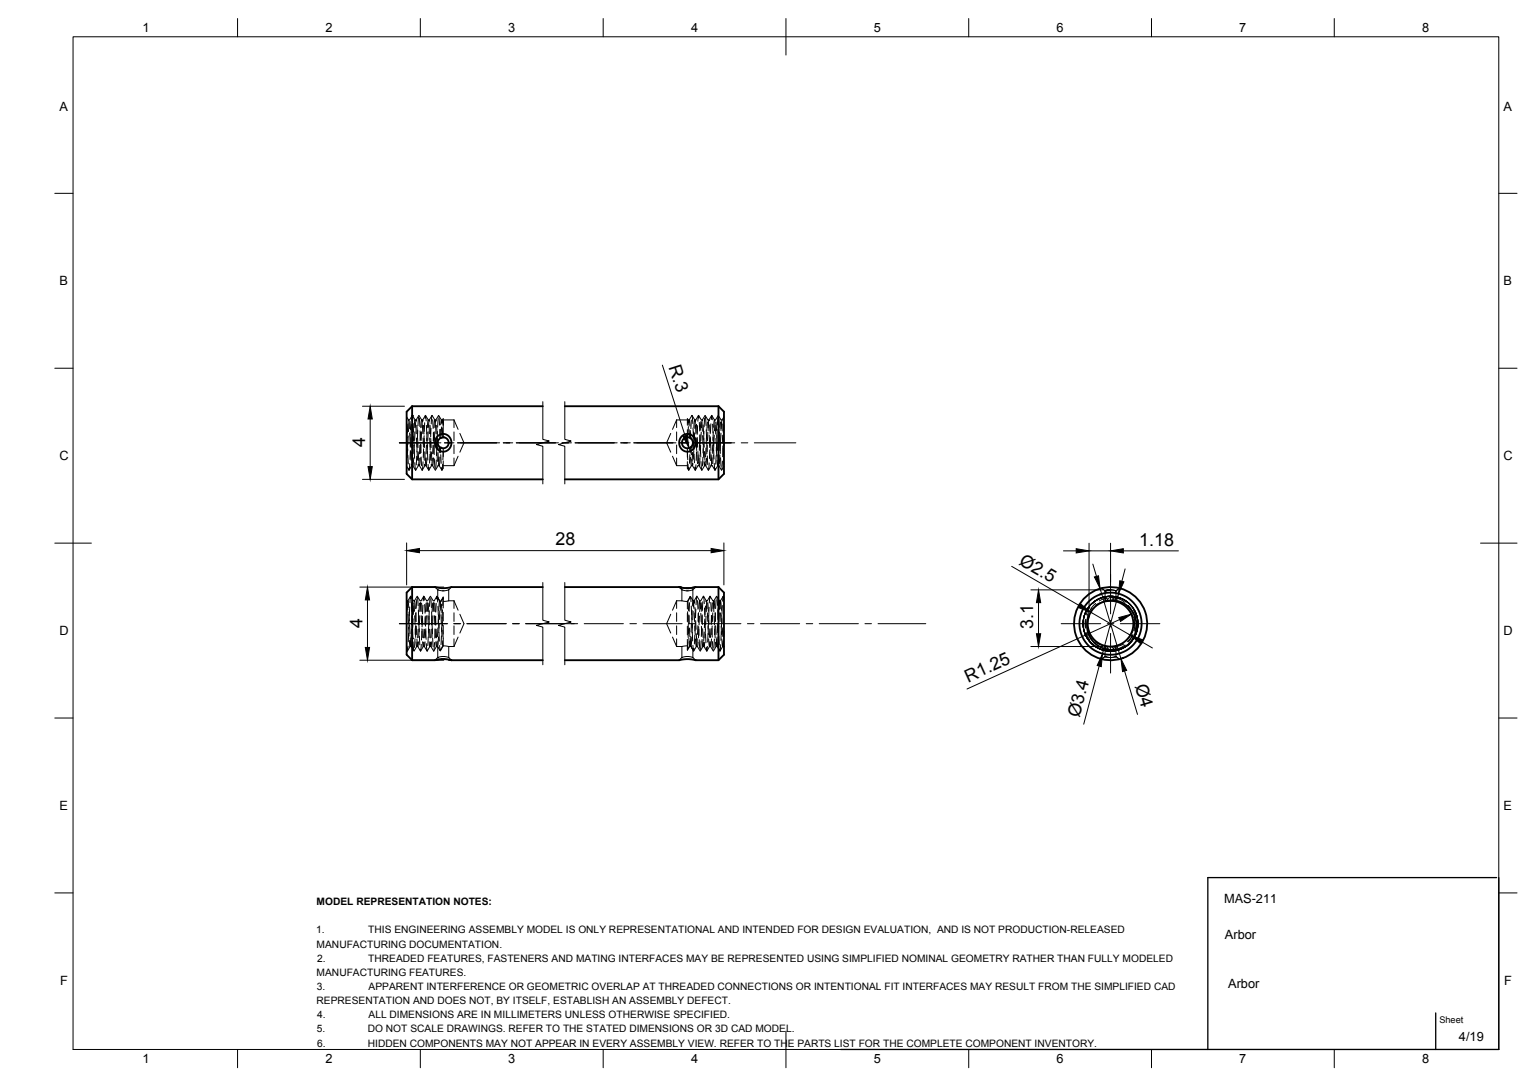
ISO-10303-21;
HEADER;
FILE_DESCRIPTION(
 (''),
 '2;1');
FILE_NAME ( 'Arbor.step', '2026-10-05T20:07:59+06:00', ( '' ), ( '' ), 'STEP AP214', 'Unspecified', '' );
FILE_SCHEMA (('AUTOMOTIVE_DESIGN { 1 0 10303 214 3 1 1 }'));
ENDSEC;
DATA;
#10=MECHANICAL_DESIGN_GEOMETRIC_PRESENTATION_REPRESENTATION('',(#320),#196741);
#311=CONICAL_SURFACE('',#8772,1.12500000002727,1.15997123047796) ;
#312=CONICAL_SURFACE('',#8775,1.12500000002727,1.15997123047796) ;
#320=STYLED_ITEM('',(#196765),#339) ;
#339=MANIFOLD_SOLID_BREP('Arbor',#8716) ;
#359=PLANE('',#8770) ;
#360=PLANE('',#8771) ;
#361=PLANE('',#8778) ;
#362=PLANE('',#8781) ;
#363=PLANE('',#8787) ;
#364=PLANE('',#8788) ;
#558=FACE_BOUND('',#1358,.T.) ;
#559=FACE_BOUND('',#1359,.T.) ;
#560=FACE_BOUND('',#1360,.T.) ;
#561=FACE_BOUND('',#1361,.T.) ;
#562=FACE_BOUND('',#1363,.T.) ;
#563=FACE_BOUND('',#1365,.T.) ;
#614=CIRCLE('',#8756,1.25000000003034) ;
#615=CIRCLE('',#8762,1.25000000003052) ;
#616=CIRCLE('',#8768,2.00000000000001) ;
#617=CIRCLE('',#8769,2.) ;
#618=CIRCLE('',#8773,1.2500000000303) ;
#619=CIRCLE('',#8774,1.2500000000303) ;
#620=CIRCLE('',#8776,1.2500000000303) ;
#621=CIRCLE('',#8777,1.2500000000303) ;
#622=CIRCLE('',#8779,1.2500000000303) ;
#623=CIRCLE('',#8782,1.25000000003031) ;
#624=CIRCLE('',#8785,1.25000000003032) ;
#625=CIRCLE('',#8786,1.25000000003029) ;
#817=B_SPLINE_SURFACE_WITH_KNOTS('',1,3,((#18888,#18889,#18890,#18891,#18892,
#18893,#18894,#18895,#18896,#18897,#18898,#18899,#18900,#18901,#18902,#18903,
#18904,#18905,#18906),(#18907,#18908,#18909,#18910,#18911,#18912,#18913,
#18914,#18915,#18916,#18917,#18918,#18919,#18920,#18921,#18922,#18923,#18924,
#18925)),.UNSPECIFIED.,.F.,.T.,.F.,(2,2),(4,1,1,1,1,1,1,1,1,1,1,1,1,1,1,
1,4),(0.,0.431146952730279),(0.,0.667571568814075,1.33514313762815,2.00271471386764,
2.67028629010714,3.33785785892123,4.00542942773531,4.67300100397479,5.34057258021427,
6.00814415645105,6.67571573268784,7.34328730150191,8.01085887031598,8.67843044655548,
9.34600202279497,10.0135735916091,10.6811451604231),.UNSPECIFIED.) ;
#818=B_SPLINE_SURFACE_WITH_KNOTS('',3,1,((#18927,#18928),(#18929,#18930),
(#18931,#18932),(#18933,#18934),(#18935,#18936),(#18937,#18938),(#18939,
#18940),(#18941,#18942),(#18943,#18944),(#18945,#18946),(#18947,#18948),
(#18949,#18950),(#18951,#18952),(#18953,#18954),(#18955,#18956),(#18957,
#18958),(#18959,#18960),(#18961,#18962),(#18963,#18964)),.UNSPECIFIED.,
 .T.,.F.,.F.,(4,1,1,1,1,1,1,1,1,1,1,1,1,1,1,1,4),(2,2),(0.,0.66757156881407,
1.33514313762814,2.00271471386764,2.67028629010714,3.33785785892123,4.00542942773532,
4.67300100397479,5.34057258021426,6.00814415645105,6.67571573268784,7.34328730150192,
8.01085887031599,8.67843044655547,9.34600202279495,10.013573591609,10.6811451604231),
(0.,0.431146952730297),.UNSPECIFIED.) ;
#819=B_SPLINE_SURFACE_WITH_KNOTS('',3,1,((#18980,#18981),(#18982,#18983),
(#18984,#18985),(#18986,#18987),(#18988,#18989),(#18990,#18991),(#18992,
#18993),(#18994,#18995),(#18996,#18997),(#18998,#18999),(#19000,#19001),
(#19002,#19003),(#19004,#19005),(#19006,#19007),(#19008,#19009),(#19010,
#19011),(#19012,#19013),(#19014,#19015),(#19016,#19017),(#19018,#19019),
(#19020,#19021),(#19022,#19023),(#19024,#19025),(#19026,#19027),(#19028,
#19029),(#19030,#19031),(#19032,#19033),(#19034,#19035),(#19036,#19037),
(#19038,#19039),(#19040,#19041),(#19042,#19043),(#19044,#19045),(#19046,
#19047),(#19048,#19049),(#19050,#19051),(#19052,#19053),(#19054,#19055),
(#19056,#19057),(#19058,#19059),(#19060,#19061),(#19062,#19063),(#19064,
#19065),(#19066,#19067),(#19068,#19069),(#19070,#19071),(#19072,#19073),
(#19074,#19075),(#19076,#19077),(#19078,#19079),(#19080,#19081),(#19082,
#19083),(#19084,#19085),(#19086,#19087),(#19088,#19089),(#19090,#19091),
(#19092,#19093),(#19094,#19095),(#19096,#19097),(#19098,#19099),(#19100,
#19101),(#19102,#19103),(#19104,#19105),(#19106,#19107),(#19108,#19109),
(#19110,#19111),(#19112,#19113),(#19114,#19115),(#19116,#19117),(#19118,
#19119),(#19120,#19121),(#19122,#19123),(#19124,#19125),(#19126,#19127),
(#19128,#19129),(#19130,#19131),(#19132,#19133),(#19134,#19135),(#19136,
#19137),(#19138,#19139),(#19140,#19141),(#19142,#19143),(#19144,#19145),
(#19146,#19147),(#19148,#19149),(#19150,#19151),(#19152,#19153),(#19154,
#19155),(#19156,#19157),(#19158,#19159),(#19160,#19161),(#19162,#19163),
(#19164,#19165),(#19166,#19167),(#19168,#19169),(#19170,#19171),(#19172,
#19173),(#19174,#19175),(#19176,#19177),(#19178,#19179),(#19180,#19181),
(#19182,#19183),(#19184,#19185),(#19186,#19187),(#19188,#19189),(#19190,
#19191),(#19192,#19193),(#19194,#19195),(#19196,#19197),(#19198,#19199),
(#19200,#19201),(#19202,#19203),(#19204,#19205),(#19206,#19207),(#19208,
#19209),(#19210,#19211),(#19212,#19213),(#19214,#19215),(#19216,#19217),
(#19218,#19219),(#19220,#19221),(#19222,#19223),(#19224,#19225),(#19226,
#19227),(#19228,#19229),(#19230,#19231),(#19232,#19233),(#19234,#19235),
(#19236,#19237),(#19238,#19239),(#19240,#19241),(#19242,#19243),(#19244,
#19245),(#19246,#19247),(#19248,#19249),(#19250,#19251),(#19252,#19253),
(#19254,#19255),(#19256,#19257),(#19258,#19259),(#19260,#19261),(#19262,
#19263),(#19264,#19265),(#19266,#19267),(#19268,#19269),(#19270,#19271),
(#19272,#19273),(#19274,#19275),(#19276,#19277),(#19278,#19279),(#19280,
#19281),(#19282,#19283),(#19284,#19285),(#19286,#19287),(#19288,#19289),
(#19290,#19291),(#19292,#19293),(#19294,#19295),(#19296,#19297),(#19298,
#19299),(#19300,#19301),(#19302,#19303),(#19304,#19305),(#19306,#19307),
(#19308,#19309),(#19310,#19311),(#19312,#19313),(#19314,#19315),(#19316,
#19317),(#19318,#19319),(#19320,#19321),(#19322,#19323),(#19324,#19325),
(#19326,#19327),(#19328,#19329),(#19330,#19331),(#19332,#19333),(#19334,
#19335),(#19336,#19337),(#19338,#19339),(#19340,#19341),(#19342,#19343),
(#19344,#19345),(#19346,#19347),(#19348,#19349),(#19350,#19351),(#19352,
#19353),(#19354,#19355),(#19356,#19357),(#19358,#19359),(#19360,#19361),
(#19362,#19363),(#19364,#19365),(#19366,#19367),(#19368,#19369),(#19370,
#19371),(#19372,#19373),(#19374,#19375),(#19376,#19377),(#19378,#19379),
(#19380,#19381),(#19382,#19383),(#19384,#19385),(#19386,#19387),(#19388,
#19389),(#19390,#19391),(#19392,#19393),(#19394,#19395),(#19396,#19397),
(#19398,#19399),(#19400,#19401),(#19402,#19403),(#19404,#19405),(#19406,
#19407),(#19408,#19409),(#19410,#19411),(#19412,#19413),(#19414,#19415),
(#19416,#19417),(#19418,#19419),(#19420,#19421),(#19422,#19423),(#19424,
#19425),(#19426,#19427),(#19428,#19429),(#19430,#19431),(#19432,#19433),
(#19434,#19435),(#19436,#19437),(#19438,#19439),(#19440,#19441),(#19442,
#19443),(#19444,#19445),(#19446,#19447),(#19448,#19449),(#19450,#19451),
(#19452,#19453),(#19454,#19455),(#19456,#19457),(#19458,#19459),(#19460,
#19461),(#19462,#19463),(#19464,#19465),(#19466,#19467),(#19468,#19469),
(#19470,#19471),(#19472,#19473),(#19474,#19475),(#19476,#19477),(#19478,
#19479),(#19480,#19481),(#19482,#19483),(#19484,#19485),(#19486,#19487),
(#19488,#19489),(#19490,#19491),(#19492,#19493),(#19494,#19495),(#19496,
#19497),(#19498,#19499),(#19500,#19501),(#19502,#19503),(#19504,#19505),
(#19506,#19507),(#19508,#19509),(#19510,#19511),(#19512,#19513),(#19514,
#19515),(#19516,#19517),(#19518,#19519),(#19520,#19521),(#19522,#19523),
(#19524,#19525),(#19526,#19527),(#19528,#19529),(#19530,#19531),(#19532,
#19533),(#19534,#19535),(#19536,#19537),(#19538,#19539),(#19540,#19541),
(#19542,#19543),(#19544,#19545),(#19546,#19547),(#19548,#19549),(#19550,
#19551),(#19552,#19553),(#19554,#19555),(#19556,#19557),(#19558,#19559),
(#19560,#19561),(#19562,#19563),(#19564,#19565),(#19566,#19567),(#19568,
#19569),(#19570,#19571),(#19572,#19573),(#19574,#19575),(#19576,#19577),
(#19578,#19579),(#19580,#19581),(#19582,#19583),(#19584,#19585),(#19586,
#19587),(#19588,#19589),(#19590,#19591),(#19592,#19593),(#19594,#19595),
(#19596,#19597),(#19598,#19599),(#19600,#19601),(#19602,#19603),(#19604,
#19605),(#19606,#19607),(#19608,#19609),(#19610,#19611),(#19612,#19613),
(#19614,#19615),(#19616,#19617),(#19618,#19619),(#19620,#19621),(#19622,
#19623),(#19624,#19625),(#19626,#19627),(#19628,#19629),(#19630,#19631),
(#19632,#19633),(#19634,#19635),(#19636,#19637),(#19638,#19639),(#19640,
#19641),(#19642,#19643),(#19644,#19645),(#19646,#19647),(#19648,#19649),
(#19650,#19651),(#19652,#19653),(#19654,#19655),(#19656,#19657),(#19658,
#19659),(#19660,#19661),(#19662,#19663),(#19664,#19665),(#19666,#19667),
(#19668,#19669),(#19670,#19671),(#19672,#19673),(#19674,#19675),(#19676,
#19677),(#19678,#19679),(#19680,#19681),(#19682,#19683),(#19684,#19685),
(#19686,#19687),(#19688,#19689),(#19690,#19691),(#19692,#19693),(#19694,
#19695),(#19696,#19697),(#19698,#19699),(#19700,#19701),(#19702,#19703),
(#19704,#19705),(#19706,#19707),(#19708,#19709),(#19710,#19711),(#19712,
#19713),(#19714,#19715),(#19716,#19717),(#19718,#19719),(#19720,#19721),
(#19722,#19723),(#19724,#19725),(#19726,#19727),(#19728,#19729),(#19730,
#19731),(#19732,#19733),(#19734,#19735),(#19736,#19737),(#19738,#19739),
(#19740,#19741),(#19742,#19743),(#19744,#19745),(#19746,#19747),(#19748,
#19749),(#19750,#19751),(#19752,#19753),(#19754,#19755),(#19756,#19757),
(#19758,#19759),(#19760,#19761),(#19762,#19763),(#19764,#19765),(#19766,
#19767),(#19768,#19769),(#19770,#19771),(#19772,#19773),(#19774,#19775),
(#19776,#19777),(#19778,#19779),(#19780,#19781),(#19782,#19783),(#19784,
#19785),(#19786,#19787),(#19788,#19789),(#19790,#19791),(#19792,#19793),
(#19794,#19795),(#19796,#19797),(#19798,#19799),(#19800,#19801),(#19802,
#19803),(#19804,#19805),(#19806,#19807),(#19808,#19809),(#19810,#19811),
(#19812,#19813),(#19814,#19815),(#19816,#19817),(#19818,#19819),(#19820,
#19821),(#19822,#19823),(#19824,#19825),(#19826,#19827),(#19828,#19829),
(#19830,#19831),(#19832,#19833),(#19834,#19835),(#19836,#19837),(#19838,
#19839),(#19840,#19841),(#19842,#19843),(#19844,#19845),(#19846,#19847),
(#19848,#19849),(#19850,#19851),(#19852,#19853),(#19854,#19855),(#19856,
#19857),(#19858,#19859),(#19860,#19861),(#19862,#19863),(#19864,#19865),
(#19866,#19867),(#19868,#19869),(#19870,#19871),(#19872,#19873),(#19874,
#19875),(#19876,#19877),(#19878,#19879),(#19880,#19881),(#19882,#19883),
(#19884,#19885),(#19886,#19887),(#19888,#19889),(#19890,#19891),(#19892,
#19893),(#19894,#19895),(#19896,#19897),(#19898,#19899),(#19900,#19901),
(#19902,#19903),(#19904,#19905),(#19906,#19907),(#19908,#19909),(#19910,
#19911),(#19912,#19913),(#19914,#19915),(#19916,#19917),(#19918,#19919),
(#19920,#19921),(#19922,#19923),(#19924,#19925),(#19926,#19927),(#19928,
#19929),(#19930,#19931),(#19932,#19933),(#19934,#19935),(#19936,#19937),
(#19938,#19939),(#19940,#19941),(#19942,#19943),(#19944,#19945),(#19946,
#19947),(#19948,#19949),(#19950,#19951),(#19952,#19953),(#19954,#19955),
(#19956,#19957),(#19958,#19959),(#19960,#19961),(#19962,#19963),(#19964,
#19965),(#19966,#19967),(#19968,#19969),(#19970,#19971),(#19972,#19973),
(#19974,#19975),(#19976,#19977),(#19978,#19979),(#19980,#19981),(#19982,
#19983),(#19984,#19985),(#19986,#19987),(#19988,#19989),(#19990,#19991),
(#19992,#19993),(#19994,#19995),(#19996,#19997),(#19998,#19999),(#20000,
#20001),(#20002,#20003),(#20004,#20005),(#20006,#20007),(#20008,#20009),
(#20010,#20011),(#20012,#20013),(#20014,#20015),(#20016,#20017),(#20018,
#20019),(#20020,#20021),(#20022,#20023),(#20024,#20025),(#20026,#20027),
(#20028,#20029),(#20030,#20031),(#20032,#20033),(#20034,#20035),(#20036,
#20037),(#20038,#20039),(#20040,#20041),(#20042,#20043),(#20044,#20045),
(#20046,#20047),(#20048,#20049),(#20050,#20051),(#20052,#20053),(#20054,
#20055),(#20056,#20057),(#20058,#20059),(#20060,#20061),(#20062,#20063),
(#20064,#20065),(#20066,#20067),(#20068,#20069),(#20070,#20071),(#20072,
#20073),(#20074,#20075),(#20076,#20077),(#20078,#20079),(#20080,#20081),
(#20082,#20083),(#20084,#20085),(#20086,#20087),(#20088,#20089),(#20090,
#20091),(#20092,#20093),(#20094,#20095),(#20096,#20097),(#20098,#20099),
(#20100,#20101),(#20102,#20103),(#20104,#20105),(#20106,#20107),(#20108,
#20109),(#20110,#20111),(#20112,#20113),(#20114,#20115),(#20116,#20117),
(#20118,#20119),(#20120,#20121),(#20122,#20123),(#20124,#20125),(#20126,
#20127),(#20128,#20129),(#20130,#20131),(#20132,#20133),(#20134,#20135),
(#20136,#20137),(#20138,#20139),(#20140,#20141),(#20142,#20143),(#20144,
#20145),(#20146,#20147),(#20148,#20149),(#20150,#20151),(#20152,#20153),
(#20154,#20155),(#20156,#20157),(#20158,#20159),(#20160,#20161),(#20162,
#20163),(#20164,#20165),(#20166,#20167),(#20168,#20169),(#20170,#20171),
(#20172,#20173),(#20174,#20175),(#20176,#20177),(#20178,#20179),(#20180,
#20181),(#20182,#20183),(#20184,#20185),(#20186,#20187),(#20188,#20189),
(#20190,#20191),(#20192,#20193),(#20194,#20195),(#20196,#20197),(#20198,
#20199),(#20200,#20201),(#20202,#20203),(#20204,#20205),(#20206,#20207),
(#20208,#20209),(#20210,#20211),(#20212,#20213),(#20214,#20215),(#20216,
#20217),(#20218,#20219),(#20220,#20221),(#20222,#20223),(#20224,#20225),
(#20226,#20227),(#20228,#20229),(#20230,#20231),(#20232,#20233),(#20234,
#20235),(#20236,#20237),(#20238,#20239),(#20240,#20241),(#20242,#20243),
(#20244,#20245),(#20246,#20247),(#20248,#20249),(#20250,#20251),(#20252,
#20253),(#20254,#20255),(#20256,#20257),(#20258,#20259),(#20260,#20261),
(#20262,#20263),(#20264,#20265),(#20266,#20267),(#20268,#20269),(#20270,
#20271),(#20272,#20273),(#20274,#20275),(#20276,#20277),(#20278,#20279),
(#20280,#20281),(#20282,#20283),(#20284,#20285),(#20286,#20287),(#20288,
#20289),(#20290,#20291),(#20292,#20293),(#20294,#20295),(#20296,#20297),
(#20298,#20299),(#20300,#20301),(#20302,#20303),(#20304,#20305),(#20306,
#20307),(#20308,#20309),(#20310,#20311),(#20312,#20313),(#20314,#20315),
(#20316,#20317),(#20318,#20319),(#20320,#20321),(#20322,#20323),(#20324,
#20325),(#20326,#20327),(#20328,#20329),(#20330,#20331),(#20332,#20333),
(#20334,#20335),(#20336,#20337),(#20338,#20339),(#20340,#20341),(#20342,
#20343),(#20344,#20345),(#20346,#20347),(#20348,#20349),(#20350,#20351),
(#20352,#20353),(#20354,#20355),(#20356,#20357),(#20358,#20359),(#20360,
#20361),(#20362,#20363),(#20364,#20365),(#20366,#20367),(#20368,#20369),
(#20370,#20371),(#20372,#20373),(#20374,#20375),(#20376,#20377),(#20378,
#20379),(#20380,#20381),(#20382,#20383),(#20384,#20385),(#20386,#20387),
(#20388,#20389),(#20390,#20391),(#20392,#20393),(#20394,#20395),(#20396,
#20397),(#20398,#20399),(#20400,#20401),(#20402,#20403),(#20404,#20405),
(#20406,#20407),(#20408,#20409),(#20410,#20411),(#20412,#20413),(#20414,
#20415),(#20416,#20417),(#20418,#20419),(#20420,#20421),(#20422,#20423),
(#20424,#20425),(#20426,#20427),(#20428,#20429),(#20430,#20431),(#20432,
#20433),(#20434,#20435),(#20436,#20437),(#20438,#20439),(#20440,#20441),
(#20442,#20443),(#20444,#20445),(#20446,#20447),(#20448,#20449),(#20450,
#20451),(#20452,#20453),(#20454,#20455),(#20456,#20457),(#20458,#20459),
(#20460,#20461),(#20462,#20463),(#20464,#20465),(#20466,#20467),(#20468,
#20469),(#20470,#20471),(#20472,#20473),(#20474,#20475),(#20476,#20477),
(#20478,#20479),(#20480,#20481),(#20482,#20483),(#20484,#20485),(#20486,
#20487),(#20488,#20489),(#20490,#20491),(#20492,#20493),(#20494,#20495),
(#20496,#20497),(#20498,#20499),(#20500,#20501),(#20502,#20503),(#20504,
#20505),(#20506,#20507),(#20508,#20509),(#20510,#20511),(#20512,#20513),
(#20514,#20515),(#20516,#20517),(#20518,#20519),(#20520,#20521),(#20522,
#20523),(#20524,#20525),(#20526,#20527),(#20528,#20529),(#20530,#20531),
(#20532,#20533),(#20534,#20535),(#20536,#20537),(#20538,#20539),(#20540,
#20541),(#20542,#20543),(#20544,#20545),(#20546,#20547),(#20548,#20549),
(#20550,#20551),(#20552,#20553),(#20554,#20555),(#20556,#20557),(#20558,
#20559),(#20560,#20561),(#20562,#20563),(#20564,#20565),(#20566,#20567),
(#20568,#20569),(#20570,#20571),(#20572,#20573),(#20574,#20575),(#20576,
#20577),(#20578,#20579),(#20580,#20581),(#20582,#20583),(#20584,#20585),
(#20586,#20587),(#20588,#20589),(#20590,#20591),(#20592,#20593),(#20594,
#20595),(#20596,#20597),(#20598,#20599),(#20600,#20601),(#20602,#20603),
(#20604,#20605),(#20606,#20607),(#20608,#20609),(#20610,#20611),(#20612,
#20613),(#20614,#20615),(#20616,#20617),(#20618,#20619),(#20620,#20621),
(#20622,#20623),(#20624,#20625),(#20626,#20627),(#20628,#20629),(#20630,
#20631),(#20632,#20633),(#20634,#20635),(#20636,#20637),(#20638,#20639),
(#20640,#20641),(#20642,#20643),(#20644,#20645),(#20646,#20647),(#20648,
#20649),(#20650,#20651),(#20652,#20653),(#20654,#20655),(#20656,#20657),
(#20658,#20659),(#20660,#20661),(#20662,#20663),(#20664,#20665),(#20666,
#20667),(#20668,#20669),(#20670,#20671),(#20672,#20673),(#20674,#20675),
(#20676,#20677),(#20678,#20679),(#20680,#20681),(#20682,#20683),(#20684,
#20685),(#20686,#20687),(#20688,#20689),(#20690,#20691),(#20692,#20693),
(#20694,#20695),(#20696,#20697),(#20698,#20699),(#20700,#20701),(#20702,
#20703),(#20704,#20705),(#20706,#20707),(#20708,#20709),(#20710,#20711),
(#20712,#20713),(#20714,#20715),(#20716,#20717),(#20718,#20719),(#20720,
#20721),(#20722,#20723),(#20724,#20725),(#20726,#20727),(#20728,#20729),
(#20730,#20731),(#20732,#20733),(#20734,#20735),(#20736,#20737),(#20738,
#20739),(#20740,#20741),(#20742,#20743),(#20744,#20745),(#20746,#20747),
(#20748,#20749),(#20750,#20751),(#20752,#20753),(#20754,#20755),(#20756,
#20757),(#20758,#20759),(#20760,#20761),(#20762,#20763),(#20764,#20765),
(#20766,#20767),(#20768,#20769),(#20770,#20771),(#20772,#20773),(#20774,
#20775),(#20776,#20777),(#20778,#20779),(#20780,#20781),(#20782,#20783),
(#20784,#20785),(#20786,#20787),(#20788,#20789),(#20790,#20791),(#20792,
#20793),(#20794,#20795),(#20796,#20797),(#20798,#20799),(#20800,#20801),
(#20802,#20803),(#20804,#20805),(#20806,#20807),(#20808,#20809),(#20810,
#20811),(#20812,#20813),(#20814,#20815),(#20816,#20817),(#20818,#20819),
(#20820,#20821),(#20822,#20823),(#20824,#20825),(#20826,#20827),(#20828,
#20829),(#20830,#20831),(#20832,#20833),(#20834,#20835),(#20836,#20837),
(#20838,#20839),(#20840,#20841),(#20842,#20843),(#20844,#20845),(#20846,
#20847),(#20848,#20849),(#20850,#20851),(#20852,#20853),(#20854,#20855),
(#20856,#20857),(#20858,#20859),(#20860,#20861),(#20862,#20863),(#20864,
#20865),(#20866,#20867),(#20868,#20869),(#20870,#20871),(#20872,#20873),
(#20874,#20875),(#20876,#20877),(#20878,#20879),(#20880,#20881),(#20882,
#20883),(#20884,#20885),(#20886,#20887),(#20888,#20889),(#20890,#20891),
(#20892,#20893),(#20894,#20895),(#20896,#20897),(#20898,#20899),(#20900,
#20901),(#20902,#20903),(#20904,#20905),(#20906,#20907),(#20908,#20909),
(#20910,#20911),(#20912,#20913),(#20914,#20915),(#20916,#20917),(#20918,
#20919),(#20920,#20921),(#20922,#20923),(#20924,#20925),(#20926,#20927),
(#20928,#20929),(#20930,#20931),(#20932,#20933),(#20934,#20935),(#20936,
#20937),(#20938,#20939),(#20940,#20941),(#20942,#20943),(#20944,#20945),
(#20946,#20947),(#20948,#20949),(#20950,#20951),(#20952,#20953),(#20954,
#20955),(#20956,#20957),(#20958,#20959),(#20960,#20961),(#20962,#20963),
(#20964,#20965),(#20966,#20967),(#20968,#20969),(#20970,#20971),(#20972,
#20973),(#20974,#20975),(#20976,#20977),(#20978,#20979),(#20980,#20981),
(#20982,#20983),(#20984,#20985),(#20986,#20987),(#20988,#20989),(#20990,
#20991),(#20992,#20993),(#20994,#20995),(#20996,#20997),(#20998,#20999),
(#21000,#21001),(#21002,#21003),(#21004,#21005),(#21006,#21007),(#21008,
#21009),(#21010,#21011),(#21012,#21013),(#21014,#21015),(#21016,#21017),
(#21018,#21019),(#21020,#21021),(#21022,#21023),(#21024,#21025),(#21026,
#21027),(#21028,#21029),(#21030,#21031),(#21032,#21033),(#21034,#21035),
(#21036,#21037),(#21038,#21039),(#21040,#21041),(#21042,#21043),(#21044,
#21045),(#21046,#21047),(#21048,#21049),(#21050,#21051),(#21052,#21053),
(#21054,#21055),(#21056,#21057),(#21058,#21059),(#21060,#21061),(#21062,
#21063),(#21064,#21065),(#21066,#21067),(#21068,#21069),(#21070,#21071),
(#21072,#21073),(#21074,#21075),(#21076,#21077),(#21078,#21079),(#21080,
#21081),(#21082,#21083),(#21084,#21085),(#21086,#21087),(#21088,#21089),
(#21090,#21091),(#21092,#21093),(#21094,#21095),(#21096,#21097),(#21098,
#21099),(#21100,#21101),(#21102,#21103),(#21104,#21105),(#21106,#21107),
(#21108,#21109),(#21110,#21111),(#21112,#21113),(#21114,#21115),(#21116,
#21117),(#21118,#21119),(#21120,#21121),(#21122,#21123),(#21124,#21125),
(#21126,#21127),(#21128,#21129),(#21130,#21131),(#21132,#21133),(#21134,
#21135),(#21136,#21137),(#21138,#21139),(#21140,#21141),(#21142,#21143),
(#21144,#21145),(#21146,#21147),(#21148,#21149),(#21150,#21151),(#21152,
#21153),(#21154,#21155),(#21156,#21157),(#21158,#21159),(#21160,#21161),
(#21162,#21163),(#21164,#21165),(#21166,#21167),(#21168,#21169),(#21170,
#21171),(#21172,#21173),(#21174,#21175),(#21176,#21177),(#21178,#21179),
(#21180,#21181),(#21182,#21183),(#21184,#21185),(#21186,#21187),(#21188,
#21189),(#21190,#21191),(#21192,#21193),(#21194,#21195),(#21196,#21197),
(#21198,#21199),(#21200,#21201),(#21202,#21203),(#21204,#21205),(#21206,
#21207),(#21208,#21209),(#21210,#21211),(#21212,#21213),(#21214,#21215),
(#21216,#21217),(#21218,#21219),(#21220,#21221),(#21222,#21223),(#21224,
#21225),(#21226,#21227),(#21228,#21229),(#21230,#21231),(#21232,#21233),
(#21234,#21235),(#21236,#21237),(#21238,#21239),(#21240,#21241),(#21242,
#21243),(#21244,#21245),(#21246,#21247),(#21248,#21249),(#21250,#21251),
(#21252,#21253),(#21254,#21255),(#21256,#21257),(#21258,#21259),(#21260,
#21261),(#21262,#21263),(#21264,#21265),(#21266,#21267),(#21268,#21269),
(#21270,#21271),(#21272,#21273),(#21274,#21275),(#21276,#21277),(#21278,
#21279),(#21280,#21281),(#21282,#21283),(#21284,#21285),(#21286,#21287),
(#21288,#21289),(#21290,#21291),(#21292,#21293),(#21294,#21295),(#21296,
#21297),(#21298,#21299),(#21300,#21301),(#21302,#21303),(#21304,#21305),
(#21306,#21307),(#21308,#21309),(#21310,#21311),(#21312,#21313),(#21314,
#21315),(#21316,#21317),(#21318,#21319),(#21320,#21321),(#21322,#21323),
(#21324,#21325),(#21326,#21327),(#21328,#21329),(#21330,#21331),(#21332,
#21333),(#21334,#21335),(#21336,#21337),(#21338,#21339),(#21340,#21341),
(#21342,#21343),(#21344,#21345),(#21346,#21347),(#21348,#21349),(#21350,
#21351),(#21352,#21353),(#21354,#21355),(#21356,#21357),(#21358,#21359),
(#21360,#21361),(#21362,#21363),(#21364,#21365),(#21366,#21367),(#21368,
#21369),(#21370,#21371),(#21372,#21373),(#21374,#21375),(#21376,#21377),
(#21378,#21379),(#21380,#21381),(#21382,#21383),(#21384,#21385),(#21386,
#21387),(#21388,#21389),(#21390,#21391),(#21392,#21393),(#21394,#21395),
(#21396,#21397),(#21398,#21399),(#21400,#21401),(#21402,#21403),(#21404,
#21405),(#21406,#21407),(#21408,#21409),(#21410,#21411),(#21412,#21413),
(#21414,#21415),(#21416,#21417),(#21418,#21419),(#21420,#21421),(#21422,
#21423),(#21424,#21425),(#21426,#21427),(#21428,#21429),(#21430,#21431),
(#21432,#21433),(#21434,#21435),(#21436,#21437),(#21438,#21439),(#21440,
#21441),(#21442,#21443),(#21444,#21445),(#21446,#21447),(#21448,#21449),
(#21450,#21451),(#21452,#21453),(#21454,#21455),(#21456,#21457),(#21458,
#21459),(#21460,#21461),(#21462,#21463),(#21464,#21465),(#21466,#21467),
(#21468,#21469),(#21470,#21471),(#21472,#21473),(#21474,#21475),(#21476,
#21477),(#21478,#21479),(#21480,#21481),(#21482,#21483),(#21484,#21485),
(#21486,#21487),(#21488,#21489),(#21490,#21491),(#21492,#21493),(#21494,
#21495),(#21496,#21497),(#21498,#21499),(#21500,#21501),(#21502,#21503),
(#21504,#21505),(#21506,#21507),(#21508,#21509),(#21510,#21511),(#21512,
#21513),(#21514,#21515),(#21516,#21517),(#21518,#21519),(#21520,#21521),
(#21522,#21523),(#21524,#21525),(#21526,#21527),(#21528,#21529),(#21530,
#21531),(#21532,#21533),(#21534,#21535),(#21536,#21537),(#21538,#21539),
(#21540,#21541),(#21542,#21543),(#21544,#21545),(#21546,#21547),(#21548,
#21549),(#21550,#21551),(#21552,#21553),(#21554,#21555),(#21556,#21557),
(#21558,#21559),(#21560,#21561),(#21562,#21563),(#21564,#21565),(#21566,
#21567),(#21568,#21569),(#21570,#21571),(#21572,#21573),(#21574,#21575),
(#21576,#21577),(#21578,#21579),(#21580,#21581),(#21582,#21583),(#21584,
#21585),(#21586,#21587),(#21588,#21589),(#21590,#21591),(#21592,#21593),
(#21594,#21595),(#21596,#21597),(#21598,#21599),(#21600,#21601),(#21602,
#21603),(#21604,#21605),(#21606,#21607),(#21608,#21609),(#21610,#21611),
(#21612,#21613),(#21614,#21615),(#21616,#21617),(#21618,#21619),(#21620,
#21621),(#21622,#21623),(#21624,#21625),(#21626,#21627),(#21628,#21629),
(#21630,#21631),(#21632,#21633),(#21634,#21635),(#21636,#21637),(#21638,
#21639),(#21640,#21641),(#21642,#21643),(#21644,#21645),(#21646,#21647),
(#21648,#21649),(#21650,#21651),(#21652,#21653),(#21654,#21655),(#21656,
#21657),(#21658,#21659),(#21660,#21661),(#21662,#21663),(#21664,#21665),
(#21666,#21667),(#21668,#21669),(#21670,#21671),(#21672,#21673),(#21674,
#21675),(#21676,#21677),(#21678,#21679),(#21680,#21681),(#21682,#21683),
(#21684,#21685),(#21686,#21687),(#21688,#21689),(#21690,#21691),(#21692,
#21693),(#21694,#21695),(#21696,#21697),(#21698,#21699),(#21700,#21701),
(#21702,#21703),(#21704,#21705),(#21706,#21707),(#21708,#21709),(#21710,
#21711),(#21712,#21713),(#21714,#21715),(#21716,#21717),(#21718,#21719),
(#21720,#21721),(#21722,#21723),(#21724,#21725),(#21726,#21727),(#21728,
#21729),(#21730,#21731),(#21732,#21733),(#21734,#21735),(#21736,#21737),
(#21738,#21739),(#21740,#21741),(#21742,#21743),(#21744,#21745),(#21746,
#21747),(#21748,#21749),(#21750,#21751),(#21752,#21753),(#21754,#21755),
(#21756,#21757),(#21758,#21759),(#21760,#21761),(#21762,#21763),(#21764,
#21765),(#21766,#21767),(#21768,#21769),(#21770,#21771),(#21772,#21773),
(#21774,#21775),(#21776,#21777),(#21778,#21779),(#21780,#21781),(#21782,
#21783),(#21784,#21785),(#21786,#21787),(#21788,#21789),(#21790,#21791),
(#21792,#21793),(#21794,#21795),(#21796,#21797),(#21798,#21799),(#21800,
#21801),(#21802,#21803),(#21804,#21805),(#21806,#21807),(#21808,#21809),
(#21810,#21811),(#21812,#21813),(#21814,#21815),(#21816,#21817),(#21818,
#21819),(#21820,#21821),(#21822,#21823),(#21824,#21825),(#21826,#21827),
(#21828,#21829),(#21830,#21831),(#21832,#21833),(#21834,#21835),(#21836,
#21837),(#21838,#21839),(#21840,#21841),(#21842,#21843),(#21844,#21845),
(#21846,#21847),(#21848,#21849),(#21850,#21851),(#21852,#21853),(#21854,
#21855),(#21856,#21857),(#21858,#21859),(#21860,#21861),(#21862,#21863),
(#21864,#21865),(#21866,#21867),(#21868,#21869),(#21870,#21871),(#21872,
#21873),(#21874,#21875),(#21876,#21877),(#21878,#21879),(#21880,#21881),
(#21882,#21883),(#21884,#21885),(#21886,#21887),(#21888,#21889),(#21890,
#21891),(#21892,#21893),(#21894,#21895),(#21896,#21897),(#21898,#21899),
(#21900,#21901),(#21902,#21903),(#21904,#21905),(#21906,#21907),(#21908,
#21909),(#21910,#21911),(#21912,#21913),(#21914,#21915),(#21916,#21917),
(#21918,#21919),(#21920,#21921),(#21922,#21923),(#21924,#21925),(#21926,
#21927),(#21928,#21929),(#21930,#21931),(#21932,#21933),(#21934,#21935),
(#21936,#21937),(#21938,#21939),(#21940,#21941),(#21942,#21943),(#21944,
#21945),(#21946,#21947),(#21948,#21949),(#21950,#21951),(#21952,#21953),
(#21954,#21955),(#21956,#21957),(#21958,#21959),(#21960,#21961),(#21962,
#21963),(#21964,#21965),(#21966,#21967),(#21968,#21969),(#21970,#21971),
(#21972,#21973),(#21974,#21975),(#21976,#21977),(#21978,#21979),(#21980,
#21981),(#21982,#21983),(#21984,#21985),(#21986,#21987),(#21988,#21989),
(#21990,#21991),(#21992,#21993),(#21994,#21995),(#21996,#21997),(#21998,
#21999),(#22000,#22001),(#22002,#22003),(#22004,#22005),(#22006,#22007),
(#22008,#22009),(#22010,#22011),(#22012,#22013),(#22014,#22015),(#22016,
#22017),(#22018,#22019),(#22020,#22021),(#22022,#22023),(#22024,#22025),
(#22026,#22027),(#22028,#22029),(#22030,#22031),(#22032,#22033),(#22034,
#22035),(#22036,#22037),(#22038,#22039),(#22040,#22041),(#22042,#22043),
(#22044,#22045),(#22046,#22047),(#22048,#22049),(#22050,#22051),(#22052,
#22053),(#22054,#22055),(#22056,#22057),(#22058,#22059),(#22060,#22061),
(#22062,#22063),(#22064,#22065),(#22066,#22067),(#22068,#22069),(#22070,
#22071),(#22072,#22073),(#22074,#22075),(#22076,#22077),(#22078,#22079),
(#22080,#22081),(#22082,#22083),(#22084,#22085),(#22086,#22087),(#22088,
#22089),(#22090,#22091),(#22092,#22093),(#22094,#22095),(#22096,#22097),
(#22098,#22099),(#22100,#22101),(#22102,#22103),(#22104,#22105),(#22106,
#22107),(#22108,#22109),(#22110,#22111),(#22112,#22113),(#22114,#22115),
(#22116,#22117),(#22118,#22119),(#22120,#22121),(#22122,#22123),(#22124,
#22125),(#22126,#22127),(#22128,#22129),(#22130,#22131),(#22132,#22133),
(#22134,#22135),(#22136,#22137),(#22138,#22139),(#22140,#22141),(#22142,
#22143),(#22144,#22145),(#22146,#22147),(#22148,#22149),(#22150,#22151),
(#22152,#22153),(#22154,#22155),(#22156,#22157),(#22158,#22159),(#22160,
#22161),(#22162,#22163),(#22164,#22165),(#22166,#22167),(#22168,#22169),
(#22170,#22171),(#22172,#22173),(#22174,#22175),(#22176,#22177),(#22178,
#22179),(#22180,#22181),(#22182,#22183),(#22184,#22185),(#22186,#22187),
(#22188,#22189),(#22190,#22191),(#22192,#22193),(#22194,#22195),(#22196,
#22197),(#22198,#22199),(#22200,#22201),(#22202,#22203),(#22204,#22205),
(#22206,#22207),(#22208,#22209),(#22210,#22211),(#22212,#22213),(#22214,
#22215),(#22216,#22217),(#22218,#22219),(#22220,#22221),(#22222,#22223),
(#22224,#22225),(#22226,#22227),(#22228,#22229),(#22230,#22231),(#22232,
#22233),(#22234,#22235),(#22236,#22237),(#22238,#22239),(#22240,#22241),
(#22242,#22243),(#22244,#22245),(#22246,#22247),(#22248,#22249),(#22250,
#22251),(#22252,#22253),(#22254,#22255),(#22256,#22257),(#22258,#22259),
(#22260,#22261),(#22262,#22263),(#22264,#22265),(#22266,#22267),(#22268,
#22269),(#22270,#22271),(#22272,#22273),(#22274,#22275),(#22276,#22277),
(#22278,#22279),(#22280,#22281),(#22282,#22283),(#22284,#22285),(#22286,
#22287),(#22288,#22289),(#22290,#22291),(#22292,#22293),(#22294,#22295),
(#22296,#22297),(#22298,#22299),(#22300,#22301),(#22302,#22303),(#22304,
#22305),(#22306,#22307),(#22308,#22309),(#22310,#22311),(#22312,#22313),
(#22314,#22315),(#22316,#22317),(#22318,#22319),(#22320,#22321),(#22322,
#22323),(#22324,#22325),(#22326,#22327),(#22328,#22329),(#22330,#22331),
(#22332,#22333),(#22334,#22335),(#22336,#22337),(#22338,#22339),(#22340,
#22341),(#22342,#22343),(#22344,#22345),(#22346,#22347),(#22348,#22349),
(#22350,#22351),(#22352,#22353),(#22354,#22355),(#22356,#22357),(#22358,
#22359),(#22360,#22361),(#22362,#22363),(#22364,#22365),(#22366,#22367),
(#22368,#22369),(#22370,#22371),(#22372,#22373),(#22374,#22375),(#22376,
#22377),(#22378,#22379),(#22380,#22381),(#22382,#22383),(#22384,#22385),
(#22386,#22387),(#22388,#22389),(#22390,#22391),(#22392,#22393),(#22394,
#22395),(#22396,#22397),(#22398,#22399),(#22400,#22401),(#22402,#22403),
(#22404,#22405),(#22406,#22407),(#22408,#22409),(#22410,#22411),(#22412,
#22413),(#22414,#22415),(#22416,#22417),(#22418,#22419),(#22420,#22421),
(#22422,#22423),(#22424,#22425),(#22426,#22427),(#22428,#22429),(#22430,
#22431),(#22432,#22433),(#22434,#22435),(#22436,#22437),(#22438,#22439),
(#22440,#22441),(#22442,#22443),(#22444,#22445),(#22446,#22447),(#22448,
#22449),(#22450,#22451),(#22452,#22453),(#22454,#22455),(#22456,#22457),
(#22458,#22459),(#22460,#22461),(#22462,#22463),(#22464,#22465),(#22466,
#22467),(#22468,#22469),(#22470,#22471),(#22472,#22473),(#22474,#22475),
(#22476,#22477),(#22478,#22479),(#22480,#22481),(#22482,#22483),(#22484,
#22485),(#22486,#22487),(#22488,#22489),(#22490,#22491),(#22492,#22493),
(#22494,#22495),(#22496,#22497),(#22498,#22499),(#22500,#22501),(#22502,
#22503),(#22504,#22505),(#22506,#22507),(#22508,#22509),(#22510,#22511),
(#22512,#22513),(#22514,#22515),(#22516,#22517),(#22518,#22519),(#22520,
#22521),(#22522,#22523),(#22524,#22525),(#22526,#22527),(#22528,#22529),
(#22530,#22531),(#22532,#22533),(#22534,#22535),(#22536,#22537),(#22538,
#22539),(#22540,#22541),(#22542,#22543),(#22544,#22545),(#22546,#22547),
(#22548,#22549),(#22550,#22551),(#22552,#22553),(#22554,#22555),(#22556,
#22557),(#22558,#22559),(#22560,#22561),(#22562,#22563),(#22564,#22565),
(#22566,#22567),(#22568,#22569),(#22570,#22571),(#22572,#22573),(#22574,
#22575),(#22576,#22577),(#22578,#22579),(#22580,#22581),(#22582,#22583),
(#22584,#22585),(#22586,#22587),(#22588,#22589),(#22590,#22591),(#22592,
#22593),(#22594,#22595),(#22596,#22597),(#22598,#22599),(#22600,#22601),
(#22602,#22603),(#22604,#22605),(#22606,#22607),(#22608,#22609),(#22610,
#22611),(#22612,#22613),(#22614,#22615),(#22616,#22617),(#22618,#22619),
(#22620,#22621),(#22622,#22623),(#22624,#22625),(#22626,#22627),(#22628,
#22629),(#22630,#22631),(#22632,#22633),(#22634,#22635),(#22636,#22637),
(#22638,#22639),(#22640,#22641),(#22642,#22643),(#22644,#22645),(#22646,
#22647),(#22648,#22649),(#22650,#22651),(#22652,#22653),(#22654,#22655),
(#22656,#22657),(#22658,#22659),(#22660,#22661),(#22662,#22663),(#22664,
#22665),(#22666,#22667),(#22668,#22669),(#22670,#22671),(#22672,#22673),
(#22674,#22675),(#22676,#22677),(#22678,#22679),(#22680,#22681),(#22682,
#22683),(#22684,#22685),(#22686,#22687),(#22688,#22689),(#22690,#22691),
(#22692,#22693),(#22694,#22695),(#22696,#22697),(#22698,#22699),(#22700,
#22701),(#22702,#22703),(#22704,#22705),(#22706,#22707),(#22708,#22709),
(#22710,#22711),(#22712,#22713),(#22714,#22715),(#22716,#22717),(#22718,
#22719),(#22720,#22721),(#22722,#22723),(#22724,#22725),(#22726,#22727),
(#22728,#22729),(#22730,#22731),(#22732,#22733),(#22734,#22735),(#22736,
#22737),(#22738,#22739),(#22740,#22741),(#22742,#22743),(#22744,#22745),
(#22746,#22747),(#22748,#22749),(#22750,#22751),(#22752,#22753),(#22754,
#22755),(#22756,#22757),(#22758,#22759),(#22760,#22761),(#22762,#22763),
(#22764,#22765),(#22766,#22767),(#22768,#22769),(#22770,#22771),(#22772,
#22773),(#22774,#22775),(#22776,#22777),(#22778,#22779),(#22780,#22781),
(#22782,#22783),(#22784,#22785),(#22786,#22787),(#22788,#22789),(#22790,
#22791),(#22792,#22793),(#22794,#22795),(#22796,#22797),(#22798,#22799),
(#22800,#22801),(#22802,#22803),(#22804,#22805),(#22806,#22807),(#22808,
#22809),(#22810,#22811),(#22812,#22813),(#22814,#22815),(#22816,#22817),
(#22818,#22819),(#22820,#22821),(#22822,#22823),(#22824,#22825),(#22826,
#22827),(#22828,#22829),(#22830,#22831),(#22832,#22833),(#22834,#22835),
(#22836,#22837),(#22838,#22839),(#22840,#22841),(#22842,#22843),(#22844,
#22845),(#22846,#22847),(#22848,#22849),(#22850,#22851),(#22852,#22853),
(#22854,#22855),(#22856,#22857),(#22858,#22859),(#22860,#22861),(#22862,
#22863),(#22864,#22865),(#22866,#22867),(#22868,#22869),(#22870,#22871),
(#22872,#22873),(#22874,#22875),(#22876,#22877),(#22878,#22879),(#22880,
#22881),(#22882,#22883),(#22884,#22885),(#22886,#22887),(#22888,#22889),
(#22890,#22891),(#22892,#22893),(#22894,#22895),(#22896,#22897),(#22898,
#22899),(#22900,#22901),(#22902,#22903),(#22904,#22905),(#22906,#22907),
(#22908,#22909),(#22910,#22911),(#22912,#22913),(#22914,#22915),(#22916,
#22917),(#22918,#22919),(#22920,#22921),(#22922,#22923),(#22924,#22925),
(#22926,#22927),(#22928,#22929),(#22930,#22931),(#22932,#22933),(#22934,
#22935),(#22936,#22937),(#22938,#22939),(#22940,#22941),(#22942,#22943),
(#22944,#22945),(#22946,#22947),(#22948,#22949),(#22950,#22951),(#22952,
#22953),(#22954,#22955),(#22956,#22957),(#22958,#22959),(#22960,#22961),
(#22962,#22963),(#22964,#22965),(#22966,#22967),(#22968,#22969),(#22970,
#22971),(#22972,#22973),(#22974,#22975),(#22976,#22977),(#22978,#22979),
(#22980,#22981),(#22982,#22983),(#22984,#22985),(#22986,#22987),(#22988,
#22989),(#22990,#22991),(#22992,#22993),(#22994,#22995),(#22996,#22997),
(#22998,#22999),(#23000,#23001),(#23002,#23003),(#23004,#23005),(#23006,
#23007),(#23008,#23009),(#23010,#23011),(#23012,#23013),(#23014,#23015),
(#23016,#23017),(#23018,#23019),(#23020,#23021),(#23022,#23023),(#23024,
#23025),(#23026,#23027),(#23028,#23029),(#23030,#23031),(#23032,#23033),
(#23034,#23035),(#23036,#23037),(#23038,#23039),(#23040,#23041),(#23042,
#23043),(#23044,#23045),(#23046,#23047),(#23048,#23049),(#23050,#23051),
(#23052,#23053),(#23054,#23055),(#23056,#23057),(#23058,#23059),(#23060,
#23061),(#23062,#23063),(#23064,#23065),(#23066,#23067),(#23068,#23069),
(#23070,#23071),(#23072,#23073),(#23074,#23075),(#23076,#23077),(#23078,
#23079),(#23080,#23081),(#23082,#23083),(#23084,#23085),(#23086,#23087),
(#23088,#23089),(#23090,#23091),(#23092,#23093),(#23094,#23095),(#23096,
#23097),(#23098,#23099),(#23100,#23101),(#23102,#23103),(#23104,#23105),
(#23106,#23107),(#23108,#23109),(#23110,#23111),(#23112,#23113),(#23114,
#23115),(#23116,#23117),(#23118,#23119),(#23120,#23121),(#23122,#23123),
(#23124,#23125),(#23126,#23127),(#23128,#23129),(#23130,#23131),(#23132,
#23133),(#23134,#23135),(#23136,#23137),(#23138,#23139),(#23140,#23141),
(#23142,#23143),(#23144,#23145),(#23146,#23147),(#23148,#23149),(#23150,
#23151),(#23152,#23153),(#23154,#23155),(#23156,#23157),(#23158,#23159),
(#23160,#23161),(#23162,#23163),(#23164,#23165),(#23166,#23167),(#23168,
#23169),(#23170,#23171),(#23172,#23173),(#23174,#23175),(#23176,#23177),
(#23178,#23179),(#23180,#23181),(#23182,#23183),(#23184,#23185),(#23186,
#23187),(#23188,#23189),(#23190,#23191),(#23192,#23193),(#23194,#23195),
(#23196,#23197),(#23198,#23199),(#23200,#23201),(#23202,#23203),(#23204,
#23205),(#23206,#23207),(#23208,#23209),(#23210,#23211),(#23212,#23213),
(#23214,#23215),(#23216,#23217),(#23218,#23219),(#23220,#23221),(#23222,
#23223),(#23224,#23225),(#23226,#23227),(#23228,#23229),(#23230,#23231),
(#23232,#23233),(#23234,#23235),(#23236,#23237),(#23238,#23239),(#23240,
#23241),(#23242,#23243),(#23244,#23245),(#23246,#23247),(#23248,#23249),
(#23250,#23251),(#23252,#23253),(#23254,#23255),(#23256,#23257),(#23258,
#23259),(#23260,#23261),(#23262,#23263),(#23264,#23265),(#23266,#23267),
(#23268,#23269),(#23270,#23271),(#23272,#23273),(#23274,#23275),(#23276,
#23277),(#23278,#23279),(#23280,#23281),(#23282,#23283),(#23284,#23285),
(#23286,#23287),(#23288,#23289),(#23290,#23291),(#23292,#23293),(#23294,
#23295),(#23296,#23297),(#23298,#23299),(#23300,#23301),(#23302,#23303),
(#23304,#23305),(#23306,#23307),(#23308,#23309),(#23310,#23311),(#23312,
#23313),(#23314,#23315),(#23316,#23317),(#23318,#23319),(#23320,#23321),
(#23322,#23323),(#23324,#23325),(#23326,#23327),(#23328,#23329),(#23330,
#23331),(#23332,#23333),(#23334,#23335),(#23336,#23337),(#23338,#23339),
(#23340,#23341),(#23342,#23343),(#23344,#23345),(#23346,#23347),(#23348,
#23349),(#23350,#23351),(#23352,#23353),(#23354,#23355),(#23356,#23357),
(#23358,#23359),(#23360,#23361),(#23362,#23363),(#23364,#23365),(#23366,
#23367),(#23368,#23369),(#23370,#23371),(#23372,#23373),(#23374,#23375),
(#23376,#23377),(#23378,#23379),(#23380,#23381),(#23382,#23383),(#23384,
#23385),(#23386,#23387),(#23388,#23389),(#23390,#23391),(#23392,#23393),
(#23394,#23395),(#23396,#23397),(#23398,#23399),(#23400,#23401),(#23402,
#23403),(#23404,#23405),(#23406,#23407),(#23408,#23409),(#23410,#23411),
(#23412,#23413),(#23414,#23415),(#23416,#23417),(#23418,#23419),(#23420,
#23421),(#23422,#23423),(#23424,#23425),(#23426,#23427),(#23428,#23429),
(#23430,#23431),(#23432,#23433),(#23434,#23435),(#23436,#23437),(#23438,
#23439),(#23440,#23441),(#23442,#23443),(#23444,#23445),(#23446,#23447),
(#23448,#23449),(#23450,#23451),(#23452,#23453),(#23454,#23455),(#23456,
#23457),(#23458,#23459),(#23460,#23461),(#23462,#23463),(#23464,#23465),
(#23466,#23467),(#23468,#23469),(#23470,#23471),(#23472,#23473),(#23474,
#23475),(#23476,#23477),(#23478,#23479),(#23480,#23481),(#23482,#23483),
(#23484,#23485),(#23486,#23487),(#23488,#23489),(#23490,#23491),(#23492,
#23493),(#23494,#23495),(#23496,#23497),(#23498,#23499),(#23500,#23501),
(#23502,#23503),(#23504,#23505),(#23506,#23507),(#23508,#23509),(#23510,
#23511),(#23512,#23513),(#23514,#23515),(#23516,#23517),(#23518,#23519),
(#23520,#23521),(#23522,#23523),(#23524,#23525),(#23526,#23527),(#23528,
#23529),(#23530,#23531),(#23532,#23533),(#23534,#23535),(#23536,#23537),
(#23538,#23539),(#23540,#23541),(#23542,#23543),(#23544,#23545),(#23546,
#23547),(#23548,#23549),(#23550,#23551),(#23552,#23553),(#23554,#23555),
(#23556,#23557),(#23558,#23559),(#23560,#23561),(#23562,#23563),(#23564,
#23565),(#23566,#23567),(#23568,#23569),(#23570,#23571),(#23572,#23573),
(#23574,#23575),(#23576,#23577),(#23578,#23579),(#23580,#23581),(#23582,
#23583),(#23584,#23585),(#23586,#23587),(#23588,#23589),(#23590,#23591),
(#23592,#23593),(#23594,#23595),(#23596,#23597),(#23598,#23599),(#23600,
#23601),(#23602,#23603),(#23604,#23605),(#23606,#23607),(#23608,#23609),
(#23610,#23611),(#23612,#23613),(#23614,#23615),(#23616,#23617),(#23618,
#23619),(#23620,#23621),(#23622,#23623),(#23624,#23625),(#23626,#23627),
(#23628,#23629),(#23630,#23631),(#23632,#23633),(#23634,#23635),(#23636,
#23637),(#23638,#23639),(#23640,#23641),(#23642,#23643),(#23644,#23645),
(#23646,#23647),(#23648,#23649),(#23650,#23651),(#23652,#23653),(#23654,
#23655),(#23656,#23657),(#23658,#23659),(#23660,#23661),(#23662,#23663),
(#23664,#23665),(#23666,#23667),(#23668,#23669),(#23670,#23671),(#23672,
#23673),(#23674,#23675),(#23676,#23677),(#23678,#23679),(#23680,#23681),
(#23682,#23683),(#23684,#23685),(#23686,#23687),(#23688,#23689),(#23690,
#23691),(#23692,#23693),(#23694,#23695),(#23696,#23697),(#23698,#23699),
(#23700,#23701),(#23702,#23703),(#23704,#23705),(#23706,#23707),(#23708,
#23709),(#23710,#23711),(#23712,#23713),(#23714,#23715),(#23716,#23717),
(#23718,#23719),(#23720,#23721),(#23722,#23723),(#23724,#23725),(#23726,
#23727),(#23728,#23729),(#23730,#23731),(#23732,#23733),(#23734,#23735),
(#23736,#23737),(#23738,#23739),(#23740,#23741),(#23742,#23743),(#23744,
#23745),(#23746,#23747),(#23748,#23749),(#23750,#23751),(#23752,#23753),
(#23754,#23755),(#23756,#23757),(#23758,#23759),(#23760,#23761),(#23762,
#23763),(#23764,#23765),(#23766,#23767),(#23768,#23769),(#23770,#23771),
(#23772,#23773),(#23774,#23775),(#23776,#23777),(#23778,#23779),(#23780,
#23781),(#23782,#23783),(#23784,#23785),(#23786,#23787),(#23788,#23789),
(#23790,#23791),(#23792,#23793),(#23794,#23795),(#23796,#23797),(#23798,
#23799),(#23800,#23801),(#23802,#23803),(#23804,#23805),(#23806,#23807),
(#23808,#23809),(#23810,#23811),(#23812,#23813),(#23814,#23815),(#23816,
#23817),(#23818,#23819),(#23820,#23821),(#23822,#23823),(#23824,#23825),
(#23826,#23827),(#23828,#23829),(#23830,#23831),(#23832,#23833),(#23834,
#23835),(#23836,#23837),(#23838,#23839),(#23840,#23841),(#23842,#23843),
(#23844,#23845),(#23846,#23847),(#23848,#23849),(#23850,#23851),(#23852,
#23853),(#23854,#23855),(#23856,#23857),(#23858,#23859),(#23860,#23861),
(#23862,#23863),(#23864,#23865),(#23866,#23867),(#23868,#23869),(#23870,
#23871),(#23872,#23873),(#23874,#23875),(#23876,#23877),(#23878,#23879),
(#23880,#23881),(#23882,#23883),(#23884,#23885),(#23886,#23887),(#23888,
#23889),(#23890,#23891),(#23892,#23893),(#23894,#23895),(#23896,#23897),
(#23898,#23899),(#23900,#23901),(#23902,#23903),(#23904,#23905),(#23906,
#23907),(#23908,#23909),(#23910,#23911),(#23912,#23913),(#23914,#23915),
(#23916,#23917),(#23918,#23919),(#23920,#23921),(#23922,#23923),(#23924,
#23925),(#23926,#23927),(#23928,#23929),(#23930,#23931),(#23932,#23933),
(#23934,#23935),(#23936,#23937),(#23938,#23939),(#23940,#23941),(#23942,
#23943),(#23944,#23945),(#23946,#23947),(#23948,#23949),(#23950,#23951),
(#23952,#23953),(#23954,#23955),(#23956,#23957),(#23958,#23959),(#23960,
#23961),(#23962,#23963),(#23964,#23965),(#23966,#23967),(#23968,#23969),
(#23970,#23971),(#23972,#23973),(#23974,#23975),(#23976,#23977),(#23978,
#23979),(#23980,#23981),(#23982,#23983),(#23984,#23985),(#23986,#23987),
(#23988,#23989),(#23990,#23991),(#23992,#23993),(#23994,#23995),(#23996,
#23997),(#23998,#23999),(#24000,#24001),(#24002,#24003),(#24004,#24005),
(#24006,#24007),(#24008,#24009),(#24010,#24011),(#24012,#24013),(#24014,
#24015),(#24016,#24017),(#24018,#24019),(#24020,#24021),(#24022,#24023),
(#24024,#24025),(#24026,#24027),(#24028,#24029),(#24030,#24031),(#24032,
#24033),(#24034,#24035),(#24036,#24037),(#24038,#24039),(#24040,#24041),
(#24042,#24043),(#24044,#24045),(#24046,#24047),(#24048,#24049),(#24050,
#24051),(#24052,#24053),(#24054,#24055),(#24056,#24057),(#24058,#24059),
(#24060,#24061),(#24062,#24063),(#24064,#24065),(#24066,#24067),(#24068,
#24069),(#24070,#24071),(#24072,#24073),(#24074,#24075),(#24076,#24077),
(#24078,#24079),(#24080,#24081),(#24082,#24083),(#24084,#24085),(#24086,
#24087),(#24088,#24089),(#24090,#24091),(#24092,#24093),(#24094,#24095),
(#24096,#24097),(#24098,#24099),(#24100,#24101),(#24102,#24103),(#24104,
#24105),(#24106,#24107),(#24108,#24109),(#24110,#24111),(#24112,#24113),
(#24114,#24115),(#24116,#24117),(#24118,#24119),(#24120,#24121),(#24122,
#24123),(#24124,#24125),(#24126,#24127),(#24128,#24129),(#24130,#24131),
(#24132,#24133),(#24134,#24135),(#24136,#24137),(#24138,#24139),(#24140,
#24141),(#24142,#24143),(#24144,#24145),(#24146,#24147),(#24148,#24149),
(#24150,#24151),(#24152,#24153),(#24154,#24155),(#24156,#24157),(#24158,
#24159),(#24160,#24161),(#24162,#24163),(#24164,#24165),(#24166,#24167),
(#24168,#24169),(#24170,#24171),(#24172,#24173),(#24174,#24175),(#24176,
#24177),(#24178,#24179),(#24180,#24181),(#24182,#24183),(#24184,#24185),
(#24186,#24187),(#24188,#24189),(#24190,#24191),(#24192,#24193),(#24194,
#24195),(#24196,#24197),(#24198,#24199),(#24200,#24201),(#24202,#24203),
(#24204,#24205),(#24206,#24207),(#24208,#24209),(#24210,#24211),(#24212,
#24213),(#24214,#24215),(#24216,#24217),(#24218,#24219),(#24220,#24221),
(#24222,#24223),(#24224,#24225),(#24226,#24227),(#24228,#24229),(#24230,
#24231),(#24232,#24233),(#24234,#24235),(#24236,#24237),(#24238,#24239),
(#24240,#24241),(#24242,#24243),(#24244,#24245),(#24246,#24247),(#24248,
#24249),(#24250,#24251),(#24252,#24253),(#24254,#24255),(#24256,#24257),
(#24258,#24259),(#24260,#24261),(#24262,#24263),(#24264,#24265),(#24266,
#24267),(#24268,#24269),(#24270,#24271),(#24272,#24273),(#24274,#24275),
(#24276,#24277),(#24278,#24279),(#24280,#24281),(#24282,#24283),(#24284,
#24285),(#24286,#24287),(#24288,#24289),(#24290,#24291),(#24292,#24293),
(#24294,#24295),(#24296,#24297),(#24298,#24299),(#24300,#24301),(#24302,
#24303),(#24304,#24305),(#24306,#24307),(#24308,#24309),(#24310,#24311),
(#24312,#24313),(#24314,#24315),(#24316,#24317),(#24318,#24319),(#24320,
#24321),(#24322,#24323),(#24324,#24325),(#24326,#24327),(#24328,#24329),
(#24330,#24331),(#24332,#24333),(#24334,#24335),(#24336,#24337),(#24338,
#24339),(#24340,#24341),(#24342,#24343),(#24344,#24345),(#24346,#24347),
(#24348,#24349),(#24350,#24351),(#24352,#24353),(#24354,#24355),(#24356,
#24357),(#24358,#24359),(#24360,#24361),(#24362,#24363),(#24364,#24365),
(#24366,#24367),(#24368,#24369),(#24370,#24371),(#24372,#24373),(#24374,
#24375),(#24376,#24377),(#24378,#24379),(#24380,#24381),(#24382,#24383),
(#24384,#24385),(#24386,#24387),(#24388,#24389),(#24390,#24391),(#24392,
#24393),(#24394,#24395),(#24396,#24397),(#24398,#24399),(#24400,#24401),
(#24402,#24403),(#24404,#24405),(#24406,#24407),(#24408,#24409),(#24410,
#24411),(#24412,#24413),(#24414,#24415),(#24416,#24417),(#24418,#24419),
(#24420,#24421),(#24422,#24423),(#24424,#24425),(#24426,#24427),(#24428,
#24429),(#24430,#24431),(#24432,#24433),(#24434,#24435),(#24436,#24437),
(#24438,#24439),(#24440,#24441),(#24442,#24443),(#24444,#24445),(#24446,
#24447),(#24448,#24449),(#24450,#24451),(#24452,#24453),(#24454,#24455),
(#24456,#24457),(#24458,#24459),(#24460,#24461),(#24462,#24463),(#24464,
#24465),(#24466,#24467),(#24468,#24469),(#24470,#24471),(#24472,#24473),
(#24474,#24475),(#24476,#24477),(#24478,#24479),(#24480,#24481),(#24482,
#24483),(#24484,#24485),(#24486,#24487),(#24488,#24489),(#24490,#24491),
(#24492,#24493),(#24494,#24495),(#24496,#24497),(#24498,#24499),(#24500,
#24501),(#24502,#24503),(#24504,#24505),(#24506,#24507),(#24508,#24509),
(#24510,#24511),(#24512,#24513),(#24514,#24515),(#24516,#24517),(#24518,
#24519),(#24520,#24521),(#24522,#24523),(#24524,#24525),(#24526,#24527),
(#24528,#24529),(#24530,#24531),(#24532,#24533),(#24534,#24535),(#24536,
#24537),(#24538,#24539),(#24540,#24541),(#24542,#24543),(#24544,#24545),
(#24546,#24547),(#24548,#24549),(#24550,#24551),(#24552,#24553),(#24554,
#24555),(#24556,#24557),(#24558,#24559),(#24560,#24561),(#24562,#24563),
(#24564,#24565),(#24566,#24567),(#24568,#24569),(#24570,#24571),(#24572,
#24573),(#24574,#24575),(#24576,#24577),(#24578,#24579),(#24580,#24581),
(#24582,#24583),(#24584,#24585),(#24586,#24587),(#24588,#24589),(#24590,
#24591),(#24592,#24593),(#24594,#24595),(#24596,#24597),(#24598,#24599),
(#24600,#24601),(#24602,#24603),(#24604,#24605),(#24606,#24607),(#24608,
#24609),(#24610,#24611),(#24612,#24613),(#24614,#24615),(#24616,#24617),
(#24618,#24619),(#24620,#24621),(#24622,#24623),(#24624,#24625),(#24626,
#24627),(#24628,#24629),(#24630,#24631),(#24632,#24633),(#24634,#24635),
(#24636,#24637),(#24638,#24639),(#24640,#24641),(#24642,#24643),(#24644,
#24645),(#24646,#24647),(#24648,#24649),(#24650,#24651),(#24652,#24653),
(#24654,#24655),(#24656,#24657),(#24658,#24659),(#24660,#24661),(#24662,
#24663),(#24664,#24665),(#24666,#24667),(#24668,#24669),(#24670,#24671),
(#24672,#24673),(#24674,#24675),(#24676,#24677),(#24678,#24679),(#24680,
#24681),(#24682,#24683),(#24684,#24685),(#24686,#24687),(#24688,#24689),
(#24690,#24691),(#24692,#24693),(#24694,#24695),(#24696,#24697),(#24698,
#24699),(#24700,#24701),(#24702,#24703),(#24704,#24705),(#24706,#24707),
(#24708,#24709),(#24710,#24711),(#24712,#24713),(#24714,#24715),(#24716,
#24717),(#24718,#24719),(#24720,#24721),(#24722,#24723),(#24724,#24725),
(#24726,#24727),(#24728,#24729),(#24730,#24731),(#24732,#24733),(#24734,
#24735),(#24736,#24737),(#24738,#24739),(#24740,#24741),(#24742,#24743),
(#24744,#24745),(#24746,#24747),(#24748,#24749),(#24750,#24751),(#24752,
#24753),(#24754,#24755),(#24756,#24757),(#24758,#24759),(#24760,#24761),
(#24762,#24763),(#24764,#24765),(#24766,#24767),(#24768,#24769),(#24770,
#24771),(#24772,#24773),(#24774,#24775),(#24776,#24777),(#24778,#24779),
(#24780,#24781),(#24782,#24783),(#24784,#24785),(#24786,#24787),(#24788,
#24789),(#24790,#24791),(#24792,#24793),(#24794,#24795),(#24796,#24797),
(#24798,#24799),(#24800,#24801),(#24802,#24803),(#24804,#24805),(#24806,
#24807),(#24808,#24809),(#24810,#24811),(#24812,#24813),(#24814,#24815),
(#24816,#24817),(#24818,#24819),(#24820,#24821),(#24822,#24823),(#24824,
#24825),(#24826,#24827),(#24828,#24829),(#24830,#24831),(#24832,#24833),
(#24834,#24835),(#24836,#24837),(#24838,#24839),(#24840,#24841),(#24842,
#24843),(#24844,#24845),(#24846,#24847),(#24848,#24849),(#24850,#24851),
(#24852,#24853),(#24854,#24855),(#24856,#24857),(#24858,#24859),(#24860,
#24861),(#24862,#24863),(#24864,#24865),(#24866,#24867),(#24868,#24869),
(#24870,#24871),(#24872,#24873),(#24874,#24875),(#24876,#24877),(#24878,
#24879),(#24880,#24881),(#24882,#24883),(#24884,#24885),(#24886,#24887),
(#24888,#24889),(#24890,#24891),(#24892,#24893),(#24894,#24895),(#24896,
#24897),(#24898,#24899),(#24900,#24901),(#24902,#24903),(#24904,#24905),
(#24906,#24907),(#24908,#24909),(#24910,#24911),(#24912,#24913),(#24914,
#24915),(#24916,#24917),(#24918,#24919),(#24920,#24921),(#24922,#24923),
(#24924,#24925),(#24926,#24927),(#24928,#24929),(#24930,#24931),(#24932,
#24933),(#24934,#24935),(#24936,#24937),(#24938,#24939),(#24940,#24941),
(#24942,#24943),(#24944,#24945),(#24946,#24947),(#24948,#24949),(#24950,
#24951),(#24952,#24953),(#24954,#24955),(#24956,#24957),(#24958,#24959),
(#24960,#24961),(#24962,#24963),(#24964,#24965),(#24966,#24967),(#24968,
#24969),(#24970,#24971),(#24972,#24973),(#24974,#24975),(#24976,#24977),
(#24978,#24979),(#24980,#24981),(#24982,#24983),(#24984,#24985),(#24986,
#24987),(#24988,#24989),(#24990,#24991),(#24992,#24993),(#24994,#24995),
(#24996,#24997),(#24998,#24999),(#25000,#25001),(#25002,#25003),(#25004,
#25005),(#25006,#25007),(#25008,#25009),(#25010,#25011),(#25012,#25013),
(#25014,#25015),(#25016,#25017),(#25018,#25019),(#25020,#25021),(#25022,
#25023),(#25024,#25025),(#25026,#25027),(#25028,#25029),(#25030,#25031),
(#25032,#25033),(#25034,#25035),(#25036,#25037),(#25038,#25039),(#25040,
#25041),(#25042,#25043),(#25044,#25045),(#25046,#25047),(#25048,#25049),
(#25050,#25051),(#25052,#25053),(#25054,#25055),(#25056,#25057),(#25058,
#25059),(#25060,#25061),(#25062,#25063),(#25064,#25065),(#25066,#25067),
(#25068,#25069),(#25070,#25071),(#25072,#25073),(#25074,#25075),(#25076,
#25077),(#25078,#25079),(#25080,#25081),(#25082,#25083),(#25084,#25085),
(#25086,#25087),(#25088,#25089),(#25090,#25091),(#25092,#25093),(#25094,
#25095),(#25096,#25097),(#25098,#25099),(#25100,#25101),(#25102,#25103),
(#25104,#25105),(#25106,#25107),(#25108,#25109),(#25110,#25111),(#25112,
#25113),(#25114,#25115),(#25116,#25117),(#25118,#25119),(#25120,#25121),
(#25122,#25123),(#25124,#25125),(#25126,#25127),(#25128,#25129),(#25130,
#25131),(#25132,#25133),(#25134,#25135),(#25136,#25137),(#25138,#25139),
(#25140,#25141),(#25142,#25143),(#25144,#25145),(#25146,#25147),(#25148,
#25149),(#25150,#25151),(#25152,#25153),(#25154,#25155),(#25156,#25157),
(#25158,#25159),(#25160,#25161),(#25162,#25163),(#25164,#25165),(#25166,
#25167),(#25168,#25169),(#25170,#25171),(#25172,#25173),(#25174,#25175),
(#25176,#25177),(#25178,#25179),(#25180,#25181),(#25182,#25183),(#25184,
#25185),(#25186,#25187),(#25188,#25189),(#25190,#25191),(#25192,#25193),
(#25194,#25195),(#25196,#25197),(#25198,#25199),(#25200,#25201),(#25202,
#25203),(#25204,#25205),(#25206,#25207),(#25208,#25209),(#25210,#25211),
(#25212,#25213),(#25214,#25215),(#25216,#25217),(#25218,#25219),(#25220,
#25221),(#25222,#25223),(#25224,#25225),(#25226,#25227),(#25228,#25229),
(#25230,#25231),(#25232,#25233),(#25234,#25235),(#25236,#25237),(#25238,
#25239),(#25240,#25241),(#25242,#25243),(#25244,#25245),(#25246,#25247),
(#25248,#25249),(#25250,#25251),(#25252,#25253),(#25254,#25255),(#25256,
#25257),(#25258,#25259),(#25260,#25261),(#25262,#25263),(#25264,#25265),
(#25266,#25267),(#25268,#25269),(#25270,#25271),(#25272,#25273),(#25274,
#25275),(#25276,#25277),(#25278,#25279),(#25280,#25281),(#25282,#25283),
(#25284,#25285),(#25286,#25287),(#25288,#25289),(#25290,#25291),(#25292,
#25293),(#25294,#25295),(#25296,#25297),(#25298,#25299),(#25300,#25301),
(#25302,#25303),(#25304,#25305),(#25306,#25307),(#25308,#25309),(#25310,
#25311),(#25312,#25313),(#25314,#25315),(#25316,#25317),(#25318,#25319),
(#25320,#25321),(#25322,#25323),(#25324,#25325),(#25326,#25327),(#25328,
#25329),(#25330,#25331),(#25332,#25333),(#25334,#25335),(#25336,#25337),
(#25338,#25339),(#25340,#25341),(#25342,#25343),(#25344,#25345),(#25346,
#25347),(#25348,#25349),(#25350,#25351),(#25352,#25353),(#25354,#25355),
(#25356,#25357),(#25358,#25359),(#25360,#25361),(#25362,#25363),(#25364,
#25365),(#25366,#25367),(#25368,#25369),(#25370,#25371),(#25372,#25373),
(#25374,#25375),(#25376,#25377),(#25378,#25379),(#25380,#25381),(#25382,
#25383),(#25384,#25385),(#25386,#25387),(#25388,#25389),(#25390,#25391),
(#25392,#25393),(#25394,#25395),(#25396,#25397),(#25398,#25399),(#25400,
#25401),(#25402,#25403),(#25404,#25405),(#25406,#25407),(#25408,#25409),
(#25410,#25411),(#25412,#25413),(#25414,#25415),(#25416,#25417),(#25418,
#25419),(#25420,#25421),(#25422,#25423),(#25424,#25425),(#25426,#25427),
(#25428,#25429),(#25430,#25431),(#25432,#25433),(#25434,#25435),(#25436,
#25437),(#25438,#25439),(#25440,#25441),(#25442,#25443),(#25444,#25445),
(#25446,#25447),(#25448,#25449),(#25450,#25451),(#25452,#25453),(#25454,
#25455),(#25456,#25457),(#25458,#25459),(#25460,#25461),(#25462,#25463),
(#25464,#25465),(#25466,#25467),(#25468,#25469),(#25470,#25471),(#25472,
#25473),(#25474,#25475),(#25476,#25477),(#25478,#25479),(#25480,#25481),
(#25482,#25483),(#25484,#25485),(#25486,#25487),(#25488,#25489),(#25490,
#25491),(#25492,#25493),(#25494,#25495),(#25496,#25497),(#25498,#25499),
(#25500,#25501),(#25502,#25503),(#25504,#25505),(#25506,#25507),(#25508,
#25509),(#25510,#25511),(#25512,#25513),(#25514,#25515),(#25516,#25517),
(#25518,#25519),(#25520,#25521),(#25522,#25523),(#25524,#25525),(#25526,
#25527),(#25528,#25529),(#25530,#25531),(#25532,#25533),(#25534,#25535),
(#25536,#25537),(#25538,#25539),(#25540,#25541),(#25542,#25543),(#25544,
#25545),(#25546,#25547),(#25548,#25549),(#25550,#25551),(#25552,#25553),
(#25554,#25555),(#25556,#25557),(#25558,#25559),(#25560,#25561),(#25562,
#25563),(#25564,#25565),(#25566,#25567),(#25568,#25569),(#25570,#25571),
(#25572,#25573),(#25574,#25575),(#25576,#25577),(#25578,#25579),(#25580,
#25581),(#25582,#25583),(#25584,#25585),(#25586,#25587),(#25588,#25589),
(#25590,#25591),(#25592,#25593),(#25594,#25595),(#25596,#25597),(#25598,
#25599),(#25600,#25601),(#25602,#25603),(#25604,#25605),(#25606,#25607),
(#25608,#25609),(#25610,#25611),(#25612,#25613),(#25614,#25615),(#25616,
#25617),(#25618,#25619),(#25620,#25621),(#25622,#25623),(#25624,#25625),
(#25626,#25627),(#25628,#25629),(#25630,#25631),(#25632,#25633),(#25634,
#25635),(#25636,#25637),(#25638,#25639),(#25640,#25641),(#25642,#25643),
(#25644,#25645),(#25646,#25647),(#25648,#25649),(#25650,#25651),(#25652,
#25653),(#25654,#25655),(#25656,#25657),(#25658,#25659),(#25660,#25661),
(#25662,#25663),(#25664,#25665),(#25666,#25667),(#25668,#25669),(#25670,
#25671),(#25672,#25673),(#25674,#25675),(#25676,#25677),(#25678,#25679),
(#25680,#25681),(#25682,#25683),(#25684,#25685),(#25686,#25687),(#25688,
#25689),(#25690,#25691),(#25692,#25693),(#25694,#25695),(#25696,#25697),
(#25698,#25699),(#25700,#25701),(#25702,#25703),(#25704,#25705),(#25706,
#25707),(#25708,#25709),(#25710,#25711),(#25712,#25713),(#25714,#25715),
(#25716,#25717),(#25718,#25719),(#25720,#25721),(#25722,#25723),(#25724,
#25725),(#25726,#25727),(#25728,#25729),(#25730,#25731),(#25732,#25733),
(#25734,#25735),(#25736,#25737),(#25738,#25739),(#25740,#25741),(#25742,
#25743),(#25744,#25745),(#25746,#25747),(#25748,#25749),(#25750,#25751),
(#25752,#25753),(#25754,#25755),(#25756,#25757),(#25758,#25759),(#25760,
#25761),(#25762,#25763),(#25764,#25765),(#25766,#25767),(#25768,#25769),
(#25770,#25771),(#25772,#25773),(#25774,#25775),(#25776,#25777),(#25778,
#25779),(#25780,#25781),(#25782,#25783),(#25784,#25785),(#25786,#25787),
(#25788,#25789),(#25790,#25791),(#25792,#25793),(#25794,#25795),(#25796,
#25797),(#25798,#25799),(#25800,#25801),(#25802,#25803),(#25804,#25805),
(#25806,#25807),(#25808,#25809),(#25810,#25811),(#25812,#25813),(#25814,
#25815),(#25816,#25817),(#25818,#25819),(#25820,#25821),(#25822,#25823),
(#25824,#25825),(#25826,#25827),(#25828,#25829),(#25830,#25831),(#25832,
#25833),(#25834,#25835),(#25836,#25837),(#25838,#25839),(#25840,#25841),
(#25842,#25843),(#25844,#25845),(#25846,#25847),(#25848,#25849),(#25850,
#25851),(#25852,#25853),(#25854,#25855),(#25856,#25857),(#25858,#25859),
(#25860,#25861),(#25862,#25863),(#25864,#25865),(#25866,#25867),(#25868,
#25869),(#25870,#25871),(#25872,#25873),(#25874,#25875),(#25876,#25877),
(#25878,#25879),(#25880,#25881),(#25882,#25883),(#25884,#25885),(#25886,
#25887),(#25888,#25889),(#25890,#25891),(#25892,#25893),(#25894,#25895),
(#25896,#25897),(#25898,#25899),(#25900,#25901),(#25902,#25903),(#25904,
#25905),(#25906,#25907),(#25908,#25909),(#25910,#25911),(#25912,#25913),
(#25914,#25915),(#25916,#25917),(#25918,#25919),(#25920,#25921),(#25922,
#25923),(#25924,#25925),(#25926,#25927),(#25928,#25929),(#25930,#25931),
(#25932,#25933),(#25934,#25935),(#25936,#25937),(#25938,#25939),(#25940,
#25941),(#25942,#25943),(#25944,#25945),(#25946,#25947),(#25948,#25949)),
 .UNSPECIFIED.,.F.,.F.,.F.,(4,1,1,1,1,1,1,1,1,1,1,1,1,1,1,1,1,1,1,1,1,1,
1,1,1,1,1,1,1,1,1,1,1,1,1,1,1,1,1,1,1,1,1,1,1,1,1,1,1,1,1,1,1,1,1,1,1,1,
1,1,1,1,1,1,1,1,1,1,1,1,1,1,1,1,1,1,1,1,1,1,1,1,1,1,1,1,1,1,1,1,1,1,1,1,
1,1,1,1,1,1,1,1,1,1,1,1,1,1,1,1,1,1,1,1,1,1,1,1,1,1,1,1,1,1,1,1,1,1,1,1,
1,1,1,1,1,1,1,1,1,1,1,1,1,1,1,1,1,1,1,1,1,1,1,1,1,1,1,1,1,1,1,1,1,1,1,1,
1,1,1,1,1,1,1,1,1,1,1,1,1,1,1,1,1,1,1,1,1,1,1,1,1,1,1,1,1,1,1,1,1,1,1,1,
1,1,1,1,1,1,1,1,1,1,1,1,1,1,1,1,1,1,1,1,1,1,1,1,1,1,1,1,1,1,1,1,1,1,1,1,
1,1,1,1,1,1,1,1,1,1,1,1,1,1,1,1,1,1,1,1,1,1,1,1,1,1,1,1,1,1,1,1,1,1,1,1,
1,1,1,1,1,1,1,1,1,1,1,1,1,1,1,1,1,1,1,1,1,1,1,1,1,1,1,1,1,1,1,1,1,1,1,1,
1,1,1,1,1,1,1,1,1,1,1,1,1,1,1,1,1,1,1,1,1,1,1,1,1,1,1,1,1,1,1,1,1,1,1,1,
1,1,1,1,1,1,1,1,1,1,1,1,1,1,1,1,1,1,1,1,1,1,1,1,1,1,1,1,1,1,1,1,1,1,1,1,
1,1,1,1,1,1,1,1,1,1,1,1,1,1,1,1,1,1,1,1,1,1,1,1,1,1,1,1,1,1,1,1,1,1,1,1,
1,1,1,1,1,1,1,1,1,1,1,1,1,1,1,1,1,1,1,1,1,1,1,1,1,1,1,1,1,1,1,1,1,1,1,1,
1,1,1,1,1,1,1,1,1,1,1,1,1,1,1,1,1,1,1,1,1,1,1,1,1,1,1,1,1,1,1,1,1,1,1,1,
1,1,1,1,1,1,1,1,1,1,1,1,1,1,1,1,1,1,1,1,1,1,1,1,1,1,1,1,1,1,1,1,1,1,1,1,
1,1,1,1,1,1,1,1,1,1,1,1,1,1,1,1,1,1,1,1,1,1,1,1,1,1,1,1,1,1,1,1,1,1,1,1,
1,1,1,1,1,1,1,1,1,1,1,1,1,1,1,1,1,1,1,1,1,1,1,1,1,1,1,1,1,1,1,1,1,1,1,1,
1,1,1,1,1,1,1,1,1,1,1,1,1,1,1,1,1,1,1,1,1,1,1,1,1,1,1,1,1,1,1,1,1,1,1,1,
1,1,1,1,1,1,1,1,1,1,1,1,1,1,1,1,1,1,1,1,1,1,1,1,1,1,1,1,1,1,1,1,1,1,1,1,
1,1,1,1,1,1,1,1,1,1,1,1,1,1,1,1,1,1,1,1,1,1,1,1,1,1,1,1,1,1,1,1,1,1,1,1,
1,1,1,1,1,1,1,1,1,1,1,1,1,1,1,1,1,1,1,1,1,1,1,1,1,1,1,1,1,1,1,1,1,1,1,1,
1,1,1,1,1,1,1,1,1,1,1,1,1,1,1,1,1,1,1,1,1,1,1,1,1,1,1,1,1,1,1,1,1,1,1,1,
1,1,1,1,1,1,1,1,1,1,1,1,1,1,1,1,1,1,1,1,1,1,1,1,1,1,1,1,1,1,1,1,1,1,1,1,
1,1,1,1,1,1,1,1,1,1,1,1,1,1,1,1,1,1,1,1,1,1,1,1,1,1,1,1,1,1,1,1,1,1,1,1,
1,1,1,1,1,1,1,1,1,1,1,1,1,1,1,1,1,1,1,1,1,1,1,1,1,1,1,1,1,1,1,1,1,1,1,1,
1,1,1,1,1,1,1,1,1,1,1,1,1,1,1,1,1,1,1,1,1,1,1,1,1,1,1,1,1,1,1,1,1,1,1,1,
1,1,1,1,1,1,1,1,1,1,1,1,1,1,1,1,1,1,1,1,1,1,1,1,1,1,1,1,1,1,1,1,1,1,1,1,
1,1,1,1,1,1,1,1,1,1,1,1,1,1,1,1,1,1,1,1,1,1,1,1,1,1,1,1,1,1,1,1,1,1,1,1,
1,1,1,1,1,1,1,1,1,1,1,1,1,1,1,1,1,1,1,1,1,1,1,1,1,1,1,1,1,1,1,1,1,1,1,1,
1,1,1,1,1,1,1,1,1,1,1,1,1,1,1,1,1,1,1,1,1,1,1,1,1,1,1,1,1,1,1,1,1,1,1,1,
1,1,1,1,1,1,1,1,1,1,1,1,1,1,1,1,1,1,1,1,1,1,1,1,1,1,1,1,1,1,1,1,1,1,1,1,
1,1,1,1,1,1,1,1,1,1,1,1,1,1,1,1,1,1,1,1,1,1,1,1,1,1,1,1,1,1,1,1,1,1,1,1,
1,1,1,1,1,1,1,1,1,1,1,1,1,1,1,1,1,1,1,1,1,1,1,1,1,1,1,1,1,1,1,1,1,1,1,1,
1,1,1,1,1,1,1,1,1,1,1,1,1,1,1,1,1,1,1,1,1,1,1,1,1,1,1,1,1,1,1,1,1,1,1,1,
1,1,1,1,1,1,1,1,1,1,1,1,1,1,1,1,1,1,1,1,1,1,1,1,1,1,1,1,1,1,1,1,1,1,1,1,
1,1,1,1,1,1,1,1,1,1,1,1,1,1,1,1,1,1,1,1,1,1,1,1,1,1,1,1,1,1,1,1,1,1,1,1,
1,1,1,1,1,1,1,1,1,1,1,1,1,1,1,1,1,1,1,1,1,1,1,1,1,1,1,1,1,1,1,1,1,1,1,1,
1,1,1,1,1,1,1,1,1,1,1,1,1,1,1,1,1,1,1,1,1,1,1,1,1,1,1,1,1,1,1,1,1,1,1,1,
1,1,1,1,1,1,1,1,1,1,1,1,1,1,1,1,1,1,1,1,1,1,1,1,1,1,1,1,1,1,1,1,1,1,1,1,
1,1,1,1,1,1,1,1,1,1,1,1,1,1,1,1,1,1,1,1,1,1,1,1,1,1,1,1,1,1,1,1,1,1,1,1,
1,1,1,1,1,1,1,1,1,1,1,1,1,1,1,1,1,1,1,1,1,1,1,1,1,1,1,1,1,1,1,1,1,1,1,1,
1,1,1,1,1,1,1,1,1,1,1,1,1,1,1,1,1,1,1,1,1,1,1,1,1,1,1,1,1,1,1,1,1,1,1,1,
1,1,1,1,1,1,1,1,1,1,1,1,1,1,1,1,1,1,1,1,1,1,1,1,1,1,1,1,1,1,1,1,1,1,1,1,
1,1,1,1,1,1,1,1,1,1,1,1,1,1,1,1,1,1,1,1,1,1,1,1,1,1,1,1,1,1,1,1,1,1,1,1,
1,1,1,1,1,1,1,1,1,1,1,1,1,1,1,1,1,1,1,1,1,1,1,1,1,1,1,1,1,1,1,1,1,1,1,1,
1,1,1,1,1,1,1,1,1,1,1,1,1,1,1,1,1,1,1,1,1,1,1,1,1,1,1,1,1,1,1,1,1,1,1,1,
1,1,1,1,1,1,1,1,1,1,1,1,1,1,1,1,1,1,1,1,1,1,1,1,1,1,1,1,1,1,1,1,1,1,1,1,
1,1,1,1,1,1,1,1,1,1,1,1,1,1,1,1,1,1,1,1,1,1,1,1,1,1,1,1,1,1,1,1,1,1,1,1,
1,1,1,1,1,1,1,1,1,1,1,1,1,1,1,1,1,1,1,1,1,1,1,1,1,1,1,1,1,1,1,1,1,1,1,1,
1,1,1,1,1,1,1,1,1,1,1,1,1,1,1,1,1,1,1,1,1,1,1,1,1,1,1,1,1,1,1,1,1,1,1,1,
1,1,1,1,1,1,1,1,1,1,1,1,1,1,1,1,1,1,1,1,1,1,1,1,1,1,1,1,1,1,1,1,1,1,1,1,
1,1,1,1,1,1,1,1,1,1,1,1,1,1,1,1,1,1,1,1,1,1,1,1,1,1,1,1,1,1,1,1,1,1,1,1,
1,1,1,1,1,1,1,1,1,1,1,1,1,1,1,1,1,1,1,1,1,1,1,1,1,1,1,1,1,1,1,1,1,1,1,1,
1,1,1,1,1,1,1,1,1,1,1,1,1,1,1,1,1,1,1,1,1,1,1,1,1,1,1,1,1,1,1,1,1,1,1,1,
1,1,1,1,1,1,1,1,1,1,1,1,1,1,1,1,1,1,1,1,1,1,1,1,1,1,1,1,1,1,1,1,1,1,1,1,
1,1,1,1,1,1,1,1,1,1,1,1,1,1,1,1,1,1,1,1,1,1,1,1,1,1,1,1,1,1,1,1,1,1,1,1,
1,1,1,1,1,1,1,1,1,1,1,1,1,1,1,1,1,1,1,1,1,1,1,1,1,1,1,1,1,1,1,1,1,1,1,1,
1,1,1,1,1,1,1,1,1,1,1,1,1,1,1,1,1,1,1,1,1,1,1,1,1,1,1,1,1,1,1,1,1,1,1,1,
1,1,1,1,1,1,1,1,1,1,1,1,1,1,1,1,1,1,1,1,1,1,1,1,1,1,1,1,1,1,1,1,1,1,1,1,
1,1,1,1,1,1,1,1,1,1,1,1,1,1,1,1,1,1,1,1,1,1,1,1,1,1,1,1,1,1,1,1,1,1,1,1,
1,1,1,1,1,1,1,1,1,1,1,1,1,1,1,1,1,1,1,1,1,1,1,1,1,1,1,1,1,1,1,1,1,1,1,1,
1,1,1,1,1,1,1,1,1,1,1,1,1,1,1,1,1,1,1,1,1,1,1,1,1,1,1,1,1,1,1,1,1,1,1,1,
1,1,1,1,1,1,1,1,1,1,1,1,1,1,1,1,1,1,1,1,1,1,1,1,1,1,1,1,1,1,1,1,1,1,1,1,
1,1,1,1,1,1,1,1,1,1,1,1,1,1,1,1,1,1,1,1,1,1,1,1,1,1,1,1,1,1,1,1,1,1,1,1,
1,1,1,1,1,1,1,1,1,1,1,1,1,1,1,1,1,1,1,1,1,1,1,1,1,1,1,1,1,1,1,1,1,1,1,1,
1,1,1,1,1,1,1,1,1,1,1,1,1,1,1,1,1,1,1,1,1,1,1,1,1,1,1,1,1,1,1,1,1,1,1,1,
1,1,1,1,1,1,1,1,1,1,1,1,1,1,1,1,1,1,1,1,1,1,1,1,1,1,1,1,1,1,1,1,1,1,1,1,
1,1,1,1,1,1,1,1,1,1,1,1,1,1,1,1,1,1,1,1,1,1,1,1,1,1,1,1,1,1,1,1,1,1,1,1,
1,1,1,1,1,1,1,1,1,1,1,1,1,1,1,1,1,1,1,1,1,1,1,1,1,1,1,1,1,1,1,1,1,1,1,1,
1,1,1,1,1,1,1,1,1,1,1,1,1,1,1,1,1,1,1,1,1,1,1,1,1,1,1,1,1,1,1,1,1,1,1,1,
1,1,1,1,1,1,1,1,1,1,1,1,1,1,1,1,1,1,1,1,1,1,1,1,1,1,1,1,1,1,1,1,1,1,1,1,
1,1,1,1,1,1,1,1,1,1,1,1,1,1,1,1,1,1,1,1,1,1,1,1,1,1,1,1,1,1,1,1,1,1,1,1,
1,1,1,1,1,1,1,1,1,1,1,1,1,1,1,1,1,1,1,1,1,1,1,1,1,1,1,1,1,1,1,1,1,1,1,1,
1,1,1,1,1,1,1,1,1,1,1,1,1,1,1,1,1,1,1,1,1,1,1,1,1,1,1,1,1,1,1,1,1,1,1,1,
1,1,1,1,1,1,1,1,1,1,1,1,1,1,1,1,1,1,1,1,1,1,1,1,1,1,1,1,1,1,1,1,1,1,1,1,
1,1,1,1,1,1,1,1,1,1,1,1,1,1,1,1,1,1,1,1,1,1,1,1,1,1,1,1,1,1,1,1,1,1,1,1,
1,1,1,1,1,1,1,1,1,1,1,1,1,1,1,1,1,1,1,1,1,1,1,1,1,1,1,1,1,1,1,1,1,1,1,1,
1,1,1,1,1,1,1,1,1,1,1,1,1,1,1,1,1,1,1,1,1,1,1,1,1,1,1,1,1,1,1,1,1,1,1,1,
1,1,1,1,1,1,1,1,1,1,1,1,1,1,1,1,1,1,1,1,1,1,1,1,1,1,1,1,1,1,1,1,1,1,1,1,
1,1,1,1,1,1,1,1,1,1,1,1,1,1,1,1,1,1,1,1,1,1,1,1,1,1,1,1,1,1,1,1,1,1,1,1,
1,1,1,1,1,1,1,1,1,1,1,1,1,1,1,1,1,1,1,1,1,1,1,1,1,1,1,1,1,1,1,1,1,1,1,1,
1,1,1,1,1,1,1,1,1,1,1,1,1,1,1,1,1,1,1,1,1,1,1,1,1,1,1,1,1,1,1,1,1,1,1,1,
1,1,1,1,1,1,1,1,1,1,1,1,1,1,1,1,1,1,1,1,1,1,1,1,1,1,1,1,1,1,1,1,1,1,1,1,
1,1,1,1,1,1,1,1,1,1,1,1,1,1,1,1,1,1,1,1,1,1,1,1,1,1,1,1,1,1,1,1,1,1,1,1,
1,1,1,1,1,1,1,1,1,1,1,1,1,1,1,1,1,1,1,1,1,1,1,1,1,1,1,1,1,1,1,1,1,1,1,1,
1,1,1,1,1,1,1,1,1,1,1,1,1,1,1,1,1,1,1,1,1,1,1,1,1,1,1,1,1,1,1,1,1,1,1,1,
1,1,1,1,1,1,1,1,1,1,1,1,1,1,1,1,1,1,1,1,1,1,1,1,1,1,1,1,1,1,1,1,1,1,1,1,
1,1,1,1,1,1,1,1,1,1,1,1,1,1,1,1,1,1,1,1,1,1,1,1,1,1,1,1,1,1,1,1,1,1,1,1,
1,1,1,1,1,1,1,1,1,1,1,1,1,1,1,1,1,1,1,1,1,1,1,1,1,1,1,1,1,1,1,1,1,1,1,1,
1,1,1,1,1,1,1,1,1,1,1,1,1,1,1,1,1,1,1,1,1,1,1,1,1,1,1,1,1,1,1,1,1,1,1,1,
1,1,1,1,1,1,1,1,1,1,1,1,1,1,1,1,1,1,1,1,1,1,1,1,1,1,1,1,1,1,1,1,1,1,1,1,
1,1,1,1,1,1,1,1,1,1,1,1,1,1,1,1,1,1,1,1,1,1,1,1,1,1,1,1,1,1,1,1,1,1,1,1,
1,1,1,1,1,1,1,1,1,1,1,1,1,1,1,1,1,1,1,1,1,1,1,1,1,1,1,1,1,1,1,1,1,1,1,1,
1,1,1,1,1,1,1,1,1,1,1,1,1,1,1,1,1,1,1,1,1,1,1,1,1,1,1,1,1,1,1,1,1,1,1,1,
1,1,1,1,1,1,1,1,1,1,1,1,1,1,1,1,1,1,1,1,1,1,1,1,1,1,1,1,1,1,1,1,1,1,1,1,
1,1,1,1,1,1,1,1,1,1,1,1,1,1,1,1,1,1,1,1,1,1,1,1,1,1,1,1,1,1,1,1,1,1,1,1,
1,1,1,1,1,1,1,1,1,1,1,1,1,1,1,1,1,1,1,1,1,1,1,1,1,1,1,1,1,1,1,1,1,1,1,1,
1,1,1,1,4),(2,2),(0.,0.869746702321014,1.7394931589914,2.60923976624962,
3.47983908319159,4.35043840179749,5.22018503077054,6.08993165951504,6.95967828799171,
7.82942491616733,8.69917154401062,9.56891817149224,10.4395174886835,11.3101168056706,
12.179863432132,13.049610058144,13.9193566836854,14.7891033087372,15.6588499332817,
16.5285965573034,17.3991958717975,18.2697951860185,18.7046684974166,19.1395418086746,
19.5744151197912,20.0092884307654,20.4441617415962,20.8790350522825,21.7487816732187,
22.1836549834672,22.6185282935685,23.0534016035221,23.4882749133276,23.9231482229848,
24.3588742245859,24.794600226187,25.2294735355468,26.0992201538203,26.5340934627341,
26.9689667714994,27.4038400801166,27.838713388586,28.2735866969081,28.7084600050832,
29.143333313112,29.5782066209952,30.0130799287334,30.4479532363275,30.8828265437783,
31.3185525442794,31.7542785447804,32.1891518519474,32.6240251589741,33.0588984658616,
33.4937717726112,33.928645079224,34.3635183857014,34.7983916920448,35.2332649982556,
35.6681383043353,36.1030116102854,36.5378849161076,36.9727582218035,37.4076315273749,
37.8425048328235,38.2782308323341,38.7139568318446,39.1488301370532,39.5837034421446,
40.0185767471208,40.4534500519838,40.8883233567357,41.3231966613787,41.7580699659148,
42.1929432703463,42.6278165746754,43.0626898789044,43.4975631830356,43.9324364870714,
44.3673097910142,44.8021830948664,45.2379090935952,45.673635092324,46.1085083960024,
46.5433816995978,46.9782550031127,47.4131283065497,47.8480016099115,48.2828749132006,
48.7177482164198,49.1526215195718,49.5874948226593,50.0223681256851,50.457241428652,
50.8921147315628,51.3269880344203,51.7618613372274,52.197587335454,52.6333133336805,
53.0681866363954,53.5030599390685,53.9379332417027,54.3728065443011,54.8076798468664,
55.2425531494018,55.6774264519101,56.1122997543943,56.5471730568575,56.9820463593026,
57.4169196617326,57.8517929641506,58.2866662665595,58.7215395689624,59.157265567009,
59.5929915650557,60.0278648674556,60.4627381698584,60.8976114722673,61.3324847746853,
61.7673580771153,62.2022313795604,62.6371046820236,63.0719779845079,63.5068512870162,
63.9417245895516,64.376597892117,64.8114711947155,65.2463444973499,65.6812178000231,
66.1169437982275,66.5526697964318,66.9875430991915,67.4224164019987,67.8572897048563,
68.2921630077673,68.7270363107343,69.1619096137603,69.5967829168479,70.0316562200001,
70.4665295232194,70.9014028265087,71.3362761298705,71.7711494333077,72.2060227368227,
72.6408960404182,73.0766220391044,73.5123480377905,73.9472213415547,74.382094645407,
74.8169679493499,75.2518412533859,75.6867145575172,76.1215878617464,76.5564611660756,
76.9913344705072,77.4262077750435,77.8610810796866,78.2959543844386,78.7308276893018,
79.1657009942781,79.6005742993696,80.0363002988208,80.4720262982719,80.9068996035997,
81.3417729090484,81.7766462146199,82.211519520316,82.6463928261383,83.0812661320886,
83.5161394381684,83.9510127443794,84.3858860507229,84.8207593572004,85.2556326638134,
85.6905059705631,86.1253792774507,86.5602525844776,86.995978584908,87.4317045853384,
87.8665778926469,88.3014512000977,88.7363245076919,89.1711978154302,89.6060711233134,
90.0409444313423,90.4758177395175,90.9106910478396,91.345564356309,91.7804376649263,
92.2153109736917,92.6501842826055,93.085057591668,93.5199309008791,93.9556569024059,
94.3913829039327,94.8262562134414,95.2611295230986,95.6960028329042,96.1308761428578,
96.5657494529591,97.0006227632077,97.4354960736028,97.870369384144,98.3052426948304,
98.7401160056612,99.1749893166354,99.6098626277522,100.04473593901,100.915335253024,
101.351061255639,101.785934567313,102.220807879124,102.655681191068,103.090554503145,
103.525427815353,104.395174440154,105.264921065453,105.699794378283,106.134667691232,
106.569541004295,107.004414317471,107.8750136343,108.745612951339,109.615359578629,
110.485106206296,111.354852834309,112.224599462639,113.094346091254,113.964092720119,
114.834692038763,115.705291357499,116.575037986826,117.444784616267,118.314531245777,
119.184277875311,120.054024504821,120.923771134261,121.794370453112,122.66496977189,
123.534716400968,124.404463029834,125.274209658448,126.143956286779,127.013702914792,
127.883449542458,128.754048859798,129.624648176939,130.494394803617,131.364141429857,
132.233888055637,133.103634680937,133.973381305737,134.843127930023,135.71372724472,
136.584326559147,137.019199870684,137.454073182083,137.888946493341,138.323819804458,
139.193566426263,140.063313047491,140.498186357887,140.933059668136,141.367932978237,
141.802806288191,142.237679597997,142.673405599673,143.109131601348,143.544004910857,
143.978878220217,144.413751529429,144.848624838491,145.283498147405,145.718371456171,
146.153244764789,146.588118073258,147.022991381581,147.457864689756,147.892737997785,
148.327611305669,148.762484613407,149.197357921002,149.633083921574,150.068809922147,
150.503683229455,150.938556536623,151.37342984365,151.808303150538,152.243176457288,
152.678049763901,153.112923070379,153.547796376722,153.982669682934,154.417542989014,
154.852416294964,155.287289600787,155.722162906483,156.157036212055,156.592762211626,
157.028488211198,157.463361516526,157.898234821735,158.333108126826,158.767981431803,
159.202854736666,159.637728041419,160.072601346062,160.507474650599,160.94234795503,
161.37722125936,161.812094563589,162.246967867721,162.681841171757,163.1167144757,
163.552440474473,163.988166473247,164.423039777011,164.85791308069,165.292786384286,
165.727659687801,166.162532991238,166.597406294601,167.03227959789,167.46715290111,
167.902026204262,168.33689950735,168.771772810376,169.206646113343,169.641519416254,
170.076392719112,170.512118717363,170.947844715614,171.382718018374,171.817591321089,
172.252464623762,172.687337926397,173.122211228996,173.557084531561,173.991957834097,
174.426831136606,174.86170443909,175.296577741554,175.731451044,176.16632434643,
176.601197648848,177.036070951258,177.471796949306,177.907522947355,178.342396249755,
178.777269552155,179.212142854558,179.647016156968,180.081889459386,180.516762761816,
180.951636064262,181.386509366726,181.82138266921,182.256255971719,182.691129274255,
183.12600257682,183.560875879419,183.995749182054,184.431475180237,184.867201178421,
185.302074481136,185.736947783896,186.171821086704,186.606694389561,187.041567692473,
187.47644099544,187.911314298466,188.346187601554,188.781060904706,189.215934207926,
189.650807511215,190.085680814577,190.520554118015,190.95542742153,191.391153420175,
191.82687941882,192.261752722499,192.696626026263,193.131499330116,193.566372634059,
194.001245938095,194.436119242227,194.870992546456,195.305865850785,195.740739155217,
196.175612459754,196.610485764397,197.045359069149,197.480232374013,197.915105678989,
198.350831678382,198.786557677775,199.221430982984,199.656304288312,200.091177593761,
200.526050899333,200.960924205029,201.395797510852,201.830670816802,202.265544122882,
202.700417429093,203.135290735437,203.570164041915,204.005037348528,204.439910655278,
204.874783962166,205.310509962526,205.746235962887,206.181109270054,206.615982577363,
207.050855884814,207.485729192409,207.920602500147,208.355475808031,208.79034911606,
209.225222424235,209.660095732558,210.094969041027,210.529842349645,210.96471565841,
211.399588967324,211.834462276387,212.27018827784,212.705914279292,213.140787588653,
213.575660898161,214.010534207819,214.880280827579,215.31515413768,215.750027447929,
216.184900758324,216.619774068866,217.054647379553,217.489520690384,218.359267312475,
219.22986662628,219.665592628826,220.100465940363,220.535339252038,220.970212563848,
221.83995918787,222.709705812416,223.579452437468,224.014325750179,224.44919906301,
225.318945689022,226.189545005688,227.060144322571,227.929890949664,228.799637577146,
229.66938420499,230.539130833166,231.408877461643,232.278624090388,233.149223408954,
234.019822727623,234.889569356878,235.759315986267,236.629062615749,237.498809245277,
238.368555874806,239.238302504287,240.108901823183,240.979501142017,241.849247771189,
242.718994400167,243.588741028911,244.458487657389,245.328234285565,246.197980913409,
247.068580230891,247.939179548182,248.80892617507,249.678672801532,250.548419427545,
251.418166053087,252.287912678139,253.157659302684,254.028258617581,254.898857932211,
255.333731243885,255.768604555423,256.203477866821,256.63835117808,257.508097800171,
258.377844421689,258.812717732231,259.247591042627,259.682464352876,260.117337662977,
260.552210972931,260.987936974682,261.858536286089,262.293409595598,262.728282904958,
263.16315621417,263.598029523233,264.032902832147,264.467776140913,264.902649449531,
265.337522758001,265.772396066323,266.207269374499,266.642142682528,267.077015990412,
267.511889298151,267.947615298795,268.383341299439,268.81821460689,269.2530879142,
269.687961221367,270.122834528394,270.557707835282,270.992581142032,271.427454448646,
271.862327755124,272.297201061468,272.732074367679,273.166947673759,273.60182097971,
274.036694285533,274.471567591229,274.907293590862,275.343019590495,275.777892895944,
276.212766201272,276.647639506481,277.082512811573,277.51738611655,277.952259421414,
278.387132726166,278.82200603081,279.256879335346,279.691752639779,280.126625944108,
280.561499248338,280.996372552469,281.431245856506,281.866971855324,282.302697854143,
282.737571157996,283.172444461761,283.60731776544,284.042191069036,284.477064372551,
284.911937675989,285.346810979351,285.781684282641,286.216557585861,286.651430889013,
287.086304192101,287.521177495128,287.956050798095,288.390924101007,288.826650099283,
289.262376097559,289.697249400366,290.132122703127,290.566996005842,291.001869308516,
291.43674261115,291.871615913749,292.306489216315,292.741362518851,293.17623582136,
293.611109123845,294.045982426308,294.480855728754,294.915729031185,295.350602333603,
295.786328331655,296.222054329707,296.65692763211,297.091800934511,297.526674236911,
297.961547539314,298.396420841724,298.831294144142,299.266167446573,299.701040749018,
300.135914051482,300.570787353967,301.005660656476,301.440533959012,301.875407261578,
302.310280564177,302.746006562341,303.181732560506,303.616605863179,304.051479165895,
304.486352468655,304.921225771462,305.35609907432,305.790972377232,306.225845680199,
306.660718983226,307.095592286314,307.530465589466,307.965338892686,308.400212195976,
308.835085499338,309.269958802776,309.705684801381,310.141410799985,310.576284103581,
311.01115740726,311.446030711025,311.880904014878,312.315777318821,312.750650622858,
313.185523926989,313.620397231219,314.055270535549,314.490143839981,314.925017144517,
315.359890449161,315.794763753913,316.229637058777,316.665363058112,317.101089057448,
317.53596236254,317.970835667749,318.405708973077,318.840582278526,319.275455584098,
319.710328889795,320.145202195618,320.580075501568,321.014948807648,321.44982211386,
321.884695420204,322.319568726682,322.754442033295,323.189315340045,323.625041340336,
324.060767340628,324.495640647655,324.930513954822,325.365387262131,325.800260569583,
326.235133877177,326.670007184916,327.1048804928,327.539753800829,327.974627109005,
328.409500417327,328.844373725797,329.279247034415,329.714120343181,330.148993652095,
330.584719653474,331.020445654852,331.455318964064,331.890192273424,332.325065582933,
332.759938892591,333.194812202397,333.629685512351,334.064558822453,334.499432132702,
334.934305443098,335.369178753639,335.804052064326,336.673798686132,337.108671997249,
337.544397999725,337.980124002201,338.4149973136,338.849870625137,339.284743936812,
340.154490560568,341.024237184854,341.459110497191,341.893983809655,342.328857122244,
342.763730434955,343.633477060735,344.504076377234,345.374675693955,346.244422320844,
347.114168948136,347.983915575803,348.853662203817,349.723408832148,350.593155460764,
351.463754779246,352.334354097839,353.204100727012,354.07384735634,354.943593985781,
355.813340615292,356.683087244827,357.552833874338,358.423433193272,359.294032512154,
360.163779141409,361.033525770489,361.903272399355,362.77301902797,363.642765656301,
364.512512284316,365.383111601936,366.253710919371,367.123457546465,367.993204173143,
368.862950799383,369.732697425164,370.602444050463,371.472190675265,372.342789990359,
373.21338930519,373.648262617,374.083135928675,374.952882551611,375.822629173987,
376.257502484962,376.692375795793,377.12724910648,377.562122417021,377.996995727417,
378.431869037666,378.866742347767,379.302468349591,379.738194351416,380.173067661222,
380.607940970879,381.042814280388,381.477687589749,381.91256089896,382.347434208023,
382.782307516937,383.217180825703,383.652054134321,384.086927442791,384.521800751113,
384.956674059289,385.391547367318,385.826420675202,386.262146675918,386.697872676635,
387.13274598423,387.567619291681,388.00249259899,388.437365906157,388.872239213185,
389.307112520073,389.741985826823,390.176859133436,390.611732439914,391.046605746258,
391.48147905247,391.91635235855,392.351225664501,392.786098970323,393.221824970019,
393.657550969714,394.092424275286,394.527297580735,394.962170886063,395.397044191272,
395.831917496364,396.266790801341,396.701664106204,397.136537410957,397.5714107156,
398.006284020137,398.441157324569,398.876030628899,399.310903933128,399.74577723726,
400.181503236126,400.617229234991,401.052102538934,401.486975842787,401.921849146551,
402.356722450231,402.791595753827,403.226469057342,403.66134236078,404.096215664142,
404.531088967432,404.965962270651,405.400835573804,405.835708876892,406.270582179918,
406.705455482886,407.141181481189,407.576907479491,408.01178078235,408.446654085157,
408.881527387917,409.316400690633,409.751273993306,410.186147295941,410.62102059854,
411.055893901106,411.490767203642,411.925640506151,412.360513808636,412.795387111099,
413.230260413545,413.665133715976,414.100859714032,414.536585712088,414.971459014498,
415.406332316901,415.841205619301,416.276078921702,416.710952224105,417.145825526515,
417.580698828933,418.015572131364,418.45044543381,418.885318736273,419.320192038758,
419.755065341267,420.189938643803,420.624811946369,421.060537944515,421.496263942662,
421.931137245297,422.36601054797,422.800883850686,423.235757153446,423.670630456253,
424.105503759112,424.540377062023,424.975250364991,425.410123668017,425.844996971105,
426.279870274258,426.714743577477,427.149616880767,427.584490184129,428.020216182695,
428.455942181261,428.890815484776,429.325688788373,429.760562092052,430.195435395816,
430.630308699669,431.065182003612,431.500055307649,431.93492861178,432.36980191601,
432.80467522034,433.239548524772,433.674421829309,434.109295133952,434.544168438705,
434.979894437984,435.415620437262,435.850493742239,436.285367047331,436.72024035254,
437.155113657869,437.589986963318,438.024860268889,438.459733574586,438.894606880409,
439.32948018636,439.76435349244,440.199226798651,440.634100104995,441.068973411473,
441.503846718087,441.939572718309,442.375298718531,442.810172025419,443.245045332447,
443.679918639614,444.114791946923,444.549665254374,444.984538561969,445.419411869708,
445.854285177591,446.289158485621,446.724031793796,447.158905102119,447.593778410589,
448.028651719207,448.463525027973,448.899251029277,449.334977030581,449.769850339644,
450.639596958216,451.074470267725,451.509343577383,451.944216887189,452.379090197143,
452.813963507244,453.248836817493,453.683710127889,454.118583438431,454.553456749117,
454.988330059949,455.423203370923,455.858929373329,456.294655375734,456.729528686993,
457.164401998391,457.599275309929,458.469021933414,458.90389524536,459.338768557437,
459.773641869646,460.208515181983,460.643388494447,461.078261807036,461.948008432578,
462.818607748906,463.689207065461,464.55895369214,465.428700319234,466.298446946716,
467.16819357456,468.037940202737,468.907686831215,469.778286149605,470.648885468116,
471.518632097196,472.388378726451,473.258125355841,474.127871985322,474.997618614851,
475.86736524438,476.737964563343,477.608563882265,478.478310511593,479.348057140765,
480.217803769743,481.087550398488,481.957297026966,482.827043655142,483.697642972895,
484.568242290469,485.43798891776,486.307735544649,487.177482171112,488.047228797125,
488.916975422667,489.78672204772,490.657321363009,491.09304736596,491.527920678038,
492.397667301793,493.267413925005,494.137160547663,494.57203385878,495.006907169755,
495.441780480586,495.876653791273,496.311527101814,496.74640041221,497.616999724357,
498.052725726255,498.487599036209,498.922472346015,499.357345655673,499.792218965182,
500.227092274542,500.661965583754,501.096838892816,501.531712201731,501.966585510497,
502.401458819114,502.836332127584,503.271205435907,503.706078744082,504.140952052112,
504.576678052901,505.01240405369,505.447277361429,505.882150669023,506.317023976474,
506.751897283783,507.186770590951,507.621643897978,508.056517204866,508.491390511616,
508.92626381823,509.361137124708,509.796010431052,510.230883737263,510.665757043344,
511.100630349294,511.536356349053,511.972082348811,512.406955654506,512.841828960076,
513.276702265523,513.711575570849,514.146448876056,514.581322181146,515.016195486121,
515.451068790983,515.885942095733,516.320815400375,516.75568870491,517.19056200934,
517.625435313668,518.060308617896,518.496034616807,518.931760615718,519.366633919752,
519.801507223694,520.236380527545,520.671253831307,521.106127134985,521.541000438579,
521.975873742092,522.410747045528,522.845620348888,523.280493652176,523.715366955394,
524.150240258545,524.585113561631,525.019986864656,525.455712862985,525.891438861313,
526.326312164223,526.761185467079,527.196058769885,527.630932072643,528.065805375356,
528.500678678029,528.935551980661,529.370425283258,529.805298585822,530.240171888356,
530.675045190863,531.109918493346,531.544791795808,531.979665098252,532.415391096312,
532.851117094373,533.285990396789,533.720863699197,534.155737001598,534.590610303997,
535.025483606395,535.460356908796,535.895230211204,536.330103513621,536.764976816049,
537.199850118493,537.634723420955,538.069596723438,538.504470025945,538.93934332848,
539.375069326608,539.810795324736,540.245668627333,540.680541929966,541.115415232637,
541.550288535351,541.985161838109,542.420035140915,542.854908443771,543.28978174668,
543.724655049646,544.15952835267,544.594401655757,545.029274958907,545.464148262125,
545.899021565413,546.334747563939,546.770473562465,547.205346865901,547.640220169415,
548.075093473009,548.509966776686,548.944840080449,549.3797133843,549.814586688241,
550.249459992276,550.684333296405,551.119206600633,551.554079904961,551.988953209391,
552.423826513926,552.858699818567,553.294425817789,553.73015181701,554.165025121872,
554.599898426846,555.034771731937,555.469645037144,555.90451834247,556.339391647917,
556.774264953487,557.209138259182,557.644011565003,558.078884870951,558.51375817703,
558.948631483239,559.383504789581,559.818378096058,560.254104096209,560.689830096361,
561.12470340311,561.559576709996,561.994450017021,562.429323324187,562.864196631494,
563.299069938943,563.733943246536,564.168816554273,564.603689862154,565.038563170182,
565.473436478355,565.908309786676,566.343183095144,566.77805640376,567.213782404988,
567.649508406216,568.084381715128,568.519255024189,568.954128333399,569.389001642757,
569.823874952264,570.258748261921,570.693621571725,571.128494881677,571.563368191777,
572.433114812417,572.867988122957,573.302861433642,573.737734744471,574.173460746804,
574.609186749136,575.044060060251,575.913806682904,576.783553306113,577.218426617922,
577.653299929865,578.08817324194,578.523046554147,579.392793178944,580.26253980424,
581.13313912039,581.568865123709,582.003738436771,582.87348506323,583.743231690115,
584.612978317402,585.482724945065,586.352471573076,587.222218201403,588.092817519691,
588.963416838109,589.833163467083,590.702910096251,591.572656725575,592.442403355013,
593.31214998452,594.181896614051,595.05249593303,595.92309525198,596.792841881366,
597.662588510618,598.532335139693,599.402081768556,600.271828397167,601.141575025495,
602.012174343369,602.882773661074,603.752520288553,604.622266915642,605.492013542317,
606.361760168553,607.23150679433,608.101253419626,608.971852735101,609.842452050322,
610.71219867434,611.581945297822,612.451691920754,612.886565232011,613.321438543126,
613.756311854099,614.191185164928,615.060931786153,615.931531098516,616.367257100486,
616.802130410586,617.237003720538,617.671877030342,618.106750339998,618.541623649505,
618.976496958863,619.411370268073,619.846243577134,620.281116886046,620.71599019481,
621.150863503426,621.585736811894,622.020610120214,622.455483428388,622.891209429248,
623.326935430108,623.761808737989,624.196682045726,624.631555353319,625.066428660769,
625.501301968075,625.936175275241,626.371048582266,626.805921889153,627.240795195901,
627.675668502512,628.110541808988,628.54541511533,628.98028842154,629.415161727618,
629.850887727438,630.286613727259,630.72148703308,631.156360338774,631.591233644344,
632.026106949791,632.460980255118,632.895853560325,633.330726865415,633.76560017039,
634.200473475251,634.635346780002,635.070220084644,635.505093389179,635.939966693609,
636.374839997937,636.810565996897,637.246291995857,637.681165299986,638.116038604021,
638.550911907962,638.985785211813,639.420658515576,639.855531819253,640.290405122847,
640.725278426361,641.160151729796,641.595025033157,642.029898336444,642.464771639662,
642.899644942813,643.334518245899,643.770244244257,644.205970242616,644.640843545581,
645.075716848491,645.510590151347,645.945463454153,646.380336756911,646.815210059625,
647.250083362296,647.684956664929,648.119829967526,648.55470327009,648.989576572624,
649.424449875131,649.859323177614,650.294196480076,650.729922478144,651.165648476212,
651.600521778641,652.035395081057,652.470268383465,652.905141685866,653.340014988265,
653.774888290663,654.209761593065,654.644634895472,655.079508197889,655.514381500318,
655.949254802762,656.384128105224,656.819001407706,657.253874710213,657.689600708326,
658.12532670644,658.560200009004,658.995073311601,659.429946614234,659.864819916905,
660.299693219619,660.734566522377,661.169439825183,661.604313128039,662.039186430948,
662.474059733914,662.908933036938,663.343806340025,663.778679643175,664.213552946393,
664.649278944883,665.085004943373,665.519878246733,665.954751550169,666.389624853683,
666.824498157277,667.259371460954,667.694244764717,668.129118068568,668.563991372509,
668.998864676544,669.433737980674,669.868611284901,670.303484589229,670.738357893659,
671.173231198194,671.608957197361,672.044683196528,672.479556501278,672.91442980614,
673.349303111115,673.784176416205,674.219049721412,674.653923026738,675.088796332185,
675.523669637755,675.95854294345,676.393416249271,676.82828955522,677.263162861298,
677.698036167508,678.13290947385,678.568635473934,679.004361474018,679.439234780629,
679.874108087377,680.308981394264,680.743854701289,681.178728008455,681.613601315762,
682.048474623211,682.483347930804,682.91822123854,683.353094546422,683.78796785445,
684.222841162623,684.657714470944,685.092587779412,685.528313780566,685.96403978172,
686.398913090483,686.833786399396,687.268659708457,687.703533017666,688.138406327025,
688.573279636532,689.008152946187,689.443026255992,689.877899565944,690.312772876043,
690.74764618629,691.182519496684,691.617392807224,692.052266117909,692.487992120169,
692.92371812243,693.358591433403,694.228338055774,694.663211367171,695.098084678707,
695.532957990379,695.967831302188,696.402704614131,696.837577926207,697.707324550749,
698.577071175797,699.011944488507,699.447670491767,699.883396495028,700.318269807975,
701.188016434211,702.057763060886,702.927509687976,703.797256315454,704.667002943295,
705.536749571467,706.407348889651,707.277948207973,708.147694836835,709.017441465911,
709.887188095163,710.756934724548,711.626681354026,712.496427983551,713.367027302543,
714.237626621516,715.107373250954,715.977119880277,716.846866509446,717.716613138419,
718.586359767161,719.456106395635,720.32670571363,721.197305031464,722.067051659126,
722.936798286414,723.806544913299,724.676291539758,725.546038165767,726.415784791305,
727.286384106969,728.156983422381,729.026730046663,729.896476670415,730.331349982088,
730.766223293624,731.201096605021,731.635969916278,732.505716538366,733.37546315988,
733.81033647042,734.246062472462,734.681788474505,735.116661784752,735.551535094852,
735.986408404804,736.421281714608,736.856155024264,737.291028333771,737.72590164313,
738.160774952339,738.5956482614,739.030521570312,739.465394879076,739.900268187692,
740.33514149616,740.77001480448,741.205740805414,741.641466806347,742.076340114374,
742.511213422256,742.946086729993,743.380960037585,743.815833345035,744.250706652341,
744.685579959507,745.120453266533,745.555326573419,745.990199880167,746.425073186778,
746.859946493254,747.294819799596,747.729693105806,748.165419105691,748.601145105576,
749.036018411525,749.470891717346,749.90576502304,750.34063832861,750.775511634057,
751.210384939384,751.645258244591,752.080131549682,752.515004854656,752.949878159518,
753.384751464269,753.81962476891,754.254498073445,754.689371377875,755.125097376885,
755.560823375895,755.995696680123,756.430569984253,756.865443288287,757.300316592228,
757.735189896079,758.170063199842,758.604936503519,759.039809807113,759.474683110627,
759.909556414062,760.344429717423,760.779303020711,761.214176323929,761.649049627079,
762.084775625469,762.520501623858,762.955374926883,763.390248229848,763.825121532758,
764.259994835614,764.694868138419,765.129741441178,765.564614743891,765.999488046563,
766.434361349196,766.869234651793,767.304107954357,767.738981256891,768.173854559398,
768.608727861881,769.044453859958,769.480179858035,769.915053160479,770.349926462907,
770.784799765324,771.219673067731,771.654546370133,772.089419672531,772.52429297493,
772.959166277331,773.394039579739,773.828912882155,774.263786184584,774.698659487028,
775.13353278949,775.568406091973,776.004132090072,776.439858088172,776.874731390706,
777.30960469327,777.744477995867,778.1793512985,778.614224601171,779.049097903885,
779.483971206643,779.918844509449,780.353717812305,780.788591115215,781.22346441818,
781.658337721205,782.093211024291,782.528084327442,782.963810325897,783.399536324352,
783.834409627639,784.269282931,784.704156234435,785.139029537949,785.573902841543,
786.00877614522,786.443649448983,786.878522752834,787.313396056775,787.74826936081,
788.183142664939,788.618015969167,789.052889273495,789.487762577925,789.923488577038,
790.359214576152,790.794087880793,791.228961185544,791.663834490406,792.098707795381,
792.533581100471,792.968454405678,793.403327711004,793.838201016451,794.273074322021,
794.707947627716,795.142820933537,795.577694239486,796.012567545564,796.447440851774,
796.883166851791,797.318892851808,797.753766158284,798.188639464895,798.623512771643,
799.058386078529,799.493259385555,799.92813269272,800.363006000027,800.797879307477,
801.232752615069,801.667625922806,802.102499230688,802.537372538715,802.972245846889,
803.40711915521,803.84284515629,804.27857115737,804.713444465985,805.148317774749,
805.583191083662,806.018064392723,806.452937701933,806.887811011291,807.322684320798,
808.192430940258,808.62730425021,809.06217756031,809.497050870557,809.931924180951,
810.36679749149,810.802523493679,811.238249495867,811.673122806697,812.542869428785,
812.977742740041,813.412616051438,813.847489362974,814.282362674646,814.717235986455,
815.152109298398,816.021855922681,816.891602547478,817.326475860065,817.762201863265,
818.197927866466,818.632801179295,819.502547805304,820.372294431763,821.242041058648,
822.111787685935,822.981534313598,823.851280941609,824.721880259681,825.5924795779,
826.462226206642,827.331972835616,828.201719464785,829.071466094109,829.941212723546,
830.810959353053,831.681558672047,832.552157991036,833.421904620514,834.2916512499,
835.161397879151,836.031144508226,836.900891137089,837.770637765701,838.641237083811,
839.511836401767,840.381583029608,841.251329657086,842.121076284176,842.990822910851,
843.860569537087,844.730316162863,845.600915478712,846.471514794314,847.341261418855,
848.211008042874,848.645881354683,849.080754666356,849.515627977891,849.950501289288,
850.82024791166,851.689994533462,852.124867844147,852.560593846263,852.996319848379,
853.431193158772,853.866066469019,854.300939779119,855.170686398875,855.605559708531,
856.040433018038,856.475306327397,856.910179636606,857.345052945667,857.77992625458,
858.214799563344,858.64967287196,859.084546180427,859.520272181434,859.95599818244,
860.390871490614,860.825744798641,861.260618106523,861.69549141426,862.130364721852,
862.565238029302,863.000111336609,863.434984643774,863.8698579508,864.304731257686,
864.739604564434,865.174477871045,865.609351177521,866.044224483863,866.479950483814,
866.915676483765,867.350549789843,867.785423095792,868.220296401613,868.655169707307,
869.090043012877,869.524916318325,869.959789623651,870.394662928858,870.829536233948,
871.264409538923,871.699282843785,872.134156148535,872.569029453177,873.003902757712,
873.439628756773,873.875354755834,874.310228060162,874.745101364389,875.179974668519,
875.614847972553,876.049721276495,876.484594580346,876.919467884108,877.354341187786,
877.78921449138,878.224087794893,878.658961098329,879.093834401689,879.528707704977,
879.963581008195,880.399307006616,880.835033005038,881.269906308124,881.704779611148,
882.139652914114,882.574526217024,883.00939951988,883.444272822685,883.879146125444,
884.314019428157,884.748892730829,885.183766033462,885.618639336059,886.053512638623,
886.488385941157,886.923259243664,887.358985241751,887.794711239839,888.2295845423,
888.664457844744,889.099331147173,889.534204449589,889.969077751997,890.403951054398,
890.838824356797,891.273697659195,891.708570961597,892.143444264004,892.578317566421,
893.01319086885,893.448064171293,893.882937473755,894.318663471843,894.75438946993,
895.189262772437,895.624136074971,896.059009377535,896.493882680132,896.928755982765,
897.363629285437,897.798502588151,898.233375890909,898.668249193715,899.103122496571,
899.53799579948,899.972869102446,900.40774240547,900.842615708556,901.278341706978,
901.714067705399,902.148941008617,902.583814311905,903.018687615265,903.453560918701,
903.888434222214,904.323307525808,904.758180829485,905.193054133248,905.627927437099,
906.06280074104,906.497674045075,906.932547349205,907.367420653433,907.80229395776,
908.238019956821,908.673745955883,909.108619260417,909.543492565059,909.978365869809,
910.413239174671,910.848112479646,911.282985784736,911.717859089943,912.152732395269,
912.587605700716,913.022479006287,913.457352311981,913.892225617802,914.327098923751,
914.761972229829,915.19769822978,915.633424229731,916.068297536072,916.503170842548,
916.93804414916,917.372917455908,917.807790762794,918.24266406982,918.677537376985,
919.112410684292,919.547283991742,919.982157299334,920.417030607071,920.851903914953,
921.28677722298,921.721650531154,922.15737653216,922.593102533167,923.027975841635,
923.46284915025,923.897722459014,924.332595767926,924.767469076987,925.202342386197,
925.637215695556,926.072089005063,926.506962314719,926.941835624523,927.376708934475,
927.811582244575,928.246455554822,928.681328865215,929.117054867331,929.987654180132,
930.422527490961,930.857400801934,931.292274113049,931.727147424306,932.162020735703,
932.596894047238,933.46664067072,934.336387294739,934.771260606945,935.20613391928,
935.641007231742,936.076733234882,936.94733255073,937.817079176507,938.686825802743,
939.556572429418,940.426319056508,941.296065683986,942.165812311827,943.036411629783,
943.907010947893,944.776757576505,945.646504205367,946.516250834443,947.385997463694,
948.25574409308,949.125490722558,949.996090041546,950.86668936054,951.736435990048,
952.606182619485,953.475929248809,954.345675877978,955.215422506951,956.085169135693,
956.955768453912,957.826367771985,958.696114399995,959.565861027658,960.435607654946,
961.305354281831,962.175100908289,963.044847534298,963.915446850328,964.786046166116,
965.655792790913,966.525539415195,966.960412727138,967.395286038947,968.265032662155,
969.134779284809,969.569652595924,970.004525906897,970.439399217726,970.875125219914,
971.310851222103,971.745724532643,972.615471153283,973.485217773335,973.920091083139,
974.354964392795,974.789837702302,975.22471101166,975.65958432087,976.094457629931,
976.529330938844,976.964204247608,977.399077556223,977.834803557303,978.270529558383,
978.705402866704,979.140276174877,979.575149482905,980.010022790786,980.444896098523,
980.879769406116,981.314642713565,981.749516020872,982.184389328038,982.619262635063,
983.05413594195,983.489009248698,983.923882555309,984.358755861785,984.794481861802,
985.230207861819,985.665081168029,986.099954474107,986.534827780056,986.969701085877,
987.404574391571,987.839447697141,988.274321002589,988.709194307915,989.144067613122,
989.578940918212,990.013814223187,990.448687528048,990.883560832799,991.31843413744,
991.754160136554,992.189886135667,992.624759440097,993.059632744425,993.494506048653,
993.929379352783,994.364252656817,994.799125960758,995.233999264609,995.668872568372,
996.103745872049,996.538619175643,996.973492479157,997.408365782593,997.843239085953,
998.278112389241,998.713838387696,999.149564386151,999.584437689301,1000.01931099239,
1000.45418429541,1000.88905759838,1001.32393090129,1001.75880420414,1002.19367750695,
1002.62855080971,1003.06342411242,1003.49829741509,1003.93317071773,1004.36804402032,
1004.80291732289,1005.23779062542,1005.67351662352,1006.10924262162,1006.5441159241,
1006.97898922656,1007.41386252901,1007.84873583144,1008.28360913385,1008.71848243626,
1009.15335573866,1009.58822904106,1010.02310234346,1010.45797564586,1010.89284894827,
1011.32772225069,1011.76259555311,1012.19746885556,1012.63319485364,1013.06892085171,
1013.5037941542,1013.9386674567,1014.37354075924,1014.8084140618,1015.2432873644,
1015.67816066703,1016.1130339697,1016.54790727242,1016.98278057517,1017.41765387798,
1017.85252718084,1018.28740048375,1018.72227378671,1019.15714708974,1019.59287308813,
1020.02859908651,1020.46347238967,1020.89834569288,1021.33321899617,1021.76809229953,
1022.20296560297,1022.63783890648,1023.07271221007,1023.50758551375,1023.94245881752,
1024.37733212137,1024.81220542531,1025.24707872935,1025.68195203348,1026.11682533771,
1026.55255133672,1026.98827733573,1027.42315064016,1027.8580239447,1028.29289724934,
1028.72777055409,1029.16264385896,1029.59751716393,1030.03239046902,1030.46726377423,
1030.90213707956,1031.33701038501,1031.77188369058,1032.20675699628,1032.6416303021,
1033.07650360805,1033.51222960793,1033.94795560782,1034.38282891403,1034.81770222038,
1035.25257552685,1035.68744883347,1036.12232214022,1036.5571954471,1036.99206875413,
1037.4269420613,1037.86181536861,1038.29668867606,1038.73156198365,1039.16643529139,
1039.60130859927,1040.0361819073,1040.47190790824,1040.90763390917,1041.34250721749,
1041.77738052596,1042.21225383458,1042.64712714334,1043.08200045226,1043.95174707053,
1044.38662037989,1044.8214936894,1045.25636699906,1045.69124030886,1046.12611361882,
1046.56098692892,1046.99586023917,1047.43158624121,1047.86731224325,1048.3021855538,
1048.73705886448,1049.17193217531,1049.60680548629,1050.0416787974,1050.47655210866,
1050.91142542006,1051.78117204327,1052.21604535508,1052.65091866703,1053.0857919791,
1053.52066529131,1053.95553860365,1054.39126460673,1055.26186392239,1056.13161054793,
1057.00135717395,1057.43623048712,1057.87110380041,1058.7408504273,1059.61059705459,
1060.48034368225,1061.35094300009,1062.22154231809,1063.09128894656,1063.96103557531,
1064.83078220429,1065.70052883346,1066.57027546278,1067.44002209222,1068.3106214112,
1069.18122073019,1070.05096735972,1070.9207139892,1071.79046061859,1072.66020724785,
1073.52995387693,1074.39970050579,1075.27029982411,1076.1408991423,1077.01064577048,
1077.88039239832,1078.7501390258,1079.61988565289,1080.48963227957,1081.35937890581,
1082.22997822202,1083.100577538,1083.97032416305,1084.84007078759,1085.70981741161,
1086.5795640351,1087.44931065803,1087.88418396929,1088.31905728041,1088.75393059138,
1089.18965659365,1089.62538259591,1090.06025590659,1090.93000252753,1091.36487583778,
1091.79974914788,1092.23462245783,1092.66949576764,1093.1043690773,1093.5392423868,
1093.97411569616,1094.40898900538,1094.84386231444,1095.27873562335,1095.71360893212,
1096.14933493327,1096.58506093443,1097.0199342429,1097.45480755122,1097.88968085939,
1098.32455416742,1098.75942747531,1099.19430078305,1099.62917409064,1100.06404739809,
1100.4989207054,1100.93379401257,1101.36866731959,1101.80354062648,1102.23841393323,
1102.67328723984,1103.10901323993,1103.54473924001,1103.97961254636,1104.41448585257,
1104.84935915865,1105.2842324646,1105.71910577042,1106.15397907612,1106.58885238169,
1107.02372568714,1107.45859899246,1107.89347229767,1108.32834560276,1108.76321890774,
1109.1980922126,1109.63296551736,1110.06869151652,1110.50441751569,1110.93929082023,
1111.37416412466,1111.80903742899,1112.24391073322,1112.67878403735,1113.11365734139,
1113.54853064533,1113.98340394918,1114.41827725295,1114.85315055662,1115.28802386022,
1115.72289716374,1116.15777046717,1116.59264377053,1117.02836976903,1117.46409576752,
1117.89896907074,1118.33384237389,1118.76871567698,1119.20358898,1119.63846228297,
1120.07333558588,1120.50820888874,1120.94308219154,1121.3779554943,1121.81282879702,
1122.24770209969,1122.68257540233,1123.11744870492,1123.55232200749,1123.98804800561,
1124.42377400372,1124.85864730623,1125.29352060871,1125.72839391118,1126.16326721362,
1126.59814051605,1127.03301381847,1127.46788712088,1127.90276042328,1128.33763372568,
1128.77250702808,1129.20738033048,1129.64225363289,1130.07712693531,1130.51200023774,
1130.94772623581,1131.38345223388,1131.81832553634,1132.25319883883,1132.68807214134,
1133.12294544387,1133.55781874644,1133.99269204904,1134.42756535167,1134.86243865434,
1135.29731195706,1135.73218525982,1136.16705856263,1136.60193186548,1137.03680516839,
1137.47167847136,1137.90740446972,1138.34313046808,1138.77800377117,1139.21287707432,
1139.64775037754,1140.08262368083,1140.51749698419,1140.95237028763,1141.38724359114,
1141.82211689474,1142.25699019842,1142.69186350218,1143.12673680603,1143.56161010998,
1143.99648341401,1144.43135671814,1144.86708271711,1145.30280871607,1145.7376820204,
1146.17255532483,1146.60742862936,1147.04230193401,1147.47717523876,1147.91204854362,
1148.3469218486,1148.78179515369,1149.2166684589,1149.65154176423,1150.08641506968,
1150.52128837525,1150.95616168094,1151.39103498677,1151.82676098659,1152.26248698641,
1152.69736029249,1153.1322335987,1153.56710690504,1154.00198021152,1154.43685351813,
1154.87172682488,1155.30660013177,1155.7414734388,1156.17634674597,1156.61122005327,
1157.04609336073,1157.48096666832,1157.91583997606,1158.35071328394,1158.7864392848,
1159.22216528566,1159.65703859384,1160.09191190216,1160.52678521063,1160.96165851925,
1161.39653182801,1161.83140513693,1162.26627844599,1162.7011517552,1163.13602506456,
1163.57089837407,1164.00577168373,1164.44064499353,1164.87551830349,1165.74611761556,
1166.18184361753,1166.61671692792,1167.05159023846,1167.48646354915,1167.92133685998,
1168.35621017096,1169.22595679333,1170.09570341627,1170.53057672794,1170.96545003975,
1171.4003233517,1171.83519666377,1172.27006997598,1172.705795979,1173.57639529447,
1174.44614191977,1174.8810152326,1175.31588854555,1176.18563517179,1177.05538179847,
1177.92512842556,1178.79487505304,1179.66547437075,1180.53607368863,1181.40582031696,
1182.27556694557,1183.14531357444,1184.01506020352,1184.88480683277,1185.75455346216,
1186.62515278112,1187.4957521001,1188.36549872963,1189.23524535914,1190.10499198858,
1190.97473861791,1191.84448524708,1192.71423187606,1193.58483119448,1194.45543051277,
1195.3251771411,1196.19492376911,1197.06467039678,1197.93441702407,1198.80416365096,
1199.67391027742,1200.5445095938,1201.41510890996,1202.28485553525,1203.15460216005,
1204.02434878434,1204.89409540809,1205.76384203131,1206.1987153427,1206.63358865396,
1207.06846196508,1207.50418796741,1208.37478728058,1209.2445339018,1209.6794072122,
1210.11428052245,1210.54915383255,1210.9840271425,1211.41890045231,1211.85377376197,
1212.28864707147,1212.72352038083,1213.15839369005,1213.59326699911,1214.02814030802,
1214.46386630925,1214.89959231048,1215.3344656191,1215.76933892757,1216.20421223589,
1216.63908554406,1217.07395885209,1217.50883215998,1217.94370546771,1218.37857877531,
1218.81345208276,1219.24832539007,1219.68319869724,1220.11807200426,1220.55294531115,
1220.9878186179,1221.42354461805,1221.85927061821,1222.29414392468,1222.72901723103,
1223.16389053724,1223.59876384332,1224.03363714927,1224.46851045509,1224.90338376079,
1225.33825706636,1225.77313037181,1226.20800367713,1226.64287698234,1227.07775028743,
1227.51262359241,1227.94749689727,1228.3832228965,1228.81894889572,1229.25382220036,
1229.6886955049,1230.12356880933,1230.55844211366,1230.99331541789,1231.42818872202,
1231.86306202606,1232.29793533,1232.73280863385,1233.16768193762,1233.60255524129,
1234.03742854489,1234.4723018484,1234.90717515184,1235.34290115037,1235.7786271489,
1236.21350045219,1236.64837375541,1237.08324705856,1237.51812036165,1237.95299366467,
1238.38786696764,1238.82274027055,1239.25761357341,1239.69248687621,1240.12736017897,
1240.56223348169,1240.99710678436,1241.431980087,1241.8668533896,1242.30257938773,
1242.73830538585,1243.17317868839,1243.6080519909,1244.04292529338,1244.47779859585,
1244.91267189829,1245.34754520072,1245.78241850314,1246.21729180555,1246.65216510795,
1247.08703841035,1247.52191171275,1247.95678501515,1248.39165831756,1248.82653161998,
1249.26225761804,1249.69798361611,1250.13285691855,1250.56773022101,1251.0026035235,
1251.43747682601,1251.87235012854,1252.30722343111,1252.74209673371,1253.17697003634,
1253.61184333901,1254.04671664173,1254.48158994449,1254.9164632473,1255.35133655015,
1255.78620985306,1256.22193585139,1256.65766184973,1257.09253515275,1257.52740845584,
1257.96228175899,1258.39715506221,1258.8320283655,1259.26690166886,1259.7017749723,
1260.13664827581,1260.57152157941,1261.00639488309,1261.44126818685,1261.8761414907,
1262.31101479465,1262.74588809868,1263.1816140976,1263.61734009651,1264.05221340074,
1264.48708670507,1264.9219600095,1265.35683331403,1265.79170661868,1266.22657992343,
1266.66145322829,1267.09632653327,1267.53119983836,1267.96607314357,1268.4009464489,
1268.83581975434,1269.27069305992,1269.70556636561,1270.14129236537,1270.57701836513,
1271.01189167108,1271.44676497716,1271.88163828337,1272.31651158971,1272.75138489619,
1273.1862582028,1273.62113150955,1274.05600481644,1274.49087812347,1274.92575143063,
1275.36062473794,1275.79549804539,1276.23037135299,1276.66524466073,1277.10097066151,
1277.5366966623,1277.97156997033,1278.40644327851,1278.84131658683,1279.2761898953,
1279.71106320392,1280.14593651268,1280.5808098216,1281.01568313066,1281.45055643987,
1281.88542974923,1282.32030305874,1282.75517636839,1283.1900496782,1283.62492298815,
1284.06064899005,1284.49637499195,1284.9312483022,1285.36612161259,1285.80099492313,
1286.23586823382,1286.67074154465,1287.54048816674,1287.975361478,1288.4102347894,
1288.84510810093,1289.27998141261,1289.71485472442,1290.14972803636,1291.02032735139,
1291.89092666668,1292.32579997914,1292.76067329173,1293.19554660444,1293.63041991727,
1294.50016654328,1295.36991316974,1296.23965979663,1297.10940642392,1297.9800057415,
1298.85060505925,1299.72035168742,1300.5900983159,1301.45984494464,1302.32959157362,
1303.19933820279,1304.06908483212,1304.93968415104,1305.81028347,1306.68003009953,
1307.54977672906,1308.41952335854,1309.28926998793,1310.15901661718,1311.02876324626,
1311.89936256477,1312.76996188316,1313.63970851164,1314.50945513981,1315.37920176765,
1316.24894839514,1317.11869502223,1317.98844164891,1318.85904096546,1319.72964028179,
1320.59938690733,1321.46913353238,1322.33888015692,1323.20862678095,1323.64350009276,
1324.07837340443,1324.51324671597,1324.94812002737,1325.81871934103,1326.68931865441,
1327.12419196524,1327.55906527593,1327.99393858647,1328.42881189686,1328.86368520711,
1329.29855851721,1329.73343182716,1330.16830513697,1330.60317844663,1331.03805175614,
1331.4729250655,1331.90779837471,1332.34267168377,1332.77839768507,1333.21412368638,
1333.64899699514,1334.08387030376,1334.51874361223,1334.95361692055,1335.38849022873,
1335.82336353676,1336.25823684464,1336.69311015238,1337.12798345997,1337.56285676742,
1337.99773007473,1338.4326033819,1338.86747668892,1339.30234999581,1339.73807599603,
1340.17380199625,1340.60867530287,1341.04354860934,1341.47842191569,1341.9132952219,
1342.34816852798,1342.78304183393,1343.21791513975,1343.65278844545,1344.08766175102,
1344.52253505647,1344.95740836179,1345.392281667,1345.82715497209,1346.26202827707,
1346.69775427635,1347.13348027563,1347.56835358038,1348.00322688502,1348.43810018956,
1348.87297349399,1349.30784679832,1349.74272010255,1350.17759340668,1350.61246671072,
1351.04734001466,1351.48221331851,1351.91708662228,1352.35195992595,1352.78683322955,
1353.22170653306,1353.65743253163,1354.09315853019,1354.52803183356,1354.96290513685,
1355.39777844007,1355.83265174322,1356.26752504631,1356.70239834933,1357.1372716523,
1357.57214495521,1358.00701825807,1358.44189156087,1358.87676486363,1359.31163816635,
1359.74651146902,1360.18138477166,1360.6171107698,1361.05283676795,1361.48771007051,
1361.92258337305,1362.35745667556,1362.79232997804,1363.2272032805,1363.66207658295,
1364.09694988538,1364.5318231878,1364.96669649021,1365.40156979261,1365.83644309501,
1366.27131639741,1366.70618969981,1367.14106300222,1367.57678900028,1368.01251499834,
1368.44738830077,1368.88226160321,1369.31713490567,1369.75200820816,1370.18688151067,
1370.6217548132,1371.05662811577,1371.49150141837,1371.926374721,1372.36124802367,
1372.79612132639,1373.23099462915,1373.66586793196,1374.10074123481,1374.53646723311,
1374.97219323142,1375.40706653438,1375.84193983741,1376.2768131405,1376.71168644365,
1377.14655974687,1377.58143305016,1378.01630635352,1378.45117965696,1378.88605296047,
1379.32092626407,1379.75579956775,1380.19067287151,1380.62554617536,1381.06041947931,
1381.49614547817,1381.93187147704,1382.36674478117,1382.8016180854,1383.23649138973,
1383.67136469416,1384.10623799869,1384.54111130334,1384.97598460809,1385.41085791295,
1385.84573121793,1386.28060452302,1386.71547782823,1387.15035113356,1387.585224439,
1388.02009774458,1388.45582374427,1388.89154974397,1389.32642304979,1389.76129635574,
1390.19616966182,1390.63104296803,1391.06591627437,1391.50078958085,1391.93566288746,
1392.37053619421,1392.8054095011,1393.24028280813,1393.6751561153,1394.1100294226,
1394.54490273005,1394.97977603765,1395.41550203836,1395.85122803908,1396.28610134696,
1396.72097465499,1397.15584796317,1397.59072127149,1398.02559457996,1398.46046788858,
1398.89534119734,1399.33021450626,1399.76508781532,1400.19996112453,1400.63483443389,
1401.50458105306,1401.93945436286,1402.37518036469,1402.81090636651,1403.24577967661,
1403.68065298686,1404.11552629725,1404.5503996078,1404.98527291848,1405.85501954029,
1406.2898928514,1406.72476616266,1407.15963947406,1407.5945127856,1408.02938609727,
1408.46425940908,1409.33485872391,1410.205458039,1410.64033135134,1411.07520466381,
1411.51007797639,1411.9449512891,1412.81469791488,1413.68444454112,1414.5541911678,
1415.42393779489,1416.29453711233,1417.16513642995,1418.03488305796,1418.90462968629,
1419.77437631491,1420.64412294377,1421.51386957285,1422.38361620211,1423.25421552099,
1424.12481483992,1424.99456146943,1425.86430809896,1426.73405472847,1427.60380135791,
1428.47354798724,1429.34329461641,1430.21389393501,1431.08449325349,1431.9542398821,
1432.82398651043,1433.69373313844,1434.56347976611,1435.4332263934,1436.30297302029,
1437.17357233701,1438.04417165351,1438.91391827929,1439.78366490459,1440.65341152939,
1441.52315815367,1441.95803146562,1442.39290477743,1442.8277780891,1443.26265140064,
1444.13325071451,1445.00385002811,1445.43872333908,1445.87359664991,1446.3084699606,
1446.74334327114,1447.17821658153,1447.61308989178,1448.48283651184,1448.91770982164,
1449.3525831313,1449.78745644081,1450.22232975017,1450.65720305938,1451.09292906076,
1451.52865506214,1451.96352837105,1452.39840167982,1452.83327498843,1453.2681482969,
1453.70302160522,1454.1378949134,1454.57276822143,1455.00764152931,1455.44251483705,
1455.87738814464,1456.31226145209,1456.7471347594,1457.18200806657,1457.6168813736,
1458.05260737389,1458.48833337418,1458.92320668093,1459.35807998754,1459.79295329402,
1460.22782660036,1460.66269990657,1461.09757321265,1461.5324465186,1461.96731982443,
1462.40219313012,1462.83706643569,1463.27193974114,1463.70681304647,1464.14168635168,
1464.57655965677,1465.0122856561,1465.44801165544,1465.8828849603,1466.31775826505,
1466.7526315697,1467.18750487423,1467.62237817866,1468.05725148299,1468.49212478722,
1468.92699809135,1469.36187139539,1469.79674469933,1470.23161800319,1470.66649130695,
1471.10136461063,1471.53623791422,1471.97196391283,1472.40768991143,1472.84256321487,
1473.27743651823,1473.71230982152,1474.14718312474,1474.58205642789,1475.01692973098,
1475.451803034,1475.88667633697,1476.32154963988,1476.75642294274,1477.19129624555,
1477.62616954831,1478.06104285102,1478.4959161537,1478.93164215186,1479.36736815002,
1479.80224145262,1480.23711475519,1480.67198805772,1481.10686136023,1481.54173466272,
1481.97660796518,1482.41148126762,1482.84635457005,1483.28122787247,1483.71610117488,
1484.15097447728,1484.58584777968,1485.02072108208,1485.45559438449,1485.89132038254,
1486.32704638059,1486.76191968301,1487.19679298544,1487.63166628788,1488.06653959035,
1488.50141289283,1488.93628619534,1489.37115949787,1489.80603280044,1490.24090610304,
1490.67577940567,1491.11065270835,1491.54552601106,1491.98039931382,1492.41527261663,
1492.8509986149,1493.28672461318,1493.72159791609,1494.15647121906,1494.59134452208,
1495.02621782517,1495.46109112832,1495.89596443154,1496.33083773483,1496.76571103819,
1497.20058434163,1497.63545764515,1498.07033094874,1498.50520425242,1498.94007755618,
1499.37495086004,1499.81067685885,1500.24640285767,1500.68127616171,1501.11614946584,
1501.55102277007,1501.9858960744,1502.42076937883,1502.85564268337,1503.29051598801,
1503.72538929276,1504.16026259762,1504.5951359026,1505.03000920769,1505.4648825129,
1505.89975581823,1506.33462912368,1506.77035512331,1507.20608112294,1507.64095442864,
1508.07582773446,1508.51070104041,1508.94557434649,1509.3804476527,1509.81532095904,
1510.25019426552,1510.68506757213,1511.11994087888,1511.55481418577,1511.9896874928,
1512.42456079996,1512.85943410727,1513.29430741472,1513.73003341537,1514.16575941601,
1514.60063272375,1515.03550603163,1515.47037933966,1515.90525264784,1516.34012595616,
1516.77499926463,1517.20987257325,1517.64474588201,1518.07961919093,1518.51449249999,
1518.9493658092,1519.38423911856,1519.81911242807,1520.25398573772,1520.68971173947,
1521.12543774122,1521.56031105118,1521.99518436128,1522.43005767153,1523.29980429246,
1523.73467760315,1524.16955091398,1524.60442422495,1525.03929753607,1525.47417084733,
1525.90904415873,1526.77879078194,1527.64939009657,1528.08511609939,1528.51998941146,
1528.95486272367,1529.38973603601,1530.25948266106,1531.1292292866,1531.99897591261,
1532.86872253907,1533.73846916596,1534.60906848325,1535.47966780073,1536.34941442858,
1537.21916105675,1538.08890768523,1538.95865431398,1539.82840094295,1540.69814757212,
1541.56874689096,1542.43934620985,1543.30909283933,1544.17883946886,1545.04858609839,
1545.91833272787,1546.78807935726,1547.65782598651,1548.52842530518,1549.39902462375,
1550.26877125249,1551.13851788097,1552.00826450914,1552.87801113699,1553.74775776447,
1554.61750439156,1555.48810370844,1556.35870302511,1557.22844965112,1558.09819627666,
1558.96794290171,1559.83768952626,1560.27256283834,1560.70743615028,1561.57718277377,
1562.44778208785,1563.31838140165,1563.75325471277,1564.18812802374,1564.62300133457,
1565.05787464526,1565.9276212662,1566.79736788655,1567.2322411965,1567.66711450631,
1568.10198781596,1568.53686112547,1568.97173443483,1569.40746043628,1569.84318643774,
1570.2780597468,1570.71293305571,1571.14780636448,1571.5826796731,1572.01755298157,
1572.45242628989,1572.88729959806,1573.32217290609,1573.75704621397,1574.19191952171,
1574.62679282931,1575.06166613676,1575.49653944407,1575.93141275123,1576.36713875159,
1576.80286475195,1577.23773805884,1577.67261136559,1578.1074846722,1578.54235797868,
1578.97723128502,1579.41210459124,1579.84697789732,1580.28185120327,1580.71672450909,
1581.15159781478,1581.58647112036,1582.0213444258,1582.45621773113,1582.89109103634,
1583.32681703573,1583.76254303513,1584.1974163401,1584.63228964497,1585.06716294972,
1585.50203625436,1585.9369095589,1586.37178286333,1586.80665616766,1587.24152947189,
1587.67640277602,1588.11127608005,1588.546149384,1588.98102268785,1589.41589599161,
1589.85076929529,1590.28649529394,1590.72222129258,1591.1570945961,1591.59196789953,
1592.0268412029,1592.46171450619,1592.8965878094,1593.33146111256,1593.76633441564,
1594.20120771867,1594.63608102164,1595.07095432455,1595.50582762741,1595.94070093021,
1596.37557423297,1596.81044753569,1597.24617353387,1597.68189953206,1598.11677283469,
1598.55164613729,1598.98651943985,1599.42139274239,1599.8562660449,1600.29113934738,
1600.72601264985,1601.16088595229,1601.59575925472,1602.03063255714,1602.46550585955,
1602.90037916195,1603.33525246435,1603.77012576675,1604.2058517648,1604.64157776285,
1605.07645106526,1605.51132436768,1605.94619767011,1606.38107097255,1606.81594427502,
1607.2508175775,1607.68569088001,1608.12056418254,1608.55543748511,1608.99031078771,
1609.42518409034,1609.86005739302,1610.29493069573,1610.72980399849,1611.16552999674,
1611.60125599499,1612.03612929785,1612.47100260076,1612.90587590373,1613.34074920675,
1613.77562250984,1614.21049581299,1614.64536911621,1615.0802424195,1615.51511572286,
1615.9499890263,1616.38486232981,1616.81973563341,1617.25460893709,1617.68948224085,
1618.12520823963,1618.5609342384,1618.99580754234,1619.43068084638,1619.86555415051,
1620.30042745474,1620.73530075907,1621.1701740635,1621.60504736804,1622.03992067268,
1622.47479397743,1622.90966728229,1623.34454058727,1623.77941389236,1624.21428719757,
1624.6491605029,1625.08488650247,1625.52061250204,1625.95548580761,1626.39035911331,
1626.82523241913,1627.26010572508,1627.69497903116,1628.12985233737,1628.56472564372,
1628.99959895019,1629.43447225681,1629.86934556356,1630.30421887044,1630.73909217747,
1631.17396548464,1631.60883879195,1632.04456479252,1632.48029079309,1632.91516410068,
1633.35003740842,1633.78491071631,1634.21978402433,1634.65465733251,1635.08953064083,
1635.5244039493,1635.95927725792,1636.39415056668,1636.8290238756,1637.26389718466,
1637.69877049387,1638.13364380323,1638.56851711274,1639.00424311442,1639.43996911609,
1639.8748424259,1640.30971573585,1640.74458904595,1641.6143356666,1642.04920897714,
1642.48408228782,1642.91895559865,1643.35382890963,1643.78870222074,1644.223575532,
1645.09332215494,1645.52819546661,1645.96392146936,1646.39964747212,1646.83452078406,
1647.26939409614,1647.70426740834,1648.57401403314,1649.44376065844,1650.31350728422,
1650.74838059729,1651.18325391046,1652.05300053714,1652.92359985428,1653.79419917162,
1654.66394579929,1655.5336924273,1656.40343905563,1657.27318568424,1658.14293231311,
1659.01267894219,1659.88327826096,1660.75387757982,1661.62362420926,1662.49337083877,
1663.3631174683,1664.23286409781,1665.10261072725,1665.97235735658,1666.84295667531,
1667.71355599396,1668.58330262282,1669.45304925143,1670.32279587976,1671.19254250778,
1672.06228913544,1672.93203576273,1673.80263507977,1674.6732343966,1675.54298102284,
1676.41272764862,1677.28247427392,1678.15222089872,1679.021967523,1679.89171414676,
1680.76231346105,1681.19803946366,1681.63291277506,1682.06778608632,1682.50265939743,
1682.93753270841,1683.37240601924,1684.24215264047,1684.67702595086,1685.11189926111,
1685.54677257121,1685.98164588116,1686.41651919097,1686.85139250063,1687.28626581014,
1687.72199181166,1688.15771781319,1688.5925911224,1689.02746443146,1689.46233774038,
1689.89721104914,1690.33208435776,1690.76695766623,1691.20183097455,1691.63670428272,
1692.07157759075,1692.50645089864,1692.94132420637,1693.37619751397,1693.81107082142,
1694.24594412873,1694.68167012916,1695.11739612959,1695.55226943662,1695.9871427435,
1696.42201605025,1696.85688935687,1697.29176266334,1697.72663596969,1698.1615092759,
1698.59638258198,1699.03125588793,1699.46612919375,1699.90100249945,1700.33587580502,
1700.77074911047,1701.20562241579,1701.64134841525,1702.0770744147,1702.51194771979,
1702.94682102476,1703.38169432963,1703.81656763438,1704.25144093902,1704.68631424356,
1705.12118754799,1705.55606085232,1705.99093415655,1706.42580746068,1706.86068076471,
1707.29555406866,1707.73042737251,1708.16530067627,1708.60102667496,1709.03675267365,
1709.47162597724,1709.90649928076,1710.34137258419,1710.77624588756,1711.21111919085,
1711.64599249406,1712.08086579722,1712.5157391003,1712.95061240333,1713.3854857063,
1713.82035900921,1714.25523231207,1714.69010561487,1715.12497891763,1715.56070491584,
1715.99643091404,1716.43130421671,1716.86617751935,1717.30105082195,1717.73592412451,
1718.17079742705,1718.60567072956,1719.04054403204,1719.4754173345,1719.91029063695,
1720.34516393938,1720.7800372418,1721.21491054421,1721.64978384661,1722.08465714901,
1722.52038314706,1722.9561091451,1723.39098244751,1723.82585574992,1724.26072905233,
1724.69560235476,1725.13047565721,1725.56534895967,1726.00022226216,1726.43509556467,
1726.8699688672,1727.30484216977,1727.73971547236,1728.174588775,1728.60946207767,
1729.04433538039,1729.48006137861,1729.91578737684,1730.35066067965,1730.78553398251,
1731.22040728542,1731.65528058838,1732.09015389141,1732.5250271945,1732.95990049765,
1733.39477380087,1733.82964710416,1734.26452040752,1734.69939371096,1735.13426701447,
1735.56914031807,1736.00401362175,1736.43973962048,1736.8754656192,1737.31033892306,
1737.745212227,1738.18008553104,1738.61495883517,1739.0498321394,1739.48470544373,
1739.91957874816,1740.35445205269,1740.78932535734,1741.22419866209,1741.65907196695,
1742.09394527193,1742.52881857702,1742.96369188223,1743.39941788174,1743.83514388125,
1744.2700171867,1744.70489049227,1745.13976379797,1745.57463710379,1746.00951040974,
1746.44438371582,1746.87925702203,1747.31413032837,1747.74900363485,1748.18387694146,
1748.61875024821,1749.0536235551,1749.48849686213,1749.92337016929,1750.3590961698,
1750.7948221703,1751.22969547775,1751.66456878534,1752.09944209308,1752.53431540096,
1752.96918870899,1753.40406201717,1753.83893532549,1754.27380863396,1754.70868194258,
1755.14355525134,1755.57842856026,1756.01330186932,1756.44817517853,1756.88304848789,
1757.31877448949,1757.75450049109,1758.18937380075,1759.05912042051,1759.49399373061,
1759.92886704086,1760.36374035125,1760.79861366179,1761.23348697248,1761.66836028331,
1762.10323359429,1762.5381069054,1763.40785352806,1763.8427268396,1764.27845284228,
1764.71417884496,1765.14905215677,1765.58392546872,1766.0187987808,1766.88854540534,
1767.75829203039,1768.1931653431,1768.62803865593,1769.06291196888,1769.49778528195,
1770.36753190841,1771.2381312254,1772.10873054259,1772.97847717007,1773.84822379791,
1774.71797042609,1775.58771705456,1776.45746368331,1777.32721031228,1778.19780963089,
1779.06840894783,1779.93815555508,1780.80790201176,1781.67764871408),(-0.58309518948453,
0.),.UNSPECIFIED.) ;
#820=B_SPLINE_SURFACE_WITH_KNOTS('',3,1,((#26267,#26268),(#26269,#26270),
(#26271,#26272),(#26273,#26274),(#26275,#26276),(#26277,#26278),(#26279,
#26280),(#26281,#26282),(#26283,#26284),(#26285,#26286),(#26287,#26288),
(#26289,#26290),(#26291,#26292),(#26293,#26294),(#26295,#26296),(#26297,
#26298),(#26299,#26300),(#26301,#26302),(#26303,#26304),(#26305,#26306),
(#26307,#26308),(#26309,#26310),(#26311,#26312),(#26313,#26314),(#26315,
#26316),(#26317,#26318),(#26319,#26320),(#26321,#26322),(#26323,#26324),
(#26325,#26326),(#26327,#26328),(#26329,#26330),(#26331,#26332),(#26333,
#26334),(#26335,#26336),(#26337,#26338),(#26339,#26340),(#26341,#26342),
(#26343,#26344),(#26345,#26346),(#26347,#26348),(#26349,#26350),(#26351,
#26352),(#26353,#26354),(#26355,#26356),(#26357,#26358),(#26359,#26360),
(#26361,#26362),(#26363,#26364),(#26365,#26366),(#26367,#26368),(#26369,
#26370),(#26371,#26372),(#26373,#26374),(#26375,#26376),(#26377,#26378),
(#26379,#26380),(#26381,#26382),(#26383,#26384),(#26385,#26386),(#26387,
#26388),(#26389,#26390),(#26391,#26392),(#26393,#26394),(#26395,#26396),
(#26397,#26398),(#26399,#26400),(#26401,#26402),(#26403,#26404),(#26405,
#26406),(#26407,#26408),(#26409,#26410),(#26411,#26412),(#26413,#26414),
(#26415,#26416),(#26417,#26418),(#26419,#26420),(#26421,#26422),(#26423,
#26424),(#26425,#26426),(#26427,#26428),(#26429,#26430),(#26431,#26432),
(#26433,#26434),(#26435,#26436),(#26437,#26438),(#26439,#26440),(#26441,
#26442),(#26443,#26444),(#26445,#26446),(#26447,#26448),(#26449,#26450),
(#26451,#26452),(#26453,#26454),(#26455,#26456),(#26457,#26458),(#26459,
#26460),(#26461,#26462),(#26463,#26464),(#26465,#26466),(#26467,#26468),
(#26469,#26470),(#26471,#26472),(#26473,#26474),(#26475,#26476),(#26477,
#26478),(#26479,#26480),(#26481,#26482),(#26483,#26484),(#26485,#26486),
(#26487,#26488),(#26489,#26490),(#26491,#26492),(#26493,#26494),(#26495,
#26496),(#26497,#26498),(#26499,#26500),(#26501,#26502),(#26503,#26504),
(#26505,#26506),(#26507,#26508),(#26509,#26510),(#26511,#26512),(#26513,
#26514),(#26515,#26516),(#26517,#26518),(#26519,#26520),(#26521,#26522),
(#26523,#26524),(#26525,#26526),(#26527,#26528),(#26529,#26530),(#26531,
#26532),(#26533,#26534),(#26535,#26536),(#26537,#26538),(#26539,#26540),
(#26541,#26542),(#26543,#26544),(#26545,#26546),(#26547,#26548),(#26549,
#26550),(#26551,#26552),(#26553,#26554),(#26555,#26556),(#26557,#26558),
(#26559,#26560),(#26561,#26562),(#26563,#26564),(#26565,#26566),(#26567,
#26568),(#26569,#26570),(#26571,#26572),(#26573,#26574),(#26575,#26576),
(#26577,#26578),(#26579,#26580),(#26581,#26582),(#26583,#26584),(#26585,
#26586),(#26587,#26588),(#26589,#26590),(#26591,#26592),(#26593,#26594),
(#26595,#26596),(#26597,#26598),(#26599,#26600),(#26601,#26602),(#26603,
#26604),(#26605,#26606),(#26607,#26608),(#26609,#26610),(#26611,#26612),
(#26613,#26614),(#26615,#26616),(#26617,#26618),(#26619,#26620),(#26621,
#26622),(#26623,#26624),(#26625,#26626),(#26627,#26628),(#26629,#26630),
(#26631,#26632),(#26633,#26634),(#26635,#26636),(#26637,#26638),(#26639,
#26640),(#26641,#26642),(#26643,#26644),(#26645,#26646),(#26647,#26648),
(#26649,#26650),(#26651,#26652),(#26653,#26654),(#26655,#26656),(#26657,
#26658),(#26659,#26660),(#26661,#26662),(#26663,#26664),(#26665,#26666),
(#26667,#26668),(#26669,#26670),(#26671,#26672),(#26673,#26674),(#26675,
#26676),(#26677,#26678),(#26679,#26680),(#26681,#26682),(#26683,#26684),
(#26685,#26686),(#26687,#26688),(#26689,#26690),(#26691,#26692),(#26693,
#26694),(#26695,#26696),(#26697,#26698),(#26699,#26700),(#26701,#26702),
(#26703,#26704),(#26705,#26706),(#26707,#26708),(#26709,#26710),(#26711,
#26712),(#26713,#26714),(#26715,#26716),(#26717,#26718),(#26719,#26720),
(#26721,#26722),(#26723,#26724),(#26725,#26726),(#26727,#26728),(#26729,
#26730),(#26731,#26732),(#26733,#26734),(#26735,#26736),(#26737,#26738),
(#26739,#26740),(#26741,#26742),(#26743,#26744),(#26745,#26746),(#26747,
#26748),(#26749,#26750),(#26751,#26752),(#26753,#26754),(#26755,#26756),
(#26757,#26758),(#26759,#26760),(#26761,#26762),(#26763,#26764),(#26765,
#26766),(#26767,#26768),(#26769,#26770),(#26771,#26772),(#26773,#26774),
(#26775,#26776),(#26777,#26778),(#26779,#26780),(#26781,#26782),(#26783,
#26784),(#26785,#26786),(#26787,#26788),(#26789,#26790),(#26791,#26792),
(#26793,#26794),(#26795,#26796),(#26797,#26798),(#26799,#26800),(#26801,
#26802),(#26803,#26804),(#26805,#26806),(#26807,#26808),(#26809,#26810),
(#26811,#26812),(#26813,#26814),(#26815,#26816),(#26817,#26818),(#26819,
#26820),(#26821,#26822),(#26823,#26824),(#26825,#26826),(#26827,#26828),
(#26829,#26830),(#26831,#26832),(#26833,#26834),(#26835,#26836),(#26837,
#26838),(#26839,#26840),(#26841,#26842),(#26843,#26844),(#26845,#26846),
(#26847,#26848),(#26849,#26850),(#26851,#26852),(#26853,#26854),(#26855,
#26856),(#26857,#26858),(#26859,#26860),(#26861,#26862),(#26863,#26864),
(#26865,#26866),(#26867,#26868),(#26869,#26870),(#26871,#26872),(#26873,
#26874),(#26875,#26876),(#26877,#26878),(#26879,#26880),(#26881,#26882),
(#26883,#26884),(#26885,#26886),(#26887,#26888),(#26889,#26890),(#26891,
#26892),(#26893,#26894),(#26895,#26896),(#26897,#26898),(#26899,#26900),
(#26901,#26902),(#26903,#26904),(#26905,#26906),(#26907,#26908),(#26909,
#26910),(#26911,#26912),(#26913,#26914),(#26915,#26916),(#26917,#26918),
(#26919,#26920),(#26921,#26922),(#26923,#26924),(#26925,#26926),(#26927,
#26928),(#26929,#26930),(#26931,#26932),(#26933,#26934),(#26935,#26936),
(#26937,#26938),(#26939,#26940),(#26941,#26942),(#26943,#26944),(#26945,
#26946),(#26947,#26948),(#26949,#26950),(#26951,#26952),(#26953,#26954),
(#26955,#26956),(#26957,#26958),(#26959,#26960),(#26961,#26962),(#26963,
#26964),(#26965,#26966),(#26967,#26968),(#26969,#26970),(#26971,#26972),
(#26973,#26974),(#26975,#26976),(#26977,#26978),(#26979,#26980),(#26981,
#26982),(#26983,#26984),(#26985,#26986),(#26987,#26988),(#26989,#26990),
(#26991,#26992),(#26993,#26994),(#26995,#26996),(#26997,#26998),(#26999,
#27000),(#27001,#27002),(#27003,#27004),(#27005,#27006),(#27007,#27008),
(#27009,#27010),(#27011,#27012),(#27013,#27014),(#27015,#27016),(#27017,
#27018),(#27019,#27020),(#27021,#27022),(#27023,#27024),(#27025,#27026),
(#27027,#27028),(#27029,#27030),(#27031,#27032),(#27033,#27034),(#27035,
#27036),(#27037,#27038),(#27039,#27040),(#27041,#27042),(#27043,#27044),
(#27045,#27046),(#27047,#27048),(#27049,#27050),(#27051,#27052),(#27053,
#27054),(#27055,#27056),(#27057,#27058),(#27059,#27060),(#27061,#27062),
(#27063,#27064),(#27065,#27066),(#27067,#27068),(#27069,#27070),(#27071,
#27072),(#27073,#27074),(#27075,#27076),(#27077,#27078),(#27079,#27080),
(#27081,#27082),(#27083,#27084),(#27085,#27086),(#27087,#27088),(#27089,
#27090),(#27091,#27092),(#27093,#27094),(#27095,#27096),(#27097,#27098),
(#27099,#27100),(#27101,#27102),(#27103,#27104),(#27105,#27106),(#27107,
#27108),(#27109,#27110),(#27111,#27112),(#27113,#27114),(#27115,#27116),
(#27117,#27118),(#27119,#27120),(#27121,#27122),(#27123,#27124),(#27125,
#27126),(#27127,#27128),(#27129,#27130),(#27131,#27132),(#27133,#27134),
(#27135,#27136),(#27137,#27138),(#27139,#27140),(#27141,#27142),(#27143,
#27144),(#27145,#27146),(#27147,#27148),(#27149,#27150),(#27151,#27152),
(#27153,#27154),(#27155,#27156),(#27157,#27158),(#27159,#27160),(#27161,
#27162),(#27163,#27164),(#27165,#27166),(#27167,#27168),(#27169,#27170),
(#27171,#27172),(#27173,#27174),(#27175,#27176),(#27177,#27178),(#27179,
#27180),(#27181,#27182),(#27183,#27184),(#27185,#27186),(#27187,#27188),
(#27189,#27190),(#27191,#27192),(#27193,#27194),(#27195,#27196),(#27197,
#27198),(#27199,#27200),(#27201,#27202),(#27203,#27204),(#27205,#27206),
(#27207,#27208),(#27209,#27210),(#27211,#27212),(#27213,#27214),(#27215,
#27216),(#27217,#27218),(#27219,#27220),(#27221,#27222),(#27223,#27224),
(#27225,#27226),(#27227,#27228),(#27229,#27230),(#27231,#27232),(#27233,
#27234),(#27235,#27236),(#27237,#27238),(#27239,#27240),(#27241,#27242),
(#27243,#27244),(#27245,#27246),(#27247,#27248),(#27249,#27250),(#27251,
#27252),(#27253,#27254),(#27255,#27256),(#27257,#27258),(#27259,#27260),
(#27261,#27262),(#27263,#27264),(#27265,#27266),(#27267,#27268),(#27269,
#27270),(#27271,#27272),(#27273,#27274),(#27275,#27276),(#27277,#27278),
(#27279,#27280),(#27281,#27282),(#27283,#27284),(#27285,#27286),(#27287,
#27288),(#27289,#27290),(#27291,#27292),(#27293,#27294),(#27295,#27296),
(#27297,#27298),(#27299,#27300),(#27301,#27302),(#27303,#27304),(#27305,
#27306),(#27307,#27308),(#27309,#27310),(#27311,#27312),(#27313,#27314),
(#27315,#27316),(#27317,#27318),(#27319,#27320),(#27321,#27322),(#27323,
#27324),(#27325,#27326),(#27327,#27328),(#27329,#27330),(#27331,#27332),
(#27333,#27334),(#27335,#27336),(#27337,#27338),(#27339,#27340),(#27341,
#27342),(#27343,#27344),(#27345,#27346),(#27347,#27348),(#27349,#27350),
(#27351,#27352),(#27353,#27354),(#27355,#27356),(#27357,#27358),(#27359,
#27360),(#27361,#27362),(#27363,#27364),(#27365,#27366),(#27367,#27368),
(#27369,#27370),(#27371,#27372),(#27373,#27374),(#27375,#27376),(#27377,
#27378),(#27379,#27380),(#27381,#27382),(#27383,#27384),(#27385,#27386),
(#27387,#27388),(#27389,#27390),(#27391,#27392),(#27393,#27394),(#27395,
#27396),(#27397,#27398),(#27399,#27400),(#27401,#27402),(#27403,#27404),
(#27405,#27406),(#27407,#27408),(#27409,#27410),(#27411,#27412),(#27413,
#27414),(#27415,#27416),(#27417,#27418),(#27419,#27420),(#27421,#27422),
(#27423,#27424),(#27425,#27426),(#27427,#27428),(#27429,#27430),(#27431,
#27432),(#27433,#27434),(#27435,#27436),(#27437,#27438),(#27439,#27440),
(#27441,#27442),(#27443,#27444),(#27445,#27446),(#27447,#27448),(#27449,
#27450),(#27451,#27452),(#27453,#27454),(#27455,#27456),(#27457,#27458),
(#27459,#27460),(#27461,#27462),(#27463,#27464),(#27465,#27466),(#27467,
#27468),(#27469,#27470),(#27471,#27472),(#27473,#27474),(#27475,#27476),
(#27477,#27478),(#27479,#27480),(#27481,#27482),(#27483,#27484),(#27485,
#27486),(#27487,#27488),(#27489,#27490),(#27491,#27492),(#27493,#27494),
(#27495,#27496),(#27497,#27498),(#27499,#27500),(#27501,#27502),(#27503,
#27504),(#27505,#27506),(#27507,#27508),(#27509,#27510),(#27511,#27512),
(#27513,#27514),(#27515,#27516),(#27517,#27518),(#27519,#27520),(#27521,
#27522),(#27523,#27524),(#27525,#27526),(#27527,#27528),(#27529,#27530),
(#27531,#27532),(#27533,#27534),(#27535,#27536),(#27537,#27538),(#27539,
#27540),(#27541,#27542),(#27543,#27544),(#27545,#27546),(#27547,#27548),
(#27549,#27550),(#27551,#27552),(#27553,#27554),(#27555,#27556),(#27557,
#27558),(#27559,#27560),(#27561,#27562),(#27563,#27564),(#27565,#27566),
(#27567,#27568),(#27569,#27570),(#27571,#27572),(#27573,#27574),(#27575,
#27576),(#27577,#27578),(#27579,#27580),(#27581,#27582),(#27583,#27584),
(#27585,#27586),(#27587,#27588),(#27589,#27590),(#27591,#27592),(#27593,
#27594),(#27595,#27596),(#27597,#27598),(#27599,#27600),(#27601,#27602),
(#27603,#27604),(#27605,#27606),(#27607,#27608),(#27609,#27610),(#27611,
#27612),(#27613,#27614),(#27615,#27616),(#27617,#27618),(#27619,#27620),
(#27621,#27622),(#27623,#27624),(#27625,#27626),(#27627,#27628),(#27629,
#27630),(#27631,#27632),(#27633,#27634),(#27635,#27636),(#27637,#27638),
(#27639,#27640),(#27641,#27642),(#27643,#27644),(#27645,#27646),(#27647,
#27648),(#27649,#27650),(#27651,#27652),(#27653,#27654),(#27655,#27656),
(#27657,#27658),(#27659,#27660),(#27661,#27662),(#27663,#27664),(#27665,
#27666),(#27667,#27668),(#27669,#27670),(#27671,#27672),(#27673,#27674),
(#27675,#27676),(#27677,#27678),(#27679,#27680),(#27681,#27682),(#27683,
#27684),(#27685,#27686),(#27687,#27688),(#27689,#27690),(#27691,#27692),
(#27693,#27694),(#27695,#27696),(#27697,#27698),(#27699,#27700),(#27701,
#27702),(#27703,#27704),(#27705,#27706),(#27707,#27708),(#27709,#27710),
(#27711,#27712),(#27713,#27714),(#27715,#27716),(#27717,#27718),(#27719,
#27720),(#27721,#27722),(#27723,#27724),(#27725,#27726),(#27727,#27728),
(#27729,#27730),(#27731,#27732),(#27733,#27734),(#27735,#27736),(#27737,
#27738),(#27739,#27740),(#27741,#27742),(#27743,#27744),(#27745,#27746),
(#27747,#27748),(#27749,#27750),(#27751,#27752),(#27753,#27754),(#27755,
#27756),(#27757,#27758),(#27759,#27760),(#27761,#27762),(#27763,#27764),
(#27765,#27766),(#27767,#27768),(#27769,#27770),(#27771,#27772),(#27773,
#27774),(#27775,#27776),(#27777,#27778),(#27779,#27780),(#27781,#27782),
(#27783,#27784),(#27785,#27786),(#27787,#27788),(#27789,#27790),(#27791,
#27792),(#27793,#27794),(#27795,#27796),(#27797,#27798),(#27799,#27800),
(#27801,#27802),(#27803,#27804),(#27805,#27806),(#27807,#27808),(#27809,
#27810),(#27811,#27812),(#27813,#27814),(#27815,#27816),(#27817,#27818),
(#27819,#27820),(#27821,#27822),(#27823,#27824),(#27825,#27826),(#27827,
#27828),(#27829,#27830),(#27831,#27832),(#27833,#27834),(#27835,#27836),
(#27837,#27838),(#27839,#27840),(#27841,#27842),(#27843,#27844),(#27845,
#27846),(#27847,#27848),(#27849,#27850),(#27851,#27852),(#27853,#27854),
(#27855,#27856),(#27857,#27858),(#27859,#27860),(#27861,#27862),(#27863,
#27864),(#27865,#27866),(#27867,#27868),(#27869,#27870),(#27871,#27872),
(#27873,#27874),(#27875,#27876),(#27877,#27878),(#27879,#27880),(#27881,
#27882),(#27883,#27884),(#27885,#27886),(#27887,#27888),(#27889,#27890),
(#27891,#27892),(#27893,#27894),(#27895,#27896),(#27897,#27898),(#27899,
#27900),(#27901,#27902),(#27903,#27904),(#27905,#27906),(#27907,#27908),
(#27909,#27910),(#27911,#27912),(#27913,#27914),(#27915,#27916),(#27917,
#27918),(#27919,#27920),(#27921,#27922),(#27923,#27924),(#27925,#27926),
(#27927,#27928),(#27929,#27930),(#27931,#27932),(#27933,#27934),(#27935,
#27936),(#27937,#27938),(#27939,#27940),(#27941,#27942),(#27943,#27944),
(#27945,#27946),(#27947,#27948),(#27949,#27950),(#27951,#27952),(#27953,
#27954),(#27955,#27956),(#27957,#27958),(#27959,#27960),(#27961,#27962),
(#27963,#27964),(#27965,#27966),(#27967,#27968),(#27969,#27970),(#27971,
#27972),(#27973,#27974),(#27975,#27976),(#27977,#27978),(#27979,#27980),
(#27981,#27982),(#27983,#27984),(#27985,#27986),(#27987,#27988),(#27989,
#27990),(#27991,#27992),(#27993,#27994),(#27995,#27996),(#27997,#27998),
(#27999,#28000),(#28001,#28002),(#28003,#28004),(#28005,#28006),(#28007,
#28008),(#28009,#28010),(#28011,#28012),(#28013,#28014),(#28015,#28016),
(#28017,#28018),(#28019,#28020),(#28021,#28022),(#28023,#28024),(#28025,
#28026),(#28027,#28028),(#28029,#28030),(#28031,#28032),(#28033,#28034),
(#28035,#28036),(#28037,#28038),(#28039,#28040),(#28041,#28042),(#28043,
#28044),(#28045,#28046),(#28047,#28048),(#28049,#28050),(#28051,#28052),
(#28053,#28054),(#28055,#28056),(#28057,#28058),(#28059,#28060),(#28061,
#28062),(#28063,#28064),(#28065,#28066),(#28067,#28068),(#28069,#28070),
(#28071,#28072),(#28073,#28074),(#28075,#28076),(#28077,#28078),(#28079,
#28080),(#28081,#28082),(#28083,#28084),(#28085,#28086),(#28087,#28088),
(#28089,#28090),(#28091,#28092),(#28093,#28094),(#28095,#28096),(#28097,
#28098),(#28099,#28100),(#28101,#28102),(#28103,#28104),(#28105,#28106),
(#28107,#28108),(#28109,#28110),(#28111,#28112),(#28113,#28114),(#28115,
#28116),(#28117,#28118),(#28119,#28120),(#28121,#28122),(#28123,#28124),
(#28125,#28126),(#28127,#28128),(#28129,#28130),(#28131,#28132),(#28133,
#28134),(#28135,#28136),(#28137,#28138),(#28139,#28140),(#28141,#28142),
(#28143,#28144),(#28145,#28146),(#28147,#28148),(#28149,#28150),(#28151,
#28152),(#28153,#28154),(#28155,#28156),(#28157,#28158),(#28159,#28160),
(#28161,#28162),(#28163,#28164),(#28165,#28166),(#28167,#28168),(#28169,
#28170),(#28171,#28172),(#28173,#28174),(#28175,#28176),(#28177,#28178),
(#28179,#28180),(#28181,#28182),(#28183,#28184),(#28185,#28186),(#28187,
#28188),(#28189,#28190),(#28191,#28192),(#28193,#28194),(#28195,#28196),
(#28197,#28198),(#28199,#28200),(#28201,#28202),(#28203,#28204),(#28205,
#28206),(#28207,#28208),(#28209,#28210),(#28211,#28212),(#28213,#28214),
(#28215,#28216),(#28217,#28218),(#28219,#28220),(#28221,#28222),(#28223,
#28224),(#28225,#28226),(#28227,#28228),(#28229,#28230),(#28231,#28232),
(#28233,#28234),(#28235,#28236),(#28237,#28238),(#28239,#28240),(#28241,
#28242),(#28243,#28244),(#28245,#28246),(#28247,#28248),(#28249,#28250),
(#28251,#28252),(#28253,#28254),(#28255,#28256),(#28257,#28258),(#28259,
#28260),(#28261,#28262),(#28263,#28264),(#28265,#28266),(#28267,#28268),
(#28269,#28270),(#28271,#28272),(#28273,#28274),(#28275,#28276),(#28277,
#28278),(#28279,#28280),(#28281,#28282),(#28283,#28284),(#28285,#28286),
(#28287,#28288),(#28289,#28290),(#28291,#28292),(#28293,#28294),(#28295,
#28296),(#28297,#28298),(#28299,#28300),(#28301,#28302),(#28303,#28304),
(#28305,#28306),(#28307,#28308),(#28309,#28310),(#28311,#28312),(#28313,
#28314),(#28315,#28316),(#28317,#28318),(#28319,#28320),(#28321,#28322),
(#28323,#28324),(#28325,#28326),(#28327,#28328),(#28329,#28330),(#28331,
#28332),(#28333,#28334),(#28335,#28336),(#28337,#28338),(#28339,#28340),
(#28341,#28342),(#28343,#28344),(#28345,#28346),(#28347,#28348),(#28349,
#28350),(#28351,#28352),(#28353,#28354),(#28355,#28356),(#28357,#28358),
(#28359,#28360),(#28361,#28362),(#28363,#28364),(#28365,#28366),(#28367,
#28368),(#28369,#28370),(#28371,#28372),(#28373,#28374),(#28375,#28376),
(#28377,#28378),(#28379,#28380),(#28381,#28382),(#28383,#28384),(#28385,
#28386),(#28387,#28388),(#28389,#28390),(#28391,#28392),(#28393,#28394),
(#28395,#28396),(#28397,#28398),(#28399,#28400),(#28401,#28402),(#28403,
#28404),(#28405,#28406),(#28407,#28408),(#28409,#28410),(#28411,#28412),
(#28413,#28414),(#28415,#28416),(#28417,#28418),(#28419,#28420),(#28421,
#28422),(#28423,#28424),(#28425,#28426),(#28427,#28428),(#28429,#28430),
(#28431,#28432),(#28433,#28434),(#28435,#28436),(#28437,#28438),(#28439,
#28440),(#28441,#28442),(#28443,#28444),(#28445,#28446),(#28447,#28448),
(#28449,#28450),(#28451,#28452),(#28453,#28454),(#28455,#28456),(#28457,
#28458),(#28459,#28460),(#28461,#28462),(#28463,#28464),(#28465,#28466),
(#28467,#28468),(#28469,#28470),(#28471,#28472),(#28473,#28474),(#28475,
#28476),(#28477,#28478),(#28479,#28480),(#28481,#28482),(#28483,#28484),
(#28485,#28486),(#28487,#28488),(#28489,#28490),(#28491,#28492),(#28493,
#28494),(#28495,#28496),(#28497,#28498),(#28499,#28500),(#28501,#28502),
(#28503,#28504),(#28505,#28506),(#28507,#28508),(#28509,#28510),(#28511,
#28512),(#28513,#28514),(#28515,#28516),(#28517,#28518),(#28519,#28520),
(#28521,#28522),(#28523,#28524),(#28525,#28526),(#28527,#28528),(#28529,
#28530),(#28531,#28532),(#28533,#28534),(#28535,#28536),(#28537,#28538),
(#28539,#28540),(#28541,#28542),(#28543,#28544),(#28545,#28546),(#28547,
#28548),(#28549,#28550),(#28551,#28552),(#28553,#28554),(#28555,#28556),
(#28557,#28558),(#28559,#28560),(#28561,#28562),(#28563,#28564),(#28565,
#28566),(#28567,#28568),(#28569,#28570),(#28571,#28572),(#28573,#28574),
(#28575,#28576),(#28577,#28578),(#28579,#28580),(#28581,#28582),(#28583,
#28584),(#28585,#28586),(#28587,#28588),(#28589,#28590),(#28591,#28592),
(#28593,#28594),(#28595,#28596),(#28597,#28598),(#28599,#28600),(#28601,
#28602),(#28603,#28604),(#28605,#28606),(#28607,#28608),(#28609,#28610),
(#28611,#28612),(#28613,#28614),(#28615,#28616),(#28617,#28618),(#28619,
#28620),(#28621,#28622),(#28623,#28624),(#28625,#28626),(#28627,#28628),
(#28629,#28630),(#28631,#28632),(#28633,#28634),(#28635,#28636),(#28637,
#28638),(#28639,#28640),(#28641,#28642),(#28643,#28644),(#28645,#28646),
(#28647,#28648),(#28649,#28650),(#28651,#28652),(#28653,#28654),(#28655,
#28656),(#28657,#28658),(#28659,#28660),(#28661,#28662),(#28663,#28664),
(#28665,#28666),(#28667,#28668),(#28669,#28670),(#28671,#28672),(#28673,
#28674),(#28675,#28676),(#28677,#28678),(#28679,#28680),(#28681,#28682),
(#28683,#28684),(#28685,#28686),(#28687,#28688),(#28689,#28690),(#28691,
#28692),(#28693,#28694),(#28695,#28696),(#28697,#28698),(#28699,#28700),
(#28701,#28702),(#28703,#28704),(#28705,#28706),(#28707,#28708),(#28709,
#28710),(#28711,#28712),(#28713,#28714),(#28715,#28716),(#28717,#28718),
(#28719,#28720),(#28721,#28722),(#28723,#28724),(#28725,#28726),(#28727,
#28728),(#28729,#28730),(#28731,#28732),(#28733,#28734),(#28735,#28736),
(#28737,#28738),(#28739,#28740),(#28741,#28742),(#28743,#28744),(#28745,
#28746),(#28747,#28748),(#28749,#28750),(#28751,#28752),(#28753,#28754),
(#28755,#28756),(#28757,#28758),(#28759,#28760),(#28761,#28762),(#28763,
#28764),(#28765,#28766),(#28767,#28768),(#28769,#28770),(#28771,#28772),
(#28773,#28774),(#28775,#28776),(#28777,#28778),(#28779,#28780),(#28781,
#28782),(#28783,#28784),(#28785,#28786),(#28787,#28788),(#28789,#28790),
(#28791,#28792),(#28793,#28794),(#28795,#28796),(#28797,#28798),(#28799,
#28800),(#28801,#28802),(#28803,#28804),(#28805,#28806),(#28807,#28808),
(#28809,#28810),(#28811,#28812),(#28813,#28814),(#28815,#28816),(#28817,
#28818),(#28819,#28820),(#28821,#28822),(#28823,#28824),(#28825,#28826),
(#28827,#28828),(#28829,#28830),(#28831,#28832),(#28833,#28834),(#28835,
#28836),(#28837,#28838),(#28839,#28840),(#28841,#28842),(#28843,#28844),
(#28845,#28846),(#28847,#28848),(#28849,#28850),(#28851,#28852),(#28853,
#28854),(#28855,#28856),(#28857,#28858),(#28859,#28860),(#28861,#28862),
(#28863,#28864),(#28865,#28866),(#28867,#28868),(#28869,#28870),(#28871,
#28872),(#28873,#28874),(#28875,#28876),(#28877,#28878),(#28879,#28880),
(#28881,#28882),(#28883,#28884),(#28885,#28886),(#28887,#28888),(#28889,
#28890),(#28891,#28892),(#28893,#28894),(#28895,#28896),(#28897,#28898),
(#28899,#28900),(#28901,#28902),(#28903,#28904),(#28905,#28906),(#28907,
#28908),(#28909,#28910),(#28911,#28912),(#28913,#28914),(#28915,#28916),
(#28917,#28918),(#28919,#28920),(#28921,#28922),(#28923,#28924),(#28925,
#28926),(#28927,#28928),(#28929,#28930),(#28931,#28932),(#28933,#28934),
(#28935,#28936),(#28937,#28938),(#28939,#28940),(#28941,#28942),(#28943,
#28944),(#28945,#28946),(#28947,#28948),(#28949,#28950),(#28951,#28952),
(#28953,#28954),(#28955,#28956),(#28957,#28958),(#28959,#28960),(#28961,
#28962),(#28963,#28964),(#28965,#28966),(#28967,#28968),(#28969,#28970),
(#28971,#28972),(#28973,#28974),(#28975,#28976),(#28977,#28978),(#28979,
#28980),(#28981,#28982),(#28983,#28984),(#28985,#28986),(#28987,#28988),
(#28989,#28990),(#28991,#28992),(#28993,#28994),(#28995,#28996),(#28997,
#28998),(#28999,#29000),(#29001,#29002),(#29003,#29004),(#29005,#29006),
(#29007,#29008),(#29009,#29010),(#29011,#29012),(#29013,#29014),(#29015,
#29016),(#29017,#29018),(#29019,#29020),(#29021,#29022),(#29023,#29024),
(#29025,#29026),(#29027,#29028),(#29029,#29030),(#29031,#29032),(#29033,
#29034),(#29035,#29036),(#29037,#29038),(#29039,#29040),(#29041,#29042),
(#29043,#29044),(#29045,#29046),(#29047,#29048),(#29049,#29050),(#29051,
#29052),(#29053,#29054),(#29055,#29056),(#29057,#29058),(#29059,#29060),
(#29061,#29062),(#29063,#29064),(#29065,#29066),(#29067,#29068),(#29069,
#29070),(#29071,#29072),(#29073,#29074),(#29075,#29076),(#29077,#29078),
(#29079,#29080),(#29081,#29082),(#29083,#29084),(#29085,#29086),(#29087,
#29088),(#29089,#29090),(#29091,#29092),(#29093,#29094),(#29095,#29096),
(#29097,#29098),(#29099,#29100),(#29101,#29102),(#29103,#29104),(#29105,
#29106),(#29107,#29108),(#29109,#29110),(#29111,#29112),(#29113,#29114),
(#29115,#29116),(#29117,#29118),(#29119,#29120),(#29121,#29122),(#29123,
#29124),(#29125,#29126),(#29127,#29128),(#29129,#29130),(#29131,#29132),
(#29133,#29134),(#29135,#29136),(#29137,#29138),(#29139,#29140),(#29141,
#29142),(#29143,#29144),(#29145,#29146),(#29147,#29148),(#29149,#29150),
(#29151,#29152),(#29153,#29154),(#29155,#29156),(#29157,#29158),(#29159,
#29160),(#29161,#29162),(#29163,#29164),(#29165,#29166),(#29167,#29168),
(#29169,#29170),(#29171,#29172),(#29173,#29174),(#29175,#29176),(#29177,
#29178),(#29179,#29180),(#29181,#29182),(#29183,#29184),(#29185,#29186),
(#29187,#29188),(#29189,#29190),(#29191,#29192),(#29193,#29194),(#29195,
#29196),(#29197,#29198),(#29199,#29200),(#29201,#29202),(#29203,#29204),
(#29205,#29206),(#29207,#29208),(#29209,#29210),(#29211,#29212),(#29213,
#29214),(#29215,#29216),(#29217,#29218),(#29219,#29220),(#29221,#29222),
(#29223,#29224),(#29225,#29226),(#29227,#29228),(#29229,#29230),(#29231,
#29232),(#29233,#29234),(#29235,#29236),(#29237,#29238),(#29239,#29240),
(#29241,#29242),(#29243,#29244),(#29245,#29246),(#29247,#29248),(#29249,
#29250),(#29251,#29252),(#29253,#29254),(#29255,#29256),(#29257,#29258),
(#29259,#29260),(#29261,#29262),(#29263,#29264),(#29265,#29266),(#29267,
#29268),(#29269,#29270),(#29271,#29272),(#29273,#29274),(#29275,#29276),
(#29277,#29278),(#29279,#29280),(#29281,#29282),(#29283,#29284),(#29285,
#29286),(#29287,#29288),(#29289,#29290),(#29291,#29292),(#29293,#29294),
(#29295,#29296),(#29297,#29298),(#29299,#29300),(#29301,#29302),(#29303,
#29304),(#29305,#29306),(#29307,#29308),(#29309,#29310),(#29311,#29312),
(#29313,#29314),(#29315,#29316),(#29317,#29318),(#29319,#29320),(#29321,
#29322),(#29323,#29324),(#29325,#29326),(#29327,#29328),(#29329,#29330),
(#29331,#29332),(#29333,#29334),(#29335,#29336),(#29337,#29338),(#29339,
#29340),(#29341,#29342),(#29343,#29344),(#29345,#29346),(#29347,#29348),
(#29349,#29350),(#29351,#29352),(#29353,#29354),(#29355,#29356),(#29357,
#29358),(#29359,#29360),(#29361,#29362),(#29363,#29364),(#29365,#29366),
(#29367,#29368),(#29369,#29370),(#29371,#29372),(#29373,#29374),(#29375,
#29376),(#29377,#29378),(#29379,#29380),(#29381,#29382),(#29383,#29384),
(#29385,#29386),(#29387,#29388),(#29389,#29390),(#29391,#29392),(#29393,
#29394),(#29395,#29396),(#29397,#29398),(#29399,#29400),(#29401,#29402),
(#29403,#29404),(#29405,#29406),(#29407,#29408),(#29409,#29410),(#29411,
#29412),(#29413,#29414),(#29415,#29416),(#29417,#29418),(#29419,#29420),
(#29421,#29422),(#29423,#29424),(#29425,#29426),(#29427,#29428),(#29429,
#29430),(#29431,#29432),(#29433,#29434),(#29435,#29436),(#29437,#29438),
(#29439,#29440),(#29441,#29442),(#29443,#29444),(#29445,#29446),(#29447,
#29448),(#29449,#29450),(#29451,#29452),(#29453,#29454),(#29455,#29456),
(#29457,#29458),(#29459,#29460),(#29461,#29462),(#29463,#29464),(#29465,
#29466),(#29467,#29468),(#29469,#29470),(#29471,#29472),(#29473,#29474),
(#29475,#29476),(#29477,#29478),(#29479,#29480),(#29481,#29482),(#29483,
#29484),(#29485,#29486),(#29487,#29488),(#29489,#29490),(#29491,#29492),
(#29493,#29494),(#29495,#29496),(#29497,#29498),(#29499,#29500),(#29501,
#29502),(#29503,#29504),(#29505,#29506),(#29507,#29508),(#29509,#29510),
(#29511,#29512),(#29513,#29514),(#29515,#29516),(#29517,#29518),(#29519,
#29520),(#29521,#29522),(#29523,#29524),(#29525,#29526),(#29527,#29528),
(#29529,#29530),(#29531,#29532),(#29533,#29534),(#29535,#29536),(#29537,
#29538),(#29539,#29540),(#29541,#29542),(#29543,#29544),(#29545,#29546),
(#29547,#29548),(#29549,#29550),(#29551,#29552),(#29553,#29554),(#29555,
#29556),(#29557,#29558),(#29559,#29560),(#29561,#29562),(#29563,#29564),
(#29565,#29566),(#29567,#29568),(#29569,#29570),(#29571,#29572),(#29573,
#29574),(#29575,#29576),(#29577,#29578),(#29579,#29580),(#29581,#29582),
(#29583,#29584),(#29585,#29586),(#29587,#29588),(#29589,#29590),(#29591,
#29592),(#29593,#29594),(#29595,#29596),(#29597,#29598),(#29599,#29600),
(#29601,#29602),(#29603,#29604),(#29605,#29606),(#29607,#29608),(#29609,
#29610),(#29611,#29612),(#29613,#29614),(#29615,#29616),(#29617,#29618),
(#29619,#29620),(#29621,#29622),(#29623,#29624),(#29625,#29626),(#29627,
#29628),(#29629,#29630),(#29631,#29632),(#29633,#29634),(#29635,#29636),
(#29637,#29638),(#29639,#29640),(#29641,#29642),(#29643,#29644),(#29645,
#29646),(#29647,#29648),(#29649,#29650),(#29651,#29652),(#29653,#29654),
(#29655,#29656),(#29657,#29658),(#29659,#29660),(#29661,#29662),(#29663,
#29664),(#29665,#29666),(#29667,#29668),(#29669,#29670),(#29671,#29672),
(#29673,#29674),(#29675,#29676),(#29677,#29678),(#29679,#29680),(#29681,
#29682),(#29683,#29684),(#29685,#29686),(#29687,#29688),(#29689,#29690),
(#29691,#29692),(#29693,#29694),(#29695,#29696),(#29697,#29698),(#29699,
#29700),(#29701,#29702),(#29703,#29704),(#29705,#29706),(#29707,#29708),
(#29709,#29710),(#29711,#29712),(#29713,#29714),(#29715,#29716),(#29717,
#29718),(#29719,#29720),(#29721,#29722),(#29723,#29724),(#29725,#29726),
(#29727,#29728),(#29729,#29730),(#29731,#29732),(#29733,#29734),(#29735,
#29736),(#29737,#29738),(#29739,#29740),(#29741,#29742),(#29743,#29744),
(#29745,#29746),(#29747,#29748),(#29749,#29750),(#29751,#29752),(#29753,
#29754),(#29755,#29756),(#29757,#29758),(#29759,#29760),(#29761,#29762),
(#29763,#29764),(#29765,#29766),(#29767,#29768),(#29769,#29770),(#29771,
#29772),(#29773,#29774),(#29775,#29776),(#29777,#29778),(#29779,#29780),
(#29781,#29782),(#29783,#29784),(#29785,#29786),(#29787,#29788),(#29789,
#29790),(#29791,#29792),(#29793,#29794),(#29795,#29796),(#29797,#29798),
(#29799,#29800),(#29801,#29802),(#29803,#29804),(#29805,#29806),(#29807,
#29808),(#29809,#29810),(#29811,#29812),(#29813,#29814),(#29815,#29816),
(#29817,#29818),(#29819,#29820),(#29821,#29822),(#29823,#29824),(#29825,
#29826),(#29827,#29828),(#29829,#29830),(#29831,#29832),(#29833,#29834),
(#29835,#29836),(#29837,#29838),(#29839,#29840),(#29841,#29842),(#29843,
#29844),(#29845,#29846),(#29847,#29848),(#29849,#29850),(#29851,#29852),
(#29853,#29854),(#29855,#29856),(#29857,#29858),(#29859,#29860),(#29861,
#29862),(#29863,#29864),(#29865,#29866),(#29867,#29868),(#29869,#29870),
(#29871,#29872),(#29873,#29874),(#29875,#29876),(#29877,#29878),(#29879,
#29880),(#29881,#29882),(#29883,#29884),(#29885,#29886),(#29887,#29888),
(#29889,#29890),(#29891,#29892),(#29893,#29894),(#29895,#29896),(#29897,
#29898),(#29899,#29900),(#29901,#29902),(#29903,#29904),(#29905,#29906),
(#29907,#29908),(#29909,#29910),(#29911,#29912),(#29913,#29914),(#29915,
#29916),(#29917,#29918),(#29919,#29920),(#29921,#29922),(#29923,#29924),
(#29925,#29926),(#29927,#29928),(#29929,#29930),(#29931,#29932),(#29933,
#29934),(#29935,#29936),(#29937,#29938),(#29939,#29940),(#29941,#29942),
(#29943,#29944),(#29945,#29946),(#29947,#29948),(#29949,#29950),(#29951,
#29952),(#29953,#29954),(#29955,#29956),(#29957,#29958),(#29959,#29960),
(#29961,#29962),(#29963,#29964),(#29965,#29966),(#29967,#29968),(#29969,
#29970),(#29971,#29972),(#29973,#29974),(#29975,#29976),(#29977,#29978),
(#29979,#29980),(#29981,#29982),(#29983,#29984),(#29985,#29986),(#29987,
#29988),(#29989,#29990),(#29991,#29992),(#29993,#29994),(#29995,#29996),
(#29997,#29998),(#29999,#30000),(#30001,#30002),(#30003,#30004),(#30005,
#30006),(#30007,#30008),(#30009,#30010),(#30011,#30012),(#30013,#30014),
(#30015,#30016),(#30017,#30018),(#30019,#30020),(#30021,#30022),(#30023,
#30024),(#30025,#30026),(#30027,#30028),(#30029,#30030),(#30031,#30032),
(#30033,#30034),(#30035,#30036),(#30037,#30038),(#30039,#30040),(#30041,
#30042),(#30043,#30044),(#30045,#30046),(#30047,#30048),(#30049,#30050),
(#30051,#30052),(#30053,#30054),(#30055,#30056),(#30057,#30058),(#30059,
#30060),(#30061,#30062),(#30063,#30064),(#30065,#30066),(#30067,#30068),
(#30069,#30070),(#30071,#30072),(#30073,#30074),(#30075,#30076),(#30077,
#30078),(#30079,#30080),(#30081,#30082),(#30083,#30084),(#30085,#30086),
(#30087,#30088),(#30089,#30090),(#30091,#30092),(#30093,#30094),(#30095,
#30096),(#30097,#30098),(#30099,#30100),(#30101,#30102),(#30103,#30104),
(#30105,#30106),(#30107,#30108),(#30109,#30110),(#30111,#30112),(#30113,
#30114),(#30115,#30116),(#30117,#30118),(#30119,#30120),(#30121,#30122),
(#30123,#30124),(#30125,#30126),(#30127,#30128),(#30129,#30130),(#30131,
#30132),(#30133,#30134),(#30135,#30136),(#30137,#30138),(#30139,#30140),
(#30141,#30142),(#30143,#30144),(#30145,#30146),(#30147,#30148),(#30149,
#30150),(#30151,#30152),(#30153,#30154),(#30155,#30156),(#30157,#30158),
(#30159,#30160),(#30161,#30162),(#30163,#30164),(#30165,#30166),(#30167,
#30168),(#30169,#30170),(#30171,#30172),(#30173,#30174),(#30175,#30176),
(#30177,#30178),(#30179,#30180),(#30181,#30182),(#30183,#30184),(#30185,
#30186),(#30187,#30188),(#30189,#30190),(#30191,#30192),(#30193,#30194),
(#30195,#30196),(#30197,#30198),(#30199,#30200),(#30201,#30202),(#30203,
#30204),(#30205,#30206),(#30207,#30208),(#30209,#30210),(#30211,#30212),
(#30213,#30214),(#30215,#30216),(#30217,#30218),(#30219,#30220),(#30221,
#30222),(#30223,#30224),(#30225,#30226),(#30227,#30228),(#30229,#30230),
(#30231,#30232),(#30233,#30234),(#30235,#30236),(#30237,#30238),(#30239,
#30240),(#30241,#30242),(#30243,#30244),(#30245,#30246),(#30247,#30248),
(#30249,#30250),(#30251,#30252),(#30253,#30254),(#30255,#30256),(#30257,
#30258),(#30259,#30260),(#30261,#30262),(#30263,#30264),(#30265,#30266),
(#30267,#30268),(#30269,#30270),(#30271,#30272),(#30273,#30274),(#30275,
#30276),(#30277,#30278),(#30279,#30280),(#30281,#30282),(#30283,#30284),
(#30285,#30286),(#30287,#30288),(#30289,#30290),(#30291,#30292),(#30293,
#30294),(#30295,#30296),(#30297,#30298),(#30299,#30300),(#30301,#30302),
(#30303,#30304),(#30305,#30306),(#30307,#30308),(#30309,#30310),(#30311,
#30312),(#30313,#30314),(#30315,#30316),(#30317,#30318),(#30319,#30320),
(#30321,#30322),(#30323,#30324),(#30325,#30326),(#30327,#30328),(#30329,
#30330),(#30331,#30332),(#30333,#30334),(#30335,#30336),(#30337,#30338),
(#30339,#30340),(#30341,#30342),(#30343,#30344),(#30345,#30346),(#30347,
#30348),(#30349,#30350),(#30351,#30352),(#30353,#30354),(#30355,#30356),
(#30357,#30358),(#30359,#30360),(#30361,#30362),(#30363,#30364),(#30365,
#30366),(#30367,#30368),(#30369,#30370),(#30371,#30372),(#30373,#30374),
(#30375,#30376),(#30377,#30378),(#30379,#30380),(#30381,#30382),(#30383,
#30384),(#30385,#30386),(#30387,#30388),(#30389,#30390),(#30391,#30392),
(#30393,#30394),(#30395,#30396),(#30397,#30398),(#30399,#30400),(#30401,
#30402),(#30403,#30404),(#30405,#30406),(#30407,#30408),(#30409,#30410),
(#30411,#30412),(#30413,#30414),(#30415,#30416),(#30417,#30418),(#30419,
#30420),(#30421,#30422),(#30423,#30424),(#30425,#30426),(#30427,#30428),
(#30429,#30430),(#30431,#30432),(#30433,#30434),(#30435,#30436),(#30437,
#30438),(#30439,#30440),(#30441,#30442),(#30443,#30444),(#30445,#30446),
(#30447,#30448),(#30449,#30450),(#30451,#30452),(#30453,#30454),(#30455,
#30456),(#30457,#30458),(#30459,#30460),(#30461,#30462),(#30463,#30464),
(#30465,#30466),(#30467,#30468),(#30469,#30470),(#30471,#30472),(#30473,
#30474),(#30475,#30476),(#30477,#30478),(#30479,#30480),(#30481,#30482),
(#30483,#30484),(#30485,#30486),(#30487,#30488),(#30489,#30490),(#30491,
#30492),(#30493,#30494),(#30495,#30496),(#30497,#30498),(#30499,#30500),
(#30501,#30502),(#30503,#30504),(#30505,#30506),(#30507,#30508),(#30509,
#30510),(#30511,#30512),(#30513,#30514),(#30515,#30516),(#30517,#30518),
(#30519,#30520),(#30521,#30522),(#30523,#30524),(#30525,#30526),(#30527,
#30528),(#30529,#30530),(#30531,#30532),(#30533,#30534),(#30535,#30536),
(#30537,#30538),(#30539,#30540),(#30541,#30542),(#30543,#30544),(#30545,
#30546),(#30547,#30548),(#30549,#30550),(#30551,#30552),(#30553,#30554),
(#30555,#30556),(#30557,#30558),(#30559,#30560),(#30561,#30562),(#30563,
#30564),(#30565,#30566),(#30567,#30568),(#30569,#30570),(#30571,#30572),
(#30573,#30574),(#30575,#30576),(#30577,#30578),(#30579,#30580),(#30581,
#30582),(#30583,#30584),(#30585,#30586),(#30587,#30588),(#30589,#30590),
(#30591,#30592),(#30593,#30594),(#30595,#30596),(#30597,#30598),(#30599,
#30600),(#30601,#30602),(#30603,#30604),(#30605,#30606),(#30607,#30608),
(#30609,#30610),(#30611,#30612),(#30613,#30614),(#30615,#30616),(#30617,
#30618),(#30619,#30620),(#30621,#30622),(#30623,#30624),(#30625,#30626),
(#30627,#30628),(#30629,#30630),(#30631,#30632),(#30633,#30634),(#30635,
#30636),(#30637,#30638),(#30639,#30640),(#30641,#30642),(#30643,#30644),
(#30645,#30646),(#30647,#30648),(#30649,#30650),(#30651,#30652),(#30653,
#30654),(#30655,#30656),(#30657,#30658),(#30659,#30660),(#30661,#30662),
(#30663,#30664),(#30665,#30666),(#30667,#30668),(#30669,#30670),(#30671,
#30672),(#30673,#30674),(#30675,#30676),(#30677,#30678),(#30679,#30680),
(#30681,#30682),(#30683,#30684),(#30685,#30686),(#30687,#30688),(#30689,
#30690),(#30691,#30692),(#30693,#30694),(#30695,#30696),(#30697,#30698),
(#30699,#30700),(#30701,#30702),(#30703,#30704),(#30705,#30706),(#30707,
#30708),(#30709,#30710),(#30711,#30712),(#30713,#30714),(#30715,#30716),
(#30717,#30718),(#30719,#30720),(#30721,#30722),(#30723,#30724),(#30725,
#30726),(#30727,#30728),(#30729,#30730),(#30731,#30732),(#30733,#30734),
(#30735,#30736),(#30737,#30738),(#30739,#30740),(#30741,#30742),(#30743,
#30744),(#30745,#30746),(#30747,#30748),(#30749,#30750),(#30751,#30752),
(#30753,#30754),(#30755,#30756),(#30757,#30758),(#30759,#30760),(#30761,
#30762),(#30763,#30764),(#30765,#30766),(#30767,#30768),(#30769,#30770),
(#30771,#30772),(#30773,#30774),(#30775,#30776),(#30777,#30778),(#30779,
#30780),(#30781,#30782),(#30783,#30784),(#30785,#30786),(#30787,#30788),
(#30789,#30790),(#30791,#30792),(#30793,#30794),(#30795,#30796),(#30797,
#30798),(#30799,#30800),(#30801,#30802),(#30803,#30804),(#30805,#30806),
(#30807,#30808),(#30809,#30810),(#30811,#30812),(#30813,#30814),(#30815,
#30816),(#30817,#30818),(#30819,#30820),(#30821,#30822),(#30823,#30824),
(#30825,#30826),(#30827,#30828),(#30829,#30830),(#30831,#30832),(#30833,
#30834),(#30835,#30836),(#30837,#30838),(#30839,#30840),(#30841,#30842),
(#30843,#30844),(#30845,#30846),(#30847,#30848),(#30849,#30850),(#30851,
#30852),(#30853,#30854),(#30855,#30856),(#30857,#30858),(#30859,#30860),
(#30861,#30862),(#30863,#30864),(#30865,#30866),(#30867,#30868),(#30869,
#30870),(#30871,#30872),(#30873,#30874),(#30875,#30876),(#30877,#30878),
(#30879,#30880),(#30881,#30882),(#30883,#30884),(#30885,#30886),(#30887,
#30888),(#30889,#30890),(#30891,#30892),(#30893,#30894),(#30895,#30896),
(#30897,#30898),(#30899,#30900),(#30901,#30902),(#30903,#30904),(#30905,
#30906),(#30907,#30908),(#30909,#30910),(#30911,#30912),(#30913,#30914),
(#30915,#30916),(#30917,#30918),(#30919,#30920),(#30921,#30922),(#30923,
#30924),(#30925,#30926),(#30927,#30928),(#30929,#30930),(#30931,#30932),
(#30933,#30934),(#30935,#30936),(#30937,#30938),(#30939,#30940),(#30941,
#30942),(#30943,#30944),(#30945,#30946),(#30947,#30948),(#30949,#30950),
(#30951,#30952),(#30953,#30954),(#30955,#30956),(#30957,#30958),(#30959,
#30960),(#30961,#30962),(#30963,#30964),(#30965,#30966),(#30967,#30968),
(#30969,#30970),(#30971,#30972),(#30973,#30974),(#30975,#30976),(#30977,
#30978),(#30979,#30980),(#30981,#30982),(#30983,#30984),(#30985,#30986),
(#30987,#30988),(#30989,#30990),(#30991,#30992),(#30993,#30994),(#30995,
#30996),(#30997,#30998),(#30999,#31000),(#31001,#31002),(#31003,#31004),
(#31005,#31006),(#31007,#31008),(#31009,#31010),(#31011,#31012),(#31013,
#31014),(#31015,#31016),(#31017,#31018),(#31019,#31020),(#31021,#31022),
(#31023,#31024),(#31025,#31026),(#31027,#31028),(#31029,#31030),(#31031,
#31032),(#31033,#31034),(#31035,#31036),(#31037,#31038),(#31039,#31040),
(#31041,#31042),(#31043,#31044),(#31045,#31046),(#31047,#31048),(#31049,
#31050),(#31051,#31052),(#31053,#31054),(#31055,#31056),(#31057,#31058),
(#31059,#31060),(#31061,#31062),(#31063,#31064),(#31065,#31066),(#31067,
#31068),(#31069,#31070),(#31071,#31072),(#31073,#31074),(#31075,#31076),
(#31077,#31078),(#31079,#31080),(#31081,#31082),(#31083,#31084),(#31085,
#31086),(#31087,#31088),(#31089,#31090),(#31091,#31092),(#31093,#31094),
(#31095,#31096),(#31097,#31098),(#31099,#31100),(#31101,#31102),(#31103,
#31104),(#31105,#31106),(#31107,#31108),(#31109,#31110),(#31111,#31112),
(#31113,#31114),(#31115,#31116),(#31117,#31118),(#31119,#31120),(#31121,
#31122),(#31123,#31124),(#31125,#31126),(#31127,#31128),(#31129,#31130),
(#31131,#31132),(#31133,#31134),(#31135,#31136),(#31137,#31138),(#31139,
#31140),(#31141,#31142),(#31143,#31144),(#31145,#31146),(#31147,#31148),
(#31149,#31150),(#31151,#31152),(#31153,#31154),(#31155,#31156),(#31157,
#31158),(#31159,#31160),(#31161,#31162),(#31163,#31164),(#31165,#31166),
(#31167,#31168),(#31169,#31170),(#31171,#31172),(#31173,#31174),(#31175,
#31176),(#31177,#31178),(#31179,#31180),(#31181,#31182),(#31183,#31184),
(#31185,#31186),(#31187,#31188),(#31189,#31190),(#31191,#31192),(#31193,
#31194),(#31195,#31196),(#31197,#31198),(#31199,#31200),(#31201,#31202),
(#31203,#31204),(#31205,#31206),(#31207,#31208),(#31209,#31210),(#31211,
#31212),(#31213,#31214),(#31215,#31216),(#31217,#31218),(#31219,#31220),
(#31221,#31222),(#31223,#31224),(#31225,#31226),(#31227,#31228),(#31229,
#31230),(#31231,#31232),(#31233,#31234),(#31235,#31236),(#31237,#31238),
(#31239,#31240),(#31241,#31242),(#31243,#31244),(#31245,#31246),(#31247,
#31248),(#31249,#31250),(#31251,#31252),(#31253,#31254),(#31255,#31256),
(#31257,#31258),(#31259,#31260),(#31261,#31262),(#31263,#31264),(#31265,
#31266),(#31267,#31268),(#31269,#31270),(#31271,#31272),(#31273,#31274),
(#31275,#31276),(#31277,#31278),(#31279,#31280),(#31281,#31282),(#31283,
#31284),(#31285,#31286),(#31287,#31288),(#31289,#31290),(#31291,#31292),
(#31293,#31294),(#31295,#31296),(#31297,#31298),(#31299,#31300),(#31301,
#31302),(#31303,#31304),(#31305,#31306),(#31307,#31308),(#31309,#31310),
(#31311,#31312),(#31313,#31314),(#31315,#31316),(#31317,#31318),(#31319,
#31320),(#31321,#31322),(#31323,#31324),(#31325,#31326),(#31327,#31328),
(#31329,#31330),(#31331,#31332),(#31333,#31334),(#31335,#31336),(#31337,
#31338),(#31339,#31340),(#31341,#31342),(#31343,#31344),(#31345,#31346),
(#31347,#31348),(#31349,#31350),(#31351,#31352),(#31353,#31354),(#31355,
#31356),(#31357,#31358),(#31359,#31360),(#31361,#31362),(#31363,#31364),
(#31365,#31366),(#31367,#31368),(#31369,#31370),(#31371,#31372),(#31373,
#31374),(#31375,#31376),(#31377,#31378),(#31379,#31380),(#31381,#31382),
(#31383,#31384),(#31385,#31386),(#31387,#31388),(#31389,#31390),(#31391,
#31392),(#31393,#31394),(#31395,#31396),(#31397,#31398),(#31399,#31400),
(#31401,#31402),(#31403,#31404),(#31405,#31406),(#31407,#31408),(#31409,
#31410),(#31411,#31412),(#31413,#31414),(#31415,#31416),(#31417,#31418),
(#31419,#31420),(#31421,#31422),(#31423,#31424),(#31425,#31426),(#31427,
#31428),(#31429,#31430),(#31431,#31432),(#31433,#31434),(#31435,#31436),
(#31437,#31438),(#31439,#31440),(#31441,#31442),(#31443,#31444),(#31445,
#31446),(#31447,#31448),(#31449,#31450),(#31451,#31452),(#31453,#31454),
(#31455,#31456),(#31457,#31458),(#31459,#31460),(#31461,#31462),(#31463,
#31464),(#31465,#31466),(#31467,#31468),(#31469,#31470),(#31471,#31472),
(#31473,#31474),(#31475,#31476),(#31477,#31478),(#31479,#31480),(#31481,
#31482),(#31483,#31484),(#31485,#31486),(#31487,#31488),(#31489,#31490),
(#31491,#31492),(#31493,#31494),(#31495,#31496),(#31497,#31498),(#31499,
#31500),(#31501,#31502),(#31503,#31504),(#31505,#31506),(#31507,#31508),
(#31509,#31510),(#31511,#31512),(#31513,#31514),(#31515,#31516),(#31517,
#31518),(#31519,#31520),(#31521,#31522),(#31523,#31524),(#31525,#31526),
(#31527,#31528),(#31529,#31530),(#31531,#31532),(#31533,#31534),(#31535,
#31536),(#31537,#31538),(#31539,#31540),(#31541,#31542),(#31543,#31544),
(#31545,#31546),(#31547,#31548),(#31549,#31550),(#31551,#31552),(#31553,
#31554),(#31555,#31556),(#31557,#31558),(#31559,#31560),(#31561,#31562),
(#31563,#31564),(#31565,#31566),(#31567,#31568),(#31569,#31570),(#31571,
#31572),(#31573,#31574),(#31575,#31576),(#31577,#31578),(#31579,#31580),
(#31581,#31582),(#31583,#31584),(#31585,#31586),(#31587,#31588),(#31589,
#31590),(#31591,#31592),(#31593,#31594),(#31595,#31596),(#31597,#31598),
(#31599,#31600),(#31601,#31602),(#31603,#31604),(#31605,#31606),(#31607,
#31608),(#31609,#31610),(#31611,#31612),(#31613,#31614),(#31615,#31616),
(#31617,#31618),(#31619,#31620),(#31621,#31622),(#31623,#31624),(#31625,
#31626),(#31627,#31628),(#31629,#31630),(#31631,#31632),(#31633,#31634),
(#31635,#31636),(#31637,#31638),(#31639,#31640),(#31641,#31642),(#31643,
#31644),(#31645,#31646),(#31647,#31648),(#31649,#31650),(#31651,#31652),
(#31653,#31654),(#31655,#31656),(#31657,#31658),(#31659,#31660),(#31661,
#31662),(#31663,#31664),(#31665,#31666),(#31667,#31668),(#31669,#31670),
(#31671,#31672),(#31673,#31674),(#31675,#31676),(#31677,#31678),(#31679,
#31680),(#31681,#31682),(#31683,#31684),(#31685,#31686),(#31687,#31688),
(#31689,#31690),(#31691,#31692),(#31693,#31694),(#31695,#31696),(#31697,
#31698),(#31699,#31700),(#31701,#31702),(#31703,#31704),(#31705,#31706),
(#31707,#31708),(#31709,#31710),(#31711,#31712),(#31713,#31714),(#31715,
#31716),(#31717,#31718),(#31719,#31720),(#31721,#31722),(#31723,#31724),
(#31725,#31726),(#31727,#31728),(#31729,#31730),(#31731,#31732),(#31733,
#31734),(#31735,#31736),(#31737,#31738),(#31739,#31740),(#31741,#31742),
(#31743,#31744),(#31745,#31746),(#31747,#31748),(#31749,#31750),(#31751,
#31752),(#31753,#31754),(#31755,#31756),(#31757,#31758),(#31759,#31760),
(#31761,#31762),(#31763,#31764),(#31765,#31766),(#31767,#31768),(#31769,
#31770),(#31771,#31772),(#31773,#31774),(#31775,#31776),(#31777,#31778),
(#31779,#31780),(#31781,#31782),(#31783,#31784),(#31785,#31786),(#31787,
#31788),(#31789,#31790),(#31791,#31792),(#31793,#31794),(#31795,#31796),
(#31797,#31798),(#31799,#31800),(#31801,#31802),(#31803,#31804),(#31805,
#31806),(#31807,#31808),(#31809,#31810),(#31811,#31812),(#31813,#31814),
(#31815,#31816),(#31817,#31818),(#31819,#31820),(#31821,#31822),(#31823,
#31824),(#31825,#31826),(#31827,#31828),(#31829,#31830),(#31831,#31832),
(#31833,#31834),(#31835,#31836),(#31837,#31838),(#31839,#31840),(#31841,
#31842),(#31843,#31844),(#31845,#31846),(#31847,#31848),(#31849,#31850),
(#31851,#31852),(#31853,#31854),(#31855,#31856),(#31857,#31858),(#31859,
#31860),(#31861,#31862),(#31863,#31864),(#31865,#31866),(#31867,#31868),
(#31869,#31870),(#31871,#31872),(#31873,#31874),(#31875,#31876),(#31877,
#31878),(#31879,#31880),(#31881,#31882),(#31883,#31884),(#31885,#31886),
(#31887,#31888),(#31889,#31890),(#31891,#31892),(#31893,#31894),(#31895,
#31896),(#31897,#31898),(#31899,#31900),(#31901,#31902),(#31903,#31904),
(#31905,#31906),(#31907,#31908),(#31909,#31910),(#31911,#31912),(#31913,
#31914),(#31915,#31916),(#31917,#31918),(#31919,#31920),(#31921,#31922),
(#31923,#31924),(#31925,#31926),(#31927,#31928),(#31929,#31930),(#31931,
#31932),(#31933,#31934),(#31935,#31936),(#31937,#31938),(#31939,#31940),
(#31941,#31942),(#31943,#31944),(#31945,#31946),(#31947,#31948),(#31949,
#31950),(#31951,#31952),(#31953,#31954),(#31955,#31956),(#31957,#31958),
(#31959,#31960),(#31961,#31962),(#31963,#31964),(#31965,#31966),(#31967,
#31968),(#31969,#31970),(#31971,#31972),(#31973,#31974),(#31975,#31976),
(#31977,#31978),(#31979,#31980),(#31981,#31982),(#31983,#31984),(#31985,
#31986),(#31987,#31988),(#31989,#31990),(#31991,#31992),(#31993,#31994),
(#31995,#31996),(#31997,#31998),(#31999,#32000),(#32001,#32002),(#32003,
#32004),(#32005,#32006),(#32007,#32008),(#32009,#32010),(#32011,#32012),
(#32013,#32014),(#32015,#32016),(#32017,#32018),(#32019,#32020),(#32021,
#32022),(#32023,#32024),(#32025,#32026),(#32027,#32028),(#32029,#32030),
(#32031,#32032),(#32033,#32034),(#32035,#32036),(#32037,#32038),(#32039,
#32040),(#32041,#32042),(#32043,#32044),(#32045,#32046),(#32047,#32048),
(#32049,#32050),(#32051,#32052),(#32053,#32054),(#32055,#32056),(#32057,
#32058),(#32059,#32060),(#32061,#32062),(#32063,#32064),(#32065,#32066),
(#32067,#32068),(#32069,#32070),(#32071,#32072),(#32073,#32074),(#32075,
#32076),(#32077,#32078),(#32079,#32080),(#32081,#32082),(#32083,#32084),
(#32085,#32086),(#32087,#32088),(#32089,#32090),(#32091,#32092),(#32093,
#32094),(#32095,#32096),(#32097,#32098),(#32099,#32100),(#32101,#32102),
(#32103,#32104),(#32105,#32106),(#32107,#32108),(#32109,#32110),(#32111,
#32112),(#32113,#32114),(#32115,#32116),(#32117,#32118),(#32119,#32120),
(#32121,#32122),(#32123,#32124),(#32125,#32126),(#32127,#32128),(#32129,
#32130),(#32131,#32132),(#32133,#32134),(#32135,#32136),(#32137,#32138),
(#32139,#32140),(#32141,#32142),(#32143,#32144),(#32145,#32146),(#32147,
#32148),(#32149,#32150),(#32151,#32152),(#32153,#32154),(#32155,#32156),
(#32157,#32158),(#32159,#32160),(#32161,#32162),(#32163,#32164),(#32165,
#32166),(#32167,#32168),(#32169,#32170),(#32171,#32172),(#32173,#32174),
(#32175,#32176),(#32177,#32178),(#32179,#32180),(#32181,#32182),(#32183,
#32184),(#32185,#32186),(#32187,#32188),(#32189,#32190),(#32191,#32192),
(#32193,#32194),(#32195,#32196),(#32197,#32198),(#32199,#32200),(#32201,
#32202),(#32203,#32204),(#32205,#32206),(#32207,#32208),(#32209,#32210),
(#32211,#32212),(#32213,#32214),(#32215,#32216),(#32217,#32218),(#32219,
#32220),(#32221,#32222),(#32223,#32224),(#32225,#32226),(#32227,#32228),
(#32229,#32230),(#32231,#32232),(#32233,#32234),(#32235,#32236),(#32237,
#32238),(#32239,#32240),(#32241,#32242),(#32243,#32244),(#32245,#32246),
(#32247,#32248),(#32249,#32250),(#32251,#32252),(#32253,#32254),(#32255,
#32256),(#32257,#32258),(#32259,#32260),(#32261,#32262),(#32263,#32264),
(#32265,#32266),(#32267,#32268),(#32269,#32270),(#32271,#32272),(#32273,
#32274),(#32275,#32276),(#32277,#32278),(#32279,#32280),(#32281,#32282),
(#32283,#32284),(#32285,#32286),(#32287,#32288),(#32289,#32290),(#32291,
#32292),(#32293,#32294),(#32295,#32296),(#32297,#32298),(#32299,#32300),
(#32301,#32302),(#32303,#32304),(#32305,#32306),(#32307,#32308),(#32309,
#32310),(#32311,#32312),(#32313,#32314),(#32315,#32316),(#32317,#32318),
(#32319,#32320),(#32321,#32322),(#32323,#32324),(#32325,#32326),(#32327,
#32328),(#32329,#32330),(#32331,#32332),(#32333,#32334),(#32335,#32336),
(#32337,#32338),(#32339,#32340),(#32341,#32342),(#32343,#32344),(#32345,
#32346),(#32347,#32348),(#32349,#32350),(#32351,#32352),(#32353,#32354),
(#32355,#32356),(#32357,#32358),(#32359,#32360),(#32361,#32362),(#32363,
#32364),(#32365,#32366),(#32367,#32368),(#32369,#32370),(#32371,#32372),
(#32373,#32374),(#32375,#32376),(#32377,#32378),(#32379,#32380),(#32381,
#32382),(#32383,#32384),(#32385,#32386),(#32387,#32388),(#32389,#32390),
(#32391,#32392),(#32393,#32394),(#32395,#32396),(#32397,#32398),(#32399,
#32400),(#32401,#32402),(#32403,#32404),(#32405,#32406),(#32407,#32408),
(#32409,#32410),(#32411,#32412),(#32413,#32414),(#32415,#32416),(#32417,
#32418),(#32419,#32420),(#32421,#32422),(#32423,#32424),(#32425,#32426),
(#32427,#32428),(#32429,#32430),(#32431,#32432),(#32433,#32434),(#32435,
#32436),(#32437,#32438),(#32439,#32440),(#32441,#32442),(#32443,#32444),
(#32445,#32446),(#32447,#32448),(#32449,#32450),(#32451,#32452),(#32453,
#32454),(#32455,#32456),(#32457,#32458),(#32459,#32460),(#32461,#32462),
(#32463,#32464),(#32465,#32466),(#32467,#32468),(#32469,#32470),(#32471,
#32472),(#32473,#32474),(#32475,#32476),(#32477,#32478),(#32479,#32480),
(#32481,#32482),(#32483,#32484),(#32485,#32486),(#32487,#32488),(#32489,
#32490),(#32491,#32492),(#32493,#32494),(#32495,#32496),(#32497,#32498),
(#32499,#32500),(#32501,#32502),(#32503,#32504),(#32505,#32506),(#32507,
#32508),(#32509,#32510),(#32511,#32512),(#32513,#32514),(#32515,#32516),
(#32517,#32518),(#32519,#32520),(#32521,#32522),(#32523,#32524),(#32525,
#32526),(#32527,#32528),(#32529,#32530),(#32531,#32532),(#32533,#32534),
(#32535,#32536),(#32537,#32538),(#32539,#32540),(#32541,#32542),(#32543,
#32544),(#32545,#32546),(#32547,#32548),(#32549,#32550),(#32551,#32552),
(#32553,#32554),(#32555,#32556),(#32557,#32558),(#32559,#32560),(#32561,
#32562),(#32563,#32564),(#32565,#32566),(#32567,#32568),(#32569,#32570),
(#32571,#32572),(#32573,#32574),(#32575,#32576),(#32577,#32578),(#32579,
#32580),(#32581,#32582),(#32583,#32584),(#32585,#32586),(#32587,#32588),
(#32589,#32590),(#32591,#32592),(#32593,#32594),(#32595,#32596),(#32597,
#32598),(#32599,#32600),(#32601,#32602),(#32603,#32604),(#32605,#32606),
(#32607,#32608),(#32609,#32610),(#32611,#32612),(#32613,#32614),(#32615,
#32616),(#32617,#32618),(#32619,#32620),(#32621,#32622),(#32623,#32624),
(#32625,#32626),(#32627,#32628),(#32629,#32630),(#32631,#32632),(#32633,
#32634),(#32635,#32636),(#32637,#32638),(#32639,#32640),(#32641,#32642),
(#32643,#32644),(#32645,#32646),(#32647,#32648),(#32649,#32650),(#32651,
#32652),(#32653,#32654),(#32655,#32656),(#32657,#32658),(#32659,#32660),
(#32661,#32662),(#32663,#32664),(#32665,#32666),(#32667,#32668),(#32669,
#32670),(#32671,#32672),(#32673,#32674),(#32675,#32676),(#32677,#32678),
(#32679,#32680),(#32681,#32682),(#32683,#32684),(#32685,#32686),(#32687,
#32688),(#32689,#32690),(#32691,#32692),(#32693,#32694),(#32695,#32696),
(#32697,#32698),(#32699,#32700),(#32701,#32702),(#32703,#32704),(#32705,
#32706),(#32707,#32708),(#32709,#32710),(#32711,#32712),(#32713,#32714),
(#32715,#32716),(#32717,#32718),(#32719,#32720),(#32721,#32722),(#32723,
#32724),(#32725,#32726),(#32727,#32728),(#32729,#32730),(#32731,#32732),
(#32733,#32734),(#32735,#32736),(#32737,#32738),(#32739,#32740),(#32741,
#32742),(#32743,#32744),(#32745,#32746),(#32747,#32748),(#32749,#32750),
(#32751,#32752),(#32753,#32754),(#32755,#32756),(#32757,#32758),(#32759,
#32760),(#32761,#32762),(#32763,#32764),(#32765,#32766),(#32767,#32768),
(#32769,#32770),(#32771,#32772),(#32773,#32774),(#32775,#32776),(#32777,
#32778),(#32779,#32780),(#32781,#32782),(#32783,#32784),(#32785,#32786),
(#32787,#32788),(#32789,#32790),(#32791,#32792),(#32793,#32794),(#32795,
#32796),(#32797,#32798),(#32799,#32800),(#32801,#32802),(#32803,#32804),
(#32805,#32806),(#32807,#32808),(#32809,#32810),(#32811,#32812),(#32813,
#32814),(#32815,#32816),(#32817,#32818),(#32819,#32820),(#32821,#32822),
(#32823,#32824),(#32825,#32826),(#32827,#32828),(#32829,#32830),(#32831,
#32832),(#32833,#32834),(#32835,#32836),(#32837,#32838),(#32839,#32840),
(#32841,#32842),(#32843,#32844),(#32845,#32846),(#32847,#32848),(#32849,
#32850),(#32851,#32852),(#32853,#32854),(#32855,#32856),(#32857,#32858),
(#32859,#32860),(#32861,#32862),(#32863,#32864),(#32865,#32866),(#32867,
#32868),(#32869,#32870),(#32871,#32872),(#32873,#32874),(#32875,#32876),
(#32877,#32878),(#32879,#32880),(#32881,#32882),(#32883,#32884),(#32885,
#32886),(#32887,#32888),(#32889,#32890),(#32891,#32892),(#32893,#32894),
(#32895,#32896),(#32897,#32898),(#32899,#32900),(#32901,#32902),(#32903,
#32904),(#32905,#32906),(#32907,#32908),(#32909,#32910),(#32911,#32912),
(#32913,#32914),(#32915,#32916),(#32917,#32918),(#32919,#32920),(#32921,
#32922),(#32923,#32924),(#32925,#32926),(#32927,#32928),(#32929,#32930),
(#32931,#32932),(#32933,#32934),(#32935,#32936),(#32937,#32938),(#32939,
#32940),(#32941,#32942),(#32943,#32944),(#32945,#32946),(#32947,#32948),
(#32949,#32950),(#32951,#32952),(#32953,#32954),(#32955,#32956),(#32957,
#32958),(#32959,#32960),(#32961,#32962),(#32963,#32964),(#32965,#32966),
(#32967,#32968),(#32969,#32970),(#32971,#32972),(#32973,#32974),(#32975,
#32976),(#32977,#32978),(#32979,#32980),(#32981,#32982),(#32983,#32984),
(#32985,#32986),(#32987,#32988),(#32989,#32990),(#32991,#32992),(#32993,
#32994),(#32995,#32996),(#32997,#32998),(#32999,#33000),(#33001,#33002),
(#33003,#33004),(#33005,#33006),(#33007,#33008),(#33009,#33010),(#33011,
#33012),(#33013,#33014),(#33015,#33016),(#33017,#33018),(#33019,#33020),
(#33021,#33022),(#33023,#33024),(#33025,#33026),(#33027,#33028),(#33029,
#33030),(#33031,#33032),(#33033,#33034),(#33035,#33036),(#33037,#33038),
(#33039,#33040),(#33041,#33042),(#33043,#33044),(#33045,#33046),(#33047,
#33048),(#33049,#33050),(#33051,#33052),(#33053,#33054),(#33055,#33056),
(#33057,#33058),(#33059,#33060),(#33061,#33062),(#33063,#33064),(#33065,
#33066),(#33067,#33068),(#33069,#33070),(#33071,#33072),(#33073,#33074),
(#33075,#33076),(#33077,#33078),(#33079,#33080),(#33081,#33082),(#33083,
#33084),(#33085,#33086),(#33087,#33088),(#33089,#33090),(#33091,#33092),
(#33093,#33094),(#33095,#33096),(#33097,#33098),(#33099,#33100),(#33101,
#33102),(#33103,#33104),(#33105,#33106),(#33107,#33108),(#33109,#33110),
(#33111,#33112),(#33113,#33114),(#33115,#33116),(#33117,#33118),(#33119,
#33120),(#33121,#33122),(#33123,#33124),(#33125,#33126),(#33127,#33128),
(#33129,#33130),(#33131,#33132),(#33133,#33134),(#33135,#33136),(#33137,
#33138),(#33139,#33140),(#33141,#33142),(#33143,#33144),(#33145,#33146),
(#33147,#33148),(#33149,#33150),(#33151,#33152),(#33153,#33154),(#33155,
#33156),(#33157,#33158),(#33159,#33160),(#33161,#33162),(#33163,#33164),
(#33165,#33166),(#33167,#33168),(#33169,#33170),(#33171,#33172),(#33173,
#33174),(#33175,#33176),(#33177,#33178),(#33179,#33180),(#33181,#33182),
(#33183,#33184),(#33185,#33186),(#33187,#33188),(#33189,#33190),(#33191,
#33192),(#33193,#33194),(#33195,#33196),(#33197,#33198),(#33199,#33200),
(#33201,#33202),(#33203,#33204),(#33205,#33206),(#33207,#33208),(#33209,
#33210),(#33211,#33212),(#33213,#33214),(#33215,#33216),(#33217,#33218),
(#33219,#33220),(#33221,#33222),(#33223,#33224),(#33225,#33226),(#33227,
#33228),(#33229,#33230),(#33231,#33232),(#33233,#33234),(#33235,#33236)),
 .UNSPECIFIED.,.F.,.F.,.F.,(4,1,1,1,1,1,1,1,1,1,1,1,1,1,1,1,1,1,1,1,1,1,
1,1,1,1,1,1,1,1,1,1,1,1,1,1,1,1,1,1,1,1,1,1,1,1,1,1,1,1,1,1,1,1,1,1,1,1,
1,1,1,1,1,1,1,1,1,1,1,1,1,1,1,1,1,1,1,1,1,1,1,1,1,1,1,1,1,1,1,1,1,1,1,1,
1,1,1,1,1,1,1,1,1,1,1,1,1,1,1,1,1,1,1,1,1,1,1,1,1,1,1,1,1,1,1,1,1,1,1,1,
1,1,1,1,1,1,1,1,1,1,1,1,1,1,1,1,1,1,1,1,1,1,1,1,1,1,1,1,1,1,1,1,1,1,1,1,
1,1,1,1,1,1,1,1,1,1,1,1,1,1,1,1,1,1,1,1,1,1,1,1,1,1,1,1,1,1,1,1,1,1,1,1,
1,1,1,1,1,1,1,1,1,1,1,1,1,1,1,1,1,1,1,1,1,1,1,1,1,1,1,1,1,1,1,1,1,1,1,1,
1,1,1,1,1,1,1,1,1,1,1,1,1,1,1,1,1,1,1,1,1,1,1,1,1,1,1,1,1,1,1,1,1,1,1,1,
1,1,1,1,1,1,1,1,1,1,1,1,1,1,1,1,1,1,1,1,1,1,1,1,1,1,1,1,1,1,1,1,1,1,1,1,
1,1,1,1,1,1,1,1,1,1,1,1,1,1,1,1,1,1,1,1,1,1,1,1,1,1,1,1,1,1,1,1,1,1,1,1,
1,1,1,1,1,1,1,1,1,1,1,1,1,1,1,1,1,1,1,1,1,1,1,1,1,1,1,1,1,1,1,1,1,1,1,1,
1,1,1,1,1,1,1,1,1,1,1,1,1,1,1,1,1,1,1,1,1,1,1,1,1,1,1,1,1,1,1,1,1,1,1,1,
1,1,1,1,1,1,1,1,1,1,1,1,1,1,1,1,1,1,1,1,1,1,1,1,1,1,1,1,1,1,1,1,1,1,1,1,
1,1,1,1,1,1,1,1,1,1,1,1,1,1,1,1,1,1,1,1,1,1,1,1,1,1,1,1,1,1,1,1,1,1,1,1,
1,1,1,1,1,1,1,1,1,1,1,1,1,1,1,1,1,1,1,1,1,1,1,1,1,1,1,1,1,1,1,1,1,1,1,1,
1,1,1,1,1,1,1,1,1,1,1,1,1,1,1,1,1,1,1,1,1,1,1,1,1,1,1,1,1,1,1,1,1,1,1,1,
1,1,1,1,1,1,1,1,1,1,1,1,1,1,1,1,1,1,1,1,1,1,1,1,1,1,1,1,1,1,1,1,1,1,1,1,
1,1,1,1,1,1,1,1,1,1,1,1,1,1,1,1,1,1,1,1,1,1,1,1,1,1,1,1,1,1,1,1,1,1,1,1,
1,1,1,1,1,1,1,1,1,1,1,1,1,1,1,1,1,1,1,1,1,1,1,1,1,1,1,1,1,1,1,1,1,1,1,1,
1,1,1,1,1,1,1,1,1,1,1,1,1,1,1,1,1,1,1,1,1,1,1,1,1,1,1,1,1,1,1,1,1,1,1,1,
1,1,1,1,1,1,1,1,1,1,1,1,1,1,1,1,1,1,1,1,1,1,1,1,1,1,1,1,1,1,1,1,1,1,1,1,
1,1,1,1,1,1,1,1,1,1,1,1,1,1,1,1,1,1,1,1,1,1,1,1,1,1,1,1,1,1,1,1,1,1,1,1,
1,1,1,1,1,1,1,1,1,1,1,1,1,1,1,1,1,1,1,1,1,1,1,1,1,1,1,1,1,1,1,1,1,1,1,1,
1,1,1,1,1,1,1,1,1,1,1,1,1,1,1,1,1,1,1,1,1,1,1,1,1,1,1,1,1,1,1,1,1,1,1,1,
1,1,1,1,1,1,1,1,1,1,1,1,1,1,1,1,1,1,1,1,1,1,1,1,1,1,1,1,1,1,1,1,1,1,1,1,
1,1,1,1,1,1,1,1,1,1,1,1,1,1,1,1,1,1,1,1,1,1,1,1,1,1,1,1,1,1,1,1,1,1,1,1,
1,1,1,1,1,1,1,1,1,1,1,1,1,1,1,1,1,1,1,1,1,1,1,1,1,1,1,1,1,1,1,1,1,1,1,1,
1,1,1,1,1,1,1,1,1,1,1,1,1,1,1,1,1,1,1,1,1,1,1,1,1,1,1,1,1,1,1,1,1,1,1,1,
1,1,1,1,1,1,1,1,1,1,1,1,1,1,1,1,1,1,1,1,1,1,1,1,1,1,1,1,1,1,1,1,1,1,1,1,
1,1,1,1,1,1,1,1,1,1,1,1,1,1,1,1,1,1,1,1,1,1,1,1,1,1,1,1,1,1,1,1,1,1,1,1,
1,1,1,1,1,1,1,1,1,1,1,1,1,1,1,1,1,1,1,1,1,1,1,1,1,1,1,1,1,1,1,1,1,1,1,1,
1,1,1,1,1,1,1,1,1,1,1,1,1,1,1,1,1,1,1,1,1,1,1,1,1,1,1,1,1,1,1,1,1,1,1,1,
1,1,1,1,1,1,1,1,1,1,1,1,1,1,1,1,1,1,1,1,1,1,1,1,1,1,1,1,1,1,1,1,1,1,1,1,
1,1,1,1,1,1,1,1,1,1,1,1,1,1,1,1,1,1,1,1,1,1,1,1,1,1,1,1,1,1,1,1,1,1,1,1,
1,1,1,1,1,1,1,1,1,1,1,1,1,1,1,1,1,1,1,1,1,1,1,1,1,1,1,1,1,1,1,1,1,1,1,1,
1,1,1,1,1,1,1,1,1,1,1,1,1,1,1,1,1,1,1,1,1,1,1,1,1,1,1,1,1,1,1,1,1,1,1,1,
1,1,1,1,1,1,1,1,1,1,1,1,1,1,1,1,1,1,1,1,1,1,1,1,1,1,1,1,1,1,1,1,1,1,1,1,
1,1,1,1,1,1,1,1,1,1,1,1,1,1,1,1,1,1,1,1,1,1,1,1,1,1,1,1,1,1,1,1,1,1,1,1,
1,1,1,1,1,1,1,1,1,1,1,1,1,1,1,1,1,1,1,1,1,1,1,1,1,1,1,1,1,1,1,1,1,1,1,1,
1,1,1,1,1,1,1,1,1,1,1,1,1,1,1,1,1,1,1,1,1,1,1,1,1,1,1,1,1,1,1,1,1,1,1,1,
1,1,1,1,1,1,1,1,1,1,1,1,1,1,1,1,1,1,1,1,1,1,1,1,1,1,1,1,1,1,1,1,1,1,1,1,
1,1,1,1,1,1,1,1,1,1,1,1,1,1,1,1,1,1,1,1,1,1,1,1,1,1,1,1,1,1,1,1,1,1,1,1,
1,1,1,1,1,1,1,1,1,1,1,1,1,1,1,1,1,1,1,1,1,1,1,1,1,1,1,1,1,1,1,1,1,1,1,1,
1,1,1,1,1,1,1,1,1,1,1,1,1,1,1,1,1,1,1,1,1,1,1,1,1,1,1,1,1,1,1,1,1,1,1,1,
1,1,1,1,1,1,1,1,1,1,1,1,1,1,1,1,1,1,1,1,1,1,1,1,1,1,1,1,1,1,1,1,1,1,1,1,
1,1,1,1,1,1,1,1,1,1,1,1,1,1,1,1,1,1,1,1,1,1,1,1,1,1,1,1,1,1,1,1,1,1,1,1,
1,1,1,1,1,1,1,1,1,1,1,1,1,1,1,1,1,1,1,1,1,1,1,1,1,1,1,1,1,1,1,1,1,1,1,1,
1,1,1,1,1,1,1,1,1,1,1,1,1,1,1,1,1,1,1,1,1,1,1,1,1,1,1,1,1,1,1,1,1,1,1,1,
1,1,1,1,1,1,1,1,1,1,1,1,1,1,1,1,1,1,1,1,1,1,1,1,1,1,1,1,1,1,1,1,1,1,1,1,
1,1,1,1,1,1,1,1,1,1,1,1,1,1,1,1,1,1,1,1,1,1,1,1,1,1,1,1,1,1,1,1,1,1,1,1,
1,1,1,1,1,1,1,1,1,1,1,1,1,1,1,1,1,1,1,1,1,1,1,1,1,1,1,1,1,1,1,1,1,1,1,1,
1,1,1,1,1,1,1,1,1,1,1,1,1,1,1,1,1,1,1,1,1,1,1,1,1,1,1,1,1,1,1,1,1,1,1,1,
1,1,1,1,1,1,1,1,1,1,1,1,1,1,1,1,1,1,1,1,1,1,1,1,1,1,1,1,1,1,1,1,1,1,1,1,
1,1,1,1,1,1,1,1,1,1,1,1,1,1,1,1,1,1,1,1,1,1,1,1,1,1,1,1,1,1,1,1,1,1,1,1,
1,1,1,1,1,1,1,1,1,1,1,1,1,1,1,1,1,1,1,1,1,1,1,1,1,1,1,1,1,1,1,1,1,1,1,1,
1,1,1,1,1,1,1,1,1,1,1,1,1,1,1,1,1,1,1,1,1,1,1,1,1,1,1,1,1,1,1,1,1,1,1,1,
1,1,1,1,1,1,1,1,1,1,1,1,1,1,1,1,1,1,1,1,1,1,1,1,1,1,1,1,1,1,1,1,1,1,1,1,
1,1,1,1,1,1,1,1,1,1,1,1,1,1,1,1,1,1,1,1,1,1,1,1,1,1,1,1,1,1,1,1,1,1,1,1,
1,1,1,1,1,1,1,1,1,1,1,1,1,1,1,1,1,1,1,1,1,1,1,1,1,1,1,1,1,1,1,1,1,1,1,1,
1,1,1,1,1,1,1,1,1,1,1,1,1,1,1,1,1,1,1,1,1,1,1,1,1,1,1,1,1,1,1,1,1,1,1,1,
1,1,1,1,1,1,1,1,1,1,1,1,1,1,1,1,1,1,1,1,1,1,1,1,1,1,1,1,1,1,1,1,1,1,1,1,
1,1,1,1,1,1,1,1,1,1,1,1,1,1,1,1,1,1,1,1,1,1,1,1,1,1,1,1,1,1,1,1,1,1,1,1,
1,1,1,1,1,1,1,1,1,1,1,1,1,1,1,1,1,1,1,1,1,1,1,1,1,1,1,1,1,1,1,1,1,1,1,1,
1,1,1,1,1,1,1,1,1,1,1,1,1,1,1,1,1,1,1,1,1,1,1,1,1,1,1,1,1,1,1,1,1,1,1,1,
1,1,1,1,1,1,1,1,1,1,1,1,1,1,1,1,1,1,1,1,1,1,1,1,1,1,1,1,1,1,1,1,1,1,1,1,
1,1,1,1,1,1,1,1,1,1,1,1,1,1,1,1,1,1,1,1,1,1,1,1,1,1,1,1,1,1,1,1,1,1,1,1,
1,1,1,1,1,1,1,1,1,1,1,1,1,1,1,1,1,1,1,1,1,1,1,1,1,1,1,1,1,1,1,1,1,1,1,1,
1,1,1,1,1,1,1,1,1,1,1,1,1,1,1,1,1,1,1,1,1,1,1,1,1,1,1,1,1,1,1,1,1,1,1,1,
1,1,1,1,1,1,1,1,1,1,1,1,1,1,1,1,1,1,1,1,1,1,1,1,1,1,1,1,1,1,1,1,1,1,1,1,
1,1,1,1,1,1,1,1,1,1,1,1,1,1,1,1,1,1,1,1,1,1,1,1,1,1,1,1,1,1,1,1,1,1,1,1,
1,1,1,1,1,1,1,1,1,1,1,1,1,1,1,1,1,1,1,1,1,1,1,1,1,1,1,1,1,1,1,1,1,1,1,1,
1,1,1,1,1,1,1,1,1,1,1,1,1,1,1,1,1,1,1,1,1,1,1,1,1,1,1,1,1,1,1,1,1,1,1,1,
1,1,1,1,1,1,1,1,1,1,1,1,1,1,1,1,1,1,1,1,1,1,1,1,1,1,1,1,1,1,1,1,1,1,1,1,
1,1,1,1,1,1,1,1,1,1,1,1,1,1,1,1,1,1,1,1,1,1,1,1,1,1,1,1,1,1,1,1,1,1,1,1,
1,1,1,1,1,1,1,1,1,1,1,1,1,1,1,1,1,1,1,1,1,1,1,1,1,1,1,1,1,1,1,1,1,1,1,1,
1,1,1,1,1,1,1,1,1,1,1,1,1,1,1,1,1,1,1,1,1,1,1,1,1,1,1,1,1,1,1,1,1,1,1,1,
1,1,1,1,1,1,1,1,1,1,1,1,1,1,1,1,1,1,1,1,1,1,1,1,1,1,1,1,1,1,1,1,1,1,1,1,
1,1,1,1,1,1,1,1,1,1,1,1,1,1,1,1,1,1,1,1,1,1,1,1,1,1,1,1,1,1,1,1,1,1,1,1,
1,1,1,1,1,1,1,1,1,1,1,1,1,1,1,1,1,1,1,1,1,1,1,1,1,1,1,1,1,1,1,1,1,1,1,1,
1,1,1,1,1,1,1,1,1,1,1,1,1,1,1,1,1,1,1,1,1,1,1,1,1,1,1,1,1,1,1,1,1,1,1,1,
1,1,1,1,1,1,1,1,1,1,1,1,1,1,1,1,1,1,1,1,1,1,1,1,1,1,1,1,1,1,1,1,1,1,1,1,
1,1,1,1,1,1,1,1,1,1,1,1,1,1,1,1,1,1,1,1,1,1,1,1,1,1,1,1,1,1,1,1,1,1,1,1,
1,1,1,1,1,1,1,1,1,1,1,1,1,1,1,1,1,1,1,1,1,1,1,1,1,1,1,1,1,1,1,1,1,1,1,1,
1,1,1,1,1,1,1,1,1,1,1,1,1,1,1,1,1,1,1,1,1,1,1,1,1,1,1,1,1,1,1,1,1,1,1,1,
1,1,1,1,1,1,1,1,1,1,1,1,1,1,1,1,1,1,1,1,1,1,1,1,1,1,1,1,1,1,1,1,1,1,1,1,
1,1,1,1,1,1,1,1,1,1,1,1,1,1,1,1,1,1,1,1,1,1,1,1,1,1,1,1,1,1,1,1,1,1,1,1,
1,1,1,1,1,1,1,1,1,1,1,1,1,1,1,1,1,1,1,1,1,1,1,1,1,1,1,1,1,1,1,1,1,1,1,1,
1,1,1,1,1,1,1,1,1,1,1,1,1,1,1,1,1,1,1,1,1,1,1,1,1,1,1,1,1,1,1,1,1,1,1,1,
1,1,1,1,1,1,1,1,1,1,1,1,1,1,1,1,1,1,1,1,1,1,1,1,1,1,1,1,1,1,1,1,1,1,1,1,
1,1,1,1,1,1,1,1,1,1,1,1,1,1,1,1,1,1,1,1,1,1,1,1,1,1,1,1,1,1,1,1,1,1,1,1,
1,1,1,1,1,1,1,1,1,1,1,1,1,1,1,1,1,1,1,1,1,1,1,1,1,1,1,1,1,1,1,1,1,1,1,1,
1,1,1,1,1,1,1,1,1,1,1,1,1,1,1,1,1,1,1,1,1,1,1,1,1,1,1,1,1,1,1,1,1,1,1,1,
1,1,1,1,1,1,1,1,1,1,1,1,1,1,1,1,1,1,1,1,1,1,1,1,1,1,1,1,1,1,1,1,1,1,1,1,
1,1,1,1,1,1,1,1,1,1,1,1,1,1,1,1,1,1,1,1,1,1,1,1,1,1,1,1,1,1,1,1,1,1,1,1,
1,1,1,1,1,1,1,1,1,1,1,1,1,1,1,1,1,1,1,1,1,1,1,1,1,1,1,1,1,1,1,1,1,1,1,1,
1,1,1,1,1,1,1,1,1,1,1,1,1,1,1,1,1,1,1,1,1,1,1,1,1,1,1,1,1,1,1,1,1,1,1,1,
1,1,1,1,1,1,1,1,1,1,1,1,1,1,1,1,1,1,1,1,1,1,1,1,1,1,1,1,1,1,1,1,1,1,1,1,
1,1,1,1,4),(2,2),(0.,0.869746702321014,1.7394931589914,2.60923976624962,
3.47983908319159,4.35043840179749,5.22018503077054,6.08993165951504,6.95967828799171,
7.82942491616733,8.69917154401062,9.56891817149224,10.4395174886835,11.3101168056706,
12.179863432132,13.049610058144,13.9193566836854,14.7891033087372,15.6588499332817,
16.5285965573034,17.3991958717975,18.2697951860185,18.7046684974166,19.1395418086746,
19.5744151197912,20.0092884307654,20.4441617415962,20.8790350522825,21.7487816732187,
22.1836549834672,22.6185282935685,23.0534016035221,23.4882749133276,23.9231482229848,
24.3588742245859,24.794600226187,25.2294735355468,26.0992201538203,26.5340934627341,
26.9689667714994,27.4038400801166,27.838713388586,28.2735866969081,28.7084600050832,
29.143333313112,29.5782066209952,30.0130799287334,30.4479532363275,30.8828265437783,
31.3185525442794,31.7542785447804,32.1891518519474,32.6240251589741,33.0588984658616,
33.4937717726112,33.928645079224,34.3635183857014,34.7983916920448,35.2332649982556,
35.6681383043353,36.1030116102854,36.5378849161076,36.9727582218035,37.4076315273749,
37.8425048328235,38.2782308323341,38.7139568318446,39.1488301370532,39.5837034421446,
40.0185767471208,40.4534500519838,40.8883233567357,41.3231966613787,41.7580699659148,
42.1929432703463,42.6278165746754,43.0626898789044,43.4975631830356,43.9324364870714,
44.3673097910142,44.8021830948664,45.2379090935952,45.673635092324,46.1085083960024,
46.5433816995978,46.9782550031127,47.4131283065497,47.8480016099115,48.2828749132006,
48.7177482164198,49.1526215195718,49.5874948226593,50.0223681256851,50.457241428652,
50.8921147315628,51.3269880344203,51.7618613372274,52.197587335454,52.6333133336805,
53.0681866363954,53.5030599390685,53.9379332417027,54.3728065443011,54.8076798468664,
55.2425531494018,55.6774264519101,56.1122997543943,56.5471730568575,56.9820463593026,
57.4169196617326,57.8517929641506,58.2866662665595,58.7215395689624,59.157265567009,
59.5929915650557,60.0278648674556,60.4627381698584,60.8976114722673,61.3324847746853,
61.7673580771153,62.2022313795604,62.6371046820236,63.0719779845079,63.5068512870162,
63.9417245895516,64.376597892117,64.8114711947155,65.2463444973499,65.6812178000231,
66.1169437982275,66.5526697964318,66.9875430991915,67.4224164019987,67.8572897048563,
68.2921630077673,68.7270363107343,69.1619096137603,69.5967829168479,70.0316562200001,
70.4665295232194,70.9014028265087,71.3362761298705,71.7711494333077,72.2060227368227,
72.6408960404182,73.0766220391044,73.5123480377905,73.9472213415547,74.382094645407,
74.8169679493499,75.2518412533859,75.6867145575172,76.1215878617464,76.5564611660756,
76.9913344705072,77.4262077750435,77.8610810796866,78.2959543844386,78.7308276893018,
79.1657009942781,79.6005742993696,80.0363002988208,80.4720262982719,80.9068996035997,
81.3417729090484,81.7766462146199,82.211519520316,82.6463928261383,83.0812661320886,
83.5161394381684,83.9510127443794,84.3858860507229,84.8207593572004,85.2556326638134,
85.6905059705631,86.1253792774507,86.5602525844776,86.995978584908,87.4317045853384,
87.8665778926469,88.3014512000977,88.7363245076919,89.1711978154302,89.6060711233134,
90.0409444313423,90.4758177395175,90.9106910478396,91.345564356309,91.7804376649263,
92.2153109736917,92.6501842826055,93.085057591668,93.5199309008791,93.9556569024059,
94.3913829039327,94.8262562134414,95.2611295230986,95.6960028329042,96.1308761428578,
96.5657494529591,97.0006227632077,97.4354960736028,97.870369384144,98.3052426948304,
98.7401160056612,99.1749893166354,99.6098626277522,100.04473593901,100.915335253024,
101.351061255639,101.785934567313,102.220807879124,102.655681191068,103.090554503145,
103.525427815353,104.395174440154,105.264921065453,105.699794378283,106.134667691232,
106.569541004295,107.004414317471,107.8750136343,108.745612951339,109.615359578629,
110.485106206296,111.354852834309,112.224599462639,113.094346091254,113.964092720119,
114.834692038763,115.705291357499,116.575037986826,117.444784616267,118.314531245777,
119.184277875311,120.054024504821,120.923771134261,121.794370453112,122.66496977189,
123.534716400968,124.404463029834,125.274209658448,126.143956286779,127.013702914792,
127.883449542458,128.754048859798,129.624648176939,130.494394803617,131.364141429857,
132.233888055637,133.103634680937,133.973381305737,134.843127930023,135.71372724472,
136.584326559147,137.019199870684,137.454073182083,137.888946493341,138.323819804458,
139.193566426263,140.063313047491,140.498186357887,140.933059668136,141.367932978237,
141.802806288191,142.237679597997,142.673405599673,143.109131601348,143.544004910857,
143.978878220217,144.413751529429,144.848624838491,145.283498147405,145.718371456171,
146.153244764789,146.588118073258,147.022991381581,147.457864689756,147.892737997785,
148.327611305669,148.762484613407,149.197357921002,149.633083921574,150.068809922147,
150.503683229455,150.938556536623,151.37342984365,151.808303150538,152.243176457288,
152.678049763901,153.112923070379,153.547796376722,153.982669682934,154.417542989014,
154.852416294964,155.287289600787,155.722162906483,156.157036212055,156.592762211626,
157.028488211198,157.463361516526,157.898234821735,158.333108126826,158.767981431803,
159.202854736666,159.637728041419,160.072601346062,160.507474650599,160.94234795503,
161.37722125936,161.812094563589,162.246967867721,162.681841171757,163.1167144757,
163.552440474473,163.988166473247,164.423039777011,164.85791308069,165.292786384286,
165.727659687801,166.162532991238,166.597406294601,167.03227959789,167.46715290111,
167.902026204262,168.33689950735,168.771772810376,169.206646113343,169.641519416254,
170.076392719112,170.512118717363,170.947844715614,171.382718018374,171.817591321089,
172.252464623762,172.687337926397,173.122211228996,173.557084531561,173.991957834097,
174.426831136606,174.86170443909,175.296577741554,175.731451044,176.16632434643,
176.601197648848,177.036070951258,177.471796949306,177.907522947355,178.342396249755,
178.777269552155,179.212142854558,179.647016156968,180.081889459386,180.516762761816,
180.951636064262,181.386509366726,181.82138266921,182.256255971719,182.691129274255,
183.12600257682,183.560875879419,183.995749182054,184.431475180237,184.867201178421,
185.302074481136,185.736947783896,186.171821086704,186.606694389561,187.041567692473,
187.47644099544,187.911314298466,188.346187601554,188.781060904706,189.215934207926,
189.650807511215,190.085680814577,190.520554118015,190.95542742153,191.391153420175,
191.82687941882,192.261752722499,192.696626026263,193.131499330116,193.566372634059,
194.001245938095,194.436119242227,194.870992546456,195.305865850785,195.740739155217,
196.175612459754,196.610485764397,197.045359069149,197.480232374013,197.915105678989,
198.350831678382,198.786557677775,199.221430982984,199.656304288312,200.091177593761,
200.526050899333,200.960924205029,201.395797510852,201.830670816802,202.265544122882,
202.700417429093,203.135290735437,203.570164041915,204.005037348528,204.439910655278,
204.874783962166,205.310509962526,205.746235962887,206.181109270054,206.615982577363,
207.050855884814,207.485729192409,207.920602500147,208.355475808031,208.79034911606,
209.225222424235,209.660095732558,210.094969041027,210.529842349645,210.96471565841,
211.399588967324,211.834462276387,212.27018827784,212.705914279292,213.140787588653,
213.575660898161,214.010534207819,214.880280827579,215.31515413768,215.750027447929,
216.184900758324,216.619774068866,217.054647379553,217.489520690384,218.359267312475,
219.22986662628,219.665592628826,220.100465940363,220.535339252038,220.970212563848,
221.83995918787,222.709705812416,223.579452437468,224.014325750179,224.44919906301,
225.318945689022,226.189545005688,227.060144322571,227.929890949664,228.799637577146,
229.66938420499,230.539130833166,231.408877461643,232.278624090388,233.149223408954,
234.019822727623,234.889569356878,235.759315986267,236.629062615749,237.498809245277,
238.368555874806,239.238302504287,240.108901823183,240.979501142017,241.849247771189,
242.718994400167,243.588741028911,244.458487657389,245.328234285565,246.197980913409,
247.068580230891,247.939179548182,248.80892617507,249.678672801532,250.548419427545,
251.418166053087,252.287912678139,253.157659302684,254.028258617581,254.898857932211,
255.333731243885,255.768604555423,256.203477866821,256.63835117808,257.508097800171,
258.377844421689,258.812717732231,259.247591042627,259.682464352876,260.117337662977,
260.552210972931,260.987936974682,261.858536286089,262.293409595598,262.728282904958,
263.16315621417,263.598029523233,264.032902832147,264.467776140913,264.902649449531,
265.337522758001,265.772396066323,266.207269374499,266.642142682528,267.077015990412,
267.511889298151,267.947615298795,268.383341299439,268.81821460689,269.2530879142,
269.687961221367,270.122834528394,270.557707835282,270.992581142032,271.427454448646,
271.862327755124,272.297201061468,272.732074367679,273.166947673759,273.60182097971,
274.036694285533,274.471567591229,274.907293590862,275.343019590495,275.777892895944,
276.212766201272,276.647639506481,277.082512811573,277.51738611655,277.952259421414,
278.387132726166,278.82200603081,279.256879335346,279.691752639779,280.126625944108,
280.561499248338,280.996372552469,281.431245856506,281.866971855324,282.302697854143,
282.737571157996,283.172444461761,283.60731776544,284.042191069036,284.477064372551,
284.911937675989,285.346810979351,285.781684282641,286.216557585861,286.651430889013,
287.086304192101,287.521177495128,287.956050798095,288.390924101007,288.826650099283,
289.262376097559,289.697249400366,290.132122703127,290.566996005842,291.001869308516,
291.43674261115,291.871615913749,292.306489216315,292.741362518851,293.17623582136,
293.611109123845,294.045982426308,294.480855728754,294.915729031185,295.350602333603,
295.786328331655,296.222054329707,296.65692763211,297.091800934511,297.526674236911,
297.961547539314,298.396420841724,298.831294144142,299.266167446573,299.701040749018,
300.135914051482,300.570787353967,301.005660656476,301.440533959012,301.875407261578,
302.310280564177,302.746006562341,303.181732560506,303.616605863179,304.051479165895,
304.486352468655,304.921225771462,305.35609907432,305.790972377232,306.225845680199,
306.660718983226,307.095592286314,307.530465589466,307.965338892686,308.400212195976,
308.835085499338,309.269958802776,309.705684801381,310.141410799985,310.576284103581,
311.01115740726,311.446030711025,311.880904014878,312.315777318821,312.750650622858,
313.185523926989,313.620397231219,314.055270535549,314.490143839981,314.925017144517,
315.359890449161,315.794763753913,316.229637058777,316.665363058112,317.101089057448,
317.53596236254,317.970835667749,318.405708973077,318.840582278526,319.275455584098,
319.710328889795,320.145202195618,320.580075501568,321.014948807648,321.44982211386,
321.884695420204,322.319568726682,322.754442033295,323.189315340045,323.625041340336,
324.060767340628,324.495640647655,324.930513954822,325.365387262131,325.800260569583,
326.235133877177,326.670007184916,327.1048804928,327.539753800829,327.974627109005,
328.409500417327,328.844373725797,329.279247034415,329.714120343181,330.148993652095,
330.584719653474,331.020445654852,331.455318964064,331.890192273424,332.325065582933,
332.759938892591,333.194812202397,333.629685512351,334.064558822453,334.499432132702,
334.934305443098,335.369178753639,335.804052064326,336.673798686132,337.108671997249,
337.544397999725,337.980124002201,338.4149973136,338.849870625137,339.284743936812,
340.154490560568,341.024237184854,341.459110497191,341.893983809655,342.328857122244,
342.763730434955,343.633477060735,344.504076377234,345.374675693955,346.244422320844,
347.114168948136,347.983915575803,348.853662203817,349.723408832148,350.593155460764,
351.463754779246,352.334354097839,353.204100727012,354.07384735634,354.943593985781,
355.813340615292,356.683087244827,357.552833874338,358.423433193272,359.294032512154,
360.163779141409,361.033525770489,361.903272399355,362.77301902797,363.642765656301,
364.512512284316,365.383111601936,366.253710919371,367.123457546465,367.993204173143,
368.862950799383,369.732697425164,370.602444050463,371.472190675265,372.342789990359,
373.21338930519,373.648262617,374.083135928675,374.952882551611,375.822629173987,
376.257502484962,376.692375795793,377.12724910648,377.562122417021,377.996995727417,
378.431869037666,378.866742347767,379.302468349591,379.738194351416,380.173067661222,
380.607940970879,381.042814280388,381.477687589749,381.91256089896,382.347434208023,
382.782307516937,383.217180825703,383.652054134321,384.086927442791,384.521800751113,
384.956674059289,385.391547367318,385.826420675202,386.262146675918,386.697872676635,
387.13274598423,387.567619291681,388.00249259899,388.437365906157,388.872239213185,
389.307112520073,389.741985826823,390.176859133436,390.611732439914,391.046605746258,
391.48147905247,391.91635235855,392.351225664501,392.786098970323,393.221824970019,
393.657550969714,394.092424275286,394.527297580735,394.962170886063,395.397044191272,
395.831917496364,396.266790801341,396.701664106204,397.136537410957,397.5714107156,
398.006284020137,398.441157324569,398.876030628899,399.310903933128,399.74577723726,
400.181503236126,400.617229234991,401.052102538934,401.486975842787,401.921849146551,
402.356722450231,402.791595753827,403.226469057342,403.66134236078,404.096215664142,
404.531088967432,404.965962270651,405.400835573804,405.835708876892,406.270582179918,
406.705455482886,407.141181481189,407.576907479491,408.01178078235,408.446654085157,
408.881527387917,409.316400690633,409.751273993306,410.186147295941,410.62102059854,
411.055893901106,411.490767203642,411.925640506151,412.360513808636,412.795387111099,
413.230260413545,413.665133715976,414.100859714032,414.536585712088,414.971459014498,
415.406332316901,415.841205619301,416.276078921702,416.710952224105,417.145825526515,
417.580698828933,418.015572131364,418.45044543381,418.885318736273,419.320192038758,
419.755065341267,420.189938643803,420.624811946369,421.060537944515,421.496263942662,
421.931137245297,422.36601054797,422.800883850686,423.235757153446,423.670630456253,
424.105503759112,424.540377062023,424.975250364991,425.410123668017,425.844996971105,
426.279870274258,426.714743577477,427.149616880767,427.584490184129,428.020216182695,
428.455942181261,428.890815484776,429.325688788373,429.760562092052,430.195435395816,
430.630308699669,431.065182003612,431.500055307649,431.93492861178,432.36980191601,
432.80467522034,433.239548524772,433.674421829309,434.109295133952,434.544168438705,
434.979894437984,435.415620437262,435.850493742239,436.285367047331,436.72024035254,
437.155113657869,437.589986963318,438.024860268889,438.459733574586,438.894606880409,
439.32948018636,439.76435349244,440.199226798651,440.634100104995,441.068973411473,
441.503846718087,441.939572718309,442.375298718531,442.810172025419,443.245045332447,
443.679918639614,444.114791946923,444.549665254374,444.984538561969,445.419411869708,
445.854285177591,446.289158485621,446.724031793796,447.158905102119,447.593778410589,
448.028651719207,448.463525027973,448.899251029277,449.334977030581,449.769850339644,
450.639596958216,451.074470267725,451.509343577383,451.944216887189,452.379090197143,
452.813963507244,453.248836817493,453.683710127889,454.118583438431,454.553456749117,
454.988330059949,455.423203370923,455.858929373329,456.294655375734,456.729528686993,
457.164401998391,457.599275309929,458.469021933414,458.90389524536,459.338768557437,
459.773641869646,460.208515181983,460.643388494447,461.078261807036,461.948008432578,
462.818607748906,463.689207065461,464.55895369214,465.428700319234,466.298446946716,
467.16819357456,468.037940202737,468.907686831215,469.778286149605,470.648885468116,
471.518632097196,472.388378726451,473.258125355841,474.127871985322,474.997618614851,
475.86736524438,476.737964563343,477.608563882265,478.478310511593,479.348057140765,
480.217803769743,481.087550398488,481.957297026966,482.827043655142,483.697642972895,
484.568242290469,485.43798891776,486.307735544649,487.177482171112,488.047228797125,
488.916975422667,489.78672204772,490.657321363009,491.09304736596,491.527920678038,
492.397667301793,493.267413925005,494.137160547663,494.57203385878,495.006907169755,
495.441780480586,495.876653791273,496.311527101814,496.74640041221,497.616999724357,
498.052725726255,498.487599036209,498.922472346015,499.357345655673,499.792218965182,
500.227092274542,500.661965583754,501.096838892816,501.531712201731,501.966585510497,
502.401458819114,502.836332127584,503.271205435907,503.706078744082,504.140952052112,
504.576678052901,505.01240405369,505.447277361429,505.882150669023,506.317023976474,
506.751897283783,507.186770590951,507.621643897978,508.056517204866,508.491390511616,
508.92626381823,509.361137124708,509.796010431052,510.230883737263,510.665757043344,
511.100630349294,511.536356349053,511.972082348811,512.406955654506,512.841828960076,
513.276702265523,513.711575570849,514.146448876056,514.581322181146,515.016195486121,
515.451068790983,515.885942095733,516.320815400375,516.75568870491,517.19056200934,
517.625435313668,518.060308617896,518.496034616807,518.931760615718,519.366633919752,
519.801507223694,520.236380527545,520.671253831307,521.106127134985,521.541000438579,
521.975873742092,522.410747045528,522.845620348888,523.280493652176,523.715366955394,
524.150240258545,524.585113561631,525.019986864656,525.455712862985,525.891438861313,
526.326312164223,526.761185467079,527.196058769885,527.630932072643,528.065805375356,
528.500678678029,528.935551980661,529.370425283258,529.805298585822,530.240171888356,
530.675045190863,531.109918493346,531.544791795808,531.979665098252,532.415391096312,
532.851117094373,533.285990396789,533.720863699197,534.155737001598,534.590610303997,
535.025483606395,535.460356908796,535.895230211204,536.330103513621,536.764976816049,
537.199850118493,537.634723420955,538.069596723438,538.504470025945,538.93934332848,
539.375069326608,539.810795324736,540.245668627333,540.680541929966,541.115415232637,
541.550288535351,541.985161838109,542.420035140915,542.854908443771,543.28978174668,
543.724655049646,544.15952835267,544.594401655757,545.029274958907,545.464148262125,
545.899021565413,546.334747563939,546.770473562465,547.205346865901,547.640220169415,
548.075093473009,548.509966776686,548.944840080449,549.3797133843,549.814586688241,
550.249459992276,550.684333296405,551.119206600633,551.554079904961,551.988953209391,
552.423826513926,552.858699818567,553.294425817789,553.73015181701,554.165025121872,
554.599898426846,555.034771731937,555.469645037144,555.90451834247,556.339391647917,
556.774264953487,557.209138259182,557.644011565003,558.078884870951,558.51375817703,
558.948631483239,559.383504789581,559.818378096058,560.254104096209,560.689830096361,
561.12470340311,561.559576709996,561.994450017021,562.429323324187,562.864196631494,
563.299069938943,563.733943246536,564.168816554273,564.603689862154,565.038563170182,
565.473436478355,565.908309786676,566.343183095144,566.77805640376,567.213782404988,
567.649508406216,568.084381715128,568.519255024189,568.954128333399,569.389001642757,
569.823874952264,570.258748261921,570.693621571725,571.128494881677,571.563368191777,
572.433114812417,572.867988122957,573.302861433642,573.737734744471,574.173460746804,
574.609186749136,575.044060060251,575.913806682904,576.783553306113,577.218426617922,
577.653299929865,578.08817324194,578.523046554147,579.392793178944,580.26253980424,
581.13313912039,581.568865123709,582.003738436771,582.87348506323,583.743231690115,
584.612978317402,585.482724945065,586.352471573076,587.222218201403,588.092817519691,
588.963416838109,589.833163467083,590.702910096251,591.572656725575,592.442403355013,
593.31214998452,594.181896614051,595.05249593303,595.92309525198,596.792841881366,
597.662588510618,598.532335139693,599.402081768556,600.271828397167,601.141575025495,
602.012174343369,602.882773661074,603.752520288553,604.622266915642,605.492013542317,
606.361760168553,607.23150679433,608.101253419626,608.971852735101,609.842452050322,
610.71219867434,611.581945297822,612.451691920754,612.886565232011,613.321438543126,
613.756311854099,614.191185164928,615.060931786153,615.931531098516,616.367257100486,
616.802130410586,617.237003720538,617.671877030342,618.106750339998,618.541623649505,
618.976496958863,619.411370268073,619.846243577134,620.281116886046,620.71599019481,
621.150863503426,621.585736811894,622.020610120214,622.455483428388,622.891209429248,
623.326935430108,623.761808737989,624.196682045726,624.631555353319,625.066428660769,
625.501301968075,625.936175275241,626.371048582266,626.805921889153,627.240795195901,
627.675668502512,628.110541808988,628.54541511533,628.98028842154,629.415161727618,
629.850887727438,630.286613727259,630.72148703308,631.156360338774,631.591233644344,
632.026106949791,632.460980255118,632.895853560325,633.330726865415,633.76560017039,
634.200473475251,634.635346780002,635.070220084644,635.505093389179,635.939966693609,
636.374839997937,636.810565996897,637.246291995857,637.681165299986,638.116038604021,
638.550911907962,638.985785211813,639.420658515576,639.855531819253,640.290405122847,
640.725278426361,641.160151729796,641.595025033157,642.029898336444,642.464771639662,
642.899644942813,643.334518245899,643.770244244257,644.205970242616,644.640843545581,
645.075716848491,645.510590151347,645.945463454153,646.380336756911,646.815210059625,
647.250083362296,647.684956664929,648.119829967526,648.55470327009,648.989576572624,
649.424449875131,649.859323177614,650.294196480076,650.729922478144,651.165648476212,
651.600521778641,652.035395081057,652.470268383465,652.905141685866,653.340014988265,
653.774888290663,654.209761593065,654.644634895472,655.079508197889,655.514381500318,
655.949254802762,656.384128105224,656.819001407706,657.253874710213,657.689600708326,
658.12532670644,658.560200009004,658.995073311601,659.429946614234,659.864819916905,
660.299693219619,660.734566522377,661.169439825183,661.604313128039,662.039186430948,
662.474059733914,662.908933036938,663.343806340025,663.778679643175,664.213552946393,
664.649278944883,665.085004943373,665.519878246733,665.954751550169,666.389624853683,
666.824498157277,667.259371460954,667.694244764717,668.129118068568,668.563991372509,
668.998864676544,669.433737980674,669.868611284901,670.303484589229,670.738357893659,
671.173231198194,671.608957197361,672.044683196528,672.479556501278,672.91442980614,
673.349303111115,673.784176416205,674.219049721412,674.653923026738,675.088796332185,
675.523669637755,675.95854294345,676.393416249271,676.82828955522,677.263162861298,
677.698036167508,678.13290947385,678.568635473934,679.004361474018,679.439234780629,
679.874108087377,680.308981394264,680.743854701289,681.178728008455,681.613601315762,
682.048474623211,682.483347930804,682.91822123854,683.353094546422,683.78796785445,
684.222841162623,684.657714470944,685.092587779412,685.528313780566,685.96403978172,
686.398913090483,686.833786399396,687.268659708457,687.703533017666,688.138406327025,
688.573279636532,689.008152946187,689.443026255992,689.877899565944,690.312772876043,
690.74764618629,691.182519496684,691.617392807224,692.052266117909,692.487992120169,
692.92371812243,693.358591433403,694.228338055774,694.663211367171,695.098084678707,
695.532957990379,695.967831302188,696.402704614131,696.837577926207,697.707324550749,
698.577071175797,699.011944488507,699.447670491767,699.883396495028,700.318269807975,
701.188016434211,702.057763060886,702.927509687976,703.797256315454,704.667002943295,
705.536749571467,706.407348889651,707.277948207973,708.147694836835,709.017441465911,
709.887188095163,710.756934724548,711.626681354026,712.496427983551,713.367027302543,
714.237626621516,715.107373250954,715.977119880277,716.846866509446,717.716613138419,
718.586359767161,719.456106395635,720.32670571363,721.197305031464,722.067051659126,
722.936798286414,723.806544913299,724.676291539758,725.546038165767,726.415784791305,
727.286384106969,728.156983422381,729.026730046663,729.896476670415,730.331349982088,
730.766223293624,731.201096605021,731.635969916278,732.505716538366,733.37546315988,
733.81033647042,734.246062472462,734.681788474505,735.116661784752,735.551535094852,
735.986408404804,736.421281714608,736.856155024264,737.291028333771,737.72590164313,
738.160774952339,738.5956482614,739.030521570312,739.465394879076,739.900268187692,
740.33514149616,740.77001480448,741.205740805414,741.641466806347,742.076340114374,
742.511213422256,742.946086729993,743.380960037585,743.815833345035,744.250706652341,
744.685579959507,745.120453266533,745.555326573419,745.990199880167,746.425073186778,
746.859946493254,747.294819799596,747.729693105806,748.165419105691,748.601145105576,
749.036018411525,749.470891717346,749.90576502304,750.34063832861,750.775511634057,
751.210384939384,751.645258244591,752.080131549682,752.515004854656,752.949878159518,
753.384751464269,753.81962476891,754.254498073445,754.689371377875,755.125097376885,
755.560823375895,755.995696680123,756.430569984253,756.865443288287,757.300316592228,
757.735189896079,758.170063199842,758.604936503519,759.039809807113,759.474683110627,
759.909556414062,760.344429717423,760.779303020711,761.214176323929,761.649049627079,
762.084775625469,762.520501623858,762.955374926883,763.390248229848,763.825121532758,
764.259994835614,764.694868138419,765.129741441178,765.564614743891,765.999488046563,
766.434361349196,766.869234651793,767.304107954357,767.738981256891,768.173854559398,
768.608727861881,769.044453859958,769.480179858035,769.915053160479,770.349926462907,
770.784799765324,771.219673067731,771.654546370133,772.089419672531,772.52429297493,
772.959166277331,773.394039579739,773.828912882155,774.263786184584,774.698659487028,
775.13353278949,775.568406091973,776.004132090072,776.439858088172,776.874731390706,
777.30960469327,777.744477995867,778.1793512985,778.614224601171,779.049097903885,
779.483971206643,779.918844509449,780.353717812305,780.788591115215,781.22346441818,
781.658337721205,782.093211024291,782.528084327442,782.963810325897,783.399536324352,
783.834409627639,784.269282931,784.704156234435,785.139029537949,785.573902841543,
786.00877614522,786.443649448983,786.878522752834,787.313396056775,787.74826936081,
788.183142664939,788.618015969167,789.052889273495,789.487762577925,789.923488577038,
790.359214576152,790.794087880793,791.228961185544,791.663834490406,792.098707795381,
792.533581100471,792.968454405678,793.403327711004,793.838201016451,794.273074322021,
794.707947627716,795.142820933537,795.577694239486,796.012567545564,796.447440851774,
796.883166851791,797.318892851808,797.753766158284,798.188639464895,798.623512771643,
799.058386078529,799.493259385555,799.92813269272,800.363006000027,800.797879307477,
801.232752615069,801.667625922806,802.102499230688,802.537372538715,802.972245846889,
803.40711915521,803.84284515629,804.27857115737,804.713444465985,805.148317774749,
805.583191083662,806.018064392723,806.452937701933,806.887811011291,807.322684320798,
808.192430940258,808.62730425021,809.06217756031,809.497050870557,809.931924180951,
810.36679749149,810.802523493679,811.238249495867,811.673122806697,812.542869428785,
812.977742740041,813.412616051438,813.847489362974,814.282362674646,814.717235986455,
815.152109298398,816.021855922681,816.891602547478,817.326475860065,817.762201863265,
818.197927866466,818.632801179295,819.502547805304,820.372294431763,821.242041058648,
822.111787685935,822.981534313598,823.851280941609,824.721880259681,825.5924795779,
826.462226206642,827.331972835616,828.201719464785,829.071466094109,829.941212723546,
830.810959353053,831.681558672047,832.552157991036,833.421904620514,834.2916512499,
835.161397879151,836.031144508226,836.900891137089,837.770637765701,838.641237083811,
839.511836401767,840.381583029608,841.251329657086,842.121076284176,842.990822910851,
843.860569537087,844.730316162863,845.600915478712,846.471514794314,847.341261418855,
848.211008042874,848.645881354683,849.080754666356,849.515627977891,849.950501289288,
850.82024791166,851.689994533462,852.124867844147,852.560593846263,852.996319848379,
853.431193158772,853.866066469019,854.300939779119,855.170686398875,855.605559708531,
856.040433018038,856.475306327397,856.910179636606,857.345052945667,857.77992625458,
858.214799563344,858.64967287196,859.084546180427,859.520272181434,859.95599818244,
860.390871490614,860.825744798641,861.260618106523,861.69549141426,862.130364721852,
862.565238029302,863.000111336609,863.434984643774,863.8698579508,864.304731257686,
864.739604564434,865.174477871045,865.609351177521,866.044224483863,866.479950483814,
866.915676483765,867.350549789843,867.785423095792,868.220296401613,868.655169707307,
869.090043012877,869.524916318325,869.959789623651,870.394662928858,870.829536233948,
871.264409538923,871.699282843785,872.134156148535,872.569029453177,873.003902757712,
873.439628756773,873.875354755834,874.310228060162,874.745101364389,875.179974668519,
875.614847972553,876.049721276495,876.484594580346,876.919467884108,877.354341187786,
877.78921449138,878.224087794893,878.658961098329,879.093834401689,879.528707704977,
879.963581008195,880.399307006616,880.835033005038,881.269906308124,881.704779611148,
882.139652914114,882.574526217024,883.00939951988,883.444272822685,883.879146125444,
884.314019428157,884.748892730829,885.183766033462,885.618639336059,886.053512638623,
886.488385941157,886.923259243664,887.358985241751,887.794711239839,888.2295845423,
888.664457844744,889.099331147173,889.534204449589,889.969077751997,890.403951054398,
890.838824356797,891.273697659195,891.708570961597,892.143444264004,892.578317566421,
893.01319086885,893.448064171293,893.882937473755,894.318663471843,894.75438946993,
895.189262772437,895.624136074971,896.059009377535,896.493882680132,896.928755982765,
897.363629285437,897.798502588151,898.233375890909,898.668249193715,899.103122496571,
899.53799579948,899.972869102446,900.40774240547,900.842615708556,901.278341706978,
901.714067705399,902.148941008617,902.583814311905,903.018687615265,903.453560918701,
903.888434222214,904.323307525808,904.758180829485,905.193054133248,905.627927437099,
906.06280074104,906.497674045075,906.932547349205,907.367420653433,907.80229395776,
908.238019956821,908.673745955883,909.108619260417,909.543492565059,909.978365869809,
910.413239174671,910.848112479646,911.282985784736,911.717859089943,912.152732395269,
912.587605700716,913.022479006287,913.457352311981,913.892225617802,914.327098923751,
914.761972229829,915.19769822978,915.633424229731,916.068297536072,916.503170842548,
916.93804414916,917.372917455908,917.807790762794,918.24266406982,918.677537376985,
919.112410684292,919.547283991742,919.982157299334,920.417030607071,920.851903914953,
921.28677722298,921.721650531154,922.15737653216,922.593102533167,923.027975841635,
923.46284915025,923.897722459014,924.332595767926,924.767469076987,925.202342386197,
925.637215695556,926.072089005063,926.506962314719,926.941835624523,927.376708934475,
927.811582244575,928.246455554822,928.681328865215,929.117054867331,929.987654180132,
930.422527490961,930.857400801934,931.292274113049,931.727147424306,932.162020735703,
932.596894047238,933.46664067072,934.336387294739,934.771260606945,935.20613391928,
935.641007231742,936.076733234882,936.94733255073,937.817079176507,938.686825802743,
939.556572429418,940.426319056508,941.296065683986,942.165812311827,943.036411629783,
943.907010947893,944.776757576505,945.646504205367,946.516250834443,947.385997463694,
948.25574409308,949.125490722558,949.996090041546,950.86668936054,951.736435990048,
952.606182619485,953.475929248809,954.345675877978,955.215422506951,956.085169135693,
956.955768453912,957.826367771985,958.696114399995,959.565861027658,960.435607654946,
961.305354281831,962.175100908289,963.044847534298,963.915446850328,964.786046166116,
965.655792790913,966.525539415195,966.960412727138,967.395286038947,968.265032662155,
969.134779284809,969.569652595924,970.004525906897,970.439399217726,970.875125219914,
971.310851222103,971.745724532643,972.615471153283,973.485217773335,973.920091083139,
974.354964392795,974.789837702302,975.22471101166,975.65958432087,976.094457629931,
976.529330938844,976.964204247608,977.399077556223,977.834803557303,978.270529558383,
978.705402866704,979.140276174877,979.575149482905,980.010022790786,980.444896098523,
980.879769406116,981.314642713565,981.749516020872,982.184389328038,982.619262635063,
983.05413594195,983.489009248698,983.923882555309,984.358755861785,984.794481861802,
985.230207861819,985.665081168029,986.099954474107,986.534827780056,986.969701085877,
987.404574391571,987.839447697141,988.274321002589,988.709194307915,989.144067613122,
989.578940918212,990.013814223187,990.448687528048,990.883560832799,991.31843413744,
991.754160136554,992.189886135667,992.624759440097,993.059632744425,993.494506048653,
993.929379352783,994.364252656817,994.799125960758,995.233999264609,995.668872568372,
996.103745872049,996.538619175643,996.973492479157,997.408365782593,997.843239085953,
998.278112389241,998.713838387696,999.149564386151,999.584437689301,1000.01931099239,
1000.45418429541,1000.88905759838,1001.32393090129,1001.75880420414,1002.19367750695,
1002.62855080971,1003.06342411242,1003.49829741509,1003.93317071773,1004.36804402032,
1004.80291732289,1005.23779062542,1005.67351662352,1006.10924262162,1006.5441159241,
1006.97898922656,1007.41386252901,1007.84873583144,1008.28360913385,1008.71848243626,
1009.15335573866,1009.58822904106,1010.02310234346,1010.45797564586,1010.89284894827,
1011.32772225069,1011.76259555311,1012.19746885556,1012.63319485364,1013.06892085171,
1013.5037941542,1013.9386674567,1014.37354075924,1014.8084140618,1015.2432873644,
1015.67816066703,1016.1130339697,1016.54790727242,1016.98278057517,1017.41765387798,
1017.85252718084,1018.28740048375,1018.72227378671,1019.15714708974,1019.59287308813,
1020.02859908651,1020.46347238967,1020.89834569288,1021.33321899617,1021.76809229953,
1022.20296560297,1022.63783890648,1023.07271221007,1023.50758551375,1023.94245881752,
1024.37733212137,1024.81220542531,1025.24707872935,1025.68195203348,1026.11682533771,
1026.55255133672,1026.98827733573,1027.42315064016,1027.8580239447,1028.29289724934,
1028.72777055409,1029.16264385896,1029.59751716393,1030.03239046902,1030.46726377423,
1030.90213707956,1031.33701038501,1031.77188369058,1032.20675699628,1032.6416303021,
1033.07650360805,1033.51222960793,1033.94795560782,1034.38282891403,1034.81770222038,
1035.25257552685,1035.68744883347,1036.12232214022,1036.5571954471,1036.99206875413,
1037.4269420613,1037.86181536861,1038.29668867606,1038.73156198365,1039.16643529139,
1039.60130859927,1040.0361819073,1040.47190790824,1040.90763390917,1041.34250721749,
1041.77738052596,1042.21225383458,1042.64712714334,1043.08200045226,1043.95174707053,
1044.38662037989,1044.8214936894,1045.25636699906,1045.69124030886,1046.12611361882,
1046.56098692892,1046.99586023917,1047.43158624121,1047.86731224325,1048.3021855538,
1048.73705886448,1049.17193217531,1049.60680548629,1050.0416787974,1050.47655210866,
1050.91142542006,1051.78117204327,1052.21604535508,1052.65091866703,1053.0857919791,
1053.52066529131,1053.95553860365,1054.39126460673,1055.26186392239,1056.13161054793,
1057.00135717395,1057.43623048712,1057.87110380041,1058.7408504273,1059.61059705459,
1060.48034368225,1061.35094300009,1062.22154231809,1063.09128894656,1063.96103557531,
1064.83078220429,1065.70052883346,1066.57027546278,1067.44002209222,1068.3106214112,
1069.18122073019,1070.05096735972,1070.9207139892,1071.79046061859,1072.66020724785,
1073.52995387693,1074.39970050579,1075.27029982411,1076.1408991423,1077.01064577048,
1077.88039239832,1078.7501390258,1079.61988565289,1080.48963227957,1081.35937890581,
1082.22997822202,1083.100577538,1083.97032416305,1084.84007078759,1085.70981741161,
1086.5795640351,1087.44931065803,1087.88418396929,1088.31905728041,1088.75393059138,
1089.18965659365,1089.62538259591,1090.06025590659,1090.93000252753,1091.36487583778,
1091.79974914788,1092.23462245783,1092.66949576764,1093.1043690773,1093.5392423868,
1093.97411569616,1094.40898900538,1094.84386231444,1095.27873562335,1095.71360893212,
1096.14933493327,1096.58506093443,1097.0199342429,1097.45480755122,1097.88968085939,
1098.32455416742,1098.75942747531,1099.19430078305,1099.62917409064,1100.06404739809,
1100.4989207054,1100.93379401257,1101.36866731959,1101.80354062648,1102.23841393323,
1102.67328723984,1103.10901323993,1103.54473924001,1103.97961254636,1104.41448585257,
1104.84935915865,1105.2842324646,1105.71910577042,1106.15397907612,1106.58885238169,
1107.02372568714,1107.45859899246,1107.89347229767,1108.32834560276,1108.76321890774,
1109.1980922126,1109.63296551736,1110.06869151652,1110.50441751569,1110.93929082023,
1111.37416412466,1111.80903742899,1112.24391073322,1112.67878403735,1113.11365734139,
1113.54853064533,1113.98340394918,1114.41827725295,1114.85315055662,1115.28802386022,
1115.72289716374,1116.15777046717,1116.59264377053,1117.02836976903,1117.46409576752,
1117.89896907074,1118.33384237389,1118.76871567698,1119.20358898,1119.63846228297,
1120.07333558588,1120.50820888874,1120.94308219154,1121.3779554943,1121.81282879702,
1122.24770209969,1122.68257540233,1123.11744870492,1123.55232200749,1123.98804800561,
1124.42377400372,1124.85864730623,1125.29352060871,1125.72839391118,1126.16326721362,
1126.59814051605,1127.03301381847,1127.46788712088,1127.90276042328,1128.33763372568,
1128.77250702808,1129.20738033048,1129.64225363289,1130.07712693531,1130.51200023774,
1130.94772623581,1131.38345223388,1131.81832553634,1132.25319883883,1132.68807214134,
1133.12294544387,1133.55781874644,1133.99269204904,1134.42756535167,1134.86243865434,
1135.29731195706,1135.73218525982,1136.16705856263,1136.60193186548,1137.03680516839,
1137.47167847136,1137.90740446972,1138.34313046808,1138.77800377117,1139.21287707432,
1139.64775037754,1140.08262368083,1140.51749698419,1140.95237028763,1141.38724359114,
1141.82211689474,1142.25699019842,1142.69186350218,1143.12673680603,1143.56161010998,
1143.99648341401,1144.43135671814,1144.86708271711,1145.30280871607,1145.7376820204,
1146.17255532483,1146.60742862936,1147.04230193401,1147.47717523876,1147.91204854362,
1148.3469218486,1148.78179515369,1149.2166684589,1149.65154176423,1150.08641506968,
1150.52128837525,1150.95616168094,1151.39103498677,1151.82676098659,1152.26248698641,
1152.69736029249,1153.1322335987,1153.56710690504,1154.00198021152,1154.43685351813,
1154.87172682488,1155.30660013177,1155.7414734388,1156.17634674597,1156.61122005327,
1157.04609336073,1157.48096666832,1157.91583997606,1158.35071328394,1158.7864392848,
1159.22216528566,1159.65703859384,1160.09191190216,1160.52678521063,1160.96165851925,
1161.39653182801,1161.83140513693,1162.26627844599,1162.7011517552,1163.13602506456,
1163.57089837407,1164.00577168373,1164.44064499353,1164.87551830349,1165.74611761556,
1166.18184361753,1166.61671692792,1167.05159023846,1167.48646354915,1167.92133685998,
1168.35621017096,1169.22595679333,1170.09570341627,1170.53057672794,1170.96545003975,
1171.4003233517,1171.83519666377,1172.27006997598,1172.705795979,1173.57639529447,
1174.44614191977,1174.8810152326,1175.31588854555,1176.18563517179,1177.05538179847,
1177.92512842556,1178.79487505304,1179.66547437075,1180.53607368863,1181.40582031696,
1182.27556694557,1183.14531357444,1184.01506020352,1184.88480683277,1185.75455346216,
1186.62515278112,1187.4957521001,1188.36549872963,1189.23524535914,1190.10499198858,
1190.97473861791,1191.84448524708,1192.71423187606,1193.58483119448,1194.45543051277,
1195.3251771411,1196.19492376911,1197.06467039678,1197.93441702407,1198.80416365096,
1199.67391027742,1200.5445095938,1201.41510890996,1202.28485553525,1203.15460216005,
1204.02434878434,1204.89409540809,1205.76384203131,1206.1987153427,1206.63358865396,
1207.06846196508,1207.50418796741,1208.37478728058,1209.2445339018,1209.6794072122,
1210.11428052245,1210.54915383255,1210.9840271425,1211.41890045231,1211.85377376197,
1212.28864707147,1212.72352038083,1213.15839369005,1213.59326699911,1214.02814030802,
1214.46386630925,1214.89959231048,1215.3344656191,1215.76933892757,1216.20421223589,
1216.63908554406,1217.07395885209,1217.50883215998,1217.94370546771,1218.37857877531,
1218.81345208276,1219.24832539007,1219.68319869724,1220.11807200426,1220.55294531115,
1220.9878186179,1221.42354461805,1221.85927061821,1222.29414392468,1222.72901723103,
1223.16389053724,1223.59876384332,1224.03363714927,1224.46851045509,1224.90338376079,
1225.33825706636,1225.77313037181,1226.20800367713,1226.64287698234,1227.07775028743,
1227.51262359241,1227.94749689727,1228.3832228965,1228.81894889572,1229.25382220036,
1229.6886955049,1230.12356880933,1230.55844211366,1230.99331541789,1231.42818872202,
1231.86306202606,1232.29793533,1232.73280863385,1233.16768193762,1233.60255524129,
1234.03742854489,1234.4723018484,1234.90717515184,1235.34290115037,1235.7786271489,
1236.21350045219,1236.64837375541,1237.08324705856,1237.51812036165,1237.95299366467,
1238.38786696764,1238.82274027055,1239.25761357341,1239.69248687621,1240.12736017897,
1240.56223348169,1240.99710678436,1241.431980087,1241.8668533896,1242.30257938773,
1242.73830538585,1243.17317868839,1243.6080519909,1244.04292529338,1244.47779859585,
1244.91267189829,1245.34754520072,1245.78241850314,1246.21729180555,1246.65216510795,
1247.08703841035,1247.52191171275,1247.95678501515,1248.39165831756,1248.82653161998,
1249.26225761804,1249.69798361611,1250.13285691855,1250.56773022101,1251.0026035235,
1251.43747682601,1251.87235012854,1252.30722343111,1252.74209673371,1253.17697003634,
1253.61184333901,1254.04671664173,1254.48158994449,1254.9164632473,1255.35133655015,
1255.78620985306,1256.22193585139,1256.65766184973,1257.09253515275,1257.52740845584,
1257.96228175899,1258.39715506221,1258.8320283655,1259.26690166886,1259.7017749723,
1260.13664827581,1260.57152157941,1261.00639488309,1261.44126818685,1261.8761414907,
1262.31101479465,1262.74588809868,1263.1816140976,1263.61734009651,1264.05221340074,
1264.48708670507,1264.9219600095,1265.35683331403,1265.79170661868,1266.22657992343,
1266.66145322829,1267.09632653327,1267.53119983836,1267.96607314357,1268.4009464489,
1268.83581975434,1269.27069305992,1269.70556636561,1270.14129236537,1270.57701836513,
1271.01189167108,1271.44676497716,1271.88163828337,1272.31651158971,1272.75138489619,
1273.1862582028,1273.62113150955,1274.05600481644,1274.49087812347,1274.92575143063,
1275.36062473794,1275.79549804539,1276.23037135299,1276.66524466073,1277.10097066151,
1277.5366966623,1277.97156997033,1278.40644327851,1278.84131658683,1279.2761898953,
1279.71106320392,1280.14593651268,1280.5808098216,1281.01568313066,1281.45055643987,
1281.88542974923,1282.32030305874,1282.75517636839,1283.1900496782,1283.62492298815,
1284.06064899005,1284.49637499195,1284.9312483022,1285.36612161259,1285.80099492313,
1286.23586823382,1286.67074154465,1287.54048816674,1287.975361478,1288.4102347894,
1288.84510810093,1289.27998141261,1289.71485472442,1290.14972803636,1291.02032735139,
1291.89092666668,1292.32579997914,1292.76067329173,1293.19554660444,1293.63041991727,
1294.50016654328,1295.36991316974,1296.23965979663,1297.10940642392,1297.9800057415,
1298.85060505925,1299.72035168742,1300.5900983159,1301.45984494464,1302.32959157362,
1303.19933820279,1304.06908483212,1304.93968415104,1305.81028347,1306.68003009953,
1307.54977672906,1308.41952335854,1309.28926998793,1310.15901661718,1311.02876324626,
1311.89936256477,1312.76996188316,1313.63970851164,1314.50945513981,1315.37920176765,
1316.24894839514,1317.11869502223,1317.98844164891,1318.85904096546,1319.72964028179,
1320.59938690733,1321.46913353238,1322.33888015692,1323.20862678095,1323.64350009276,
1324.07837340443,1324.51324671597,1324.94812002737,1325.81871934103,1326.68931865441,
1327.12419196524,1327.55906527593,1327.99393858647,1328.42881189686,1328.86368520711,
1329.29855851721,1329.73343182716,1330.16830513697,1330.60317844663,1331.03805175614,
1331.4729250655,1331.90779837471,1332.34267168377,1332.77839768507,1333.21412368638,
1333.64899699514,1334.08387030376,1334.51874361223,1334.95361692055,1335.38849022873,
1335.82336353676,1336.25823684464,1336.69311015238,1337.12798345997,1337.56285676742,
1337.99773007473,1338.4326033819,1338.86747668892,1339.30234999581,1339.73807599603,
1340.17380199625,1340.60867530287,1341.04354860934,1341.47842191569,1341.9132952219,
1342.34816852798,1342.78304183393,1343.21791513975,1343.65278844545,1344.08766175102,
1344.52253505647,1344.95740836179,1345.392281667,1345.82715497209,1346.26202827707,
1346.69775427635,1347.13348027563,1347.56835358038,1348.00322688502,1348.43810018956,
1348.87297349399,1349.30784679832,1349.74272010255,1350.17759340668,1350.61246671072,
1351.04734001466,1351.48221331851,1351.91708662228,1352.35195992595,1352.78683322955,
1353.22170653306,1353.65743253163,1354.09315853019,1354.52803183356,1354.96290513685,
1355.39777844007,1355.83265174322,1356.26752504631,1356.70239834933,1357.1372716523,
1357.57214495521,1358.00701825807,1358.44189156087,1358.87676486363,1359.31163816635,
1359.74651146902,1360.18138477166,1360.6171107698,1361.05283676795,1361.48771007051,
1361.92258337305,1362.35745667556,1362.79232997804,1363.2272032805,1363.66207658295,
1364.09694988538,1364.5318231878,1364.96669649021,1365.40156979261,1365.83644309501,
1366.27131639741,1366.70618969981,1367.14106300222,1367.57678900028,1368.01251499834,
1368.44738830077,1368.88226160321,1369.31713490567,1369.75200820816,1370.18688151067,
1370.6217548132,1371.05662811577,1371.49150141837,1371.926374721,1372.36124802367,
1372.79612132639,1373.23099462915,1373.66586793196,1374.10074123481,1374.53646723311,
1374.97219323142,1375.40706653438,1375.84193983741,1376.2768131405,1376.71168644365,
1377.14655974687,1377.58143305016,1378.01630635352,1378.45117965696,1378.88605296047,
1379.32092626407,1379.75579956775,1380.19067287151,1380.62554617536,1381.06041947931,
1381.49614547817,1381.93187147704,1382.36674478117,1382.8016180854,1383.23649138973,
1383.67136469416,1384.10623799869,1384.54111130334,1384.97598460809,1385.41085791295,
1385.84573121793,1386.28060452302,1386.71547782823,1387.15035113356,1387.585224439,
1388.02009774458,1388.45582374427,1388.89154974397,1389.32642304979,1389.76129635574,
1390.19616966182,1390.63104296803,1391.06591627437,1391.50078958085,1391.93566288746,
1392.37053619421,1392.8054095011,1393.24028280813,1393.6751561153,1394.1100294226,
1394.54490273005,1394.97977603765,1395.41550203836,1395.85122803908,1396.28610134696,
1396.72097465499,1397.15584796317,1397.59072127149,1398.02559457996,1398.46046788858,
1398.89534119734,1399.33021450626,1399.76508781532,1400.19996112453,1400.63483443389,
1401.50458105306,1401.93945436286,1402.37518036469,1402.81090636651,1403.24577967661,
1403.68065298686,1404.11552629725,1404.5503996078,1404.98527291848,1405.85501954029,
1406.2898928514,1406.72476616266,1407.15963947406,1407.5945127856,1408.02938609727,
1408.46425940908,1409.33485872391,1410.205458039,1410.64033135134,1411.07520466381,
1411.51007797639,1411.9449512891,1412.81469791488,1413.68444454112,1414.5541911678,
1415.42393779489,1416.29453711233,1417.16513642995,1418.03488305796,1418.90462968629,
1419.77437631491,1420.64412294377,1421.51386957285,1422.38361620211,1423.25421552099,
1424.12481483992,1424.99456146943,1425.86430809896,1426.73405472847,1427.60380135791,
1428.47354798724,1429.34329461641,1430.21389393501,1431.08449325349,1431.9542398821,
1432.82398651043,1433.69373313844,1434.56347976611,1435.4332263934,1436.30297302029,
1437.17357233701,1438.04417165351,1438.91391827929,1439.78366490459,1440.65341152939,
1441.52315815367,1441.95803146562,1442.39290477743,1442.8277780891,1443.26265140064,
1444.13325071451,1445.00385002811,1445.43872333908,1445.87359664991,1446.3084699606,
1446.74334327114,1447.17821658153,1447.61308989178,1448.48283651184,1448.91770982164,
1449.3525831313,1449.78745644081,1450.22232975017,1450.65720305938,1451.09292906076,
1451.52865506214,1451.96352837105,1452.39840167982,1452.83327498843,1453.2681482969,
1453.70302160522,1454.1378949134,1454.57276822143,1455.00764152931,1455.44251483705,
1455.87738814464,1456.31226145209,1456.7471347594,1457.18200806657,1457.6168813736,
1458.05260737389,1458.48833337418,1458.92320668093,1459.35807998754,1459.79295329402,
1460.22782660036,1460.66269990657,1461.09757321265,1461.5324465186,1461.96731982443,
1462.40219313012,1462.83706643569,1463.27193974114,1463.70681304647,1464.14168635168,
1464.57655965677,1465.0122856561,1465.44801165544,1465.8828849603,1466.31775826505,
1466.7526315697,1467.18750487423,1467.62237817866,1468.05725148299,1468.49212478722,
1468.92699809135,1469.36187139539,1469.79674469933,1470.23161800319,1470.66649130695,
1471.10136461063,1471.53623791422,1471.97196391283,1472.40768991143,1472.84256321487,
1473.27743651823,1473.71230982152,1474.14718312474,1474.58205642789,1475.01692973098,
1475.451803034,1475.88667633697,1476.32154963988,1476.75642294274,1477.19129624555,
1477.62616954831,1478.06104285102,1478.4959161537,1478.93164215186,1479.36736815002,
1479.80224145262,1480.23711475519,1480.67198805772,1481.10686136023,1481.54173466272,
1481.97660796518,1482.41148126762,1482.84635457005,1483.28122787247,1483.71610117488,
1484.15097447728,1484.58584777968,1485.02072108208,1485.45559438449,1485.89132038254,
1486.32704638059,1486.76191968301,1487.19679298544,1487.63166628788,1488.06653959035,
1488.50141289283,1488.93628619534,1489.37115949787,1489.80603280044,1490.24090610304,
1490.67577940567,1491.11065270835,1491.54552601106,1491.98039931382,1492.41527261663,
1492.8509986149,1493.28672461318,1493.72159791609,1494.15647121906,1494.59134452208,
1495.02621782517,1495.46109112832,1495.89596443154,1496.33083773483,1496.76571103819,
1497.20058434163,1497.63545764515,1498.07033094874,1498.50520425242,1498.94007755618,
1499.37495086004,1499.81067685885,1500.24640285767,1500.68127616171,1501.11614946584,
1501.55102277007,1501.9858960744,1502.42076937883,1502.85564268337,1503.29051598801,
1503.72538929276,1504.16026259762,1504.5951359026,1505.03000920769,1505.4648825129,
1505.89975581823,1506.33462912368,1506.77035512331,1507.20608112294,1507.64095442864,
1508.07582773446,1508.51070104041,1508.94557434649,1509.3804476527,1509.81532095904,
1510.25019426552,1510.68506757213,1511.11994087888,1511.55481418577,1511.9896874928,
1512.42456079996,1512.85943410727,1513.29430741472,1513.73003341537,1514.16575941601,
1514.60063272375,1515.03550603163,1515.47037933966,1515.90525264784,1516.34012595616,
1516.77499926463,1517.20987257325,1517.64474588201,1518.07961919093,1518.51449249999,
1518.9493658092,1519.38423911856,1519.81911242807,1520.25398573772,1520.68971173947,
1521.12543774122,1521.56031105118,1521.99518436128,1522.43005767153,1523.29980429246,
1523.73467760315,1524.16955091398,1524.60442422495,1525.03929753607,1525.47417084733,
1525.90904415873,1526.77879078194,1527.64939009657,1528.08511609939,1528.51998941146,
1528.95486272367,1529.38973603601,1530.25948266106,1531.1292292866,1531.99897591261,
1532.86872253907,1533.73846916596,1534.60906848325,1535.47966780073,1536.34941442858,
1537.21916105675,1538.08890768523,1538.95865431398,1539.82840094295,1540.69814757212,
1541.56874689096,1542.43934620985,1543.30909283933,1544.17883946886,1545.04858609839,
1545.91833272787,1546.78807935726,1547.65782598651,1548.52842530518,1549.39902462375,
1550.26877125249,1551.13851788097,1552.00826450914,1552.87801113699,1553.74775776447,
1554.61750439156,1555.48810370844,1556.35870302511,1557.22844965112,1558.09819627666,
1558.96794290171,1559.83768952626,1560.27256283834,1560.70743615028,1561.57718277377,
1562.44778208785,1563.31838140165,1563.75325471277,1564.18812802374,1564.62300133457,
1565.05787464526,1565.9276212662,1566.79736788655,1567.2322411965,1567.66711450631,
1568.10198781596,1568.53686112547,1568.97173443483,1569.40746043628,1569.84318643774,
1570.2780597468,1570.71293305571,1571.14780636448,1571.5826796731,1572.01755298157,
1572.45242628989,1572.88729959806,1573.32217290609,1573.75704621397,1574.19191952171,
1574.62679282931,1575.06166613676,1575.49653944407,1575.93141275123,1576.36713875159,
1576.80286475195,1577.23773805884,1577.67261136559,1578.1074846722,1578.54235797868,
1578.97723128502,1579.41210459124,1579.84697789732,1580.28185120327,1580.71672450909,
1581.15159781478,1581.58647112036,1582.0213444258,1582.45621773113,1582.89109103634,
1583.32681703573,1583.76254303513,1584.1974163401,1584.63228964497,1585.06716294972,
1585.50203625436,1585.9369095589,1586.37178286333,1586.80665616766,1587.24152947189,
1587.67640277602,1588.11127608005,1588.546149384,1588.98102268785,1589.41589599161,
1589.85076929529,1590.28649529394,1590.72222129258,1591.1570945961,1591.59196789953,
1592.0268412029,1592.46171450619,1592.8965878094,1593.33146111256,1593.76633441564,
1594.20120771867,1594.63608102164,1595.07095432455,1595.50582762741,1595.94070093021,
1596.37557423297,1596.81044753569,1597.24617353387,1597.68189953206,1598.11677283469,
1598.55164613729,1598.98651943985,1599.42139274239,1599.8562660449,1600.29113934738,
1600.72601264985,1601.16088595229,1601.59575925472,1602.03063255714,1602.46550585955,
1602.90037916195,1603.33525246435,1603.77012576675,1604.2058517648,1604.64157776285,
1605.07645106526,1605.51132436768,1605.94619767011,1606.38107097255,1606.81594427502,
1607.2508175775,1607.68569088001,1608.12056418254,1608.55543748511,1608.99031078771,
1609.42518409034,1609.86005739302,1610.29493069573,1610.72980399849,1611.16552999674,
1611.60125599499,1612.03612929785,1612.47100260076,1612.90587590373,1613.34074920675,
1613.77562250984,1614.21049581299,1614.64536911621,1615.0802424195,1615.51511572286,
1615.9499890263,1616.38486232981,1616.81973563341,1617.25460893709,1617.68948224085,
1618.12520823963,1618.5609342384,1618.99580754234,1619.43068084638,1619.86555415051,
1620.30042745474,1620.73530075907,1621.1701740635,1621.60504736804,1622.03992067268,
1622.47479397743,1622.90966728229,1623.34454058727,1623.77941389236,1624.21428719757,
1624.6491605029,1625.08488650247,1625.52061250204,1625.95548580761,1626.39035911331,
1626.82523241913,1627.26010572508,1627.69497903116,1628.12985233737,1628.56472564372,
1628.99959895019,1629.43447225681,1629.86934556356,1630.30421887044,1630.73909217747,
1631.17396548464,1631.60883879195,1632.04456479252,1632.48029079309,1632.91516410068,
1633.35003740842,1633.78491071631,1634.21978402433,1634.65465733251,1635.08953064083,
1635.5244039493,1635.95927725792,1636.39415056668,1636.8290238756,1637.26389718466,
1637.69877049387,1638.13364380323,1638.56851711274,1639.00424311442,1639.43996911609,
1639.8748424259,1640.30971573585,1640.74458904595,1641.6143356666,1642.04920897714,
1642.48408228782,1642.91895559865,1643.35382890963,1643.78870222074,1644.223575532,
1645.09332215494,1645.52819546661,1645.96392146936,1646.39964747212,1646.83452078406,
1647.26939409614,1647.70426740834,1648.57401403314,1649.44376065844,1650.31350728422,
1650.74838059729,1651.18325391046,1652.05300053714,1652.92359985428,1653.79419917162,
1654.66394579929,1655.5336924273,1656.40343905563,1657.27318568424,1658.14293231311,
1659.01267894219,1659.88327826096,1660.75387757982,1661.62362420926,1662.49337083877,
1663.3631174683,1664.23286409781,1665.10261072725,1665.97235735658,1666.84295667531,
1667.71355599396,1668.58330262282,1669.45304925143,1670.32279587976,1671.19254250778,
1672.06228913544,1672.93203576273,1673.80263507977,1674.6732343966,1675.54298102284,
1676.41272764862,1677.28247427392,1678.15222089872,1679.021967523,1679.89171414676,
1680.76231346105,1681.19803946366,1681.63291277506,1682.06778608632,1682.50265939743,
1682.93753270841,1683.37240601924,1684.24215264047,1684.67702595086,1685.11189926111,
1685.54677257121,1685.98164588116,1686.41651919097,1686.85139250063,1687.28626581014,
1687.72199181166,1688.15771781319,1688.5925911224,1689.02746443146,1689.46233774038,
1689.89721104914,1690.33208435776,1690.76695766623,1691.20183097455,1691.63670428272,
1692.07157759075,1692.50645089864,1692.94132420637,1693.37619751397,1693.81107082142,
1694.24594412873,1694.68167012916,1695.11739612959,1695.55226943662,1695.9871427435,
1696.42201605025,1696.85688935687,1697.29176266334,1697.72663596969,1698.1615092759,
1698.59638258198,1699.03125588793,1699.46612919375,1699.90100249945,1700.33587580502,
1700.77074911047,1701.20562241579,1701.64134841525,1702.0770744147,1702.51194771979,
1702.94682102476,1703.38169432963,1703.81656763438,1704.25144093902,1704.68631424356,
1705.12118754799,1705.55606085232,1705.99093415655,1706.42580746068,1706.86068076471,
1707.29555406866,1707.73042737251,1708.16530067627,1708.60102667496,1709.03675267365,
1709.47162597724,1709.90649928076,1710.34137258419,1710.77624588756,1711.21111919085,
1711.64599249406,1712.08086579722,1712.5157391003,1712.95061240333,1713.3854857063,
1713.82035900921,1714.25523231207,1714.69010561487,1715.12497891763,1715.56070491584,
1715.99643091404,1716.43130421671,1716.86617751935,1717.30105082195,1717.73592412451,
1718.17079742705,1718.60567072956,1719.04054403204,1719.4754173345,1719.91029063695,
1720.34516393938,1720.7800372418,1721.21491054421,1721.64978384661,1722.08465714901,
1722.52038314706,1722.9561091451,1723.39098244751,1723.82585574992,1724.26072905233,
1724.69560235476,1725.13047565721,1725.56534895967,1726.00022226216,1726.43509556467,
1726.8699688672,1727.30484216977,1727.73971547236,1728.174588775,1728.60946207767,
1729.04433538039,1729.48006137861,1729.91578737684,1730.35066067965,1730.78553398251,
1731.22040728542,1731.65528058838,1732.09015389141,1732.5250271945,1732.95990049765,
1733.39477380087,1733.82964710416,1734.26452040752,1734.69939371096,1735.13426701447,
1735.56914031807,1736.00401362175,1736.43973962048,1736.8754656192,1737.31033892306,
1737.745212227,1738.18008553104,1738.61495883517,1739.0498321394,1739.48470544373,
1739.91957874816,1740.35445205269,1740.78932535734,1741.22419866209,1741.65907196695,
1742.09394527193,1742.52881857702,1742.96369188223,1743.39941788174,1743.83514388125,
1744.2700171867,1744.70489049227,1745.13976379797,1745.57463710379,1746.00951040974,
1746.44438371582,1746.87925702203,1747.31413032837,1747.74900363485,1748.18387694146,
1748.61875024821,1749.0536235551,1749.48849686213,1749.92337016929,1750.3590961698,
1750.7948221703,1751.22969547775,1751.66456878534,1752.09944209308,1752.53431540096,
1752.96918870899,1753.40406201717,1753.83893532549,1754.27380863396,1754.70868194258,
1755.14355525134,1755.57842856026,1756.01330186932,1756.44817517853,1756.88304848789,
1757.31877448949,1757.75450049109,1758.18937380075,1759.05912042051,1759.49399373061,
1759.92886704086,1760.36374035125,1760.79861366179,1761.23348697248,1761.66836028331,
1762.10323359429,1762.5381069054,1763.40785352806,1763.8427268396,1764.27845284228,
1764.71417884496,1765.14905215677,1765.58392546872,1766.0187987808,1766.88854540534,
1767.75829203039,1768.1931653431,1768.62803865593,1769.06291196888,1769.49778528195,
1770.36753190841,1771.2381312254,1772.10873054259,1772.97847717007,1773.84822379791,
1774.71797042609,1775.58771705456,1776.45746368331,1777.32721031228,1778.19780963089,
1779.06840894783,1779.93815555508,1780.80790201176,1781.67764871408),(-1.76619037896906,
-1.18309518948453),.UNSPECIFIED.) ;
#821=B_SPLINE_SURFACE_WITH_KNOTS('',3,1,((#34258,#34259),(#34260,#34261),
(#34262,#34263),(#34264,#34265),(#34266,#34267),(#34268,#34269),(#34270,
#34271),(#34272,#34273),(#34274,#34275),(#34276,#34277),(#34278,#34279),
(#34280,#34281),(#34282,#34283),(#34284,#34285),(#34286,#34287),(#34288,
#34289),(#34290,#34291),(#34292,#34293),(#34294,#34295),(#34296,#34297),
(#34298,#34299),(#34300,#34301),(#34302,#34303),(#34304,#34305),(#34306,
#34307),(#34308,#34309),(#34310,#34311),(#34312,#34313),(#34314,#34315),
(#34316,#34317),(#34318,#34319),(#34320,#34321),(#34322,#34323),(#34324,
#34325),(#34326,#34327),(#34328,#34329),(#34330,#34331),(#34332,#34333),
(#34334,#34335),(#34336,#34337),(#34338,#34339),(#34340,#34341),(#34342,
#34343),(#34344,#34345),(#34346,#34347),(#34348,#34349),(#34350,#34351),
(#34352,#34353),(#34354,#34355),(#34356,#34357),(#34358,#34359),(#34360,
#34361),(#34362,#34363),(#34364,#34365),(#34366,#34367),(#34368,#34369),
(#34370,#34371),(#34372,#34373),(#34374,#34375),(#34376,#34377),(#34378,
#34379),(#34380,#34381),(#34382,#34383),(#34384,#34385),(#34386,#34387),
(#34388,#34389),(#34390,#34391),(#34392,#34393),(#34394,#34395),(#34396,
#34397),(#34398,#34399),(#34400,#34401),(#34402,#34403),(#34404,#34405),
(#34406,#34407),(#34408,#34409),(#34410,#34411),(#34412,#34413),(#34414,
#34415),(#34416,#34417),(#34418,#34419),(#34420,#34421),(#34422,#34423),
(#34424,#34425),(#34426,#34427),(#34428,#34429),(#34430,#34431),(#34432,
#34433),(#34434,#34435),(#34436,#34437),(#34438,#34439),(#34440,#34441),
(#34442,#34443),(#34444,#34445),(#34446,#34447),(#34448,#34449),(#34450,
#34451),(#34452,#34453),(#34454,#34455),(#34456,#34457),(#34458,#34459),
(#34460,#34461),(#34462,#34463),(#34464,#34465),(#34466,#34467),(#34468,
#34469),(#34470,#34471),(#34472,#34473),(#34474,#34475),(#34476,#34477),
(#34478,#34479),(#34480,#34481),(#34482,#34483),(#34484,#34485),(#34486,
#34487),(#34488,#34489),(#34490,#34491),(#34492,#34493),(#34494,#34495),
(#34496,#34497),(#34498,#34499),(#34500,#34501),(#34502,#34503),(#34504,
#34505),(#34506,#34507),(#34508,#34509),(#34510,#34511),(#34512,#34513),
(#34514,#34515),(#34516,#34517),(#34518,#34519),(#34520,#34521),(#34522,
#34523),(#34524,#34525),(#34526,#34527),(#34528,#34529),(#34530,#34531),
(#34532,#34533),(#34534,#34535),(#34536,#34537),(#34538,#34539),(#34540,
#34541),(#34542,#34543),(#34544,#34545),(#34546,#34547),(#34548,#34549),
(#34550,#34551),(#34552,#34553),(#34554,#34555),(#34556,#34557),(#34558,
#34559),(#34560,#34561),(#34562,#34563),(#34564,#34565),(#34566,#34567),
(#34568,#34569),(#34570,#34571),(#34572,#34573),(#34574,#34575),(#34576,
#34577),(#34578,#34579),(#34580,#34581),(#34582,#34583),(#34584,#34585),
(#34586,#34587),(#34588,#34589),(#34590,#34591),(#34592,#34593),(#34594,
#34595),(#34596,#34597),(#34598,#34599),(#34600,#34601),(#34602,#34603),
(#34604,#34605),(#34606,#34607),(#34608,#34609),(#34610,#34611),(#34612,
#34613),(#34614,#34615),(#34616,#34617),(#34618,#34619),(#34620,#34621),
(#34622,#34623),(#34624,#34625),(#34626,#34627),(#34628,#34629),(#34630,
#34631),(#34632,#34633),(#34634,#34635),(#34636,#34637),(#34638,#34639),
(#34640,#34641),(#34642,#34643),(#34644,#34645),(#34646,#34647),(#34648,
#34649),(#34650,#34651),(#34652,#34653),(#34654,#34655),(#34656,#34657),
(#34658,#34659),(#34660,#34661),(#34662,#34663),(#34664,#34665),(#34666,
#34667),(#34668,#34669),(#34670,#34671),(#34672,#34673),(#34674,#34675),
(#34676,#34677),(#34678,#34679),(#34680,#34681),(#34682,#34683),(#34684,
#34685),(#34686,#34687),(#34688,#34689),(#34690,#34691),(#34692,#34693),
(#34694,#34695),(#34696,#34697),(#34698,#34699),(#34700,#34701),(#34702,
#34703),(#34704,#34705),(#34706,#34707),(#34708,#34709),(#34710,#34711),
(#34712,#34713),(#34714,#34715),(#34716,#34717),(#34718,#34719),(#34720,
#34721),(#34722,#34723),(#34724,#34725),(#34726,#34727),(#34728,#34729),
(#34730,#34731),(#34732,#34733),(#34734,#34735),(#34736,#34737),(#34738,
#34739),(#34740,#34741),(#34742,#34743),(#34744,#34745),(#34746,#34747),
(#34748,#34749),(#34750,#34751),(#34752,#34753),(#34754,#34755),(#34756,
#34757),(#34758,#34759),(#34760,#34761),(#34762,#34763),(#34764,#34765),
(#34766,#34767),(#34768,#34769),(#34770,#34771),(#34772,#34773),(#34774,
#34775),(#34776,#34777),(#34778,#34779),(#34780,#34781),(#34782,#34783),
(#34784,#34785),(#34786,#34787),(#34788,#34789),(#34790,#34791),(#34792,
#34793),(#34794,#34795),(#34796,#34797),(#34798,#34799),(#34800,#34801),
(#34802,#34803),(#34804,#34805),(#34806,#34807),(#34808,#34809),(#34810,
#34811),(#34812,#34813),(#34814,#34815),(#34816,#34817),(#34818,#34819),
(#34820,#34821),(#34822,#34823),(#34824,#34825),(#34826,#34827),(#34828,
#34829),(#34830,#34831),(#34832,#34833),(#34834,#34835),(#34836,#34837),
(#34838,#34839),(#34840,#34841),(#34842,#34843),(#34844,#34845),(#34846,
#34847),(#34848,#34849),(#34850,#34851),(#34852,#34853),(#34854,#34855),
(#34856,#34857),(#34858,#34859),(#34860,#34861),(#34862,#34863),(#34864,
#34865),(#34866,#34867),(#34868,#34869),(#34870,#34871),(#34872,#34873),
(#34874,#34875),(#34876,#34877),(#34878,#34879),(#34880,#34881),(#34882,
#34883),(#34884,#34885),(#34886,#34887),(#34888,#34889),(#34890,#34891),
(#34892,#34893),(#34894,#34895),(#34896,#34897),(#34898,#34899),(#34900,
#34901),(#34902,#34903),(#34904,#34905),(#34906,#34907),(#34908,#34909),
(#34910,#34911),(#34912,#34913),(#34914,#34915),(#34916,#34917),(#34918,
#34919),(#34920,#34921),(#34922,#34923),(#34924,#34925),(#34926,#34927),
(#34928,#34929),(#34930,#34931),(#34932,#34933),(#34934,#34935),(#34936,
#34937),(#34938,#34939),(#34940,#34941),(#34942,#34943),(#34944,#34945),
(#34946,#34947),(#34948,#34949),(#34950,#34951),(#34952,#34953),(#34954,
#34955),(#34956,#34957),(#34958,#34959),(#34960,#34961),(#34962,#34963),
(#34964,#34965),(#34966,#34967),(#34968,#34969),(#34970,#34971),(#34972,
#34973),(#34974,#34975),(#34976,#34977),(#34978,#34979),(#34980,#34981),
(#34982,#34983),(#34984,#34985),(#34986,#34987),(#34988,#34989),(#34990,
#34991),(#34992,#34993),(#34994,#34995),(#34996,#34997),(#34998,#34999),
(#35000,#35001),(#35002,#35003),(#35004,#35005),(#35006,#35007),(#35008,
#35009),(#35010,#35011),(#35012,#35013),(#35014,#35015),(#35016,#35017),
(#35018,#35019),(#35020,#35021),(#35022,#35023),(#35024,#35025),(#35026,
#35027),(#35028,#35029),(#35030,#35031),(#35032,#35033),(#35034,#35035),
(#35036,#35037),(#35038,#35039),(#35040,#35041),(#35042,#35043),(#35044,
#35045),(#35046,#35047),(#35048,#35049),(#35050,#35051),(#35052,#35053),
(#35054,#35055),(#35056,#35057),(#35058,#35059),(#35060,#35061),(#35062,
#35063),(#35064,#35065),(#35066,#35067),(#35068,#35069),(#35070,#35071),
(#35072,#35073),(#35074,#35075),(#35076,#35077),(#35078,#35079),(#35080,
#35081),(#35082,#35083),(#35084,#35085),(#35086,#35087),(#35088,#35089),
(#35090,#35091),(#35092,#35093),(#35094,#35095),(#35096,#35097),(#35098,
#35099),(#35100,#35101),(#35102,#35103),(#35104,#35105),(#35106,#35107),
(#35108,#35109),(#35110,#35111),(#35112,#35113),(#35114,#35115),(#35116,
#35117),(#35118,#35119),(#35120,#35121),(#35122,#35123),(#35124,#35125),
(#35126,#35127),(#35128,#35129),(#35130,#35131),(#35132,#35133),(#35134,
#35135),(#35136,#35137),(#35138,#35139),(#35140,#35141),(#35142,#35143),
(#35144,#35145),(#35146,#35147),(#35148,#35149),(#35150,#35151),(#35152,
#35153),(#35154,#35155),(#35156,#35157),(#35158,#35159),(#35160,#35161),
(#35162,#35163),(#35164,#35165),(#35166,#35167),(#35168,#35169),(#35170,
#35171),(#35172,#35173),(#35174,#35175),(#35176,#35177),(#35178,#35179),
(#35180,#35181),(#35182,#35183),(#35184,#35185),(#35186,#35187),(#35188,
#35189),(#35190,#35191),(#35192,#35193),(#35194,#35195),(#35196,#35197),
(#35198,#35199),(#35200,#35201),(#35202,#35203),(#35204,#35205),(#35206,
#35207),(#35208,#35209),(#35210,#35211),(#35212,#35213),(#35214,#35215),
(#35216,#35217),(#35218,#35219),(#35220,#35221),(#35222,#35223),(#35224,
#35225),(#35226,#35227),(#35228,#35229),(#35230,#35231),(#35232,#35233),
(#35234,#35235),(#35236,#35237),(#35238,#35239),(#35240,#35241),(#35242,
#35243),(#35244,#35245),(#35246,#35247),(#35248,#35249),(#35250,#35251),
(#35252,#35253),(#35254,#35255),(#35256,#35257),(#35258,#35259),(#35260,
#35261),(#35262,#35263),(#35264,#35265),(#35266,#35267),(#35268,#35269),
(#35270,#35271),(#35272,#35273),(#35274,#35275),(#35276,#35277),(#35278,
#35279),(#35280,#35281),(#35282,#35283),(#35284,#35285),(#35286,#35287),
(#35288,#35289),(#35290,#35291),(#35292,#35293),(#35294,#35295),(#35296,
#35297),(#35298,#35299),(#35300,#35301),(#35302,#35303),(#35304,#35305),
(#35306,#35307),(#35308,#35309),(#35310,#35311),(#35312,#35313),(#35314,
#35315),(#35316,#35317),(#35318,#35319),(#35320,#35321),(#35322,#35323),
(#35324,#35325),(#35326,#35327),(#35328,#35329),(#35330,#35331),(#35332,
#35333),(#35334,#35335),(#35336,#35337),(#35338,#35339),(#35340,#35341),
(#35342,#35343),(#35344,#35345),(#35346,#35347),(#35348,#35349),(#35350,
#35351),(#35352,#35353),(#35354,#35355),(#35356,#35357),(#35358,#35359),
(#35360,#35361),(#35362,#35363),(#35364,#35365),(#35366,#35367),(#35368,
#35369),(#35370,#35371),(#35372,#35373),(#35374,#35375),(#35376,#35377),
(#35378,#35379),(#35380,#35381),(#35382,#35383),(#35384,#35385),(#35386,
#35387),(#35388,#35389),(#35390,#35391),(#35392,#35393),(#35394,#35395),
(#35396,#35397),(#35398,#35399),(#35400,#35401),(#35402,#35403),(#35404,
#35405),(#35406,#35407),(#35408,#35409),(#35410,#35411),(#35412,#35413),
(#35414,#35415),(#35416,#35417),(#35418,#35419),(#35420,#35421),(#35422,
#35423),(#35424,#35425),(#35426,#35427),(#35428,#35429),(#35430,#35431),
(#35432,#35433),(#35434,#35435),(#35436,#35437),(#35438,#35439),(#35440,
#35441),(#35442,#35443),(#35444,#35445),(#35446,#35447),(#35448,#35449),
(#35450,#35451),(#35452,#35453),(#35454,#35455),(#35456,#35457),(#35458,
#35459),(#35460,#35461),(#35462,#35463),(#35464,#35465),(#35466,#35467),
(#35468,#35469),(#35470,#35471),(#35472,#35473),(#35474,#35475),(#35476,
#35477),(#35478,#35479),(#35480,#35481),(#35482,#35483),(#35484,#35485),
(#35486,#35487),(#35488,#35489),(#35490,#35491),(#35492,#35493),(#35494,
#35495),(#35496,#35497),(#35498,#35499),(#35500,#35501),(#35502,#35503),
(#35504,#35505),(#35506,#35507),(#35508,#35509),(#35510,#35511),(#35512,
#35513),(#35514,#35515),(#35516,#35517),(#35518,#35519),(#35520,#35521),
(#35522,#35523),(#35524,#35525),(#35526,#35527),(#35528,#35529),(#35530,
#35531),(#35532,#35533),(#35534,#35535),(#35536,#35537),(#35538,#35539),
(#35540,#35541),(#35542,#35543),(#35544,#35545),(#35546,#35547),(#35548,
#35549),(#35550,#35551),(#35552,#35553),(#35554,#35555),(#35556,#35557),
(#35558,#35559),(#35560,#35561),(#35562,#35563),(#35564,#35565),(#35566,
#35567),(#35568,#35569),(#35570,#35571),(#35572,#35573),(#35574,#35575),
(#35576,#35577),(#35578,#35579),(#35580,#35581),(#35582,#35583),(#35584,
#35585),(#35586,#35587),(#35588,#35589),(#35590,#35591),(#35592,#35593),
(#35594,#35595),(#35596,#35597),(#35598,#35599),(#35600,#35601),(#35602,
#35603),(#35604,#35605),(#35606,#35607),(#35608,#35609),(#35610,#35611),
(#35612,#35613),(#35614,#35615),(#35616,#35617),(#35618,#35619),(#35620,
#35621),(#35622,#35623),(#35624,#35625),(#35626,#35627),(#35628,#35629),
(#35630,#35631),(#35632,#35633),(#35634,#35635),(#35636,#35637),(#35638,
#35639),(#35640,#35641),(#35642,#35643),(#35644,#35645),(#35646,#35647),
(#35648,#35649),(#35650,#35651),(#35652,#35653),(#35654,#35655),(#35656,
#35657),(#35658,#35659),(#35660,#35661),(#35662,#35663),(#35664,#35665),
(#35666,#35667),(#35668,#35669),(#35670,#35671),(#35672,#35673),(#35674,
#35675),(#35676,#35677),(#35678,#35679),(#35680,#35681),(#35682,#35683),
(#35684,#35685),(#35686,#35687),(#35688,#35689),(#35690,#35691),(#35692,
#35693),(#35694,#35695),(#35696,#35697),(#35698,#35699),(#35700,#35701),
(#35702,#35703),(#35704,#35705),(#35706,#35707),(#35708,#35709),(#35710,
#35711),(#35712,#35713),(#35714,#35715),(#35716,#35717),(#35718,#35719),
(#35720,#35721),(#35722,#35723),(#35724,#35725),(#35726,#35727),(#35728,
#35729),(#35730,#35731),(#35732,#35733),(#35734,#35735),(#35736,#35737),
(#35738,#35739),(#35740,#35741),(#35742,#35743),(#35744,#35745),(#35746,
#35747),(#35748,#35749),(#35750,#35751),(#35752,#35753),(#35754,#35755),
(#35756,#35757),(#35758,#35759),(#35760,#35761),(#35762,#35763),(#35764,
#35765),(#35766,#35767),(#35768,#35769),(#35770,#35771),(#35772,#35773),
(#35774,#35775),(#35776,#35777),(#35778,#35779),(#35780,#35781),(#35782,
#35783),(#35784,#35785),(#35786,#35787),(#35788,#35789),(#35790,#35791),
(#35792,#35793),(#35794,#35795),(#35796,#35797),(#35798,#35799),(#35800,
#35801),(#35802,#35803),(#35804,#35805),(#35806,#35807),(#35808,#35809),
(#35810,#35811),(#35812,#35813),(#35814,#35815),(#35816,#35817),(#35818,
#35819),(#35820,#35821),(#35822,#35823),(#35824,#35825),(#35826,#35827),
(#35828,#35829),(#35830,#35831),(#35832,#35833),(#35834,#35835),(#35836,
#35837),(#35838,#35839),(#35840,#35841),(#35842,#35843),(#35844,#35845),
(#35846,#35847),(#35848,#35849),(#35850,#35851),(#35852,#35853),(#35854,
#35855),(#35856,#35857),(#35858,#35859),(#35860,#35861),(#35862,#35863),
(#35864,#35865),(#35866,#35867),(#35868,#35869),(#35870,#35871),(#35872,
#35873),(#35874,#35875),(#35876,#35877),(#35878,#35879),(#35880,#35881),
(#35882,#35883),(#35884,#35885),(#35886,#35887),(#35888,#35889),(#35890,
#35891),(#35892,#35893),(#35894,#35895),(#35896,#35897),(#35898,#35899),
(#35900,#35901),(#35902,#35903),(#35904,#35905),(#35906,#35907),(#35908,
#35909),(#35910,#35911),(#35912,#35913),(#35914,#35915),(#35916,#35917),
(#35918,#35919),(#35920,#35921),(#35922,#35923),(#35924,#35925),(#35926,
#35927),(#35928,#35929),(#35930,#35931),(#35932,#35933),(#35934,#35935),
(#35936,#35937),(#35938,#35939),(#35940,#35941),(#35942,#35943),(#35944,
#35945),(#35946,#35947),(#35948,#35949),(#35950,#35951),(#35952,#35953),
(#35954,#35955),(#35956,#35957),(#35958,#35959),(#35960,#35961),(#35962,
#35963),(#35964,#35965),(#35966,#35967),(#35968,#35969),(#35970,#35971),
(#35972,#35973),(#35974,#35975),(#35976,#35977),(#35978,#35979),(#35980,
#35981),(#35982,#35983),(#35984,#35985),(#35986,#35987),(#35988,#35989),
(#35990,#35991),(#35992,#35993),(#35994,#35995),(#35996,#35997),(#35998,
#35999),(#36000,#36001),(#36002,#36003),(#36004,#36005),(#36006,#36007),
(#36008,#36009),(#36010,#36011),(#36012,#36013),(#36014,#36015),(#36016,
#36017),(#36018,#36019),(#36020,#36021),(#36022,#36023),(#36024,#36025),
(#36026,#36027),(#36028,#36029),(#36030,#36031),(#36032,#36033),(#36034,
#36035),(#36036,#36037),(#36038,#36039),(#36040,#36041),(#36042,#36043),
(#36044,#36045),(#36046,#36047),(#36048,#36049),(#36050,#36051),(#36052,
#36053),(#36054,#36055),(#36056,#36057),(#36058,#36059),(#36060,#36061),
(#36062,#36063),(#36064,#36065),(#36066,#36067),(#36068,#36069),(#36070,
#36071),(#36072,#36073),(#36074,#36075),(#36076,#36077),(#36078,#36079),
(#36080,#36081),(#36082,#36083),(#36084,#36085),(#36086,#36087),(#36088,
#36089),(#36090,#36091),(#36092,#36093),(#36094,#36095),(#36096,#36097),
(#36098,#36099),(#36100,#36101),(#36102,#36103),(#36104,#36105),(#36106,
#36107),(#36108,#36109),(#36110,#36111),(#36112,#36113),(#36114,#36115),
(#36116,#36117),(#36118,#36119),(#36120,#36121),(#36122,#36123),(#36124,
#36125),(#36126,#36127),(#36128,#36129),(#36130,#36131),(#36132,#36133),
(#36134,#36135),(#36136,#36137),(#36138,#36139),(#36140,#36141),(#36142,
#36143),(#36144,#36145),(#36146,#36147),(#36148,#36149),(#36150,#36151),
(#36152,#36153),(#36154,#36155),(#36156,#36157),(#36158,#36159),(#36160,
#36161),(#36162,#36163),(#36164,#36165),(#36166,#36167),(#36168,#36169),
(#36170,#36171),(#36172,#36173),(#36174,#36175),(#36176,#36177),(#36178,
#36179),(#36180,#36181),(#36182,#36183),(#36184,#36185),(#36186,#36187),
(#36188,#36189),(#36190,#36191),(#36192,#36193),(#36194,#36195),(#36196,
#36197),(#36198,#36199),(#36200,#36201),(#36202,#36203),(#36204,#36205),
(#36206,#36207),(#36208,#36209),(#36210,#36211),(#36212,#36213),(#36214,
#36215),(#36216,#36217),(#36218,#36219),(#36220,#36221),(#36222,#36223),
(#36224,#36225),(#36226,#36227),(#36228,#36229),(#36230,#36231),(#36232,
#36233),(#36234,#36235),(#36236,#36237),(#36238,#36239),(#36240,#36241),
(#36242,#36243),(#36244,#36245),(#36246,#36247),(#36248,#36249),(#36250,
#36251),(#36252,#36253),(#36254,#36255),(#36256,#36257),(#36258,#36259),
(#36260,#36261),(#36262,#36263),(#36264,#36265),(#36266,#36267),(#36268,
#36269),(#36270,#36271),(#36272,#36273),(#36274,#36275),(#36276,#36277),
(#36278,#36279),(#36280,#36281),(#36282,#36283),(#36284,#36285),(#36286,
#36287),(#36288,#36289),(#36290,#36291),(#36292,#36293),(#36294,#36295),
(#36296,#36297),(#36298,#36299),(#36300,#36301),(#36302,#36303),(#36304,
#36305),(#36306,#36307),(#36308,#36309),(#36310,#36311),(#36312,#36313),
(#36314,#36315),(#36316,#36317),(#36318,#36319),(#36320,#36321),(#36322,
#36323),(#36324,#36325),(#36326,#36327),(#36328,#36329),(#36330,#36331),
(#36332,#36333),(#36334,#36335),(#36336,#36337),(#36338,#36339),(#36340,
#36341),(#36342,#36343),(#36344,#36345),(#36346,#36347),(#36348,#36349),
(#36350,#36351),(#36352,#36353),(#36354,#36355),(#36356,#36357),(#36358,
#36359),(#36360,#36361),(#36362,#36363),(#36364,#36365),(#36366,#36367),
(#36368,#36369),(#36370,#36371),(#36372,#36373),(#36374,#36375),(#36376,
#36377),(#36378,#36379),(#36380,#36381),(#36382,#36383),(#36384,#36385),
(#36386,#36387),(#36388,#36389),(#36390,#36391),(#36392,#36393),(#36394,
#36395),(#36396,#36397),(#36398,#36399),(#36400,#36401),(#36402,#36403),
(#36404,#36405),(#36406,#36407),(#36408,#36409),(#36410,#36411),(#36412,
#36413),(#36414,#36415),(#36416,#36417),(#36418,#36419),(#36420,#36421),
(#36422,#36423),(#36424,#36425),(#36426,#36427),(#36428,#36429),(#36430,
#36431),(#36432,#36433),(#36434,#36435),(#36436,#36437),(#36438,#36439),
(#36440,#36441),(#36442,#36443),(#36444,#36445),(#36446,#36447),(#36448,
#36449),(#36450,#36451),(#36452,#36453),(#36454,#36455),(#36456,#36457),
(#36458,#36459),(#36460,#36461),(#36462,#36463),(#36464,#36465),(#36466,
#36467),(#36468,#36469),(#36470,#36471),(#36472,#36473),(#36474,#36475),
(#36476,#36477),(#36478,#36479),(#36480,#36481),(#36482,#36483),(#36484,
#36485),(#36486,#36487),(#36488,#36489),(#36490,#36491),(#36492,#36493),
(#36494,#36495),(#36496,#36497),(#36498,#36499),(#36500,#36501),(#36502,
#36503),(#36504,#36505),(#36506,#36507),(#36508,#36509),(#36510,#36511),
(#36512,#36513),(#36514,#36515),(#36516,#36517),(#36518,#36519),(#36520,
#36521),(#36522,#36523),(#36524,#36525),(#36526,#36527),(#36528,#36529),
(#36530,#36531),(#36532,#36533),(#36534,#36535),(#36536,#36537),(#36538,
#36539),(#36540,#36541),(#36542,#36543),(#36544,#36545),(#36546,#36547),
(#36548,#36549),(#36550,#36551),(#36552,#36553),(#36554,#36555),(#36556,
#36557),(#36558,#36559),(#36560,#36561),(#36562,#36563),(#36564,#36565),
(#36566,#36567),(#36568,#36569),(#36570,#36571),(#36572,#36573),(#36574,
#36575),(#36576,#36577),(#36578,#36579),(#36580,#36581),(#36582,#36583),
(#36584,#36585),(#36586,#36587),(#36588,#36589),(#36590,#36591),(#36592,
#36593),(#36594,#36595),(#36596,#36597),(#36598,#36599),(#36600,#36601),
(#36602,#36603),(#36604,#36605),(#36606,#36607),(#36608,#36609),(#36610,
#36611),(#36612,#36613),(#36614,#36615),(#36616,#36617),(#36618,#36619),
(#36620,#36621),(#36622,#36623),(#36624,#36625),(#36626,#36627),(#36628,
#36629),(#36630,#36631),(#36632,#36633),(#36634,#36635),(#36636,#36637),
(#36638,#36639),(#36640,#36641),(#36642,#36643),(#36644,#36645),(#36646,
#36647),(#36648,#36649),(#36650,#36651),(#36652,#36653),(#36654,#36655),
(#36656,#36657),(#36658,#36659),(#36660,#36661),(#36662,#36663),(#36664,
#36665),(#36666,#36667),(#36668,#36669),(#36670,#36671),(#36672,#36673),
(#36674,#36675),(#36676,#36677),(#36678,#36679),(#36680,#36681),(#36682,
#36683),(#36684,#36685),(#36686,#36687),(#36688,#36689),(#36690,#36691),
(#36692,#36693),(#36694,#36695),(#36696,#36697),(#36698,#36699),(#36700,
#36701),(#36702,#36703),(#36704,#36705),(#36706,#36707),(#36708,#36709),
(#36710,#36711),(#36712,#36713),(#36714,#36715),(#36716,#36717),(#36718,
#36719),(#36720,#36721),(#36722,#36723),(#36724,#36725),(#36726,#36727),
(#36728,#36729),(#36730,#36731),(#36732,#36733),(#36734,#36735),(#36736,
#36737),(#36738,#36739),(#36740,#36741),(#36742,#36743),(#36744,#36745),
(#36746,#36747),(#36748,#36749),(#36750,#36751),(#36752,#36753),(#36754,
#36755),(#36756,#36757),(#36758,#36759),(#36760,#36761),(#36762,#36763),
(#36764,#36765),(#36766,#36767),(#36768,#36769),(#36770,#36771),(#36772,
#36773),(#36774,#36775),(#36776,#36777),(#36778,#36779),(#36780,#36781),
(#36782,#36783),(#36784,#36785),(#36786,#36787),(#36788,#36789),(#36790,
#36791),(#36792,#36793),(#36794,#36795),(#36796,#36797),(#36798,#36799),
(#36800,#36801),(#36802,#36803),(#36804,#36805),(#36806,#36807),(#36808,
#36809),(#36810,#36811),(#36812,#36813),(#36814,#36815),(#36816,#36817),
(#36818,#36819),(#36820,#36821),(#36822,#36823),(#36824,#36825),(#36826,
#36827),(#36828,#36829),(#36830,#36831),(#36832,#36833),(#36834,#36835),
(#36836,#36837),(#36838,#36839),(#36840,#36841),(#36842,#36843),(#36844,
#36845),(#36846,#36847),(#36848,#36849),(#36850,#36851),(#36852,#36853),
(#36854,#36855),(#36856,#36857),(#36858,#36859),(#36860,#36861),(#36862,
#36863),(#36864,#36865),(#36866,#36867),(#36868,#36869),(#36870,#36871),
(#36872,#36873),(#36874,#36875),(#36876,#36877),(#36878,#36879),(#36880,
#36881),(#36882,#36883),(#36884,#36885),(#36886,#36887),(#36888,#36889),
(#36890,#36891),(#36892,#36893),(#36894,#36895),(#36896,#36897),(#36898,
#36899),(#36900,#36901),(#36902,#36903),(#36904,#36905),(#36906,#36907),
(#36908,#36909),(#36910,#36911),(#36912,#36913),(#36914,#36915),(#36916,
#36917),(#36918,#36919),(#36920,#36921),(#36922,#36923),(#36924,#36925),
(#36926,#36927),(#36928,#36929),(#36930,#36931),(#36932,#36933),(#36934,
#36935),(#36936,#36937),(#36938,#36939),(#36940,#36941),(#36942,#36943),
(#36944,#36945),(#36946,#36947),(#36948,#36949),(#36950,#36951),(#36952,
#36953),(#36954,#36955),(#36956,#36957),(#36958,#36959),(#36960,#36961),
(#36962,#36963),(#36964,#36965),(#36966,#36967),(#36968,#36969),(#36970,
#36971),(#36972,#36973),(#36974,#36975),(#36976,#36977),(#36978,#36979),
(#36980,#36981),(#36982,#36983),(#36984,#36985),(#36986,#36987),(#36988,
#36989),(#36990,#36991),(#36992,#36993),(#36994,#36995),(#36996,#36997),
(#36998,#36999),(#37000,#37001),(#37002,#37003),(#37004,#37005),(#37006,
#37007),(#37008,#37009),(#37010,#37011),(#37012,#37013),(#37014,#37015),
(#37016,#37017),(#37018,#37019),(#37020,#37021),(#37022,#37023),(#37024,
#37025),(#37026,#37027),(#37028,#37029),(#37030,#37031),(#37032,#37033),
(#37034,#37035),(#37036,#37037),(#37038,#37039),(#37040,#37041),(#37042,
#37043),(#37044,#37045),(#37046,#37047),(#37048,#37049),(#37050,#37051),
(#37052,#37053),(#37054,#37055),(#37056,#37057),(#37058,#37059),(#37060,
#37061),(#37062,#37063),(#37064,#37065),(#37066,#37067),(#37068,#37069),
(#37070,#37071),(#37072,#37073),(#37074,#37075),(#37076,#37077),(#37078,
#37079),(#37080,#37081),(#37082,#37083),(#37084,#37085),(#37086,#37087),
(#37088,#37089),(#37090,#37091),(#37092,#37093),(#37094,#37095),(#37096,
#37097),(#37098,#37099),(#37100,#37101),(#37102,#37103),(#37104,#37105),
(#37106,#37107),(#37108,#37109),(#37110,#37111),(#37112,#37113),(#37114,
#37115),(#37116,#37117),(#37118,#37119),(#37120,#37121),(#37122,#37123),
(#37124,#37125),(#37126,#37127),(#37128,#37129),(#37130,#37131),(#37132,
#37133),(#37134,#37135),(#37136,#37137),(#37138,#37139),(#37140,#37141),
(#37142,#37143),(#37144,#37145),(#37146,#37147),(#37148,#37149),(#37150,
#37151),(#37152,#37153),(#37154,#37155),(#37156,#37157),(#37158,#37159),
(#37160,#37161),(#37162,#37163),(#37164,#37165),(#37166,#37167),(#37168,
#37169),(#37170,#37171),(#37172,#37173),(#37174,#37175),(#37176,#37177),
(#37178,#37179),(#37180,#37181),(#37182,#37183),(#37184,#37185),(#37186,
#37187),(#37188,#37189),(#37190,#37191),(#37192,#37193),(#37194,#37195),
(#37196,#37197),(#37198,#37199),(#37200,#37201),(#37202,#37203),(#37204,
#37205),(#37206,#37207),(#37208,#37209),(#37210,#37211),(#37212,#37213),
(#37214,#37215),(#37216,#37217),(#37218,#37219),(#37220,#37221),(#37222,
#37223),(#37224,#37225),(#37226,#37227),(#37228,#37229),(#37230,#37231),
(#37232,#37233),(#37234,#37235),(#37236,#37237),(#37238,#37239),(#37240,
#37241),(#37242,#37243),(#37244,#37245),(#37246,#37247),(#37248,#37249),
(#37250,#37251),(#37252,#37253),(#37254,#37255),(#37256,#37257),(#37258,
#37259),(#37260,#37261),(#37262,#37263),(#37264,#37265),(#37266,#37267),
(#37268,#37269),(#37270,#37271),(#37272,#37273),(#37274,#37275),(#37276,
#37277),(#37278,#37279),(#37280,#37281),(#37282,#37283),(#37284,#37285),
(#37286,#37287),(#37288,#37289),(#37290,#37291),(#37292,#37293),(#37294,
#37295),(#37296,#37297),(#37298,#37299),(#37300,#37301),(#37302,#37303),
(#37304,#37305),(#37306,#37307),(#37308,#37309),(#37310,#37311),(#37312,
#37313),(#37314,#37315),(#37316,#37317),(#37318,#37319),(#37320,#37321),
(#37322,#37323),(#37324,#37325),(#37326,#37327),(#37328,#37329),(#37330,
#37331),(#37332,#37333),(#37334,#37335),(#37336,#37337),(#37338,#37339),
(#37340,#37341),(#37342,#37343),(#37344,#37345),(#37346,#37347),(#37348,
#37349),(#37350,#37351),(#37352,#37353),(#37354,#37355),(#37356,#37357),
(#37358,#37359),(#37360,#37361),(#37362,#37363),(#37364,#37365),(#37366,
#37367),(#37368,#37369),(#37370,#37371),(#37372,#37373),(#37374,#37375),
(#37376,#37377),(#37378,#37379),(#37380,#37381),(#37382,#37383),(#37384,
#37385),(#37386,#37387),(#37388,#37389),(#37390,#37391),(#37392,#37393),
(#37394,#37395),(#37396,#37397),(#37398,#37399),(#37400,#37401),(#37402,
#37403),(#37404,#37405),(#37406,#37407),(#37408,#37409),(#37410,#37411),
(#37412,#37413),(#37414,#37415),(#37416,#37417),(#37418,#37419),(#37420,
#37421),(#37422,#37423),(#37424,#37425),(#37426,#37427),(#37428,#37429),
(#37430,#37431),(#37432,#37433),(#37434,#37435),(#37436,#37437),(#37438,
#37439),(#37440,#37441),(#37442,#37443),(#37444,#37445),(#37446,#37447),
(#37448,#37449),(#37450,#37451),(#37452,#37453),(#37454,#37455),(#37456,
#37457),(#37458,#37459),(#37460,#37461),(#37462,#37463),(#37464,#37465),
(#37466,#37467),(#37468,#37469),(#37470,#37471),(#37472,#37473),(#37474,
#37475),(#37476,#37477),(#37478,#37479),(#37480,#37481),(#37482,#37483),
(#37484,#37485),(#37486,#37487),(#37488,#37489),(#37490,#37491),(#37492,
#37493),(#37494,#37495),(#37496,#37497),(#37498,#37499),(#37500,#37501),
(#37502,#37503),(#37504,#37505),(#37506,#37507),(#37508,#37509),(#37510,
#37511),(#37512,#37513),(#37514,#37515),(#37516,#37517),(#37518,#37519),
(#37520,#37521),(#37522,#37523),(#37524,#37525),(#37526,#37527),(#37528,
#37529),(#37530,#37531),(#37532,#37533),(#37534,#37535),(#37536,#37537),
(#37538,#37539),(#37540,#37541),(#37542,#37543),(#37544,#37545),(#37546,
#37547),(#37548,#37549),(#37550,#37551),(#37552,#37553),(#37554,#37555),
(#37556,#37557),(#37558,#37559),(#37560,#37561),(#37562,#37563),(#37564,
#37565),(#37566,#37567),(#37568,#37569),(#37570,#37571),(#37572,#37573),
(#37574,#37575),(#37576,#37577),(#37578,#37579),(#37580,#37581),(#37582,
#37583),(#37584,#37585),(#37586,#37587),(#37588,#37589),(#37590,#37591),
(#37592,#37593),(#37594,#37595),(#37596,#37597),(#37598,#37599),(#37600,
#37601),(#37602,#37603),(#37604,#37605),(#37606,#37607),(#37608,#37609),
(#37610,#37611),(#37612,#37613),(#37614,#37615),(#37616,#37617),(#37618,
#37619),(#37620,#37621),(#37622,#37623),(#37624,#37625),(#37626,#37627),
(#37628,#37629),(#37630,#37631),(#37632,#37633),(#37634,#37635),(#37636,
#37637),(#37638,#37639),(#37640,#37641),(#37642,#37643),(#37644,#37645),
(#37646,#37647),(#37648,#37649),(#37650,#37651),(#37652,#37653),(#37654,
#37655),(#37656,#37657),(#37658,#37659),(#37660,#37661),(#37662,#37663),
(#37664,#37665),(#37666,#37667),(#37668,#37669),(#37670,#37671),(#37672,
#37673),(#37674,#37675),(#37676,#37677),(#37678,#37679),(#37680,#37681),
(#37682,#37683),(#37684,#37685),(#37686,#37687),(#37688,#37689),(#37690,
#37691),(#37692,#37693),(#37694,#37695),(#37696,#37697),(#37698,#37699),
(#37700,#37701),(#37702,#37703),(#37704,#37705),(#37706,#37707),(#37708,
#37709),(#37710,#37711),(#37712,#37713),(#37714,#37715),(#37716,#37717),
(#37718,#37719),(#37720,#37721),(#37722,#37723),(#37724,#37725),(#37726,
#37727),(#37728,#37729),(#37730,#37731),(#37732,#37733),(#37734,#37735),
(#37736,#37737),(#37738,#37739),(#37740,#37741),(#37742,#37743),(#37744,
#37745),(#37746,#37747),(#37748,#37749),(#37750,#37751),(#37752,#37753),
(#37754,#37755),(#37756,#37757),(#37758,#37759),(#37760,#37761),(#37762,
#37763),(#37764,#37765),(#37766,#37767),(#37768,#37769),(#37770,#37771),
(#37772,#37773),(#37774,#37775),(#37776,#37777),(#37778,#37779),(#37780,
#37781),(#37782,#37783),(#37784,#37785),(#37786,#37787),(#37788,#37789),
(#37790,#37791),(#37792,#37793),(#37794,#37795),(#37796,#37797),(#37798,
#37799),(#37800,#37801),(#37802,#37803),(#37804,#37805),(#37806,#37807),
(#37808,#37809),(#37810,#37811),(#37812,#37813),(#37814,#37815),(#37816,
#37817),(#37818,#37819),(#37820,#37821),(#37822,#37823),(#37824,#37825),
(#37826,#37827),(#37828,#37829),(#37830,#37831),(#37832,#37833),(#37834,
#37835),(#37836,#37837),(#37838,#37839),(#37840,#37841),(#37842,#37843),
(#37844,#37845),(#37846,#37847),(#37848,#37849),(#37850,#37851),(#37852,
#37853),(#37854,#37855),(#37856,#37857),(#37858,#37859),(#37860,#37861),
(#37862,#37863),(#37864,#37865),(#37866,#37867),(#37868,#37869),(#37870,
#37871),(#37872,#37873),(#37874,#37875),(#37876,#37877),(#37878,#37879),
(#37880,#37881),(#37882,#37883),(#37884,#37885),(#37886,#37887),(#37888,
#37889),(#37890,#37891),(#37892,#37893),(#37894,#37895),(#37896,#37897),
(#37898,#37899),(#37900,#37901),(#37902,#37903),(#37904,#37905),(#37906,
#37907),(#37908,#37909),(#37910,#37911),(#37912,#37913),(#37914,#37915),
(#37916,#37917),(#37918,#37919),(#37920,#37921),(#37922,#37923),(#37924,
#37925),(#37926,#37927),(#37928,#37929),(#37930,#37931),(#37932,#37933),
(#37934,#37935),(#37936,#37937),(#37938,#37939),(#37940,#37941),(#37942,
#37943),(#37944,#37945),(#37946,#37947),(#37948,#37949),(#37950,#37951),
(#37952,#37953),(#37954,#37955),(#37956,#37957),(#37958,#37959),(#37960,
#37961),(#37962,#37963),(#37964,#37965),(#37966,#37967),(#37968,#37969),
(#37970,#37971),(#37972,#37973),(#37974,#37975),(#37976,#37977),(#37978,
#37979),(#37980,#37981),(#37982,#37983),(#37984,#37985),(#37986,#37987),
(#37988,#37989),(#37990,#37991),(#37992,#37993),(#37994,#37995),(#37996,
#37997),(#37998,#37999),(#38000,#38001),(#38002,#38003),(#38004,#38005),
(#38006,#38007),(#38008,#38009),(#38010,#38011),(#38012,#38013),(#38014,
#38015),(#38016,#38017),(#38018,#38019),(#38020,#38021),(#38022,#38023),
(#38024,#38025),(#38026,#38027),(#38028,#38029),(#38030,#38031),(#38032,
#38033),(#38034,#38035),(#38036,#38037),(#38038,#38039),(#38040,#38041),
(#38042,#38043),(#38044,#38045),(#38046,#38047),(#38048,#38049),(#38050,
#38051),(#38052,#38053),(#38054,#38055),(#38056,#38057),(#38058,#38059),
(#38060,#38061),(#38062,#38063),(#38064,#38065),(#38066,#38067),(#38068,
#38069),(#38070,#38071),(#38072,#38073),(#38074,#38075),(#38076,#38077),
(#38078,#38079),(#38080,#38081),(#38082,#38083),(#38084,#38085),(#38086,
#38087),(#38088,#38089),(#38090,#38091),(#38092,#38093),(#38094,#38095),
(#38096,#38097),(#38098,#38099),(#38100,#38101),(#38102,#38103),(#38104,
#38105),(#38106,#38107),(#38108,#38109),(#38110,#38111),(#38112,#38113),
(#38114,#38115),(#38116,#38117),(#38118,#38119),(#38120,#38121),(#38122,
#38123),(#38124,#38125),(#38126,#38127),(#38128,#38129),(#38130,#38131),
(#38132,#38133),(#38134,#38135),(#38136,#38137),(#38138,#38139),(#38140,
#38141),(#38142,#38143),(#38144,#38145),(#38146,#38147),(#38148,#38149),
(#38150,#38151),(#38152,#38153),(#38154,#38155),(#38156,#38157),(#38158,
#38159),(#38160,#38161),(#38162,#38163),(#38164,#38165),(#38166,#38167),
(#38168,#38169),(#38170,#38171),(#38172,#38173),(#38174,#38175),(#38176,
#38177),(#38178,#38179),(#38180,#38181),(#38182,#38183),(#38184,#38185),
(#38186,#38187),(#38188,#38189),(#38190,#38191),(#38192,#38193),(#38194,
#38195),(#38196,#38197),(#38198,#38199),(#38200,#38201),(#38202,#38203),
(#38204,#38205),(#38206,#38207),(#38208,#38209),(#38210,#38211),(#38212,
#38213),(#38214,#38215),(#38216,#38217),(#38218,#38219),(#38220,#38221),
(#38222,#38223),(#38224,#38225),(#38226,#38227),(#38228,#38229),(#38230,
#38231),(#38232,#38233),(#38234,#38235),(#38236,#38237),(#38238,#38239),
(#38240,#38241),(#38242,#38243),(#38244,#38245),(#38246,#38247),(#38248,
#38249),(#38250,#38251),(#38252,#38253),(#38254,#38255),(#38256,#38257),
(#38258,#38259),(#38260,#38261),(#38262,#38263),(#38264,#38265),(#38266,
#38267),(#38268,#38269),(#38270,#38271),(#38272,#38273),(#38274,#38275),
(#38276,#38277),(#38278,#38279),(#38280,#38281),(#38282,#38283),(#38284,
#38285),(#38286,#38287),(#38288,#38289),(#38290,#38291),(#38292,#38293),
(#38294,#38295),(#38296,#38297),(#38298,#38299),(#38300,#38301),(#38302,
#38303),(#38304,#38305),(#38306,#38307),(#38308,#38309),(#38310,#38311),
(#38312,#38313),(#38314,#38315),(#38316,#38317),(#38318,#38319),(#38320,
#38321),(#38322,#38323),(#38324,#38325),(#38326,#38327),(#38328,#38329),
(#38330,#38331),(#38332,#38333),(#38334,#38335),(#38336,#38337),(#38338,
#38339),(#38340,#38341),(#38342,#38343),(#38344,#38345),(#38346,#38347),
(#38348,#38349),(#38350,#38351),(#38352,#38353),(#38354,#38355),(#38356,
#38357),(#38358,#38359),(#38360,#38361),(#38362,#38363),(#38364,#38365),
(#38366,#38367),(#38368,#38369),(#38370,#38371),(#38372,#38373),(#38374,
#38375),(#38376,#38377),(#38378,#38379),(#38380,#38381),(#38382,#38383),
(#38384,#38385),(#38386,#38387),(#38388,#38389),(#38390,#38391),(#38392,
#38393),(#38394,#38395),(#38396,#38397),(#38398,#38399),(#38400,#38401),
(#38402,#38403),(#38404,#38405),(#38406,#38407),(#38408,#38409),(#38410,
#38411),(#38412,#38413),(#38414,#38415),(#38416,#38417),(#38418,#38419),
(#38420,#38421),(#38422,#38423),(#38424,#38425),(#38426,#38427),(#38428,
#38429),(#38430,#38431),(#38432,#38433),(#38434,#38435),(#38436,#38437),
(#38438,#38439),(#38440,#38441),(#38442,#38443),(#38444,#38445),(#38446,
#38447),(#38448,#38449),(#38450,#38451),(#38452,#38453),(#38454,#38455),
(#38456,#38457),(#38458,#38459),(#38460,#38461),(#38462,#38463),(#38464,
#38465),(#38466,#38467),(#38468,#38469),(#38470,#38471),(#38472,#38473),
(#38474,#38475),(#38476,#38477),(#38478,#38479),(#38480,#38481),(#38482,
#38483),(#38484,#38485),(#38486,#38487),(#38488,#38489),(#38490,#38491),
(#38492,#38493),(#38494,#38495),(#38496,#38497),(#38498,#38499),(#38500,
#38501),(#38502,#38503),(#38504,#38505),(#38506,#38507),(#38508,#38509),
(#38510,#38511),(#38512,#38513),(#38514,#38515),(#38516,#38517),(#38518,
#38519),(#38520,#38521),(#38522,#38523),(#38524,#38525),(#38526,#38527),
(#38528,#38529),(#38530,#38531),(#38532,#38533),(#38534,#38535),(#38536,
#38537),(#38538,#38539),(#38540,#38541),(#38542,#38543),(#38544,#38545),
(#38546,#38547),(#38548,#38549),(#38550,#38551),(#38552,#38553),(#38554,
#38555),(#38556,#38557),(#38558,#38559),(#38560,#38561),(#38562,#38563),
(#38564,#38565),(#38566,#38567),(#38568,#38569),(#38570,#38571),(#38572,
#38573),(#38574,#38575),(#38576,#38577),(#38578,#38579),(#38580,#38581),
(#38582,#38583),(#38584,#38585),(#38586,#38587),(#38588,#38589),(#38590,
#38591),(#38592,#38593),(#38594,#38595),(#38596,#38597),(#38598,#38599),
(#38600,#38601),(#38602,#38603),(#38604,#38605),(#38606,#38607),(#38608,
#38609),(#38610,#38611),(#38612,#38613),(#38614,#38615),(#38616,#38617),
(#38618,#38619),(#38620,#38621),(#38622,#38623),(#38624,#38625),(#38626,
#38627),(#38628,#38629),(#38630,#38631),(#38632,#38633),(#38634,#38635),
(#38636,#38637),(#38638,#38639),(#38640,#38641),(#38642,#38643),(#38644,
#38645),(#38646,#38647),(#38648,#38649),(#38650,#38651),(#38652,#38653),
(#38654,#38655),(#38656,#38657),(#38658,#38659),(#38660,#38661),(#38662,
#38663),(#38664,#38665),(#38666,#38667),(#38668,#38669),(#38670,#38671),
(#38672,#38673),(#38674,#38675),(#38676,#38677),(#38678,#38679),(#38680,
#38681),(#38682,#38683),(#38684,#38685),(#38686,#38687),(#38688,#38689),
(#38690,#38691),(#38692,#38693),(#38694,#38695),(#38696,#38697),(#38698,
#38699),(#38700,#38701),(#38702,#38703),(#38704,#38705),(#38706,#38707),
(#38708,#38709),(#38710,#38711),(#38712,#38713),(#38714,#38715),(#38716,
#38717),(#38718,#38719),(#38720,#38721),(#38722,#38723),(#38724,#38725),
(#38726,#38727),(#38728,#38729),(#38730,#38731),(#38732,#38733),(#38734,
#38735),(#38736,#38737),(#38738,#38739),(#38740,#38741),(#38742,#38743),
(#38744,#38745),(#38746,#38747),(#38748,#38749),(#38750,#38751),(#38752,
#38753),(#38754,#38755),(#38756,#38757),(#38758,#38759),(#38760,#38761),
(#38762,#38763),(#38764,#38765),(#38766,#38767),(#38768,#38769),(#38770,
#38771),(#38772,#38773),(#38774,#38775),(#38776,#38777),(#38778,#38779),
(#38780,#38781),(#38782,#38783),(#38784,#38785),(#38786,#38787),(#38788,
#38789),(#38790,#38791),(#38792,#38793),(#38794,#38795),(#38796,#38797),
(#38798,#38799),(#38800,#38801),(#38802,#38803),(#38804,#38805),(#38806,
#38807),(#38808,#38809),(#38810,#38811),(#38812,#38813),(#38814,#38815),
(#38816,#38817),(#38818,#38819),(#38820,#38821),(#38822,#38823),(#38824,
#38825),(#38826,#38827),(#38828,#38829),(#38830,#38831),(#38832,#38833),
(#38834,#38835),(#38836,#38837),(#38838,#38839),(#38840,#38841),(#38842,
#38843),(#38844,#38845),(#38846,#38847),(#38848,#38849),(#38850,#38851),
(#38852,#38853),(#38854,#38855),(#38856,#38857),(#38858,#38859),(#38860,
#38861),(#38862,#38863),(#38864,#38865),(#38866,#38867),(#38868,#38869),
(#38870,#38871),(#38872,#38873),(#38874,#38875),(#38876,#38877),(#38878,
#38879),(#38880,#38881),(#38882,#38883),(#38884,#38885),(#38886,#38887),
(#38888,#38889),(#38890,#38891),(#38892,#38893),(#38894,#38895),(#38896,
#38897),(#38898,#38899),(#38900,#38901),(#38902,#38903),(#38904,#38905),
(#38906,#38907),(#38908,#38909),(#38910,#38911),(#38912,#38913),(#38914,
#38915),(#38916,#38917),(#38918,#38919),(#38920,#38921),(#38922,#38923),
(#38924,#38925),(#38926,#38927),(#38928,#38929),(#38930,#38931),(#38932,
#38933),(#38934,#38935),(#38936,#38937),(#38938,#38939),(#38940,#38941),
(#38942,#38943),(#38944,#38945),(#38946,#38947),(#38948,#38949),(#38950,
#38951),(#38952,#38953),(#38954,#38955),(#38956,#38957),(#38958,#38959),
(#38960,#38961),(#38962,#38963),(#38964,#38965),(#38966,#38967),(#38968,
#38969),(#38970,#38971),(#38972,#38973),(#38974,#38975),(#38976,#38977),
(#38978,#38979),(#38980,#38981),(#38982,#38983),(#38984,#38985),(#38986,
#38987),(#38988,#38989),(#38990,#38991),(#38992,#38993),(#38994,#38995),
(#38996,#38997),(#38998,#38999),(#39000,#39001),(#39002,#39003),(#39004,
#39005),(#39006,#39007),(#39008,#39009),(#39010,#39011),(#39012,#39013),
(#39014,#39015),(#39016,#39017),(#39018,#39019),(#39020,#39021),(#39022,
#39023),(#39024,#39025),(#39026,#39027),(#39028,#39029),(#39030,#39031),
(#39032,#39033),(#39034,#39035),(#39036,#39037),(#39038,#39039),(#39040,
#39041),(#39042,#39043),(#39044,#39045),(#39046,#39047),(#39048,#39049),
(#39050,#39051),(#39052,#39053),(#39054,#39055),(#39056,#39057),(#39058,
#39059),(#39060,#39061),(#39062,#39063),(#39064,#39065),(#39066,#39067),
(#39068,#39069),(#39070,#39071),(#39072,#39073),(#39074,#39075),(#39076,
#39077),(#39078,#39079),(#39080,#39081),(#39082,#39083),(#39084,#39085),
(#39086,#39087),(#39088,#39089),(#39090,#39091),(#39092,#39093),(#39094,
#39095),(#39096,#39097),(#39098,#39099),(#39100,#39101),(#39102,#39103),
(#39104,#39105),(#39106,#39107),(#39108,#39109),(#39110,#39111),(#39112,
#39113),(#39114,#39115),(#39116,#39117),(#39118,#39119),(#39120,#39121),
(#39122,#39123),(#39124,#39125),(#39126,#39127),(#39128,#39129),(#39130,
#39131),(#39132,#39133),(#39134,#39135),(#39136,#39137),(#39138,#39139),
(#39140,#39141),(#39142,#39143),(#39144,#39145),(#39146,#39147),(#39148,
#39149),(#39150,#39151),(#39152,#39153),(#39154,#39155),(#39156,#39157),
(#39158,#39159),(#39160,#39161),(#39162,#39163),(#39164,#39165),(#39166,
#39167),(#39168,#39169),(#39170,#39171),(#39172,#39173),(#39174,#39175),
(#39176,#39177),(#39178,#39179),(#39180,#39181),(#39182,#39183),(#39184,
#39185),(#39186,#39187),(#39188,#39189),(#39190,#39191),(#39192,#39193),
(#39194,#39195),(#39196,#39197),(#39198,#39199),(#39200,#39201),(#39202,
#39203),(#39204,#39205),(#39206,#39207),(#39208,#39209),(#39210,#39211),
(#39212,#39213),(#39214,#39215),(#39216,#39217),(#39218,#39219),(#39220,
#39221),(#39222,#39223),(#39224,#39225),(#39226,#39227),(#39228,#39229),
(#39230,#39231),(#39232,#39233),(#39234,#39235),(#39236,#39237),(#39238,
#39239),(#39240,#39241),(#39242,#39243),(#39244,#39245),(#39246,#39247),
(#39248,#39249),(#39250,#39251),(#39252,#39253),(#39254,#39255),(#39256,
#39257),(#39258,#39259),(#39260,#39261),(#39262,#39263),(#39264,#39265),
(#39266,#39267),(#39268,#39269),(#39270,#39271),(#39272,#39273),(#39274,
#39275),(#39276,#39277),(#39278,#39279),(#39280,#39281),(#39282,#39283),
(#39284,#39285),(#39286,#39287),(#39288,#39289),(#39290,#39291),(#39292,
#39293),(#39294,#39295),(#39296,#39297),(#39298,#39299),(#39300,#39301),
(#39302,#39303),(#39304,#39305),(#39306,#39307),(#39308,#39309),(#39310,
#39311),(#39312,#39313),(#39314,#39315),(#39316,#39317),(#39318,#39319),
(#39320,#39321),(#39322,#39323),(#39324,#39325),(#39326,#39327),(#39328,
#39329),(#39330,#39331),(#39332,#39333),(#39334,#39335),(#39336,#39337),
(#39338,#39339),(#39340,#39341),(#39342,#39343),(#39344,#39345),(#39346,
#39347),(#39348,#39349),(#39350,#39351),(#39352,#39353),(#39354,#39355),
(#39356,#39357),(#39358,#39359),(#39360,#39361),(#39362,#39363),(#39364,
#39365),(#39366,#39367),(#39368,#39369),(#39370,#39371),(#39372,#39373),
(#39374,#39375),(#39376,#39377),(#39378,#39379),(#39380,#39381),(#39382,
#39383),(#39384,#39385),(#39386,#39387),(#39388,#39389),(#39390,#39391),
(#39392,#39393),(#39394,#39395),(#39396,#39397),(#39398,#39399),(#39400,
#39401),(#39402,#39403),(#39404,#39405),(#39406,#39407),(#39408,#39409),
(#39410,#39411),(#39412,#39413),(#39414,#39415),(#39416,#39417),(#39418,
#39419),(#39420,#39421),(#39422,#39423),(#39424,#39425),(#39426,#39427),
(#39428,#39429),(#39430,#39431),(#39432,#39433),(#39434,#39435),(#39436,
#39437),(#39438,#39439),(#39440,#39441),(#39442,#39443),(#39444,#39445),
(#39446,#39447),(#39448,#39449),(#39450,#39451),(#39452,#39453),(#39454,
#39455),(#39456,#39457),(#39458,#39459),(#39460,#39461),(#39462,#39463),
(#39464,#39465),(#39466,#39467),(#39468,#39469),(#39470,#39471),(#39472,
#39473),(#39474,#39475),(#39476,#39477),(#39478,#39479),(#39480,#39481),
(#39482,#39483),(#39484,#39485),(#39486,#39487),(#39488,#39489),(#39490,
#39491),(#39492,#39493),(#39494,#39495),(#39496,#39497),(#39498,#39499),
(#39500,#39501),(#39502,#39503),(#39504,#39505),(#39506,#39507),(#39508,
#39509),(#39510,#39511),(#39512,#39513),(#39514,#39515),(#39516,#39517),
(#39518,#39519),(#39520,#39521),(#39522,#39523),(#39524,#39525),(#39526,
#39527),(#39528,#39529),(#39530,#39531),(#39532,#39533),(#39534,#39535),
(#39536,#39537),(#39538,#39539),(#39540,#39541),(#39542,#39543),(#39544,
#39545),(#39546,#39547),(#39548,#39549),(#39550,#39551),(#39552,#39553),
(#39554,#39555),(#39556,#39557),(#39558,#39559),(#39560,#39561),(#39562,
#39563),(#39564,#39565),(#39566,#39567),(#39568,#39569),(#39570,#39571),
(#39572,#39573),(#39574,#39575),(#39576,#39577),(#39578,#39579),(#39580,
#39581),(#39582,#39583),(#39584,#39585),(#39586,#39587),(#39588,#39589),
(#39590,#39591),(#39592,#39593),(#39594,#39595),(#39596,#39597),(#39598,
#39599),(#39600,#39601),(#39602,#39603),(#39604,#39605),(#39606,#39607),
(#39608,#39609),(#39610,#39611),(#39612,#39613),(#39614,#39615),(#39616,
#39617),(#39618,#39619),(#39620,#39621),(#39622,#39623),(#39624,#39625),
(#39626,#39627),(#39628,#39629),(#39630,#39631),(#39632,#39633),(#39634,
#39635),(#39636,#39637),(#39638,#39639),(#39640,#39641),(#39642,#39643),
(#39644,#39645),(#39646,#39647),(#39648,#39649),(#39650,#39651),(#39652,
#39653),(#39654,#39655),(#39656,#39657),(#39658,#39659),(#39660,#39661),
(#39662,#39663),(#39664,#39665),(#39666,#39667),(#39668,#39669),(#39670,
#39671),(#39672,#39673),(#39674,#39675),(#39676,#39677),(#39678,#39679),
(#39680,#39681),(#39682,#39683),(#39684,#39685),(#39686,#39687),(#39688,
#39689),(#39690,#39691),(#39692,#39693),(#39694,#39695),(#39696,#39697),
(#39698,#39699),(#39700,#39701),(#39702,#39703),(#39704,#39705),(#39706,
#39707),(#39708,#39709),(#39710,#39711),(#39712,#39713),(#39714,#39715),
(#39716,#39717),(#39718,#39719),(#39720,#39721),(#39722,#39723),(#39724,
#39725),(#39726,#39727),(#39728,#39729),(#39730,#39731),(#39732,#39733),
(#39734,#39735),(#39736,#39737),(#39738,#39739),(#39740,#39741),(#39742,
#39743),(#39744,#39745),(#39746,#39747),(#39748,#39749),(#39750,#39751),
(#39752,#39753),(#39754,#39755),(#39756,#39757),(#39758,#39759),(#39760,
#39761),(#39762,#39763),(#39764,#39765),(#39766,#39767),(#39768,#39769),
(#39770,#39771),(#39772,#39773),(#39774,#39775),(#39776,#39777),(#39778,
#39779),(#39780,#39781),(#39782,#39783),(#39784,#39785),(#39786,#39787),
(#39788,#39789),(#39790,#39791),(#39792,#39793),(#39794,#39795),(#39796,
#39797),(#39798,#39799),(#39800,#39801),(#39802,#39803),(#39804,#39805),
(#39806,#39807),(#39808,#39809),(#39810,#39811),(#39812,#39813),(#39814,
#39815),(#39816,#39817),(#39818,#39819),(#39820,#39821),(#39822,#39823),
(#39824,#39825),(#39826,#39827),(#39828,#39829),(#39830,#39831),(#39832,
#39833),(#39834,#39835),(#39836,#39837),(#39838,#39839),(#39840,#39841),
(#39842,#39843),(#39844,#39845),(#39846,#39847),(#39848,#39849),(#39850,
#39851),(#39852,#39853),(#39854,#39855),(#39856,#39857),(#39858,#39859),
(#39860,#39861),(#39862,#39863),(#39864,#39865),(#39866,#39867),(#39868,
#39869),(#39870,#39871),(#39872,#39873),(#39874,#39875),(#39876,#39877),
(#39878,#39879),(#39880,#39881),(#39882,#39883),(#39884,#39885),(#39886,
#39887),(#39888,#39889),(#39890,#39891),(#39892,#39893),(#39894,#39895),
(#39896,#39897),(#39898,#39899),(#39900,#39901),(#39902,#39903),(#39904,
#39905),(#39906,#39907),(#39908,#39909),(#39910,#39911),(#39912,#39913),
(#39914,#39915),(#39916,#39917),(#39918,#39919),(#39920,#39921),(#39922,
#39923),(#39924,#39925),(#39926,#39927),(#39928,#39929),(#39930,#39931),
(#39932,#39933),(#39934,#39935),(#39936,#39937),(#39938,#39939),(#39940,
#39941),(#39942,#39943),(#39944,#39945),(#39946,#39947),(#39948,#39949),
(#39950,#39951),(#39952,#39953),(#39954,#39955),(#39956,#39957),(#39958,
#39959),(#39960,#39961),(#39962,#39963),(#39964,#39965),(#39966,#39967),
(#39968,#39969),(#39970,#39971),(#39972,#39973),(#39974,#39975),(#39976,
#39977),(#39978,#39979),(#39980,#39981),(#39982,#39983),(#39984,#39985),
(#39986,#39987),(#39988,#39989),(#39990,#39991),(#39992,#39993),(#39994,
#39995),(#39996,#39997),(#39998,#39999),(#40000,#40001),(#40002,#40003),
(#40004,#40005),(#40006,#40007),(#40008,#40009),(#40010,#40011),(#40012,
#40013),(#40014,#40015),(#40016,#40017),(#40018,#40019),(#40020,#40021),
(#40022,#40023),(#40024,#40025),(#40026,#40027),(#40028,#40029),(#40030,
#40031),(#40032,#40033),(#40034,#40035),(#40036,#40037),(#40038,#40039),
(#40040,#40041),(#40042,#40043),(#40044,#40045),(#40046,#40047),(#40048,
#40049),(#40050,#40051),(#40052,#40053),(#40054,#40055),(#40056,#40057),
(#40058,#40059),(#40060,#40061),(#40062,#40063),(#40064,#40065),(#40066,
#40067),(#40068,#40069),(#40070,#40071),(#40072,#40073),(#40074,#40075),
(#40076,#40077),(#40078,#40079),(#40080,#40081),(#40082,#40083),(#40084,
#40085),(#40086,#40087),(#40088,#40089),(#40090,#40091),(#40092,#40093),
(#40094,#40095),(#40096,#40097),(#40098,#40099),(#40100,#40101),(#40102,
#40103),(#40104,#40105),(#40106,#40107),(#40108,#40109),(#40110,#40111),
(#40112,#40113),(#40114,#40115),(#40116,#40117),(#40118,#40119),(#40120,
#40121),(#40122,#40123),(#40124,#40125),(#40126,#40127),(#40128,#40129),
(#40130,#40131),(#40132,#40133),(#40134,#40135),(#40136,#40137),(#40138,
#40139),(#40140,#40141),(#40142,#40143),(#40144,#40145),(#40146,#40147),
(#40148,#40149),(#40150,#40151),(#40152,#40153),(#40154,#40155),(#40156,
#40157),(#40158,#40159),(#40160,#40161),(#40162,#40163),(#40164,#40165),
(#40166,#40167),(#40168,#40169),(#40170,#40171),(#40172,#40173),(#40174,
#40175),(#40176,#40177),(#40178,#40179),(#40180,#40181),(#40182,#40183),
(#40184,#40185),(#40186,#40187),(#40188,#40189),(#40190,#40191),(#40192,
#40193),(#40194,#40195),(#40196,#40197),(#40198,#40199),(#40200,#40201),
(#40202,#40203),(#40204,#40205),(#40206,#40207),(#40208,#40209),(#40210,
#40211),(#40212,#40213),(#40214,#40215),(#40216,#40217),(#40218,#40219),
(#40220,#40221),(#40222,#40223),(#40224,#40225),(#40226,#40227),(#40228,
#40229),(#40230,#40231),(#40232,#40233),(#40234,#40235),(#40236,#40237),
(#40238,#40239),(#40240,#40241),(#40242,#40243),(#40244,#40245),(#40246,
#40247),(#40248,#40249),(#40250,#40251),(#40252,#40253),(#40254,#40255),
(#40256,#40257),(#40258,#40259),(#40260,#40261),(#40262,#40263),(#40264,
#40265),(#40266,#40267),(#40268,#40269),(#40270,#40271),(#40272,#40273),
(#40274,#40275),(#40276,#40277),(#40278,#40279),(#40280,#40281),(#40282,
#40283),(#40284,#40285),(#40286,#40287),(#40288,#40289),(#40290,#40291),
(#40292,#40293),(#40294,#40295),(#40296,#40297),(#40298,#40299),(#40300,
#40301),(#40302,#40303),(#40304,#40305),(#40306,#40307),(#40308,#40309),
(#40310,#40311),(#40312,#40313),(#40314,#40315),(#40316,#40317),(#40318,
#40319),(#40320,#40321),(#40322,#40323),(#40324,#40325),(#40326,#40327),
(#40328,#40329),(#40330,#40331),(#40332,#40333),(#40334,#40335),(#40336,
#40337),(#40338,#40339),(#40340,#40341),(#40342,#40343),(#40344,#40345),
(#40346,#40347),(#40348,#40349),(#40350,#40351),(#40352,#40353),(#40354,
#40355),(#40356,#40357),(#40358,#40359),(#40360,#40361),(#40362,#40363),
(#40364,#40365),(#40366,#40367),(#40368,#40369),(#40370,#40371),(#40372,
#40373),(#40374,#40375),(#40376,#40377),(#40378,#40379),(#40380,#40381),
(#40382,#40383),(#40384,#40385),(#40386,#40387),(#40388,#40389),(#40390,
#40391),(#40392,#40393),(#40394,#40395),(#40396,#40397),(#40398,#40399),
(#40400,#40401),(#40402,#40403),(#40404,#40405),(#40406,#40407),(#40408,
#40409),(#40410,#40411),(#40412,#40413),(#40414,#40415),(#40416,#40417),
(#40418,#40419),(#40420,#40421),(#40422,#40423),(#40424,#40425),(#40426,
#40427),(#40428,#40429),(#40430,#40431),(#40432,#40433),(#40434,#40435),
(#40436,#40437),(#40438,#40439),(#40440,#40441),(#40442,#40443),(#40444,
#40445),(#40446,#40447),(#40448,#40449),(#40450,#40451),(#40452,#40453),
(#40454,#40455),(#40456,#40457),(#40458,#40459),(#40460,#40461),(#40462,
#40463),(#40464,#40465),(#40466,#40467),(#40468,#40469),(#40470,#40471),
(#40472,#40473),(#40474,#40475),(#40476,#40477),(#40478,#40479),(#40480,
#40481),(#40482,#40483),(#40484,#40485),(#40486,#40487),(#40488,#40489),
(#40490,#40491),(#40492,#40493),(#40494,#40495),(#40496,#40497),(#40498,
#40499),(#40500,#40501),(#40502,#40503),(#40504,#40505),(#40506,#40507),
(#40508,#40509),(#40510,#40511),(#40512,#40513),(#40514,#40515),(#40516,
#40517),(#40518,#40519),(#40520,#40521),(#40522,#40523),(#40524,#40525),
(#40526,#40527),(#40528,#40529),(#40530,#40531),(#40532,#40533),(#40534,
#40535),(#40536,#40537),(#40538,#40539),(#40540,#40541),(#40542,#40543),
(#40544,#40545),(#40546,#40547),(#40548,#40549),(#40550,#40551),(#40552,
#40553),(#40554,#40555),(#40556,#40557),(#40558,#40559),(#40560,#40561),
(#40562,#40563),(#40564,#40565),(#40566,#40567),(#40568,#40569),(#40570,
#40571),(#40572,#40573),(#40574,#40575),(#40576,#40577),(#40578,#40579),
(#40580,#40581),(#40582,#40583),(#40584,#40585),(#40586,#40587),(#40588,
#40589),(#40590,#40591),(#40592,#40593),(#40594,#40595),(#40596,#40597),
(#40598,#40599),(#40600,#40601),(#40602,#40603),(#40604,#40605),(#40606,
#40607),(#40608,#40609),(#40610,#40611),(#40612,#40613),(#40614,#40615),
(#40616,#40617),(#40618,#40619),(#40620,#40621),(#40622,#40623),(#40624,
#40625),(#40626,#40627),(#40628,#40629),(#40630,#40631),(#40632,#40633),
(#40634,#40635),(#40636,#40637),(#40638,#40639),(#40640,#40641),(#40642,
#40643),(#40644,#40645),(#40646,#40647),(#40648,#40649),(#40650,#40651),
(#40652,#40653),(#40654,#40655),(#40656,#40657),(#40658,#40659),(#40660,
#40661),(#40662,#40663),(#40664,#40665),(#40666,#40667),(#40668,#40669),
(#40670,#40671),(#40672,#40673),(#40674,#40675),(#40676,#40677),(#40678,
#40679),(#40680,#40681),(#40682,#40683),(#40684,#40685),(#40686,#40687),
(#40688,#40689),(#40690,#40691),(#40692,#40693),(#40694,#40695),(#40696,
#40697),(#40698,#40699),(#40700,#40701),(#40702,#40703),(#40704,#40705),
(#40706,#40707),(#40708,#40709),(#40710,#40711),(#40712,#40713),(#40714,
#40715),(#40716,#40717),(#40718,#40719),(#40720,#40721),(#40722,#40723),
(#40724,#40725),(#40726,#40727),(#40728,#40729),(#40730,#40731),(#40732,
#40733),(#40734,#40735),(#40736,#40737),(#40738,#40739),(#40740,#40741),
(#40742,#40743),(#40744,#40745),(#40746,#40747),(#40748,#40749),(#40750,
#40751),(#40752,#40753),(#40754,#40755),(#40756,#40757),(#40758,#40759),
(#40760,#40761),(#40762,#40763),(#40764,#40765),(#40766,#40767),(#40768,
#40769),(#40770,#40771),(#40772,#40773),(#40774,#40775),(#40776,#40777),
(#40778,#40779),(#40780,#40781),(#40782,#40783),(#40784,#40785),(#40786,
#40787),(#40788,#40789),(#40790,#40791),(#40792,#40793),(#40794,#40795),
(#40796,#40797),(#40798,#40799),(#40800,#40801),(#40802,#40803),(#40804,
#40805),(#40806,#40807),(#40808,#40809),(#40810,#40811),(#40812,#40813),
(#40814,#40815),(#40816,#40817),(#40818,#40819),(#40820,#40821),(#40822,
#40823),(#40824,#40825),(#40826,#40827),(#40828,#40829),(#40830,#40831),
(#40832,#40833),(#40834,#40835),(#40836,#40837),(#40838,#40839),(#40840,
#40841),(#40842,#40843),(#40844,#40845),(#40846,#40847),(#40848,#40849),
(#40850,#40851),(#40852,#40853),(#40854,#40855),(#40856,#40857),(#40858,
#40859),(#40860,#40861),(#40862,#40863),(#40864,#40865),(#40866,#40867),
(#40868,#40869),(#40870,#40871),(#40872,#40873),(#40874,#40875),(#40876,
#40877),(#40878,#40879),(#40880,#40881),(#40882,#40883),(#40884,#40885),
(#40886,#40887),(#40888,#40889),(#40890,#40891),(#40892,#40893),(#40894,
#40895),(#40896,#40897),(#40898,#40899),(#40900,#40901),(#40902,#40903),
(#40904,#40905),(#40906,#40907),(#40908,#40909),(#40910,#40911),(#40912,
#40913),(#40914,#40915),(#40916,#40917),(#40918,#40919),(#40920,#40921),
(#40922,#40923),(#40924,#40925),(#40926,#40927),(#40928,#40929),(#40930,
#40931),(#40932,#40933),(#40934,#40935),(#40936,#40937),(#40938,#40939),
(#40940,#40941),(#40942,#40943),(#40944,#40945),(#40946,#40947),(#40948,
#40949),(#40950,#40951),(#40952,#40953),(#40954,#40955),(#40956,#40957),
(#40958,#40959),(#40960,#40961),(#40962,#40963),(#40964,#40965),(#40966,
#40967),(#40968,#40969),(#40970,#40971),(#40972,#40973),(#40974,#40975),
(#40976,#40977),(#40978,#40979),(#40980,#40981),(#40982,#40983),(#40984,
#40985),(#40986,#40987),(#40988,#40989),(#40990,#40991),(#40992,#40993),
(#40994,#40995),(#40996,#40997),(#40998,#40999),(#41000,#41001),(#41002,
#41003),(#41004,#41005),(#41006,#41007),(#41008,#41009),(#41010,#41011),
(#41012,#41013),(#41014,#41015),(#41016,#41017),(#41018,#41019),(#41020,
#41021),(#41022,#41023),(#41024,#41025),(#41026,#41027),(#41028,#41029),
(#41030,#41031),(#41032,#41033),(#41034,#41035),(#41036,#41037),(#41038,
#41039),(#41040,#41041),(#41042,#41043),(#41044,#41045),(#41046,#41047),
(#41048,#41049),(#41050,#41051),(#41052,#41053),(#41054,#41055),(#41056,
#41057),(#41058,#41059),(#41060,#41061),(#41062,#41063),(#41064,#41065),
(#41066,#41067),(#41068,#41069),(#41070,#41071),(#41072,#41073),(#41074,
#41075),(#41076,#41077),(#41078,#41079),(#41080,#41081),(#41082,#41083),
(#41084,#41085),(#41086,#41087),(#41088,#41089),(#41090,#41091),(#41092,
#41093),(#41094,#41095),(#41096,#41097),(#41098,#41099),(#41100,#41101),
(#41102,#41103),(#41104,#41105),(#41106,#41107),(#41108,#41109),(#41110,
#41111),(#41112,#41113),(#41114,#41115),(#41116,#41117),(#41118,#41119),
(#41120,#41121),(#41122,#41123),(#41124,#41125),(#41126,#41127),(#41128,
#41129),(#41130,#41131),(#41132,#41133),(#41134,#41135),(#41136,#41137),
(#41138,#41139),(#41140,#41141),(#41142,#41143),(#41144,#41145),(#41146,
#41147),(#41148,#41149),(#41150,#41151),(#41152,#41153),(#41154,#41155),
(#41156,#41157),(#41158,#41159),(#41160,#41161),(#41162,#41163),(#41164,
#41165),(#41166,#41167),(#41168,#41169),(#41170,#41171),(#41172,#41173),
(#41174,#41175),(#41176,#41177),(#41178,#41179),(#41180,#41181),(#41182,
#41183),(#41184,#41185),(#41186,#41187),(#41188,#41189),(#41190,#41191),
(#41192,#41193),(#41194,#41195),(#41196,#41197),(#41198,#41199),(#41200,
#41201),(#41202,#41203),(#41204,#41205),(#41206,#41207),(#41208,#41209),
(#41210,#41211),(#41212,#41213),(#41214,#41215),(#41216,#41217),(#41218,
#41219),(#41220,#41221),(#41222,#41223),(#41224,#41225),(#41226,#41227)),
 .UNSPECIFIED.,.F.,.F.,.F.,(4,1,1,1,1,1,1,1,1,1,1,1,1,1,1,1,1,1,1,1,1,1,
1,1,1,1,1,1,1,1,1,1,1,1,1,1,1,1,1,1,1,1,1,1,1,1,1,1,1,1,1,1,1,1,1,1,1,1,
1,1,1,1,1,1,1,1,1,1,1,1,1,1,1,1,1,1,1,1,1,1,1,1,1,1,1,1,1,1,1,1,1,1,1,1,
1,1,1,1,1,1,1,1,1,1,1,1,1,1,1,1,1,1,1,1,1,1,1,1,1,1,1,1,1,1,1,1,1,1,1,1,
1,1,1,1,1,1,1,1,1,1,1,1,1,1,1,1,1,1,1,1,1,1,1,1,1,1,1,1,1,1,1,1,1,1,1,1,
1,1,1,1,1,1,1,1,1,1,1,1,1,1,1,1,1,1,1,1,1,1,1,1,1,1,1,1,1,1,1,1,1,1,1,1,
1,1,1,1,1,1,1,1,1,1,1,1,1,1,1,1,1,1,1,1,1,1,1,1,1,1,1,1,1,1,1,1,1,1,1,1,
1,1,1,1,1,1,1,1,1,1,1,1,1,1,1,1,1,1,1,1,1,1,1,1,1,1,1,1,1,1,1,1,1,1,1,1,
1,1,1,1,1,1,1,1,1,1,1,1,1,1,1,1,1,1,1,1,1,1,1,1,1,1,1,1,1,1,1,1,1,1,1,1,
1,1,1,1,1,1,1,1,1,1,1,1,1,1,1,1,1,1,1,1,1,1,1,1,1,1,1,1,1,1,1,1,1,1,1,1,
1,1,1,1,1,1,1,1,1,1,1,1,1,1,1,1,1,1,1,1,1,1,1,1,1,1,1,1,1,1,1,1,1,1,1,1,
1,1,1,1,1,1,1,1,1,1,1,1,1,1,1,1,1,1,1,1,1,1,1,1,1,1,1,1,1,1,1,1,1,1,1,1,
1,1,1,1,1,1,1,1,1,1,1,1,1,1,1,1,1,1,1,1,1,1,1,1,1,1,1,1,1,1,1,1,1,1,1,1,
1,1,1,1,1,1,1,1,1,1,1,1,1,1,1,1,1,1,1,1,1,1,1,1,1,1,1,1,1,1,1,1,1,1,1,1,
1,1,1,1,1,1,1,1,1,1,1,1,1,1,1,1,1,1,1,1,1,1,1,1,1,1,1,1,1,1,1,1,1,1,1,1,
1,1,1,1,1,1,1,1,1,1,1,1,1,1,1,1,1,1,1,1,1,1,1,1,1,1,1,1,1,1,1,1,1,1,1,1,
1,1,1,1,1,1,1,1,1,1,1,1,1,1,1,1,1,1,1,1,1,1,1,1,1,1,1,1,1,1,1,1,1,1,1,1,
1,1,1,1,1,1,1,1,1,1,1,1,1,1,1,1,1,1,1,1,1,1,1,1,1,1,1,1,1,1,1,1,1,1,1,1,
1,1,1,1,1,1,1,1,1,1,1,1,1,1,1,1,1,1,1,1,1,1,1,1,1,1,1,1,1,1,1,1,1,1,1,1,
1,1,1,1,1,1,1,1,1,1,1,1,1,1,1,1,1,1,1,1,1,1,1,1,1,1,1,1,1,1,1,1,1,1,1,1,
1,1,1,1,1,1,1,1,1,1,1,1,1,1,1,1,1,1,1,1,1,1,1,1,1,1,1,1,1,1,1,1,1,1,1,1,
1,1,1,1,1,1,1,1,1,1,1,1,1,1,1,1,1,1,1,1,1,1,1,1,1,1,1,1,1,1,1,1,1,1,1,1,
1,1,1,1,1,1,1,1,1,1,1,1,1,1,1,1,1,1,1,1,1,1,1,1,1,1,1,1,1,1,1,1,1,1,1,1,
1,1,1,1,1,1,1,1,1,1,1,1,1,1,1,1,1,1,1,1,1,1,1,1,1,1,1,1,1,1,1,1,1,1,1,1,
1,1,1,1,1,1,1,1,1,1,1,1,1,1,1,1,1,1,1,1,1,1,1,1,1,1,1,1,1,1,1,1,1,1,1,1,
1,1,1,1,1,1,1,1,1,1,1,1,1,1,1,1,1,1,1,1,1,1,1,1,1,1,1,1,1,1,1,1,1,1,1,1,
1,1,1,1,1,1,1,1,1,1,1,1,1,1,1,1,1,1,1,1,1,1,1,1,1,1,1,1,1,1,1,1,1,1,1,1,
1,1,1,1,1,1,1,1,1,1,1,1,1,1,1,1,1,1,1,1,1,1,1,1,1,1,1,1,1,1,1,1,1,1,1,1,
1,1,1,1,1,1,1,1,1,1,1,1,1,1,1,1,1,1,1,1,1,1,1,1,1,1,1,1,1,1,1,1,1,1,1,1,
1,1,1,1,1,1,1,1,1,1,1,1,1,1,1,1,1,1,1,1,1,1,1,1,1,1,1,1,1,1,1,1,1,1,1,1,
1,1,1,1,1,1,1,1,1,1,1,1,1,1,1,1,1,1,1,1,1,1,1,1,1,1,1,1,1,1,1,1,1,1,1,1,
1,1,1,1,1,1,1,1,1,1,1,1,1,1,1,1,1,1,1,1,1,1,1,1,1,1,1,1,1,1,1,1,1,1,1,1,
1,1,1,1,1,1,1,1,1,1,1,1,1,1,1,1,1,1,1,1,1,1,1,1,1,1,1,1,1,1,1,1,1,1,1,1,
1,1,1,1,1,1,1,1,1,1,1,1,1,1,1,1,1,1,1,1,1,1,1,1,1,1,1,1,1,1,1,1,1,1,1,1,
1,1,1,1,1,1,1,1,1,1,1,1,1,1,1,1,1,1,1,1,1,1,1,1,1,1,1,1,1,1,1,1,1,1,1,1,
1,1,1,1,1,1,1,1,1,1,1,1,1,1,1,1,1,1,1,1,1,1,1,1,1,1,1,1,1,1,1,1,1,1,1,1,
1,1,1,1,1,1,1,1,1,1,1,1,1,1,1,1,1,1,1,1,1,1,1,1,1,1,1,1,1,1,1,1,1,1,1,1,
1,1,1,1,1,1,1,1,1,1,1,1,1,1,1,1,1,1,1,1,1,1,1,1,1,1,1,1,1,1,1,1,1,1,1,1,
1,1,1,1,1,1,1,1,1,1,1,1,1,1,1,1,1,1,1,1,1,1,1,1,1,1,1,1,1,1,1,1,1,1,1,1,
1,1,1,1,1,1,1,1,1,1,1,1,1,1,1,1,1,1,1,1,1,1,1,1,1,1,1,1,1,1,1,1,1,1,1,1,
1,1,1,1,1,1,1,1,1,1,1,1,1,1,1,1,1,1,1,1,1,1,1,1,1,1,1,1,1,1,1,1,1,1,1,1,
1,1,1,1,1,1,1,1,1,1,1,1,1,1,1,1,1,1,1,1,1,1,1,1,1,1,1,1,1,1,1,1,1,1,1,1,
1,1,1,1,1,1,1,1,1,1,1,1,1,1,1,1,1,1,1,1,1,1,1,1,1,1,1,1,1,1,1,1,1,1,1,1,
1,1,1,1,1,1,1,1,1,1,1,1,1,1,1,1,1,1,1,1,1,1,1,1,1,1,1,1,1,1,1,1,1,1,1,1,
1,1,1,1,1,1,1,1,1,1,1,1,1,1,1,1,1,1,1,1,1,1,1,1,1,1,1,1,1,1,1,1,1,1,1,1,
1,1,1,1,1,1,1,1,1,1,1,1,1,1,1,1,1,1,1,1,1,1,1,1,1,1,1,1,1,1,1,1,1,1,1,1,
1,1,1,1,1,1,1,1,1,1,1,1,1,1,1,1,1,1,1,1,1,1,1,1,1,1,1,1,1,1,1,1,1,1,1,1,
1,1,1,1,1,1,1,1,1,1,1,1,1,1,1,1,1,1,1,1,1,1,1,1,1,1,1,1,1,1,1,1,1,1,1,1,
1,1,1,1,1,1,1,1,1,1,1,1,1,1,1,1,1,1,1,1,1,1,1,1,1,1,1,1,1,1,1,1,1,1,1,1,
1,1,1,1,1,1,1,1,1,1,1,1,1,1,1,1,1,1,1,1,1,1,1,1,1,1,1,1,1,1,1,1,1,1,1,1,
1,1,1,1,1,1,1,1,1,1,1,1,1,1,1,1,1,1,1,1,1,1,1,1,1,1,1,1,1,1,1,1,1,1,1,1,
1,1,1,1,1,1,1,1,1,1,1,1,1,1,1,1,1,1,1,1,1,1,1,1,1,1,1,1,1,1,1,1,1,1,1,1,
1,1,1,1,1,1,1,1,1,1,1,1,1,1,1,1,1,1,1,1,1,1,1,1,1,1,1,1,1,1,1,1,1,1,1,1,
1,1,1,1,1,1,1,1,1,1,1,1,1,1,1,1,1,1,1,1,1,1,1,1,1,1,1,1,1,1,1,1,1,1,1,1,
1,1,1,1,1,1,1,1,1,1,1,1,1,1,1,1,1,1,1,1,1,1,1,1,1,1,1,1,1,1,1,1,1,1,1,1,
1,1,1,1,1,1,1,1,1,1,1,1,1,1,1,1,1,1,1,1,1,1,1,1,1,1,1,1,1,1,1,1,1,1,1,1,
1,1,1,1,1,1,1,1,1,1,1,1,1,1,1,1,1,1,1,1,1,1,1,1,1,1,1,1,1,1,1,1,1,1,1,1,
1,1,1,1,1,1,1,1,1,1,1,1,1,1,1,1,1,1,1,1,1,1,1,1,1,1,1,1,1,1,1,1,1,1,1,1,
1,1,1,1,1,1,1,1,1,1,1,1,1,1,1,1,1,1,1,1,1,1,1,1,1,1,1,1,1,1,1,1,1,1,1,1,
1,1,1,1,1,1,1,1,1,1,1,1,1,1,1,1,1,1,1,1,1,1,1,1,1,1,1,1,1,1,1,1,1,1,1,1,
1,1,1,1,1,1,1,1,1,1,1,1,1,1,1,1,1,1,1,1,1,1,1,1,1,1,1,1,1,1,1,1,1,1,1,1,
1,1,1,1,1,1,1,1,1,1,1,1,1,1,1,1,1,1,1,1,1,1,1,1,1,1,1,1,1,1,1,1,1,1,1,1,
1,1,1,1,1,1,1,1,1,1,1,1,1,1,1,1,1,1,1,1,1,1,1,1,1,1,1,1,1,1,1,1,1,1,1,1,
1,1,1,1,1,1,1,1,1,1,1,1,1,1,1,1,1,1,1,1,1,1,1,1,1,1,1,1,1,1,1,1,1,1,1,1,
1,1,1,1,1,1,1,1,1,1,1,1,1,1,1,1,1,1,1,1,1,1,1,1,1,1,1,1,1,1,1,1,1,1,1,1,
1,1,1,1,1,1,1,1,1,1,1,1,1,1,1,1,1,1,1,1,1,1,1,1,1,1,1,1,1,1,1,1,1,1,1,1,
1,1,1,1,1,1,1,1,1,1,1,1,1,1,1,1,1,1,1,1,1,1,1,1,1,1,1,1,1,1,1,1,1,1,1,1,
1,1,1,1,1,1,1,1,1,1,1,1,1,1,1,1,1,1,1,1,1,1,1,1,1,1,1,1,1,1,1,1,1,1,1,1,
1,1,1,1,1,1,1,1,1,1,1,1,1,1,1,1,1,1,1,1,1,1,1,1,1,1,1,1,1,1,1,1,1,1,1,1,
1,1,1,1,1,1,1,1,1,1,1,1,1,1,1,1,1,1,1,1,1,1,1,1,1,1,1,1,1,1,1,1,1,1,1,1,
1,1,1,1,1,1,1,1,1,1,1,1,1,1,1,1,1,1,1,1,1,1,1,1,1,1,1,1,1,1,1,1,1,1,1,1,
1,1,1,1,1,1,1,1,1,1,1,1,1,1,1,1,1,1,1,1,1,1,1,1,1,1,1,1,1,1,1,1,1,1,1,1,
1,1,1,1,1,1,1,1,1,1,1,1,1,1,1,1,1,1,1,1,1,1,1,1,1,1,1,1,1,1,1,1,1,1,1,1,
1,1,1,1,1,1,1,1,1,1,1,1,1,1,1,1,1,1,1,1,1,1,1,1,1,1,1,1,1,1,1,1,1,1,1,1,
1,1,1,1,1,1,1,1,1,1,1,1,1,1,1,1,1,1,1,1,1,1,1,1,1,1,1,1,1,1,1,1,1,1,1,1,
1,1,1,1,1,1,1,1,1,1,1,1,1,1,1,1,1,1,1,1,1,1,1,1,1,1,1,1,1,1,1,1,1,1,1,1,
1,1,1,1,1,1,1,1,1,1,1,1,1,1,1,1,1,1,1,1,1,1,1,1,1,1,1,1,1,1,1,1,1,1,1,1,
1,1,1,1,1,1,1,1,1,1,1,1,1,1,1,1,1,1,1,1,1,1,1,1,1,1,1,1,1,1,1,1,1,1,1,1,
1,1,1,1,1,1,1,1,1,1,1,1,1,1,1,1,1,1,1,1,1,1,1,1,1,1,1,1,1,1,1,1,1,1,1,1,
1,1,1,1,1,1,1,1,1,1,1,1,1,1,1,1,1,1,1,1,1,1,1,1,1,1,1,1,1,1,1,1,1,1,1,1,
1,1,1,1,1,1,1,1,1,1,1,1,1,1,1,1,1,1,1,1,1,1,1,1,1,1,1,1,1,1,1,1,1,1,1,1,
1,1,1,1,1,1,1,1,1,1,1,1,1,1,1,1,1,1,1,1,1,1,1,1,1,1,1,1,1,1,1,1,1,1,1,1,
1,1,1,1,1,1,1,1,1,1,1,1,1,1,1,1,1,1,1,1,1,1,1,1,1,1,1,1,1,1,1,1,1,1,1,1,
1,1,1,1,1,1,1,1,1,1,1,1,1,1,1,1,1,1,1,1,1,1,1,1,1,1,1,1,1,1,1,1,1,1,1,1,
1,1,1,1,1,1,1,1,1,1,1,1,1,1,1,1,1,1,1,1,1,1,1,1,1,1,1,1,1,1,1,1,1,1,1,1,
1,1,1,1,1,1,1,1,1,1,1,1,1,1,1,1,1,1,1,1,1,1,1,1,1,1,1,1,1,1,1,1,1,1,1,1,
1,1,1,1,1,1,1,1,1,1,1,1,1,1,1,1,1,1,1,1,1,1,1,1,1,1,1,1,1,1,1,1,1,1,1,1,
1,1,1,1,1,1,1,1,1,1,1,1,1,1,1,1,1,1,1,1,1,1,1,1,1,1,1,1,1,1,1,1,1,1,1,1,
1,1,1,1,1,1,1,1,1,1,1,1,1,1,1,1,1,1,1,1,1,1,1,1,1,1,1,1,1,1,1,1,1,1,1,1,
1,1,1,1,1,1,1,1,1,1,1,1,1,1,1,1,1,1,1,1,1,1,1,1,1,1,1,1,1,1,1,1,1,1,1,1,
1,1,1,1,1,1,1,1,1,1,1,1,1,1,1,1,1,1,1,1,1,1,1,1,1,1,1,1,1,1,1,1,1,1,1,1,
1,1,1,1,1,1,1,1,1,1,1,1,1,1,1,1,1,1,1,1,1,1,1,1,1,1,1,1,1,1,1,1,1,1,1,1,
1,1,1,1,1,1,1,1,1,1,1,1,1,1,1,1,1,1,1,1,1,1,1,1,1,1,1,1,1,1,1,1,1,1,1,1,
1,1,1,1,1,1,1,1,1,1,1,1,1,1,1,1,1,1,1,1,1,1,1,1,1,1,1,1,1,1,1,1,1,1,1,1,
1,1,1,1,1,1,1,1,1,1,1,1,1,1,1,1,1,1,1,1,1,1,1,1,1,1,1,1,1,1,1,1,1,1,1,1,
1,1,1,1,1,1,1,1,1,1,1,1,1,1,1,1,1,1,1,1,1,1,1,1,1,1,1,1,1,1,1,1,1,1,1,1,
1,1,1,1,1,1,1,1,1,1,1,1,1,1,1,1,1,1,1,1,1,1,1,1,1,1,1,1,1,1,1,1,1,1,1,1,
1,1,1,1,4),(2,2),(0.,0.869746702321014,1.7394931589914,2.60923976624962,
3.47983908319159,4.35043840179749,5.22018503077054,6.08993165951504,6.95967828799171,
7.82942491616733,8.69917154401062,9.56891817149224,10.4395174886835,11.3101168056706,
12.179863432132,13.049610058144,13.9193566836854,14.7891033087372,15.6588499332817,
16.5285965573034,17.3991958717975,18.2697951860185,18.7046684974166,19.1395418086746,
19.5744151197912,20.0092884307654,20.4441617415962,20.8790350522825,21.7487816732187,
22.1836549834672,22.6185282935685,23.0534016035221,23.4882749133276,23.9231482229848,
24.3588742245859,24.794600226187,25.2294735355468,26.0992201538203,26.5340934627341,
26.9689667714994,27.4038400801166,27.838713388586,28.2735866969081,28.7084600050832,
29.143333313112,29.5782066209952,30.0130799287334,30.4479532363275,30.8828265437783,
31.3185525442794,31.7542785447804,32.1891518519474,32.6240251589741,33.0588984658616,
33.4937717726112,33.928645079224,34.3635183857014,34.7983916920448,35.2332649982556,
35.6681383043353,36.1030116102854,36.5378849161076,36.9727582218035,37.4076315273749,
37.8425048328235,38.2782308323341,38.7139568318446,39.1488301370532,39.5837034421446,
40.0185767471208,40.4534500519838,40.8883233567357,41.3231966613787,41.7580699659148,
42.1929432703463,42.6278165746754,43.0626898789044,43.4975631830356,43.9324364870714,
44.3673097910142,44.8021830948664,45.2379090935952,45.673635092324,46.1085083960024,
46.5433816995978,46.9782550031127,47.4131283065497,47.8480016099115,48.2828749132006,
48.7177482164198,49.1526215195718,49.5874948226593,50.0223681256851,50.457241428652,
50.8921147315628,51.3269880344203,51.7618613372274,52.197587335454,52.6333133336805,
53.0681866363954,53.5030599390685,53.9379332417027,54.3728065443011,54.8076798468664,
55.2425531494018,55.6774264519101,56.1122997543943,56.5471730568575,56.9820463593026,
57.4169196617326,57.8517929641506,58.2866662665595,58.7215395689624,59.157265567009,
59.5929915650557,60.0278648674556,60.4627381698584,60.8976114722673,61.3324847746853,
61.7673580771153,62.2022313795604,62.6371046820236,63.0719779845079,63.5068512870162,
63.9417245895516,64.376597892117,64.8114711947155,65.2463444973499,65.6812178000231,
66.1169437982275,66.5526697964318,66.9875430991915,67.4224164019987,67.8572897048563,
68.2921630077673,68.7270363107343,69.1619096137603,69.5967829168479,70.0316562200001,
70.4665295232194,70.9014028265087,71.3362761298705,71.7711494333077,72.2060227368227,
72.6408960404182,73.0766220391044,73.5123480377905,73.9472213415547,74.382094645407,
74.8169679493499,75.2518412533859,75.6867145575172,76.1215878617464,76.5564611660756,
76.9913344705072,77.4262077750435,77.8610810796866,78.2959543844386,78.7308276893018,
79.1657009942781,79.6005742993696,80.0363002988208,80.4720262982719,80.9068996035997,
81.3417729090484,81.7766462146199,82.211519520316,82.6463928261383,83.0812661320886,
83.5161394381684,83.9510127443794,84.3858860507229,84.8207593572004,85.2556326638134,
85.6905059705631,86.1253792774507,86.5602525844776,86.995978584908,87.4317045853384,
87.8665778926469,88.3014512000977,88.7363245076919,89.1711978154302,89.6060711233134,
90.0409444313423,90.4758177395175,90.9106910478396,91.345564356309,91.7804376649263,
92.2153109736917,92.6501842826055,93.085057591668,93.5199309008791,93.9556569024059,
94.3913829039327,94.8262562134414,95.2611295230986,95.6960028329042,96.1308761428578,
96.5657494529591,97.0006227632077,97.4354960736028,97.870369384144,98.3052426948304,
98.7401160056612,99.1749893166354,99.6098626277522,100.04473593901,100.915335253024,
101.351061255639,101.785934567313,102.220807879124,102.655681191068,103.090554503145,
103.525427815353,104.395174440154,105.264921065453,105.699794378283,106.134667691232,
106.569541004295,107.004414317471,107.8750136343,108.745612951339,109.615359578629,
110.485106206296,111.354852834309,112.224599462639,113.094346091254,113.964092720119,
114.834692038763,115.705291357499,116.575037986826,117.444784616267,118.314531245777,
119.184277875311,120.054024504821,120.923771134261,121.794370453112,122.66496977189,
123.534716400968,124.404463029834,125.274209658448,126.143956286779,127.013702914792,
127.883449542458,128.754048859798,129.624648176939,130.494394803617,131.364141429857,
132.233888055637,133.103634680937,133.973381305737,134.843127930023,135.71372724472,
136.584326559147,137.019199870684,137.454073182083,137.888946493341,138.323819804458,
139.193566426263,140.063313047491,140.498186357887,140.933059668136,141.367932978237,
141.802806288191,142.237679597997,142.673405599673,143.109131601348,143.544004910857,
143.978878220217,144.413751529429,144.848624838491,145.283498147405,145.718371456171,
146.153244764789,146.588118073258,147.022991381581,147.457864689756,147.892737997785,
148.327611305669,148.762484613407,149.197357921002,149.633083921574,150.068809922147,
150.503683229455,150.938556536623,151.37342984365,151.808303150538,152.243176457288,
152.678049763901,153.112923070379,153.547796376722,153.982669682934,154.417542989014,
154.852416294964,155.287289600787,155.722162906483,156.157036212055,156.592762211626,
157.028488211198,157.463361516526,157.898234821735,158.333108126826,158.767981431803,
159.202854736666,159.637728041419,160.072601346062,160.507474650599,160.94234795503,
161.37722125936,161.812094563589,162.246967867721,162.681841171757,163.1167144757,
163.552440474473,163.988166473247,164.423039777011,164.85791308069,165.292786384286,
165.727659687801,166.162532991238,166.597406294601,167.03227959789,167.46715290111,
167.902026204262,168.33689950735,168.771772810376,169.206646113343,169.641519416254,
170.076392719112,170.512118717363,170.947844715614,171.382718018374,171.817591321089,
172.252464623762,172.687337926397,173.122211228996,173.557084531561,173.991957834097,
174.426831136606,174.86170443909,175.296577741554,175.731451044,176.16632434643,
176.601197648848,177.036070951258,177.471796949306,177.907522947355,178.342396249755,
178.777269552155,179.212142854558,179.647016156968,180.081889459386,180.516762761816,
180.951636064262,181.386509366726,181.82138266921,182.256255971719,182.691129274255,
183.12600257682,183.560875879419,183.995749182054,184.431475180237,184.867201178421,
185.302074481136,185.736947783896,186.171821086704,186.606694389561,187.041567692473,
187.47644099544,187.911314298466,188.346187601554,188.781060904706,189.215934207926,
189.650807511215,190.085680814577,190.520554118015,190.95542742153,191.391153420175,
191.82687941882,192.261752722499,192.696626026263,193.131499330116,193.566372634059,
194.001245938095,194.436119242227,194.870992546456,195.305865850785,195.740739155217,
196.175612459754,196.610485764397,197.045359069149,197.480232374013,197.915105678989,
198.350831678382,198.786557677775,199.221430982984,199.656304288312,200.091177593761,
200.526050899333,200.960924205029,201.395797510852,201.830670816802,202.265544122882,
202.700417429093,203.135290735437,203.570164041915,204.005037348528,204.439910655278,
204.874783962166,205.310509962526,205.746235962887,206.181109270054,206.615982577363,
207.050855884814,207.485729192409,207.920602500147,208.355475808031,208.79034911606,
209.225222424235,209.660095732558,210.094969041027,210.529842349645,210.96471565841,
211.399588967324,211.834462276387,212.27018827784,212.705914279292,213.140787588653,
213.575660898161,214.010534207819,214.880280827579,215.31515413768,215.750027447929,
216.184900758324,216.619774068866,217.054647379553,217.489520690384,218.359267312475,
219.22986662628,219.665592628826,220.100465940363,220.535339252038,220.970212563848,
221.83995918787,222.709705812416,223.579452437468,224.014325750179,224.44919906301,
225.318945689022,226.189545005688,227.060144322571,227.929890949664,228.799637577146,
229.66938420499,230.539130833166,231.408877461643,232.278624090388,233.149223408954,
234.019822727623,234.889569356878,235.759315986267,236.629062615749,237.498809245277,
238.368555874806,239.238302504287,240.108901823183,240.979501142017,241.849247771189,
242.718994400167,243.588741028911,244.458487657389,245.328234285565,246.197980913409,
247.068580230891,247.939179548182,248.80892617507,249.678672801532,250.548419427545,
251.418166053087,252.287912678139,253.157659302684,254.028258617581,254.898857932211,
255.333731243885,255.768604555423,256.203477866821,256.63835117808,257.508097800171,
258.377844421689,258.812717732231,259.247591042627,259.682464352876,260.117337662977,
260.552210972931,260.987936974682,261.858536286089,262.293409595598,262.728282904958,
263.16315621417,263.598029523233,264.032902832147,264.467776140913,264.902649449531,
265.337522758001,265.772396066323,266.207269374499,266.642142682528,267.077015990412,
267.511889298151,267.947615298795,268.383341299439,268.81821460689,269.2530879142,
269.687961221367,270.122834528394,270.557707835282,270.992581142032,271.427454448646,
271.862327755124,272.297201061468,272.732074367679,273.166947673759,273.60182097971,
274.036694285533,274.471567591229,274.907293590862,275.343019590495,275.777892895944,
276.212766201272,276.647639506481,277.082512811573,277.51738611655,277.952259421414,
278.387132726166,278.82200603081,279.256879335346,279.691752639779,280.126625944108,
280.561499248338,280.996372552469,281.431245856506,281.866971855324,282.302697854143,
282.737571157996,283.172444461761,283.60731776544,284.042191069036,284.477064372551,
284.911937675989,285.346810979351,285.781684282641,286.216557585861,286.651430889013,
287.086304192101,287.521177495128,287.956050798095,288.390924101007,288.826650099283,
289.262376097559,289.697249400366,290.132122703127,290.566996005842,291.001869308516,
291.43674261115,291.871615913749,292.306489216315,292.741362518851,293.17623582136,
293.611109123845,294.045982426308,294.480855728754,294.915729031185,295.350602333603,
295.786328331655,296.222054329707,296.65692763211,297.091800934511,297.526674236911,
297.961547539314,298.396420841724,298.831294144142,299.266167446573,299.701040749018,
300.135914051482,300.570787353967,301.005660656476,301.440533959012,301.875407261578,
302.310280564177,302.746006562341,303.181732560506,303.616605863179,304.051479165895,
304.486352468655,304.921225771462,305.35609907432,305.790972377232,306.225845680199,
306.660718983226,307.095592286314,307.530465589466,307.965338892686,308.400212195976,
308.835085499338,309.269958802776,309.705684801381,310.141410799985,310.576284103581,
311.01115740726,311.446030711025,311.880904014878,312.315777318821,312.750650622858,
313.185523926989,313.620397231219,314.055270535549,314.490143839981,314.925017144517,
315.359890449161,315.794763753913,316.229637058777,316.665363058112,317.101089057448,
317.53596236254,317.970835667749,318.405708973077,318.840582278526,319.275455584098,
319.710328889795,320.145202195618,320.580075501568,321.014948807648,321.44982211386,
321.884695420204,322.319568726682,322.754442033295,323.189315340045,323.625041340336,
324.060767340628,324.495640647655,324.930513954822,325.365387262131,325.800260569583,
326.235133877177,326.670007184916,327.1048804928,327.539753800829,327.974627109005,
328.409500417327,328.844373725797,329.279247034415,329.714120343181,330.148993652095,
330.584719653474,331.020445654852,331.455318964064,331.890192273424,332.325065582933,
332.759938892591,333.194812202397,333.629685512351,334.064558822453,334.499432132702,
334.934305443098,335.369178753639,335.804052064326,336.673798686132,337.108671997249,
337.544397999725,337.980124002201,338.4149973136,338.849870625137,339.284743936812,
340.154490560568,341.024237184854,341.459110497191,341.893983809655,342.328857122244,
342.763730434955,343.633477060735,344.504076377234,345.374675693955,346.244422320844,
347.114168948136,347.983915575803,348.853662203817,349.723408832148,350.593155460764,
351.463754779246,352.334354097839,353.204100727012,354.07384735634,354.943593985781,
355.813340615292,356.683087244827,357.552833874338,358.423433193272,359.294032512154,
360.163779141409,361.033525770489,361.903272399355,362.77301902797,363.642765656301,
364.512512284316,365.383111601936,366.253710919371,367.123457546465,367.993204173143,
368.862950799383,369.732697425164,370.602444050463,371.472190675265,372.342789990359,
373.21338930519,373.648262617,374.083135928675,374.952882551611,375.822629173987,
376.257502484962,376.692375795793,377.12724910648,377.562122417021,377.996995727417,
378.431869037666,378.866742347767,379.302468349591,379.738194351416,380.173067661222,
380.607940970879,381.042814280388,381.477687589749,381.91256089896,382.347434208023,
382.782307516937,383.217180825703,383.652054134321,384.086927442791,384.521800751113,
384.956674059289,385.391547367318,385.826420675202,386.262146675918,386.697872676635,
387.13274598423,387.567619291681,388.00249259899,388.437365906157,388.872239213185,
389.307112520073,389.741985826823,390.176859133436,390.611732439914,391.046605746258,
391.48147905247,391.91635235855,392.351225664501,392.786098970323,393.221824970019,
393.657550969714,394.092424275286,394.527297580735,394.962170886063,395.397044191272,
395.831917496364,396.266790801341,396.701664106204,397.136537410957,397.5714107156,
398.006284020137,398.441157324569,398.876030628899,399.310903933128,399.74577723726,
400.181503236126,400.617229234991,401.052102538934,401.486975842787,401.921849146551,
402.356722450231,402.791595753827,403.226469057342,403.66134236078,404.096215664142,
404.531088967432,404.965962270651,405.400835573804,405.835708876892,406.270582179918,
406.705455482886,407.141181481189,407.576907479491,408.01178078235,408.446654085157,
408.881527387917,409.316400690633,409.751273993306,410.186147295941,410.62102059854,
411.055893901106,411.490767203642,411.925640506151,412.360513808636,412.795387111099,
413.230260413545,413.665133715976,414.100859714032,414.536585712088,414.971459014498,
415.406332316901,415.841205619301,416.276078921702,416.710952224105,417.145825526515,
417.580698828933,418.015572131364,418.45044543381,418.885318736273,419.320192038758,
419.755065341267,420.189938643803,420.624811946369,421.060537944515,421.496263942662,
421.931137245297,422.36601054797,422.800883850686,423.235757153446,423.670630456253,
424.105503759112,424.540377062023,424.975250364991,425.410123668017,425.844996971105,
426.279870274258,426.714743577477,427.149616880767,427.584490184129,428.020216182695,
428.455942181261,428.890815484776,429.325688788373,429.760562092052,430.195435395816,
430.630308699669,431.065182003612,431.500055307649,431.93492861178,432.36980191601,
432.80467522034,433.239548524772,433.674421829309,434.109295133952,434.544168438705,
434.979894437984,435.415620437262,435.850493742239,436.285367047331,436.72024035254,
437.155113657869,437.589986963318,438.024860268889,438.459733574586,438.894606880409,
439.32948018636,439.76435349244,440.199226798651,440.634100104995,441.068973411473,
441.503846718087,441.939572718309,442.375298718531,442.810172025419,443.245045332447,
443.679918639614,444.114791946923,444.549665254374,444.984538561969,445.419411869708,
445.854285177591,446.289158485621,446.724031793796,447.158905102119,447.593778410589,
448.028651719207,448.463525027973,448.899251029277,449.334977030581,449.769850339644,
450.639596958216,451.074470267725,451.509343577383,451.944216887189,452.379090197143,
452.813963507244,453.248836817493,453.683710127889,454.118583438431,454.553456749117,
454.988330059949,455.423203370923,455.858929373329,456.294655375734,456.729528686993,
457.164401998391,457.599275309929,458.469021933414,458.90389524536,459.338768557437,
459.773641869646,460.208515181983,460.643388494447,461.078261807036,461.948008432578,
462.818607748906,463.689207065461,464.55895369214,465.428700319234,466.298446946716,
467.16819357456,468.037940202737,468.907686831215,469.778286149605,470.648885468116,
471.518632097196,472.388378726451,473.258125355841,474.127871985322,474.997618614851,
475.86736524438,476.737964563343,477.608563882265,478.478310511593,479.348057140765,
480.217803769743,481.087550398488,481.957297026966,482.827043655142,483.697642972895,
484.568242290469,485.43798891776,486.307735544649,487.177482171112,488.047228797125,
488.916975422667,489.78672204772,490.657321363009,491.09304736596,491.527920678038,
492.397667301793,493.267413925005,494.137160547663,494.57203385878,495.006907169755,
495.441780480586,495.876653791273,496.311527101814,496.74640041221,497.616999724357,
498.052725726255,498.487599036209,498.922472346015,499.357345655673,499.792218965182,
500.227092274542,500.661965583754,501.096838892816,501.531712201731,501.966585510497,
502.401458819114,502.836332127584,503.271205435907,503.706078744082,504.140952052112,
504.576678052901,505.01240405369,505.447277361429,505.882150669023,506.317023976474,
506.751897283783,507.186770590951,507.621643897978,508.056517204866,508.491390511616,
508.92626381823,509.361137124708,509.796010431052,510.230883737263,510.665757043344,
511.100630349294,511.536356349053,511.972082348811,512.406955654506,512.841828960076,
513.276702265523,513.711575570849,514.146448876056,514.581322181146,515.016195486121,
515.451068790983,515.885942095733,516.320815400375,516.75568870491,517.19056200934,
517.625435313668,518.060308617896,518.496034616807,518.931760615718,519.366633919752,
519.801507223694,520.236380527545,520.671253831307,521.106127134985,521.541000438579,
521.975873742092,522.410747045528,522.845620348888,523.280493652176,523.715366955394,
524.150240258545,524.585113561631,525.019986864656,525.455712862985,525.891438861313,
526.326312164223,526.761185467079,527.196058769885,527.630932072643,528.065805375356,
528.500678678029,528.935551980661,529.370425283258,529.805298585822,530.240171888356,
530.675045190863,531.109918493346,531.544791795808,531.979665098252,532.415391096312,
532.851117094373,533.285990396789,533.720863699197,534.155737001598,534.590610303997,
535.025483606395,535.460356908796,535.895230211204,536.330103513621,536.764976816049,
537.199850118493,537.634723420955,538.069596723438,538.504470025945,538.93934332848,
539.375069326608,539.810795324736,540.245668627333,540.680541929966,541.115415232637,
541.550288535351,541.985161838109,542.420035140915,542.854908443771,543.28978174668,
543.724655049646,544.15952835267,544.594401655757,545.029274958907,545.464148262125,
545.899021565413,546.334747563939,546.770473562465,547.205346865901,547.640220169415,
548.075093473009,548.509966776686,548.944840080449,549.3797133843,549.814586688241,
550.249459992276,550.684333296405,551.119206600633,551.554079904961,551.988953209391,
552.423826513926,552.858699818567,553.294425817789,553.73015181701,554.165025121872,
554.599898426846,555.034771731937,555.469645037144,555.90451834247,556.339391647917,
556.774264953487,557.209138259182,557.644011565003,558.078884870951,558.51375817703,
558.948631483239,559.383504789581,559.818378096058,560.254104096209,560.689830096361,
561.12470340311,561.559576709996,561.994450017021,562.429323324187,562.864196631494,
563.299069938943,563.733943246536,564.168816554273,564.603689862154,565.038563170182,
565.473436478355,565.908309786676,566.343183095144,566.77805640376,567.213782404988,
567.649508406216,568.084381715128,568.519255024189,568.954128333399,569.389001642757,
569.823874952264,570.258748261921,570.693621571725,571.128494881677,571.563368191777,
572.433114812417,572.867988122957,573.302861433642,573.737734744471,574.173460746804,
574.609186749136,575.044060060251,575.913806682904,576.783553306113,577.218426617922,
577.653299929865,578.08817324194,578.523046554147,579.392793178944,580.26253980424,
581.13313912039,581.568865123709,582.003738436771,582.87348506323,583.743231690115,
584.612978317402,585.482724945065,586.352471573076,587.222218201403,588.092817519691,
588.963416838109,589.833163467083,590.702910096251,591.572656725575,592.442403355013,
593.31214998452,594.181896614051,595.05249593303,595.92309525198,596.792841881366,
597.662588510618,598.532335139693,599.402081768556,600.271828397167,601.141575025495,
602.012174343369,602.882773661074,603.752520288553,604.622266915642,605.492013542317,
606.361760168553,607.23150679433,608.101253419626,608.971852735101,609.842452050322,
610.71219867434,611.581945297822,612.451691920754,612.886565232011,613.321438543126,
613.756311854099,614.191185164928,615.060931786153,615.931531098516,616.367257100486,
616.802130410586,617.237003720538,617.671877030342,618.106750339998,618.541623649505,
618.976496958863,619.411370268073,619.846243577134,620.281116886046,620.71599019481,
621.150863503426,621.585736811894,622.020610120214,622.455483428388,622.891209429248,
623.326935430108,623.761808737989,624.196682045726,624.631555353319,625.066428660769,
625.501301968075,625.936175275241,626.371048582266,626.805921889153,627.240795195901,
627.675668502512,628.110541808988,628.54541511533,628.98028842154,629.415161727618,
629.850887727438,630.286613727259,630.72148703308,631.156360338774,631.591233644344,
632.026106949791,632.460980255118,632.895853560325,633.330726865415,633.76560017039,
634.200473475251,634.635346780002,635.070220084644,635.505093389179,635.939966693609,
636.374839997937,636.810565996897,637.246291995857,637.681165299986,638.116038604021,
638.550911907962,638.985785211813,639.420658515576,639.855531819253,640.290405122847,
640.725278426361,641.160151729796,641.595025033157,642.029898336444,642.464771639662,
642.899644942813,643.334518245899,643.770244244257,644.205970242616,644.640843545581,
645.075716848491,645.510590151347,645.945463454153,646.380336756911,646.815210059625,
647.250083362296,647.684956664929,648.119829967526,648.55470327009,648.989576572624,
649.424449875131,649.859323177614,650.294196480076,650.729922478144,651.165648476212,
651.600521778641,652.035395081057,652.470268383465,652.905141685866,653.340014988265,
653.774888290663,654.209761593065,654.644634895472,655.079508197889,655.514381500318,
655.949254802762,656.384128105224,656.819001407706,657.253874710213,657.689600708326,
658.12532670644,658.560200009004,658.995073311601,659.429946614234,659.864819916905,
660.299693219619,660.734566522377,661.169439825183,661.604313128039,662.039186430948,
662.474059733914,662.908933036938,663.343806340025,663.778679643175,664.213552946393,
664.649278944883,665.085004943373,665.519878246733,665.954751550169,666.389624853683,
666.824498157277,667.259371460954,667.694244764717,668.129118068568,668.563991372509,
668.998864676544,669.433737980674,669.868611284901,670.303484589229,670.738357893659,
671.173231198194,671.608957197361,672.044683196528,672.479556501278,672.91442980614,
673.349303111115,673.784176416205,674.219049721412,674.653923026738,675.088796332185,
675.523669637755,675.95854294345,676.393416249271,676.82828955522,677.263162861298,
677.698036167508,678.13290947385,678.568635473934,679.004361474018,679.439234780629,
679.874108087377,680.308981394264,680.743854701289,681.178728008455,681.613601315762,
682.048474623211,682.483347930804,682.91822123854,683.353094546422,683.78796785445,
684.222841162623,684.657714470944,685.092587779412,685.528313780566,685.96403978172,
686.398913090483,686.833786399396,687.268659708457,687.703533017666,688.138406327025,
688.573279636532,689.008152946187,689.443026255992,689.877899565944,690.312772876043,
690.74764618629,691.182519496684,691.617392807224,692.052266117909,692.487992120169,
692.92371812243,693.358591433403,694.228338055774,694.663211367171,695.098084678707,
695.532957990379,695.967831302188,696.402704614131,696.837577926207,697.707324550749,
698.577071175797,699.011944488507,699.447670491767,699.883396495028,700.318269807975,
701.188016434211,702.057763060886,702.927509687976,703.797256315454,704.667002943295,
705.536749571467,706.407348889651,707.277948207973,708.147694836835,709.017441465911,
709.887188095163,710.756934724548,711.626681354026,712.496427983551,713.367027302543,
714.237626621516,715.107373250954,715.977119880277,716.846866509446,717.716613138419,
718.586359767161,719.456106395635,720.32670571363,721.197305031464,722.067051659126,
722.936798286414,723.806544913299,724.676291539758,725.546038165767,726.415784791305,
727.286384106969,728.156983422381,729.026730046663,729.896476670415,730.331349982088,
730.766223293624,731.201096605021,731.635969916278,732.505716538366,733.37546315988,
733.81033647042,734.246062472462,734.681788474505,735.116661784752,735.551535094852,
735.986408404804,736.421281714608,736.856155024264,737.291028333771,737.72590164313,
738.160774952339,738.5956482614,739.030521570312,739.465394879076,739.900268187692,
740.33514149616,740.77001480448,741.205740805414,741.641466806347,742.076340114374,
742.511213422256,742.946086729993,743.380960037585,743.815833345035,744.250706652341,
744.685579959507,745.120453266533,745.555326573419,745.990199880167,746.425073186778,
746.859946493254,747.294819799596,747.729693105806,748.165419105691,748.601145105576,
749.036018411525,749.470891717346,749.90576502304,750.34063832861,750.775511634057,
751.210384939384,751.645258244591,752.080131549682,752.515004854656,752.949878159518,
753.384751464269,753.81962476891,754.254498073445,754.689371377875,755.125097376885,
755.560823375895,755.995696680123,756.430569984253,756.865443288287,757.300316592228,
757.735189896079,758.170063199842,758.604936503519,759.039809807113,759.474683110627,
759.909556414062,760.344429717423,760.779303020711,761.214176323929,761.649049627079,
762.084775625469,762.520501623858,762.955374926883,763.390248229848,763.825121532758,
764.259994835614,764.694868138419,765.129741441178,765.564614743891,765.999488046563,
766.434361349196,766.869234651793,767.304107954357,767.738981256891,768.173854559398,
768.608727861881,769.044453859958,769.480179858035,769.915053160479,770.349926462907,
770.784799765324,771.219673067731,771.654546370133,772.089419672531,772.52429297493,
772.959166277331,773.394039579739,773.828912882155,774.263786184584,774.698659487028,
775.13353278949,775.568406091973,776.004132090072,776.439858088172,776.874731390706,
777.30960469327,777.744477995867,778.1793512985,778.614224601171,779.049097903885,
779.483971206643,779.918844509449,780.353717812305,780.788591115215,781.22346441818,
781.658337721205,782.093211024291,782.528084327442,782.963810325897,783.399536324352,
783.834409627639,784.269282931,784.704156234435,785.139029537949,785.573902841543,
786.00877614522,786.443649448983,786.878522752834,787.313396056775,787.74826936081,
788.183142664939,788.618015969167,789.052889273495,789.487762577925,789.923488577038,
790.359214576152,790.794087880793,791.228961185544,791.663834490406,792.098707795381,
792.533581100471,792.968454405678,793.403327711004,793.838201016451,794.273074322021,
794.707947627716,795.142820933537,795.577694239486,796.012567545564,796.447440851774,
796.883166851791,797.318892851808,797.753766158284,798.188639464895,798.623512771643,
799.058386078529,799.493259385555,799.92813269272,800.363006000027,800.797879307477,
801.232752615069,801.667625922806,802.102499230688,802.537372538715,802.972245846889,
803.40711915521,803.84284515629,804.27857115737,804.713444465985,805.148317774749,
805.583191083662,806.018064392723,806.452937701933,806.887811011291,807.322684320798,
808.192430940258,808.62730425021,809.06217756031,809.497050870557,809.931924180951,
810.36679749149,810.802523493679,811.238249495867,811.673122806697,812.542869428785,
812.977742740041,813.412616051438,813.847489362974,814.282362674646,814.717235986455,
815.152109298398,816.021855922681,816.891602547478,817.326475860065,817.762201863265,
818.197927866466,818.632801179295,819.502547805304,820.372294431763,821.242041058648,
822.111787685935,822.981534313598,823.851280941609,824.721880259681,825.5924795779,
826.462226206642,827.331972835616,828.201719464785,829.071466094109,829.941212723546,
830.810959353053,831.681558672047,832.552157991036,833.421904620514,834.2916512499,
835.161397879151,836.031144508226,836.900891137089,837.770637765701,838.641237083811,
839.511836401767,840.381583029608,841.251329657086,842.121076284176,842.990822910851,
843.860569537087,844.730316162863,845.600915478712,846.471514794314,847.341261418855,
848.211008042874,848.645881354683,849.080754666356,849.515627977891,849.950501289288,
850.82024791166,851.689994533462,852.124867844147,852.560593846263,852.996319848379,
853.431193158772,853.866066469019,854.300939779119,855.170686398875,855.605559708531,
856.040433018038,856.475306327397,856.910179636606,857.345052945667,857.77992625458,
858.214799563344,858.64967287196,859.084546180427,859.520272181434,859.95599818244,
860.390871490614,860.825744798641,861.260618106523,861.69549141426,862.130364721852,
862.565238029302,863.000111336609,863.434984643774,863.8698579508,864.304731257686,
864.739604564434,865.174477871045,865.609351177521,866.044224483863,866.479950483814,
866.915676483765,867.350549789843,867.785423095792,868.220296401613,868.655169707307,
869.090043012877,869.524916318325,869.959789623651,870.394662928858,870.829536233948,
871.264409538923,871.699282843785,872.134156148535,872.569029453177,873.003902757712,
873.439628756773,873.875354755834,874.310228060162,874.745101364389,875.179974668519,
875.614847972553,876.049721276495,876.484594580346,876.919467884108,877.354341187786,
877.78921449138,878.224087794893,878.658961098329,879.093834401689,879.528707704977,
879.963581008195,880.399307006616,880.835033005038,881.269906308124,881.704779611148,
882.139652914114,882.574526217024,883.00939951988,883.444272822685,883.879146125444,
884.314019428157,884.748892730829,885.183766033462,885.618639336059,886.053512638623,
886.488385941157,886.923259243664,887.358985241751,887.794711239839,888.2295845423,
888.664457844744,889.099331147173,889.534204449589,889.969077751997,890.403951054398,
890.838824356797,891.273697659195,891.708570961597,892.143444264004,892.578317566421,
893.01319086885,893.448064171293,893.882937473755,894.318663471843,894.75438946993,
895.189262772437,895.624136074971,896.059009377535,896.493882680132,896.928755982765,
897.363629285437,897.798502588151,898.233375890909,898.668249193715,899.103122496571,
899.53799579948,899.972869102446,900.40774240547,900.842615708556,901.278341706978,
901.714067705399,902.148941008617,902.583814311905,903.018687615265,903.453560918701,
903.888434222214,904.323307525808,904.758180829485,905.193054133248,905.627927437099,
906.06280074104,906.497674045075,906.932547349205,907.367420653433,907.80229395776,
908.238019956821,908.673745955883,909.108619260417,909.543492565059,909.978365869809,
910.413239174671,910.848112479646,911.282985784736,911.717859089943,912.152732395269,
912.587605700716,913.022479006287,913.457352311981,913.892225617802,914.327098923751,
914.761972229829,915.19769822978,915.633424229731,916.068297536072,916.503170842548,
916.93804414916,917.372917455908,917.807790762794,918.24266406982,918.677537376985,
919.112410684292,919.547283991742,919.982157299334,920.417030607071,920.851903914953,
921.28677722298,921.721650531154,922.15737653216,922.593102533167,923.027975841635,
923.46284915025,923.897722459014,924.332595767926,924.767469076987,925.202342386197,
925.637215695556,926.072089005063,926.506962314719,926.941835624523,927.376708934475,
927.811582244575,928.246455554822,928.681328865215,929.117054867331,929.987654180132,
930.422527490961,930.857400801934,931.292274113049,931.727147424306,932.162020735703,
932.596894047238,933.46664067072,934.336387294739,934.771260606945,935.20613391928,
935.641007231742,936.076733234882,936.94733255073,937.817079176507,938.686825802743,
939.556572429418,940.426319056508,941.296065683986,942.165812311827,943.036411629783,
943.907010947893,944.776757576505,945.646504205367,946.516250834443,947.385997463694,
948.25574409308,949.125490722558,949.996090041546,950.86668936054,951.736435990048,
952.606182619485,953.475929248809,954.345675877978,955.215422506951,956.085169135693,
956.955768453912,957.826367771985,958.696114399995,959.565861027658,960.435607654946,
961.305354281831,962.175100908289,963.044847534298,963.915446850328,964.786046166116,
965.655792790913,966.525539415195,966.960412727138,967.395286038947,968.265032662155,
969.134779284809,969.569652595924,970.004525906897,970.439399217726,970.875125219914,
971.310851222103,971.745724532643,972.615471153283,973.485217773335,973.920091083139,
974.354964392795,974.789837702302,975.22471101166,975.65958432087,976.094457629931,
976.529330938844,976.964204247608,977.399077556223,977.834803557303,978.270529558383,
978.705402866704,979.140276174877,979.575149482905,980.010022790786,980.444896098523,
980.879769406116,981.314642713565,981.749516020872,982.184389328038,982.619262635063,
983.05413594195,983.489009248698,983.923882555309,984.358755861785,984.794481861802,
985.230207861819,985.665081168029,986.099954474107,986.534827780056,986.969701085877,
987.404574391571,987.839447697141,988.274321002589,988.709194307915,989.144067613122,
989.578940918212,990.013814223187,990.448687528048,990.883560832799,991.31843413744,
991.754160136554,992.189886135667,992.624759440097,993.059632744425,993.494506048653,
993.929379352783,994.364252656817,994.799125960758,995.233999264609,995.668872568372,
996.103745872049,996.538619175643,996.973492479157,997.408365782593,997.843239085953,
998.278112389241,998.713838387696,999.149564386151,999.584437689301,1000.01931099239,
1000.45418429541,1000.88905759838,1001.32393090129,1001.75880420414,1002.19367750695,
1002.62855080971,1003.06342411242,1003.49829741509,1003.93317071773,1004.36804402032,
1004.80291732289,1005.23779062542,1005.67351662352,1006.10924262162,1006.5441159241,
1006.97898922656,1007.41386252901,1007.84873583144,1008.28360913385,1008.71848243626,
1009.15335573866,1009.58822904106,1010.02310234346,1010.45797564586,1010.89284894827,
1011.32772225069,1011.76259555311,1012.19746885556,1012.63319485364,1013.06892085171,
1013.5037941542,1013.9386674567,1014.37354075924,1014.8084140618,1015.2432873644,
1015.67816066703,1016.1130339697,1016.54790727242,1016.98278057517,1017.41765387798,
1017.85252718084,1018.28740048375,1018.72227378671,1019.15714708974,1019.59287308813,
1020.02859908651,1020.46347238967,1020.89834569288,1021.33321899617,1021.76809229953,
1022.20296560297,1022.63783890648,1023.07271221007,1023.50758551375,1023.94245881752,
1024.37733212137,1024.81220542531,1025.24707872935,1025.68195203348,1026.11682533771,
1026.55255133672,1026.98827733573,1027.42315064016,1027.8580239447,1028.29289724934,
1028.72777055409,1029.16264385896,1029.59751716393,1030.03239046902,1030.46726377423,
1030.90213707956,1031.33701038501,1031.77188369058,1032.20675699628,1032.6416303021,
1033.07650360805,1033.51222960793,1033.94795560782,1034.38282891403,1034.81770222038,
1035.25257552685,1035.68744883347,1036.12232214022,1036.5571954471,1036.99206875413,
1037.4269420613,1037.86181536861,1038.29668867606,1038.73156198365,1039.16643529139,
1039.60130859927,1040.0361819073,1040.47190790824,1040.90763390917,1041.34250721749,
1041.77738052596,1042.21225383458,1042.64712714334,1043.08200045226,1043.95174707053,
1044.38662037989,1044.8214936894,1045.25636699906,1045.69124030886,1046.12611361882,
1046.56098692892,1046.99586023917,1047.43158624121,1047.86731224325,1048.3021855538,
1048.73705886448,1049.17193217531,1049.60680548629,1050.0416787974,1050.47655210866,
1050.91142542006,1051.78117204327,1052.21604535508,1052.65091866703,1053.0857919791,
1053.52066529131,1053.95553860365,1054.39126460673,1055.26186392239,1056.13161054793,
1057.00135717395,1057.43623048712,1057.87110380041,1058.7408504273,1059.61059705459,
1060.48034368225,1061.35094300009,1062.22154231809,1063.09128894656,1063.96103557531,
1064.83078220429,1065.70052883346,1066.57027546278,1067.44002209222,1068.3106214112,
1069.18122073019,1070.05096735972,1070.9207139892,1071.79046061859,1072.66020724785,
1073.52995387693,1074.39970050579,1075.27029982411,1076.1408991423,1077.01064577048,
1077.88039239832,1078.7501390258,1079.61988565289,1080.48963227957,1081.35937890581,
1082.22997822202,1083.100577538,1083.97032416305,1084.84007078759,1085.70981741161,
1086.5795640351,1087.44931065803,1087.88418396929,1088.31905728041,1088.75393059138,
1089.18965659365,1089.62538259591,1090.06025590659,1090.93000252753,1091.36487583778,
1091.79974914788,1092.23462245783,1092.66949576764,1093.1043690773,1093.5392423868,
1093.97411569616,1094.40898900538,1094.84386231444,1095.27873562335,1095.71360893212,
1096.14933493327,1096.58506093443,1097.0199342429,1097.45480755122,1097.88968085939,
1098.32455416742,1098.75942747531,1099.19430078305,1099.62917409064,1100.06404739809,
1100.4989207054,1100.93379401257,1101.36866731959,1101.80354062648,1102.23841393323,
1102.67328723984,1103.10901323993,1103.54473924001,1103.97961254636,1104.41448585257,
1104.84935915865,1105.2842324646,1105.71910577042,1106.15397907612,1106.58885238169,
1107.02372568714,1107.45859899246,1107.89347229767,1108.32834560276,1108.76321890774,
1109.1980922126,1109.63296551736,1110.06869151652,1110.50441751569,1110.93929082023,
1111.37416412466,1111.80903742899,1112.24391073322,1112.67878403735,1113.11365734139,
1113.54853064533,1113.98340394918,1114.41827725295,1114.85315055662,1115.28802386022,
1115.72289716374,1116.15777046717,1116.59264377053,1117.02836976903,1117.46409576752,
1117.89896907074,1118.33384237389,1118.76871567698,1119.20358898,1119.63846228297,
1120.07333558588,1120.50820888874,1120.94308219154,1121.3779554943,1121.81282879702,
1122.24770209969,1122.68257540233,1123.11744870492,1123.55232200749,1123.98804800561,
1124.42377400372,1124.85864730623,1125.29352060871,1125.72839391118,1126.16326721362,
1126.59814051605,1127.03301381847,1127.46788712088,1127.90276042328,1128.33763372568,
1128.77250702808,1129.20738033048,1129.64225363289,1130.07712693531,1130.51200023774,
1130.94772623581,1131.38345223388,1131.81832553634,1132.25319883883,1132.68807214134,
1133.12294544387,1133.55781874644,1133.99269204904,1134.42756535167,1134.86243865434,
1135.29731195706,1135.73218525982,1136.16705856263,1136.60193186548,1137.03680516839,
1137.47167847136,1137.90740446972,1138.34313046808,1138.77800377117,1139.21287707432,
1139.64775037754,1140.08262368083,1140.51749698419,1140.95237028763,1141.38724359114,
1141.82211689474,1142.25699019842,1142.69186350218,1143.12673680603,1143.56161010998,
1143.99648341401,1144.43135671814,1144.86708271711,1145.30280871607,1145.7376820204,
1146.17255532483,1146.60742862936,1147.04230193401,1147.47717523876,1147.91204854362,
1148.3469218486,1148.78179515369,1149.2166684589,1149.65154176423,1150.08641506968,
1150.52128837525,1150.95616168094,1151.39103498677,1151.82676098659,1152.26248698641,
1152.69736029249,1153.1322335987,1153.56710690504,1154.00198021152,1154.43685351813,
1154.87172682488,1155.30660013177,1155.7414734388,1156.17634674597,1156.61122005327,
1157.04609336073,1157.48096666832,1157.91583997606,1158.35071328394,1158.7864392848,
1159.22216528566,1159.65703859384,1160.09191190216,1160.52678521063,1160.96165851925,
1161.39653182801,1161.83140513693,1162.26627844599,1162.7011517552,1163.13602506456,
1163.57089837407,1164.00577168373,1164.44064499353,1164.87551830349,1165.74611761556,
1166.18184361753,1166.61671692792,1167.05159023846,1167.48646354915,1167.92133685998,
1168.35621017096,1169.22595679333,1170.09570341627,1170.53057672794,1170.96545003975,
1171.4003233517,1171.83519666377,1172.27006997598,1172.705795979,1173.57639529447,
1174.44614191977,1174.8810152326,1175.31588854555,1176.18563517179,1177.05538179847,
1177.92512842556,1178.79487505304,1179.66547437075,1180.53607368863,1181.40582031696,
1182.27556694557,1183.14531357444,1184.01506020352,1184.88480683277,1185.75455346216,
1186.62515278112,1187.4957521001,1188.36549872963,1189.23524535914,1190.10499198858,
1190.97473861791,1191.84448524708,1192.71423187606,1193.58483119448,1194.45543051277,
1195.3251771411,1196.19492376911,1197.06467039678,1197.93441702407,1198.80416365096,
1199.67391027742,1200.5445095938,1201.41510890996,1202.28485553525,1203.15460216005,
1204.02434878434,1204.89409540809,1205.76384203131,1206.1987153427,1206.63358865396,
1207.06846196508,1207.50418796741,1208.37478728058,1209.2445339018,1209.6794072122,
1210.11428052245,1210.54915383255,1210.9840271425,1211.41890045231,1211.85377376197,
1212.28864707147,1212.72352038083,1213.15839369005,1213.59326699911,1214.02814030802,
1214.46386630925,1214.89959231048,1215.3344656191,1215.76933892757,1216.20421223589,
1216.63908554406,1217.07395885209,1217.50883215998,1217.94370546771,1218.37857877531,
1218.81345208276,1219.24832539007,1219.68319869724,1220.11807200426,1220.55294531115,
1220.9878186179,1221.42354461805,1221.85927061821,1222.29414392468,1222.72901723103,
1223.16389053724,1223.59876384332,1224.03363714927,1224.46851045509,1224.90338376079,
1225.33825706636,1225.77313037181,1226.20800367713,1226.64287698234,1227.07775028743,
1227.51262359241,1227.94749689727,1228.3832228965,1228.81894889572,1229.25382220036,
1229.6886955049,1230.12356880933,1230.55844211366,1230.99331541789,1231.42818872202,
1231.86306202606,1232.29793533,1232.73280863385,1233.16768193762,1233.60255524129,
1234.03742854489,1234.4723018484,1234.90717515184,1235.34290115037,1235.7786271489,
1236.21350045219,1236.64837375541,1237.08324705856,1237.51812036165,1237.95299366467,
1238.38786696764,1238.82274027055,1239.25761357341,1239.69248687621,1240.12736017897,
1240.56223348169,1240.99710678436,1241.431980087,1241.8668533896,1242.30257938773,
1242.73830538585,1243.17317868839,1243.6080519909,1244.04292529338,1244.47779859585,
1244.91267189829,1245.34754520072,1245.78241850314,1246.21729180555,1246.65216510795,
1247.08703841035,1247.52191171275,1247.95678501515,1248.39165831756,1248.82653161998,
1249.26225761804,1249.69798361611,1250.13285691855,1250.56773022101,1251.0026035235,
1251.43747682601,1251.87235012854,1252.30722343111,1252.74209673371,1253.17697003634,
1253.61184333901,1254.04671664173,1254.48158994449,1254.9164632473,1255.35133655015,
1255.78620985306,1256.22193585139,1256.65766184973,1257.09253515275,1257.52740845584,
1257.96228175899,1258.39715506221,1258.8320283655,1259.26690166886,1259.7017749723,
1260.13664827581,1260.57152157941,1261.00639488309,1261.44126818685,1261.8761414907,
1262.31101479465,1262.74588809868,1263.1816140976,1263.61734009651,1264.05221340074,
1264.48708670507,1264.9219600095,1265.35683331403,1265.79170661868,1266.22657992343,
1266.66145322829,1267.09632653327,1267.53119983836,1267.96607314357,1268.4009464489,
1268.83581975434,1269.27069305992,1269.70556636561,1270.14129236537,1270.57701836513,
1271.01189167108,1271.44676497716,1271.88163828337,1272.31651158971,1272.75138489619,
1273.1862582028,1273.62113150955,1274.05600481644,1274.49087812347,1274.92575143063,
1275.36062473794,1275.79549804539,1276.23037135299,1276.66524466073,1277.10097066151,
1277.5366966623,1277.97156997033,1278.40644327851,1278.84131658683,1279.2761898953,
1279.71106320392,1280.14593651268,1280.5808098216,1281.01568313066,1281.45055643987,
1281.88542974923,1282.32030305874,1282.75517636839,1283.1900496782,1283.62492298815,
1284.06064899005,1284.49637499195,1284.9312483022,1285.36612161259,1285.80099492313,
1286.23586823382,1286.67074154465,1287.54048816674,1287.975361478,1288.4102347894,
1288.84510810093,1289.27998141261,1289.71485472442,1290.14972803636,1291.02032735139,
1291.89092666668,1292.32579997914,1292.76067329173,1293.19554660444,1293.63041991727,
1294.50016654328,1295.36991316974,1296.23965979663,1297.10940642392,1297.9800057415,
1298.85060505925,1299.72035168742,1300.5900983159,1301.45984494464,1302.32959157362,
1303.19933820279,1304.06908483212,1304.93968415104,1305.81028347,1306.68003009953,
1307.54977672906,1308.41952335854,1309.28926998793,1310.15901661718,1311.02876324626,
1311.89936256477,1312.76996188316,1313.63970851164,1314.50945513981,1315.37920176765,
1316.24894839514,1317.11869502223,1317.98844164891,1318.85904096546,1319.72964028179,
1320.59938690733,1321.46913353238,1322.33888015692,1323.20862678095,1323.64350009276,
1324.07837340443,1324.51324671597,1324.94812002737,1325.81871934103,1326.68931865441,
1327.12419196524,1327.55906527593,1327.99393858647,1328.42881189686,1328.86368520711,
1329.29855851721,1329.73343182716,1330.16830513697,1330.60317844663,1331.03805175614,
1331.4729250655,1331.90779837471,1332.34267168377,1332.77839768507,1333.21412368638,
1333.64899699514,1334.08387030376,1334.51874361223,1334.95361692055,1335.38849022873,
1335.82336353676,1336.25823684464,1336.69311015238,1337.12798345997,1337.56285676742,
1337.99773007473,1338.4326033819,1338.86747668892,1339.30234999581,1339.73807599603,
1340.17380199625,1340.60867530287,1341.04354860934,1341.47842191569,1341.9132952219,
1342.34816852798,1342.78304183393,1343.21791513975,1343.65278844545,1344.08766175102,
1344.52253505647,1344.95740836179,1345.392281667,1345.82715497209,1346.26202827707,
1346.69775427635,1347.13348027563,1347.56835358038,1348.00322688502,1348.43810018956,
1348.87297349399,1349.30784679832,1349.74272010255,1350.17759340668,1350.61246671072,
1351.04734001466,1351.48221331851,1351.91708662228,1352.35195992595,1352.78683322955,
1353.22170653306,1353.65743253163,1354.09315853019,1354.52803183356,1354.96290513685,
1355.39777844007,1355.83265174322,1356.26752504631,1356.70239834933,1357.1372716523,
1357.57214495521,1358.00701825807,1358.44189156087,1358.87676486363,1359.31163816635,
1359.74651146902,1360.18138477166,1360.6171107698,1361.05283676795,1361.48771007051,
1361.92258337305,1362.35745667556,1362.79232997804,1363.2272032805,1363.66207658295,
1364.09694988538,1364.5318231878,1364.96669649021,1365.40156979261,1365.83644309501,
1366.27131639741,1366.70618969981,1367.14106300222,1367.57678900028,1368.01251499834,
1368.44738830077,1368.88226160321,1369.31713490567,1369.75200820816,1370.18688151067,
1370.6217548132,1371.05662811577,1371.49150141837,1371.926374721,1372.36124802367,
1372.79612132639,1373.23099462915,1373.66586793196,1374.10074123481,1374.53646723311,
1374.97219323142,1375.40706653438,1375.84193983741,1376.2768131405,1376.71168644365,
1377.14655974687,1377.58143305016,1378.01630635352,1378.45117965696,1378.88605296047,
1379.32092626407,1379.75579956775,1380.19067287151,1380.62554617536,1381.06041947931,
1381.49614547817,1381.93187147704,1382.36674478117,1382.8016180854,1383.23649138973,
1383.67136469416,1384.10623799869,1384.54111130334,1384.97598460809,1385.41085791295,
1385.84573121793,1386.28060452302,1386.71547782823,1387.15035113356,1387.585224439,
1388.02009774458,1388.45582374427,1388.89154974397,1389.32642304979,1389.76129635574,
1390.19616966182,1390.63104296803,1391.06591627437,1391.50078958085,1391.93566288746,
1392.37053619421,1392.8054095011,1393.24028280813,1393.6751561153,1394.1100294226,
1394.54490273005,1394.97977603765,1395.41550203836,1395.85122803908,1396.28610134696,
1396.72097465499,1397.15584796317,1397.59072127149,1398.02559457996,1398.46046788858,
1398.89534119734,1399.33021450626,1399.76508781532,1400.19996112453,1400.63483443389,
1401.50458105306,1401.93945436286,1402.37518036469,1402.81090636651,1403.24577967661,
1403.68065298686,1404.11552629725,1404.5503996078,1404.98527291848,1405.85501954029,
1406.2898928514,1406.72476616266,1407.15963947406,1407.5945127856,1408.02938609727,
1408.46425940908,1409.33485872391,1410.205458039,1410.64033135134,1411.07520466381,
1411.51007797639,1411.9449512891,1412.81469791488,1413.68444454112,1414.5541911678,
1415.42393779489,1416.29453711233,1417.16513642995,1418.03488305796,1418.90462968629,
1419.77437631491,1420.64412294377,1421.51386957285,1422.38361620211,1423.25421552099,
1424.12481483992,1424.99456146943,1425.86430809896,1426.73405472847,1427.60380135791,
1428.47354798724,1429.34329461641,1430.21389393501,1431.08449325349,1431.9542398821,
1432.82398651043,1433.69373313844,1434.56347976611,1435.4332263934,1436.30297302029,
1437.17357233701,1438.04417165351,1438.91391827929,1439.78366490459,1440.65341152939,
1441.52315815367,1441.95803146562,1442.39290477743,1442.8277780891,1443.26265140064,
1444.13325071451,1445.00385002811,1445.43872333908,1445.87359664991,1446.3084699606,
1446.74334327114,1447.17821658153,1447.61308989178,1448.48283651184,1448.91770982164,
1449.3525831313,1449.78745644081,1450.22232975017,1450.65720305938,1451.09292906076,
1451.52865506214,1451.96352837105,1452.39840167982,1452.83327498843,1453.2681482969,
1453.70302160522,1454.1378949134,1454.57276822143,1455.00764152931,1455.44251483705,
1455.87738814464,1456.31226145209,1456.7471347594,1457.18200806657,1457.6168813736,
1458.05260737389,1458.48833337418,1458.92320668093,1459.35807998754,1459.79295329402,
1460.22782660036,1460.66269990657,1461.09757321265,1461.5324465186,1461.96731982443,
1462.40219313012,1462.83706643569,1463.27193974114,1463.70681304647,1464.14168635168,
1464.57655965677,1465.0122856561,1465.44801165544,1465.8828849603,1466.31775826505,
1466.7526315697,1467.18750487423,1467.62237817866,1468.05725148299,1468.49212478722,
1468.92699809135,1469.36187139539,1469.79674469933,1470.23161800319,1470.66649130695,
1471.10136461063,1471.53623791422,1471.97196391283,1472.40768991143,1472.84256321487,
1473.27743651823,1473.71230982152,1474.14718312474,1474.58205642789,1475.01692973098,
1475.451803034,1475.88667633697,1476.32154963988,1476.75642294274,1477.19129624555,
1477.62616954831,1478.06104285102,1478.4959161537,1478.93164215186,1479.36736815002,
1479.80224145262,1480.23711475519,1480.67198805772,1481.10686136023,1481.54173466272,
1481.97660796518,1482.41148126762,1482.84635457005,1483.28122787247,1483.71610117488,
1484.15097447728,1484.58584777968,1485.02072108208,1485.45559438449,1485.89132038254,
1486.32704638059,1486.76191968301,1487.19679298544,1487.63166628788,1488.06653959035,
1488.50141289283,1488.93628619534,1489.37115949787,1489.80603280044,1490.24090610304,
1490.67577940567,1491.11065270835,1491.54552601106,1491.98039931382,1492.41527261663,
1492.8509986149,1493.28672461318,1493.72159791609,1494.15647121906,1494.59134452208,
1495.02621782517,1495.46109112832,1495.89596443154,1496.33083773483,1496.76571103819,
1497.20058434163,1497.63545764515,1498.07033094874,1498.50520425242,1498.94007755618,
1499.37495086004,1499.81067685885,1500.24640285767,1500.68127616171,1501.11614946584,
1501.55102277007,1501.9858960744,1502.42076937883,1502.85564268337,1503.29051598801,
1503.72538929276,1504.16026259762,1504.5951359026,1505.03000920769,1505.4648825129,
1505.89975581823,1506.33462912368,1506.77035512331,1507.20608112294,1507.64095442864,
1508.07582773446,1508.51070104041,1508.94557434649,1509.3804476527,1509.81532095904,
1510.25019426552,1510.68506757213,1511.11994087888,1511.55481418577,1511.9896874928,
1512.42456079996,1512.85943410727,1513.29430741472,1513.73003341537,1514.16575941601,
1514.60063272375,1515.03550603163,1515.47037933966,1515.90525264784,1516.34012595616,
1516.77499926463,1517.20987257325,1517.64474588201,1518.07961919093,1518.51449249999,
1518.9493658092,1519.38423911856,1519.81911242807,1520.25398573772,1520.68971173947,
1521.12543774122,1521.56031105118,1521.99518436128,1522.43005767153,1523.29980429246,
1523.73467760315,1524.16955091398,1524.60442422495,1525.03929753607,1525.47417084733,
1525.90904415873,1526.77879078194,1527.64939009657,1528.08511609939,1528.51998941146,
1528.95486272367,1529.38973603601,1530.25948266106,1531.1292292866,1531.99897591261,
1532.86872253907,1533.73846916596,1534.60906848325,1535.47966780073,1536.34941442858,
1537.21916105675,1538.08890768523,1538.95865431398,1539.82840094295,1540.69814757212,
1541.56874689096,1542.43934620985,1543.30909283933,1544.17883946886,1545.04858609839,
1545.91833272787,1546.78807935726,1547.65782598651,1548.52842530518,1549.39902462375,
1550.26877125249,1551.13851788097,1552.00826450914,1552.87801113699,1553.74775776447,
1554.61750439156,1555.48810370844,1556.35870302511,1557.22844965112,1558.09819627666,
1558.96794290171,1559.83768952626,1560.27256283834,1560.70743615028,1561.57718277377,
1562.44778208785,1563.31838140165,1563.75325471277,1564.18812802374,1564.62300133457,
1565.05787464526,1565.9276212662,1566.79736788655,1567.2322411965,1567.66711450631,
1568.10198781596,1568.53686112547,1568.97173443483,1569.40746043628,1569.84318643774,
1570.2780597468,1570.71293305571,1571.14780636448,1571.5826796731,1572.01755298157,
1572.45242628989,1572.88729959806,1573.32217290609,1573.75704621397,1574.19191952171,
1574.62679282931,1575.06166613676,1575.49653944407,1575.93141275123,1576.36713875159,
1576.80286475195,1577.23773805884,1577.67261136559,1578.1074846722,1578.54235797868,
1578.97723128502,1579.41210459124,1579.84697789732,1580.28185120327,1580.71672450909,
1581.15159781478,1581.58647112036,1582.0213444258,1582.45621773113,1582.89109103634,
1583.32681703573,1583.76254303513,1584.1974163401,1584.63228964497,1585.06716294972,
1585.50203625436,1585.9369095589,1586.37178286333,1586.80665616766,1587.24152947189,
1587.67640277602,1588.11127608005,1588.546149384,1588.98102268785,1589.41589599161,
1589.85076929529,1590.28649529394,1590.72222129258,1591.1570945961,1591.59196789953,
1592.0268412029,1592.46171450619,1592.8965878094,1593.33146111256,1593.76633441564,
1594.20120771867,1594.63608102164,1595.07095432455,1595.50582762741,1595.94070093021,
1596.37557423297,1596.81044753569,1597.24617353387,1597.68189953206,1598.11677283469,
1598.55164613729,1598.98651943985,1599.42139274239,1599.8562660449,1600.29113934738,
1600.72601264985,1601.16088595229,1601.59575925472,1602.03063255714,1602.46550585955,
1602.90037916195,1603.33525246435,1603.77012576675,1604.2058517648,1604.64157776285,
1605.07645106526,1605.51132436768,1605.94619767011,1606.38107097255,1606.81594427502,
1607.2508175775,1607.68569088001,1608.12056418254,1608.55543748511,1608.99031078771,
1609.42518409034,1609.86005739302,1610.29493069573,1610.72980399849,1611.16552999674,
1611.60125599499,1612.03612929785,1612.47100260076,1612.90587590373,1613.34074920675,
1613.77562250984,1614.21049581299,1614.64536911621,1615.0802424195,1615.51511572286,
1615.9499890263,1616.38486232981,1616.81973563341,1617.25460893709,1617.68948224085,
1618.12520823963,1618.5609342384,1618.99580754234,1619.43068084638,1619.86555415051,
1620.30042745474,1620.73530075907,1621.1701740635,1621.60504736804,1622.03992067268,
1622.47479397743,1622.90966728229,1623.34454058727,1623.77941389236,1624.21428719757,
1624.6491605029,1625.08488650247,1625.52061250204,1625.95548580761,1626.39035911331,
1626.82523241913,1627.26010572508,1627.69497903116,1628.12985233737,1628.56472564372,
1628.99959895019,1629.43447225681,1629.86934556356,1630.30421887044,1630.73909217747,
1631.17396548464,1631.60883879195,1632.04456479252,1632.48029079309,1632.91516410068,
1633.35003740842,1633.78491071631,1634.21978402433,1634.65465733251,1635.08953064083,
1635.5244039493,1635.95927725792,1636.39415056668,1636.8290238756,1637.26389718466,
1637.69877049387,1638.13364380323,1638.56851711274,1639.00424311442,1639.43996911609,
1639.8748424259,1640.30971573585,1640.74458904595,1641.6143356666,1642.04920897714,
1642.48408228782,1642.91895559865,1643.35382890963,1643.78870222074,1644.223575532,
1645.09332215494,1645.52819546661,1645.96392146936,1646.39964747212,1646.83452078406,
1647.26939409614,1647.70426740834,1648.57401403314,1649.44376065844,1650.31350728422,
1650.74838059729,1651.18325391046,1652.05300053714,1652.92359985428,1653.79419917162,
1654.66394579929,1655.5336924273,1656.40343905563,1657.27318568424,1658.14293231311,
1659.01267894219,1659.88327826096,1660.75387757982,1661.62362420926,1662.49337083877,
1663.3631174683,1664.23286409781,1665.10261072725,1665.97235735658,1666.84295667531,
1667.71355599396,1668.58330262282,1669.45304925143,1670.32279587976,1671.19254250778,
1672.06228913544,1672.93203576273,1673.80263507977,1674.6732343966,1675.54298102284,
1676.41272764862,1677.28247427392,1678.15222089872,1679.021967523,1679.89171414676,
1680.76231346105,1681.19803946366,1681.63291277506,1682.06778608632,1682.50265939743,
1682.93753270841,1683.37240601924,1684.24215264047,1684.67702595086,1685.11189926111,
1685.54677257121,1685.98164588116,1686.41651919097,1686.85139250063,1687.28626581014,
1687.72199181166,1688.15771781319,1688.5925911224,1689.02746443146,1689.46233774038,
1689.89721104914,1690.33208435776,1690.76695766623,1691.20183097455,1691.63670428272,
1692.07157759075,1692.50645089864,1692.94132420637,1693.37619751397,1693.81107082142,
1694.24594412873,1694.68167012916,1695.11739612959,1695.55226943662,1695.9871427435,
1696.42201605025,1696.85688935687,1697.29176266334,1697.72663596969,1698.1615092759,
1698.59638258198,1699.03125588793,1699.46612919375,1699.90100249945,1700.33587580502,
1700.77074911047,1701.20562241579,1701.64134841525,1702.0770744147,1702.51194771979,
1702.94682102476,1703.38169432963,1703.81656763438,1704.25144093902,1704.68631424356,
1705.12118754799,1705.55606085232,1705.99093415655,1706.42580746068,1706.86068076471,
1707.29555406866,1707.73042737251,1708.16530067627,1708.60102667496,1709.03675267365,
1709.47162597724,1709.90649928076,1710.34137258419,1710.77624588756,1711.21111919085,
1711.64599249406,1712.08086579722,1712.5157391003,1712.95061240333,1713.3854857063,
1713.82035900921,1714.25523231207,1714.69010561487,1715.12497891763,1715.56070491584,
1715.99643091404,1716.43130421671,1716.86617751935,1717.30105082195,1717.73592412451,
1718.17079742705,1718.60567072956,1719.04054403204,1719.4754173345,1719.91029063695,
1720.34516393938,1720.7800372418,1721.21491054421,1721.64978384661,1722.08465714901,
1722.52038314706,1722.9561091451,1723.39098244751,1723.82585574992,1724.26072905233,
1724.69560235476,1725.13047565721,1725.56534895967,1726.00022226216,1726.43509556467,
1726.8699688672,1727.30484216977,1727.73971547236,1728.174588775,1728.60946207767,
1729.04433538039,1729.48006137861,1729.91578737684,1730.35066067965,1730.78553398251,
1731.22040728542,1731.65528058838,1732.09015389141,1732.5250271945,1732.95990049765,
1733.39477380087,1733.82964710416,1734.26452040752,1734.69939371096,1735.13426701447,
1735.56914031807,1736.00401362175,1736.43973962048,1736.8754656192,1737.31033892306,
1737.745212227,1738.18008553104,1738.61495883517,1739.0498321394,1739.48470544373,
1739.91957874816,1740.35445205269,1740.78932535734,1741.22419866209,1741.65907196695,
1742.09394527193,1742.52881857702,1742.96369188223,1743.39941788174,1743.83514388125,
1744.2700171867,1744.70489049227,1745.13976379797,1745.57463710379,1746.00951040974,
1746.44438371582,1746.87925702203,1747.31413032837,1747.74900363485,1748.18387694146,
1748.61875024821,1749.0536235551,1749.48849686213,1749.92337016929,1750.3590961698,
1750.7948221703,1751.22969547775,1751.66456878534,1752.09944209308,1752.53431540096,
1752.96918870899,1753.40406201717,1753.83893532549,1754.27380863396,1754.70868194258,
1755.14355525134,1755.57842856026,1756.01330186932,1756.44817517853,1756.88304848789,
1757.31877448949,1757.75450049109,1758.18937380075,1759.05912042051,1759.49399373061,
1759.92886704086,1760.36374035125,1760.79861366179,1761.23348697248,1761.66836028331,
1762.10323359429,1762.5381069054,1763.40785352806,1763.8427268396,1764.27845284228,
1764.71417884496,1765.14905215677,1765.58392546872,1766.0187987808,1766.88854540534,
1767.75829203039,1768.1931653431,1768.62803865593,1769.06291196888,1769.49778528195,
1770.36753190841,1771.2381312254,1772.10873054259,1772.97847717007,1773.84822379791,
1774.71797042609,1775.58771705456,1776.45746368331,1777.32721031228,1778.19780963089,
1779.06840894783,1779.93815555508,1780.80790201176,1781.67764871408),(-0.58309518948453,
1.5208938731769E-10),.UNSPECIFIED.) ;
#822=B_SPLINE_SURFACE_WITH_KNOTS('',3,1,((#43253,#43254),(#43255,#43256),
(#43257,#43258),(#43259,#43260),(#43261,#43262),(#43263,#43264),(#43265,
#43266),(#43267,#43268),(#43269,#43270),(#43271,#43272),(#43273,#43274),
(#43275,#43276),(#43277,#43278),(#43279,#43280),(#43281,#43282),(#43283,
#43284),(#43285,#43286),(#43287,#43288),(#43289,#43290),(#43291,#43292),
(#43293,#43294),(#43295,#43296),(#43297,#43298),(#43299,#43300),(#43301,
#43302),(#43303,#43304),(#43305,#43306),(#43307,#43308),(#43309,#43310),
(#43311,#43312),(#43313,#43314),(#43315,#43316),(#43317,#43318),(#43319,
#43320),(#43321,#43322),(#43323,#43324),(#43325,#43326),(#43327,#43328),
(#43329,#43330),(#43331,#43332),(#43333,#43334),(#43335,#43336),(#43337,
#43338),(#43339,#43340),(#43341,#43342),(#43343,#43344),(#43345,#43346),
(#43347,#43348),(#43349,#43350),(#43351,#43352),(#43353,#43354),(#43355,
#43356),(#43357,#43358),(#43359,#43360),(#43361,#43362),(#43363,#43364),
(#43365,#43366),(#43367,#43368),(#43369,#43370),(#43371,#43372),(#43373,
#43374),(#43375,#43376),(#43377,#43378),(#43379,#43380),(#43381,#43382),
(#43383,#43384),(#43385,#43386),(#43387,#43388),(#43389,#43390),(#43391,
#43392),(#43393,#43394),(#43395,#43396),(#43397,#43398),(#43399,#43400),
(#43401,#43402),(#43403,#43404),(#43405,#43406),(#43407,#43408),(#43409,
#43410),(#43411,#43412),(#43413,#43414),(#43415,#43416),(#43417,#43418),
(#43419,#43420),(#43421,#43422),(#43423,#43424),(#43425,#43426),(#43427,
#43428),(#43429,#43430),(#43431,#43432),(#43433,#43434),(#43435,#43436),
(#43437,#43438),(#43439,#43440),(#43441,#43442),(#43443,#43444),(#43445,
#43446),(#43447,#43448),(#43449,#43450),(#43451,#43452),(#43453,#43454),
(#43455,#43456),(#43457,#43458),(#43459,#43460),(#43461,#43462),(#43463,
#43464),(#43465,#43466),(#43467,#43468),(#43469,#43470),(#43471,#43472),
(#43473,#43474),(#43475,#43476),(#43477,#43478),(#43479,#43480),(#43481,
#43482),(#43483,#43484),(#43485,#43486),(#43487,#43488),(#43489,#43490),
(#43491,#43492),(#43493,#43494),(#43495,#43496),(#43497,#43498),(#43499,
#43500),(#43501,#43502),(#43503,#43504),(#43505,#43506),(#43507,#43508),
(#43509,#43510),(#43511,#43512),(#43513,#43514),(#43515,#43516),(#43517,
#43518),(#43519,#43520),(#43521,#43522),(#43523,#43524),(#43525,#43526),
(#43527,#43528),(#43529,#43530),(#43531,#43532),(#43533,#43534),(#43535,
#43536),(#43537,#43538),(#43539,#43540),(#43541,#43542),(#43543,#43544),
(#43545,#43546),(#43547,#43548),(#43549,#43550),(#43551,#43552),(#43553,
#43554),(#43555,#43556),(#43557,#43558),(#43559,#43560),(#43561,#43562),
(#43563,#43564),(#43565,#43566),(#43567,#43568),(#43569,#43570),(#43571,
#43572),(#43573,#43574),(#43575,#43576),(#43577,#43578),(#43579,#43580),
(#43581,#43582),(#43583,#43584),(#43585,#43586),(#43587,#43588),(#43589,
#43590),(#43591,#43592),(#43593,#43594),(#43595,#43596),(#43597,#43598),
(#43599,#43600),(#43601,#43602),(#43603,#43604),(#43605,#43606),(#43607,
#43608),(#43609,#43610),(#43611,#43612),(#43613,#43614),(#43615,#43616),
(#43617,#43618),(#43619,#43620),(#43621,#43622),(#43623,#43624),(#43625,
#43626),(#43627,#43628),(#43629,#43630),(#43631,#43632),(#43633,#43634),
(#43635,#43636),(#43637,#43638),(#43639,#43640),(#43641,#43642),(#43643,
#43644),(#43645,#43646),(#43647,#43648),(#43649,#43650),(#43651,#43652),
(#43653,#43654),(#43655,#43656),(#43657,#43658),(#43659,#43660),(#43661,
#43662),(#43663,#43664),(#43665,#43666),(#43667,#43668),(#43669,#43670),
(#43671,#43672),(#43673,#43674),(#43675,#43676),(#43677,#43678),(#43679,
#43680),(#43681,#43682),(#43683,#43684),(#43685,#43686),(#43687,#43688),
(#43689,#43690),(#43691,#43692),(#43693,#43694),(#43695,#43696),(#43697,
#43698),(#43699,#43700),(#43701,#43702),(#43703,#43704),(#43705,#43706),
(#43707,#43708),(#43709,#43710),(#43711,#43712),(#43713,#43714),(#43715,
#43716),(#43717,#43718),(#43719,#43720),(#43721,#43722),(#43723,#43724),
(#43725,#43726),(#43727,#43728),(#43729,#43730),(#43731,#43732),(#43733,
#43734),(#43735,#43736),(#43737,#43738),(#43739,#43740),(#43741,#43742),
(#43743,#43744),(#43745,#43746),(#43747,#43748),(#43749,#43750),(#43751,
#43752),(#43753,#43754),(#43755,#43756),(#43757,#43758),(#43759,#43760),
(#43761,#43762),(#43763,#43764),(#43765,#43766),(#43767,#43768),(#43769,
#43770),(#43771,#43772),(#43773,#43774),(#43775,#43776),(#43777,#43778),
(#43779,#43780),(#43781,#43782),(#43783,#43784),(#43785,#43786),(#43787,
#43788),(#43789,#43790),(#43791,#43792),(#43793,#43794),(#43795,#43796),
(#43797,#43798),(#43799,#43800),(#43801,#43802),(#43803,#43804),(#43805,
#43806),(#43807,#43808),(#43809,#43810),(#43811,#43812),(#43813,#43814),
(#43815,#43816),(#43817,#43818),(#43819,#43820),(#43821,#43822),(#43823,
#43824),(#43825,#43826),(#43827,#43828),(#43829,#43830),(#43831,#43832),
(#43833,#43834),(#43835,#43836),(#43837,#43838),(#43839,#43840),(#43841,
#43842),(#43843,#43844),(#43845,#43846),(#43847,#43848),(#43849,#43850),
(#43851,#43852),(#43853,#43854),(#43855,#43856),(#43857,#43858),(#43859,
#43860),(#43861,#43862),(#43863,#43864),(#43865,#43866),(#43867,#43868),
(#43869,#43870),(#43871,#43872),(#43873,#43874),(#43875,#43876),(#43877,
#43878),(#43879,#43880),(#43881,#43882),(#43883,#43884),(#43885,#43886),
(#43887,#43888),(#43889,#43890),(#43891,#43892),(#43893,#43894),(#43895,
#43896),(#43897,#43898),(#43899,#43900),(#43901,#43902),(#43903,#43904),
(#43905,#43906),(#43907,#43908),(#43909,#43910),(#43911,#43912),(#43913,
#43914),(#43915,#43916),(#43917,#43918),(#43919,#43920),(#43921,#43922),
(#43923,#43924),(#43925,#43926),(#43927,#43928),(#43929,#43930),(#43931,
#43932),(#43933,#43934),(#43935,#43936),(#43937,#43938),(#43939,#43940),
(#43941,#43942),(#43943,#43944),(#43945,#43946),(#43947,#43948),(#43949,
#43950),(#43951,#43952),(#43953,#43954),(#43955,#43956),(#43957,#43958),
(#43959,#43960),(#43961,#43962),(#43963,#43964),(#43965,#43966),(#43967,
#43968),(#43969,#43970),(#43971,#43972),(#43973,#43974),(#43975,#43976),
(#43977,#43978),(#43979,#43980),(#43981,#43982),(#43983,#43984),(#43985,
#43986),(#43987,#43988),(#43989,#43990),(#43991,#43992),(#43993,#43994),
(#43995,#43996),(#43997,#43998),(#43999,#44000),(#44001,#44002),(#44003,
#44004),(#44005,#44006),(#44007,#44008),(#44009,#44010),(#44011,#44012),
(#44013,#44014),(#44015,#44016),(#44017,#44018),(#44019,#44020),(#44021,
#44022),(#44023,#44024),(#44025,#44026),(#44027,#44028),(#44029,#44030),
(#44031,#44032),(#44033,#44034),(#44035,#44036),(#44037,#44038),(#44039,
#44040),(#44041,#44042),(#44043,#44044),(#44045,#44046),(#44047,#44048),
(#44049,#44050),(#44051,#44052),(#44053,#44054),(#44055,#44056),(#44057,
#44058),(#44059,#44060),(#44061,#44062),(#44063,#44064),(#44065,#44066),
(#44067,#44068),(#44069,#44070),(#44071,#44072),(#44073,#44074),(#44075,
#44076),(#44077,#44078),(#44079,#44080),(#44081,#44082),(#44083,#44084),
(#44085,#44086),(#44087,#44088),(#44089,#44090),(#44091,#44092),(#44093,
#44094),(#44095,#44096),(#44097,#44098),(#44099,#44100),(#44101,#44102),
(#44103,#44104),(#44105,#44106),(#44107,#44108),(#44109,#44110),(#44111,
#44112),(#44113,#44114),(#44115,#44116),(#44117,#44118),(#44119,#44120),
(#44121,#44122),(#44123,#44124),(#44125,#44126),(#44127,#44128),(#44129,
#44130),(#44131,#44132),(#44133,#44134),(#44135,#44136),(#44137,#44138),
(#44139,#44140),(#44141,#44142),(#44143,#44144),(#44145,#44146),(#44147,
#44148),(#44149,#44150),(#44151,#44152),(#44153,#44154),(#44155,#44156),
(#44157,#44158),(#44159,#44160),(#44161,#44162),(#44163,#44164),(#44165,
#44166),(#44167,#44168),(#44169,#44170),(#44171,#44172),(#44173,#44174),
(#44175,#44176),(#44177,#44178),(#44179,#44180),(#44181,#44182),(#44183,
#44184),(#44185,#44186),(#44187,#44188),(#44189,#44190),(#44191,#44192),
(#44193,#44194),(#44195,#44196),(#44197,#44198),(#44199,#44200),(#44201,
#44202),(#44203,#44204),(#44205,#44206),(#44207,#44208),(#44209,#44210),
(#44211,#44212),(#44213,#44214),(#44215,#44216),(#44217,#44218),(#44219,
#44220),(#44221,#44222),(#44223,#44224),(#44225,#44226),(#44227,#44228),
(#44229,#44230),(#44231,#44232),(#44233,#44234),(#44235,#44236),(#44237,
#44238),(#44239,#44240),(#44241,#44242),(#44243,#44244),(#44245,#44246),
(#44247,#44248),(#44249,#44250),(#44251,#44252),(#44253,#44254),(#44255,
#44256),(#44257,#44258),(#44259,#44260),(#44261,#44262),(#44263,#44264),
(#44265,#44266),(#44267,#44268),(#44269,#44270),(#44271,#44272),(#44273,
#44274),(#44275,#44276),(#44277,#44278),(#44279,#44280),(#44281,#44282),
(#44283,#44284),(#44285,#44286),(#44287,#44288),(#44289,#44290),(#44291,
#44292),(#44293,#44294),(#44295,#44296),(#44297,#44298),(#44299,#44300),
(#44301,#44302),(#44303,#44304),(#44305,#44306),(#44307,#44308),(#44309,
#44310),(#44311,#44312),(#44313,#44314),(#44315,#44316),(#44317,#44318),
(#44319,#44320),(#44321,#44322),(#44323,#44324),(#44325,#44326),(#44327,
#44328),(#44329,#44330),(#44331,#44332),(#44333,#44334),(#44335,#44336),
(#44337,#44338),(#44339,#44340),(#44341,#44342),(#44343,#44344),(#44345,
#44346),(#44347,#44348),(#44349,#44350),(#44351,#44352),(#44353,#44354),
(#44355,#44356),(#44357,#44358),(#44359,#44360),(#44361,#44362),(#44363,
#44364),(#44365,#44366),(#44367,#44368),(#44369,#44370),(#44371,#44372),
(#44373,#44374),(#44375,#44376),(#44377,#44378),(#44379,#44380),(#44381,
#44382),(#44383,#44384),(#44385,#44386),(#44387,#44388),(#44389,#44390),
(#44391,#44392),(#44393,#44394),(#44395,#44396),(#44397,#44398),(#44399,
#44400),(#44401,#44402),(#44403,#44404),(#44405,#44406),(#44407,#44408),
(#44409,#44410),(#44411,#44412),(#44413,#44414),(#44415,#44416),(#44417,
#44418),(#44419,#44420),(#44421,#44422),(#44423,#44424),(#44425,#44426),
(#44427,#44428),(#44429,#44430),(#44431,#44432),(#44433,#44434),(#44435,
#44436),(#44437,#44438),(#44439,#44440),(#44441,#44442),(#44443,#44444),
(#44445,#44446),(#44447,#44448),(#44449,#44450),(#44451,#44452),(#44453,
#44454),(#44455,#44456),(#44457,#44458),(#44459,#44460),(#44461,#44462),
(#44463,#44464),(#44465,#44466),(#44467,#44468),(#44469,#44470),(#44471,
#44472),(#44473,#44474),(#44475,#44476),(#44477,#44478),(#44479,#44480),
(#44481,#44482),(#44483,#44484),(#44485,#44486),(#44487,#44488),(#44489,
#44490),(#44491,#44492),(#44493,#44494),(#44495,#44496),(#44497,#44498),
(#44499,#44500),(#44501,#44502),(#44503,#44504),(#44505,#44506),(#44507,
#44508),(#44509,#44510),(#44511,#44512),(#44513,#44514),(#44515,#44516),
(#44517,#44518),(#44519,#44520),(#44521,#44522),(#44523,#44524),(#44525,
#44526),(#44527,#44528),(#44529,#44530),(#44531,#44532),(#44533,#44534),
(#44535,#44536),(#44537,#44538),(#44539,#44540),(#44541,#44542),(#44543,
#44544),(#44545,#44546),(#44547,#44548),(#44549,#44550),(#44551,#44552),
(#44553,#44554),(#44555,#44556),(#44557,#44558),(#44559,#44560),(#44561,
#44562),(#44563,#44564),(#44565,#44566),(#44567,#44568),(#44569,#44570),
(#44571,#44572),(#44573,#44574),(#44575,#44576),(#44577,#44578),(#44579,
#44580),(#44581,#44582),(#44583,#44584),(#44585,#44586),(#44587,#44588),
(#44589,#44590),(#44591,#44592),(#44593,#44594),(#44595,#44596),(#44597,
#44598),(#44599,#44600),(#44601,#44602),(#44603,#44604),(#44605,#44606),
(#44607,#44608),(#44609,#44610),(#44611,#44612),(#44613,#44614),(#44615,
#44616),(#44617,#44618),(#44619,#44620),(#44621,#44622),(#44623,#44624),
(#44625,#44626),(#44627,#44628),(#44629,#44630),(#44631,#44632),(#44633,
#44634),(#44635,#44636),(#44637,#44638),(#44639,#44640),(#44641,#44642),
(#44643,#44644),(#44645,#44646),(#44647,#44648),(#44649,#44650),(#44651,
#44652),(#44653,#44654),(#44655,#44656),(#44657,#44658),(#44659,#44660),
(#44661,#44662),(#44663,#44664),(#44665,#44666),(#44667,#44668),(#44669,
#44670),(#44671,#44672),(#44673,#44674),(#44675,#44676),(#44677,#44678),
(#44679,#44680),(#44681,#44682),(#44683,#44684),(#44685,#44686),(#44687,
#44688),(#44689,#44690),(#44691,#44692),(#44693,#44694),(#44695,#44696),
(#44697,#44698),(#44699,#44700),(#44701,#44702),(#44703,#44704),(#44705,
#44706),(#44707,#44708),(#44709,#44710),(#44711,#44712),(#44713,#44714),
(#44715,#44716),(#44717,#44718),(#44719,#44720),(#44721,#44722),(#44723,
#44724),(#44725,#44726),(#44727,#44728),(#44729,#44730),(#44731,#44732),
(#44733,#44734),(#44735,#44736),(#44737,#44738),(#44739,#44740),(#44741,
#44742),(#44743,#44744),(#44745,#44746),(#44747,#44748),(#44749,#44750),
(#44751,#44752),(#44753,#44754),(#44755,#44756),(#44757,#44758),(#44759,
#44760),(#44761,#44762),(#44763,#44764),(#44765,#44766),(#44767,#44768),
(#44769,#44770),(#44771,#44772),(#44773,#44774),(#44775,#44776),(#44777,
#44778),(#44779,#44780),(#44781,#44782),(#44783,#44784),(#44785,#44786),
(#44787,#44788),(#44789,#44790),(#44791,#44792),(#44793,#44794),(#44795,
#44796),(#44797,#44798),(#44799,#44800),(#44801,#44802),(#44803,#44804),
(#44805,#44806),(#44807,#44808),(#44809,#44810),(#44811,#44812),(#44813,
#44814),(#44815,#44816),(#44817,#44818),(#44819,#44820),(#44821,#44822),
(#44823,#44824),(#44825,#44826),(#44827,#44828),(#44829,#44830),(#44831,
#44832),(#44833,#44834),(#44835,#44836),(#44837,#44838),(#44839,#44840),
(#44841,#44842),(#44843,#44844),(#44845,#44846),(#44847,#44848),(#44849,
#44850),(#44851,#44852),(#44853,#44854),(#44855,#44856),(#44857,#44858),
(#44859,#44860),(#44861,#44862),(#44863,#44864),(#44865,#44866),(#44867,
#44868),(#44869,#44870),(#44871,#44872),(#44873,#44874),(#44875,#44876),
(#44877,#44878),(#44879,#44880),(#44881,#44882),(#44883,#44884),(#44885,
#44886),(#44887,#44888),(#44889,#44890),(#44891,#44892),(#44893,#44894),
(#44895,#44896),(#44897,#44898),(#44899,#44900),(#44901,#44902),(#44903,
#44904),(#44905,#44906),(#44907,#44908),(#44909,#44910),(#44911,#44912),
(#44913,#44914),(#44915,#44916),(#44917,#44918),(#44919,#44920),(#44921,
#44922),(#44923,#44924),(#44925,#44926),(#44927,#44928),(#44929,#44930),
(#44931,#44932),(#44933,#44934),(#44935,#44936),(#44937,#44938),(#44939,
#44940),(#44941,#44942),(#44943,#44944),(#44945,#44946),(#44947,#44948),
(#44949,#44950),(#44951,#44952),(#44953,#44954),(#44955,#44956),(#44957,
#44958),(#44959,#44960),(#44961,#44962),(#44963,#44964),(#44965,#44966),
(#44967,#44968),(#44969,#44970),(#44971,#44972),(#44973,#44974),(#44975,
#44976),(#44977,#44978),(#44979,#44980),(#44981,#44982),(#44983,#44984),
(#44985,#44986),(#44987,#44988),(#44989,#44990),(#44991,#44992),(#44993,
#44994),(#44995,#44996),(#44997,#44998),(#44999,#45000),(#45001,#45002),
(#45003,#45004),(#45005,#45006),(#45007,#45008),(#45009,#45010),(#45011,
#45012),(#45013,#45014),(#45015,#45016),(#45017,#45018),(#45019,#45020),
(#45021,#45022),(#45023,#45024),(#45025,#45026),(#45027,#45028),(#45029,
#45030),(#45031,#45032),(#45033,#45034),(#45035,#45036),(#45037,#45038),
(#45039,#45040),(#45041,#45042),(#45043,#45044),(#45045,#45046),(#45047,
#45048),(#45049,#45050),(#45051,#45052),(#45053,#45054),(#45055,#45056),
(#45057,#45058),(#45059,#45060),(#45061,#45062),(#45063,#45064),(#45065,
#45066),(#45067,#45068),(#45069,#45070),(#45071,#45072),(#45073,#45074),
(#45075,#45076),(#45077,#45078),(#45079,#45080),(#45081,#45082),(#45083,
#45084),(#45085,#45086),(#45087,#45088),(#45089,#45090),(#45091,#45092),
(#45093,#45094),(#45095,#45096),(#45097,#45098),(#45099,#45100),(#45101,
#45102),(#45103,#45104),(#45105,#45106),(#45107,#45108),(#45109,#45110),
(#45111,#45112),(#45113,#45114),(#45115,#45116),(#45117,#45118),(#45119,
#45120),(#45121,#45122),(#45123,#45124),(#45125,#45126),(#45127,#45128),
(#45129,#45130),(#45131,#45132),(#45133,#45134),(#45135,#45136),(#45137,
#45138),(#45139,#45140),(#45141,#45142),(#45143,#45144),(#45145,#45146),
(#45147,#45148),(#45149,#45150),(#45151,#45152),(#45153,#45154),(#45155,
#45156),(#45157,#45158),(#45159,#45160),(#45161,#45162),(#45163,#45164),
(#45165,#45166),(#45167,#45168),(#45169,#45170),(#45171,#45172),(#45173,
#45174),(#45175,#45176),(#45177,#45178),(#45179,#45180),(#45181,#45182),
(#45183,#45184),(#45185,#45186),(#45187,#45188),(#45189,#45190),(#45191,
#45192),(#45193,#45194),(#45195,#45196),(#45197,#45198),(#45199,#45200),
(#45201,#45202),(#45203,#45204),(#45205,#45206),(#45207,#45208),(#45209,
#45210),(#45211,#45212),(#45213,#45214),(#45215,#45216),(#45217,#45218),
(#45219,#45220),(#45221,#45222),(#45223,#45224),(#45225,#45226),(#45227,
#45228),(#45229,#45230),(#45231,#45232),(#45233,#45234),(#45235,#45236),
(#45237,#45238),(#45239,#45240),(#45241,#45242),(#45243,#45244),(#45245,
#45246),(#45247,#45248),(#45249,#45250),(#45251,#45252),(#45253,#45254),
(#45255,#45256),(#45257,#45258),(#45259,#45260),(#45261,#45262),(#45263,
#45264),(#45265,#45266),(#45267,#45268),(#45269,#45270),(#45271,#45272),
(#45273,#45274),(#45275,#45276),(#45277,#45278),(#45279,#45280),(#45281,
#45282),(#45283,#45284),(#45285,#45286),(#45287,#45288),(#45289,#45290),
(#45291,#45292),(#45293,#45294),(#45295,#45296),(#45297,#45298),(#45299,
#45300),(#45301,#45302),(#45303,#45304),(#45305,#45306),(#45307,#45308),
(#45309,#45310),(#45311,#45312),(#45313,#45314),(#45315,#45316),(#45317,
#45318),(#45319,#45320),(#45321,#45322),(#45323,#45324),(#45325,#45326),
(#45327,#45328),(#45329,#45330),(#45331,#45332),(#45333,#45334),(#45335,
#45336),(#45337,#45338),(#45339,#45340),(#45341,#45342),(#45343,#45344),
(#45345,#45346),(#45347,#45348),(#45349,#45350),(#45351,#45352),(#45353,
#45354),(#45355,#45356),(#45357,#45358),(#45359,#45360),(#45361,#45362),
(#45363,#45364),(#45365,#45366),(#45367,#45368),(#45369,#45370),(#45371,
#45372),(#45373,#45374),(#45375,#45376),(#45377,#45378),(#45379,#45380),
(#45381,#45382),(#45383,#45384),(#45385,#45386),(#45387,#45388),(#45389,
#45390),(#45391,#45392),(#45393,#45394),(#45395,#45396),(#45397,#45398),
(#45399,#45400),(#45401,#45402),(#45403,#45404),(#45405,#45406),(#45407,
#45408),(#45409,#45410),(#45411,#45412),(#45413,#45414),(#45415,#45416),
(#45417,#45418),(#45419,#45420),(#45421,#45422),(#45423,#45424),(#45425,
#45426),(#45427,#45428),(#45429,#45430),(#45431,#45432),(#45433,#45434),
(#45435,#45436),(#45437,#45438),(#45439,#45440),(#45441,#45442),(#45443,
#45444),(#45445,#45446),(#45447,#45448),(#45449,#45450),(#45451,#45452),
(#45453,#45454),(#45455,#45456),(#45457,#45458),(#45459,#45460),(#45461,
#45462),(#45463,#45464),(#45465,#45466),(#45467,#45468),(#45469,#45470),
(#45471,#45472),(#45473,#45474),(#45475,#45476),(#45477,#45478),(#45479,
#45480),(#45481,#45482),(#45483,#45484),(#45485,#45486),(#45487,#45488),
(#45489,#45490),(#45491,#45492),(#45493,#45494),(#45495,#45496),(#45497,
#45498),(#45499,#45500),(#45501,#45502),(#45503,#45504),(#45505,#45506),
(#45507,#45508),(#45509,#45510),(#45511,#45512),(#45513,#45514),(#45515,
#45516),(#45517,#45518),(#45519,#45520),(#45521,#45522),(#45523,#45524),
(#45525,#45526),(#45527,#45528),(#45529,#45530),(#45531,#45532),(#45533,
#45534),(#45535,#45536),(#45537,#45538),(#45539,#45540),(#45541,#45542),
(#45543,#45544),(#45545,#45546),(#45547,#45548),(#45549,#45550),(#45551,
#45552),(#45553,#45554),(#45555,#45556),(#45557,#45558),(#45559,#45560),
(#45561,#45562),(#45563,#45564),(#45565,#45566),(#45567,#45568),(#45569,
#45570),(#45571,#45572),(#45573,#45574),(#45575,#45576),(#45577,#45578),
(#45579,#45580),(#45581,#45582),(#45583,#45584),(#45585,#45586),(#45587,
#45588),(#45589,#45590),(#45591,#45592),(#45593,#45594),(#45595,#45596),
(#45597,#45598),(#45599,#45600),(#45601,#45602),(#45603,#45604),(#45605,
#45606),(#45607,#45608),(#45609,#45610),(#45611,#45612),(#45613,#45614),
(#45615,#45616),(#45617,#45618),(#45619,#45620),(#45621,#45622),(#45623,
#45624),(#45625,#45626),(#45627,#45628),(#45629,#45630),(#45631,#45632),
(#45633,#45634),(#45635,#45636),(#45637,#45638),(#45639,#45640),(#45641,
#45642),(#45643,#45644),(#45645,#45646),(#45647,#45648),(#45649,#45650),
(#45651,#45652),(#45653,#45654),(#45655,#45656),(#45657,#45658),(#45659,
#45660),(#45661,#45662),(#45663,#45664),(#45665,#45666),(#45667,#45668),
(#45669,#45670),(#45671,#45672),(#45673,#45674),(#45675,#45676),(#45677,
#45678),(#45679,#45680),(#45681,#45682),(#45683,#45684),(#45685,#45686),
(#45687,#45688),(#45689,#45690),(#45691,#45692),(#45693,#45694),(#45695,
#45696),(#45697,#45698),(#45699,#45700),(#45701,#45702),(#45703,#45704),
(#45705,#45706),(#45707,#45708),(#45709,#45710),(#45711,#45712),(#45713,
#45714),(#45715,#45716),(#45717,#45718),(#45719,#45720),(#45721,#45722),
(#45723,#45724),(#45725,#45726),(#45727,#45728),(#45729,#45730),(#45731,
#45732),(#45733,#45734),(#45735,#45736),(#45737,#45738),(#45739,#45740),
(#45741,#45742),(#45743,#45744),(#45745,#45746),(#45747,#45748),(#45749,
#45750),(#45751,#45752),(#45753,#45754),(#45755,#45756),(#45757,#45758),
(#45759,#45760),(#45761,#45762),(#45763,#45764),(#45765,#45766),(#45767,
#45768),(#45769,#45770),(#45771,#45772),(#45773,#45774),(#45775,#45776),
(#45777,#45778),(#45779,#45780),(#45781,#45782),(#45783,#45784),(#45785,
#45786),(#45787,#45788),(#45789,#45790),(#45791,#45792),(#45793,#45794),
(#45795,#45796),(#45797,#45798),(#45799,#45800),(#45801,#45802),(#45803,
#45804),(#45805,#45806),(#45807,#45808),(#45809,#45810),(#45811,#45812),
(#45813,#45814),(#45815,#45816),(#45817,#45818),(#45819,#45820),(#45821,
#45822),(#45823,#45824),(#45825,#45826),(#45827,#45828),(#45829,#45830),
(#45831,#45832),(#45833,#45834),(#45835,#45836),(#45837,#45838),(#45839,
#45840),(#45841,#45842),(#45843,#45844),(#45845,#45846),(#45847,#45848),
(#45849,#45850),(#45851,#45852),(#45853,#45854),(#45855,#45856),(#45857,
#45858),(#45859,#45860),(#45861,#45862),(#45863,#45864),(#45865,#45866),
(#45867,#45868),(#45869,#45870),(#45871,#45872),(#45873,#45874),(#45875,
#45876),(#45877,#45878),(#45879,#45880),(#45881,#45882),(#45883,#45884),
(#45885,#45886),(#45887,#45888),(#45889,#45890),(#45891,#45892),(#45893,
#45894),(#45895,#45896),(#45897,#45898),(#45899,#45900),(#45901,#45902),
(#45903,#45904),(#45905,#45906),(#45907,#45908),(#45909,#45910),(#45911,
#45912),(#45913,#45914),(#45915,#45916),(#45917,#45918),(#45919,#45920),
(#45921,#45922),(#45923,#45924),(#45925,#45926),(#45927,#45928),(#45929,
#45930),(#45931,#45932),(#45933,#45934),(#45935,#45936),(#45937,#45938),
(#45939,#45940),(#45941,#45942),(#45943,#45944),(#45945,#45946),(#45947,
#45948),(#45949,#45950),(#45951,#45952),(#45953,#45954),(#45955,#45956),
(#45957,#45958),(#45959,#45960),(#45961,#45962),(#45963,#45964),(#45965,
#45966),(#45967,#45968),(#45969,#45970),(#45971,#45972),(#45973,#45974),
(#45975,#45976),(#45977,#45978),(#45979,#45980),(#45981,#45982),(#45983,
#45984),(#45985,#45986),(#45987,#45988),(#45989,#45990),(#45991,#45992),
(#45993,#45994),(#45995,#45996),(#45997,#45998),(#45999,#46000),(#46001,
#46002),(#46003,#46004),(#46005,#46006),(#46007,#46008),(#46009,#46010),
(#46011,#46012),(#46013,#46014),(#46015,#46016),(#46017,#46018),(#46019,
#46020),(#46021,#46022),(#46023,#46024),(#46025,#46026),(#46027,#46028),
(#46029,#46030),(#46031,#46032),(#46033,#46034),(#46035,#46036),(#46037,
#46038),(#46039,#46040),(#46041,#46042),(#46043,#46044),(#46045,#46046),
(#46047,#46048),(#46049,#46050),(#46051,#46052),(#46053,#46054),(#46055,
#46056),(#46057,#46058),(#46059,#46060),(#46061,#46062),(#46063,#46064),
(#46065,#46066),(#46067,#46068),(#46069,#46070),(#46071,#46072),(#46073,
#46074),(#46075,#46076),(#46077,#46078),(#46079,#46080),(#46081,#46082),
(#46083,#46084),(#46085,#46086),(#46087,#46088),(#46089,#46090),(#46091,
#46092),(#46093,#46094),(#46095,#46096),(#46097,#46098),(#46099,#46100),
(#46101,#46102),(#46103,#46104),(#46105,#46106),(#46107,#46108),(#46109,
#46110),(#46111,#46112),(#46113,#46114),(#46115,#46116),(#46117,#46118),
(#46119,#46120),(#46121,#46122),(#46123,#46124),(#46125,#46126),(#46127,
#46128),(#46129,#46130),(#46131,#46132),(#46133,#46134),(#46135,#46136),
(#46137,#46138),(#46139,#46140),(#46141,#46142),(#46143,#46144),(#46145,
#46146),(#46147,#46148),(#46149,#46150),(#46151,#46152),(#46153,#46154),
(#46155,#46156),(#46157,#46158),(#46159,#46160),(#46161,#46162),(#46163,
#46164),(#46165,#46166),(#46167,#46168),(#46169,#46170),(#46171,#46172),
(#46173,#46174),(#46175,#46176),(#46177,#46178),(#46179,#46180),(#46181,
#46182),(#46183,#46184),(#46185,#46186),(#46187,#46188),(#46189,#46190),
(#46191,#46192),(#46193,#46194),(#46195,#46196),(#46197,#46198),(#46199,
#46200),(#46201,#46202),(#46203,#46204),(#46205,#46206),(#46207,#46208),
(#46209,#46210),(#46211,#46212),(#46213,#46214),(#46215,#46216),(#46217,
#46218),(#46219,#46220),(#46221,#46222),(#46223,#46224),(#46225,#46226),
(#46227,#46228),(#46229,#46230),(#46231,#46232),(#46233,#46234),(#46235,
#46236),(#46237,#46238),(#46239,#46240),(#46241,#46242),(#46243,#46244),
(#46245,#46246),(#46247,#46248),(#46249,#46250),(#46251,#46252),(#46253,
#46254),(#46255,#46256),(#46257,#46258),(#46259,#46260),(#46261,#46262),
(#46263,#46264),(#46265,#46266),(#46267,#46268),(#46269,#46270),(#46271,
#46272),(#46273,#46274),(#46275,#46276),(#46277,#46278),(#46279,#46280),
(#46281,#46282),(#46283,#46284),(#46285,#46286),(#46287,#46288),(#46289,
#46290),(#46291,#46292),(#46293,#46294),(#46295,#46296),(#46297,#46298),
(#46299,#46300),(#46301,#46302),(#46303,#46304),(#46305,#46306),(#46307,
#46308),(#46309,#46310),(#46311,#46312),(#46313,#46314),(#46315,#46316),
(#46317,#46318),(#46319,#46320),(#46321,#46322),(#46323,#46324),(#46325,
#46326),(#46327,#46328),(#46329,#46330),(#46331,#46332),(#46333,#46334),
(#46335,#46336),(#46337,#46338),(#46339,#46340),(#46341,#46342),(#46343,
#46344),(#46345,#46346),(#46347,#46348),(#46349,#46350),(#46351,#46352),
(#46353,#46354),(#46355,#46356),(#46357,#46358),(#46359,#46360),(#46361,
#46362),(#46363,#46364),(#46365,#46366),(#46367,#46368),(#46369,#46370),
(#46371,#46372),(#46373,#46374),(#46375,#46376),(#46377,#46378),(#46379,
#46380),(#46381,#46382),(#46383,#46384),(#46385,#46386),(#46387,#46388),
(#46389,#46390),(#46391,#46392),(#46393,#46394),(#46395,#46396),(#46397,
#46398),(#46399,#46400),(#46401,#46402),(#46403,#46404),(#46405,#46406),
(#46407,#46408),(#46409,#46410),(#46411,#46412),(#46413,#46414),(#46415,
#46416),(#46417,#46418),(#46419,#46420),(#46421,#46422),(#46423,#46424),
(#46425,#46426),(#46427,#46428),(#46429,#46430),(#46431,#46432),(#46433,
#46434),(#46435,#46436),(#46437,#46438),(#46439,#46440),(#46441,#46442),
(#46443,#46444),(#46445,#46446),(#46447,#46448),(#46449,#46450),(#46451,
#46452),(#46453,#46454),(#46455,#46456),(#46457,#46458),(#46459,#46460),
(#46461,#46462),(#46463,#46464),(#46465,#46466),(#46467,#46468),(#46469,
#46470),(#46471,#46472),(#46473,#46474),(#46475,#46476),(#46477,#46478),
(#46479,#46480),(#46481,#46482),(#46483,#46484),(#46485,#46486),(#46487,
#46488),(#46489,#46490),(#46491,#46492),(#46493,#46494),(#46495,#46496),
(#46497,#46498),(#46499,#46500),(#46501,#46502),(#46503,#46504),(#46505,
#46506),(#46507,#46508),(#46509,#46510),(#46511,#46512),(#46513,#46514),
(#46515,#46516),(#46517,#46518),(#46519,#46520),(#46521,#46522),(#46523,
#46524),(#46525,#46526),(#46527,#46528),(#46529,#46530),(#46531,#46532),
(#46533,#46534),(#46535,#46536),(#46537,#46538),(#46539,#46540),(#46541,
#46542),(#46543,#46544),(#46545,#46546),(#46547,#46548),(#46549,#46550),
(#46551,#46552),(#46553,#46554),(#46555,#46556),(#46557,#46558),(#46559,
#46560),(#46561,#46562),(#46563,#46564),(#46565,#46566),(#46567,#46568),
(#46569,#46570),(#46571,#46572),(#46573,#46574),(#46575,#46576),(#46577,
#46578),(#46579,#46580),(#46581,#46582),(#46583,#46584),(#46585,#46586),
(#46587,#46588),(#46589,#46590),(#46591,#46592),(#46593,#46594),(#46595,
#46596),(#46597,#46598),(#46599,#46600),(#46601,#46602),(#46603,#46604),
(#46605,#46606),(#46607,#46608),(#46609,#46610),(#46611,#46612),(#46613,
#46614),(#46615,#46616),(#46617,#46618),(#46619,#46620),(#46621,#46622),
(#46623,#46624),(#46625,#46626),(#46627,#46628),(#46629,#46630),(#46631,
#46632),(#46633,#46634),(#46635,#46636),(#46637,#46638),(#46639,#46640),
(#46641,#46642),(#46643,#46644),(#46645,#46646),(#46647,#46648),(#46649,
#46650),(#46651,#46652),(#46653,#46654),(#46655,#46656),(#46657,#46658),
(#46659,#46660),(#46661,#46662),(#46663,#46664),(#46665,#46666),(#46667,
#46668),(#46669,#46670),(#46671,#46672),(#46673,#46674),(#46675,#46676),
(#46677,#46678),(#46679,#46680),(#46681,#46682),(#46683,#46684),(#46685,
#46686),(#46687,#46688),(#46689,#46690),(#46691,#46692),(#46693,#46694),
(#46695,#46696),(#46697,#46698),(#46699,#46700),(#46701,#46702),(#46703,
#46704),(#46705,#46706),(#46707,#46708),(#46709,#46710),(#46711,#46712),
(#46713,#46714),(#46715,#46716),(#46717,#46718),(#46719,#46720),(#46721,
#46722),(#46723,#46724),(#46725,#46726),(#46727,#46728),(#46729,#46730),
(#46731,#46732),(#46733,#46734),(#46735,#46736),(#46737,#46738),(#46739,
#46740),(#46741,#46742),(#46743,#46744),(#46745,#46746),(#46747,#46748),
(#46749,#46750),(#46751,#46752),(#46753,#46754),(#46755,#46756),(#46757,
#46758),(#46759,#46760),(#46761,#46762),(#46763,#46764),(#46765,#46766),
(#46767,#46768),(#46769,#46770),(#46771,#46772),(#46773,#46774),(#46775,
#46776),(#46777,#46778),(#46779,#46780),(#46781,#46782),(#46783,#46784),
(#46785,#46786),(#46787,#46788),(#46789,#46790),(#46791,#46792),(#46793,
#46794),(#46795,#46796),(#46797,#46798),(#46799,#46800),(#46801,#46802),
(#46803,#46804),(#46805,#46806),(#46807,#46808),(#46809,#46810),(#46811,
#46812),(#46813,#46814),(#46815,#46816),(#46817,#46818),(#46819,#46820),
(#46821,#46822),(#46823,#46824),(#46825,#46826),(#46827,#46828),(#46829,
#46830),(#46831,#46832),(#46833,#46834),(#46835,#46836),(#46837,#46838),
(#46839,#46840),(#46841,#46842),(#46843,#46844),(#46845,#46846),(#46847,
#46848),(#46849,#46850),(#46851,#46852),(#46853,#46854),(#46855,#46856),
(#46857,#46858),(#46859,#46860),(#46861,#46862),(#46863,#46864),(#46865,
#46866),(#46867,#46868),(#46869,#46870),(#46871,#46872),(#46873,#46874),
(#46875,#46876),(#46877,#46878),(#46879,#46880),(#46881,#46882),(#46883,
#46884),(#46885,#46886),(#46887,#46888),(#46889,#46890),(#46891,#46892),
(#46893,#46894),(#46895,#46896),(#46897,#46898),(#46899,#46900),(#46901,
#46902),(#46903,#46904),(#46905,#46906),(#46907,#46908),(#46909,#46910),
(#46911,#46912),(#46913,#46914),(#46915,#46916),(#46917,#46918),(#46919,
#46920),(#46921,#46922),(#46923,#46924),(#46925,#46926),(#46927,#46928),
(#46929,#46930),(#46931,#46932),(#46933,#46934),(#46935,#46936),(#46937,
#46938),(#46939,#46940),(#46941,#46942),(#46943,#46944),(#46945,#46946),
(#46947,#46948),(#46949,#46950),(#46951,#46952),(#46953,#46954),(#46955,
#46956),(#46957,#46958),(#46959,#46960),(#46961,#46962),(#46963,#46964),
(#46965,#46966),(#46967,#46968),(#46969,#46970),(#46971,#46972),(#46973,
#46974),(#46975,#46976),(#46977,#46978),(#46979,#46980),(#46981,#46982),
(#46983,#46984),(#46985,#46986),(#46987,#46988),(#46989,#46990),(#46991,
#46992),(#46993,#46994),(#46995,#46996),(#46997,#46998),(#46999,#47000),
(#47001,#47002),(#47003,#47004),(#47005,#47006),(#47007,#47008),(#47009,
#47010),(#47011,#47012),(#47013,#47014),(#47015,#47016),(#47017,#47018),
(#47019,#47020),(#47021,#47022),(#47023,#47024),(#47025,#47026),(#47027,
#47028),(#47029,#47030),(#47031,#47032),(#47033,#47034),(#47035,#47036),
(#47037,#47038),(#47039,#47040),(#47041,#47042),(#47043,#47044),(#47045,
#47046),(#47047,#47048),(#47049,#47050),(#47051,#47052),(#47053,#47054),
(#47055,#47056),(#47057,#47058),(#47059,#47060),(#47061,#47062),(#47063,
#47064),(#47065,#47066),(#47067,#47068),(#47069,#47070),(#47071,#47072),
(#47073,#47074),(#47075,#47076),(#47077,#47078),(#47079,#47080),(#47081,
#47082),(#47083,#47084),(#47085,#47086),(#47087,#47088),(#47089,#47090),
(#47091,#47092),(#47093,#47094),(#47095,#47096),(#47097,#47098),(#47099,
#47100),(#47101,#47102),(#47103,#47104),(#47105,#47106),(#47107,#47108),
(#47109,#47110),(#47111,#47112),(#47113,#47114),(#47115,#47116),(#47117,
#47118),(#47119,#47120),(#47121,#47122),(#47123,#47124),(#47125,#47126),
(#47127,#47128),(#47129,#47130),(#47131,#47132),(#47133,#47134),(#47135,
#47136),(#47137,#47138),(#47139,#47140),(#47141,#47142),(#47143,#47144),
(#47145,#47146),(#47147,#47148),(#47149,#47150),(#47151,#47152),(#47153,
#47154),(#47155,#47156),(#47157,#47158),(#47159,#47160),(#47161,#47162),
(#47163,#47164),(#47165,#47166),(#47167,#47168),(#47169,#47170),(#47171,
#47172),(#47173,#47174),(#47175,#47176),(#47177,#47178),(#47179,#47180),
(#47181,#47182),(#47183,#47184),(#47185,#47186),(#47187,#47188),(#47189,
#47190),(#47191,#47192),(#47193,#47194),(#47195,#47196),(#47197,#47198),
(#47199,#47200),(#47201,#47202),(#47203,#47204),(#47205,#47206),(#47207,
#47208),(#47209,#47210),(#47211,#47212),(#47213,#47214),(#47215,#47216),
(#47217,#47218),(#47219,#47220),(#47221,#47222),(#47223,#47224),(#47225,
#47226),(#47227,#47228),(#47229,#47230),(#47231,#47232),(#47233,#47234),
(#47235,#47236),(#47237,#47238),(#47239,#47240),(#47241,#47242),(#47243,
#47244),(#47245,#47246),(#47247,#47248),(#47249,#47250),(#47251,#47252),
(#47253,#47254),(#47255,#47256),(#47257,#47258),(#47259,#47260),(#47261,
#47262),(#47263,#47264),(#47265,#47266),(#47267,#47268),(#47269,#47270),
(#47271,#47272),(#47273,#47274),(#47275,#47276),(#47277,#47278),(#47279,
#47280),(#47281,#47282),(#47283,#47284),(#47285,#47286),(#47287,#47288),
(#47289,#47290),(#47291,#47292),(#47293,#47294),(#47295,#47296),(#47297,
#47298),(#47299,#47300),(#47301,#47302),(#47303,#47304),(#47305,#47306),
(#47307,#47308),(#47309,#47310),(#47311,#47312),(#47313,#47314),(#47315,
#47316),(#47317,#47318),(#47319,#47320),(#47321,#47322),(#47323,#47324),
(#47325,#47326),(#47327,#47328),(#47329,#47330),(#47331,#47332),(#47333,
#47334),(#47335,#47336),(#47337,#47338),(#47339,#47340),(#47341,#47342),
(#47343,#47344),(#47345,#47346),(#47347,#47348),(#47349,#47350),(#47351,
#47352),(#47353,#47354),(#47355,#47356),(#47357,#47358),(#47359,#47360),
(#47361,#47362),(#47363,#47364),(#47365,#47366),(#47367,#47368),(#47369,
#47370),(#47371,#47372),(#47373,#47374),(#47375,#47376),(#47377,#47378),
(#47379,#47380),(#47381,#47382),(#47383,#47384),(#47385,#47386),(#47387,
#47388),(#47389,#47390),(#47391,#47392),(#47393,#47394),(#47395,#47396),
(#47397,#47398),(#47399,#47400),(#47401,#47402),(#47403,#47404),(#47405,
#47406),(#47407,#47408),(#47409,#47410),(#47411,#47412),(#47413,#47414),
(#47415,#47416),(#47417,#47418),(#47419,#47420),(#47421,#47422),(#47423,
#47424),(#47425,#47426),(#47427,#47428),(#47429,#47430),(#47431,#47432),
(#47433,#47434),(#47435,#47436),(#47437,#47438),(#47439,#47440),(#47441,
#47442),(#47443,#47444),(#47445,#47446),(#47447,#47448),(#47449,#47450),
(#47451,#47452),(#47453,#47454),(#47455,#47456),(#47457,#47458),(#47459,
#47460),(#47461,#47462),(#47463,#47464),(#47465,#47466),(#47467,#47468),
(#47469,#47470),(#47471,#47472),(#47473,#47474),(#47475,#47476),(#47477,
#47478),(#47479,#47480),(#47481,#47482),(#47483,#47484),(#47485,#47486),
(#47487,#47488),(#47489,#47490),(#47491,#47492),(#47493,#47494),(#47495,
#47496),(#47497,#47498),(#47499,#47500),(#47501,#47502),(#47503,#47504),
(#47505,#47506),(#47507,#47508),(#47509,#47510),(#47511,#47512),(#47513,
#47514),(#47515,#47516),(#47517,#47518),(#47519,#47520),(#47521,#47522),
(#47523,#47524),(#47525,#47526),(#47527,#47528),(#47529,#47530),(#47531,
#47532),(#47533,#47534),(#47535,#47536),(#47537,#47538),(#47539,#47540),
(#47541,#47542),(#47543,#47544),(#47545,#47546),(#47547,#47548),(#47549,
#47550),(#47551,#47552),(#47553,#47554),(#47555,#47556),(#47557,#47558),
(#47559,#47560),(#47561,#47562),(#47563,#47564),(#47565,#47566),(#47567,
#47568),(#47569,#47570),(#47571,#47572),(#47573,#47574),(#47575,#47576),
(#47577,#47578),(#47579,#47580),(#47581,#47582),(#47583,#47584),(#47585,
#47586),(#47587,#47588),(#47589,#47590),(#47591,#47592),(#47593,#47594),
(#47595,#47596),(#47597,#47598),(#47599,#47600),(#47601,#47602),(#47603,
#47604),(#47605,#47606),(#47607,#47608),(#47609,#47610),(#47611,#47612),
(#47613,#47614),(#47615,#47616),(#47617,#47618),(#47619,#47620),(#47621,
#47622),(#47623,#47624),(#47625,#47626),(#47627,#47628),(#47629,#47630),
(#47631,#47632),(#47633,#47634),(#47635,#47636),(#47637,#47638),(#47639,
#47640),(#47641,#47642),(#47643,#47644),(#47645,#47646),(#47647,#47648),
(#47649,#47650),(#47651,#47652),(#47653,#47654),(#47655,#47656),(#47657,
#47658),(#47659,#47660),(#47661,#47662),(#47663,#47664),(#47665,#47666),
(#47667,#47668),(#47669,#47670),(#47671,#47672),(#47673,#47674),(#47675,
#47676),(#47677,#47678),(#47679,#47680),(#47681,#47682),(#47683,#47684),
(#47685,#47686),(#47687,#47688),(#47689,#47690),(#47691,#47692),(#47693,
#47694),(#47695,#47696),(#47697,#47698),(#47699,#47700),(#47701,#47702),
(#47703,#47704),(#47705,#47706),(#47707,#47708),(#47709,#47710),(#47711,
#47712),(#47713,#47714),(#47715,#47716),(#47717,#47718),(#47719,#47720),
(#47721,#47722),(#47723,#47724),(#47725,#47726),(#47727,#47728),(#47729,
#47730),(#47731,#47732),(#47733,#47734),(#47735,#47736),(#47737,#47738),
(#47739,#47740),(#47741,#47742),(#47743,#47744),(#47745,#47746),(#47747,
#47748),(#47749,#47750),(#47751,#47752),(#47753,#47754),(#47755,#47756),
(#47757,#47758),(#47759,#47760),(#47761,#47762),(#47763,#47764),(#47765,
#47766),(#47767,#47768),(#47769,#47770),(#47771,#47772),(#47773,#47774),
(#47775,#47776),(#47777,#47778),(#47779,#47780),(#47781,#47782),(#47783,
#47784),(#47785,#47786),(#47787,#47788),(#47789,#47790),(#47791,#47792),
(#47793,#47794),(#47795,#47796),(#47797,#47798),(#47799,#47800),(#47801,
#47802),(#47803,#47804),(#47805,#47806),(#47807,#47808),(#47809,#47810),
(#47811,#47812),(#47813,#47814),(#47815,#47816),(#47817,#47818),(#47819,
#47820),(#47821,#47822),(#47823,#47824),(#47825,#47826),(#47827,#47828),
(#47829,#47830),(#47831,#47832),(#47833,#47834),(#47835,#47836),(#47837,
#47838),(#47839,#47840),(#47841,#47842),(#47843,#47844),(#47845,#47846),
(#47847,#47848),(#47849,#47850),(#47851,#47852),(#47853,#47854),(#47855,
#47856),(#47857,#47858),(#47859,#47860),(#47861,#47862),(#47863,#47864),
(#47865,#47866),(#47867,#47868),(#47869,#47870),(#47871,#47872),(#47873,
#47874),(#47875,#47876),(#47877,#47878),(#47879,#47880),(#47881,#47882),
(#47883,#47884),(#47885,#47886),(#47887,#47888),(#47889,#47890),(#47891,
#47892),(#47893,#47894),(#47895,#47896),(#47897,#47898),(#47899,#47900),
(#47901,#47902),(#47903,#47904),(#47905,#47906),(#47907,#47908),(#47909,
#47910),(#47911,#47912),(#47913,#47914),(#47915,#47916),(#47917,#47918),
(#47919,#47920),(#47921,#47922),(#47923,#47924),(#47925,#47926),(#47927,
#47928),(#47929,#47930),(#47931,#47932),(#47933,#47934),(#47935,#47936),
(#47937,#47938),(#47939,#47940),(#47941,#47942),(#47943,#47944),(#47945,
#47946),(#47947,#47948),(#47949,#47950),(#47951,#47952),(#47953,#47954),
(#47955,#47956),(#47957,#47958),(#47959,#47960),(#47961,#47962),(#47963,
#47964),(#47965,#47966),(#47967,#47968),(#47969,#47970),(#47971,#47972),
(#47973,#47974),(#47975,#47976),(#47977,#47978),(#47979,#47980),(#47981,
#47982),(#47983,#47984),(#47985,#47986),(#47987,#47988),(#47989,#47990),
(#47991,#47992),(#47993,#47994),(#47995,#47996),(#47997,#47998),(#47999,
#48000),(#48001,#48002),(#48003,#48004),(#48005,#48006),(#48007,#48008),
(#48009,#48010),(#48011,#48012),(#48013,#48014),(#48015,#48016),(#48017,
#48018),(#48019,#48020),(#48021,#48022),(#48023,#48024),(#48025,#48026),
(#48027,#48028),(#48029,#48030),(#48031,#48032),(#48033,#48034),(#48035,
#48036),(#48037,#48038),(#48039,#48040),(#48041,#48042),(#48043,#48044),
(#48045,#48046),(#48047,#48048),(#48049,#48050),(#48051,#48052),(#48053,
#48054),(#48055,#48056),(#48057,#48058),(#48059,#48060),(#48061,#48062),
(#48063,#48064),(#48065,#48066),(#48067,#48068),(#48069,#48070),(#48071,
#48072),(#48073,#48074),(#48075,#48076),(#48077,#48078),(#48079,#48080),
(#48081,#48082),(#48083,#48084),(#48085,#48086),(#48087,#48088),(#48089,
#48090),(#48091,#48092),(#48093,#48094),(#48095,#48096),(#48097,#48098),
(#48099,#48100),(#48101,#48102),(#48103,#48104),(#48105,#48106),(#48107,
#48108),(#48109,#48110),(#48111,#48112),(#48113,#48114),(#48115,#48116),
(#48117,#48118),(#48119,#48120),(#48121,#48122),(#48123,#48124),(#48125,
#48126),(#48127,#48128),(#48129,#48130),(#48131,#48132),(#48133,#48134),
(#48135,#48136),(#48137,#48138),(#48139,#48140),(#48141,#48142),(#48143,
#48144),(#48145,#48146),(#48147,#48148),(#48149,#48150),(#48151,#48152),
(#48153,#48154),(#48155,#48156),(#48157,#48158),(#48159,#48160),(#48161,
#48162),(#48163,#48164),(#48165,#48166),(#48167,#48168),(#48169,#48170),
(#48171,#48172),(#48173,#48174),(#48175,#48176),(#48177,#48178),(#48179,
#48180),(#48181,#48182),(#48183,#48184),(#48185,#48186),(#48187,#48188),
(#48189,#48190),(#48191,#48192),(#48193,#48194),(#48195,#48196),(#48197,
#48198),(#48199,#48200),(#48201,#48202),(#48203,#48204),(#48205,#48206),
(#48207,#48208),(#48209,#48210),(#48211,#48212),(#48213,#48214),(#48215,
#48216),(#48217,#48218),(#48219,#48220),(#48221,#48222),(#48223,#48224),
(#48225,#48226),(#48227,#48228),(#48229,#48230),(#48231,#48232),(#48233,
#48234),(#48235,#48236),(#48237,#48238),(#48239,#48240),(#48241,#48242),
(#48243,#48244),(#48245,#48246),(#48247,#48248),(#48249,#48250),(#48251,
#48252),(#48253,#48254),(#48255,#48256),(#48257,#48258),(#48259,#48260),
(#48261,#48262),(#48263,#48264),(#48265,#48266),(#48267,#48268),(#48269,
#48270),(#48271,#48272),(#48273,#48274),(#48275,#48276),(#48277,#48278),
(#48279,#48280),(#48281,#48282),(#48283,#48284),(#48285,#48286),(#48287,
#48288),(#48289,#48290),(#48291,#48292),(#48293,#48294),(#48295,#48296),
(#48297,#48298),(#48299,#48300),(#48301,#48302),(#48303,#48304),(#48305,
#48306),(#48307,#48308),(#48309,#48310),(#48311,#48312),(#48313,#48314),
(#48315,#48316),(#48317,#48318),(#48319,#48320),(#48321,#48322),(#48323,
#48324),(#48325,#48326),(#48327,#48328),(#48329,#48330),(#48331,#48332),
(#48333,#48334),(#48335,#48336),(#48337,#48338),(#48339,#48340),(#48341,
#48342),(#48343,#48344),(#48345,#48346),(#48347,#48348),(#48349,#48350),
(#48351,#48352),(#48353,#48354),(#48355,#48356),(#48357,#48358),(#48359,
#48360),(#48361,#48362),(#48363,#48364),(#48365,#48366),(#48367,#48368),
(#48369,#48370),(#48371,#48372),(#48373,#48374),(#48375,#48376),(#48377,
#48378),(#48379,#48380),(#48381,#48382),(#48383,#48384),(#48385,#48386),
(#48387,#48388),(#48389,#48390),(#48391,#48392),(#48393,#48394),(#48395,
#48396),(#48397,#48398),(#48399,#48400),(#48401,#48402),(#48403,#48404),
(#48405,#48406),(#48407,#48408),(#48409,#48410),(#48411,#48412),(#48413,
#48414),(#48415,#48416),(#48417,#48418),(#48419,#48420),(#48421,#48422),
(#48423,#48424),(#48425,#48426),(#48427,#48428),(#48429,#48430),(#48431,
#48432),(#48433,#48434),(#48435,#48436),(#48437,#48438),(#48439,#48440),
(#48441,#48442),(#48443,#48444),(#48445,#48446),(#48447,#48448),(#48449,
#48450),(#48451,#48452),(#48453,#48454),(#48455,#48456),(#48457,#48458),
(#48459,#48460),(#48461,#48462),(#48463,#48464),(#48465,#48466),(#48467,
#48468),(#48469,#48470),(#48471,#48472),(#48473,#48474),(#48475,#48476),
(#48477,#48478),(#48479,#48480),(#48481,#48482),(#48483,#48484),(#48485,
#48486),(#48487,#48488),(#48489,#48490),(#48491,#48492),(#48493,#48494),
(#48495,#48496),(#48497,#48498),(#48499,#48500),(#48501,#48502),(#48503,
#48504),(#48505,#48506),(#48507,#48508),(#48509,#48510),(#48511,#48512),
(#48513,#48514),(#48515,#48516),(#48517,#48518),(#48519,#48520),(#48521,
#48522),(#48523,#48524),(#48525,#48526),(#48527,#48528),(#48529,#48530),
(#48531,#48532),(#48533,#48534),(#48535,#48536),(#48537,#48538),(#48539,
#48540),(#48541,#48542),(#48543,#48544),(#48545,#48546),(#48547,#48548),
(#48549,#48550),(#48551,#48552),(#48553,#48554),(#48555,#48556),(#48557,
#48558),(#48559,#48560),(#48561,#48562),(#48563,#48564),(#48565,#48566),
(#48567,#48568),(#48569,#48570),(#48571,#48572),(#48573,#48574),(#48575,
#48576),(#48577,#48578),(#48579,#48580),(#48581,#48582),(#48583,#48584),
(#48585,#48586),(#48587,#48588),(#48589,#48590),(#48591,#48592),(#48593,
#48594),(#48595,#48596),(#48597,#48598),(#48599,#48600),(#48601,#48602),
(#48603,#48604),(#48605,#48606),(#48607,#48608),(#48609,#48610),(#48611,
#48612),(#48613,#48614),(#48615,#48616),(#48617,#48618),(#48619,#48620),
(#48621,#48622),(#48623,#48624),(#48625,#48626),(#48627,#48628),(#48629,
#48630),(#48631,#48632),(#48633,#48634),(#48635,#48636),(#48637,#48638),
(#48639,#48640),(#48641,#48642),(#48643,#48644),(#48645,#48646),(#48647,
#48648),(#48649,#48650),(#48651,#48652),(#48653,#48654),(#48655,#48656),
(#48657,#48658),(#48659,#48660),(#48661,#48662),(#48663,#48664),(#48665,
#48666),(#48667,#48668),(#48669,#48670),(#48671,#48672),(#48673,#48674),
(#48675,#48676),(#48677,#48678),(#48679,#48680),(#48681,#48682),(#48683,
#48684),(#48685,#48686),(#48687,#48688),(#48689,#48690),(#48691,#48692),
(#48693,#48694),(#48695,#48696),(#48697,#48698),(#48699,#48700),(#48701,
#48702),(#48703,#48704),(#48705,#48706),(#48707,#48708),(#48709,#48710),
(#48711,#48712),(#48713,#48714),(#48715,#48716),(#48717,#48718),(#48719,
#48720),(#48721,#48722),(#48723,#48724),(#48725,#48726),(#48727,#48728),
(#48729,#48730),(#48731,#48732),(#48733,#48734),(#48735,#48736),(#48737,
#48738),(#48739,#48740),(#48741,#48742),(#48743,#48744),(#48745,#48746),
(#48747,#48748),(#48749,#48750),(#48751,#48752),(#48753,#48754),(#48755,
#48756),(#48757,#48758),(#48759,#48760),(#48761,#48762),(#48763,#48764),
(#48765,#48766),(#48767,#48768),(#48769,#48770),(#48771,#48772),(#48773,
#48774),(#48775,#48776),(#48777,#48778),(#48779,#48780),(#48781,#48782),
(#48783,#48784),(#48785,#48786),(#48787,#48788),(#48789,#48790),(#48791,
#48792),(#48793,#48794),(#48795,#48796),(#48797,#48798),(#48799,#48800),
(#48801,#48802),(#48803,#48804),(#48805,#48806),(#48807,#48808),(#48809,
#48810),(#48811,#48812),(#48813,#48814),(#48815,#48816),(#48817,#48818),
(#48819,#48820),(#48821,#48822),(#48823,#48824),(#48825,#48826),(#48827,
#48828),(#48829,#48830),(#48831,#48832),(#48833,#48834),(#48835,#48836),
(#48837,#48838),(#48839,#48840),(#48841,#48842),(#48843,#48844),(#48845,
#48846),(#48847,#48848),(#48849,#48850),(#48851,#48852),(#48853,#48854),
(#48855,#48856),(#48857,#48858),(#48859,#48860),(#48861,#48862),(#48863,
#48864),(#48865,#48866),(#48867,#48868),(#48869,#48870),(#48871,#48872),
(#48873,#48874),(#48875,#48876),(#48877,#48878),(#48879,#48880),(#48881,
#48882),(#48883,#48884),(#48885,#48886),(#48887,#48888),(#48889,#48890),
(#48891,#48892),(#48893,#48894),(#48895,#48896),(#48897,#48898),(#48899,
#48900),(#48901,#48902),(#48903,#48904),(#48905,#48906),(#48907,#48908),
(#48909,#48910),(#48911,#48912),(#48913,#48914),(#48915,#48916),(#48917,
#48918),(#48919,#48920),(#48921,#48922),(#48923,#48924),(#48925,#48926),
(#48927,#48928),(#48929,#48930),(#48931,#48932),(#48933,#48934),(#48935,
#48936),(#48937,#48938),(#48939,#48940),(#48941,#48942),(#48943,#48944),
(#48945,#48946),(#48947,#48948),(#48949,#48950),(#48951,#48952),(#48953,
#48954),(#48955,#48956),(#48957,#48958),(#48959,#48960),(#48961,#48962),
(#48963,#48964),(#48965,#48966),(#48967,#48968),(#48969,#48970),(#48971,
#48972),(#48973,#48974),(#48975,#48976),(#48977,#48978),(#48979,#48980),
(#48981,#48982),(#48983,#48984),(#48985,#48986),(#48987,#48988),(#48989,
#48990),(#48991,#48992),(#48993,#48994),(#48995,#48996),(#48997,#48998),
(#48999,#49000),(#49001,#49002),(#49003,#49004),(#49005,#49006),(#49007,
#49008),(#49009,#49010),(#49011,#49012),(#49013,#49014),(#49015,#49016),
(#49017,#49018),(#49019,#49020),(#49021,#49022),(#49023,#49024),(#49025,
#49026),(#49027,#49028),(#49029,#49030),(#49031,#49032),(#49033,#49034),
(#49035,#49036),(#49037,#49038),(#49039,#49040),(#49041,#49042),(#49043,
#49044),(#49045,#49046),(#49047,#49048),(#49049,#49050),(#49051,#49052),
(#49053,#49054),(#49055,#49056),(#49057,#49058),(#49059,#49060),(#49061,
#49062),(#49063,#49064),(#49065,#49066),(#49067,#49068),(#49069,#49070),
(#49071,#49072),(#49073,#49074),(#49075,#49076),(#49077,#49078),(#49079,
#49080),(#49081,#49082),(#49083,#49084),(#49085,#49086),(#49087,#49088),
(#49089,#49090),(#49091,#49092),(#49093,#49094),(#49095,#49096),(#49097,
#49098),(#49099,#49100),(#49101,#49102),(#49103,#49104),(#49105,#49106),
(#49107,#49108),(#49109,#49110),(#49111,#49112),(#49113,#49114),(#49115,
#49116),(#49117,#49118),(#49119,#49120),(#49121,#49122),(#49123,#49124),
(#49125,#49126),(#49127,#49128),(#49129,#49130),(#49131,#49132),(#49133,
#49134),(#49135,#49136),(#49137,#49138),(#49139,#49140),(#49141,#49142),
(#49143,#49144),(#49145,#49146),(#49147,#49148),(#49149,#49150),(#49151,
#49152),(#49153,#49154),(#49155,#49156),(#49157,#49158),(#49159,#49160),
(#49161,#49162),(#49163,#49164),(#49165,#49166),(#49167,#49168),(#49169,
#49170),(#49171,#49172),(#49173,#49174),(#49175,#49176),(#49177,#49178),
(#49179,#49180),(#49181,#49182),(#49183,#49184),(#49185,#49186),(#49187,
#49188),(#49189,#49190),(#49191,#49192),(#49193,#49194),(#49195,#49196),
(#49197,#49198),(#49199,#49200),(#49201,#49202),(#49203,#49204),(#49205,
#49206),(#49207,#49208),(#49209,#49210),(#49211,#49212),(#49213,#49214),
(#49215,#49216),(#49217,#49218),(#49219,#49220),(#49221,#49222),(#49223,
#49224),(#49225,#49226),(#49227,#49228),(#49229,#49230),(#49231,#49232),
(#49233,#49234),(#49235,#49236),(#49237,#49238),(#49239,#49240),(#49241,
#49242),(#49243,#49244),(#49245,#49246),(#49247,#49248),(#49249,#49250),
(#49251,#49252),(#49253,#49254),(#49255,#49256),(#49257,#49258),(#49259,
#49260),(#49261,#49262),(#49263,#49264),(#49265,#49266),(#49267,#49268),
(#49269,#49270),(#49271,#49272),(#49273,#49274),(#49275,#49276),(#49277,
#49278),(#49279,#49280),(#49281,#49282),(#49283,#49284),(#49285,#49286),
(#49287,#49288),(#49289,#49290),(#49291,#49292),(#49293,#49294),(#49295,
#49296),(#49297,#49298),(#49299,#49300),(#49301,#49302),(#49303,#49304),
(#49305,#49306),(#49307,#49308),(#49309,#49310),(#49311,#49312),(#49313,
#49314),(#49315,#49316),(#49317,#49318),(#49319,#49320),(#49321,#49322),
(#49323,#49324),(#49325,#49326),(#49327,#49328),(#49329,#49330),(#49331,
#49332),(#49333,#49334),(#49335,#49336),(#49337,#49338),(#49339,#49340),
(#49341,#49342),(#49343,#49344),(#49345,#49346),(#49347,#49348),(#49349,
#49350),(#49351,#49352),(#49353,#49354),(#49355,#49356),(#49357,#49358),
(#49359,#49360),(#49361,#49362),(#49363,#49364),(#49365,#49366),(#49367,
#49368),(#49369,#49370),(#49371,#49372),(#49373,#49374),(#49375,#49376),
(#49377,#49378),(#49379,#49380),(#49381,#49382),(#49383,#49384),(#49385,
#49386),(#49387,#49388),(#49389,#49390),(#49391,#49392),(#49393,#49394),
(#49395,#49396),(#49397,#49398),(#49399,#49400),(#49401,#49402),(#49403,
#49404),(#49405,#49406),(#49407,#49408),(#49409,#49410),(#49411,#49412),
(#49413,#49414),(#49415,#49416),(#49417,#49418),(#49419,#49420),(#49421,
#49422),(#49423,#49424),(#49425,#49426),(#49427,#49428),(#49429,#49430),
(#49431,#49432),(#49433,#49434),(#49435,#49436),(#49437,#49438),(#49439,
#49440),(#49441,#49442),(#49443,#49444),(#49445,#49446),(#49447,#49448),
(#49449,#49450),(#49451,#49452),(#49453,#49454),(#49455,#49456),(#49457,
#49458),(#49459,#49460),(#49461,#49462),(#49463,#49464),(#49465,#49466),
(#49467,#49468),(#49469,#49470),(#49471,#49472),(#49473,#49474),(#49475,
#49476),(#49477,#49478),(#49479,#49480),(#49481,#49482),(#49483,#49484),
(#49485,#49486),(#49487,#49488),(#49489,#49490),(#49491,#49492),(#49493,
#49494),(#49495,#49496),(#49497,#49498),(#49499,#49500),(#49501,#49502),
(#49503,#49504),(#49505,#49506),(#49507,#49508),(#49509,#49510),(#49511,
#49512),(#49513,#49514),(#49515,#49516),(#49517,#49518),(#49519,#49520),
(#49521,#49522),(#49523,#49524),(#49525,#49526),(#49527,#49528),(#49529,
#49530),(#49531,#49532),(#49533,#49534),(#49535,#49536),(#49537,#49538),
(#49539,#49540),(#49541,#49542),(#49543,#49544),(#49545,#49546),(#49547,
#49548),(#49549,#49550),(#49551,#49552),(#49553,#49554),(#49555,#49556),
(#49557,#49558),(#49559,#49560),(#49561,#49562),(#49563,#49564),(#49565,
#49566),(#49567,#49568),(#49569,#49570),(#49571,#49572),(#49573,#49574),
(#49575,#49576),(#49577,#49578),(#49579,#49580),(#49581,#49582),(#49583,
#49584),(#49585,#49586),(#49587,#49588),(#49589,#49590),(#49591,#49592),
(#49593,#49594),(#49595,#49596),(#49597,#49598),(#49599,#49600),(#49601,
#49602),(#49603,#49604),(#49605,#49606),(#49607,#49608),(#49609,#49610),
(#49611,#49612),(#49613,#49614),(#49615,#49616),(#49617,#49618),(#49619,
#49620),(#49621,#49622),(#49623,#49624),(#49625,#49626),(#49627,#49628),
(#49629,#49630),(#49631,#49632),(#49633,#49634),(#49635,#49636),(#49637,
#49638),(#49639,#49640),(#49641,#49642),(#49643,#49644),(#49645,#49646),
(#49647,#49648),(#49649,#49650),(#49651,#49652),(#49653,#49654),(#49655,
#49656),(#49657,#49658),(#49659,#49660),(#49661,#49662),(#49663,#49664),
(#49665,#49666),(#49667,#49668),(#49669,#49670),(#49671,#49672),(#49673,
#49674),(#49675,#49676),(#49677,#49678),(#49679,#49680),(#49681,#49682),
(#49683,#49684),(#49685,#49686),(#49687,#49688),(#49689,#49690),(#49691,
#49692),(#49693,#49694),(#49695,#49696),(#49697,#49698),(#49699,#49700),
(#49701,#49702),(#49703,#49704),(#49705,#49706),(#49707,#49708),(#49709,
#49710),(#49711,#49712),(#49713,#49714),(#49715,#49716),(#49717,#49718),
(#49719,#49720),(#49721,#49722),(#49723,#49724),(#49725,#49726),(#49727,
#49728),(#49729,#49730),(#49731,#49732),(#49733,#49734),(#49735,#49736),
(#49737,#49738),(#49739,#49740),(#49741,#49742),(#49743,#49744),(#49745,
#49746),(#49747,#49748),(#49749,#49750),(#49751,#49752),(#49753,#49754),
(#49755,#49756),(#49757,#49758),(#49759,#49760),(#49761,#49762),(#49763,
#49764),(#49765,#49766),(#49767,#49768),(#49769,#49770),(#49771,#49772),
(#49773,#49774),(#49775,#49776),(#49777,#49778),(#49779,#49780),(#49781,
#49782),(#49783,#49784),(#49785,#49786),(#49787,#49788),(#49789,#49790),
(#49791,#49792),(#49793,#49794),(#49795,#49796),(#49797,#49798),(#49799,
#49800),(#49801,#49802),(#49803,#49804),(#49805,#49806),(#49807,#49808),
(#49809,#49810),(#49811,#49812),(#49813,#49814),(#49815,#49816),(#49817,
#49818),(#49819,#49820),(#49821,#49822),(#49823,#49824),(#49825,#49826),
(#49827,#49828),(#49829,#49830),(#49831,#49832),(#49833,#49834),(#49835,
#49836),(#49837,#49838),(#49839,#49840),(#49841,#49842),(#49843,#49844),
(#49845,#49846),(#49847,#49848),(#49849,#49850),(#49851,#49852),(#49853,
#49854),(#49855,#49856),(#49857,#49858),(#49859,#49860),(#49861,#49862),
(#49863,#49864),(#49865,#49866),(#49867,#49868),(#49869,#49870),(#49871,
#49872),(#49873,#49874),(#49875,#49876),(#49877,#49878),(#49879,#49880),
(#49881,#49882),(#49883,#49884),(#49885,#49886),(#49887,#49888),(#49889,
#49890),(#49891,#49892),(#49893,#49894),(#49895,#49896),(#49897,#49898),
(#49899,#49900),(#49901,#49902),(#49903,#49904),(#49905,#49906),(#49907,
#49908),(#49909,#49910),(#49911,#49912),(#49913,#49914),(#49915,#49916),
(#49917,#49918),(#49919,#49920),(#49921,#49922),(#49923,#49924),(#49925,
#49926),(#49927,#49928),(#49929,#49930),(#49931,#49932),(#49933,#49934),
(#49935,#49936),(#49937,#49938),(#49939,#49940),(#49941,#49942),(#49943,
#49944),(#49945,#49946),(#49947,#49948),(#49949,#49950),(#49951,#49952),
(#49953,#49954),(#49955,#49956),(#49957,#49958),(#49959,#49960),(#49961,
#49962),(#49963,#49964),(#49965,#49966),(#49967,#49968),(#49969,#49970),
(#49971,#49972),(#49973,#49974),(#49975,#49976),(#49977,#49978),(#49979,
#49980),(#49981,#49982),(#49983,#49984),(#49985,#49986),(#49987,#49988),
(#49989,#49990),(#49991,#49992),(#49993,#49994),(#49995,#49996),(#49997,
#49998),(#49999,#50000),(#50001,#50002),(#50003,#50004),(#50005,#50006),
(#50007,#50008),(#50009,#50010),(#50011,#50012),(#50013,#50014),(#50015,
#50016),(#50017,#50018),(#50019,#50020),(#50021,#50022),(#50023,#50024),
(#50025,#50026),(#50027,#50028),(#50029,#50030),(#50031,#50032),(#50033,
#50034),(#50035,#50036),(#50037,#50038),(#50039,#50040),(#50041,#50042),
(#50043,#50044),(#50045,#50046),(#50047,#50048),(#50049,#50050),(#50051,
#50052),(#50053,#50054),(#50055,#50056),(#50057,#50058),(#50059,#50060),
(#50061,#50062),(#50063,#50064),(#50065,#50066),(#50067,#50068),(#50069,
#50070),(#50071,#50072),(#50073,#50074),(#50075,#50076),(#50077,#50078),
(#50079,#50080),(#50081,#50082),(#50083,#50084),(#50085,#50086),(#50087,
#50088),(#50089,#50090),(#50091,#50092),(#50093,#50094),(#50095,#50096),
(#50097,#50098),(#50099,#50100),(#50101,#50102),(#50103,#50104),(#50105,
#50106),(#50107,#50108),(#50109,#50110),(#50111,#50112),(#50113,#50114),
(#50115,#50116),(#50117,#50118),(#50119,#50120),(#50121,#50122),(#50123,
#50124),(#50125,#50126),(#50127,#50128),(#50129,#50130),(#50131,#50132),
(#50133,#50134),(#50135,#50136),(#50137,#50138),(#50139,#50140),(#50141,
#50142),(#50143,#50144),(#50145,#50146),(#50147,#50148),(#50149,#50150),
(#50151,#50152),(#50153,#50154),(#50155,#50156),(#50157,#50158),(#50159,
#50160),(#50161,#50162),(#50163,#50164),(#50165,#50166),(#50167,#50168),
(#50169,#50170),(#50171,#50172),(#50173,#50174),(#50175,#50176),(#50177,
#50178),(#50179,#50180),(#50181,#50182),(#50183,#50184),(#50185,#50186),
(#50187,#50188),(#50189,#50190),(#50191,#50192),(#50193,#50194),(#50195,
#50196),(#50197,#50198),(#50199,#50200),(#50201,#50202),(#50203,#50204),
(#50205,#50206),(#50207,#50208),(#50209,#50210),(#50211,#50212),(#50213,
#50214),(#50215,#50216),(#50217,#50218),(#50219,#50220),(#50221,#50222)),
 .UNSPECIFIED.,.F.,.F.,.F.,(4,1,1,1,1,1,1,1,1,1,1,1,1,1,1,1,1,1,1,1,1,1,
1,1,1,1,1,1,1,1,1,1,1,1,1,1,1,1,1,1,1,1,1,1,1,1,1,1,1,1,1,1,1,1,1,1,1,1,
1,1,1,1,1,1,1,1,1,1,1,1,1,1,1,1,1,1,1,1,1,1,1,1,1,1,1,1,1,1,1,1,1,1,1,1,
1,1,1,1,1,1,1,1,1,1,1,1,1,1,1,1,1,1,1,1,1,1,1,1,1,1,1,1,1,1,1,1,1,1,1,1,
1,1,1,1,1,1,1,1,1,1,1,1,1,1,1,1,1,1,1,1,1,1,1,1,1,1,1,1,1,1,1,1,1,1,1,1,
1,1,1,1,1,1,1,1,1,1,1,1,1,1,1,1,1,1,1,1,1,1,1,1,1,1,1,1,1,1,1,1,1,1,1,1,
1,1,1,1,1,1,1,1,1,1,1,1,1,1,1,1,1,1,1,1,1,1,1,1,1,1,1,1,1,1,1,1,1,1,1,1,
1,1,1,1,1,1,1,1,1,1,1,1,1,1,1,1,1,1,1,1,1,1,1,1,1,1,1,1,1,1,1,1,1,1,1,1,
1,1,1,1,1,1,1,1,1,1,1,1,1,1,1,1,1,1,1,1,1,1,1,1,1,1,1,1,1,1,1,1,1,1,1,1,
1,1,1,1,1,1,1,1,1,1,1,1,1,1,1,1,1,1,1,1,1,1,1,1,1,1,1,1,1,1,1,1,1,1,1,1,
1,1,1,1,1,1,1,1,1,1,1,1,1,1,1,1,1,1,1,1,1,1,1,1,1,1,1,1,1,1,1,1,1,1,1,1,
1,1,1,1,1,1,1,1,1,1,1,1,1,1,1,1,1,1,1,1,1,1,1,1,1,1,1,1,1,1,1,1,1,1,1,1,
1,1,1,1,1,1,1,1,1,1,1,1,1,1,1,1,1,1,1,1,1,1,1,1,1,1,1,1,1,1,1,1,1,1,1,1,
1,1,1,1,1,1,1,1,1,1,1,1,1,1,1,1,1,1,1,1,1,1,1,1,1,1,1,1,1,1,1,1,1,1,1,1,
1,1,1,1,1,1,1,1,1,1,1,1,1,1,1,1,1,1,1,1,1,1,1,1,1,1,1,1,1,1,1,1,1,1,1,1,
1,1,1,1,1,1,1,1,1,1,1,1,1,1,1,1,1,1,1,1,1,1,1,1,1,1,1,1,1,1,1,1,1,1,1,1,
1,1,1,1,1,1,1,1,1,1,1,1,1,1,1,1,1,1,1,1,1,1,1,1,1,1,1,1,1,1,1,1,1,1,1,1,
1,1,1,1,1,1,1,1,1,1,1,1,1,1,1,1,1,1,1,1,1,1,1,1,1,1,1,1,1,1,1,1,1,1,1,1,
1,1,1,1,1,1,1,1,1,1,1,1,1,1,1,1,1,1,1,1,1,1,1,1,1,1,1,1,1,1,1,1,1,1,1,1,
1,1,1,1,1,1,1,1,1,1,1,1,1,1,1,1,1,1,1,1,1,1,1,1,1,1,1,1,1,1,1,1,1,1,1,1,
1,1,1,1,1,1,1,1,1,1,1,1,1,1,1,1,1,1,1,1,1,1,1,1,1,1,1,1,1,1,1,1,1,1,1,1,
1,1,1,1,1,1,1,1,1,1,1,1,1,1,1,1,1,1,1,1,1,1,1,1,1,1,1,1,1,1,1,1,1,1,1,1,
1,1,1,1,1,1,1,1,1,1,1,1,1,1,1,1,1,1,1,1,1,1,1,1,1,1,1,1,1,1,1,1,1,1,1,1,
1,1,1,1,1,1,1,1,1,1,1,1,1,1,1,1,1,1,1,1,1,1,1,1,1,1,1,1,1,1,1,1,1,1,1,1,
1,1,1,1,1,1,1,1,1,1,1,1,1,1,1,1,1,1,1,1,1,1,1,1,1,1,1,1,1,1,1,1,1,1,1,1,
1,1,1,1,1,1,1,1,1,1,1,1,1,1,1,1,1,1,1,1,1,1,1,1,1,1,1,1,1,1,1,1,1,1,1,1,
1,1,1,1,1,1,1,1,1,1,1,1,1,1,1,1,1,1,1,1,1,1,1,1,1,1,1,1,1,1,1,1,1,1,1,1,
1,1,1,1,1,1,1,1,1,1,1,1,1,1,1,1,1,1,1,1,1,1,1,1,1,1,1,1,1,1,1,1,1,1,1,1,
1,1,1,1,1,1,1,1,1,1,1,1,1,1,1,1,1,1,1,1,1,1,1,1,1,1,1,1,1,1,1,1,1,1,1,1,
1,1,1,1,1,1,1,1,1,1,1,1,1,1,1,1,1,1,1,1,1,1,1,1,1,1,1,1,1,1,1,1,1,1,1,1,
1,1,1,1,1,1,1,1,1,1,1,1,1,1,1,1,1,1,1,1,1,1,1,1,1,1,1,1,1,1,1,1,1,1,1,1,
1,1,1,1,1,1,1,1,1,1,1,1,1,1,1,1,1,1,1,1,1,1,1,1,1,1,1,1,1,1,1,1,1,1,1,1,
1,1,1,1,1,1,1,1,1,1,1,1,1,1,1,1,1,1,1,1,1,1,1,1,1,1,1,1,1,1,1,1,1,1,1,1,
1,1,1,1,1,1,1,1,1,1,1,1,1,1,1,1,1,1,1,1,1,1,1,1,1,1,1,1,1,1,1,1,1,1,1,1,
1,1,1,1,1,1,1,1,1,1,1,1,1,1,1,1,1,1,1,1,1,1,1,1,1,1,1,1,1,1,1,1,1,1,1,1,
1,1,1,1,1,1,1,1,1,1,1,1,1,1,1,1,1,1,1,1,1,1,1,1,1,1,1,1,1,1,1,1,1,1,1,1,
1,1,1,1,1,1,1,1,1,1,1,1,1,1,1,1,1,1,1,1,1,1,1,1,1,1,1,1,1,1,1,1,1,1,1,1,
1,1,1,1,1,1,1,1,1,1,1,1,1,1,1,1,1,1,1,1,1,1,1,1,1,1,1,1,1,1,1,1,1,1,1,1,
1,1,1,1,1,1,1,1,1,1,1,1,1,1,1,1,1,1,1,1,1,1,1,1,1,1,1,1,1,1,1,1,1,1,1,1,
1,1,1,1,1,1,1,1,1,1,1,1,1,1,1,1,1,1,1,1,1,1,1,1,1,1,1,1,1,1,1,1,1,1,1,1,
1,1,1,1,1,1,1,1,1,1,1,1,1,1,1,1,1,1,1,1,1,1,1,1,1,1,1,1,1,1,1,1,1,1,1,1,
1,1,1,1,1,1,1,1,1,1,1,1,1,1,1,1,1,1,1,1,1,1,1,1,1,1,1,1,1,1,1,1,1,1,1,1,
1,1,1,1,1,1,1,1,1,1,1,1,1,1,1,1,1,1,1,1,1,1,1,1,1,1,1,1,1,1,1,1,1,1,1,1,
1,1,1,1,1,1,1,1,1,1,1,1,1,1,1,1,1,1,1,1,1,1,1,1,1,1,1,1,1,1,1,1,1,1,1,1,
1,1,1,1,1,1,1,1,1,1,1,1,1,1,1,1,1,1,1,1,1,1,1,1,1,1,1,1,1,1,1,1,1,1,1,1,
1,1,1,1,1,1,1,1,1,1,1,1,1,1,1,1,1,1,1,1,1,1,1,1,1,1,1,1,1,1,1,1,1,1,1,1,
1,1,1,1,1,1,1,1,1,1,1,1,1,1,1,1,1,1,1,1,1,1,1,1,1,1,1,1,1,1,1,1,1,1,1,1,
1,1,1,1,1,1,1,1,1,1,1,1,1,1,1,1,1,1,1,1,1,1,1,1,1,1,1,1,1,1,1,1,1,1,1,1,
1,1,1,1,1,1,1,1,1,1,1,1,1,1,1,1,1,1,1,1,1,1,1,1,1,1,1,1,1,1,1,1,1,1,1,1,
1,1,1,1,1,1,1,1,1,1,1,1,1,1,1,1,1,1,1,1,1,1,1,1,1,1,1,1,1,1,1,1,1,1,1,1,
1,1,1,1,1,1,1,1,1,1,1,1,1,1,1,1,1,1,1,1,1,1,1,1,1,1,1,1,1,1,1,1,1,1,1,1,
1,1,1,1,1,1,1,1,1,1,1,1,1,1,1,1,1,1,1,1,1,1,1,1,1,1,1,1,1,1,1,1,1,1,1,1,
1,1,1,1,1,1,1,1,1,1,1,1,1,1,1,1,1,1,1,1,1,1,1,1,1,1,1,1,1,1,1,1,1,1,1,1,
1,1,1,1,1,1,1,1,1,1,1,1,1,1,1,1,1,1,1,1,1,1,1,1,1,1,1,1,1,1,1,1,1,1,1,1,
1,1,1,1,1,1,1,1,1,1,1,1,1,1,1,1,1,1,1,1,1,1,1,1,1,1,1,1,1,1,1,1,1,1,1,1,
1,1,1,1,1,1,1,1,1,1,1,1,1,1,1,1,1,1,1,1,1,1,1,1,1,1,1,1,1,1,1,1,1,1,1,1,
1,1,1,1,1,1,1,1,1,1,1,1,1,1,1,1,1,1,1,1,1,1,1,1,1,1,1,1,1,1,1,1,1,1,1,1,
1,1,1,1,1,1,1,1,1,1,1,1,1,1,1,1,1,1,1,1,1,1,1,1,1,1,1,1,1,1,1,1,1,1,1,1,
1,1,1,1,1,1,1,1,1,1,1,1,1,1,1,1,1,1,1,1,1,1,1,1,1,1,1,1,1,1,1,1,1,1,1,1,
1,1,1,1,1,1,1,1,1,1,1,1,1,1,1,1,1,1,1,1,1,1,1,1,1,1,1,1,1,1,1,1,1,1,1,1,
1,1,1,1,1,1,1,1,1,1,1,1,1,1,1,1,1,1,1,1,1,1,1,1,1,1,1,1,1,1,1,1,1,1,1,1,
1,1,1,1,1,1,1,1,1,1,1,1,1,1,1,1,1,1,1,1,1,1,1,1,1,1,1,1,1,1,1,1,1,1,1,1,
1,1,1,1,1,1,1,1,1,1,1,1,1,1,1,1,1,1,1,1,1,1,1,1,1,1,1,1,1,1,1,1,1,1,1,1,
1,1,1,1,1,1,1,1,1,1,1,1,1,1,1,1,1,1,1,1,1,1,1,1,1,1,1,1,1,1,1,1,1,1,1,1,
1,1,1,1,1,1,1,1,1,1,1,1,1,1,1,1,1,1,1,1,1,1,1,1,1,1,1,1,1,1,1,1,1,1,1,1,
1,1,1,1,1,1,1,1,1,1,1,1,1,1,1,1,1,1,1,1,1,1,1,1,1,1,1,1,1,1,1,1,1,1,1,1,
1,1,1,1,1,1,1,1,1,1,1,1,1,1,1,1,1,1,1,1,1,1,1,1,1,1,1,1,1,1,1,1,1,1,1,1,
1,1,1,1,1,1,1,1,1,1,1,1,1,1,1,1,1,1,1,1,1,1,1,1,1,1,1,1,1,1,1,1,1,1,1,1,
1,1,1,1,1,1,1,1,1,1,1,1,1,1,1,1,1,1,1,1,1,1,1,1,1,1,1,1,1,1,1,1,1,1,1,1,
1,1,1,1,1,1,1,1,1,1,1,1,1,1,1,1,1,1,1,1,1,1,1,1,1,1,1,1,1,1,1,1,1,1,1,1,
1,1,1,1,1,1,1,1,1,1,1,1,1,1,1,1,1,1,1,1,1,1,1,1,1,1,1,1,1,1,1,1,1,1,1,1,
1,1,1,1,1,1,1,1,1,1,1,1,1,1,1,1,1,1,1,1,1,1,1,1,1,1,1,1,1,1,1,1,1,1,1,1,
1,1,1,1,1,1,1,1,1,1,1,1,1,1,1,1,1,1,1,1,1,1,1,1,1,1,1,1,1,1,1,1,1,1,1,1,
1,1,1,1,1,1,1,1,1,1,1,1,1,1,1,1,1,1,1,1,1,1,1,1,1,1,1,1,1,1,1,1,1,1,1,1,
1,1,1,1,1,1,1,1,1,1,1,1,1,1,1,1,1,1,1,1,1,1,1,1,1,1,1,1,1,1,1,1,1,1,1,1,
1,1,1,1,1,1,1,1,1,1,1,1,1,1,1,1,1,1,1,1,1,1,1,1,1,1,1,1,1,1,1,1,1,1,1,1,
1,1,1,1,1,1,1,1,1,1,1,1,1,1,1,1,1,1,1,1,1,1,1,1,1,1,1,1,1,1,1,1,1,1,1,1,
1,1,1,1,1,1,1,1,1,1,1,1,1,1,1,1,1,1,1,1,1,1,1,1,1,1,1,1,1,1,1,1,1,1,1,1,
1,1,1,1,1,1,1,1,1,1,1,1,1,1,1,1,1,1,1,1,1,1,1,1,1,1,1,1,1,1,1,1,1,1,1,1,
1,1,1,1,1,1,1,1,1,1,1,1,1,1,1,1,1,1,1,1,1,1,1,1,1,1,1,1,1,1,1,1,1,1,1,1,
1,1,1,1,1,1,1,1,1,1,1,1,1,1,1,1,1,1,1,1,1,1,1,1,1,1,1,1,1,1,1,1,1,1,1,1,
1,1,1,1,1,1,1,1,1,1,1,1,1,1,1,1,1,1,1,1,1,1,1,1,1,1,1,1,1,1,1,1,1,1,1,1,
1,1,1,1,1,1,1,1,1,1,1,1,1,1,1,1,1,1,1,1,1,1,1,1,1,1,1,1,1,1,1,1,1,1,1,1,
1,1,1,1,1,1,1,1,1,1,1,1,1,1,1,1,1,1,1,1,1,1,1,1,1,1,1,1,1,1,1,1,1,1,1,1,
1,1,1,1,1,1,1,1,1,1,1,1,1,1,1,1,1,1,1,1,1,1,1,1,1,1,1,1,1,1,1,1,1,1,1,1,
1,1,1,1,1,1,1,1,1,1,1,1,1,1,1,1,1,1,1,1,1,1,1,1,1,1,1,1,1,1,1,1,1,1,1,1,
1,1,1,1,1,1,1,1,1,1,1,1,1,1,1,1,1,1,1,1,1,1,1,1,1,1,1,1,1,1,1,1,1,1,1,1,
1,1,1,1,1,1,1,1,1,1,1,1,1,1,1,1,1,1,1,1,1,1,1,1,1,1,1,1,1,1,1,1,1,1,1,1,
1,1,1,1,1,1,1,1,1,1,1,1,1,1,1,1,1,1,1,1,1,1,1,1,1,1,1,1,1,1,1,1,1,1,1,1,
1,1,1,1,1,1,1,1,1,1,1,1,1,1,1,1,1,1,1,1,1,1,1,1,1,1,1,1,1,1,1,1,1,1,1,1,
1,1,1,1,1,1,1,1,1,1,1,1,1,1,1,1,1,1,1,1,1,1,1,1,1,1,1,1,1,1,1,1,1,1,1,1,
1,1,1,1,1,1,1,1,1,1,1,1,1,1,1,1,1,1,1,1,1,1,1,1,1,1,1,1,1,1,1,1,1,1,1,1,
1,1,1,1,1,1,1,1,1,1,1,1,1,1,1,1,1,1,1,1,1,1,1,1,1,1,1,1,1,1,1,1,1,1,1,1,
1,1,1,1,1,1,1,1,1,1,1,1,1,1,1,1,1,1,1,1,1,1,1,1,1,1,1,1,1,1,1,1,1,1,1,1,
1,1,1,1,1,1,1,1,1,1,1,1,1,1,1,1,1,1,1,1,1,1,1,1,1,1,1,1,1,1,1,1,1,1,1,1,
1,1,1,1,1,1,1,1,1,1,1,1,1,1,1,1,1,1,1,1,1,1,1,1,1,1,1,1,1,1,1,1,1,1,1,1,
1,1,1,1,1,1,1,1,1,1,1,1,1,1,1,1,1,1,1,1,1,1,1,1,1,1,1,1,1,1,1,1,1,1,1,1,
1,1,1,1,4),(2,2),(0.,0.869746702321014,1.7394931589914,2.60923976624962,
3.47983908319159,4.35043840179749,5.22018503077054,6.08993165951504,6.95967828799171,
7.82942491616733,8.69917154401062,9.56891817149224,10.4395174886835,11.3101168056706,
12.179863432132,13.049610058144,13.9193566836854,14.7891033087372,15.6588499332817,
16.5285965573034,17.3991958717975,18.2697951860185,18.7046684974166,19.1395418086746,
19.5744151197912,20.0092884307654,20.4441617415962,20.8790350522825,21.7487816732187,
22.1836549834672,22.6185282935685,23.0534016035221,23.4882749133276,23.9231482229848,
24.3588742245859,24.794600226187,25.2294735355468,26.0992201538203,26.5340934627341,
26.9689667714994,27.4038400801166,27.838713388586,28.2735866969081,28.7084600050832,
29.143333313112,29.5782066209952,30.0130799287334,30.4479532363275,30.8828265437783,
31.3185525442794,31.7542785447804,32.1891518519474,32.6240251589741,33.0588984658616,
33.4937717726112,33.928645079224,34.3635183857014,34.7983916920448,35.2332649982556,
35.6681383043353,36.1030116102854,36.5378849161076,36.9727582218035,37.4076315273749,
37.8425048328235,38.2782308323341,38.7139568318446,39.1488301370532,39.5837034421446,
40.0185767471208,40.4534500519838,40.8883233567357,41.3231966613787,41.7580699659148,
42.1929432703463,42.6278165746754,43.0626898789044,43.4975631830356,43.9324364870714,
44.3673097910142,44.8021830948664,45.2379090935952,45.673635092324,46.1085083960024,
46.5433816995978,46.9782550031127,47.4131283065497,47.8480016099115,48.2828749132006,
48.7177482164198,49.1526215195718,49.5874948226593,50.0223681256851,50.457241428652,
50.8921147315628,51.3269880344203,51.7618613372274,52.197587335454,52.6333133336805,
53.0681866363954,53.5030599390685,53.9379332417027,54.3728065443011,54.8076798468664,
55.2425531494018,55.6774264519101,56.1122997543943,56.5471730568575,56.9820463593026,
57.4169196617326,57.8517929641506,58.2866662665595,58.7215395689624,59.157265567009,
59.5929915650557,60.0278648674556,60.4627381698584,60.8976114722673,61.3324847746853,
61.7673580771153,62.2022313795604,62.6371046820236,63.0719779845079,63.5068512870162,
63.9417245895516,64.376597892117,64.8114711947155,65.2463444973499,65.6812178000231,
66.1169437982275,66.5526697964318,66.9875430991915,67.4224164019987,67.8572897048563,
68.2921630077673,68.7270363107343,69.1619096137603,69.5967829168479,70.0316562200001,
70.4665295232194,70.9014028265087,71.3362761298705,71.7711494333077,72.2060227368227,
72.6408960404182,73.0766220391044,73.5123480377905,73.9472213415547,74.382094645407,
74.8169679493499,75.2518412533859,75.6867145575172,76.1215878617464,76.5564611660756,
76.9913344705072,77.4262077750435,77.8610810796866,78.2959543844386,78.7308276893018,
79.1657009942781,79.6005742993696,80.0363002988208,80.4720262982719,80.9068996035997,
81.3417729090484,81.7766462146199,82.211519520316,82.6463928261383,83.0812661320886,
83.5161394381684,83.9510127443794,84.3858860507229,84.8207593572004,85.2556326638134,
85.6905059705631,86.1253792774507,86.5602525844776,86.995978584908,87.4317045853384,
87.8665778926469,88.3014512000977,88.7363245076919,89.1711978154302,89.6060711233134,
90.0409444313423,90.4758177395175,90.9106910478396,91.345564356309,91.7804376649263,
92.2153109736917,92.6501842826055,93.085057591668,93.5199309008791,93.9556569024059,
94.3913829039327,94.8262562134414,95.2611295230986,95.6960028329042,96.1308761428578,
96.5657494529591,97.0006227632077,97.4354960736028,97.870369384144,98.3052426948304,
98.7401160056612,99.1749893166354,99.6098626277522,100.04473593901,100.915335253024,
101.351061255639,101.785934567313,102.220807879124,102.655681191068,103.090554503145,
103.525427815353,104.395174440154,105.264921065453,105.699794378283,106.134667691232,
106.569541004295,107.004414317471,107.8750136343,108.745612951339,109.615359578629,
110.485106206296,111.354852834309,112.224599462639,113.094346091254,113.964092720119,
114.834692038763,115.705291357499,116.575037986826,117.444784616267,118.314531245777,
119.184277875311,120.054024504821,120.923771134261,121.794370453112,122.66496977189,
123.534716400968,124.404463029834,125.274209658448,126.143956286779,127.013702914792,
127.883449542458,128.754048859798,129.624648176939,130.494394803617,131.364141429857,
132.233888055637,133.103634680937,133.973381305737,134.843127930023,135.71372724472,
136.584326559147,137.019199870684,137.454073182083,137.888946493341,138.323819804458,
139.193566426263,140.063313047491,140.498186357887,140.933059668136,141.367932978237,
141.802806288191,142.237679597997,142.673405599673,143.109131601348,143.544004910857,
143.978878220217,144.413751529429,144.848624838491,145.283498147405,145.718371456171,
146.153244764789,146.588118073258,147.022991381581,147.457864689756,147.892737997785,
148.327611305669,148.762484613407,149.197357921002,149.633083921574,150.068809922147,
150.503683229455,150.938556536623,151.37342984365,151.808303150538,152.243176457288,
152.678049763901,153.112923070379,153.547796376722,153.982669682934,154.417542989014,
154.852416294964,155.287289600787,155.722162906483,156.157036212055,156.592762211626,
157.028488211198,157.463361516526,157.898234821735,158.333108126826,158.767981431803,
159.202854736666,159.637728041419,160.072601346062,160.507474650599,160.94234795503,
161.37722125936,161.812094563589,162.246967867721,162.681841171757,163.1167144757,
163.552440474473,163.988166473247,164.423039777011,164.85791308069,165.292786384286,
165.727659687801,166.162532991238,166.597406294601,167.03227959789,167.46715290111,
167.902026204262,168.33689950735,168.771772810376,169.206646113343,169.641519416254,
170.076392719112,170.512118717363,170.947844715614,171.382718018374,171.817591321089,
172.252464623762,172.687337926397,173.122211228996,173.557084531561,173.991957834097,
174.426831136606,174.86170443909,175.296577741554,175.731451044,176.16632434643,
176.601197648848,177.036070951258,177.471796949306,177.907522947355,178.342396249755,
178.777269552155,179.212142854558,179.647016156968,180.081889459386,180.516762761816,
180.951636064262,181.386509366726,181.82138266921,182.256255971719,182.691129274255,
183.12600257682,183.560875879419,183.995749182054,184.431475180237,184.867201178421,
185.302074481136,185.736947783896,186.171821086704,186.606694389561,187.041567692473,
187.47644099544,187.911314298466,188.346187601554,188.781060904706,189.215934207926,
189.650807511215,190.085680814577,190.520554118015,190.95542742153,191.391153420175,
191.82687941882,192.261752722499,192.696626026263,193.131499330116,193.566372634059,
194.001245938095,194.436119242227,194.870992546456,195.305865850785,195.740739155217,
196.175612459754,196.610485764397,197.045359069149,197.480232374013,197.915105678989,
198.350831678382,198.786557677775,199.221430982984,199.656304288312,200.091177593761,
200.526050899333,200.960924205029,201.395797510852,201.830670816802,202.265544122882,
202.700417429093,203.135290735437,203.570164041915,204.005037348528,204.439910655278,
204.874783962166,205.310509962526,205.746235962887,206.181109270054,206.615982577363,
207.050855884814,207.485729192409,207.920602500147,208.355475808031,208.79034911606,
209.225222424235,209.660095732558,210.094969041027,210.529842349645,210.96471565841,
211.399588967324,211.834462276387,212.27018827784,212.705914279292,213.140787588653,
213.575660898161,214.010534207819,214.880280827579,215.31515413768,215.750027447929,
216.184900758324,216.619774068866,217.054647379553,217.489520690384,218.359267312475,
219.22986662628,219.665592628826,220.100465940363,220.535339252038,220.970212563848,
221.83995918787,222.709705812416,223.579452437468,224.014325750179,224.44919906301,
225.318945689022,226.189545005688,227.060144322571,227.929890949664,228.799637577146,
229.66938420499,230.539130833166,231.408877461643,232.278624090388,233.149223408954,
234.019822727623,234.889569356878,235.759315986267,236.629062615749,237.498809245277,
238.368555874806,239.238302504287,240.108901823183,240.979501142017,241.849247771189,
242.718994400167,243.588741028911,244.458487657389,245.328234285565,246.197980913409,
247.068580230891,247.939179548182,248.80892617507,249.678672801532,250.548419427545,
251.418166053087,252.287912678139,253.157659302684,254.028258617581,254.898857932211,
255.333731243885,255.768604555423,256.203477866821,256.63835117808,257.508097800171,
258.377844421689,258.812717732231,259.247591042627,259.682464352876,260.117337662977,
260.552210972931,260.987936974682,261.858536286089,262.293409595598,262.728282904958,
263.16315621417,263.598029523233,264.032902832147,264.467776140913,264.902649449531,
265.337522758001,265.772396066323,266.207269374499,266.642142682528,267.077015990412,
267.511889298151,267.947615298795,268.383341299439,268.81821460689,269.2530879142,
269.687961221367,270.122834528394,270.557707835282,270.992581142032,271.427454448646,
271.862327755124,272.297201061468,272.732074367679,273.166947673759,273.60182097971,
274.036694285533,274.471567591229,274.907293590862,275.343019590495,275.777892895944,
276.212766201272,276.647639506481,277.082512811573,277.51738611655,277.952259421414,
278.387132726166,278.82200603081,279.256879335346,279.691752639779,280.126625944108,
280.561499248338,280.996372552469,281.431245856506,281.866971855324,282.302697854143,
282.737571157996,283.172444461761,283.60731776544,284.042191069036,284.477064372551,
284.911937675989,285.346810979351,285.781684282641,286.216557585861,286.651430889013,
287.086304192101,287.521177495128,287.956050798095,288.390924101007,288.826650099283,
289.262376097559,289.697249400366,290.132122703127,290.566996005842,291.001869308516,
291.43674261115,291.871615913749,292.306489216315,292.741362518851,293.17623582136,
293.611109123845,294.045982426308,294.480855728754,294.915729031185,295.350602333603,
295.786328331655,296.222054329707,296.65692763211,297.091800934511,297.526674236911,
297.961547539314,298.396420841724,298.831294144142,299.266167446573,299.701040749018,
300.135914051482,300.570787353967,301.005660656476,301.440533959012,301.875407261578,
302.310280564177,302.746006562341,303.181732560506,303.616605863179,304.051479165895,
304.486352468655,304.921225771462,305.35609907432,305.790972377232,306.225845680199,
306.660718983226,307.095592286314,307.530465589466,307.965338892686,308.400212195976,
308.835085499338,309.269958802776,309.705684801381,310.141410799985,310.576284103581,
311.01115740726,311.446030711025,311.880904014878,312.315777318821,312.750650622858,
313.185523926989,313.620397231219,314.055270535549,314.490143839981,314.925017144517,
315.359890449161,315.794763753913,316.229637058777,316.665363058112,317.101089057448,
317.53596236254,317.970835667749,318.405708973077,318.840582278526,319.275455584098,
319.710328889795,320.145202195618,320.580075501568,321.014948807648,321.44982211386,
321.884695420204,322.319568726682,322.754442033295,323.189315340045,323.625041340336,
324.060767340628,324.495640647655,324.930513954822,325.365387262131,325.800260569583,
326.235133877177,326.670007184916,327.1048804928,327.539753800829,327.974627109005,
328.409500417327,328.844373725797,329.279247034415,329.714120343181,330.148993652095,
330.584719653474,331.020445654852,331.455318964064,331.890192273424,332.325065582933,
332.759938892591,333.194812202397,333.629685512351,334.064558822453,334.499432132702,
334.934305443098,335.369178753639,335.804052064326,336.673798686132,337.108671997249,
337.544397999725,337.980124002201,338.4149973136,338.849870625137,339.284743936812,
340.154490560568,341.024237184854,341.459110497191,341.893983809655,342.328857122244,
342.763730434955,343.633477060735,344.504076377234,345.374675693955,346.244422320844,
347.114168948136,347.983915575803,348.853662203817,349.723408832148,350.593155460764,
351.463754779246,352.334354097839,353.204100727012,354.07384735634,354.943593985781,
355.813340615292,356.683087244827,357.552833874338,358.423433193272,359.294032512154,
360.163779141409,361.033525770489,361.903272399355,362.77301902797,363.642765656301,
364.512512284316,365.383111601936,366.253710919371,367.123457546465,367.993204173143,
368.862950799383,369.732697425164,370.602444050463,371.472190675265,372.342789990359,
373.21338930519,373.648262617,374.083135928675,374.952882551611,375.822629173987,
376.257502484962,376.692375795793,377.12724910648,377.562122417021,377.996995727417,
378.431869037666,378.866742347767,379.302468349591,379.738194351416,380.173067661222,
380.607940970879,381.042814280388,381.477687589749,381.91256089896,382.347434208023,
382.782307516937,383.217180825703,383.652054134321,384.086927442791,384.521800751113,
384.956674059289,385.391547367318,385.826420675202,386.262146675918,386.697872676635,
387.13274598423,387.567619291681,388.00249259899,388.437365906157,388.872239213185,
389.307112520073,389.741985826823,390.176859133436,390.611732439914,391.046605746258,
391.48147905247,391.91635235855,392.351225664501,392.786098970323,393.221824970019,
393.657550969714,394.092424275286,394.527297580735,394.962170886063,395.397044191272,
395.831917496364,396.266790801341,396.701664106204,397.136537410957,397.5714107156,
398.006284020137,398.441157324569,398.876030628899,399.310903933128,399.74577723726,
400.181503236126,400.617229234991,401.052102538934,401.486975842787,401.921849146551,
402.356722450231,402.791595753827,403.226469057342,403.66134236078,404.096215664142,
404.531088967432,404.965962270651,405.400835573804,405.835708876892,406.270582179918,
406.705455482886,407.141181481189,407.576907479491,408.01178078235,408.446654085157,
408.881527387917,409.316400690633,409.751273993306,410.186147295941,410.62102059854,
411.055893901106,411.490767203642,411.925640506151,412.360513808636,412.795387111099,
413.230260413545,413.665133715976,414.100859714032,414.536585712088,414.971459014498,
415.406332316901,415.841205619301,416.276078921702,416.710952224105,417.145825526515,
417.580698828933,418.015572131364,418.45044543381,418.885318736273,419.320192038758,
419.755065341267,420.189938643803,420.624811946369,421.060537944515,421.496263942662,
421.931137245297,422.36601054797,422.800883850686,423.235757153446,423.670630456253,
424.105503759112,424.540377062023,424.975250364991,425.410123668017,425.844996971105,
426.279870274258,426.714743577477,427.149616880767,427.584490184129,428.020216182695,
428.455942181261,428.890815484776,429.325688788373,429.760562092052,430.195435395816,
430.630308699669,431.065182003612,431.500055307649,431.93492861178,432.36980191601,
432.80467522034,433.239548524772,433.674421829309,434.109295133952,434.544168438705,
434.979894437984,435.415620437262,435.850493742239,436.285367047331,436.72024035254,
437.155113657869,437.589986963318,438.024860268889,438.459733574586,438.894606880409,
439.32948018636,439.76435349244,440.199226798651,440.634100104995,441.068973411473,
441.503846718087,441.939572718309,442.375298718531,442.810172025419,443.245045332447,
443.679918639614,444.114791946923,444.549665254374,444.984538561969,445.419411869708,
445.854285177591,446.289158485621,446.724031793796,447.158905102119,447.593778410589,
448.028651719207,448.463525027973,448.899251029277,449.334977030581,449.769850339644,
450.639596958216,451.074470267725,451.509343577383,451.944216887189,452.379090197143,
452.813963507244,453.248836817493,453.683710127889,454.118583438431,454.553456749117,
454.988330059949,455.423203370923,455.858929373329,456.294655375734,456.729528686993,
457.164401998391,457.599275309929,458.469021933414,458.90389524536,459.338768557437,
459.773641869646,460.208515181983,460.643388494447,461.078261807036,461.948008432578,
462.818607748906,463.689207065461,464.55895369214,465.428700319234,466.298446946716,
467.16819357456,468.037940202737,468.907686831215,469.778286149605,470.648885468116,
471.518632097196,472.388378726451,473.258125355841,474.127871985322,474.997618614851,
475.86736524438,476.737964563343,477.608563882265,478.478310511593,479.348057140765,
480.217803769743,481.087550398488,481.957297026966,482.827043655142,483.697642972895,
484.568242290469,485.43798891776,486.307735544649,487.177482171112,488.047228797125,
488.916975422667,489.78672204772,490.657321363009,491.09304736596,491.527920678038,
492.397667301793,493.267413925005,494.137160547663,494.57203385878,495.006907169755,
495.441780480586,495.876653791273,496.311527101814,496.74640041221,497.616999724357,
498.052725726255,498.487599036209,498.922472346015,499.357345655673,499.792218965182,
500.227092274542,500.661965583754,501.096838892816,501.531712201731,501.966585510497,
502.401458819114,502.836332127584,503.271205435907,503.706078744082,504.140952052112,
504.576678052901,505.01240405369,505.447277361429,505.882150669023,506.317023976474,
506.751897283783,507.186770590951,507.621643897978,508.056517204866,508.491390511616,
508.92626381823,509.361137124708,509.796010431052,510.230883737263,510.665757043344,
511.100630349294,511.536356349053,511.972082348811,512.406955654506,512.841828960076,
513.276702265523,513.711575570849,514.146448876056,514.581322181146,515.016195486121,
515.451068790983,515.885942095733,516.320815400375,516.75568870491,517.19056200934,
517.625435313668,518.060308617896,518.496034616807,518.931760615718,519.366633919752,
519.801507223694,520.236380527545,520.671253831307,521.106127134985,521.541000438579,
521.975873742092,522.410747045528,522.845620348888,523.280493652176,523.715366955394,
524.150240258545,524.585113561631,525.019986864656,525.455712862985,525.891438861313,
526.326312164223,526.761185467079,527.196058769885,527.630932072643,528.065805375356,
528.500678678029,528.935551980661,529.370425283258,529.805298585822,530.240171888356,
530.675045190863,531.109918493346,531.544791795808,531.979665098252,532.415391096312,
532.851117094373,533.285990396789,533.720863699197,534.155737001598,534.590610303997,
535.025483606395,535.460356908796,535.895230211204,536.330103513621,536.764976816049,
537.199850118493,537.634723420955,538.069596723438,538.504470025945,538.93934332848,
539.375069326608,539.810795324736,540.245668627333,540.680541929966,541.115415232637,
541.550288535351,541.985161838109,542.420035140915,542.854908443771,543.28978174668,
543.724655049646,544.15952835267,544.594401655757,545.029274958907,545.464148262125,
545.899021565413,546.334747563939,546.770473562465,547.205346865901,547.640220169415,
548.075093473009,548.509966776686,548.944840080449,549.3797133843,549.814586688241,
550.249459992276,550.684333296405,551.119206600633,551.554079904961,551.988953209391,
552.423826513926,552.858699818567,553.294425817789,553.73015181701,554.165025121872,
554.599898426846,555.034771731937,555.469645037144,555.90451834247,556.339391647917,
556.774264953487,557.209138259182,557.644011565003,558.078884870951,558.51375817703,
558.948631483239,559.383504789581,559.818378096058,560.254104096209,560.689830096361,
561.12470340311,561.559576709996,561.994450017021,562.429323324187,562.864196631494,
563.299069938943,563.733943246536,564.168816554273,564.603689862154,565.038563170182,
565.473436478355,565.908309786676,566.343183095144,566.77805640376,567.213782404988,
567.649508406216,568.084381715128,568.519255024189,568.954128333399,569.389001642757,
569.823874952264,570.258748261921,570.693621571725,571.128494881677,571.563368191777,
572.433114812417,572.867988122957,573.302861433642,573.737734744471,574.173460746804,
574.609186749136,575.044060060251,575.913806682904,576.783553306113,577.218426617922,
577.653299929865,578.08817324194,578.523046554147,579.392793178944,580.26253980424,
581.13313912039,581.568865123709,582.003738436771,582.87348506323,583.743231690115,
584.612978317402,585.482724945065,586.352471573076,587.222218201403,588.092817519691,
588.963416838109,589.833163467083,590.702910096251,591.572656725575,592.442403355013,
593.31214998452,594.181896614051,595.05249593303,595.92309525198,596.792841881366,
597.662588510618,598.532335139693,599.402081768556,600.271828397167,601.141575025495,
602.012174343369,602.882773661074,603.752520288553,604.622266915642,605.492013542317,
606.361760168553,607.23150679433,608.101253419626,608.971852735101,609.842452050322,
610.71219867434,611.581945297822,612.451691920754,612.886565232011,613.321438543126,
613.756311854099,614.191185164928,615.060931786153,615.931531098516,616.367257100486,
616.802130410586,617.237003720538,617.671877030342,618.106750339998,618.541623649505,
618.976496958863,619.411370268073,619.846243577134,620.281116886046,620.71599019481,
621.150863503426,621.585736811894,622.020610120214,622.455483428388,622.891209429248,
623.326935430108,623.761808737989,624.196682045726,624.631555353319,625.066428660769,
625.501301968075,625.936175275241,626.371048582266,626.805921889153,627.240795195901,
627.675668502512,628.110541808988,628.54541511533,628.98028842154,629.415161727618,
629.850887727438,630.286613727259,630.72148703308,631.156360338774,631.591233644344,
632.026106949791,632.460980255118,632.895853560325,633.330726865415,633.76560017039,
634.200473475251,634.635346780002,635.070220084644,635.505093389179,635.939966693609,
636.374839997937,636.810565996897,637.246291995857,637.681165299986,638.116038604021,
638.550911907962,638.985785211813,639.420658515576,639.855531819253,640.290405122847,
640.725278426361,641.160151729796,641.595025033157,642.029898336444,642.464771639662,
642.899644942813,643.334518245899,643.770244244257,644.205970242616,644.640843545581,
645.075716848491,645.510590151347,645.945463454153,646.380336756911,646.815210059625,
647.250083362296,647.684956664929,648.119829967526,648.55470327009,648.989576572624,
649.424449875131,649.859323177614,650.294196480076,650.729922478144,651.165648476212,
651.600521778641,652.035395081057,652.470268383465,652.905141685866,653.340014988265,
653.774888290663,654.209761593065,654.644634895472,655.079508197889,655.514381500318,
655.949254802762,656.384128105224,656.819001407706,657.253874710213,657.689600708326,
658.12532670644,658.560200009004,658.995073311601,659.429946614234,659.864819916905,
660.299693219619,660.734566522377,661.169439825183,661.604313128039,662.039186430948,
662.474059733914,662.908933036938,663.343806340025,663.778679643175,664.213552946393,
664.649278944883,665.085004943373,665.519878246733,665.954751550169,666.389624853683,
666.824498157277,667.259371460954,667.694244764717,668.129118068568,668.563991372509,
668.998864676544,669.433737980674,669.868611284901,670.303484589229,670.738357893659,
671.173231198194,671.608957197361,672.044683196528,672.479556501278,672.91442980614,
673.349303111115,673.784176416205,674.219049721412,674.653923026738,675.088796332185,
675.523669637755,675.95854294345,676.393416249271,676.82828955522,677.263162861298,
677.698036167508,678.13290947385,678.568635473934,679.004361474018,679.439234780629,
679.874108087377,680.308981394264,680.743854701289,681.178728008455,681.613601315762,
682.048474623211,682.483347930804,682.91822123854,683.353094546422,683.78796785445,
684.222841162623,684.657714470944,685.092587779412,685.528313780566,685.96403978172,
686.398913090483,686.833786399396,687.268659708457,687.703533017666,688.138406327025,
688.573279636532,689.008152946187,689.443026255992,689.877899565944,690.312772876043,
690.74764618629,691.182519496684,691.617392807224,692.052266117909,692.487992120169,
692.92371812243,693.358591433403,694.228338055774,694.663211367171,695.098084678707,
695.532957990379,695.967831302188,696.402704614131,696.837577926207,697.707324550749,
698.577071175797,699.011944488507,699.447670491767,699.883396495028,700.318269807975,
701.188016434211,702.057763060886,702.927509687976,703.797256315454,704.667002943295,
705.536749571467,706.407348889651,707.277948207973,708.147694836835,709.017441465911,
709.887188095163,710.756934724548,711.626681354026,712.496427983551,713.367027302543,
714.237626621516,715.107373250954,715.977119880277,716.846866509446,717.716613138419,
718.586359767161,719.456106395635,720.32670571363,721.197305031464,722.067051659126,
722.936798286414,723.806544913299,724.676291539758,725.546038165767,726.415784791305,
727.286384106969,728.156983422381,729.026730046663,729.896476670415,730.331349982088,
730.766223293624,731.201096605021,731.635969916278,732.505716538366,733.37546315988,
733.81033647042,734.246062472462,734.681788474505,735.116661784752,735.551535094852,
735.986408404804,736.421281714608,736.856155024264,737.291028333771,737.72590164313,
738.160774952339,738.5956482614,739.030521570312,739.465394879076,739.900268187692,
740.33514149616,740.77001480448,741.205740805414,741.641466806347,742.076340114374,
742.511213422256,742.946086729993,743.380960037585,743.815833345035,744.250706652341,
744.685579959507,745.120453266533,745.555326573419,745.990199880167,746.425073186778,
746.859946493254,747.294819799596,747.729693105806,748.165419105691,748.601145105576,
749.036018411525,749.470891717346,749.90576502304,750.34063832861,750.775511634057,
751.210384939384,751.645258244591,752.080131549682,752.515004854656,752.949878159518,
753.384751464269,753.81962476891,754.254498073445,754.689371377875,755.125097376885,
755.560823375895,755.995696680123,756.430569984253,756.865443288287,757.300316592228,
757.735189896079,758.170063199842,758.604936503519,759.039809807113,759.474683110627,
759.909556414062,760.344429717423,760.779303020711,761.214176323929,761.649049627079,
762.084775625469,762.520501623858,762.955374926883,763.390248229848,763.825121532758,
764.259994835614,764.694868138419,765.129741441178,765.564614743891,765.999488046563,
766.434361349196,766.869234651793,767.304107954357,767.738981256891,768.173854559398,
768.608727861881,769.044453859958,769.480179858035,769.915053160479,770.349926462907,
770.784799765324,771.219673067731,771.654546370133,772.089419672531,772.52429297493,
772.959166277331,773.394039579739,773.828912882155,774.263786184584,774.698659487028,
775.13353278949,775.568406091973,776.004132090072,776.439858088172,776.874731390706,
777.30960469327,777.744477995867,778.1793512985,778.614224601171,779.049097903885,
779.483971206643,779.918844509449,780.353717812305,780.788591115215,781.22346441818,
781.658337721205,782.093211024291,782.528084327442,782.963810325897,783.399536324352,
783.834409627639,784.269282931,784.704156234435,785.139029537949,785.573902841543,
786.00877614522,786.443649448983,786.878522752834,787.313396056775,787.74826936081,
788.183142664939,788.618015969167,789.052889273495,789.487762577925,789.923488577038,
790.359214576152,790.794087880793,791.228961185544,791.663834490406,792.098707795381,
792.533581100471,792.968454405678,793.403327711004,793.838201016451,794.273074322021,
794.707947627716,795.142820933537,795.577694239486,796.012567545564,796.447440851774,
796.883166851791,797.318892851808,797.753766158284,798.188639464895,798.623512771643,
799.058386078529,799.493259385555,799.92813269272,800.363006000027,800.797879307477,
801.232752615069,801.667625922806,802.102499230688,802.537372538715,802.972245846889,
803.40711915521,803.84284515629,804.27857115737,804.713444465985,805.148317774749,
805.583191083662,806.018064392723,806.452937701933,806.887811011291,807.322684320798,
808.192430940258,808.62730425021,809.06217756031,809.497050870557,809.931924180951,
810.36679749149,810.802523493679,811.238249495867,811.673122806697,812.542869428785,
812.977742740041,813.412616051438,813.847489362974,814.282362674646,814.717235986455,
815.152109298398,816.021855922681,816.891602547478,817.326475860065,817.762201863265,
818.197927866466,818.632801179295,819.502547805304,820.372294431763,821.242041058648,
822.111787685935,822.981534313598,823.851280941609,824.721880259681,825.5924795779,
826.462226206642,827.331972835616,828.201719464785,829.071466094109,829.941212723546,
830.810959353053,831.681558672047,832.552157991036,833.421904620514,834.2916512499,
835.161397879151,836.031144508226,836.900891137089,837.770637765701,838.641237083811,
839.511836401767,840.381583029608,841.251329657086,842.121076284176,842.990822910851,
843.860569537087,844.730316162863,845.600915478712,846.471514794314,847.341261418855,
848.211008042874,848.645881354683,849.080754666356,849.515627977891,849.950501289288,
850.82024791166,851.689994533462,852.124867844147,852.560593846263,852.996319848379,
853.431193158772,853.866066469019,854.300939779119,855.170686398875,855.605559708531,
856.040433018038,856.475306327397,856.910179636606,857.345052945667,857.77992625458,
858.214799563344,858.64967287196,859.084546180427,859.520272181434,859.95599818244,
860.390871490614,860.825744798641,861.260618106523,861.69549141426,862.130364721852,
862.565238029302,863.000111336609,863.434984643774,863.8698579508,864.304731257686,
864.739604564434,865.174477871045,865.609351177521,866.044224483863,866.479950483814,
866.915676483765,867.350549789843,867.785423095792,868.220296401613,868.655169707307,
869.090043012877,869.524916318325,869.959789623651,870.394662928858,870.829536233948,
871.264409538923,871.699282843785,872.134156148535,872.569029453177,873.003902757712,
873.439628756773,873.875354755834,874.310228060162,874.745101364389,875.179974668519,
875.614847972553,876.049721276495,876.484594580346,876.919467884108,877.354341187786,
877.78921449138,878.224087794893,878.658961098329,879.093834401689,879.528707704977,
879.963581008195,880.399307006616,880.835033005038,881.269906308124,881.704779611148,
882.139652914114,882.574526217024,883.00939951988,883.444272822685,883.879146125444,
884.314019428157,884.748892730829,885.183766033462,885.618639336059,886.053512638623,
886.488385941157,886.923259243664,887.358985241751,887.794711239839,888.2295845423,
888.664457844744,889.099331147173,889.534204449589,889.969077751997,890.403951054398,
890.838824356797,891.273697659195,891.708570961597,892.143444264004,892.578317566421,
893.01319086885,893.448064171293,893.882937473755,894.318663471843,894.75438946993,
895.189262772437,895.624136074971,896.059009377535,896.493882680132,896.928755982765,
897.363629285437,897.798502588151,898.233375890909,898.668249193715,899.103122496571,
899.53799579948,899.972869102446,900.40774240547,900.842615708556,901.278341706978,
901.714067705399,902.148941008617,902.583814311905,903.018687615265,903.453560918701,
903.888434222214,904.323307525808,904.758180829485,905.193054133248,905.627927437099,
906.06280074104,906.497674045075,906.932547349205,907.367420653433,907.80229395776,
908.238019956821,908.673745955883,909.108619260417,909.543492565059,909.978365869809,
910.413239174671,910.848112479646,911.282985784736,911.717859089943,912.152732395269,
912.587605700716,913.022479006287,913.457352311981,913.892225617802,914.327098923751,
914.761972229829,915.19769822978,915.633424229731,916.068297536072,916.503170842548,
916.93804414916,917.372917455908,917.807790762794,918.24266406982,918.677537376985,
919.112410684292,919.547283991742,919.982157299334,920.417030607071,920.851903914953,
921.28677722298,921.721650531154,922.15737653216,922.593102533167,923.027975841635,
923.46284915025,923.897722459014,924.332595767926,924.767469076987,925.202342386197,
925.637215695556,926.072089005063,926.506962314719,926.941835624523,927.376708934475,
927.811582244575,928.246455554822,928.681328865215,929.117054867331,929.987654180132,
930.422527490961,930.857400801934,931.292274113049,931.727147424306,932.162020735703,
932.596894047238,933.46664067072,934.336387294739,934.771260606945,935.20613391928,
935.641007231742,936.076733234882,936.94733255073,937.817079176507,938.686825802743,
939.556572429418,940.426319056508,941.296065683986,942.165812311827,943.036411629783,
943.907010947893,944.776757576505,945.646504205367,946.516250834443,947.385997463694,
948.25574409308,949.125490722558,949.996090041546,950.86668936054,951.736435990048,
952.606182619485,953.475929248809,954.345675877978,955.215422506951,956.085169135693,
956.955768453912,957.826367771985,958.696114399995,959.565861027658,960.435607654946,
961.305354281831,962.175100908289,963.044847534298,963.915446850328,964.786046166116,
965.655792790913,966.525539415195,966.960412727138,967.395286038947,968.265032662155,
969.134779284809,969.569652595924,970.004525906897,970.439399217726,970.875125219914,
971.310851222103,971.745724532643,972.615471153283,973.485217773335,973.920091083139,
974.354964392795,974.789837702302,975.22471101166,975.65958432087,976.094457629931,
976.529330938844,976.964204247608,977.399077556223,977.834803557303,978.270529558383,
978.705402866704,979.140276174877,979.575149482905,980.010022790786,980.444896098523,
980.879769406116,981.314642713565,981.749516020872,982.184389328038,982.619262635063,
983.05413594195,983.489009248698,983.923882555309,984.358755861785,984.794481861802,
985.230207861819,985.665081168029,986.099954474107,986.534827780056,986.969701085877,
987.404574391571,987.839447697141,988.274321002589,988.709194307915,989.144067613122,
989.578940918212,990.013814223187,990.448687528048,990.883560832799,991.31843413744,
991.754160136554,992.189886135667,992.624759440097,993.059632744425,993.494506048653,
993.929379352783,994.364252656817,994.799125960758,995.233999264609,995.668872568372,
996.103745872049,996.538619175643,996.973492479157,997.408365782593,997.843239085953,
998.278112389241,998.713838387696,999.149564386151,999.584437689301,1000.01931099239,
1000.45418429541,1000.88905759838,1001.32393090129,1001.75880420414,1002.19367750695,
1002.62855080971,1003.06342411242,1003.49829741509,1003.93317071773,1004.36804402032,
1004.80291732289,1005.23779062542,1005.67351662352,1006.10924262162,1006.5441159241,
1006.97898922656,1007.41386252901,1007.84873583144,1008.28360913385,1008.71848243626,
1009.15335573866,1009.58822904106,1010.02310234346,1010.45797564586,1010.89284894827,
1011.32772225069,1011.76259555311,1012.19746885556,1012.63319485364,1013.06892085171,
1013.5037941542,1013.9386674567,1014.37354075924,1014.8084140618,1015.2432873644,
1015.67816066703,1016.1130339697,1016.54790727242,1016.98278057517,1017.41765387798,
1017.85252718084,1018.28740048375,1018.72227378671,1019.15714708974,1019.59287308813,
1020.02859908651,1020.46347238967,1020.89834569288,1021.33321899617,1021.76809229953,
1022.20296560297,1022.63783890648,1023.07271221007,1023.50758551375,1023.94245881752,
1024.37733212137,1024.81220542531,1025.24707872935,1025.68195203348,1026.11682533771,
1026.55255133672,1026.98827733573,1027.42315064016,1027.8580239447,1028.29289724934,
1028.72777055409,1029.16264385896,1029.59751716393,1030.03239046902,1030.46726377423,
1030.90213707956,1031.33701038501,1031.77188369058,1032.20675699628,1032.6416303021,
1033.07650360805,1033.51222960793,1033.94795560782,1034.38282891403,1034.81770222038,
1035.25257552685,1035.68744883347,1036.12232214022,1036.5571954471,1036.99206875413,
1037.4269420613,1037.86181536861,1038.29668867606,1038.73156198365,1039.16643529139,
1039.60130859927,1040.0361819073,1040.47190790824,1040.90763390917,1041.34250721749,
1041.77738052596,1042.21225383458,1042.64712714334,1043.08200045226,1043.95174707053,
1044.38662037989,1044.8214936894,1045.25636699906,1045.69124030886,1046.12611361882,
1046.56098692892,1046.99586023917,1047.43158624121,1047.86731224325,1048.3021855538,
1048.73705886448,1049.17193217531,1049.60680548629,1050.0416787974,1050.47655210866,
1050.91142542006,1051.78117204327,1052.21604535508,1052.65091866703,1053.0857919791,
1053.52066529131,1053.95553860365,1054.39126460673,1055.26186392239,1056.13161054793,
1057.00135717395,1057.43623048712,1057.87110380041,1058.7408504273,1059.61059705459,
1060.48034368225,1061.35094300009,1062.22154231809,1063.09128894656,1063.96103557531,
1064.83078220429,1065.70052883346,1066.57027546278,1067.44002209222,1068.3106214112,
1069.18122073019,1070.05096735972,1070.9207139892,1071.79046061859,1072.66020724785,
1073.52995387693,1074.39970050579,1075.27029982411,1076.1408991423,1077.01064577048,
1077.88039239832,1078.7501390258,1079.61988565289,1080.48963227957,1081.35937890581,
1082.22997822202,1083.100577538,1083.97032416305,1084.84007078759,1085.70981741161,
1086.5795640351,1087.44931065803,1087.88418396929,1088.31905728041,1088.75393059138,
1089.18965659365,1089.62538259591,1090.06025590659,1090.93000252753,1091.36487583778,
1091.79974914788,1092.23462245783,1092.66949576764,1093.1043690773,1093.5392423868,
1093.97411569616,1094.40898900538,1094.84386231444,1095.27873562335,1095.71360893212,
1096.14933493327,1096.58506093443,1097.0199342429,1097.45480755122,1097.88968085939,
1098.32455416742,1098.75942747531,1099.19430078305,1099.62917409064,1100.06404739809,
1100.4989207054,1100.93379401257,1101.36866731959,1101.80354062648,1102.23841393323,
1102.67328723984,1103.10901323993,1103.54473924001,1103.97961254636,1104.41448585257,
1104.84935915865,1105.2842324646,1105.71910577042,1106.15397907612,1106.58885238169,
1107.02372568714,1107.45859899246,1107.89347229767,1108.32834560276,1108.76321890774,
1109.1980922126,1109.63296551736,1110.06869151652,1110.50441751569,1110.93929082023,
1111.37416412466,1111.80903742899,1112.24391073322,1112.67878403735,1113.11365734139,
1113.54853064533,1113.98340394918,1114.41827725295,1114.85315055662,1115.28802386022,
1115.72289716374,1116.15777046717,1116.59264377053,1117.02836976903,1117.46409576752,
1117.89896907074,1118.33384237389,1118.76871567698,1119.20358898,1119.63846228297,
1120.07333558588,1120.50820888874,1120.94308219154,1121.3779554943,1121.81282879702,
1122.24770209969,1122.68257540233,1123.11744870492,1123.55232200749,1123.98804800561,
1124.42377400372,1124.85864730623,1125.29352060871,1125.72839391118,1126.16326721362,
1126.59814051605,1127.03301381847,1127.46788712088,1127.90276042328,1128.33763372568,
1128.77250702808,1129.20738033048,1129.64225363289,1130.07712693531,1130.51200023774,
1130.94772623581,1131.38345223388,1131.81832553634,1132.25319883883,1132.68807214134,
1133.12294544387,1133.55781874644,1133.99269204904,1134.42756535167,1134.86243865434,
1135.29731195706,1135.73218525982,1136.16705856263,1136.60193186548,1137.03680516839,
1137.47167847136,1137.90740446972,1138.34313046808,1138.77800377117,1139.21287707432,
1139.64775037754,1140.08262368083,1140.51749698419,1140.95237028763,1141.38724359114,
1141.82211689474,1142.25699019842,1142.69186350218,1143.12673680603,1143.56161010998,
1143.99648341401,1144.43135671814,1144.86708271711,1145.30280871607,1145.7376820204,
1146.17255532483,1146.60742862936,1147.04230193401,1147.47717523876,1147.91204854362,
1148.3469218486,1148.78179515369,1149.2166684589,1149.65154176423,1150.08641506968,
1150.52128837525,1150.95616168094,1151.39103498677,1151.82676098659,1152.26248698641,
1152.69736029249,1153.1322335987,1153.56710690504,1154.00198021152,1154.43685351813,
1154.87172682488,1155.30660013177,1155.7414734388,1156.17634674597,1156.61122005327,
1157.04609336073,1157.48096666832,1157.91583997606,1158.35071328394,1158.7864392848,
1159.22216528566,1159.65703859384,1160.09191190216,1160.52678521063,1160.96165851925,
1161.39653182801,1161.83140513693,1162.26627844599,1162.7011517552,1163.13602506456,
1163.57089837407,1164.00577168373,1164.44064499353,1164.87551830349,1165.74611761556,
1166.18184361753,1166.61671692792,1167.05159023846,1167.48646354915,1167.92133685998,
1168.35621017096,1169.22595679333,1170.09570341627,1170.53057672794,1170.96545003975,
1171.4003233517,1171.83519666377,1172.27006997598,1172.705795979,1173.57639529447,
1174.44614191977,1174.8810152326,1175.31588854555,1176.18563517179,1177.05538179847,
1177.92512842556,1178.79487505304,1179.66547437075,1180.53607368863,1181.40582031696,
1182.27556694557,1183.14531357444,1184.01506020352,1184.88480683277,1185.75455346216,
1186.62515278112,1187.4957521001,1188.36549872963,1189.23524535914,1190.10499198858,
1190.97473861791,1191.84448524708,1192.71423187606,1193.58483119448,1194.45543051277,
1195.3251771411,1196.19492376911,1197.06467039678,1197.93441702407,1198.80416365096,
1199.67391027742,1200.5445095938,1201.41510890996,1202.28485553525,1203.15460216005,
1204.02434878434,1204.89409540809,1205.76384203131,1206.1987153427,1206.63358865396,
1207.06846196508,1207.50418796741,1208.37478728058,1209.2445339018,1209.6794072122,
1210.11428052245,1210.54915383255,1210.9840271425,1211.41890045231,1211.85377376197,
1212.28864707147,1212.72352038083,1213.15839369005,1213.59326699911,1214.02814030802,
1214.46386630925,1214.89959231048,1215.3344656191,1215.76933892757,1216.20421223589,
1216.63908554406,1217.07395885209,1217.50883215998,1217.94370546771,1218.37857877531,
1218.81345208276,1219.24832539007,1219.68319869724,1220.11807200426,1220.55294531115,
1220.9878186179,1221.42354461805,1221.85927061821,1222.29414392468,1222.72901723103,
1223.16389053724,1223.59876384332,1224.03363714927,1224.46851045509,1224.90338376079,
1225.33825706636,1225.77313037181,1226.20800367713,1226.64287698234,1227.07775028743,
1227.51262359241,1227.94749689727,1228.3832228965,1228.81894889572,1229.25382220036,
1229.6886955049,1230.12356880933,1230.55844211366,1230.99331541789,1231.42818872202,
1231.86306202606,1232.29793533,1232.73280863385,1233.16768193762,1233.60255524129,
1234.03742854489,1234.4723018484,1234.90717515184,1235.34290115037,1235.7786271489,
1236.21350045219,1236.64837375541,1237.08324705856,1237.51812036165,1237.95299366467,
1238.38786696764,1238.82274027055,1239.25761357341,1239.69248687621,1240.12736017897,
1240.56223348169,1240.99710678436,1241.431980087,1241.8668533896,1242.30257938773,
1242.73830538585,1243.17317868839,1243.6080519909,1244.04292529338,1244.47779859585,
1244.91267189829,1245.34754520072,1245.78241850314,1246.21729180555,1246.65216510795,
1247.08703841035,1247.52191171275,1247.95678501515,1248.39165831756,1248.82653161998,
1249.26225761804,1249.69798361611,1250.13285691855,1250.56773022101,1251.0026035235,
1251.43747682601,1251.87235012854,1252.30722343111,1252.74209673371,1253.17697003634,
1253.61184333901,1254.04671664173,1254.48158994449,1254.9164632473,1255.35133655015,
1255.78620985306,1256.22193585139,1256.65766184973,1257.09253515275,1257.52740845584,
1257.96228175899,1258.39715506221,1258.8320283655,1259.26690166886,1259.7017749723,
1260.13664827581,1260.57152157941,1261.00639488309,1261.44126818685,1261.8761414907,
1262.31101479465,1262.74588809868,1263.1816140976,1263.61734009651,1264.05221340074,
1264.48708670507,1264.9219600095,1265.35683331403,1265.79170661868,1266.22657992343,
1266.66145322829,1267.09632653327,1267.53119983836,1267.96607314357,1268.4009464489,
1268.83581975434,1269.27069305992,1269.70556636561,1270.14129236537,1270.57701836513,
1271.01189167108,1271.44676497716,1271.88163828337,1272.31651158971,1272.75138489619,
1273.1862582028,1273.62113150955,1274.05600481644,1274.49087812347,1274.92575143063,
1275.36062473794,1275.79549804539,1276.23037135299,1276.66524466073,1277.10097066151,
1277.5366966623,1277.97156997033,1278.40644327851,1278.84131658683,1279.2761898953,
1279.71106320392,1280.14593651268,1280.5808098216,1281.01568313066,1281.45055643987,
1281.88542974923,1282.32030305874,1282.75517636839,1283.1900496782,1283.62492298815,
1284.06064899005,1284.49637499195,1284.9312483022,1285.36612161259,1285.80099492313,
1286.23586823382,1286.67074154465,1287.54048816674,1287.975361478,1288.4102347894,
1288.84510810093,1289.27998141261,1289.71485472442,1290.14972803636,1291.02032735139,
1291.89092666668,1292.32579997914,1292.76067329173,1293.19554660444,1293.63041991727,
1294.50016654328,1295.36991316974,1296.23965979663,1297.10940642392,1297.9800057415,
1298.85060505925,1299.72035168742,1300.5900983159,1301.45984494464,1302.32959157362,
1303.19933820279,1304.06908483212,1304.93968415104,1305.81028347,1306.68003009953,
1307.54977672906,1308.41952335854,1309.28926998793,1310.15901661718,1311.02876324626,
1311.89936256477,1312.76996188316,1313.63970851164,1314.50945513981,1315.37920176765,
1316.24894839514,1317.11869502223,1317.98844164891,1318.85904096546,1319.72964028179,
1320.59938690733,1321.46913353238,1322.33888015692,1323.20862678095,1323.64350009276,
1324.07837340443,1324.51324671597,1324.94812002737,1325.81871934103,1326.68931865441,
1327.12419196524,1327.55906527593,1327.99393858647,1328.42881189686,1328.86368520711,
1329.29855851721,1329.73343182716,1330.16830513697,1330.60317844663,1331.03805175614,
1331.4729250655,1331.90779837471,1332.34267168377,1332.77839768507,1333.21412368638,
1333.64899699514,1334.08387030376,1334.51874361223,1334.95361692055,1335.38849022873,
1335.82336353676,1336.25823684464,1336.69311015238,1337.12798345997,1337.56285676742,
1337.99773007473,1338.4326033819,1338.86747668892,1339.30234999581,1339.73807599603,
1340.17380199625,1340.60867530287,1341.04354860934,1341.47842191569,1341.9132952219,
1342.34816852798,1342.78304183393,1343.21791513975,1343.65278844545,1344.08766175102,
1344.52253505647,1344.95740836179,1345.392281667,1345.82715497209,1346.26202827707,
1346.69775427635,1347.13348027563,1347.56835358038,1348.00322688502,1348.43810018956,
1348.87297349399,1349.30784679832,1349.74272010255,1350.17759340668,1350.61246671072,
1351.04734001466,1351.48221331851,1351.91708662228,1352.35195992595,1352.78683322955,
1353.22170653306,1353.65743253163,1354.09315853019,1354.52803183356,1354.96290513685,
1355.39777844007,1355.83265174322,1356.26752504631,1356.70239834933,1357.1372716523,
1357.57214495521,1358.00701825807,1358.44189156087,1358.87676486363,1359.31163816635,
1359.74651146902,1360.18138477166,1360.6171107698,1361.05283676795,1361.48771007051,
1361.92258337305,1362.35745667556,1362.79232997804,1363.2272032805,1363.66207658295,
1364.09694988538,1364.5318231878,1364.96669649021,1365.40156979261,1365.83644309501,
1366.27131639741,1366.70618969981,1367.14106300222,1367.57678900028,1368.01251499834,
1368.44738830077,1368.88226160321,1369.31713490567,1369.75200820816,1370.18688151067,
1370.6217548132,1371.05662811577,1371.49150141837,1371.926374721,1372.36124802367,
1372.79612132639,1373.23099462915,1373.66586793196,1374.10074123481,1374.53646723311,
1374.97219323142,1375.40706653438,1375.84193983741,1376.2768131405,1376.71168644365,
1377.14655974687,1377.58143305016,1378.01630635352,1378.45117965696,1378.88605296047,
1379.32092626407,1379.75579956775,1380.19067287151,1380.62554617536,1381.06041947931,
1381.49614547817,1381.93187147704,1382.36674478117,1382.8016180854,1383.23649138973,
1383.67136469416,1384.10623799869,1384.54111130334,1384.97598460809,1385.41085791295,
1385.84573121793,1386.28060452302,1386.71547782823,1387.15035113356,1387.585224439,
1388.02009774458,1388.45582374427,1388.89154974397,1389.32642304979,1389.76129635574,
1390.19616966182,1390.63104296803,1391.06591627437,1391.50078958085,1391.93566288746,
1392.37053619421,1392.8054095011,1393.24028280813,1393.6751561153,1394.1100294226,
1394.54490273005,1394.97977603765,1395.41550203836,1395.85122803908,1396.28610134696,
1396.72097465499,1397.15584796317,1397.59072127149,1398.02559457996,1398.46046788858,
1398.89534119734,1399.33021450626,1399.76508781532,1400.19996112453,1400.63483443389,
1401.50458105306,1401.93945436286,1402.37518036469,1402.81090636651,1403.24577967661,
1403.68065298686,1404.11552629725,1404.5503996078,1404.98527291848,1405.85501954029,
1406.2898928514,1406.72476616266,1407.15963947406,1407.5945127856,1408.02938609727,
1408.46425940908,1409.33485872391,1410.205458039,1410.64033135134,1411.07520466381,
1411.51007797639,1411.9449512891,1412.81469791488,1413.68444454112,1414.5541911678,
1415.42393779489,1416.29453711233,1417.16513642995,1418.03488305796,1418.90462968629,
1419.77437631491,1420.64412294377,1421.51386957285,1422.38361620211,1423.25421552099,
1424.12481483992,1424.99456146943,1425.86430809896,1426.73405472847,1427.60380135791,
1428.47354798724,1429.34329461641,1430.21389393501,1431.08449325349,1431.9542398821,
1432.82398651043,1433.69373313844,1434.56347976611,1435.4332263934,1436.30297302029,
1437.17357233701,1438.04417165351,1438.91391827929,1439.78366490459,1440.65341152939,
1441.52315815367,1441.95803146562,1442.39290477743,1442.8277780891,1443.26265140064,
1444.13325071451,1445.00385002811,1445.43872333908,1445.87359664991,1446.3084699606,
1446.74334327114,1447.17821658153,1447.61308989178,1448.48283651184,1448.91770982164,
1449.3525831313,1449.78745644081,1450.22232975017,1450.65720305938,1451.09292906076,
1451.52865506214,1451.96352837105,1452.39840167982,1452.83327498843,1453.2681482969,
1453.70302160522,1454.1378949134,1454.57276822143,1455.00764152931,1455.44251483705,
1455.87738814464,1456.31226145209,1456.7471347594,1457.18200806657,1457.6168813736,
1458.05260737389,1458.48833337418,1458.92320668093,1459.35807998754,1459.79295329402,
1460.22782660036,1460.66269990657,1461.09757321265,1461.5324465186,1461.96731982443,
1462.40219313012,1462.83706643569,1463.27193974114,1463.70681304647,1464.14168635168,
1464.57655965677,1465.0122856561,1465.44801165544,1465.8828849603,1466.31775826505,
1466.7526315697,1467.18750487423,1467.62237817866,1468.05725148299,1468.49212478722,
1468.92699809135,1469.36187139539,1469.79674469933,1470.23161800319,1470.66649130695,
1471.10136461063,1471.53623791422,1471.97196391283,1472.40768991143,1472.84256321487,
1473.27743651823,1473.71230982152,1474.14718312474,1474.58205642789,1475.01692973098,
1475.451803034,1475.88667633697,1476.32154963988,1476.75642294274,1477.19129624555,
1477.62616954831,1478.06104285102,1478.4959161537,1478.93164215186,1479.36736815002,
1479.80224145262,1480.23711475519,1480.67198805772,1481.10686136023,1481.54173466272,
1481.97660796518,1482.41148126762,1482.84635457005,1483.28122787247,1483.71610117488,
1484.15097447728,1484.58584777968,1485.02072108208,1485.45559438449,1485.89132038254,
1486.32704638059,1486.76191968301,1487.19679298544,1487.63166628788,1488.06653959035,
1488.50141289283,1488.93628619534,1489.37115949787,1489.80603280044,1490.24090610304,
1490.67577940567,1491.11065270835,1491.54552601106,1491.98039931382,1492.41527261663,
1492.8509986149,1493.28672461318,1493.72159791609,1494.15647121906,1494.59134452208,
1495.02621782517,1495.46109112832,1495.89596443154,1496.33083773483,1496.76571103819,
1497.20058434163,1497.63545764515,1498.07033094874,1498.50520425242,1498.94007755618,
1499.37495086004,1499.81067685885,1500.24640285767,1500.68127616171,1501.11614946584,
1501.55102277007,1501.9858960744,1502.42076937883,1502.85564268337,1503.29051598801,
1503.72538929276,1504.16026259762,1504.5951359026,1505.03000920769,1505.4648825129,
1505.89975581823,1506.33462912368,1506.77035512331,1507.20608112294,1507.64095442864,
1508.07582773446,1508.51070104041,1508.94557434649,1509.3804476527,1509.81532095904,
1510.25019426552,1510.68506757213,1511.11994087888,1511.55481418577,1511.9896874928,
1512.42456079996,1512.85943410727,1513.29430741472,1513.73003341537,1514.16575941601,
1514.60063272375,1515.03550603163,1515.47037933966,1515.90525264784,1516.34012595616,
1516.77499926463,1517.20987257325,1517.64474588201,1518.07961919093,1518.51449249999,
1518.9493658092,1519.38423911856,1519.81911242807,1520.25398573772,1520.68971173947,
1521.12543774122,1521.56031105118,1521.99518436128,1522.43005767153,1523.29980429246,
1523.73467760315,1524.16955091398,1524.60442422495,1525.03929753607,1525.47417084733,
1525.90904415873,1526.77879078194,1527.64939009657,1528.08511609939,1528.51998941146,
1528.95486272367,1529.38973603601,1530.25948266106,1531.1292292866,1531.99897591261,
1532.86872253907,1533.73846916596,1534.60906848325,1535.47966780073,1536.34941442858,
1537.21916105675,1538.08890768523,1538.95865431398,1539.82840094295,1540.69814757212,
1541.56874689096,1542.43934620985,1543.30909283933,1544.17883946886,1545.04858609839,
1545.91833272787,1546.78807935726,1547.65782598651,1548.52842530518,1549.39902462375,
1550.26877125249,1551.13851788097,1552.00826450914,1552.87801113699,1553.74775776447,
1554.61750439156,1555.48810370844,1556.35870302511,1557.22844965112,1558.09819627666,
1558.96794290171,1559.83768952626,1560.27256283834,1560.70743615028,1561.57718277377,
1562.44778208785,1563.31838140165,1563.75325471277,1564.18812802374,1564.62300133457,
1565.05787464526,1565.9276212662,1566.79736788655,1567.2322411965,1567.66711450631,
1568.10198781596,1568.53686112547,1568.97173443483,1569.40746043628,1569.84318643774,
1570.2780597468,1570.71293305571,1571.14780636448,1571.5826796731,1572.01755298157,
1572.45242628989,1572.88729959806,1573.32217290609,1573.75704621397,1574.19191952171,
1574.62679282931,1575.06166613676,1575.49653944407,1575.93141275123,1576.36713875159,
1576.80286475195,1577.23773805884,1577.67261136559,1578.1074846722,1578.54235797868,
1578.97723128502,1579.41210459124,1579.84697789732,1580.28185120327,1580.71672450909,
1581.15159781478,1581.58647112036,1582.0213444258,1582.45621773113,1582.89109103634,
1583.32681703573,1583.76254303513,1584.1974163401,1584.63228964497,1585.06716294972,
1585.50203625436,1585.9369095589,1586.37178286333,1586.80665616766,1587.24152947189,
1587.67640277602,1588.11127608005,1588.546149384,1588.98102268785,1589.41589599161,
1589.85076929529,1590.28649529394,1590.72222129258,1591.1570945961,1591.59196789953,
1592.0268412029,1592.46171450619,1592.8965878094,1593.33146111256,1593.76633441564,
1594.20120771867,1594.63608102164,1595.07095432455,1595.50582762741,1595.94070093021,
1596.37557423297,1596.81044753569,1597.24617353387,1597.68189953206,1598.11677283469,
1598.55164613729,1598.98651943985,1599.42139274239,1599.8562660449,1600.29113934738,
1600.72601264985,1601.16088595229,1601.59575925472,1602.03063255714,1602.46550585955,
1602.90037916195,1603.33525246435,1603.77012576675,1604.2058517648,1604.64157776285,
1605.07645106526,1605.51132436768,1605.94619767011,1606.38107097255,1606.81594427502,
1607.2508175775,1607.68569088001,1608.12056418254,1608.55543748511,1608.99031078771,
1609.42518409034,1609.86005739302,1610.29493069573,1610.72980399849,1611.16552999674,
1611.60125599499,1612.03612929785,1612.47100260076,1612.90587590373,1613.34074920675,
1613.77562250984,1614.21049581299,1614.64536911621,1615.0802424195,1615.51511572286,
1615.9499890263,1616.38486232981,1616.81973563341,1617.25460893709,1617.68948224085,
1618.12520823963,1618.5609342384,1618.99580754234,1619.43068084638,1619.86555415051,
1620.30042745474,1620.73530075907,1621.1701740635,1621.60504736804,1622.03992067268,
1622.47479397743,1622.90966728229,1623.34454058727,1623.77941389236,1624.21428719757,
1624.6491605029,1625.08488650247,1625.52061250204,1625.95548580761,1626.39035911331,
1626.82523241913,1627.26010572508,1627.69497903116,1628.12985233737,1628.56472564372,
1628.99959895019,1629.43447225681,1629.86934556356,1630.30421887044,1630.73909217747,
1631.17396548464,1631.60883879195,1632.04456479252,1632.48029079309,1632.91516410068,
1633.35003740842,1633.78491071631,1634.21978402433,1634.65465733251,1635.08953064083,
1635.5244039493,1635.95927725792,1636.39415056668,1636.8290238756,1637.26389718466,
1637.69877049387,1638.13364380323,1638.56851711274,1639.00424311442,1639.43996911609,
1639.8748424259,1640.30971573585,1640.74458904595,1641.6143356666,1642.04920897714,
1642.48408228782,1642.91895559865,1643.35382890963,1643.78870222074,1644.223575532,
1645.09332215494,1645.52819546661,1645.96392146936,1646.39964747212,1646.83452078406,
1647.26939409614,1647.70426740834,1648.57401403314,1649.44376065844,1650.31350728422,
1650.74838059729,1651.18325391046,1652.05300053714,1652.92359985428,1653.79419917162,
1654.66394579929,1655.5336924273,1656.40343905563,1657.27318568424,1658.14293231311,
1659.01267894219,1659.88327826096,1660.75387757982,1661.62362420926,1662.49337083877,
1663.3631174683,1664.23286409781,1665.10261072725,1665.97235735658,1666.84295667531,
1667.71355599396,1668.58330262282,1669.45304925143,1670.32279587976,1671.19254250778,
1672.06228913544,1672.93203576273,1673.80263507977,1674.6732343966,1675.54298102284,
1676.41272764862,1677.28247427392,1678.15222089872,1679.021967523,1679.89171414676,
1680.76231346105,1681.19803946366,1681.63291277506,1682.06778608632,1682.50265939743,
1682.93753270841,1683.37240601924,1684.24215264047,1684.67702595086,1685.11189926111,
1685.54677257121,1685.98164588116,1686.41651919097,1686.85139250063,1687.28626581014,
1687.72199181166,1688.15771781319,1688.5925911224,1689.02746443146,1689.46233774038,
1689.89721104914,1690.33208435776,1690.76695766623,1691.20183097455,1691.63670428272,
1692.07157759075,1692.50645089864,1692.94132420637,1693.37619751397,1693.81107082142,
1694.24594412873,1694.68167012916,1695.11739612959,1695.55226943662,1695.9871427435,
1696.42201605025,1696.85688935687,1697.29176266334,1697.72663596969,1698.1615092759,
1698.59638258198,1699.03125588793,1699.46612919375,1699.90100249945,1700.33587580502,
1700.77074911047,1701.20562241579,1701.64134841525,1702.0770744147,1702.51194771979,
1702.94682102476,1703.38169432963,1703.81656763438,1704.25144093902,1704.68631424356,
1705.12118754799,1705.55606085232,1705.99093415655,1706.42580746068,1706.86068076471,
1707.29555406866,1707.73042737251,1708.16530067627,1708.60102667496,1709.03675267365,
1709.47162597724,1709.90649928076,1710.34137258419,1710.77624588756,1711.21111919085,
1711.64599249406,1712.08086579722,1712.5157391003,1712.95061240333,1713.3854857063,
1713.82035900921,1714.25523231207,1714.69010561487,1715.12497891763,1715.56070491584,
1715.99643091404,1716.43130421671,1716.86617751935,1717.30105082195,1717.73592412451,
1718.17079742705,1718.60567072956,1719.04054403204,1719.4754173345,1719.91029063695,
1720.34516393938,1720.7800372418,1721.21491054421,1721.64978384661,1722.08465714901,
1722.52038314706,1722.9561091451,1723.39098244751,1723.82585574992,1724.26072905233,
1724.69560235476,1725.13047565721,1725.56534895967,1726.00022226216,1726.43509556467,
1726.8699688672,1727.30484216977,1727.73971547236,1728.174588775,1728.60946207767,
1729.04433538039,1729.48006137861,1729.91578737684,1730.35066067965,1730.78553398251,
1731.22040728542,1731.65528058838,1732.09015389141,1732.5250271945,1732.95990049765,
1733.39477380087,1733.82964710416,1734.26452040752,1734.69939371096,1735.13426701447,
1735.56914031807,1736.00401362175,1736.43973962048,1736.8754656192,1737.31033892306,
1737.745212227,1738.18008553104,1738.61495883517,1739.0498321394,1739.48470544373,
1739.91957874816,1740.35445205269,1740.78932535734,1741.22419866209,1741.65907196695,
1742.09394527193,1742.52881857702,1742.96369188223,1743.39941788174,1743.83514388125,
1744.2700171867,1744.70489049227,1745.13976379797,1745.57463710379,1746.00951040974,
1746.44438371582,1746.87925702203,1747.31413032837,1747.74900363485,1748.18387694146,
1748.61875024821,1749.0536235551,1749.48849686213,1749.92337016929,1750.3590961698,
1750.7948221703,1751.22969547775,1751.66456878534,1752.09944209308,1752.53431540096,
1752.96918870899,1753.40406201717,1753.83893532549,1754.27380863396,1754.70868194258,
1755.14355525134,1755.57842856026,1756.01330186932,1756.44817517853,1756.88304848789,
1757.31877448949,1757.75450049109,1758.18937380075,1759.05912042051,1759.49399373061,
1759.92886704086,1760.36374035125,1760.79861366179,1761.23348697248,1761.66836028331,
1762.10323359429,1762.5381069054,1763.40785352806,1763.8427268396,1764.27845284228,
1764.71417884496,1765.14905215677,1765.58392546872,1766.0187987808,1766.88854540534,
1767.75829203039,1768.1931653431,1768.62803865593,1769.06291196888,1769.49778528195,
1770.36753190841,1771.2381312254,1772.10873054259,1772.97847717007,1773.84822379791,
1774.71797042609,1775.58771705456,1776.45746368331,1777.32721031228,1778.19780963089,
1779.06840894783,1779.93815555508,1780.80790201176,1781.67764871408),(-0.58309518948453,
0.),.UNSPECIFIED.) ;
#823=B_SPLINE_SURFACE_WITH_KNOTS('',3,1,((#50304,#50305),(#50306,#50307),
(#50308,#50309),(#50310,#50311),(#50312,#50313),(#50314,#50315),(#50316,
#50317),(#50318,#50319),(#50320,#50321),(#50322,#50323),(#50324,#50325),
(#50326,#50327),(#50328,#50329),(#50330,#50331),(#50332,#50333),(#50334,
#50335),(#50336,#50337),(#50338,#50339),(#50340,#50341),(#50342,#50343),
(#50344,#50345),(#50346,#50347),(#50348,#50349),(#50350,#50351),(#50352,
#50353),(#50354,#50355),(#50356,#50357),(#50358,#50359),(#50360,#50361),
(#50362,#50363),(#50364,#50365),(#50366,#50367),(#50368,#50369),(#50370,
#50371),(#50372,#50373),(#50374,#50375),(#50376,#50377),(#50378,#50379),
(#50380,#50381),(#50382,#50383),(#50384,#50385),(#50386,#50387),(#50388,
#50389),(#50390,#50391),(#50392,#50393),(#50394,#50395),(#50396,#50397),
(#50398,#50399),(#50400,#50401),(#50402,#50403),(#50404,#50405),(#50406,
#50407),(#50408,#50409),(#50410,#50411),(#50412,#50413),(#50414,#50415),
(#50416,#50417),(#50418,#50419),(#50420,#50421),(#50422,#50423),(#50424,
#50425),(#50426,#50427),(#50428,#50429),(#50430,#50431),(#50432,#50433),
(#50434,#50435),(#50436,#50437),(#50438,#50439),(#50440,#50441),(#50442,
#50443),(#50444,#50445),(#50446,#50447),(#50448,#50449),(#50450,#50451),
(#50452,#50453),(#50454,#50455),(#50456,#50457),(#50458,#50459),(#50460,
#50461),(#50462,#50463),(#50464,#50465),(#50466,#50467),(#50468,#50469),
(#50470,#50471),(#50472,#50473),(#50474,#50475),(#50476,#50477),(#50478,
#50479),(#50480,#50481),(#50482,#50483),(#50484,#50485),(#50486,#50487),
(#50488,#50489),(#50490,#50491),(#50492,#50493),(#50494,#50495),(#50496,
#50497),(#50498,#50499),(#50500,#50501),(#50502,#50503),(#50504,#50505),
(#50506,#50507),(#50508,#50509),(#50510,#50511),(#50512,#50513),(#50514,
#50515),(#50516,#50517),(#50518,#50519),(#50520,#50521),(#50522,#50523),
(#50524,#50525),(#50526,#50527),(#50528,#50529),(#50530,#50531),(#50532,
#50533),(#50534,#50535),(#50536,#50537),(#50538,#50539),(#50540,#50541),
(#50542,#50543),(#50544,#50545),(#50546,#50547),(#50548,#50549),(#50550,
#50551),(#50552,#50553),(#50554,#50555),(#50556,#50557),(#50558,#50559),
(#50560,#50561),(#50562,#50563),(#50564,#50565),(#50566,#50567),(#50568,
#50569),(#50570,#50571),(#50572,#50573),(#50574,#50575),(#50576,#50577),
(#50578,#50579),(#50580,#50581),(#50582,#50583),(#50584,#50585),(#50586,
#50587),(#50588,#50589),(#50590,#50591),(#50592,#50593),(#50594,#50595),
(#50596,#50597),(#50598,#50599),(#50600,#50601),(#50602,#50603),(#50604,
#50605),(#50606,#50607),(#50608,#50609),(#50610,#50611),(#50612,#50613),
(#50614,#50615),(#50616,#50617),(#50618,#50619),(#50620,#50621),(#50622,
#50623),(#50624,#50625),(#50626,#50627),(#50628,#50629),(#50630,#50631),
(#50632,#50633),(#50634,#50635),(#50636,#50637),(#50638,#50639),(#50640,
#50641),(#50642,#50643),(#50644,#50645),(#50646,#50647),(#50648,#50649),
(#50650,#50651),(#50652,#50653),(#50654,#50655),(#50656,#50657),(#50658,
#50659),(#50660,#50661),(#50662,#50663),(#50664,#50665),(#50666,#50667),
(#50668,#50669),(#50670,#50671),(#50672,#50673),(#50674,#50675),(#50676,
#50677),(#50678,#50679),(#50680,#50681),(#50682,#50683),(#50684,#50685),
(#50686,#50687),(#50688,#50689),(#50690,#50691),(#50692,#50693),(#50694,
#50695),(#50696,#50697),(#50698,#50699),(#50700,#50701),(#50702,#50703),
(#50704,#50705),(#50706,#50707),(#50708,#50709),(#50710,#50711),(#50712,
#50713),(#50714,#50715),(#50716,#50717),(#50718,#50719),(#50720,#50721),
(#50722,#50723),(#50724,#50725),(#50726,#50727),(#50728,#50729),(#50730,
#50731),(#50732,#50733),(#50734,#50735),(#50736,#50737),(#50738,#50739),
(#50740,#50741),(#50742,#50743),(#50744,#50745),(#50746,#50747),(#50748,
#50749),(#50750,#50751),(#50752,#50753),(#50754,#50755),(#50756,#50757),
(#50758,#50759),(#50760,#50761),(#50762,#50763),(#50764,#50765),(#50766,
#50767),(#50768,#50769),(#50770,#50771),(#50772,#50773),(#50774,#50775),
(#50776,#50777),(#50778,#50779),(#50780,#50781),(#50782,#50783),(#50784,
#50785),(#50786,#50787),(#50788,#50789),(#50790,#50791),(#50792,#50793),
(#50794,#50795),(#50796,#50797),(#50798,#50799),(#50800,#50801),(#50802,
#50803),(#50804,#50805),(#50806,#50807),(#50808,#50809),(#50810,#50811),
(#50812,#50813),(#50814,#50815),(#50816,#50817),(#50818,#50819),(#50820,
#50821),(#50822,#50823),(#50824,#50825),(#50826,#50827),(#50828,#50829),
(#50830,#50831),(#50832,#50833),(#50834,#50835),(#50836,#50837),(#50838,
#50839),(#50840,#50841),(#50842,#50843),(#50844,#50845),(#50846,#50847),
(#50848,#50849),(#50850,#50851),(#50852,#50853),(#50854,#50855),(#50856,
#50857),(#50858,#50859),(#50860,#50861),(#50862,#50863),(#50864,#50865),
(#50866,#50867),(#50868,#50869),(#50870,#50871),(#50872,#50873),(#50874,
#50875),(#50876,#50877),(#50878,#50879),(#50880,#50881),(#50882,#50883),
(#50884,#50885),(#50886,#50887),(#50888,#50889),(#50890,#50891),(#50892,
#50893),(#50894,#50895),(#50896,#50897),(#50898,#50899),(#50900,#50901),
(#50902,#50903),(#50904,#50905),(#50906,#50907),(#50908,#50909),(#50910,
#50911),(#50912,#50913),(#50914,#50915),(#50916,#50917),(#50918,#50919),
(#50920,#50921),(#50922,#50923),(#50924,#50925),(#50926,#50927),(#50928,
#50929),(#50930,#50931),(#50932,#50933),(#50934,#50935),(#50936,#50937),
(#50938,#50939),(#50940,#50941),(#50942,#50943),(#50944,#50945),(#50946,
#50947),(#50948,#50949),(#50950,#50951),(#50952,#50953),(#50954,#50955),
(#50956,#50957),(#50958,#50959),(#50960,#50961),(#50962,#50963),(#50964,
#50965),(#50966,#50967),(#50968,#50969),(#50970,#50971),(#50972,#50973),
(#50974,#50975),(#50976,#50977),(#50978,#50979),(#50980,#50981),(#50982,
#50983),(#50984,#50985),(#50986,#50987),(#50988,#50989),(#50990,#50991),
(#50992,#50993),(#50994,#50995),(#50996,#50997),(#50998,#50999),(#51000,
#51001),(#51002,#51003),(#51004,#51005),(#51006,#51007),(#51008,#51009),
(#51010,#51011),(#51012,#51013),(#51014,#51015),(#51016,#51017),(#51018,
#51019),(#51020,#51021),(#51022,#51023),(#51024,#51025),(#51026,#51027),
(#51028,#51029),(#51030,#51031),(#51032,#51033),(#51034,#51035),(#51036,
#51037),(#51038,#51039),(#51040,#51041),(#51042,#51043),(#51044,#51045),
(#51046,#51047),(#51048,#51049),(#51050,#51051),(#51052,#51053),(#51054,
#51055),(#51056,#51057),(#51058,#51059),(#51060,#51061),(#51062,#51063),
(#51064,#51065),(#51066,#51067),(#51068,#51069),(#51070,#51071),(#51072,
#51073),(#51074,#51075),(#51076,#51077),(#51078,#51079),(#51080,#51081),
(#51082,#51083),(#51084,#51085),(#51086,#51087),(#51088,#51089),(#51090,
#51091),(#51092,#51093),(#51094,#51095),(#51096,#51097),(#51098,#51099),
(#51100,#51101),(#51102,#51103),(#51104,#51105),(#51106,#51107),(#51108,
#51109),(#51110,#51111),(#51112,#51113),(#51114,#51115),(#51116,#51117),
(#51118,#51119),(#51120,#51121),(#51122,#51123),(#51124,#51125),(#51126,
#51127),(#51128,#51129),(#51130,#51131),(#51132,#51133),(#51134,#51135),
(#51136,#51137),(#51138,#51139),(#51140,#51141),(#51142,#51143),(#51144,
#51145),(#51146,#51147),(#51148,#51149),(#51150,#51151),(#51152,#51153),
(#51154,#51155),(#51156,#51157),(#51158,#51159),(#51160,#51161),(#51162,
#51163),(#51164,#51165),(#51166,#51167),(#51168,#51169),(#51170,#51171),
(#51172,#51173),(#51174,#51175),(#51176,#51177),(#51178,#51179),(#51180,
#51181),(#51182,#51183),(#51184,#51185),(#51186,#51187),(#51188,#51189),
(#51190,#51191),(#51192,#51193),(#51194,#51195),(#51196,#51197),(#51198,
#51199),(#51200,#51201),(#51202,#51203),(#51204,#51205),(#51206,#51207),
(#51208,#51209),(#51210,#51211),(#51212,#51213),(#51214,#51215),(#51216,
#51217),(#51218,#51219),(#51220,#51221),(#51222,#51223),(#51224,#51225),
(#51226,#51227),(#51228,#51229),(#51230,#51231),(#51232,#51233),(#51234,
#51235),(#51236,#51237),(#51238,#51239),(#51240,#51241),(#51242,#51243),
(#51244,#51245),(#51246,#51247),(#51248,#51249),(#51250,#51251),(#51252,
#51253),(#51254,#51255),(#51256,#51257),(#51258,#51259),(#51260,#51261),
(#51262,#51263),(#51264,#51265),(#51266,#51267),(#51268,#51269),(#51270,
#51271),(#51272,#51273),(#51274,#51275),(#51276,#51277),(#51278,#51279),
(#51280,#51281),(#51282,#51283),(#51284,#51285),(#51286,#51287),(#51288,
#51289),(#51290,#51291),(#51292,#51293),(#51294,#51295),(#51296,#51297),
(#51298,#51299),(#51300,#51301),(#51302,#51303),(#51304,#51305),(#51306,
#51307),(#51308,#51309),(#51310,#51311),(#51312,#51313),(#51314,#51315),
(#51316,#51317),(#51318,#51319),(#51320,#51321),(#51322,#51323),(#51324,
#51325),(#51326,#51327),(#51328,#51329),(#51330,#51331),(#51332,#51333),
(#51334,#51335),(#51336,#51337),(#51338,#51339),(#51340,#51341),(#51342,
#51343),(#51344,#51345),(#51346,#51347),(#51348,#51349),(#51350,#51351),
(#51352,#51353),(#51354,#51355),(#51356,#51357),(#51358,#51359),(#51360,
#51361),(#51362,#51363),(#51364,#51365),(#51366,#51367),(#51368,#51369),
(#51370,#51371),(#51372,#51373),(#51374,#51375),(#51376,#51377),(#51378,
#51379),(#51380,#51381),(#51382,#51383),(#51384,#51385),(#51386,#51387),
(#51388,#51389),(#51390,#51391),(#51392,#51393),(#51394,#51395),(#51396,
#51397),(#51398,#51399),(#51400,#51401),(#51402,#51403),(#51404,#51405),
(#51406,#51407),(#51408,#51409),(#51410,#51411),(#51412,#51413),(#51414,
#51415),(#51416,#51417),(#51418,#51419),(#51420,#51421),(#51422,#51423),
(#51424,#51425),(#51426,#51427),(#51428,#51429),(#51430,#51431),(#51432,
#51433),(#51434,#51435),(#51436,#51437),(#51438,#51439),(#51440,#51441),
(#51442,#51443),(#51444,#51445),(#51446,#51447),(#51448,#51449),(#51450,
#51451),(#51452,#51453),(#51454,#51455),(#51456,#51457),(#51458,#51459),
(#51460,#51461),(#51462,#51463),(#51464,#51465),(#51466,#51467),(#51468,
#51469),(#51470,#51471),(#51472,#51473),(#51474,#51475),(#51476,#51477),
(#51478,#51479),(#51480,#51481),(#51482,#51483),(#51484,#51485),(#51486,
#51487),(#51488,#51489),(#51490,#51491),(#51492,#51493),(#51494,#51495),
(#51496,#51497),(#51498,#51499),(#51500,#51501),(#51502,#51503),(#51504,
#51505),(#51506,#51507),(#51508,#51509),(#51510,#51511),(#51512,#51513),
(#51514,#51515),(#51516,#51517),(#51518,#51519),(#51520,#51521),(#51522,
#51523),(#51524,#51525),(#51526,#51527),(#51528,#51529),(#51530,#51531),
(#51532,#51533),(#51534,#51535),(#51536,#51537),(#51538,#51539),(#51540,
#51541),(#51542,#51543),(#51544,#51545),(#51546,#51547),(#51548,#51549),
(#51550,#51551),(#51552,#51553),(#51554,#51555),(#51556,#51557),(#51558,
#51559),(#51560,#51561),(#51562,#51563),(#51564,#51565),(#51566,#51567),
(#51568,#51569),(#51570,#51571),(#51572,#51573),(#51574,#51575),(#51576,
#51577),(#51578,#51579),(#51580,#51581),(#51582,#51583),(#51584,#51585),
(#51586,#51587),(#51588,#51589),(#51590,#51591),(#51592,#51593),(#51594,
#51595),(#51596,#51597),(#51598,#51599),(#51600,#51601),(#51602,#51603),
(#51604,#51605),(#51606,#51607),(#51608,#51609),(#51610,#51611),(#51612,
#51613),(#51614,#51615),(#51616,#51617),(#51618,#51619),(#51620,#51621),
(#51622,#51623),(#51624,#51625),(#51626,#51627),(#51628,#51629),(#51630,
#51631),(#51632,#51633),(#51634,#51635),(#51636,#51637),(#51638,#51639),
(#51640,#51641),(#51642,#51643),(#51644,#51645),(#51646,#51647),(#51648,
#51649),(#51650,#51651),(#51652,#51653),(#51654,#51655),(#51656,#51657),
(#51658,#51659),(#51660,#51661),(#51662,#51663),(#51664,#51665),(#51666,
#51667),(#51668,#51669),(#51670,#51671),(#51672,#51673),(#51674,#51675),
(#51676,#51677),(#51678,#51679),(#51680,#51681),(#51682,#51683),(#51684,
#51685),(#51686,#51687),(#51688,#51689),(#51690,#51691),(#51692,#51693),
(#51694,#51695),(#51696,#51697),(#51698,#51699),(#51700,#51701),(#51702,
#51703),(#51704,#51705),(#51706,#51707),(#51708,#51709),(#51710,#51711),
(#51712,#51713),(#51714,#51715),(#51716,#51717),(#51718,#51719),(#51720,
#51721),(#51722,#51723),(#51724,#51725),(#51726,#51727),(#51728,#51729),
(#51730,#51731),(#51732,#51733),(#51734,#51735),(#51736,#51737),(#51738,
#51739),(#51740,#51741),(#51742,#51743),(#51744,#51745),(#51746,#51747),
(#51748,#51749),(#51750,#51751),(#51752,#51753),(#51754,#51755),(#51756,
#51757),(#51758,#51759),(#51760,#51761),(#51762,#51763),(#51764,#51765),
(#51766,#51767),(#51768,#51769),(#51770,#51771),(#51772,#51773),(#51774,
#51775),(#51776,#51777),(#51778,#51779),(#51780,#51781),(#51782,#51783),
(#51784,#51785),(#51786,#51787),(#51788,#51789),(#51790,#51791),(#51792,
#51793),(#51794,#51795),(#51796,#51797),(#51798,#51799),(#51800,#51801),
(#51802,#51803),(#51804,#51805),(#51806,#51807),(#51808,#51809),(#51810,
#51811),(#51812,#51813),(#51814,#51815),(#51816,#51817),(#51818,#51819),
(#51820,#51821),(#51822,#51823),(#51824,#51825),(#51826,#51827),(#51828,
#51829),(#51830,#51831),(#51832,#51833),(#51834,#51835),(#51836,#51837),
(#51838,#51839),(#51840,#51841),(#51842,#51843),(#51844,#51845),(#51846,
#51847),(#51848,#51849),(#51850,#51851),(#51852,#51853),(#51854,#51855),
(#51856,#51857),(#51858,#51859),(#51860,#51861),(#51862,#51863),(#51864,
#51865),(#51866,#51867),(#51868,#51869),(#51870,#51871),(#51872,#51873),
(#51874,#51875),(#51876,#51877),(#51878,#51879),(#51880,#51881),(#51882,
#51883),(#51884,#51885),(#51886,#51887),(#51888,#51889),(#51890,#51891),
(#51892,#51893),(#51894,#51895),(#51896,#51897),(#51898,#51899),(#51900,
#51901),(#51902,#51903),(#51904,#51905),(#51906,#51907),(#51908,#51909),
(#51910,#51911),(#51912,#51913),(#51914,#51915),(#51916,#51917),(#51918,
#51919),(#51920,#51921),(#51922,#51923),(#51924,#51925),(#51926,#51927),
(#51928,#51929),(#51930,#51931),(#51932,#51933),(#51934,#51935),(#51936,
#51937),(#51938,#51939),(#51940,#51941),(#51942,#51943),(#51944,#51945),
(#51946,#51947),(#51948,#51949),(#51950,#51951),(#51952,#51953),(#51954,
#51955),(#51956,#51957),(#51958,#51959),(#51960,#51961),(#51962,#51963),
(#51964,#51965),(#51966,#51967),(#51968,#51969),(#51970,#51971),(#51972,
#51973),(#51974,#51975),(#51976,#51977),(#51978,#51979),(#51980,#51981),
(#51982,#51983),(#51984,#51985),(#51986,#51987),(#51988,#51989),(#51990,
#51991),(#51992,#51993),(#51994,#51995),(#51996,#51997),(#51998,#51999),
(#52000,#52001),(#52002,#52003),(#52004,#52005),(#52006,#52007),(#52008,
#52009),(#52010,#52011),(#52012,#52013),(#52014,#52015),(#52016,#52017),
(#52018,#52019),(#52020,#52021),(#52022,#52023),(#52024,#52025),(#52026,
#52027),(#52028,#52029),(#52030,#52031),(#52032,#52033),(#52034,#52035),
(#52036,#52037),(#52038,#52039),(#52040,#52041),(#52042,#52043),(#52044,
#52045),(#52046,#52047),(#52048,#52049),(#52050,#52051),(#52052,#52053),
(#52054,#52055),(#52056,#52057),(#52058,#52059),(#52060,#52061),(#52062,
#52063),(#52064,#52065),(#52066,#52067),(#52068,#52069),(#52070,#52071),
(#52072,#52073),(#52074,#52075),(#52076,#52077),(#52078,#52079),(#52080,
#52081),(#52082,#52083),(#52084,#52085),(#52086,#52087),(#52088,#52089),
(#52090,#52091),(#52092,#52093),(#52094,#52095),(#52096,#52097),(#52098,
#52099),(#52100,#52101),(#52102,#52103),(#52104,#52105),(#52106,#52107),
(#52108,#52109),(#52110,#52111),(#52112,#52113),(#52114,#52115),(#52116,
#52117),(#52118,#52119),(#52120,#52121),(#52122,#52123),(#52124,#52125),
(#52126,#52127),(#52128,#52129),(#52130,#52131),(#52132,#52133),(#52134,
#52135),(#52136,#52137),(#52138,#52139),(#52140,#52141),(#52142,#52143),
(#52144,#52145),(#52146,#52147),(#52148,#52149),(#52150,#52151),(#52152,
#52153),(#52154,#52155),(#52156,#52157),(#52158,#52159),(#52160,#52161),
(#52162,#52163),(#52164,#52165),(#52166,#52167),(#52168,#52169),(#52170,
#52171),(#52172,#52173),(#52174,#52175),(#52176,#52177),(#52178,#52179),
(#52180,#52181),(#52182,#52183),(#52184,#52185),(#52186,#52187),(#52188,
#52189),(#52190,#52191),(#52192,#52193),(#52194,#52195),(#52196,#52197),
(#52198,#52199),(#52200,#52201),(#52202,#52203),(#52204,#52205),(#52206,
#52207),(#52208,#52209),(#52210,#52211),(#52212,#52213),(#52214,#52215),
(#52216,#52217),(#52218,#52219),(#52220,#52221),(#52222,#52223),(#52224,
#52225),(#52226,#52227),(#52228,#52229),(#52230,#52231),(#52232,#52233),
(#52234,#52235),(#52236,#52237),(#52238,#52239),(#52240,#52241),(#52242,
#52243),(#52244,#52245),(#52246,#52247),(#52248,#52249),(#52250,#52251),
(#52252,#52253),(#52254,#52255),(#52256,#52257),(#52258,#52259),(#52260,
#52261),(#52262,#52263),(#52264,#52265),(#52266,#52267),(#52268,#52269),
(#52270,#52271),(#52272,#52273),(#52274,#52275),(#52276,#52277),(#52278,
#52279),(#52280,#52281),(#52282,#52283),(#52284,#52285),(#52286,#52287),
(#52288,#52289),(#52290,#52291),(#52292,#52293),(#52294,#52295),(#52296,
#52297),(#52298,#52299),(#52300,#52301),(#52302,#52303),(#52304,#52305),
(#52306,#52307),(#52308,#52309),(#52310,#52311),(#52312,#52313),(#52314,
#52315),(#52316,#52317),(#52318,#52319),(#52320,#52321),(#52322,#52323),
(#52324,#52325),(#52326,#52327),(#52328,#52329),(#52330,#52331),(#52332,
#52333),(#52334,#52335),(#52336,#52337),(#52338,#52339),(#52340,#52341),
(#52342,#52343),(#52344,#52345),(#52346,#52347),(#52348,#52349),(#52350,
#52351),(#52352,#52353),(#52354,#52355),(#52356,#52357),(#52358,#52359),
(#52360,#52361),(#52362,#52363),(#52364,#52365),(#52366,#52367),(#52368,
#52369),(#52370,#52371),(#52372,#52373),(#52374,#52375),(#52376,#52377),
(#52378,#52379),(#52380,#52381),(#52382,#52383),(#52384,#52385),(#52386,
#52387),(#52388,#52389),(#52390,#52391),(#52392,#52393),(#52394,#52395),
(#52396,#52397),(#52398,#52399),(#52400,#52401),(#52402,#52403),(#52404,
#52405),(#52406,#52407),(#52408,#52409),(#52410,#52411),(#52412,#52413),
(#52414,#52415),(#52416,#52417),(#52418,#52419),(#52420,#52421),(#52422,
#52423),(#52424,#52425),(#52426,#52427),(#52428,#52429),(#52430,#52431),
(#52432,#52433),(#52434,#52435),(#52436,#52437),(#52438,#52439),(#52440,
#52441),(#52442,#52443),(#52444,#52445),(#52446,#52447),(#52448,#52449),
(#52450,#52451),(#52452,#52453),(#52454,#52455),(#52456,#52457),(#52458,
#52459),(#52460,#52461),(#52462,#52463),(#52464,#52465),(#52466,#52467),
(#52468,#52469),(#52470,#52471),(#52472,#52473),(#52474,#52475),(#52476,
#52477),(#52478,#52479),(#52480,#52481),(#52482,#52483),(#52484,#52485),
(#52486,#52487),(#52488,#52489),(#52490,#52491),(#52492,#52493),(#52494,
#52495),(#52496,#52497),(#52498,#52499),(#52500,#52501),(#52502,#52503),
(#52504,#52505),(#52506,#52507),(#52508,#52509),(#52510,#52511),(#52512,
#52513),(#52514,#52515),(#52516,#52517),(#52518,#52519),(#52520,#52521),
(#52522,#52523),(#52524,#52525),(#52526,#52527),(#52528,#52529),(#52530,
#52531),(#52532,#52533),(#52534,#52535),(#52536,#52537),(#52538,#52539),
(#52540,#52541),(#52542,#52543),(#52544,#52545),(#52546,#52547),(#52548,
#52549),(#52550,#52551),(#52552,#52553),(#52554,#52555),(#52556,#52557),
(#52558,#52559),(#52560,#52561),(#52562,#52563),(#52564,#52565),(#52566,
#52567),(#52568,#52569),(#52570,#52571),(#52572,#52573),(#52574,#52575),
(#52576,#52577),(#52578,#52579),(#52580,#52581),(#52582,#52583),(#52584,
#52585),(#52586,#52587),(#52588,#52589),(#52590,#52591),(#52592,#52593),
(#52594,#52595),(#52596,#52597),(#52598,#52599),(#52600,#52601),(#52602,
#52603),(#52604,#52605),(#52606,#52607),(#52608,#52609),(#52610,#52611),
(#52612,#52613),(#52614,#52615),(#52616,#52617),(#52618,#52619),(#52620,
#52621),(#52622,#52623),(#52624,#52625),(#52626,#52627),(#52628,#52629),
(#52630,#52631),(#52632,#52633),(#52634,#52635),(#52636,#52637),(#52638,
#52639),(#52640,#52641),(#52642,#52643),(#52644,#52645),(#52646,#52647),
(#52648,#52649),(#52650,#52651),(#52652,#52653),(#52654,#52655),(#52656,
#52657),(#52658,#52659),(#52660,#52661),(#52662,#52663),(#52664,#52665),
(#52666,#52667),(#52668,#52669),(#52670,#52671),(#52672,#52673),(#52674,
#52675),(#52676,#52677),(#52678,#52679),(#52680,#52681),(#52682,#52683),
(#52684,#52685),(#52686,#52687),(#52688,#52689),(#52690,#52691),(#52692,
#52693),(#52694,#52695),(#52696,#52697),(#52698,#52699),(#52700,#52701),
(#52702,#52703),(#52704,#52705),(#52706,#52707),(#52708,#52709),(#52710,
#52711),(#52712,#52713),(#52714,#52715),(#52716,#52717),(#52718,#52719),
(#52720,#52721),(#52722,#52723),(#52724,#52725),(#52726,#52727),(#52728,
#52729),(#52730,#52731),(#52732,#52733),(#52734,#52735),(#52736,#52737),
(#52738,#52739),(#52740,#52741),(#52742,#52743),(#52744,#52745),(#52746,
#52747),(#52748,#52749),(#52750,#52751),(#52752,#52753),(#52754,#52755),
(#52756,#52757),(#52758,#52759),(#52760,#52761),(#52762,#52763),(#52764,
#52765),(#52766,#52767),(#52768,#52769),(#52770,#52771),(#52772,#52773),
(#52774,#52775),(#52776,#52777),(#52778,#52779),(#52780,#52781),(#52782,
#52783),(#52784,#52785),(#52786,#52787),(#52788,#52789),(#52790,#52791),
(#52792,#52793),(#52794,#52795),(#52796,#52797),(#52798,#52799),(#52800,
#52801),(#52802,#52803),(#52804,#52805),(#52806,#52807),(#52808,#52809),
(#52810,#52811),(#52812,#52813),(#52814,#52815),(#52816,#52817),(#52818,
#52819),(#52820,#52821),(#52822,#52823),(#52824,#52825),(#52826,#52827),
(#52828,#52829),(#52830,#52831),(#52832,#52833),(#52834,#52835),(#52836,
#52837),(#52838,#52839),(#52840,#52841),(#52842,#52843),(#52844,#52845),
(#52846,#52847),(#52848,#52849),(#52850,#52851),(#52852,#52853),(#52854,
#52855),(#52856,#52857),(#52858,#52859),(#52860,#52861),(#52862,#52863),
(#52864,#52865),(#52866,#52867),(#52868,#52869),(#52870,#52871),(#52872,
#52873),(#52874,#52875),(#52876,#52877),(#52878,#52879),(#52880,#52881),
(#52882,#52883),(#52884,#52885),(#52886,#52887),(#52888,#52889),(#52890,
#52891),(#52892,#52893),(#52894,#52895),(#52896,#52897),(#52898,#52899),
(#52900,#52901),(#52902,#52903),(#52904,#52905),(#52906,#52907),(#52908,
#52909),(#52910,#52911),(#52912,#52913),(#52914,#52915),(#52916,#52917),
(#52918,#52919),(#52920,#52921),(#52922,#52923),(#52924,#52925),(#52926,
#52927),(#52928,#52929),(#52930,#52931),(#52932,#52933),(#52934,#52935),
(#52936,#52937),(#52938,#52939),(#52940,#52941),(#52942,#52943),(#52944,
#52945),(#52946,#52947),(#52948,#52949),(#52950,#52951),(#52952,#52953),
(#52954,#52955),(#52956,#52957),(#52958,#52959),(#52960,#52961),(#52962,
#52963),(#52964,#52965),(#52966,#52967),(#52968,#52969),(#52970,#52971),
(#52972,#52973),(#52974,#52975),(#52976,#52977),(#52978,#52979),(#52980,
#52981),(#52982,#52983),(#52984,#52985),(#52986,#52987),(#52988,#52989),
(#52990,#52991),(#52992,#52993),(#52994,#52995),(#52996,#52997),(#52998,
#52999),(#53000,#53001),(#53002,#53003),(#53004,#53005),(#53006,#53007),
(#53008,#53009),(#53010,#53011),(#53012,#53013),(#53014,#53015),(#53016,
#53017),(#53018,#53019),(#53020,#53021),(#53022,#53023),(#53024,#53025),
(#53026,#53027),(#53028,#53029),(#53030,#53031),(#53032,#53033),(#53034,
#53035),(#53036,#53037),(#53038,#53039),(#53040,#53041),(#53042,#53043),
(#53044,#53045),(#53046,#53047),(#53048,#53049),(#53050,#53051),(#53052,
#53053),(#53054,#53055),(#53056,#53057),(#53058,#53059),(#53060,#53061),
(#53062,#53063),(#53064,#53065),(#53066,#53067),(#53068,#53069),(#53070,
#53071),(#53072,#53073),(#53074,#53075),(#53076,#53077),(#53078,#53079),
(#53080,#53081),(#53082,#53083),(#53084,#53085),(#53086,#53087),(#53088,
#53089),(#53090,#53091),(#53092,#53093),(#53094,#53095),(#53096,#53097),
(#53098,#53099),(#53100,#53101),(#53102,#53103),(#53104,#53105),(#53106,
#53107),(#53108,#53109),(#53110,#53111),(#53112,#53113),(#53114,#53115),
(#53116,#53117),(#53118,#53119),(#53120,#53121),(#53122,#53123),(#53124,
#53125),(#53126,#53127),(#53128,#53129),(#53130,#53131),(#53132,#53133),
(#53134,#53135),(#53136,#53137),(#53138,#53139),(#53140,#53141),(#53142,
#53143),(#53144,#53145),(#53146,#53147),(#53148,#53149),(#53150,#53151),
(#53152,#53153),(#53154,#53155),(#53156,#53157),(#53158,#53159),(#53160,
#53161),(#53162,#53163),(#53164,#53165),(#53166,#53167),(#53168,#53169),
(#53170,#53171),(#53172,#53173),(#53174,#53175),(#53176,#53177),(#53178,
#53179),(#53180,#53181),(#53182,#53183),(#53184,#53185),(#53186,#53187),
(#53188,#53189),(#53190,#53191),(#53192,#53193),(#53194,#53195),(#53196,
#53197),(#53198,#53199),(#53200,#53201),(#53202,#53203),(#53204,#53205),
(#53206,#53207),(#53208,#53209),(#53210,#53211),(#53212,#53213),(#53214,
#53215),(#53216,#53217),(#53218,#53219),(#53220,#53221),(#53222,#53223),
(#53224,#53225),(#53226,#53227),(#53228,#53229),(#53230,#53231),(#53232,
#53233),(#53234,#53235),(#53236,#53237),(#53238,#53239),(#53240,#53241),
(#53242,#53243),(#53244,#53245),(#53246,#53247),(#53248,#53249),(#53250,
#53251),(#53252,#53253),(#53254,#53255),(#53256,#53257),(#53258,#53259),
(#53260,#53261),(#53262,#53263),(#53264,#53265),(#53266,#53267),(#53268,
#53269),(#53270,#53271),(#53272,#53273),(#53274,#53275),(#53276,#53277),
(#53278,#53279),(#53280,#53281),(#53282,#53283),(#53284,#53285),(#53286,
#53287),(#53288,#53289),(#53290,#53291),(#53292,#53293),(#53294,#53295),
(#53296,#53297),(#53298,#53299),(#53300,#53301),(#53302,#53303),(#53304,
#53305),(#53306,#53307),(#53308,#53309),(#53310,#53311),(#53312,#53313),
(#53314,#53315),(#53316,#53317),(#53318,#53319),(#53320,#53321),(#53322,
#53323),(#53324,#53325),(#53326,#53327),(#53328,#53329),(#53330,#53331),
(#53332,#53333),(#53334,#53335),(#53336,#53337),(#53338,#53339),(#53340,
#53341),(#53342,#53343),(#53344,#53345),(#53346,#53347),(#53348,#53349),
(#53350,#53351),(#53352,#53353),(#53354,#53355),(#53356,#53357),(#53358,
#53359),(#53360,#53361),(#53362,#53363),(#53364,#53365),(#53366,#53367),
(#53368,#53369),(#53370,#53371),(#53372,#53373),(#53374,#53375),(#53376,
#53377),(#53378,#53379),(#53380,#53381),(#53382,#53383),(#53384,#53385),
(#53386,#53387),(#53388,#53389),(#53390,#53391),(#53392,#53393),(#53394,
#53395),(#53396,#53397),(#53398,#53399),(#53400,#53401),(#53402,#53403),
(#53404,#53405),(#53406,#53407),(#53408,#53409),(#53410,#53411),(#53412,
#53413),(#53414,#53415),(#53416,#53417),(#53418,#53419),(#53420,#53421),
(#53422,#53423),(#53424,#53425),(#53426,#53427),(#53428,#53429),(#53430,
#53431),(#53432,#53433),(#53434,#53435),(#53436,#53437),(#53438,#53439),
(#53440,#53441),(#53442,#53443),(#53444,#53445),(#53446,#53447),(#53448,
#53449),(#53450,#53451),(#53452,#53453),(#53454,#53455),(#53456,#53457),
(#53458,#53459),(#53460,#53461),(#53462,#53463),(#53464,#53465),(#53466,
#53467),(#53468,#53469),(#53470,#53471),(#53472,#53473),(#53474,#53475),
(#53476,#53477),(#53478,#53479),(#53480,#53481),(#53482,#53483),(#53484,
#53485),(#53486,#53487),(#53488,#53489),(#53490,#53491),(#53492,#53493),
(#53494,#53495),(#53496,#53497),(#53498,#53499),(#53500,#53501),(#53502,
#53503),(#53504,#53505),(#53506,#53507),(#53508,#53509),(#53510,#53511),
(#53512,#53513),(#53514,#53515),(#53516,#53517),(#53518,#53519),(#53520,
#53521),(#53522,#53523),(#53524,#53525),(#53526,#53527),(#53528,#53529),
(#53530,#53531),(#53532,#53533),(#53534,#53535),(#53536,#53537),(#53538,
#53539),(#53540,#53541),(#53542,#53543),(#53544,#53545),(#53546,#53547),
(#53548,#53549),(#53550,#53551),(#53552,#53553),(#53554,#53555),(#53556,
#53557),(#53558,#53559),(#53560,#53561),(#53562,#53563),(#53564,#53565),
(#53566,#53567),(#53568,#53569),(#53570,#53571),(#53572,#53573),(#53574,
#53575),(#53576,#53577),(#53578,#53579),(#53580,#53581),(#53582,#53583),
(#53584,#53585),(#53586,#53587),(#53588,#53589),(#53590,#53591),(#53592,
#53593),(#53594,#53595),(#53596,#53597),(#53598,#53599),(#53600,#53601),
(#53602,#53603),(#53604,#53605),(#53606,#53607),(#53608,#53609),(#53610,
#53611),(#53612,#53613),(#53614,#53615),(#53616,#53617),(#53618,#53619),
(#53620,#53621),(#53622,#53623),(#53624,#53625),(#53626,#53627),(#53628,
#53629),(#53630,#53631),(#53632,#53633),(#53634,#53635),(#53636,#53637),
(#53638,#53639),(#53640,#53641),(#53642,#53643),(#53644,#53645),(#53646,
#53647),(#53648,#53649),(#53650,#53651),(#53652,#53653),(#53654,#53655),
(#53656,#53657),(#53658,#53659),(#53660,#53661),(#53662,#53663),(#53664,
#53665),(#53666,#53667),(#53668,#53669),(#53670,#53671),(#53672,#53673),
(#53674,#53675),(#53676,#53677),(#53678,#53679),(#53680,#53681),(#53682,
#53683),(#53684,#53685),(#53686,#53687),(#53688,#53689),(#53690,#53691),
(#53692,#53693),(#53694,#53695),(#53696,#53697),(#53698,#53699),(#53700,
#53701),(#53702,#53703),(#53704,#53705),(#53706,#53707),(#53708,#53709),
(#53710,#53711),(#53712,#53713),(#53714,#53715),(#53716,#53717),(#53718,
#53719),(#53720,#53721),(#53722,#53723),(#53724,#53725),(#53726,#53727),
(#53728,#53729),(#53730,#53731),(#53732,#53733),(#53734,#53735),(#53736,
#53737),(#53738,#53739),(#53740,#53741),(#53742,#53743),(#53744,#53745),
(#53746,#53747),(#53748,#53749),(#53750,#53751),(#53752,#53753),(#53754,
#53755),(#53756,#53757),(#53758,#53759),(#53760,#53761),(#53762,#53763),
(#53764,#53765),(#53766,#53767),(#53768,#53769),(#53770,#53771),(#53772,
#53773),(#53774,#53775),(#53776,#53777),(#53778,#53779),(#53780,#53781),
(#53782,#53783),(#53784,#53785),(#53786,#53787),(#53788,#53789),(#53790,
#53791),(#53792,#53793),(#53794,#53795),(#53796,#53797),(#53798,#53799),
(#53800,#53801),(#53802,#53803),(#53804,#53805),(#53806,#53807),(#53808,
#53809),(#53810,#53811),(#53812,#53813),(#53814,#53815),(#53816,#53817),
(#53818,#53819),(#53820,#53821),(#53822,#53823),(#53824,#53825),(#53826,
#53827),(#53828,#53829),(#53830,#53831),(#53832,#53833),(#53834,#53835),
(#53836,#53837),(#53838,#53839),(#53840,#53841),(#53842,#53843),(#53844,
#53845),(#53846,#53847),(#53848,#53849),(#53850,#53851),(#53852,#53853),
(#53854,#53855),(#53856,#53857),(#53858,#53859),(#53860,#53861),(#53862,
#53863),(#53864,#53865),(#53866,#53867),(#53868,#53869),(#53870,#53871),
(#53872,#53873),(#53874,#53875),(#53876,#53877),(#53878,#53879),(#53880,
#53881),(#53882,#53883),(#53884,#53885),(#53886,#53887),(#53888,#53889),
(#53890,#53891),(#53892,#53893),(#53894,#53895),(#53896,#53897),(#53898,
#53899),(#53900,#53901),(#53902,#53903),(#53904,#53905),(#53906,#53907),
(#53908,#53909),(#53910,#53911),(#53912,#53913),(#53914,#53915),(#53916,
#53917),(#53918,#53919),(#53920,#53921),(#53922,#53923),(#53924,#53925),
(#53926,#53927),(#53928,#53929),(#53930,#53931),(#53932,#53933),(#53934,
#53935),(#53936,#53937),(#53938,#53939),(#53940,#53941),(#53942,#53943),
(#53944,#53945),(#53946,#53947),(#53948,#53949),(#53950,#53951),(#53952,
#53953),(#53954,#53955),(#53956,#53957),(#53958,#53959),(#53960,#53961),
(#53962,#53963),(#53964,#53965),(#53966,#53967),(#53968,#53969),(#53970,
#53971),(#53972,#53973),(#53974,#53975),(#53976,#53977),(#53978,#53979),
(#53980,#53981),(#53982,#53983),(#53984,#53985),(#53986,#53987),(#53988,
#53989),(#53990,#53991),(#53992,#53993),(#53994,#53995),(#53996,#53997),
(#53998,#53999),(#54000,#54001),(#54002,#54003),(#54004,#54005),(#54006,
#54007),(#54008,#54009),(#54010,#54011),(#54012,#54013),(#54014,#54015),
(#54016,#54017),(#54018,#54019),(#54020,#54021),(#54022,#54023),(#54024,
#54025),(#54026,#54027),(#54028,#54029),(#54030,#54031),(#54032,#54033),
(#54034,#54035),(#54036,#54037),(#54038,#54039),(#54040,#54041),(#54042,
#54043),(#54044,#54045),(#54046,#54047),(#54048,#54049),(#54050,#54051),
(#54052,#54053),(#54054,#54055),(#54056,#54057),(#54058,#54059),(#54060,
#54061),(#54062,#54063),(#54064,#54065),(#54066,#54067),(#54068,#54069),
(#54070,#54071),(#54072,#54073),(#54074,#54075),(#54076,#54077),(#54078,
#54079),(#54080,#54081),(#54082,#54083),(#54084,#54085),(#54086,#54087),
(#54088,#54089),(#54090,#54091),(#54092,#54093),(#54094,#54095),(#54096,
#54097),(#54098,#54099),(#54100,#54101),(#54102,#54103),(#54104,#54105),
(#54106,#54107),(#54108,#54109),(#54110,#54111),(#54112,#54113),(#54114,
#54115),(#54116,#54117),(#54118,#54119),(#54120,#54121),(#54122,#54123),
(#54124,#54125),(#54126,#54127),(#54128,#54129),(#54130,#54131),(#54132,
#54133),(#54134,#54135),(#54136,#54137),(#54138,#54139),(#54140,#54141),
(#54142,#54143),(#54144,#54145),(#54146,#54147),(#54148,#54149),(#54150,
#54151),(#54152,#54153),(#54154,#54155),(#54156,#54157),(#54158,#54159),
(#54160,#54161),(#54162,#54163),(#54164,#54165),(#54166,#54167),(#54168,
#54169),(#54170,#54171),(#54172,#54173),(#54174,#54175),(#54176,#54177),
(#54178,#54179),(#54180,#54181),(#54182,#54183),(#54184,#54185),(#54186,
#54187),(#54188,#54189),(#54190,#54191),(#54192,#54193),(#54194,#54195),
(#54196,#54197),(#54198,#54199),(#54200,#54201),(#54202,#54203),(#54204,
#54205),(#54206,#54207),(#54208,#54209),(#54210,#54211),(#54212,#54213),
(#54214,#54215),(#54216,#54217),(#54218,#54219),(#54220,#54221),(#54222,
#54223),(#54224,#54225),(#54226,#54227),(#54228,#54229),(#54230,#54231),
(#54232,#54233),(#54234,#54235),(#54236,#54237),(#54238,#54239),(#54240,
#54241),(#54242,#54243),(#54244,#54245),(#54246,#54247),(#54248,#54249),
(#54250,#54251),(#54252,#54253),(#54254,#54255),(#54256,#54257),(#54258,
#54259),(#54260,#54261),(#54262,#54263),(#54264,#54265),(#54266,#54267),
(#54268,#54269),(#54270,#54271),(#54272,#54273),(#54274,#54275),(#54276,
#54277),(#54278,#54279),(#54280,#54281),(#54282,#54283),(#54284,#54285),
(#54286,#54287),(#54288,#54289),(#54290,#54291),(#54292,#54293),(#54294,
#54295),(#54296,#54297),(#54298,#54299),(#54300,#54301),(#54302,#54303),
(#54304,#54305),(#54306,#54307),(#54308,#54309),(#54310,#54311),(#54312,
#54313),(#54314,#54315),(#54316,#54317),(#54318,#54319),(#54320,#54321),
(#54322,#54323),(#54324,#54325),(#54326,#54327),(#54328,#54329),(#54330,
#54331),(#54332,#54333),(#54334,#54335),(#54336,#54337),(#54338,#54339),
(#54340,#54341),(#54342,#54343),(#54344,#54345),(#54346,#54347),(#54348,
#54349),(#54350,#54351),(#54352,#54353),(#54354,#54355),(#54356,#54357),
(#54358,#54359),(#54360,#54361),(#54362,#54363),(#54364,#54365),(#54366,
#54367),(#54368,#54369),(#54370,#54371),(#54372,#54373),(#54374,#54375),
(#54376,#54377),(#54378,#54379),(#54380,#54381),(#54382,#54383),(#54384,
#54385),(#54386,#54387),(#54388,#54389),(#54390,#54391),(#54392,#54393),
(#54394,#54395),(#54396,#54397),(#54398,#54399),(#54400,#54401),(#54402,
#54403),(#54404,#54405),(#54406,#54407),(#54408,#54409),(#54410,#54411),
(#54412,#54413),(#54414,#54415),(#54416,#54417),(#54418,#54419),(#54420,
#54421),(#54422,#54423),(#54424,#54425),(#54426,#54427),(#54428,#54429),
(#54430,#54431),(#54432,#54433),(#54434,#54435),(#54436,#54437),(#54438,
#54439),(#54440,#54441),(#54442,#54443),(#54444,#54445),(#54446,#54447),
(#54448,#54449),(#54450,#54451),(#54452,#54453),(#54454,#54455),(#54456,
#54457),(#54458,#54459),(#54460,#54461),(#54462,#54463),(#54464,#54465),
(#54466,#54467),(#54468,#54469),(#54470,#54471),(#54472,#54473),(#54474,
#54475),(#54476,#54477),(#54478,#54479),(#54480,#54481),(#54482,#54483),
(#54484,#54485),(#54486,#54487),(#54488,#54489),(#54490,#54491),(#54492,
#54493),(#54494,#54495),(#54496,#54497),(#54498,#54499),(#54500,#54501),
(#54502,#54503),(#54504,#54505),(#54506,#54507),(#54508,#54509),(#54510,
#54511),(#54512,#54513),(#54514,#54515),(#54516,#54517),(#54518,#54519),
(#54520,#54521),(#54522,#54523),(#54524,#54525),(#54526,#54527),(#54528,
#54529),(#54530,#54531),(#54532,#54533),(#54534,#54535),(#54536,#54537),
(#54538,#54539),(#54540,#54541),(#54542,#54543),(#54544,#54545),(#54546,
#54547),(#54548,#54549),(#54550,#54551),(#54552,#54553),(#54554,#54555),
(#54556,#54557),(#54558,#54559),(#54560,#54561),(#54562,#54563),(#54564,
#54565),(#54566,#54567),(#54568,#54569),(#54570,#54571),(#54572,#54573),
(#54574,#54575),(#54576,#54577),(#54578,#54579),(#54580,#54581),(#54582,
#54583),(#54584,#54585),(#54586,#54587),(#54588,#54589),(#54590,#54591),
(#54592,#54593),(#54594,#54595),(#54596,#54597),(#54598,#54599),(#54600,
#54601),(#54602,#54603),(#54604,#54605),(#54606,#54607),(#54608,#54609),
(#54610,#54611),(#54612,#54613),(#54614,#54615),(#54616,#54617),(#54618,
#54619),(#54620,#54621),(#54622,#54623),(#54624,#54625),(#54626,#54627),
(#54628,#54629),(#54630,#54631),(#54632,#54633),(#54634,#54635),(#54636,
#54637),(#54638,#54639),(#54640,#54641),(#54642,#54643),(#54644,#54645),
(#54646,#54647),(#54648,#54649),(#54650,#54651),(#54652,#54653),(#54654,
#54655),(#54656,#54657),(#54658,#54659),(#54660,#54661),(#54662,#54663),
(#54664,#54665),(#54666,#54667),(#54668,#54669),(#54670,#54671),(#54672,
#54673),(#54674,#54675),(#54676,#54677),(#54678,#54679),(#54680,#54681),
(#54682,#54683),(#54684,#54685),(#54686,#54687),(#54688,#54689),(#54690,
#54691),(#54692,#54693),(#54694,#54695),(#54696,#54697),(#54698,#54699),
(#54700,#54701),(#54702,#54703),(#54704,#54705),(#54706,#54707),(#54708,
#54709),(#54710,#54711),(#54712,#54713),(#54714,#54715),(#54716,#54717),
(#54718,#54719),(#54720,#54721),(#54722,#54723),(#54724,#54725),(#54726,
#54727),(#54728,#54729),(#54730,#54731),(#54732,#54733),(#54734,#54735),
(#54736,#54737),(#54738,#54739),(#54740,#54741),(#54742,#54743),(#54744,
#54745),(#54746,#54747),(#54748,#54749),(#54750,#54751),(#54752,#54753),
(#54754,#54755),(#54756,#54757),(#54758,#54759),(#54760,#54761),(#54762,
#54763),(#54764,#54765),(#54766,#54767),(#54768,#54769),(#54770,#54771),
(#54772,#54773),(#54774,#54775),(#54776,#54777),(#54778,#54779),(#54780,
#54781),(#54782,#54783),(#54784,#54785),(#54786,#54787),(#54788,#54789),
(#54790,#54791),(#54792,#54793),(#54794,#54795),(#54796,#54797),(#54798,
#54799),(#54800,#54801),(#54802,#54803),(#54804,#54805),(#54806,#54807),
(#54808,#54809),(#54810,#54811),(#54812,#54813),(#54814,#54815),(#54816,
#54817),(#54818,#54819),(#54820,#54821),(#54822,#54823),(#54824,#54825),
(#54826,#54827),(#54828,#54829),(#54830,#54831),(#54832,#54833),(#54834,
#54835),(#54836,#54837),(#54838,#54839),(#54840,#54841),(#54842,#54843),
(#54844,#54845),(#54846,#54847),(#54848,#54849),(#54850,#54851),(#54852,
#54853),(#54854,#54855),(#54856,#54857),(#54858,#54859),(#54860,#54861),
(#54862,#54863),(#54864,#54865),(#54866,#54867),(#54868,#54869),(#54870,
#54871),(#54872,#54873),(#54874,#54875),(#54876,#54877),(#54878,#54879),
(#54880,#54881),(#54882,#54883),(#54884,#54885),(#54886,#54887),(#54888,
#54889),(#54890,#54891),(#54892,#54893),(#54894,#54895),(#54896,#54897),
(#54898,#54899),(#54900,#54901),(#54902,#54903),(#54904,#54905),(#54906,
#54907),(#54908,#54909),(#54910,#54911),(#54912,#54913),(#54914,#54915),
(#54916,#54917),(#54918,#54919),(#54920,#54921),(#54922,#54923),(#54924,
#54925),(#54926,#54927),(#54928,#54929),(#54930,#54931),(#54932,#54933),
(#54934,#54935),(#54936,#54937),(#54938,#54939),(#54940,#54941),(#54942,
#54943),(#54944,#54945),(#54946,#54947),(#54948,#54949),(#54950,#54951),
(#54952,#54953),(#54954,#54955),(#54956,#54957),(#54958,#54959),(#54960,
#54961),(#54962,#54963),(#54964,#54965),(#54966,#54967),(#54968,#54969),
(#54970,#54971),(#54972,#54973),(#54974,#54975),(#54976,#54977),(#54978,
#54979),(#54980,#54981),(#54982,#54983),(#54984,#54985),(#54986,#54987),
(#54988,#54989),(#54990,#54991),(#54992,#54993),(#54994,#54995),(#54996,
#54997),(#54998,#54999),(#55000,#55001),(#55002,#55003),(#55004,#55005),
(#55006,#55007),(#55008,#55009),(#55010,#55011),(#55012,#55013),(#55014,
#55015),(#55016,#55017),(#55018,#55019),(#55020,#55021),(#55022,#55023),
(#55024,#55025),(#55026,#55027),(#55028,#55029),(#55030,#55031),(#55032,
#55033),(#55034,#55035),(#55036,#55037),(#55038,#55039),(#55040,#55041),
(#55042,#55043),(#55044,#55045),(#55046,#55047),(#55048,#55049),(#55050,
#55051),(#55052,#55053),(#55054,#55055),(#55056,#55057),(#55058,#55059),
(#55060,#55061),(#55062,#55063),(#55064,#55065),(#55066,#55067),(#55068,
#55069),(#55070,#55071),(#55072,#55073),(#55074,#55075),(#55076,#55077),
(#55078,#55079),(#55080,#55081),(#55082,#55083),(#55084,#55085),(#55086,
#55087),(#55088,#55089),(#55090,#55091),(#55092,#55093),(#55094,#55095),
(#55096,#55097),(#55098,#55099),(#55100,#55101),(#55102,#55103),(#55104,
#55105),(#55106,#55107),(#55108,#55109),(#55110,#55111),(#55112,#55113),
(#55114,#55115),(#55116,#55117),(#55118,#55119),(#55120,#55121),(#55122,
#55123),(#55124,#55125),(#55126,#55127),(#55128,#55129),(#55130,#55131),
(#55132,#55133),(#55134,#55135),(#55136,#55137),(#55138,#55139),(#55140,
#55141),(#55142,#55143),(#55144,#55145),(#55146,#55147),(#55148,#55149),
(#55150,#55151),(#55152,#55153),(#55154,#55155),(#55156,#55157),(#55158,
#55159),(#55160,#55161),(#55162,#55163),(#55164,#55165),(#55166,#55167),
(#55168,#55169),(#55170,#55171),(#55172,#55173),(#55174,#55175),(#55176,
#55177),(#55178,#55179),(#55180,#55181),(#55182,#55183),(#55184,#55185),
(#55186,#55187),(#55188,#55189),(#55190,#55191),(#55192,#55193),(#55194,
#55195),(#55196,#55197),(#55198,#55199),(#55200,#55201),(#55202,#55203),
(#55204,#55205),(#55206,#55207),(#55208,#55209),(#55210,#55211),(#55212,
#55213),(#55214,#55215),(#55216,#55217),(#55218,#55219),(#55220,#55221),
(#55222,#55223),(#55224,#55225),(#55226,#55227),(#55228,#55229),(#55230,
#55231),(#55232,#55233),(#55234,#55235),(#55236,#55237),(#55238,#55239),
(#55240,#55241),(#55242,#55243),(#55244,#55245),(#55246,#55247),(#55248,
#55249),(#55250,#55251),(#55252,#55253),(#55254,#55255),(#55256,#55257),
(#55258,#55259),(#55260,#55261),(#55262,#55263),(#55264,#55265),(#55266,
#55267),(#55268,#55269),(#55270,#55271),(#55272,#55273),(#55274,#55275),
(#55276,#55277),(#55278,#55279),(#55280,#55281),(#55282,#55283),(#55284,
#55285),(#55286,#55287),(#55288,#55289),(#55290,#55291),(#55292,#55293),
(#55294,#55295),(#55296,#55297),(#55298,#55299),(#55300,#55301),(#55302,
#55303),(#55304,#55305),(#55306,#55307),(#55308,#55309),(#55310,#55311),
(#55312,#55313),(#55314,#55315),(#55316,#55317),(#55318,#55319),(#55320,
#55321),(#55322,#55323),(#55324,#55325),(#55326,#55327),(#55328,#55329),
(#55330,#55331),(#55332,#55333),(#55334,#55335),(#55336,#55337),(#55338,
#55339),(#55340,#55341),(#55342,#55343),(#55344,#55345),(#55346,#55347),
(#55348,#55349),(#55350,#55351),(#55352,#55353),(#55354,#55355),(#55356,
#55357),(#55358,#55359),(#55360,#55361),(#55362,#55363),(#55364,#55365),
(#55366,#55367),(#55368,#55369),(#55370,#55371),(#55372,#55373),(#55374,
#55375),(#55376,#55377),(#55378,#55379),(#55380,#55381),(#55382,#55383),
(#55384,#55385),(#55386,#55387),(#55388,#55389),(#55390,#55391),(#55392,
#55393),(#55394,#55395),(#55396,#55397),(#55398,#55399),(#55400,#55401),
(#55402,#55403),(#55404,#55405),(#55406,#55407),(#55408,#55409),(#55410,
#55411),(#55412,#55413),(#55414,#55415),(#55416,#55417),(#55418,#55419),
(#55420,#55421),(#55422,#55423),(#55424,#55425),(#55426,#55427),(#55428,
#55429),(#55430,#55431),(#55432,#55433),(#55434,#55435),(#55436,#55437),
(#55438,#55439),(#55440,#55441),(#55442,#55443),(#55444,#55445),(#55446,
#55447),(#55448,#55449),(#55450,#55451),(#55452,#55453),(#55454,#55455),
(#55456,#55457),(#55458,#55459),(#55460,#55461),(#55462,#55463),(#55464,
#55465),(#55466,#55467),(#55468,#55469),(#55470,#55471),(#55472,#55473),
(#55474,#55475),(#55476,#55477),(#55478,#55479),(#55480,#55481),(#55482,
#55483),(#55484,#55485),(#55486,#55487),(#55488,#55489),(#55490,#55491),
(#55492,#55493),(#55494,#55495),(#55496,#55497),(#55498,#55499),(#55500,
#55501),(#55502,#55503),(#55504,#55505),(#55506,#55507),(#55508,#55509),
(#55510,#55511),(#55512,#55513),(#55514,#55515),(#55516,#55517),(#55518,
#55519),(#55520,#55521),(#55522,#55523),(#55524,#55525),(#55526,#55527),
(#55528,#55529),(#55530,#55531),(#55532,#55533),(#55534,#55535),(#55536,
#55537),(#55538,#55539),(#55540,#55541),(#55542,#55543),(#55544,#55545),
(#55546,#55547),(#55548,#55549),(#55550,#55551),(#55552,#55553),(#55554,
#55555),(#55556,#55557),(#55558,#55559),(#55560,#55561),(#55562,#55563),
(#55564,#55565),(#55566,#55567),(#55568,#55569),(#55570,#55571),(#55572,
#55573),(#55574,#55575),(#55576,#55577),(#55578,#55579),(#55580,#55581),
(#55582,#55583),(#55584,#55585),(#55586,#55587),(#55588,#55589),(#55590,
#55591),(#55592,#55593),(#55594,#55595),(#55596,#55597),(#55598,#55599),
(#55600,#55601),(#55602,#55603),(#55604,#55605),(#55606,#55607),(#55608,
#55609),(#55610,#55611),(#55612,#55613),(#55614,#55615),(#55616,#55617),
(#55618,#55619),(#55620,#55621),(#55622,#55623),(#55624,#55625),(#55626,
#55627),(#55628,#55629),(#55630,#55631),(#55632,#55633),(#55634,#55635),
(#55636,#55637),(#55638,#55639),(#55640,#55641),(#55642,#55643),(#55644,
#55645),(#55646,#55647),(#55648,#55649),(#55650,#55651),(#55652,#55653),
(#55654,#55655),(#55656,#55657),(#55658,#55659),(#55660,#55661),(#55662,
#55663),(#55664,#55665),(#55666,#55667),(#55668,#55669),(#55670,#55671),
(#55672,#55673),(#55674,#55675),(#55676,#55677),(#55678,#55679),(#55680,
#55681),(#55682,#55683),(#55684,#55685),(#55686,#55687),(#55688,#55689),
(#55690,#55691),(#55692,#55693),(#55694,#55695),(#55696,#55697),(#55698,
#55699),(#55700,#55701),(#55702,#55703),(#55704,#55705),(#55706,#55707),
(#55708,#55709),(#55710,#55711),(#55712,#55713),(#55714,#55715),(#55716,
#55717),(#55718,#55719),(#55720,#55721),(#55722,#55723),(#55724,#55725),
(#55726,#55727),(#55728,#55729),(#55730,#55731),(#55732,#55733),(#55734,
#55735),(#55736,#55737),(#55738,#55739),(#55740,#55741),(#55742,#55743),
(#55744,#55745),(#55746,#55747),(#55748,#55749),(#55750,#55751),(#55752,
#55753),(#55754,#55755),(#55756,#55757),(#55758,#55759),(#55760,#55761),
(#55762,#55763),(#55764,#55765),(#55766,#55767),(#55768,#55769),(#55770,
#55771),(#55772,#55773),(#55774,#55775),(#55776,#55777),(#55778,#55779),
(#55780,#55781),(#55782,#55783),(#55784,#55785),(#55786,#55787),(#55788,
#55789),(#55790,#55791),(#55792,#55793),(#55794,#55795),(#55796,#55797),
(#55798,#55799),(#55800,#55801),(#55802,#55803),(#55804,#55805),(#55806,
#55807),(#55808,#55809),(#55810,#55811),(#55812,#55813),(#55814,#55815),
(#55816,#55817),(#55818,#55819),(#55820,#55821),(#55822,#55823),(#55824,
#55825),(#55826,#55827),(#55828,#55829),(#55830,#55831),(#55832,#55833),
(#55834,#55835),(#55836,#55837),(#55838,#55839),(#55840,#55841),(#55842,
#55843),(#55844,#55845),(#55846,#55847),(#55848,#55849),(#55850,#55851),
(#55852,#55853),(#55854,#55855),(#55856,#55857),(#55858,#55859),(#55860,
#55861),(#55862,#55863),(#55864,#55865),(#55866,#55867),(#55868,#55869),
(#55870,#55871),(#55872,#55873),(#55874,#55875),(#55876,#55877),(#55878,
#55879),(#55880,#55881),(#55882,#55883),(#55884,#55885),(#55886,#55887),
(#55888,#55889),(#55890,#55891),(#55892,#55893),(#55894,#55895),(#55896,
#55897),(#55898,#55899),(#55900,#55901),(#55902,#55903),(#55904,#55905),
(#55906,#55907),(#55908,#55909),(#55910,#55911),(#55912,#55913),(#55914,
#55915),(#55916,#55917),(#55918,#55919),(#55920,#55921),(#55922,#55923),
(#55924,#55925),(#55926,#55927),(#55928,#55929),(#55930,#55931),(#55932,
#55933),(#55934,#55935),(#55936,#55937),(#55938,#55939),(#55940,#55941),
(#55942,#55943),(#55944,#55945),(#55946,#55947),(#55948,#55949),(#55950,
#55951),(#55952,#55953),(#55954,#55955),(#55956,#55957),(#55958,#55959),
(#55960,#55961),(#55962,#55963),(#55964,#55965),(#55966,#55967),(#55968,
#55969),(#55970,#55971),(#55972,#55973),(#55974,#55975),(#55976,#55977),
(#55978,#55979),(#55980,#55981),(#55982,#55983),(#55984,#55985),(#55986,
#55987),(#55988,#55989),(#55990,#55991),(#55992,#55993),(#55994,#55995),
(#55996,#55997),(#55998,#55999),(#56000,#56001),(#56002,#56003),(#56004,
#56005),(#56006,#56007),(#56008,#56009),(#56010,#56011),(#56012,#56013),
(#56014,#56015),(#56016,#56017),(#56018,#56019),(#56020,#56021),(#56022,
#56023),(#56024,#56025),(#56026,#56027),(#56028,#56029),(#56030,#56031),
(#56032,#56033),(#56034,#56035),(#56036,#56037),(#56038,#56039),(#56040,
#56041),(#56042,#56043),(#56044,#56045),(#56046,#56047),(#56048,#56049),
(#56050,#56051),(#56052,#56053),(#56054,#56055),(#56056,#56057),(#56058,
#56059),(#56060,#56061),(#56062,#56063),(#56064,#56065),(#56066,#56067),
(#56068,#56069),(#56070,#56071),(#56072,#56073),(#56074,#56075),(#56076,
#56077),(#56078,#56079),(#56080,#56081),(#56082,#56083),(#56084,#56085),
(#56086,#56087),(#56088,#56089),(#56090,#56091),(#56092,#56093),(#56094,
#56095),(#56096,#56097),(#56098,#56099),(#56100,#56101),(#56102,#56103),
(#56104,#56105),(#56106,#56107),(#56108,#56109),(#56110,#56111),(#56112,
#56113),(#56114,#56115),(#56116,#56117),(#56118,#56119),(#56120,#56121),
(#56122,#56123),(#56124,#56125),(#56126,#56127),(#56128,#56129),(#56130,
#56131),(#56132,#56133),(#56134,#56135),(#56136,#56137),(#56138,#56139),
(#56140,#56141),(#56142,#56143),(#56144,#56145),(#56146,#56147),(#56148,
#56149),(#56150,#56151),(#56152,#56153),(#56154,#56155),(#56156,#56157),
(#56158,#56159),(#56160,#56161),(#56162,#56163),(#56164,#56165),(#56166,
#56167),(#56168,#56169),(#56170,#56171),(#56172,#56173),(#56174,#56175),
(#56176,#56177),(#56178,#56179),(#56180,#56181),(#56182,#56183),(#56184,
#56185),(#56186,#56187),(#56188,#56189),(#56190,#56191),(#56192,#56193),
(#56194,#56195),(#56196,#56197),(#56198,#56199),(#56200,#56201),(#56202,
#56203),(#56204,#56205),(#56206,#56207),(#56208,#56209),(#56210,#56211),
(#56212,#56213),(#56214,#56215),(#56216,#56217),(#56218,#56219),(#56220,
#56221),(#56222,#56223),(#56224,#56225),(#56226,#56227),(#56228,#56229),
(#56230,#56231),(#56232,#56233),(#56234,#56235),(#56236,#56237),(#56238,
#56239),(#56240,#56241),(#56242,#56243),(#56244,#56245),(#56246,#56247),
(#56248,#56249),(#56250,#56251),(#56252,#56253),(#56254,#56255),(#56256,
#56257),(#56258,#56259),(#56260,#56261),(#56262,#56263),(#56264,#56265),
(#56266,#56267),(#56268,#56269),(#56270,#56271),(#56272,#56273),(#56274,
#56275),(#56276,#56277),(#56278,#56279),(#56280,#56281),(#56282,#56283),
(#56284,#56285),(#56286,#56287),(#56288,#56289),(#56290,#56291),(#56292,
#56293),(#56294,#56295),(#56296,#56297),(#56298,#56299),(#56300,#56301),
(#56302,#56303),(#56304,#56305),(#56306,#56307),(#56308,#56309),(#56310,
#56311),(#56312,#56313),(#56314,#56315),(#56316,#56317),(#56318,#56319),
(#56320,#56321),(#56322,#56323),(#56324,#56325),(#56326,#56327),(#56328,
#56329),(#56330,#56331),(#56332,#56333),(#56334,#56335),(#56336,#56337),
(#56338,#56339),(#56340,#56341),(#56342,#56343),(#56344,#56345),(#56346,
#56347),(#56348,#56349),(#56350,#56351),(#56352,#56353),(#56354,#56355),
(#56356,#56357),(#56358,#56359),(#56360,#56361),(#56362,#56363),(#56364,
#56365),(#56366,#56367),(#56368,#56369),(#56370,#56371),(#56372,#56373),
(#56374,#56375),(#56376,#56377),(#56378,#56379),(#56380,#56381),(#56382,
#56383),(#56384,#56385),(#56386,#56387),(#56388,#56389),(#56390,#56391),
(#56392,#56393),(#56394,#56395),(#56396,#56397),(#56398,#56399),(#56400,
#56401),(#56402,#56403),(#56404,#56405),(#56406,#56407),(#56408,#56409),
(#56410,#56411),(#56412,#56413),(#56414,#56415),(#56416,#56417),(#56418,
#56419),(#56420,#56421),(#56422,#56423),(#56424,#56425),(#56426,#56427),
(#56428,#56429),(#56430,#56431),(#56432,#56433),(#56434,#56435),(#56436,
#56437),(#56438,#56439),(#56440,#56441),(#56442,#56443),(#56444,#56445),
(#56446,#56447),(#56448,#56449),(#56450,#56451),(#56452,#56453),(#56454,
#56455),(#56456,#56457),(#56458,#56459),(#56460,#56461),(#56462,#56463),
(#56464,#56465),(#56466,#56467),(#56468,#56469),(#56470,#56471),(#56472,
#56473),(#56474,#56475),(#56476,#56477),(#56478,#56479),(#56480,#56481),
(#56482,#56483),(#56484,#56485),(#56486,#56487),(#56488,#56489),(#56490,
#56491),(#56492,#56493),(#56494,#56495),(#56496,#56497),(#56498,#56499),
(#56500,#56501),(#56502,#56503),(#56504,#56505),(#56506,#56507),(#56508,
#56509),(#56510,#56511),(#56512,#56513),(#56514,#56515),(#56516,#56517),
(#56518,#56519),(#56520,#56521),(#56522,#56523),(#56524,#56525),(#56526,
#56527),(#56528,#56529),(#56530,#56531),(#56532,#56533),(#56534,#56535),
(#56536,#56537),(#56538,#56539),(#56540,#56541),(#56542,#56543),(#56544,
#56545),(#56546,#56547),(#56548,#56549),(#56550,#56551),(#56552,#56553),
(#56554,#56555),(#56556,#56557),(#56558,#56559),(#56560,#56561),(#56562,
#56563),(#56564,#56565),(#56566,#56567),(#56568,#56569),(#56570,#56571),
(#56572,#56573),(#56574,#56575),(#56576,#56577),(#56578,#56579),(#56580,
#56581),(#56582,#56583),(#56584,#56585),(#56586,#56587),(#56588,#56589),
(#56590,#56591),(#56592,#56593),(#56594,#56595),(#56596,#56597),(#56598,
#56599),(#56600,#56601),(#56602,#56603),(#56604,#56605),(#56606,#56607),
(#56608,#56609),(#56610,#56611),(#56612,#56613),(#56614,#56615),(#56616,
#56617),(#56618,#56619),(#56620,#56621),(#56622,#56623),(#56624,#56625),
(#56626,#56627),(#56628,#56629),(#56630,#56631),(#56632,#56633),(#56634,
#56635),(#56636,#56637),(#56638,#56639),(#56640,#56641),(#56642,#56643),
(#56644,#56645),(#56646,#56647),(#56648,#56649),(#56650,#56651),(#56652,
#56653),(#56654,#56655),(#56656,#56657),(#56658,#56659),(#56660,#56661),
(#56662,#56663),(#56664,#56665),(#56666,#56667),(#56668,#56669),(#56670,
#56671),(#56672,#56673),(#56674,#56675),(#56676,#56677),(#56678,#56679),
(#56680,#56681),(#56682,#56683),(#56684,#56685),(#56686,#56687),(#56688,
#56689),(#56690,#56691),(#56692,#56693),(#56694,#56695),(#56696,#56697),
(#56698,#56699),(#56700,#56701),(#56702,#56703),(#56704,#56705),(#56706,
#56707),(#56708,#56709),(#56710,#56711),(#56712,#56713),(#56714,#56715),
(#56716,#56717),(#56718,#56719),(#56720,#56721),(#56722,#56723),(#56724,
#56725),(#56726,#56727),(#56728,#56729),(#56730,#56731),(#56732,#56733),
(#56734,#56735),(#56736,#56737),(#56738,#56739),(#56740,#56741),(#56742,
#56743),(#56744,#56745),(#56746,#56747),(#56748,#56749),(#56750,#56751),
(#56752,#56753),(#56754,#56755),(#56756,#56757),(#56758,#56759),(#56760,
#56761),(#56762,#56763),(#56764,#56765),(#56766,#56767),(#56768,#56769),
(#56770,#56771),(#56772,#56773),(#56774,#56775),(#56776,#56777),(#56778,
#56779),(#56780,#56781),(#56782,#56783),(#56784,#56785),(#56786,#56787),
(#56788,#56789),(#56790,#56791),(#56792,#56793),(#56794,#56795),(#56796,
#56797),(#56798,#56799),(#56800,#56801),(#56802,#56803),(#56804,#56805),
(#56806,#56807),(#56808,#56809),(#56810,#56811),(#56812,#56813),(#56814,
#56815),(#56816,#56817),(#56818,#56819),(#56820,#56821),(#56822,#56823),
(#56824,#56825),(#56826,#56827),(#56828,#56829),(#56830,#56831),(#56832,
#56833),(#56834,#56835),(#56836,#56837),(#56838,#56839),(#56840,#56841),
(#56842,#56843),(#56844,#56845),(#56846,#56847),(#56848,#56849),(#56850,
#56851),(#56852,#56853),(#56854,#56855),(#56856,#56857),(#56858,#56859),
(#56860,#56861),(#56862,#56863),(#56864,#56865),(#56866,#56867),(#56868,
#56869),(#56870,#56871),(#56872,#56873),(#56874,#56875),(#56876,#56877),
(#56878,#56879),(#56880,#56881),(#56882,#56883),(#56884,#56885),(#56886,
#56887),(#56888,#56889),(#56890,#56891),(#56892,#56893),(#56894,#56895),
(#56896,#56897),(#56898,#56899),(#56900,#56901),(#56902,#56903),(#56904,
#56905),(#56906,#56907),(#56908,#56909),(#56910,#56911),(#56912,#56913),
(#56914,#56915),(#56916,#56917),(#56918,#56919),(#56920,#56921),(#56922,
#56923),(#56924,#56925),(#56926,#56927),(#56928,#56929),(#56930,#56931),
(#56932,#56933),(#56934,#56935),(#56936,#56937),(#56938,#56939),(#56940,
#56941),(#56942,#56943),(#56944,#56945),(#56946,#56947),(#56948,#56949),
(#56950,#56951),(#56952,#56953),(#56954,#56955),(#56956,#56957),(#56958,
#56959),(#56960,#56961),(#56962,#56963),(#56964,#56965),(#56966,#56967),
(#56968,#56969),(#56970,#56971),(#56972,#56973),(#56974,#56975),(#56976,
#56977),(#56978,#56979),(#56980,#56981),(#56982,#56983),(#56984,#56985),
(#56986,#56987),(#56988,#56989),(#56990,#56991),(#56992,#56993),(#56994,
#56995),(#56996,#56997),(#56998,#56999),(#57000,#57001),(#57002,#57003),
(#57004,#57005),(#57006,#57007),(#57008,#57009),(#57010,#57011),(#57012,
#57013),(#57014,#57015),(#57016,#57017),(#57018,#57019),(#57020,#57021),
(#57022,#57023),(#57024,#57025),(#57026,#57027),(#57028,#57029),(#57030,
#57031),(#57032,#57033),(#57034,#57035),(#57036,#57037),(#57038,#57039),
(#57040,#57041),(#57042,#57043),(#57044,#57045),(#57046,#57047),(#57048,
#57049),(#57050,#57051),(#57052,#57053),(#57054,#57055),(#57056,#57057),
(#57058,#57059),(#57060,#57061),(#57062,#57063),(#57064,#57065),(#57066,
#57067),(#57068,#57069),(#57070,#57071),(#57072,#57073),(#57074,#57075),
(#57076,#57077),(#57078,#57079),(#57080,#57081),(#57082,#57083),(#57084,
#57085),(#57086,#57087),(#57088,#57089),(#57090,#57091),(#57092,#57093),
(#57094,#57095),(#57096,#57097),(#57098,#57099),(#57100,#57101),(#57102,
#57103),(#57104,#57105),(#57106,#57107),(#57108,#57109),(#57110,#57111),
(#57112,#57113),(#57114,#57115),(#57116,#57117),(#57118,#57119),(#57120,
#57121),(#57122,#57123),(#57124,#57125),(#57126,#57127),(#57128,#57129),
(#57130,#57131),(#57132,#57133),(#57134,#57135),(#57136,#57137),(#57138,
#57139),(#57140,#57141),(#57142,#57143),(#57144,#57145),(#57146,#57147),
(#57148,#57149),(#57150,#57151),(#57152,#57153),(#57154,#57155),(#57156,
#57157),(#57158,#57159),(#57160,#57161),(#57162,#57163),(#57164,#57165),
(#57166,#57167),(#57168,#57169),(#57170,#57171),(#57172,#57173),(#57174,
#57175),(#57176,#57177),(#57178,#57179),(#57180,#57181),(#57182,#57183),
(#57184,#57185),(#57186,#57187),(#57188,#57189),(#57190,#57191),(#57192,
#57193),(#57194,#57195),(#57196,#57197),(#57198,#57199),(#57200,#57201),
(#57202,#57203),(#57204,#57205),(#57206,#57207),(#57208,#57209),(#57210,
#57211),(#57212,#57213),(#57214,#57215),(#57216,#57217),(#57218,#57219),
(#57220,#57221),(#57222,#57223),(#57224,#57225),(#57226,#57227),(#57228,
#57229),(#57230,#57231),(#57232,#57233),(#57234,#57235),(#57236,#57237),
(#57238,#57239),(#57240,#57241),(#57242,#57243),(#57244,#57245),(#57246,
#57247),(#57248,#57249),(#57250,#57251),(#57252,#57253),(#57254,#57255),
(#57256,#57257),(#57258,#57259),(#57260,#57261),(#57262,#57263),(#57264,
#57265),(#57266,#57267),(#57268,#57269),(#57270,#57271),(#57272,#57273)),
 .UNSPECIFIED.,.F.,.F.,.F.,(4,1,1,1,1,1,1,1,1,1,1,1,1,1,1,1,1,1,1,1,1,1,
1,1,1,1,1,1,1,1,1,1,1,1,1,1,1,1,1,1,1,1,1,1,1,1,1,1,1,1,1,1,1,1,1,1,1,1,
1,1,1,1,1,1,1,1,1,1,1,1,1,1,1,1,1,1,1,1,1,1,1,1,1,1,1,1,1,1,1,1,1,1,1,1,
1,1,1,1,1,1,1,1,1,1,1,1,1,1,1,1,1,1,1,1,1,1,1,1,1,1,1,1,1,1,1,1,1,1,1,1,
1,1,1,1,1,1,1,1,1,1,1,1,1,1,1,1,1,1,1,1,1,1,1,1,1,1,1,1,1,1,1,1,1,1,1,1,
1,1,1,1,1,1,1,1,1,1,1,1,1,1,1,1,1,1,1,1,1,1,1,1,1,1,1,1,1,1,1,1,1,1,1,1,
1,1,1,1,1,1,1,1,1,1,1,1,1,1,1,1,1,1,1,1,1,1,1,1,1,1,1,1,1,1,1,1,1,1,1,1,
1,1,1,1,1,1,1,1,1,1,1,1,1,1,1,1,1,1,1,1,1,1,1,1,1,1,1,1,1,1,1,1,1,1,1,1,
1,1,1,1,1,1,1,1,1,1,1,1,1,1,1,1,1,1,1,1,1,1,1,1,1,1,1,1,1,1,1,1,1,1,1,1,
1,1,1,1,1,1,1,1,1,1,1,1,1,1,1,1,1,1,1,1,1,1,1,1,1,1,1,1,1,1,1,1,1,1,1,1,
1,1,1,1,1,1,1,1,1,1,1,1,1,1,1,1,1,1,1,1,1,1,1,1,1,1,1,1,1,1,1,1,1,1,1,1,
1,1,1,1,1,1,1,1,1,1,1,1,1,1,1,1,1,1,1,1,1,1,1,1,1,1,1,1,1,1,1,1,1,1,1,1,
1,1,1,1,1,1,1,1,1,1,1,1,1,1,1,1,1,1,1,1,1,1,1,1,1,1,1,1,1,1,1,1,1,1,1,1,
1,1,1,1,1,1,1,1,1,1,1,1,1,1,1,1,1,1,1,1,1,1,1,1,1,1,1,1,1,1,1,1,1,1,1,1,
1,1,1,1,1,1,1,1,1,1,1,1,1,1,1,1,1,1,1,1,1,1,1,1,1,1,1,1,1,1,1,1,1,1,1,1,
1,1,1,1,1,1,1,1,1,1,1,1,1,1,1,1,1,1,1,1,1,1,1,1,1,1,1,1,1,1,1,1,1,1,1,1,
1,1,1,1,1,1,1,1,1,1,1,1,1,1,1,1,1,1,1,1,1,1,1,1,1,1,1,1,1,1,1,1,1,1,1,1,
1,1,1,1,1,1,1,1,1,1,1,1,1,1,1,1,1,1,1,1,1,1,1,1,1,1,1,1,1,1,1,1,1,1,1,1,
1,1,1,1,1,1,1,1,1,1,1,1,1,1,1,1,1,1,1,1,1,1,1,1,1,1,1,1,1,1,1,1,1,1,1,1,
1,1,1,1,1,1,1,1,1,1,1,1,1,1,1,1,1,1,1,1,1,1,1,1,1,1,1,1,1,1,1,1,1,1,1,1,
1,1,1,1,1,1,1,1,1,1,1,1,1,1,1,1,1,1,1,1,1,1,1,1,1,1,1,1,1,1,1,1,1,1,1,1,
1,1,1,1,1,1,1,1,1,1,1,1,1,1,1,1,1,1,1,1,1,1,1,1,1,1,1,1,1,1,1,1,1,1,1,1,
1,1,1,1,1,1,1,1,1,1,1,1,1,1,1,1,1,1,1,1,1,1,1,1,1,1,1,1,1,1,1,1,1,1,1,1,
1,1,1,1,1,1,1,1,1,1,1,1,1,1,1,1,1,1,1,1,1,1,1,1,1,1,1,1,1,1,1,1,1,1,1,1,
1,1,1,1,1,1,1,1,1,1,1,1,1,1,1,1,1,1,1,1,1,1,1,1,1,1,1,1,1,1,1,1,1,1,1,1,
1,1,1,1,1,1,1,1,1,1,1,1,1,1,1,1,1,1,1,1,1,1,1,1,1,1,1,1,1,1,1,1,1,1,1,1,
1,1,1,1,1,1,1,1,1,1,1,1,1,1,1,1,1,1,1,1,1,1,1,1,1,1,1,1,1,1,1,1,1,1,1,1,
1,1,1,1,1,1,1,1,1,1,1,1,1,1,1,1,1,1,1,1,1,1,1,1,1,1,1,1,1,1,1,1,1,1,1,1,
1,1,1,1,1,1,1,1,1,1,1,1,1,1,1,1,1,1,1,1,1,1,1,1,1,1,1,1,1,1,1,1,1,1,1,1,
1,1,1,1,1,1,1,1,1,1,1,1,1,1,1,1,1,1,1,1,1,1,1,1,1,1,1,1,1,1,1,1,1,1,1,1,
1,1,1,1,1,1,1,1,1,1,1,1,1,1,1,1,1,1,1,1,1,1,1,1,1,1,1,1,1,1,1,1,1,1,1,1,
1,1,1,1,1,1,1,1,1,1,1,1,1,1,1,1,1,1,1,1,1,1,1,1,1,1,1,1,1,1,1,1,1,1,1,1,
1,1,1,1,1,1,1,1,1,1,1,1,1,1,1,1,1,1,1,1,1,1,1,1,1,1,1,1,1,1,1,1,1,1,1,1,
1,1,1,1,1,1,1,1,1,1,1,1,1,1,1,1,1,1,1,1,1,1,1,1,1,1,1,1,1,1,1,1,1,1,1,1,
1,1,1,1,1,1,1,1,1,1,1,1,1,1,1,1,1,1,1,1,1,1,1,1,1,1,1,1,1,1,1,1,1,1,1,1,
1,1,1,1,1,1,1,1,1,1,1,1,1,1,1,1,1,1,1,1,1,1,1,1,1,1,1,1,1,1,1,1,1,1,1,1,
1,1,1,1,1,1,1,1,1,1,1,1,1,1,1,1,1,1,1,1,1,1,1,1,1,1,1,1,1,1,1,1,1,1,1,1,
1,1,1,1,1,1,1,1,1,1,1,1,1,1,1,1,1,1,1,1,1,1,1,1,1,1,1,1,1,1,1,1,1,1,1,1,
1,1,1,1,1,1,1,1,1,1,1,1,1,1,1,1,1,1,1,1,1,1,1,1,1,1,1,1,1,1,1,1,1,1,1,1,
1,1,1,1,1,1,1,1,1,1,1,1,1,1,1,1,1,1,1,1,1,1,1,1,1,1,1,1,1,1,1,1,1,1,1,1,
1,1,1,1,1,1,1,1,1,1,1,1,1,1,1,1,1,1,1,1,1,1,1,1,1,1,1,1,1,1,1,1,1,1,1,1,
1,1,1,1,1,1,1,1,1,1,1,1,1,1,1,1,1,1,1,1,1,1,1,1,1,1,1,1,1,1,1,1,1,1,1,1,
1,1,1,1,1,1,1,1,1,1,1,1,1,1,1,1,1,1,1,1,1,1,1,1,1,1,1,1,1,1,1,1,1,1,1,1,
1,1,1,1,1,1,1,1,1,1,1,1,1,1,1,1,1,1,1,1,1,1,1,1,1,1,1,1,1,1,1,1,1,1,1,1,
1,1,1,1,1,1,1,1,1,1,1,1,1,1,1,1,1,1,1,1,1,1,1,1,1,1,1,1,1,1,1,1,1,1,1,1,
1,1,1,1,1,1,1,1,1,1,1,1,1,1,1,1,1,1,1,1,1,1,1,1,1,1,1,1,1,1,1,1,1,1,1,1,
1,1,1,1,1,1,1,1,1,1,1,1,1,1,1,1,1,1,1,1,1,1,1,1,1,1,1,1,1,1,1,1,1,1,1,1,
1,1,1,1,1,1,1,1,1,1,1,1,1,1,1,1,1,1,1,1,1,1,1,1,1,1,1,1,1,1,1,1,1,1,1,1,
1,1,1,1,1,1,1,1,1,1,1,1,1,1,1,1,1,1,1,1,1,1,1,1,1,1,1,1,1,1,1,1,1,1,1,1,
1,1,1,1,1,1,1,1,1,1,1,1,1,1,1,1,1,1,1,1,1,1,1,1,1,1,1,1,1,1,1,1,1,1,1,1,
1,1,1,1,1,1,1,1,1,1,1,1,1,1,1,1,1,1,1,1,1,1,1,1,1,1,1,1,1,1,1,1,1,1,1,1,
1,1,1,1,1,1,1,1,1,1,1,1,1,1,1,1,1,1,1,1,1,1,1,1,1,1,1,1,1,1,1,1,1,1,1,1,
1,1,1,1,1,1,1,1,1,1,1,1,1,1,1,1,1,1,1,1,1,1,1,1,1,1,1,1,1,1,1,1,1,1,1,1,
1,1,1,1,1,1,1,1,1,1,1,1,1,1,1,1,1,1,1,1,1,1,1,1,1,1,1,1,1,1,1,1,1,1,1,1,
1,1,1,1,1,1,1,1,1,1,1,1,1,1,1,1,1,1,1,1,1,1,1,1,1,1,1,1,1,1,1,1,1,1,1,1,
1,1,1,1,1,1,1,1,1,1,1,1,1,1,1,1,1,1,1,1,1,1,1,1,1,1,1,1,1,1,1,1,1,1,1,1,
1,1,1,1,1,1,1,1,1,1,1,1,1,1,1,1,1,1,1,1,1,1,1,1,1,1,1,1,1,1,1,1,1,1,1,1,
1,1,1,1,1,1,1,1,1,1,1,1,1,1,1,1,1,1,1,1,1,1,1,1,1,1,1,1,1,1,1,1,1,1,1,1,
1,1,1,1,1,1,1,1,1,1,1,1,1,1,1,1,1,1,1,1,1,1,1,1,1,1,1,1,1,1,1,1,1,1,1,1,
1,1,1,1,1,1,1,1,1,1,1,1,1,1,1,1,1,1,1,1,1,1,1,1,1,1,1,1,1,1,1,1,1,1,1,1,
1,1,1,1,1,1,1,1,1,1,1,1,1,1,1,1,1,1,1,1,1,1,1,1,1,1,1,1,1,1,1,1,1,1,1,1,
1,1,1,1,1,1,1,1,1,1,1,1,1,1,1,1,1,1,1,1,1,1,1,1,1,1,1,1,1,1,1,1,1,1,1,1,
1,1,1,1,1,1,1,1,1,1,1,1,1,1,1,1,1,1,1,1,1,1,1,1,1,1,1,1,1,1,1,1,1,1,1,1,
1,1,1,1,1,1,1,1,1,1,1,1,1,1,1,1,1,1,1,1,1,1,1,1,1,1,1,1,1,1,1,1,1,1,1,1,
1,1,1,1,1,1,1,1,1,1,1,1,1,1,1,1,1,1,1,1,1,1,1,1,1,1,1,1,1,1,1,1,1,1,1,1,
1,1,1,1,1,1,1,1,1,1,1,1,1,1,1,1,1,1,1,1,1,1,1,1,1,1,1,1,1,1,1,1,1,1,1,1,
1,1,1,1,1,1,1,1,1,1,1,1,1,1,1,1,1,1,1,1,1,1,1,1,1,1,1,1,1,1,1,1,1,1,1,1,
1,1,1,1,1,1,1,1,1,1,1,1,1,1,1,1,1,1,1,1,1,1,1,1,1,1,1,1,1,1,1,1,1,1,1,1,
1,1,1,1,1,1,1,1,1,1,1,1,1,1,1,1,1,1,1,1,1,1,1,1,1,1,1,1,1,1,1,1,1,1,1,1,
1,1,1,1,1,1,1,1,1,1,1,1,1,1,1,1,1,1,1,1,1,1,1,1,1,1,1,1,1,1,1,1,1,1,1,1,
1,1,1,1,1,1,1,1,1,1,1,1,1,1,1,1,1,1,1,1,1,1,1,1,1,1,1,1,1,1,1,1,1,1,1,1,
1,1,1,1,1,1,1,1,1,1,1,1,1,1,1,1,1,1,1,1,1,1,1,1,1,1,1,1,1,1,1,1,1,1,1,1,
1,1,1,1,1,1,1,1,1,1,1,1,1,1,1,1,1,1,1,1,1,1,1,1,1,1,1,1,1,1,1,1,1,1,1,1,
1,1,1,1,1,1,1,1,1,1,1,1,1,1,1,1,1,1,1,1,1,1,1,1,1,1,1,1,1,1,1,1,1,1,1,1,
1,1,1,1,1,1,1,1,1,1,1,1,1,1,1,1,1,1,1,1,1,1,1,1,1,1,1,1,1,1,1,1,1,1,1,1,
1,1,1,1,1,1,1,1,1,1,1,1,1,1,1,1,1,1,1,1,1,1,1,1,1,1,1,1,1,1,1,1,1,1,1,1,
1,1,1,1,1,1,1,1,1,1,1,1,1,1,1,1,1,1,1,1,1,1,1,1,1,1,1,1,1,1,1,1,1,1,1,1,
1,1,1,1,1,1,1,1,1,1,1,1,1,1,1,1,1,1,1,1,1,1,1,1,1,1,1,1,1,1,1,1,1,1,1,1,
1,1,1,1,1,1,1,1,1,1,1,1,1,1,1,1,1,1,1,1,1,1,1,1,1,1,1,1,1,1,1,1,1,1,1,1,
1,1,1,1,1,1,1,1,1,1,1,1,1,1,1,1,1,1,1,1,1,1,1,1,1,1,1,1,1,1,1,1,1,1,1,1,
1,1,1,1,1,1,1,1,1,1,1,1,1,1,1,1,1,1,1,1,1,1,1,1,1,1,1,1,1,1,1,1,1,1,1,1,
1,1,1,1,1,1,1,1,1,1,1,1,1,1,1,1,1,1,1,1,1,1,1,1,1,1,1,1,1,1,1,1,1,1,1,1,
1,1,1,1,1,1,1,1,1,1,1,1,1,1,1,1,1,1,1,1,1,1,1,1,1,1,1,1,1,1,1,1,1,1,1,1,
1,1,1,1,1,1,1,1,1,1,1,1,1,1,1,1,1,1,1,1,1,1,1,1,1,1,1,1,1,1,1,1,1,1,1,1,
1,1,1,1,1,1,1,1,1,1,1,1,1,1,1,1,1,1,1,1,1,1,1,1,1,1,1,1,1,1,1,1,1,1,1,1,
1,1,1,1,1,1,1,1,1,1,1,1,1,1,1,1,1,1,1,1,1,1,1,1,1,1,1,1,1,1,1,1,1,1,1,1,
1,1,1,1,1,1,1,1,1,1,1,1,1,1,1,1,1,1,1,1,1,1,1,1,1,1,1,1,1,1,1,1,1,1,1,1,
1,1,1,1,1,1,1,1,1,1,1,1,1,1,1,1,1,1,1,1,1,1,1,1,1,1,1,1,1,1,1,1,1,1,1,1,
1,1,1,1,1,1,1,1,1,1,1,1,1,1,1,1,1,1,1,1,1,1,1,1,1,1,1,1,1,1,1,1,1,1,1,1,
1,1,1,1,1,1,1,1,1,1,1,1,1,1,1,1,1,1,1,1,1,1,1,1,1,1,1,1,1,1,1,1,1,1,1,1,
1,1,1,1,1,1,1,1,1,1,1,1,1,1,1,1,1,1,1,1,1,1,1,1,1,1,1,1,1,1,1,1,1,1,1,1,
1,1,1,1,1,1,1,1,1,1,1,1,1,1,1,1,1,1,1,1,1,1,1,1,1,1,1,1,1,1,1,1,1,1,1,1,
1,1,1,1,1,1,1,1,1,1,1,1,1,1,1,1,1,1,1,1,1,1,1,1,1,1,1,1,1,1,1,1,1,1,1,1,
1,1,1,1,1,1,1,1,1,1,1,1,1,1,1,1,1,1,1,1,1,1,1,1,1,1,1,1,1,1,1,1,1,1,1,1,
1,1,1,1,1,1,1,1,1,1,1,1,1,1,1,1,1,1,1,1,1,1,1,1,1,1,1,1,1,1,1,1,1,1,1,1,
1,1,1,1,1,1,1,1,1,1,1,1,1,1,1,1,1,1,1,1,1,1,1,1,1,1,1,1,1,1,1,1,1,1,1,1,
1,1,1,1,1,1,1,1,1,1,1,1,1,1,1,1,1,1,1,1,1,1,1,1,1,1,1,1,1,1,1,1,1,1,1,1,
1,1,1,1,4),(2,2),(0.,0.869746702321014,1.7394931589914,2.60923976624962,
3.47983908319159,4.35043840179749,5.22018503077054,6.08993165951504,6.95967828799171,
7.82942491616733,8.69917154401062,9.56891817149224,10.4395174886835,11.3101168056706,
12.179863432132,13.049610058144,13.9193566836854,14.7891033087372,15.6588499332817,
16.5285965573034,17.3991958717975,18.2697951860185,18.7046684974166,19.1395418086746,
19.5744151197912,20.0092884307654,20.4441617415962,20.8790350522825,21.7487816732187,
22.1836549834672,22.6185282935685,23.0534016035221,23.4882749133276,23.9231482229848,
24.3588742245859,24.794600226187,25.2294735355468,26.0992201538203,26.5340934627341,
26.9689667714994,27.4038400801166,27.838713388586,28.2735866969081,28.7084600050832,
29.143333313112,29.5782066209952,30.0130799287334,30.4479532363275,30.8828265437783,
31.3185525442794,31.7542785447804,32.1891518519474,32.6240251589741,33.0588984658616,
33.4937717726112,33.928645079224,34.3635183857014,34.7983916920448,35.2332649982556,
35.6681383043353,36.1030116102854,36.5378849161076,36.9727582218035,37.4076315273749,
37.8425048328235,38.2782308323341,38.7139568318446,39.1488301370532,39.5837034421446,
40.0185767471208,40.4534500519838,40.8883233567357,41.3231966613787,41.7580699659148,
42.1929432703463,42.6278165746754,43.0626898789044,43.4975631830356,43.9324364870714,
44.3673097910142,44.8021830948664,45.2379090935952,45.673635092324,46.1085083960024,
46.5433816995978,46.9782550031127,47.4131283065497,47.8480016099115,48.2828749132006,
48.7177482164198,49.1526215195718,49.5874948226593,50.0223681256851,50.457241428652,
50.8921147315628,51.3269880344203,51.7618613372274,52.197587335454,52.6333133336805,
53.0681866363954,53.5030599390685,53.9379332417027,54.3728065443011,54.8076798468664,
55.2425531494018,55.6774264519101,56.1122997543943,56.5471730568575,56.9820463593026,
57.4169196617326,57.8517929641506,58.2866662665595,58.7215395689624,59.157265567009,
59.5929915650557,60.0278648674556,60.4627381698584,60.8976114722673,61.3324847746853,
61.7673580771153,62.2022313795604,62.6371046820236,63.0719779845079,63.5068512870162,
63.9417245895516,64.376597892117,64.8114711947155,65.2463444973499,65.6812178000231,
66.1169437982275,66.5526697964318,66.9875430991915,67.4224164019987,67.8572897048563,
68.2921630077673,68.7270363107343,69.1619096137603,69.5967829168479,70.0316562200001,
70.4665295232194,70.9014028265087,71.3362761298705,71.7711494333077,72.2060227368227,
72.6408960404182,73.0766220391044,73.5123480377905,73.9472213415547,74.382094645407,
74.8169679493499,75.2518412533859,75.6867145575172,76.1215878617464,76.5564611660756,
76.9913344705072,77.4262077750435,77.8610810796866,78.2959543844386,78.7308276893018,
79.1657009942781,79.6005742993696,80.0363002988208,80.4720262982719,80.9068996035997,
81.3417729090484,81.7766462146199,82.211519520316,82.6463928261383,83.0812661320886,
83.5161394381684,83.9510127443794,84.3858860507229,84.8207593572004,85.2556326638134,
85.6905059705631,86.1253792774507,86.5602525844776,86.995978584908,87.4317045853384,
87.8665778926469,88.3014512000977,88.7363245076919,89.1711978154302,89.6060711233134,
90.0409444313423,90.4758177395175,90.9106910478396,91.345564356309,91.7804376649263,
92.2153109736917,92.6501842826055,93.085057591668,93.5199309008791,93.9556569024059,
94.3913829039327,94.8262562134414,95.2611295230986,95.6960028329042,96.1308761428578,
96.5657494529591,97.0006227632077,97.4354960736028,97.870369384144,98.3052426948304,
98.7401160056612,99.1749893166354,99.6098626277522,100.04473593901,100.915335253024,
101.351061255639,101.785934567313,102.220807879124,102.655681191068,103.090554503145,
103.525427815353,104.395174440154,105.264921065453,105.699794378283,106.134667691232,
106.569541004295,107.004414317471,107.8750136343,108.745612951339,109.615359578629,
110.485106206296,111.354852834309,112.224599462639,113.094346091254,113.964092720119,
114.834692038763,115.705291357499,116.575037986826,117.444784616267,118.314531245777,
119.184277875311,120.054024504821,120.923771134261,121.794370453112,122.66496977189,
123.534716400968,124.404463029834,125.274209658448,126.143956286779,127.013702914792,
127.883449542458,128.754048859798,129.624648176939,130.494394803617,131.364141429857,
132.233888055637,133.103634680937,133.973381305737,134.843127930023,135.71372724472,
136.584326559147,137.019199870684,137.454073182083,137.888946493341,138.323819804458,
139.193566426263,140.063313047491,140.498186357887,140.933059668136,141.367932978237,
141.802806288191,142.237679597997,142.673405599673,143.109131601348,143.544004910857,
143.978878220217,144.413751529429,144.848624838491,145.283498147405,145.718371456171,
146.153244764789,146.588118073258,147.022991381581,147.457864689756,147.892737997785,
148.327611305669,148.762484613407,149.197357921002,149.633083921574,150.068809922147,
150.503683229455,150.938556536623,151.37342984365,151.808303150538,152.243176457288,
152.678049763901,153.112923070379,153.547796376722,153.982669682934,154.417542989014,
154.852416294964,155.287289600787,155.722162906483,156.157036212055,156.592762211626,
157.028488211198,157.463361516526,157.898234821735,158.333108126826,158.767981431803,
159.202854736666,159.637728041419,160.072601346062,160.507474650599,160.94234795503,
161.37722125936,161.812094563589,162.246967867721,162.681841171757,163.1167144757,
163.552440474473,163.988166473247,164.423039777011,164.85791308069,165.292786384286,
165.727659687801,166.162532991238,166.597406294601,167.03227959789,167.46715290111,
167.902026204262,168.33689950735,168.771772810376,169.206646113343,169.641519416254,
170.076392719112,170.512118717363,170.947844715614,171.382718018374,171.817591321089,
172.252464623762,172.687337926397,173.122211228996,173.557084531561,173.991957834097,
174.426831136606,174.86170443909,175.296577741554,175.731451044,176.16632434643,
176.601197648848,177.036070951258,177.471796949306,177.907522947355,178.342396249755,
178.777269552155,179.212142854558,179.647016156968,180.081889459386,180.516762761816,
180.951636064262,181.386509366726,181.82138266921,182.256255971719,182.691129274255,
183.12600257682,183.560875879419,183.995749182054,184.431475180237,184.867201178421,
185.302074481136,185.736947783896,186.171821086704,186.606694389561,187.041567692473,
187.47644099544,187.911314298466,188.346187601554,188.781060904706,189.215934207926,
189.650807511215,190.085680814577,190.520554118015,190.95542742153,191.391153420175,
191.82687941882,192.261752722499,192.696626026263,193.131499330116,193.566372634059,
194.001245938095,194.436119242227,194.870992546456,195.305865850785,195.740739155217,
196.175612459754,196.610485764397,197.045359069149,197.480232374013,197.915105678989,
198.350831678382,198.786557677775,199.221430982984,199.656304288312,200.091177593761,
200.526050899333,200.960924205029,201.395797510852,201.830670816802,202.265544122882,
202.700417429093,203.135290735437,203.570164041915,204.005037348528,204.439910655278,
204.874783962166,205.310509962526,205.746235962887,206.181109270054,206.615982577363,
207.050855884814,207.485729192409,207.920602500147,208.355475808031,208.79034911606,
209.225222424235,209.660095732558,210.094969041027,210.529842349645,210.96471565841,
211.399588967324,211.834462276387,212.27018827784,212.705914279292,213.140787588653,
213.575660898161,214.010534207819,214.880280827579,215.31515413768,215.750027447929,
216.184900758324,216.619774068866,217.054647379553,217.489520690384,218.359267312475,
219.22986662628,219.665592628826,220.100465940363,220.535339252038,220.970212563848,
221.83995918787,222.709705812416,223.579452437468,224.014325750179,224.44919906301,
225.318945689022,226.189545005688,227.060144322571,227.929890949664,228.799637577146,
229.66938420499,230.539130833166,231.408877461643,232.278624090388,233.149223408954,
234.019822727623,234.889569356878,235.759315986267,236.629062615749,237.498809245277,
238.368555874806,239.238302504287,240.108901823183,240.979501142017,241.849247771189,
242.718994400167,243.588741028911,244.458487657389,245.328234285565,246.197980913409,
247.068580230891,247.939179548182,248.80892617507,249.678672801532,250.548419427545,
251.418166053087,252.287912678139,253.157659302684,254.028258617581,254.898857932211,
255.333731243885,255.768604555423,256.203477866821,256.63835117808,257.508097800171,
258.377844421689,258.812717732231,259.247591042627,259.682464352876,260.117337662977,
260.552210972931,260.987936974682,261.858536286089,262.293409595598,262.728282904958,
263.16315621417,263.598029523233,264.032902832147,264.467776140913,264.902649449531,
265.337522758001,265.772396066323,266.207269374499,266.642142682528,267.077015990412,
267.511889298151,267.947615298795,268.383341299439,268.81821460689,269.2530879142,
269.687961221367,270.122834528394,270.557707835282,270.992581142032,271.427454448646,
271.862327755124,272.297201061468,272.732074367679,273.166947673759,273.60182097971,
274.036694285533,274.471567591229,274.907293590862,275.343019590495,275.777892895944,
276.212766201272,276.647639506481,277.082512811573,277.51738611655,277.952259421414,
278.387132726166,278.82200603081,279.256879335346,279.691752639779,280.126625944108,
280.561499248338,280.996372552469,281.431245856506,281.866971855324,282.302697854143,
282.737571157996,283.172444461761,283.60731776544,284.042191069036,284.477064372551,
284.911937675989,285.346810979351,285.781684282641,286.216557585861,286.651430889013,
287.086304192101,287.521177495128,287.956050798095,288.390924101007,288.826650099283,
289.262376097559,289.697249400366,290.132122703127,290.566996005842,291.001869308516,
291.43674261115,291.871615913749,292.306489216315,292.741362518851,293.17623582136,
293.611109123845,294.045982426308,294.480855728754,294.915729031185,295.350602333603,
295.786328331655,296.222054329707,296.65692763211,297.091800934511,297.526674236911,
297.961547539314,298.396420841724,298.831294144142,299.266167446573,299.701040749018,
300.135914051482,300.570787353967,301.005660656476,301.440533959012,301.875407261578,
302.310280564177,302.746006562341,303.181732560506,303.616605863179,304.051479165895,
304.486352468655,304.921225771462,305.35609907432,305.790972377232,306.225845680199,
306.660718983226,307.095592286314,307.530465589466,307.965338892686,308.400212195976,
308.835085499338,309.269958802776,309.705684801381,310.141410799985,310.576284103581,
311.01115740726,311.446030711025,311.880904014878,312.315777318821,312.750650622858,
313.185523926989,313.620397231219,314.055270535549,314.490143839981,314.925017144517,
315.359890449161,315.794763753913,316.229637058777,316.665363058112,317.101089057448,
317.53596236254,317.970835667749,318.405708973077,318.840582278526,319.275455584098,
319.710328889795,320.145202195618,320.580075501568,321.014948807648,321.44982211386,
321.884695420204,322.319568726682,322.754442033295,323.189315340045,323.625041340336,
324.060767340628,324.495640647655,324.930513954822,325.365387262131,325.800260569583,
326.235133877177,326.670007184916,327.1048804928,327.539753800829,327.974627109005,
328.409500417327,328.844373725797,329.279247034415,329.714120343181,330.148993652095,
330.584719653474,331.020445654852,331.455318964064,331.890192273424,332.325065582933,
332.759938892591,333.194812202397,333.629685512351,334.064558822453,334.499432132702,
334.934305443098,335.369178753639,335.804052064326,336.673798686132,337.108671997249,
337.544397999725,337.980124002201,338.4149973136,338.849870625137,339.284743936812,
340.154490560568,341.024237184854,341.459110497191,341.893983809655,342.328857122244,
342.763730434955,343.633477060735,344.504076377234,345.374675693955,346.244422320844,
347.114168948136,347.983915575803,348.853662203817,349.723408832148,350.593155460764,
351.463754779246,352.334354097839,353.204100727012,354.07384735634,354.943593985781,
355.813340615292,356.683087244827,357.552833874338,358.423433193272,359.294032512154,
360.163779141409,361.033525770489,361.903272399355,362.77301902797,363.642765656301,
364.512512284316,365.383111601936,366.253710919371,367.123457546465,367.993204173143,
368.862950799383,369.732697425164,370.602444050463,371.472190675265,372.342789990359,
373.21338930519,373.648262617,374.083135928675,374.952882551611,375.822629173987,
376.257502484962,376.692375795793,377.12724910648,377.562122417021,377.996995727417,
378.431869037666,378.866742347767,379.302468349591,379.738194351416,380.173067661222,
380.607940970879,381.042814280388,381.477687589749,381.91256089896,382.347434208023,
382.782307516937,383.217180825703,383.652054134321,384.086927442791,384.521800751113,
384.956674059289,385.391547367318,385.826420675202,386.262146675918,386.697872676635,
387.13274598423,387.567619291681,388.00249259899,388.437365906157,388.872239213185,
389.307112520073,389.741985826823,390.176859133436,390.611732439914,391.046605746258,
391.48147905247,391.91635235855,392.351225664501,392.786098970323,393.221824970019,
393.657550969714,394.092424275286,394.527297580735,394.962170886063,395.397044191272,
395.831917496364,396.266790801341,396.701664106204,397.136537410957,397.5714107156,
398.006284020137,398.441157324569,398.876030628899,399.310903933128,399.74577723726,
400.181503236126,400.617229234991,401.052102538934,401.486975842787,401.921849146551,
402.356722450231,402.791595753827,403.226469057342,403.66134236078,404.096215664142,
404.531088967432,404.965962270651,405.400835573804,405.835708876892,406.270582179918,
406.705455482886,407.141181481189,407.576907479491,408.01178078235,408.446654085157,
408.881527387917,409.316400690633,409.751273993306,410.186147295941,410.62102059854,
411.055893901106,411.490767203642,411.925640506151,412.360513808636,412.795387111099,
413.230260413545,413.665133715976,414.100859714032,414.536585712088,414.971459014498,
415.406332316901,415.841205619301,416.276078921702,416.710952224105,417.145825526515,
417.580698828933,418.015572131364,418.45044543381,418.885318736273,419.320192038758,
419.755065341267,420.189938643803,420.624811946369,421.060537944515,421.496263942662,
421.931137245297,422.36601054797,422.800883850686,423.235757153446,423.670630456253,
424.105503759112,424.540377062023,424.975250364991,425.410123668017,425.844996971105,
426.279870274258,426.714743577477,427.149616880767,427.584490184129,428.020216182695,
428.455942181261,428.890815484776,429.325688788373,429.760562092052,430.195435395816,
430.630308699669,431.065182003612,431.500055307649,431.93492861178,432.36980191601,
432.80467522034,433.239548524772,433.674421829309,434.109295133952,434.544168438705,
434.979894437984,435.415620437262,435.850493742239,436.285367047331,436.72024035254,
437.155113657869,437.589986963318,438.024860268889,438.459733574586,438.894606880409,
439.32948018636,439.76435349244,440.199226798651,440.634100104995,441.068973411473,
441.503846718087,441.939572718309,442.375298718531,442.810172025419,443.245045332447,
443.679918639614,444.114791946923,444.549665254374,444.984538561969,445.419411869708,
445.854285177591,446.289158485621,446.724031793796,447.158905102119,447.593778410589,
448.028651719207,448.463525027973,448.899251029277,449.334977030581,449.769850339644,
450.639596958216,451.074470267725,451.509343577383,451.944216887189,452.379090197143,
452.813963507244,453.248836817493,453.683710127889,454.118583438431,454.553456749117,
454.988330059949,455.423203370923,455.858929373329,456.294655375734,456.729528686993,
457.164401998391,457.599275309929,458.469021933414,458.90389524536,459.338768557437,
459.773641869646,460.208515181983,460.643388494447,461.078261807036,461.948008432578,
462.818607748906,463.689207065461,464.55895369214,465.428700319234,466.298446946716,
467.16819357456,468.037940202737,468.907686831215,469.778286149605,470.648885468116,
471.518632097196,472.388378726451,473.258125355841,474.127871985322,474.997618614851,
475.86736524438,476.737964563343,477.608563882265,478.478310511593,479.348057140765,
480.217803769743,481.087550398488,481.957297026966,482.827043655142,483.697642972895,
484.568242290469,485.43798891776,486.307735544649,487.177482171112,488.047228797125,
488.916975422667,489.78672204772,490.657321363009,491.09304736596,491.527920678038,
492.397667301793,493.267413925005,494.137160547663,494.57203385878,495.006907169755,
495.441780480586,495.876653791273,496.311527101814,496.74640041221,497.616999724357,
498.052725726255,498.487599036209,498.922472346015,499.357345655673,499.792218965182,
500.227092274542,500.661965583754,501.096838892816,501.531712201731,501.966585510497,
502.401458819114,502.836332127584,503.271205435907,503.706078744082,504.140952052112,
504.576678052901,505.01240405369,505.447277361429,505.882150669023,506.317023976474,
506.751897283783,507.186770590951,507.621643897978,508.056517204866,508.491390511616,
508.92626381823,509.361137124708,509.796010431052,510.230883737263,510.665757043344,
511.100630349294,511.536356349053,511.972082348811,512.406955654506,512.841828960076,
513.276702265523,513.711575570849,514.146448876056,514.581322181146,515.016195486121,
515.451068790983,515.885942095733,516.320815400375,516.75568870491,517.19056200934,
517.625435313668,518.060308617896,518.496034616807,518.931760615718,519.366633919752,
519.801507223694,520.236380527545,520.671253831307,521.106127134985,521.541000438579,
521.975873742092,522.410747045528,522.845620348888,523.280493652176,523.715366955394,
524.150240258545,524.585113561631,525.019986864656,525.455712862985,525.891438861313,
526.326312164223,526.761185467079,527.196058769885,527.630932072643,528.065805375356,
528.500678678029,528.935551980661,529.370425283258,529.805298585822,530.240171888356,
530.675045190863,531.109918493346,531.544791795808,531.979665098252,532.415391096312,
532.851117094373,533.285990396789,533.720863699197,534.155737001598,534.590610303997,
535.025483606395,535.460356908796,535.895230211204,536.330103513621,536.764976816049,
537.199850118493,537.634723420955,538.069596723438,538.504470025945,538.93934332848,
539.375069326608,539.810795324736,540.245668627333,540.680541929966,541.115415232637,
541.550288535351,541.985161838109,542.420035140915,542.854908443771,543.28978174668,
543.724655049646,544.15952835267,544.594401655757,545.029274958907,545.464148262125,
545.899021565413,546.334747563939,546.770473562465,547.205346865901,547.640220169415,
548.075093473009,548.509966776686,548.944840080449,549.3797133843,549.814586688241,
550.249459992276,550.684333296405,551.119206600633,551.554079904961,551.988953209391,
552.423826513926,552.858699818567,553.294425817789,553.73015181701,554.165025121872,
554.599898426846,555.034771731937,555.469645037144,555.90451834247,556.339391647917,
556.774264953487,557.209138259182,557.644011565003,558.078884870951,558.51375817703,
558.948631483239,559.383504789581,559.818378096058,560.254104096209,560.689830096361,
561.12470340311,561.559576709996,561.994450017021,562.429323324187,562.864196631494,
563.299069938943,563.733943246536,564.168816554273,564.603689862154,565.038563170182,
565.473436478355,565.908309786676,566.343183095144,566.77805640376,567.213782404988,
567.649508406216,568.084381715128,568.519255024189,568.954128333399,569.389001642757,
569.823874952264,570.258748261921,570.693621571725,571.128494881677,571.563368191777,
572.433114812417,572.867988122957,573.302861433642,573.737734744471,574.173460746804,
574.609186749136,575.044060060251,575.913806682904,576.783553306113,577.218426617922,
577.653299929865,578.08817324194,578.523046554147,579.392793178944,580.26253980424,
581.13313912039,581.568865123709,582.003738436771,582.87348506323,583.743231690115,
584.612978317402,585.482724945065,586.352471573076,587.222218201403,588.092817519691,
588.963416838109,589.833163467083,590.702910096251,591.572656725575,592.442403355013,
593.31214998452,594.181896614051,595.05249593303,595.92309525198,596.792841881366,
597.662588510618,598.532335139693,599.402081768556,600.271828397167,601.141575025495,
602.012174343369,602.882773661074,603.752520288553,604.622266915642,605.492013542317,
606.361760168553,607.23150679433,608.101253419626,608.971852735101,609.842452050322,
610.71219867434,611.581945297822,612.451691920754,612.886565232011,613.321438543126,
613.756311854099,614.191185164928,615.060931786153,615.931531098516,616.367257100486,
616.802130410586,617.237003720538,617.671877030342,618.106750339998,618.541623649505,
618.976496958863,619.411370268073,619.846243577134,620.281116886046,620.71599019481,
621.150863503426,621.585736811894,622.020610120214,622.455483428388,622.891209429248,
623.326935430108,623.761808737989,624.196682045726,624.631555353319,625.066428660769,
625.501301968075,625.936175275241,626.371048582266,626.805921889153,627.240795195901,
627.675668502512,628.110541808988,628.54541511533,628.98028842154,629.415161727618,
629.850887727438,630.286613727259,630.72148703308,631.156360338774,631.591233644344,
632.026106949791,632.460980255118,632.895853560325,633.330726865415,633.76560017039,
634.200473475251,634.635346780002,635.070220084644,635.505093389179,635.939966693609,
636.374839997937,636.810565996897,637.246291995857,637.681165299986,638.116038604021,
638.550911907962,638.985785211813,639.420658515576,639.855531819253,640.290405122847,
640.725278426361,641.160151729796,641.595025033157,642.029898336444,642.464771639662,
642.899644942813,643.334518245899,643.770244244257,644.205970242616,644.640843545581,
645.075716848491,645.510590151347,645.945463454153,646.380336756911,646.815210059625,
647.250083362296,647.684956664929,648.119829967526,648.55470327009,648.989576572624,
649.424449875131,649.859323177614,650.294196480076,650.729922478144,651.165648476212,
651.600521778641,652.035395081057,652.470268383465,652.905141685866,653.340014988265,
653.774888290663,654.209761593065,654.644634895472,655.079508197889,655.514381500318,
655.949254802762,656.384128105224,656.819001407706,657.253874710213,657.689600708326,
658.12532670644,658.560200009004,658.995073311601,659.429946614234,659.864819916905,
660.299693219619,660.734566522377,661.169439825183,661.604313128039,662.039186430948,
662.474059733914,662.908933036938,663.343806340025,663.778679643175,664.213552946393,
664.649278944883,665.085004943373,665.519878246733,665.954751550169,666.389624853683,
666.824498157277,667.259371460954,667.694244764717,668.129118068568,668.563991372509,
668.998864676544,669.433737980674,669.868611284901,670.303484589229,670.738357893659,
671.173231198194,671.608957197361,672.044683196528,672.479556501278,672.91442980614,
673.349303111115,673.784176416205,674.219049721412,674.653923026738,675.088796332185,
675.523669637755,675.95854294345,676.393416249271,676.82828955522,677.263162861298,
677.698036167508,678.13290947385,678.568635473934,679.004361474018,679.439234780629,
679.874108087377,680.308981394264,680.743854701289,681.178728008455,681.613601315762,
682.048474623211,682.483347930804,682.91822123854,683.353094546422,683.78796785445,
684.222841162623,684.657714470944,685.092587779412,685.528313780566,685.96403978172,
686.398913090483,686.833786399396,687.268659708457,687.703533017666,688.138406327025,
688.573279636532,689.008152946187,689.443026255992,689.877899565944,690.312772876043,
690.74764618629,691.182519496684,691.617392807224,692.052266117909,692.487992120169,
692.92371812243,693.358591433403,694.228338055774,694.663211367171,695.098084678707,
695.532957990379,695.967831302188,696.402704614131,696.837577926207,697.707324550749,
698.577071175797,699.011944488507,699.447670491767,699.883396495028,700.318269807975,
701.188016434211,702.057763060886,702.927509687976,703.797256315454,704.667002943295,
705.536749571467,706.407348889651,707.277948207973,708.147694836835,709.017441465911,
709.887188095163,710.756934724548,711.626681354026,712.496427983551,713.367027302543,
714.237626621516,715.107373250954,715.977119880277,716.846866509446,717.716613138419,
718.586359767161,719.456106395635,720.32670571363,721.197305031464,722.067051659126,
722.936798286414,723.806544913299,724.676291539758,725.546038165767,726.415784791305,
727.286384106969,728.156983422381,729.026730046663,729.896476670415,730.331349982088,
730.766223293624,731.201096605021,731.635969916278,732.505716538366,733.37546315988,
733.81033647042,734.246062472462,734.681788474505,735.116661784752,735.551535094852,
735.986408404804,736.421281714608,736.856155024264,737.291028333771,737.72590164313,
738.160774952339,738.5956482614,739.030521570312,739.465394879076,739.900268187692,
740.33514149616,740.77001480448,741.205740805414,741.641466806347,742.076340114374,
742.511213422256,742.946086729993,743.380960037585,743.815833345035,744.250706652341,
744.685579959507,745.120453266533,745.555326573419,745.990199880167,746.425073186778,
746.859946493254,747.294819799596,747.729693105806,748.165419105691,748.601145105576,
749.036018411525,749.470891717346,749.90576502304,750.34063832861,750.775511634057,
751.210384939384,751.645258244591,752.080131549682,752.515004854656,752.949878159518,
753.384751464269,753.81962476891,754.254498073445,754.689371377875,755.125097376885,
755.560823375895,755.995696680123,756.430569984253,756.865443288287,757.300316592228,
757.735189896079,758.170063199842,758.604936503519,759.039809807113,759.474683110627,
759.909556414062,760.344429717423,760.779303020711,761.214176323929,761.649049627079,
762.084775625469,762.520501623858,762.955374926883,763.390248229848,763.825121532758,
764.259994835614,764.694868138419,765.129741441178,765.564614743891,765.999488046563,
766.434361349196,766.869234651793,767.304107954357,767.738981256891,768.173854559398,
768.608727861881,769.044453859958,769.480179858035,769.915053160479,770.349926462907,
770.784799765324,771.219673067731,771.654546370133,772.089419672531,772.52429297493,
772.959166277331,773.394039579739,773.828912882155,774.263786184584,774.698659487028,
775.13353278949,775.568406091973,776.004132090072,776.439858088172,776.874731390706,
777.30960469327,777.744477995867,778.1793512985,778.614224601171,779.049097903885,
779.483971206643,779.918844509449,780.353717812305,780.788591115215,781.22346441818,
781.658337721205,782.093211024291,782.528084327442,782.963810325897,783.399536324352,
783.834409627639,784.269282931,784.704156234435,785.139029537949,785.573902841543,
786.00877614522,786.443649448983,786.878522752834,787.313396056775,787.74826936081,
788.183142664939,788.618015969167,789.052889273495,789.487762577925,789.923488577038,
790.359214576152,790.794087880793,791.228961185544,791.663834490406,792.098707795381,
792.533581100471,792.968454405678,793.403327711004,793.838201016451,794.273074322021,
794.707947627716,795.142820933537,795.577694239486,796.012567545564,796.447440851774,
796.883166851791,797.318892851808,797.753766158284,798.188639464895,798.623512771643,
799.058386078529,799.493259385555,799.92813269272,800.363006000027,800.797879307477,
801.232752615069,801.667625922806,802.102499230688,802.537372538715,802.972245846889,
803.40711915521,803.84284515629,804.27857115737,804.713444465985,805.148317774749,
805.583191083662,806.018064392723,806.452937701933,806.887811011291,807.322684320798,
808.192430940258,808.62730425021,809.06217756031,809.497050870557,809.931924180951,
810.36679749149,810.802523493679,811.238249495867,811.673122806697,812.542869428785,
812.977742740041,813.412616051438,813.847489362974,814.282362674646,814.717235986455,
815.152109298398,816.021855922681,816.891602547478,817.326475860065,817.762201863265,
818.197927866466,818.632801179295,819.502547805304,820.372294431763,821.242041058648,
822.111787685935,822.981534313598,823.851280941609,824.721880259681,825.5924795779,
826.462226206642,827.331972835616,828.201719464785,829.071466094109,829.941212723546,
830.810959353053,831.681558672047,832.552157991036,833.421904620514,834.2916512499,
835.161397879151,836.031144508226,836.900891137089,837.770637765701,838.641237083811,
839.511836401767,840.381583029608,841.251329657086,842.121076284176,842.990822910851,
843.860569537087,844.730316162863,845.600915478712,846.471514794314,847.341261418855,
848.211008042874,848.645881354683,849.080754666356,849.515627977891,849.950501289288,
850.82024791166,851.689994533462,852.124867844147,852.560593846263,852.996319848379,
853.431193158772,853.866066469019,854.300939779119,855.170686398875,855.605559708531,
856.040433018038,856.475306327397,856.910179636606,857.345052945667,857.77992625458,
858.214799563344,858.64967287196,859.084546180427,859.520272181434,859.95599818244,
860.390871490614,860.825744798641,861.260618106523,861.69549141426,862.130364721852,
862.565238029302,863.000111336609,863.434984643774,863.8698579508,864.304731257686,
864.739604564434,865.174477871045,865.609351177521,866.044224483863,866.479950483814,
866.915676483765,867.350549789843,867.785423095792,868.220296401613,868.655169707307,
869.090043012877,869.524916318325,869.959789623651,870.394662928858,870.829536233948,
871.264409538923,871.699282843785,872.134156148535,872.569029453177,873.003902757712,
873.439628756773,873.875354755834,874.310228060162,874.745101364389,875.179974668519,
875.614847972553,876.049721276495,876.484594580346,876.919467884108,877.354341187786,
877.78921449138,878.224087794893,878.658961098329,879.093834401689,879.528707704977,
879.963581008195,880.399307006616,880.835033005038,881.269906308124,881.704779611148,
882.139652914114,882.574526217024,883.00939951988,883.444272822685,883.879146125444,
884.314019428157,884.748892730829,885.183766033462,885.618639336059,886.053512638623,
886.488385941157,886.923259243664,887.358985241751,887.794711239839,888.2295845423,
888.664457844744,889.099331147173,889.534204449589,889.969077751997,890.403951054398,
890.838824356797,891.273697659195,891.708570961597,892.143444264004,892.578317566421,
893.01319086885,893.448064171293,893.882937473755,894.318663471843,894.75438946993,
895.189262772437,895.624136074971,896.059009377535,896.493882680132,896.928755982765,
897.363629285437,897.798502588151,898.233375890909,898.668249193715,899.103122496571,
899.53799579948,899.972869102446,900.40774240547,900.842615708556,901.278341706978,
901.714067705399,902.148941008617,902.583814311905,903.018687615265,903.453560918701,
903.888434222214,904.323307525808,904.758180829485,905.193054133248,905.627927437099,
906.06280074104,906.497674045075,906.932547349205,907.367420653433,907.80229395776,
908.238019956821,908.673745955883,909.108619260417,909.543492565059,909.978365869809,
910.413239174671,910.848112479646,911.282985784736,911.717859089943,912.152732395269,
912.587605700716,913.022479006287,913.457352311981,913.892225617802,914.327098923751,
914.761972229829,915.19769822978,915.633424229731,916.068297536072,916.503170842548,
916.93804414916,917.372917455908,917.807790762794,918.24266406982,918.677537376985,
919.112410684292,919.547283991742,919.982157299334,920.417030607071,920.851903914953,
921.28677722298,921.721650531154,922.15737653216,922.593102533167,923.027975841635,
923.46284915025,923.897722459014,924.332595767926,924.767469076987,925.202342386197,
925.637215695556,926.072089005063,926.506962314719,926.941835624523,927.376708934475,
927.811582244575,928.246455554822,928.681328865215,929.117054867331,929.987654180132,
930.422527490961,930.857400801934,931.292274113049,931.727147424306,932.162020735703,
932.596894047238,933.46664067072,934.336387294739,934.771260606945,935.20613391928,
935.641007231742,936.076733234882,936.94733255073,937.817079176507,938.686825802743,
939.556572429418,940.426319056508,941.296065683986,942.165812311827,943.036411629783,
943.907010947893,944.776757576505,945.646504205367,946.516250834443,947.385997463694,
948.25574409308,949.125490722558,949.996090041546,950.86668936054,951.736435990048,
952.606182619485,953.475929248809,954.345675877978,955.215422506951,956.085169135693,
956.955768453912,957.826367771985,958.696114399995,959.565861027658,960.435607654946,
961.305354281831,962.175100908289,963.044847534298,963.915446850328,964.786046166116,
965.655792790913,966.525539415195,966.960412727138,967.395286038947,968.265032662155,
969.134779284809,969.569652595924,970.004525906897,970.439399217726,970.875125219914,
971.310851222103,971.745724532643,972.615471153283,973.485217773335,973.920091083139,
974.354964392795,974.789837702302,975.22471101166,975.65958432087,976.094457629931,
976.529330938844,976.964204247608,977.399077556223,977.834803557303,978.270529558383,
978.705402866704,979.140276174877,979.575149482905,980.010022790786,980.444896098523,
980.879769406116,981.314642713565,981.749516020872,982.184389328038,982.619262635063,
983.05413594195,983.489009248698,983.923882555309,984.358755861785,984.794481861802,
985.230207861819,985.665081168029,986.099954474107,986.534827780056,986.969701085877,
987.404574391571,987.839447697141,988.274321002589,988.709194307915,989.144067613122,
989.578940918212,990.013814223187,990.448687528048,990.883560832799,991.31843413744,
991.754160136554,992.189886135667,992.624759440097,993.059632744425,993.494506048653,
993.929379352783,994.364252656817,994.799125960758,995.233999264609,995.668872568372,
996.103745872049,996.538619175643,996.973492479157,997.408365782593,997.843239085953,
998.278112389241,998.713838387696,999.149564386151,999.584437689301,1000.01931099239,
1000.45418429541,1000.88905759838,1001.32393090129,1001.75880420414,1002.19367750695,
1002.62855080971,1003.06342411242,1003.49829741509,1003.93317071773,1004.36804402032,
1004.80291732289,1005.23779062542,1005.67351662352,1006.10924262162,1006.5441159241,
1006.97898922656,1007.41386252901,1007.84873583144,1008.28360913385,1008.71848243626,
1009.15335573866,1009.58822904106,1010.02310234346,1010.45797564586,1010.89284894827,
1011.32772225069,1011.76259555311,1012.19746885556,1012.63319485364,1013.06892085171,
1013.5037941542,1013.9386674567,1014.37354075924,1014.8084140618,1015.2432873644,
1015.67816066703,1016.1130339697,1016.54790727242,1016.98278057517,1017.41765387798,
1017.85252718084,1018.28740048375,1018.72227378671,1019.15714708974,1019.59287308813,
1020.02859908651,1020.46347238967,1020.89834569288,1021.33321899617,1021.76809229953,
1022.20296560297,1022.63783890648,1023.07271221007,1023.50758551375,1023.94245881752,
1024.37733212137,1024.81220542531,1025.24707872935,1025.68195203348,1026.11682533771,
1026.55255133672,1026.98827733573,1027.42315064016,1027.8580239447,1028.29289724934,
1028.72777055409,1029.16264385896,1029.59751716393,1030.03239046902,1030.46726377423,
1030.90213707956,1031.33701038501,1031.77188369058,1032.20675699628,1032.6416303021,
1033.07650360805,1033.51222960793,1033.94795560782,1034.38282891403,1034.81770222038,
1035.25257552685,1035.68744883347,1036.12232214022,1036.5571954471,1036.99206875413,
1037.4269420613,1037.86181536861,1038.29668867606,1038.73156198365,1039.16643529139,
1039.60130859927,1040.0361819073,1040.47190790824,1040.90763390917,1041.34250721749,
1041.77738052596,1042.21225383458,1042.64712714334,1043.08200045226,1043.95174707053,
1044.38662037989,1044.8214936894,1045.25636699906,1045.69124030886,1046.12611361882,
1046.56098692892,1046.99586023917,1047.43158624121,1047.86731224325,1048.3021855538,
1048.73705886448,1049.17193217531,1049.60680548629,1050.0416787974,1050.47655210866,
1050.91142542006,1051.78117204327,1052.21604535508,1052.65091866703,1053.0857919791,
1053.52066529131,1053.95553860365,1054.39126460673,1055.26186392239,1056.13161054793,
1057.00135717395,1057.43623048712,1057.87110380041,1058.7408504273,1059.61059705459,
1060.48034368225,1061.35094300009,1062.22154231809,1063.09128894656,1063.96103557531,
1064.83078220429,1065.70052883346,1066.57027546278,1067.44002209222,1068.3106214112,
1069.18122073019,1070.05096735972,1070.9207139892,1071.79046061859,1072.66020724785,
1073.52995387693,1074.39970050579,1075.27029982411,1076.1408991423,1077.01064577048,
1077.88039239832,1078.7501390258,1079.61988565289,1080.48963227957,1081.35937890581,
1082.22997822202,1083.100577538,1083.97032416305,1084.84007078759,1085.70981741161,
1086.5795640351,1087.44931065803,1087.88418396929,1088.31905728041,1088.75393059138,
1089.18965659365,1089.62538259591,1090.06025590659,1090.93000252753,1091.36487583778,
1091.79974914788,1092.23462245783,1092.66949576764,1093.1043690773,1093.5392423868,
1093.97411569616,1094.40898900538,1094.84386231444,1095.27873562335,1095.71360893212,
1096.14933493327,1096.58506093443,1097.0199342429,1097.45480755122,1097.88968085939,
1098.32455416742,1098.75942747531,1099.19430078305,1099.62917409064,1100.06404739809,
1100.4989207054,1100.93379401257,1101.36866731959,1101.80354062648,1102.23841393323,
1102.67328723984,1103.10901323993,1103.54473924001,1103.97961254636,1104.41448585257,
1104.84935915865,1105.2842324646,1105.71910577042,1106.15397907612,1106.58885238169,
1107.02372568714,1107.45859899246,1107.89347229767,1108.32834560276,1108.76321890774,
1109.1980922126,1109.63296551736,1110.06869151652,1110.50441751569,1110.93929082023,
1111.37416412466,1111.80903742899,1112.24391073322,1112.67878403735,1113.11365734139,
1113.54853064533,1113.98340394918,1114.41827725295,1114.85315055662,1115.28802386022,
1115.72289716374,1116.15777046717,1116.59264377053,1117.02836976903,1117.46409576752,
1117.89896907074,1118.33384237389,1118.76871567698,1119.20358898,1119.63846228297,
1120.07333558588,1120.50820888874,1120.94308219154,1121.3779554943,1121.81282879702,
1122.24770209969,1122.68257540233,1123.11744870492,1123.55232200749,1123.98804800561,
1124.42377400372,1124.85864730623,1125.29352060871,1125.72839391118,1126.16326721362,
1126.59814051605,1127.03301381847,1127.46788712088,1127.90276042328,1128.33763372568,
1128.77250702808,1129.20738033048,1129.64225363289,1130.07712693531,1130.51200023774,
1130.94772623581,1131.38345223388,1131.81832553634,1132.25319883883,1132.68807214134,
1133.12294544387,1133.55781874644,1133.99269204904,1134.42756535167,1134.86243865434,
1135.29731195706,1135.73218525982,1136.16705856263,1136.60193186548,1137.03680516839,
1137.47167847136,1137.90740446972,1138.34313046808,1138.77800377117,1139.21287707432,
1139.64775037754,1140.08262368083,1140.51749698419,1140.95237028763,1141.38724359114,
1141.82211689474,1142.25699019842,1142.69186350218,1143.12673680603,1143.56161010998,
1143.99648341401,1144.43135671814,1144.86708271711,1145.30280871607,1145.7376820204,
1146.17255532483,1146.60742862936,1147.04230193401,1147.47717523876,1147.91204854362,
1148.3469218486,1148.78179515369,1149.2166684589,1149.65154176423,1150.08641506968,
1150.52128837525,1150.95616168094,1151.39103498677,1151.82676098659,1152.26248698641,
1152.69736029249,1153.1322335987,1153.56710690504,1154.00198021152,1154.43685351813,
1154.87172682488,1155.30660013177,1155.7414734388,1156.17634674597,1156.61122005327,
1157.04609336073,1157.48096666832,1157.91583997606,1158.35071328394,1158.7864392848,
1159.22216528566,1159.65703859384,1160.09191190216,1160.52678521063,1160.96165851925,
1161.39653182801,1161.83140513693,1162.26627844599,1162.7011517552,1163.13602506456,
1163.57089837407,1164.00577168373,1164.44064499353,1164.87551830349,1165.74611761556,
1166.18184361753,1166.61671692792,1167.05159023846,1167.48646354915,1167.92133685998,
1168.35621017096,1169.22595679333,1170.09570341627,1170.53057672794,1170.96545003975,
1171.4003233517,1171.83519666377,1172.27006997598,1172.705795979,1173.57639529447,
1174.44614191977,1174.8810152326,1175.31588854555,1176.18563517179,1177.05538179847,
1177.92512842556,1178.79487505304,1179.66547437075,1180.53607368863,1181.40582031696,
1182.27556694557,1183.14531357444,1184.01506020352,1184.88480683277,1185.75455346216,
1186.62515278112,1187.4957521001,1188.36549872963,1189.23524535914,1190.10499198858,
1190.97473861791,1191.84448524708,1192.71423187606,1193.58483119448,1194.45543051277,
1195.3251771411,1196.19492376911,1197.06467039678,1197.93441702407,1198.80416365096,
1199.67391027742,1200.5445095938,1201.41510890996,1202.28485553525,1203.15460216005,
1204.02434878434,1204.89409540809,1205.76384203131,1206.1987153427,1206.63358865396,
1207.06846196508,1207.50418796741,1208.37478728058,1209.2445339018,1209.6794072122,
1210.11428052245,1210.54915383255,1210.9840271425,1211.41890045231,1211.85377376197,
1212.28864707147,1212.72352038083,1213.15839369005,1213.59326699911,1214.02814030802,
1214.46386630925,1214.89959231048,1215.3344656191,1215.76933892757,1216.20421223589,
1216.63908554406,1217.07395885209,1217.50883215998,1217.94370546771,1218.37857877531,
1218.81345208276,1219.24832539007,1219.68319869724,1220.11807200426,1220.55294531115,
1220.9878186179,1221.42354461805,1221.85927061821,1222.29414392468,1222.72901723103,
1223.16389053724,1223.59876384332,1224.03363714927,1224.46851045509,1224.90338376079,
1225.33825706636,1225.77313037181,1226.20800367713,1226.64287698234,1227.07775028743,
1227.51262359241,1227.94749689727,1228.3832228965,1228.81894889572,1229.25382220036,
1229.6886955049,1230.12356880933,1230.55844211366,1230.99331541789,1231.42818872202,
1231.86306202606,1232.29793533,1232.73280863385,1233.16768193762,1233.60255524129,
1234.03742854489,1234.4723018484,1234.90717515184,1235.34290115037,1235.7786271489,
1236.21350045219,1236.64837375541,1237.08324705856,1237.51812036165,1237.95299366467,
1238.38786696764,1238.82274027055,1239.25761357341,1239.69248687621,1240.12736017897,
1240.56223348169,1240.99710678436,1241.431980087,1241.8668533896,1242.30257938773,
1242.73830538585,1243.17317868839,1243.6080519909,1244.04292529338,1244.47779859585,
1244.91267189829,1245.34754520072,1245.78241850314,1246.21729180555,1246.65216510795,
1247.08703841035,1247.52191171275,1247.95678501515,1248.39165831756,1248.82653161998,
1249.26225761804,1249.69798361611,1250.13285691855,1250.56773022101,1251.0026035235,
1251.43747682601,1251.87235012854,1252.30722343111,1252.74209673371,1253.17697003634,
1253.61184333901,1254.04671664173,1254.48158994449,1254.9164632473,1255.35133655015,
1255.78620985306,1256.22193585139,1256.65766184973,1257.09253515275,1257.52740845584,
1257.96228175899,1258.39715506221,1258.8320283655,1259.26690166886,1259.7017749723,
1260.13664827581,1260.57152157941,1261.00639488309,1261.44126818685,1261.8761414907,
1262.31101479465,1262.74588809868,1263.1816140976,1263.61734009651,1264.05221340074,
1264.48708670507,1264.9219600095,1265.35683331403,1265.79170661868,1266.22657992343,
1266.66145322829,1267.09632653327,1267.53119983836,1267.96607314357,1268.4009464489,
1268.83581975434,1269.27069305992,1269.70556636561,1270.14129236537,1270.57701836513,
1271.01189167108,1271.44676497716,1271.88163828337,1272.31651158971,1272.75138489619,
1273.1862582028,1273.62113150955,1274.05600481644,1274.49087812347,1274.92575143063,
1275.36062473794,1275.79549804539,1276.23037135299,1276.66524466073,1277.10097066151,
1277.5366966623,1277.97156997033,1278.40644327851,1278.84131658683,1279.2761898953,
1279.71106320392,1280.14593651268,1280.5808098216,1281.01568313066,1281.45055643987,
1281.88542974923,1282.32030305874,1282.75517636839,1283.1900496782,1283.62492298815,
1284.06064899005,1284.49637499195,1284.9312483022,1285.36612161259,1285.80099492313,
1286.23586823382,1286.67074154465,1287.54048816674,1287.975361478,1288.4102347894,
1288.84510810093,1289.27998141261,1289.71485472442,1290.14972803636,1291.02032735139,
1291.89092666668,1292.32579997914,1292.76067329173,1293.19554660444,1293.63041991727,
1294.50016654328,1295.36991316974,1296.23965979663,1297.10940642392,1297.9800057415,
1298.85060505925,1299.72035168742,1300.5900983159,1301.45984494464,1302.32959157362,
1303.19933820279,1304.06908483212,1304.93968415104,1305.81028347,1306.68003009953,
1307.54977672906,1308.41952335854,1309.28926998793,1310.15901661718,1311.02876324626,
1311.89936256477,1312.76996188316,1313.63970851164,1314.50945513981,1315.37920176765,
1316.24894839514,1317.11869502223,1317.98844164891,1318.85904096546,1319.72964028179,
1320.59938690733,1321.46913353238,1322.33888015692,1323.20862678095,1323.64350009276,
1324.07837340443,1324.51324671597,1324.94812002737,1325.81871934103,1326.68931865441,
1327.12419196524,1327.55906527593,1327.99393858647,1328.42881189686,1328.86368520711,
1329.29855851721,1329.73343182716,1330.16830513697,1330.60317844663,1331.03805175614,
1331.4729250655,1331.90779837471,1332.34267168377,1332.77839768507,1333.21412368638,
1333.64899699514,1334.08387030376,1334.51874361223,1334.95361692055,1335.38849022873,
1335.82336353676,1336.25823684464,1336.69311015238,1337.12798345997,1337.56285676742,
1337.99773007473,1338.4326033819,1338.86747668892,1339.30234999581,1339.73807599603,
1340.17380199625,1340.60867530287,1341.04354860934,1341.47842191569,1341.9132952219,
1342.34816852798,1342.78304183393,1343.21791513975,1343.65278844545,1344.08766175102,
1344.52253505647,1344.95740836179,1345.392281667,1345.82715497209,1346.26202827707,
1346.69775427635,1347.13348027563,1347.56835358038,1348.00322688502,1348.43810018956,
1348.87297349399,1349.30784679832,1349.74272010255,1350.17759340668,1350.61246671072,
1351.04734001466,1351.48221331851,1351.91708662228,1352.35195992595,1352.78683322955,
1353.22170653306,1353.65743253163,1354.09315853019,1354.52803183356,1354.96290513685,
1355.39777844007,1355.83265174322,1356.26752504631,1356.70239834933,1357.1372716523,
1357.57214495521,1358.00701825807,1358.44189156087,1358.87676486363,1359.31163816635,
1359.74651146902,1360.18138477166,1360.6171107698,1361.05283676795,1361.48771007051,
1361.92258337305,1362.35745667556,1362.79232997804,1363.2272032805,1363.66207658295,
1364.09694988538,1364.5318231878,1364.96669649021,1365.40156979261,1365.83644309501,
1366.27131639741,1366.70618969981,1367.14106300222,1367.57678900028,1368.01251499834,
1368.44738830077,1368.88226160321,1369.31713490567,1369.75200820816,1370.18688151067,
1370.6217548132,1371.05662811577,1371.49150141837,1371.926374721,1372.36124802367,
1372.79612132639,1373.23099462915,1373.66586793196,1374.10074123481,1374.53646723311,
1374.97219323142,1375.40706653438,1375.84193983741,1376.2768131405,1376.71168644365,
1377.14655974687,1377.58143305016,1378.01630635352,1378.45117965696,1378.88605296047,
1379.32092626407,1379.75579956775,1380.19067287151,1380.62554617536,1381.06041947931,
1381.49614547817,1381.93187147704,1382.36674478117,1382.8016180854,1383.23649138973,
1383.67136469416,1384.10623799869,1384.54111130334,1384.97598460809,1385.41085791295,
1385.84573121793,1386.28060452302,1386.71547782823,1387.15035113356,1387.585224439,
1388.02009774458,1388.45582374427,1388.89154974397,1389.32642304979,1389.76129635574,
1390.19616966182,1390.63104296803,1391.06591627437,1391.50078958085,1391.93566288746,
1392.37053619421,1392.8054095011,1393.24028280813,1393.6751561153,1394.1100294226,
1394.54490273005,1394.97977603765,1395.41550203836,1395.85122803908,1396.28610134696,
1396.72097465499,1397.15584796317,1397.59072127149,1398.02559457996,1398.46046788858,
1398.89534119734,1399.33021450626,1399.76508781532,1400.19996112453,1400.63483443389,
1401.50458105306,1401.93945436286,1402.37518036469,1402.81090636651,1403.24577967661,
1403.68065298686,1404.11552629725,1404.5503996078,1404.98527291848,1405.85501954029,
1406.2898928514,1406.72476616266,1407.15963947406,1407.5945127856,1408.02938609727,
1408.46425940908,1409.33485872391,1410.205458039,1410.64033135134,1411.07520466381,
1411.51007797639,1411.9449512891,1412.81469791488,1413.68444454112,1414.5541911678,
1415.42393779489,1416.29453711233,1417.16513642995,1418.03488305796,1418.90462968629,
1419.77437631491,1420.64412294377,1421.51386957285,1422.38361620211,1423.25421552099,
1424.12481483992,1424.99456146943,1425.86430809896,1426.73405472847,1427.60380135791,
1428.47354798724,1429.34329461641,1430.21389393501,1431.08449325349,1431.9542398821,
1432.82398651043,1433.69373313844,1434.56347976611,1435.4332263934,1436.30297302029,
1437.17357233701,1438.04417165351,1438.91391827929,1439.78366490459,1440.65341152939,
1441.52315815367,1441.95803146562,1442.39290477743,1442.8277780891,1443.26265140064,
1444.13325071451,1445.00385002811,1445.43872333908,1445.87359664991,1446.3084699606,
1446.74334327114,1447.17821658153,1447.61308989178,1448.48283651184,1448.91770982164,
1449.3525831313,1449.78745644081,1450.22232975017,1450.65720305938,1451.09292906076,
1451.52865506214,1451.96352837105,1452.39840167982,1452.83327498843,1453.2681482969,
1453.70302160522,1454.1378949134,1454.57276822143,1455.00764152931,1455.44251483705,
1455.87738814464,1456.31226145209,1456.7471347594,1457.18200806657,1457.6168813736,
1458.05260737389,1458.48833337418,1458.92320668093,1459.35807998754,1459.79295329402,
1460.22782660036,1460.66269990657,1461.09757321265,1461.5324465186,1461.96731982443,
1462.40219313012,1462.83706643569,1463.27193974114,1463.70681304647,1464.14168635168,
1464.57655965677,1465.0122856561,1465.44801165544,1465.8828849603,1466.31775826505,
1466.7526315697,1467.18750487423,1467.62237817866,1468.05725148299,1468.49212478722,
1468.92699809135,1469.36187139539,1469.79674469933,1470.23161800319,1470.66649130695,
1471.10136461063,1471.53623791422,1471.97196391283,1472.40768991143,1472.84256321487,
1473.27743651823,1473.71230982152,1474.14718312474,1474.58205642789,1475.01692973098,
1475.451803034,1475.88667633697,1476.32154963988,1476.75642294274,1477.19129624555,
1477.62616954831,1478.06104285102,1478.4959161537,1478.93164215186,1479.36736815002,
1479.80224145262,1480.23711475519,1480.67198805772,1481.10686136023,1481.54173466272,
1481.97660796518,1482.41148126762,1482.84635457005,1483.28122787247,1483.71610117488,
1484.15097447728,1484.58584777968,1485.02072108208,1485.45559438449,1485.89132038254,
1486.32704638059,1486.76191968301,1487.19679298544,1487.63166628788,1488.06653959035,
1488.50141289283,1488.93628619534,1489.37115949787,1489.80603280044,1490.24090610304,
1490.67577940567,1491.11065270835,1491.54552601106,1491.98039931382,1492.41527261663,
1492.8509986149,1493.28672461318,1493.72159791609,1494.15647121906,1494.59134452208,
1495.02621782517,1495.46109112832,1495.89596443154,1496.33083773483,1496.76571103819,
1497.20058434163,1497.63545764515,1498.07033094874,1498.50520425242,1498.94007755618,
1499.37495086004,1499.81067685885,1500.24640285767,1500.68127616171,1501.11614946584,
1501.55102277007,1501.9858960744,1502.42076937883,1502.85564268337,1503.29051598801,
1503.72538929276,1504.16026259762,1504.5951359026,1505.03000920769,1505.4648825129,
1505.89975581823,1506.33462912368,1506.77035512331,1507.20608112294,1507.64095442864,
1508.07582773446,1508.51070104041,1508.94557434649,1509.3804476527,1509.81532095904,
1510.25019426552,1510.68506757213,1511.11994087888,1511.55481418577,1511.9896874928,
1512.42456079996,1512.85943410727,1513.29430741472,1513.73003341537,1514.16575941601,
1514.60063272375,1515.03550603163,1515.47037933966,1515.90525264784,1516.34012595616,
1516.77499926463,1517.20987257325,1517.64474588201,1518.07961919093,1518.51449249999,
1518.9493658092,1519.38423911856,1519.81911242807,1520.25398573772,1520.68971173947,
1521.12543774122,1521.56031105118,1521.99518436128,1522.43005767153,1523.29980429246,
1523.73467760315,1524.16955091398,1524.60442422495,1525.03929753607,1525.47417084733,
1525.90904415873,1526.77879078194,1527.64939009657,1528.08511609939,1528.51998941146,
1528.95486272367,1529.38973603601,1530.25948266106,1531.1292292866,1531.99897591261,
1532.86872253907,1533.73846916596,1534.60906848325,1535.47966780073,1536.34941442858,
1537.21916105675,1538.08890768523,1538.95865431398,1539.82840094295,1540.69814757212,
1541.56874689096,1542.43934620985,1543.30909283933,1544.17883946886,1545.04858609839,
1545.91833272787,1546.78807935726,1547.65782598651,1548.52842530518,1549.39902462375,
1550.26877125249,1551.13851788097,1552.00826450914,1552.87801113699,1553.74775776447,
1554.61750439156,1555.48810370844,1556.35870302511,1557.22844965112,1558.09819627666,
1558.96794290171,1559.83768952626,1560.27256283834,1560.70743615028,1561.57718277377,
1562.44778208785,1563.31838140165,1563.75325471277,1564.18812802374,1564.62300133457,
1565.05787464526,1565.9276212662,1566.79736788655,1567.2322411965,1567.66711450631,
1568.10198781596,1568.53686112547,1568.97173443483,1569.40746043628,1569.84318643774,
1570.2780597468,1570.71293305571,1571.14780636448,1571.5826796731,1572.01755298157,
1572.45242628989,1572.88729959806,1573.32217290609,1573.75704621397,1574.19191952171,
1574.62679282931,1575.06166613676,1575.49653944407,1575.93141275123,1576.36713875159,
1576.80286475195,1577.23773805884,1577.67261136559,1578.1074846722,1578.54235797868,
1578.97723128502,1579.41210459124,1579.84697789732,1580.28185120327,1580.71672450909,
1581.15159781478,1581.58647112036,1582.0213444258,1582.45621773113,1582.89109103634,
1583.32681703573,1583.76254303513,1584.1974163401,1584.63228964497,1585.06716294972,
1585.50203625436,1585.9369095589,1586.37178286333,1586.80665616766,1587.24152947189,
1587.67640277602,1588.11127608005,1588.546149384,1588.98102268785,1589.41589599161,
1589.85076929529,1590.28649529394,1590.72222129258,1591.1570945961,1591.59196789953,
1592.0268412029,1592.46171450619,1592.8965878094,1593.33146111256,1593.76633441564,
1594.20120771867,1594.63608102164,1595.07095432455,1595.50582762741,1595.94070093021,
1596.37557423297,1596.81044753569,1597.24617353387,1597.68189953206,1598.11677283469,
1598.55164613729,1598.98651943985,1599.42139274239,1599.8562660449,1600.29113934738,
1600.72601264985,1601.16088595229,1601.59575925472,1602.03063255714,1602.46550585955,
1602.90037916195,1603.33525246435,1603.77012576675,1604.2058517648,1604.64157776285,
1605.07645106526,1605.51132436768,1605.94619767011,1606.38107097255,1606.81594427502,
1607.2508175775,1607.68569088001,1608.12056418254,1608.55543748511,1608.99031078771,
1609.42518409034,1609.86005739302,1610.29493069573,1610.72980399849,1611.16552999674,
1611.60125599499,1612.03612929785,1612.47100260076,1612.90587590373,1613.34074920675,
1613.77562250984,1614.21049581299,1614.64536911621,1615.0802424195,1615.51511572286,
1615.9499890263,1616.38486232981,1616.81973563341,1617.25460893709,1617.68948224085,
1618.12520823963,1618.5609342384,1618.99580754234,1619.43068084638,1619.86555415051,
1620.30042745474,1620.73530075907,1621.1701740635,1621.60504736804,1622.03992067268,
1622.47479397743,1622.90966728229,1623.34454058727,1623.77941389236,1624.21428719757,
1624.6491605029,1625.08488650247,1625.52061250204,1625.95548580761,1626.39035911331,
1626.82523241913,1627.26010572508,1627.69497903116,1628.12985233737,1628.56472564372,
1628.99959895019,1629.43447225681,1629.86934556356,1630.30421887044,1630.73909217747,
1631.17396548464,1631.60883879195,1632.04456479252,1632.48029079309,1632.91516410068,
1633.35003740842,1633.78491071631,1634.21978402433,1634.65465733251,1635.08953064083,
1635.5244039493,1635.95927725792,1636.39415056668,1636.8290238756,1637.26389718466,
1637.69877049387,1638.13364380323,1638.56851711274,1639.00424311442,1639.43996911609,
1639.8748424259,1640.30971573585,1640.74458904595,1641.6143356666,1642.04920897714,
1642.48408228782,1642.91895559865,1643.35382890963,1643.78870222074,1644.223575532,
1645.09332215494,1645.52819546661,1645.96392146936,1646.39964747212,1646.83452078406,
1647.26939409614,1647.70426740834,1648.57401403314,1649.44376065844,1650.31350728422,
1650.74838059729,1651.18325391046,1652.05300053714,1652.92359985428,1653.79419917162,
1654.66394579929,1655.5336924273,1656.40343905563,1657.27318568424,1658.14293231311,
1659.01267894219,1659.88327826096,1660.75387757982,1661.62362420926,1662.49337083877,
1663.3631174683,1664.23286409781,1665.10261072725,1665.97235735658,1666.84295667531,
1667.71355599396,1668.58330262282,1669.45304925143,1670.32279587976,1671.19254250778,
1672.06228913544,1672.93203576273,1673.80263507977,1674.6732343966,1675.54298102284,
1676.41272764862,1677.28247427392,1678.15222089872,1679.021967523,1679.89171414676,
1680.76231346105,1681.19803946366,1681.63291277506,1682.06778608632,1682.50265939743,
1682.93753270841,1683.37240601924,1684.24215264047,1684.67702595086,1685.11189926111,
1685.54677257121,1685.98164588116,1686.41651919097,1686.85139250063,1687.28626581014,
1687.72199181166,1688.15771781319,1688.5925911224,1689.02746443146,1689.46233774038,
1689.89721104914,1690.33208435776,1690.76695766623,1691.20183097455,1691.63670428272,
1692.07157759075,1692.50645089864,1692.94132420637,1693.37619751397,1693.81107082142,
1694.24594412873,1694.68167012916,1695.11739612959,1695.55226943662,1695.9871427435,
1696.42201605025,1696.85688935687,1697.29176266334,1697.72663596969,1698.1615092759,
1698.59638258198,1699.03125588793,1699.46612919375,1699.90100249945,1700.33587580502,
1700.77074911047,1701.20562241579,1701.64134841525,1702.0770744147,1702.51194771979,
1702.94682102476,1703.38169432963,1703.81656763438,1704.25144093902,1704.68631424356,
1705.12118754799,1705.55606085232,1705.99093415655,1706.42580746068,1706.86068076471,
1707.29555406866,1707.73042737251,1708.16530067627,1708.60102667496,1709.03675267365,
1709.47162597724,1709.90649928076,1710.34137258419,1710.77624588756,1711.21111919085,
1711.64599249406,1712.08086579722,1712.5157391003,1712.95061240333,1713.3854857063,
1713.82035900921,1714.25523231207,1714.69010561487,1715.12497891763,1715.56070491584,
1715.99643091404,1716.43130421671,1716.86617751935,1717.30105082195,1717.73592412451,
1718.17079742705,1718.60567072956,1719.04054403204,1719.4754173345,1719.91029063695,
1720.34516393938,1720.7800372418,1721.21491054421,1721.64978384661,1722.08465714901,
1722.52038314706,1722.9561091451,1723.39098244751,1723.82585574992,1724.26072905233,
1724.69560235476,1725.13047565721,1725.56534895967,1726.00022226216,1726.43509556467,
1726.8699688672,1727.30484216977,1727.73971547236,1728.174588775,1728.60946207767,
1729.04433538039,1729.48006137861,1729.91578737684,1730.35066067965,1730.78553398251,
1731.22040728542,1731.65528058838,1732.09015389141,1732.5250271945,1732.95990049765,
1733.39477380087,1733.82964710416,1734.26452040752,1734.69939371096,1735.13426701447,
1735.56914031807,1736.00401362175,1736.43973962048,1736.8754656192,1737.31033892306,
1737.745212227,1738.18008553104,1738.61495883517,1739.0498321394,1739.48470544373,
1739.91957874816,1740.35445205269,1740.78932535734,1741.22419866209,1741.65907196695,
1742.09394527193,1742.52881857702,1742.96369188223,1743.39941788174,1743.83514388125,
1744.2700171867,1744.70489049227,1745.13976379797,1745.57463710379,1746.00951040974,
1746.44438371582,1746.87925702203,1747.31413032837,1747.74900363485,1748.18387694146,
1748.61875024821,1749.0536235551,1749.48849686213,1749.92337016929,1750.3590961698,
1750.7948221703,1751.22969547775,1751.66456878534,1752.09944209308,1752.53431540096,
1752.96918870899,1753.40406201717,1753.83893532549,1754.27380863396,1754.70868194258,
1755.14355525134,1755.57842856026,1756.01330186932,1756.44817517853,1756.88304848789,
1757.31877448949,1757.75450049109,1758.18937380075,1759.05912042051,1759.49399373061,
1759.92886704086,1760.36374035125,1760.79861366179,1761.23348697248,1761.66836028331,
1762.10323359429,1762.5381069054,1763.40785352806,1763.8427268396,1764.27845284228,
1764.71417884496,1765.14905215677,1765.58392546872,1766.0187987808,1766.88854540534,
1767.75829203039,1768.1931653431,1768.62803865593,1769.06291196888,1769.49778528195,
1770.36753190841,1771.2381312254,1772.10873054259,1772.97847717007,1773.84822379791,
1774.71797042609,1775.58771705456,1776.45746368331,1777.32721031228,1778.19780963089,
1779.06840894783,1779.93815555508,1780.80790201176,1781.67764871408),(-0.58309518948453,
3.80976832182013E-10),.UNSPECIFIED.) ;
#824=B_SPLINE_SURFACE_WITH_KNOTS('',3,1,((#57502,#57503),(#57504,#57505),
(#57506,#57507),(#57508,#57509),(#57510,#57511),(#57512,#57513),(#57514,
#57515),(#57516,#57517),(#57518,#57519),(#57520,#57521),(#57522,#57523),
(#57524,#57525),(#57526,#57527),(#57528,#57529),(#57530,#57531),(#57532,
#57533),(#57534,#57535),(#57536,#57537),(#57538,#57539),(#57540,#57541),
(#57542,#57543),(#57544,#57545),(#57546,#57547),(#57548,#57549),(#57550,
#57551),(#57552,#57553),(#57554,#57555),(#57556,#57557),(#57558,#57559),
(#57560,#57561),(#57562,#57563),(#57564,#57565),(#57566,#57567),(#57568,
#57569),(#57570,#57571),(#57572,#57573),(#57574,#57575),(#57576,#57577),
(#57578,#57579),(#57580,#57581),(#57582,#57583),(#57584,#57585),(#57586,
#57587),(#57588,#57589),(#57590,#57591),(#57592,#57593),(#57594,#57595),
(#57596,#57597),(#57598,#57599),(#57600,#57601),(#57602,#57603),(#57604,
#57605),(#57606,#57607),(#57608,#57609),(#57610,#57611),(#57612,#57613),
(#57614,#57615),(#57616,#57617),(#57618,#57619),(#57620,#57621),(#57622,
#57623),(#57624,#57625),(#57626,#57627),(#57628,#57629),(#57630,#57631),
(#57632,#57633),(#57634,#57635),(#57636,#57637),(#57638,#57639),(#57640,
#57641),(#57642,#57643),(#57644,#57645),(#57646,#57647),(#57648,#57649),
(#57650,#57651),(#57652,#57653),(#57654,#57655),(#57656,#57657),(#57658,
#57659),(#57660,#57661),(#57662,#57663),(#57664,#57665),(#57666,#57667),
(#57668,#57669),(#57670,#57671),(#57672,#57673),(#57674,#57675),(#57676,
#57677),(#57678,#57679),(#57680,#57681),(#57682,#57683),(#57684,#57685),
(#57686,#57687),(#57688,#57689),(#57690,#57691),(#57692,#57693),(#57694,
#57695),(#57696,#57697),(#57698,#57699),(#57700,#57701),(#57702,#57703),
(#57704,#57705),(#57706,#57707),(#57708,#57709),(#57710,#57711),(#57712,
#57713),(#57714,#57715),(#57716,#57717),(#57718,#57719),(#57720,#57721),
(#57722,#57723),(#57724,#57725),(#57726,#57727),(#57728,#57729),(#57730,
#57731),(#57732,#57733),(#57734,#57735),(#57736,#57737),(#57738,#57739),
(#57740,#57741),(#57742,#57743),(#57744,#57745),(#57746,#57747),(#57748,
#57749),(#57750,#57751),(#57752,#57753),(#57754,#57755),(#57756,#57757),
(#57758,#57759),(#57760,#57761),(#57762,#57763),(#57764,#57765),(#57766,
#57767),(#57768,#57769),(#57770,#57771),(#57772,#57773),(#57774,#57775),
(#57776,#57777),(#57778,#57779),(#57780,#57781),(#57782,#57783),(#57784,
#57785),(#57786,#57787),(#57788,#57789),(#57790,#57791),(#57792,#57793),
(#57794,#57795),(#57796,#57797),(#57798,#57799),(#57800,#57801),(#57802,
#57803),(#57804,#57805),(#57806,#57807),(#57808,#57809),(#57810,#57811),
(#57812,#57813),(#57814,#57815),(#57816,#57817),(#57818,#57819),(#57820,
#57821),(#57822,#57823),(#57824,#57825),(#57826,#57827),(#57828,#57829),
(#57830,#57831),(#57832,#57833),(#57834,#57835),(#57836,#57837),(#57838,
#57839),(#57840,#57841),(#57842,#57843),(#57844,#57845),(#57846,#57847),
(#57848,#57849),(#57850,#57851),(#57852,#57853),(#57854,#57855),(#57856,
#57857),(#57858,#57859),(#57860,#57861),(#57862,#57863),(#57864,#57865),
(#57866,#57867),(#57868,#57869),(#57870,#57871),(#57872,#57873),(#57874,
#57875),(#57876,#57877),(#57878,#57879),(#57880,#57881),(#57882,#57883),
(#57884,#57885),(#57886,#57887),(#57888,#57889),(#57890,#57891),(#57892,
#57893),(#57894,#57895),(#57896,#57897),(#57898,#57899),(#57900,#57901),
(#57902,#57903),(#57904,#57905),(#57906,#57907),(#57908,#57909),(#57910,
#57911),(#57912,#57913),(#57914,#57915),(#57916,#57917),(#57918,#57919),
(#57920,#57921),(#57922,#57923),(#57924,#57925),(#57926,#57927),(#57928,
#57929),(#57930,#57931),(#57932,#57933),(#57934,#57935),(#57936,#57937),
(#57938,#57939),(#57940,#57941),(#57942,#57943),(#57944,#57945),(#57946,
#57947),(#57948,#57949),(#57950,#57951),(#57952,#57953),(#57954,#57955),
(#57956,#57957),(#57958,#57959),(#57960,#57961),(#57962,#57963),(#57964,
#57965),(#57966,#57967),(#57968,#57969),(#57970,#57971),(#57972,#57973),
(#57974,#57975),(#57976,#57977),(#57978,#57979),(#57980,#57981),(#57982,
#57983),(#57984,#57985),(#57986,#57987),(#57988,#57989),(#57990,#57991),
(#57992,#57993),(#57994,#57995),(#57996,#57997),(#57998,#57999),(#58000,
#58001),(#58002,#58003),(#58004,#58005),(#58006,#58007),(#58008,#58009),
(#58010,#58011),(#58012,#58013),(#58014,#58015),(#58016,#58017),(#58018,
#58019),(#58020,#58021),(#58022,#58023),(#58024,#58025),(#58026,#58027),
(#58028,#58029),(#58030,#58031),(#58032,#58033),(#58034,#58035),(#58036,
#58037),(#58038,#58039),(#58040,#58041),(#58042,#58043),(#58044,#58045),
(#58046,#58047),(#58048,#58049),(#58050,#58051),(#58052,#58053),(#58054,
#58055),(#58056,#58057),(#58058,#58059),(#58060,#58061),(#58062,#58063),
(#58064,#58065),(#58066,#58067),(#58068,#58069),(#58070,#58071),(#58072,
#58073),(#58074,#58075),(#58076,#58077),(#58078,#58079),(#58080,#58081),
(#58082,#58083),(#58084,#58085),(#58086,#58087),(#58088,#58089),(#58090,
#58091),(#58092,#58093),(#58094,#58095),(#58096,#58097),(#58098,#58099),
(#58100,#58101),(#58102,#58103),(#58104,#58105),(#58106,#58107),(#58108,
#58109),(#58110,#58111),(#58112,#58113),(#58114,#58115),(#58116,#58117),
(#58118,#58119),(#58120,#58121),(#58122,#58123),(#58124,#58125),(#58126,
#58127),(#58128,#58129),(#58130,#58131),(#58132,#58133),(#58134,#58135),
(#58136,#58137),(#58138,#58139),(#58140,#58141),(#58142,#58143),(#58144,
#58145),(#58146,#58147),(#58148,#58149),(#58150,#58151),(#58152,#58153),
(#58154,#58155),(#58156,#58157),(#58158,#58159),(#58160,#58161),(#58162,
#58163),(#58164,#58165),(#58166,#58167),(#58168,#58169),(#58170,#58171),
(#58172,#58173),(#58174,#58175),(#58176,#58177),(#58178,#58179),(#58180,
#58181),(#58182,#58183),(#58184,#58185),(#58186,#58187),(#58188,#58189),
(#58190,#58191),(#58192,#58193),(#58194,#58195),(#58196,#58197),(#58198,
#58199),(#58200,#58201),(#58202,#58203),(#58204,#58205),(#58206,#58207),
(#58208,#58209),(#58210,#58211),(#58212,#58213),(#58214,#58215),(#58216,
#58217),(#58218,#58219),(#58220,#58221),(#58222,#58223),(#58224,#58225),
(#58226,#58227),(#58228,#58229),(#58230,#58231),(#58232,#58233),(#58234,
#58235),(#58236,#58237),(#58238,#58239),(#58240,#58241),(#58242,#58243),
(#58244,#58245),(#58246,#58247),(#58248,#58249),(#58250,#58251),(#58252,
#58253),(#58254,#58255),(#58256,#58257),(#58258,#58259),(#58260,#58261),
(#58262,#58263),(#58264,#58265),(#58266,#58267),(#58268,#58269),(#58270,
#58271),(#58272,#58273),(#58274,#58275),(#58276,#58277),(#58278,#58279),
(#58280,#58281),(#58282,#58283),(#58284,#58285),(#58286,#58287),(#58288,
#58289),(#58290,#58291),(#58292,#58293),(#58294,#58295),(#58296,#58297),
(#58298,#58299),(#58300,#58301),(#58302,#58303),(#58304,#58305),(#58306,
#58307),(#58308,#58309),(#58310,#58311),(#58312,#58313),(#58314,#58315),
(#58316,#58317),(#58318,#58319),(#58320,#58321),(#58322,#58323),(#58324,
#58325),(#58326,#58327),(#58328,#58329),(#58330,#58331),(#58332,#58333),
(#58334,#58335),(#58336,#58337),(#58338,#58339),(#58340,#58341),(#58342,
#58343),(#58344,#58345),(#58346,#58347),(#58348,#58349),(#58350,#58351),
(#58352,#58353),(#58354,#58355),(#58356,#58357),(#58358,#58359),(#58360,
#58361),(#58362,#58363),(#58364,#58365),(#58366,#58367),(#58368,#58369),
(#58370,#58371),(#58372,#58373),(#58374,#58375),(#58376,#58377),(#58378,
#58379),(#58380,#58381),(#58382,#58383),(#58384,#58385),(#58386,#58387),
(#58388,#58389),(#58390,#58391),(#58392,#58393),(#58394,#58395),(#58396,
#58397),(#58398,#58399),(#58400,#58401),(#58402,#58403),(#58404,#58405),
(#58406,#58407),(#58408,#58409),(#58410,#58411),(#58412,#58413),(#58414,
#58415),(#58416,#58417),(#58418,#58419),(#58420,#58421),(#58422,#58423),
(#58424,#58425),(#58426,#58427),(#58428,#58429),(#58430,#58431),(#58432,
#58433),(#58434,#58435),(#58436,#58437),(#58438,#58439),(#58440,#58441),
(#58442,#58443),(#58444,#58445),(#58446,#58447),(#58448,#58449),(#58450,
#58451),(#58452,#58453),(#58454,#58455),(#58456,#58457),(#58458,#58459),
(#58460,#58461),(#58462,#58463),(#58464,#58465),(#58466,#58467),(#58468,
#58469),(#58470,#58471),(#58472,#58473),(#58474,#58475),(#58476,#58477),
(#58478,#58479),(#58480,#58481),(#58482,#58483),(#58484,#58485),(#58486,
#58487),(#58488,#58489),(#58490,#58491),(#58492,#58493),(#58494,#58495),
(#58496,#58497),(#58498,#58499),(#58500,#58501),(#58502,#58503),(#58504,
#58505),(#58506,#58507),(#58508,#58509),(#58510,#58511),(#58512,#58513),
(#58514,#58515),(#58516,#58517),(#58518,#58519),(#58520,#58521),(#58522,
#58523),(#58524,#58525),(#58526,#58527),(#58528,#58529),(#58530,#58531),
(#58532,#58533),(#58534,#58535),(#58536,#58537),(#58538,#58539),(#58540,
#58541),(#58542,#58543),(#58544,#58545),(#58546,#58547),(#58548,#58549),
(#58550,#58551),(#58552,#58553),(#58554,#58555),(#58556,#58557),(#58558,
#58559),(#58560,#58561),(#58562,#58563),(#58564,#58565),(#58566,#58567),
(#58568,#58569),(#58570,#58571),(#58572,#58573),(#58574,#58575),(#58576,
#58577),(#58578,#58579),(#58580,#58581),(#58582,#58583),(#58584,#58585),
(#58586,#58587),(#58588,#58589),(#58590,#58591),(#58592,#58593),(#58594,
#58595),(#58596,#58597),(#58598,#58599),(#58600,#58601),(#58602,#58603),
(#58604,#58605),(#58606,#58607),(#58608,#58609),(#58610,#58611),(#58612,
#58613),(#58614,#58615),(#58616,#58617),(#58618,#58619),(#58620,#58621),
(#58622,#58623),(#58624,#58625),(#58626,#58627),(#58628,#58629),(#58630,
#58631),(#58632,#58633),(#58634,#58635),(#58636,#58637),(#58638,#58639),
(#58640,#58641),(#58642,#58643),(#58644,#58645),(#58646,#58647),(#58648,
#58649),(#58650,#58651),(#58652,#58653),(#58654,#58655),(#58656,#58657),
(#58658,#58659),(#58660,#58661),(#58662,#58663),(#58664,#58665),(#58666,
#58667),(#58668,#58669),(#58670,#58671),(#58672,#58673),(#58674,#58675),
(#58676,#58677),(#58678,#58679),(#58680,#58681),(#58682,#58683),(#58684,
#58685),(#58686,#58687),(#58688,#58689),(#58690,#58691),(#58692,#58693),
(#58694,#58695),(#58696,#58697),(#58698,#58699),(#58700,#58701),(#58702,
#58703),(#58704,#58705),(#58706,#58707),(#58708,#58709),(#58710,#58711),
(#58712,#58713),(#58714,#58715),(#58716,#58717),(#58718,#58719),(#58720,
#58721),(#58722,#58723),(#58724,#58725),(#58726,#58727),(#58728,#58729),
(#58730,#58731),(#58732,#58733),(#58734,#58735),(#58736,#58737),(#58738,
#58739),(#58740,#58741),(#58742,#58743),(#58744,#58745),(#58746,#58747),
(#58748,#58749),(#58750,#58751),(#58752,#58753),(#58754,#58755),(#58756,
#58757),(#58758,#58759),(#58760,#58761),(#58762,#58763),(#58764,#58765),
(#58766,#58767),(#58768,#58769),(#58770,#58771),(#58772,#58773),(#58774,
#58775),(#58776,#58777),(#58778,#58779),(#58780,#58781),(#58782,#58783),
(#58784,#58785),(#58786,#58787),(#58788,#58789),(#58790,#58791),(#58792,
#58793),(#58794,#58795),(#58796,#58797),(#58798,#58799),(#58800,#58801),
(#58802,#58803),(#58804,#58805),(#58806,#58807),(#58808,#58809),(#58810,
#58811),(#58812,#58813),(#58814,#58815),(#58816,#58817),(#58818,#58819),
(#58820,#58821),(#58822,#58823),(#58824,#58825),(#58826,#58827),(#58828,
#58829),(#58830,#58831),(#58832,#58833),(#58834,#58835),(#58836,#58837),
(#58838,#58839),(#58840,#58841),(#58842,#58843),(#58844,#58845),(#58846,
#58847),(#58848,#58849),(#58850,#58851),(#58852,#58853),(#58854,#58855),
(#58856,#58857),(#58858,#58859),(#58860,#58861),(#58862,#58863),(#58864,
#58865),(#58866,#58867),(#58868,#58869),(#58870,#58871),(#58872,#58873),
(#58874,#58875),(#58876,#58877),(#58878,#58879),(#58880,#58881),(#58882,
#58883),(#58884,#58885),(#58886,#58887),(#58888,#58889),(#58890,#58891),
(#58892,#58893),(#58894,#58895),(#58896,#58897),(#58898,#58899),(#58900,
#58901),(#58902,#58903),(#58904,#58905),(#58906,#58907),(#58908,#58909),
(#58910,#58911),(#58912,#58913),(#58914,#58915),(#58916,#58917),(#58918,
#58919),(#58920,#58921),(#58922,#58923),(#58924,#58925),(#58926,#58927),
(#58928,#58929),(#58930,#58931),(#58932,#58933),(#58934,#58935),(#58936,
#58937),(#58938,#58939),(#58940,#58941),(#58942,#58943),(#58944,#58945),
(#58946,#58947),(#58948,#58949),(#58950,#58951),(#58952,#58953),(#58954,
#58955),(#58956,#58957),(#58958,#58959),(#58960,#58961),(#58962,#58963),
(#58964,#58965),(#58966,#58967),(#58968,#58969),(#58970,#58971),(#58972,
#58973),(#58974,#58975),(#58976,#58977),(#58978,#58979),(#58980,#58981),
(#58982,#58983),(#58984,#58985),(#58986,#58987),(#58988,#58989),(#58990,
#58991),(#58992,#58993),(#58994,#58995),(#58996,#58997),(#58998,#58999),
(#59000,#59001),(#59002,#59003),(#59004,#59005),(#59006,#59007),(#59008,
#59009),(#59010,#59011),(#59012,#59013),(#59014,#59015),(#59016,#59017),
(#59018,#59019),(#59020,#59021),(#59022,#59023),(#59024,#59025),(#59026,
#59027),(#59028,#59029),(#59030,#59031),(#59032,#59033),(#59034,#59035),
(#59036,#59037),(#59038,#59039),(#59040,#59041),(#59042,#59043),(#59044,
#59045),(#59046,#59047),(#59048,#59049),(#59050,#59051),(#59052,#59053),
(#59054,#59055),(#59056,#59057),(#59058,#59059),(#59060,#59061),(#59062,
#59063),(#59064,#59065),(#59066,#59067),(#59068,#59069),(#59070,#59071),
(#59072,#59073),(#59074,#59075),(#59076,#59077),(#59078,#59079),(#59080,
#59081),(#59082,#59083),(#59084,#59085),(#59086,#59087),(#59088,#59089),
(#59090,#59091),(#59092,#59093),(#59094,#59095),(#59096,#59097),(#59098,
#59099),(#59100,#59101),(#59102,#59103),(#59104,#59105),(#59106,#59107),
(#59108,#59109),(#59110,#59111),(#59112,#59113),(#59114,#59115),(#59116,
#59117),(#59118,#59119),(#59120,#59121),(#59122,#59123),(#59124,#59125),
(#59126,#59127),(#59128,#59129),(#59130,#59131),(#59132,#59133),(#59134,
#59135),(#59136,#59137),(#59138,#59139),(#59140,#59141),(#59142,#59143),
(#59144,#59145),(#59146,#59147),(#59148,#59149),(#59150,#59151),(#59152,
#59153),(#59154,#59155),(#59156,#59157),(#59158,#59159),(#59160,#59161),
(#59162,#59163),(#59164,#59165),(#59166,#59167),(#59168,#59169),(#59170,
#59171),(#59172,#59173),(#59174,#59175),(#59176,#59177),(#59178,#59179),
(#59180,#59181),(#59182,#59183),(#59184,#59185),(#59186,#59187),(#59188,
#59189),(#59190,#59191),(#59192,#59193),(#59194,#59195),(#59196,#59197),
(#59198,#59199),(#59200,#59201),(#59202,#59203),(#59204,#59205),(#59206,
#59207),(#59208,#59209),(#59210,#59211),(#59212,#59213),(#59214,#59215),
(#59216,#59217),(#59218,#59219),(#59220,#59221),(#59222,#59223),(#59224,
#59225),(#59226,#59227),(#59228,#59229),(#59230,#59231),(#59232,#59233),
(#59234,#59235),(#59236,#59237),(#59238,#59239),(#59240,#59241),(#59242,
#59243),(#59244,#59245),(#59246,#59247),(#59248,#59249),(#59250,#59251),
(#59252,#59253),(#59254,#59255),(#59256,#59257),(#59258,#59259),(#59260,
#59261),(#59262,#59263),(#59264,#59265),(#59266,#59267),(#59268,#59269),
(#59270,#59271),(#59272,#59273),(#59274,#59275),(#59276,#59277),(#59278,
#59279),(#59280,#59281),(#59282,#59283),(#59284,#59285),(#59286,#59287),
(#59288,#59289),(#59290,#59291),(#59292,#59293),(#59294,#59295),(#59296,
#59297),(#59298,#59299),(#59300,#59301),(#59302,#59303),(#59304,#59305),
(#59306,#59307),(#59308,#59309),(#59310,#59311),(#59312,#59313),(#59314,
#59315),(#59316,#59317),(#59318,#59319),(#59320,#59321),(#59322,#59323),
(#59324,#59325),(#59326,#59327),(#59328,#59329),(#59330,#59331),(#59332,
#59333),(#59334,#59335),(#59336,#59337),(#59338,#59339),(#59340,#59341),
(#59342,#59343),(#59344,#59345),(#59346,#59347),(#59348,#59349),(#59350,
#59351),(#59352,#59353),(#59354,#59355),(#59356,#59357),(#59358,#59359),
(#59360,#59361),(#59362,#59363),(#59364,#59365),(#59366,#59367),(#59368,
#59369),(#59370,#59371),(#59372,#59373),(#59374,#59375),(#59376,#59377),
(#59378,#59379),(#59380,#59381),(#59382,#59383),(#59384,#59385),(#59386,
#59387),(#59388,#59389),(#59390,#59391),(#59392,#59393),(#59394,#59395),
(#59396,#59397),(#59398,#59399),(#59400,#59401),(#59402,#59403),(#59404,
#59405),(#59406,#59407),(#59408,#59409),(#59410,#59411),(#59412,#59413),
(#59414,#59415),(#59416,#59417),(#59418,#59419),(#59420,#59421),(#59422,
#59423),(#59424,#59425),(#59426,#59427),(#59428,#59429),(#59430,#59431),
(#59432,#59433),(#59434,#59435),(#59436,#59437),(#59438,#59439),(#59440,
#59441),(#59442,#59443),(#59444,#59445),(#59446,#59447),(#59448,#59449),
(#59450,#59451),(#59452,#59453),(#59454,#59455),(#59456,#59457),(#59458,
#59459),(#59460,#59461),(#59462,#59463),(#59464,#59465),(#59466,#59467),
(#59468,#59469),(#59470,#59471),(#59472,#59473),(#59474,#59475),(#59476,
#59477),(#59478,#59479),(#59480,#59481),(#59482,#59483),(#59484,#59485),
(#59486,#59487),(#59488,#59489),(#59490,#59491),(#59492,#59493),(#59494,
#59495),(#59496,#59497),(#59498,#59499),(#59500,#59501),(#59502,#59503),
(#59504,#59505),(#59506,#59507),(#59508,#59509),(#59510,#59511),(#59512,
#59513),(#59514,#59515),(#59516,#59517),(#59518,#59519),(#59520,#59521),
(#59522,#59523),(#59524,#59525),(#59526,#59527),(#59528,#59529),(#59530,
#59531),(#59532,#59533),(#59534,#59535),(#59536,#59537),(#59538,#59539),
(#59540,#59541),(#59542,#59543),(#59544,#59545),(#59546,#59547),(#59548,
#59549),(#59550,#59551),(#59552,#59553),(#59554,#59555),(#59556,#59557),
(#59558,#59559),(#59560,#59561),(#59562,#59563),(#59564,#59565),(#59566,
#59567),(#59568,#59569),(#59570,#59571),(#59572,#59573),(#59574,#59575),
(#59576,#59577),(#59578,#59579),(#59580,#59581),(#59582,#59583),(#59584,
#59585),(#59586,#59587),(#59588,#59589),(#59590,#59591),(#59592,#59593),
(#59594,#59595),(#59596,#59597),(#59598,#59599),(#59600,#59601),(#59602,
#59603),(#59604,#59605),(#59606,#59607),(#59608,#59609),(#59610,#59611),
(#59612,#59613),(#59614,#59615),(#59616,#59617),(#59618,#59619),(#59620,
#59621),(#59622,#59623),(#59624,#59625),(#59626,#59627),(#59628,#59629),
(#59630,#59631),(#59632,#59633),(#59634,#59635),(#59636,#59637),(#59638,
#59639),(#59640,#59641),(#59642,#59643),(#59644,#59645),(#59646,#59647),
(#59648,#59649),(#59650,#59651),(#59652,#59653),(#59654,#59655),(#59656,
#59657),(#59658,#59659),(#59660,#59661),(#59662,#59663),(#59664,#59665),
(#59666,#59667),(#59668,#59669),(#59670,#59671),(#59672,#59673),(#59674,
#59675),(#59676,#59677),(#59678,#59679),(#59680,#59681),(#59682,#59683),
(#59684,#59685),(#59686,#59687),(#59688,#59689),(#59690,#59691),(#59692,
#59693),(#59694,#59695),(#59696,#59697),(#59698,#59699),(#59700,#59701),
(#59702,#59703),(#59704,#59705),(#59706,#59707),(#59708,#59709),(#59710,
#59711),(#59712,#59713),(#59714,#59715),(#59716,#59717),(#59718,#59719),
(#59720,#59721),(#59722,#59723),(#59724,#59725),(#59726,#59727),(#59728,
#59729),(#59730,#59731),(#59732,#59733),(#59734,#59735),(#59736,#59737),
(#59738,#59739),(#59740,#59741),(#59742,#59743),(#59744,#59745),(#59746,
#59747),(#59748,#59749),(#59750,#59751),(#59752,#59753),(#59754,#59755),
(#59756,#59757),(#59758,#59759),(#59760,#59761),(#59762,#59763),(#59764,
#59765),(#59766,#59767),(#59768,#59769),(#59770,#59771),(#59772,#59773),
(#59774,#59775),(#59776,#59777),(#59778,#59779),(#59780,#59781),(#59782,
#59783),(#59784,#59785),(#59786,#59787),(#59788,#59789),(#59790,#59791),
(#59792,#59793),(#59794,#59795),(#59796,#59797),(#59798,#59799),(#59800,
#59801),(#59802,#59803),(#59804,#59805),(#59806,#59807),(#59808,#59809),
(#59810,#59811),(#59812,#59813),(#59814,#59815),(#59816,#59817),(#59818,
#59819),(#59820,#59821),(#59822,#59823),(#59824,#59825),(#59826,#59827),
(#59828,#59829),(#59830,#59831),(#59832,#59833),(#59834,#59835),(#59836,
#59837),(#59838,#59839),(#59840,#59841),(#59842,#59843),(#59844,#59845),
(#59846,#59847),(#59848,#59849),(#59850,#59851),(#59852,#59853),(#59854,
#59855),(#59856,#59857),(#59858,#59859),(#59860,#59861),(#59862,#59863),
(#59864,#59865),(#59866,#59867),(#59868,#59869),(#59870,#59871),(#59872,
#59873),(#59874,#59875),(#59876,#59877),(#59878,#59879),(#59880,#59881),
(#59882,#59883),(#59884,#59885),(#59886,#59887),(#59888,#59889),(#59890,
#59891),(#59892,#59893),(#59894,#59895),(#59896,#59897),(#59898,#59899),
(#59900,#59901),(#59902,#59903),(#59904,#59905),(#59906,#59907),(#59908,
#59909),(#59910,#59911),(#59912,#59913),(#59914,#59915),(#59916,#59917),
(#59918,#59919),(#59920,#59921),(#59922,#59923),(#59924,#59925),(#59926,
#59927),(#59928,#59929),(#59930,#59931),(#59932,#59933),(#59934,#59935),
(#59936,#59937),(#59938,#59939),(#59940,#59941),(#59942,#59943),(#59944,
#59945),(#59946,#59947),(#59948,#59949),(#59950,#59951),(#59952,#59953),
(#59954,#59955),(#59956,#59957),(#59958,#59959),(#59960,#59961),(#59962,
#59963),(#59964,#59965),(#59966,#59967),(#59968,#59969),(#59970,#59971),
(#59972,#59973),(#59974,#59975),(#59976,#59977),(#59978,#59979),(#59980,
#59981),(#59982,#59983),(#59984,#59985),(#59986,#59987),(#59988,#59989),
(#59990,#59991),(#59992,#59993),(#59994,#59995),(#59996,#59997),(#59998,
#59999),(#60000,#60001),(#60002,#60003),(#60004,#60005),(#60006,#60007),
(#60008,#60009),(#60010,#60011),(#60012,#60013),(#60014,#60015),(#60016,
#60017),(#60018,#60019),(#60020,#60021),(#60022,#60023),(#60024,#60025),
(#60026,#60027),(#60028,#60029),(#60030,#60031),(#60032,#60033),(#60034,
#60035),(#60036,#60037),(#60038,#60039),(#60040,#60041),(#60042,#60043),
(#60044,#60045),(#60046,#60047),(#60048,#60049),(#60050,#60051),(#60052,
#60053),(#60054,#60055),(#60056,#60057),(#60058,#60059),(#60060,#60061),
(#60062,#60063),(#60064,#60065),(#60066,#60067),(#60068,#60069),(#60070,
#60071),(#60072,#60073),(#60074,#60075),(#60076,#60077),(#60078,#60079),
(#60080,#60081),(#60082,#60083),(#60084,#60085),(#60086,#60087),(#60088,
#60089),(#60090,#60091),(#60092,#60093),(#60094,#60095),(#60096,#60097),
(#60098,#60099),(#60100,#60101),(#60102,#60103),(#60104,#60105),(#60106,
#60107),(#60108,#60109),(#60110,#60111),(#60112,#60113),(#60114,#60115),
(#60116,#60117),(#60118,#60119),(#60120,#60121),(#60122,#60123),(#60124,
#60125),(#60126,#60127),(#60128,#60129),(#60130,#60131),(#60132,#60133),
(#60134,#60135),(#60136,#60137),(#60138,#60139),(#60140,#60141),(#60142,
#60143),(#60144,#60145),(#60146,#60147),(#60148,#60149),(#60150,#60151),
(#60152,#60153),(#60154,#60155),(#60156,#60157),(#60158,#60159),(#60160,
#60161),(#60162,#60163),(#60164,#60165),(#60166,#60167),(#60168,#60169),
(#60170,#60171),(#60172,#60173),(#60174,#60175),(#60176,#60177),(#60178,
#60179),(#60180,#60181),(#60182,#60183),(#60184,#60185),(#60186,#60187),
(#60188,#60189),(#60190,#60191),(#60192,#60193),(#60194,#60195),(#60196,
#60197),(#60198,#60199),(#60200,#60201),(#60202,#60203),(#60204,#60205),
(#60206,#60207),(#60208,#60209),(#60210,#60211),(#60212,#60213),(#60214,
#60215),(#60216,#60217),(#60218,#60219),(#60220,#60221),(#60222,#60223),
(#60224,#60225),(#60226,#60227),(#60228,#60229),(#60230,#60231),(#60232,
#60233),(#60234,#60235),(#60236,#60237),(#60238,#60239),(#60240,#60241),
(#60242,#60243),(#60244,#60245),(#60246,#60247),(#60248,#60249),(#60250,
#60251),(#60252,#60253),(#60254,#60255),(#60256,#60257),(#60258,#60259),
(#60260,#60261),(#60262,#60263),(#60264,#60265),(#60266,#60267),(#60268,
#60269),(#60270,#60271),(#60272,#60273),(#60274,#60275),(#60276,#60277),
(#60278,#60279),(#60280,#60281),(#60282,#60283),(#60284,#60285),(#60286,
#60287),(#60288,#60289),(#60290,#60291),(#60292,#60293),(#60294,#60295),
(#60296,#60297),(#60298,#60299),(#60300,#60301),(#60302,#60303),(#60304,
#60305),(#60306,#60307),(#60308,#60309),(#60310,#60311),(#60312,#60313),
(#60314,#60315),(#60316,#60317),(#60318,#60319),(#60320,#60321),(#60322,
#60323),(#60324,#60325),(#60326,#60327),(#60328,#60329),(#60330,#60331),
(#60332,#60333),(#60334,#60335),(#60336,#60337),(#60338,#60339),(#60340,
#60341),(#60342,#60343),(#60344,#60345),(#60346,#60347),(#60348,#60349),
(#60350,#60351),(#60352,#60353),(#60354,#60355),(#60356,#60357),(#60358,
#60359),(#60360,#60361),(#60362,#60363),(#60364,#60365),(#60366,#60367),
(#60368,#60369),(#60370,#60371),(#60372,#60373),(#60374,#60375),(#60376,
#60377),(#60378,#60379),(#60380,#60381),(#60382,#60383),(#60384,#60385),
(#60386,#60387),(#60388,#60389),(#60390,#60391),(#60392,#60393),(#60394,
#60395),(#60396,#60397),(#60398,#60399),(#60400,#60401),(#60402,#60403),
(#60404,#60405),(#60406,#60407),(#60408,#60409),(#60410,#60411),(#60412,
#60413),(#60414,#60415),(#60416,#60417),(#60418,#60419),(#60420,#60421),
(#60422,#60423),(#60424,#60425),(#60426,#60427),(#60428,#60429),(#60430,
#60431),(#60432,#60433),(#60434,#60435),(#60436,#60437),(#60438,#60439),
(#60440,#60441),(#60442,#60443),(#60444,#60445),(#60446,#60447),(#60448,
#60449),(#60450,#60451),(#60452,#60453),(#60454,#60455),(#60456,#60457),
(#60458,#60459),(#60460,#60461),(#60462,#60463),(#60464,#60465),(#60466,
#60467),(#60468,#60469),(#60470,#60471),(#60472,#60473),(#60474,#60475),
(#60476,#60477),(#60478,#60479),(#60480,#60481),(#60482,#60483),(#60484,
#60485),(#60486,#60487),(#60488,#60489),(#60490,#60491),(#60492,#60493),
(#60494,#60495),(#60496,#60497),(#60498,#60499),(#60500,#60501),(#60502,
#60503),(#60504,#60505),(#60506,#60507),(#60508,#60509),(#60510,#60511),
(#60512,#60513),(#60514,#60515),(#60516,#60517),(#60518,#60519),(#60520,
#60521),(#60522,#60523),(#60524,#60525),(#60526,#60527),(#60528,#60529),
(#60530,#60531),(#60532,#60533),(#60534,#60535),(#60536,#60537),(#60538,
#60539),(#60540,#60541),(#60542,#60543),(#60544,#60545),(#60546,#60547),
(#60548,#60549),(#60550,#60551),(#60552,#60553),(#60554,#60555),(#60556,
#60557),(#60558,#60559),(#60560,#60561),(#60562,#60563),(#60564,#60565),
(#60566,#60567),(#60568,#60569),(#60570,#60571),(#60572,#60573),(#60574,
#60575),(#60576,#60577),(#60578,#60579),(#60580,#60581),(#60582,#60583),
(#60584,#60585),(#60586,#60587),(#60588,#60589),(#60590,#60591),(#60592,
#60593),(#60594,#60595),(#60596,#60597),(#60598,#60599),(#60600,#60601),
(#60602,#60603),(#60604,#60605),(#60606,#60607),(#60608,#60609),(#60610,
#60611),(#60612,#60613),(#60614,#60615),(#60616,#60617),(#60618,#60619),
(#60620,#60621),(#60622,#60623),(#60624,#60625),(#60626,#60627),(#60628,
#60629),(#60630,#60631),(#60632,#60633),(#60634,#60635),(#60636,#60637),
(#60638,#60639),(#60640,#60641),(#60642,#60643),(#60644,#60645),(#60646,
#60647),(#60648,#60649),(#60650,#60651),(#60652,#60653),(#60654,#60655),
(#60656,#60657),(#60658,#60659),(#60660,#60661),(#60662,#60663),(#60664,
#60665),(#60666,#60667),(#60668,#60669),(#60670,#60671),(#60672,#60673),
(#60674,#60675),(#60676,#60677),(#60678,#60679),(#60680,#60681),(#60682,
#60683),(#60684,#60685),(#60686,#60687),(#60688,#60689),(#60690,#60691),
(#60692,#60693),(#60694,#60695),(#60696,#60697),(#60698,#60699),(#60700,
#60701),(#60702,#60703),(#60704,#60705),(#60706,#60707),(#60708,#60709),
(#60710,#60711),(#60712,#60713),(#60714,#60715),(#60716,#60717),(#60718,
#60719),(#60720,#60721),(#60722,#60723),(#60724,#60725),(#60726,#60727),
(#60728,#60729),(#60730,#60731),(#60732,#60733),(#60734,#60735),(#60736,
#60737),(#60738,#60739),(#60740,#60741),(#60742,#60743),(#60744,#60745),
(#60746,#60747),(#60748,#60749),(#60750,#60751),(#60752,#60753),(#60754,
#60755),(#60756,#60757),(#60758,#60759),(#60760,#60761),(#60762,#60763),
(#60764,#60765),(#60766,#60767),(#60768,#60769),(#60770,#60771),(#60772,
#60773),(#60774,#60775),(#60776,#60777),(#60778,#60779),(#60780,#60781),
(#60782,#60783),(#60784,#60785),(#60786,#60787),(#60788,#60789),(#60790,
#60791),(#60792,#60793),(#60794,#60795),(#60796,#60797),(#60798,#60799),
(#60800,#60801),(#60802,#60803),(#60804,#60805),(#60806,#60807),(#60808,
#60809),(#60810,#60811),(#60812,#60813),(#60814,#60815),(#60816,#60817),
(#60818,#60819),(#60820,#60821),(#60822,#60823),(#60824,#60825),(#60826,
#60827),(#60828,#60829),(#60830,#60831),(#60832,#60833),(#60834,#60835),
(#60836,#60837),(#60838,#60839),(#60840,#60841),(#60842,#60843),(#60844,
#60845),(#60846,#60847),(#60848,#60849),(#60850,#60851),(#60852,#60853),
(#60854,#60855),(#60856,#60857),(#60858,#60859),(#60860,#60861),(#60862,
#60863),(#60864,#60865),(#60866,#60867),(#60868,#60869),(#60870,#60871),
(#60872,#60873),(#60874,#60875),(#60876,#60877),(#60878,#60879),(#60880,
#60881),(#60882,#60883),(#60884,#60885),(#60886,#60887),(#60888,#60889),
(#60890,#60891),(#60892,#60893),(#60894,#60895),(#60896,#60897),(#60898,
#60899),(#60900,#60901),(#60902,#60903),(#60904,#60905),(#60906,#60907),
(#60908,#60909),(#60910,#60911),(#60912,#60913),(#60914,#60915),(#60916,
#60917),(#60918,#60919),(#60920,#60921),(#60922,#60923),(#60924,#60925),
(#60926,#60927),(#60928,#60929),(#60930,#60931),(#60932,#60933),(#60934,
#60935),(#60936,#60937),(#60938,#60939),(#60940,#60941),(#60942,#60943),
(#60944,#60945),(#60946,#60947),(#60948,#60949),(#60950,#60951),(#60952,
#60953),(#60954,#60955),(#60956,#60957),(#60958,#60959),(#60960,#60961),
(#60962,#60963),(#60964,#60965),(#60966,#60967),(#60968,#60969),(#60970,
#60971),(#60972,#60973),(#60974,#60975),(#60976,#60977),(#60978,#60979),
(#60980,#60981),(#60982,#60983),(#60984,#60985),(#60986,#60987),(#60988,
#60989),(#60990,#60991),(#60992,#60993),(#60994,#60995),(#60996,#60997),
(#60998,#60999),(#61000,#61001),(#61002,#61003),(#61004,#61005),(#61006,
#61007),(#61008,#61009),(#61010,#61011),(#61012,#61013),(#61014,#61015),
(#61016,#61017),(#61018,#61019),(#61020,#61021),(#61022,#61023),(#61024,
#61025),(#61026,#61027),(#61028,#61029),(#61030,#61031),(#61032,#61033),
(#61034,#61035),(#61036,#61037),(#61038,#61039),(#61040,#61041),(#61042,
#61043),(#61044,#61045),(#61046,#61047),(#61048,#61049),(#61050,#61051),
(#61052,#61053),(#61054,#61055),(#61056,#61057),(#61058,#61059),(#61060,
#61061),(#61062,#61063),(#61064,#61065),(#61066,#61067),(#61068,#61069),
(#61070,#61071),(#61072,#61073),(#61074,#61075),(#61076,#61077),(#61078,
#61079),(#61080,#61081),(#61082,#61083),(#61084,#61085),(#61086,#61087),
(#61088,#61089),(#61090,#61091),(#61092,#61093),(#61094,#61095),(#61096,
#61097),(#61098,#61099),(#61100,#61101),(#61102,#61103),(#61104,#61105),
(#61106,#61107),(#61108,#61109),(#61110,#61111),(#61112,#61113),(#61114,
#61115),(#61116,#61117),(#61118,#61119),(#61120,#61121),(#61122,#61123),
(#61124,#61125),(#61126,#61127),(#61128,#61129),(#61130,#61131),(#61132,
#61133),(#61134,#61135),(#61136,#61137),(#61138,#61139),(#61140,#61141),
(#61142,#61143),(#61144,#61145),(#61146,#61147),(#61148,#61149),(#61150,
#61151),(#61152,#61153),(#61154,#61155),(#61156,#61157),(#61158,#61159),
(#61160,#61161),(#61162,#61163),(#61164,#61165),(#61166,#61167),(#61168,
#61169),(#61170,#61171),(#61172,#61173),(#61174,#61175),(#61176,#61177),
(#61178,#61179),(#61180,#61181),(#61182,#61183),(#61184,#61185),(#61186,
#61187),(#61188,#61189),(#61190,#61191),(#61192,#61193),(#61194,#61195),
(#61196,#61197),(#61198,#61199),(#61200,#61201),(#61202,#61203),(#61204,
#61205),(#61206,#61207),(#61208,#61209),(#61210,#61211),(#61212,#61213),
(#61214,#61215),(#61216,#61217),(#61218,#61219),(#61220,#61221),(#61222,
#61223),(#61224,#61225),(#61226,#61227),(#61228,#61229),(#61230,#61231),
(#61232,#61233),(#61234,#61235),(#61236,#61237),(#61238,#61239),(#61240,
#61241),(#61242,#61243),(#61244,#61245),(#61246,#61247),(#61248,#61249),
(#61250,#61251),(#61252,#61253),(#61254,#61255),(#61256,#61257),(#61258,
#61259),(#61260,#61261),(#61262,#61263),(#61264,#61265),(#61266,#61267),
(#61268,#61269),(#61270,#61271),(#61272,#61273),(#61274,#61275),(#61276,
#61277),(#61278,#61279),(#61280,#61281),(#61282,#61283),(#61284,#61285),
(#61286,#61287),(#61288,#61289),(#61290,#61291),(#61292,#61293),(#61294,
#61295),(#61296,#61297),(#61298,#61299),(#61300,#61301),(#61302,#61303),
(#61304,#61305),(#61306,#61307),(#61308,#61309),(#61310,#61311),(#61312,
#61313),(#61314,#61315),(#61316,#61317),(#61318,#61319),(#61320,#61321),
(#61322,#61323),(#61324,#61325),(#61326,#61327),(#61328,#61329),(#61330,
#61331),(#61332,#61333),(#61334,#61335),(#61336,#61337),(#61338,#61339),
(#61340,#61341),(#61342,#61343),(#61344,#61345),(#61346,#61347),(#61348,
#61349),(#61350,#61351),(#61352,#61353),(#61354,#61355),(#61356,#61357),
(#61358,#61359),(#61360,#61361),(#61362,#61363),(#61364,#61365),(#61366,
#61367),(#61368,#61369),(#61370,#61371),(#61372,#61373),(#61374,#61375),
(#61376,#61377),(#61378,#61379),(#61380,#61381),(#61382,#61383),(#61384,
#61385),(#61386,#61387),(#61388,#61389),(#61390,#61391),(#61392,#61393),
(#61394,#61395),(#61396,#61397),(#61398,#61399),(#61400,#61401),(#61402,
#61403),(#61404,#61405),(#61406,#61407),(#61408,#61409),(#61410,#61411),
(#61412,#61413),(#61414,#61415),(#61416,#61417),(#61418,#61419),(#61420,
#61421),(#61422,#61423),(#61424,#61425),(#61426,#61427),(#61428,#61429),
(#61430,#61431),(#61432,#61433),(#61434,#61435),(#61436,#61437),(#61438,
#61439),(#61440,#61441),(#61442,#61443),(#61444,#61445),(#61446,#61447),
(#61448,#61449),(#61450,#61451),(#61452,#61453),(#61454,#61455),(#61456,
#61457),(#61458,#61459),(#61460,#61461),(#61462,#61463),(#61464,#61465),
(#61466,#61467),(#61468,#61469),(#61470,#61471),(#61472,#61473),(#61474,
#61475),(#61476,#61477),(#61478,#61479),(#61480,#61481),(#61482,#61483),
(#61484,#61485),(#61486,#61487),(#61488,#61489),(#61490,#61491),(#61492,
#61493),(#61494,#61495),(#61496,#61497),(#61498,#61499),(#61500,#61501),
(#61502,#61503),(#61504,#61505),(#61506,#61507),(#61508,#61509),(#61510,
#61511),(#61512,#61513),(#61514,#61515),(#61516,#61517),(#61518,#61519),
(#61520,#61521),(#61522,#61523),(#61524,#61525),(#61526,#61527),(#61528,
#61529),(#61530,#61531),(#61532,#61533),(#61534,#61535),(#61536,#61537),
(#61538,#61539),(#61540,#61541),(#61542,#61543),(#61544,#61545),(#61546,
#61547),(#61548,#61549),(#61550,#61551),(#61552,#61553),(#61554,#61555),
(#61556,#61557),(#61558,#61559),(#61560,#61561),(#61562,#61563),(#61564,
#61565),(#61566,#61567),(#61568,#61569),(#61570,#61571),(#61572,#61573),
(#61574,#61575),(#61576,#61577),(#61578,#61579),(#61580,#61581),(#61582,
#61583),(#61584,#61585),(#61586,#61587),(#61588,#61589),(#61590,#61591),
(#61592,#61593),(#61594,#61595),(#61596,#61597),(#61598,#61599),(#61600,
#61601),(#61602,#61603),(#61604,#61605),(#61606,#61607),(#61608,#61609),
(#61610,#61611),(#61612,#61613),(#61614,#61615),(#61616,#61617),(#61618,
#61619),(#61620,#61621),(#61622,#61623),(#61624,#61625),(#61626,#61627),
(#61628,#61629),(#61630,#61631),(#61632,#61633),(#61634,#61635),(#61636,
#61637),(#61638,#61639),(#61640,#61641),(#61642,#61643),(#61644,#61645),
(#61646,#61647),(#61648,#61649),(#61650,#61651),(#61652,#61653),(#61654,
#61655),(#61656,#61657),(#61658,#61659),(#61660,#61661),(#61662,#61663),
(#61664,#61665),(#61666,#61667),(#61668,#61669),(#61670,#61671),(#61672,
#61673),(#61674,#61675),(#61676,#61677),(#61678,#61679),(#61680,#61681),
(#61682,#61683),(#61684,#61685),(#61686,#61687),(#61688,#61689),(#61690,
#61691),(#61692,#61693),(#61694,#61695),(#61696,#61697),(#61698,#61699),
(#61700,#61701),(#61702,#61703),(#61704,#61705),(#61706,#61707),(#61708,
#61709),(#61710,#61711),(#61712,#61713),(#61714,#61715),(#61716,#61717),
(#61718,#61719),(#61720,#61721),(#61722,#61723),(#61724,#61725),(#61726,
#61727),(#61728,#61729),(#61730,#61731),(#61732,#61733),(#61734,#61735),
(#61736,#61737),(#61738,#61739),(#61740,#61741),(#61742,#61743),(#61744,
#61745),(#61746,#61747),(#61748,#61749),(#61750,#61751),(#61752,#61753),
(#61754,#61755),(#61756,#61757),(#61758,#61759),(#61760,#61761),(#61762,
#61763),(#61764,#61765),(#61766,#61767),(#61768,#61769),(#61770,#61771),
(#61772,#61773),(#61774,#61775),(#61776,#61777),(#61778,#61779),(#61780,
#61781),(#61782,#61783),(#61784,#61785),(#61786,#61787),(#61788,#61789),
(#61790,#61791),(#61792,#61793),(#61794,#61795),(#61796,#61797),(#61798,
#61799),(#61800,#61801),(#61802,#61803),(#61804,#61805),(#61806,#61807),
(#61808,#61809),(#61810,#61811),(#61812,#61813),(#61814,#61815),(#61816,
#61817),(#61818,#61819),(#61820,#61821),(#61822,#61823),(#61824,#61825),
(#61826,#61827),(#61828,#61829),(#61830,#61831),(#61832,#61833),(#61834,
#61835),(#61836,#61837),(#61838,#61839),(#61840,#61841),(#61842,#61843),
(#61844,#61845),(#61846,#61847),(#61848,#61849),(#61850,#61851),(#61852,
#61853),(#61854,#61855),(#61856,#61857),(#61858,#61859),(#61860,#61861),
(#61862,#61863),(#61864,#61865),(#61866,#61867),(#61868,#61869),(#61870,
#61871),(#61872,#61873),(#61874,#61875),(#61876,#61877),(#61878,#61879),
(#61880,#61881),(#61882,#61883),(#61884,#61885),(#61886,#61887),(#61888,
#61889),(#61890,#61891),(#61892,#61893),(#61894,#61895),(#61896,#61897),
(#61898,#61899),(#61900,#61901),(#61902,#61903),(#61904,#61905),(#61906,
#61907),(#61908,#61909),(#61910,#61911),(#61912,#61913),(#61914,#61915),
(#61916,#61917),(#61918,#61919),(#61920,#61921),(#61922,#61923),(#61924,
#61925),(#61926,#61927),(#61928,#61929),(#61930,#61931),(#61932,#61933),
(#61934,#61935),(#61936,#61937),(#61938,#61939),(#61940,#61941),(#61942,
#61943),(#61944,#61945),(#61946,#61947),(#61948,#61949),(#61950,#61951),
(#61952,#61953),(#61954,#61955),(#61956,#61957),(#61958,#61959),(#61960,
#61961),(#61962,#61963),(#61964,#61965),(#61966,#61967),(#61968,#61969),
(#61970,#61971),(#61972,#61973),(#61974,#61975),(#61976,#61977),(#61978,
#61979),(#61980,#61981),(#61982,#61983),(#61984,#61985),(#61986,#61987),
(#61988,#61989),(#61990,#61991),(#61992,#61993),(#61994,#61995),(#61996,
#61997),(#61998,#61999),(#62000,#62001),(#62002,#62003),(#62004,#62005),
(#62006,#62007),(#62008,#62009),(#62010,#62011),(#62012,#62013),(#62014,
#62015),(#62016,#62017),(#62018,#62019),(#62020,#62021),(#62022,#62023),
(#62024,#62025),(#62026,#62027),(#62028,#62029),(#62030,#62031),(#62032,
#62033),(#62034,#62035),(#62036,#62037),(#62038,#62039),(#62040,#62041),
(#62042,#62043),(#62044,#62045),(#62046,#62047),(#62048,#62049),(#62050,
#62051),(#62052,#62053),(#62054,#62055),(#62056,#62057),(#62058,#62059),
(#62060,#62061),(#62062,#62063),(#62064,#62065),(#62066,#62067),(#62068,
#62069),(#62070,#62071),(#62072,#62073),(#62074,#62075),(#62076,#62077),
(#62078,#62079),(#62080,#62081),(#62082,#62083),(#62084,#62085),(#62086,
#62087),(#62088,#62089),(#62090,#62091),(#62092,#62093),(#62094,#62095),
(#62096,#62097),(#62098,#62099),(#62100,#62101),(#62102,#62103),(#62104,
#62105),(#62106,#62107),(#62108,#62109),(#62110,#62111),(#62112,#62113),
(#62114,#62115),(#62116,#62117),(#62118,#62119),(#62120,#62121),(#62122,
#62123),(#62124,#62125),(#62126,#62127),(#62128,#62129),(#62130,#62131),
(#62132,#62133),(#62134,#62135),(#62136,#62137),(#62138,#62139),(#62140,
#62141),(#62142,#62143),(#62144,#62145),(#62146,#62147),(#62148,#62149),
(#62150,#62151),(#62152,#62153),(#62154,#62155),(#62156,#62157),(#62158,
#62159),(#62160,#62161),(#62162,#62163),(#62164,#62165),(#62166,#62167),
(#62168,#62169),(#62170,#62171),(#62172,#62173),(#62174,#62175),(#62176,
#62177),(#62178,#62179),(#62180,#62181),(#62182,#62183),(#62184,#62185),
(#62186,#62187),(#62188,#62189),(#62190,#62191),(#62192,#62193),(#62194,
#62195),(#62196,#62197),(#62198,#62199),(#62200,#62201),(#62202,#62203),
(#62204,#62205),(#62206,#62207),(#62208,#62209),(#62210,#62211),(#62212,
#62213),(#62214,#62215),(#62216,#62217),(#62218,#62219),(#62220,#62221),
(#62222,#62223),(#62224,#62225),(#62226,#62227),(#62228,#62229),(#62230,
#62231),(#62232,#62233),(#62234,#62235),(#62236,#62237),(#62238,#62239),
(#62240,#62241),(#62242,#62243),(#62244,#62245),(#62246,#62247),(#62248,
#62249),(#62250,#62251),(#62252,#62253),(#62254,#62255),(#62256,#62257),
(#62258,#62259),(#62260,#62261),(#62262,#62263),(#62264,#62265),(#62266,
#62267),(#62268,#62269),(#62270,#62271),(#62272,#62273),(#62274,#62275),
(#62276,#62277),(#62278,#62279),(#62280,#62281),(#62282,#62283),(#62284,
#62285),(#62286,#62287),(#62288,#62289),(#62290,#62291),(#62292,#62293),
(#62294,#62295),(#62296,#62297),(#62298,#62299),(#62300,#62301),(#62302,
#62303),(#62304,#62305),(#62306,#62307),(#62308,#62309),(#62310,#62311),
(#62312,#62313),(#62314,#62315),(#62316,#62317),(#62318,#62319),(#62320,
#62321),(#62322,#62323),(#62324,#62325),(#62326,#62327),(#62328,#62329),
(#62330,#62331),(#62332,#62333),(#62334,#62335),(#62336,#62337),(#62338,
#62339),(#62340,#62341),(#62342,#62343),(#62344,#62345),(#62346,#62347),
(#62348,#62349),(#62350,#62351),(#62352,#62353),(#62354,#62355),(#62356,
#62357),(#62358,#62359),(#62360,#62361),(#62362,#62363),(#62364,#62365),
(#62366,#62367),(#62368,#62369),(#62370,#62371),(#62372,#62373),(#62374,
#62375),(#62376,#62377),(#62378,#62379),(#62380,#62381),(#62382,#62383),
(#62384,#62385),(#62386,#62387),(#62388,#62389),(#62390,#62391),(#62392,
#62393),(#62394,#62395),(#62396,#62397),(#62398,#62399),(#62400,#62401),
(#62402,#62403),(#62404,#62405),(#62406,#62407),(#62408,#62409),(#62410,
#62411),(#62412,#62413),(#62414,#62415),(#62416,#62417),(#62418,#62419),
(#62420,#62421),(#62422,#62423),(#62424,#62425),(#62426,#62427),(#62428,
#62429),(#62430,#62431),(#62432,#62433),(#62434,#62435),(#62436,#62437),
(#62438,#62439),(#62440,#62441),(#62442,#62443),(#62444,#62445),(#62446,
#62447),(#62448,#62449),(#62450,#62451),(#62452,#62453),(#62454,#62455),
(#62456,#62457),(#62458,#62459),(#62460,#62461),(#62462,#62463),(#62464,
#62465),(#62466,#62467),(#62468,#62469),(#62470,#62471),(#62472,#62473),
(#62474,#62475),(#62476,#62477),(#62478,#62479),(#62480,#62481),(#62482,
#62483),(#62484,#62485),(#62486,#62487),(#62488,#62489),(#62490,#62491),
(#62492,#62493),(#62494,#62495),(#62496,#62497),(#62498,#62499),(#62500,
#62501),(#62502,#62503),(#62504,#62505),(#62506,#62507),(#62508,#62509),
(#62510,#62511),(#62512,#62513),(#62514,#62515),(#62516,#62517),(#62518,
#62519),(#62520,#62521),(#62522,#62523),(#62524,#62525),(#62526,#62527),
(#62528,#62529),(#62530,#62531),(#62532,#62533),(#62534,#62535),(#62536,
#62537),(#62538,#62539),(#62540,#62541),(#62542,#62543),(#62544,#62545),
(#62546,#62547),(#62548,#62549),(#62550,#62551),(#62552,#62553),(#62554,
#62555),(#62556,#62557),(#62558,#62559),(#62560,#62561),(#62562,#62563),
(#62564,#62565),(#62566,#62567),(#62568,#62569),(#62570,#62571),(#62572,
#62573),(#62574,#62575),(#62576,#62577),(#62578,#62579),(#62580,#62581),
(#62582,#62583),(#62584,#62585),(#62586,#62587),(#62588,#62589),(#62590,
#62591),(#62592,#62593),(#62594,#62595),(#62596,#62597),(#62598,#62599),
(#62600,#62601),(#62602,#62603),(#62604,#62605),(#62606,#62607),(#62608,
#62609),(#62610,#62611),(#62612,#62613),(#62614,#62615),(#62616,#62617),
(#62618,#62619),(#62620,#62621),(#62622,#62623),(#62624,#62625),(#62626,
#62627),(#62628,#62629),(#62630,#62631),(#62632,#62633),(#62634,#62635),
(#62636,#62637),(#62638,#62639),(#62640,#62641),(#62642,#62643),(#62644,
#62645),(#62646,#62647),(#62648,#62649),(#62650,#62651),(#62652,#62653),
(#62654,#62655),(#62656,#62657),(#62658,#62659),(#62660,#62661),(#62662,
#62663),(#62664,#62665),(#62666,#62667),(#62668,#62669),(#62670,#62671),
(#62672,#62673),(#62674,#62675),(#62676,#62677),(#62678,#62679),(#62680,
#62681),(#62682,#62683),(#62684,#62685),(#62686,#62687),(#62688,#62689),
(#62690,#62691),(#62692,#62693),(#62694,#62695),(#62696,#62697),(#62698,
#62699),(#62700,#62701),(#62702,#62703),(#62704,#62705),(#62706,#62707),
(#62708,#62709),(#62710,#62711),(#62712,#62713),(#62714,#62715),(#62716,
#62717),(#62718,#62719),(#62720,#62721),(#62722,#62723),(#62724,#62725),
(#62726,#62727),(#62728,#62729),(#62730,#62731),(#62732,#62733),(#62734,
#62735),(#62736,#62737),(#62738,#62739),(#62740,#62741),(#62742,#62743),
(#62744,#62745),(#62746,#62747),(#62748,#62749),(#62750,#62751),(#62752,
#62753),(#62754,#62755),(#62756,#62757),(#62758,#62759),(#62760,#62761),
(#62762,#62763),(#62764,#62765),(#62766,#62767),(#62768,#62769),(#62770,
#62771),(#62772,#62773),(#62774,#62775),(#62776,#62777),(#62778,#62779),
(#62780,#62781),(#62782,#62783),(#62784,#62785),(#62786,#62787),(#62788,
#62789),(#62790,#62791),(#62792,#62793),(#62794,#62795),(#62796,#62797),
(#62798,#62799),(#62800,#62801),(#62802,#62803),(#62804,#62805),(#62806,
#62807),(#62808,#62809),(#62810,#62811),(#62812,#62813),(#62814,#62815),
(#62816,#62817),(#62818,#62819),(#62820,#62821),(#62822,#62823),(#62824,
#62825),(#62826,#62827),(#62828,#62829),(#62830,#62831),(#62832,#62833),
(#62834,#62835),(#62836,#62837),(#62838,#62839),(#62840,#62841),(#62842,
#62843),(#62844,#62845),(#62846,#62847),(#62848,#62849),(#62850,#62851),
(#62852,#62853),(#62854,#62855),(#62856,#62857),(#62858,#62859),(#62860,
#62861),(#62862,#62863),(#62864,#62865),(#62866,#62867),(#62868,#62869),
(#62870,#62871),(#62872,#62873),(#62874,#62875),(#62876,#62877),(#62878,
#62879),(#62880,#62881),(#62882,#62883),(#62884,#62885),(#62886,#62887),
(#62888,#62889),(#62890,#62891),(#62892,#62893),(#62894,#62895),(#62896,
#62897),(#62898,#62899),(#62900,#62901),(#62902,#62903),(#62904,#62905),
(#62906,#62907),(#62908,#62909),(#62910,#62911),(#62912,#62913),(#62914,
#62915),(#62916,#62917),(#62918,#62919),(#62920,#62921),(#62922,#62923),
(#62924,#62925),(#62926,#62927),(#62928,#62929),(#62930,#62931),(#62932,
#62933),(#62934,#62935),(#62936,#62937),(#62938,#62939),(#62940,#62941),
(#62942,#62943),(#62944,#62945),(#62946,#62947),(#62948,#62949),(#62950,
#62951),(#62952,#62953),(#62954,#62955),(#62956,#62957),(#62958,#62959),
(#62960,#62961),(#62962,#62963),(#62964,#62965),(#62966,#62967),(#62968,
#62969),(#62970,#62971),(#62972,#62973),(#62974,#62975),(#62976,#62977),
(#62978,#62979),(#62980,#62981),(#62982,#62983),(#62984,#62985),(#62986,
#62987),(#62988,#62989),(#62990,#62991),(#62992,#62993),(#62994,#62995),
(#62996,#62997),(#62998,#62999),(#63000,#63001),(#63002,#63003),(#63004,
#63005),(#63006,#63007),(#63008,#63009),(#63010,#63011),(#63012,#63013),
(#63014,#63015),(#63016,#63017),(#63018,#63019),(#63020,#63021),(#63022,
#63023),(#63024,#63025),(#63026,#63027),(#63028,#63029),(#63030,#63031),
(#63032,#63033),(#63034,#63035),(#63036,#63037),(#63038,#63039),(#63040,
#63041),(#63042,#63043),(#63044,#63045),(#63046,#63047),(#63048,#63049),
(#63050,#63051),(#63052,#63053),(#63054,#63055),(#63056,#63057),(#63058,
#63059),(#63060,#63061),(#63062,#63063),(#63064,#63065),(#63066,#63067),
(#63068,#63069),(#63070,#63071),(#63072,#63073),(#63074,#63075),(#63076,
#63077),(#63078,#63079),(#63080,#63081),(#63082,#63083),(#63084,#63085),
(#63086,#63087),(#63088,#63089),(#63090,#63091),(#63092,#63093),(#63094,
#63095),(#63096,#63097),(#63098,#63099),(#63100,#63101),(#63102,#63103),
(#63104,#63105),(#63106,#63107),(#63108,#63109),(#63110,#63111),(#63112,
#63113),(#63114,#63115),(#63116,#63117),(#63118,#63119),(#63120,#63121),
(#63122,#63123),(#63124,#63125),(#63126,#63127),(#63128,#63129),(#63130,
#63131),(#63132,#63133),(#63134,#63135),(#63136,#63137),(#63138,#63139),
(#63140,#63141),(#63142,#63143),(#63144,#63145),(#63146,#63147),(#63148,
#63149),(#63150,#63151),(#63152,#63153),(#63154,#63155),(#63156,#63157),
(#63158,#63159),(#63160,#63161),(#63162,#63163),(#63164,#63165),(#63166,
#63167),(#63168,#63169),(#63170,#63171),(#63172,#63173),(#63174,#63175),
(#63176,#63177),(#63178,#63179),(#63180,#63181),(#63182,#63183),(#63184,
#63185),(#63186,#63187),(#63188,#63189),(#63190,#63191),(#63192,#63193),
(#63194,#63195),(#63196,#63197),(#63198,#63199),(#63200,#63201),(#63202,
#63203),(#63204,#63205),(#63206,#63207),(#63208,#63209),(#63210,#63211),
(#63212,#63213),(#63214,#63215),(#63216,#63217),(#63218,#63219),(#63220,
#63221),(#63222,#63223),(#63224,#63225),(#63226,#63227),(#63228,#63229),
(#63230,#63231),(#63232,#63233),(#63234,#63235),(#63236,#63237),(#63238,
#63239),(#63240,#63241),(#63242,#63243),(#63244,#63245),(#63246,#63247),
(#63248,#63249),(#63250,#63251),(#63252,#63253),(#63254,#63255),(#63256,
#63257),(#63258,#63259),(#63260,#63261),(#63262,#63263),(#63264,#63265),
(#63266,#63267),(#63268,#63269),(#63270,#63271),(#63272,#63273),(#63274,
#63275),(#63276,#63277),(#63278,#63279),(#63280,#63281),(#63282,#63283),
(#63284,#63285),(#63286,#63287),(#63288,#63289),(#63290,#63291),(#63292,
#63293),(#63294,#63295),(#63296,#63297),(#63298,#63299),(#63300,#63301),
(#63302,#63303),(#63304,#63305),(#63306,#63307),(#63308,#63309),(#63310,
#63311),(#63312,#63313),(#63314,#63315),(#63316,#63317),(#63318,#63319),
(#63320,#63321),(#63322,#63323),(#63324,#63325),(#63326,#63327),(#63328,
#63329),(#63330,#63331),(#63332,#63333),(#63334,#63335),(#63336,#63337),
(#63338,#63339),(#63340,#63341),(#63342,#63343),(#63344,#63345),(#63346,
#63347),(#63348,#63349),(#63350,#63351),(#63352,#63353),(#63354,#63355),
(#63356,#63357),(#63358,#63359),(#63360,#63361),(#63362,#63363),(#63364,
#63365),(#63366,#63367),(#63368,#63369),(#63370,#63371),(#63372,#63373),
(#63374,#63375),(#63376,#63377),(#63378,#63379),(#63380,#63381),(#63382,
#63383),(#63384,#63385),(#63386,#63387),(#63388,#63389),(#63390,#63391),
(#63392,#63393),(#63394,#63395),(#63396,#63397),(#63398,#63399),(#63400,
#63401),(#63402,#63403),(#63404,#63405),(#63406,#63407),(#63408,#63409),
(#63410,#63411),(#63412,#63413),(#63414,#63415),(#63416,#63417),(#63418,
#63419),(#63420,#63421),(#63422,#63423),(#63424,#63425),(#63426,#63427),
(#63428,#63429),(#63430,#63431),(#63432,#63433),(#63434,#63435),(#63436,
#63437),(#63438,#63439),(#63440,#63441),(#63442,#63443),(#63444,#63445),
(#63446,#63447),(#63448,#63449),(#63450,#63451),(#63452,#63453),(#63454,
#63455),(#63456,#63457),(#63458,#63459),(#63460,#63461),(#63462,#63463),
(#63464,#63465),(#63466,#63467),(#63468,#63469),(#63470,#63471),(#63472,
#63473),(#63474,#63475),(#63476,#63477),(#63478,#63479),(#63480,#63481),
(#63482,#63483),(#63484,#63485),(#63486,#63487),(#63488,#63489),(#63490,
#63491),(#63492,#63493),(#63494,#63495),(#63496,#63497),(#63498,#63499),
(#63500,#63501),(#63502,#63503),(#63504,#63505),(#63506,#63507),(#63508,
#63509),(#63510,#63511),(#63512,#63513),(#63514,#63515),(#63516,#63517),
(#63518,#63519),(#63520,#63521),(#63522,#63523),(#63524,#63525),(#63526,
#63527),(#63528,#63529),(#63530,#63531),(#63532,#63533),(#63534,#63535),
(#63536,#63537),(#63538,#63539),(#63540,#63541),(#63542,#63543),(#63544,
#63545),(#63546,#63547),(#63548,#63549),(#63550,#63551),(#63552,#63553),
(#63554,#63555),(#63556,#63557),(#63558,#63559),(#63560,#63561),(#63562,
#63563),(#63564,#63565),(#63566,#63567),(#63568,#63569),(#63570,#63571),
(#63572,#63573),(#63574,#63575),(#63576,#63577),(#63578,#63579),(#63580,
#63581),(#63582,#63583),(#63584,#63585),(#63586,#63587),(#63588,#63589),
(#63590,#63591),(#63592,#63593),(#63594,#63595),(#63596,#63597),(#63598,
#63599),(#63600,#63601),(#63602,#63603),(#63604,#63605),(#63606,#63607),
(#63608,#63609),(#63610,#63611),(#63612,#63613),(#63614,#63615),(#63616,
#63617),(#63618,#63619),(#63620,#63621),(#63622,#63623),(#63624,#63625),
(#63626,#63627),(#63628,#63629),(#63630,#63631),(#63632,#63633),(#63634,
#63635),(#63636,#63637),(#63638,#63639),(#63640,#63641),(#63642,#63643),
(#63644,#63645),(#63646,#63647),(#63648,#63649),(#63650,#63651),(#63652,
#63653),(#63654,#63655),(#63656,#63657),(#63658,#63659),(#63660,#63661),
(#63662,#63663),(#63664,#63665),(#63666,#63667),(#63668,#63669),(#63670,
#63671),(#63672,#63673),(#63674,#63675),(#63676,#63677),(#63678,#63679),
(#63680,#63681),(#63682,#63683),(#63684,#63685),(#63686,#63687),(#63688,
#63689),(#63690,#63691),(#63692,#63693),(#63694,#63695),(#63696,#63697),
(#63698,#63699),(#63700,#63701),(#63702,#63703),(#63704,#63705),(#63706,
#63707),(#63708,#63709),(#63710,#63711),(#63712,#63713),(#63714,#63715),
(#63716,#63717),(#63718,#63719),(#63720,#63721),(#63722,#63723),(#63724,
#63725),(#63726,#63727),(#63728,#63729),(#63730,#63731),(#63732,#63733),
(#63734,#63735),(#63736,#63737),(#63738,#63739),(#63740,#63741),(#63742,
#63743),(#63744,#63745),(#63746,#63747),(#63748,#63749),(#63750,#63751),
(#63752,#63753),(#63754,#63755),(#63756,#63757),(#63758,#63759),(#63760,
#63761),(#63762,#63763),(#63764,#63765),(#63766,#63767),(#63768,#63769),
(#63770,#63771),(#63772,#63773),(#63774,#63775),(#63776,#63777),(#63778,
#63779),(#63780,#63781),(#63782,#63783),(#63784,#63785),(#63786,#63787),
(#63788,#63789),(#63790,#63791),(#63792,#63793),(#63794,#63795),(#63796,
#63797),(#63798,#63799),(#63800,#63801),(#63802,#63803),(#63804,#63805),
(#63806,#63807),(#63808,#63809),(#63810,#63811),(#63812,#63813),(#63814,
#63815),(#63816,#63817),(#63818,#63819),(#63820,#63821),(#63822,#63823),
(#63824,#63825),(#63826,#63827),(#63828,#63829),(#63830,#63831),(#63832,
#63833),(#63834,#63835),(#63836,#63837),(#63838,#63839),(#63840,#63841),
(#63842,#63843),(#63844,#63845),(#63846,#63847),(#63848,#63849),(#63850,
#63851),(#63852,#63853),(#63854,#63855),(#63856,#63857),(#63858,#63859),
(#63860,#63861),(#63862,#63863),(#63864,#63865),(#63866,#63867),(#63868,
#63869),(#63870,#63871),(#63872,#63873),(#63874,#63875),(#63876,#63877),
(#63878,#63879),(#63880,#63881),(#63882,#63883),(#63884,#63885),(#63886,
#63887),(#63888,#63889),(#63890,#63891),(#63892,#63893),(#63894,#63895),
(#63896,#63897),(#63898,#63899),(#63900,#63901),(#63902,#63903),(#63904,
#63905),(#63906,#63907),(#63908,#63909),(#63910,#63911),(#63912,#63913),
(#63914,#63915),(#63916,#63917),(#63918,#63919),(#63920,#63921),(#63922,
#63923),(#63924,#63925),(#63926,#63927),(#63928,#63929),(#63930,#63931),
(#63932,#63933),(#63934,#63935),(#63936,#63937),(#63938,#63939),(#63940,
#63941),(#63942,#63943),(#63944,#63945),(#63946,#63947),(#63948,#63949),
(#63950,#63951),(#63952,#63953),(#63954,#63955),(#63956,#63957),(#63958,
#63959),(#63960,#63961),(#63962,#63963),(#63964,#63965),(#63966,#63967),
(#63968,#63969),(#63970,#63971),(#63972,#63973),(#63974,#63975),(#63976,
#63977),(#63978,#63979),(#63980,#63981),(#63982,#63983),(#63984,#63985),
(#63986,#63987),(#63988,#63989),(#63990,#63991),(#63992,#63993),(#63994,
#63995),(#63996,#63997),(#63998,#63999),(#64000,#64001),(#64002,#64003),
(#64004,#64005),(#64006,#64007),(#64008,#64009),(#64010,#64011),(#64012,
#64013),(#64014,#64015),(#64016,#64017),(#64018,#64019),(#64020,#64021),
(#64022,#64023),(#64024,#64025),(#64026,#64027),(#64028,#64029),(#64030,
#64031),(#64032,#64033),(#64034,#64035),(#64036,#64037),(#64038,#64039),
(#64040,#64041),(#64042,#64043),(#64044,#64045),(#64046,#64047),(#64048,
#64049),(#64050,#64051),(#64052,#64053),(#64054,#64055),(#64056,#64057),
(#64058,#64059),(#64060,#64061),(#64062,#64063),(#64064,#64065),(#64066,
#64067),(#64068,#64069),(#64070,#64071),(#64072,#64073),(#64074,#64075),
(#64076,#64077),(#64078,#64079),(#64080,#64081),(#64082,#64083),(#64084,
#64085),(#64086,#64087),(#64088,#64089),(#64090,#64091),(#64092,#64093),
(#64094,#64095),(#64096,#64097),(#64098,#64099),(#64100,#64101),(#64102,
#64103),(#64104,#64105),(#64106,#64107),(#64108,#64109),(#64110,#64111),
(#64112,#64113),(#64114,#64115),(#64116,#64117),(#64118,#64119),(#64120,
#64121),(#64122,#64123),(#64124,#64125),(#64126,#64127),(#64128,#64129),
(#64130,#64131),(#64132,#64133),(#64134,#64135),(#64136,#64137),(#64138,
#64139),(#64140,#64141),(#64142,#64143),(#64144,#64145),(#64146,#64147),
(#64148,#64149),(#64150,#64151),(#64152,#64153),(#64154,#64155),(#64156,
#64157),(#64158,#64159),(#64160,#64161),(#64162,#64163),(#64164,#64165),
(#64166,#64167),(#64168,#64169),(#64170,#64171),(#64172,#64173),(#64174,
#64175),(#64176,#64177),(#64178,#64179),(#64180,#64181),(#64182,#64183),
(#64184,#64185),(#64186,#64187),(#64188,#64189),(#64190,#64191),(#64192,
#64193),(#64194,#64195),(#64196,#64197),(#64198,#64199),(#64200,#64201),
(#64202,#64203),(#64204,#64205),(#64206,#64207),(#64208,#64209),(#64210,
#64211),(#64212,#64213),(#64214,#64215),(#64216,#64217),(#64218,#64219),
(#64220,#64221),(#64222,#64223),(#64224,#64225),(#64226,#64227),(#64228,
#64229),(#64230,#64231),(#64232,#64233),(#64234,#64235),(#64236,#64237),
(#64238,#64239),(#64240,#64241),(#64242,#64243),(#64244,#64245),(#64246,
#64247),(#64248,#64249),(#64250,#64251),(#64252,#64253),(#64254,#64255),
(#64256,#64257),(#64258,#64259),(#64260,#64261),(#64262,#64263),(#64264,
#64265),(#64266,#64267),(#64268,#64269),(#64270,#64271),(#64272,#64273),
(#64274,#64275),(#64276,#64277),(#64278,#64279),(#64280,#64281),(#64282,
#64283),(#64284,#64285),(#64286,#64287),(#64288,#64289),(#64290,#64291),
(#64292,#64293),(#64294,#64295),(#64296,#64297),(#64298,#64299),(#64300,
#64301),(#64302,#64303),(#64304,#64305),(#64306,#64307),(#64308,#64309),
(#64310,#64311),(#64312,#64313),(#64314,#64315),(#64316,#64317),(#64318,
#64319),(#64320,#64321),(#64322,#64323),(#64324,#64325),(#64326,#64327),
(#64328,#64329),(#64330,#64331),(#64332,#64333),(#64334,#64335),(#64336,
#64337),(#64338,#64339),(#64340,#64341),(#64342,#64343),(#64344,#64345),
(#64346,#64347),(#64348,#64349),(#64350,#64351),(#64352,#64353),(#64354,
#64355),(#64356,#64357),(#64358,#64359),(#64360,#64361),(#64362,#64363),
(#64364,#64365),(#64366,#64367),(#64368,#64369),(#64370,#64371),(#64372,
#64373),(#64374,#64375),(#64376,#64377),(#64378,#64379),(#64380,#64381),
(#64382,#64383),(#64384,#64385),(#64386,#64387),(#64388,#64389),(#64390,
#64391),(#64392,#64393),(#64394,#64395),(#64396,#64397),(#64398,#64399),
(#64400,#64401),(#64402,#64403),(#64404,#64405),(#64406,#64407),(#64408,
#64409),(#64410,#64411),(#64412,#64413),(#64414,#64415),(#64416,#64417),
(#64418,#64419),(#64420,#64421),(#64422,#64423),(#64424,#64425),(#64426,
#64427),(#64428,#64429),(#64430,#64431),(#64432,#64433),(#64434,#64435),
(#64436,#64437),(#64438,#64439),(#64440,#64441),(#64442,#64443),(#64444,
#64445),(#64446,#64447),(#64448,#64449),(#64450,#64451),(#64452,#64453),
(#64454,#64455),(#64456,#64457),(#64458,#64459),(#64460,#64461),(#64462,
#64463),(#64464,#64465),(#64466,#64467),(#64468,#64469),(#64470,#64471)),
 .UNSPECIFIED.,.F.,.F.,.F.,(4,1,1,1,1,1,1,1,1,1,1,1,1,1,1,1,1,1,1,1,1,1,
1,1,1,1,1,1,1,1,1,1,1,1,1,1,1,1,1,1,1,1,1,1,1,1,1,1,1,1,1,1,1,1,1,1,1,1,
1,1,1,1,1,1,1,1,1,1,1,1,1,1,1,1,1,1,1,1,1,1,1,1,1,1,1,1,1,1,1,1,1,1,1,1,
1,1,1,1,1,1,1,1,1,1,1,1,1,1,1,1,1,1,1,1,1,1,1,1,1,1,1,1,1,1,1,1,1,1,1,1,
1,1,1,1,1,1,1,1,1,1,1,1,1,1,1,1,1,1,1,1,1,1,1,1,1,1,1,1,1,1,1,1,1,1,1,1,
1,1,1,1,1,1,1,1,1,1,1,1,1,1,1,1,1,1,1,1,1,1,1,1,1,1,1,1,1,1,1,1,1,1,1,1,
1,1,1,1,1,1,1,1,1,1,1,1,1,1,1,1,1,1,1,1,1,1,1,1,1,1,1,1,1,1,1,1,1,1,1,1,
1,1,1,1,1,1,1,1,1,1,1,1,1,1,1,1,1,1,1,1,1,1,1,1,1,1,1,1,1,1,1,1,1,1,1,1,
1,1,1,1,1,1,1,1,1,1,1,1,1,1,1,1,1,1,1,1,1,1,1,1,1,1,1,1,1,1,1,1,1,1,1,1,
1,1,1,1,1,1,1,1,1,1,1,1,1,1,1,1,1,1,1,1,1,1,1,1,1,1,1,1,1,1,1,1,1,1,1,1,
1,1,1,1,1,1,1,1,1,1,1,1,1,1,1,1,1,1,1,1,1,1,1,1,1,1,1,1,1,1,1,1,1,1,1,1,
1,1,1,1,1,1,1,1,1,1,1,1,1,1,1,1,1,1,1,1,1,1,1,1,1,1,1,1,1,1,1,1,1,1,1,1,
1,1,1,1,1,1,1,1,1,1,1,1,1,1,1,1,1,1,1,1,1,1,1,1,1,1,1,1,1,1,1,1,1,1,1,1,
1,1,1,1,1,1,1,1,1,1,1,1,1,1,1,1,1,1,1,1,1,1,1,1,1,1,1,1,1,1,1,1,1,1,1,1,
1,1,1,1,1,1,1,1,1,1,1,1,1,1,1,1,1,1,1,1,1,1,1,1,1,1,1,1,1,1,1,1,1,1,1,1,
1,1,1,1,1,1,1,1,1,1,1,1,1,1,1,1,1,1,1,1,1,1,1,1,1,1,1,1,1,1,1,1,1,1,1,1,
1,1,1,1,1,1,1,1,1,1,1,1,1,1,1,1,1,1,1,1,1,1,1,1,1,1,1,1,1,1,1,1,1,1,1,1,
1,1,1,1,1,1,1,1,1,1,1,1,1,1,1,1,1,1,1,1,1,1,1,1,1,1,1,1,1,1,1,1,1,1,1,1,
1,1,1,1,1,1,1,1,1,1,1,1,1,1,1,1,1,1,1,1,1,1,1,1,1,1,1,1,1,1,1,1,1,1,1,1,
1,1,1,1,1,1,1,1,1,1,1,1,1,1,1,1,1,1,1,1,1,1,1,1,1,1,1,1,1,1,1,1,1,1,1,1,
1,1,1,1,1,1,1,1,1,1,1,1,1,1,1,1,1,1,1,1,1,1,1,1,1,1,1,1,1,1,1,1,1,1,1,1,
1,1,1,1,1,1,1,1,1,1,1,1,1,1,1,1,1,1,1,1,1,1,1,1,1,1,1,1,1,1,1,1,1,1,1,1,
1,1,1,1,1,1,1,1,1,1,1,1,1,1,1,1,1,1,1,1,1,1,1,1,1,1,1,1,1,1,1,1,1,1,1,1,
1,1,1,1,1,1,1,1,1,1,1,1,1,1,1,1,1,1,1,1,1,1,1,1,1,1,1,1,1,1,1,1,1,1,1,1,
1,1,1,1,1,1,1,1,1,1,1,1,1,1,1,1,1,1,1,1,1,1,1,1,1,1,1,1,1,1,1,1,1,1,1,1,
1,1,1,1,1,1,1,1,1,1,1,1,1,1,1,1,1,1,1,1,1,1,1,1,1,1,1,1,1,1,1,1,1,1,1,1,
1,1,1,1,1,1,1,1,1,1,1,1,1,1,1,1,1,1,1,1,1,1,1,1,1,1,1,1,1,1,1,1,1,1,1,1,
1,1,1,1,1,1,1,1,1,1,1,1,1,1,1,1,1,1,1,1,1,1,1,1,1,1,1,1,1,1,1,1,1,1,1,1,
1,1,1,1,1,1,1,1,1,1,1,1,1,1,1,1,1,1,1,1,1,1,1,1,1,1,1,1,1,1,1,1,1,1,1,1,
1,1,1,1,1,1,1,1,1,1,1,1,1,1,1,1,1,1,1,1,1,1,1,1,1,1,1,1,1,1,1,1,1,1,1,1,
1,1,1,1,1,1,1,1,1,1,1,1,1,1,1,1,1,1,1,1,1,1,1,1,1,1,1,1,1,1,1,1,1,1,1,1,
1,1,1,1,1,1,1,1,1,1,1,1,1,1,1,1,1,1,1,1,1,1,1,1,1,1,1,1,1,1,1,1,1,1,1,1,
1,1,1,1,1,1,1,1,1,1,1,1,1,1,1,1,1,1,1,1,1,1,1,1,1,1,1,1,1,1,1,1,1,1,1,1,
1,1,1,1,1,1,1,1,1,1,1,1,1,1,1,1,1,1,1,1,1,1,1,1,1,1,1,1,1,1,1,1,1,1,1,1,
1,1,1,1,1,1,1,1,1,1,1,1,1,1,1,1,1,1,1,1,1,1,1,1,1,1,1,1,1,1,1,1,1,1,1,1,
1,1,1,1,1,1,1,1,1,1,1,1,1,1,1,1,1,1,1,1,1,1,1,1,1,1,1,1,1,1,1,1,1,1,1,1,
1,1,1,1,1,1,1,1,1,1,1,1,1,1,1,1,1,1,1,1,1,1,1,1,1,1,1,1,1,1,1,1,1,1,1,1,
1,1,1,1,1,1,1,1,1,1,1,1,1,1,1,1,1,1,1,1,1,1,1,1,1,1,1,1,1,1,1,1,1,1,1,1,
1,1,1,1,1,1,1,1,1,1,1,1,1,1,1,1,1,1,1,1,1,1,1,1,1,1,1,1,1,1,1,1,1,1,1,1,
1,1,1,1,1,1,1,1,1,1,1,1,1,1,1,1,1,1,1,1,1,1,1,1,1,1,1,1,1,1,1,1,1,1,1,1,
1,1,1,1,1,1,1,1,1,1,1,1,1,1,1,1,1,1,1,1,1,1,1,1,1,1,1,1,1,1,1,1,1,1,1,1,
1,1,1,1,1,1,1,1,1,1,1,1,1,1,1,1,1,1,1,1,1,1,1,1,1,1,1,1,1,1,1,1,1,1,1,1,
1,1,1,1,1,1,1,1,1,1,1,1,1,1,1,1,1,1,1,1,1,1,1,1,1,1,1,1,1,1,1,1,1,1,1,1,
1,1,1,1,1,1,1,1,1,1,1,1,1,1,1,1,1,1,1,1,1,1,1,1,1,1,1,1,1,1,1,1,1,1,1,1,
1,1,1,1,1,1,1,1,1,1,1,1,1,1,1,1,1,1,1,1,1,1,1,1,1,1,1,1,1,1,1,1,1,1,1,1,
1,1,1,1,1,1,1,1,1,1,1,1,1,1,1,1,1,1,1,1,1,1,1,1,1,1,1,1,1,1,1,1,1,1,1,1,
1,1,1,1,1,1,1,1,1,1,1,1,1,1,1,1,1,1,1,1,1,1,1,1,1,1,1,1,1,1,1,1,1,1,1,1,
1,1,1,1,1,1,1,1,1,1,1,1,1,1,1,1,1,1,1,1,1,1,1,1,1,1,1,1,1,1,1,1,1,1,1,1,
1,1,1,1,1,1,1,1,1,1,1,1,1,1,1,1,1,1,1,1,1,1,1,1,1,1,1,1,1,1,1,1,1,1,1,1,
1,1,1,1,1,1,1,1,1,1,1,1,1,1,1,1,1,1,1,1,1,1,1,1,1,1,1,1,1,1,1,1,1,1,1,1,
1,1,1,1,1,1,1,1,1,1,1,1,1,1,1,1,1,1,1,1,1,1,1,1,1,1,1,1,1,1,1,1,1,1,1,1,
1,1,1,1,1,1,1,1,1,1,1,1,1,1,1,1,1,1,1,1,1,1,1,1,1,1,1,1,1,1,1,1,1,1,1,1,
1,1,1,1,1,1,1,1,1,1,1,1,1,1,1,1,1,1,1,1,1,1,1,1,1,1,1,1,1,1,1,1,1,1,1,1,
1,1,1,1,1,1,1,1,1,1,1,1,1,1,1,1,1,1,1,1,1,1,1,1,1,1,1,1,1,1,1,1,1,1,1,1,
1,1,1,1,1,1,1,1,1,1,1,1,1,1,1,1,1,1,1,1,1,1,1,1,1,1,1,1,1,1,1,1,1,1,1,1,
1,1,1,1,1,1,1,1,1,1,1,1,1,1,1,1,1,1,1,1,1,1,1,1,1,1,1,1,1,1,1,1,1,1,1,1,
1,1,1,1,1,1,1,1,1,1,1,1,1,1,1,1,1,1,1,1,1,1,1,1,1,1,1,1,1,1,1,1,1,1,1,1,
1,1,1,1,1,1,1,1,1,1,1,1,1,1,1,1,1,1,1,1,1,1,1,1,1,1,1,1,1,1,1,1,1,1,1,1,
1,1,1,1,1,1,1,1,1,1,1,1,1,1,1,1,1,1,1,1,1,1,1,1,1,1,1,1,1,1,1,1,1,1,1,1,
1,1,1,1,1,1,1,1,1,1,1,1,1,1,1,1,1,1,1,1,1,1,1,1,1,1,1,1,1,1,1,1,1,1,1,1,
1,1,1,1,1,1,1,1,1,1,1,1,1,1,1,1,1,1,1,1,1,1,1,1,1,1,1,1,1,1,1,1,1,1,1,1,
1,1,1,1,1,1,1,1,1,1,1,1,1,1,1,1,1,1,1,1,1,1,1,1,1,1,1,1,1,1,1,1,1,1,1,1,
1,1,1,1,1,1,1,1,1,1,1,1,1,1,1,1,1,1,1,1,1,1,1,1,1,1,1,1,1,1,1,1,1,1,1,1,
1,1,1,1,1,1,1,1,1,1,1,1,1,1,1,1,1,1,1,1,1,1,1,1,1,1,1,1,1,1,1,1,1,1,1,1,
1,1,1,1,1,1,1,1,1,1,1,1,1,1,1,1,1,1,1,1,1,1,1,1,1,1,1,1,1,1,1,1,1,1,1,1,
1,1,1,1,1,1,1,1,1,1,1,1,1,1,1,1,1,1,1,1,1,1,1,1,1,1,1,1,1,1,1,1,1,1,1,1,
1,1,1,1,1,1,1,1,1,1,1,1,1,1,1,1,1,1,1,1,1,1,1,1,1,1,1,1,1,1,1,1,1,1,1,1,
1,1,1,1,1,1,1,1,1,1,1,1,1,1,1,1,1,1,1,1,1,1,1,1,1,1,1,1,1,1,1,1,1,1,1,1,
1,1,1,1,1,1,1,1,1,1,1,1,1,1,1,1,1,1,1,1,1,1,1,1,1,1,1,1,1,1,1,1,1,1,1,1,
1,1,1,1,1,1,1,1,1,1,1,1,1,1,1,1,1,1,1,1,1,1,1,1,1,1,1,1,1,1,1,1,1,1,1,1,
1,1,1,1,1,1,1,1,1,1,1,1,1,1,1,1,1,1,1,1,1,1,1,1,1,1,1,1,1,1,1,1,1,1,1,1,
1,1,1,1,1,1,1,1,1,1,1,1,1,1,1,1,1,1,1,1,1,1,1,1,1,1,1,1,1,1,1,1,1,1,1,1,
1,1,1,1,1,1,1,1,1,1,1,1,1,1,1,1,1,1,1,1,1,1,1,1,1,1,1,1,1,1,1,1,1,1,1,1,
1,1,1,1,1,1,1,1,1,1,1,1,1,1,1,1,1,1,1,1,1,1,1,1,1,1,1,1,1,1,1,1,1,1,1,1,
1,1,1,1,1,1,1,1,1,1,1,1,1,1,1,1,1,1,1,1,1,1,1,1,1,1,1,1,1,1,1,1,1,1,1,1,
1,1,1,1,1,1,1,1,1,1,1,1,1,1,1,1,1,1,1,1,1,1,1,1,1,1,1,1,1,1,1,1,1,1,1,1,
1,1,1,1,1,1,1,1,1,1,1,1,1,1,1,1,1,1,1,1,1,1,1,1,1,1,1,1,1,1,1,1,1,1,1,1,
1,1,1,1,1,1,1,1,1,1,1,1,1,1,1,1,1,1,1,1,1,1,1,1,1,1,1,1,1,1,1,1,1,1,1,1,
1,1,1,1,1,1,1,1,1,1,1,1,1,1,1,1,1,1,1,1,1,1,1,1,1,1,1,1,1,1,1,1,1,1,1,1,
1,1,1,1,1,1,1,1,1,1,1,1,1,1,1,1,1,1,1,1,1,1,1,1,1,1,1,1,1,1,1,1,1,1,1,1,
1,1,1,1,1,1,1,1,1,1,1,1,1,1,1,1,1,1,1,1,1,1,1,1,1,1,1,1,1,1,1,1,1,1,1,1,
1,1,1,1,1,1,1,1,1,1,1,1,1,1,1,1,1,1,1,1,1,1,1,1,1,1,1,1,1,1,1,1,1,1,1,1,
1,1,1,1,1,1,1,1,1,1,1,1,1,1,1,1,1,1,1,1,1,1,1,1,1,1,1,1,1,1,1,1,1,1,1,1,
1,1,1,1,1,1,1,1,1,1,1,1,1,1,1,1,1,1,1,1,1,1,1,1,1,1,1,1,1,1,1,1,1,1,1,1,
1,1,1,1,1,1,1,1,1,1,1,1,1,1,1,1,1,1,1,1,1,1,1,1,1,1,1,1,1,1,1,1,1,1,1,1,
1,1,1,1,1,1,1,1,1,1,1,1,1,1,1,1,1,1,1,1,1,1,1,1,1,1,1,1,1,1,1,1,1,1,1,1,
1,1,1,1,1,1,1,1,1,1,1,1,1,1,1,1,1,1,1,1,1,1,1,1,1,1,1,1,1,1,1,1,1,1,1,1,
1,1,1,1,1,1,1,1,1,1,1,1,1,1,1,1,1,1,1,1,1,1,1,1,1,1,1,1,1,1,1,1,1,1,1,1,
1,1,1,1,1,1,1,1,1,1,1,1,1,1,1,1,1,1,1,1,1,1,1,1,1,1,1,1,1,1,1,1,1,1,1,1,
1,1,1,1,1,1,1,1,1,1,1,1,1,1,1,1,1,1,1,1,1,1,1,1,1,1,1,1,1,1,1,1,1,1,1,1,
1,1,1,1,1,1,1,1,1,1,1,1,1,1,1,1,1,1,1,1,1,1,1,1,1,1,1,1,1,1,1,1,1,1,1,1,
1,1,1,1,1,1,1,1,1,1,1,1,1,1,1,1,1,1,1,1,1,1,1,1,1,1,1,1,1,1,1,1,1,1,1,1,
1,1,1,1,1,1,1,1,1,1,1,1,1,1,1,1,1,1,1,1,1,1,1,1,1,1,1,1,1,1,1,1,1,1,1,1,
1,1,1,1,1,1,1,1,1,1,1,1,1,1,1,1,1,1,1,1,1,1,1,1,1,1,1,1,1,1,1,1,1,1,1,1,
1,1,1,1,1,1,1,1,1,1,1,1,1,1,1,1,1,1,1,1,1,1,1,1,1,1,1,1,1,1,1,1,1,1,1,1,
1,1,1,1,1,1,1,1,1,1,1,1,1,1,1,1,1,1,1,1,1,1,1,1,1,1,1,1,1,1,1,1,1,1,1,1,
1,1,1,1,1,1,1,1,1,1,1,1,1,1,1,1,1,1,1,1,1,1,1,1,1,1,1,1,1,1,1,1,1,1,1,1,
1,1,1,1,4),(2,2),(0.,0.869746702321014,1.7394931589914,2.60923976624962,
3.47983908319159,4.35043840179749,5.22018503077054,6.08993165951504,6.95967828799171,
7.82942491616733,8.69917154401062,9.56891817149224,10.4395174886835,11.3101168056706,
12.179863432132,13.049610058144,13.9193566836854,14.7891033087372,15.6588499332817,
16.5285965573034,17.3991958717975,18.2697951860185,18.7046684974166,19.1395418086746,
19.5744151197912,20.0092884307654,20.4441617415962,20.8790350522825,21.7487816732187,
22.1836549834672,22.6185282935685,23.0534016035221,23.4882749133276,23.9231482229848,
24.3588742245859,24.794600226187,25.2294735355468,26.0992201538203,26.5340934627341,
26.9689667714994,27.4038400801166,27.838713388586,28.2735866969081,28.7084600050832,
29.143333313112,29.5782066209952,30.0130799287334,30.4479532363275,30.8828265437783,
31.3185525442794,31.7542785447804,32.1891518519474,32.6240251589741,33.0588984658616,
33.4937717726112,33.928645079224,34.3635183857014,34.7983916920448,35.2332649982556,
35.6681383043353,36.1030116102854,36.5378849161076,36.9727582218035,37.4076315273749,
37.8425048328235,38.2782308323341,38.7139568318446,39.1488301370532,39.5837034421446,
40.0185767471208,40.4534500519838,40.8883233567357,41.3231966613787,41.7580699659148,
42.1929432703463,42.6278165746754,43.0626898789044,43.4975631830356,43.9324364870714,
44.3673097910142,44.8021830948664,45.2379090935952,45.673635092324,46.1085083960024,
46.5433816995978,46.9782550031127,47.4131283065497,47.8480016099115,48.2828749132006,
48.7177482164198,49.1526215195718,49.5874948226593,50.0223681256851,50.457241428652,
50.8921147315628,51.3269880344203,51.7618613372274,52.197587335454,52.6333133336805,
53.0681866363954,53.5030599390685,53.9379332417027,54.3728065443011,54.8076798468664,
55.2425531494018,55.6774264519101,56.1122997543943,56.5471730568575,56.9820463593026,
57.4169196617326,57.8517929641506,58.2866662665595,58.7215395689624,59.157265567009,
59.5929915650557,60.0278648674556,60.4627381698584,60.8976114722673,61.3324847746853,
61.7673580771153,62.2022313795604,62.6371046820236,63.0719779845079,63.5068512870162,
63.9417245895516,64.376597892117,64.8114711947155,65.2463444973499,65.6812178000231,
66.1169437982275,66.5526697964318,66.9875430991915,67.4224164019987,67.8572897048563,
68.2921630077673,68.7270363107343,69.1619096137603,69.5967829168479,70.0316562200001,
70.4665295232194,70.9014028265087,71.3362761298705,71.7711494333077,72.2060227368227,
72.6408960404182,73.0766220391044,73.5123480377905,73.9472213415547,74.382094645407,
74.8169679493499,75.2518412533859,75.6867145575172,76.1215878617464,76.5564611660756,
76.9913344705072,77.4262077750435,77.8610810796866,78.2959543844386,78.7308276893018,
79.1657009942781,79.6005742993696,80.0363002988208,80.4720262982719,80.9068996035997,
81.3417729090484,81.7766462146199,82.211519520316,82.6463928261383,83.0812661320886,
83.5161394381684,83.9510127443794,84.3858860507229,84.8207593572004,85.2556326638134,
85.6905059705631,86.1253792774507,86.5602525844776,86.995978584908,87.4317045853384,
87.8665778926469,88.3014512000977,88.7363245076919,89.1711978154302,89.6060711233134,
90.0409444313423,90.4758177395175,90.9106910478396,91.345564356309,91.7804376649263,
92.2153109736917,92.6501842826055,93.085057591668,93.5199309008791,93.9556569024059,
94.3913829039327,94.8262562134414,95.2611295230986,95.6960028329042,96.1308761428578,
96.5657494529591,97.0006227632077,97.4354960736028,97.870369384144,98.3052426948304,
98.7401160056612,99.1749893166354,99.6098626277522,100.04473593901,100.915335253024,
101.351061255639,101.785934567313,102.220807879124,102.655681191068,103.090554503145,
103.525427815353,104.395174440154,105.264921065453,105.699794378283,106.134667691232,
106.569541004295,107.004414317471,107.8750136343,108.745612951339,109.615359578629,
110.485106206296,111.354852834309,112.224599462639,113.094346091254,113.964092720119,
114.834692038763,115.705291357499,116.575037986826,117.444784616267,118.314531245777,
119.184277875311,120.054024504821,120.923771134261,121.794370453112,122.66496977189,
123.534716400968,124.404463029834,125.274209658448,126.143956286779,127.013702914792,
127.883449542458,128.754048859798,129.624648176939,130.494394803617,131.364141429857,
132.233888055637,133.103634680937,133.973381305737,134.843127930023,135.71372724472,
136.584326559147,137.019199870684,137.454073182083,137.888946493341,138.323819804458,
139.193566426263,140.063313047491,140.498186357887,140.933059668136,141.367932978237,
141.802806288191,142.237679597997,142.673405599673,143.109131601348,143.544004910857,
143.978878220217,144.413751529429,144.848624838491,145.283498147405,145.718371456171,
146.153244764789,146.588118073258,147.022991381581,147.457864689756,147.892737997785,
148.327611305669,148.762484613407,149.197357921002,149.633083921574,150.068809922147,
150.503683229455,150.938556536623,151.37342984365,151.808303150538,152.243176457288,
152.678049763901,153.112923070379,153.547796376722,153.982669682934,154.417542989014,
154.852416294964,155.287289600787,155.722162906483,156.157036212055,156.592762211626,
157.028488211198,157.463361516526,157.898234821735,158.333108126826,158.767981431803,
159.202854736666,159.637728041419,160.072601346062,160.507474650599,160.94234795503,
161.37722125936,161.812094563589,162.246967867721,162.681841171757,163.1167144757,
163.552440474473,163.988166473247,164.423039777011,164.85791308069,165.292786384286,
165.727659687801,166.162532991238,166.597406294601,167.03227959789,167.46715290111,
167.902026204262,168.33689950735,168.771772810376,169.206646113343,169.641519416254,
170.076392719112,170.512118717363,170.947844715614,171.382718018374,171.817591321089,
172.252464623762,172.687337926397,173.122211228996,173.557084531561,173.991957834097,
174.426831136606,174.86170443909,175.296577741554,175.731451044,176.16632434643,
176.601197648848,177.036070951258,177.471796949306,177.907522947355,178.342396249755,
178.777269552155,179.212142854558,179.647016156968,180.081889459386,180.516762761816,
180.951636064262,181.386509366726,181.82138266921,182.256255971719,182.691129274255,
183.12600257682,183.560875879419,183.995749182054,184.431475180237,184.867201178421,
185.302074481136,185.736947783896,186.171821086704,186.606694389561,187.041567692473,
187.47644099544,187.911314298466,188.346187601554,188.781060904706,189.215934207926,
189.650807511215,190.085680814577,190.520554118015,190.95542742153,191.391153420175,
191.82687941882,192.261752722499,192.696626026263,193.131499330116,193.566372634059,
194.001245938095,194.436119242227,194.870992546456,195.305865850785,195.740739155217,
196.175612459754,196.610485764397,197.045359069149,197.480232374013,197.915105678989,
198.350831678382,198.786557677775,199.221430982984,199.656304288312,200.091177593761,
200.526050899333,200.960924205029,201.395797510852,201.830670816802,202.265544122882,
202.700417429093,203.135290735437,203.570164041915,204.005037348528,204.439910655278,
204.874783962166,205.310509962526,205.746235962887,206.181109270054,206.615982577363,
207.050855884814,207.485729192409,207.920602500147,208.355475808031,208.79034911606,
209.225222424235,209.660095732558,210.094969041027,210.529842349645,210.96471565841,
211.399588967324,211.834462276387,212.27018827784,212.705914279292,213.140787588653,
213.575660898161,214.010534207819,214.880280827579,215.31515413768,215.750027447929,
216.184900758324,216.619774068866,217.054647379553,217.489520690384,218.359267312475,
219.22986662628,219.665592628826,220.100465940363,220.535339252038,220.970212563848,
221.83995918787,222.709705812416,223.579452437468,224.014325750179,224.44919906301,
225.318945689022,226.189545005688,227.060144322571,227.929890949664,228.799637577146,
229.66938420499,230.539130833166,231.408877461643,232.278624090388,233.149223408954,
234.019822727623,234.889569356878,235.759315986267,236.629062615749,237.498809245277,
238.368555874806,239.238302504287,240.108901823183,240.979501142017,241.849247771189,
242.718994400167,243.588741028911,244.458487657389,245.328234285565,246.197980913409,
247.068580230891,247.939179548182,248.80892617507,249.678672801532,250.548419427545,
251.418166053087,252.287912678139,253.157659302684,254.028258617581,254.898857932211,
255.333731243885,255.768604555423,256.203477866821,256.63835117808,257.508097800171,
258.377844421689,258.812717732231,259.247591042627,259.682464352876,260.117337662977,
260.552210972931,260.987936974682,261.858536286089,262.293409595598,262.728282904958,
263.16315621417,263.598029523233,264.032902832147,264.467776140913,264.902649449531,
265.337522758001,265.772396066323,266.207269374499,266.642142682528,267.077015990412,
267.511889298151,267.947615298795,268.383341299439,268.81821460689,269.2530879142,
269.687961221367,270.122834528394,270.557707835282,270.992581142032,271.427454448646,
271.862327755124,272.297201061468,272.732074367679,273.166947673759,273.60182097971,
274.036694285533,274.471567591229,274.907293590862,275.343019590495,275.777892895944,
276.212766201272,276.647639506481,277.082512811573,277.51738611655,277.952259421414,
278.387132726166,278.82200603081,279.256879335346,279.691752639779,280.126625944108,
280.561499248338,280.996372552469,281.431245856506,281.866971855324,282.302697854143,
282.737571157996,283.172444461761,283.60731776544,284.042191069036,284.477064372551,
284.911937675989,285.346810979351,285.781684282641,286.216557585861,286.651430889013,
287.086304192101,287.521177495128,287.956050798095,288.390924101007,288.826650099283,
289.262376097559,289.697249400366,290.132122703127,290.566996005842,291.001869308516,
291.43674261115,291.871615913749,292.306489216315,292.741362518851,293.17623582136,
293.611109123845,294.045982426308,294.480855728754,294.915729031185,295.350602333603,
295.786328331655,296.222054329707,296.65692763211,297.091800934511,297.526674236911,
297.961547539314,298.396420841724,298.831294144142,299.266167446573,299.701040749018,
300.135914051482,300.570787353967,301.005660656476,301.440533959012,301.875407261578,
302.310280564177,302.746006562341,303.181732560506,303.616605863179,304.051479165895,
304.486352468655,304.921225771462,305.35609907432,305.790972377232,306.225845680199,
306.660718983226,307.095592286314,307.530465589466,307.965338892686,308.400212195976,
308.835085499338,309.269958802776,309.705684801381,310.141410799985,310.576284103581,
311.01115740726,311.446030711025,311.880904014878,312.315777318821,312.750650622858,
313.185523926989,313.620397231219,314.055270535549,314.490143839981,314.925017144517,
315.359890449161,315.794763753913,316.229637058777,316.665363058112,317.101089057448,
317.53596236254,317.970835667749,318.405708973077,318.840582278526,319.275455584098,
319.710328889795,320.145202195618,320.580075501568,321.014948807648,321.44982211386,
321.884695420204,322.319568726682,322.754442033295,323.189315340045,323.625041340336,
324.060767340628,324.495640647655,324.930513954822,325.365387262131,325.800260569583,
326.235133877177,326.670007184916,327.1048804928,327.539753800829,327.974627109005,
328.409500417327,328.844373725797,329.279247034415,329.714120343181,330.148993652095,
330.584719653474,331.020445654852,331.455318964064,331.890192273424,332.325065582933,
332.759938892591,333.194812202397,333.629685512351,334.064558822453,334.499432132702,
334.934305443098,335.369178753639,335.804052064326,336.673798686132,337.108671997249,
337.544397999725,337.980124002201,338.4149973136,338.849870625137,339.284743936812,
340.154490560568,341.024237184854,341.459110497191,341.893983809655,342.328857122244,
342.763730434955,343.633477060735,344.504076377234,345.374675693955,346.244422320844,
347.114168948136,347.983915575803,348.853662203817,349.723408832148,350.593155460764,
351.463754779246,352.334354097839,353.204100727012,354.07384735634,354.943593985781,
355.813340615292,356.683087244827,357.552833874338,358.423433193272,359.294032512154,
360.163779141409,361.033525770489,361.903272399355,362.77301902797,363.642765656301,
364.512512284316,365.383111601936,366.253710919371,367.123457546465,367.993204173143,
368.862950799383,369.732697425164,370.602444050463,371.472190675265,372.342789990359,
373.21338930519,373.648262617,374.083135928675,374.952882551611,375.822629173987,
376.257502484962,376.692375795793,377.12724910648,377.562122417021,377.996995727417,
378.431869037666,378.866742347767,379.302468349591,379.738194351416,380.173067661222,
380.607940970879,381.042814280388,381.477687589749,381.91256089896,382.347434208023,
382.782307516937,383.217180825703,383.652054134321,384.086927442791,384.521800751113,
384.956674059289,385.391547367318,385.826420675202,386.262146675918,386.697872676635,
387.13274598423,387.567619291681,388.00249259899,388.437365906157,388.872239213185,
389.307112520073,389.741985826823,390.176859133436,390.611732439914,391.046605746258,
391.48147905247,391.91635235855,392.351225664501,392.786098970323,393.221824970019,
393.657550969714,394.092424275286,394.527297580735,394.962170886063,395.397044191272,
395.831917496364,396.266790801341,396.701664106204,397.136537410957,397.5714107156,
398.006284020137,398.441157324569,398.876030628899,399.310903933128,399.74577723726,
400.181503236126,400.617229234991,401.052102538934,401.486975842787,401.921849146551,
402.356722450231,402.791595753827,403.226469057342,403.66134236078,404.096215664142,
404.531088967432,404.965962270651,405.400835573804,405.835708876892,406.270582179918,
406.705455482886,407.141181481189,407.576907479491,408.01178078235,408.446654085157,
408.881527387917,409.316400690633,409.751273993306,410.186147295941,410.62102059854,
411.055893901106,411.490767203642,411.925640506151,412.360513808636,412.795387111099,
413.230260413545,413.665133715976,414.100859714032,414.536585712088,414.971459014498,
415.406332316901,415.841205619301,416.276078921702,416.710952224105,417.145825526515,
417.580698828933,418.015572131364,418.45044543381,418.885318736273,419.320192038758,
419.755065341267,420.189938643803,420.624811946369,421.060537944515,421.496263942662,
421.931137245297,422.36601054797,422.800883850686,423.235757153446,423.670630456253,
424.105503759112,424.540377062023,424.975250364991,425.410123668017,425.844996971105,
426.279870274258,426.714743577477,427.149616880767,427.584490184129,428.020216182695,
428.455942181261,428.890815484776,429.325688788373,429.760562092052,430.195435395816,
430.630308699669,431.065182003612,431.500055307649,431.93492861178,432.36980191601,
432.80467522034,433.239548524772,433.674421829309,434.109295133952,434.544168438705,
434.979894437984,435.415620437262,435.850493742239,436.285367047331,436.72024035254,
437.155113657869,437.589986963318,438.024860268889,438.459733574586,438.894606880409,
439.32948018636,439.76435349244,440.199226798651,440.634100104995,441.068973411473,
441.503846718087,441.939572718309,442.375298718531,442.810172025419,443.245045332447,
443.679918639614,444.114791946923,444.549665254374,444.984538561969,445.419411869708,
445.854285177591,446.289158485621,446.724031793796,447.158905102119,447.593778410589,
448.028651719207,448.463525027973,448.899251029277,449.334977030581,449.769850339644,
450.639596958216,451.074470267725,451.509343577383,451.944216887189,452.379090197143,
452.813963507244,453.248836817493,453.683710127889,454.118583438431,454.553456749117,
454.988330059949,455.423203370923,455.858929373329,456.294655375734,456.729528686993,
457.164401998391,457.599275309929,458.469021933414,458.90389524536,459.338768557437,
459.773641869646,460.208515181983,460.643388494447,461.078261807036,461.948008432578,
462.818607748906,463.689207065461,464.55895369214,465.428700319234,466.298446946716,
467.16819357456,468.037940202737,468.907686831215,469.778286149605,470.648885468116,
471.518632097196,472.388378726451,473.258125355841,474.127871985322,474.997618614851,
475.86736524438,476.737964563343,477.608563882265,478.478310511593,479.348057140765,
480.217803769743,481.087550398488,481.957297026966,482.827043655142,483.697642972895,
484.568242290469,485.43798891776,486.307735544649,487.177482171112,488.047228797125,
488.916975422667,489.78672204772,490.657321363009,491.09304736596,491.527920678038,
492.397667301793,493.267413925005,494.137160547663,494.57203385878,495.006907169755,
495.441780480586,495.876653791273,496.311527101814,496.74640041221,497.616999724357,
498.052725726255,498.487599036209,498.922472346015,499.357345655673,499.792218965182,
500.227092274542,500.661965583754,501.096838892816,501.531712201731,501.966585510497,
502.401458819114,502.836332127584,503.271205435907,503.706078744082,504.140952052112,
504.576678052901,505.01240405369,505.447277361429,505.882150669023,506.317023976474,
506.751897283783,507.186770590951,507.621643897978,508.056517204866,508.491390511616,
508.92626381823,509.361137124708,509.796010431052,510.230883737263,510.665757043344,
511.100630349294,511.536356349053,511.972082348811,512.406955654506,512.841828960076,
513.276702265523,513.711575570849,514.146448876056,514.581322181146,515.016195486121,
515.451068790983,515.885942095733,516.320815400375,516.75568870491,517.19056200934,
517.625435313668,518.060308617896,518.496034616807,518.931760615718,519.366633919752,
519.801507223694,520.236380527545,520.671253831307,521.106127134985,521.541000438579,
521.975873742092,522.410747045528,522.845620348888,523.280493652176,523.715366955394,
524.150240258545,524.585113561631,525.019986864656,525.455712862985,525.891438861313,
526.326312164223,526.761185467079,527.196058769885,527.630932072643,528.065805375356,
528.500678678029,528.935551980661,529.370425283258,529.805298585822,530.240171888356,
530.675045190863,531.109918493346,531.544791795808,531.979665098252,532.415391096312,
532.851117094373,533.285990396789,533.720863699197,534.155737001598,534.590610303997,
535.025483606395,535.460356908796,535.895230211204,536.330103513621,536.764976816049,
537.199850118493,537.634723420955,538.069596723438,538.504470025945,538.93934332848,
539.375069326608,539.810795324736,540.245668627333,540.680541929966,541.115415232637,
541.550288535351,541.985161838109,542.420035140915,542.854908443771,543.28978174668,
543.724655049646,544.15952835267,544.594401655757,545.029274958907,545.464148262125,
545.899021565413,546.334747563939,546.770473562465,547.205346865901,547.640220169415,
548.075093473009,548.509966776686,548.944840080449,549.3797133843,549.814586688241,
550.249459992276,550.684333296405,551.119206600633,551.554079904961,551.988953209391,
552.423826513926,552.858699818567,553.294425817789,553.73015181701,554.165025121872,
554.599898426846,555.034771731937,555.469645037144,555.90451834247,556.339391647917,
556.774264953487,557.209138259182,557.644011565003,558.078884870951,558.51375817703,
558.948631483239,559.383504789581,559.818378096058,560.254104096209,560.689830096361,
561.12470340311,561.559576709996,561.994450017021,562.429323324187,562.864196631494,
563.299069938943,563.733943246536,564.168816554273,564.603689862154,565.038563170182,
565.473436478355,565.908309786676,566.343183095144,566.77805640376,567.213782404988,
567.649508406216,568.084381715128,568.519255024189,568.954128333399,569.389001642757,
569.823874952264,570.258748261921,570.693621571725,571.128494881677,571.563368191777,
572.433114812417,572.867988122957,573.302861433642,573.737734744471,574.173460746804,
574.609186749136,575.044060060251,575.913806682904,576.783553306113,577.218426617922,
577.653299929865,578.08817324194,578.523046554147,579.392793178944,580.26253980424,
581.13313912039,581.568865123709,582.003738436771,582.87348506323,583.743231690115,
584.612978317402,585.482724945065,586.352471573076,587.222218201403,588.092817519691,
588.963416838109,589.833163467083,590.702910096251,591.572656725575,592.442403355013,
593.31214998452,594.181896614051,595.05249593303,595.92309525198,596.792841881366,
597.662588510618,598.532335139693,599.402081768556,600.271828397167,601.141575025495,
602.012174343369,602.882773661074,603.752520288553,604.622266915642,605.492013542317,
606.361760168553,607.23150679433,608.101253419626,608.971852735101,609.842452050322,
610.71219867434,611.581945297822,612.451691920754,612.886565232011,613.321438543126,
613.756311854099,614.191185164928,615.060931786153,615.931531098516,616.367257100486,
616.802130410586,617.237003720538,617.671877030342,618.106750339998,618.541623649505,
618.976496958863,619.411370268073,619.846243577134,620.281116886046,620.71599019481,
621.150863503426,621.585736811894,622.020610120214,622.455483428388,622.891209429248,
623.326935430108,623.761808737989,624.196682045726,624.631555353319,625.066428660769,
625.501301968075,625.936175275241,626.371048582266,626.805921889153,627.240795195901,
627.675668502512,628.110541808988,628.54541511533,628.98028842154,629.415161727618,
629.850887727438,630.286613727259,630.72148703308,631.156360338774,631.591233644344,
632.026106949791,632.460980255118,632.895853560325,633.330726865415,633.76560017039,
634.200473475251,634.635346780002,635.070220084644,635.505093389179,635.939966693609,
636.374839997937,636.810565996897,637.246291995857,637.681165299986,638.116038604021,
638.550911907962,638.985785211813,639.420658515576,639.855531819253,640.290405122847,
640.725278426361,641.160151729796,641.595025033157,642.029898336444,642.464771639662,
642.899644942813,643.334518245899,643.770244244257,644.205970242616,644.640843545581,
645.075716848491,645.510590151347,645.945463454153,646.380336756911,646.815210059625,
647.250083362296,647.684956664929,648.119829967526,648.55470327009,648.989576572624,
649.424449875131,649.859323177614,650.294196480076,650.729922478144,651.165648476212,
651.600521778641,652.035395081057,652.470268383465,652.905141685866,653.340014988265,
653.774888290663,654.209761593065,654.644634895472,655.079508197889,655.514381500318,
655.949254802762,656.384128105224,656.819001407706,657.253874710213,657.689600708326,
658.12532670644,658.560200009004,658.995073311601,659.429946614234,659.864819916905,
660.299693219619,660.734566522377,661.169439825183,661.604313128039,662.039186430948,
662.474059733914,662.908933036938,663.343806340025,663.778679643175,664.213552946393,
664.649278944883,665.085004943373,665.519878246733,665.954751550169,666.389624853683,
666.824498157277,667.259371460954,667.694244764717,668.129118068568,668.563991372509,
668.998864676544,669.433737980674,669.868611284901,670.303484589229,670.738357893659,
671.173231198194,671.608957197361,672.044683196528,672.479556501278,672.91442980614,
673.349303111115,673.784176416205,674.219049721412,674.653923026738,675.088796332185,
675.523669637755,675.95854294345,676.393416249271,676.82828955522,677.263162861298,
677.698036167508,678.13290947385,678.568635473934,679.004361474018,679.439234780629,
679.874108087377,680.308981394264,680.743854701289,681.178728008455,681.613601315762,
682.048474623211,682.483347930804,682.91822123854,683.353094546422,683.78796785445,
684.222841162623,684.657714470944,685.092587779412,685.528313780566,685.96403978172,
686.398913090483,686.833786399396,687.268659708457,687.703533017666,688.138406327025,
688.573279636532,689.008152946187,689.443026255992,689.877899565944,690.312772876043,
690.74764618629,691.182519496684,691.617392807224,692.052266117909,692.487992120169,
692.92371812243,693.358591433403,694.228338055774,694.663211367171,695.098084678707,
695.532957990379,695.967831302188,696.402704614131,696.837577926207,697.707324550749,
698.577071175797,699.011944488507,699.447670491767,699.883396495028,700.318269807975,
701.188016434211,702.057763060886,702.927509687976,703.797256315454,704.667002943295,
705.536749571467,706.407348889651,707.277948207973,708.147694836835,709.017441465911,
709.887188095163,710.756934724548,711.626681354026,712.496427983551,713.367027302543,
714.237626621516,715.107373250954,715.977119880277,716.846866509446,717.716613138419,
718.586359767161,719.456106395635,720.32670571363,721.197305031464,722.067051659126,
722.936798286414,723.806544913299,724.676291539758,725.546038165767,726.415784791305,
727.286384106969,728.156983422381,729.026730046663,729.896476670415,730.331349982088,
730.766223293624,731.201096605021,731.635969916278,732.505716538366,733.37546315988,
733.81033647042,734.246062472462,734.681788474505,735.116661784752,735.551535094852,
735.986408404804,736.421281714608,736.856155024264,737.291028333771,737.72590164313,
738.160774952339,738.5956482614,739.030521570312,739.465394879076,739.900268187692,
740.33514149616,740.77001480448,741.205740805414,741.641466806347,742.076340114374,
742.511213422256,742.946086729993,743.380960037585,743.815833345035,744.250706652341,
744.685579959507,745.120453266533,745.555326573419,745.990199880167,746.425073186778,
746.859946493254,747.294819799596,747.729693105806,748.165419105691,748.601145105576,
749.036018411525,749.470891717346,749.90576502304,750.34063832861,750.775511634057,
751.210384939384,751.645258244591,752.080131549682,752.515004854656,752.949878159518,
753.384751464269,753.81962476891,754.254498073445,754.689371377875,755.125097376885,
755.560823375895,755.995696680123,756.430569984253,756.865443288287,757.300316592228,
757.735189896079,758.170063199842,758.604936503519,759.039809807113,759.474683110627,
759.909556414062,760.344429717423,760.779303020711,761.214176323929,761.649049627079,
762.084775625469,762.520501623858,762.955374926883,763.390248229848,763.825121532758,
764.259994835614,764.694868138419,765.129741441178,765.564614743891,765.999488046563,
766.434361349196,766.869234651793,767.304107954357,767.738981256891,768.173854559398,
768.608727861881,769.044453859958,769.480179858035,769.915053160479,770.349926462907,
770.784799765324,771.219673067731,771.654546370133,772.089419672531,772.52429297493,
772.959166277331,773.394039579739,773.828912882155,774.263786184584,774.698659487028,
775.13353278949,775.568406091973,776.004132090072,776.439858088172,776.874731390706,
777.30960469327,777.744477995867,778.1793512985,778.614224601171,779.049097903885,
779.483971206643,779.918844509449,780.353717812305,780.788591115215,781.22346441818,
781.658337721205,782.093211024291,782.528084327442,782.963810325897,783.399536324352,
783.834409627639,784.269282931,784.704156234435,785.139029537949,785.573902841543,
786.00877614522,786.443649448983,786.878522752834,787.313396056775,787.74826936081,
788.183142664939,788.618015969167,789.052889273495,789.487762577925,789.923488577038,
790.359214576152,790.794087880793,791.228961185544,791.663834490406,792.098707795381,
792.533581100471,792.968454405678,793.403327711004,793.838201016451,794.273074322021,
794.707947627716,795.142820933537,795.577694239486,796.012567545564,796.447440851774,
796.883166851791,797.318892851808,797.753766158284,798.188639464895,798.623512771643,
799.058386078529,799.493259385555,799.92813269272,800.363006000027,800.797879307477,
801.232752615069,801.667625922806,802.102499230688,802.537372538715,802.972245846889,
803.40711915521,803.84284515629,804.27857115737,804.713444465985,805.148317774749,
805.583191083662,806.018064392723,806.452937701933,806.887811011291,807.322684320798,
808.192430940258,808.62730425021,809.06217756031,809.497050870557,809.931924180951,
810.36679749149,810.802523493679,811.238249495867,811.673122806697,812.542869428785,
812.977742740041,813.412616051438,813.847489362974,814.282362674646,814.717235986455,
815.152109298398,816.021855922681,816.891602547478,817.326475860065,817.762201863265,
818.197927866466,818.632801179295,819.502547805304,820.372294431763,821.242041058648,
822.111787685935,822.981534313598,823.851280941609,824.721880259681,825.5924795779,
826.462226206642,827.331972835616,828.201719464785,829.071466094109,829.941212723546,
830.810959353053,831.681558672047,832.552157991036,833.421904620514,834.2916512499,
835.161397879151,836.031144508226,836.900891137089,837.770637765701,838.641237083811,
839.511836401767,840.381583029608,841.251329657086,842.121076284176,842.990822910851,
843.860569537087,844.730316162863,845.600915478712,846.471514794314,847.341261418855,
848.211008042874,848.645881354683,849.080754666356,849.515627977891,849.950501289288,
850.82024791166,851.689994533462,852.124867844147,852.560593846263,852.996319848379,
853.431193158772,853.866066469019,854.300939779119,855.170686398875,855.605559708531,
856.040433018038,856.475306327397,856.910179636606,857.345052945667,857.77992625458,
858.214799563344,858.64967287196,859.084546180427,859.520272181434,859.95599818244,
860.390871490614,860.825744798641,861.260618106523,861.69549141426,862.130364721852,
862.565238029302,863.000111336609,863.434984643774,863.8698579508,864.304731257686,
864.739604564434,865.174477871045,865.609351177521,866.044224483863,866.479950483814,
866.915676483765,867.350549789843,867.785423095792,868.220296401613,868.655169707307,
869.090043012877,869.524916318325,869.959789623651,870.394662928858,870.829536233948,
871.264409538923,871.699282843785,872.134156148535,872.569029453177,873.003902757712,
873.439628756773,873.875354755834,874.310228060162,874.745101364389,875.179974668519,
875.614847972553,876.049721276495,876.484594580346,876.919467884108,877.354341187786,
877.78921449138,878.224087794893,878.658961098329,879.093834401689,879.528707704977,
879.963581008195,880.399307006616,880.835033005038,881.269906308124,881.704779611148,
882.139652914114,882.574526217024,883.00939951988,883.444272822685,883.879146125444,
884.314019428157,884.748892730829,885.183766033462,885.618639336059,886.053512638623,
886.488385941157,886.923259243664,887.358985241751,887.794711239839,888.2295845423,
888.664457844744,889.099331147173,889.534204449589,889.969077751997,890.403951054398,
890.838824356797,891.273697659195,891.708570961597,892.143444264004,892.578317566421,
893.01319086885,893.448064171293,893.882937473755,894.318663471843,894.75438946993,
895.189262772437,895.624136074971,896.059009377535,896.493882680132,896.928755982765,
897.363629285437,897.798502588151,898.233375890909,898.668249193715,899.103122496571,
899.53799579948,899.972869102446,900.40774240547,900.842615708556,901.278341706978,
901.714067705399,902.148941008617,902.583814311905,903.018687615265,903.453560918701,
903.888434222214,904.323307525808,904.758180829485,905.193054133248,905.627927437099,
906.06280074104,906.497674045075,906.932547349205,907.367420653433,907.80229395776,
908.238019956821,908.673745955883,909.108619260417,909.543492565059,909.978365869809,
910.413239174671,910.848112479646,911.282985784736,911.717859089943,912.152732395269,
912.587605700716,913.022479006287,913.457352311981,913.892225617802,914.327098923751,
914.761972229829,915.19769822978,915.633424229731,916.068297536072,916.503170842548,
916.93804414916,917.372917455908,917.807790762794,918.24266406982,918.677537376985,
919.112410684292,919.547283991742,919.982157299334,920.417030607071,920.851903914953,
921.28677722298,921.721650531154,922.15737653216,922.593102533167,923.027975841635,
923.46284915025,923.897722459014,924.332595767926,924.767469076987,925.202342386197,
925.637215695556,926.072089005063,926.506962314719,926.941835624523,927.376708934475,
927.811582244575,928.246455554822,928.681328865215,929.117054867331,929.987654180132,
930.422527490961,930.857400801934,931.292274113049,931.727147424306,932.162020735703,
932.596894047238,933.46664067072,934.336387294739,934.771260606945,935.20613391928,
935.641007231742,936.076733234882,936.94733255073,937.817079176507,938.686825802743,
939.556572429418,940.426319056508,941.296065683986,942.165812311827,943.036411629783,
943.907010947893,944.776757576505,945.646504205367,946.516250834443,947.385997463694,
948.25574409308,949.125490722558,949.996090041546,950.86668936054,951.736435990048,
952.606182619485,953.475929248809,954.345675877978,955.215422506951,956.085169135693,
956.955768453912,957.826367771985,958.696114399995,959.565861027658,960.435607654946,
961.305354281831,962.175100908289,963.044847534298,963.915446850328,964.786046166116,
965.655792790913,966.525539415195,966.960412727138,967.395286038947,968.265032662155,
969.134779284809,969.569652595924,970.004525906897,970.439399217726,970.875125219914,
971.310851222103,971.745724532643,972.615471153283,973.485217773335,973.920091083139,
974.354964392795,974.789837702302,975.22471101166,975.65958432087,976.094457629931,
976.529330938844,976.964204247608,977.399077556223,977.834803557303,978.270529558383,
978.705402866704,979.140276174877,979.575149482905,980.010022790786,980.444896098523,
980.879769406116,981.314642713565,981.749516020872,982.184389328038,982.619262635063,
983.05413594195,983.489009248698,983.923882555309,984.358755861785,984.794481861802,
985.230207861819,985.665081168029,986.099954474107,986.534827780056,986.969701085877,
987.404574391571,987.839447697141,988.274321002589,988.709194307915,989.144067613122,
989.578940918212,990.013814223187,990.448687528048,990.883560832799,991.31843413744,
991.754160136554,992.189886135667,992.624759440097,993.059632744425,993.494506048653,
993.929379352783,994.364252656817,994.799125960758,995.233999264609,995.668872568372,
996.103745872049,996.538619175643,996.973492479157,997.408365782593,997.843239085953,
998.278112389241,998.713838387696,999.149564386151,999.584437689301,1000.01931099239,
1000.45418429541,1000.88905759838,1001.32393090129,1001.75880420414,1002.19367750695,
1002.62855080971,1003.06342411242,1003.49829741509,1003.93317071773,1004.36804402032,
1004.80291732289,1005.23779062542,1005.67351662352,1006.10924262162,1006.5441159241,
1006.97898922656,1007.41386252901,1007.84873583144,1008.28360913385,1008.71848243626,
1009.15335573866,1009.58822904106,1010.02310234346,1010.45797564586,1010.89284894827,
1011.32772225069,1011.76259555311,1012.19746885556,1012.63319485364,1013.06892085171,
1013.5037941542,1013.9386674567,1014.37354075924,1014.8084140618,1015.2432873644,
1015.67816066703,1016.1130339697,1016.54790727242,1016.98278057517,1017.41765387798,
1017.85252718084,1018.28740048375,1018.72227378671,1019.15714708974,1019.59287308813,
1020.02859908651,1020.46347238967,1020.89834569288,1021.33321899617,1021.76809229953,
1022.20296560297,1022.63783890648,1023.07271221007,1023.50758551375,1023.94245881752,
1024.37733212137,1024.81220542531,1025.24707872935,1025.68195203348,1026.11682533771,
1026.55255133672,1026.98827733573,1027.42315064016,1027.8580239447,1028.29289724934,
1028.72777055409,1029.16264385896,1029.59751716393,1030.03239046902,1030.46726377423,
1030.90213707956,1031.33701038501,1031.77188369058,1032.20675699628,1032.6416303021,
1033.07650360805,1033.51222960793,1033.94795560782,1034.38282891403,1034.81770222038,
1035.25257552685,1035.68744883347,1036.12232214022,1036.5571954471,1036.99206875413,
1037.4269420613,1037.86181536861,1038.29668867606,1038.73156198365,1039.16643529139,
1039.60130859927,1040.0361819073,1040.47190790824,1040.90763390917,1041.34250721749,
1041.77738052596,1042.21225383458,1042.64712714334,1043.08200045226,1043.95174707053,
1044.38662037989,1044.8214936894,1045.25636699906,1045.69124030886,1046.12611361882,
1046.56098692892,1046.99586023917,1047.43158624121,1047.86731224325,1048.3021855538,
1048.73705886448,1049.17193217531,1049.60680548629,1050.0416787974,1050.47655210866,
1050.91142542006,1051.78117204327,1052.21604535508,1052.65091866703,1053.0857919791,
1053.52066529131,1053.95553860365,1054.39126460673,1055.26186392239,1056.13161054793,
1057.00135717395,1057.43623048712,1057.87110380041,1058.7408504273,1059.61059705459,
1060.48034368225,1061.35094300009,1062.22154231809,1063.09128894656,1063.96103557531,
1064.83078220429,1065.70052883346,1066.57027546278,1067.44002209222,1068.3106214112,
1069.18122073019,1070.05096735972,1070.9207139892,1071.79046061859,1072.66020724785,
1073.52995387693,1074.39970050579,1075.27029982411,1076.1408991423,1077.01064577048,
1077.88039239832,1078.7501390258,1079.61988565289,1080.48963227957,1081.35937890581,
1082.22997822202,1083.100577538,1083.97032416305,1084.84007078759,1085.70981741161,
1086.5795640351,1087.44931065803,1087.88418396929,1088.31905728041,1088.75393059138,
1089.18965659365,1089.62538259591,1090.06025590659,1090.93000252753,1091.36487583778,
1091.79974914788,1092.23462245783,1092.66949576764,1093.1043690773,1093.5392423868,
1093.97411569616,1094.40898900538,1094.84386231444,1095.27873562335,1095.71360893212,
1096.14933493327,1096.58506093443,1097.0199342429,1097.45480755122,1097.88968085939,
1098.32455416742,1098.75942747531,1099.19430078305,1099.62917409064,1100.06404739809,
1100.4989207054,1100.93379401257,1101.36866731959,1101.80354062648,1102.23841393323,
1102.67328723984,1103.10901323993,1103.54473924001,1103.97961254636,1104.41448585257,
1104.84935915865,1105.2842324646,1105.71910577042,1106.15397907612,1106.58885238169,
1107.02372568714,1107.45859899246,1107.89347229767,1108.32834560276,1108.76321890774,
1109.1980922126,1109.63296551736,1110.06869151652,1110.50441751569,1110.93929082023,
1111.37416412466,1111.80903742899,1112.24391073322,1112.67878403735,1113.11365734139,
1113.54853064533,1113.98340394918,1114.41827725295,1114.85315055662,1115.28802386022,
1115.72289716374,1116.15777046717,1116.59264377053,1117.02836976903,1117.46409576752,
1117.89896907074,1118.33384237389,1118.76871567698,1119.20358898,1119.63846228297,
1120.07333558588,1120.50820888874,1120.94308219154,1121.3779554943,1121.81282879702,
1122.24770209969,1122.68257540233,1123.11744870492,1123.55232200749,1123.98804800561,
1124.42377400372,1124.85864730623,1125.29352060871,1125.72839391118,1126.16326721362,
1126.59814051605,1127.03301381847,1127.46788712088,1127.90276042328,1128.33763372568,
1128.77250702808,1129.20738033048,1129.64225363289,1130.07712693531,1130.51200023774,
1130.94772623581,1131.38345223388,1131.81832553634,1132.25319883883,1132.68807214134,
1133.12294544387,1133.55781874644,1133.99269204904,1134.42756535167,1134.86243865434,
1135.29731195706,1135.73218525982,1136.16705856263,1136.60193186548,1137.03680516839,
1137.47167847136,1137.90740446972,1138.34313046808,1138.77800377117,1139.21287707432,
1139.64775037754,1140.08262368083,1140.51749698419,1140.95237028763,1141.38724359114,
1141.82211689474,1142.25699019842,1142.69186350218,1143.12673680603,1143.56161010998,
1143.99648341401,1144.43135671814,1144.86708271711,1145.30280871607,1145.7376820204,
1146.17255532483,1146.60742862936,1147.04230193401,1147.47717523876,1147.91204854362,
1148.3469218486,1148.78179515369,1149.2166684589,1149.65154176423,1150.08641506968,
1150.52128837525,1150.95616168094,1151.39103498677,1151.82676098659,1152.26248698641,
1152.69736029249,1153.1322335987,1153.56710690504,1154.00198021152,1154.43685351813,
1154.87172682488,1155.30660013177,1155.7414734388,1156.17634674597,1156.61122005327,
1157.04609336073,1157.48096666832,1157.91583997606,1158.35071328394,1158.7864392848,
1159.22216528566,1159.65703859384,1160.09191190216,1160.52678521063,1160.96165851925,
1161.39653182801,1161.83140513693,1162.26627844599,1162.7011517552,1163.13602506456,
1163.57089837407,1164.00577168373,1164.44064499353,1164.87551830349,1165.74611761556,
1166.18184361753,1166.61671692792,1167.05159023846,1167.48646354915,1167.92133685998,
1168.35621017096,1169.22595679333,1170.09570341627,1170.53057672794,1170.96545003975,
1171.4003233517,1171.83519666377,1172.27006997598,1172.705795979,1173.57639529447,
1174.44614191977,1174.8810152326,1175.31588854555,1176.18563517179,1177.05538179847,
1177.92512842556,1178.79487505304,1179.66547437075,1180.53607368863,1181.40582031696,
1182.27556694557,1183.14531357444,1184.01506020352,1184.88480683277,1185.75455346216,
1186.62515278112,1187.4957521001,1188.36549872963,1189.23524535914,1190.10499198858,
1190.97473861791,1191.84448524708,1192.71423187606,1193.58483119448,1194.45543051277,
1195.3251771411,1196.19492376911,1197.06467039678,1197.93441702407,1198.80416365096,
1199.67391027742,1200.5445095938,1201.41510890996,1202.28485553525,1203.15460216005,
1204.02434878434,1204.89409540809,1205.76384203131,1206.1987153427,1206.63358865396,
1207.06846196508,1207.50418796741,1208.37478728058,1209.2445339018,1209.6794072122,
1210.11428052245,1210.54915383255,1210.9840271425,1211.41890045231,1211.85377376197,
1212.28864707147,1212.72352038083,1213.15839369005,1213.59326699911,1214.02814030802,
1214.46386630925,1214.89959231048,1215.3344656191,1215.76933892757,1216.20421223589,
1216.63908554406,1217.07395885209,1217.50883215998,1217.94370546771,1218.37857877531,
1218.81345208276,1219.24832539007,1219.68319869724,1220.11807200426,1220.55294531115,
1220.9878186179,1221.42354461805,1221.85927061821,1222.29414392468,1222.72901723103,
1223.16389053724,1223.59876384332,1224.03363714927,1224.46851045509,1224.90338376079,
1225.33825706636,1225.77313037181,1226.20800367713,1226.64287698234,1227.07775028743,
1227.51262359241,1227.94749689727,1228.3832228965,1228.81894889572,1229.25382220036,
1229.6886955049,1230.12356880933,1230.55844211366,1230.99331541789,1231.42818872202,
1231.86306202606,1232.29793533,1232.73280863385,1233.16768193762,1233.60255524129,
1234.03742854489,1234.4723018484,1234.90717515184,1235.34290115037,1235.7786271489,
1236.21350045219,1236.64837375541,1237.08324705856,1237.51812036165,1237.95299366467,
1238.38786696764,1238.82274027055,1239.25761357341,1239.69248687621,1240.12736017897,
1240.56223348169,1240.99710678436,1241.431980087,1241.8668533896,1242.30257938773,
1242.73830538585,1243.17317868839,1243.6080519909,1244.04292529338,1244.47779859585,
1244.91267189829,1245.34754520072,1245.78241850314,1246.21729180555,1246.65216510795,
1247.08703841035,1247.52191171275,1247.95678501515,1248.39165831756,1248.82653161998,
1249.26225761804,1249.69798361611,1250.13285691855,1250.56773022101,1251.0026035235,
1251.43747682601,1251.87235012854,1252.30722343111,1252.74209673371,1253.17697003634,
1253.61184333901,1254.04671664173,1254.48158994449,1254.9164632473,1255.35133655015,
1255.78620985306,1256.22193585139,1256.65766184973,1257.09253515275,1257.52740845584,
1257.96228175899,1258.39715506221,1258.8320283655,1259.26690166886,1259.7017749723,
1260.13664827581,1260.57152157941,1261.00639488309,1261.44126818685,1261.8761414907,
1262.31101479465,1262.74588809868,1263.1816140976,1263.61734009651,1264.05221340074,
1264.48708670507,1264.9219600095,1265.35683331403,1265.79170661868,1266.22657992343,
1266.66145322829,1267.09632653327,1267.53119983836,1267.96607314357,1268.4009464489,
1268.83581975434,1269.27069305992,1269.70556636561,1270.14129236537,1270.57701836513,
1271.01189167108,1271.44676497716,1271.88163828337,1272.31651158971,1272.75138489619,
1273.1862582028,1273.62113150955,1274.05600481644,1274.49087812347,1274.92575143063,
1275.36062473794,1275.79549804539,1276.23037135299,1276.66524466073,1277.10097066151,
1277.5366966623,1277.97156997033,1278.40644327851,1278.84131658683,1279.2761898953,
1279.71106320392,1280.14593651268,1280.5808098216,1281.01568313066,1281.45055643987,
1281.88542974923,1282.32030305874,1282.75517636839,1283.1900496782,1283.62492298815,
1284.06064899005,1284.49637499195,1284.9312483022,1285.36612161259,1285.80099492313,
1286.23586823382,1286.67074154465,1287.54048816674,1287.975361478,1288.4102347894,
1288.84510810093,1289.27998141261,1289.71485472442,1290.14972803636,1291.02032735139,
1291.89092666668,1292.32579997914,1292.76067329173,1293.19554660444,1293.63041991727,
1294.50016654328,1295.36991316974,1296.23965979663,1297.10940642392,1297.9800057415,
1298.85060505925,1299.72035168742,1300.5900983159,1301.45984494464,1302.32959157362,
1303.19933820279,1304.06908483212,1304.93968415104,1305.81028347,1306.68003009953,
1307.54977672906,1308.41952335854,1309.28926998793,1310.15901661718,1311.02876324626,
1311.89936256477,1312.76996188316,1313.63970851164,1314.50945513981,1315.37920176765,
1316.24894839514,1317.11869502223,1317.98844164891,1318.85904096546,1319.72964028179,
1320.59938690733,1321.46913353238,1322.33888015692,1323.20862678095,1323.64350009276,
1324.07837340443,1324.51324671597,1324.94812002737,1325.81871934103,1326.68931865441,
1327.12419196524,1327.55906527593,1327.99393858647,1328.42881189686,1328.86368520711,
1329.29855851721,1329.73343182716,1330.16830513697,1330.60317844663,1331.03805175614,
1331.4729250655,1331.90779837471,1332.34267168377,1332.77839768507,1333.21412368638,
1333.64899699514,1334.08387030376,1334.51874361223,1334.95361692055,1335.38849022873,
1335.82336353676,1336.25823684464,1336.69311015238,1337.12798345997,1337.56285676742,
1337.99773007473,1338.4326033819,1338.86747668892,1339.30234999581,1339.73807599603,
1340.17380199625,1340.60867530287,1341.04354860934,1341.47842191569,1341.9132952219,
1342.34816852798,1342.78304183393,1343.21791513975,1343.65278844545,1344.08766175102,
1344.52253505647,1344.95740836179,1345.392281667,1345.82715497209,1346.26202827707,
1346.69775427635,1347.13348027563,1347.56835358038,1348.00322688502,1348.43810018956,
1348.87297349399,1349.30784679832,1349.74272010255,1350.17759340668,1350.61246671072,
1351.04734001466,1351.48221331851,1351.91708662228,1352.35195992595,1352.78683322955,
1353.22170653306,1353.65743253163,1354.09315853019,1354.52803183356,1354.96290513685,
1355.39777844007,1355.83265174322,1356.26752504631,1356.70239834933,1357.1372716523,
1357.57214495521,1358.00701825807,1358.44189156087,1358.87676486363,1359.31163816635,
1359.74651146902,1360.18138477166,1360.6171107698,1361.05283676795,1361.48771007051,
1361.92258337305,1362.35745667556,1362.79232997804,1363.2272032805,1363.66207658295,
1364.09694988538,1364.5318231878,1364.96669649021,1365.40156979261,1365.83644309501,
1366.27131639741,1366.70618969981,1367.14106300222,1367.57678900028,1368.01251499834,
1368.44738830077,1368.88226160321,1369.31713490567,1369.75200820816,1370.18688151067,
1370.6217548132,1371.05662811577,1371.49150141837,1371.926374721,1372.36124802367,
1372.79612132639,1373.23099462915,1373.66586793196,1374.10074123481,1374.53646723311,
1374.97219323142,1375.40706653438,1375.84193983741,1376.2768131405,1376.71168644365,
1377.14655974687,1377.58143305016,1378.01630635352,1378.45117965696,1378.88605296047,
1379.32092626407,1379.75579956775,1380.19067287151,1380.62554617536,1381.06041947931,
1381.49614547817,1381.93187147704,1382.36674478117,1382.8016180854,1383.23649138973,
1383.67136469416,1384.10623799869,1384.54111130334,1384.97598460809,1385.41085791295,
1385.84573121793,1386.28060452302,1386.71547782823,1387.15035113356,1387.585224439,
1388.02009774458,1388.45582374427,1388.89154974397,1389.32642304979,1389.76129635574,
1390.19616966182,1390.63104296803,1391.06591627437,1391.50078958085,1391.93566288746,
1392.37053619421,1392.8054095011,1393.24028280813,1393.6751561153,1394.1100294226,
1394.54490273005,1394.97977603765,1395.41550203836,1395.85122803908,1396.28610134696,
1396.72097465499,1397.15584796317,1397.59072127149,1398.02559457996,1398.46046788858,
1398.89534119734,1399.33021450626,1399.76508781532,1400.19996112453,1400.63483443389,
1401.50458105306,1401.93945436286,1402.37518036469,1402.81090636651,1403.24577967661,
1403.68065298686,1404.11552629725,1404.5503996078,1404.98527291848,1405.85501954029,
1406.2898928514,1406.72476616266,1407.15963947406,1407.5945127856,1408.02938609727,
1408.46425940908,1409.33485872391,1410.205458039,1410.64033135134,1411.07520466381,
1411.51007797639,1411.9449512891,1412.81469791488,1413.68444454112,1414.5541911678,
1415.42393779489,1416.29453711233,1417.16513642995,1418.03488305796,1418.90462968629,
1419.77437631491,1420.64412294377,1421.51386957285,1422.38361620211,1423.25421552099,
1424.12481483992,1424.99456146943,1425.86430809896,1426.73405472847,1427.60380135791,
1428.47354798724,1429.34329461641,1430.21389393501,1431.08449325349,1431.9542398821,
1432.82398651043,1433.69373313844,1434.56347976611,1435.4332263934,1436.30297302029,
1437.17357233701,1438.04417165351,1438.91391827929,1439.78366490459,1440.65341152939,
1441.52315815367,1441.95803146562,1442.39290477743,1442.8277780891,1443.26265140064,
1444.13325071451,1445.00385002811,1445.43872333908,1445.87359664991,1446.3084699606,
1446.74334327114,1447.17821658153,1447.61308989178,1448.48283651184,1448.91770982164,
1449.3525831313,1449.78745644081,1450.22232975017,1450.65720305938,1451.09292906076,
1451.52865506214,1451.96352837105,1452.39840167982,1452.83327498843,1453.2681482969,
1453.70302160522,1454.1378949134,1454.57276822143,1455.00764152931,1455.44251483705,
1455.87738814464,1456.31226145209,1456.7471347594,1457.18200806657,1457.6168813736,
1458.05260737389,1458.48833337418,1458.92320668093,1459.35807998754,1459.79295329402,
1460.22782660036,1460.66269990657,1461.09757321265,1461.5324465186,1461.96731982443,
1462.40219313012,1462.83706643569,1463.27193974114,1463.70681304647,1464.14168635168,
1464.57655965677,1465.0122856561,1465.44801165544,1465.8828849603,1466.31775826505,
1466.7526315697,1467.18750487423,1467.62237817866,1468.05725148299,1468.49212478722,
1468.92699809135,1469.36187139539,1469.79674469933,1470.23161800319,1470.66649130695,
1471.10136461063,1471.53623791422,1471.97196391283,1472.40768991143,1472.84256321487,
1473.27743651823,1473.71230982152,1474.14718312474,1474.58205642789,1475.01692973098,
1475.451803034,1475.88667633697,1476.32154963988,1476.75642294274,1477.19129624555,
1477.62616954831,1478.06104285102,1478.4959161537,1478.93164215186,1479.36736815002,
1479.80224145262,1480.23711475519,1480.67198805772,1481.10686136023,1481.54173466272,
1481.97660796518,1482.41148126762,1482.84635457005,1483.28122787247,1483.71610117488,
1484.15097447728,1484.58584777968,1485.02072108208,1485.45559438449,1485.89132038254,
1486.32704638059,1486.76191968301,1487.19679298544,1487.63166628788,1488.06653959035,
1488.50141289283,1488.93628619534,1489.37115949787,1489.80603280044,1490.24090610304,
1490.67577940567,1491.11065270835,1491.54552601106,1491.98039931382,1492.41527261663,
1492.8509986149,1493.28672461318,1493.72159791609,1494.15647121906,1494.59134452208,
1495.02621782517,1495.46109112832,1495.89596443154,1496.33083773483,1496.76571103819,
1497.20058434163,1497.63545764515,1498.07033094874,1498.50520425242,1498.94007755618,
1499.37495086004,1499.81067685885,1500.24640285767,1500.68127616171,1501.11614946584,
1501.55102277007,1501.9858960744,1502.42076937883,1502.85564268337,1503.29051598801,
1503.72538929276,1504.16026259762,1504.5951359026,1505.03000920769,1505.4648825129,
1505.89975581823,1506.33462912368,1506.77035512331,1507.20608112294,1507.64095442864,
1508.07582773446,1508.51070104041,1508.94557434649,1509.3804476527,1509.81532095904,
1510.25019426552,1510.68506757213,1511.11994087888,1511.55481418577,1511.9896874928,
1512.42456079996,1512.85943410727,1513.29430741472,1513.73003341537,1514.16575941601,
1514.60063272375,1515.03550603163,1515.47037933966,1515.90525264784,1516.34012595616,
1516.77499926463,1517.20987257325,1517.64474588201,1518.07961919093,1518.51449249999,
1518.9493658092,1519.38423911856,1519.81911242807,1520.25398573772,1520.68971173947,
1521.12543774122,1521.56031105118,1521.99518436128,1522.43005767153,1523.29980429246,
1523.73467760315,1524.16955091398,1524.60442422495,1525.03929753607,1525.47417084733,
1525.90904415873,1526.77879078194,1527.64939009657,1528.08511609939,1528.51998941146,
1528.95486272367,1529.38973603601,1530.25948266106,1531.1292292866,1531.99897591261,
1532.86872253907,1533.73846916596,1534.60906848325,1535.47966780073,1536.34941442858,
1537.21916105675,1538.08890768523,1538.95865431398,1539.82840094295,1540.69814757212,
1541.56874689096,1542.43934620985,1543.30909283933,1544.17883946886,1545.04858609839,
1545.91833272787,1546.78807935726,1547.65782598651,1548.52842530518,1549.39902462375,
1550.26877125249,1551.13851788097,1552.00826450914,1552.87801113699,1553.74775776447,
1554.61750439156,1555.48810370844,1556.35870302511,1557.22844965112,1558.09819627666,
1558.96794290171,1559.83768952626,1560.27256283834,1560.70743615028,1561.57718277377,
1562.44778208785,1563.31838140165,1563.75325471277,1564.18812802374,1564.62300133457,
1565.05787464526,1565.9276212662,1566.79736788655,1567.2322411965,1567.66711450631,
1568.10198781596,1568.53686112547,1568.97173443483,1569.40746043628,1569.84318643774,
1570.2780597468,1570.71293305571,1571.14780636448,1571.5826796731,1572.01755298157,
1572.45242628989,1572.88729959806,1573.32217290609,1573.75704621397,1574.19191952171,
1574.62679282931,1575.06166613676,1575.49653944407,1575.93141275123,1576.36713875159,
1576.80286475195,1577.23773805884,1577.67261136559,1578.1074846722,1578.54235797868,
1578.97723128502,1579.41210459124,1579.84697789732,1580.28185120327,1580.71672450909,
1581.15159781478,1581.58647112036,1582.0213444258,1582.45621773113,1582.89109103634,
1583.32681703573,1583.76254303513,1584.1974163401,1584.63228964497,1585.06716294972,
1585.50203625436,1585.9369095589,1586.37178286333,1586.80665616766,1587.24152947189,
1587.67640277602,1588.11127608005,1588.546149384,1588.98102268785,1589.41589599161,
1589.85076929529,1590.28649529394,1590.72222129258,1591.1570945961,1591.59196789953,
1592.0268412029,1592.46171450619,1592.8965878094,1593.33146111256,1593.76633441564,
1594.20120771867,1594.63608102164,1595.07095432455,1595.50582762741,1595.94070093021,
1596.37557423297,1596.81044753569,1597.24617353387,1597.68189953206,1598.11677283469,
1598.55164613729,1598.98651943985,1599.42139274239,1599.8562660449,1600.29113934738,
1600.72601264985,1601.16088595229,1601.59575925472,1602.03063255714,1602.46550585955,
1602.90037916195,1603.33525246435,1603.77012576675,1604.2058517648,1604.64157776285,
1605.07645106526,1605.51132436768,1605.94619767011,1606.38107097255,1606.81594427502,
1607.2508175775,1607.68569088001,1608.12056418254,1608.55543748511,1608.99031078771,
1609.42518409034,1609.86005739302,1610.29493069573,1610.72980399849,1611.16552999674,
1611.60125599499,1612.03612929785,1612.47100260076,1612.90587590373,1613.34074920675,
1613.77562250984,1614.21049581299,1614.64536911621,1615.0802424195,1615.51511572286,
1615.9499890263,1616.38486232981,1616.81973563341,1617.25460893709,1617.68948224085,
1618.12520823963,1618.5609342384,1618.99580754234,1619.43068084638,1619.86555415051,
1620.30042745474,1620.73530075907,1621.1701740635,1621.60504736804,1622.03992067268,
1622.47479397743,1622.90966728229,1623.34454058727,1623.77941389236,1624.21428719757,
1624.6491605029,1625.08488650247,1625.52061250204,1625.95548580761,1626.39035911331,
1626.82523241913,1627.26010572508,1627.69497903116,1628.12985233737,1628.56472564372,
1628.99959895019,1629.43447225681,1629.86934556356,1630.30421887044,1630.73909217747,
1631.17396548464,1631.60883879195,1632.04456479252,1632.48029079309,1632.91516410068,
1633.35003740842,1633.78491071631,1634.21978402433,1634.65465733251,1635.08953064083,
1635.5244039493,1635.95927725792,1636.39415056668,1636.8290238756,1637.26389718466,
1637.69877049387,1638.13364380323,1638.56851711274,1639.00424311442,1639.43996911609,
1639.8748424259,1640.30971573585,1640.74458904595,1641.6143356666,1642.04920897714,
1642.48408228782,1642.91895559865,1643.35382890963,1643.78870222074,1644.223575532,
1645.09332215494,1645.52819546661,1645.96392146936,1646.39964747212,1646.83452078406,
1647.26939409614,1647.70426740834,1648.57401403314,1649.44376065844,1650.31350728422,
1650.74838059729,1651.18325391046,1652.05300053714,1652.92359985428,1653.79419917162,
1654.66394579929,1655.5336924273,1656.40343905563,1657.27318568424,1658.14293231311,
1659.01267894219,1659.88327826096,1660.75387757982,1661.62362420926,1662.49337083877,
1663.3631174683,1664.23286409781,1665.10261072725,1665.97235735658,1666.84295667531,
1667.71355599396,1668.58330262282,1669.45304925143,1670.32279587976,1671.19254250778,
1672.06228913544,1672.93203576273,1673.80263507977,1674.6732343966,1675.54298102284,
1676.41272764862,1677.28247427392,1678.15222089872,1679.021967523,1679.89171414676,
1680.76231346105,1681.19803946366,1681.63291277506,1682.06778608632,1682.50265939743,
1682.93753270841,1683.37240601924,1684.24215264047,1684.67702595086,1685.11189926111,
1685.54677257121,1685.98164588116,1686.41651919097,1686.85139250063,1687.28626581014,
1687.72199181166,1688.15771781319,1688.5925911224,1689.02746443146,1689.46233774038,
1689.89721104914,1690.33208435776,1690.76695766623,1691.20183097455,1691.63670428272,
1692.07157759075,1692.50645089864,1692.94132420637,1693.37619751397,1693.81107082142,
1694.24594412873,1694.68167012916,1695.11739612959,1695.55226943662,1695.9871427435,
1696.42201605025,1696.85688935687,1697.29176266334,1697.72663596969,1698.1615092759,
1698.59638258198,1699.03125588793,1699.46612919375,1699.90100249945,1700.33587580502,
1700.77074911047,1701.20562241579,1701.64134841525,1702.0770744147,1702.51194771979,
1702.94682102476,1703.38169432963,1703.81656763438,1704.25144093902,1704.68631424356,
1705.12118754799,1705.55606085232,1705.99093415655,1706.42580746068,1706.86068076471,
1707.29555406866,1707.73042737251,1708.16530067627,1708.60102667496,1709.03675267365,
1709.47162597724,1709.90649928076,1710.34137258419,1710.77624588756,1711.21111919085,
1711.64599249406,1712.08086579722,1712.5157391003,1712.95061240333,1713.3854857063,
1713.82035900921,1714.25523231207,1714.69010561487,1715.12497891763,1715.56070491584,
1715.99643091404,1716.43130421671,1716.86617751935,1717.30105082195,1717.73592412451,
1718.17079742705,1718.60567072956,1719.04054403204,1719.4754173345,1719.91029063695,
1720.34516393938,1720.7800372418,1721.21491054421,1721.64978384661,1722.08465714901,
1722.52038314706,1722.9561091451,1723.39098244751,1723.82585574992,1724.26072905233,
1724.69560235476,1725.13047565721,1725.56534895967,1726.00022226216,1726.43509556467,
1726.8699688672,1727.30484216977,1727.73971547236,1728.174588775,1728.60946207767,
1729.04433538039,1729.48006137861,1729.91578737684,1730.35066067965,1730.78553398251,
1731.22040728542,1731.65528058838,1732.09015389141,1732.5250271945,1732.95990049765,
1733.39477380087,1733.82964710416,1734.26452040752,1734.69939371096,1735.13426701447,
1735.56914031807,1736.00401362175,1736.43973962048,1736.8754656192,1737.31033892306,
1737.745212227,1738.18008553104,1738.61495883517,1739.0498321394,1739.48470544373,
1739.91957874816,1740.35445205269,1740.78932535734,1741.22419866209,1741.65907196695,
1742.09394527193,1742.52881857702,1742.96369188223,1743.39941788174,1743.83514388125,
1744.2700171867,1744.70489049227,1745.13976379797,1745.57463710379,1746.00951040974,
1746.44438371582,1746.87925702203,1747.31413032837,1747.74900363485,1748.18387694146,
1748.61875024821,1749.0536235551,1749.48849686213,1749.92337016929,1750.3590961698,
1750.7948221703,1751.22969547775,1751.66456878534,1752.09944209308,1752.53431540096,
1752.96918870899,1753.40406201717,1753.83893532549,1754.27380863396,1754.70868194258,
1755.14355525134,1755.57842856026,1756.01330186932,1756.44817517853,1756.88304848789,
1757.31877448949,1757.75450049109,1758.18937380075,1759.05912042051,1759.49399373061,
1759.92886704086,1760.36374035125,1760.79861366179,1761.23348697248,1761.66836028331,
1762.10323359429,1762.5381069054,1763.40785352806,1763.8427268396,1764.27845284228,
1764.71417884496,1765.14905215677,1765.58392546872,1766.0187987808,1766.88854540534,
1767.75829203039,1768.1931653431,1768.62803865593,1769.06291196888,1769.49778528195,
1770.36753190841,1771.2381312254,1772.10873054259,1772.97847717007,1773.84822379791,
1774.71797042609,1775.58771705456,1776.45746368331,1777.32721031228,1778.19780963089,
1779.06840894783,1779.93815555508,1780.80790201176,1781.67764871408),(-1.76619037896906,
-1.18309518948453),.UNSPECIFIED.) ;
#825=B_SPLINE_SURFACE_WITH_KNOTS('',3,1,((#64564,#64565),(#64566,#64567),
(#64568,#64569),(#64570,#64571),(#64572,#64573),(#64574,#64575),(#64576,
#64577),(#64578,#64579),(#64580,#64581),(#64582,#64583),(#64584,#64585),
(#64586,#64587),(#64588,#64589),(#64590,#64591),(#64592,#64593),(#64594,
#64595),(#64596,#64597),(#64598,#64599),(#64600,#64601),(#64602,#64603),
(#64604,#64605),(#64606,#64607),(#64608,#64609),(#64610,#64611),(#64612,
#64613),(#64614,#64615),(#64616,#64617),(#64618,#64619),(#64620,#64621),
(#64622,#64623),(#64624,#64625),(#64626,#64627),(#64628,#64629),(#64630,
#64631),(#64632,#64633),(#64634,#64635),(#64636,#64637),(#64638,#64639),
(#64640,#64641),(#64642,#64643),(#64644,#64645),(#64646,#64647),(#64648,
#64649),(#64650,#64651),(#64652,#64653),(#64654,#64655),(#64656,#64657),
(#64658,#64659),(#64660,#64661),(#64662,#64663),(#64664,#64665),(#64666,
#64667),(#64668,#64669),(#64670,#64671),(#64672,#64673),(#64674,#64675),
(#64676,#64677),(#64678,#64679),(#64680,#64681),(#64682,#64683),(#64684,
#64685),(#64686,#64687),(#64688,#64689),(#64690,#64691),(#64692,#64693),
(#64694,#64695),(#64696,#64697),(#64698,#64699),(#64700,#64701),(#64702,
#64703),(#64704,#64705),(#64706,#64707),(#64708,#64709),(#64710,#64711),
(#64712,#64713),(#64714,#64715),(#64716,#64717),(#64718,#64719),(#64720,
#64721),(#64722,#64723),(#64724,#64725),(#64726,#64727),(#64728,#64729),
(#64730,#64731),(#64732,#64733),(#64734,#64735),(#64736,#64737),(#64738,
#64739),(#64740,#64741),(#64742,#64743),(#64744,#64745),(#64746,#64747),
(#64748,#64749),(#64750,#64751),(#64752,#64753),(#64754,#64755),(#64756,
#64757),(#64758,#64759),(#64760,#64761),(#64762,#64763),(#64764,#64765),
(#64766,#64767),(#64768,#64769),(#64770,#64771),(#64772,#64773),(#64774,
#64775),(#64776,#64777),(#64778,#64779),(#64780,#64781),(#64782,#64783),
(#64784,#64785),(#64786,#64787),(#64788,#64789),(#64790,#64791),(#64792,
#64793),(#64794,#64795),(#64796,#64797),(#64798,#64799),(#64800,#64801),
(#64802,#64803),(#64804,#64805),(#64806,#64807),(#64808,#64809),(#64810,
#64811),(#64812,#64813),(#64814,#64815),(#64816,#64817),(#64818,#64819),
(#64820,#64821),(#64822,#64823),(#64824,#64825),(#64826,#64827),(#64828,
#64829),(#64830,#64831),(#64832,#64833),(#64834,#64835),(#64836,#64837),
(#64838,#64839),(#64840,#64841),(#64842,#64843),(#64844,#64845),(#64846,
#64847),(#64848,#64849),(#64850,#64851),(#64852,#64853),(#64854,#64855),
(#64856,#64857),(#64858,#64859),(#64860,#64861),(#64862,#64863),(#64864,
#64865),(#64866,#64867),(#64868,#64869),(#64870,#64871),(#64872,#64873),
(#64874,#64875),(#64876,#64877),(#64878,#64879),(#64880,#64881),(#64882,
#64883),(#64884,#64885),(#64886,#64887),(#64888,#64889),(#64890,#64891),
(#64892,#64893),(#64894,#64895),(#64896,#64897),(#64898,#64899),(#64900,
#64901),(#64902,#64903),(#64904,#64905),(#64906,#64907),(#64908,#64909),
(#64910,#64911),(#64912,#64913),(#64914,#64915),(#64916,#64917),(#64918,
#64919),(#64920,#64921),(#64922,#64923),(#64924,#64925),(#64926,#64927),
(#64928,#64929),(#64930,#64931),(#64932,#64933),(#64934,#64935),(#64936,
#64937),(#64938,#64939),(#64940,#64941),(#64942,#64943),(#64944,#64945),
(#64946,#64947),(#64948,#64949),(#64950,#64951),(#64952,#64953),(#64954,
#64955),(#64956,#64957),(#64958,#64959),(#64960,#64961),(#64962,#64963),
(#64964,#64965),(#64966,#64967),(#64968,#64969),(#64970,#64971),(#64972,
#64973),(#64974,#64975),(#64976,#64977),(#64978,#64979),(#64980,#64981),
(#64982,#64983),(#64984,#64985),(#64986,#64987),(#64988,#64989),(#64990,
#64991),(#64992,#64993),(#64994,#64995),(#64996,#64997),(#64998,#64999),
(#65000,#65001),(#65002,#65003),(#65004,#65005),(#65006,#65007),(#65008,
#65009),(#65010,#65011),(#65012,#65013),(#65014,#65015),(#65016,#65017),
(#65018,#65019),(#65020,#65021),(#65022,#65023),(#65024,#65025),(#65026,
#65027),(#65028,#65029),(#65030,#65031),(#65032,#65033),(#65034,#65035),
(#65036,#65037),(#65038,#65039),(#65040,#65041),(#65042,#65043),(#65044,
#65045),(#65046,#65047),(#65048,#65049),(#65050,#65051),(#65052,#65053),
(#65054,#65055),(#65056,#65057),(#65058,#65059),(#65060,#65061),(#65062,
#65063),(#65064,#65065),(#65066,#65067),(#65068,#65069),(#65070,#65071),
(#65072,#65073),(#65074,#65075),(#65076,#65077),(#65078,#65079),(#65080,
#65081),(#65082,#65083),(#65084,#65085),(#65086,#65087),(#65088,#65089),
(#65090,#65091),(#65092,#65093),(#65094,#65095),(#65096,#65097),(#65098,
#65099),(#65100,#65101),(#65102,#65103),(#65104,#65105),(#65106,#65107),
(#65108,#65109),(#65110,#65111),(#65112,#65113),(#65114,#65115),(#65116,
#65117),(#65118,#65119),(#65120,#65121),(#65122,#65123),(#65124,#65125),
(#65126,#65127),(#65128,#65129),(#65130,#65131),(#65132,#65133),(#65134,
#65135),(#65136,#65137),(#65138,#65139),(#65140,#65141),(#65142,#65143),
(#65144,#65145),(#65146,#65147),(#65148,#65149),(#65150,#65151),(#65152,
#65153),(#65154,#65155),(#65156,#65157),(#65158,#65159),(#65160,#65161),
(#65162,#65163),(#65164,#65165),(#65166,#65167),(#65168,#65169),(#65170,
#65171),(#65172,#65173),(#65174,#65175),(#65176,#65177),(#65178,#65179),
(#65180,#65181),(#65182,#65183),(#65184,#65185),(#65186,#65187),(#65188,
#65189),(#65190,#65191),(#65192,#65193),(#65194,#65195),(#65196,#65197),
(#65198,#65199),(#65200,#65201),(#65202,#65203),(#65204,#65205),(#65206,
#65207),(#65208,#65209),(#65210,#65211),(#65212,#65213),(#65214,#65215),
(#65216,#65217),(#65218,#65219),(#65220,#65221),(#65222,#65223),(#65224,
#65225),(#65226,#65227),(#65228,#65229),(#65230,#65231),(#65232,#65233),
(#65234,#65235),(#65236,#65237),(#65238,#65239),(#65240,#65241),(#65242,
#65243),(#65244,#65245),(#65246,#65247),(#65248,#65249),(#65250,#65251),
(#65252,#65253),(#65254,#65255),(#65256,#65257),(#65258,#65259),(#65260,
#65261),(#65262,#65263),(#65264,#65265),(#65266,#65267),(#65268,#65269),
(#65270,#65271),(#65272,#65273),(#65274,#65275),(#65276,#65277),(#65278,
#65279),(#65280,#65281),(#65282,#65283),(#65284,#65285),(#65286,#65287),
(#65288,#65289),(#65290,#65291),(#65292,#65293),(#65294,#65295),(#65296,
#65297),(#65298,#65299),(#65300,#65301),(#65302,#65303),(#65304,#65305),
(#65306,#65307),(#65308,#65309),(#65310,#65311),(#65312,#65313),(#65314,
#65315),(#65316,#65317),(#65318,#65319),(#65320,#65321),(#65322,#65323),
(#65324,#65325),(#65326,#65327),(#65328,#65329),(#65330,#65331),(#65332,
#65333),(#65334,#65335),(#65336,#65337),(#65338,#65339),(#65340,#65341),
(#65342,#65343),(#65344,#65345),(#65346,#65347),(#65348,#65349),(#65350,
#65351),(#65352,#65353),(#65354,#65355),(#65356,#65357),(#65358,#65359),
(#65360,#65361),(#65362,#65363),(#65364,#65365),(#65366,#65367),(#65368,
#65369),(#65370,#65371),(#65372,#65373),(#65374,#65375),(#65376,#65377),
(#65378,#65379),(#65380,#65381),(#65382,#65383),(#65384,#65385),(#65386,
#65387),(#65388,#65389),(#65390,#65391),(#65392,#65393),(#65394,#65395),
(#65396,#65397),(#65398,#65399),(#65400,#65401),(#65402,#65403),(#65404,
#65405),(#65406,#65407),(#65408,#65409),(#65410,#65411),(#65412,#65413),
(#65414,#65415),(#65416,#65417),(#65418,#65419),(#65420,#65421),(#65422,
#65423),(#65424,#65425),(#65426,#65427),(#65428,#65429),(#65430,#65431),
(#65432,#65433),(#65434,#65435),(#65436,#65437),(#65438,#65439),(#65440,
#65441),(#65442,#65443),(#65444,#65445),(#65446,#65447),(#65448,#65449),
(#65450,#65451),(#65452,#65453),(#65454,#65455),(#65456,#65457),(#65458,
#65459),(#65460,#65461),(#65462,#65463),(#65464,#65465),(#65466,#65467),
(#65468,#65469),(#65470,#65471),(#65472,#65473),(#65474,#65475),(#65476,
#65477),(#65478,#65479),(#65480,#65481),(#65482,#65483),(#65484,#65485),
(#65486,#65487),(#65488,#65489),(#65490,#65491),(#65492,#65493),(#65494,
#65495),(#65496,#65497),(#65498,#65499),(#65500,#65501),(#65502,#65503),
(#65504,#65505),(#65506,#65507),(#65508,#65509),(#65510,#65511),(#65512,
#65513),(#65514,#65515),(#65516,#65517),(#65518,#65519),(#65520,#65521),
(#65522,#65523),(#65524,#65525),(#65526,#65527),(#65528,#65529),(#65530,
#65531),(#65532,#65533),(#65534,#65535),(#65536,#65537),(#65538,#65539),
(#65540,#65541),(#65542,#65543),(#65544,#65545),(#65546,#65547),(#65548,
#65549),(#65550,#65551),(#65552,#65553),(#65554,#65555),(#65556,#65557),
(#65558,#65559),(#65560,#65561),(#65562,#65563),(#65564,#65565),(#65566,
#65567),(#65568,#65569),(#65570,#65571),(#65572,#65573),(#65574,#65575),
(#65576,#65577),(#65578,#65579),(#65580,#65581),(#65582,#65583),(#65584,
#65585),(#65586,#65587),(#65588,#65589),(#65590,#65591),(#65592,#65593),
(#65594,#65595),(#65596,#65597),(#65598,#65599),(#65600,#65601),(#65602,
#65603),(#65604,#65605),(#65606,#65607),(#65608,#65609),(#65610,#65611),
(#65612,#65613),(#65614,#65615),(#65616,#65617),(#65618,#65619),(#65620,
#65621),(#65622,#65623),(#65624,#65625),(#65626,#65627),(#65628,#65629),
(#65630,#65631),(#65632,#65633),(#65634,#65635),(#65636,#65637),(#65638,
#65639),(#65640,#65641),(#65642,#65643),(#65644,#65645),(#65646,#65647),
(#65648,#65649),(#65650,#65651),(#65652,#65653),(#65654,#65655),(#65656,
#65657),(#65658,#65659),(#65660,#65661),(#65662,#65663),(#65664,#65665),
(#65666,#65667),(#65668,#65669),(#65670,#65671),(#65672,#65673),(#65674,
#65675),(#65676,#65677),(#65678,#65679),(#65680,#65681),(#65682,#65683),
(#65684,#65685),(#65686,#65687),(#65688,#65689),(#65690,#65691),(#65692,
#65693),(#65694,#65695),(#65696,#65697),(#65698,#65699),(#65700,#65701),
(#65702,#65703),(#65704,#65705),(#65706,#65707),(#65708,#65709),(#65710,
#65711),(#65712,#65713),(#65714,#65715),(#65716,#65717),(#65718,#65719),
(#65720,#65721),(#65722,#65723),(#65724,#65725),(#65726,#65727),(#65728,
#65729),(#65730,#65731),(#65732,#65733),(#65734,#65735),(#65736,#65737),
(#65738,#65739),(#65740,#65741),(#65742,#65743),(#65744,#65745),(#65746,
#65747),(#65748,#65749),(#65750,#65751),(#65752,#65753),(#65754,#65755),
(#65756,#65757),(#65758,#65759),(#65760,#65761),(#65762,#65763),(#65764,
#65765),(#65766,#65767),(#65768,#65769),(#65770,#65771),(#65772,#65773),
(#65774,#65775),(#65776,#65777),(#65778,#65779),(#65780,#65781),(#65782,
#65783),(#65784,#65785),(#65786,#65787),(#65788,#65789),(#65790,#65791),
(#65792,#65793),(#65794,#65795),(#65796,#65797),(#65798,#65799),(#65800,
#65801),(#65802,#65803),(#65804,#65805),(#65806,#65807),(#65808,#65809),
(#65810,#65811),(#65812,#65813),(#65814,#65815),(#65816,#65817),(#65818,
#65819),(#65820,#65821),(#65822,#65823),(#65824,#65825),(#65826,#65827),
(#65828,#65829),(#65830,#65831),(#65832,#65833),(#65834,#65835),(#65836,
#65837),(#65838,#65839),(#65840,#65841),(#65842,#65843),(#65844,#65845),
(#65846,#65847),(#65848,#65849),(#65850,#65851),(#65852,#65853),(#65854,
#65855),(#65856,#65857),(#65858,#65859),(#65860,#65861),(#65862,#65863),
(#65864,#65865),(#65866,#65867),(#65868,#65869),(#65870,#65871),(#65872,
#65873),(#65874,#65875),(#65876,#65877),(#65878,#65879),(#65880,#65881),
(#65882,#65883),(#65884,#65885),(#65886,#65887),(#65888,#65889),(#65890,
#65891),(#65892,#65893),(#65894,#65895),(#65896,#65897),(#65898,#65899),
(#65900,#65901),(#65902,#65903),(#65904,#65905),(#65906,#65907),(#65908,
#65909),(#65910,#65911),(#65912,#65913),(#65914,#65915),(#65916,#65917),
(#65918,#65919),(#65920,#65921),(#65922,#65923),(#65924,#65925),(#65926,
#65927),(#65928,#65929),(#65930,#65931),(#65932,#65933),(#65934,#65935),
(#65936,#65937),(#65938,#65939),(#65940,#65941),(#65942,#65943),(#65944,
#65945),(#65946,#65947),(#65948,#65949),(#65950,#65951),(#65952,#65953),
(#65954,#65955),(#65956,#65957),(#65958,#65959),(#65960,#65961),(#65962,
#65963),(#65964,#65965),(#65966,#65967),(#65968,#65969),(#65970,#65971),
(#65972,#65973),(#65974,#65975),(#65976,#65977),(#65978,#65979),(#65980,
#65981),(#65982,#65983),(#65984,#65985),(#65986,#65987),(#65988,#65989),
(#65990,#65991),(#65992,#65993),(#65994,#65995),(#65996,#65997),(#65998,
#65999),(#66000,#66001),(#66002,#66003),(#66004,#66005),(#66006,#66007),
(#66008,#66009),(#66010,#66011),(#66012,#66013),(#66014,#66015),(#66016,
#66017),(#66018,#66019),(#66020,#66021),(#66022,#66023),(#66024,#66025),
(#66026,#66027),(#66028,#66029),(#66030,#66031),(#66032,#66033),(#66034,
#66035),(#66036,#66037),(#66038,#66039),(#66040,#66041),(#66042,#66043),
(#66044,#66045),(#66046,#66047),(#66048,#66049),(#66050,#66051),(#66052,
#66053),(#66054,#66055),(#66056,#66057),(#66058,#66059),(#66060,#66061),
(#66062,#66063),(#66064,#66065),(#66066,#66067),(#66068,#66069),(#66070,
#66071),(#66072,#66073),(#66074,#66075),(#66076,#66077),(#66078,#66079),
(#66080,#66081),(#66082,#66083),(#66084,#66085),(#66086,#66087),(#66088,
#66089),(#66090,#66091),(#66092,#66093),(#66094,#66095),(#66096,#66097),
(#66098,#66099),(#66100,#66101),(#66102,#66103),(#66104,#66105),(#66106,
#66107),(#66108,#66109),(#66110,#66111),(#66112,#66113),(#66114,#66115),
(#66116,#66117),(#66118,#66119),(#66120,#66121),(#66122,#66123),(#66124,
#66125),(#66126,#66127),(#66128,#66129),(#66130,#66131),(#66132,#66133),
(#66134,#66135),(#66136,#66137),(#66138,#66139),(#66140,#66141),(#66142,
#66143),(#66144,#66145),(#66146,#66147),(#66148,#66149),(#66150,#66151),
(#66152,#66153),(#66154,#66155),(#66156,#66157),(#66158,#66159),(#66160,
#66161),(#66162,#66163),(#66164,#66165),(#66166,#66167),(#66168,#66169),
(#66170,#66171),(#66172,#66173),(#66174,#66175),(#66176,#66177),(#66178,
#66179),(#66180,#66181),(#66182,#66183),(#66184,#66185),(#66186,#66187),
(#66188,#66189),(#66190,#66191),(#66192,#66193),(#66194,#66195),(#66196,
#66197),(#66198,#66199),(#66200,#66201),(#66202,#66203),(#66204,#66205),
(#66206,#66207),(#66208,#66209),(#66210,#66211),(#66212,#66213),(#66214,
#66215),(#66216,#66217),(#66218,#66219),(#66220,#66221),(#66222,#66223),
(#66224,#66225),(#66226,#66227),(#66228,#66229),(#66230,#66231),(#66232,
#66233),(#66234,#66235),(#66236,#66237),(#66238,#66239),(#66240,#66241),
(#66242,#66243),(#66244,#66245),(#66246,#66247),(#66248,#66249),(#66250,
#66251),(#66252,#66253),(#66254,#66255),(#66256,#66257),(#66258,#66259),
(#66260,#66261),(#66262,#66263),(#66264,#66265),(#66266,#66267),(#66268,
#66269),(#66270,#66271),(#66272,#66273),(#66274,#66275),(#66276,#66277),
(#66278,#66279),(#66280,#66281),(#66282,#66283),(#66284,#66285),(#66286,
#66287),(#66288,#66289),(#66290,#66291),(#66292,#66293),(#66294,#66295),
(#66296,#66297),(#66298,#66299),(#66300,#66301),(#66302,#66303),(#66304,
#66305),(#66306,#66307),(#66308,#66309),(#66310,#66311),(#66312,#66313),
(#66314,#66315),(#66316,#66317),(#66318,#66319),(#66320,#66321),(#66322,
#66323),(#66324,#66325),(#66326,#66327),(#66328,#66329),(#66330,#66331),
(#66332,#66333),(#66334,#66335),(#66336,#66337),(#66338,#66339),(#66340,
#66341),(#66342,#66343),(#66344,#66345),(#66346,#66347),(#66348,#66349),
(#66350,#66351),(#66352,#66353),(#66354,#66355),(#66356,#66357),(#66358,
#66359),(#66360,#66361),(#66362,#66363),(#66364,#66365),(#66366,#66367),
(#66368,#66369),(#66370,#66371),(#66372,#66373),(#66374,#66375),(#66376,
#66377),(#66378,#66379),(#66380,#66381),(#66382,#66383),(#66384,#66385),
(#66386,#66387),(#66388,#66389),(#66390,#66391),(#66392,#66393),(#66394,
#66395),(#66396,#66397),(#66398,#66399),(#66400,#66401),(#66402,#66403),
(#66404,#66405),(#66406,#66407),(#66408,#66409),(#66410,#66411),(#66412,
#66413),(#66414,#66415),(#66416,#66417),(#66418,#66419),(#66420,#66421),
(#66422,#66423),(#66424,#66425),(#66426,#66427),(#66428,#66429),(#66430,
#66431),(#66432,#66433),(#66434,#66435),(#66436,#66437),(#66438,#66439),
(#66440,#66441),(#66442,#66443),(#66444,#66445),(#66446,#66447),(#66448,
#66449),(#66450,#66451),(#66452,#66453),(#66454,#66455),(#66456,#66457),
(#66458,#66459),(#66460,#66461),(#66462,#66463),(#66464,#66465),(#66466,
#66467),(#66468,#66469),(#66470,#66471),(#66472,#66473),(#66474,#66475),
(#66476,#66477),(#66478,#66479),(#66480,#66481),(#66482,#66483),(#66484,
#66485),(#66486,#66487),(#66488,#66489),(#66490,#66491),(#66492,#66493),
(#66494,#66495),(#66496,#66497),(#66498,#66499),(#66500,#66501),(#66502,
#66503),(#66504,#66505),(#66506,#66507),(#66508,#66509),(#66510,#66511),
(#66512,#66513),(#66514,#66515),(#66516,#66517),(#66518,#66519),(#66520,
#66521),(#66522,#66523),(#66524,#66525),(#66526,#66527),(#66528,#66529),
(#66530,#66531),(#66532,#66533),(#66534,#66535),(#66536,#66537),(#66538,
#66539),(#66540,#66541),(#66542,#66543),(#66544,#66545),(#66546,#66547),
(#66548,#66549),(#66550,#66551),(#66552,#66553),(#66554,#66555),(#66556,
#66557),(#66558,#66559),(#66560,#66561),(#66562,#66563),(#66564,#66565),
(#66566,#66567),(#66568,#66569),(#66570,#66571),(#66572,#66573),(#66574,
#66575),(#66576,#66577),(#66578,#66579),(#66580,#66581),(#66582,#66583),
(#66584,#66585),(#66586,#66587),(#66588,#66589),(#66590,#66591),(#66592,
#66593),(#66594,#66595),(#66596,#66597),(#66598,#66599),(#66600,#66601),
(#66602,#66603),(#66604,#66605),(#66606,#66607),(#66608,#66609),(#66610,
#66611),(#66612,#66613),(#66614,#66615),(#66616,#66617),(#66618,#66619),
(#66620,#66621),(#66622,#66623),(#66624,#66625),(#66626,#66627),(#66628,
#66629),(#66630,#66631),(#66632,#66633),(#66634,#66635),(#66636,#66637),
(#66638,#66639),(#66640,#66641),(#66642,#66643),(#66644,#66645),(#66646,
#66647),(#66648,#66649),(#66650,#66651),(#66652,#66653),(#66654,#66655),
(#66656,#66657),(#66658,#66659),(#66660,#66661),(#66662,#66663),(#66664,
#66665),(#66666,#66667),(#66668,#66669),(#66670,#66671),(#66672,#66673),
(#66674,#66675),(#66676,#66677),(#66678,#66679),(#66680,#66681),(#66682,
#66683),(#66684,#66685),(#66686,#66687),(#66688,#66689),(#66690,#66691),
(#66692,#66693),(#66694,#66695),(#66696,#66697),(#66698,#66699),(#66700,
#66701),(#66702,#66703),(#66704,#66705),(#66706,#66707),(#66708,#66709),
(#66710,#66711),(#66712,#66713),(#66714,#66715),(#66716,#66717),(#66718,
#66719),(#66720,#66721),(#66722,#66723),(#66724,#66725),(#66726,#66727),
(#66728,#66729),(#66730,#66731),(#66732,#66733),(#66734,#66735),(#66736,
#66737),(#66738,#66739),(#66740,#66741),(#66742,#66743),(#66744,#66745),
(#66746,#66747),(#66748,#66749),(#66750,#66751),(#66752,#66753),(#66754,
#66755),(#66756,#66757),(#66758,#66759),(#66760,#66761),(#66762,#66763),
(#66764,#66765),(#66766,#66767),(#66768,#66769),(#66770,#66771),(#66772,
#66773),(#66774,#66775),(#66776,#66777),(#66778,#66779),(#66780,#66781),
(#66782,#66783),(#66784,#66785),(#66786,#66787),(#66788,#66789),(#66790,
#66791),(#66792,#66793),(#66794,#66795),(#66796,#66797),(#66798,#66799),
(#66800,#66801),(#66802,#66803),(#66804,#66805),(#66806,#66807),(#66808,
#66809),(#66810,#66811),(#66812,#66813),(#66814,#66815),(#66816,#66817),
(#66818,#66819),(#66820,#66821),(#66822,#66823),(#66824,#66825),(#66826,
#66827),(#66828,#66829),(#66830,#66831),(#66832,#66833),(#66834,#66835),
(#66836,#66837),(#66838,#66839),(#66840,#66841),(#66842,#66843),(#66844,
#66845),(#66846,#66847),(#66848,#66849),(#66850,#66851),(#66852,#66853),
(#66854,#66855),(#66856,#66857),(#66858,#66859),(#66860,#66861),(#66862,
#66863),(#66864,#66865),(#66866,#66867),(#66868,#66869),(#66870,#66871),
(#66872,#66873),(#66874,#66875),(#66876,#66877),(#66878,#66879),(#66880,
#66881),(#66882,#66883),(#66884,#66885),(#66886,#66887),(#66888,#66889),
(#66890,#66891),(#66892,#66893),(#66894,#66895),(#66896,#66897),(#66898,
#66899),(#66900,#66901),(#66902,#66903),(#66904,#66905),(#66906,#66907),
(#66908,#66909),(#66910,#66911),(#66912,#66913),(#66914,#66915),(#66916,
#66917),(#66918,#66919),(#66920,#66921),(#66922,#66923),(#66924,#66925),
(#66926,#66927),(#66928,#66929),(#66930,#66931),(#66932,#66933),(#66934,
#66935),(#66936,#66937),(#66938,#66939),(#66940,#66941),(#66942,#66943),
(#66944,#66945),(#66946,#66947),(#66948,#66949),(#66950,#66951),(#66952,
#66953),(#66954,#66955),(#66956,#66957),(#66958,#66959),(#66960,#66961),
(#66962,#66963),(#66964,#66965),(#66966,#66967),(#66968,#66969),(#66970,
#66971),(#66972,#66973),(#66974,#66975),(#66976,#66977),(#66978,#66979),
(#66980,#66981),(#66982,#66983),(#66984,#66985),(#66986,#66987),(#66988,
#66989),(#66990,#66991),(#66992,#66993),(#66994,#66995),(#66996,#66997),
(#66998,#66999),(#67000,#67001),(#67002,#67003),(#67004,#67005),(#67006,
#67007),(#67008,#67009),(#67010,#67011),(#67012,#67013),(#67014,#67015),
(#67016,#67017),(#67018,#67019),(#67020,#67021),(#67022,#67023),(#67024,
#67025),(#67026,#67027),(#67028,#67029),(#67030,#67031),(#67032,#67033),
(#67034,#67035),(#67036,#67037),(#67038,#67039),(#67040,#67041),(#67042,
#67043),(#67044,#67045),(#67046,#67047),(#67048,#67049),(#67050,#67051),
(#67052,#67053),(#67054,#67055),(#67056,#67057),(#67058,#67059),(#67060,
#67061),(#67062,#67063),(#67064,#67065),(#67066,#67067),(#67068,#67069),
(#67070,#67071),(#67072,#67073),(#67074,#67075),(#67076,#67077),(#67078,
#67079),(#67080,#67081),(#67082,#67083),(#67084,#67085),(#67086,#67087),
(#67088,#67089),(#67090,#67091),(#67092,#67093),(#67094,#67095),(#67096,
#67097),(#67098,#67099),(#67100,#67101),(#67102,#67103),(#67104,#67105),
(#67106,#67107),(#67108,#67109),(#67110,#67111),(#67112,#67113),(#67114,
#67115),(#67116,#67117),(#67118,#67119),(#67120,#67121),(#67122,#67123),
(#67124,#67125),(#67126,#67127),(#67128,#67129),(#67130,#67131),(#67132,
#67133),(#67134,#67135),(#67136,#67137),(#67138,#67139),(#67140,#67141),
(#67142,#67143),(#67144,#67145),(#67146,#67147),(#67148,#67149),(#67150,
#67151),(#67152,#67153),(#67154,#67155),(#67156,#67157),(#67158,#67159),
(#67160,#67161),(#67162,#67163),(#67164,#67165),(#67166,#67167),(#67168,
#67169),(#67170,#67171),(#67172,#67173),(#67174,#67175),(#67176,#67177),
(#67178,#67179),(#67180,#67181),(#67182,#67183),(#67184,#67185),(#67186,
#67187),(#67188,#67189),(#67190,#67191),(#67192,#67193),(#67194,#67195),
(#67196,#67197),(#67198,#67199),(#67200,#67201),(#67202,#67203),(#67204,
#67205),(#67206,#67207),(#67208,#67209),(#67210,#67211),(#67212,#67213),
(#67214,#67215),(#67216,#67217),(#67218,#67219),(#67220,#67221),(#67222,
#67223),(#67224,#67225),(#67226,#67227),(#67228,#67229),(#67230,#67231),
(#67232,#67233),(#67234,#67235),(#67236,#67237),(#67238,#67239),(#67240,
#67241),(#67242,#67243),(#67244,#67245),(#67246,#67247),(#67248,#67249),
(#67250,#67251),(#67252,#67253),(#67254,#67255),(#67256,#67257),(#67258,
#67259),(#67260,#67261),(#67262,#67263),(#67264,#67265),(#67266,#67267),
(#67268,#67269),(#67270,#67271),(#67272,#67273),(#67274,#67275),(#67276,
#67277),(#67278,#67279),(#67280,#67281),(#67282,#67283),(#67284,#67285),
(#67286,#67287),(#67288,#67289),(#67290,#67291),(#67292,#67293),(#67294,
#67295),(#67296,#67297),(#67298,#67299),(#67300,#67301),(#67302,#67303),
(#67304,#67305),(#67306,#67307),(#67308,#67309),(#67310,#67311),(#67312,
#67313),(#67314,#67315),(#67316,#67317),(#67318,#67319),(#67320,#67321),
(#67322,#67323),(#67324,#67325),(#67326,#67327),(#67328,#67329),(#67330,
#67331),(#67332,#67333),(#67334,#67335),(#67336,#67337),(#67338,#67339),
(#67340,#67341),(#67342,#67343),(#67344,#67345),(#67346,#67347),(#67348,
#67349),(#67350,#67351),(#67352,#67353),(#67354,#67355),(#67356,#67357),
(#67358,#67359),(#67360,#67361),(#67362,#67363),(#67364,#67365),(#67366,
#67367),(#67368,#67369),(#67370,#67371),(#67372,#67373),(#67374,#67375),
(#67376,#67377),(#67378,#67379),(#67380,#67381),(#67382,#67383),(#67384,
#67385),(#67386,#67387),(#67388,#67389),(#67390,#67391),(#67392,#67393),
(#67394,#67395),(#67396,#67397),(#67398,#67399),(#67400,#67401),(#67402,
#67403),(#67404,#67405),(#67406,#67407),(#67408,#67409),(#67410,#67411),
(#67412,#67413),(#67414,#67415),(#67416,#67417),(#67418,#67419),(#67420,
#67421),(#67422,#67423),(#67424,#67425),(#67426,#67427),(#67428,#67429),
(#67430,#67431),(#67432,#67433),(#67434,#67435),(#67436,#67437),(#67438,
#67439),(#67440,#67441),(#67442,#67443),(#67444,#67445),(#67446,#67447),
(#67448,#67449),(#67450,#67451),(#67452,#67453),(#67454,#67455),(#67456,
#67457),(#67458,#67459),(#67460,#67461),(#67462,#67463),(#67464,#67465),
(#67466,#67467),(#67468,#67469),(#67470,#67471),(#67472,#67473),(#67474,
#67475),(#67476,#67477),(#67478,#67479),(#67480,#67481),(#67482,#67483),
(#67484,#67485),(#67486,#67487),(#67488,#67489),(#67490,#67491),(#67492,
#67493),(#67494,#67495),(#67496,#67497),(#67498,#67499),(#67500,#67501),
(#67502,#67503),(#67504,#67505),(#67506,#67507),(#67508,#67509),(#67510,
#67511),(#67512,#67513),(#67514,#67515),(#67516,#67517),(#67518,#67519),
(#67520,#67521),(#67522,#67523),(#67524,#67525),(#67526,#67527),(#67528,
#67529),(#67530,#67531),(#67532,#67533),(#67534,#67535),(#67536,#67537),
(#67538,#67539),(#67540,#67541),(#67542,#67543),(#67544,#67545),(#67546,
#67547),(#67548,#67549),(#67550,#67551),(#67552,#67553),(#67554,#67555),
(#67556,#67557),(#67558,#67559),(#67560,#67561),(#67562,#67563),(#67564,
#67565),(#67566,#67567),(#67568,#67569),(#67570,#67571),(#67572,#67573),
(#67574,#67575),(#67576,#67577),(#67578,#67579),(#67580,#67581),(#67582,
#67583),(#67584,#67585),(#67586,#67587),(#67588,#67589),(#67590,#67591),
(#67592,#67593),(#67594,#67595),(#67596,#67597),(#67598,#67599),(#67600,
#67601),(#67602,#67603),(#67604,#67605),(#67606,#67607),(#67608,#67609),
(#67610,#67611),(#67612,#67613),(#67614,#67615),(#67616,#67617),(#67618,
#67619),(#67620,#67621),(#67622,#67623),(#67624,#67625),(#67626,#67627),
(#67628,#67629),(#67630,#67631),(#67632,#67633),(#67634,#67635),(#67636,
#67637),(#67638,#67639),(#67640,#67641),(#67642,#67643),(#67644,#67645),
(#67646,#67647),(#67648,#67649),(#67650,#67651),(#67652,#67653),(#67654,
#67655),(#67656,#67657),(#67658,#67659),(#67660,#67661),(#67662,#67663),
(#67664,#67665),(#67666,#67667),(#67668,#67669),(#67670,#67671),(#67672,
#67673),(#67674,#67675),(#67676,#67677),(#67678,#67679),(#67680,#67681),
(#67682,#67683),(#67684,#67685),(#67686,#67687),(#67688,#67689),(#67690,
#67691),(#67692,#67693),(#67694,#67695),(#67696,#67697),(#67698,#67699),
(#67700,#67701),(#67702,#67703),(#67704,#67705),(#67706,#67707),(#67708,
#67709),(#67710,#67711),(#67712,#67713),(#67714,#67715),(#67716,#67717),
(#67718,#67719),(#67720,#67721),(#67722,#67723),(#67724,#67725),(#67726,
#67727),(#67728,#67729),(#67730,#67731),(#67732,#67733),(#67734,#67735),
(#67736,#67737),(#67738,#67739),(#67740,#67741),(#67742,#67743),(#67744,
#67745),(#67746,#67747),(#67748,#67749),(#67750,#67751),(#67752,#67753),
(#67754,#67755),(#67756,#67757),(#67758,#67759),(#67760,#67761),(#67762,
#67763),(#67764,#67765),(#67766,#67767),(#67768,#67769),(#67770,#67771),
(#67772,#67773),(#67774,#67775),(#67776,#67777),(#67778,#67779),(#67780,
#67781),(#67782,#67783),(#67784,#67785),(#67786,#67787),(#67788,#67789),
(#67790,#67791),(#67792,#67793),(#67794,#67795),(#67796,#67797),(#67798,
#67799),(#67800,#67801),(#67802,#67803),(#67804,#67805),(#67806,#67807),
(#67808,#67809),(#67810,#67811),(#67812,#67813),(#67814,#67815),(#67816,
#67817),(#67818,#67819),(#67820,#67821),(#67822,#67823),(#67824,#67825),
(#67826,#67827),(#67828,#67829),(#67830,#67831),(#67832,#67833),(#67834,
#67835),(#67836,#67837),(#67838,#67839),(#67840,#67841),(#67842,#67843),
(#67844,#67845),(#67846,#67847),(#67848,#67849),(#67850,#67851),(#67852,
#67853),(#67854,#67855),(#67856,#67857),(#67858,#67859),(#67860,#67861),
(#67862,#67863),(#67864,#67865),(#67866,#67867),(#67868,#67869),(#67870,
#67871),(#67872,#67873),(#67874,#67875),(#67876,#67877),(#67878,#67879),
(#67880,#67881),(#67882,#67883),(#67884,#67885),(#67886,#67887),(#67888,
#67889),(#67890,#67891),(#67892,#67893),(#67894,#67895),(#67896,#67897),
(#67898,#67899),(#67900,#67901),(#67902,#67903),(#67904,#67905),(#67906,
#67907),(#67908,#67909),(#67910,#67911),(#67912,#67913),(#67914,#67915),
(#67916,#67917),(#67918,#67919),(#67920,#67921),(#67922,#67923),(#67924,
#67925),(#67926,#67927),(#67928,#67929),(#67930,#67931),(#67932,#67933),
(#67934,#67935),(#67936,#67937),(#67938,#67939),(#67940,#67941),(#67942,
#67943),(#67944,#67945),(#67946,#67947),(#67948,#67949),(#67950,#67951),
(#67952,#67953),(#67954,#67955),(#67956,#67957),(#67958,#67959),(#67960,
#67961),(#67962,#67963),(#67964,#67965),(#67966,#67967),(#67968,#67969),
(#67970,#67971),(#67972,#67973),(#67974,#67975),(#67976,#67977),(#67978,
#67979),(#67980,#67981),(#67982,#67983),(#67984,#67985),(#67986,#67987),
(#67988,#67989),(#67990,#67991),(#67992,#67993),(#67994,#67995),(#67996,
#67997),(#67998,#67999),(#68000,#68001),(#68002,#68003),(#68004,#68005),
(#68006,#68007),(#68008,#68009),(#68010,#68011),(#68012,#68013),(#68014,
#68015),(#68016,#68017),(#68018,#68019),(#68020,#68021),(#68022,#68023),
(#68024,#68025),(#68026,#68027),(#68028,#68029),(#68030,#68031),(#68032,
#68033),(#68034,#68035),(#68036,#68037),(#68038,#68039),(#68040,#68041),
(#68042,#68043),(#68044,#68045),(#68046,#68047),(#68048,#68049),(#68050,
#68051),(#68052,#68053),(#68054,#68055),(#68056,#68057),(#68058,#68059),
(#68060,#68061),(#68062,#68063),(#68064,#68065),(#68066,#68067),(#68068,
#68069),(#68070,#68071),(#68072,#68073),(#68074,#68075),(#68076,#68077),
(#68078,#68079),(#68080,#68081),(#68082,#68083),(#68084,#68085),(#68086,
#68087),(#68088,#68089),(#68090,#68091),(#68092,#68093),(#68094,#68095),
(#68096,#68097),(#68098,#68099),(#68100,#68101),(#68102,#68103),(#68104,
#68105),(#68106,#68107),(#68108,#68109),(#68110,#68111),(#68112,#68113),
(#68114,#68115),(#68116,#68117),(#68118,#68119),(#68120,#68121),(#68122,
#68123),(#68124,#68125),(#68126,#68127),(#68128,#68129),(#68130,#68131),
(#68132,#68133),(#68134,#68135),(#68136,#68137),(#68138,#68139),(#68140,
#68141),(#68142,#68143),(#68144,#68145),(#68146,#68147),(#68148,#68149),
(#68150,#68151),(#68152,#68153),(#68154,#68155),(#68156,#68157),(#68158,
#68159),(#68160,#68161),(#68162,#68163),(#68164,#68165),(#68166,#68167),
(#68168,#68169),(#68170,#68171),(#68172,#68173),(#68174,#68175),(#68176,
#68177),(#68178,#68179),(#68180,#68181),(#68182,#68183),(#68184,#68185),
(#68186,#68187),(#68188,#68189),(#68190,#68191),(#68192,#68193),(#68194,
#68195),(#68196,#68197),(#68198,#68199),(#68200,#68201),(#68202,#68203),
(#68204,#68205),(#68206,#68207),(#68208,#68209),(#68210,#68211),(#68212,
#68213),(#68214,#68215),(#68216,#68217),(#68218,#68219),(#68220,#68221),
(#68222,#68223),(#68224,#68225),(#68226,#68227),(#68228,#68229),(#68230,
#68231),(#68232,#68233),(#68234,#68235),(#68236,#68237),(#68238,#68239),
(#68240,#68241),(#68242,#68243),(#68244,#68245),(#68246,#68247),(#68248,
#68249),(#68250,#68251),(#68252,#68253),(#68254,#68255),(#68256,#68257),
(#68258,#68259),(#68260,#68261),(#68262,#68263),(#68264,#68265),(#68266,
#68267),(#68268,#68269),(#68270,#68271),(#68272,#68273),(#68274,#68275),
(#68276,#68277),(#68278,#68279),(#68280,#68281),(#68282,#68283),(#68284,
#68285),(#68286,#68287),(#68288,#68289),(#68290,#68291),(#68292,#68293),
(#68294,#68295),(#68296,#68297),(#68298,#68299),(#68300,#68301),(#68302,
#68303),(#68304,#68305),(#68306,#68307),(#68308,#68309),(#68310,#68311),
(#68312,#68313),(#68314,#68315),(#68316,#68317),(#68318,#68319),(#68320,
#68321),(#68322,#68323),(#68324,#68325),(#68326,#68327),(#68328,#68329),
(#68330,#68331),(#68332,#68333),(#68334,#68335),(#68336,#68337),(#68338,
#68339),(#68340,#68341),(#68342,#68343),(#68344,#68345),(#68346,#68347),
(#68348,#68349),(#68350,#68351),(#68352,#68353),(#68354,#68355),(#68356,
#68357),(#68358,#68359),(#68360,#68361),(#68362,#68363),(#68364,#68365),
(#68366,#68367),(#68368,#68369),(#68370,#68371),(#68372,#68373),(#68374,
#68375),(#68376,#68377),(#68378,#68379),(#68380,#68381),(#68382,#68383),
(#68384,#68385),(#68386,#68387),(#68388,#68389),(#68390,#68391),(#68392,
#68393),(#68394,#68395),(#68396,#68397),(#68398,#68399),(#68400,#68401),
(#68402,#68403),(#68404,#68405),(#68406,#68407),(#68408,#68409),(#68410,
#68411),(#68412,#68413),(#68414,#68415),(#68416,#68417),(#68418,#68419),
(#68420,#68421),(#68422,#68423),(#68424,#68425),(#68426,#68427),(#68428,
#68429),(#68430,#68431),(#68432,#68433),(#68434,#68435),(#68436,#68437),
(#68438,#68439),(#68440,#68441),(#68442,#68443),(#68444,#68445),(#68446,
#68447),(#68448,#68449),(#68450,#68451),(#68452,#68453),(#68454,#68455),
(#68456,#68457),(#68458,#68459),(#68460,#68461),(#68462,#68463),(#68464,
#68465),(#68466,#68467),(#68468,#68469),(#68470,#68471),(#68472,#68473),
(#68474,#68475),(#68476,#68477),(#68478,#68479),(#68480,#68481),(#68482,
#68483),(#68484,#68485),(#68486,#68487),(#68488,#68489),(#68490,#68491),
(#68492,#68493),(#68494,#68495),(#68496,#68497),(#68498,#68499),(#68500,
#68501),(#68502,#68503),(#68504,#68505),(#68506,#68507),(#68508,#68509),
(#68510,#68511),(#68512,#68513),(#68514,#68515),(#68516,#68517),(#68518,
#68519),(#68520,#68521),(#68522,#68523),(#68524,#68525),(#68526,#68527),
(#68528,#68529),(#68530,#68531),(#68532,#68533),(#68534,#68535),(#68536,
#68537),(#68538,#68539),(#68540,#68541),(#68542,#68543),(#68544,#68545),
(#68546,#68547),(#68548,#68549),(#68550,#68551),(#68552,#68553),(#68554,
#68555),(#68556,#68557),(#68558,#68559),(#68560,#68561),(#68562,#68563),
(#68564,#68565),(#68566,#68567),(#68568,#68569),(#68570,#68571),(#68572,
#68573),(#68574,#68575),(#68576,#68577),(#68578,#68579),(#68580,#68581),
(#68582,#68583),(#68584,#68585),(#68586,#68587),(#68588,#68589),(#68590,
#68591),(#68592,#68593),(#68594,#68595),(#68596,#68597),(#68598,#68599),
(#68600,#68601),(#68602,#68603),(#68604,#68605),(#68606,#68607),(#68608,
#68609),(#68610,#68611),(#68612,#68613),(#68614,#68615),(#68616,#68617),
(#68618,#68619),(#68620,#68621),(#68622,#68623),(#68624,#68625),(#68626,
#68627),(#68628,#68629),(#68630,#68631),(#68632,#68633),(#68634,#68635),
(#68636,#68637),(#68638,#68639),(#68640,#68641),(#68642,#68643),(#68644,
#68645),(#68646,#68647),(#68648,#68649),(#68650,#68651),(#68652,#68653),
(#68654,#68655),(#68656,#68657),(#68658,#68659),(#68660,#68661),(#68662,
#68663),(#68664,#68665),(#68666,#68667),(#68668,#68669),(#68670,#68671),
(#68672,#68673),(#68674,#68675),(#68676,#68677),(#68678,#68679),(#68680,
#68681),(#68682,#68683),(#68684,#68685),(#68686,#68687),(#68688,#68689),
(#68690,#68691),(#68692,#68693),(#68694,#68695),(#68696,#68697),(#68698,
#68699),(#68700,#68701),(#68702,#68703),(#68704,#68705),(#68706,#68707),
(#68708,#68709),(#68710,#68711),(#68712,#68713),(#68714,#68715),(#68716,
#68717),(#68718,#68719),(#68720,#68721),(#68722,#68723),(#68724,#68725),
(#68726,#68727),(#68728,#68729),(#68730,#68731),(#68732,#68733),(#68734,
#68735),(#68736,#68737),(#68738,#68739),(#68740,#68741),(#68742,#68743),
(#68744,#68745),(#68746,#68747),(#68748,#68749),(#68750,#68751),(#68752,
#68753),(#68754,#68755),(#68756,#68757),(#68758,#68759),(#68760,#68761),
(#68762,#68763),(#68764,#68765),(#68766,#68767),(#68768,#68769),(#68770,
#68771),(#68772,#68773),(#68774,#68775),(#68776,#68777),(#68778,#68779),
(#68780,#68781),(#68782,#68783),(#68784,#68785),(#68786,#68787),(#68788,
#68789),(#68790,#68791),(#68792,#68793),(#68794,#68795),(#68796,#68797),
(#68798,#68799),(#68800,#68801),(#68802,#68803),(#68804,#68805),(#68806,
#68807),(#68808,#68809),(#68810,#68811),(#68812,#68813),(#68814,#68815),
(#68816,#68817),(#68818,#68819),(#68820,#68821),(#68822,#68823),(#68824,
#68825),(#68826,#68827),(#68828,#68829),(#68830,#68831),(#68832,#68833),
(#68834,#68835),(#68836,#68837),(#68838,#68839),(#68840,#68841),(#68842,
#68843),(#68844,#68845),(#68846,#68847),(#68848,#68849),(#68850,#68851),
(#68852,#68853),(#68854,#68855),(#68856,#68857),(#68858,#68859),(#68860,
#68861),(#68862,#68863),(#68864,#68865),(#68866,#68867),(#68868,#68869),
(#68870,#68871),(#68872,#68873),(#68874,#68875),(#68876,#68877),(#68878,
#68879),(#68880,#68881),(#68882,#68883),(#68884,#68885),(#68886,#68887),
(#68888,#68889),(#68890,#68891),(#68892,#68893),(#68894,#68895),(#68896,
#68897),(#68898,#68899),(#68900,#68901),(#68902,#68903),(#68904,#68905),
(#68906,#68907),(#68908,#68909),(#68910,#68911),(#68912,#68913),(#68914,
#68915),(#68916,#68917),(#68918,#68919),(#68920,#68921),(#68922,#68923),
(#68924,#68925),(#68926,#68927),(#68928,#68929),(#68930,#68931),(#68932,
#68933),(#68934,#68935),(#68936,#68937),(#68938,#68939),(#68940,#68941),
(#68942,#68943),(#68944,#68945),(#68946,#68947),(#68948,#68949),(#68950,
#68951),(#68952,#68953),(#68954,#68955),(#68956,#68957),(#68958,#68959),
(#68960,#68961),(#68962,#68963),(#68964,#68965),(#68966,#68967),(#68968,
#68969),(#68970,#68971),(#68972,#68973),(#68974,#68975),(#68976,#68977),
(#68978,#68979),(#68980,#68981),(#68982,#68983),(#68984,#68985),(#68986,
#68987),(#68988,#68989),(#68990,#68991),(#68992,#68993),(#68994,#68995),
(#68996,#68997),(#68998,#68999),(#69000,#69001),(#69002,#69003),(#69004,
#69005),(#69006,#69007),(#69008,#69009),(#69010,#69011),(#69012,#69013),
(#69014,#69015),(#69016,#69017),(#69018,#69019),(#69020,#69021),(#69022,
#69023),(#69024,#69025),(#69026,#69027),(#69028,#69029),(#69030,#69031),
(#69032,#69033),(#69034,#69035),(#69036,#69037),(#69038,#69039),(#69040,
#69041),(#69042,#69043),(#69044,#69045),(#69046,#69047),(#69048,#69049),
(#69050,#69051),(#69052,#69053),(#69054,#69055),(#69056,#69057),(#69058,
#69059),(#69060,#69061),(#69062,#69063),(#69064,#69065),(#69066,#69067),
(#69068,#69069),(#69070,#69071),(#69072,#69073),(#69074,#69075),(#69076,
#69077),(#69078,#69079),(#69080,#69081),(#69082,#69083),(#69084,#69085),
(#69086,#69087),(#69088,#69089),(#69090,#69091),(#69092,#69093),(#69094,
#69095),(#69096,#69097),(#69098,#69099),(#69100,#69101),(#69102,#69103),
(#69104,#69105),(#69106,#69107),(#69108,#69109),(#69110,#69111),(#69112,
#69113),(#69114,#69115),(#69116,#69117),(#69118,#69119),(#69120,#69121),
(#69122,#69123),(#69124,#69125),(#69126,#69127),(#69128,#69129),(#69130,
#69131),(#69132,#69133),(#69134,#69135),(#69136,#69137),(#69138,#69139),
(#69140,#69141),(#69142,#69143),(#69144,#69145),(#69146,#69147),(#69148,
#69149),(#69150,#69151),(#69152,#69153),(#69154,#69155),(#69156,#69157),
(#69158,#69159),(#69160,#69161),(#69162,#69163),(#69164,#69165),(#69166,
#69167),(#69168,#69169),(#69170,#69171),(#69172,#69173),(#69174,#69175),
(#69176,#69177),(#69178,#69179),(#69180,#69181),(#69182,#69183),(#69184,
#69185),(#69186,#69187),(#69188,#69189),(#69190,#69191),(#69192,#69193),
(#69194,#69195),(#69196,#69197),(#69198,#69199),(#69200,#69201),(#69202,
#69203),(#69204,#69205),(#69206,#69207),(#69208,#69209),(#69210,#69211),
(#69212,#69213),(#69214,#69215),(#69216,#69217),(#69218,#69219),(#69220,
#69221),(#69222,#69223),(#69224,#69225),(#69226,#69227),(#69228,#69229),
(#69230,#69231),(#69232,#69233),(#69234,#69235),(#69236,#69237),(#69238,
#69239),(#69240,#69241),(#69242,#69243),(#69244,#69245),(#69246,#69247),
(#69248,#69249),(#69250,#69251),(#69252,#69253),(#69254,#69255),(#69256,
#69257),(#69258,#69259),(#69260,#69261),(#69262,#69263),(#69264,#69265),
(#69266,#69267),(#69268,#69269),(#69270,#69271),(#69272,#69273),(#69274,
#69275),(#69276,#69277),(#69278,#69279),(#69280,#69281),(#69282,#69283),
(#69284,#69285),(#69286,#69287),(#69288,#69289),(#69290,#69291),(#69292,
#69293),(#69294,#69295),(#69296,#69297),(#69298,#69299),(#69300,#69301),
(#69302,#69303),(#69304,#69305),(#69306,#69307),(#69308,#69309),(#69310,
#69311),(#69312,#69313),(#69314,#69315),(#69316,#69317),(#69318,#69319),
(#69320,#69321),(#69322,#69323),(#69324,#69325),(#69326,#69327),(#69328,
#69329),(#69330,#69331),(#69332,#69333),(#69334,#69335),(#69336,#69337),
(#69338,#69339),(#69340,#69341),(#69342,#69343),(#69344,#69345),(#69346,
#69347),(#69348,#69349),(#69350,#69351),(#69352,#69353),(#69354,#69355),
(#69356,#69357),(#69358,#69359),(#69360,#69361),(#69362,#69363),(#69364,
#69365),(#69366,#69367),(#69368,#69369),(#69370,#69371),(#69372,#69373),
(#69374,#69375),(#69376,#69377),(#69378,#69379),(#69380,#69381),(#69382,
#69383),(#69384,#69385),(#69386,#69387),(#69388,#69389),(#69390,#69391),
(#69392,#69393),(#69394,#69395),(#69396,#69397),(#69398,#69399),(#69400,
#69401),(#69402,#69403),(#69404,#69405),(#69406,#69407),(#69408,#69409),
(#69410,#69411),(#69412,#69413),(#69414,#69415),(#69416,#69417),(#69418,
#69419),(#69420,#69421),(#69422,#69423),(#69424,#69425),(#69426,#69427),
(#69428,#69429),(#69430,#69431),(#69432,#69433),(#69434,#69435),(#69436,
#69437),(#69438,#69439),(#69440,#69441),(#69442,#69443),(#69444,#69445),
(#69446,#69447),(#69448,#69449),(#69450,#69451),(#69452,#69453),(#69454,
#69455),(#69456,#69457),(#69458,#69459),(#69460,#69461),(#69462,#69463),
(#69464,#69465),(#69466,#69467),(#69468,#69469),(#69470,#69471),(#69472,
#69473),(#69474,#69475),(#69476,#69477),(#69478,#69479),(#69480,#69481),
(#69482,#69483),(#69484,#69485),(#69486,#69487),(#69488,#69489),(#69490,
#69491),(#69492,#69493),(#69494,#69495),(#69496,#69497),(#69498,#69499),
(#69500,#69501),(#69502,#69503),(#69504,#69505),(#69506,#69507),(#69508,
#69509),(#69510,#69511),(#69512,#69513),(#69514,#69515),(#69516,#69517),
(#69518,#69519),(#69520,#69521),(#69522,#69523),(#69524,#69525),(#69526,
#69527),(#69528,#69529),(#69530,#69531),(#69532,#69533),(#69534,#69535),
(#69536,#69537),(#69538,#69539),(#69540,#69541),(#69542,#69543),(#69544,
#69545),(#69546,#69547),(#69548,#69549),(#69550,#69551),(#69552,#69553),
(#69554,#69555),(#69556,#69557),(#69558,#69559),(#69560,#69561),(#69562,
#69563),(#69564,#69565),(#69566,#69567),(#69568,#69569),(#69570,#69571),
(#69572,#69573),(#69574,#69575),(#69576,#69577),(#69578,#69579),(#69580,
#69581),(#69582,#69583),(#69584,#69585),(#69586,#69587),(#69588,#69589),
(#69590,#69591),(#69592,#69593),(#69594,#69595),(#69596,#69597),(#69598,
#69599),(#69600,#69601),(#69602,#69603),(#69604,#69605),(#69606,#69607),
(#69608,#69609),(#69610,#69611),(#69612,#69613),(#69614,#69615),(#69616,
#69617),(#69618,#69619),(#69620,#69621),(#69622,#69623),(#69624,#69625),
(#69626,#69627),(#69628,#69629),(#69630,#69631),(#69632,#69633),(#69634,
#69635),(#69636,#69637),(#69638,#69639),(#69640,#69641),(#69642,#69643),
(#69644,#69645),(#69646,#69647),(#69648,#69649),(#69650,#69651),(#69652,
#69653),(#69654,#69655),(#69656,#69657),(#69658,#69659),(#69660,#69661),
(#69662,#69663),(#69664,#69665),(#69666,#69667),(#69668,#69669),(#69670,
#69671),(#69672,#69673),(#69674,#69675),(#69676,#69677),(#69678,#69679),
(#69680,#69681),(#69682,#69683),(#69684,#69685),(#69686,#69687),(#69688,
#69689),(#69690,#69691),(#69692,#69693),(#69694,#69695),(#69696,#69697),
(#69698,#69699),(#69700,#69701),(#69702,#69703),(#69704,#69705),(#69706,
#69707),(#69708,#69709),(#69710,#69711),(#69712,#69713),(#69714,#69715),
(#69716,#69717),(#69718,#69719),(#69720,#69721),(#69722,#69723),(#69724,
#69725),(#69726,#69727),(#69728,#69729),(#69730,#69731),(#69732,#69733),
(#69734,#69735),(#69736,#69737),(#69738,#69739),(#69740,#69741),(#69742,
#69743),(#69744,#69745),(#69746,#69747),(#69748,#69749),(#69750,#69751),
(#69752,#69753),(#69754,#69755),(#69756,#69757),(#69758,#69759),(#69760,
#69761),(#69762,#69763),(#69764,#69765),(#69766,#69767),(#69768,#69769),
(#69770,#69771),(#69772,#69773),(#69774,#69775),(#69776,#69777),(#69778,
#69779),(#69780,#69781),(#69782,#69783),(#69784,#69785),(#69786,#69787),
(#69788,#69789),(#69790,#69791),(#69792,#69793),(#69794,#69795),(#69796,
#69797),(#69798,#69799),(#69800,#69801),(#69802,#69803),(#69804,#69805),
(#69806,#69807),(#69808,#69809),(#69810,#69811),(#69812,#69813),(#69814,
#69815),(#69816,#69817),(#69818,#69819),(#69820,#69821),(#69822,#69823),
(#69824,#69825),(#69826,#69827),(#69828,#69829),(#69830,#69831),(#69832,
#69833),(#69834,#69835),(#69836,#69837),(#69838,#69839),(#69840,#69841),
(#69842,#69843),(#69844,#69845),(#69846,#69847),(#69848,#69849),(#69850,
#69851),(#69852,#69853),(#69854,#69855),(#69856,#69857),(#69858,#69859),
(#69860,#69861),(#69862,#69863),(#69864,#69865),(#69866,#69867),(#69868,
#69869),(#69870,#69871),(#69872,#69873),(#69874,#69875),(#69876,#69877),
(#69878,#69879),(#69880,#69881),(#69882,#69883),(#69884,#69885),(#69886,
#69887),(#69888,#69889),(#69890,#69891),(#69892,#69893),(#69894,#69895),
(#69896,#69897),(#69898,#69899),(#69900,#69901),(#69902,#69903),(#69904,
#69905),(#69906,#69907),(#69908,#69909),(#69910,#69911),(#69912,#69913),
(#69914,#69915),(#69916,#69917),(#69918,#69919),(#69920,#69921),(#69922,
#69923),(#69924,#69925),(#69926,#69927),(#69928,#69929),(#69930,#69931),
(#69932,#69933),(#69934,#69935),(#69936,#69937),(#69938,#69939),(#69940,
#69941),(#69942,#69943),(#69944,#69945),(#69946,#69947),(#69948,#69949),
(#69950,#69951),(#69952,#69953),(#69954,#69955),(#69956,#69957),(#69958,
#69959),(#69960,#69961),(#69962,#69963),(#69964,#69965),(#69966,#69967),
(#69968,#69969),(#69970,#69971),(#69972,#69973),(#69974,#69975),(#69976,
#69977),(#69978,#69979),(#69980,#69981),(#69982,#69983),(#69984,#69985),
(#69986,#69987),(#69988,#69989),(#69990,#69991),(#69992,#69993),(#69994,
#69995),(#69996,#69997),(#69998,#69999),(#70000,#70001),(#70002,#70003),
(#70004,#70005),(#70006,#70007),(#70008,#70009),(#70010,#70011),(#70012,
#70013),(#70014,#70015),(#70016,#70017),(#70018,#70019),(#70020,#70021),
(#70022,#70023),(#70024,#70025),(#70026,#70027),(#70028,#70029),(#70030,
#70031),(#70032,#70033),(#70034,#70035),(#70036,#70037),(#70038,#70039),
(#70040,#70041),(#70042,#70043),(#70044,#70045),(#70046,#70047),(#70048,
#70049),(#70050,#70051),(#70052,#70053),(#70054,#70055),(#70056,#70057),
(#70058,#70059),(#70060,#70061),(#70062,#70063),(#70064,#70065),(#70066,
#70067),(#70068,#70069),(#70070,#70071),(#70072,#70073),(#70074,#70075),
(#70076,#70077),(#70078,#70079),(#70080,#70081),(#70082,#70083),(#70084,
#70085),(#70086,#70087),(#70088,#70089),(#70090,#70091),(#70092,#70093),
(#70094,#70095),(#70096,#70097),(#70098,#70099),(#70100,#70101),(#70102,
#70103),(#70104,#70105),(#70106,#70107),(#70108,#70109),(#70110,#70111),
(#70112,#70113),(#70114,#70115),(#70116,#70117),(#70118,#70119),(#70120,
#70121),(#70122,#70123),(#70124,#70125),(#70126,#70127),(#70128,#70129),
(#70130,#70131),(#70132,#70133),(#70134,#70135),(#70136,#70137),(#70138,
#70139),(#70140,#70141),(#70142,#70143),(#70144,#70145),(#70146,#70147),
(#70148,#70149),(#70150,#70151),(#70152,#70153),(#70154,#70155),(#70156,
#70157),(#70158,#70159),(#70160,#70161),(#70162,#70163),(#70164,#70165),
(#70166,#70167),(#70168,#70169),(#70170,#70171),(#70172,#70173),(#70174,
#70175),(#70176,#70177),(#70178,#70179),(#70180,#70181),(#70182,#70183),
(#70184,#70185),(#70186,#70187),(#70188,#70189),(#70190,#70191),(#70192,
#70193),(#70194,#70195),(#70196,#70197),(#70198,#70199),(#70200,#70201),
(#70202,#70203),(#70204,#70205),(#70206,#70207),(#70208,#70209),(#70210,
#70211),(#70212,#70213),(#70214,#70215),(#70216,#70217),(#70218,#70219),
(#70220,#70221),(#70222,#70223),(#70224,#70225),(#70226,#70227),(#70228,
#70229),(#70230,#70231),(#70232,#70233),(#70234,#70235),(#70236,#70237),
(#70238,#70239),(#70240,#70241),(#70242,#70243),(#70244,#70245),(#70246,
#70247),(#70248,#70249),(#70250,#70251),(#70252,#70253),(#70254,#70255),
(#70256,#70257),(#70258,#70259),(#70260,#70261),(#70262,#70263),(#70264,
#70265),(#70266,#70267),(#70268,#70269),(#70270,#70271),(#70272,#70273),
(#70274,#70275),(#70276,#70277),(#70278,#70279),(#70280,#70281),(#70282,
#70283),(#70284,#70285),(#70286,#70287),(#70288,#70289),(#70290,#70291),
(#70292,#70293),(#70294,#70295),(#70296,#70297),(#70298,#70299),(#70300,
#70301),(#70302,#70303),(#70304,#70305),(#70306,#70307),(#70308,#70309),
(#70310,#70311),(#70312,#70313),(#70314,#70315),(#70316,#70317),(#70318,
#70319),(#70320,#70321),(#70322,#70323),(#70324,#70325),(#70326,#70327),
(#70328,#70329),(#70330,#70331),(#70332,#70333),(#70334,#70335),(#70336,
#70337),(#70338,#70339),(#70340,#70341),(#70342,#70343),(#70344,#70345),
(#70346,#70347),(#70348,#70349),(#70350,#70351),(#70352,#70353),(#70354,
#70355),(#70356,#70357),(#70358,#70359),(#70360,#70361),(#70362,#70363),
(#70364,#70365),(#70366,#70367),(#70368,#70369),(#70370,#70371),(#70372,
#70373),(#70374,#70375),(#70376,#70377),(#70378,#70379),(#70380,#70381),
(#70382,#70383),(#70384,#70385),(#70386,#70387),(#70388,#70389),(#70390,
#70391),(#70392,#70393),(#70394,#70395),(#70396,#70397),(#70398,#70399),
(#70400,#70401),(#70402,#70403),(#70404,#70405),(#70406,#70407),(#70408,
#70409),(#70410,#70411),(#70412,#70413),(#70414,#70415),(#70416,#70417),
(#70418,#70419),(#70420,#70421),(#70422,#70423),(#70424,#70425),(#70426,
#70427),(#70428,#70429),(#70430,#70431),(#70432,#70433),(#70434,#70435),
(#70436,#70437),(#70438,#70439),(#70440,#70441),(#70442,#70443),(#70444,
#70445),(#70446,#70447),(#70448,#70449),(#70450,#70451),(#70452,#70453),
(#70454,#70455),(#70456,#70457),(#70458,#70459),(#70460,#70461),(#70462,
#70463),(#70464,#70465),(#70466,#70467),(#70468,#70469),(#70470,#70471),
(#70472,#70473),(#70474,#70475),(#70476,#70477),(#70478,#70479),(#70480,
#70481),(#70482,#70483),(#70484,#70485),(#70486,#70487),(#70488,#70489),
(#70490,#70491),(#70492,#70493),(#70494,#70495),(#70496,#70497),(#70498,
#70499),(#70500,#70501),(#70502,#70503),(#70504,#70505),(#70506,#70507),
(#70508,#70509),(#70510,#70511),(#70512,#70513),(#70514,#70515),(#70516,
#70517),(#70518,#70519),(#70520,#70521),(#70522,#70523),(#70524,#70525),
(#70526,#70527),(#70528,#70529),(#70530,#70531),(#70532,#70533),(#70534,
#70535),(#70536,#70537),(#70538,#70539),(#70540,#70541),(#70542,#70543),
(#70544,#70545),(#70546,#70547),(#70548,#70549),(#70550,#70551),(#70552,
#70553),(#70554,#70555),(#70556,#70557),(#70558,#70559),(#70560,#70561),
(#70562,#70563),(#70564,#70565),(#70566,#70567),(#70568,#70569),(#70570,
#70571),(#70572,#70573),(#70574,#70575),(#70576,#70577),(#70578,#70579),
(#70580,#70581),(#70582,#70583),(#70584,#70585),(#70586,#70587),(#70588,
#70589),(#70590,#70591),(#70592,#70593),(#70594,#70595),(#70596,#70597),
(#70598,#70599),(#70600,#70601),(#70602,#70603),(#70604,#70605),(#70606,
#70607),(#70608,#70609),(#70610,#70611),(#70612,#70613),(#70614,#70615),
(#70616,#70617),(#70618,#70619),(#70620,#70621),(#70622,#70623),(#70624,
#70625),(#70626,#70627),(#70628,#70629),(#70630,#70631),(#70632,#70633),
(#70634,#70635),(#70636,#70637),(#70638,#70639),(#70640,#70641),(#70642,
#70643),(#70644,#70645),(#70646,#70647),(#70648,#70649),(#70650,#70651),
(#70652,#70653),(#70654,#70655),(#70656,#70657),(#70658,#70659),(#70660,
#70661),(#70662,#70663),(#70664,#70665),(#70666,#70667),(#70668,#70669),
(#70670,#70671),(#70672,#70673),(#70674,#70675),(#70676,#70677),(#70678,
#70679),(#70680,#70681),(#70682,#70683),(#70684,#70685),(#70686,#70687),
(#70688,#70689),(#70690,#70691),(#70692,#70693),(#70694,#70695),(#70696,
#70697),(#70698,#70699),(#70700,#70701),(#70702,#70703),(#70704,#70705),
(#70706,#70707),(#70708,#70709),(#70710,#70711),(#70712,#70713),(#70714,
#70715),(#70716,#70717),(#70718,#70719),(#70720,#70721),(#70722,#70723),
(#70724,#70725),(#70726,#70727),(#70728,#70729),(#70730,#70731),(#70732,
#70733),(#70734,#70735),(#70736,#70737),(#70738,#70739),(#70740,#70741),
(#70742,#70743),(#70744,#70745),(#70746,#70747),(#70748,#70749),(#70750,
#70751),(#70752,#70753),(#70754,#70755),(#70756,#70757),(#70758,#70759),
(#70760,#70761),(#70762,#70763),(#70764,#70765),(#70766,#70767),(#70768,
#70769),(#70770,#70771),(#70772,#70773),(#70774,#70775),(#70776,#70777),
(#70778,#70779),(#70780,#70781),(#70782,#70783),(#70784,#70785),(#70786,
#70787),(#70788,#70789),(#70790,#70791),(#70792,#70793),(#70794,#70795),
(#70796,#70797),(#70798,#70799),(#70800,#70801),(#70802,#70803),(#70804,
#70805),(#70806,#70807),(#70808,#70809),(#70810,#70811),(#70812,#70813),
(#70814,#70815),(#70816,#70817),(#70818,#70819),(#70820,#70821),(#70822,
#70823),(#70824,#70825),(#70826,#70827),(#70828,#70829),(#70830,#70831),
(#70832,#70833),(#70834,#70835),(#70836,#70837),(#70838,#70839),(#70840,
#70841),(#70842,#70843),(#70844,#70845),(#70846,#70847),(#70848,#70849),
(#70850,#70851),(#70852,#70853),(#70854,#70855),(#70856,#70857),(#70858,
#70859),(#70860,#70861),(#70862,#70863),(#70864,#70865),(#70866,#70867),
(#70868,#70869),(#70870,#70871),(#70872,#70873),(#70874,#70875),(#70876,
#70877),(#70878,#70879),(#70880,#70881),(#70882,#70883),(#70884,#70885),
(#70886,#70887),(#70888,#70889),(#70890,#70891),(#70892,#70893),(#70894,
#70895),(#70896,#70897),(#70898,#70899),(#70900,#70901),(#70902,#70903),
(#70904,#70905),(#70906,#70907),(#70908,#70909),(#70910,#70911),(#70912,
#70913),(#70914,#70915),(#70916,#70917),(#70918,#70919),(#70920,#70921),
(#70922,#70923),(#70924,#70925),(#70926,#70927),(#70928,#70929),(#70930,
#70931),(#70932,#70933),(#70934,#70935),(#70936,#70937),(#70938,#70939),
(#70940,#70941),(#70942,#70943),(#70944,#70945),(#70946,#70947),(#70948,
#70949),(#70950,#70951),(#70952,#70953),(#70954,#70955),(#70956,#70957),
(#70958,#70959),(#70960,#70961),(#70962,#70963),(#70964,#70965),(#70966,
#70967),(#70968,#70969),(#70970,#70971),(#70972,#70973),(#70974,#70975),
(#70976,#70977),(#70978,#70979),(#70980,#70981),(#70982,#70983),(#70984,
#70985),(#70986,#70987),(#70988,#70989),(#70990,#70991),(#70992,#70993),
(#70994,#70995),(#70996,#70997),(#70998,#70999),(#71000,#71001),(#71002,
#71003),(#71004,#71005),(#71006,#71007),(#71008,#71009),(#71010,#71011),
(#71012,#71013),(#71014,#71015),(#71016,#71017),(#71018,#71019),(#71020,
#71021),(#71022,#71023),(#71024,#71025),(#71026,#71027),(#71028,#71029),
(#71030,#71031),(#71032,#71033),(#71034,#71035),(#71036,#71037),(#71038,
#71039),(#71040,#71041),(#71042,#71043),(#71044,#71045),(#71046,#71047),
(#71048,#71049),(#71050,#71051),(#71052,#71053),(#71054,#71055),(#71056,
#71057),(#71058,#71059),(#71060,#71061),(#71062,#71063),(#71064,#71065),
(#71066,#71067),(#71068,#71069),(#71070,#71071),(#71072,#71073),(#71074,
#71075),(#71076,#71077),(#71078,#71079),(#71080,#71081),(#71082,#71083),
(#71084,#71085),(#71086,#71087),(#71088,#71089),(#71090,#71091),(#71092,
#71093),(#71094,#71095),(#71096,#71097),(#71098,#71099),(#71100,#71101),
(#71102,#71103),(#71104,#71105),(#71106,#71107),(#71108,#71109),(#71110,
#71111),(#71112,#71113),(#71114,#71115),(#71116,#71117),(#71118,#71119),
(#71120,#71121),(#71122,#71123),(#71124,#71125),(#71126,#71127),(#71128,
#71129),(#71130,#71131),(#71132,#71133),(#71134,#71135),(#71136,#71137),
(#71138,#71139),(#71140,#71141),(#71142,#71143),(#71144,#71145),(#71146,
#71147),(#71148,#71149),(#71150,#71151),(#71152,#71153),(#71154,#71155),
(#71156,#71157),(#71158,#71159),(#71160,#71161),(#71162,#71163),(#71164,
#71165),(#71166,#71167),(#71168,#71169),(#71170,#71171),(#71172,#71173),
(#71174,#71175),(#71176,#71177),(#71178,#71179),(#71180,#71181),(#71182,
#71183),(#71184,#71185),(#71186,#71187),(#71188,#71189),(#71190,#71191),
(#71192,#71193),(#71194,#71195),(#71196,#71197),(#71198,#71199),(#71200,
#71201),(#71202,#71203),(#71204,#71205),(#71206,#71207),(#71208,#71209),
(#71210,#71211),(#71212,#71213),(#71214,#71215),(#71216,#71217),(#71218,
#71219),(#71220,#71221),(#71222,#71223),(#71224,#71225),(#71226,#71227),
(#71228,#71229),(#71230,#71231),(#71232,#71233),(#71234,#71235),(#71236,
#71237),(#71238,#71239),(#71240,#71241),(#71242,#71243),(#71244,#71245),
(#71246,#71247),(#71248,#71249),(#71250,#71251),(#71252,#71253),(#71254,
#71255),(#71256,#71257),(#71258,#71259),(#71260,#71261),(#71262,#71263),
(#71264,#71265),(#71266,#71267),(#71268,#71269),(#71270,#71271),(#71272,
#71273),(#71274,#71275),(#71276,#71277),(#71278,#71279),(#71280,#71281),
(#71282,#71283),(#71284,#71285),(#71286,#71287),(#71288,#71289),(#71290,
#71291),(#71292,#71293),(#71294,#71295),(#71296,#71297),(#71298,#71299),
(#71300,#71301),(#71302,#71303),(#71304,#71305),(#71306,#71307),(#71308,
#71309),(#71310,#71311),(#71312,#71313),(#71314,#71315),(#71316,#71317),
(#71318,#71319),(#71320,#71321),(#71322,#71323),(#71324,#71325),(#71326,
#71327),(#71328,#71329),(#71330,#71331),(#71332,#71333),(#71334,#71335),
(#71336,#71337),(#71338,#71339),(#71340,#71341),(#71342,#71343),(#71344,
#71345),(#71346,#71347),(#71348,#71349),(#71350,#71351),(#71352,#71353),
(#71354,#71355),(#71356,#71357),(#71358,#71359),(#71360,#71361),(#71362,
#71363),(#71364,#71365),(#71366,#71367),(#71368,#71369),(#71370,#71371),
(#71372,#71373),(#71374,#71375),(#71376,#71377),(#71378,#71379),(#71380,
#71381),(#71382,#71383),(#71384,#71385),(#71386,#71387),(#71388,#71389),
(#71390,#71391),(#71392,#71393),(#71394,#71395),(#71396,#71397),(#71398,
#71399),(#71400,#71401),(#71402,#71403),(#71404,#71405),(#71406,#71407),
(#71408,#71409),(#71410,#71411),(#71412,#71413),(#71414,#71415),(#71416,
#71417),(#71418,#71419),(#71420,#71421),(#71422,#71423),(#71424,#71425),
(#71426,#71427),(#71428,#71429),(#71430,#71431),(#71432,#71433),(#71434,
#71435),(#71436,#71437),(#71438,#71439),(#71440,#71441),(#71442,#71443),
(#71444,#71445),(#71446,#71447),(#71448,#71449),(#71450,#71451),(#71452,
#71453),(#71454,#71455),(#71456,#71457),(#71458,#71459),(#71460,#71461),
(#71462,#71463),(#71464,#71465),(#71466,#71467),(#71468,#71469),(#71470,
#71471),(#71472,#71473),(#71474,#71475),(#71476,#71477),(#71478,#71479),
(#71480,#71481),(#71482,#71483),(#71484,#71485),(#71486,#71487),(#71488,
#71489),(#71490,#71491),(#71492,#71493),(#71494,#71495),(#71496,#71497),
(#71498,#71499),(#71500,#71501),(#71502,#71503),(#71504,#71505),(#71506,
#71507),(#71508,#71509),(#71510,#71511),(#71512,#71513),(#71514,#71515),
(#71516,#71517),(#71518,#71519),(#71520,#71521),(#71522,#71523),(#71524,
#71525),(#71526,#71527),(#71528,#71529),(#71530,#71531),(#71532,#71533)),
 .UNSPECIFIED.,.F.,.F.,.F.,(4,1,1,1,1,1,1,1,1,1,1,1,1,1,1,1,1,1,1,1,1,1,
1,1,1,1,1,1,1,1,1,1,1,1,1,1,1,1,1,1,1,1,1,1,1,1,1,1,1,1,1,1,1,1,1,1,1,1,
1,1,1,1,1,1,1,1,1,1,1,1,1,1,1,1,1,1,1,1,1,1,1,1,1,1,1,1,1,1,1,1,1,1,1,1,
1,1,1,1,1,1,1,1,1,1,1,1,1,1,1,1,1,1,1,1,1,1,1,1,1,1,1,1,1,1,1,1,1,1,1,1,
1,1,1,1,1,1,1,1,1,1,1,1,1,1,1,1,1,1,1,1,1,1,1,1,1,1,1,1,1,1,1,1,1,1,1,1,
1,1,1,1,1,1,1,1,1,1,1,1,1,1,1,1,1,1,1,1,1,1,1,1,1,1,1,1,1,1,1,1,1,1,1,1,
1,1,1,1,1,1,1,1,1,1,1,1,1,1,1,1,1,1,1,1,1,1,1,1,1,1,1,1,1,1,1,1,1,1,1,1,
1,1,1,1,1,1,1,1,1,1,1,1,1,1,1,1,1,1,1,1,1,1,1,1,1,1,1,1,1,1,1,1,1,1,1,1,
1,1,1,1,1,1,1,1,1,1,1,1,1,1,1,1,1,1,1,1,1,1,1,1,1,1,1,1,1,1,1,1,1,1,1,1,
1,1,1,1,1,1,1,1,1,1,1,1,1,1,1,1,1,1,1,1,1,1,1,1,1,1,1,1,1,1,1,1,1,1,1,1,
1,1,1,1,1,1,1,1,1,1,1,1,1,1,1,1,1,1,1,1,1,1,1,1,1,1,1,1,1,1,1,1,1,1,1,1,
1,1,1,1,1,1,1,1,1,1,1,1,1,1,1,1,1,1,1,1,1,1,1,1,1,1,1,1,1,1,1,1,1,1,1,1,
1,1,1,1,1,1,1,1,1,1,1,1,1,1,1,1,1,1,1,1,1,1,1,1,1,1,1,1,1,1,1,1,1,1,1,1,
1,1,1,1,1,1,1,1,1,1,1,1,1,1,1,1,1,1,1,1,1,1,1,1,1,1,1,1,1,1,1,1,1,1,1,1,
1,1,1,1,1,1,1,1,1,1,1,1,1,1,1,1,1,1,1,1,1,1,1,1,1,1,1,1,1,1,1,1,1,1,1,1,
1,1,1,1,1,1,1,1,1,1,1,1,1,1,1,1,1,1,1,1,1,1,1,1,1,1,1,1,1,1,1,1,1,1,1,1,
1,1,1,1,1,1,1,1,1,1,1,1,1,1,1,1,1,1,1,1,1,1,1,1,1,1,1,1,1,1,1,1,1,1,1,1,
1,1,1,1,1,1,1,1,1,1,1,1,1,1,1,1,1,1,1,1,1,1,1,1,1,1,1,1,1,1,1,1,1,1,1,1,
1,1,1,1,1,1,1,1,1,1,1,1,1,1,1,1,1,1,1,1,1,1,1,1,1,1,1,1,1,1,1,1,1,1,1,1,
1,1,1,1,1,1,1,1,1,1,1,1,1,1,1,1,1,1,1,1,1,1,1,1,1,1,1,1,1,1,1,1,1,1,1,1,
1,1,1,1,1,1,1,1,1,1,1,1,1,1,1,1,1,1,1,1,1,1,1,1,1,1,1,1,1,1,1,1,1,1,1,1,
1,1,1,1,1,1,1,1,1,1,1,1,1,1,1,1,1,1,1,1,1,1,1,1,1,1,1,1,1,1,1,1,1,1,1,1,
1,1,1,1,1,1,1,1,1,1,1,1,1,1,1,1,1,1,1,1,1,1,1,1,1,1,1,1,1,1,1,1,1,1,1,1,
1,1,1,1,1,1,1,1,1,1,1,1,1,1,1,1,1,1,1,1,1,1,1,1,1,1,1,1,1,1,1,1,1,1,1,1,
1,1,1,1,1,1,1,1,1,1,1,1,1,1,1,1,1,1,1,1,1,1,1,1,1,1,1,1,1,1,1,1,1,1,1,1,
1,1,1,1,1,1,1,1,1,1,1,1,1,1,1,1,1,1,1,1,1,1,1,1,1,1,1,1,1,1,1,1,1,1,1,1,
1,1,1,1,1,1,1,1,1,1,1,1,1,1,1,1,1,1,1,1,1,1,1,1,1,1,1,1,1,1,1,1,1,1,1,1,
1,1,1,1,1,1,1,1,1,1,1,1,1,1,1,1,1,1,1,1,1,1,1,1,1,1,1,1,1,1,1,1,1,1,1,1,
1,1,1,1,1,1,1,1,1,1,1,1,1,1,1,1,1,1,1,1,1,1,1,1,1,1,1,1,1,1,1,1,1,1,1,1,
1,1,1,1,1,1,1,1,1,1,1,1,1,1,1,1,1,1,1,1,1,1,1,1,1,1,1,1,1,1,1,1,1,1,1,1,
1,1,1,1,1,1,1,1,1,1,1,1,1,1,1,1,1,1,1,1,1,1,1,1,1,1,1,1,1,1,1,1,1,1,1,1,
1,1,1,1,1,1,1,1,1,1,1,1,1,1,1,1,1,1,1,1,1,1,1,1,1,1,1,1,1,1,1,1,1,1,1,1,
1,1,1,1,1,1,1,1,1,1,1,1,1,1,1,1,1,1,1,1,1,1,1,1,1,1,1,1,1,1,1,1,1,1,1,1,
1,1,1,1,1,1,1,1,1,1,1,1,1,1,1,1,1,1,1,1,1,1,1,1,1,1,1,1,1,1,1,1,1,1,1,1,
1,1,1,1,1,1,1,1,1,1,1,1,1,1,1,1,1,1,1,1,1,1,1,1,1,1,1,1,1,1,1,1,1,1,1,1,
1,1,1,1,1,1,1,1,1,1,1,1,1,1,1,1,1,1,1,1,1,1,1,1,1,1,1,1,1,1,1,1,1,1,1,1,
1,1,1,1,1,1,1,1,1,1,1,1,1,1,1,1,1,1,1,1,1,1,1,1,1,1,1,1,1,1,1,1,1,1,1,1,
1,1,1,1,1,1,1,1,1,1,1,1,1,1,1,1,1,1,1,1,1,1,1,1,1,1,1,1,1,1,1,1,1,1,1,1,
1,1,1,1,1,1,1,1,1,1,1,1,1,1,1,1,1,1,1,1,1,1,1,1,1,1,1,1,1,1,1,1,1,1,1,1,
1,1,1,1,1,1,1,1,1,1,1,1,1,1,1,1,1,1,1,1,1,1,1,1,1,1,1,1,1,1,1,1,1,1,1,1,
1,1,1,1,1,1,1,1,1,1,1,1,1,1,1,1,1,1,1,1,1,1,1,1,1,1,1,1,1,1,1,1,1,1,1,1,
1,1,1,1,1,1,1,1,1,1,1,1,1,1,1,1,1,1,1,1,1,1,1,1,1,1,1,1,1,1,1,1,1,1,1,1,
1,1,1,1,1,1,1,1,1,1,1,1,1,1,1,1,1,1,1,1,1,1,1,1,1,1,1,1,1,1,1,1,1,1,1,1,
1,1,1,1,1,1,1,1,1,1,1,1,1,1,1,1,1,1,1,1,1,1,1,1,1,1,1,1,1,1,1,1,1,1,1,1,
1,1,1,1,1,1,1,1,1,1,1,1,1,1,1,1,1,1,1,1,1,1,1,1,1,1,1,1,1,1,1,1,1,1,1,1,
1,1,1,1,1,1,1,1,1,1,1,1,1,1,1,1,1,1,1,1,1,1,1,1,1,1,1,1,1,1,1,1,1,1,1,1,
1,1,1,1,1,1,1,1,1,1,1,1,1,1,1,1,1,1,1,1,1,1,1,1,1,1,1,1,1,1,1,1,1,1,1,1,
1,1,1,1,1,1,1,1,1,1,1,1,1,1,1,1,1,1,1,1,1,1,1,1,1,1,1,1,1,1,1,1,1,1,1,1,
1,1,1,1,1,1,1,1,1,1,1,1,1,1,1,1,1,1,1,1,1,1,1,1,1,1,1,1,1,1,1,1,1,1,1,1,
1,1,1,1,1,1,1,1,1,1,1,1,1,1,1,1,1,1,1,1,1,1,1,1,1,1,1,1,1,1,1,1,1,1,1,1,
1,1,1,1,1,1,1,1,1,1,1,1,1,1,1,1,1,1,1,1,1,1,1,1,1,1,1,1,1,1,1,1,1,1,1,1,
1,1,1,1,1,1,1,1,1,1,1,1,1,1,1,1,1,1,1,1,1,1,1,1,1,1,1,1,1,1,1,1,1,1,1,1,
1,1,1,1,1,1,1,1,1,1,1,1,1,1,1,1,1,1,1,1,1,1,1,1,1,1,1,1,1,1,1,1,1,1,1,1,
1,1,1,1,1,1,1,1,1,1,1,1,1,1,1,1,1,1,1,1,1,1,1,1,1,1,1,1,1,1,1,1,1,1,1,1,
1,1,1,1,1,1,1,1,1,1,1,1,1,1,1,1,1,1,1,1,1,1,1,1,1,1,1,1,1,1,1,1,1,1,1,1,
1,1,1,1,1,1,1,1,1,1,1,1,1,1,1,1,1,1,1,1,1,1,1,1,1,1,1,1,1,1,1,1,1,1,1,1,
1,1,1,1,1,1,1,1,1,1,1,1,1,1,1,1,1,1,1,1,1,1,1,1,1,1,1,1,1,1,1,1,1,1,1,1,
1,1,1,1,1,1,1,1,1,1,1,1,1,1,1,1,1,1,1,1,1,1,1,1,1,1,1,1,1,1,1,1,1,1,1,1,
1,1,1,1,1,1,1,1,1,1,1,1,1,1,1,1,1,1,1,1,1,1,1,1,1,1,1,1,1,1,1,1,1,1,1,1,
1,1,1,1,1,1,1,1,1,1,1,1,1,1,1,1,1,1,1,1,1,1,1,1,1,1,1,1,1,1,1,1,1,1,1,1,
1,1,1,1,1,1,1,1,1,1,1,1,1,1,1,1,1,1,1,1,1,1,1,1,1,1,1,1,1,1,1,1,1,1,1,1,
1,1,1,1,1,1,1,1,1,1,1,1,1,1,1,1,1,1,1,1,1,1,1,1,1,1,1,1,1,1,1,1,1,1,1,1,
1,1,1,1,1,1,1,1,1,1,1,1,1,1,1,1,1,1,1,1,1,1,1,1,1,1,1,1,1,1,1,1,1,1,1,1,
1,1,1,1,1,1,1,1,1,1,1,1,1,1,1,1,1,1,1,1,1,1,1,1,1,1,1,1,1,1,1,1,1,1,1,1,
1,1,1,1,1,1,1,1,1,1,1,1,1,1,1,1,1,1,1,1,1,1,1,1,1,1,1,1,1,1,1,1,1,1,1,1,
1,1,1,1,1,1,1,1,1,1,1,1,1,1,1,1,1,1,1,1,1,1,1,1,1,1,1,1,1,1,1,1,1,1,1,1,
1,1,1,1,1,1,1,1,1,1,1,1,1,1,1,1,1,1,1,1,1,1,1,1,1,1,1,1,1,1,1,1,1,1,1,1,
1,1,1,1,1,1,1,1,1,1,1,1,1,1,1,1,1,1,1,1,1,1,1,1,1,1,1,1,1,1,1,1,1,1,1,1,
1,1,1,1,1,1,1,1,1,1,1,1,1,1,1,1,1,1,1,1,1,1,1,1,1,1,1,1,1,1,1,1,1,1,1,1,
1,1,1,1,1,1,1,1,1,1,1,1,1,1,1,1,1,1,1,1,1,1,1,1,1,1,1,1,1,1,1,1,1,1,1,1,
1,1,1,1,1,1,1,1,1,1,1,1,1,1,1,1,1,1,1,1,1,1,1,1,1,1,1,1,1,1,1,1,1,1,1,1,
1,1,1,1,1,1,1,1,1,1,1,1,1,1,1,1,1,1,1,1,1,1,1,1,1,1,1,1,1,1,1,1,1,1,1,1,
1,1,1,1,1,1,1,1,1,1,1,1,1,1,1,1,1,1,1,1,1,1,1,1,1,1,1,1,1,1,1,1,1,1,1,1,
1,1,1,1,1,1,1,1,1,1,1,1,1,1,1,1,1,1,1,1,1,1,1,1,1,1,1,1,1,1,1,1,1,1,1,1,
1,1,1,1,1,1,1,1,1,1,1,1,1,1,1,1,1,1,1,1,1,1,1,1,1,1,1,1,1,1,1,1,1,1,1,1,
1,1,1,1,1,1,1,1,1,1,1,1,1,1,1,1,1,1,1,1,1,1,1,1,1,1,1,1,1,1,1,1,1,1,1,1,
1,1,1,1,1,1,1,1,1,1,1,1,1,1,1,1,1,1,1,1,1,1,1,1,1,1,1,1,1,1,1,1,1,1,1,1,
1,1,1,1,1,1,1,1,1,1,1,1,1,1,1,1,1,1,1,1,1,1,1,1,1,1,1,1,1,1,1,1,1,1,1,1,
1,1,1,1,1,1,1,1,1,1,1,1,1,1,1,1,1,1,1,1,1,1,1,1,1,1,1,1,1,1,1,1,1,1,1,1,
1,1,1,1,1,1,1,1,1,1,1,1,1,1,1,1,1,1,1,1,1,1,1,1,1,1,1,1,1,1,1,1,1,1,1,1,
1,1,1,1,1,1,1,1,1,1,1,1,1,1,1,1,1,1,1,1,1,1,1,1,1,1,1,1,1,1,1,1,1,1,1,1,
1,1,1,1,1,1,1,1,1,1,1,1,1,1,1,1,1,1,1,1,1,1,1,1,1,1,1,1,1,1,1,1,1,1,1,1,
1,1,1,1,1,1,1,1,1,1,1,1,1,1,1,1,1,1,1,1,1,1,1,1,1,1,1,1,1,1,1,1,1,1,1,1,
1,1,1,1,1,1,1,1,1,1,1,1,1,1,1,1,1,1,1,1,1,1,1,1,1,1,1,1,1,1,1,1,1,1,1,1,
1,1,1,1,1,1,1,1,1,1,1,1,1,1,1,1,1,1,1,1,1,1,1,1,1,1,1,1,1,1,1,1,1,1,1,1,
1,1,1,1,1,1,1,1,1,1,1,1,1,1,1,1,1,1,1,1,1,1,1,1,1,1,1,1,1,1,1,1,1,1,1,1,
1,1,1,1,1,1,1,1,1,1,1,1,1,1,1,1,1,1,1,1,1,1,1,1,1,1,1,1,1,1,1,1,1,1,1,1,
1,1,1,1,1,1,1,1,1,1,1,1,1,1,1,1,1,1,1,1,1,1,1,1,1,1,1,1,1,1,1,1,1,1,1,1,
1,1,1,1,1,1,1,1,1,1,1,1,1,1,1,1,1,1,1,1,1,1,1,1,1,1,1,1,1,1,1,1,1,1,1,1,
1,1,1,1,1,1,1,1,1,1,1,1,1,1,1,1,1,1,1,1,1,1,1,1,1,1,1,1,1,1,1,1,1,1,1,1,
1,1,1,1,1,1,1,1,1,1,1,1,1,1,1,1,1,1,1,1,1,1,1,1,1,1,1,1,1,1,1,1,1,1,1,1,
1,1,1,1,1,1,1,1,1,1,1,1,1,1,1,1,1,1,1,1,1,1,1,1,1,1,1,1,1,1,1,1,1,1,1,1,
1,1,1,1,1,1,1,1,1,1,1,1,1,1,1,1,1,1,1,1,1,1,1,1,1,1,1,1,1,1,1,1,1,1,1,1,
1,1,1,1,1,1,1,1,1,1,1,1,1,1,1,1,1,1,1,1,1,1,1,1,1,1,1,1,1,1,1,1,1,1,1,1,
1,1,1,1,1,1,1,1,1,1,1,1,1,1,1,1,1,1,1,1,1,1,1,1,1,1,1,1,1,1,1,1,1,1,1,1,
1,1,1,1,1,1,1,1,1,1,1,1,1,1,1,1,1,1,1,1,1,1,1,1,1,1,1,1,1,1,1,1,1,1,1,1,
1,1,1,1,1,1,1,1,1,1,1,1,1,1,1,1,1,1,1,1,1,1,1,1,1,1,1,1,1,1,1,1,1,1,1,1,
1,1,1,1,4),(2,2),(0.,0.869746702321014,1.7394931589914,2.60923976624962,
3.47983908319159,4.35043840179749,5.22018503077054,6.08993165951504,6.95967828799171,
7.82942491616733,8.69917154401062,9.56891817149224,10.4395174886835,11.3101168056706,
12.179863432132,13.049610058144,13.9193566836854,14.7891033087372,15.6588499332817,
16.5285965573034,17.3991958717975,18.2697951860185,18.7046684974166,19.1395418086746,
19.5744151197912,20.0092884307654,20.4441617415962,20.8790350522825,21.7487816732187,
22.1836549834672,22.6185282935685,23.0534016035221,23.4882749133276,23.9231482229848,
24.3588742245859,24.794600226187,25.2294735355468,26.0992201538203,26.5340934627341,
26.9689667714994,27.4038400801166,27.838713388586,28.2735866969081,28.7084600050832,
29.143333313112,29.5782066209952,30.0130799287334,30.4479532363275,30.8828265437783,
31.3185525442794,31.7542785447804,32.1891518519474,32.6240251589741,33.0588984658616,
33.4937717726112,33.928645079224,34.3635183857014,34.7983916920448,35.2332649982556,
35.6681383043353,36.1030116102854,36.5378849161076,36.9727582218035,37.4076315273749,
37.8425048328235,38.2782308323341,38.7139568318446,39.1488301370532,39.5837034421446,
40.0185767471208,40.4534500519838,40.8883233567357,41.3231966613787,41.7580699659148,
42.1929432703463,42.6278165746754,43.0626898789044,43.4975631830356,43.9324364870714,
44.3673097910142,44.8021830948664,45.2379090935952,45.673635092324,46.1085083960024,
46.5433816995978,46.9782550031127,47.4131283065497,47.8480016099115,48.2828749132006,
48.7177482164198,49.1526215195718,49.5874948226593,50.0223681256851,50.457241428652,
50.8921147315628,51.3269880344203,51.7618613372274,52.197587335454,52.6333133336805,
53.0681866363954,53.5030599390685,53.9379332417027,54.3728065443011,54.8076798468664,
55.2425531494018,55.6774264519101,56.1122997543943,56.5471730568575,56.9820463593026,
57.4169196617326,57.8517929641506,58.2866662665595,58.7215395689624,59.157265567009,
59.5929915650557,60.0278648674556,60.4627381698584,60.8976114722673,61.3324847746853,
61.7673580771153,62.2022313795604,62.6371046820236,63.0719779845079,63.5068512870162,
63.9417245895516,64.376597892117,64.8114711947155,65.2463444973499,65.6812178000231,
66.1169437982275,66.5526697964318,66.9875430991915,67.4224164019987,67.8572897048563,
68.2921630077673,68.7270363107343,69.1619096137603,69.5967829168479,70.0316562200001,
70.4665295232194,70.9014028265087,71.3362761298705,71.7711494333077,72.2060227368227,
72.6408960404182,73.0766220391044,73.5123480377905,73.9472213415547,74.382094645407,
74.8169679493499,75.2518412533859,75.6867145575172,76.1215878617464,76.5564611660756,
76.9913344705072,77.4262077750435,77.8610810796866,78.2959543844386,78.7308276893018,
79.1657009942781,79.6005742993696,80.0363002988208,80.4720262982719,80.9068996035997,
81.3417729090484,81.7766462146199,82.211519520316,82.6463928261383,83.0812661320886,
83.5161394381684,83.9510127443794,84.3858860507229,84.8207593572004,85.2556326638134,
85.6905059705631,86.1253792774507,86.5602525844776,86.995978584908,87.4317045853384,
87.8665778926469,88.3014512000977,88.7363245076919,89.1711978154302,89.6060711233134,
90.0409444313423,90.4758177395175,90.9106910478396,91.345564356309,91.7804376649263,
92.2153109736917,92.6501842826055,93.085057591668,93.5199309008791,93.9556569024059,
94.3913829039327,94.8262562134414,95.2611295230986,95.6960028329042,96.1308761428578,
96.5657494529591,97.0006227632077,97.4354960736028,97.870369384144,98.3052426948304,
98.7401160056612,99.1749893166354,99.6098626277522,100.04473593901,100.915335253024,
101.351061255639,101.785934567313,102.220807879124,102.655681191068,103.090554503145,
103.525427815353,104.395174440154,105.264921065453,105.699794378283,106.134667691232,
106.569541004295,107.004414317471,107.8750136343,108.745612951339,109.615359578629,
110.485106206296,111.354852834309,112.224599462639,113.094346091254,113.964092720119,
114.834692038763,115.705291357499,116.575037986826,117.444784616267,118.314531245777,
119.184277875311,120.054024504821,120.923771134261,121.794370453112,122.66496977189,
123.534716400968,124.404463029834,125.274209658448,126.143956286779,127.013702914792,
127.883449542458,128.754048859798,129.624648176939,130.494394803617,131.364141429857,
132.233888055637,133.103634680937,133.973381305737,134.843127930023,135.71372724472,
136.584326559147,137.019199870684,137.454073182083,137.888946493341,138.323819804458,
139.193566426263,140.063313047491,140.498186357887,140.933059668136,141.367932978237,
141.802806288191,142.237679597997,142.673405599673,143.109131601348,143.544004910857,
143.978878220217,144.413751529429,144.848624838491,145.283498147405,145.718371456171,
146.153244764789,146.588118073258,147.022991381581,147.457864689756,147.892737997785,
148.327611305669,148.762484613407,149.197357921002,149.633083921574,150.068809922147,
150.503683229455,150.938556536623,151.37342984365,151.808303150538,152.243176457288,
152.678049763901,153.112923070379,153.547796376722,153.982669682934,154.417542989014,
154.852416294964,155.287289600787,155.722162906483,156.157036212055,156.592762211626,
157.028488211198,157.463361516526,157.898234821735,158.333108126826,158.767981431803,
159.202854736666,159.637728041419,160.072601346062,160.507474650599,160.94234795503,
161.37722125936,161.812094563589,162.246967867721,162.681841171757,163.1167144757,
163.552440474473,163.988166473247,164.423039777011,164.85791308069,165.292786384286,
165.727659687801,166.162532991238,166.597406294601,167.03227959789,167.46715290111,
167.902026204262,168.33689950735,168.771772810376,169.206646113343,169.641519416254,
170.076392719112,170.512118717363,170.947844715614,171.382718018374,171.817591321089,
172.252464623762,172.687337926397,173.122211228996,173.557084531561,173.991957834097,
174.426831136606,174.86170443909,175.296577741554,175.731451044,176.16632434643,
176.601197648848,177.036070951258,177.471796949306,177.907522947355,178.342396249755,
178.777269552155,179.212142854558,179.647016156968,180.081889459386,180.516762761816,
180.951636064262,181.386509366726,181.82138266921,182.256255971719,182.691129274255,
183.12600257682,183.560875879419,183.995749182054,184.431475180237,184.867201178421,
185.302074481136,185.736947783896,186.171821086704,186.606694389561,187.041567692473,
187.47644099544,187.911314298466,188.346187601554,188.781060904706,189.215934207926,
189.650807511215,190.085680814577,190.520554118015,190.95542742153,191.391153420175,
191.82687941882,192.261752722499,192.696626026263,193.131499330116,193.566372634059,
194.001245938095,194.436119242227,194.870992546456,195.305865850785,195.740739155217,
196.175612459754,196.610485764397,197.045359069149,197.480232374013,197.915105678989,
198.350831678382,198.786557677775,199.221430982984,199.656304288312,200.091177593761,
200.526050899333,200.960924205029,201.395797510852,201.830670816802,202.265544122882,
202.700417429093,203.135290735437,203.570164041915,204.005037348528,204.439910655278,
204.874783962166,205.310509962526,205.746235962887,206.181109270054,206.615982577363,
207.050855884814,207.485729192409,207.920602500147,208.355475808031,208.79034911606,
209.225222424235,209.660095732558,210.094969041027,210.529842349645,210.96471565841,
211.399588967324,211.834462276387,212.27018827784,212.705914279292,213.140787588653,
213.575660898161,214.010534207819,214.880280827579,215.31515413768,215.750027447929,
216.184900758324,216.619774068866,217.054647379553,217.489520690384,218.359267312475,
219.22986662628,219.665592628826,220.100465940363,220.535339252038,220.970212563848,
221.83995918787,222.709705812416,223.579452437468,224.014325750179,224.44919906301,
225.318945689022,226.189545005688,227.060144322571,227.929890949664,228.799637577146,
229.66938420499,230.539130833166,231.408877461643,232.278624090388,233.149223408954,
234.019822727623,234.889569356878,235.759315986267,236.629062615749,237.498809245277,
238.368555874806,239.238302504287,240.108901823183,240.979501142017,241.849247771189,
242.718994400167,243.588741028911,244.458487657389,245.328234285565,246.197980913409,
247.068580230891,247.939179548182,248.80892617507,249.678672801532,250.548419427545,
251.418166053087,252.287912678139,253.157659302684,254.028258617581,254.898857932211,
255.333731243885,255.768604555423,256.203477866821,256.63835117808,257.508097800171,
258.377844421689,258.812717732231,259.247591042627,259.682464352876,260.117337662977,
260.552210972931,260.987936974682,261.858536286089,262.293409595598,262.728282904958,
263.16315621417,263.598029523233,264.032902832147,264.467776140913,264.902649449531,
265.337522758001,265.772396066323,266.207269374499,266.642142682528,267.077015990412,
267.511889298151,267.947615298795,268.383341299439,268.81821460689,269.2530879142,
269.687961221367,270.122834528394,270.557707835282,270.992581142032,271.427454448646,
271.862327755124,272.297201061468,272.732074367679,273.166947673759,273.60182097971,
274.036694285533,274.471567591229,274.907293590862,275.343019590495,275.777892895944,
276.212766201272,276.647639506481,277.082512811573,277.51738611655,277.952259421414,
278.387132726166,278.82200603081,279.256879335346,279.691752639779,280.126625944108,
280.561499248338,280.996372552469,281.431245856506,281.866971855324,282.302697854143,
282.737571157996,283.172444461761,283.60731776544,284.042191069036,284.477064372551,
284.911937675989,285.346810979351,285.781684282641,286.216557585861,286.651430889013,
287.086304192101,287.521177495128,287.956050798095,288.390924101007,288.826650099283,
289.262376097559,289.697249400366,290.132122703127,290.566996005842,291.001869308516,
291.43674261115,291.871615913749,292.306489216315,292.741362518851,293.17623582136,
293.611109123845,294.045982426308,294.480855728754,294.915729031185,295.350602333603,
295.786328331655,296.222054329707,296.65692763211,297.091800934511,297.526674236911,
297.961547539314,298.396420841724,298.831294144142,299.266167446573,299.701040749018,
300.135914051482,300.570787353967,301.005660656476,301.440533959012,301.875407261578,
302.310280564177,302.746006562341,303.181732560506,303.616605863179,304.051479165895,
304.486352468655,304.921225771462,305.35609907432,305.790972377232,306.225845680199,
306.660718983226,307.095592286314,307.530465589466,307.965338892686,308.400212195976,
308.835085499338,309.269958802776,309.705684801381,310.141410799985,310.576284103581,
311.01115740726,311.446030711025,311.880904014878,312.315777318821,312.750650622858,
313.185523926989,313.620397231219,314.055270535549,314.490143839981,314.925017144517,
315.359890449161,315.794763753913,316.229637058777,316.665363058112,317.101089057448,
317.53596236254,317.970835667749,318.405708973077,318.840582278526,319.275455584098,
319.710328889795,320.145202195618,320.580075501568,321.014948807648,321.44982211386,
321.884695420204,322.319568726682,322.754442033295,323.189315340045,323.625041340336,
324.060767340628,324.495640647655,324.930513954822,325.365387262131,325.800260569583,
326.235133877177,326.670007184916,327.1048804928,327.539753800829,327.974627109005,
328.409500417327,328.844373725797,329.279247034415,329.714120343181,330.148993652095,
330.584719653474,331.020445654852,331.455318964064,331.890192273424,332.325065582933,
332.759938892591,333.194812202397,333.629685512351,334.064558822453,334.499432132702,
334.934305443098,335.369178753639,335.804052064326,336.673798686132,337.108671997249,
337.544397999725,337.980124002201,338.4149973136,338.849870625137,339.284743936812,
340.154490560568,341.024237184854,341.459110497191,341.893983809655,342.328857122244,
342.763730434955,343.633477060735,344.504076377234,345.374675693955,346.244422320844,
347.114168948136,347.983915575803,348.853662203817,349.723408832148,350.593155460764,
351.463754779246,352.334354097839,353.204100727012,354.07384735634,354.943593985781,
355.813340615292,356.683087244827,357.552833874338,358.423433193272,359.294032512154,
360.163779141409,361.033525770489,361.903272399355,362.77301902797,363.642765656301,
364.512512284316,365.383111601936,366.253710919371,367.123457546465,367.993204173143,
368.862950799383,369.732697425164,370.602444050463,371.472190675265,372.342789990359,
373.21338930519,373.648262617,374.083135928675,374.952882551611,375.822629173987,
376.257502484962,376.692375795793,377.12724910648,377.562122417021,377.996995727417,
378.431869037666,378.866742347767,379.302468349591,379.738194351416,380.173067661222,
380.607940970879,381.042814280388,381.477687589749,381.91256089896,382.347434208023,
382.782307516937,383.217180825703,383.652054134321,384.086927442791,384.521800751113,
384.956674059289,385.391547367318,385.826420675202,386.262146675918,386.697872676635,
387.13274598423,387.567619291681,388.00249259899,388.437365906157,388.872239213185,
389.307112520073,389.741985826823,390.176859133436,390.611732439914,391.046605746258,
391.48147905247,391.91635235855,392.351225664501,392.786098970323,393.221824970019,
393.657550969714,394.092424275286,394.527297580735,394.962170886063,395.397044191272,
395.831917496364,396.266790801341,396.701664106204,397.136537410957,397.5714107156,
398.006284020137,398.441157324569,398.876030628899,399.310903933128,399.74577723726,
400.181503236126,400.617229234991,401.052102538934,401.486975842787,401.921849146551,
402.356722450231,402.791595753827,403.226469057342,403.66134236078,404.096215664142,
404.531088967432,404.965962270651,405.400835573804,405.835708876892,406.270582179918,
406.705455482886,407.141181481189,407.576907479491,408.01178078235,408.446654085157,
408.881527387917,409.316400690633,409.751273993306,410.186147295941,410.62102059854,
411.055893901106,411.490767203642,411.925640506151,412.360513808636,412.795387111099,
413.230260413545,413.665133715976,414.100859714032,414.536585712088,414.971459014498,
415.406332316901,415.841205619301,416.276078921702,416.710952224105,417.145825526515,
417.580698828933,418.015572131364,418.45044543381,418.885318736273,419.320192038758,
419.755065341267,420.189938643803,420.624811946369,421.060537944515,421.496263942662,
421.931137245297,422.36601054797,422.800883850686,423.235757153446,423.670630456253,
424.105503759112,424.540377062023,424.975250364991,425.410123668017,425.844996971105,
426.279870274258,426.714743577477,427.149616880767,427.584490184129,428.020216182695,
428.455942181261,428.890815484776,429.325688788373,429.760562092052,430.195435395816,
430.630308699669,431.065182003612,431.500055307649,431.93492861178,432.36980191601,
432.80467522034,433.239548524772,433.674421829309,434.109295133952,434.544168438705,
434.979894437984,435.415620437262,435.850493742239,436.285367047331,436.72024035254,
437.155113657869,437.589986963318,438.024860268889,438.459733574586,438.894606880409,
439.32948018636,439.76435349244,440.199226798651,440.634100104995,441.068973411473,
441.503846718087,441.939572718309,442.375298718531,442.810172025419,443.245045332447,
443.679918639614,444.114791946923,444.549665254374,444.984538561969,445.419411869708,
445.854285177591,446.289158485621,446.724031793796,447.158905102119,447.593778410589,
448.028651719207,448.463525027973,448.899251029277,449.334977030581,449.769850339644,
450.639596958216,451.074470267725,451.509343577383,451.944216887189,452.379090197143,
452.813963507244,453.248836817493,453.683710127889,454.118583438431,454.553456749117,
454.988330059949,455.423203370923,455.858929373329,456.294655375734,456.729528686993,
457.164401998391,457.599275309929,458.469021933414,458.90389524536,459.338768557437,
459.773641869646,460.208515181983,460.643388494447,461.078261807036,461.948008432578,
462.818607748906,463.689207065461,464.55895369214,465.428700319234,466.298446946716,
467.16819357456,468.037940202737,468.907686831215,469.778286149605,470.648885468116,
471.518632097196,472.388378726451,473.258125355841,474.127871985322,474.997618614851,
475.86736524438,476.737964563343,477.608563882265,478.478310511593,479.348057140765,
480.217803769743,481.087550398488,481.957297026966,482.827043655142,483.697642972895,
484.568242290469,485.43798891776,486.307735544649,487.177482171112,488.047228797125,
488.916975422667,489.78672204772,490.657321363009,491.09304736596,491.527920678038,
492.397667301793,493.267413925005,494.137160547663,494.57203385878,495.006907169755,
495.441780480586,495.876653791273,496.311527101814,496.74640041221,497.616999724357,
498.052725726255,498.487599036209,498.922472346015,499.357345655673,499.792218965182,
500.227092274542,500.661965583754,501.096838892816,501.531712201731,501.966585510497,
502.401458819114,502.836332127584,503.271205435907,503.706078744082,504.140952052112,
504.576678052901,505.01240405369,505.447277361429,505.882150669023,506.317023976474,
506.751897283783,507.186770590951,507.621643897978,508.056517204866,508.491390511616,
508.92626381823,509.361137124708,509.796010431052,510.230883737263,510.665757043344,
511.100630349294,511.536356349053,511.972082348811,512.406955654506,512.841828960076,
513.276702265523,513.711575570849,514.146448876056,514.581322181146,515.016195486121,
515.451068790983,515.885942095733,516.320815400375,516.75568870491,517.19056200934,
517.625435313668,518.060308617896,518.496034616807,518.931760615718,519.366633919752,
519.801507223694,520.236380527545,520.671253831307,521.106127134985,521.541000438579,
521.975873742092,522.410747045528,522.845620348888,523.280493652176,523.715366955394,
524.150240258545,524.585113561631,525.019986864656,525.455712862985,525.891438861313,
526.326312164223,526.761185467079,527.196058769885,527.630932072643,528.065805375356,
528.500678678029,528.935551980661,529.370425283258,529.805298585822,530.240171888356,
530.675045190863,531.109918493346,531.544791795808,531.979665098252,532.415391096312,
532.851117094373,533.285990396789,533.720863699197,534.155737001598,534.590610303997,
535.025483606395,535.460356908796,535.895230211204,536.330103513621,536.764976816049,
537.199850118493,537.634723420955,538.069596723438,538.504470025945,538.93934332848,
539.375069326608,539.810795324736,540.245668627333,540.680541929966,541.115415232637,
541.550288535351,541.985161838109,542.420035140915,542.854908443771,543.28978174668,
543.724655049646,544.15952835267,544.594401655757,545.029274958907,545.464148262125,
545.899021565413,546.334747563939,546.770473562465,547.205346865901,547.640220169415,
548.075093473009,548.509966776686,548.944840080449,549.3797133843,549.814586688241,
550.249459992276,550.684333296405,551.119206600633,551.554079904961,551.988953209391,
552.423826513926,552.858699818567,553.294425817789,553.73015181701,554.165025121872,
554.599898426846,555.034771731937,555.469645037144,555.90451834247,556.339391647917,
556.774264953487,557.209138259182,557.644011565003,558.078884870951,558.51375817703,
558.948631483239,559.383504789581,559.818378096058,560.254104096209,560.689830096361,
561.12470340311,561.559576709996,561.994450017021,562.429323324187,562.864196631494,
563.299069938943,563.733943246536,564.168816554273,564.603689862154,565.038563170182,
565.473436478355,565.908309786676,566.343183095144,566.77805640376,567.213782404988,
567.649508406216,568.084381715128,568.519255024189,568.954128333399,569.389001642757,
569.823874952264,570.258748261921,570.693621571725,571.128494881677,571.563368191777,
572.433114812417,572.867988122957,573.302861433642,573.737734744471,574.173460746804,
574.609186749136,575.044060060251,575.913806682904,576.783553306113,577.218426617922,
577.653299929865,578.08817324194,578.523046554147,579.392793178944,580.26253980424,
581.13313912039,581.568865123709,582.003738436771,582.87348506323,583.743231690115,
584.612978317402,585.482724945065,586.352471573076,587.222218201403,588.092817519691,
588.963416838109,589.833163467083,590.702910096251,591.572656725575,592.442403355013,
593.31214998452,594.181896614051,595.05249593303,595.92309525198,596.792841881366,
597.662588510618,598.532335139693,599.402081768556,600.271828397167,601.141575025495,
602.012174343369,602.882773661074,603.752520288553,604.622266915642,605.492013542317,
606.361760168553,607.23150679433,608.101253419626,608.971852735101,609.842452050322,
610.71219867434,611.581945297822,612.451691920754,612.886565232011,613.321438543126,
613.756311854099,614.191185164928,615.060931786153,615.931531098516,616.367257100486,
616.802130410586,617.237003720538,617.671877030342,618.106750339998,618.541623649505,
618.976496958863,619.411370268073,619.846243577134,620.281116886046,620.71599019481,
621.150863503426,621.585736811894,622.020610120214,622.455483428388,622.891209429248,
623.326935430108,623.761808737989,624.196682045726,624.631555353319,625.066428660769,
625.501301968075,625.936175275241,626.371048582266,626.805921889153,627.240795195901,
627.675668502512,628.110541808988,628.54541511533,628.98028842154,629.415161727618,
629.850887727438,630.286613727259,630.72148703308,631.156360338774,631.591233644344,
632.026106949791,632.460980255118,632.895853560325,633.330726865415,633.76560017039,
634.200473475251,634.635346780002,635.070220084644,635.505093389179,635.939966693609,
636.374839997937,636.810565996897,637.246291995857,637.681165299986,638.116038604021,
638.550911907962,638.985785211813,639.420658515576,639.855531819253,640.290405122847,
640.725278426361,641.160151729796,641.595025033157,642.029898336444,642.464771639662,
642.899644942813,643.334518245899,643.770244244257,644.205970242616,644.640843545581,
645.075716848491,645.510590151347,645.945463454153,646.380336756911,646.815210059625,
647.250083362296,647.684956664929,648.119829967526,648.55470327009,648.989576572624,
649.424449875131,649.859323177614,650.294196480076,650.729922478144,651.165648476212,
651.600521778641,652.035395081057,652.470268383465,652.905141685866,653.340014988265,
653.774888290663,654.209761593065,654.644634895472,655.079508197889,655.514381500318,
655.949254802762,656.384128105224,656.819001407706,657.253874710213,657.689600708326,
658.12532670644,658.560200009004,658.995073311601,659.429946614234,659.864819916905,
660.299693219619,660.734566522377,661.169439825183,661.604313128039,662.039186430948,
662.474059733914,662.908933036938,663.343806340025,663.778679643175,664.213552946393,
664.649278944883,665.085004943373,665.519878246733,665.954751550169,666.389624853683,
666.824498157277,667.259371460954,667.694244764717,668.129118068568,668.563991372509,
668.998864676544,669.433737980674,669.868611284901,670.303484589229,670.738357893659,
671.173231198194,671.608957197361,672.044683196528,672.479556501278,672.91442980614,
673.349303111115,673.784176416205,674.219049721412,674.653923026738,675.088796332185,
675.523669637755,675.95854294345,676.393416249271,676.82828955522,677.263162861298,
677.698036167508,678.13290947385,678.568635473934,679.004361474018,679.439234780629,
679.874108087377,680.308981394264,680.743854701289,681.178728008455,681.613601315762,
682.048474623211,682.483347930804,682.91822123854,683.353094546422,683.78796785445,
684.222841162623,684.657714470944,685.092587779412,685.528313780566,685.96403978172,
686.398913090483,686.833786399396,687.268659708457,687.703533017666,688.138406327025,
688.573279636532,689.008152946187,689.443026255992,689.877899565944,690.312772876043,
690.74764618629,691.182519496684,691.617392807224,692.052266117909,692.487992120169,
692.92371812243,693.358591433403,694.228338055774,694.663211367171,695.098084678707,
695.532957990379,695.967831302188,696.402704614131,696.837577926207,697.707324550749,
698.577071175797,699.011944488507,699.447670491767,699.883396495028,700.318269807975,
701.188016434211,702.057763060886,702.927509687976,703.797256315454,704.667002943295,
705.536749571467,706.407348889651,707.277948207973,708.147694836835,709.017441465911,
709.887188095163,710.756934724548,711.626681354026,712.496427983551,713.367027302543,
714.237626621516,715.107373250954,715.977119880277,716.846866509446,717.716613138419,
718.586359767161,719.456106395635,720.32670571363,721.197305031464,722.067051659126,
722.936798286414,723.806544913299,724.676291539758,725.546038165767,726.415784791305,
727.286384106969,728.156983422381,729.026730046663,729.896476670415,730.331349982088,
730.766223293624,731.201096605021,731.635969916278,732.505716538366,733.37546315988,
733.81033647042,734.246062472462,734.681788474505,735.116661784752,735.551535094852,
735.986408404804,736.421281714608,736.856155024264,737.291028333771,737.72590164313,
738.160774952339,738.5956482614,739.030521570312,739.465394879076,739.900268187692,
740.33514149616,740.77001480448,741.205740805414,741.641466806347,742.076340114374,
742.511213422256,742.946086729993,743.380960037585,743.815833345035,744.250706652341,
744.685579959507,745.120453266533,745.555326573419,745.990199880167,746.425073186778,
746.859946493254,747.294819799596,747.729693105806,748.165419105691,748.601145105576,
749.036018411525,749.470891717346,749.90576502304,750.34063832861,750.775511634057,
751.210384939384,751.645258244591,752.080131549682,752.515004854656,752.949878159518,
753.384751464269,753.81962476891,754.254498073445,754.689371377875,755.125097376885,
755.560823375895,755.995696680123,756.430569984253,756.865443288287,757.300316592228,
757.735189896079,758.170063199842,758.604936503519,759.039809807113,759.474683110627,
759.909556414062,760.344429717423,760.779303020711,761.214176323929,761.649049627079,
762.084775625469,762.520501623858,762.955374926883,763.390248229848,763.825121532758,
764.259994835614,764.694868138419,765.129741441178,765.564614743891,765.999488046563,
766.434361349196,766.869234651793,767.304107954357,767.738981256891,768.173854559398,
768.608727861881,769.044453859958,769.480179858035,769.915053160479,770.349926462907,
770.784799765324,771.219673067731,771.654546370133,772.089419672531,772.52429297493,
772.959166277331,773.394039579739,773.828912882155,774.263786184584,774.698659487028,
775.13353278949,775.568406091973,776.004132090072,776.439858088172,776.874731390706,
777.30960469327,777.744477995867,778.1793512985,778.614224601171,779.049097903885,
779.483971206643,779.918844509449,780.353717812305,780.788591115215,781.22346441818,
781.658337721205,782.093211024291,782.528084327442,782.963810325897,783.399536324352,
783.834409627639,784.269282931,784.704156234435,785.139029537949,785.573902841543,
786.00877614522,786.443649448983,786.878522752834,787.313396056775,787.74826936081,
788.183142664939,788.618015969167,789.052889273495,789.487762577925,789.923488577038,
790.359214576152,790.794087880793,791.228961185544,791.663834490406,792.098707795381,
792.533581100471,792.968454405678,793.403327711004,793.838201016451,794.273074322021,
794.707947627716,795.142820933537,795.577694239486,796.012567545564,796.447440851774,
796.883166851791,797.318892851808,797.753766158284,798.188639464895,798.623512771643,
799.058386078529,799.493259385555,799.92813269272,800.363006000027,800.797879307477,
801.232752615069,801.667625922806,802.102499230688,802.537372538715,802.972245846889,
803.40711915521,803.84284515629,804.27857115737,804.713444465985,805.148317774749,
805.583191083662,806.018064392723,806.452937701933,806.887811011291,807.322684320798,
808.192430940258,808.62730425021,809.06217756031,809.497050870557,809.931924180951,
810.36679749149,810.802523493679,811.238249495867,811.673122806697,812.542869428785,
812.977742740041,813.412616051438,813.847489362974,814.282362674646,814.717235986455,
815.152109298398,816.021855922681,816.891602547478,817.326475860065,817.762201863265,
818.197927866466,818.632801179295,819.502547805304,820.372294431763,821.242041058648,
822.111787685935,822.981534313598,823.851280941609,824.721880259681,825.5924795779,
826.462226206642,827.331972835616,828.201719464785,829.071466094109,829.941212723546,
830.810959353053,831.681558672047,832.552157991036,833.421904620514,834.2916512499,
835.161397879151,836.031144508226,836.900891137089,837.770637765701,838.641237083811,
839.511836401767,840.381583029608,841.251329657086,842.121076284176,842.990822910851,
843.860569537087,844.730316162863,845.600915478712,846.471514794314,847.341261418855,
848.211008042874,848.645881354683,849.080754666356,849.515627977891,849.950501289288,
850.82024791166,851.689994533462,852.124867844147,852.560593846263,852.996319848379,
853.431193158772,853.866066469019,854.300939779119,855.170686398875,855.605559708531,
856.040433018038,856.475306327397,856.910179636606,857.345052945667,857.77992625458,
858.214799563344,858.64967287196,859.084546180427,859.520272181434,859.95599818244,
860.390871490614,860.825744798641,861.260618106523,861.69549141426,862.130364721852,
862.565238029302,863.000111336609,863.434984643774,863.8698579508,864.304731257686,
864.739604564434,865.174477871045,865.609351177521,866.044224483863,866.479950483814,
866.915676483765,867.350549789843,867.785423095792,868.220296401613,868.655169707307,
869.090043012877,869.524916318325,869.959789623651,870.394662928858,870.829536233948,
871.264409538923,871.699282843785,872.134156148535,872.569029453177,873.003902757712,
873.439628756773,873.875354755834,874.310228060162,874.745101364389,875.179974668519,
875.614847972553,876.049721276495,876.484594580346,876.919467884108,877.354341187786,
877.78921449138,878.224087794893,878.658961098329,879.093834401689,879.528707704977,
879.963581008195,880.399307006616,880.835033005038,881.269906308124,881.704779611148,
882.139652914114,882.574526217024,883.00939951988,883.444272822685,883.879146125444,
884.314019428157,884.748892730829,885.183766033462,885.618639336059,886.053512638623,
886.488385941157,886.923259243664,887.358985241751,887.794711239839,888.2295845423,
888.664457844744,889.099331147173,889.534204449589,889.969077751997,890.403951054398,
890.838824356797,891.273697659195,891.708570961597,892.143444264004,892.578317566421,
893.01319086885,893.448064171293,893.882937473755,894.318663471843,894.75438946993,
895.189262772437,895.624136074971,896.059009377535,896.493882680132,896.928755982765,
897.363629285437,897.798502588151,898.233375890909,898.668249193715,899.103122496571,
899.53799579948,899.972869102446,900.40774240547,900.842615708556,901.278341706978,
901.714067705399,902.148941008617,902.583814311905,903.018687615265,903.453560918701,
903.888434222214,904.323307525808,904.758180829485,905.193054133248,905.627927437099,
906.06280074104,906.497674045075,906.932547349205,907.367420653433,907.80229395776,
908.238019956821,908.673745955883,909.108619260417,909.543492565059,909.978365869809,
910.413239174671,910.848112479646,911.282985784736,911.717859089943,912.152732395269,
912.587605700716,913.022479006287,913.457352311981,913.892225617802,914.327098923751,
914.761972229829,915.19769822978,915.633424229731,916.068297536072,916.503170842548,
916.93804414916,917.372917455908,917.807790762794,918.24266406982,918.677537376985,
919.112410684292,919.547283991742,919.982157299334,920.417030607071,920.851903914953,
921.28677722298,921.721650531154,922.15737653216,922.593102533167,923.027975841635,
923.46284915025,923.897722459014,924.332595767926,924.767469076987,925.202342386197,
925.637215695556,926.072089005063,926.506962314719,926.941835624523,927.376708934475,
927.811582244575,928.246455554822,928.681328865215,929.117054867331,929.987654180132,
930.422527490961,930.857400801934,931.292274113049,931.727147424306,932.162020735703,
932.596894047238,933.46664067072,934.336387294739,934.771260606945,935.20613391928,
935.641007231742,936.076733234882,936.94733255073,937.817079176507,938.686825802743,
939.556572429418,940.426319056508,941.296065683986,942.165812311827,943.036411629783,
943.907010947893,944.776757576505,945.646504205367,946.516250834443,947.385997463694,
948.25574409308,949.125490722558,949.996090041546,950.86668936054,951.736435990048,
952.606182619485,953.475929248809,954.345675877978,955.215422506951,956.085169135693,
956.955768453912,957.826367771985,958.696114399995,959.565861027658,960.435607654946,
961.305354281831,962.175100908289,963.044847534298,963.915446850328,964.786046166116,
965.655792790913,966.525539415195,966.960412727138,967.395286038947,968.265032662155,
969.134779284809,969.569652595924,970.004525906897,970.439399217726,970.875125219914,
971.310851222103,971.745724532643,972.615471153283,973.485217773335,973.920091083139,
974.354964392795,974.789837702302,975.22471101166,975.65958432087,976.094457629931,
976.529330938844,976.964204247608,977.399077556223,977.834803557303,978.270529558383,
978.705402866704,979.140276174877,979.575149482905,980.010022790786,980.444896098523,
980.879769406116,981.314642713565,981.749516020872,982.184389328038,982.619262635063,
983.05413594195,983.489009248698,983.923882555309,984.358755861785,984.794481861802,
985.230207861819,985.665081168029,986.099954474107,986.534827780056,986.969701085877,
987.404574391571,987.839447697141,988.274321002589,988.709194307915,989.144067613122,
989.578940918212,990.013814223187,990.448687528048,990.883560832799,991.31843413744,
991.754160136554,992.189886135667,992.624759440097,993.059632744425,993.494506048653,
993.929379352783,994.364252656817,994.799125960758,995.233999264609,995.668872568372,
996.103745872049,996.538619175643,996.973492479157,997.408365782593,997.843239085953,
998.278112389241,998.713838387696,999.149564386151,999.584437689301,1000.01931099239,
1000.45418429541,1000.88905759838,1001.32393090129,1001.75880420414,1002.19367750695,
1002.62855080971,1003.06342411242,1003.49829741509,1003.93317071773,1004.36804402032,
1004.80291732289,1005.23779062542,1005.67351662352,1006.10924262162,1006.5441159241,
1006.97898922656,1007.41386252901,1007.84873583144,1008.28360913385,1008.71848243626,
1009.15335573866,1009.58822904106,1010.02310234346,1010.45797564586,1010.89284894827,
1011.32772225069,1011.76259555311,1012.19746885556,1012.63319485364,1013.06892085171,
1013.5037941542,1013.9386674567,1014.37354075924,1014.8084140618,1015.2432873644,
1015.67816066703,1016.1130339697,1016.54790727242,1016.98278057517,1017.41765387798,
1017.85252718084,1018.28740048375,1018.72227378671,1019.15714708974,1019.59287308813,
1020.02859908651,1020.46347238967,1020.89834569288,1021.33321899617,1021.76809229953,
1022.20296560297,1022.63783890648,1023.07271221007,1023.50758551375,1023.94245881752,
1024.37733212137,1024.81220542531,1025.24707872935,1025.68195203348,1026.11682533771,
1026.55255133672,1026.98827733573,1027.42315064016,1027.8580239447,1028.29289724934,
1028.72777055409,1029.16264385896,1029.59751716393,1030.03239046902,1030.46726377423,
1030.90213707956,1031.33701038501,1031.77188369058,1032.20675699628,1032.6416303021,
1033.07650360805,1033.51222960793,1033.94795560782,1034.38282891403,1034.81770222038,
1035.25257552685,1035.68744883347,1036.12232214022,1036.5571954471,1036.99206875413,
1037.4269420613,1037.86181536861,1038.29668867606,1038.73156198365,1039.16643529139,
1039.60130859927,1040.0361819073,1040.47190790824,1040.90763390917,1041.34250721749,
1041.77738052596,1042.21225383458,1042.64712714334,1043.08200045226,1043.95174707053,
1044.38662037989,1044.8214936894,1045.25636699906,1045.69124030886,1046.12611361882,
1046.56098692892,1046.99586023917,1047.43158624121,1047.86731224325,1048.3021855538,
1048.73705886448,1049.17193217531,1049.60680548629,1050.0416787974,1050.47655210866,
1050.91142542006,1051.78117204327,1052.21604535508,1052.65091866703,1053.0857919791,
1053.52066529131,1053.95553860365,1054.39126460673,1055.26186392239,1056.13161054793,
1057.00135717395,1057.43623048712,1057.87110380041,1058.7408504273,1059.61059705459,
1060.48034368225,1061.35094300009,1062.22154231809,1063.09128894656,1063.96103557531,
1064.83078220429,1065.70052883346,1066.57027546278,1067.44002209222,1068.3106214112,
1069.18122073019,1070.05096735972,1070.9207139892,1071.79046061859,1072.66020724785,
1073.52995387693,1074.39970050579,1075.27029982411,1076.1408991423,1077.01064577048,
1077.88039239832,1078.7501390258,1079.61988565289,1080.48963227957,1081.35937890581,
1082.22997822202,1083.100577538,1083.97032416305,1084.84007078759,1085.70981741161,
1086.5795640351,1087.44931065803,1087.88418396929,1088.31905728041,1088.75393059138,
1089.18965659365,1089.62538259591,1090.06025590659,1090.93000252753,1091.36487583778,
1091.79974914788,1092.23462245783,1092.66949576764,1093.1043690773,1093.5392423868,
1093.97411569616,1094.40898900538,1094.84386231444,1095.27873562335,1095.71360893212,
1096.14933493327,1096.58506093443,1097.0199342429,1097.45480755122,1097.88968085939,
1098.32455416742,1098.75942747531,1099.19430078305,1099.62917409064,1100.06404739809,
1100.4989207054,1100.93379401257,1101.36866731959,1101.80354062648,1102.23841393323,
1102.67328723984,1103.10901323993,1103.54473924001,1103.97961254636,1104.41448585257,
1104.84935915865,1105.2842324646,1105.71910577042,1106.15397907612,1106.58885238169,
1107.02372568714,1107.45859899246,1107.89347229767,1108.32834560276,1108.76321890774,
1109.1980922126,1109.63296551736,1110.06869151652,1110.50441751569,1110.93929082023,
1111.37416412466,1111.80903742899,1112.24391073322,1112.67878403735,1113.11365734139,
1113.54853064533,1113.98340394918,1114.41827725295,1114.85315055662,1115.28802386022,
1115.72289716374,1116.15777046717,1116.59264377053,1117.02836976903,1117.46409576752,
1117.89896907074,1118.33384237389,1118.76871567698,1119.20358898,1119.63846228297,
1120.07333558588,1120.50820888874,1120.94308219154,1121.3779554943,1121.81282879702,
1122.24770209969,1122.68257540233,1123.11744870492,1123.55232200749,1123.98804800561,
1124.42377400372,1124.85864730623,1125.29352060871,1125.72839391118,1126.16326721362,
1126.59814051605,1127.03301381847,1127.46788712088,1127.90276042328,1128.33763372568,
1128.77250702808,1129.20738033048,1129.64225363289,1130.07712693531,1130.51200023774,
1130.94772623581,1131.38345223388,1131.81832553634,1132.25319883883,1132.68807214134,
1133.12294544387,1133.55781874644,1133.99269204904,1134.42756535167,1134.86243865434,
1135.29731195706,1135.73218525982,1136.16705856263,1136.60193186548,1137.03680516839,
1137.47167847136,1137.90740446972,1138.34313046808,1138.77800377117,1139.21287707432,
1139.64775037754,1140.08262368083,1140.51749698419,1140.95237028763,1141.38724359114,
1141.82211689474,1142.25699019842,1142.69186350218,1143.12673680603,1143.56161010998,
1143.99648341401,1144.43135671814,1144.86708271711,1145.30280871607,1145.7376820204,
1146.17255532483,1146.60742862936,1147.04230193401,1147.47717523876,1147.91204854362,
1148.3469218486,1148.78179515369,1149.2166684589,1149.65154176423,1150.08641506968,
1150.52128837525,1150.95616168094,1151.39103498677,1151.82676098659,1152.26248698641,
1152.69736029249,1153.1322335987,1153.56710690504,1154.00198021152,1154.43685351813,
1154.87172682488,1155.30660013177,1155.7414734388,1156.17634674597,1156.61122005327,
1157.04609336073,1157.48096666832,1157.91583997606,1158.35071328394,1158.7864392848,
1159.22216528566,1159.65703859384,1160.09191190216,1160.52678521063,1160.96165851925,
1161.39653182801,1161.83140513693,1162.26627844599,1162.7011517552,1163.13602506456,
1163.57089837407,1164.00577168373,1164.44064499353,1164.87551830349,1165.74611761556,
1166.18184361753,1166.61671692792,1167.05159023846,1167.48646354915,1167.92133685998,
1168.35621017096,1169.22595679333,1170.09570341627,1170.53057672794,1170.96545003975,
1171.4003233517,1171.83519666377,1172.27006997598,1172.705795979,1173.57639529447,
1174.44614191977,1174.8810152326,1175.31588854555,1176.18563517179,1177.05538179847,
1177.92512842556,1178.79487505304,1179.66547437075,1180.53607368863,1181.40582031696,
1182.27556694557,1183.14531357444,1184.01506020352,1184.88480683277,1185.75455346216,
1186.62515278112,1187.4957521001,1188.36549872963,1189.23524535914,1190.10499198858,
1190.97473861791,1191.84448524708,1192.71423187606,1193.58483119448,1194.45543051277,
1195.3251771411,1196.19492376911,1197.06467039678,1197.93441702407,1198.80416365096,
1199.67391027742,1200.5445095938,1201.41510890996,1202.28485553525,1203.15460216005,
1204.02434878434,1204.89409540809,1205.76384203131,1206.1987153427,1206.63358865396,
1207.06846196508,1207.50418796741,1208.37478728058,1209.2445339018,1209.6794072122,
1210.11428052245,1210.54915383255,1210.9840271425,1211.41890045231,1211.85377376197,
1212.28864707147,1212.72352038083,1213.15839369005,1213.59326699911,1214.02814030802,
1214.46386630925,1214.89959231048,1215.3344656191,1215.76933892757,1216.20421223589,
1216.63908554406,1217.07395885209,1217.50883215998,1217.94370546771,1218.37857877531,
1218.81345208276,1219.24832539007,1219.68319869724,1220.11807200426,1220.55294531115,
1220.9878186179,1221.42354461805,1221.85927061821,1222.29414392468,1222.72901723103,
1223.16389053724,1223.59876384332,1224.03363714927,1224.46851045509,1224.90338376079,
1225.33825706636,1225.77313037181,1226.20800367713,1226.64287698234,1227.07775028743,
1227.51262359241,1227.94749689727,1228.3832228965,1228.81894889572,1229.25382220036,
1229.6886955049,1230.12356880933,1230.55844211366,1230.99331541789,1231.42818872202,
1231.86306202606,1232.29793533,1232.73280863385,1233.16768193762,1233.60255524129,
1234.03742854489,1234.4723018484,1234.90717515184,1235.34290115037,1235.7786271489,
1236.21350045219,1236.64837375541,1237.08324705856,1237.51812036165,1237.95299366467,
1238.38786696764,1238.82274027055,1239.25761357341,1239.69248687621,1240.12736017897,
1240.56223348169,1240.99710678436,1241.431980087,1241.8668533896,1242.30257938773,
1242.73830538585,1243.17317868839,1243.6080519909,1244.04292529338,1244.47779859585,
1244.91267189829,1245.34754520072,1245.78241850314,1246.21729180555,1246.65216510795,
1247.08703841035,1247.52191171275,1247.95678501515,1248.39165831756,1248.82653161998,
1249.26225761804,1249.69798361611,1250.13285691855,1250.56773022101,1251.0026035235,
1251.43747682601,1251.87235012854,1252.30722343111,1252.74209673371,1253.17697003634,
1253.61184333901,1254.04671664173,1254.48158994449,1254.9164632473,1255.35133655015,
1255.78620985306,1256.22193585139,1256.65766184973,1257.09253515275,1257.52740845584,
1257.96228175899,1258.39715506221,1258.8320283655,1259.26690166886,1259.7017749723,
1260.13664827581,1260.57152157941,1261.00639488309,1261.44126818685,1261.8761414907,
1262.31101479465,1262.74588809868,1263.1816140976,1263.61734009651,1264.05221340074,
1264.48708670507,1264.9219600095,1265.35683331403,1265.79170661868,1266.22657992343,
1266.66145322829,1267.09632653327,1267.53119983836,1267.96607314357,1268.4009464489,
1268.83581975434,1269.27069305992,1269.70556636561,1270.14129236537,1270.57701836513,
1271.01189167108,1271.44676497716,1271.88163828337,1272.31651158971,1272.75138489619,
1273.1862582028,1273.62113150955,1274.05600481644,1274.49087812347,1274.92575143063,
1275.36062473794,1275.79549804539,1276.23037135299,1276.66524466073,1277.10097066151,
1277.5366966623,1277.97156997033,1278.40644327851,1278.84131658683,1279.2761898953,
1279.71106320392,1280.14593651268,1280.5808098216,1281.01568313066,1281.45055643987,
1281.88542974923,1282.32030305874,1282.75517636839,1283.1900496782,1283.62492298815,
1284.06064899005,1284.49637499195,1284.9312483022,1285.36612161259,1285.80099492313,
1286.23586823382,1286.67074154465,1287.54048816674,1287.975361478,1288.4102347894,
1288.84510810093,1289.27998141261,1289.71485472442,1290.14972803636,1291.02032735139,
1291.89092666668,1292.32579997914,1292.76067329173,1293.19554660444,1293.63041991727,
1294.50016654328,1295.36991316974,1296.23965979663,1297.10940642392,1297.9800057415,
1298.85060505925,1299.72035168742,1300.5900983159,1301.45984494464,1302.32959157362,
1303.19933820279,1304.06908483212,1304.93968415104,1305.81028347,1306.68003009953,
1307.54977672906,1308.41952335854,1309.28926998793,1310.15901661718,1311.02876324626,
1311.89936256477,1312.76996188316,1313.63970851164,1314.50945513981,1315.37920176765,
1316.24894839514,1317.11869502223,1317.98844164891,1318.85904096546,1319.72964028179,
1320.59938690733,1321.46913353238,1322.33888015692,1323.20862678095,1323.64350009276,
1324.07837340443,1324.51324671597,1324.94812002737,1325.81871934103,1326.68931865441,
1327.12419196524,1327.55906527593,1327.99393858647,1328.42881189686,1328.86368520711,
1329.29855851721,1329.73343182716,1330.16830513697,1330.60317844663,1331.03805175614,
1331.4729250655,1331.90779837471,1332.34267168377,1332.77839768507,1333.21412368638,
1333.64899699514,1334.08387030376,1334.51874361223,1334.95361692055,1335.38849022873,
1335.82336353676,1336.25823684464,1336.69311015238,1337.12798345997,1337.56285676742,
1337.99773007473,1338.4326033819,1338.86747668892,1339.30234999581,1339.73807599603,
1340.17380199625,1340.60867530287,1341.04354860934,1341.47842191569,1341.9132952219,
1342.34816852798,1342.78304183393,1343.21791513975,1343.65278844545,1344.08766175102,
1344.52253505647,1344.95740836179,1345.392281667,1345.82715497209,1346.26202827707,
1346.69775427635,1347.13348027563,1347.56835358038,1348.00322688502,1348.43810018956,
1348.87297349399,1349.30784679832,1349.74272010255,1350.17759340668,1350.61246671072,
1351.04734001466,1351.48221331851,1351.91708662228,1352.35195992595,1352.78683322955,
1353.22170653306,1353.65743253163,1354.09315853019,1354.52803183356,1354.96290513685,
1355.39777844007,1355.83265174322,1356.26752504631,1356.70239834933,1357.1372716523,
1357.57214495521,1358.00701825807,1358.44189156087,1358.87676486363,1359.31163816635,
1359.74651146902,1360.18138477166,1360.6171107698,1361.05283676795,1361.48771007051,
1361.92258337305,1362.35745667556,1362.79232997804,1363.2272032805,1363.66207658295,
1364.09694988538,1364.5318231878,1364.96669649021,1365.40156979261,1365.83644309501,
1366.27131639741,1366.70618969981,1367.14106300222,1367.57678900028,1368.01251499834,
1368.44738830077,1368.88226160321,1369.31713490567,1369.75200820816,1370.18688151067,
1370.6217548132,1371.05662811577,1371.49150141837,1371.926374721,1372.36124802367,
1372.79612132639,1373.23099462915,1373.66586793196,1374.10074123481,1374.53646723311,
1374.97219323142,1375.40706653438,1375.84193983741,1376.2768131405,1376.71168644365,
1377.14655974687,1377.58143305016,1378.01630635352,1378.45117965696,1378.88605296047,
1379.32092626407,1379.75579956775,1380.19067287151,1380.62554617536,1381.06041947931,
1381.49614547817,1381.93187147704,1382.36674478117,1382.8016180854,1383.23649138973,
1383.67136469416,1384.10623799869,1384.54111130334,1384.97598460809,1385.41085791295,
1385.84573121793,1386.28060452302,1386.71547782823,1387.15035113356,1387.585224439,
1388.02009774458,1388.45582374427,1388.89154974397,1389.32642304979,1389.76129635574,
1390.19616966182,1390.63104296803,1391.06591627437,1391.50078958085,1391.93566288746,
1392.37053619421,1392.8054095011,1393.24028280813,1393.6751561153,1394.1100294226,
1394.54490273005,1394.97977603765,1395.41550203836,1395.85122803908,1396.28610134696,
1396.72097465499,1397.15584796317,1397.59072127149,1398.02559457996,1398.46046788858,
1398.89534119734,1399.33021450626,1399.76508781532,1400.19996112453,1400.63483443389,
1401.50458105306,1401.93945436286,1402.37518036469,1402.81090636651,1403.24577967661,
1403.68065298686,1404.11552629725,1404.5503996078,1404.98527291848,1405.85501954029,
1406.2898928514,1406.72476616266,1407.15963947406,1407.5945127856,1408.02938609727,
1408.46425940908,1409.33485872391,1410.205458039,1410.64033135134,1411.07520466381,
1411.51007797639,1411.9449512891,1412.81469791488,1413.68444454112,1414.5541911678,
1415.42393779489,1416.29453711233,1417.16513642995,1418.03488305796,1418.90462968629,
1419.77437631491,1420.64412294377,1421.51386957285,1422.38361620211,1423.25421552099,
1424.12481483992,1424.99456146943,1425.86430809896,1426.73405472847,1427.60380135791,
1428.47354798724,1429.34329461641,1430.21389393501,1431.08449325349,1431.9542398821,
1432.82398651043,1433.69373313844,1434.56347976611,1435.4332263934,1436.30297302029,
1437.17357233701,1438.04417165351,1438.91391827929,1439.78366490459,1440.65341152939,
1441.52315815367,1441.95803146562,1442.39290477743,1442.8277780891,1443.26265140064,
1444.13325071451,1445.00385002811,1445.43872333908,1445.87359664991,1446.3084699606,
1446.74334327114,1447.17821658153,1447.61308989178,1448.48283651184,1448.91770982164,
1449.3525831313,1449.78745644081,1450.22232975017,1450.65720305938,1451.09292906076,
1451.52865506214,1451.96352837105,1452.39840167982,1452.83327498843,1453.2681482969,
1453.70302160522,1454.1378949134,1454.57276822143,1455.00764152931,1455.44251483705,
1455.87738814464,1456.31226145209,1456.7471347594,1457.18200806657,1457.6168813736,
1458.05260737389,1458.48833337418,1458.92320668093,1459.35807998754,1459.79295329402,
1460.22782660036,1460.66269990657,1461.09757321265,1461.5324465186,1461.96731982443,
1462.40219313012,1462.83706643569,1463.27193974114,1463.70681304647,1464.14168635168,
1464.57655965677,1465.0122856561,1465.44801165544,1465.8828849603,1466.31775826505,
1466.7526315697,1467.18750487423,1467.62237817866,1468.05725148299,1468.49212478722,
1468.92699809135,1469.36187139539,1469.79674469933,1470.23161800319,1470.66649130695,
1471.10136461063,1471.53623791422,1471.97196391283,1472.40768991143,1472.84256321487,
1473.27743651823,1473.71230982152,1474.14718312474,1474.58205642789,1475.01692973098,
1475.451803034,1475.88667633697,1476.32154963988,1476.75642294274,1477.19129624555,
1477.62616954831,1478.06104285102,1478.4959161537,1478.93164215186,1479.36736815002,
1479.80224145262,1480.23711475519,1480.67198805772,1481.10686136023,1481.54173466272,
1481.97660796518,1482.41148126762,1482.84635457005,1483.28122787247,1483.71610117488,
1484.15097447728,1484.58584777968,1485.02072108208,1485.45559438449,1485.89132038254,
1486.32704638059,1486.76191968301,1487.19679298544,1487.63166628788,1488.06653959035,
1488.50141289283,1488.93628619534,1489.37115949787,1489.80603280044,1490.24090610304,
1490.67577940567,1491.11065270835,1491.54552601106,1491.98039931382,1492.41527261663,
1492.8509986149,1493.28672461318,1493.72159791609,1494.15647121906,1494.59134452208,
1495.02621782517,1495.46109112832,1495.89596443154,1496.33083773483,1496.76571103819,
1497.20058434163,1497.63545764515,1498.07033094874,1498.50520425242,1498.94007755618,
1499.37495086004,1499.81067685885,1500.24640285767,1500.68127616171,1501.11614946584,
1501.55102277007,1501.9858960744,1502.42076937883,1502.85564268337,1503.29051598801,
1503.72538929276,1504.16026259762,1504.5951359026,1505.03000920769,1505.4648825129,
1505.89975581823,1506.33462912368,1506.77035512331,1507.20608112294,1507.64095442864,
1508.07582773446,1508.51070104041,1508.94557434649,1509.3804476527,1509.81532095904,
1510.25019426552,1510.68506757213,1511.11994087888,1511.55481418577,1511.9896874928,
1512.42456079996,1512.85943410727,1513.29430741472,1513.73003341537,1514.16575941601,
1514.60063272375,1515.03550603163,1515.47037933966,1515.90525264784,1516.34012595616,
1516.77499926463,1517.20987257325,1517.64474588201,1518.07961919093,1518.51449249999,
1518.9493658092,1519.38423911856,1519.81911242807,1520.25398573772,1520.68971173947,
1521.12543774122,1521.56031105118,1521.99518436128,1522.43005767153,1523.29980429246,
1523.73467760315,1524.16955091398,1524.60442422495,1525.03929753607,1525.47417084733,
1525.90904415873,1526.77879078194,1527.64939009657,1528.08511609939,1528.51998941146,
1528.95486272367,1529.38973603601,1530.25948266106,1531.1292292866,1531.99897591261,
1532.86872253907,1533.73846916596,1534.60906848325,1535.47966780073,1536.34941442858,
1537.21916105675,1538.08890768523,1538.95865431398,1539.82840094295,1540.69814757212,
1541.56874689096,1542.43934620985,1543.30909283933,1544.17883946886,1545.04858609839,
1545.91833272787,1546.78807935726,1547.65782598651,1548.52842530518,1549.39902462375,
1550.26877125249,1551.13851788097,1552.00826450914,1552.87801113699,1553.74775776447,
1554.61750439156,1555.48810370844,1556.35870302511,1557.22844965112,1558.09819627666,
1558.96794290171,1559.83768952626,1560.27256283834,1560.70743615028,1561.57718277377,
1562.44778208785,1563.31838140165,1563.75325471277,1564.18812802374,1564.62300133457,
1565.05787464526,1565.9276212662,1566.79736788655,1567.2322411965,1567.66711450631,
1568.10198781596,1568.53686112547,1568.97173443483,1569.40746043628,1569.84318643774,
1570.2780597468,1570.71293305571,1571.14780636448,1571.5826796731,1572.01755298157,
1572.45242628989,1572.88729959806,1573.32217290609,1573.75704621397,1574.19191952171,
1574.62679282931,1575.06166613676,1575.49653944407,1575.93141275123,1576.36713875159,
1576.80286475195,1577.23773805884,1577.67261136559,1578.1074846722,1578.54235797868,
1578.97723128502,1579.41210459124,1579.84697789732,1580.28185120327,1580.71672450909,
1581.15159781478,1581.58647112036,1582.0213444258,1582.45621773113,1582.89109103634,
1583.32681703573,1583.76254303513,1584.1974163401,1584.63228964497,1585.06716294972,
1585.50203625436,1585.9369095589,1586.37178286333,1586.80665616766,1587.24152947189,
1587.67640277602,1588.11127608005,1588.546149384,1588.98102268785,1589.41589599161,
1589.85076929529,1590.28649529394,1590.72222129258,1591.1570945961,1591.59196789953,
1592.0268412029,1592.46171450619,1592.8965878094,1593.33146111256,1593.76633441564,
1594.20120771867,1594.63608102164,1595.07095432455,1595.50582762741,1595.94070093021,
1596.37557423297,1596.81044753569,1597.24617353387,1597.68189953206,1598.11677283469,
1598.55164613729,1598.98651943985,1599.42139274239,1599.8562660449,1600.29113934738,
1600.72601264985,1601.16088595229,1601.59575925472,1602.03063255714,1602.46550585955,
1602.90037916195,1603.33525246435,1603.77012576675,1604.2058517648,1604.64157776285,
1605.07645106526,1605.51132436768,1605.94619767011,1606.38107097255,1606.81594427502,
1607.2508175775,1607.68569088001,1608.12056418254,1608.55543748511,1608.99031078771,
1609.42518409034,1609.86005739302,1610.29493069573,1610.72980399849,1611.16552999674,
1611.60125599499,1612.03612929785,1612.47100260076,1612.90587590373,1613.34074920675,
1613.77562250984,1614.21049581299,1614.64536911621,1615.0802424195,1615.51511572286,
1615.9499890263,1616.38486232981,1616.81973563341,1617.25460893709,1617.68948224085,
1618.12520823963,1618.5609342384,1618.99580754234,1619.43068084638,1619.86555415051,
1620.30042745474,1620.73530075907,1621.1701740635,1621.60504736804,1622.03992067268,
1622.47479397743,1622.90966728229,1623.34454058727,1623.77941389236,1624.21428719757,
1624.6491605029,1625.08488650247,1625.52061250204,1625.95548580761,1626.39035911331,
1626.82523241913,1627.26010572508,1627.69497903116,1628.12985233737,1628.56472564372,
1628.99959895019,1629.43447225681,1629.86934556356,1630.30421887044,1630.73909217747,
1631.17396548464,1631.60883879195,1632.04456479252,1632.48029079309,1632.91516410068,
1633.35003740842,1633.78491071631,1634.21978402433,1634.65465733251,1635.08953064083,
1635.5244039493,1635.95927725792,1636.39415056668,1636.8290238756,1637.26389718466,
1637.69877049387,1638.13364380323,1638.56851711274,1639.00424311442,1639.43996911609,
1639.8748424259,1640.30971573585,1640.74458904595,1641.6143356666,1642.04920897714,
1642.48408228782,1642.91895559865,1643.35382890963,1643.78870222074,1644.223575532,
1645.09332215494,1645.52819546661,1645.96392146936,1646.39964747212,1646.83452078406,
1647.26939409614,1647.70426740834,1648.57401403314,1649.44376065844,1650.31350728422,
1650.74838059729,1651.18325391046,1652.05300053714,1652.92359985428,1653.79419917162,
1654.66394579929,1655.5336924273,1656.40343905563,1657.27318568424,1658.14293231311,
1659.01267894219,1659.88327826096,1660.75387757982,1661.62362420926,1662.49337083877,
1663.3631174683,1664.23286409781,1665.10261072725,1665.97235735658,1666.84295667531,
1667.71355599396,1668.58330262282,1669.45304925143,1670.32279587976,1671.19254250778,
1672.06228913544,1672.93203576273,1673.80263507977,1674.6732343966,1675.54298102284,
1676.41272764862,1677.28247427392,1678.15222089872,1679.021967523,1679.89171414676,
1680.76231346105,1681.19803946366,1681.63291277506,1682.06778608632,1682.50265939743,
1682.93753270841,1683.37240601924,1684.24215264047,1684.67702595086,1685.11189926111,
1685.54677257121,1685.98164588116,1686.41651919097,1686.85139250063,1687.28626581014,
1687.72199181166,1688.15771781319,1688.5925911224,1689.02746443146,1689.46233774038,
1689.89721104914,1690.33208435776,1690.76695766623,1691.20183097455,1691.63670428272,
1692.07157759075,1692.50645089864,1692.94132420637,1693.37619751397,1693.81107082142,
1694.24594412873,1694.68167012916,1695.11739612959,1695.55226943662,1695.9871427435,
1696.42201605025,1696.85688935687,1697.29176266334,1697.72663596969,1698.1615092759,
1698.59638258198,1699.03125588793,1699.46612919375,1699.90100249945,1700.33587580502,
1700.77074911047,1701.20562241579,1701.64134841525,1702.0770744147,1702.51194771979,
1702.94682102476,1703.38169432963,1703.81656763438,1704.25144093902,1704.68631424356,
1705.12118754799,1705.55606085232,1705.99093415655,1706.42580746068,1706.86068076471,
1707.29555406866,1707.73042737251,1708.16530067627,1708.60102667496,1709.03675267365,
1709.47162597724,1709.90649928076,1710.34137258419,1710.77624588756,1711.21111919085,
1711.64599249406,1712.08086579722,1712.5157391003,1712.95061240333,1713.3854857063,
1713.82035900921,1714.25523231207,1714.69010561487,1715.12497891763,1715.56070491584,
1715.99643091404,1716.43130421671,1716.86617751935,1717.30105082195,1717.73592412451,
1718.17079742705,1718.60567072956,1719.04054403204,1719.4754173345,1719.91029063695,
1720.34516393938,1720.7800372418,1721.21491054421,1721.64978384661,1722.08465714901,
1722.52038314706,1722.9561091451,1723.39098244751,1723.82585574992,1724.26072905233,
1724.69560235476,1725.13047565721,1725.56534895967,1726.00022226216,1726.43509556467,
1726.8699688672,1727.30484216977,1727.73971547236,1728.174588775,1728.60946207767,
1729.04433538039,1729.48006137861,1729.91578737684,1730.35066067965,1730.78553398251,
1731.22040728542,1731.65528058838,1732.09015389141,1732.5250271945,1732.95990049765,
1733.39477380087,1733.82964710416,1734.26452040752,1734.69939371096,1735.13426701447,
1735.56914031807,1736.00401362175,1736.43973962048,1736.8754656192,1737.31033892306,
1737.745212227,1738.18008553104,1738.61495883517,1739.0498321394,1739.48470544373,
1739.91957874816,1740.35445205269,1740.78932535734,1741.22419866209,1741.65907196695,
1742.09394527193,1742.52881857702,1742.96369188223,1743.39941788174,1743.83514388125,
1744.2700171867,1744.70489049227,1745.13976379797,1745.57463710379,1746.00951040974,
1746.44438371582,1746.87925702203,1747.31413032837,1747.74900363485,1748.18387694146,
1748.61875024821,1749.0536235551,1749.48849686213,1749.92337016929,1750.3590961698,
1750.7948221703,1751.22969547775,1751.66456878534,1752.09944209308,1752.53431540096,
1752.96918870899,1753.40406201717,1753.83893532549,1754.27380863396,1754.70868194258,
1755.14355525134,1755.57842856026,1756.01330186932,1756.44817517853,1756.88304848789,
1757.31877448949,1757.75450049109,1758.18937380075,1759.05912042051,1759.49399373061,
1759.92886704086,1760.36374035125,1760.79861366179,1761.23348697248,1761.66836028331,
1762.10323359429,1762.5381069054,1763.40785352806,1763.8427268396,1764.27845284228,
1764.71417884496,1765.14905215677,1765.58392546872,1766.0187987808,1766.88854540534,
1767.75829203039,1768.1931653431,1768.62803865593,1769.06291196888,1769.49778528195,
1770.36753190841,1771.2381312254,1772.10873054259,1772.97847717007,1773.84822379791,
1774.71797042609,1775.58771705456,1776.45746368331,1777.32721031228,1778.19780963089,
1779.06840894783,1779.93815555508,1780.80790201176,1781.67764871408),(-1.76619037896906,
-1.18309518948453),.UNSPECIFIED.) ;
#826=B_SPLINE_SURFACE_WITH_KNOTS('',3,1,((#72010,#72011),(#72012,#72013),
(#72014,#72015),(#72016,#72017),(#72018,#72019),(#72020,#72021),(#72022,
#72023),(#72024,#72025),(#72026,#72027),(#72028,#72029),(#72030,#72031),
(#72032,#72033),(#72034,#72035),(#72036,#72037),(#72038,#72039),(#72040,
#72041),(#72042,#72043),(#72044,#72045),(#72046,#72047),(#72048,#72049),
(#72050,#72051),(#72052,#72053),(#72054,#72055),(#72056,#72057),(#72058,
#72059),(#72060,#72061),(#72062,#72063),(#72064,#72065),(#72066,#72067),
(#72068,#72069),(#72070,#72071),(#72072,#72073),(#72074,#72075),(#72076,
#72077),(#72078,#72079),(#72080,#72081),(#72082,#72083),(#72084,#72085),
(#72086,#72087),(#72088,#72089),(#72090,#72091),(#72092,#72093),(#72094,
#72095),(#72096,#72097),(#72098,#72099),(#72100,#72101),(#72102,#72103),
(#72104,#72105),(#72106,#72107),(#72108,#72109),(#72110,#72111),(#72112,
#72113),(#72114,#72115),(#72116,#72117),(#72118,#72119),(#72120,#72121),
(#72122,#72123),(#72124,#72125),(#72126,#72127),(#72128,#72129),(#72130,
#72131),(#72132,#72133),(#72134,#72135),(#72136,#72137),(#72138,#72139),
(#72140,#72141),(#72142,#72143),(#72144,#72145),(#72146,#72147),(#72148,
#72149),(#72150,#72151),(#72152,#72153),(#72154,#72155),(#72156,#72157),
(#72158,#72159),(#72160,#72161),(#72162,#72163),(#72164,#72165),(#72166,
#72167),(#72168,#72169),(#72170,#72171),(#72172,#72173),(#72174,#72175),
(#72176,#72177),(#72178,#72179),(#72180,#72181),(#72182,#72183),(#72184,
#72185),(#72186,#72187),(#72188,#72189),(#72190,#72191),(#72192,#72193),
(#72194,#72195),(#72196,#72197),(#72198,#72199),(#72200,#72201),(#72202,
#72203),(#72204,#72205),(#72206,#72207),(#72208,#72209),(#72210,#72211),
(#72212,#72213),(#72214,#72215),(#72216,#72217),(#72218,#72219),(#72220,
#72221),(#72222,#72223),(#72224,#72225),(#72226,#72227),(#72228,#72229),
(#72230,#72231),(#72232,#72233),(#72234,#72235),(#72236,#72237),(#72238,
#72239),(#72240,#72241),(#72242,#72243),(#72244,#72245),(#72246,#72247),
(#72248,#72249),(#72250,#72251),(#72252,#72253),(#72254,#72255),(#72256,
#72257),(#72258,#72259),(#72260,#72261),(#72262,#72263),(#72264,#72265),
(#72266,#72267),(#72268,#72269),(#72270,#72271),(#72272,#72273),(#72274,
#72275),(#72276,#72277),(#72278,#72279),(#72280,#72281),(#72282,#72283),
(#72284,#72285),(#72286,#72287),(#72288,#72289),(#72290,#72291),(#72292,
#72293),(#72294,#72295),(#72296,#72297),(#72298,#72299),(#72300,#72301),
(#72302,#72303),(#72304,#72305),(#72306,#72307),(#72308,#72309),(#72310,
#72311),(#72312,#72313),(#72314,#72315),(#72316,#72317),(#72318,#72319),
(#72320,#72321),(#72322,#72323),(#72324,#72325),(#72326,#72327),(#72328,
#72329),(#72330,#72331),(#72332,#72333),(#72334,#72335),(#72336,#72337),
(#72338,#72339),(#72340,#72341),(#72342,#72343),(#72344,#72345),(#72346,
#72347),(#72348,#72349),(#72350,#72351),(#72352,#72353),(#72354,#72355),
(#72356,#72357),(#72358,#72359),(#72360,#72361),(#72362,#72363),(#72364,
#72365),(#72366,#72367),(#72368,#72369),(#72370,#72371),(#72372,#72373),
(#72374,#72375),(#72376,#72377),(#72378,#72379),(#72380,#72381),(#72382,
#72383),(#72384,#72385),(#72386,#72387),(#72388,#72389),(#72390,#72391),
(#72392,#72393),(#72394,#72395),(#72396,#72397),(#72398,#72399),(#72400,
#72401),(#72402,#72403),(#72404,#72405),(#72406,#72407),(#72408,#72409),
(#72410,#72411),(#72412,#72413),(#72414,#72415),(#72416,#72417),(#72418,
#72419),(#72420,#72421),(#72422,#72423),(#72424,#72425),(#72426,#72427),
(#72428,#72429),(#72430,#72431),(#72432,#72433),(#72434,#72435),(#72436,
#72437),(#72438,#72439),(#72440,#72441),(#72442,#72443),(#72444,#72445),
(#72446,#72447),(#72448,#72449),(#72450,#72451),(#72452,#72453),(#72454,
#72455),(#72456,#72457),(#72458,#72459),(#72460,#72461),(#72462,#72463),
(#72464,#72465),(#72466,#72467),(#72468,#72469),(#72470,#72471),(#72472,
#72473),(#72474,#72475),(#72476,#72477),(#72478,#72479),(#72480,#72481),
(#72482,#72483),(#72484,#72485),(#72486,#72487),(#72488,#72489),(#72490,
#72491),(#72492,#72493),(#72494,#72495),(#72496,#72497),(#72498,#72499),
(#72500,#72501),(#72502,#72503),(#72504,#72505),(#72506,#72507),(#72508,
#72509),(#72510,#72511),(#72512,#72513),(#72514,#72515),(#72516,#72517),
(#72518,#72519),(#72520,#72521),(#72522,#72523),(#72524,#72525),(#72526,
#72527),(#72528,#72529),(#72530,#72531),(#72532,#72533),(#72534,#72535),
(#72536,#72537),(#72538,#72539),(#72540,#72541),(#72542,#72543),(#72544,
#72545),(#72546,#72547),(#72548,#72549),(#72550,#72551),(#72552,#72553),
(#72554,#72555),(#72556,#72557),(#72558,#72559),(#72560,#72561),(#72562,
#72563),(#72564,#72565),(#72566,#72567),(#72568,#72569),(#72570,#72571),
(#72572,#72573),(#72574,#72575),(#72576,#72577),(#72578,#72579),(#72580,
#72581),(#72582,#72583),(#72584,#72585),(#72586,#72587),(#72588,#72589),
(#72590,#72591),(#72592,#72593),(#72594,#72595),(#72596,#72597),(#72598,
#72599),(#72600,#72601),(#72602,#72603),(#72604,#72605),(#72606,#72607),
(#72608,#72609),(#72610,#72611),(#72612,#72613),(#72614,#72615),(#72616,
#72617),(#72618,#72619),(#72620,#72621),(#72622,#72623),(#72624,#72625),
(#72626,#72627),(#72628,#72629),(#72630,#72631),(#72632,#72633),(#72634,
#72635),(#72636,#72637),(#72638,#72639),(#72640,#72641),(#72642,#72643),
(#72644,#72645),(#72646,#72647),(#72648,#72649),(#72650,#72651),(#72652,
#72653),(#72654,#72655),(#72656,#72657),(#72658,#72659),(#72660,#72661),
(#72662,#72663),(#72664,#72665),(#72666,#72667),(#72668,#72669),(#72670,
#72671),(#72672,#72673),(#72674,#72675),(#72676,#72677),(#72678,#72679),
(#72680,#72681),(#72682,#72683),(#72684,#72685),(#72686,#72687),(#72688,
#72689),(#72690,#72691),(#72692,#72693),(#72694,#72695),(#72696,#72697),
(#72698,#72699),(#72700,#72701),(#72702,#72703),(#72704,#72705),(#72706,
#72707),(#72708,#72709),(#72710,#72711),(#72712,#72713),(#72714,#72715),
(#72716,#72717),(#72718,#72719),(#72720,#72721),(#72722,#72723),(#72724,
#72725),(#72726,#72727),(#72728,#72729),(#72730,#72731),(#72732,#72733),
(#72734,#72735),(#72736,#72737),(#72738,#72739),(#72740,#72741),(#72742,
#72743),(#72744,#72745),(#72746,#72747),(#72748,#72749),(#72750,#72751),
(#72752,#72753),(#72754,#72755),(#72756,#72757),(#72758,#72759),(#72760,
#72761),(#72762,#72763),(#72764,#72765),(#72766,#72767),(#72768,#72769),
(#72770,#72771),(#72772,#72773),(#72774,#72775),(#72776,#72777),(#72778,
#72779),(#72780,#72781),(#72782,#72783),(#72784,#72785),(#72786,#72787),
(#72788,#72789),(#72790,#72791),(#72792,#72793),(#72794,#72795),(#72796,
#72797),(#72798,#72799),(#72800,#72801),(#72802,#72803),(#72804,#72805),
(#72806,#72807),(#72808,#72809),(#72810,#72811),(#72812,#72813),(#72814,
#72815),(#72816,#72817),(#72818,#72819),(#72820,#72821),(#72822,#72823),
(#72824,#72825),(#72826,#72827),(#72828,#72829),(#72830,#72831),(#72832,
#72833),(#72834,#72835),(#72836,#72837),(#72838,#72839),(#72840,#72841),
(#72842,#72843),(#72844,#72845),(#72846,#72847),(#72848,#72849),(#72850,
#72851),(#72852,#72853),(#72854,#72855),(#72856,#72857),(#72858,#72859),
(#72860,#72861),(#72862,#72863),(#72864,#72865),(#72866,#72867),(#72868,
#72869),(#72870,#72871),(#72872,#72873),(#72874,#72875),(#72876,#72877),
(#72878,#72879),(#72880,#72881),(#72882,#72883),(#72884,#72885),(#72886,
#72887),(#72888,#72889),(#72890,#72891),(#72892,#72893),(#72894,#72895),
(#72896,#72897),(#72898,#72899),(#72900,#72901),(#72902,#72903),(#72904,
#72905),(#72906,#72907),(#72908,#72909),(#72910,#72911),(#72912,#72913),
(#72914,#72915),(#72916,#72917),(#72918,#72919),(#72920,#72921),(#72922,
#72923),(#72924,#72925),(#72926,#72927),(#72928,#72929),(#72930,#72931),
(#72932,#72933),(#72934,#72935),(#72936,#72937),(#72938,#72939),(#72940,
#72941),(#72942,#72943),(#72944,#72945),(#72946,#72947),(#72948,#72949),
(#72950,#72951),(#72952,#72953),(#72954,#72955),(#72956,#72957),(#72958,
#72959),(#72960,#72961),(#72962,#72963),(#72964,#72965),(#72966,#72967),
(#72968,#72969),(#72970,#72971),(#72972,#72973),(#72974,#72975),(#72976,
#72977),(#72978,#72979),(#72980,#72981),(#72982,#72983),(#72984,#72985),
(#72986,#72987),(#72988,#72989),(#72990,#72991),(#72992,#72993),(#72994,
#72995),(#72996,#72997),(#72998,#72999),(#73000,#73001),(#73002,#73003),
(#73004,#73005),(#73006,#73007),(#73008,#73009),(#73010,#73011),(#73012,
#73013),(#73014,#73015),(#73016,#73017),(#73018,#73019),(#73020,#73021),
(#73022,#73023),(#73024,#73025),(#73026,#73027),(#73028,#73029),(#73030,
#73031),(#73032,#73033),(#73034,#73035),(#73036,#73037),(#73038,#73039),
(#73040,#73041),(#73042,#73043),(#73044,#73045),(#73046,#73047),(#73048,
#73049),(#73050,#73051),(#73052,#73053),(#73054,#73055),(#73056,#73057),
(#73058,#73059),(#73060,#73061),(#73062,#73063),(#73064,#73065),(#73066,
#73067),(#73068,#73069),(#73070,#73071),(#73072,#73073),(#73074,#73075),
(#73076,#73077),(#73078,#73079),(#73080,#73081),(#73082,#73083),(#73084,
#73085),(#73086,#73087),(#73088,#73089),(#73090,#73091),(#73092,#73093),
(#73094,#73095),(#73096,#73097),(#73098,#73099),(#73100,#73101),(#73102,
#73103),(#73104,#73105),(#73106,#73107),(#73108,#73109),(#73110,#73111),
(#73112,#73113),(#73114,#73115),(#73116,#73117),(#73118,#73119),(#73120,
#73121),(#73122,#73123),(#73124,#73125),(#73126,#73127),(#73128,#73129),
(#73130,#73131),(#73132,#73133),(#73134,#73135),(#73136,#73137),(#73138,
#73139),(#73140,#73141),(#73142,#73143),(#73144,#73145),(#73146,#73147),
(#73148,#73149),(#73150,#73151),(#73152,#73153),(#73154,#73155),(#73156,
#73157),(#73158,#73159),(#73160,#73161),(#73162,#73163),(#73164,#73165),
(#73166,#73167),(#73168,#73169),(#73170,#73171),(#73172,#73173),(#73174,
#73175),(#73176,#73177),(#73178,#73179),(#73180,#73181),(#73182,#73183),
(#73184,#73185),(#73186,#73187),(#73188,#73189),(#73190,#73191),(#73192,
#73193),(#73194,#73195),(#73196,#73197),(#73198,#73199),(#73200,#73201),
(#73202,#73203),(#73204,#73205),(#73206,#73207),(#73208,#73209),(#73210,
#73211),(#73212,#73213),(#73214,#73215),(#73216,#73217),(#73218,#73219),
(#73220,#73221),(#73222,#73223),(#73224,#73225),(#73226,#73227),(#73228,
#73229),(#73230,#73231),(#73232,#73233),(#73234,#73235),(#73236,#73237),
(#73238,#73239),(#73240,#73241),(#73242,#73243),(#73244,#73245),(#73246,
#73247),(#73248,#73249),(#73250,#73251),(#73252,#73253),(#73254,#73255),
(#73256,#73257),(#73258,#73259),(#73260,#73261),(#73262,#73263),(#73264,
#73265),(#73266,#73267),(#73268,#73269),(#73270,#73271),(#73272,#73273),
(#73274,#73275),(#73276,#73277),(#73278,#73279),(#73280,#73281),(#73282,
#73283),(#73284,#73285),(#73286,#73287),(#73288,#73289),(#73290,#73291),
(#73292,#73293),(#73294,#73295),(#73296,#73297),(#73298,#73299),(#73300,
#73301),(#73302,#73303),(#73304,#73305),(#73306,#73307),(#73308,#73309),
(#73310,#73311),(#73312,#73313),(#73314,#73315),(#73316,#73317),(#73318,
#73319),(#73320,#73321),(#73322,#73323),(#73324,#73325),(#73326,#73327),
(#73328,#73329),(#73330,#73331),(#73332,#73333),(#73334,#73335),(#73336,
#73337),(#73338,#73339),(#73340,#73341),(#73342,#73343),(#73344,#73345),
(#73346,#73347),(#73348,#73349),(#73350,#73351),(#73352,#73353),(#73354,
#73355),(#73356,#73357),(#73358,#73359),(#73360,#73361),(#73362,#73363),
(#73364,#73365),(#73366,#73367),(#73368,#73369),(#73370,#73371),(#73372,
#73373),(#73374,#73375),(#73376,#73377),(#73378,#73379),(#73380,#73381),
(#73382,#73383),(#73384,#73385),(#73386,#73387),(#73388,#73389),(#73390,
#73391),(#73392,#73393),(#73394,#73395),(#73396,#73397),(#73398,#73399),
(#73400,#73401),(#73402,#73403),(#73404,#73405),(#73406,#73407),(#73408,
#73409),(#73410,#73411),(#73412,#73413),(#73414,#73415),(#73416,#73417),
(#73418,#73419),(#73420,#73421),(#73422,#73423),(#73424,#73425),(#73426,
#73427),(#73428,#73429),(#73430,#73431),(#73432,#73433),(#73434,#73435),
(#73436,#73437),(#73438,#73439),(#73440,#73441),(#73442,#73443),(#73444,
#73445),(#73446,#73447),(#73448,#73449),(#73450,#73451),(#73452,#73453),
(#73454,#73455),(#73456,#73457),(#73458,#73459),(#73460,#73461),(#73462,
#73463),(#73464,#73465),(#73466,#73467),(#73468,#73469),(#73470,#73471),
(#73472,#73473),(#73474,#73475),(#73476,#73477),(#73478,#73479),(#73480,
#73481),(#73482,#73483),(#73484,#73485),(#73486,#73487),(#73488,#73489),
(#73490,#73491),(#73492,#73493),(#73494,#73495),(#73496,#73497),(#73498,
#73499),(#73500,#73501),(#73502,#73503),(#73504,#73505),(#73506,#73507),
(#73508,#73509),(#73510,#73511),(#73512,#73513),(#73514,#73515),(#73516,
#73517),(#73518,#73519),(#73520,#73521),(#73522,#73523),(#73524,#73525),
(#73526,#73527),(#73528,#73529),(#73530,#73531),(#73532,#73533),(#73534,
#73535),(#73536,#73537),(#73538,#73539),(#73540,#73541),(#73542,#73543),
(#73544,#73545),(#73546,#73547),(#73548,#73549),(#73550,#73551),(#73552,
#73553),(#73554,#73555),(#73556,#73557),(#73558,#73559),(#73560,#73561),
(#73562,#73563),(#73564,#73565),(#73566,#73567),(#73568,#73569),(#73570,
#73571),(#73572,#73573),(#73574,#73575),(#73576,#73577),(#73578,#73579),
(#73580,#73581),(#73582,#73583),(#73584,#73585),(#73586,#73587),(#73588,
#73589),(#73590,#73591),(#73592,#73593),(#73594,#73595),(#73596,#73597),
(#73598,#73599),(#73600,#73601),(#73602,#73603),(#73604,#73605),(#73606,
#73607),(#73608,#73609),(#73610,#73611),(#73612,#73613),(#73614,#73615),
(#73616,#73617),(#73618,#73619),(#73620,#73621),(#73622,#73623),(#73624,
#73625),(#73626,#73627),(#73628,#73629),(#73630,#73631),(#73632,#73633),
(#73634,#73635),(#73636,#73637),(#73638,#73639),(#73640,#73641),(#73642,
#73643),(#73644,#73645),(#73646,#73647),(#73648,#73649),(#73650,#73651),
(#73652,#73653),(#73654,#73655),(#73656,#73657),(#73658,#73659),(#73660,
#73661),(#73662,#73663),(#73664,#73665),(#73666,#73667),(#73668,#73669),
(#73670,#73671),(#73672,#73673),(#73674,#73675),(#73676,#73677),(#73678,
#73679),(#73680,#73681),(#73682,#73683),(#73684,#73685),(#73686,#73687),
(#73688,#73689),(#73690,#73691),(#73692,#73693),(#73694,#73695),(#73696,
#73697),(#73698,#73699),(#73700,#73701),(#73702,#73703),(#73704,#73705),
(#73706,#73707),(#73708,#73709),(#73710,#73711),(#73712,#73713),(#73714,
#73715),(#73716,#73717),(#73718,#73719),(#73720,#73721),(#73722,#73723),
(#73724,#73725),(#73726,#73727),(#73728,#73729),(#73730,#73731),(#73732,
#73733),(#73734,#73735),(#73736,#73737),(#73738,#73739),(#73740,#73741),
(#73742,#73743),(#73744,#73745),(#73746,#73747),(#73748,#73749),(#73750,
#73751),(#73752,#73753),(#73754,#73755),(#73756,#73757),(#73758,#73759),
(#73760,#73761),(#73762,#73763),(#73764,#73765),(#73766,#73767),(#73768,
#73769),(#73770,#73771),(#73772,#73773),(#73774,#73775),(#73776,#73777),
(#73778,#73779),(#73780,#73781),(#73782,#73783),(#73784,#73785),(#73786,
#73787),(#73788,#73789),(#73790,#73791),(#73792,#73793),(#73794,#73795),
(#73796,#73797),(#73798,#73799),(#73800,#73801),(#73802,#73803),(#73804,
#73805),(#73806,#73807),(#73808,#73809),(#73810,#73811),(#73812,#73813),
(#73814,#73815),(#73816,#73817),(#73818,#73819),(#73820,#73821),(#73822,
#73823),(#73824,#73825),(#73826,#73827),(#73828,#73829),(#73830,#73831),
(#73832,#73833),(#73834,#73835),(#73836,#73837),(#73838,#73839),(#73840,
#73841),(#73842,#73843),(#73844,#73845),(#73846,#73847),(#73848,#73849),
(#73850,#73851),(#73852,#73853),(#73854,#73855),(#73856,#73857),(#73858,
#73859),(#73860,#73861),(#73862,#73863),(#73864,#73865),(#73866,#73867),
(#73868,#73869),(#73870,#73871),(#73872,#73873),(#73874,#73875),(#73876,
#73877),(#73878,#73879),(#73880,#73881),(#73882,#73883),(#73884,#73885),
(#73886,#73887),(#73888,#73889),(#73890,#73891),(#73892,#73893),(#73894,
#73895),(#73896,#73897),(#73898,#73899),(#73900,#73901),(#73902,#73903),
(#73904,#73905),(#73906,#73907),(#73908,#73909),(#73910,#73911),(#73912,
#73913),(#73914,#73915),(#73916,#73917),(#73918,#73919),(#73920,#73921),
(#73922,#73923),(#73924,#73925),(#73926,#73927),(#73928,#73929),(#73930,
#73931),(#73932,#73933),(#73934,#73935),(#73936,#73937),(#73938,#73939),
(#73940,#73941),(#73942,#73943),(#73944,#73945),(#73946,#73947),(#73948,
#73949),(#73950,#73951),(#73952,#73953),(#73954,#73955),(#73956,#73957),
(#73958,#73959),(#73960,#73961),(#73962,#73963),(#73964,#73965),(#73966,
#73967),(#73968,#73969),(#73970,#73971),(#73972,#73973),(#73974,#73975),
(#73976,#73977),(#73978,#73979),(#73980,#73981),(#73982,#73983),(#73984,
#73985),(#73986,#73987),(#73988,#73989),(#73990,#73991),(#73992,#73993),
(#73994,#73995),(#73996,#73997),(#73998,#73999),(#74000,#74001),(#74002,
#74003),(#74004,#74005),(#74006,#74007),(#74008,#74009),(#74010,#74011),
(#74012,#74013),(#74014,#74015),(#74016,#74017),(#74018,#74019),(#74020,
#74021),(#74022,#74023),(#74024,#74025),(#74026,#74027),(#74028,#74029),
(#74030,#74031),(#74032,#74033),(#74034,#74035),(#74036,#74037),(#74038,
#74039),(#74040,#74041),(#74042,#74043),(#74044,#74045),(#74046,#74047),
(#74048,#74049),(#74050,#74051),(#74052,#74053),(#74054,#74055),(#74056,
#74057),(#74058,#74059),(#74060,#74061),(#74062,#74063),(#74064,#74065),
(#74066,#74067),(#74068,#74069),(#74070,#74071),(#74072,#74073),(#74074,
#74075),(#74076,#74077),(#74078,#74079),(#74080,#74081),(#74082,#74083),
(#74084,#74085),(#74086,#74087),(#74088,#74089),(#74090,#74091),(#74092,
#74093),(#74094,#74095),(#74096,#74097),(#74098,#74099),(#74100,#74101),
(#74102,#74103),(#74104,#74105),(#74106,#74107),(#74108,#74109),(#74110,
#74111),(#74112,#74113),(#74114,#74115),(#74116,#74117),(#74118,#74119),
(#74120,#74121),(#74122,#74123),(#74124,#74125),(#74126,#74127),(#74128,
#74129),(#74130,#74131),(#74132,#74133),(#74134,#74135),(#74136,#74137),
(#74138,#74139),(#74140,#74141),(#74142,#74143),(#74144,#74145),(#74146,
#74147),(#74148,#74149),(#74150,#74151),(#74152,#74153),(#74154,#74155),
(#74156,#74157),(#74158,#74159),(#74160,#74161),(#74162,#74163),(#74164,
#74165),(#74166,#74167),(#74168,#74169),(#74170,#74171),(#74172,#74173),
(#74174,#74175),(#74176,#74177),(#74178,#74179),(#74180,#74181),(#74182,
#74183),(#74184,#74185),(#74186,#74187),(#74188,#74189),(#74190,#74191),
(#74192,#74193),(#74194,#74195),(#74196,#74197),(#74198,#74199),(#74200,
#74201),(#74202,#74203),(#74204,#74205),(#74206,#74207),(#74208,#74209),
(#74210,#74211),(#74212,#74213),(#74214,#74215),(#74216,#74217),(#74218,
#74219),(#74220,#74221),(#74222,#74223),(#74224,#74225),(#74226,#74227),
(#74228,#74229),(#74230,#74231),(#74232,#74233),(#74234,#74235),(#74236,
#74237),(#74238,#74239),(#74240,#74241),(#74242,#74243),(#74244,#74245),
(#74246,#74247),(#74248,#74249),(#74250,#74251),(#74252,#74253),(#74254,
#74255),(#74256,#74257),(#74258,#74259),(#74260,#74261),(#74262,#74263),
(#74264,#74265),(#74266,#74267),(#74268,#74269),(#74270,#74271),(#74272,
#74273),(#74274,#74275),(#74276,#74277),(#74278,#74279),(#74280,#74281),
(#74282,#74283),(#74284,#74285),(#74286,#74287),(#74288,#74289),(#74290,
#74291),(#74292,#74293),(#74294,#74295),(#74296,#74297),(#74298,#74299),
(#74300,#74301),(#74302,#74303),(#74304,#74305),(#74306,#74307),(#74308,
#74309),(#74310,#74311),(#74312,#74313),(#74314,#74315),(#74316,#74317),
(#74318,#74319),(#74320,#74321),(#74322,#74323),(#74324,#74325),(#74326,
#74327),(#74328,#74329),(#74330,#74331),(#74332,#74333),(#74334,#74335),
(#74336,#74337),(#74338,#74339),(#74340,#74341),(#74342,#74343),(#74344,
#74345),(#74346,#74347),(#74348,#74349),(#74350,#74351),(#74352,#74353),
(#74354,#74355),(#74356,#74357),(#74358,#74359),(#74360,#74361),(#74362,
#74363),(#74364,#74365),(#74366,#74367),(#74368,#74369),(#74370,#74371),
(#74372,#74373),(#74374,#74375),(#74376,#74377),(#74378,#74379),(#74380,
#74381),(#74382,#74383),(#74384,#74385),(#74386,#74387),(#74388,#74389),
(#74390,#74391),(#74392,#74393),(#74394,#74395),(#74396,#74397),(#74398,
#74399),(#74400,#74401),(#74402,#74403),(#74404,#74405),(#74406,#74407),
(#74408,#74409),(#74410,#74411),(#74412,#74413),(#74414,#74415),(#74416,
#74417),(#74418,#74419),(#74420,#74421),(#74422,#74423),(#74424,#74425),
(#74426,#74427),(#74428,#74429),(#74430,#74431),(#74432,#74433),(#74434,
#74435),(#74436,#74437),(#74438,#74439),(#74440,#74441),(#74442,#74443),
(#74444,#74445),(#74446,#74447),(#74448,#74449),(#74450,#74451),(#74452,
#74453),(#74454,#74455),(#74456,#74457),(#74458,#74459),(#74460,#74461),
(#74462,#74463),(#74464,#74465),(#74466,#74467),(#74468,#74469),(#74470,
#74471),(#74472,#74473),(#74474,#74475),(#74476,#74477),(#74478,#74479),
(#74480,#74481),(#74482,#74483),(#74484,#74485),(#74486,#74487),(#74488,
#74489),(#74490,#74491),(#74492,#74493),(#74494,#74495),(#74496,#74497),
(#74498,#74499),(#74500,#74501),(#74502,#74503),(#74504,#74505),(#74506,
#74507),(#74508,#74509),(#74510,#74511),(#74512,#74513),(#74514,#74515),
(#74516,#74517),(#74518,#74519),(#74520,#74521),(#74522,#74523),(#74524,
#74525),(#74526,#74527),(#74528,#74529),(#74530,#74531),(#74532,#74533),
(#74534,#74535),(#74536,#74537),(#74538,#74539),(#74540,#74541),(#74542,
#74543),(#74544,#74545),(#74546,#74547),(#74548,#74549),(#74550,#74551),
(#74552,#74553),(#74554,#74555),(#74556,#74557),(#74558,#74559),(#74560,
#74561),(#74562,#74563),(#74564,#74565),(#74566,#74567),(#74568,#74569),
(#74570,#74571),(#74572,#74573),(#74574,#74575),(#74576,#74577),(#74578,
#74579),(#74580,#74581),(#74582,#74583),(#74584,#74585),(#74586,#74587),
(#74588,#74589),(#74590,#74591),(#74592,#74593),(#74594,#74595),(#74596,
#74597),(#74598,#74599),(#74600,#74601),(#74602,#74603),(#74604,#74605),
(#74606,#74607),(#74608,#74609),(#74610,#74611),(#74612,#74613),(#74614,
#74615),(#74616,#74617),(#74618,#74619),(#74620,#74621),(#74622,#74623),
(#74624,#74625),(#74626,#74627),(#74628,#74629),(#74630,#74631),(#74632,
#74633),(#74634,#74635),(#74636,#74637),(#74638,#74639),(#74640,#74641),
(#74642,#74643),(#74644,#74645),(#74646,#74647),(#74648,#74649),(#74650,
#74651),(#74652,#74653),(#74654,#74655),(#74656,#74657),(#74658,#74659),
(#74660,#74661),(#74662,#74663),(#74664,#74665),(#74666,#74667),(#74668,
#74669),(#74670,#74671),(#74672,#74673),(#74674,#74675),(#74676,#74677),
(#74678,#74679),(#74680,#74681),(#74682,#74683),(#74684,#74685),(#74686,
#74687),(#74688,#74689),(#74690,#74691),(#74692,#74693),(#74694,#74695),
(#74696,#74697),(#74698,#74699),(#74700,#74701),(#74702,#74703),(#74704,
#74705),(#74706,#74707),(#74708,#74709),(#74710,#74711),(#74712,#74713),
(#74714,#74715),(#74716,#74717),(#74718,#74719),(#74720,#74721),(#74722,
#74723),(#74724,#74725),(#74726,#74727),(#74728,#74729),(#74730,#74731),
(#74732,#74733),(#74734,#74735),(#74736,#74737),(#74738,#74739),(#74740,
#74741),(#74742,#74743),(#74744,#74745),(#74746,#74747),(#74748,#74749),
(#74750,#74751),(#74752,#74753),(#74754,#74755),(#74756,#74757),(#74758,
#74759),(#74760,#74761),(#74762,#74763),(#74764,#74765),(#74766,#74767),
(#74768,#74769),(#74770,#74771),(#74772,#74773),(#74774,#74775),(#74776,
#74777),(#74778,#74779),(#74780,#74781),(#74782,#74783),(#74784,#74785),
(#74786,#74787),(#74788,#74789),(#74790,#74791),(#74792,#74793),(#74794,
#74795),(#74796,#74797),(#74798,#74799),(#74800,#74801),(#74802,#74803),
(#74804,#74805),(#74806,#74807),(#74808,#74809),(#74810,#74811),(#74812,
#74813),(#74814,#74815),(#74816,#74817),(#74818,#74819),(#74820,#74821),
(#74822,#74823),(#74824,#74825),(#74826,#74827),(#74828,#74829),(#74830,
#74831),(#74832,#74833),(#74834,#74835),(#74836,#74837),(#74838,#74839),
(#74840,#74841),(#74842,#74843),(#74844,#74845),(#74846,#74847),(#74848,
#74849),(#74850,#74851),(#74852,#74853),(#74854,#74855),(#74856,#74857),
(#74858,#74859),(#74860,#74861),(#74862,#74863),(#74864,#74865),(#74866,
#74867),(#74868,#74869),(#74870,#74871),(#74872,#74873),(#74874,#74875),
(#74876,#74877),(#74878,#74879),(#74880,#74881),(#74882,#74883),(#74884,
#74885),(#74886,#74887),(#74888,#74889),(#74890,#74891),(#74892,#74893),
(#74894,#74895),(#74896,#74897),(#74898,#74899),(#74900,#74901),(#74902,
#74903),(#74904,#74905),(#74906,#74907),(#74908,#74909),(#74910,#74911),
(#74912,#74913),(#74914,#74915),(#74916,#74917),(#74918,#74919),(#74920,
#74921),(#74922,#74923),(#74924,#74925),(#74926,#74927),(#74928,#74929),
(#74930,#74931),(#74932,#74933),(#74934,#74935),(#74936,#74937),(#74938,
#74939),(#74940,#74941),(#74942,#74943),(#74944,#74945),(#74946,#74947),
(#74948,#74949),(#74950,#74951),(#74952,#74953),(#74954,#74955),(#74956,
#74957),(#74958,#74959),(#74960,#74961),(#74962,#74963),(#74964,#74965),
(#74966,#74967),(#74968,#74969),(#74970,#74971),(#74972,#74973),(#74974,
#74975),(#74976,#74977),(#74978,#74979),(#74980,#74981),(#74982,#74983),
(#74984,#74985),(#74986,#74987),(#74988,#74989),(#74990,#74991),(#74992,
#74993),(#74994,#74995),(#74996,#74997),(#74998,#74999),(#75000,#75001),
(#75002,#75003),(#75004,#75005),(#75006,#75007),(#75008,#75009),(#75010,
#75011),(#75012,#75013),(#75014,#75015),(#75016,#75017),(#75018,#75019),
(#75020,#75021),(#75022,#75023),(#75024,#75025),(#75026,#75027),(#75028,
#75029),(#75030,#75031),(#75032,#75033),(#75034,#75035),(#75036,#75037),
(#75038,#75039),(#75040,#75041),(#75042,#75043),(#75044,#75045),(#75046,
#75047),(#75048,#75049),(#75050,#75051),(#75052,#75053),(#75054,#75055),
(#75056,#75057),(#75058,#75059),(#75060,#75061),(#75062,#75063),(#75064,
#75065),(#75066,#75067),(#75068,#75069),(#75070,#75071),(#75072,#75073),
(#75074,#75075),(#75076,#75077),(#75078,#75079),(#75080,#75081),(#75082,
#75083),(#75084,#75085),(#75086,#75087),(#75088,#75089),(#75090,#75091),
(#75092,#75093),(#75094,#75095),(#75096,#75097),(#75098,#75099),(#75100,
#75101),(#75102,#75103),(#75104,#75105),(#75106,#75107),(#75108,#75109),
(#75110,#75111),(#75112,#75113),(#75114,#75115),(#75116,#75117),(#75118,
#75119),(#75120,#75121),(#75122,#75123),(#75124,#75125),(#75126,#75127),
(#75128,#75129),(#75130,#75131),(#75132,#75133),(#75134,#75135),(#75136,
#75137),(#75138,#75139),(#75140,#75141),(#75142,#75143),(#75144,#75145),
(#75146,#75147),(#75148,#75149),(#75150,#75151),(#75152,#75153),(#75154,
#75155),(#75156,#75157),(#75158,#75159),(#75160,#75161),(#75162,#75163),
(#75164,#75165),(#75166,#75167),(#75168,#75169),(#75170,#75171),(#75172,
#75173),(#75174,#75175),(#75176,#75177),(#75178,#75179),(#75180,#75181),
(#75182,#75183),(#75184,#75185),(#75186,#75187),(#75188,#75189),(#75190,
#75191),(#75192,#75193),(#75194,#75195),(#75196,#75197),(#75198,#75199),
(#75200,#75201),(#75202,#75203),(#75204,#75205),(#75206,#75207),(#75208,
#75209),(#75210,#75211),(#75212,#75213),(#75214,#75215),(#75216,#75217),
(#75218,#75219),(#75220,#75221),(#75222,#75223),(#75224,#75225),(#75226,
#75227),(#75228,#75229),(#75230,#75231),(#75232,#75233),(#75234,#75235),
(#75236,#75237),(#75238,#75239),(#75240,#75241),(#75242,#75243),(#75244,
#75245),(#75246,#75247),(#75248,#75249),(#75250,#75251),(#75252,#75253),
(#75254,#75255),(#75256,#75257),(#75258,#75259),(#75260,#75261),(#75262,
#75263),(#75264,#75265),(#75266,#75267),(#75268,#75269),(#75270,#75271),
(#75272,#75273),(#75274,#75275),(#75276,#75277),(#75278,#75279),(#75280,
#75281),(#75282,#75283),(#75284,#75285),(#75286,#75287),(#75288,#75289),
(#75290,#75291),(#75292,#75293),(#75294,#75295),(#75296,#75297),(#75298,
#75299),(#75300,#75301),(#75302,#75303),(#75304,#75305),(#75306,#75307),
(#75308,#75309),(#75310,#75311),(#75312,#75313),(#75314,#75315),(#75316,
#75317),(#75318,#75319),(#75320,#75321),(#75322,#75323),(#75324,#75325),
(#75326,#75327),(#75328,#75329),(#75330,#75331),(#75332,#75333),(#75334,
#75335),(#75336,#75337),(#75338,#75339),(#75340,#75341),(#75342,#75343),
(#75344,#75345),(#75346,#75347),(#75348,#75349),(#75350,#75351),(#75352,
#75353),(#75354,#75355),(#75356,#75357),(#75358,#75359),(#75360,#75361),
(#75362,#75363),(#75364,#75365),(#75366,#75367),(#75368,#75369),(#75370,
#75371),(#75372,#75373),(#75374,#75375),(#75376,#75377),(#75378,#75379),
(#75380,#75381),(#75382,#75383),(#75384,#75385),(#75386,#75387),(#75388,
#75389),(#75390,#75391),(#75392,#75393),(#75394,#75395),(#75396,#75397),
(#75398,#75399),(#75400,#75401),(#75402,#75403),(#75404,#75405),(#75406,
#75407),(#75408,#75409),(#75410,#75411),(#75412,#75413),(#75414,#75415),
(#75416,#75417),(#75418,#75419),(#75420,#75421),(#75422,#75423),(#75424,
#75425),(#75426,#75427),(#75428,#75429),(#75430,#75431),(#75432,#75433),
(#75434,#75435),(#75436,#75437),(#75438,#75439),(#75440,#75441),(#75442,
#75443),(#75444,#75445),(#75446,#75447),(#75448,#75449),(#75450,#75451),
(#75452,#75453),(#75454,#75455),(#75456,#75457),(#75458,#75459),(#75460,
#75461),(#75462,#75463),(#75464,#75465),(#75466,#75467),(#75468,#75469),
(#75470,#75471),(#75472,#75473),(#75474,#75475),(#75476,#75477),(#75478,
#75479),(#75480,#75481),(#75482,#75483),(#75484,#75485),(#75486,#75487),
(#75488,#75489),(#75490,#75491),(#75492,#75493),(#75494,#75495),(#75496,
#75497),(#75498,#75499),(#75500,#75501),(#75502,#75503),(#75504,#75505),
(#75506,#75507),(#75508,#75509),(#75510,#75511),(#75512,#75513),(#75514,
#75515),(#75516,#75517),(#75518,#75519),(#75520,#75521),(#75522,#75523),
(#75524,#75525),(#75526,#75527),(#75528,#75529),(#75530,#75531),(#75532,
#75533),(#75534,#75535),(#75536,#75537),(#75538,#75539),(#75540,#75541),
(#75542,#75543),(#75544,#75545),(#75546,#75547),(#75548,#75549),(#75550,
#75551),(#75552,#75553),(#75554,#75555),(#75556,#75557),(#75558,#75559),
(#75560,#75561),(#75562,#75563),(#75564,#75565),(#75566,#75567),(#75568,
#75569),(#75570,#75571),(#75572,#75573),(#75574,#75575),(#75576,#75577),
(#75578,#75579),(#75580,#75581),(#75582,#75583),(#75584,#75585),(#75586,
#75587),(#75588,#75589),(#75590,#75591),(#75592,#75593),(#75594,#75595),
(#75596,#75597),(#75598,#75599),(#75600,#75601),(#75602,#75603),(#75604,
#75605),(#75606,#75607),(#75608,#75609),(#75610,#75611),(#75612,#75613),
(#75614,#75615),(#75616,#75617),(#75618,#75619),(#75620,#75621),(#75622,
#75623),(#75624,#75625),(#75626,#75627),(#75628,#75629),(#75630,#75631),
(#75632,#75633),(#75634,#75635),(#75636,#75637),(#75638,#75639),(#75640,
#75641),(#75642,#75643),(#75644,#75645),(#75646,#75647),(#75648,#75649),
(#75650,#75651),(#75652,#75653),(#75654,#75655),(#75656,#75657),(#75658,
#75659),(#75660,#75661),(#75662,#75663),(#75664,#75665),(#75666,#75667),
(#75668,#75669),(#75670,#75671),(#75672,#75673),(#75674,#75675),(#75676,
#75677),(#75678,#75679),(#75680,#75681),(#75682,#75683),(#75684,#75685),
(#75686,#75687),(#75688,#75689),(#75690,#75691),(#75692,#75693),(#75694,
#75695),(#75696,#75697),(#75698,#75699),(#75700,#75701),(#75702,#75703),
(#75704,#75705),(#75706,#75707),(#75708,#75709),(#75710,#75711),(#75712,
#75713),(#75714,#75715),(#75716,#75717),(#75718,#75719),(#75720,#75721),
(#75722,#75723),(#75724,#75725),(#75726,#75727),(#75728,#75729),(#75730,
#75731),(#75732,#75733),(#75734,#75735),(#75736,#75737),(#75738,#75739),
(#75740,#75741),(#75742,#75743),(#75744,#75745),(#75746,#75747),(#75748,
#75749),(#75750,#75751),(#75752,#75753),(#75754,#75755),(#75756,#75757),
(#75758,#75759),(#75760,#75761),(#75762,#75763),(#75764,#75765),(#75766,
#75767),(#75768,#75769),(#75770,#75771),(#75772,#75773),(#75774,#75775),
(#75776,#75777),(#75778,#75779),(#75780,#75781),(#75782,#75783),(#75784,
#75785),(#75786,#75787),(#75788,#75789),(#75790,#75791),(#75792,#75793),
(#75794,#75795),(#75796,#75797),(#75798,#75799),(#75800,#75801),(#75802,
#75803),(#75804,#75805),(#75806,#75807),(#75808,#75809),(#75810,#75811),
(#75812,#75813),(#75814,#75815),(#75816,#75817),(#75818,#75819),(#75820,
#75821),(#75822,#75823),(#75824,#75825),(#75826,#75827),(#75828,#75829),
(#75830,#75831),(#75832,#75833),(#75834,#75835),(#75836,#75837),(#75838,
#75839),(#75840,#75841),(#75842,#75843),(#75844,#75845),(#75846,#75847),
(#75848,#75849),(#75850,#75851),(#75852,#75853),(#75854,#75855),(#75856,
#75857),(#75858,#75859),(#75860,#75861),(#75862,#75863),(#75864,#75865),
(#75866,#75867),(#75868,#75869),(#75870,#75871),(#75872,#75873),(#75874,
#75875),(#75876,#75877),(#75878,#75879),(#75880,#75881),(#75882,#75883),
(#75884,#75885),(#75886,#75887),(#75888,#75889),(#75890,#75891),(#75892,
#75893),(#75894,#75895),(#75896,#75897),(#75898,#75899),(#75900,#75901),
(#75902,#75903),(#75904,#75905),(#75906,#75907),(#75908,#75909),(#75910,
#75911),(#75912,#75913),(#75914,#75915),(#75916,#75917),(#75918,#75919),
(#75920,#75921),(#75922,#75923),(#75924,#75925),(#75926,#75927),(#75928,
#75929),(#75930,#75931),(#75932,#75933),(#75934,#75935),(#75936,#75937),
(#75938,#75939),(#75940,#75941),(#75942,#75943),(#75944,#75945),(#75946,
#75947),(#75948,#75949),(#75950,#75951),(#75952,#75953),(#75954,#75955),
(#75956,#75957),(#75958,#75959),(#75960,#75961),(#75962,#75963),(#75964,
#75965),(#75966,#75967),(#75968,#75969),(#75970,#75971),(#75972,#75973),
(#75974,#75975),(#75976,#75977),(#75978,#75979),(#75980,#75981),(#75982,
#75983),(#75984,#75985),(#75986,#75987),(#75988,#75989),(#75990,#75991),
(#75992,#75993),(#75994,#75995),(#75996,#75997),(#75998,#75999),(#76000,
#76001),(#76002,#76003),(#76004,#76005),(#76006,#76007),(#76008,#76009),
(#76010,#76011),(#76012,#76013),(#76014,#76015),(#76016,#76017),(#76018,
#76019),(#76020,#76021),(#76022,#76023),(#76024,#76025),(#76026,#76027),
(#76028,#76029),(#76030,#76031),(#76032,#76033),(#76034,#76035),(#76036,
#76037),(#76038,#76039),(#76040,#76041),(#76042,#76043),(#76044,#76045),
(#76046,#76047),(#76048,#76049),(#76050,#76051),(#76052,#76053),(#76054,
#76055),(#76056,#76057),(#76058,#76059),(#76060,#76061),(#76062,#76063),
(#76064,#76065),(#76066,#76067),(#76068,#76069),(#76070,#76071),(#76072,
#76073),(#76074,#76075),(#76076,#76077),(#76078,#76079),(#76080,#76081),
(#76082,#76083),(#76084,#76085),(#76086,#76087),(#76088,#76089),(#76090,
#76091),(#76092,#76093),(#76094,#76095),(#76096,#76097),(#76098,#76099),
(#76100,#76101),(#76102,#76103),(#76104,#76105),(#76106,#76107),(#76108,
#76109),(#76110,#76111),(#76112,#76113),(#76114,#76115),(#76116,#76117),
(#76118,#76119),(#76120,#76121),(#76122,#76123),(#76124,#76125),(#76126,
#76127),(#76128,#76129),(#76130,#76131),(#76132,#76133),(#76134,#76135),
(#76136,#76137),(#76138,#76139),(#76140,#76141),(#76142,#76143),(#76144,
#76145),(#76146,#76147),(#76148,#76149),(#76150,#76151),(#76152,#76153),
(#76154,#76155),(#76156,#76157),(#76158,#76159),(#76160,#76161),(#76162,
#76163),(#76164,#76165),(#76166,#76167),(#76168,#76169),(#76170,#76171),
(#76172,#76173),(#76174,#76175),(#76176,#76177),(#76178,#76179),(#76180,
#76181),(#76182,#76183),(#76184,#76185),(#76186,#76187),(#76188,#76189),
(#76190,#76191),(#76192,#76193),(#76194,#76195),(#76196,#76197),(#76198,
#76199),(#76200,#76201),(#76202,#76203),(#76204,#76205),(#76206,#76207),
(#76208,#76209),(#76210,#76211),(#76212,#76213),(#76214,#76215),(#76216,
#76217),(#76218,#76219),(#76220,#76221),(#76222,#76223),(#76224,#76225),
(#76226,#76227),(#76228,#76229),(#76230,#76231),(#76232,#76233),(#76234,
#76235),(#76236,#76237),(#76238,#76239),(#76240,#76241),(#76242,#76243),
(#76244,#76245),(#76246,#76247),(#76248,#76249),(#76250,#76251),(#76252,
#76253),(#76254,#76255),(#76256,#76257),(#76258,#76259),(#76260,#76261),
(#76262,#76263),(#76264,#76265),(#76266,#76267),(#76268,#76269),(#76270,
#76271),(#76272,#76273),(#76274,#76275),(#76276,#76277),(#76278,#76279),
(#76280,#76281),(#76282,#76283),(#76284,#76285),(#76286,#76287),(#76288,
#76289),(#76290,#76291),(#76292,#76293),(#76294,#76295),(#76296,#76297),
(#76298,#76299),(#76300,#76301),(#76302,#76303),(#76304,#76305),(#76306,
#76307),(#76308,#76309),(#76310,#76311),(#76312,#76313),(#76314,#76315),
(#76316,#76317),(#76318,#76319),(#76320,#76321),(#76322,#76323),(#76324,
#76325),(#76326,#76327),(#76328,#76329),(#76330,#76331),(#76332,#76333),
(#76334,#76335),(#76336,#76337),(#76338,#76339),(#76340,#76341),(#76342,
#76343),(#76344,#76345),(#76346,#76347),(#76348,#76349),(#76350,#76351),
(#76352,#76353),(#76354,#76355),(#76356,#76357),(#76358,#76359),(#76360,
#76361),(#76362,#76363),(#76364,#76365),(#76366,#76367),(#76368,#76369),
(#76370,#76371),(#76372,#76373),(#76374,#76375),(#76376,#76377),(#76378,
#76379),(#76380,#76381),(#76382,#76383),(#76384,#76385),(#76386,#76387),
(#76388,#76389),(#76390,#76391),(#76392,#76393),(#76394,#76395),(#76396,
#76397),(#76398,#76399),(#76400,#76401),(#76402,#76403),(#76404,#76405),
(#76406,#76407),(#76408,#76409),(#76410,#76411),(#76412,#76413),(#76414,
#76415),(#76416,#76417),(#76418,#76419),(#76420,#76421),(#76422,#76423),
(#76424,#76425),(#76426,#76427),(#76428,#76429),(#76430,#76431),(#76432,
#76433),(#76434,#76435),(#76436,#76437),(#76438,#76439),(#76440,#76441),
(#76442,#76443),(#76444,#76445),(#76446,#76447),(#76448,#76449),(#76450,
#76451),(#76452,#76453),(#76454,#76455),(#76456,#76457),(#76458,#76459),
(#76460,#76461),(#76462,#76463),(#76464,#76465),(#76466,#76467),(#76468,
#76469),(#76470,#76471),(#76472,#76473),(#76474,#76475),(#76476,#76477),
(#76478,#76479),(#76480,#76481),(#76482,#76483),(#76484,#76485),(#76486,
#76487),(#76488,#76489),(#76490,#76491),(#76492,#76493),(#76494,#76495),
(#76496,#76497),(#76498,#76499),(#76500,#76501),(#76502,#76503),(#76504,
#76505),(#76506,#76507),(#76508,#76509),(#76510,#76511),(#76512,#76513),
(#76514,#76515),(#76516,#76517),(#76518,#76519),(#76520,#76521),(#76522,
#76523),(#76524,#76525),(#76526,#76527),(#76528,#76529),(#76530,#76531),
(#76532,#76533),(#76534,#76535),(#76536,#76537),(#76538,#76539),(#76540,
#76541),(#76542,#76543),(#76544,#76545),(#76546,#76547),(#76548,#76549),
(#76550,#76551),(#76552,#76553),(#76554,#76555),(#76556,#76557),(#76558,
#76559),(#76560,#76561),(#76562,#76563),(#76564,#76565),(#76566,#76567),
(#76568,#76569),(#76570,#76571),(#76572,#76573),(#76574,#76575),(#76576,
#76577),(#76578,#76579),(#76580,#76581),(#76582,#76583),(#76584,#76585),
(#76586,#76587),(#76588,#76589),(#76590,#76591),(#76592,#76593),(#76594,
#76595),(#76596,#76597),(#76598,#76599),(#76600,#76601),(#76602,#76603),
(#76604,#76605),(#76606,#76607),(#76608,#76609),(#76610,#76611),(#76612,
#76613),(#76614,#76615),(#76616,#76617),(#76618,#76619),(#76620,#76621),
(#76622,#76623),(#76624,#76625),(#76626,#76627),(#76628,#76629),(#76630,
#76631),(#76632,#76633),(#76634,#76635),(#76636,#76637),(#76638,#76639),
(#76640,#76641),(#76642,#76643),(#76644,#76645),(#76646,#76647),(#76648,
#76649),(#76650,#76651),(#76652,#76653),(#76654,#76655),(#76656,#76657),
(#76658,#76659),(#76660,#76661),(#76662,#76663),(#76664,#76665),(#76666,
#76667),(#76668,#76669),(#76670,#76671),(#76672,#76673),(#76674,#76675),
(#76676,#76677),(#76678,#76679),(#76680,#76681),(#76682,#76683),(#76684,
#76685),(#76686,#76687),(#76688,#76689),(#76690,#76691),(#76692,#76693),
(#76694,#76695),(#76696,#76697),(#76698,#76699),(#76700,#76701),(#76702,
#76703),(#76704,#76705),(#76706,#76707),(#76708,#76709),(#76710,#76711),
(#76712,#76713),(#76714,#76715),(#76716,#76717),(#76718,#76719),(#76720,
#76721),(#76722,#76723),(#76724,#76725),(#76726,#76727),(#76728,#76729),
(#76730,#76731),(#76732,#76733),(#76734,#76735),(#76736,#76737),(#76738,
#76739),(#76740,#76741),(#76742,#76743),(#76744,#76745),(#76746,#76747),
(#76748,#76749),(#76750,#76751),(#76752,#76753),(#76754,#76755),(#76756,
#76757),(#76758,#76759),(#76760,#76761),(#76762,#76763),(#76764,#76765),
(#76766,#76767),(#76768,#76769),(#76770,#76771),(#76772,#76773),(#76774,
#76775),(#76776,#76777),(#76778,#76779),(#76780,#76781),(#76782,#76783),
(#76784,#76785),(#76786,#76787),(#76788,#76789),(#76790,#76791),(#76792,
#76793),(#76794,#76795),(#76796,#76797),(#76798,#76799),(#76800,#76801),
(#76802,#76803),(#76804,#76805),(#76806,#76807),(#76808,#76809),(#76810,
#76811),(#76812,#76813),(#76814,#76815),(#76816,#76817),(#76818,#76819),
(#76820,#76821),(#76822,#76823),(#76824,#76825),(#76826,#76827),(#76828,
#76829),(#76830,#76831),(#76832,#76833),(#76834,#76835),(#76836,#76837),
(#76838,#76839),(#76840,#76841),(#76842,#76843),(#76844,#76845),(#76846,
#76847),(#76848,#76849),(#76850,#76851),(#76852,#76853),(#76854,#76855),
(#76856,#76857),(#76858,#76859),(#76860,#76861),(#76862,#76863),(#76864,
#76865),(#76866,#76867),(#76868,#76869),(#76870,#76871),(#76872,#76873),
(#76874,#76875),(#76876,#76877),(#76878,#76879),(#76880,#76881),(#76882,
#76883),(#76884,#76885),(#76886,#76887),(#76888,#76889),(#76890,#76891),
(#76892,#76893),(#76894,#76895),(#76896,#76897),(#76898,#76899),(#76900,
#76901),(#76902,#76903),(#76904,#76905),(#76906,#76907),(#76908,#76909),
(#76910,#76911),(#76912,#76913),(#76914,#76915),(#76916,#76917),(#76918,
#76919),(#76920,#76921),(#76922,#76923),(#76924,#76925),(#76926,#76927),
(#76928,#76929),(#76930,#76931),(#76932,#76933),(#76934,#76935),(#76936,
#76937),(#76938,#76939),(#76940,#76941),(#76942,#76943),(#76944,#76945),
(#76946,#76947),(#76948,#76949),(#76950,#76951),(#76952,#76953),(#76954,
#76955),(#76956,#76957),(#76958,#76959),(#76960,#76961),(#76962,#76963),
(#76964,#76965),(#76966,#76967),(#76968,#76969),(#76970,#76971),(#76972,
#76973),(#76974,#76975),(#76976,#76977),(#76978,#76979),(#76980,#76981),
(#76982,#76983),(#76984,#76985),(#76986,#76987),(#76988,#76989),(#76990,
#76991),(#76992,#76993),(#76994,#76995),(#76996,#76997),(#76998,#76999),
(#77000,#77001),(#77002,#77003),(#77004,#77005),(#77006,#77007),(#77008,
#77009),(#77010,#77011),(#77012,#77013),(#77014,#77015),(#77016,#77017),
(#77018,#77019),(#77020,#77021),(#77022,#77023),(#77024,#77025),(#77026,
#77027),(#77028,#77029),(#77030,#77031),(#77032,#77033),(#77034,#77035),
(#77036,#77037),(#77038,#77039),(#77040,#77041),(#77042,#77043),(#77044,
#77045),(#77046,#77047),(#77048,#77049),(#77050,#77051),(#77052,#77053),
(#77054,#77055),(#77056,#77057),(#77058,#77059),(#77060,#77061),(#77062,
#77063),(#77064,#77065),(#77066,#77067),(#77068,#77069),(#77070,#77071),
(#77072,#77073),(#77074,#77075),(#77076,#77077),(#77078,#77079),(#77080,
#77081),(#77082,#77083),(#77084,#77085),(#77086,#77087),(#77088,#77089),
(#77090,#77091),(#77092,#77093),(#77094,#77095),(#77096,#77097),(#77098,
#77099),(#77100,#77101),(#77102,#77103),(#77104,#77105),(#77106,#77107),
(#77108,#77109),(#77110,#77111),(#77112,#77113),(#77114,#77115),(#77116,
#77117),(#77118,#77119),(#77120,#77121),(#77122,#77123),(#77124,#77125),
(#77126,#77127),(#77128,#77129),(#77130,#77131),(#77132,#77133),(#77134,
#77135),(#77136,#77137),(#77138,#77139),(#77140,#77141),(#77142,#77143),
(#77144,#77145),(#77146,#77147),(#77148,#77149),(#77150,#77151),(#77152,
#77153),(#77154,#77155),(#77156,#77157),(#77158,#77159),(#77160,#77161),
(#77162,#77163),(#77164,#77165),(#77166,#77167),(#77168,#77169),(#77170,
#77171),(#77172,#77173),(#77174,#77175),(#77176,#77177),(#77178,#77179),
(#77180,#77181),(#77182,#77183),(#77184,#77185),(#77186,#77187),(#77188,
#77189),(#77190,#77191),(#77192,#77193),(#77194,#77195),(#77196,#77197),
(#77198,#77199),(#77200,#77201),(#77202,#77203),(#77204,#77205),(#77206,
#77207),(#77208,#77209),(#77210,#77211),(#77212,#77213),(#77214,#77215),
(#77216,#77217),(#77218,#77219),(#77220,#77221),(#77222,#77223),(#77224,
#77225),(#77226,#77227),(#77228,#77229),(#77230,#77231),(#77232,#77233),
(#77234,#77235),(#77236,#77237),(#77238,#77239),(#77240,#77241),(#77242,
#77243),(#77244,#77245),(#77246,#77247),(#77248,#77249),(#77250,#77251),
(#77252,#77253),(#77254,#77255),(#77256,#77257),(#77258,#77259),(#77260,
#77261),(#77262,#77263),(#77264,#77265),(#77266,#77267),(#77268,#77269),
(#77270,#77271),(#77272,#77273),(#77274,#77275),(#77276,#77277),(#77278,
#77279),(#77280,#77281),(#77282,#77283),(#77284,#77285),(#77286,#77287),
(#77288,#77289),(#77290,#77291),(#77292,#77293),(#77294,#77295),(#77296,
#77297),(#77298,#77299),(#77300,#77301),(#77302,#77303),(#77304,#77305),
(#77306,#77307),(#77308,#77309),(#77310,#77311),(#77312,#77313),(#77314,
#77315),(#77316,#77317),(#77318,#77319),(#77320,#77321),(#77322,#77323),
(#77324,#77325),(#77326,#77327),(#77328,#77329),(#77330,#77331),(#77332,
#77333),(#77334,#77335),(#77336,#77337),(#77338,#77339),(#77340,#77341),
(#77342,#77343),(#77344,#77345),(#77346,#77347),(#77348,#77349),(#77350,
#77351),(#77352,#77353),(#77354,#77355),(#77356,#77357),(#77358,#77359),
(#77360,#77361),(#77362,#77363),(#77364,#77365),(#77366,#77367),(#77368,
#77369),(#77370,#77371),(#77372,#77373),(#77374,#77375),(#77376,#77377),
(#77378,#77379),(#77380,#77381),(#77382,#77383),(#77384,#77385),(#77386,
#77387),(#77388,#77389),(#77390,#77391),(#77392,#77393),(#77394,#77395),
(#77396,#77397),(#77398,#77399),(#77400,#77401),(#77402,#77403),(#77404,
#77405),(#77406,#77407),(#77408,#77409),(#77410,#77411),(#77412,#77413),
(#77414,#77415),(#77416,#77417),(#77418,#77419),(#77420,#77421),(#77422,
#77423),(#77424,#77425),(#77426,#77427),(#77428,#77429),(#77430,#77431),
(#77432,#77433),(#77434,#77435),(#77436,#77437),(#77438,#77439),(#77440,
#77441),(#77442,#77443),(#77444,#77445),(#77446,#77447),(#77448,#77449),
(#77450,#77451),(#77452,#77453),(#77454,#77455),(#77456,#77457),(#77458,
#77459),(#77460,#77461),(#77462,#77463),(#77464,#77465),(#77466,#77467),
(#77468,#77469),(#77470,#77471),(#77472,#77473),(#77474,#77475),(#77476,
#77477),(#77478,#77479),(#77480,#77481),(#77482,#77483),(#77484,#77485),
(#77486,#77487),(#77488,#77489),(#77490,#77491),(#77492,#77493),(#77494,
#77495),(#77496,#77497),(#77498,#77499),(#77500,#77501),(#77502,#77503),
(#77504,#77505),(#77506,#77507),(#77508,#77509),(#77510,#77511),(#77512,
#77513),(#77514,#77515),(#77516,#77517),(#77518,#77519),(#77520,#77521),
(#77522,#77523),(#77524,#77525),(#77526,#77527),(#77528,#77529),(#77530,
#77531),(#77532,#77533),(#77534,#77535),(#77536,#77537),(#77538,#77539),
(#77540,#77541),(#77542,#77543),(#77544,#77545),(#77546,#77547),(#77548,
#77549),(#77550,#77551),(#77552,#77553),(#77554,#77555),(#77556,#77557),
(#77558,#77559),(#77560,#77561),(#77562,#77563),(#77564,#77565),(#77566,
#77567),(#77568,#77569),(#77570,#77571),(#77572,#77573),(#77574,#77575),
(#77576,#77577),(#77578,#77579),(#77580,#77581),(#77582,#77583),(#77584,
#77585),(#77586,#77587),(#77588,#77589),(#77590,#77591),(#77592,#77593),
(#77594,#77595),(#77596,#77597),(#77598,#77599),(#77600,#77601),(#77602,
#77603),(#77604,#77605),(#77606,#77607),(#77608,#77609),(#77610,#77611),
(#77612,#77613),(#77614,#77615),(#77616,#77617),(#77618,#77619),(#77620,
#77621),(#77622,#77623),(#77624,#77625),(#77626,#77627),(#77628,#77629),
(#77630,#77631),(#77632,#77633),(#77634,#77635),(#77636,#77637),(#77638,
#77639),(#77640,#77641),(#77642,#77643),(#77644,#77645),(#77646,#77647),
(#77648,#77649),(#77650,#77651),(#77652,#77653),(#77654,#77655),(#77656,
#77657),(#77658,#77659),(#77660,#77661),(#77662,#77663),(#77664,#77665),
(#77666,#77667),(#77668,#77669),(#77670,#77671),(#77672,#77673),(#77674,
#77675),(#77676,#77677),(#77678,#77679),(#77680,#77681),(#77682,#77683),
(#77684,#77685),(#77686,#77687),(#77688,#77689),(#77690,#77691),(#77692,
#77693),(#77694,#77695),(#77696,#77697),(#77698,#77699),(#77700,#77701),
(#77702,#77703),(#77704,#77705),(#77706,#77707),(#77708,#77709),(#77710,
#77711),(#77712,#77713),(#77714,#77715),(#77716,#77717),(#77718,#77719),
(#77720,#77721),(#77722,#77723),(#77724,#77725),(#77726,#77727),(#77728,
#77729),(#77730,#77731),(#77732,#77733),(#77734,#77735),(#77736,#77737),
(#77738,#77739),(#77740,#77741),(#77742,#77743),(#77744,#77745),(#77746,
#77747),(#77748,#77749),(#77750,#77751),(#77752,#77753),(#77754,#77755),
(#77756,#77757),(#77758,#77759),(#77760,#77761),(#77762,#77763),(#77764,
#77765),(#77766,#77767),(#77768,#77769),(#77770,#77771),(#77772,#77773),
(#77774,#77775),(#77776,#77777),(#77778,#77779),(#77780,#77781),(#77782,
#77783),(#77784,#77785),(#77786,#77787),(#77788,#77789),(#77790,#77791),
(#77792,#77793),(#77794,#77795),(#77796,#77797),(#77798,#77799),(#77800,
#77801),(#77802,#77803),(#77804,#77805),(#77806,#77807),(#77808,#77809),
(#77810,#77811),(#77812,#77813),(#77814,#77815),(#77816,#77817),(#77818,
#77819),(#77820,#77821),(#77822,#77823),(#77824,#77825),(#77826,#77827),
(#77828,#77829),(#77830,#77831),(#77832,#77833),(#77834,#77835),(#77836,
#77837),(#77838,#77839),(#77840,#77841),(#77842,#77843),(#77844,#77845),
(#77846,#77847),(#77848,#77849),(#77850,#77851),(#77852,#77853),(#77854,
#77855),(#77856,#77857),(#77858,#77859),(#77860,#77861),(#77862,#77863),
(#77864,#77865),(#77866,#77867),(#77868,#77869),(#77870,#77871),(#77872,
#77873),(#77874,#77875),(#77876,#77877),(#77878,#77879),(#77880,#77881),
(#77882,#77883),(#77884,#77885),(#77886,#77887),(#77888,#77889),(#77890,
#77891),(#77892,#77893),(#77894,#77895),(#77896,#77897),(#77898,#77899),
(#77900,#77901),(#77902,#77903),(#77904,#77905),(#77906,#77907),(#77908,
#77909),(#77910,#77911),(#77912,#77913),(#77914,#77915),(#77916,#77917),
(#77918,#77919),(#77920,#77921),(#77922,#77923),(#77924,#77925),(#77926,
#77927),(#77928,#77929),(#77930,#77931),(#77932,#77933),(#77934,#77935),
(#77936,#77937),(#77938,#77939),(#77940,#77941),(#77942,#77943),(#77944,
#77945),(#77946,#77947),(#77948,#77949),(#77950,#77951),(#77952,#77953),
(#77954,#77955),(#77956,#77957),(#77958,#77959),(#77960,#77961),(#77962,
#77963),(#77964,#77965),(#77966,#77967),(#77968,#77969),(#77970,#77971),
(#77972,#77973),(#77974,#77975),(#77976,#77977),(#77978,#77979),(#77980,
#77981),(#77982,#77983),(#77984,#77985),(#77986,#77987),(#77988,#77989),
(#77990,#77991),(#77992,#77993),(#77994,#77995),(#77996,#77997),(#77998,
#77999),(#78000,#78001),(#78002,#78003),(#78004,#78005),(#78006,#78007),
(#78008,#78009),(#78010,#78011),(#78012,#78013),(#78014,#78015),(#78016,
#78017),(#78018,#78019),(#78020,#78021),(#78022,#78023),(#78024,#78025),
(#78026,#78027),(#78028,#78029),(#78030,#78031),(#78032,#78033),(#78034,
#78035),(#78036,#78037),(#78038,#78039),(#78040,#78041),(#78042,#78043),
(#78044,#78045),(#78046,#78047),(#78048,#78049),(#78050,#78051),(#78052,
#78053),(#78054,#78055),(#78056,#78057),(#78058,#78059),(#78060,#78061),
(#78062,#78063),(#78064,#78065),(#78066,#78067),(#78068,#78069),(#78070,
#78071),(#78072,#78073),(#78074,#78075),(#78076,#78077),(#78078,#78079),
(#78080,#78081),(#78082,#78083),(#78084,#78085),(#78086,#78087),(#78088,
#78089),(#78090,#78091),(#78092,#78093),(#78094,#78095),(#78096,#78097),
(#78098,#78099),(#78100,#78101),(#78102,#78103),(#78104,#78105),(#78106,
#78107),(#78108,#78109),(#78110,#78111),(#78112,#78113),(#78114,#78115),
(#78116,#78117),(#78118,#78119),(#78120,#78121),(#78122,#78123),(#78124,
#78125),(#78126,#78127),(#78128,#78129),(#78130,#78131),(#78132,#78133),
(#78134,#78135),(#78136,#78137),(#78138,#78139),(#78140,#78141),(#78142,
#78143),(#78144,#78145),(#78146,#78147),(#78148,#78149),(#78150,#78151),
(#78152,#78153),(#78154,#78155),(#78156,#78157),(#78158,#78159),(#78160,
#78161),(#78162,#78163),(#78164,#78165),(#78166,#78167),(#78168,#78169),
(#78170,#78171),(#78172,#78173),(#78174,#78175),(#78176,#78177),(#78178,
#78179),(#78180,#78181),(#78182,#78183),(#78184,#78185),(#78186,#78187),
(#78188,#78189),(#78190,#78191),(#78192,#78193),(#78194,#78195),(#78196,
#78197),(#78198,#78199),(#78200,#78201),(#78202,#78203),(#78204,#78205),
(#78206,#78207),(#78208,#78209),(#78210,#78211),(#78212,#78213),(#78214,
#78215),(#78216,#78217),(#78218,#78219),(#78220,#78221),(#78222,#78223),
(#78224,#78225),(#78226,#78227),(#78228,#78229),(#78230,#78231),(#78232,
#78233),(#78234,#78235),(#78236,#78237),(#78238,#78239),(#78240,#78241),
(#78242,#78243),(#78244,#78245),(#78246,#78247),(#78248,#78249),(#78250,
#78251),(#78252,#78253),(#78254,#78255),(#78256,#78257),(#78258,#78259),
(#78260,#78261),(#78262,#78263),(#78264,#78265),(#78266,#78267),(#78268,
#78269),(#78270,#78271),(#78272,#78273),(#78274,#78275),(#78276,#78277),
(#78278,#78279),(#78280,#78281),(#78282,#78283),(#78284,#78285),(#78286,
#78287),(#78288,#78289),(#78290,#78291),(#78292,#78293),(#78294,#78295),
(#78296,#78297),(#78298,#78299),(#78300,#78301),(#78302,#78303),(#78304,
#78305),(#78306,#78307),(#78308,#78309),(#78310,#78311),(#78312,#78313),
(#78314,#78315),(#78316,#78317),(#78318,#78319),(#78320,#78321),(#78322,
#78323),(#78324,#78325),(#78326,#78327),(#78328,#78329),(#78330,#78331),
(#78332,#78333),(#78334,#78335),(#78336,#78337),(#78338,#78339),(#78340,
#78341),(#78342,#78343),(#78344,#78345),(#78346,#78347),(#78348,#78349),
(#78350,#78351),(#78352,#78353),(#78354,#78355),(#78356,#78357),(#78358,
#78359),(#78360,#78361),(#78362,#78363),(#78364,#78365),(#78366,#78367),
(#78368,#78369),(#78370,#78371),(#78372,#78373),(#78374,#78375),(#78376,
#78377),(#78378,#78379),(#78380,#78381),(#78382,#78383),(#78384,#78385),
(#78386,#78387),(#78388,#78389),(#78390,#78391),(#78392,#78393),(#78394,
#78395),(#78396,#78397),(#78398,#78399),(#78400,#78401),(#78402,#78403),
(#78404,#78405),(#78406,#78407),(#78408,#78409),(#78410,#78411),(#78412,
#78413),(#78414,#78415),(#78416,#78417),(#78418,#78419),(#78420,#78421),
(#78422,#78423),(#78424,#78425),(#78426,#78427),(#78428,#78429),(#78430,
#78431),(#78432,#78433),(#78434,#78435),(#78436,#78437),(#78438,#78439),
(#78440,#78441),(#78442,#78443),(#78444,#78445),(#78446,#78447),(#78448,
#78449),(#78450,#78451),(#78452,#78453),(#78454,#78455),(#78456,#78457),
(#78458,#78459),(#78460,#78461),(#78462,#78463),(#78464,#78465),(#78466,
#78467),(#78468,#78469),(#78470,#78471),(#78472,#78473),(#78474,#78475),
(#78476,#78477),(#78478,#78479),(#78480,#78481),(#78482,#78483),(#78484,
#78485),(#78486,#78487),(#78488,#78489),(#78490,#78491),(#78492,#78493),
(#78494,#78495),(#78496,#78497),(#78498,#78499),(#78500,#78501),(#78502,
#78503),(#78504,#78505),(#78506,#78507),(#78508,#78509),(#78510,#78511),
(#78512,#78513),(#78514,#78515),(#78516,#78517),(#78518,#78519),(#78520,
#78521),(#78522,#78523),(#78524,#78525),(#78526,#78527),(#78528,#78529),
(#78530,#78531),(#78532,#78533),(#78534,#78535),(#78536,#78537),(#78538,
#78539),(#78540,#78541),(#78542,#78543),(#78544,#78545),(#78546,#78547),
(#78548,#78549),(#78550,#78551),(#78552,#78553),(#78554,#78555),(#78556,
#78557),(#78558,#78559),(#78560,#78561),(#78562,#78563),(#78564,#78565),
(#78566,#78567),(#78568,#78569),(#78570,#78571),(#78572,#78573),(#78574,
#78575),(#78576,#78577),(#78578,#78579),(#78580,#78581),(#78582,#78583),
(#78584,#78585),(#78586,#78587),(#78588,#78589),(#78590,#78591),(#78592,
#78593),(#78594,#78595),(#78596,#78597),(#78598,#78599),(#78600,#78601),
(#78602,#78603),(#78604,#78605),(#78606,#78607),(#78608,#78609),(#78610,
#78611),(#78612,#78613),(#78614,#78615),(#78616,#78617),(#78618,#78619),
(#78620,#78621),(#78622,#78623),(#78624,#78625),(#78626,#78627),(#78628,
#78629),(#78630,#78631),(#78632,#78633),(#78634,#78635),(#78636,#78637),
(#78638,#78639),(#78640,#78641),(#78642,#78643),(#78644,#78645),(#78646,
#78647),(#78648,#78649),(#78650,#78651),(#78652,#78653),(#78654,#78655),
(#78656,#78657),(#78658,#78659),(#78660,#78661),(#78662,#78663),(#78664,
#78665),(#78666,#78667),(#78668,#78669),(#78670,#78671),(#78672,#78673),
(#78674,#78675),(#78676,#78677),(#78678,#78679),(#78680,#78681),(#78682,
#78683),(#78684,#78685),(#78686,#78687),(#78688,#78689),(#78690,#78691),
(#78692,#78693),(#78694,#78695),(#78696,#78697),(#78698,#78699),(#78700,
#78701),(#78702,#78703),(#78704,#78705),(#78706,#78707),(#78708,#78709),
(#78710,#78711),(#78712,#78713),(#78714,#78715),(#78716,#78717),(#78718,
#78719),(#78720,#78721),(#78722,#78723),(#78724,#78725),(#78726,#78727),
(#78728,#78729),(#78730,#78731),(#78732,#78733),(#78734,#78735),(#78736,
#78737),(#78738,#78739),(#78740,#78741),(#78742,#78743),(#78744,#78745),
(#78746,#78747),(#78748,#78749),(#78750,#78751),(#78752,#78753),(#78754,
#78755),(#78756,#78757),(#78758,#78759),(#78760,#78761),(#78762,#78763),
(#78764,#78765),(#78766,#78767),(#78768,#78769),(#78770,#78771),(#78772,
#78773),(#78774,#78775),(#78776,#78777),(#78778,#78779),(#78780,#78781),
(#78782,#78783),(#78784,#78785),(#78786,#78787),(#78788,#78789),(#78790,
#78791),(#78792,#78793),(#78794,#78795),(#78796,#78797),(#78798,#78799),
(#78800,#78801),(#78802,#78803),(#78804,#78805),(#78806,#78807),(#78808,
#78809),(#78810,#78811),(#78812,#78813),(#78814,#78815),(#78816,#78817),
(#78818,#78819),(#78820,#78821),(#78822,#78823),(#78824,#78825),(#78826,
#78827),(#78828,#78829),(#78830,#78831),(#78832,#78833),(#78834,#78835),
(#78836,#78837),(#78838,#78839),(#78840,#78841),(#78842,#78843),(#78844,
#78845),(#78846,#78847),(#78848,#78849),(#78850,#78851),(#78852,#78853),
(#78854,#78855),(#78856,#78857),(#78858,#78859),(#78860,#78861),(#78862,
#78863),(#78864,#78865),(#78866,#78867),(#78868,#78869),(#78870,#78871),
(#78872,#78873),(#78874,#78875),(#78876,#78877),(#78878,#78879),(#78880,
#78881),(#78882,#78883),(#78884,#78885),(#78886,#78887),(#78888,#78889),
(#78890,#78891),(#78892,#78893),(#78894,#78895),(#78896,#78897),(#78898,
#78899),(#78900,#78901),(#78902,#78903),(#78904,#78905),(#78906,#78907),
(#78908,#78909),(#78910,#78911),(#78912,#78913),(#78914,#78915),(#78916,
#78917),(#78918,#78919),(#78920,#78921),(#78922,#78923),(#78924,#78925),
(#78926,#78927),(#78928,#78929),(#78930,#78931),(#78932,#78933),(#78934,
#78935),(#78936,#78937),(#78938,#78939),(#78940,#78941),(#78942,#78943),
(#78944,#78945),(#78946,#78947),(#78948,#78949),(#78950,#78951),(#78952,
#78953),(#78954,#78955),(#78956,#78957),(#78958,#78959),(#78960,#78961),
(#78962,#78963),(#78964,#78965),(#78966,#78967),(#78968,#78969),(#78970,
#78971),(#78972,#78973),(#78974,#78975),(#78976,#78977),(#78978,#78979)),
 .UNSPECIFIED.,.F.,.F.,.F.,(4,1,1,1,1,1,1,1,1,1,1,1,1,1,1,1,1,1,1,1,1,1,
1,1,1,1,1,1,1,1,1,1,1,1,1,1,1,1,1,1,1,1,1,1,1,1,1,1,1,1,1,1,1,1,1,1,1,1,
1,1,1,1,1,1,1,1,1,1,1,1,1,1,1,1,1,1,1,1,1,1,1,1,1,1,1,1,1,1,1,1,1,1,1,1,
1,1,1,1,1,1,1,1,1,1,1,1,1,1,1,1,1,1,1,1,1,1,1,1,1,1,1,1,1,1,1,1,1,1,1,1,
1,1,1,1,1,1,1,1,1,1,1,1,1,1,1,1,1,1,1,1,1,1,1,1,1,1,1,1,1,1,1,1,1,1,1,1,
1,1,1,1,1,1,1,1,1,1,1,1,1,1,1,1,1,1,1,1,1,1,1,1,1,1,1,1,1,1,1,1,1,1,1,1,
1,1,1,1,1,1,1,1,1,1,1,1,1,1,1,1,1,1,1,1,1,1,1,1,1,1,1,1,1,1,1,1,1,1,1,1,
1,1,1,1,1,1,1,1,1,1,1,1,1,1,1,1,1,1,1,1,1,1,1,1,1,1,1,1,1,1,1,1,1,1,1,1,
1,1,1,1,1,1,1,1,1,1,1,1,1,1,1,1,1,1,1,1,1,1,1,1,1,1,1,1,1,1,1,1,1,1,1,1,
1,1,1,1,1,1,1,1,1,1,1,1,1,1,1,1,1,1,1,1,1,1,1,1,1,1,1,1,1,1,1,1,1,1,1,1,
1,1,1,1,1,1,1,1,1,1,1,1,1,1,1,1,1,1,1,1,1,1,1,1,1,1,1,1,1,1,1,1,1,1,1,1,
1,1,1,1,1,1,1,1,1,1,1,1,1,1,1,1,1,1,1,1,1,1,1,1,1,1,1,1,1,1,1,1,1,1,1,1,
1,1,1,1,1,1,1,1,1,1,1,1,1,1,1,1,1,1,1,1,1,1,1,1,1,1,1,1,1,1,1,1,1,1,1,1,
1,1,1,1,1,1,1,1,1,1,1,1,1,1,1,1,1,1,1,1,1,1,1,1,1,1,1,1,1,1,1,1,1,1,1,1,
1,1,1,1,1,1,1,1,1,1,1,1,1,1,1,1,1,1,1,1,1,1,1,1,1,1,1,1,1,1,1,1,1,1,1,1,
1,1,1,1,1,1,1,1,1,1,1,1,1,1,1,1,1,1,1,1,1,1,1,1,1,1,1,1,1,1,1,1,1,1,1,1,
1,1,1,1,1,1,1,1,1,1,1,1,1,1,1,1,1,1,1,1,1,1,1,1,1,1,1,1,1,1,1,1,1,1,1,1,
1,1,1,1,1,1,1,1,1,1,1,1,1,1,1,1,1,1,1,1,1,1,1,1,1,1,1,1,1,1,1,1,1,1,1,1,
1,1,1,1,1,1,1,1,1,1,1,1,1,1,1,1,1,1,1,1,1,1,1,1,1,1,1,1,1,1,1,1,1,1,1,1,
1,1,1,1,1,1,1,1,1,1,1,1,1,1,1,1,1,1,1,1,1,1,1,1,1,1,1,1,1,1,1,1,1,1,1,1,
1,1,1,1,1,1,1,1,1,1,1,1,1,1,1,1,1,1,1,1,1,1,1,1,1,1,1,1,1,1,1,1,1,1,1,1,
1,1,1,1,1,1,1,1,1,1,1,1,1,1,1,1,1,1,1,1,1,1,1,1,1,1,1,1,1,1,1,1,1,1,1,1,
1,1,1,1,1,1,1,1,1,1,1,1,1,1,1,1,1,1,1,1,1,1,1,1,1,1,1,1,1,1,1,1,1,1,1,1,
1,1,1,1,1,1,1,1,1,1,1,1,1,1,1,1,1,1,1,1,1,1,1,1,1,1,1,1,1,1,1,1,1,1,1,1,
1,1,1,1,1,1,1,1,1,1,1,1,1,1,1,1,1,1,1,1,1,1,1,1,1,1,1,1,1,1,1,1,1,1,1,1,
1,1,1,1,1,1,1,1,1,1,1,1,1,1,1,1,1,1,1,1,1,1,1,1,1,1,1,1,1,1,1,1,1,1,1,1,
1,1,1,1,1,1,1,1,1,1,1,1,1,1,1,1,1,1,1,1,1,1,1,1,1,1,1,1,1,1,1,1,1,1,1,1,
1,1,1,1,1,1,1,1,1,1,1,1,1,1,1,1,1,1,1,1,1,1,1,1,1,1,1,1,1,1,1,1,1,1,1,1,
1,1,1,1,1,1,1,1,1,1,1,1,1,1,1,1,1,1,1,1,1,1,1,1,1,1,1,1,1,1,1,1,1,1,1,1,
1,1,1,1,1,1,1,1,1,1,1,1,1,1,1,1,1,1,1,1,1,1,1,1,1,1,1,1,1,1,1,1,1,1,1,1,
1,1,1,1,1,1,1,1,1,1,1,1,1,1,1,1,1,1,1,1,1,1,1,1,1,1,1,1,1,1,1,1,1,1,1,1,
1,1,1,1,1,1,1,1,1,1,1,1,1,1,1,1,1,1,1,1,1,1,1,1,1,1,1,1,1,1,1,1,1,1,1,1,
1,1,1,1,1,1,1,1,1,1,1,1,1,1,1,1,1,1,1,1,1,1,1,1,1,1,1,1,1,1,1,1,1,1,1,1,
1,1,1,1,1,1,1,1,1,1,1,1,1,1,1,1,1,1,1,1,1,1,1,1,1,1,1,1,1,1,1,1,1,1,1,1,
1,1,1,1,1,1,1,1,1,1,1,1,1,1,1,1,1,1,1,1,1,1,1,1,1,1,1,1,1,1,1,1,1,1,1,1,
1,1,1,1,1,1,1,1,1,1,1,1,1,1,1,1,1,1,1,1,1,1,1,1,1,1,1,1,1,1,1,1,1,1,1,1,
1,1,1,1,1,1,1,1,1,1,1,1,1,1,1,1,1,1,1,1,1,1,1,1,1,1,1,1,1,1,1,1,1,1,1,1,
1,1,1,1,1,1,1,1,1,1,1,1,1,1,1,1,1,1,1,1,1,1,1,1,1,1,1,1,1,1,1,1,1,1,1,1,
1,1,1,1,1,1,1,1,1,1,1,1,1,1,1,1,1,1,1,1,1,1,1,1,1,1,1,1,1,1,1,1,1,1,1,1,
1,1,1,1,1,1,1,1,1,1,1,1,1,1,1,1,1,1,1,1,1,1,1,1,1,1,1,1,1,1,1,1,1,1,1,1,
1,1,1,1,1,1,1,1,1,1,1,1,1,1,1,1,1,1,1,1,1,1,1,1,1,1,1,1,1,1,1,1,1,1,1,1,
1,1,1,1,1,1,1,1,1,1,1,1,1,1,1,1,1,1,1,1,1,1,1,1,1,1,1,1,1,1,1,1,1,1,1,1,
1,1,1,1,1,1,1,1,1,1,1,1,1,1,1,1,1,1,1,1,1,1,1,1,1,1,1,1,1,1,1,1,1,1,1,1,
1,1,1,1,1,1,1,1,1,1,1,1,1,1,1,1,1,1,1,1,1,1,1,1,1,1,1,1,1,1,1,1,1,1,1,1,
1,1,1,1,1,1,1,1,1,1,1,1,1,1,1,1,1,1,1,1,1,1,1,1,1,1,1,1,1,1,1,1,1,1,1,1,
1,1,1,1,1,1,1,1,1,1,1,1,1,1,1,1,1,1,1,1,1,1,1,1,1,1,1,1,1,1,1,1,1,1,1,1,
1,1,1,1,1,1,1,1,1,1,1,1,1,1,1,1,1,1,1,1,1,1,1,1,1,1,1,1,1,1,1,1,1,1,1,1,
1,1,1,1,1,1,1,1,1,1,1,1,1,1,1,1,1,1,1,1,1,1,1,1,1,1,1,1,1,1,1,1,1,1,1,1,
1,1,1,1,1,1,1,1,1,1,1,1,1,1,1,1,1,1,1,1,1,1,1,1,1,1,1,1,1,1,1,1,1,1,1,1,
1,1,1,1,1,1,1,1,1,1,1,1,1,1,1,1,1,1,1,1,1,1,1,1,1,1,1,1,1,1,1,1,1,1,1,1,
1,1,1,1,1,1,1,1,1,1,1,1,1,1,1,1,1,1,1,1,1,1,1,1,1,1,1,1,1,1,1,1,1,1,1,1,
1,1,1,1,1,1,1,1,1,1,1,1,1,1,1,1,1,1,1,1,1,1,1,1,1,1,1,1,1,1,1,1,1,1,1,1,
1,1,1,1,1,1,1,1,1,1,1,1,1,1,1,1,1,1,1,1,1,1,1,1,1,1,1,1,1,1,1,1,1,1,1,1,
1,1,1,1,1,1,1,1,1,1,1,1,1,1,1,1,1,1,1,1,1,1,1,1,1,1,1,1,1,1,1,1,1,1,1,1,
1,1,1,1,1,1,1,1,1,1,1,1,1,1,1,1,1,1,1,1,1,1,1,1,1,1,1,1,1,1,1,1,1,1,1,1,
1,1,1,1,1,1,1,1,1,1,1,1,1,1,1,1,1,1,1,1,1,1,1,1,1,1,1,1,1,1,1,1,1,1,1,1,
1,1,1,1,1,1,1,1,1,1,1,1,1,1,1,1,1,1,1,1,1,1,1,1,1,1,1,1,1,1,1,1,1,1,1,1,
1,1,1,1,1,1,1,1,1,1,1,1,1,1,1,1,1,1,1,1,1,1,1,1,1,1,1,1,1,1,1,1,1,1,1,1,
1,1,1,1,1,1,1,1,1,1,1,1,1,1,1,1,1,1,1,1,1,1,1,1,1,1,1,1,1,1,1,1,1,1,1,1,
1,1,1,1,1,1,1,1,1,1,1,1,1,1,1,1,1,1,1,1,1,1,1,1,1,1,1,1,1,1,1,1,1,1,1,1,
1,1,1,1,1,1,1,1,1,1,1,1,1,1,1,1,1,1,1,1,1,1,1,1,1,1,1,1,1,1,1,1,1,1,1,1,
1,1,1,1,1,1,1,1,1,1,1,1,1,1,1,1,1,1,1,1,1,1,1,1,1,1,1,1,1,1,1,1,1,1,1,1,
1,1,1,1,1,1,1,1,1,1,1,1,1,1,1,1,1,1,1,1,1,1,1,1,1,1,1,1,1,1,1,1,1,1,1,1,
1,1,1,1,1,1,1,1,1,1,1,1,1,1,1,1,1,1,1,1,1,1,1,1,1,1,1,1,1,1,1,1,1,1,1,1,
1,1,1,1,1,1,1,1,1,1,1,1,1,1,1,1,1,1,1,1,1,1,1,1,1,1,1,1,1,1,1,1,1,1,1,1,
1,1,1,1,1,1,1,1,1,1,1,1,1,1,1,1,1,1,1,1,1,1,1,1,1,1,1,1,1,1,1,1,1,1,1,1,
1,1,1,1,1,1,1,1,1,1,1,1,1,1,1,1,1,1,1,1,1,1,1,1,1,1,1,1,1,1,1,1,1,1,1,1,
1,1,1,1,1,1,1,1,1,1,1,1,1,1,1,1,1,1,1,1,1,1,1,1,1,1,1,1,1,1,1,1,1,1,1,1,
1,1,1,1,1,1,1,1,1,1,1,1,1,1,1,1,1,1,1,1,1,1,1,1,1,1,1,1,1,1,1,1,1,1,1,1,
1,1,1,1,1,1,1,1,1,1,1,1,1,1,1,1,1,1,1,1,1,1,1,1,1,1,1,1,1,1,1,1,1,1,1,1,
1,1,1,1,1,1,1,1,1,1,1,1,1,1,1,1,1,1,1,1,1,1,1,1,1,1,1,1,1,1,1,1,1,1,1,1,
1,1,1,1,1,1,1,1,1,1,1,1,1,1,1,1,1,1,1,1,1,1,1,1,1,1,1,1,1,1,1,1,1,1,1,1,
1,1,1,1,1,1,1,1,1,1,1,1,1,1,1,1,1,1,1,1,1,1,1,1,1,1,1,1,1,1,1,1,1,1,1,1,
1,1,1,1,1,1,1,1,1,1,1,1,1,1,1,1,1,1,1,1,1,1,1,1,1,1,1,1,1,1,1,1,1,1,1,1,
1,1,1,1,1,1,1,1,1,1,1,1,1,1,1,1,1,1,1,1,1,1,1,1,1,1,1,1,1,1,1,1,1,1,1,1,
1,1,1,1,1,1,1,1,1,1,1,1,1,1,1,1,1,1,1,1,1,1,1,1,1,1,1,1,1,1,1,1,1,1,1,1,
1,1,1,1,1,1,1,1,1,1,1,1,1,1,1,1,1,1,1,1,1,1,1,1,1,1,1,1,1,1,1,1,1,1,1,1,
1,1,1,1,1,1,1,1,1,1,1,1,1,1,1,1,1,1,1,1,1,1,1,1,1,1,1,1,1,1,1,1,1,1,1,1,
1,1,1,1,1,1,1,1,1,1,1,1,1,1,1,1,1,1,1,1,1,1,1,1,1,1,1,1,1,1,1,1,1,1,1,1,
1,1,1,1,1,1,1,1,1,1,1,1,1,1,1,1,1,1,1,1,1,1,1,1,1,1,1,1,1,1,1,1,1,1,1,1,
1,1,1,1,1,1,1,1,1,1,1,1,1,1,1,1,1,1,1,1,1,1,1,1,1,1,1,1,1,1,1,1,1,1,1,1,
1,1,1,1,1,1,1,1,1,1,1,1,1,1,1,1,1,1,1,1,1,1,1,1,1,1,1,1,1,1,1,1,1,1,1,1,
1,1,1,1,1,1,1,1,1,1,1,1,1,1,1,1,1,1,1,1,1,1,1,1,1,1,1,1,1,1,1,1,1,1,1,1,
1,1,1,1,1,1,1,1,1,1,1,1,1,1,1,1,1,1,1,1,1,1,1,1,1,1,1,1,1,1,1,1,1,1,1,1,
1,1,1,1,1,1,1,1,1,1,1,1,1,1,1,1,1,1,1,1,1,1,1,1,1,1,1,1,1,1,1,1,1,1,1,1,
1,1,1,1,1,1,1,1,1,1,1,1,1,1,1,1,1,1,1,1,1,1,1,1,1,1,1,1,1,1,1,1,1,1,1,1,
1,1,1,1,1,1,1,1,1,1,1,1,1,1,1,1,1,1,1,1,1,1,1,1,1,1,1,1,1,1,1,1,1,1,1,1,
1,1,1,1,1,1,1,1,1,1,1,1,1,1,1,1,1,1,1,1,1,1,1,1,1,1,1,1,1,1,1,1,1,1,1,1,
1,1,1,1,1,1,1,1,1,1,1,1,1,1,1,1,1,1,1,1,1,1,1,1,1,1,1,1,1,1,1,1,1,1,1,1,
1,1,1,1,1,1,1,1,1,1,1,1,1,1,1,1,1,1,1,1,1,1,1,1,1,1,1,1,1,1,1,1,1,1,1,1,
1,1,1,1,1,1,1,1,1,1,1,1,1,1,1,1,1,1,1,1,1,1,1,1,1,1,1,1,1,1,1,1,1,1,1,1,
1,1,1,1,1,1,1,1,1,1,1,1,1,1,1,1,1,1,1,1,1,1,1,1,1,1,1,1,1,1,1,1,1,1,1,1,
1,1,1,1,1,1,1,1,1,1,1,1,1,1,1,1,1,1,1,1,1,1,1,1,1,1,1,1,1,1,1,1,1,1,1,1,
1,1,1,1,1,1,1,1,1,1,1,1,1,1,1,1,1,1,1,1,1,1,1,1,1,1,1,1,1,1,1,1,1,1,1,1,
1,1,1,1,1,1,1,1,1,1,1,1,1,1,1,1,1,1,1,1,1,1,1,1,1,1,1,1,1,1,1,1,1,1,1,1,
1,1,1,1,1,1,1,1,1,1,1,1,1,1,1,1,1,1,1,1,1,1,1,1,1,1,1,1,1,1,1,1,1,1,1,1,
1,1,1,1,1,1,1,1,1,1,1,1,1,1,1,1,1,1,1,1,1,1,1,1,1,1,1,1,1,1,1,1,1,1,1,1,
1,1,1,1,4),(2,2),(0.,0.869746702321014,1.7394931589914,2.60923976624962,
3.47983908319159,4.35043840179749,5.22018503077054,6.08993165951504,6.95967828799171,
7.82942491616733,8.69917154401062,9.56891817149224,10.4395174886835,11.3101168056706,
12.179863432132,13.049610058144,13.9193566836854,14.7891033087372,15.6588499332817,
16.5285965573034,17.3991958717975,18.2697951860185,18.7046684974166,19.1395418086746,
19.5744151197912,20.0092884307654,20.4441617415962,20.8790350522825,21.7487816732187,
22.1836549834672,22.6185282935685,23.0534016035221,23.4882749133276,23.9231482229848,
24.3588742245859,24.794600226187,25.2294735355468,26.0992201538203,26.5340934627341,
26.9689667714994,27.4038400801166,27.838713388586,28.2735866969081,28.7084600050832,
29.143333313112,29.5782066209952,30.0130799287334,30.4479532363275,30.8828265437783,
31.3185525442794,31.7542785447804,32.1891518519474,32.6240251589741,33.0588984658616,
33.4937717726112,33.928645079224,34.3635183857014,34.7983916920448,35.2332649982556,
35.6681383043353,36.1030116102854,36.5378849161076,36.9727582218035,37.4076315273749,
37.8425048328235,38.2782308323341,38.7139568318446,39.1488301370532,39.5837034421446,
40.0185767471208,40.4534500519838,40.8883233567357,41.3231966613787,41.7580699659148,
42.1929432703463,42.6278165746754,43.0626898789044,43.4975631830356,43.9324364870714,
44.3673097910142,44.8021830948664,45.2379090935952,45.673635092324,46.1085083960024,
46.5433816995978,46.9782550031127,47.4131283065497,47.8480016099115,48.2828749132006,
48.7177482164198,49.1526215195718,49.5874948226593,50.0223681256851,50.457241428652,
50.8921147315628,51.3269880344203,51.7618613372274,52.197587335454,52.6333133336805,
53.0681866363954,53.5030599390685,53.9379332417027,54.3728065443011,54.8076798468664,
55.2425531494018,55.6774264519101,56.1122997543943,56.5471730568575,56.9820463593026,
57.4169196617326,57.8517929641506,58.2866662665595,58.7215395689624,59.157265567009,
59.5929915650557,60.0278648674556,60.4627381698584,60.8976114722673,61.3324847746853,
61.7673580771153,62.2022313795604,62.6371046820236,63.0719779845079,63.5068512870162,
63.9417245895516,64.376597892117,64.8114711947155,65.2463444973499,65.6812178000231,
66.1169437982275,66.5526697964318,66.9875430991915,67.4224164019987,67.8572897048563,
68.2921630077673,68.7270363107343,69.1619096137603,69.5967829168479,70.0316562200001,
70.4665295232194,70.9014028265087,71.3362761298705,71.7711494333077,72.2060227368227,
72.6408960404182,73.0766220391044,73.5123480377905,73.9472213415547,74.382094645407,
74.8169679493499,75.2518412533859,75.6867145575172,76.1215878617464,76.5564611660756,
76.9913344705072,77.4262077750435,77.8610810796866,78.2959543844386,78.7308276893018,
79.1657009942781,79.6005742993696,80.0363002988208,80.4720262982719,80.9068996035997,
81.3417729090484,81.7766462146199,82.211519520316,82.6463928261383,83.0812661320886,
83.5161394381684,83.9510127443794,84.3858860507229,84.8207593572004,85.2556326638134,
85.6905059705631,86.1253792774507,86.5602525844776,86.995978584908,87.4317045853384,
87.8665778926469,88.3014512000977,88.7363245076919,89.1711978154302,89.6060711233134,
90.0409444313423,90.4758177395175,90.9106910478396,91.345564356309,91.7804376649263,
92.2153109736917,92.6501842826055,93.085057591668,93.5199309008791,93.9556569024059,
94.3913829039327,94.8262562134414,95.2611295230986,95.6960028329042,96.1308761428578,
96.5657494529591,97.0006227632077,97.4354960736028,97.870369384144,98.3052426948304,
98.7401160056612,99.1749893166354,99.6098626277522,100.04473593901,100.915335253024,
101.351061255639,101.785934567313,102.220807879124,102.655681191068,103.090554503145,
103.525427815353,104.395174440154,105.264921065453,105.699794378283,106.134667691232,
106.569541004295,107.004414317471,107.8750136343,108.745612951339,109.615359578629,
110.485106206296,111.354852834309,112.224599462639,113.094346091254,113.964092720119,
114.834692038763,115.705291357499,116.575037986826,117.444784616267,118.314531245777,
119.184277875311,120.054024504821,120.923771134261,121.794370453112,122.66496977189,
123.534716400968,124.404463029834,125.274209658448,126.143956286779,127.013702914792,
127.883449542458,128.754048859798,129.624648176939,130.494394803617,131.364141429857,
132.233888055637,133.103634680937,133.973381305737,134.843127930023,135.71372724472,
136.584326559147,137.019199870684,137.454073182083,137.888946493341,138.323819804458,
139.193566426263,140.063313047491,140.498186357887,140.933059668136,141.367932978237,
141.802806288191,142.237679597997,142.673405599673,143.109131601348,143.544004910857,
143.978878220217,144.413751529429,144.848624838491,145.283498147405,145.718371456171,
146.153244764789,146.588118073258,147.022991381581,147.457864689756,147.892737997785,
148.327611305669,148.762484613407,149.197357921002,149.633083921574,150.068809922147,
150.503683229455,150.938556536623,151.37342984365,151.808303150538,152.243176457288,
152.678049763901,153.112923070379,153.547796376722,153.982669682934,154.417542989014,
154.852416294964,155.287289600787,155.722162906483,156.157036212055,156.592762211626,
157.028488211198,157.463361516526,157.898234821735,158.333108126826,158.767981431803,
159.202854736666,159.637728041419,160.072601346062,160.507474650599,160.94234795503,
161.37722125936,161.812094563589,162.246967867721,162.681841171757,163.1167144757,
163.552440474473,163.988166473247,164.423039777011,164.85791308069,165.292786384286,
165.727659687801,166.162532991238,166.597406294601,167.03227959789,167.46715290111,
167.902026204262,168.33689950735,168.771772810376,169.206646113343,169.641519416254,
170.076392719112,170.512118717363,170.947844715614,171.382718018374,171.817591321089,
172.252464623762,172.687337926397,173.122211228996,173.557084531561,173.991957834097,
174.426831136606,174.86170443909,175.296577741554,175.731451044,176.16632434643,
176.601197648848,177.036070951258,177.471796949306,177.907522947355,178.342396249755,
178.777269552155,179.212142854558,179.647016156968,180.081889459386,180.516762761816,
180.951636064262,181.386509366726,181.82138266921,182.256255971719,182.691129274255,
183.12600257682,183.560875879419,183.995749182054,184.431475180237,184.867201178421,
185.302074481136,185.736947783896,186.171821086704,186.606694389561,187.041567692473,
187.47644099544,187.911314298466,188.346187601554,188.781060904706,189.215934207926,
189.650807511215,190.085680814577,190.520554118015,190.95542742153,191.391153420175,
191.82687941882,192.261752722499,192.696626026263,193.131499330116,193.566372634059,
194.001245938095,194.436119242227,194.870992546456,195.305865850785,195.740739155217,
196.175612459754,196.610485764397,197.045359069149,197.480232374013,197.915105678989,
198.350831678382,198.786557677775,199.221430982984,199.656304288312,200.091177593761,
200.526050899333,200.960924205029,201.395797510852,201.830670816802,202.265544122882,
202.700417429093,203.135290735437,203.570164041915,204.005037348528,204.439910655278,
204.874783962166,205.310509962526,205.746235962887,206.181109270054,206.615982577363,
207.050855884814,207.485729192409,207.920602500147,208.355475808031,208.79034911606,
209.225222424235,209.660095732558,210.094969041027,210.529842349645,210.96471565841,
211.399588967324,211.834462276387,212.27018827784,212.705914279292,213.140787588653,
213.575660898161,214.010534207819,214.880280827579,215.31515413768,215.750027447929,
216.184900758324,216.619774068866,217.054647379553,217.489520690384,218.359267312475,
219.22986662628,219.665592628826,220.100465940363,220.535339252038,220.970212563848,
221.83995918787,222.709705812416,223.579452437468,224.014325750179,224.44919906301,
225.318945689022,226.189545005688,227.060144322571,227.929890949664,228.799637577146,
229.66938420499,230.539130833166,231.408877461643,232.278624090388,233.149223408954,
234.019822727623,234.889569356878,235.759315986267,236.629062615749,237.498809245277,
238.368555874806,239.238302504287,240.108901823183,240.979501142017,241.849247771189,
242.718994400167,243.588741028911,244.458487657389,245.328234285565,246.197980913409,
247.068580230891,247.939179548182,248.80892617507,249.678672801532,250.548419427545,
251.418166053087,252.287912678139,253.157659302684,254.028258617581,254.898857932211,
255.333731243885,255.768604555423,256.203477866821,256.63835117808,257.508097800171,
258.377844421689,258.812717732231,259.247591042627,259.682464352876,260.117337662977,
260.552210972931,260.987936974682,261.858536286089,262.293409595598,262.728282904958,
263.16315621417,263.598029523233,264.032902832147,264.467776140913,264.902649449531,
265.337522758001,265.772396066323,266.207269374499,266.642142682528,267.077015990412,
267.511889298151,267.947615298795,268.383341299439,268.81821460689,269.2530879142,
269.687961221367,270.122834528394,270.557707835282,270.992581142032,271.427454448646,
271.862327755124,272.297201061468,272.732074367679,273.166947673759,273.60182097971,
274.036694285533,274.471567591229,274.907293590862,275.343019590495,275.777892895944,
276.212766201272,276.647639506481,277.082512811573,277.51738611655,277.952259421414,
278.387132726166,278.82200603081,279.256879335346,279.691752639779,280.126625944108,
280.561499248338,280.996372552469,281.431245856506,281.866971855324,282.302697854143,
282.737571157996,283.172444461761,283.60731776544,284.042191069036,284.477064372551,
284.911937675989,285.346810979351,285.781684282641,286.216557585861,286.651430889013,
287.086304192101,287.521177495128,287.956050798095,288.390924101007,288.826650099283,
289.262376097559,289.697249400366,290.132122703127,290.566996005842,291.001869308516,
291.43674261115,291.871615913749,292.306489216315,292.741362518851,293.17623582136,
293.611109123845,294.045982426308,294.480855728754,294.915729031185,295.350602333603,
295.786328331655,296.222054329707,296.65692763211,297.091800934511,297.526674236911,
297.961547539314,298.396420841724,298.831294144142,299.266167446573,299.701040749018,
300.135914051482,300.570787353967,301.005660656476,301.440533959012,301.875407261578,
302.310280564177,302.746006562341,303.181732560506,303.616605863179,304.051479165895,
304.486352468655,304.921225771462,305.35609907432,305.790972377232,306.225845680199,
306.660718983226,307.095592286314,307.530465589466,307.965338892686,308.400212195976,
308.835085499338,309.269958802776,309.705684801381,310.141410799985,310.576284103581,
311.01115740726,311.446030711025,311.880904014878,312.315777318821,312.750650622858,
313.185523926989,313.620397231219,314.055270535549,314.490143839981,314.925017144517,
315.359890449161,315.794763753913,316.229637058777,316.665363058112,317.101089057448,
317.53596236254,317.970835667749,318.405708973077,318.840582278526,319.275455584098,
319.710328889795,320.145202195618,320.580075501568,321.014948807648,321.44982211386,
321.884695420204,322.319568726682,322.754442033295,323.189315340045,323.625041340336,
324.060767340628,324.495640647655,324.930513954822,325.365387262131,325.800260569583,
326.235133877177,326.670007184916,327.1048804928,327.539753800829,327.974627109005,
328.409500417327,328.844373725797,329.279247034415,329.714120343181,330.148993652095,
330.584719653474,331.020445654852,331.455318964064,331.890192273424,332.325065582933,
332.759938892591,333.194812202397,333.629685512351,334.064558822453,334.499432132702,
334.934305443098,335.369178753639,335.804052064326,336.673798686132,337.108671997249,
337.544397999725,337.980124002201,338.4149973136,338.849870625137,339.284743936812,
340.154490560568,341.024237184854,341.459110497191,341.893983809655,342.328857122244,
342.763730434955,343.633477060735,344.504076377234,345.374675693955,346.244422320844,
347.114168948136,347.983915575803,348.853662203817,349.723408832148,350.593155460764,
351.463754779246,352.334354097839,353.204100727012,354.07384735634,354.943593985781,
355.813340615292,356.683087244827,357.552833874338,358.423433193272,359.294032512154,
360.163779141409,361.033525770489,361.903272399355,362.77301902797,363.642765656301,
364.512512284316,365.383111601936,366.253710919371,367.123457546465,367.993204173143,
368.862950799383,369.732697425164,370.602444050463,371.472190675265,372.342789990359,
373.21338930519,373.648262617,374.083135928675,374.952882551611,375.822629173987,
376.257502484962,376.692375795793,377.12724910648,377.562122417021,377.996995727417,
378.431869037666,378.866742347767,379.302468349591,379.738194351416,380.173067661222,
380.607940970879,381.042814280388,381.477687589749,381.91256089896,382.347434208023,
382.782307516937,383.217180825703,383.652054134321,384.086927442791,384.521800751113,
384.956674059289,385.391547367318,385.826420675202,386.262146675918,386.697872676635,
387.13274598423,387.567619291681,388.00249259899,388.437365906157,388.872239213185,
389.307112520073,389.741985826823,390.176859133436,390.611732439914,391.046605746258,
391.48147905247,391.91635235855,392.351225664501,392.786098970323,393.221824970019,
393.657550969714,394.092424275286,394.527297580735,394.962170886063,395.397044191272,
395.831917496364,396.266790801341,396.701664106204,397.136537410957,397.5714107156,
398.006284020137,398.441157324569,398.876030628899,399.310903933128,399.74577723726,
400.181503236126,400.617229234991,401.052102538934,401.486975842787,401.921849146551,
402.356722450231,402.791595753827,403.226469057342,403.66134236078,404.096215664142,
404.531088967432,404.965962270651,405.400835573804,405.835708876892,406.270582179918,
406.705455482886,407.141181481189,407.576907479491,408.01178078235,408.446654085157,
408.881527387917,409.316400690633,409.751273993306,410.186147295941,410.62102059854,
411.055893901106,411.490767203642,411.925640506151,412.360513808636,412.795387111099,
413.230260413545,413.665133715976,414.100859714032,414.536585712088,414.971459014498,
415.406332316901,415.841205619301,416.276078921702,416.710952224105,417.145825526515,
417.580698828933,418.015572131364,418.45044543381,418.885318736273,419.320192038758,
419.755065341267,420.189938643803,420.624811946369,421.060537944515,421.496263942662,
421.931137245297,422.36601054797,422.800883850686,423.235757153446,423.670630456253,
424.105503759112,424.540377062023,424.975250364991,425.410123668017,425.844996971105,
426.279870274258,426.714743577477,427.149616880767,427.584490184129,428.020216182695,
428.455942181261,428.890815484776,429.325688788373,429.760562092052,430.195435395816,
430.630308699669,431.065182003612,431.500055307649,431.93492861178,432.36980191601,
432.80467522034,433.239548524772,433.674421829309,434.109295133952,434.544168438705,
434.979894437984,435.415620437262,435.850493742239,436.285367047331,436.72024035254,
437.155113657869,437.589986963318,438.024860268889,438.459733574586,438.894606880409,
439.32948018636,439.76435349244,440.199226798651,440.634100104995,441.068973411473,
441.503846718087,441.939572718309,442.375298718531,442.810172025419,443.245045332447,
443.679918639614,444.114791946923,444.549665254374,444.984538561969,445.419411869708,
445.854285177591,446.289158485621,446.724031793796,447.158905102119,447.593778410589,
448.028651719207,448.463525027973,448.899251029277,449.334977030581,449.769850339644,
450.639596958216,451.074470267725,451.509343577383,451.944216887189,452.379090197143,
452.813963507244,453.248836817493,453.683710127889,454.118583438431,454.553456749117,
454.988330059949,455.423203370923,455.858929373329,456.294655375734,456.729528686993,
457.164401998391,457.599275309929,458.469021933414,458.90389524536,459.338768557437,
459.773641869646,460.208515181983,460.643388494447,461.078261807036,461.948008432578,
462.818607748906,463.689207065461,464.55895369214,465.428700319234,466.298446946716,
467.16819357456,468.037940202737,468.907686831215,469.778286149605,470.648885468116,
471.518632097196,472.388378726451,473.258125355841,474.127871985322,474.997618614851,
475.86736524438,476.737964563343,477.608563882265,478.478310511593,479.348057140765,
480.217803769743,481.087550398488,481.957297026966,482.827043655142,483.697642972895,
484.568242290469,485.43798891776,486.307735544649,487.177482171112,488.047228797125,
488.916975422667,489.78672204772,490.657321363009,491.09304736596,491.527920678038,
492.397667301793,493.267413925005,494.137160547663,494.57203385878,495.006907169755,
495.441780480586,495.876653791273,496.311527101814,496.74640041221,497.616999724357,
498.052725726255,498.487599036209,498.922472346015,499.357345655673,499.792218965182,
500.227092274542,500.661965583754,501.096838892816,501.531712201731,501.966585510497,
502.401458819114,502.836332127584,503.271205435907,503.706078744082,504.140952052112,
504.576678052901,505.01240405369,505.447277361429,505.882150669023,506.317023976474,
506.751897283783,507.186770590951,507.621643897978,508.056517204866,508.491390511616,
508.92626381823,509.361137124708,509.796010431052,510.230883737263,510.665757043344,
511.100630349294,511.536356349053,511.972082348811,512.406955654506,512.841828960076,
513.276702265523,513.711575570849,514.146448876056,514.581322181146,515.016195486121,
515.451068790983,515.885942095733,516.320815400375,516.75568870491,517.19056200934,
517.625435313668,518.060308617896,518.496034616807,518.931760615718,519.366633919752,
519.801507223694,520.236380527545,520.671253831307,521.106127134985,521.541000438579,
521.975873742092,522.410747045528,522.845620348888,523.280493652176,523.715366955394,
524.150240258545,524.585113561631,525.019986864656,525.455712862985,525.891438861313,
526.326312164223,526.761185467079,527.196058769885,527.630932072643,528.065805375356,
528.500678678029,528.935551980661,529.370425283258,529.805298585822,530.240171888356,
530.675045190863,531.109918493346,531.544791795808,531.979665098252,532.415391096312,
532.851117094373,533.285990396789,533.720863699197,534.155737001598,534.590610303997,
535.025483606395,535.460356908796,535.895230211204,536.330103513621,536.764976816049,
537.199850118493,537.634723420955,538.069596723438,538.504470025945,538.93934332848,
539.375069326608,539.810795324736,540.245668627333,540.680541929966,541.115415232637,
541.550288535351,541.985161838109,542.420035140915,542.854908443771,543.28978174668,
543.724655049646,544.15952835267,544.594401655757,545.029274958907,545.464148262125,
545.899021565413,546.334747563939,546.770473562465,547.205346865901,547.640220169415,
548.075093473009,548.509966776686,548.944840080449,549.3797133843,549.814586688241,
550.249459992276,550.684333296405,551.119206600633,551.554079904961,551.988953209391,
552.423826513926,552.858699818567,553.294425817789,553.73015181701,554.165025121872,
554.599898426846,555.034771731937,555.469645037144,555.90451834247,556.339391647917,
556.774264953487,557.209138259182,557.644011565003,558.078884870951,558.51375817703,
558.948631483239,559.383504789581,559.818378096058,560.254104096209,560.689830096361,
561.12470340311,561.559576709996,561.994450017021,562.429323324187,562.864196631494,
563.299069938943,563.733943246536,564.168816554273,564.603689862154,565.038563170182,
565.473436478355,565.908309786676,566.343183095144,566.77805640376,567.213782404988,
567.649508406216,568.084381715128,568.519255024189,568.954128333399,569.389001642757,
569.823874952264,570.258748261921,570.693621571725,571.128494881677,571.563368191777,
572.433114812417,572.867988122957,573.302861433642,573.737734744471,574.173460746804,
574.609186749136,575.044060060251,575.913806682904,576.783553306113,577.218426617922,
577.653299929865,578.08817324194,578.523046554147,579.392793178944,580.26253980424,
581.13313912039,581.568865123709,582.003738436771,582.87348506323,583.743231690115,
584.612978317402,585.482724945065,586.352471573076,587.222218201403,588.092817519691,
588.963416838109,589.833163467083,590.702910096251,591.572656725575,592.442403355013,
593.31214998452,594.181896614051,595.05249593303,595.92309525198,596.792841881366,
597.662588510618,598.532335139693,599.402081768556,600.271828397167,601.141575025495,
602.012174343369,602.882773661074,603.752520288553,604.622266915642,605.492013542317,
606.361760168553,607.23150679433,608.101253419626,608.971852735101,609.842452050322,
610.71219867434,611.581945297822,612.451691920754,612.886565232011,613.321438543126,
613.756311854099,614.191185164928,615.060931786153,615.931531098516,616.367257100486,
616.802130410586,617.237003720538,617.671877030342,618.106750339998,618.541623649505,
618.976496958863,619.411370268073,619.846243577134,620.281116886046,620.71599019481,
621.150863503426,621.585736811894,622.020610120214,622.455483428388,622.891209429248,
623.326935430108,623.761808737989,624.196682045726,624.631555353319,625.066428660769,
625.501301968075,625.936175275241,626.371048582266,626.805921889153,627.240795195901,
627.675668502512,628.110541808988,628.54541511533,628.98028842154,629.415161727618,
629.850887727438,630.286613727259,630.72148703308,631.156360338774,631.591233644344,
632.026106949791,632.460980255118,632.895853560325,633.330726865415,633.76560017039,
634.200473475251,634.635346780002,635.070220084644,635.505093389179,635.939966693609,
636.374839997937,636.810565996897,637.246291995857,637.681165299986,638.116038604021,
638.550911907962,638.985785211813,639.420658515576,639.855531819253,640.290405122847,
640.725278426361,641.160151729796,641.595025033157,642.029898336444,642.464771639662,
642.899644942813,643.334518245899,643.770244244257,644.205970242616,644.640843545581,
645.075716848491,645.510590151347,645.945463454153,646.380336756911,646.815210059625,
647.250083362296,647.684956664929,648.119829967526,648.55470327009,648.989576572624,
649.424449875131,649.859323177614,650.294196480076,650.729922478144,651.165648476212,
651.600521778641,652.035395081057,652.470268383465,652.905141685866,653.340014988265,
653.774888290663,654.209761593065,654.644634895472,655.079508197889,655.514381500318,
655.949254802762,656.384128105224,656.819001407706,657.253874710213,657.689600708326,
658.12532670644,658.560200009004,658.995073311601,659.429946614234,659.864819916905,
660.299693219619,660.734566522377,661.169439825183,661.604313128039,662.039186430948,
662.474059733914,662.908933036938,663.343806340025,663.778679643175,664.213552946393,
664.649278944883,665.085004943373,665.519878246733,665.954751550169,666.389624853683,
666.824498157277,667.259371460954,667.694244764717,668.129118068568,668.563991372509,
668.998864676544,669.433737980674,669.868611284901,670.303484589229,670.738357893659,
671.173231198194,671.608957197361,672.044683196528,672.479556501278,672.91442980614,
673.349303111115,673.784176416205,674.219049721412,674.653923026738,675.088796332185,
675.523669637755,675.95854294345,676.393416249271,676.82828955522,677.263162861298,
677.698036167508,678.13290947385,678.568635473934,679.004361474018,679.439234780629,
679.874108087377,680.308981394264,680.743854701289,681.178728008455,681.613601315762,
682.048474623211,682.483347930804,682.91822123854,683.353094546422,683.78796785445,
684.222841162623,684.657714470944,685.092587779412,685.528313780566,685.96403978172,
686.398913090483,686.833786399396,687.268659708457,687.703533017666,688.138406327025,
688.573279636532,689.008152946187,689.443026255992,689.877899565944,690.312772876043,
690.74764618629,691.182519496684,691.617392807224,692.052266117909,692.487992120169,
692.92371812243,693.358591433403,694.228338055774,694.663211367171,695.098084678707,
695.532957990379,695.967831302188,696.402704614131,696.837577926207,697.707324550749,
698.577071175797,699.011944488507,699.447670491767,699.883396495028,700.318269807975,
701.188016434211,702.057763060886,702.927509687976,703.797256315454,704.667002943295,
705.536749571467,706.407348889651,707.277948207973,708.147694836835,709.017441465911,
709.887188095163,710.756934724548,711.626681354026,712.496427983551,713.367027302543,
714.237626621516,715.107373250954,715.977119880277,716.846866509446,717.716613138419,
718.586359767161,719.456106395635,720.32670571363,721.197305031464,722.067051659126,
722.936798286414,723.806544913299,724.676291539758,725.546038165767,726.415784791305,
727.286384106969,728.156983422381,729.026730046663,729.896476670415,730.331349982088,
730.766223293624,731.201096605021,731.635969916278,732.505716538366,733.37546315988,
733.81033647042,734.246062472462,734.681788474505,735.116661784752,735.551535094852,
735.986408404804,736.421281714608,736.856155024264,737.291028333771,737.72590164313,
738.160774952339,738.5956482614,739.030521570312,739.465394879076,739.900268187692,
740.33514149616,740.77001480448,741.205740805414,741.641466806347,742.076340114374,
742.511213422256,742.946086729993,743.380960037585,743.815833345035,744.250706652341,
744.685579959507,745.120453266533,745.555326573419,745.990199880167,746.425073186778,
746.859946493254,747.294819799596,747.729693105806,748.165419105691,748.601145105576,
749.036018411525,749.470891717346,749.90576502304,750.34063832861,750.775511634057,
751.210384939384,751.645258244591,752.080131549682,752.515004854656,752.949878159518,
753.384751464269,753.81962476891,754.254498073445,754.689371377875,755.125097376885,
755.560823375895,755.995696680123,756.430569984253,756.865443288287,757.300316592228,
757.735189896079,758.170063199842,758.604936503519,759.039809807113,759.474683110627,
759.909556414062,760.344429717423,760.779303020711,761.214176323929,761.649049627079,
762.084775625469,762.520501623858,762.955374926883,763.390248229848,763.825121532758,
764.259994835614,764.694868138419,765.129741441178,765.564614743891,765.999488046563,
766.434361349196,766.869234651793,767.304107954357,767.738981256891,768.173854559398,
768.608727861881,769.044453859958,769.480179858035,769.915053160479,770.349926462907,
770.784799765324,771.219673067731,771.654546370133,772.089419672531,772.52429297493,
772.959166277331,773.394039579739,773.828912882155,774.263786184584,774.698659487028,
775.13353278949,775.568406091973,776.004132090072,776.439858088172,776.874731390706,
777.30960469327,777.744477995867,778.1793512985,778.614224601171,779.049097903885,
779.483971206643,779.918844509449,780.353717812305,780.788591115215,781.22346441818,
781.658337721205,782.093211024291,782.528084327442,782.963810325897,783.399536324352,
783.834409627639,784.269282931,784.704156234435,785.139029537949,785.573902841543,
786.00877614522,786.443649448983,786.878522752834,787.313396056775,787.74826936081,
788.183142664939,788.618015969167,789.052889273495,789.487762577925,789.923488577038,
790.359214576152,790.794087880793,791.228961185544,791.663834490406,792.098707795381,
792.533581100471,792.968454405678,793.403327711004,793.838201016451,794.273074322021,
794.707947627716,795.142820933537,795.577694239486,796.012567545564,796.447440851774,
796.883166851791,797.318892851808,797.753766158284,798.188639464895,798.623512771643,
799.058386078529,799.493259385555,799.92813269272,800.363006000027,800.797879307477,
801.232752615069,801.667625922806,802.102499230688,802.537372538715,802.972245846889,
803.40711915521,803.84284515629,804.27857115737,804.713444465985,805.148317774749,
805.583191083662,806.018064392723,806.452937701933,806.887811011291,807.322684320798,
808.192430940258,808.62730425021,809.06217756031,809.497050870557,809.931924180951,
810.36679749149,810.802523493679,811.238249495867,811.673122806697,812.542869428785,
812.977742740041,813.412616051438,813.847489362974,814.282362674646,814.717235986455,
815.152109298398,816.021855922681,816.891602547478,817.326475860065,817.762201863265,
818.197927866466,818.632801179295,819.502547805304,820.372294431763,821.242041058648,
822.111787685935,822.981534313598,823.851280941609,824.721880259681,825.5924795779,
826.462226206642,827.331972835616,828.201719464785,829.071466094109,829.941212723546,
830.810959353053,831.681558672047,832.552157991036,833.421904620514,834.2916512499,
835.161397879151,836.031144508226,836.900891137089,837.770637765701,838.641237083811,
839.511836401767,840.381583029608,841.251329657086,842.121076284176,842.990822910851,
843.860569537087,844.730316162863,845.600915478712,846.471514794314,847.341261418855,
848.211008042874,848.645881354683,849.080754666356,849.515627977891,849.950501289288,
850.82024791166,851.689994533462,852.124867844147,852.560593846263,852.996319848379,
853.431193158772,853.866066469019,854.300939779119,855.170686398875,855.605559708531,
856.040433018038,856.475306327397,856.910179636606,857.345052945667,857.77992625458,
858.214799563344,858.64967287196,859.084546180427,859.520272181434,859.95599818244,
860.390871490614,860.825744798641,861.260618106523,861.69549141426,862.130364721852,
862.565238029302,863.000111336609,863.434984643774,863.8698579508,864.304731257686,
864.739604564434,865.174477871045,865.609351177521,866.044224483863,866.479950483814,
866.915676483765,867.350549789843,867.785423095792,868.220296401613,868.655169707307,
869.090043012877,869.524916318325,869.959789623651,870.394662928858,870.829536233948,
871.264409538923,871.699282843785,872.134156148535,872.569029453177,873.003902757712,
873.439628756773,873.875354755834,874.310228060162,874.745101364389,875.179974668519,
875.614847972553,876.049721276495,876.484594580346,876.919467884108,877.354341187786,
877.78921449138,878.224087794893,878.658961098329,879.093834401689,879.528707704977,
879.963581008195,880.399307006616,880.835033005038,881.269906308124,881.704779611148,
882.139652914114,882.574526217024,883.00939951988,883.444272822685,883.879146125444,
884.314019428157,884.748892730829,885.183766033462,885.618639336059,886.053512638623,
886.488385941157,886.923259243664,887.358985241751,887.794711239839,888.2295845423,
888.664457844744,889.099331147173,889.534204449589,889.969077751997,890.403951054398,
890.838824356797,891.273697659195,891.708570961597,892.143444264004,892.578317566421,
893.01319086885,893.448064171293,893.882937473755,894.318663471843,894.75438946993,
895.189262772437,895.624136074971,896.059009377535,896.493882680132,896.928755982765,
897.363629285437,897.798502588151,898.233375890909,898.668249193715,899.103122496571,
899.53799579948,899.972869102446,900.40774240547,900.842615708556,901.278341706978,
901.714067705399,902.148941008617,902.583814311905,903.018687615265,903.453560918701,
903.888434222214,904.323307525808,904.758180829485,905.193054133248,905.627927437099,
906.06280074104,906.497674045075,906.932547349205,907.367420653433,907.80229395776,
908.238019956821,908.673745955883,909.108619260417,909.543492565059,909.978365869809,
910.413239174671,910.848112479646,911.282985784736,911.717859089943,912.152732395269,
912.587605700716,913.022479006287,913.457352311981,913.892225617802,914.327098923751,
914.761972229829,915.19769822978,915.633424229731,916.068297536072,916.503170842548,
916.93804414916,917.372917455908,917.807790762794,918.24266406982,918.677537376985,
919.112410684292,919.547283991742,919.982157299334,920.417030607071,920.851903914953,
921.28677722298,921.721650531154,922.15737653216,922.593102533167,923.027975841635,
923.46284915025,923.897722459014,924.332595767926,924.767469076987,925.202342386197,
925.637215695556,926.072089005063,926.506962314719,926.941835624523,927.376708934475,
927.811582244575,928.246455554822,928.681328865215,929.117054867331,929.987654180132,
930.422527490961,930.857400801934,931.292274113049,931.727147424306,932.162020735703,
932.596894047238,933.46664067072,934.336387294739,934.771260606945,935.20613391928,
935.641007231742,936.076733234882,936.94733255073,937.817079176507,938.686825802743,
939.556572429418,940.426319056508,941.296065683986,942.165812311827,943.036411629783,
943.907010947893,944.776757576505,945.646504205367,946.516250834443,947.385997463694,
948.25574409308,949.125490722558,949.996090041546,950.86668936054,951.736435990048,
952.606182619485,953.475929248809,954.345675877978,955.215422506951,956.085169135693,
956.955768453912,957.826367771985,958.696114399995,959.565861027658,960.435607654946,
961.305354281831,962.175100908289,963.044847534298,963.915446850328,964.786046166116,
965.655792790913,966.525539415195,966.960412727138,967.395286038947,968.265032662155,
969.134779284809,969.569652595924,970.004525906897,970.439399217726,970.875125219914,
971.310851222103,971.745724532643,972.615471153283,973.485217773335,973.920091083139,
974.354964392795,974.789837702302,975.22471101166,975.65958432087,976.094457629931,
976.529330938844,976.964204247608,977.399077556223,977.834803557303,978.270529558383,
978.705402866704,979.140276174877,979.575149482905,980.010022790786,980.444896098523,
980.879769406116,981.314642713565,981.749516020872,982.184389328038,982.619262635063,
983.05413594195,983.489009248698,983.923882555309,984.358755861785,984.794481861802,
985.230207861819,985.665081168029,986.099954474107,986.534827780056,986.969701085877,
987.404574391571,987.839447697141,988.274321002589,988.709194307915,989.144067613122,
989.578940918212,990.013814223187,990.448687528048,990.883560832799,991.31843413744,
991.754160136554,992.189886135667,992.624759440097,993.059632744425,993.494506048653,
993.929379352783,994.364252656817,994.799125960758,995.233999264609,995.668872568372,
996.103745872049,996.538619175643,996.973492479157,997.408365782593,997.843239085953,
998.278112389241,998.713838387696,999.149564386151,999.584437689301,1000.01931099239,
1000.45418429541,1000.88905759838,1001.32393090129,1001.75880420414,1002.19367750695,
1002.62855080971,1003.06342411242,1003.49829741509,1003.93317071773,1004.36804402032,
1004.80291732289,1005.23779062542,1005.67351662352,1006.10924262162,1006.5441159241,
1006.97898922656,1007.41386252901,1007.84873583144,1008.28360913385,1008.71848243626,
1009.15335573866,1009.58822904106,1010.02310234346,1010.45797564586,1010.89284894827,
1011.32772225069,1011.76259555311,1012.19746885556,1012.63319485364,1013.06892085171,
1013.5037941542,1013.9386674567,1014.37354075924,1014.8084140618,1015.2432873644,
1015.67816066703,1016.1130339697,1016.54790727242,1016.98278057517,1017.41765387798,
1017.85252718084,1018.28740048375,1018.72227378671,1019.15714708974,1019.59287308813,
1020.02859908651,1020.46347238967,1020.89834569288,1021.33321899617,1021.76809229953,
1022.20296560297,1022.63783890648,1023.07271221007,1023.50758551375,1023.94245881752,
1024.37733212137,1024.81220542531,1025.24707872935,1025.68195203348,1026.11682533771,
1026.55255133672,1026.98827733573,1027.42315064016,1027.8580239447,1028.29289724934,
1028.72777055409,1029.16264385896,1029.59751716393,1030.03239046902,1030.46726377423,
1030.90213707956,1031.33701038501,1031.77188369058,1032.20675699628,1032.6416303021,
1033.07650360805,1033.51222960793,1033.94795560782,1034.38282891403,1034.81770222038,
1035.25257552685,1035.68744883347,1036.12232214022,1036.5571954471,1036.99206875413,
1037.4269420613,1037.86181536861,1038.29668867606,1038.73156198365,1039.16643529139,
1039.60130859927,1040.0361819073,1040.47190790824,1040.90763390917,1041.34250721749,
1041.77738052596,1042.21225383458,1042.64712714334,1043.08200045226,1043.95174707053,
1044.38662037989,1044.8214936894,1045.25636699906,1045.69124030886,1046.12611361882,
1046.56098692892,1046.99586023917,1047.43158624121,1047.86731224325,1048.3021855538,
1048.73705886448,1049.17193217531,1049.60680548629,1050.0416787974,1050.47655210866,
1050.91142542006,1051.78117204327,1052.21604535508,1052.65091866703,1053.0857919791,
1053.52066529131,1053.95553860365,1054.39126460673,1055.26186392239,1056.13161054793,
1057.00135717395,1057.43623048712,1057.87110380041,1058.7408504273,1059.61059705459,
1060.48034368225,1061.35094300009,1062.22154231809,1063.09128894656,1063.96103557531,
1064.83078220429,1065.70052883346,1066.57027546278,1067.44002209222,1068.3106214112,
1069.18122073019,1070.05096735972,1070.9207139892,1071.79046061859,1072.66020724785,
1073.52995387693,1074.39970050579,1075.27029982411,1076.1408991423,1077.01064577048,
1077.88039239832,1078.7501390258,1079.61988565289,1080.48963227957,1081.35937890581,
1082.22997822202,1083.100577538,1083.97032416305,1084.84007078759,1085.70981741161,
1086.5795640351,1087.44931065803,1087.88418396929,1088.31905728041,1088.75393059138,
1089.18965659365,1089.62538259591,1090.06025590659,1090.93000252753,1091.36487583778,
1091.79974914788,1092.23462245783,1092.66949576764,1093.1043690773,1093.5392423868,
1093.97411569616,1094.40898900538,1094.84386231444,1095.27873562335,1095.71360893212,
1096.14933493327,1096.58506093443,1097.0199342429,1097.45480755122,1097.88968085939,
1098.32455416742,1098.75942747531,1099.19430078305,1099.62917409064,1100.06404739809,
1100.4989207054,1100.93379401257,1101.36866731959,1101.80354062648,1102.23841393323,
1102.67328723984,1103.10901323993,1103.54473924001,1103.97961254636,1104.41448585257,
1104.84935915865,1105.2842324646,1105.71910577042,1106.15397907612,1106.58885238169,
1107.02372568714,1107.45859899246,1107.89347229767,1108.32834560276,1108.76321890774,
1109.1980922126,1109.63296551736,1110.06869151652,1110.50441751569,1110.93929082023,
1111.37416412466,1111.80903742899,1112.24391073322,1112.67878403735,1113.11365734139,
1113.54853064533,1113.98340394918,1114.41827725295,1114.85315055662,1115.28802386022,
1115.72289716374,1116.15777046717,1116.59264377053,1117.02836976903,1117.46409576752,
1117.89896907074,1118.33384237389,1118.76871567698,1119.20358898,1119.63846228297,
1120.07333558588,1120.50820888874,1120.94308219154,1121.3779554943,1121.81282879702,
1122.24770209969,1122.68257540233,1123.11744870492,1123.55232200749,1123.98804800561,
1124.42377400372,1124.85864730623,1125.29352060871,1125.72839391118,1126.16326721362,
1126.59814051605,1127.03301381847,1127.46788712088,1127.90276042328,1128.33763372568,
1128.77250702808,1129.20738033048,1129.64225363289,1130.07712693531,1130.51200023774,
1130.94772623581,1131.38345223388,1131.81832553634,1132.25319883883,1132.68807214134,
1133.12294544387,1133.55781874644,1133.99269204904,1134.42756535167,1134.86243865434,
1135.29731195706,1135.73218525982,1136.16705856263,1136.60193186548,1137.03680516839,
1137.47167847136,1137.90740446972,1138.34313046808,1138.77800377117,1139.21287707432,
1139.64775037754,1140.08262368083,1140.51749698419,1140.95237028763,1141.38724359114,
1141.82211689474,1142.25699019842,1142.69186350218,1143.12673680603,1143.56161010998,
1143.99648341401,1144.43135671814,1144.86708271711,1145.30280871607,1145.7376820204,
1146.17255532483,1146.60742862936,1147.04230193401,1147.47717523876,1147.91204854362,
1148.3469218486,1148.78179515369,1149.2166684589,1149.65154176423,1150.08641506968,
1150.52128837525,1150.95616168094,1151.39103498677,1151.82676098659,1152.26248698641,
1152.69736029249,1153.1322335987,1153.56710690504,1154.00198021152,1154.43685351813,
1154.87172682488,1155.30660013177,1155.7414734388,1156.17634674597,1156.61122005327,
1157.04609336073,1157.48096666832,1157.91583997606,1158.35071328394,1158.7864392848,
1159.22216528566,1159.65703859384,1160.09191190216,1160.52678521063,1160.96165851925,
1161.39653182801,1161.83140513693,1162.26627844599,1162.7011517552,1163.13602506456,
1163.57089837407,1164.00577168373,1164.44064499353,1164.87551830349,1165.74611761556,
1166.18184361753,1166.61671692792,1167.05159023846,1167.48646354915,1167.92133685998,
1168.35621017096,1169.22595679333,1170.09570341627,1170.53057672794,1170.96545003975,
1171.4003233517,1171.83519666377,1172.27006997598,1172.705795979,1173.57639529447,
1174.44614191977,1174.8810152326,1175.31588854555,1176.18563517179,1177.05538179847,
1177.92512842556,1178.79487505304,1179.66547437075,1180.53607368863,1181.40582031696,
1182.27556694557,1183.14531357444,1184.01506020352,1184.88480683277,1185.75455346216,
1186.62515278112,1187.4957521001,1188.36549872963,1189.23524535914,1190.10499198858,
1190.97473861791,1191.84448524708,1192.71423187606,1193.58483119448,1194.45543051277,
1195.3251771411,1196.19492376911,1197.06467039678,1197.93441702407,1198.80416365096,
1199.67391027742,1200.5445095938,1201.41510890996,1202.28485553525,1203.15460216005,
1204.02434878434,1204.89409540809,1205.76384203131,1206.1987153427,1206.63358865396,
1207.06846196508,1207.50418796741,1208.37478728058,1209.2445339018,1209.6794072122,
1210.11428052245,1210.54915383255,1210.9840271425,1211.41890045231,1211.85377376197,
1212.28864707147,1212.72352038083,1213.15839369005,1213.59326699911,1214.02814030802,
1214.46386630925,1214.89959231048,1215.3344656191,1215.76933892757,1216.20421223589,
1216.63908554406,1217.07395885209,1217.50883215998,1217.94370546771,1218.37857877531,
1218.81345208276,1219.24832539007,1219.68319869724,1220.11807200426,1220.55294531115,
1220.9878186179,1221.42354461805,1221.85927061821,1222.29414392468,1222.72901723103,
1223.16389053724,1223.59876384332,1224.03363714927,1224.46851045509,1224.90338376079,
1225.33825706636,1225.77313037181,1226.20800367713,1226.64287698234,1227.07775028743,
1227.51262359241,1227.94749689727,1228.3832228965,1228.81894889572,1229.25382220036,
1229.6886955049,1230.12356880933,1230.55844211366,1230.99331541789,1231.42818872202,
1231.86306202606,1232.29793533,1232.73280863385,1233.16768193762,1233.60255524129,
1234.03742854489,1234.4723018484,1234.90717515184,1235.34290115037,1235.7786271489,
1236.21350045219,1236.64837375541,1237.08324705856,1237.51812036165,1237.95299366467,
1238.38786696764,1238.82274027055,1239.25761357341,1239.69248687621,1240.12736017897,
1240.56223348169,1240.99710678436,1241.431980087,1241.8668533896,1242.30257938773,
1242.73830538585,1243.17317868839,1243.6080519909,1244.04292529338,1244.47779859585,
1244.91267189829,1245.34754520072,1245.78241850314,1246.21729180555,1246.65216510795,
1247.08703841035,1247.52191171275,1247.95678501515,1248.39165831756,1248.82653161998,
1249.26225761804,1249.69798361611,1250.13285691855,1250.56773022101,1251.0026035235,
1251.43747682601,1251.87235012854,1252.30722343111,1252.74209673371,1253.17697003634,
1253.61184333901,1254.04671664173,1254.48158994449,1254.9164632473,1255.35133655015,
1255.78620985306,1256.22193585139,1256.65766184973,1257.09253515275,1257.52740845584,
1257.96228175899,1258.39715506221,1258.8320283655,1259.26690166886,1259.7017749723,
1260.13664827581,1260.57152157941,1261.00639488309,1261.44126818685,1261.8761414907,
1262.31101479465,1262.74588809868,1263.1816140976,1263.61734009651,1264.05221340074,
1264.48708670507,1264.9219600095,1265.35683331403,1265.79170661868,1266.22657992343,
1266.66145322829,1267.09632653327,1267.53119983836,1267.96607314357,1268.4009464489,
1268.83581975434,1269.27069305992,1269.70556636561,1270.14129236537,1270.57701836513,
1271.01189167108,1271.44676497716,1271.88163828337,1272.31651158971,1272.75138489619,
1273.1862582028,1273.62113150955,1274.05600481644,1274.49087812347,1274.92575143063,
1275.36062473794,1275.79549804539,1276.23037135299,1276.66524466073,1277.10097066151,
1277.5366966623,1277.97156997033,1278.40644327851,1278.84131658683,1279.2761898953,
1279.71106320392,1280.14593651268,1280.5808098216,1281.01568313066,1281.45055643987,
1281.88542974923,1282.32030305874,1282.75517636839,1283.1900496782,1283.62492298815,
1284.06064899005,1284.49637499195,1284.9312483022,1285.36612161259,1285.80099492313,
1286.23586823382,1286.67074154465,1287.54048816674,1287.975361478,1288.4102347894,
1288.84510810093,1289.27998141261,1289.71485472442,1290.14972803636,1291.02032735139,
1291.89092666668,1292.32579997914,1292.76067329173,1293.19554660444,1293.63041991727,
1294.50016654328,1295.36991316974,1296.23965979663,1297.10940642392,1297.9800057415,
1298.85060505925,1299.72035168742,1300.5900983159,1301.45984494464,1302.32959157362,
1303.19933820279,1304.06908483212,1304.93968415104,1305.81028347,1306.68003009953,
1307.54977672906,1308.41952335854,1309.28926998793,1310.15901661718,1311.02876324626,
1311.89936256477,1312.76996188316,1313.63970851164,1314.50945513981,1315.37920176765,
1316.24894839514,1317.11869502223,1317.98844164891,1318.85904096546,1319.72964028179,
1320.59938690733,1321.46913353238,1322.33888015692,1323.20862678095,1323.64350009276,
1324.07837340443,1324.51324671597,1324.94812002737,1325.81871934103,1326.68931865441,
1327.12419196524,1327.55906527593,1327.99393858647,1328.42881189686,1328.86368520711,
1329.29855851721,1329.73343182716,1330.16830513697,1330.60317844663,1331.03805175614,
1331.4729250655,1331.90779837471,1332.34267168377,1332.77839768507,1333.21412368638,
1333.64899699514,1334.08387030376,1334.51874361223,1334.95361692055,1335.38849022873,
1335.82336353676,1336.25823684464,1336.69311015238,1337.12798345997,1337.56285676742,
1337.99773007473,1338.4326033819,1338.86747668892,1339.30234999581,1339.73807599603,
1340.17380199625,1340.60867530287,1341.04354860934,1341.47842191569,1341.9132952219,
1342.34816852798,1342.78304183393,1343.21791513975,1343.65278844545,1344.08766175102,
1344.52253505647,1344.95740836179,1345.392281667,1345.82715497209,1346.26202827707,
1346.69775427635,1347.13348027563,1347.56835358038,1348.00322688502,1348.43810018956,
1348.87297349399,1349.30784679832,1349.74272010255,1350.17759340668,1350.61246671072,
1351.04734001466,1351.48221331851,1351.91708662228,1352.35195992595,1352.78683322955,
1353.22170653306,1353.65743253163,1354.09315853019,1354.52803183356,1354.96290513685,
1355.39777844007,1355.83265174322,1356.26752504631,1356.70239834933,1357.1372716523,
1357.57214495521,1358.00701825807,1358.44189156087,1358.87676486363,1359.31163816635,
1359.74651146902,1360.18138477166,1360.6171107698,1361.05283676795,1361.48771007051,
1361.92258337305,1362.35745667556,1362.79232997804,1363.2272032805,1363.66207658295,
1364.09694988538,1364.5318231878,1364.96669649021,1365.40156979261,1365.83644309501,
1366.27131639741,1366.70618969981,1367.14106300222,1367.57678900028,1368.01251499834,
1368.44738830077,1368.88226160321,1369.31713490567,1369.75200820816,1370.18688151067,
1370.6217548132,1371.05662811577,1371.49150141837,1371.926374721,1372.36124802367,
1372.79612132639,1373.23099462915,1373.66586793196,1374.10074123481,1374.53646723311,
1374.97219323142,1375.40706653438,1375.84193983741,1376.2768131405,1376.71168644365,
1377.14655974687,1377.58143305016,1378.01630635352,1378.45117965696,1378.88605296047,
1379.32092626407,1379.75579956775,1380.19067287151,1380.62554617536,1381.06041947931,
1381.49614547817,1381.93187147704,1382.36674478117,1382.8016180854,1383.23649138973,
1383.67136469416,1384.10623799869,1384.54111130334,1384.97598460809,1385.41085791295,
1385.84573121793,1386.28060452302,1386.71547782823,1387.15035113356,1387.585224439,
1388.02009774458,1388.45582374427,1388.89154974397,1389.32642304979,1389.76129635574,
1390.19616966182,1390.63104296803,1391.06591627437,1391.50078958085,1391.93566288746,
1392.37053619421,1392.8054095011,1393.24028280813,1393.6751561153,1394.1100294226,
1394.54490273005,1394.97977603765,1395.41550203836,1395.85122803908,1396.28610134696,
1396.72097465499,1397.15584796317,1397.59072127149,1398.02559457996,1398.46046788858,
1398.89534119734,1399.33021450626,1399.76508781532,1400.19996112453,1400.63483443389,
1401.50458105306,1401.93945436286,1402.37518036469,1402.81090636651,1403.24577967661,
1403.68065298686,1404.11552629725,1404.5503996078,1404.98527291848,1405.85501954029,
1406.2898928514,1406.72476616266,1407.15963947406,1407.5945127856,1408.02938609727,
1408.46425940908,1409.33485872391,1410.205458039,1410.64033135134,1411.07520466381,
1411.51007797639,1411.9449512891,1412.81469791488,1413.68444454112,1414.5541911678,
1415.42393779489,1416.29453711233,1417.16513642995,1418.03488305796,1418.90462968629,
1419.77437631491,1420.64412294377,1421.51386957285,1422.38361620211,1423.25421552099,
1424.12481483992,1424.99456146943,1425.86430809896,1426.73405472847,1427.60380135791,
1428.47354798724,1429.34329461641,1430.21389393501,1431.08449325349,1431.9542398821,
1432.82398651043,1433.69373313844,1434.56347976611,1435.4332263934,1436.30297302029,
1437.17357233701,1438.04417165351,1438.91391827929,1439.78366490459,1440.65341152939,
1441.52315815367,1441.95803146562,1442.39290477743,1442.8277780891,1443.26265140064,
1444.13325071451,1445.00385002811,1445.43872333908,1445.87359664991,1446.3084699606,
1446.74334327114,1447.17821658153,1447.61308989178,1448.48283651184,1448.91770982164,
1449.3525831313,1449.78745644081,1450.22232975017,1450.65720305938,1451.09292906076,
1451.52865506214,1451.96352837105,1452.39840167982,1452.83327498843,1453.2681482969,
1453.70302160522,1454.1378949134,1454.57276822143,1455.00764152931,1455.44251483705,
1455.87738814464,1456.31226145209,1456.7471347594,1457.18200806657,1457.6168813736,
1458.05260737389,1458.48833337418,1458.92320668093,1459.35807998754,1459.79295329402,
1460.22782660036,1460.66269990657,1461.09757321265,1461.5324465186,1461.96731982443,
1462.40219313012,1462.83706643569,1463.27193974114,1463.70681304647,1464.14168635168,
1464.57655965677,1465.0122856561,1465.44801165544,1465.8828849603,1466.31775826505,
1466.7526315697,1467.18750487423,1467.62237817866,1468.05725148299,1468.49212478722,
1468.92699809135,1469.36187139539,1469.79674469933,1470.23161800319,1470.66649130695,
1471.10136461063,1471.53623791422,1471.97196391283,1472.40768991143,1472.84256321487,
1473.27743651823,1473.71230982152,1474.14718312474,1474.58205642789,1475.01692973098,
1475.451803034,1475.88667633697,1476.32154963988,1476.75642294274,1477.19129624555,
1477.62616954831,1478.06104285102,1478.4959161537,1478.93164215186,1479.36736815002,
1479.80224145262,1480.23711475519,1480.67198805772,1481.10686136023,1481.54173466272,
1481.97660796518,1482.41148126762,1482.84635457005,1483.28122787247,1483.71610117488,
1484.15097447728,1484.58584777968,1485.02072108208,1485.45559438449,1485.89132038254,
1486.32704638059,1486.76191968301,1487.19679298544,1487.63166628788,1488.06653959035,
1488.50141289283,1488.93628619534,1489.37115949787,1489.80603280044,1490.24090610304,
1490.67577940567,1491.11065270835,1491.54552601106,1491.98039931382,1492.41527261663,
1492.8509986149,1493.28672461318,1493.72159791609,1494.15647121906,1494.59134452208,
1495.02621782517,1495.46109112832,1495.89596443154,1496.33083773483,1496.76571103819,
1497.20058434163,1497.63545764515,1498.07033094874,1498.50520425242,1498.94007755618,
1499.37495086004,1499.81067685885,1500.24640285767,1500.68127616171,1501.11614946584,
1501.55102277007,1501.9858960744,1502.42076937883,1502.85564268337,1503.29051598801,
1503.72538929276,1504.16026259762,1504.5951359026,1505.03000920769,1505.4648825129,
1505.89975581823,1506.33462912368,1506.77035512331,1507.20608112294,1507.64095442864,
1508.07582773446,1508.51070104041,1508.94557434649,1509.3804476527,1509.81532095904,
1510.25019426552,1510.68506757213,1511.11994087888,1511.55481418577,1511.9896874928,
1512.42456079996,1512.85943410727,1513.29430741472,1513.73003341537,1514.16575941601,
1514.60063272375,1515.03550603163,1515.47037933966,1515.90525264784,1516.34012595616,
1516.77499926463,1517.20987257325,1517.64474588201,1518.07961919093,1518.51449249999,
1518.9493658092,1519.38423911856,1519.81911242807,1520.25398573772,1520.68971173947,
1521.12543774122,1521.56031105118,1521.99518436128,1522.43005767153,1523.29980429246,
1523.73467760315,1524.16955091398,1524.60442422495,1525.03929753607,1525.47417084733,
1525.90904415873,1526.77879078194,1527.64939009657,1528.08511609939,1528.51998941146,
1528.95486272367,1529.38973603601,1530.25948266106,1531.1292292866,1531.99897591261,
1532.86872253907,1533.73846916596,1534.60906848325,1535.47966780073,1536.34941442858,
1537.21916105675,1538.08890768523,1538.95865431398,1539.82840094295,1540.69814757212,
1541.56874689096,1542.43934620985,1543.30909283933,1544.17883946886,1545.04858609839,
1545.91833272787,1546.78807935726,1547.65782598651,1548.52842530518,1549.39902462375,
1550.26877125249,1551.13851788097,1552.00826450914,1552.87801113699,1553.74775776447,
1554.61750439156,1555.48810370844,1556.35870302511,1557.22844965112,1558.09819627666,
1558.96794290171,1559.83768952626,1560.27256283834,1560.70743615028,1561.57718277377,
1562.44778208785,1563.31838140165,1563.75325471277,1564.18812802374,1564.62300133457,
1565.05787464526,1565.9276212662,1566.79736788655,1567.2322411965,1567.66711450631,
1568.10198781596,1568.53686112547,1568.97173443483,1569.40746043628,1569.84318643774,
1570.2780597468,1570.71293305571,1571.14780636448,1571.5826796731,1572.01755298157,
1572.45242628989,1572.88729959806,1573.32217290609,1573.75704621397,1574.19191952171,
1574.62679282931,1575.06166613676,1575.49653944407,1575.93141275123,1576.36713875159,
1576.80286475195,1577.23773805884,1577.67261136559,1578.1074846722,1578.54235797868,
1578.97723128502,1579.41210459124,1579.84697789732,1580.28185120327,1580.71672450909,
1581.15159781478,1581.58647112036,1582.0213444258,1582.45621773113,1582.89109103634,
1583.32681703573,1583.76254303513,1584.1974163401,1584.63228964497,1585.06716294972,
1585.50203625436,1585.9369095589,1586.37178286333,1586.80665616766,1587.24152947189,
1587.67640277602,1588.11127608005,1588.546149384,1588.98102268785,1589.41589599161,
1589.85076929529,1590.28649529394,1590.72222129258,1591.1570945961,1591.59196789953,
1592.0268412029,1592.46171450619,1592.8965878094,1593.33146111256,1593.76633441564,
1594.20120771867,1594.63608102164,1595.07095432455,1595.50582762741,1595.94070093021,
1596.37557423297,1596.81044753569,1597.24617353387,1597.68189953206,1598.11677283469,
1598.55164613729,1598.98651943985,1599.42139274239,1599.8562660449,1600.29113934738,
1600.72601264985,1601.16088595229,1601.59575925472,1602.03063255714,1602.46550585955,
1602.90037916195,1603.33525246435,1603.77012576675,1604.2058517648,1604.64157776285,
1605.07645106526,1605.51132436768,1605.94619767011,1606.38107097255,1606.81594427502,
1607.2508175775,1607.68569088001,1608.12056418254,1608.55543748511,1608.99031078771,
1609.42518409034,1609.86005739302,1610.29493069573,1610.72980399849,1611.16552999674,
1611.60125599499,1612.03612929785,1612.47100260076,1612.90587590373,1613.34074920675,
1613.77562250984,1614.21049581299,1614.64536911621,1615.0802424195,1615.51511572286,
1615.9499890263,1616.38486232981,1616.81973563341,1617.25460893709,1617.68948224085,
1618.12520823963,1618.5609342384,1618.99580754234,1619.43068084638,1619.86555415051,
1620.30042745474,1620.73530075907,1621.1701740635,1621.60504736804,1622.03992067268,
1622.47479397743,1622.90966728229,1623.34454058727,1623.77941389236,1624.21428719757,
1624.6491605029,1625.08488650247,1625.52061250204,1625.95548580761,1626.39035911331,
1626.82523241913,1627.26010572508,1627.69497903116,1628.12985233737,1628.56472564372,
1628.99959895019,1629.43447225681,1629.86934556356,1630.30421887044,1630.73909217747,
1631.17396548464,1631.60883879195,1632.04456479252,1632.48029079309,1632.91516410068,
1633.35003740842,1633.78491071631,1634.21978402433,1634.65465733251,1635.08953064083,
1635.5244039493,1635.95927725792,1636.39415056668,1636.8290238756,1637.26389718466,
1637.69877049387,1638.13364380323,1638.56851711274,1639.00424311442,1639.43996911609,
1639.8748424259,1640.30971573585,1640.74458904595,1641.6143356666,1642.04920897714,
1642.48408228782,1642.91895559865,1643.35382890963,1643.78870222074,1644.223575532,
1645.09332215494,1645.52819546661,1645.96392146936,1646.39964747212,1646.83452078406,
1647.26939409614,1647.70426740834,1648.57401403314,1649.44376065844,1650.31350728422,
1650.74838059729,1651.18325391046,1652.05300053714,1652.92359985428,1653.79419917162,
1654.66394579929,1655.5336924273,1656.40343905563,1657.27318568424,1658.14293231311,
1659.01267894219,1659.88327826096,1660.75387757982,1661.62362420926,1662.49337083877,
1663.3631174683,1664.23286409781,1665.10261072725,1665.97235735658,1666.84295667531,
1667.71355599396,1668.58330262282,1669.45304925143,1670.32279587976,1671.19254250778,
1672.06228913544,1672.93203576273,1673.80263507977,1674.6732343966,1675.54298102284,
1676.41272764862,1677.28247427392,1678.15222089872,1679.021967523,1679.89171414676,
1680.76231346105,1681.19803946366,1681.63291277506,1682.06778608632,1682.50265939743,
1682.93753270841,1683.37240601924,1684.24215264047,1684.67702595086,1685.11189926111,
1685.54677257121,1685.98164588116,1686.41651919097,1686.85139250063,1687.28626581014,
1687.72199181166,1688.15771781319,1688.5925911224,1689.02746443146,1689.46233774038,
1689.89721104914,1690.33208435776,1690.76695766623,1691.20183097455,1691.63670428272,
1692.07157759075,1692.50645089864,1692.94132420637,1693.37619751397,1693.81107082142,
1694.24594412873,1694.68167012916,1695.11739612959,1695.55226943662,1695.9871427435,
1696.42201605025,1696.85688935687,1697.29176266334,1697.72663596969,1698.1615092759,
1698.59638258198,1699.03125588793,1699.46612919375,1699.90100249945,1700.33587580502,
1700.77074911047,1701.20562241579,1701.64134841525,1702.0770744147,1702.51194771979,
1702.94682102476,1703.38169432963,1703.81656763438,1704.25144093902,1704.68631424356,
1705.12118754799,1705.55606085232,1705.99093415655,1706.42580746068,1706.86068076471,
1707.29555406866,1707.73042737251,1708.16530067627,1708.60102667496,1709.03675267365,
1709.47162597724,1709.90649928076,1710.34137258419,1710.77624588756,1711.21111919085,
1711.64599249406,1712.08086579722,1712.5157391003,1712.95061240333,1713.3854857063,
1713.82035900921,1714.25523231207,1714.69010561487,1715.12497891763,1715.56070491584,
1715.99643091404,1716.43130421671,1716.86617751935,1717.30105082195,1717.73592412451,
1718.17079742705,1718.60567072956,1719.04054403204,1719.4754173345,1719.91029063695,
1720.34516393938,1720.7800372418,1721.21491054421,1721.64978384661,1722.08465714901,
1722.52038314706,1722.9561091451,1723.39098244751,1723.82585574992,1724.26072905233,
1724.69560235476,1725.13047565721,1725.56534895967,1726.00022226216,1726.43509556467,
1726.8699688672,1727.30484216977,1727.73971547236,1728.174588775,1728.60946207767,
1729.04433538039,1729.48006137861,1729.91578737684,1730.35066067965,1730.78553398251,
1731.22040728542,1731.65528058838,1732.09015389141,1732.5250271945,1732.95990049765,
1733.39477380087,1733.82964710416,1734.26452040752,1734.69939371096,1735.13426701447,
1735.56914031807,1736.00401362175,1736.43973962048,1736.8754656192,1737.31033892306,
1737.745212227,1738.18008553104,1738.61495883517,1739.0498321394,1739.48470544373,
1739.91957874816,1740.35445205269,1740.78932535734,1741.22419866209,1741.65907196695,
1742.09394527193,1742.52881857702,1742.96369188223,1743.39941788174,1743.83514388125,
1744.2700171867,1744.70489049227,1745.13976379797,1745.57463710379,1746.00951040974,
1746.44438371582,1746.87925702203,1747.31413032837,1747.74900363485,1748.18387694146,
1748.61875024821,1749.0536235551,1749.48849686213,1749.92337016929,1750.3590961698,
1750.7948221703,1751.22969547775,1751.66456878534,1752.09944209308,1752.53431540096,
1752.96918870899,1753.40406201717,1753.83893532549,1754.27380863396,1754.70868194258,
1755.14355525134,1755.57842856026,1756.01330186932,1756.44817517853,1756.88304848789,
1757.31877448949,1757.75450049109,1758.18937380075,1759.05912042051,1759.49399373061,
1759.92886704086,1760.36374035125,1760.79861366179,1761.23348697248,1761.66836028331,
1762.10323359429,1762.5381069054,1763.40785352806,1763.8427268396,1764.27845284228,
1764.71417884496,1765.14905215677,1765.58392546872,1766.0187987808,1766.88854540534,
1767.75829203039,1768.1931653431,1768.62803865593,1769.06291196888,1769.49778528195,
1770.36753190841,1771.2381312254,1772.10873054259,1772.97847717007,1773.84822379791,
1774.71797042609,1775.58771705456,1776.45746368331,1777.32721031228,1778.19780963089,
1779.06840894783,1779.93815555508,1780.80790201176,1781.67764871408),(-1.76619037915008,
-1.18309518948453),.UNSPECIFIED.) ;
#827=B_SPLINE_SURFACE_WITH_KNOTS('',1,3,((#79059,#79060,#79061,#79062,#79063,
#79064,#79065,#79066,#79067,#79068,#79069,#79070,#79071,#79072,#79073,#79074),
(#79075,#79076,#79077,#79078,#79079,#79080,#79081,#79082,#79083,#79084,
#79085,#79086,#79087,#79088,#79089,#79090)),.UNSPECIFIED.,.F.,.T.,.F.,(2,
2),(4,1,1,1,1,1,1,1,1,1,1,1,1,4),(0.,0.248609854147285),(0.,0.520304865070705,
0.709542561390409,0.804161409708611,0.898780258026813,1.15893269056541,
1.419085123104,1.67923755563226,1.93938998816052,2.03400883639567,2.12862768463082,
2.31786538114359,2.57801781366682,2.83817024619004),.UNSPECIFIED.) ;
#828=B_SPLINE_SURFACE_WITH_KNOTS('',1,3,((#79115,#79116,#79117,#79118,#79119,
#79120,#79121,#79122,#79123,#79124,#79125,#79126,#79127,#79128,#79129,#79130),
(#79131,#79132,#79133,#79134,#79135,#79136,#79137,#79138,#79139,#79140,
#79141,#79142,#79143,#79144,#79145,#79146)),.UNSPECIFIED.,.F.,.T.,.F.,(2,
2),(4,1,1,1,1,1,1,1,1,1,1,1,1,4),(0.,0.248609854327075),(0.,0.520304865043955,
0.70954256158844,0.804161409794499,0.898780258000557,1.15893269054429,1.41908512308802,
1.67923755561058,1.93938998813313,2.03400883648099,2.12862768482886,2.3178653810957,
2.57801781365659,2.83817024621747),.UNSPECIFIED.) ;
#829=B_SPLINE_SURFACE_WITH_KNOTS('',1,3,((#79194,#79195,#79196,#79197,#79198,
#79199,#79200,#79201,#79202,#79203,#79204,#79205,#79206,#79207,#79208,#79209),
(#79210,#79211,#79212,#79213,#79214,#79215,#79216,#79217,#79218,#79219,
#79220,#79221,#79222,#79223,#79224,#79225)),.UNSPECIFIED.,.F.,.T.,.F.,(2,
2),(4,1,1,1,1,1,1,1,1,1,1,1,1,4),(0.,0.248609853678558),(0.,0.520304865114576,
0.709542561608101,0.804161409843274,0.898780258078447,1.1589326906067,1.41908512313495,
1.67923755567353,1.9393899882121,2.03400883653032,2.12862768484853,2.31786538116822,
2.57801781373375,2.83817024629929),.UNSPECIFIED.) ;
#830=B_SPLINE_SURFACE_WITH_KNOTS('',1,3,((#79227,#79228,#79229,#79230,#79231,
#79232,#79233,#79234,#79235,#79236,#79237,#79238,#79239,#79240,#79241,#79242),
(#79243,#79244,#79245,#79246,#79247,#79248,#79249,#79250,#79251,#79252,
#79253,#79254,#79255,#79256,#79257,#79258)),.UNSPECIFIED.,.F.,.T.,.F.,(2,
2),(4,1,1,1,1,1,1,1,1,1,1,1,1,4),(0.,0.248609854201188),(0.,0.520304864990006,
0.709542561256855,0.80416140961432,0.898780257971786,1.15893269048473,1.41908512299766,
1.67923755554141,1.93938998808516,2.03400883629124,2.12862768449733,2.31786538104175,
2.57801781362961,2.83817024621746),.UNSPECIFIED.) ;
#870=FACE_OUTER_BOUND('',#1347,.T.) ;
#871=FACE_OUTER_BOUND('',#1348,.T.) ;
#872=FACE_OUTER_BOUND('',#1349,.T.) ;
#873=FACE_OUTER_BOUND('',#1350,.T.) ;
#874=FACE_OUTER_BOUND('',#1351,.T.) ;
#875=FACE_OUTER_BOUND('',#1352,.T.) ;
#876=FACE_OUTER_BOUND('',#1353,.T.) ;
#877=FACE_OUTER_BOUND('',#1354,.T.) ;
#878=FACE_OUTER_BOUND('',#1355,.T.) ;
#879=FACE_OUTER_BOUND('',#1356,.T.) ;
#880=FACE_OUTER_BOUND('',#1357,.T.) ;
#881=FACE_OUTER_BOUND('',#1362,.T.) ;
#882=FACE_OUTER_BOUND('',#1364,.T.) ;
#883=FACE_OUTER_BOUND('',#1366,.T.) ;
#884=FACE_OUTER_BOUND('',#1367,.T.) ;
#885=FACE_OUTER_BOUND('',#1368,.T.) ;
#886=FACE_OUTER_BOUND('',#1369,.T.) ;
#887=FACE_OUTER_BOUND('',#1370,.T.) ;
#888=FACE_OUTER_BOUND('',#1371,.T.) ;
#889=FACE_OUTER_BOUND('',#1372,.T.) ;
#890=FACE_OUTER_BOUND('',#1373,.T.) ;
#891=FACE_OUTER_BOUND('',#1374,.T.) ;
#892=FACE_OUTER_BOUND('',#1375,.T.) ;
#893=FACE_OUTER_BOUND('',#1376,.T.) ;
#894=FACE_OUTER_BOUND('',#1377,.T.) ;
#895=FACE_OUTER_BOUND('',#1378,.T.) ;
#896=FACE_OUTER_BOUND('',#1379,.T.) ;
#897=FACE_OUTER_BOUND('',#1380,.T.) ;
#898=FACE_OUTER_BOUND('',#1381,.T.) ;
#899=FACE_OUTER_BOUND('',#1382,.T.) ;
#900=FACE_OUTER_BOUND('',#1383,.T.) ;
#901=FACE_OUTER_BOUND('',#1384,.T.) ;
#902=FACE_OUTER_BOUND('',#1385,.T.) ;
#903=FACE_OUTER_BOUND('',#1386,.T.) ;
#904=FACE_OUTER_BOUND('',#1387,.T.) ;
#905=FACE_OUTER_BOUND('',#1388,.T.) ;
#906=FACE_OUTER_BOUND('',#1389,.T.) ;
#907=FACE_OUTER_BOUND('',#1390,.T.) ;
#908=FACE_OUTER_BOUND('',#1391,.T.) ;
#909=FACE_OUTER_BOUND('',#1392,.T.) ;
#910=FACE_OUTER_BOUND('',#1393,.T.) ;
#1347=EDGE_LOOP('',(#5618,#5619,#5620,#5621,#5622,#5623)) ;
#1348=EDGE_LOOP('',(#5624,#5625,#5626,#5627,#5628,#5629)) ;
#1349=EDGE_LOOP('',(#5630,#5631,#5632,#5633,#5634,#5635)) ;
#1350=EDGE_LOOP('',(#5636,#5637,#5638,#5639,#5640,#5641)) ;
#1351=EDGE_LOOP('',(#5642,#5643,#5644,#5645)) ;
#1352=EDGE_LOOP('',(#5646,#5647,#5648,#5649)) ;
#1353=EDGE_LOOP('',(#5650,#5651,#5652,#5653)) ;
#1354=EDGE_LOOP('',(#5654,#5655,#5656,#5657)) ;
#1355=EDGE_LOOP('',(#5658,#5659,#5660,#5661)) ;
#1356=EDGE_LOOP('',(#5662,#5663,#5664,#5665)) ;
#1357=EDGE_LOOP('',(#5666,#5667,#5668,#5669)) ;
#1358=EDGE_LOOP('',(#5670)) ;
#1359=EDGE_LOOP('',(#5671)) ;
#1360=EDGE_LOOP('',(#5672)) ;
#1361=EDGE_LOOP('',(#5673)) ;
#1362=EDGE_LOOP('',(#5674)) ;
#1363=EDGE_LOOP('',(#5675,#5676,#5677)) ;
#1364=EDGE_LOOP('',(#5678)) ;
#1365=EDGE_LOOP('',(#5679,#5680,#5681)) ;
#1366=EDGE_LOOP('',(#5682,#5683,#5684,#5685)) ;
#1367=EDGE_LOOP('',(#5686,#5687,#5688,#5689)) ;
#1368=EDGE_LOOP('',(#5690,#5691,#5692,#5693)) ;
#1369=EDGE_LOOP('',(#5694,#5695,#5696,#5697)) ;
#1370=EDGE_LOOP('',(#5698,#5699,#5700)) ;
#1371=EDGE_LOOP('',(#5701,#5702,#5703)) ;
#1372=EDGE_LOOP('',(#5704,#5705,#5706,#5707,#5708)) ;
#1373=EDGE_LOOP('',(#5709,#5710,#5711,#5712)) ;
#1374=EDGE_LOOP('',(#5713,#5714,#5715,#5716,#5717,#5718,#5719,#5720,#5721,
#5722,#5723,#5724)) ;
#1375=EDGE_LOOP('',(#5725,#5726,#5727)) ;
#1376=EDGE_LOOP('',(#5728,#5729,#5730,#5731,#5732,#5733)) ;
#1377=EDGE_LOOP('',(#5734,#5735,#5736,#5737,#5738,#5739,#5740,#5741,#5742,
#5743,#5744,#5745,#5746)) ;
#1378=EDGE_LOOP('',(#5747,#5748,#5749)) ;
#1379=EDGE_LOOP('',(#5750,#5751,#5752,#5753,#5754,#5755,#5756,#5757,#5758,
#5759,#5760,#5761,#5762,#5763,#5764,#5765,#5766)) ;
#1380=EDGE_LOOP('',(#5767,#5768,#5769)) ;
#1381=EDGE_LOOP('',(#5770,#5771,#5772)) ;
#1382=EDGE_LOOP('',(#5773,#5774,#5775,#5776,#5777)) ;
#1383=EDGE_LOOP('',(#5778,#5779,#5780,#5781,#5782,#5783,#5784,#5785,#5786,
#5787,#5788)) ;
#1384=EDGE_LOOP('',(#5789,#5790,#5791,#5792,#5793,#5794,#5795,#5796,#5797,
#5798,#5799,#5800,#5801)) ;
#1385=EDGE_LOOP('',(#5802,#5803,#5804,#5805,#5806,#5807,#5808,#5809,#5810,
#5811,#5812,#5813,#5814,#5815,#5816,#5817)) ;
#1386=EDGE_LOOP('',(#5818,#5819,#5820,#5821,#5822,#5823,#5824,#5825,#5826,
#5827)) ;
#1387=EDGE_LOOP('',(#5828,#5829,#5830,#5831,#5832)) ;
#1388=EDGE_LOOP('',(#5833,#5834,#5835,#5836,#5837,#5838,#5839,#5840,#5841,
#5842,#5843,#5844,#5845)) ;
#1389=EDGE_LOOP('',(#5846,#5847,#5848,#5849,#5850)) ;
#1390=EDGE_LOOP('',(#5851,#5852,#5853,#5854,#5855,#5856,#5857,#5858,#5859,
#5860)) ;
#1391=EDGE_LOOP('',(#5861,#5862,#5863,#5864,#5865,#5866,#5867,#5868,#5869,
#5870,#5871,#5872,#5873)) ;
#1392=EDGE_LOOP('',(#5874,#5875,#5876,#5877,#5878)) ;
#1393=EDGE_LOOP('',(#5879,#5880,#5881,#5882,#5883)) ;
#1872=LINE('',#12443,#2575) ;
#1873=LINE('',#12710,#2576) ;
#1874=LINE('',#12984,#2577) ;
#1875=LINE('',#13955,#2578) ;
#1876=LINE('',#15019,#2579) ;
#1877=LINE('',#15157,#2580) ;
#1878=LINE('',#15764,#2581) ;
#1879=LINE('',#16034,#2582) ;
#1880=LINE('',#16289,#2583) ;
#1881=LINE('',#17911,#2584) ;
#1882=LINE('',#18440,#2585) ;
#1883=LINE('',#18926,#2586) ;
#1884=LINE('',#18965,#2587) ;
#1885=LINE('',#18969,#2588) ;
#1886=LINE('',#18978,#2589) ;
#1887=LINE('',#33347,#2590) ;
#1888=LINE('',#33351,#2591) ;
#1889=LINE('',#41430,#2592) ;
#1890=LINE('',#43252,#2593) ;
#1891=LINE('',#64560,#2594) ;
#1892=LINE('',#64562,#2595) ;
#1893=LINE('',#64563,#2596) ;
#1894=LINE('',#71962,#2597) ;
#1895=LINE('',#79048,#2598) ;
#1896=LINE('',#79091,#2599) ;
#1897=LINE('',#79094,#2600) ;
#1898=LINE('',#79147,#2601) ;
#1899=LINE('',#79150,#2602) ;
#1900=LINE('',#79183,#2603) ;
#1901=LINE('',#79226,#2604) ;
#1902=LINE('',#79259,#2605) ;
#2575=VECTOR('',#9484,1.2500000000303) ;
#2576=VECTOR('',#9489,1.2500000000303) ;
#2577=VECTOR('',#9492,1.2500000000303) ;
#2578=VECTOR('',#9495,1.2500000000303) ;
#2579=VECTOR('',#9498,1.2500000000303) ;
#2580=VECTOR('',#9501,1.25000000003033) ;
#2581=VECTOR('',#9506,1.25000000003033) ;
#2582=VECTOR('',#9509,1.25000000003033) ;
#2583=VECTOR('',#9512,1.25000000003033) ;
#2584=VECTOR('',#9515,1.25000000003033) ;
#2585=VECTOR('',#9520,2.00000000000006) ;
#2586=VECTOR('',#9527,10.) ;
#2587=VECTOR('',#9528,10.) ;
#2588=VECTOR('',#9531,1.12500000002727) ;
#2589=VECTOR('',#9540,1.12500000002727) ;
#2590=VECTOR('',#9545,10.) ;
#2591=VECTOR('',#9548,10.) ;
#2592=VECTOR('',#9553,10.) ;
#2593=VECTOR('',#9564,1.2500000000303) ;
#2594=VECTOR('',#9567,10.) ;
#2595=VECTOR('',#9570,10.) ;
#2596=VECTOR('',#9571,10.) ;
#2597=VECTOR('',#9574,1.25000000003033) ;
#2598=VECTOR('',#9577,0.300000000000011) ;
#2599=VECTOR('',#9578,10.) ;
#2600=VECTOR('',#9581,0.300000000000011) ;
#2601=VECTOR('',#9582,10.) ;
#2602=VECTOR('',#9585,0.299999999999991) ;
#2603=VECTOR('',#9588,0.299999999999991) ;
#2604=VECTOR('',#9589,10.) ;
#2605=VECTOR('',#9590,10.) ;
#3283=B_SPLINE_CURVE_WITH_KNOTS('',3,(#12445,#12446,#12447,#12448,#12449,
#12450,#12451,#12452,#12453,#12454,#12455,#12456,#12457,#12458,#12459,#12460,
#12461,#12462,#12463,#12464,#12465,#12466,#12467,#12468,#12469,#12470,#12471,
#12472,#12473,#12474,#12475,#12476,#12477,#12478,#12479,#12480,#12481,#12482,
#12483,#12484,#12485,#12486,#12487,#12488,#12489,#12490,#12491,#12492,#12493,
#12494,#12495,#12496,#12497,#12498,#12499,#12500,#12501,#12502,#12503,#12504,
#12505,#12506,#12507,#12508,#12509,#12510,#12511),.UNSPECIFIED.,.F.,.F.,
(4,3,3,3,3,3,3,3,3,3,3,3,3,3,3,3,3,3,3,3,3,3,4),(3.9356112509829,4.03938538435145,
4.25784115129902,4.47513630847502,4.69377120659221,4.91046481666321,4.91951265349917,
5.12906709974552,5.34636177928887,5.56439507544428,5.78215798493518,5.90340082783371,
5.99918563324319,6.21796471286197,6.43674372019706,6.6534047490877,6.87204193031312,
6.88730285777762,7.08914731456076,7.30660608033134,7.52524368403693,7.7424025902883,
7.87117652775501),.UNSPECIFIED.) ;
#3284=B_SPLINE_CURVE_WITH_KNOTS('',3,(#12513,#12514,#12515,#12516,#12517,
#12518,#12519,#12520,#12521,#12522),.UNSPECIFIED.,.F.,.F.,(4,2,2,2,4),(-0.0222585247231994,
-0.013985790625096,-0.011129717560957,-0.00783049479114727,-1.0000000337726E-6),
 .UNSPECIFIED.) ;
#3285=B_SPLINE_CURVE_WITH_KNOTS('',3,(#12526,#12527,#12528,#12529,#12530,
#12531,#12532,#12533,#12534,#12535,#12536,#12537,#12538,#12539,#12540,#12541,
#12542,#12543,#12544,#12545,#12546,#12547,#12548,#12549,#12550,#12551,#12552,
#12553,#12554,#12555,#12556,#12557,#12558,#12559,#12560,#12561,#12562,#12563,
#12564,#12565,#12566,#12567,#12568,#12569,#12570,#12571,#12572,#12573,#12574,
#12575,#12576,#12577,#12578,#12579,#12580,#12581,#12582,#12583,#12584,#12585,
#12586,#12587,#12588,#12589,#12590,#12591,#12592,#12593,#12594,#12595,#12596,
#12597,#12598,#12599,#12600,#12601,#12602,#12603,#12604,#12605,#12606,#12607,
#12608,#12609,#12610,#12611,#12612,#12613,#12614,#12615,#12616,#12617,#12618,
#12619,#12620,#12621,#12622,#12623,#12624,#12625,#12626,#12627,#12628,#12629,
#12630,#12631,#12632,#12633,#12634,#12635,#12636,#12637,#12638,#12639),
 .UNSPECIFIED.,.F.,.F.,(4,2,2,2,2,2,2,2,2,2,2,2,2,2,2,2,2,2,2,2,2,2,2,2,
2,2,2,2,2,2,2,2,2,2,2,2,2,2,2,2,2,2,2,2,2,2,2,2,2,2,2,2,2,2,2,2,4),(-0.153462776225972,
-0.152324705127337,-0.151118454999884,-0.149333742371031,-0.145003214516893,
-0.13835659712187,-0.133835373411754,-0.132745313227134,-0.131847384401116,
-0.13097205154426,-0.129823508837882,-0.127628091775407,-0.119960423600932,
-0.115469114271048,-0.113272377032872,-0.111856947000151,-0.110720541727474,
-0.109751593502618,-0.108578093950052,-0.106442248036253,-0.0998082973084651,
-0.0941484535210442,-0.0917783941701622,-0.0915983015956296,-0.091502767009933,
-0.0913135982719603,-0.0911645589693218,-0.0910481152418994,-0.090957691313955,
-0.0908877816714908,-0.0894531021162402,-0.0883725557521577,-0.0873006436271552,
-0.0858223201796501,-0.0808094581085911,-0.0767363546008492,-0.0716521834197286,
-0.0692343146257553,-0.0676572673759575,-0.0657419763951433,-0.0633985116058406,
-0.0593409392751851,-0.0518183669518645,-0.0482968499863042,-0.0448444812234441,
-0.0386199857778131,-0.035642628427599,-0.0334832603615144,-0.0314977259350848,
-0.0263932638373145,-0.0225987907781864,-0.0202713898632133,-0.0181006589461003,
-0.0127737986074514,-0.00352391886801092,-0.00160881093620446,-1.00000000588518E-6),
 .UNSPECIFIED.) ;
#3286=B_SPLINE_CURVE_WITH_KNOTS('',3,(#12640,#12641,#12642,#12643,#12644,
#12645,#12646,#12647,#12648,#12649,#12650,#12651,#12652,#12653,#12654,#12655,
#12656,#12657,#12658,#12659,#12660,#12661,#12662,#12663,#12664,#12665,#12666,
#12667,#12668,#12669,#12670,#12671,#12672,#12673,#12674,#12675,#12676,#12677,
#12678,#12679,#12680,#12681,#12682,#12683,#12684,#12685,#12686,#12687,#12688,
#12689,#12690,#12691,#12692,#12693,#12694,#12695,#12696,#12697,#12698,#12699,
#12700,#12701,#12702,#12703,#12704,#12705,#12706),.UNSPECIFIED.,.F.,.F.,
(4,3,3,3,3,3,3,3,3,3,3,3,3,3,3,3,3,3,3,3,3,3,4),(0.,0.0975869658197039,
0.316224629921226,0.533974482508371,0.751791450250512,0.970571090053128,
0.983904149333616,1.18687637804593,1.40551330231184,1.62363563448458,1.84012907539297,
1.967779663268,2.05856366171448,2.27719954675489,2.49400168139467,2.71263709677618,
2.93000716182069,2.9516727955564,3.1476956812641,3.36438759275314,3.58302233313812,
3.80139773207559,3.93553521981785),.UNSPECIFIED.) ;
#3287=B_SPLINE_CURVE_WITH_KNOTS('',3,(#12712,#12713,#12714,#12715,#12716,
#12717,#12718,#12719,#12720,#12721,#12722,#12723,#12724,#12725,#12726,#12727,
#12728,#12729,#12730,#12731,#12732,#12733,#12734,#12735,#12736,#12737,#12738,
#12739,#12740,#12741,#12742,#12743,#12744,#12745,#12746,#12747,#12748,#12749,
#12750,#12751,#12752,#12753,#12754,#12755,#12756,#12757,#12758,#12759,#12760,
#12761,#12762,#12763,#12764,#12765,#12766,#12767,#12768,#12769,#12770,#12771,
#12772,#12773,#12774,#12775,#12776,#12777,#12778),.UNSPECIFIED.,.F.,.F.,
(4,3,3,3,3,3,3,3,3,3,3,3,3,3,3,3,3,3,3,3,3,3,4),(3.93547251278037,4.06961094858131,
4.28798638030629,4.50662115468534,4.72331312294551,4.91933700306806,4.94100170508307,
5.15837184749187,5.37700734464929,5.59380956446693,5.8124455505454,5.90323061785796,
6.03088023023819,6.24737376267269,6.46549619232503,6.6841331895427,6.88710479223812,
6.90043854814402,7.11921826246268,7.33703527512716,7.55478517165104,7.77342285580172,
7.87100799512254),.UNSPECIFIED.) ;
#3288=B_SPLINE_CURVE_WITH_KNOTS('',3,(#12779,#12780,#12781,#12782,#12783,
#12784,#12785,#12786,#12787,#12788,#12789,#12790,#12791,#12792,#12793,#12794,
#12795,#12796,#12797,#12798,#12799,#12800,#12801,#12802,#12803,#12804,#12805,
#12806,#12807,#12808,#12809,#12810,#12811,#12812,#12813,#12814,#12815,#12816,
#12817,#12818,#12819,#12820,#12821,#12822,#12823,#12824,#12825,#12826,#12827,
#12828,#12829,#12830,#12831,#12832,#12833,#12834,#12835,#12836,#12837,#12838,
#12839,#12840,#12841,#12842,#12843,#12844,#12845),.UNSPECIFIED.,.F.,.F.,
(4,3,3,3,3,3,3,3,3,3,3,3,3,3,3,3,3,3,3,3,3,3,4),(4.35954652862245E-7,0.119372163261154,
0.337345459789608,0.555020195428233,0.772262251650588,0.983893434075418,
0.990873877762923,1.2084306792763,1.42706758547165,1.64356117973995,1.86123472757703,
1.96779535009552,2.07966351227983,2.29690397078676,2.51539695630481,2.73254404906778,
2.95093109100352,2.95170382931863,3.16941983526542,3.38648900257636,3.60512375286946,
3.82170107768877,3.9356112509829),.UNSPECIFIED.) ;
#3289=B_SPLINE_CURVE_WITH_KNOTS('',3,(#12847,#12848,#12849,#12850,#12851,
#12852,#12853,#12854,#12855,#12856,#12857,#12858,#12859,#12860,#12861,#12862,
#12863,#12864,#12865,#12866,#12867,#12868,#12869,#12870,#12871,#12872,#12873,
#12874,#12875,#12876,#12877,#12878,#12879,#12880,#12881,#12882,#12883,#12884,
#12885,#12886,#12887,#12888,#12889,#12890,#12891,#12892,#12893,#12894,#12895,
#12896,#12897,#12898,#12899,#12900,#12901,#12902,#12903,#12904,#12905,#12906,
#12907,#12908,#12909,#12910,#12911,#12912,#12913),.UNSPECIFIED.,.F.,.F.,
(4,3,3,3,3,3,3,3,3,3,3,3,3,3,3,3,3,3,3,3,3,3,4),(3.93553521981785,4.0186166507456,
4.237394066808,4.45524637685516,4.67168228798332,4.89031731534065,4.91942511752289,
5.10777744143641,5.32641286545437,5.54365324976844,5.76132642843505,5.90327971137444,
5.97977375285268,6.19626741280715,6.41490412589105,6.6327957250643,6.85047016051711,
6.88716122923848,7.06685121073668,7.28548870358118,7.5039832238531,7.72224969150007,
7.87100730541593),.UNSPECIFIED.) ;
#3290=B_SPLINE_CURVE_WITH_KNOTS('',3,(#12914,#12915,#12916,#12917,#12918,
#12919,#12920,#12921,#12922,#12923,#12924,#12925,#12926,#12927,#12928,#12929,
#12930,#12931,#12932,#12933,#12934,#12935,#12936,#12937,#12938,#12939,#12940,
#12941,#12942,#12943,#12944,#12945,#12946,#12947,#12948,#12949,#12950,#12951,
#12952,#12953,#12954,#12955,#12956,#12957,#12958,#12959,#12960,#12961,#12962,
#12963,#12964,#12965,#12966,#12967,#12968,#12969,#12970,#12971,#12972,#12973,
#12974,#12975,#12976,#12977,#12978,#12979,#12980),.UNSPECIFIED.,.F.,.F.,
(4,3,3,3,3,3,3,3,3,3,3,3,3,3,3,3,3,3,3,3,3,3,4),(0.,0.0677050049383632,
0.286200456928864,0.504838070208805,0.721642294535249,0.940279670301964,
0.983887911634322,1.15752095782385,1.37528509523392,1.59197913143046,1.81061559832354,
1.96772752945778,2.02908413902557,2.24679594232941,2.46337476541722,2.6820102099624,
2.89990017557006,2.95160837635821,3.11728168426501,3.33539505176439,3.55269408023814,
3.77118616997486,3.9354465321173),.UNSPECIFIED.) ;
#3291=B_SPLINE_CURVE_WITH_KNOTS('',3,(#12986,#12987,#12988,#12989,#12990,
#12991,#12992,#12993,#12994,#12995,#12996,#12997,#12998,#12999,#13000,#13001,
#13002,#13003,#13004,#13005,#13006,#13007,#13008,#13009,#13010,#13011,#13012,
#13013,#13014,#13015,#13016,#13017,#13018,#13019,#13020,#13021,#13022,#13023,
#13024,#13025,#13026,#13027,#13028,#13029,#13030,#13031,#13032,#13033,#13034,
#13035,#13036,#13037,#13038,#13039,#13040,#13041,#13042,#13043,#13044,#13045,
#13046,#13047,#13048,#13049,#13050,#13051,#13052,#13053,#13054,#13055,#13056,
#13057,#13058,#13059,#13060,#13061,#13062,#13063,#13064,#13065,#13066,#13067,
#13068,#13069,#13070,#13071,#13072,#13073,#13074,#13075,#13076,#13077,#13078,
#13079,#13080,#13081,#13082,#13083,#13084,#13085,#13086,#13087,#13088,#13089,
#13090,#13091,#13092,#13093,#13094,#13095,#13096,#13097,#13098,#13099,#13100,
#13101,#13102,#13103,#13104,#13105,#13106,#13107,#13108,#13109,#13110,#13111,
#13112,#13113,#13114,#13115,#13116,#13117,#13118,#13119,#13120,#13121,#13122,
#13123,#13124,#13125,#13126,#13127,#13128,#13129,#13130,#13131,#13132,#13133,
#13134,#13135,#13136,#13137,#13138,#13139,#13140,#13141,#13142,#13143,#13144,
#13145,#13146,#13147,#13148,#13149,#13150,#13151,#13152,#13153,#13154,#13155,
#13156,#13157,#13158,#13159,#13160,#13161,#13162,#13163,#13164,#13165,#13166,
#13167,#13168,#13169,#13170,#13171,#13172,#13173,#13174,#13175,#13176,#13177,
#13178,#13179,#13180,#13181,#13182,#13183,#13184,#13185,#13186,#13187,#13188,
#13189,#13190,#13191,#13192,#13193,#13194,#13195,#13196,#13197,#13198,#13199,
#13200,#13201,#13202,#13203,#13204,#13205,#13206,#13207,#13208,#13209,#13210,
#13211,#13212,#13213,#13214,#13215,#13216,#13217,#13218,#13219,#13220,#13221,
#13222,#13223,#13224,#13225,#13226,#13227,#13228,#13229,#13230,#13231,#13232,
#13233,#13234,#13235,#13236,#13237,#13238,#13239,#13240,#13241,#13242,#13243,
#13244,#13245,#13246,#13247,#13248,#13249,#13250,#13251,#13252,#13253,#13254,
#13255,#13256,#13257,#13258,#13259,#13260,#13261,#13262,#13263,#13264,#13265,
#13266,#13267,#13268,#13269,#13270,#13271,#13272,#13273,#13274,#13275,#13276,
#13277,#13278,#13279,#13280,#13281,#13282,#13283,#13284,#13285,#13286,#13287,
#13288,#13289,#13290,#13291,#13292,#13293,#13294,#13295,#13296,#13297,#13298,
#13299,#13300,#13301,#13302,#13303,#13304,#13305,#13306,#13307,#13308,#13309,
#13310,#13311,#13312,#13313,#13314,#13315,#13316,#13317,#13318,#13319,#13320,
#13321,#13322,#13323,#13324,#13325,#13326,#13327,#13328,#13329,#13330,#13331,
#13332,#13333,#13334,#13335,#13336,#13337,#13338,#13339,#13340,#13341,#13342,
#13343,#13344,#13345,#13346,#13347,#13348,#13349,#13350,#13351,#13352,#13353,
#13354,#13355,#13356,#13357,#13358,#13359,#13360,#13361,#13362,#13363,#13364,
#13365,#13366,#13367,#13368,#13369,#13370,#13371,#13372,#13373,#13374,#13375,
#13376,#13377,#13378,#13379,#13380,#13381,#13382,#13383,#13384,#13385,#13386,
#13387,#13388,#13389,#13390,#13391,#13392,#13393,#13394,#13395,#13396,#13397,
#13398,#13399,#13400,#13401,#13402,#13403,#13404,#13405,#13406,#13407,#13408,
#13409,#13410,#13411,#13412,#13413,#13414,#13415,#13416,#13417,#13418,#13419,
#13420,#13421,#13422,#13423,#13424,#13425,#13426,#13427,#13428,#13429,#13430,
#13431,#13432,#13433,#13434,#13435,#13436,#13437,#13438,#13439,#13440,#13441,
#13442,#13443,#13444,#13445,#13446,#13447,#13448,#13449,#13450,#13451,#13452,
#13453,#13454,#13455,#13456,#13457,#13458,#13459,#13460,#13461,#13462,#13463,
#13464,#13465,#13466,#13467,#13468,#13469,#13470,#13471,#13472,#13473,#13474,
#13475,#13476,#13477,#13478,#13479,#13480,#13481,#13482,#13483,#13484,#13485,
#13486,#13487,#13488,#13489,#13490,#13491,#13492,#13493,#13494,#13495,#13496,
#13497,#13498,#13499,#13500,#13501,#13502,#13503,#13504,#13505,#13506,#13507,
#13508,#13509,#13510,#13511,#13512,#13513,#13514,#13515,#13516,#13517,#13518,
#13519,#13520,#13521,#13522,#13523,#13524,#13525,#13526,#13527,#13528,#13529,
#13530,#13531,#13532,#13533,#13534,#13535,#13536,#13537,#13538,#13539,#13540,
#13541,#13542,#13543,#13544,#13545),.UNSPECIFIED.,.F.,.F.,(4,2,2,2,2,2,
2,2,2,2,2,2,2,2,2,2,2,2,2,2,2,2,2,2,2,2,2,2,2,2,2,2,2,2,2,2,2,2,2,2,2,2,
2,2,2,2,2,2,2,2,2,2,2,2,2,2,2,2,2,2,2,2,2,2,2,2,2,2,2,2,2,2,2,2,2,2,2,2,
2,2,2,2,2,2,2,2,2,2,2,2,2,2,2,2,2,2,2,2,2,2,2,2,2,2,2,2,2,2,2,2,2,2,2,2,
2,2,2,2,2,2,2,2,2,2,2,2,2,2,2,2,2,2,2,2,2,2,2,2,2,2,2,2,2,2,2,2,2,2,2,2,
2,2,2,2,2,2,2,2,2,2,2,2,2,2,2,2,2,2,2,2,2,2,2,2,2,2,2,2,2,2,2,2,2,2,2,2,
2,2,2,2,2,2,2,2,2,2,2,2,2,2,2,2,2,2,2,2,2,2,2,2,2,2,2,2,2,2,2,2,2,2,2,2,
2,2,2,2,2,2,2,2,2,2,2,2,2,2,2,2,2,2,2,2,2,2,2,2,2,2,2,2,2,2,2,2,2,2,2,2,
2,2,2,2,2,2,2,2,2,2,2,2,2,2,2,2,2,2,2,2,2,4),(-0.393137881593438,-0.389064719683897,
-0.386009163097905,-0.385981265578937,-0.385945108836368,-0.385909794020154,
-0.385875282553561,-0.385841538154784,-0.385808526670231,-0.385776215945061,
-0.385744575643447,-0.385713577137668,-0.385683193419207,-0.385653398899929,
-0.385624169353304,-0.3855954818173,-0.385567314554562,-0.385539646925394,
-0.385512459300206,-0.38548573304274,-0.385459450436866,-0.385433594604264,
-0.385408149413348,-0.38538309950479,-0.385358430245372,-0.385334127660716,
-0.385310178392478,-0.385286569649997,-0.385263289186791,-0.385240325295512,
-0.385217666806629,-0.385195302950154,-0.385173223392286,-0.385151418221862,
-0.385129877964114,-0.38510859346962,-0.385087555927281,-0.38506675688553,
-0.382193288159145,-0.378643776553383,-0.372987032673473,-0.370532901093016,
-0.367420038226476,-0.365735167603049,-0.364371223425476,-0.362805195776009,
-0.360769131760525,-0.357030669202214,-0.347953392087648,-0.345637025624622,
-0.343909370054482,-0.343898550497168,-0.343887881487955,-0.343877358895261,
-0.343866978617838,-0.343856737143705,-0.343846630668866,-0.342404946987773,
-0.342399739837498,-0.340389768977736,-0.337225312112191,-0.328012436212014,
-0.325339571894854,-0.323238491998288,-0.321074407389107,-0.312876297699838,
-0.309143304068466,-0.305494730244086,-0.292360872563278,-0.287021783224246,
-0.278556287551638,-0.276295069825672,-0.273635629426088,-0.273603569246504,
-0.273571755268592,-0.273540177451555,-0.273508826072954,-0.27347769171537,
-0.273446765245543,-0.273416037711126,-0.2733855003582,-0.27335514473055,
-0.273324962374537,-0.273294945231453,-0.273265085345797,-0.273235374864648,
-0.273205806152832,-0.273176371752135,-0.273147064283172,-0.273117876550817,
-0.273088801554495,-0.270488295678629,-0.267434391112323,-0.260733533799063,
-0.258124972448113,-0.25665576277279,-0.255967011402266,-0.254691877630724,
-0.253222721618945,-0.250969687319429,-0.245996994877722,-0.244458155047862,
-0.238929481981041,-0.237109779149582,-0.23562893190682,-0.235114669270249,
-0.23510527824484,-0.235095943200605,-0.23508666243864,-0.235077434592277,
-0.235068258329171,-0.23505913223512,-0.235050054796457,-0.235041024921968,
-0.23503204133481,-0.235023102795624,-0.23501420791345,-0.233317826364142,
-0.231331108821098,-0.227772701309594,-0.218656615672096,-0.215977453808853,
-0.215758282067611,-0.215512652033937,-0.215205754365662,-0.214758261696359,
-0.213155418319634,-0.210596281508668,-0.207035169697749,-0.19705905462199,
-0.191068766209985,-0.186517849648799,-0.182774919494473,-0.176531897491971,
-0.171684381933814,-0.169802781088252,-0.168531950096097,-0.167101615381119,
-0.165419900551934,-0.162807962076873,-0.156713689775964,-0.151097233777737,
-0.149355284868497,-0.147974374870866,-0.146676446306276,-0.146662048893367,
-0.146647590455199,-0.146633067451535,-0.146618476015309,-0.146603812396323,
-0.146589072896078,-0.1465742536766,-0.146559350880369,-0.146544360644392,
-0.146529279061066,-0.146514102176747,-0.146498826032116,-0.146483446528305,
-0.145022506404609,-0.1428831304497,-0.138743236588388,-0.130193530613127,
-0.128000750207622,-0.126822307669245,-0.125989676753377,-0.125972568843055,
-0.125957448615906,-0.12594411680296,-0.125932386946588,-0.125922086452357,
-0.125907945915367,-0.12589422147439,-0.125880906743579,-0.125867995017865,
-0.125855479563493,-0.125843353406085,-0.125831609296632,-0.124545889979032,
-0.123054230407459,-0.120618083045251,-0.114738096948853,-0.109085202066367,
-0.106461472196433,-0.104957436840786,-0.103756569812449,-0.103727129216677,
-0.103698167169185,-0.103669631891777,-0.103641475317349,-0.103613652549213,
-0.103586121444439,-0.103558842369885,-0.103531777824728,-0.10350489215023,
-0.103478151347447,-0.103451522768268,-0.10342497499356,-0.103398477630204,
-0.103372001174486,-0.103345516866451,-0.103318996425612,-0.10329241209262,
-0.10326573648879,-0.103238942402091,-0.103212002790916,-0.103184890572307,
-0.103157578580833,-0.103130039536487,-0.103102245868264,-0.103074169644922,
-0.103045782494817,-0.103017055491307,-0.102987959086974,-0.102958463062207,
-0.101523800085531,-0.0994324376486281,-0.0955430038437078,-0.0911201356083864,
-0.0854236788472147,-0.0839197154323816,-0.0830250946066951,-0.0821241714122678,
-0.0821135781755158,-0.0821031876279128,-0.0820929993889011,-0.0820830128687592,
-0.082073227467589,-0.0820636423483411,-0.0820542568396713,-0.0820450699627639,
-0.0820360806242098,-0.0820272876877643,-0.0807182497594875,-0.0792099620321136,
-0.0764044814883249,-0.0661392203353249,-0.0637492916655484,-0.0624181589015095,
-0.0613871859981794,-0.0612864336191271,-0.0612080546638962,-0.0611437934676291,
-0.0610891162320329,-0.0610412637399253,-0.0609984305477696,-0.0609593679774651,
-0.060923172538446,-0.0608891645204566,-0.060856814182384,-0.0608256946310408,
-0.0607954502793569,-0.0607657749375909,-0.0607363960142241,-0.0607070623707868,
-0.0606775346441359,-0.0606475771504467,-0.0606169504604617,-0.0605854041988785,
-0.060552669831555,-0.060518452696715,-0.0596102459314531,-0.0578951459211566,
-0.0547051042139423,-0.0471683111335125,-0.0440718493941549,-0.0424328101440815,
-0.0407738146829186,-0.0385041307164526,-0.0355007232875941,-0.0296701859213648,
-0.0284423965395485,-0.0274091206939878,-0.0259781110431152,-0.0245484004838547,
-0.0188048286315949,-0.0164738907366568,-0.0146236725297017,-0.0128934667137873,
-0.0108113783584484,-1.00000004499279E-6),.UNSPECIFIED.) ;
#3292=B_SPLINE_CURVE_WITH_KNOTS('',3,(#13546,#13547,#13548,#13549,#13550,
#13551,#13552,#13553,#13554,#13555,#13556,#13557,#13558,#13559,#13560,#13561,
#13562,#13563,#13564,#13565,#13566,#13567,#13568,#13569,#13570,#13571,#13572,
#13573,#13574,#13575,#13576,#13577,#13578,#13579,#13580,#13581,#13582,#13583,
#13584,#13585,#13586,#13587,#13588,#13589,#13590,#13591,#13592,#13593,#13594,
#13595,#13596,#13597,#13598,#13599,#13600,#13601,#13602,#13603,#13604,#13605,
#13606,#13607,#13608,#13609,#13610,#13611,#13612),.UNSPECIFIED.,.F.,.F.,
(4,3,3,3,3,3,3,3,3,3,3,3,3,3,3,3,3,3,3,3,3,3,4),(8.59967866152634E-7,0.148759741016015,
0.367026201262003,0.585520705308296,0.804158161069697,0.983846684918452,
1.02053917198305,1.23821355501075,1.45610509475366,1.67474173516512,1.89123532545487,
1.96773238352147,2.10968257916154,2.32735567819506,2.5445960047733,2.76323136417574,
2.95158227043394,2.98069144299397,3.19932642889525,3.41576230303415,3.63361460867738,
3.85239201540518,3.93547251278037),.UNSPECIFIED.) ;
#3293=B_SPLINE_CURVE_WITH_KNOTS('',3,(#13614,#13615,#13616,#13617,#13618,
#13619,#13620,#13621,#13622,#13623,#13624,#13625,#13626,#13627,#13628,#13629,
#13630,#13631,#13632,#13633,#13634,#13635,#13636,#13637,#13638,#13639,#13640,
#13641,#13642,#13643,#13644,#13645,#13646,#13647,#13648,#13649,#13650,#13651,
#13652,#13653,#13654,#13655,#13656,#13657,#13658,#13659,#13660,#13661,#13662,
#13663,#13664,#13665,#13666,#13667,#13668,#13669,#13670,#13671,#13672,#13673,
#13674,#13675,#13676,#13677),.UNSPECIFIED.,.F.,.F.,(4,3,3,3,3,3,3,3,3,3,
3,3,3,3,3,3,3,3,3,3,3,4),(3.9354465321173,3.98915356100037,4.20712406009794,
4.42428050568497,4.64267699059911,4.91961240864166,5.07847247943613,5.35085269365423,
5.51424929699302,5.73192619675865,5.90507510819469,5.95042577873663,6.16906217982155,
6.37457560045768,6.38686811203847,6.65623297772514,6.82404441772877,6.89060319718431,
7.2601083892678,7.53715824562949,7.69704795638202,7.87704726288776),
 .UNSPECIFIED.) ;
#3294=B_SPLINE_CURVE_WITH_KNOTS('',3,(#13678,#13679,#13680,#13681,#13682,
#13683,#13684,#13685,#13686,#13687,#13688,#13689,#13690,#13691,#13692,#13693,
#13694,#13695,#13696,#13697,#13698,#13699,#13700,#13701,#13702,#13703,#13704,
#13705,#13706,#13707,#13708,#13709,#13710,#13711,#13712,#13713,#13714,#13715,
#13716,#13717,#13718,#13719,#13720,#13721,#13722,#13723,#13724,#13725,#13726,
#13727,#13728,#13729,#13730,#13731,#13732,#13733,#13734,#13735,#13736,#13737,
#13738,#13739,#13740,#13741,#13742,#13743,#13744,#13745,#13746,#13747,#13748,
#13749,#13750,#13751,#13752,#13753,#13754,#13755,#13756,#13757,#13758,#13759,
#13760,#13761,#13762,#13763,#13764,#13765,#13766,#13767,#13768,#13769,#13770,
#13771,#13772,#13773,#13774,#13775,#13776,#13777,#13778,#13779,#13780,#13781,
#13782,#13783,#13784,#13785,#13786,#13787,#13788,#13789,#13790,#13791,#13792,
#13793,#13794,#13795,#13796,#13797,#13798,#13799,#13800,#13801,#13802,#13803,
#13804,#13805,#13806,#13807,#13808,#13809,#13810,#13811,#13812,#13813,#13814,
#13815,#13816,#13817,#13818,#13819,#13820,#13821,#13822,#13823,#13824,#13825,
#13826,#13827,#13828,#13829,#13830,#13831,#13832,#13833,#13834,#13835,#13836,
#13837,#13838,#13839,#13840,#13841,#13842,#13843,#13844,#13845,#13846,#13847,
#13848,#13849,#13850,#13851,#13852,#13853,#13854,#13855,#13856,#13857,#13858,
#13859,#13860,#13861,#13862,#13863,#13864,#13865,#13866,#13867,#13868,#13869,
#13870,#13871,#13872,#13873,#13874,#13875,#13876,#13877,#13878,#13879,#13880,
#13881,#13882,#13883,#13884,#13885,#13886,#13887,#13888,#13889,#13890,#13891,
#13892,#13893,#13894,#13895,#13896,#13897,#13898,#13899,#13900,#13901,#13902,
#13903,#13904,#13905,#13906,#13907,#13908,#13909,#13910,#13911,#13912,#13913,
#13914,#13915,#13916,#13917,#13918,#13919,#13920,#13921,#13922,#13923,#13924,
#13925,#13926,#13927,#13928,#13929,#13930,#13931,#13932,#13933,#13934,#13935,
#13936,#13937,#13938,#13939,#13940,#13941,#13942,#13943,#13944,#13945,#13946,
#13947,#13948,#13949,#13950,#13951),.UNSPECIFIED.,.F.,.F.,(4,2,2,2,2,2,
2,2,2,2,2,2,2,2,2,2,2,2,2,2,2,2,2,2,2,2,2,2,2,2,2,2,2,2,2,2,2,2,2,2,2,2,
2,2,2,2,2,2,2,2,2,2,2,2,2,2,2,2,2,2,2,2,2,2,2,2,2,2,2,2,2,2,2,2,2,2,2,2,
2,2,2,2,2,2,2,2,2,2,2,2,2,2,2,2,2,2,2,2,2,2,2,2,2,2,2,2,2,2,2,2,2,2,2,2,
2,2,2,2,2,2,2,2,2,2,2,2,2,2,2,2,2,2,2,2,2,2,4),(-0.78638743863695,-0.783865136144057,
-0.781227861189557,-0.775152455613647,-0.766097510440291,-0.764097187693509,
-0.762309586971155,-0.760388178638292,-0.750981145966468,-0.742556535881132,
-0.740397682240013,-0.738484603898096,-0.736428582945787,-0.733875728280658,
-0.720932434032318,-0.717090859955029,-0.713389531042879,-0.710543028580515,
-0.693217343571822,-0.684636960856421,-0.680602460523877,-0.677007808154327,
-0.672649036269041,-0.661361827188727,-0.657367118065297,-0.654995127670715,
-0.653194778532826,-0.651398773584184,-0.649592474131525,-0.646251677215004,
-0.633032827345746,-0.62900903821384,-0.625374040640956,-0.62420154344307,
-0.617366718673342,-0.604222248212363,-0.597956446250104,-0.593485626003035,
-0.590208461213278,-0.585652486573894,-0.579451808375542,-0.572217577000446,
-0.569040010266564,-0.567102499947043,-0.565627562365034,-0.564173918933921,
-0.562517093097831,-0.559749200122382,-0.547987375366625,-0.540992348486649,
-0.53597161103656,-0.531601371432412,-0.530959041091284,-0.524707311709599,
-0.515867392725084,-0.507259310520406,-0.491002889787648,-0.486333349667312,
-0.483720612002522,-0.481821745073192,-0.480034700172722,-0.478257691761641,
-0.47576159989498,-0.465424549016278,-0.460609133799591,-0.458532191954113,
-0.457272245676355,-0.457266970231644,-0.457261751543754,-0.457256589587902,
-0.457251483390092,-0.457246432456842,-0.457241436079759,-0.457236493736514,
-0.457231604579641,-0.4572267678496,-0.457221983074196,-0.457217249922691,
-0.457212567335756,-0.457207935019405,-0.457203352445893,-0.457198818836132,
-0.457194333613499,-0.457189896411029,-0.457185506733976,-0.457181163236356,
-0.457176865874477,-0.457172614534079,-0.457168408126551,-0.457164246157086,
-0.45716012841437,-0.45715605432794,-0.457152023024765,-0.457148034407447,
-0.457144087795822,-0.457140182898109,-0.457136319059025,-0.457132495711979,
-0.457128712683886,-0.457124969589037,-0.457121265258414,-0.457117599629425,
-0.457113972289284,-0.45711038266605,-0.457106830488197,-0.45710331530434,
-0.457099836483116,-0.457096393787484,-0.457092987007351,-0.457089615480539,
-0.457086278913952,-0.457082976598086,-0.457079708498414,-0.457076474003513,
-0.457073272275524,-0.457070103696024,-0.457066968019619,-0.457063864356098,
-0.457060791889488,-0.457057751060048,-0.457054740955454,-0.45705176175811,
-0.457047854051728,-0.456092813665629,-0.455001710574267,-0.45314295087414,
-0.446964288888894,-0.441277563909847,-0.437106277410539,-0.434669623740107,
-0.432822778663546,-0.430965724317635,-0.428823650941757,-0.425037202595733,
-0.408253975266002,-0.39869121832428,-0.393164256152506),.UNSPECIFIED.) ;
#3295=B_SPLINE_CURVE_WITH_KNOTS('',3,(#13957,#13958,#13959,#13960,#13961,
#13962,#13963,#13964,#13965,#13966,#13967,#13968,#13969,#13970,#13971,#13972,
#13973,#13974,#13975,#13976,#13977,#13978,#13979,#13980,#13981,#13982,#13983,
#13984,#13985,#13986,#13987,#13988,#13989,#13990,#13991,#13992,#13993,#13994,
#13995,#13996,#13997,#13998,#13999,#14000,#14001,#14002,#14003,#14004,#14005,
#14006,#14007,#14008,#14009,#14010,#14011,#14012,#14013,#14014,#14015,#14016,
#14017,#14018,#14019,#14020,#14021,#14022,#14023,#14024,#14025,#14026,#14027,
#14028,#14029,#14030,#14031,#14032,#14033,#14034,#14035,#14036,#14037,#14038,
#14039,#14040,#14041,#14042,#14043,#14044,#14045,#14046,#14047,#14048,#14049,
#14050,#14051,#14052,#14053,#14054,#14055,#14056,#14057,#14058,#14059,#14060,
#14061,#14062,#14063,#14064,#14065,#14066,#14067,#14068,#14069,#14070,#14071,
#14072,#14073,#14074,#14075,#14076,#14077,#14078,#14079,#14080,#14081,#14082,
#14083,#14084,#14085,#14086,#14087,#14088,#14089,#14090,#14091,#14092,#14093,
#14094,#14095,#14096,#14097,#14098,#14099,#14100,#14101,#14102,#14103,#14104,
#14105,#14106,#14107,#14108,#14109,#14110,#14111,#14112,#14113,#14114,#14115,
#14116,#14117,#14118,#14119,#14120,#14121,#14122,#14123,#14124,#14125,#14126,
#14127,#14128,#14129,#14130,#14131,#14132,#14133,#14134,#14135,#14136,#14137,
#14138,#14139,#14140,#14141,#14142,#14143,#14144,#14145,#14146,#14147,#14148,
#14149,#14150,#14151,#14152,#14153,#14154,#14155,#14156,#14157,#14158,#14159,
#14160,#14161,#14162,#14163,#14164,#14165,#14166,#14167,#14168,#14169,#14170,
#14171,#14172,#14173,#14174,#14175,#14176,#14177,#14178,#14179,#14180,#14181,
#14182,#14183,#14184,#14185,#14186,#14187,#14188,#14189,#14190,#14191,#14192,
#14193,#14194,#14195,#14196,#14197,#14198,#14199,#14200,#14201,#14202,#14203,
#14204,#14205,#14206,#14207,#14208,#14209,#14210,#14211,#14212,#14213,#14214,
#14215,#14216,#14217,#14218,#14219,#14220,#14221,#14222,#14223,#14224,#14225,
#14226,#14227,#14228,#14229,#14230),.UNSPECIFIED.,.F.,.F.,(4,2,2,2,2,2,
2,2,2,2,2,2,2,2,2,2,2,2,2,2,2,2,2,2,2,2,2,2,2,2,2,2,2,2,2,2,2,2,2,2,2,2,
2,2,2,2,2,2,2,2,2,2,2,2,2,2,2,2,2,2,2,2,2,2,2,2,2,2,2,2,2,2,2,2,2,2,2,2,
2,2,2,2,2,2,2,2,2,2,2,2,2,2,2,2,2,2,2,2,2,2,2,2,2,2,2,2,2,2,2,2,2,2,2,2,
2,2,2,2,2,2,2,2,2,2,2,2,2,2,2,2,2,2,2,2,2,2,4),(-0.393155650627907,-0.387629727924683,
-0.378068230731882,-0.361287776199656,-0.357500578681126,-0.355358535505596,
-0.353501602296624,-0.351655080524313,-0.349219040259675,-0.345049209213823,
-0.33936278735035,-0.333183989104826,-0.331325463430025,-0.3302344953374,
-0.329279567659575,-0.329275660740877,-0.329272683216366,-0.329269675131916,
-0.32926663546163,-0.32926356446945,-0.329260461873318,-0.329257326950647,
-0.329254159310184,-0.329250959069278,-0.329247725451569,-0.32924445849536,
-0.329241157598115,-0.329237822001912,-0.329234451827529,-0.329231046267257,
-0.329227605084572,-0.329224127780796,-0.329220614096719,-0.329217063471653,
-0.329213475265059,-0.329209849357973,-0.329206185080382,-0.329202481745933,
-0.329198739421806,-0.329194957807482,-0.329191135890187,-0.329187273587689,
-0.329183370094182,-0.329179424994815,-0.329175437803989,-0.329171407809548,
-0.329167335082706,-0.329163219015704,-0.329159058468777,-0.329154853485093,
-0.329150603751954,-0.329146308354663,-0.329141966379954,-0.329137577978438,
-0.329133142276796,-0.329128658730507,-0.329124126752042,-0.329119546000515,
-0.329114915761884,-0.329110235079655,-0.329105503478469,-0.329100720530011,
-0.329095885784316,-0.329090998346089,-0.329086057751377,-0.329081063161586,
-0.32907601396187,-0.329070909730608,-0.32906574975319,-0.329060533062429,
-0.329055259360269,-0.327795550975526,-0.325719003041814,-0.320904544524618,
-0.31056875890951,-0.30807314487149,-0.306296471718684,-0.304509772629784,
-0.302611272054989,-0.299999045073864,-0.29533043182203,-0.279076934495437,
-0.270470430520659,-0.261632120091862,-0.255381771120378,-0.254739617695096,
-0.250371737921051,-0.245351992063265,-0.238358876007113,-0.226596184096797,
-0.22382905230438,-0.222172585951009,-0.220719246692206,-0.219244572248415,
-0.217307373489516,-0.214130264922035,-0.206896736850026,-0.200696423966184,
-0.196142809980264,-0.192866381682365,-0.188395571634731,-0.182128464896467,
-0.168982401357977,-0.162153235280996,-0.16098254727699,-0.157348466548358,
-0.153324497182617,-0.140139096102638,-0.136783434587749,-0.134974848879064,
-0.133177422459453,-0.131378834625872,-0.12901199397723,-0.125031635429469,
-0.11386010124943,-0.10942740329141,-0.10584250125783,-0.101838714256601,
-0.0935015891921936,-0.0755843737492411,-0.0724654902868474,-0.0692767199008584,
-0.0654317269939601,-0.0525099573245685,-0.0499547679711224,-0.0478985120680001,
-0.0459856695307695,-0.0438283325047181,-0.0353950616692065,-0.0259975052079688,
-0.0240759710615349,-0.0222886006567847,-0.0202890763344258,-0.0112347913638698,
-0.00515985773145303,-0.00252293204832874,-1.00000001163059E-6),
 .UNSPECIFIED.) ;
#3296=B_SPLINE_CURVE_WITH_KNOTS('',3,(#14231,#14232,#14233,#14234,#14235,
#14236,#14237,#14238,#14239,#14240,#14241,#14242,#14243,#14244,#14245,#14246,
#14247,#14248,#14249,#14250,#14251,#14252,#14253,#14254,#14255,#14256,#14257,
#14258,#14259,#14260,#14261,#14262,#14263,#14264,#14265,#14266,#14267,#14268,
#14269,#14270,#14271,#14272,#14273,#14274,#14275,#14276,#14277,#14278,#14279,
#14280,#14281,#14282,#14283,#14284,#14285,#14286,#14287,#14288,#14289,#14290,
#14291,#14292,#14293,#14294,#14295,#14296,#14297,#14298,#14299,#14300,#14301,
#14302,#14303,#14304,#14305,#14306,#14307,#14308,#14309,#14310,#14311,#14312,
#14313,#14314,#14315,#14316,#14317,#14318,#14319,#14320,#14321,#14322,#14323,
#14324,#14325,#14326,#14327,#14328,#14329,#14330,#14331,#14332,#14333,#14334,
#14335,#14336,#14337,#14338,#14339,#14340,#14341,#14342,#14343,#14344,#14345,
#14346,#14347,#14348,#14349,#14350,#14351,#14352,#14353,#14354,#14355,#14356,
#14357,#14358,#14359,#14360,#14361,#14362,#14363,#14364,#14365,#14366,#14367,
#14368,#14369,#14370,#14371,#14372,#14373,#14374,#14375,#14376,#14377,#14378,
#14379,#14380,#14381,#14382,#14383,#14384,#14385,#14386,#14387,#14388,#14389,
#14390,#14391,#14392,#14393,#14394,#14395,#14396,#14397,#14398,#14399,#14400,
#14401,#14402,#14403,#14404,#14405,#14406,#14407,#14408,#14409,#14410,#14411,
#14412,#14413,#14414,#14415,#14416,#14417,#14418,#14419,#14420,#14421,#14422,
#14423,#14424,#14425,#14426,#14427,#14428,#14429,#14430,#14431,#14432,#14433,
#14434,#14435,#14436,#14437,#14438,#14439,#14440,#14441,#14442,#14443,#14444,
#14445,#14446,#14447,#14448,#14449,#14450),.UNSPECIFIED.,.F.,.F.,(4,2,2,
2,2,2,2,2,2,2,2,2,2,2,2,2,2,2,2,2,2,2,2,2,2,2,2,2,2,2,2,2,2,2,2,2,2,2,2,
2,2,2,2,2,2,2,2,2,2,2,2,2,2,2,2,2,2,2,2,2,2,2,2,2,2,2,2,2,2,2,2,2,2,2,2,
2,2,2,2,2,2,2,2,2,2,2,2,2,2,2,2,2,2,2,2,2,2,2,2,2,2,2,2,2,2,2,2,2,2,4),
(-0.786273343435783,-0.773001471184209,-0.770573001975978,-0.768742355216508,
-0.766587767425843,-0.75899866934865,-0.75313139285783,-0.748699410766708,
-0.745705140539268,-0.742153195664726,-0.733428079293303,-0.728390926211773,
-0.726047785065597,-0.724277512874789,-0.722102272001067,-0.716420527903919,
-0.708093128085561,-0.704303759993659,-0.700288158954778,-0.691004273053775,
-0.686295144006975,-0.683880403467859,-0.682049599009929,-0.680014623759397,
-0.674617926078111,-0.667788657679692,-0.6643712859418,-0.661781895527913,
-0.65932165481377,-0.656051581552829,-0.647904383004953,-0.640525521808526,
-0.637756931237378,-0.635428184108743,-0.633020815526334,-0.631055785105423,
-0.6248745021367,-0.610275329302061,-0.606383693716128,-0.598297144223019,
-0.595215862502454,-0.592298706664051,-0.58606470101389,-0.581297788829462,
-0.569557635011832,-0.559040071782923,-0.55432033337968,-0.550634954450769,
-0.545470871844967,-0.537097023751534,-0.53129252517215,-0.526638712070383,
-0.515594536656462,-0.511360598200319,-0.508800616753945,-0.506335217761588,
-0.500095809376638,-0.493827715412358,-0.491575074254936,-0.491064556932098,
-0.487643095843383,-0.483876584508024,-0.475691649455891,-0.46980958524541,
-0.467180697532896,-0.465388922663278,-0.464200231400658,-0.462022156132893,
-0.455997116918477,-0.453227582516795,-0.453121577243071,-0.453023566146825,
-0.452932655182824,-0.452848051936698,-0.452769051778779,-0.452695026002403,
-0.452625411547095,-0.450412176489763,-0.447942918212535,-0.439410964102818,
-0.435408352651825,-0.432844648959021,-0.430509129130819,-0.427850578028832,
-0.422648173050742,-0.416008935206783,-0.414077849275576,-0.411778535426679,
-0.411736691025614,-0.411696134004543,-0.411656802430231,-0.411618637158931,
-0.411581581737191,-0.411545582241584,-0.411510587133983,-0.41147654712428,
-0.411443415053054,-0.411411145749891,-0.411379695948769,-0.411349024162954,
-0.411319090573825,-0.41128985691958,-0.411261286449138,-0.411233343753753,
-0.411205994709181,-0.409143892858475,-0.40678019535758,-0.398862602884172,
-0.393445365823776,-0.393137881593438),.UNSPECIFIED.) ;
#3297=B_SPLINE_CURVE_WITH_KNOTS('',3,(#14452,#14453,#14454,#14455,#14456,
#14457,#14458,#14459,#14460,#14461,#14462,#14463,#14464,#14465,#14466,#14467,
#14468,#14469,#14470,#14471,#14472,#14473,#14474,#14475,#14476,#14477,#14478,
#14479,#14480,#14481,#14482,#14483,#14484,#14485,#14486,#14487,#14488,#14489,
#14490,#14491,#14492,#14493,#14494,#14495,#14496,#14497,#14498,#14499,#14500,
#14501,#14502,#14503,#14504,#14505,#14506,#14507,#14508,#14509,#14510,#14511,
#14512,#14513,#14514,#14515,#14516,#14517,#14518,#14519,#14520,#14521,#14522,
#14523,#14524,#14525,#14526,#14527,#14528,#14529,#14530,#14531,#14532,#14533,
#14534,#14535,#14536,#14537,#14538,#14539,#14540,#14541,#14542,#14543,#14544,
#14545,#14546,#14547,#14548,#14549,#14550,#14551,#14552,#14553,#14554,#14555,
#14556,#14557,#14558,#14559,#14560,#14561,#14562,#14563,#14564,#14565,#14566,
#14567,#14568,#14569,#14570,#14571,#14572,#14573,#14574,#14575,#14576,#14577,
#14578,#14579,#14580,#14581,#14582,#14583,#14584,#14585,#14586,#14587,#14588,
#14589,#14590,#14591,#14592,#14593,#14594,#14595,#14596,#14597,#14598,#14599,
#14600,#14601,#14602,#14603,#14604,#14605,#14606,#14607,#14608,#14609,#14610,
#14611,#14612,#14613,#14614,#14615,#14616,#14617,#14618,#14619,#14620,#14621,
#14622,#14623,#14624,#14625,#14626,#14627,#14628,#14629,#14630,#14631,#14632,
#14633,#14634,#14635,#14636,#14637,#14638,#14639,#14640,#14641,#14642,#14643,
#14644,#14645,#14646,#14647,#14648,#14649,#14650,#14651,#14652,#14653,#14654,
#14655,#14656,#14657,#14658,#14659,#14660,#14661,#14662,#14663,#14664,#14665,
#14666,#14667,#14668,#14669,#14670,#14671,#14672,#14673,#14674,#14675,#14676,
#14677,#14678,#14679,#14680,#14681,#14682,#14683,#14684,#14685,#14686,#14687,
#14688,#14689,#14690,#14691,#14692,#14693,#14694,#14695,#14696,#14697,#14698,
#14699,#14700,#14701,#14702,#14703,#14704,#14705,#14706,#14707,#14708,#14709,
#14710,#14711,#14712,#14713,#14714,#14715,#14716,#14717,#14718,#14719,#14720,
#14721,#14722,#14723),.UNSPECIFIED.,.F.,.F.,(4,2,2,2,2,2,2,2,2,2,2,2,2,
2,2,2,2,2,2,2,2,2,2,2,2,2,2,2,2,2,2,2,2,2,2,2,2,2,2,2,2,2,2,2,2,2,2,2,2,
2,2,2,2,2,2,2,2,2,2,2,2,2,2,2,2,2,2,2,2,2,2,2,2,2,2,2,2,2,2,2,2,2,2,2,2,
2,2,2,2,2,2,2,2,2,2,2,2,2,2,2,2,2,2,2,2,2,2,2,2,2,2,2,2,2,2,2,2,2,2,2,2,
2,2,2,2,2,2,2,2,2,2,2,2,2,2,4),(-0.393164256152506,-0.393156152264836,-0.388938949432386,
-0.386265586580309,-0.383320173841496,-0.380395963431555,-0.376729005749432,
-0.371225094645901,-0.360152076233212,-0.359495928794148,-0.358457912062503,
-0.350172848148019,-0.348316579230778,-0.347232091080918,-0.346281049832906,
-0.346279673121862,-0.346278295983329,-0.346276918614931,-0.346275541127419,
-0.346274163250002,-0.346272785147417,-0.346271406528979,-0.346270027636126,
-0.346268648580951,-0.346267269146959,-0.346265889522371,-0.346264509669902,
-0.346263129235698,-0.346261748432,-0.346260367379516,-0.346258985988669,
-0.346257604455402,-0.346256222575073,-0.346254840150813,-0.346253457297103,
-0.346252074157025,-0.346250690734408,-0.34624930702275,-0.346247922935139,
-0.346246538512013,-0.34624515358407,-0.346243768164284,-0.346242382584822,
-0.345151799848308,-0.343908139441378,-0.341920247788448,-0.337956361559221,
-0.325679469518384,-0.310845004075075,-0.306934033755646,-0.304680164208461,
-0.302801175364782,-0.300978183146279,-0.298749352050761,-0.295444848040455,
-0.28956265258177,-0.276417330167695,-0.275987654395813,-0.275612833232664,
-0.274946863498535,-0.27473675522648,-0.26425374347445,-0.262358110176394,
-0.261275001979622,-0.260436280330363,-0.259409419544499,-0.257693939132142,
-0.255516662923331,-0.250898764044614,-0.24098180353912,-0.240281267024552,
-0.230388301428365,-0.226809991025846,-0.224075699166215,-0.222030371261093,
-0.218905053144269,-0.21453036929629,-0.206387136316234,-0.189252459249222,
-0.181314015113157,-0.178316431191022,-0.176070457873785,-0.173676731992705,
-0.173570406462553,-0.173456483631081,-0.17333413848094,-0.17320245484236,
-0.173060415341428,-0.173015442866163,-0.169896516950465,-0.163995443686111,
-0.15590441049969,-0.154020787739337,-0.153227388479005,-0.152166946028985,
-0.151030334603398,-0.147191849426399,-0.139235580187801,-0.131672951160756,
-0.129497194643878,-0.12793351650616,-0.126359598583563,-0.126344644150439,
-0.126329505815758,-0.126314172451892,-0.126298632774915,-0.126282875117486,
-0.126266887628018,-0.126250657965286,-0.126234173291891,-0.126217420453576,
-0.126200385837139,-0.124081559057585,-0.121493031922308,-0.116659863047585,
-0.0969684848948,-0.0894745904169614,-0.0846281110938773,-0.0808440649500737,
-0.0771927026387058,-0.0730338453367011,-0.0673537441420915,-0.0575039506960627,
-0.0470669286143805,-0.0449139771380755,-0.0437353206561605,-0.0425621832511658,
-0.0414144769472923,-0.0399527651585903,-0.0335830466459723,-0.0263176670026784,
-0.0177262246232782,-0.0144866405770614,-0.01173305256724,-0.00884924094737548,
-1.00000003500078E-6),.UNSPECIFIED.) ;
#3298=B_SPLINE_CURVE_WITH_KNOTS('',3,(#14724,#14725,#14726,#14727,#14728,
#14729,#14730,#14731,#14732,#14733,#14734,#14735,#14736,#14737,#14738,#14739,
#14740,#14741,#14742,#14743,#14744,#14745,#14746,#14747,#14748,#14749,#14750,
#14751,#14752,#14753,#14754,#14755,#14756,#14757,#14758,#14759,#14760,#14761,
#14762,#14763,#14764,#14765,#14766,#14767,#14768,#14769,#14770,#14771,#14772,
#14773,#14774,#14775,#14776,#14777,#14778,#14779,#14780,#14781,#14782,#14783,
#14784,#14785,#14786,#14787,#14788,#14789,#14790,#14791,#14792,#14793,#14794,
#14795,#14796,#14797,#14798,#14799,#14800,#14801,#14802,#14803,#14804,#14805,
#14806,#14807,#14808,#14809,#14810,#14811,#14812,#14813,#14814,#14815,#14816,
#14817,#14818,#14819,#14820,#14821,#14822,#14823,#14824,#14825,#14826,#14827,
#14828,#14829,#14830,#14831,#14832,#14833,#14834,#14835,#14836,#14837,#14838,
#14839,#14840,#14841,#14842,#14843,#14844,#14845,#14846,#14847,#14848,#14849,
#14850,#14851,#14852,#14853,#14854,#14855,#14856,#14857,#14858,#14859,#14860,
#14861,#14862,#14863,#14864,#14865,#14866,#14867,#14868,#14869,#14870,#14871,
#14872,#14873,#14874,#14875,#14876,#14877,#14878,#14879,#14880,#14881,#14882,
#14883,#14884,#14885,#14886,#14887,#14888,#14889,#14890,#14891,#14892,#14893,
#14894,#14895,#14896,#14897,#14898,#14899,#14900,#14901,#14902,#14903,#14904,
#14905,#14906,#14907,#14908,#14909,#14910,#14911,#14912,#14913,#14914,#14915,
#14916,#14917,#14918,#14919,#14920,#14921,#14922,#14923,#14924,#14925,#14926,
#14927,#14928,#14929,#14930,#14931,#14932,#14933,#14934,#14935,#14936,#14937,
#14938,#14939,#14940,#14941,#14942,#14943,#14944,#14945,#14946,#14947,#14948,
#14949,#14950,#14951,#14952,#14953,#14954,#14955,#14956,#14957,#14958,#14959,
#14960,#14961,#14962,#14963,#14964,#14965,#14966,#14967,#14968,#14969,#14970,
#14971,#14972,#14973,#14974,#14975,#14976,#14977,#14978,#14979,#14980,#14981,
#14982,#14983,#14984,#14985,#14986,#14987,#14988,#14989,#14990,#14991,#14992,
#14993,#14994,#14995,#14996,#14997,#14998,#14999,#15000,#15001,#15002,#15003,
#15004,#15005,#15006,#15007,#15008,#15009,#15010,#15011,#15012,#15013,#15014,
#15015),.UNSPECIFIED.,.F.,.F.,(4,2,2,2,2,2,2,2,2,2,2,2,2,2,2,2,2,2,2,2,
2,2,2,2,2,2,2,2,2,2,2,2,2,2,2,2,2,2,2,2,2,2,2,2,2,2,2,2,2,2,2,2,2,2,2,2,
2,2,2,2,2,2,2,2,2,2,2,2,2,2,2,2,2,2,2,2,2,2,2,2,2,2,2,2,2,2,2,2,2,2,2,2,
2,2,2,2,2,2,2,2,2,2,2,2,2,2,2,2,2,2,2,2,2,2,2,2,2,2,2,2,2,2,2,2,2,2,2,2,
2,2,2,2,2,2,2,2,2,2,2,2,2,2,2,2,2,4),(-0.786022802871508,-0.768208391277082,
-0.763296722099367,-0.757186840663637,-0.75093170811864,-0.747225332449611,
-0.743905579872729,-0.740546897014286,-0.73185450926267,-0.726296817827928,
-0.724605742925792,-0.722303472397469,-0.720646718297841,-0.718724450613038,
-0.711455389107924,-0.705359271837876,-0.702173637914158,-0.699807373883381,
-0.697387336668927,-0.694511206888103,-0.682603384706928,-0.679874821745708,
-0.676710642978271,-0.675083487318463,-0.673061951590874,-0.667330703143089,
-0.66053982472266,-0.656745501355214,-0.653484751976131,-0.650041026217191,
-0.642502460686856,-0.637046930977787,-0.634551112042692,-0.634475703136425,
-0.634422827534395,-0.634223891009373,-0.632239064452856,-0.629556314284553,
-0.620535120589472,-0.615777865121373,-0.61214503033578,-0.608261969470558,
-0.601555762042765,-0.594682091290462,-0.591844291769375,-0.591705496878947,
-0.591590627759353,-0.591494422149133,-0.591412906803809,-0.591343059299871,
-0.591282560900992,-0.591229616366297,-0.591182822316312,-0.591141070986382,
-0.591103479109329,-0.590996465223403,-0.58899879027378,-0.586182374600085,
-0.577064642147933,-0.572925971795207,-0.569140395517931,-0.56566768116009,
-0.55830252646824,-0.553871378565928,-0.551778210504473,-0.550396353791058,
-0.550323305434506,-0.550257444769354,-0.550197898458933,-0.55014391307928,
-0.550094837425834,-0.550050107588255,-0.550009234239916,-0.549971791816349,
-0.549937409460509,-0.549905763214133,-0.549876569464195,-0.549849579383786,
-0.549824574062461,-0.549801360514304,-0.549747414988473,-0.549695035134528,
-0.549644094807515,-0.54959447268028,-0.549546051397069,-0.549498717001692,
-0.549452358011198,-0.549406864822056,-0.54936212879158,-0.549318041362475,
-0.549274493079106,-0.549231372549108,-0.549188565089277,-0.549145951308499,
-0.549103405201313,-0.549060792152727,-0.549017966223606,-0.548974766892577,
-0.548931014636352,-0.548886505578638,-0.548841003937325,-0.548810962831153,
-0.548775373822835,-0.548732207959483,-0.548678123648267,-0.548606993145874,
-0.548541215849835,-0.546858935013925,-0.544928489758558,-0.539051063893007,
-0.533660931450951,-0.529338828586779,-0.526766798122483,-0.524756341531112,
-0.52283096277006,-0.520358847255927,-0.515244234843112,-0.505374289116286,
-0.502432187854402,-0.499446953973203,-0.49679495803258,-0.488455684056152,
-0.481023080017612,-0.467166537041728,-0.465270642042361,-0.462197285389915,
-0.459358861956419,-0.448994350869757,-0.44406330904248,-0.441103527746636,
-0.43868771315956,-0.436928935739463,-0.433877369930967,-0.426667677105355,
-0.418914757875739,-0.415739113566393,-0.414563685772318,-0.414553954324598,
-0.414544121933321,-0.414534185879021,-0.412512888141889,-0.407947107053795,
-0.400787576798566,-0.396835168124836,-0.393317147110158,-0.393065589708965),
 .UNSPECIFIED.) ;
#3299=B_SPLINE_CURVE_WITH_KNOTS('',3,(#15021,#15022,#15023,#15024,#15025,
#15026,#15027,#15028,#15029,#15030,#15031,#15032,#15033,#15034,#15035,#15036,
#15037,#15038,#15039,#15040,#15041,#15042,#15043,#15044,#15045,#15046,#15047,
#15048,#15049,#15050,#15051,#15052,#15053,#15054,#15055,#15056,#15057,#15058,
#15059,#15060,#15061,#15062,#15063,#15064,#15065,#15066,#15067,#15068,#15069,
#15070,#15071,#15072,#15073,#15074,#15075,#15076,#15077,#15078,#15079,#15080,
#15081,#15082,#15083,#15084),.UNSPECIFIED.,.F.,.F.,(4,3,3,3,3,3,3,3,3,3,
3,3,3,3,3,3,3,3,3,3,3,4),(3.93630690328113,4.11724533165042,4.33575257891902,
4.55311970215515,4.77079199021923,4.9201517619774,4.98858562151644,5.20574250287809,
5.42437800924309,5.64193365524723,5.85917452767311,5.90403230788466,6.07767534345593,
6.29534921278535,6.51184332341465,6.73048034262916,6.88787068095903,6.94820765270011,
7.16588235847274,7.38437758735345,7.60101478480632,7.60494227637848),
 .UNSPECIFIED.) ;
#3300=B_SPLINE_CURVE_WITH_KNOTS('',3,(#15086,#15087,#15088,#15089),
 .UNSPECIFIED.,.F.,.F.,(4,4),(0.25650513994809,0.329185416412502),
 .UNSPECIFIED.) ;
#3301=B_SPLINE_CURVE_WITH_KNOTS('',3,(#15090,#15091,#15092,#15093,#15094,
#15095,#15096,#15097,#15098,#15099,#15100,#15101,#15102,#15103,#15104,#15105,
#15106,#15107,#15108,#15109,#15110,#15111,#15112,#15113,#15114,#15115,#15116,
#15117,#15118,#15119,#15120,#15121,#15122,#15123,#15124,#15125,#15126,#15127,
#15128,#15129,#15130,#15131,#15132,#15133,#15134,#15135,#15136,#15137,#15138,
#15139,#15140,#15141,#15142,#15143,#15144,#15145,#15146,#15147,#15148,#15149,
#15150,#15151,#15152,#15153),.UNSPECIFIED.,.F.,.F.,(4,3,3,3,3,3,3,3,3,3,
3,3,3,3,3,3,3,3,3,3,3,4),(0.22510769815198,0.240322510068551,0.457482031297778,
0.674954946885662,0.984379771580828,1.11093076282781,1.38674777666684,1.54798490231427,
1.76619070002112,1.9698969082463,1.98477429053038,2.20178016056029,2.40580968662646,
2.41912725698171,2.6950269478308,2.85804930678088,2.95545595902922,3.29359733834846,
3.57495096587053,3.73048057044676,3.92985084354011,3.94168901841607),
 .UNSPECIFIED.) ;
#3302=B_SPLINE_CURVE_WITH_KNOTS('',3,(#15159,#15160,#15161,#15162,#15163,
#15164,#15165,#15166,#15167,#15168,#15169,#15170,#15171,#15172,#15173,#15174,
#15175,#15176,#15177,#15178,#15179,#15180,#15181,#15182,#15183,#15184,#15185,
#15186,#15187,#15188,#15189,#15190,#15191,#15192,#15193,#15194,#15195,#15196,
#15197,#15198,#15199,#15200,#15201,#15202,#15203,#15204,#15205,#15206,#15207,
#15208,#15209,#15210,#15211,#15212,#15213,#15214,#15215,#15216,#15217,#15218,
#15219,#15220,#15221,#15222,#15223,#15224,#15225,#15226,#15227,#15228,#15229,
#15230,#15231,#15232,#15233,#15234,#15235,#15236,#15237,#15238,#15239,#15240,
#15241,#15242,#15243,#15244,#15245,#15246,#15247,#15248,#15249,#15250,#15251,
#15252,#15253,#15254,#15255,#15256,#15257,#15258,#15259,#15260,#15261,#15262,
#15263,#15264,#15265,#15266,#15267,#15268,#15269,#15270,#15271,#15272,#15273,
#15274,#15275,#15276,#15277,#15278,#15279,#15280,#15281,#15282,#15283,#15284,
#15285,#15286,#15287,#15288,#15289,#15290,#15291,#15292,#15293,#15294,#15295,
#15296,#15297,#15298,#15299,#15300,#15301,#15302,#15303,#15304,#15305,#15306,
#15307,#15308,#15309,#15310,#15311,#15312,#15313,#15314,#15315,#15316,#15317,
#15318,#15319,#15320,#15321,#15322,#15323,#15324,#15325,#15326,#15327,#15328,
#15329,#15330,#15331,#15332,#15333,#15334,#15335,#15336,#15337,#15338,#15339,
#15340,#15341,#15342,#15343,#15344,#15345,#15346,#15347,#15348,#15349,#15350,
#15351,#15352,#15353,#15354,#15355,#15356,#15357,#15358,#15359,#15360,#15361,
#15362,#15363,#15364,#15365,#15366,#15367,#15368,#15369,#15370,#15371,#15372,
#15373,#15374,#15375,#15376,#15377,#15378,#15379,#15380,#15381,#15382,#15383,
#15384,#15385,#15386,#15387,#15388,#15389,#15390,#15391,#15392,#15393,#15394,
#15395,#15396,#15397,#15398,#15399,#15400,#15401,#15402,#15403,#15404,#15405,
#15406,#15407,#15408,#15409,#15410,#15411,#15412,#15413,#15414,#15415,#15416,
#15417,#15418,#15419,#15420,#15421,#15422,#15423,#15424,#15425,#15426,#15427,
#15428,#15429,#15430,#15431,#15432,#15433,#15434,#15435,#15436,#15437,#15438,
#15439,#15440,#15441,#15442,#15443,#15444,#15445,#15446,#15447,#15448,#15449,
#15450,#15451,#15452,#15453,#15454,#15455,#15456,#15457,#15458,#15459,#15460,
#15461,#15462,#15463,#15464,#15465,#15466,#15467,#15468,#15469,#15470,#15471,
#15472,#15473,#15474,#15475,#15476,#15477,#15478,#15479,#15480,#15481,#15482,
#15483,#15484,#15485,#15486,#15487,#15488,#15489,#15490,#15491,#15492,#15493,
#15494,#15495,#15496,#15497,#15498,#15499,#15500,#15501,#15502,#15503,#15504,
#15505,#15506,#15507,#15508,#15509,#15510,#15511,#15512,#15513,#15514,#15515,
#15516,#15517,#15518,#15519,#15520,#15521,#15522,#15523,#15524,#15525,#15526,
#15527,#15528,#15529,#15530,#15531,#15532,#15533,#15534,#15535,#15536,#15537,
#15538,#15539,#15540,#15541,#15542,#15543,#15544,#15545,#15546,#15547,#15548,
#15549,#15550,#15551,#15552,#15553,#15554,#15555,#15556,#15557,#15558,#15559,
#15560,#15561,#15562,#15563,#15564,#15565,#15566,#15567,#15568,#15569,#15570,
#15571,#15572,#15573,#15574,#15575,#15576,#15577,#15578,#15579,#15580,#15581,
#15582,#15583,#15584,#15585,#15586,#15587,#15588,#15589,#15590,#15591,#15592,
#15593,#15594,#15595,#15596,#15597,#15598,#15599,#15600,#15601,#15602,#15603,
#15604,#15605,#15606,#15607,#15608,#15609,#15610,#15611,#15612,#15613,#15614,
#15615,#15616,#15617,#15618,#15619,#15620,#15621,#15622,#15623,#15624,#15625,
#15626,#15627,#15628,#15629,#15630,#15631,#15632,#15633,#15634,#15635,#15636,
#15637,#15638,#15639,#15640,#15641,#15642,#15643,#15644,#15645,#15646,#15647,
#15648,#15649,#15650,#15651,#15652,#15653,#15654,#15655,#15656,#15657,#15658,
#15659,#15660,#15661,#15662,#15663,#15664),.UNSPECIFIED.,.F.,.F.,(4,2,2,
2,2,2,2,2,2,2,2,2,2,2,2,2,2,2,2,2,2,2,2,2,2,2,2,2,2,2,2,2,2,2,2,2,2,2,2,
2,2,2,2,2,2,2,2,2,2,2,2,2,2,2,2,2,2,2,2,2,2,2,2,2,2,2,2,2,2,2,2,2,2,2,2,
2,2,2,2,2,2,2,2,2,2,2,2,2,2,2,2,2,2,2,2,2,2,2,2,2,2,2,2,2,2,2,2,2,2,2,2,
2,2,2,2,2,2,2,2,2,2,2,2,2,2,2,2,2,2,2,2,2,2,2,2,2,2,2,2,2,2,2,2,2,2,2,2,
2,2,2,2,2,2,2,2,2,2,2,2,2,2,2,2,2,2,2,2,2,2,2,2,2,2,2,2,2,2,2,2,2,2,2,2,
2,2,2,2,2,2,2,2,2,2,2,2,2,2,2,2,2,2,2,2,2,2,2,2,2,2,2,2,2,2,2,2,2,2,2,2,
2,2,2,2,2,2,2,2,2,2,2,2,2,2,2,2,2,2,2,2,2,2,2,2,2,2,2,2,2,2,2,2,2,4),(1.00000003107423E-6,
0.00758606072509173,0.0108710041624833,0.0143247956209498,0.0208239252769082,
0.0238927515787191,0.025810946333015,0.0279968188605102,0.0322345528750677,
0.0395986954574018,0.0425303421829458,0.0444500125162114,0.0461115855658382,
0.0478838537588698,0.0500607856817371,0.0592963885234545,0.0627047199517135,
0.064622625326492,0.0648433029942763,0.0649485267661199,0.0652108824895925,
0.0664993508235049,0.0678956190543377,0.069811362557096,0.0756151563130678,
0.0786721051827159,0.080996393366047,0.0835317885474625,0.0863732180528683,
0.0869090580287054,0.0943028183611597,0.0972479917582445,0.0998375264261362,
0.103450546780153,0.105746011255335,0.109557527772641,0.111773137679787,
0.113627818652749,0.115575090925519,0.117914649082595,0.126168573624676,
0.129469211199501,0.13113763966929,0.13228382018154,0.132297312089743,0.13231060790101,
0.132323711586497,0.132336627190269,0.132349358728273,0.132361910085438,
0.132374285113824,0.132386487393706,0.132398520751075,0.132410388821155,
0.132422095081156,0.132433642971765,0.13244503604532,0.132456277667125,
0.132467371078024,0.132478319353107,0.132489125877747,0.13249979378649,
0.132510326272213,0.132520726360938,0.132530996921134,0.132541140947748,
0.1325511614019,0.13256106116734,0.132570842850748,0.132580509282205,0.13259006330926,
0.132599507761533,0.132608845029195,0.132618077622391,0.132627208339874,
0.132636239878902,0.132645174451087,0.132654014587419,0.132662762780079,
0.133613078114437,0.134551756083437,0.136110283322514,0.141852140131374,
0.148152804730228,0.150696769179636,0.152207144948827,0.153332525120183,
0.154409950910943,0.155483588439527,0.156995117321235,0.163049020974393,
0.163318457712006,0.163487701093404,0.164044551813098,0.164239980931453,
0.169149440464479,0.171578832349428,0.173224310715876,0.173251122196248,
0.173275938182836,0.173298920277962,0.173320215933595,0.173339959524006,
0.173358273909484,0.173375271145134,0.173391053637524,0.173405715092009,
0.173419341274785,0.173457076411221,0.173493888724844,0.173529818902391,
0.173564906375431,0.173599189408022,0.173632705162844,0.173665489762294,
0.173697578453696,0.173729005422107,0.173759804091931,0.173790007159945,
0.175268608390759,0.17678317453679,0.179789230807408,0.185554972527963,
0.187485508647762,0.189489597414659,0.192290189644725,0.195571422944641,
0.201512834159888,0.207699189548433,0.214772626482893,0.222893420645628,
0.231588205447433,0.239730868305575,0.247641715027393,0.250223966606402,
0.252707032278387,0.255056200826789,0.263002130010397,0.265124646036926,
0.266879034859959,0.266949731973928,0.267021738327771,0.267095384335621,
0.267171007261269,0.267248955942809,0.269253037243444,0.272675869547824,
0.280388839190857,0.283981695096317,0.28562709367168,0.286337355946282,
0.287405356306157,0.288739948714158,0.290511659225286,0.29343858183247,
0.300314970243317,0.305179804900724,0.306560366801992,0.307367316534436,
0.308143086373136,0.308147292379295,0.30815149937488,0.30815570830479,0.308159919595909,
0.308164134087966,0.308168352790471,0.308172576588967,0.308176806155979,
0.308181042011112,0.308185285035802,0.308189536275606,0.308193796370424,
0.308198065979394,0.308202345949028,0.308206637056553,0.308210940072838,
0.308215255698035,0.308219584583216,0.308223927699764,0.30822828584424,
0.308232659615481,0.308237050159465,0.308241458313446,0.308245884278854,
0.308250329065134,0.308254793672125,0.308259279029154,0.308263785619111,
0.308268314266151,0.308272865990642,0.308277441596114,0.308282041749382,
0.308286667336892,0.308291319331838,0.308295998550959,0.308300705727866,
0.30830544197662,0.308310208408059,0.308315005715939,0.308319834658204,
0.30832469627586,0.308329591497877,0.308334521189614,0.308339486557809,
0.308344488696937,0.308349528192487,0.308354606294887,0.308359724188747,
0.308364882756052,0.308370082986239,0.308375326102076,0.308380613269204,
0.308385945504728,0.309501917416463,0.310849978670979,0.313302695335476,
0.32009880250983,0.321329313609062,0.326371209895372,0.32780966818185,0.328628411435736,
0.329447103513662,0.330268560056833,0.331331652992355,0.333024686442496,
0.336492955832328,0.341319027081028,0.347789982837823,0.349234163989716,
0.350039436967057,0.350844033296672,0.351809623999787,0.353532641840576,
0.355968223308192,0.363358431133201,0.368385057144218,0.370026937325979,
0.371198454251677,0.37238817065583,0.373634585993347,0.375332328479082,
0.378325953913608,0.386222929491161,0.389566981420992,0.391526002698366,
0.393264196242751,0.395926836584615,0.399549882620271,0.404261552877088,
0.40553618279537,0.406849244156398,0.408634596324438,0.415419114930417),
 .UNSPECIFIED.) ;
#3303=B_SPLINE_CURVE_WITH_KNOTS('',3,(#15667,#15668,#15669,#15670,#15671,
#15672,#15673,#15674,#15675,#15676,#15677,#15678,#15679,#15680,#15681,#15682,
#15683,#15684,#15685,#15686,#15687,#15688,#15689,#15690,#15691,#15692,#15693,
#15694,#15695,#15696,#15697,#15698,#15699,#15700,#15701,#15702,#15703,#15704,
#15705,#15706,#15707,#15708,#15709,#15710,#15711,#15712,#15713,#15714,#15715,
#15716,#15717,#15718,#15719,#15720,#15721,#15722,#15723,#15724,#15725,#15726,
#15727,#15728,#15729,#15730,#15731,#15732,#15733,#15734,#15735,#15736,#15737,
#15738,#15739,#15740,#15741,#15742,#15743,#15744,#15745,#15746,#15747,#15748,
#15749,#15750,#15751,#15752,#15753,#15754,#15755,#15756,#15757,#15758,#15759,
#15760),.UNSPECIFIED.,.F.,.F.,(4,3,3,3,3,3,3,3,3,3,3,3,3,3,3,3,3,3,3,3,
3,3,3,3,3,3,3,3,3,3,3,4),(0.,0.134125242113495,0.352509078655641,0.571152133448733,
0.78785206804089,0.983887078909349,1.00554836450288,1.22292581387916,1.44156822673879,
1.6583768279816,1.87701872585698,1.967805066204,2.0954587923726,2.31195714336637,
2.53008391262842,2.74872480101196,2.95170543670643,2.96503359632297,3.18381638618427,
3.40163618034529,3.61938862784145,3.83802875124856,3.9356342331213,4.05498887068103,
4.27296461086581,4.49064193752331,4.70788679226362,4.91955051441669,4.92650165651424,
5.144061943285,5.36270278817282,5.47192428281431),.UNSPECIFIED.) ;
#3304=B_SPLINE_CURVE_WITH_KNOTS('',3,(#15765,#15766,#15767,#15768,#15769,
#15770,#15771,#15772,#15773,#15774,#15775,#15776,#15777,#15778,#15779,#15780,
#15781,#15782,#15783,#15784,#15785,#15786,#15787,#15788,#15789,#15790,#15791,
#15792,#15793,#15794,#15795,#15796,#15797,#15798,#15799,#15800,#15801,#15802,
#15803,#15804,#15805,#15806,#15807,#15808,#15809,#15810,#15811,#15812,#15813,
#15814,#15815,#15816,#15817,#15818,#15819,#15820,#15821,#15822,#15823,#15824,
#15825,#15826,#15827,#15828,#15829,#15830,#15831,#15832,#15833,#15834,#15835,
#15836,#15837,#15838,#15839,#15840,#15841,#15842,#15843,#15844,#15845,#15846,
#15847,#15848,#15849,#15850,#15851,#15852,#15853,#15854,#15855,#15856,#15857,
#15858,#15859,#15860,#15861,#15862,#15863,#15864,#15865,#15866,#15867,#15868,
#15869,#15870,#15871,#15872,#15873,#15874,#15875,#15876,#15877,#15878,#15879,
#15880,#15881,#15882,#15883,#15884,#15885,#15886,#15887,#15888,#15889,#15890,
#15891,#15892,#15893,#15894,#15895,#15896,#15897),.UNSPECIFIED.,.F.,.F.,
(4,3,3,3,3,3,3,3,3,3,3,3,3,3,3,3,3,3,3,3,3,3,3,3,3,3,3,3,3,3,3,3,3,3,3,
3,3,3,3,3,3,3,3,3,4),(2.23946037462874E-7,0.113928974459155,0.33050927421389,
0.549146903932351,0.766218720390714,0.98390723300321,0.984709727674719,
1.20309877951712,1.42024744924451,1.63874154934289,1.85598261279694,1.96781599695643,
2.07441147807449,2.29208458319818,2.50857722956503,2.72721269324237,2.94476761865918,
2.95171824854718,3.16337707976576,3.38061656346098,3.59828848338828,3.81625880634713,
3.93561230171815,4.03321351484648,4.25184816680328,4.4695951611072,4.68740947514502,
4.90618676612606,4.91951528184525,5.12249010119948,5.3411254552712,5.55924671538816,
5.77573958537857,5.90338904849895,5.99417411953157,6.21281048992181,6.42961360201299,
6.64825048695635,6.86562245257652,6.887282253509,7.08331326234648,7.30000775290474,
7.51864531750287,7.73702369701646,7.87114652979459),.UNSPECIFIED.) ;
#3305=B_SPLINE_CURVE_WITH_KNOTS('',3,(#15898,#15899,#15900,#15901,#15902,
#15903,#15904,#15905,#15906,#15907,#15908,#15909,#15910,#15911,#15912,#15913,
#15914,#15915,#15916,#15917,#15918,#15919,#15920,#15921,#15922,#15923,#15924,
#15925,#15926,#15927,#15928,#15929,#15930,#15931,#15932,#15933,#15934,#15935,
#15936,#15937,#15938,#15939,#15940,#15941,#15942,#15943,#15944,#15945,#15946,
#15947,#15948,#15949,#15950,#15951,#15952,#15953,#15954,#15955,#15956,#15957,
#15958,#15959,#15960,#15961,#15962,#15963,#15964,#15965,#15966,#15967,#15968,
#15969,#15970,#15971,#15972,#15973,#15974,#15975,#15976,#15977,#15978,#15979,
#15980,#15981,#15982,#15983,#15984,#15985,#15986,#15987,#15988,#15989,#15990,
#15991,#15992,#15993,#15994,#15995,#15996,#15997,#15998,#15999,#16000,#16001,
#16002,#16003,#16004,#16005,#16006,#16007,#16008,#16009,#16010,#16011,#16012,
#16013,#16014,#16015,#16016,#16017,#16018,#16019,#16020,#16021,#16022,#16023,
#16024,#16025,#16026,#16027,#16028,#16029,#16030),.UNSPECIFIED.,.F.,.F.,
(4,3,3,3,3,3,3,3,3,3,3,3,3,3,3,3,3,3,3,3,3,3,3,3,3,3,3,3,3,3,3,3,3,3,3,
3,3,3,3,3,3,3,3,3,4),(0.,0.1642451678838,0.382740226136021,0.600042062652495,
0.81815801878653,0.983838204133042,1.03554180687826,1.25343367267224,1.4720705861592,
1.68865038754616,1.90636266602205,1.96771931508277,2.12483115640474,2.34346704485423,
2.56016000368955,2.7779225847442,2.95155919736311,2.99516190669561,3.2137969189207,
3.43059850228283,3.6492332319301,3.86772566803192,3.93544715914144,4.08418625839254,
4.30244973018225,4.5209413905342,4.73957624737208,4.9192941129049,4.95595506538896,
5.17362755082564,5.39151762976199,5.61015329739374,5.82664642703676,5.90317527296924,
6.04509370180904,6.2627673956939,6.48000880082162,6.69864573210573,6.88702953663498,
6.91610786953944,7.13474521426614,7.35118372095701,7.56903886818247,7.78781927394833,
7.8709187028199),.UNSPECIFIED.) ;
#3306=B_SPLINE_CURVE_WITH_KNOTS('',3,(#16035,#16036,#16037,#16038,#16039,
#16040,#16041,#16042,#16043,#16044,#16045,#16046,#16047,#16048,#16049,#16050,
#16051,#16052,#16053,#16054,#16055,#16056,#16057,#16058,#16059,#16060,#16061,
#16062,#16063,#16064,#16065,#16066,#16067,#16068,#16069,#16070,#16071,#16072,
#16073,#16074,#16075,#16076,#16077,#16078,#16079,#16080,#16081,#16082,#16083,
#16084,#16085,#16086,#16087,#16088,#16089,#16090,#16091,#16092,#16093,#16094,
#16095,#16096,#16097,#16098,#16099,#16100,#16101,#16102,#16103,#16104,#16105,
#16106,#16107,#16108,#16109,#16110,#16111,#16112,#16113,#16114,#16115,#16116,
#16117,#16118,#16119,#16120,#16121,#16122,#16123,#16124,#16125,#16126,#16127,
#16128,#16129,#16130,#16131,#16132,#16133,#16134,#16135,#16136,#16137,#16138,
#16139,#16140,#16141,#16142,#16143,#16144,#16145,#16146,#16147,#16148,#16149,
#16150,#16151,#16152,#16153,#16154,#16155,#16156,#16157,#16158,#16159,#16160,
#16161,#16162,#16163,#16164,#16165,#16166,#16167),.UNSPECIFIED.,.F.,.F.,
(4,3,3,3,3,3,3,3,3,3,3,3,3,3,3,3,3,3,3,3,3,3,3,3,3,3,3,3,3,3,3,3,3,3,3,
3,3,3,3,3,3,3,3,3,4),(6.47843382475931E-7,0.0830984389275147,0.301878860860896,
0.519734057113125,0.736172606010294,0.954810013303583,0.983889730856414,
1.17227222785097,1.39090923664682,1.60815073803404,1.82582451472097,1.96773996380494,
2.04427188534893,2.26076510838228,2.47940086131416,2.6972910267807,2.91496358979538,
2.95162597969021,3.13134247828944,3.3499773857217,3.56846909158646,3.78673258995452,
3.93547366988932,4.00319319004644,4.22168561989418,4.44032034293354,4.65712189547432,
4.87575686542146,4.91936143024466,5.09299614077408,5.31075866271332,5.5274515595306,
5.74608737246715,5.90319990585872,5.96455578971764,6.1822680007672,6.39884773442802,
6.61748458072403,6.835376397882,6.88707997267627,7.0527601418454,7.27087606613454,
7.48817787698011,7.70667292996054,7.87091906976138),.UNSPECIFIED.) ;
#3307=B_SPLINE_CURVE_WITH_KNOTS('',3,(#16168,#16169,#16170,#16171,#16172,
#16173,#16174,#16175,#16176,#16177,#16178,#16179,#16180,#16181,#16182,#16183,
#16184,#16185,#16186,#16187,#16188,#16189,#16190,#16191,#16192,#16193,#16194,
#16195,#16196,#16197,#16198,#16199,#16200,#16201,#16202,#16203,#16204,#16205,
#16206,#16207,#16208,#16209,#16210,#16211,#16212,#16213,#16214,#16215,#16216,
#16217,#16218,#16219,#16220,#16221,#16222,#16223,#16224,#16225,#16226,#16227,
#16228,#16229,#16230,#16231,#16232,#16233,#16234,#16235,#16236,#16237,#16238,
#16239,#16240,#16241,#16242,#16243,#16244,#16245,#16246,#16247,#16248,#16249,
#16250,#16251,#16252,#16253,#16254,#16255,#16256,#16257,#16258,#16259,#16260,
#16261,#16262,#16263,#16264,#16265,#16266,#16267,#16268,#16269,#16270,#16271,
#16272,#16273,#16274,#16275,#16276,#16277,#16278,#16279,#16280,#16281,#16282,
#16283,#16284,#16285),.UNSPECIFIED.,.F.,.F.,(4,3,3,3,3,3,3,3,3,3,3,3,3,
3,3,3,3,3,3,3,3,3,3,3,3,3,3,3,3,3,3,3,3,3,3,3,3,3,3,4),(0.,0.194263872696949,
0.474398180042492,0.631922336312114,0.986336477555327,1.06871325737457,
1.35894643553535,1.50494696278201,1.94274749763261,1.97350601102964,2.37925229361138,
2.66802896959778,2.81675030786879,2.96031018031642,3.25226766112055,3.52559369118093,
3.69031672560053,3.93266213911079,3.94639008315669,4.1263712743904,4.39764408223475,
4.56330498068008,4.93283600994182,4.99936437452894,5.25968459515218,5.43653729304416,
5.64205095182849,5.65434225145359,5.87297818907955,5.91836368727623,6.09147775928523,
6.30915524874002,6.58118775056185,6.74493474743988,6.90382603695033,7.18073446312476,
7.39913360227665,7.61629290065923,7.834266390535,7.88799015781433),
 .UNSPECIFIED.) ;
#3308=B_SPLINE_CURVE_WITH_KNOTS('',3,(#16290,#16291,#16292,#16293,#16294,
#16295,#16296,#16297,#16298,#16299,#16300,#16301,#16302,#16303,#16304,#16305,
#16306,#16307,#16308,#16309,#16310,#16311,#16312,#16313,#16314,#16315,#16316,
#16317,#16318,#16319,#16320,#16321,#16322,#16323,#16324,#16325,#16326,#16327,
#16328,#16329,#16330,#16331,#16332,#16333,#16334,#16335,#16336,#16337,#16338,
#16339,#16340,#16341,#16342,#16343,#16344,#16345,#16346,#16347,#16348,#16349,
#16350,#16351,#16352,#16353,#16354,#16355,#16356,#16357,#16358,#16359,#16360,
#16361,#16362,#16363,#16364,#16365,#16366,#16367,#16368,#16369,#16370,#16371,
#16372,#16373,#16374,#16375,#16376,#16377,#16378,#16379,#16380,#16381,#16382,
#16383,#16384,#16385,#16386,#16387,#16388,#16389,#16390,#16391,#16392,#16393,
#16394,#16395,#16396,#16397,#16398,#16399,#16400,#16401,#16402,#16403,#16404,
#16405,#16406,#16407,#16408,#16409,#16410,#16411,#16412,#16413,#16414,#16415,
#16416,#16417,#16418,#16419,#16420,#16421,#16422,#16423,#16424,#16425,#16426,
#16427,#16428,#16429,#16430,#16431,#16432,#16433,#16434,#16435,#16436,#16437,
#16438,#16439,#16440,#16441,#16442,#16443,#16444,#16445,#16446,#16447,#16448,
#16449,#16450,#16451,#16452,#16453,#16454,#16455,#16456,#16457,#16458,#16459,
#16460,#16461,#16462,#16463,#16464,#16465,#16466,#16467,#16468,#16469,#16470,
#16471,#16472,#16473,#16474,#16475,#16476,#16477,#16478,#16479,#16480,#16481,
#16482,#16483,#16484,#16485,#16486,#16487,#16488,#16489,#16490,#16491,#16492,
#16493,#16494,#16495,#16496,#16497,#16498,#16499,#16500,#16501,#16502,#16503,
#16504,#16505,#16506,#16507,#16508,#16509,#16510,#16511,#16512,#16513,#16514,
#16515,#16516,#16517,#16518,#16519,#16520,#16521,#16522,#16523,#16524,#16525,
#16526,#16527,#16528,#16529,#16530,#16531,#16532,#16533,#16534,#16535,#16536,
#16537,#16538,#16539,#16540,#16541,#16542,#16543,#16544,#16545,#16546,#16547,
#16548,#16549,#16550,#16551,#16552,#16553,#16554,#16555,#16556,#16557,#16558,
#16559,#16560,#16561,#16562,#16563,#16564,#16565,#16566,#16567,#16568,#16569,
#16570,#16571,#16572,#16573,#16574,#16575,#16576,#16577,#16578,#16579,#16580,
#16581,#16582,#16583,#16584,#16585,#16586,#16587,#16588,#16589,#16590,#16591,
#16592,#16593,#16594,#16595,#16596,#16597,#16598,#16599,#16600,#16601,#16602,
#16603,#16604,#16605,#16606,#16607,#16608,#16609,#16610,#16611,#16612,#16613,
#16614,#16615,#16616,#16617,#16618,#16619,#16620,#16621,#16622,#16623,#16624,
#16625,#16626,#16627,#16628,#16629,#16630,#16631,#16632,#16633,#16634,#16635,
#16636,#16637,#16638,#16639,#16640,#16641,#16642,#16643,#16644,#16645,#16646,
#16647,#16648,#16649,#16650,#16651,#16652,#16653,#16654,#16655,#16656,#16657,
#16658,#16659,#16660,#16661,#16662,#16663,#16664,#16665,#16666,#16667,#16668,
#16669,#16670,#16671,#16672,#16673,#16674,#16675,#16676,#16677,#16678,#16679,
#16680,#16681,#16682,#16683,#16684,#16685,#16686,#16687,#16688,#16689,#16690,
#16691,#16692,#16693,#16694,#16695,#16696,#16697,#16698,#16699,#16700,#16701,
#16702,#16703,#16704,#16705,#16706,#16707,#16708,#16709,#16710,#16711,#16712,
#16713,#16714,#16715,#16716,#16717,#16718,#16719,#16720,#16721,#16722,#16723,
#16724,#16725,#16726,#16727,#16728,#16729,#16730,#16731,#16732,#16733,#16734,
#16735,#16736,#16737,#16738,#16739,#16740,#16741,#16742,#16743,#16744,#16745,
#16746,#16747,#16748,#16749,#16750,#16751,#16752,#16753,#16754,#16755,#16756,
#16757,#16758,#16759,#16760,#16761,#16762,#16763,#16764,#16765,#16766,#16767,
#16768,#16769,#16770,#16771,#16772,#16773,#16774,#16775,#16776,#16777,#16778,
#16779,#16780,#16781,#16782,#16783,#16784,#16785,#16786,#16787,#16788,#16789,
#16790,#16791,#16792,#16793,#16794,#16795,#16796,#16797,#16798,#16799,#16800,
#16801,#16802,#16803,#16804,#16805,#16806,#16807,#16808,#16809,#16810,#16811,
#16812,#16813,#16814,#16815,#16816,#16817,#16818,#16819,#16820,#16821,#16822,
#16823,#16824,#16825,#16826,#16827,#16828,#16829,#16830,#16831,#16832,#16833,
#16834,#16835,#16836,#16837,#16838,#16839,#16840,#16841,#16842,#16843,#16844,
#16845,#16846,#16847,#16848,#16849,#16850,#16851,#16852,#16853,#16854,#16855,
#16856,#16857,#16858,#16859,#16860,#16861,#16862,#16863,#16864,#16865,#16866,
#16867,#16868,#16869,#16870,#16871,#16872,#16873,#16874,#16875,#16876,#16877,
#16878,#16879,#16880,#16881,#16882,#16883,#16884,#16885,#16886,#16887,#16888,
#16889,#16890,#16891,#16892,#16893,#16894,#16895,#16896,#16897,#16898,#16899,
#16900,#16901,#16902,#16903,#16904,#16905,#16906,#16907,#16908,#16909,#16910,
#16911,#16912,#16913,#16914,#16915,#16916,#16917,#16918,#16919,#16920,#16921,
#16922,#16923,#16924,#16925,#16926,#16927,#16928,#16929,#16930,#16931,#16932,
#16933,#16934,#16935,#16936,#16937,#16938,#16939,#16940,#16941,#16942,#16943,
#16944,#16945,#16946,#16947,#16948,#16949,#16950,#16951,#16952,#16953,#16954,
#16955,#16956,#16957,#16958,#16959,#16960,#16961,#16962,#16963,#16964,#16965,
#16966,#16967,#16968,#16969,#16970,#16971,#16972,#16973,#16974,#16975,#16976,
#16977,#16978,#16979,#16980,#16981,#16982,#16983,#16984,#16985,#16986,#16987,
#16988,#16989,#16990,#16991,#16992,#16993,#16994,#16995,#16996,#16997,#16998,
#16999,#17000,#17001,#17002,#17003,#17004,#17005,#17006,#17007,#17008,#17009,
#17010,#17011,#17012,#17013,#17014,#17015,#17016,#17017,#17018,#17019,#17020,
#17021,#17022,#17023,#17024,#17025,#17026,#17027,#17028,#17029,#17030,#17031,
#17032,#17033,#17034,#17035,#17036,#17037,#17038,#17039,#17040,#17041,#17042,
#17043,#17044,#17045,#17046,#17047,#17048,#17049,#17050,#17051,#17052,#17053,
#17054,#17055,#17056,#17057,#17058,#17059,#17060,#17061,#17062,#17063,#17064,
#17065,#17066,#17067,#17068,#17069,#17070,#17071,#17072,#17073,#17074,#17075,
#17076,#17077,#17078,#17079,#17080,#17081,#17082,#17083),.UNSPECIFIED.,
 .F.,.F.,(4,2,2,2,2,2,2,2,2,2,2,2,2,2,2,2,2,2,2,2,2,2,2,2,2,2,2,2,2,2,2,
2,2,2,2,2,2,2,2,2,2,2,2,2,2,2,2,2,2,2,2,2,2,2,2,2,2,2,2,2,2,2,2,2,2,2,2,
2,2,2,2,2,2,2,2,2,2,2,2,2,2,2,2,2,2,2,2,2,2,2,2,2,2,2,2,2,2,2,2,2,2,2,2,
2,2,2,2,2,2,2,2,2,2,2,2,2,2,2,2,2,2,2,2,2,2,2,2,2,2,2,2,2,2,2,2,2,2,2,2,
2,2,2,2,2,2,2,2,2,2,2,2,2,2,2,2,2,2,2,2,2,2,2,2,2,2,2,2,2,2,2,2,2,2,2,2,
2,2,2,2,2,2,2,2,2,2,2,2,2,2,2,2,2,2,2,2,2,2,2,2,2,2,2,2,2,2,2,2,2,2,2,2,
2,2,2,2,2,2,2,2,2,2,2,2,2,2,2,2,2,2,2,2,2,2,2,2,2,2,2,2,2,2,2,2,2,2,2,2,
2,2,2,2,2,2,2,2,2,2,2,2,2,2,2,2,2,2,2,2,2,2,2,2,2,2,2,2,2,2,2,2,2,2,2,2,
2,2,2,2,2,2,2,2,2,2,2,2,2,2,2,2,2,2,2,2,2,2,2,2,2,2,2,2,2,2,2,2,2,2,2,2,
2,2,2,2,2,2,2,2,2,2,2,2,2,2,2,2,2,2,2,2,2,2,2,2,2,2,2,2,2,2,2,2,2,2,2,2,
2,2,2,2,2,2,2,2,2,2,2,2,2,2,2,2,2,2,2,2,2,2,2,2,2,2,2,2,2,2,2,2,2,2,2,2,
2,2,2,2,2,4),(1.00000004678006E-6,0.0117981715776559,0.0141765875756427,
0.0161778548407407,0.0183214071210216,0.0216752514139586,0.0301257972670827,
0.0348883544478171,0.0372044521983115,0.0396682123971428,0.0428351898584976,
0.0509548013683551,0.0540302919194078,0.0564902514800823,0.0569992489011105,
0.057287635005279,0.0596896934386391,0.0647023908037505,0.0685970451669697,
0.0703360089238731,0.0705977297608284,0.0708618611263078,0.071867870856269,
0.0720514717888028,0.0742827147117976,0.0805882325797279,0.0872943976943436,
0.091128938430779,0.0937663735205952,0.0974692052344555,0.104677080693303,
0.110711199443734,0.113344221830045,0.113646001252761,0.113916590354331,
0.114250483372622,0.116287598685056,0.117104608580213,0.124391044251081,
0.130776892737506,0.135721936028525,0.136240568959361,0.136626232832928,
0.137108340071238,0.142825704139786,0.153865841947984,0.157348106984969,
0.157506960055344,0.157710572204959,0.158010479345694,0.15850669968298,
0.158878674540749,0.159347000758451,0.161532073514973,0.1720516846647,0.186215337037974,
0.190388529976153,0.190614963879188,0.201007120766463,0.206502849534112,
0.212828239653974,0.216632075569862,0.231244010368758,0.236061569493539,
0.236281020116368,0.23645410139097,0.23659200928394,0.236702897493482,0.236792780489028,
0.236866152563208,0.237052886302177,0.237226032123925,0.23738759982428,
0.237539361728887,0.237682899697175,0.237819646663956,0.237950924855777,
0.238077982687932,0.238202032570825,0.238324292626211,0.238446036229072,
0.238568655782945,0.23869375107223,0.238823260437904,0.238959669574263,
0.239029954464892,0.239146602253067,0.239517792197664,0.242077886644829,
0.244485969598382,0.254160824240424,0.260059855551496,0.263362599291692,
0.266361995925271,0.267949647995184,0.271025158298437,0.278007528704527,
0.285633683849564,0.287605018779196,0.287613733831114,0.287622288629389,
0.287630687375141,0.287638934034966,0.287647032406389,0.287654986251203,
0.287662799264217,0.287670474845409,0.287678016451467,0.287685427327927,
0.28769271074535,0.287699869641961,0.287712045364945,0.287724131601217,
0.287736129806356,0.287748041536514,0.287759868211534,0.287771611400497,
0.28778327247071,0.287794852852654,0.287806354058216,0.28781777741181,0.287829124241842,
0.2878403959326,0.287851593861463,0.287862719306652,0.287873773675878,0.287884758248309,
0.287895674233595,0.287906522873875,0.287917305479812,0.287928023241506,
0.287938677551452,0.287949269494109,0.287959800296564,0.28797027113837,
0.287980683122077,0.287991037486362,0.288001335428267,0.288011578116628,
0.288021766660132,0.288031902186019,0.288041985818963,0.288052018663478,
0.288062001850122,0.288071936449968,0.288081823552528,0.288091664187382,
0.288101459456185,0.288111210684049,0.28812092061002,0.288130592218129,
0.288140228407355,0.288149832177158,0.28815940654576,0.288168954459302,
0.288178478887028,0.288187982703064,0.28819746885464,0.288206940299735,
0.288216443475015,0.288225985215775,0.28823556627346,0.288245187451109,
0.288254849694628,0.288264553892017,0.288274300984802,0.288284091802487,
0.288293927281936,0.288303808366235,0.288313735947895,0.288323711024387,
0.288333734690832,0.288343807933894,0.288353931706565,0.288364107083035,
0.288374335136366,0.288384617030569,0.288394953825097,0.288405346697891,
0.288415796846845,0.288426305396853,0.288436873568455,0.288447502560683,
0.288458193667055,0.288468948077633,0.288479767132306,0.288490652188274,
0.288501604697995,0.288512626015545,0.288523717528315,0.288532425454214,
0.288541351952106,0.288550504837793,0.288559892422303,0.2885695234194,0.288579406955357,
0.288589552524787,0.288599970218165,0.288610670750819,0.28862166529466,
0.288632965629541,0.288644584315021,0.28865653447984,0.288668830106218,
0.288681485909634,0.28869451761888,0.288707941849257,0.288721776254907,
0.288736039507445,0.288750751595507,0.288765933733784,0.288781608601664,
0.288797800313895,0.28881453475341,0.288831839572732,0.288849744441903,
0.288868281230161,0.288887484152688,0.288907390099895,0.288928038818334,
0.288949473235584,0.291126502648353,0.295963668354246,0.303254745760134,
0.308370978615938,0.312352732402771,0.318935052213715,0.328136385741887,
0.328169070943261,0.328199862403885,0.328228893261674,0.328256285487696,
0.328282150978216,0.32830659252777,0.328329704637812,0.32835157435535,0.328372281895868,
0.328391901306064,0.328410500993111,0.328428144189227,0.328444889484998,
0.328480976124107,0.328516301480781,0.32855089593913,0.328584788546575,
0.330847670834751,0.332832671674803,0.336802722254229,0.34519558457925,
0.349089120984497,0.352558092535757,0.353797947175991,0.357218607553165,
0.362990062524411,0.370451452940245,0.372381352886408,0.374933898929131,
0.374939788970267,0.374945669020018,0.374951539223768,0.374957399789569,
0.374963250868975,0.374969092572663,0.37497492509504,0.374980748617456,
0.374986563312461,0.374992369363712,0.374998166923447,0.375003956114768,
0.375009737085523,0.375015510117237,0.375021275344455,0.375027032882029,
0.375032782879761,0.37503852556205,0.37555694324117,0.375567269909854,0.377720868258857,
0.382365610442631,0.389375752076264,0.393379859296447,0.397296294500328,
0.401104978004888,0.406777661015277,0.407621523137426,0.410289752320065,
0.414582856926883,0.416603986028205,0.416614002572225,0.416623915413951,
0.416633726692027,0.416643438635818,0.416653053555611,0.416662573535574,
0.41667200056114,0.416681336581605,0.417485878291613,0.419087625363594,
0.421142700497735,0.42574136377725,0.436836636891112,0.439393831152882,
0.441472131292074,0.441660590835585,0.441686489525662,0.441710955310895,
0.441733714646402,0.441754835741431,0.441774391036881,0.441792456284458,
0.441809109423203,0.441824429579624,0.441838496273588,0.441851388648489,
0.441864292124513,0.441876924177411,0.4418892852421,0.441901377148708,0.441913200097161,
0.442256322994076,0.44419768240756,0.446645761483289,0.450636427945831,
0.46174540541876,0.465759700949354,0.469658104524871,0.49693467769608,0.50102995100839,
0.504817827829038,0.508390463552266,0.520691704899558,0.524782833308149,
0.526948147955865,0.528135983758028,0.528194582201978,0.528236735318638,
0.528272546690989,0.528302637777417,0.52832766942319,0.528348305856086,
0.528365185038294,0.528386703464043,0.528407214203401,0.528426731725113,
0.52844527322612,0.528462858526146,0.530200604517233,0.53232457793843,0.535618772997076,
0.542794734749739,0.549350793127886,0.553775944069864,0.558191678735382,
0.564327245393766,0.579709110085063,0.581430465521649,0.584689685628003,
0.588301379998283,0.593186366960729,0.606838048654737,0.611786897883082,
0.61365258879985,0.615185280153268,0.616555647458888,0.618102750025953,
0.620251819405073,0.623997558833745,0.633926477995027,0.642866787177593,
0.648363892796145,0.654054532993876,0.66300241029919,0.671853890072724,
0.681717989235355,0.69435239117764,0.697366964678845,0.699144929545757,
0.700941910234864,0.702848675596833,0.705486500230046,0.71031582254622,
0.720212043330027,0.722204552175948,0.723328187639032,0.724052318599337,
0.725114703915184,0.728173669291402,0.737248207422731,0.744046114323223,
0.746546722674751,0.748393098439738,0.750149368261651,0.75220221465179,
0.755246063676816,0.768062546023172,0.778797336791404,0.786297940368581),
 .UNSPECIFIED.) ;
#3309=B_SPLINE_CURVE_WITH_KNOTS('',3,(#17084,#17085,#17086,#17087,#17088,
#17089,#17090,#17091,#17092,#17093,#17094,#17095,#17096,#17097,#17098,#17099,
#17100,#17101,#17102,#17103,#17104,#17105,#17106,#17107,#17108,#17109,#17110,
#17111,#17112,#17113,#17114,#17115,#17116,#17117,#17118,#17119,#17120,#17121,
#17122,#17123,#17124,#17125,#17126,#17127,#17128,#17129,#17130,#17131,#17132,
#17133,#17134,#17135,#17136,#17137,#17138,#17139,#17140,#17141,#17142,#17143,
#17144,#17145,#17146,#17147,#17148,#17149,#17150,#17151,#17152,#17153,#17154,
#17155,#17156,#17157,#17158,#17159,#17160,#17161,#17162,#17163,#17164,#17165,
#17166,#17167,#17168,#17169,#17170,#17171,#17172,#17173,#17174,#17175,#17176,
#17177,#17178,#17179,#17180,#17181,#17182,#17183,#17184,#17185,#17186,#17187,
#17188,#17189,#17190,#17191,#17192,#17193,#17194,#17195,#17196,#17197,#17198,
#17199,#17200,#17201,#17202,#17203,#17204,#17205,#17206,#17207,#17208,#17209,
#17210,#17211,#17212,#17213,#17214,#17215,#17216,#17217,#17218,#17219,#17220,
#17221,#17222,#17223,#17224,#17225,#17226,#17227,#17228,#17229,#17230,#17231,
#17232,#17233,#17234,#17235,#17236,#17237,#17238,#17239,#17240,#17241,#17242,
#17243,#17244,#17245,#17246,#17247,#17248,#17249,#17250,#17251,#17252,#17253,
#17254,#17255,#17256,#17257,#17258,#17259,#17260,#17261,#17262,#17263,#17264,
#17265,#17266,#17267,#17268,#17269,#17270,#17271,#17272,#17273,#17274,#17275,
#17276,#17277,#17278,#17279,#17280,#17281,#17282,#17283,#17284,#17285,#17286,
#17287,#17288,#17289,#17290,#17291,#17292,#17293,#17294,#17295,#17296,#17297,
#17298,#17299,#17300,#17301,#17302,#17303,#17304,#17305,#17306,#17307,#17308,
#17309,#17310,#17311,#17312,#17313,#17314,#17315,#17316,#17317,#17318,#17319,
#17320,#17321,#17322,#17323,#17324,#17325,#17326,#17327,#17328,#17329,#17330,
#17331,#17332,#17333,#17334,#17335,#17336,#17337,#17338,#17339,#17340,#17341,
#17342,#17343,#17344,#17345,#17346,#17347,#17348,#17349,#17350,#17351,#17352,
#17353,#17354,#17355,#17356,#17357,#17358,#17359,#17360,#17361,#17362,#17363,
#17364,#17365,#17366,#17367,#17368,#17369,#17370,#17371,#17372,#17373,#17374,
#17375,#17376,#17377,#17378,#17379,#17380,#17381,#17382,#17383,#17384,#17385,
#17386,#17387,#17388,#17389,#17390,#17391,#17392,#17393,#17394,#17395,#17396,
#17397,#17398,#17399,#17400,#17401,#17402,#17403,#17404,#17405,#17406,#17407,
#17408,#17409,#17410,#17411,#17412,#17413,#17414,#17415,#17416,#17417,#17418,
#17419,#17420,#17421,#17422,#17423,#17424,#17425,#17426,#17427,#17428,#17429,
#17430,#17431,#17432,#17433,#17434,#17435,#17436,#17437,#17438,#17439,#17440,
#17441,#17442,#17443,#17444,#17445,#17446,#17447,#17448,#17449,#17450,#17451,
#17452,#17453,#17454,#17455,#17456,#17457,#17458,#17459,#17460,#17461,#17462,
#17463,#17464,#17465,#17466,#17467,#17468,#17469,#17470,#17471,#17472,#17473,
#17474,#17475,#17476,#17477,#17478,#17479,#17480,#17481,#17482,#17483,#17484,
#17485,#17486,#17487,#17488,#17489,#17490,#17491,#17492,#17493,#17494,#17495,
#17496,#17497,#17498,#17499,#17500,#17501,#17502,#17503,#17504,#17505,#17506,
#17507,#17508,#17509,#17510,#17511,#17512,#17513,#17514,#17515,#17516,#17517,
#17518,#17519,#17520,#17521,#17522,#17523,#17524,#17525,#17526,#17527,#17528,
#17529,#17530,#17531,#17532,#17533,#17534,#17535,#17536,#17537,#17538,#17539,
#17540,#17541,#17542,#17543,#17544,#17545,#17546,#17547,#17548,#17549,#17550,
#17551,#17552,#17553,#17554,#17555,#17556,#17557,#17558,#17559,#17560,#17561,
#17562,#17563,#17564,#17565,#17566,#17567,#17568,#17569,#17570,#17571,#17572,
#17573,#17574,#17575,#17576,#17577,#17578,#17579,#17580,#17581,#17582,#17583,
#17584,#17585,#17586,#17587,#17588,#17589,#17590,#17591,#17592,#17593,#17594,
#17595,#17596,#17597,#17598,#17599,#17600,#17601,#17602,#17603,#17604,#17605,
#17606,#17607,#17608,#17609,#17610,#17611,#17612,#17613,#17614,#17615,#17616,
#17617,#17618,#17619,#17620,#17621,#17622,#17623,#17624,#17625,#17626,#17627,
#17628,#17629,#17630,#17631,#17632,#17633,#17634,#17635,#17636,#17637,#17638,
#17639,#17640,#17641,#17642,#17643,#17644,#17645,#17646,#17647,#17648,#17649,
#17650,#17651,#17652,#17653,#17654,#17655,#17656,#17657,#17658,#17659,#17660,
#17661,#17662,#17663,#17664,#17665,#17666,#17667,#17668,#17669,#17670,#17671,
#17672,#17673,#17674,#17675,#17676,#17677,#17678,#17679,#17680,#17681,#17682,
#17683,#17684,#17685,#17686,#17687,#17688,#17689,#17690,#17691,#17692,#17693,
#17694,#17695,#17696,#17697,#17698,#17699,#17700,#17701,#17702,#17703,#17704,
#17705,#17706,#17707,#17708,#17709,#17710,#17711,#17712,#17713,#17714,#17715,
#17716,#17717,#17718,#17719,#17720,#17721,#17722,#17723,#17724,#17725,#17726,
#17727,#17728,#17729,#17730,#17731,#17732,#17733,#17734,#17735,#17736,#17737,
#17738,#17739,#17740,#17741,#17742,#17743,#17744,#17745,#17746,#17747,#17748,
#17749,#17750,#17751,#17752,#17753,#17754,#17755,#17756,#17757,#17758,#17759,
#17760,#17761,#17762,#17763,#17764,#17765,#17766,#17767,#17768,#17769,#17770,
#17771,#17772,#17773,#17774,#17775,#17776,#17777,#17778,#17779,#17780,#17781,
#17782,#17783,#17784,#17785,#17786,#17787,#17788,#17789,#17790,#17791,#17792,
#17793,#17794,#17795,#17796,#17797,#17798,#17799,#17800,#17801,#17802,#17803,
#17804,#17805,#17806,#17807,#17808,#17809,#17810,#17811,#17812,#17813,#17814,
#17815,#17816,#17817,#17818,#17819,#17820,#17821,#17822,#17823,#17824,#17825,
#17826,#17827,#17828,#17829,#17830,#17831,#17832,#17833,#17834,#17835,#17836,
#17837,#17838,#17839,#17840,#17841,#17842,#17843,#17844,#17845,#17846,#17847,
#17848,#17849,#17850,#17851,#17852,#17853,#17854,#17855,#17856,#17857,#17858,
#17859,#17860,#17861,#17862,#17863,#17864,#17865,#17866,#17867,#17868,#17869,
#17870,#17871,#17872,#17873,#17874,#17875,#17876,#17877,#17878,#17879,#17880,
#17881,#17882,#17883,#17884,#17885,#17886,#17887,#17888,#17889,#17890,#17891,
#17892,#17893,#17894,#17895,#17896,#17897,#17898,#17899,#17900,#17901,#17902,
#17903,#17904,#17905,#17906,#17907),.UNSPECIFIED.,.F.,.F.,(4,2,2,2,2,2,
2,2,2,2,2,2,2,2,2,2,2,2,2,2,2,2,2,2,2,2,2,2,2,2,2,2,2,2,2,2,2,2,2,2,2,2,
2,2,2,2,2,2,2,2,2,2,2,2,2,2,2,2,2,2,2,2,2,2,2,2,2,2,2,2,2,2,2,2,2,2,2,2,
2,2,2,2,2,2,2,2,2,2,2,2,2,2,2,2,2,2,2,2,2,2,2,2,2,2,2,2,2,2,2,2,2,2,2,2,
2,2,2,2,2,2,2,2,2,2,2,2,2,2,2,2,2,2,2,2,2,2,2,2,2,2,2,2,2,2,2,2,2,2,2,2,
2,2,2,2,2,2,2,2,2,2,2,2,2,2,2,2,2,2,2,2,2,2,2,2,2,2,2,2,2,2,2,2,2,2,2,2,
2,2,2,2,2,2,2,2,2,2,2,2,2,2,2,2,2,2,2,2,2,2,2,2,2,2,2,2,2,2,2,2,2,2,2,2,
2,2,2,2,2,2,2,2,2,2,2,2,2,2,2,2,2,2,2,2,2,2,2,2,2,2,2,2,2,2,2,2,2,2,2,2,
2,2,2,2,2,2,2,2,2,2,2,2,2,2,2,2,2,2,2,2,2,2,2,2,2,2,2,2,2,2,2,2,2,2,2,2,
2,2,2,2,2,2,2,2,2,2,2,2,2,2,2,2,2,2,2,2,2,2,2,2,2,2,2,2,2,2,2,2,2,2,2,2,
2,2,2,2,2,2,2,2,2,2,2,2,2,2,2,2,2,2,2,2,2,2,2,2,2,2,2,2,2,2,2,2,2,2,2,2,
2,2,2,2,2,2,2,2,2,2,2,2,2,2,2,2,2,2,2,2,2,2,2,2,2,2,2,2,2,2,2,2,2,2,2,2,
2,2,2,2,2,2,2,2,2,4),(1.00000001482342E-6,0.00387989849434221,0.00965386819778096,
0.0176277349044153,0.0198228806392684,0.0215745100882533,0.0234954630887238,
0.0326569349317571,0.0381640880605481,0.0412771457430435,0.0437174423764869,
0.0460848193585393,0.0492269609407735,0.0597163419065942,0.0643745621454506,
0.0675782334901951,0.0706959462422394,0.0779496778758638,0.0854439807223627,
0.0967604007439808,0.1017462689883,0.104731705765129,0.107252769730566,
0.11050523777754,0.119128871523756,0.124155399590182,0.126948898947171,
0.129018506668542,0.13105495250947,0.133405969259583,0.137725506561563,
0.148374618351109,0.151398280693758,0.153022907801174,0.154584281070802,
0.156423523520727,0.159912810261316,0.168481393143192,0.172565032640693,
0.175979545017129,0.179474515418626,0.189923792638977,0.193606348045477,
0.195687984992599,0.197706494688502,0.201164926123051,0.210217465380377,
0.214516682735599,0.218161996317371,0.221575844802789,0.232859886545185,
0.236588502397511,0.237112183316485,0.237411445158013,0.237578601813748,
0.237812638940346,0.239669627823577,0.241846153267194,0.247729815668176,
0.254523650730061,0.258167238498117,0.261688169648363,0.265918859928784,
0.276015561687705,0.27919245215231,0.281131484656794,0.282764054070061,
0.28459325304176,0.29344444708349,0.29879950755727,0.301799582589062,0.304123994276168,
0.306331369678783,0.309271856388809,0.320388661309048,0.324406343497094,
0.326367042094413,0.327914004120641,0.329700603105548,0.332765620440067,
0.335628650198325,0.337586531364092,0.344251170297893,0.348039110161335,
0.351365114431158,0.35489880382105,0.367359725472494,0.371399937256882,
0.380412495938149,0.393134782655627,0.403099644508735,0.40508617683676,
0.407722466949874,0.411122928841098,0.413016861815729,0.417678939999058,
0.432169368736004,0.43460346715269,0.435986161393044,0.437055341926396,
0.438233032937166,0.440330685773129,0.44298732252709,0.448720658143859,
0.466783984856216,0.471891219704659,0.475893582739653,0.479540483978466,
0.483861659422546,0.489514996798002,0.497347682092197,0.50903104119785,
0.51682119557004,0.519348403601593,0.520899994807651,0.522427103623144,
0.522431787674928,0.52243647891577,0.522441177308973,0.522445883339716,
0.522450597559427,0.522455319884319,0.522460050461944,0.522464789274641,
0.522469536791856,0.522474293569499,0.522479059583391,0.522483834861456,
0.522488620124326,0.522493415196993,0.522498220428804,0.522503036158753,
0.522507862278447,0.522512699215363,0.522517547179921,0.522522406468298,
0.522527277271925,0.522532160166779,0.52253705511781,0.522541962203414,
0.52254688191372,0.522551814514536,0.522556759960928,0.522561718587701,
0.522566690784472,0.522571676669936,0.52257667669236,0.52258169111907,0.522586720088111,
0.52259176374344,0.52259682253021,0.52260189634087,0.522606985649322,0.522612090817191,
0.522617212052831,0.522622349747412,0.522627504114795,0.522632675210603,
0.522637863360016,0.522643068897424,0.522648292262694,0.522653533546729,
0.522658793019039,0.522664071057127,0.522669367992304,0.522674683784087,
0.522680018881375,0.522685373651308,0.522690748552824,0.522696143694737,
0.52270155933062,0.522706995583814,0.522712453088174,0.522717932181592,
0.522723432857887,0.522728955413582,0.522734500378407,0.522740068108535,
0.52274565865659,0.522751272301079,0.522756909715616,0.522762570965939,
0.52276825654844,0.522773966889108,0.522779702246598,0.522785462863514,
0.522791249089045,0.52279706110555,0.522802899318917,0.522808764336661,
0.522814656363363,0.522820575614543,0.522826522575855,0.5228324974654,0.522838500862241,
0.52284453302179,0.522850594541565,0.522856685652069,0.522862806491349,
0.522868957545056,0.522875139471389,0.522881352428205,0.52288759698738,
0.522893873361063,0.522900181887687,0.522906523096759,0.522912897641791,
0.522919305649913,0.522925747550841,0.522932223934683,0.522938735130323,
0.522945281471344,0.522951863499161,0.522958481746644,0.522965136549655,
0.522971828363516,0.522978557605635,0.522985324817749,0.522992130433628,
0.522998974720019,0.523005858407542,0.523012782263043,0.523019746339463,
0.523026751225562,0.523033797426523,0.52304088550161,0.523048016135177,
0.523055189612988,0.523062406526519,0.523069667487326,0.523076972971153,
0.523084323472904,0.523091719682342,0.523099162013879,0.523106651015868,
0.523114187409881,0.523121771672841,0.523129404352956,0.523137086141206,
0.523144817633374,0.523152599363097,0.523160432004689,0.523168316071842,
0.523176252241407,0.523184241238915,0.523192283561949,0.523200380014055,
0.523208531216622,0.523216737875416,0.523225000632802,0.52323332020029,
0.523241697237135,0.523250132351368,0.523258626267659,0.523267179883397,
0.523275793851081,0.523284468965726,0.523293205898434,0.523302005342351,
0.523310868144507,0.523319795135524,0.523328787112698,0.523337844609226,
0.525978329323283,0.52959315606768,0.539115577091703,0.543835608239035,
0.545295680478062,0.545809802699583,0.546175058277946,0.547035020420134,
0.5483658270704,0.552881944968185,0.5629338284468,0.567349268951828,0.569636419430082,
0.571432686149489,0.571460440690088,0.571488096926663,0.571515667013946,
0.571543162713895,0.571570595505927,0.57159797647101,0.571625316334739,
0.57165262571796,0.571679914952057,0.571707194185741,0.571734473230971,
0.571761761761505,0.571789069348269,0.571816405330517,0.571843778985032,
0.571871199411981,0.571898675640363,0.571926216664993,0.571953831241164,
0.571981528180434,0.572009316259056,0.572037204205928,0.572065200618897,
0.57209331418374,0.572121553515515,0.572149927236589,0.572178443919876,
0.57220711230649,0.572235941083895,0.57226493891177,0.572294114588136,0.572323476896052,
0.572353034710167,0.572382797035703,0.572412772774587,0.572426819780976,
0.572441086189964,0.57245558087268,0.572470312916514,0.572485292018211,
0.572500528125015,0.572516031533396,0.572531813070026,0.572547883881441,
0.572564255805886,0.57258094096377,0.572597952081772,0.572615302426087,
0.572633005952118,0.57265107696426,0.57266953071676,0.57268838302498,0.572707650473353,
0.572727350232543,0.572747500466581,0.572768120205924,0.572789229388394,
0.572810848881148,0.572833000584883,0.572855707402202,0.572878993504638,
0.572902884225224,0.572927406145922,0.572952587234879,0.572978456979052,
0.573005046218774,0.5730323875944,0.573060515399895,0.573089465738324,0.573119276593467,
0.573149988169945,0.573181642778997,0.573214284998644,0.573247961904776,
0.57328272327948,0.573318621533535,0.573355712098979,0.57339405364296,0.573433708146859,
0.573474741030373,0.573517221578279,0.57356122312896,0.573606823301819,
0.573654104213617,0.573703152837347,0.573754061329939,0.573806927315289,
0.573861854260396,0.57391895190319,0.57397833652038,0.574040131475568,0.574104467637211,
0.57417148389872,0.577309791806326,0.583080868621443,0.605652753316221,
0.612431293337457,0.615878906316043,0.618876085243178,0.622649759553554,
0.631024122802069,0.643566397937766,0.65091863530742,0.652711902868909,
0.653761218994568,0.654673164993293,0.655825679584042,0.658039015136198,
0.665059029463612,0.685081295501266,0.691942522026095,0.694517354357912,
0.69636003364943,0.698151941485855,0.700025555889807,0.702422402367053,
0.706124226071868,0.713014604662016,0.722224740795031,0.725099045298787,
0.736565942202035,0.738505519027787,0.739619753857818,0.740483629436549,
0.741391023405732,0.742497960887426,0.745906515753753,0.748912421752995,
0.759518825586065,0.766546640638556,0.773314070429204,0.776970573531812,
0.780124271143675,0.783011593288301,0.786304990770929),.UNSPECIFIED.) ;
#3310=B_SPLINE_CURVE_WITH_KNOTS('',3,(#17913,#17914,#17915,#17916,#17917,
#17918,#17919,#17920,#17921,#17922,#17923,#17924,#17925,#17926,#17927,#17928,
#17929,#17930,#17931,#17932,#17933,#17934,#17935,#17936,#17937,#17938,#17939,
#17940,#17941,#17942,#17943,#17944,#17945,#17946,#17947,#17948,#17949,#17950,
#17951,#17952,#17953,#17954,#17955,#17956,#17957,#17958,#17959,#17960,#17961,
#17962,#17963,#17964,#17965,#17966,#17967,#17968,#17969,#17970,#17971,#17972,
#17973,#17974,#17975,#17976,#17977,#17978,#17979,#17980,#17981,#17982,#17983,
#17984,#17985,#17986,#17987,#17988,#17989,#17990,#17991,#17992,#17993,#17994,
#17995,#17996,#17997,#17998,#17999,#18000,#18001,#18002,#18003,#18004,#18005,
#18006,#18007,#18008,#18009,#18010,#18011,#18012,#18013,#18014,#18015,#18016,
#18017,#18018,#18019,#18020,#18021,#18022,#18023,#18024,#18025,#18026,#18027,
#18028,#18029,#18030,#18031,#18032,#18033,#18034,#18035,#18036,#18037,#18038,
#18039,#18040,#18041,#18042,#18043,#18044,#18045,#18046,#18047,#18048,#18049,
#18050,#18051,#18052,#18053,#18054,#18055,#18056,#18057,#18058,#18059,#18060,
#18061,#18062,#18063,#18064,#18065,#18066,#18067,#18068,#18069,#18070,#18071,
#18072,#18073,#18074,#18075,#18076,#18077,#18078,#18079,#18080,#18081,#18082,
#18083,#18084,#18085,#18086,#18087,#18088,#18089,#18090,#18091,#18092,#18093,
#18094,#18095,#18096,#18097,#18098,#18099,#18100,#18101,#18102,#18103,#18104,
#18105,#18106,#18107,#18108,#18109,#18110,#18111,#18112,#18113,#18114,#18115,
#18116,#18117,#18118,#18119,#18120,#18121,#18122,#18123,#18124,#18125,#18126,
#18127,#18128,#18129,#18130,#18131,#18132,#18133,#18134,#18135,#18136,#18137,
#18138,#18139,#18140,#18141,#18142,#18143,#18144,#18145,#18146,#18147,#18148,
#18149,#18150,#18151,#18152,#18153,#18154,#18155,#18156,#18157,#18158,#18159,
#18160,#18161,#18162,#18163,#18164,#18165,#18166,#18167,#18168,#18169,#18170,
#18171,#18172,#18173,#18174,#18175,#18176,#18177,#18178,#18179,#18180,#18181,
#18182,#18183,#18184),.UNSPECIFIED.,.F.,.F.,(4,2,2,2,2,2,2,2,2,2,2,2,2,
2,2,2,2,2,2,2,2,2,2,2,2,2,2,2,2,2,2,2,2,2,2,2,2,2,2,2,2,2,2,2,2,2,2,2,2,
2,2,2,2,2,2,2,2,2,2,2,2,2,2,2,2,2,2,2,2,2,2,2,2,2,2,2,2,2,2,2,2,2,2,2,2,
2,2,2,2,2,2,2,2,2,2,2,2,2,2,2,2,2,2,2,2,2,2,2,2,2,2,2,2,2,2,2,2,2,2,2,2,
2,2,2,2,2,2,2,2,2,2,2,2,2,2,4),(1.00045753387877E-6,0.00842574258640645,
0.00972187540196538,0.0107115335657187,0.0116939906523298,0.0128170038292646,
0.0147243601837294,0.0215802725329028,0.0218748824183406,0.0269639747780574,
0.0291600262320035,0.0309012301160614,0.0309974238262923,0.0319926874072608,
0.0329785506518943,0.034294784905869,0.0372283069439382,0.038495401808696,
0.0441001690701221,0.0470165251449591,0.0497371711014842,0.0514932927041807,
0.0524315775376868,0.0534223086733845,0.0620991752675434,0.0650098235845182,
0.0652392200391438,0.0655582062101748,0.0676666166423386,0.0725489952146196,
0.0792874801163711,0.082412773806087,0.0850633816542351,0.0921119307833907,
0.0951721742366237,0.0969128579231273,0.0969476794878039,0.0969817376180178,
0.0970150806129788,0.0970477543459423,0.0970798024757228,0.0971112666319582,
0.0971421865730741,0.0971726002560678,0.0972025441603608,0.0972320533420131,
0.0986070463085602,0.0998164535194011,0.101545167401429,0.104608187854877,
0.111301015631071,0.11464694352377,0.117315886137275,0.118995585269948,
0.119617034933218,0.119948992792079,0.122025190823821,0.129033278289205,
0.132916033136038,0.135637083878071,0.135730605089018,0.135825237093655,
0.135921367094742,0.136019410332923,0.138398653533622,0.141309989037906,
0.148182546878764,0.151303116506634,0.15307225252019,0.157548254583598,
0.161220813611117,0.161356628742213,0.161482682807114,0.161600697766164,
0.161712100649152,0.161818095844787,0.161919719087912,0.16201787898814,
0.162113389929729,0.162206999116378,0.162299409747552,0.162391301834548,
0.162483352012097,0.162576253731141,0.164998922977395,0.165350175185979,
0.165513711754882,0.166873479807214,0.17275334136621,0.179112615094698,
0.183240259013787,0.194097109397645,0.195675735372543,0.200127934149792,
0.208329337367673,0.209725031547082,0.21258176570396,0.212716443836338,
0.215791274067457,0.218730443793863,0.226421270971432,0.228229406166425,
0.229464330404538,0.230921769963285,0.232826206626257,0.235360160744058,
0.241566937320219,0.246786042138185,0.249039996753663,0.250651677162911,
0.252552014854883,0.252615301035394,0.252681953760395,0.252752366350411,
0.252826979118717,0.252906286511062,0.255250205896054,0.259565120371384,
0.267809753877705,0.270257819100499,0.272207478810114,0.274503758004808,
0.277516463423376,0.283377219011778,0.286962777096555,0.295636502516541,
0.327358048750501,0.338653043172959,0.344423924466601,0.34720348970197,
0.353062618927892,0.357882761955244,0.360027136520687,0.361867165314252,
0.363867606408137,0.366518801123044),.UNSPECIFIED.) ;
#3311=B_SPLINE_CURVE_WITH_KNOTS('',3,(#18186,#18187,#18188,#18189),
 .UNSPECIFIED.,.F.,.F.,(4,4),(1.57753970984684,1.64973532704643),
 .UNSPECIFIED.) ;
#3312=B_SPLINE_CURVE_WITH_KNOTS('',3,(#18190,#18191,#18192,#18193,#18194,
#18195,#18196,#18197,#18198,#18199,#18200,#18201,#18202,#18203,#18204,#18205,
#18206,#18207,#18208,#18209,#18210,#18211,#18212,#18213,#18214,#18215,#18216,
#18217,#18218,#18219,#18220,#18221,#18222,#18223,#18224,#18225,#18226,#18227,
#18228,#18229,#18230,#18231,#18232,#18233,#18234,#18235,#18236,#18237,#18238,
#18239,#18240,#18241,#18242,#18243,#18244,#18245,#18246,#18247,#18248,#18249,
#18250,#18251,#18252,#18253,#18254,#18255,#18256,#18257,#18258,#18259,#18260,
#18261,#18262,#18263,#18264,#18265,#18266,#18267,#18268,#18269,#18270,#18271,
#18272,#18273,#18274,#18275,#18276,#18277,#18278,#18279,#18280,#18281,#18282,
#18283,#18284,#18285,#18286,#18287,#18288,#18289,#18290,#18291,#18292,#18293,
#18294,#18295,#18296,#18297,#18298,#18299,#18300,#18301,#18302,#18303,#18304,
#18305,#18306,#18307,#18308,#18309,#18310,#18311,#18312,#18313,#18314,#18315,
#18316,#18317,#18318,#18319,#18320,#18321,#18322,#18323,#18324,#18325,#18326,
#18327,#18328,#18329,#18330,#18331,#18332,#18333,#18334,#18335,#18336,#18337,
#18338,#18339,#18340,#18341,#18342,#18343,#18344,#18345,#18346,#18347,#18348,
#18349,#18350,#18351,#18352,#18353,#18354,#18355,#18356,#18357,#18358,#18359,
#18360,#18361,#18362,#18363,#18364,#18365,#18366,#18367,#18368,#18369,#18370,
#18371,#18372,#18373,#18374,#18375,#18376,#18377,#18378,#18379,#18380,#18381,
#18382,#18383,#18384,#18385,#18386,#18387,#18388,#18389,#18390,#18391,#18392,
#18393,#18394,#18395,#18396,#18397,#18398,#18399,#18400,#18401,#18402,#18403,
#18404,#18405,#18406,#18407,#18408,#18409,#18410,#18411,#18412,#18413,#18414,
#18415,#18416,#18417,#18418,#18419,#18420,#18421,#18422,#18423,#18424,#18425,
#18426,#18427,#18428,#18429,#18430,#18431,#18432,#18433,#18434,#18435),
 .UNSPECIFIED.,.F.,.F.,(4,2,2,2,2,2,2,2,2,2,2,2,2,2,2,2,2,2,2,2,2,2,2,2,
2,2,2,2,2,2,2,2,2,2,2,2,2,2,2,2,2,2,2,2,2,2,2,2,2,2,2,2,2,2,2,2,2,2,2,2,
2,2,2,2,2,2,2,2,2,2,2,2,2,2,2,2,2,2,2,2,2,2,2,2,2,2,2,2,2,2,2,2,2,2,2,2,
2,2,2,2,2,2,2,2,2,2,2,2,2,2,2,2,2,2,2,2,2,2,2,2,2,2,4),(1.00000001215618E-6,
0.00318509854600134,0.0129825347919774,0.0161655928261109,0.0181412012449489,
0.0198749291596257,0.0217270011136096,0.027707503078466,0.0396795572268528,
0.0419643725085689,0.0439360536928425,0.0460388807219774,0.0485916927504747,
0.0564492253007152,0.0645252079856154,0.0726409997678784,0.0841201028158781,
0.0914142858167252,0.0972082175898708,0.102273990648958,0.11246729967127,
0.119786567755532,0.122835110716931,0.12464124579374,0.125528329059267,
0.125562447011711,0.125595423621323,0.125627296775938,0.125658103323062,
0.125687879117623,0.125716658934808,0.125744476687226,0.125771365263028,
0.125797356637172,0.125822481953175,0.125846771389411,0.125870254353946,
0.125892959249474,0.125914913765058,0.125936144796729,0.125956678238446,
0.125976539390029,0.125995752768358,0.12601434203994,0.127279720261118,
0.128529548359017,0.130252307020754,0.135073159299629,0.13562333022193,
0.147756262536827,0.150769938843763,0.152296404982632,0.153444191401216,
0.154524046101334,0.155740524253793,0.157326395380975,0.164922423718007,
0.171721896110145,0.173399919221211,0.175450903838611,0.181038689856756,
0.185234452374922,0.185944160403659,0.187391980760904,0.190317421502036,
0.193934746168347,0.198342189104919,0.203544452516594,0.205689344812316,
0.20587443456203,0.207753117213519,0.207766443193314,0.207779613291745,
0.207792636216129,0.207805520255973,0.20781827348019,0.207830903622127,
0.210936143326028,0.215230566120306,0.225185429159629,0.231109341320472,
0.235206707196223,0.237029262167199,0.248215449135854,0.255908396838854,
0.259423652157063,0.262992881970404,0.263559828116157,0.265002078884858,
0.270395037063474,0.278966392081394,0.27937082880019,0.279812755485324,
0.280328522021279,0.281237571128015,0.283215844598803,0.285602684967694,
0.291240687814322,0.298563836950327,0.301598944092377,0.304073300045832,
0.30475905916055,0.305444187575203,0.306030104505483,0.312713720904449,
0.317760280930702,0.323566375723472,0.32540416659242,0.326816560433781,
0.329048274516511,0.33418691579389,0.339295415530195,0.341572983271978,
0.343355722688849,0.346097461408071,0.347784540996557,0.353350479362486,
0.357419122602839,0.359260829175887,0.360777612445794,0.362205588068618,
0.363994474172703,0.370434870678895),.UNSPECIFIED.) ;
#3313=B_SPLINE_CURVE_WITH_KNOTS('',3,(#18443,#18444,#18445,#18446,#18447,
#18448,#18449,#18450,#18451,#18452,#18453,#18454,#18455,#18456,#18457,#18458),
 .UNSPECIFIED.,.T.,.F.,(4,1,1,1,1,1,1,1,1,1,1,1,1,4),(0.,0.520304865070705,
0.709542561390409,0.804161409708611,0.898780258026813,1.15893269056541,
1.419085123104,1.67923755563226,1.93938998816052,2.03400883639567,2.12862768463082,
2.31786538114359,2.57801781366682,2.83817024619004),.UNSPECIFIED.) ;
#3314=B_SPLINE_CURVE_WITH_KNOTS('',3,(#18460,#18461,#18462,#18463,#18464,
#18465,#18466,#18467,#18468,#18469,#18470,#18471,#18472,#18473,#18474,#18475),
 .UNSPECIFIED.,.T.,.F.,(4,1,1,1,1,1,1,1,1,1,1,1,1,4),(0.,0.520304865043955,
0.70954256158844,0.804161409794499,0.898780258000557,1.15893269054429,1.41908512308802,
1.67923755561058,1.93938998813313,2.03400883648099,2.12862768482886,2.3178653810957,
2.57801781365659,2.83817024621747),.UNSPECIFIED.) ;
#3315=B_SPLINE_CURVE_WITH_KNOTS('',3,(#18477,#18478,#18479,#18480,#18481,
#18482,#18483,#18484,#18485,#18486,#18487,#18488,#18489,#18490,#18491,#18492),
 .UNSPECIFIED.,.T.,.F.,(4,1,1,1,1,1,1,1,1,1,1,1,1,4),(0.,0.520304864990006,
0.709542561256855,0.80416140961432,0.898780257971786,1.15893269048473,1.41908512299766,
1.67923755554141,1.93938998808516,2.03400883629124,2.12862768449733,2.31786538104175,
2.57801781362961,2.83817024621746),.UNSPECIFIED.) ;
#3316=B_SPLINE_CURVE_WITH_KNOTS('',3,(#18494,#18495,#18496,#18497,#18498,
#18499,#18500,#18501,#18502,#18503,#18504,#18505,#18506,#18507,#18508,#18509),
 .UNSPECIFIED.,.T.,.F.,(4,1,1,1,1,1,1,1,1,1,1,1,1,4),(0.,0.520304865114576,
0.709542561608101,0.804161409843274,0.898780258078447,1.1589326906067,1.41908512313495,
1.67923755567353,1.9393899882121,2.03400883653032,2.12862768484853,2.31786538116822,
2.57801781373375,2.83817024629929),.UNSPECIFIED.) ;
#3317=B_SPLINE_CURVE_WITH_KNOTS('',3,(#18512,#18513,#18514,#18515,#18516,
#18517,#18518,#18519,#18520,#18521,#18522,#18523,#18524,#18525,#18526,#18527,
#18528,#18529,#18530),.UNSPECIFIED.,.T.,.F.,(4,1,1,1,1,1,1,1,1,1,1,1,1,
1,1,1,4),(0.,0.667571568814075,1.33514313762815,2.00271471386764,2.67028629010714,
3.33785785892123,4.00542942773531,4.67300100397479,5.34057258021427,6.00814415645105,
6.67571573268784,7.34328730150191,8.01085887031598,8.67843044655548,9.34600202279497,
10.0135735916091,10.6811451604231),.UNSPECIFIED.) ;
#3318=B_SPLINE_CURVE_WITH_KNOTS('',3,(#18532,#18533,#18534,#18535,#18536,
#18537,#18538,#18539,#18540,#18541,#18542,#18543,#18544,#18545,#18546,#18547,
#18548,#18549,#18550,#18551,#18552,#18553,#18554,#18555,#18556,#18557,#18558,
#18559,#18560,#18561,#18562,#18563,#18564,#18565,#18566,#18567,#18568,#18569,
#18570,#18571,#18572,#18573,#18574,#18575,#18576,#18577,#18578,#18579,#18580,
#18581,#18582,#18583,#18584,#18585,#18586,#18587,#18588,#18589,#18590,#18591,
#18592,#18593,#18594,#18595,#18596,#18597,#18598,#18599,#18600,#18601,#18602,
#18603,#18604,#18605,#18606,#18607),.UNSPECIFIED.,.F.,.F.,(4,3,3,3,3,3,
3,3,3,3,3,3,3,3,3,3,3,3,3,3,3,3,3,3,3,4),(0.645166102166136,0.779260260223949,
0.953432776292934,1.00087899502182,1.2245538215817,1.38792237623853,1.45262949361123,
1.68236582634801,1.91465733457253,2.07687507662671,2.15140541324293,2.35410717544614,
2.38890591237544,2.56658916175515,2.63160106806682,2.84272353227155,2.87721416966982,
3.12396628424627,3.34224298985172,3.37420303087565,3.57733400929029,3.62763142462921,
3.88309575096213,4.05946355048951,4.14300211392098,4.256701237387),
 .UNSPECIFIED.) ;
#3319=B_SPLINE_CURVE_WITH_KNOTS('',3,(#18608,#18609,#18610,#18611,#18612,
#18613,#18614,#18615,#18616,#18617,#18618,#18619,#18620,#18621,#18622,#18623,
#18624,#18625,#18626,#18627,#18628,#18629,#18630,#18631,#18632,#18633,#18634,
#18635,#18636,#18637,#18638,#18639,#18640,#18641,#18642,#18643,#18644,#18645,
#18646,#18647,#18648,#18649,#18650,#18651,#18652,#18653,#18654,#18655,#18656,
#18657,#18658,#18659,#18660,#18661,#18662,#18663,#18664,#18665,#18666,#18667,
#18668,#18669,#18670,#18671,#18672,#18673,#18674,#18675,#18676,#18677,#18678,
#18679,#18680,#18681,#18682,#18683,#18684,#18685,#18686,#18687,#18688,#18689,
#18690,#18691,#18692,#18693,#18694,#18695,#18696,#18697,#18698),
 .UNSPECIFIED.,.F.,.F.,(4,3,3,3,3,3,3,3,3,3,3,3,3,3,3,3,3,3,3,3,3,3,3,3,
3,3,3,3,3,3,4),(2.65072463961435E-14,0.145660370872957,0.320807895379567,
0.40519534671499,0.64591367467841,0.660293540743808,0.857679476426317,0.913841563973973,
1.11044144600034,1.16384460786289,1.38186603893937,1.40950020307555,1.5735409420364,
1.65456863850231,1.8674834420843,1.89503815818863,2.07745338563794,2.13417126051133,
2.32367309259648,2.37029532866498,2.58949458425784,2.60221850258879,2.76061048665942,
2.83266354337296,3.04253537567105,3.05893725264363,3.22614498180073,3.28375110259138,
3.46729051496174,3.5046955288712,3.61218581593466),.UNSPECIFIED.) ;
#3320=B_SPLINE_CURVE_WITH_KNOTS('',3,(#18701,#18702,#18703,#18704,#18705,
#18706,#18707,#18708,#18709,#18710,#18711,#18712,#18713,#18714,#18715,#18716,
#18717,#18718,#18719),.UNSPECIFIED.,.T.,.F.,(4,1,1,1,1,1,1,1,1,1,1,1,1,
1,1,1,4),(0.,0.66757156881407,1.33514313762814,2.00271471386764,2.67028629010714,
3.33785785892123,4.00542942773532,4.67300100397479,5.34057258021426,6.00814415645105,
6.67571573268784,7.34328730150192,8.01085887031599,8.67843044655547,9.34600202279495,
10.013573591609,10.6811451604231),.UNSPECIFIED.) ;
#3321=B_SPLINE_CURVE_WITH_KNOTS('',3,(#18721,#18722,#18723,#18724,#18725,
#18726,#18727,#18728,#18729,#18730,#18731,#18732,#18733,#18734,#18735,#18736,
#18737,#18738,#18739,#18740,#18741,#18742,#18743,#18744,#18745,#18746,#18747,
#18748,#18749,#18750,#18751,#18752,#18753,#18754,#18755,#18756,#18757,#18758,
#18759,#18760,#18761,#18762,#18763,#18764,#18765,#18766,#18767,#18768,#18769,
#18770,#18771,#18772,#18773,#18774,#18775,#18776,#18777,#18778,#18779,#18780,
#18781,#18782,#18783,#18784,#18785,#18786,#18787,#18788,#18789,#18790,#18791,
#18792,#18793,#18794,#18795,#18796),.UNSPECIFIED.,.F.,.F.,(4,3,3,3,3,3,
3,3,3,3,3,3,3,3,3,3,3,3,3,3,3,3,3,3,3,4),(0.,0.113699105245172,0.290066601932432,
0.373605432506589,0.629069723752491,0.832200318202323,0.882498082698975,
1.10077464959384,1.13273479495996,1.37948687564694,1.59060880287217,1.62509994351725,
1.80278299829912,1.86779506587701,2.07049658686577,2.10529553239169,2.26751302289565,
2.34204357854793,2.5743350548707,2.80407135605698,2.96743995792939,3.03214699676444,
3.25582179260699,3.42999406441784,3.47744049697027,3.61176015724593),
 .UNSPECIFIED.) ;
#3322=B_SPLINE_CURVE_WITH_KNOTS('',3,(#18797,#18798,#18799,#18800,#18801,
#18802,#18803,#18804,#18805,#18806,#18807,#18808,#18809,#18810,#18811,#18812,
#18813,#18814,#18815,#18816,#18817,#18818,#18819,#18820,#18821,#18822,#18823,
#18824,#18825,#18826,#18827,#18828,#18829,#18830,#18831,#18832,#18833,#18834,
#18835,#18836,#18837,#18838,#18839,#18840,#18841,#18842,#18843,#18844,#18845,
#18846,#18847,#18848,#18849,#18850,#18851,#18852,#18853,#18854,#18855,#18856,
#18857,#18858,#18859,#18860,#18861,#18862,#18863,#18864,#18865,#18866,#18867,
#18868,#18869,#18870,#18871,#18872,#18873,#18874,#18875,#18876,#18877,#18878,
#18879,#18880,#18881,#18882,#18883,#18884,#18885,#18886,#18887),
 .UNSPECIFIED.,.F.,.F.,(4,3,3,3,3,3,3,3,3,3,3,3,3,3,3,3,3,3,3,3,3,3,3,3,
3,3,3,3,3,3,4),(0.644441410779395,0.75200920201523,0.935549149058043,0.972953628075139,
1.14016174570414,1.1977674777995,1.40763894920845,1.4240411868457,1.58243323607625,
1.65448622740162,1.8736850500751,1.88640940109609,2.07591169111657,2.12253346901659,
2.3049493882588,2.36166657110351,2.57458028242975,2.6021360905531,2.76617690465824,
2.84720452573892,3.06522545761094,3.09286012071041,3.28946054370769,3.34286316435422,
3.54024970390616,3.59641118733614,3.8371274811361,3.85150938111551,4.02665714187106,
4.11104435670409,4.25670473004031),.UNSPECIFIED.) ;
#3323=B_SPLINE_CURVE_WITH_KNOTS('',3,(#25952,#25953,#25954,#25955,#25956,
#25957,#25958,#25959,#25960,#25961,#25962,#25963,#25964),.UNSPECIFIED.,
 .F.,.F.,(4,3,3,3,4),(0.00254885090942774,0.0798589394093864,0.156372123655699,
0.227373986667402,0.232885307902011),.UNSPECIFIED.) ;
#3324=B_SPLINE_CURVE_WITH_KNOTS('',3,(#25966,#25967,#25968,#25969,#25970,
#25971,#25972,#25973,#25974,#25975,#25976,#25977,#25978,#25979,#25980,#25981,
#25982,#25983,#25984,#25985,#25986,#25987,#25988,#25989,#25990,#25991,#25992,
#25993,#25994,#25995,#25996,#25997,#25998,#25999,#26000,#26001,#26002,#26003,
#26004,#26005,#26006,#26007,#26008,#26009,#26010,#26011,#26012,#26013,#26014,
#26015,#26016,#26017,#26018,#26019,#26020,#26021,#26022,#26023,#26024,#26025,
#26026,#26027,#26028,#26029,#26030,#26031,#26032),.UNSPECIFIED.,.F.,.F.,
(4,3,3,3,3,3,3,3,3,3,3,3,3,3,3,3,3,3,3,3,3,3,4),(0.827865437902791,0.969498970179885,
1.21799523287345,1.38410983938184,1.46526269189611,1.66145193054325,1.70762278107361,
1.87143425230401,1.94910503522581,2.16981824391288,2.18634151562757,2.36300905408328,
2.42204214196616,2.61858944195816,2.65392288419624,2.88181125820872,3.05474643104765,
3.10884237347622,3.2820669169133,3.33241696329946,3.53151864647208,3.55138037599939,
3.61142664742073),.UNSPECIFIED.) ;
#3325=B_SPLINE_CURVE_WITH_KNOTS('',3,(#26033,#26034,#26035,#26036,#26037,
#26038,#26039,#26040,#26041,#26042,#26043,#26044,#26045,#26046,#26047,#26048,
#26049,#26050,#26051,#26052,#26053,#26054,#26055,#26056,#26057,#26058,#26059,
#26060,#26061,#26062,#26063,#26064,#26065,#26066,#26067,#26068,#26069,#26070,
#26071,#26072,#26073,#26074,#26075,#26076,#26077,#26078,#26079,#26080,#26081,
#26082,#26083,#26084,#26085,#26086,#26087,#26088,#26089,#26090,#26091,#26092,
#26093,#26094,#26095,#26096,#26097,#26098,#26099,#26100,#26101,#26102,#26103,
#26104,#26105,#26106,#26107,#26108,#26109,#26110,#26111,#26112,#26113,#26114,
#26115,#26116,#26117,#26118,#26119,#26120,#26121,#26122,#26123,#26124,#26125,
#26126,#26127,#26128,#26129,#26130,#26131,#26132,#26133,#26134,#26135,#26136,
#26137,#26138,#26139,#26140,#26141,#26142,#26143,#26144,#26145,#26146,#26147,
#26148,#26149,#26150,#26151,#26152,#26153,#26154,#26155,#26156,#26157,#26158,
#26159,#26160,#26161,#26162,#26163,#26164,#26165,#26166,#26167,#26168,#26169,
#26170,#26171,#26172,#26173,#26174,#26175,#26176,#26177,#26178,#26179,#26180,
#26181,#26182,#26183,#26184,#26185,#26186,#26187,#26188,#26189,#26190,#26191,
#26192,#26193,#26194,#26195,#26196,#26197,#26198,#26199,#26200,#26201,#26202,
#26203,#26204,#26205,#26206,#26207,#26208,#26209,#26210,#26211,#26212,#26213,
#26214,#26215,#26216,#26217,#26218,#26219,#26220,#26221,#26222,#26223,#26224,
#26225,#26226,#26227,#26228,#26229,#26230,#26231,#26232,#26233,#26234,#26235,
#26236,#26237,#26238,#26239,#26240,#26241,#26242,#26243,#26244,#26245,#26246,
#26247,#26248,#26249,#26250,#26251,#26252,#26253,#26254,#26255,#26256,#26257,
#26258,#26259,#26260,#26261,#26262,#26263,#26264,#26265,#26266),
 .UNSPECIFIED.,.F.,.F.,(4,2,2,2,2,2,2,2,2,2,2,2,2,2,2,2,2,2,2,2,2,2,2,2,
2,2,2,2,2,2,2,2,2,2,2,2,2,2,2,2,2,2,2,2,2,2,2,2,2,2,2,2,2,2,2,2,2,2,2,2,
2,2,2,2,2,2,2,2,2,2,2,2,2,2,2,2,2,2,2,2,2,2,2,2,2,2,2,2,2,2,2,2,2,2,2,2,
2,2,2,2,2,2,2,2,2,2,2,2,2,2,2,2,2,2,2,2,4),(1.00011841232436E-6,0.00211487568124348,
0.00573504524170948,0.0105552052984136,0.013206038817188,0.0149819498688102,
0.0165674239395606,0.0182978612274979,0.0210987487537411,0.0278207031606176,
0.0325576793304593,0.0349535909101199,0.0374295225247761,0.0441510043973029,
0.0467789452193183,0.0486016307238571,0.0500606344083361,0.0531874431833309,
0.0585847367877814,0.061095445986784,0.0630628385785719,0.0657374888256804,
0.0741503815625694,0.0773889156137434,0.0796579552177498,0.0807688356105725,
0.0831046581995265,0.0871216394910236,0.0924688277337361,0.0956070243899364,
0.0989528606039263,0.106157070817436,0.109664151060947,0.112189673083253,
0.114183844036864,0.120195774072755,0.123225376896897,0.125013914410265,
0.125072206216835,0.125127793145369,0.125180993795639,0.125232100146867,
0.125281381546994,0.125329088683266,0.125375457257543,0.125420711238155,
0.125465066274631,0.125508733230266,0.125551921586471,0.125594843368815,
0.125637717537804,0.125680774972013,0.125724264618053,0.125768461261691,
0.125813675253946,0.125860265868866,0.125908659536032,0.125959375243851,
0.126013062148227,0.126070556325349,0.126132970718823,0.126201845154774,
0.126259063080509,0.126393996284037,0.127819373950443,0.129258214424421,
0.131110074945505,0.134186015138983,0.143305528015856,0.146054540687782,
0.147480969448531,0.148562805052782,0.149680232155087,0.149737317074787,
0.149799262331264,0.149866431189701,0.149894352585556,0.149929710577313,
0.151384856346816,0.153687973533875,0.158498449384403,0.166624947623936,
0.168158596691493,0.168993930820365,0.16982272504412,0.170635089478444,
0.171279550802086,0.172645679114621,0.175150864479718,0.182316618022404,
0.182679082917977,0.188178400224613,0.18968495109763,0.190545811688084,
0.191407957865223,0.192485536340025,0.194677082028042,0.197748855900557,
0.2033441185278,0.209436941624861,0.210950745000197,0.211819874549075,0.21269313079068,
0.213580580305497,0.213868320544485,0.214583360312335,0.216366268847191,
0.220199054862944,0.228694348237006,0.230899224185619,0.232466907354201,
0.234074279046871,0.23578755192576,0.244157487005655,0.250074754468557,
0.25296313407621,0.255635388345462),.UNSPECIFIED.) ;
#3326=B_SPLINE_CURVE_WITH_KNOTS('',3,(#33239,#33240,#33241,#33242,#33243,
#33244,#33245,#33246,#33247,#33248,#33249,#33250,#33251),.UNSPECIFIED.,
 .F.,.F.,(4,3,3,3,4),(0.,0.077810894493114,0.156406594156863,0.238224767252187,
0.302239126484708),.UNSPECIFIED.) ;
#3327=B_SPLINE_CURVE_WITH_KNOTS('',3,(#33253,#33254,#33255,#33256,#33257,
#33258,#33259,#33260,#33261,#33262,#33263,#33264,#33265,#33266,#33267,#33268,
#33269,#33270,#33271,#33272,#33273,#33274,#33275,#33276,#33277,#33278,#33279,
#33280,#33281,#33282,#33283,#33284,#33285,#33286,#33287,#33288,#33289,#33290,
#33291,#33292,#33293,#33294,#33295,#33296,#33297,#33298,#33299,#33300,#33301,
#33302,#33303,#33304,#33305,#33306,#33307,#33308,#33309,#33310,#33311,#33312,
#33313,#33314,#33315,#33316,#33317,#33318,#33319,#33320,#33321,#33322,#33323,
#33324,#33325),.UNSPECIFIED.,.F.,.F.,(4,3,3,3,3,3,3,3,3,3,3,3,3,3,3,3,3,
3,3,3,3,3,3,3,4),(0.730465481580954,0.828645125064015,1.05028297683292,
1.25837815007314,1.27510983870171,1.45572385055039,1.50312162767456,1.73316624271265,
1.90167574230091,1.96765453876245,2.20387853992391,2.44262970595965,2.62527594874775,
2.68580352301486,2.90417726727137,2.9307933308959,3.16390700344848,3.17732285394432,
3.35312908465983,3.42916468918551,3.68305064914715,3.93956813737863,4.12212044382143,
4.19992860565306,4.25678609882998),.UNSPECIFIED.) ;
#3328=B_SPLINE_CURVE_WITH_KNOTS('',3,(#33326,#33327,#33328,#33329,#33330,
#33331,#33332,#33333,#33334,#33335,#33336,#33337,#33338,#33339,#33340,#33341,
#33342,#33343,#33344),.UNSPECIFIED.,.F.,.F.,(4,1,1,1,1,1,1,1,1,1,1,1,1,
1,1,1,4),(87.336489761411,87.4317045853384,87.8665778926469,88.3014512000977,
88.7363245076919,89.1711978154302,89.6060711233134,90.0409444313423,90.4758177395175,
90.9106910478396,91.345564356309,91.7804376649263,92.2153109736917,92.6501842826055,
93.085057591668,93.5199309008791,93.8817096841969),.UNSPECIFIED.) ;
#3329=B_SPLINE_CURVE_WITH_KNOTS('',3,(#33352,#33353,#33354,#33355,#33356,
#33357),.UNSPECIFIED.,.F.,.F.,(4,2,4),(-0.0221113024783476,-0.0110566426889343,
-1.00008409958761E-6),.UNSPECIFIED.) ;
#3330=B_SPLINE_CURVE_WITH_KNOTS('',3,(#33359,#33360,#33361,#33362,#33363,
#33364,#33365,#33366,#33367,#33368,#33369,#33370,#33371,#33372,#33373,#33374,
#33375,#33376,#33377,#33378,#33379,#33380,#33381,#33382,#33383,#33384,#33385,
#33386,#33387,#33388,#33389,#33390,#33391,#33392,#33393,#33394,#33395,#33396,
#33397,#33398,#33399,#33400,#33401,#33402,#33403,#33404,#33405,#33406,#33407,
#33408,#33409,#33410,#33411,#33412,#33413,#33414,#33415,#33416,#33417,#33418,
#33419,#33420,#33421,#33422,#33423,#33424,#33425,#33426,#33427,#33428,#33429,
#33430,#33431,#33432,#33433,#33434,#33435,#33436,#33437,#33438,#33439,#33440,
#33441,#33442,#33443,#33444,#33445,#33446,#33447,#33448,#33449,#33450,#33451,
#33452,#33453,#33454,#33455,#33456,#33457,#33458,#33459,#33460,#33461,#33462,
#33463,#33464,#33465,#33466,#33467,#33468,#33469,#33470,#33471,#33472,#33473,
#33474,#33475,#33476,#33477,#33478,#33479,#33480,#33481,#33482,#33483,#33484,
#33485,#33486,#33487,#33488,#33489,#33490,#33491,#33492,#33493,#33494,#33495,
#33496,#33497,#33498,#33499,#33500,#33501,#33502,#33503,#33504,#33505,#33506,
#33507,#33508,#33509,#33510,#33511,#33512,#33513,#33514,#33515,#33516,#33517,
#33518,#33519,#33520,#33521,#33522,#33523,#33524,#33525,#33526,#33527,#33528,
#33529,#33530,#33531,#33532,#33533,#33534,#33535,#33536,#33537,#33538,#33539,
#33540,#33541,#33542,#33543,#33544,#33545,#33546,#33547,#33548,#33549,#33550,
#33551,#33552,#33553,#33554,#33555,#33556,#33557,#33558,#33559,#33560,#33561,
#33562,#33563,#33564,#33565,#33566,#33567,#33568,#33569,#33570,#33571,#33572,
#33573,#33574,#33575,#33576,#33577,#33578,#33579,#33580,#33581,#33582,#33583,
#33584,#33585,#33586,#33587,#33588,#33589,#33590,#33591,#33592,#33593,#33594,
#33595,#33596,#33597,#33598,#33599,#33600,#33601,#33602,#33603,#33604,#33605,
#33606,#33607,#33608,#33609,#33610,#33611,#33612,#33613,#33614,#33615,#33616,
#33617,#33618,#33619,#33620,#33621,#33622,#33623,#33624,#33625,#33626,#33627,
#33628,#33629,#33630,#33631,#33632,#33633,#33634,#33635,#33636,#33637,#33638,
#33639,#33640,#33641,#33642,#33643,#33644,#33645,#33646,#33647,#33648,#33649,
#33650,#33651,#33652,#33653,#33654,#33655,#33656,#33657,#33658,#33659,#33660,
#33661,#33662,#33663,#33664,#33665,#33666,#33667,#33668,#33669,#33670,#33671,
#33672,#33673,#33674,#33675,#33676,#33677,#33678,#33679,#33680,#33681,#33682,
#33683,#33684,#33685,#33686,#33687,#33688,#33689,#33690,#33691,#33692,#33693,
#33694,#33695,#33696,#33697,#33698,#33699,#33700,#33701,#33702,#33703,#33704,
#33705,#33706,#33707,#33708,#33709,#33710,#33711,#33712,#33713,#33714,#33715,
#33716,#33717,#33718,#33719,#33720,#33721,#33722,#33723,#33724,#33725,#33726,
#33727,#33728,#33729,#33730,#33731,#33732,#33733,#33734,#33735,#33736,#33737,
#33738,#33739,#33740,#33741,#33742,#33743,#33744,#33745,#33746,#33747,#33748,
#33749,#33750,#33751,#33752,#33753,#33754,#33755,#33756,#33757,#33758,#33759,
#33760,#33761,#33762,#33763,#33764,#33765,#33766,#33767,#33768,#33769,#33770,
#33771,#33772,#33773,#33774,#33775,#33776,#33777,#33778,#33779,#33780,#33781,
#33782,#33783,#33784,#33785,#33786,#33787,#33788,#33789,#33790,#33791,#33792,
#33793,#33794,#33795,#33796,#33797,#33798,#33799,#33800,#33801,#33802,#33803,
#33804,#33805,#33806,#33807,#33808,#33809,#33810,#33811,#33812,#33813,#33814,
#33815,#33816,#33817,#33818,#33819,#33820,#33821,#33822,#33823,#33824,#33825,
#33826,#33827,#33828,#33829,#33830,#33831,#33832,#33833,#33834,#33835,#33836,
#33837,#33838,#33839,#33840,#33841,#33842,#33843,#33844,#33845,#33846,#33847,
#33848,#33849,#33850,#33851,#33852,#33853,#33854,#33855,#33856,#33857,#33858,
#33859,#33860,#33861,#33862,#33863,#33864,#33865,#33866,#33867,#33868,#33869,
#33870,#33871,#33872,#33873,#33874,#33875,#33876,#33877,#33878,#33879,#33880,
#33881,#33882,#33883,#33884,#33885,#33886,#33887,#33888,#33889,#33890,#33891,
#33892,#33893,#33894,#33895,#33896,#33897,#33898,#33899,#33900,#33901,#33902,
#33903,#33904,#33905,#33906,#33907,#33908,#33909,#33910,#33911,#33912,#33913,
#33914,#33915,#33916,#33917,#33918,#33919,#33920,#33921,#33922,#33923,#33924,
#33925,#33926,#33927,#33928,#33929,#33930,#33931,#33932,#33933,#33934,#33935,
#33936,#33937,#33938,#33939,#33940,#33941,#33942,#33943,#33944,#33945,#33946,
#33947,#33948,#33949,#33950,#33951,#33952,#33953,#33954,#33955,#33956,#33957,
#33958,#33959,#33960,#33961,#33962,#33963,#33964,#33965,#33966,#33967,#33968,
#33969,#33970,#33971,#33972,#33973,#33974,#33975,#33976,#33977,#33978,#33979,
#33980,#33981,#33982,#33983,#33984,#33985,#33986,#33987,#33988,#33989,#33990,
#33991,#33992,#33993,#33994,#33995,#33996,#33997,#33998,#33999,#34000,#34001,
#34002,#34003,#34004,#34005,#34006,#34007,#34008,#34009,#34010,#34011,#34012,
#34013,#34014,#34015,#34016,#34017,#34018,#34019,#34020,#34021,#34022,#34023,
#34024,#34025,#34026,#34027,#34028,#34029,#34030,#34031,#34032,#34033,#34034,
#34035,#34036,#34037,#34038,#34039,#34040,#34041,#34042,#34043,#34044,#34045,
#34046,#34047,#34048,#34049,#34050,#34051,#34052,#34053,#34054,#34055,#34056,
#34057,#34058,#34059,#34060,#34061,#34062,#34063,#34064,#34065,#34066,#34067,
#34068,#34069,#34070,#34071,#34072,#34073,#34074,#34075,#34076,#34077,#34078,
#34079,#34080,#34081,#34082,#34083,#34084,#34085,#34086,#34087,#34088,#34089,
#34090,#34091,#34092,#34093,#34094,#34095,#34096,#34097,#34098,#34099,#34100,
#34101,#34102,#34103,#34104,#34105,#34106,#34107,#34108,#34109,#34110,#34111,
#34112,#34113,#34114,#34115,#34116,#34117,#34118,#34119,#34120,#34121,#34122,
#34123,#34124,#34125,#34126,#34127,#34128,#34129,#34130,#34131,#34132,#34133,
#34134,#34135,#34136,#34137,#34138,#34139,#34140,#34141,#34142),
 .UNSPECIFIED.,.F.,.F.,(4,2,2,2,2,2,2,2,2,2,2,2,2,2,2,2,2,2,2,2,2,2,2,2,
2,2,2,2,2,2,2,2,2,2,2,2,2,2,2,2,2,2,2,2,2,2,2,2,2,2,2,2,2,2,2,2,2,2,2,2,
2,2,2,2,2,2,2,2,2,2,2,2,2,2,2,2,2,2,2,2,2,2,2,2,2,2,2,2,2,2,2,2,2,2,2,2,
2,2,2,2,2,2,2,2,2,2,2,2,2,2,2,2,2,2,2,2,2,2,2,2,2,2,2,2,2,2,2,2,2,2,2,2,
2,2,2,2,2,2,2,2,2,2,2,2,2,2,2,2,2,2,2,2,2,2,2,2,2,2,2,2,2,2,2,2,2,2,2,2,
2,2,2,2,2,2,2,2,2,2,2,2,2,2,2,2,2,2,2,2,2,2,2,2,2,2,2,2,2,2,2,2,2,2,2,2,
2,2,2,2,2,2,2,2,2,2,2,2,2,2,2,2,2,2,2,2,2,2,2,2,2,2,2,2,2,2,2,2,2,2,2,2,
2,2,2,2,2,2,2,2,2,2,2,2,2,2,2,2,2,2,2,2,2,2,2,2,2,2,2,2,2,2,2,2,2,2,2,2,
2,2,2,2,2,2,2,2,2,2,2,2,2,2,2,2,2,2,2,2,2,2,2,2,2,2,2,2,2,2,2,2,2,2,2,2,
2,2,2,2,2,2,2,2,2,2,2,2,2,2,2,2,2,2,2,2,2,2,2,2,2,2,2,2,2,2,2,2,2,2,2,2,
2,2,2,2,2,2,2,2,2,2,2,2,2,2,2,2,2,2,2,2,2,2,2,2,2,2,2,2,2,2,2,2,2,2,2,2,
2,2,2,2,2,2,2,4),(1.00000001682088E-6,0.00412378435184989,0.00720393598231871,
0.0103717437260683,0.0145585560623559,0.0244680661083784,0.0329545253558829,
0.0425764562482095,0.0440725730601049,0.0451152033327152,0.0460124834422306,
0.046934990694426,0.0481632294947072,0.050724122983898,0.0630557572617355,
0.0756411641465513,0.0813714533000482,0.0846115376600266,0.0868137062066845,
0.0886335553345215,0.0903716139373155,0.0926078484500323,0.0964385758774219,
0.110549659029758,0.121459739409565,0.129033302174599,0.130760319639646,
0.131651475686724,0.13256791807344,0.133625596671386,0.135410993071053,
0.142996697469524,0.155349098660419,0.163677401609616,0.167444141957419,
0.170440984965391,0.173893558787823,0.180700035175655,0.203153850559646,
0.208964366471218,0.212113722160231,0.212181573822733,0.212246701945834,
0.212309247893573,0.212369344911492,0.212427118577817,0.212482687279601,
0.212536162672608,0.212587650052935,0.212637248730231,0.212685052495241,
0.212731149867509,0.212775624407095,0.212818555053062,0.212860016364252,
0.212900078783675,0.212938809005543,0.212976269956484,0.213012521237669,
0.213047619261203,0.213081617320833,0.213114566013228,0.213146513186833,
0.213177504145674,0.213207581900862,0.213236787245495,0.213265158841159,
0.213292733336209,0.213319545600158,0.213345628689971,0.213371014017961,
0.213395731397533,0.213419809318236,0.213443274783266,0.213466153519028,
0.213488469935302,0.213510247310883,0.213531507949612,0.213552272981879,
0.213572562581441,0.213592396070832,0.213611791795321,0.213630767294437,
0.213649339348355,0.21366752401514,0.213685336572033,0.213702791695819,
0.213719903515766,0.213736685484902,0.213753150432965,0.213769310728772,
0.21378517818009,0.21380076423114,0.213816079672839,0.213831134968361,0.213845940413858,
0.213860505553586,0.213874839687762,0.213888951851384,0.213902850598825,
0.213932756139912,0.213962451140244,0.213991944588857,0.214021245372558,
0.214050362396523,0.21407930444072,0.21410808025762,0.214136698534644,0.214165167899702,
0.214193497034036,0.214221694551859,0.2142497691563,0.216316764564342,0.21852724166571,
0.222391601619717,0.233412192448542,0.237938484265656,0.239269823749761,
0.240130520900268,0.240495793723779,0.241009367005868,0.242468317341029,
0.247176360858102,0.256709502061751,0.260325910001816,0.262967487383116,
0.262976550055926,0.262985547006863,0.262994478949593,0.263003346688414,
0.263012151095934,0.263020892846339,0.263029572691251,0.263038191357084,
0.263046749477224,0.263055247941868,0.263063687659736,0.263072069032241,
0.263080392853637,0.263088659913182,0.263096870891574,0.263105026435826,
0.263113127286558,0.263121173964806,0.263129167089014,0.263137107431365,
0.263144995519346,0.263152832068115,0.263160617799678,0.263168353033123,
0.263176038461129,0.263183674782712,0.26319126272822,0.263198802642571,
0.263206295194712,0.263213741094152,0.263221140664439,0.263228494507098,
0.263235803269919,0.263243067523899,0.263250287803804,0.263257464673431,
0.263264598540779,0.263271689890335,0.263278739290234,0.263285747295609,
0.263292714458167,0.263299641321257,0.263306528372713,0.26331337601404,
0.263320184523784,0.263326954678803,0.263333686681642,0.263340381199479,
0.263347038813512,0.263353659761591,0.263360244580434,0.263366793603721,
0.26337330735734,0.263379786216298,0.263386230638156,0.26339264105942,0.263399017864931,
0.263405361587141,0.263411672563466,0.263417951327975,0.263424198117529,
0.263430413386007,0.263436597660909,0.263442751083506,0.263448874031492,
0.263454967274796,0.263461030978515,0.263467065444312,0.263473071031463,
0.263479048115547,0.26348499719065,0.263490918600648,0.263496812378503,
0.263502679415271,0.263508519888591,0.263514334030613,0.263520121950217,
0.263525884178365,0.263531621317426,0.263537333562649,0.263543021217466,
0.263548684527306,0.26355432378257,0.263559939476474,0.26356553220086,0.263571101903078,
0.26357664882651,0.263582173188598,0.263587675623338,0.263593156231263,
0.263598615319778,0.263604053269746,0.263609470391771,0.263614866889543,
0.26362024322544,0.263625599643742,0.263630936585898,0.263636254096805,
0.263641552456102,0.263646831847872,0.263652092608879,0.263657335218632,
0.263662559954704,0.263667766857738,0.263672956340642,0.263678128674226,
0.263683284231555,0.263688422961633,0.263693545507355,0.263698652084501,
0.263703742717273,0.263708818049715,0.263713878119357,0.263718922833078,
0.26372395284085,0.26372896824138,0.263733969297089,0.263738956503716,0.263743929821177,
0.263748889334407,0.263753835587936,0.263758768884115,0.263763689325482,
0.263768597440996,0.263773493243255,0.263778377033001,0.263783249035293,
0.263788109318664,0.263792958270771,0.263797796190937,0.263802623000511,
0.263807439149299,0.263812244968126,0.263817040702161,0.263821826455816,
0.263826602693428,0.263831369545261,0.263836126972638,0.263840875287213,
0.2638456147326,0.263850345569688,0.263855068225747,0.263859782816834,0.263864489633565,
0.263869188717774,0.263873880213536,0.265401600255821,0.266952459355332,
0.269475389911629,0.277313206724315,0.28897782029383,0.29680510177015,0.302454562050922,
0.306773756205715,0.310418199298673,0.314420940817946,0.319531495145557,
0.337589015000251,0.343318491153592,0.345973977396469,0.348070856727646,
0.34924830229069,0.350317526017165,0.351700343117464,0.354135128192724,
0.368622453128095,0.37328553484783,0.375179706387552,0.378580431548132,
0.381216461170867,0.383203158061469,0.393168494486374,0.405892027088247,
0.414901388307961,0.418941628677775,0.431399265051532,0.434934023162209,
0.43826011895309,0.442047228602453,0.448707942327242,0.450636832431272,
0.455673185951709,0.457711421550039,0.459369612802801,0.459393312537367,
0.459418300524679,0.459444670008319,0.461107089664572,0.464102834781033,
0.474294649944849,0.478469544933861,0.480777478216863,0.483091943086908,
0.485584314396763,0.489201048388902,0.49743706517905,0.498560540151176,
0.502130853319476,0.503676616615559,0.505311218089556,0.507306934747305,
0.510681185550213,0.522412328781764,0.524853424365672,0.52832725682492,
0.532028675715041,0.538308483071323,0.544544439139152,0.546692055961045,
0.548563315398212,0.548816900362078,0.549061281778513,0.549493119504176,
0.552992927585461,0.565070061983992,0.568331469467836,0.57196600242079,
0.576351091695299,0.581912985310773,0.58757768752732,0.589810159141457,
0.591607083077002,0.591973682452946,0.592227919713621,0.595420724217392,
0.605818271537551,0.609795976107658,0.613252592277516,0.617136578941486,
0.624359334370696,0.629340571199528,0.631327527801954,0.632953647429156,
0.634520487477763,0.637129649028583,0.644471683708734,0.651701706861225,
0.654404126261276,0.656417672709504,0.658388187756684,0.660761646549056,
0.66447217565491,0.673649019142133,0.677975885884396,0.680721260710457,
0.683544414440198,0.68754435673873,0.700974075705117,0.708499933748802,
0.71587279908506,0.718924768869659,0.722413104893756,0.72800993542403,0.737282377918865,
0.740350329593211,0.742684396226621,0.745136271957237,0.748306111782994,
0.754030433416531,0.762682415799703,0.764638709251022,0.766387126543181,
0.768545119657253,0.776581200999748,0.782397828470698,0.786290042297251),
 .UNSPECIFIED.) ;
#3331=B_SPLINE_CURVE_WITH_KNOTS('',3,(#34143,#34144,#34145,#34146,#34147,
#34148,#34149,#34150,#34151,#34152,#34153,#34154,#34155,#34156,#34157,#34158,
#34159,#34160,#34161,#34162,#34163,#34164,#34165,#34166,#34167,#34168,#34169,
#34170,#34171,#34172,#34173,#34174,#34175,#34176,#34177,#34178,#34179,#34180,
#34181,#34182,#34183,#34184,#34185,#34186,#34187,#34188,#34189,#34190,#34191,
#34192,#34193,#34194,#34195,#34196,#34197,#34198,#34199,#34200,#34201,#34202,
#34203,#34204,#34205,#34206,#34207,#34208,#34209,#34210,#34211,#34212,#34213,
#34214,#34215,#34216,#34217,#34218,#34219,#34220,#34221,#34222,#34223,#34224,
#34225,#34226,#34227,#34228,#34229,#34230,#34231,#34232,#34233,#34234,#34235,
#34236,#34237,#34238,#34239,#34240,#34241,#34242,#34243,#34244,#34245,#34246,
#34247,#34248,#34249,#34250,#34251,#34252,#34253,#34254,#34255,#34256,#34257),
 .UNSPECIFIED.,.F.,.F.,(4,3,3,3,3,3,3,3,3,3,3,3,3,3,3,3,3,3,3,3,3,3,3,3,
3,3,3,3,3,3,3,3,3,3,3,3,3,3,4),(0.,0.0377030535869255,0.254567771787473,
0.472814106637255,0.691451692099905,0.908523894195214,0.983882498076101,
1.12697364238926,1.34346828606356,1.5611425742692,1.7797791811067,1.96773553890813,
1.9969257592614,2.21556187156847,2.43217608081115,2.65081168252064,2.86814667737748,
2.95162325710805,3.30465282917188,3.52319094343164,3.74168240699446,3.93630861076791,
3.95797636096931,4.17661107076291,4.39376768198014,4.61123898216608,4.92068696075518,
5.04720928317926,5.48426176171593,5.70246546995195,5.90620613535479,5.92104893161303,
6.13805509181114,6.35540620614376,6.79432818927802,6.89176793866042,7.22988061248286,
7.66676952770389,7.87799350781472),.UNSPECIFIED.) ;
#3332=B_SPLINE_CURVE_WITH_KNOTS('',3,(#41229,#41230,#41231,#41232,#41233,
#41234,#41235,#41236,#41237,#41238,#41239,#41240,#41241,#41242,#41243,#41244,
#41245,#41246,#41247,#41248,#41249,#41250,#41251,#41252,#41253,#41254,#41255,
#41256,#41257,#41258,#41259,#41260,#41261,#41262,#41263,#41264,#41265,#41266,
#41267,#41268,#41269,#41270,#41271,#41272),.UNSPECIFIED.,.F.,.F.,(4,2,2,
2,2,2,2,2,2,2,2,2,2,2,2,2,2,2,2,2,2,4),(0.,0.00971482468978479,0.0203872474063451,
0.0279236293697992,0.0332114727556085,0.0367480813478895,0.0382588296076648,
0.0385204656750401,0.0385321923580342,0.0385402608458808,0.0385454131009185,
0.0385482839226327,0.0385506929760014,0.0385535216348412,0.0385585725934473,
0.0385811991469328,0.0386219012951342,0.0407407599450427,0.0444803773101447,
0.0498412534615488,0.0574206915439498,0.0744461764183355),.UNSPECIFIED.) ;
#3333=B_SPLINE_CURVE_WITH_KNOTS('',3,(#41273,#41274,#41275,#41276,#41277,
#41278),.UNSPECIFIED.,.F.,.F.,(4,2,4),(9.99929898480087E-7,0.0141909886738071,
0.027570872690399),.UNSPECIFIED.) ;
#3334=B_SPLINE_CURVE_WITH_KNOTS('',3,(#41279,#41280,#41281,#41282,#41283,
#41284,#41285,#41286,#41287,#41288,#41289,#41290,#41291,#41292,#41293,#41294,
#41295,#41296,#41297,#41298,#41299,#41300,#41301,#41302,#41303,#41304,#41305,
#41306,#41307,#41308,#41309,#41310,#41311,#41312,#41313,#41314,#41315,#41316,
#41317,#41318,#41319,#41320,#41321,#41322,#41323,#41324,#41325,#41326,#41327,
#41328,#41329,#41330,#41331,#41332,#41333,#41334,#41335,#41336,#41337,#41338,
#41339,#41340,#41341,#41342,#41343,#41344,#41345,#41346,#41347,#41348,#41349,
#41350,#41351,#41352,#41353,#41354,#41355,#41356,#41357,#41358,#41359,#41360,
#41361,#41362,#41363,#41364,#41365,#41366,#41367,#41368,#41369,#41370,#41371,
#41372,#41373,#41374,#41375,#41376,#41377,#41378,#41379,#41380,#41381,#41382,
#41383,#41384,#41385,#41386,#41387,#41388,#41389,#41390,#41391,#41392,#41393,
#41394,#41395,#41396,#41397,#41398,#41399,#41400,#41401,#41402,#41403,#41404,
#41405,#41406,#41407,#41408,#41409,#41410,#41411,#41412,#41413,#41414,#41415,
#41416,#41417,#41418,#41419,#41420,#41421,#41422,#41423,#41424,#41425,#41426,
#41427),.UNSPECIFIED.,.F.,.F.,(4,1,1,1,1,1,1,1,1,1,1,1,1,1,1,1,1,1,1,1,
1,1,1,1,1,1,1,1,1,1,1,1,1,1,1,1,1,1,1,1,1,1,1,1,1,1,1,1,1,1,1,1,1,1,1,1,
1,1,1,1,1,1,1,1,1,1,1,1,1,1,1,1,1,1,1,1,1,1,1,1,1,1,1,1,1,1,1,1,1,1,1,1,
1,1,1,1,1,1,1,1,1,1,1,1,1,1,1,1,1,1,1,1,1,1,1,1,1,1,1,1,1,1,1,1,1,1,1,1,
1,1,1,1,1,1,1,1,1,1,1,1,1,1,1,1,1,1,4),(94.7323961409497,94.8262562134414,
95.2611295230986,95.6960028329042,96.1308761428578,96.5657494529591,97.0006227632077,
97.4354960736028,97.870369384144,98.3052426948304,98.7401160056612,99.1749893166354,
99.6098626277522,100.04473593901,100.915335253024,101.351061255639,101.785934567313,
102.220807879124,102.655681191068,103.090554503145,103.525427815353,104.395174440154,
105.264921065453,105.699794378283,106.134667691232,106.569541004295,107.004414317471,
107.8750136343,108.745612951339,109.615359578629,110.485106206296,111.354852834309,
112.224599462639,113.094346091254,113.964092720119,114.834692038763,115.705291357499,
116.575037986826,117.444784616267,118.314531245777,119.184277875311,120.054024504821,
120.923771134261,121.794370453112,122.66496977189,123.534716400968,124.404463029834,
125.274209658448,126.143956286779,127.013702914792,127.883449542458,128.754048859798,
129.624648176939,130.494394803617,131.364141429857,132.233888055637,133.103634680937,
133.973381305737,134.843127930023,135.71372724472,136.584326559147,137.019199870684,
137.454073182083,137.888946493341,138.323819804458,139.193566426263,140.063313047491,
140.498186357887,140.933059668136,141.367932978237,141.802806288191,142.237679597997,
142.673405599673,143.109131601348,143.544004910857,143.978878220217,144.413751529429,
144.848624838491,145.283498147405,145.718371456171,146.153244764789,146.588118073258,
147.022991381581,147.457864689756,147.892737997785,148.327611305669,148.762484613407,
149.197357921002,149.633083921574,150.068809922147,150.503683229455,150.938556536623,
151.37342984365,151.808303150538,152.243176457288,152.678049763901,153.112923070379,
153.547796376722,153.982669682934,154.417542989014,154.852416294964,155.287289600787,
155.722162906483,156.157036212055,156.592762211626,157.028488211198,157.463361516526,
157.898234821735,158.333108126826,158.767981431803,159.202854736666,159.637728041419,
160.072601346062,160.507474650599,160.94234795503,161.37722125936,161.812094563589,
162.246967867721,162.681841171757,163.1167144757,163.552440474473,163.988166473247,
164.423039777011,164.85791308069,165.292786384286,165.727659687801,166.162532991238,
166.597406294601,167.03227959789,167.46715290111,167.902026204262,168.33689950735,
168.771772810376,169.206646113343,169.641519416254,170.076392719112,170.512118717363,
170.947844715614,171.382718018374,171.817591321089,172.252464623762,172.687337926397,
173.122211228996,173.557084531561,173.991957834097,174.426831136606,174.671174277229),
 .UNSPECIFIED.) ;
#3335=B_SPLINE_CURVE_WITH_KNOTS('',3,(#41434,#41435,#41436,#41437,#41438,
#41439,#41440,#41441,#41442,#41443,#41444,#41445,#41446,#41447,#41448,#41449,
#41450,#41451,#41452,#41453,#41454,#41455,#41456,#41457,#41458,#41459,#41460,
#41461,#41462,#41463,#41464,#41465,#41466,#41467,#41468,#41469,#41470,#41471,
#41472,#41473,#41474,#41475,#41476,#41477,#41478,#41479,#41480,#41481,#41482,
#41483,#41484,#41485,#41486,#41487,#41488,#41489,#41490,#41491),
 .UNSPECIFIED.,.F.,.F.,(4,3,3,3,3,3,3,3,3,3,3,3,3,3,3,3,3,3,3,4),(3.94168901841607,
4.15261423848637,4.16618665983574,4.44281737539361,4.60337687546477,4.92785564904694,
5.03898230867997,5.31950967594945,5.47698109930275,5.91441694228828,5.91506511246863,
6.35152427416674,6.66153035873348,6.78902235094994,6.90225579028163,7.22528631210598,
7.50348627263337,7.66193049212852,7.87484757961294,7.8884094762389),
 .UNSPECIFIED.) ;
#3336=B_SPLINE_CURVE_WITH_KNOTS('',3,(#41492,#41493,#41494,#41495,#41496,
#41497,#41498,#41499,#41500,#41501,#41502,#41503,#41504,#41505,#41506,#41507,
#41508,#41509,#41510,#41511,#41512,#41513,#41514,#41515,#41516,#41517,#41518,
#41519,#41520,#41521,#41522,#41523,#41524,#41525,#41526,#41527,#41528,#41529,
#41530,#41531,#41532,#41533,#41534,#41535,#41536,#41537,#41538,#41539,#41540,
#41541,#41542,#41543,#41544,#41545,#41546,#41547,#41548,#41549,#41550,#41551,
#41552,#41553,#41554,#41555,#41556,#41557,#41558,#41559,#41560,#41561,#41562,
#41563,#41564,#41565,#41566,#41567,#41568,#41569,#41570,#41571,#41572,#41573,
#41574,#41575,#41576,#41577,#41578,#41579,#41580,#41581,#41582,#41583,#41584,
#41585,#41586,#41587,#41588,#41589,#41590,#41591,#41592,#41593,#41594,#41595,
#41596,#41597,#41598,#41599,#41600,#41601,#41602,#41603,#41604,#41605,#41606,
#41607,#41608,#41609,#41610,#41611,#41612,#41613,#41614,#41615,#41616,#41617,
#41618,#41619,#41620,#41621,#41622,#41623,#41624,#41625,#41626,#41627,#41628,
#41629,#41630,#41631,#41632,#41633,#41634,#41635,#41636,#41637,#41638,#41639,
#41640,#41641,#41642,#41643,#41644,#41645,#41646,#41647,#41648,#41649,#41650,
#41651,#41652,#41653,#41654,#41655,#41656,#41657,#41658,#41659,#41660,#41661,
#41662,#41663,#41664,#41665,#41666,#41667,#41668,#41669,#41670,#41671,#41672,
#41673,#41674,#41675,#41676,#41677,#41678,#41679,#41680,#41681,#41682,#41683,
#41684,#41685,#41686,#41687,#41688,#41689,#41690,#41691,#41692,#41693,#41694,
#41695,#41696,#41697,#41698,#41699,#41700,#41701,#41702,#41703,#41704,#41705,
#41706,#41707,#41708,#41709,#41710,#41711,#41712,#41713,#41714,#41715,#41716,
#41717,#41718,#41719,#41720,#41721,#41722,#41723,#41724,#41725,#41726,#41727,
#41728,#41729,#41730,#41731,#41732,#41733,#41734,#41735,#41736,#41737,#41738,
#41739,#41740,#41741,#41742,#41743,#41744,#41745,#41746,#41747,#41748,#41749,
#41750,#41751,#41752,#41753,#41754,#41755,#41756,#41757,#41758,#41759,#41760,
#41761,#41762,#41763,#41764,#41765,#41766,#41767,#41768,#41769,#41770,#41771,
#41772,#41773,#41774,#41775,#41776,#41777,#41778,#41779,#41780,#41781,#41782,
#41783,#41784,#41785,#41786,#41787,#41788,#41789,#41790,#41791,#41792,#41793,
#41794,#41795,#41796,#41797,#41798,#41799,#41800,#41801),.UNSPECIFIED.,
 .F.,.F.,(4,2,2,2,2,2,2,2,2,2,2,2,2,2,2,2,2,2,2,2,2,2,2,2,2,2,2,2,2,2,2,
2,2,2,2,2,2,2,2,2,2,2,2,2,2,2,2,2,2,2,2,2,2,2,2,2,2,2,2,2,2,2,2,2,2,2,2,
2,2,2,2,2,2,2,2,2,2,2,2,2,2,2,2,2,2,2,2,2,2,2,2,2,2,2,2,2,2,2,2,2,2,2,2,
2,2,2,2,2,2,2,2,2,2,2,2,2,2,2,2,2,2,2,2,2,2,2,2,2,2,2,2,2,2,2,2,2,2,2,2,
2,2,2,2,2,2,2,2,2,2,2,2,2,2,2,4),(-0.786310854402765,-0.777462697274128,
-0.774578872863381,-0.771825253196008,-0.768585597468488,-0.759993654801992,
-0.752727637017471,-0.7463579158524,-0.744896183621603,-0.743748465546371,
-0.742575316626439,-0.741396655378143,-0.739243693561859,-0.729650287374014,
-0.719309564515478,-0.713515223997535,-0.709308158995403,-0.705651448980889,
-0.701940572141836,-0.697184946732764,-0.689928898172377,-0.675431880047376,
-0.667047856015395,-0.661931638796638,-0.661855545681514,-0.661787040240191,
-0.66172535466873,-0.661669797262891,-0.661619745923069,-0.661574641880017,
-0.661533983714326,-0.661497321699181,-0.66146425256561,-0.661434414874798,
-0.661407484600269,-0.661383171233308,-0.66136121431376,-0.661341380105068,
-0.661323458728828,-0.661307261727949,-0.661292619899717,-0.661242260347798,
-0.661193672018736,-0.661146774937757,-0.661101492920444,-0.660256710115307,
-0.660237022592094,-0.660217738911895,-0.660198840980835,-0.660180311218699,
-0.660162132911044,-0.660144290023941,-0.660126766947141,-0.660109548839258,
-0.660092621243659,-0.660075970239275,-0.660059582355764,-0.660043444656213,
-0.660027544568104,-0.660011869881863,-0.659996408737286,-0.659981149545176,
-0.659966081292558,-0.659951193024744,-0.65993647410584,-0.659921913985125,
-0.658343782751553,-0.656773017784948,-0.654567106743606,-0.647058060570245,
-0.639120195852277,-0.63528599385772,-0.634149487673151,-0.633089154912727,
-0.632295462749806,-0.630410887711222,-0.622332241191278,-0.616425079464459,
-0.613304633882996,-0.613259122205537,-0.613116914942923,-0.612985080125594,
-0.6128625987091,-0.612748553021981,-0.612642116711313,-0.612542545427062,
-0.612449168349521,-0.612361380429204,-0.612278635424558,-0.612200439406071,
-0.612126344955206,-0.612055945993218,-0.611988872963505,-0.611924788505522,
-0.611863383584545,-0.611804373914465,-0.61174749668639,-0.611692507596376,
-0.611639177998426,-0.611587292280063,-0.611536645440485,-0.611487040473534,
-0.611438286141007,-0.611390194205315,-0.611342577007589,-0.611295244644771,
-0.609030554233093,-0.606771899712746,-0.602625644752582,-0.58350798549645,
-0.573412898727784,-0.568397100365427,-0.565069075724267,-0.564230906277338,
-0.5619812954031,-0.559213833044693,-0.554692116549716,-0.54296895675803,
-0.533313904284,-0.529881127000282,-0.528101707580342,-0.526672538331252,
-0.525674820049849,-0.524770311635361,-0.523580015442259,-0.521028765004709,
-0.509643894233779,-0.496661773228539,-0.490823463523767,-0.487536687466684,
-0.485315312582905,-0.483494100654152,-0.481615236879797,-0.479353551751606,
-0.475409067681439,-0.460110760829431,-0.448244360047109,-0.444342287175839,
-0.442375723309685,-0.441140763404031,-0.440041468532887,-0.439091864624069,
-0.437996200865361,-0.43614029059331,-0.427858512292576,-0.426819130476898,
-0.426163596147315,-0.415092050513689,-0.409588944069834,-0.405922479428505,
-0.402998655796344,-0.40005364938589,-0.397380628838706,-0.393164021180743,
-0.393155650627907),.UNSPECIFIED.) ;
#3337=B_SPLINE_CURVE_WITH_KNOTS('',3,(#41803,#41804,#41805,#41806,#41807,
#41808,#41809,#41810,#41811,#41812,#41813,#41814,#41815,#41816,#41817,#41818,
#41819,#41820,#41821,#41822,#41823,#41824,#41825,#41826,#41827,#41828,#41829,
#41830,#41831,#41832,#41833,#41834,#41835,#41836,#41837,#41838,#41839,#41840,
#41841,#41842,#41843,#41844,#41845,#41846,#41847,#41848,#41849,#41850,#41851,
#41852,#41853,#41854,#41855,#41856,#41857,#41858,#41859,#41860,#41861,#41862,
#41863,#41864,#41865,#41866,#41867,#41868,#41869,#41870,#41871,#41872,#41873,
#41874,#41875,#41876,#41877,#41878,#41879,#41880,#41881,#41882,#41883,#41884,
#41885,#41886,#41887,#41888,#41889,#41890,#41891,#41892,#41893,#41894,#41895,
#41896,#41897,#41898,#41899,#41900,#41901,#41902,#41903,#41904,#41905,#41906,
#41907,#41908,#41909,#41910,#41911,#41912,#41913,#41914,#41915,#41916,#41917,
#41918,#41919,#41920,#41921,#41922,#41923,#41924,#41925,#41926,#41927,#41928,
#41929,#41930,#41931,#41932,#41933,#41934,#41935,#41936,#41937,#41938,#41939,
#41940,#41941,#41942,#41943,#41944,#41945,#41946,#41947,#41948,#41949,#41950,
#41951,#41952,#41953,#41954,#41955,#41956,#41957,#41958,#41959,#41960,#41961,
#41962,#41963,#41964,#41965,#41966,#41967,#41968,#41969,#41970,#41971,#41972,
#41973,#41974,#41975,#41976,#41977,#41978,#41979,#41980,#41981,#41982,#41983,
#41984,#41985,#41986,#41987,#41988,#41989,#41990,#41991,#41992,#41993,#41994,
#41995,#41996,#41997,#41998,#41999,#42000,#42001,#42002,#42003,#42004,#42005,
#42006,#42007,#42008,#42009,#42010,#42011,#42012,#42013,#42014,#42015,#42016,
#42017,#42018,#42019,#42020,#42021,#42022,#42023,#42024,#42025,#42026,#42027,
#42028,#42029,#42030,#42031,#42032,#42033,#42034,#42035,#42036,#42037,#42038,
#42039,#42040,#42041,#42042,#42043,#42044,#42045,#42046,#42047,#42048,#42049,
#42050,#42051,#42052,#42053,#42054,#42055,#42056,#42057,#42058,#42059,#42060,
#42061,#42062,#42063,#42064,#42065,#42066,#42067,#42068,#42069,#42070,#42071,
#42072,#42073,#42074,#42075,#42076,#42077,#42078,#42079,#42080,#42081,#42082,
#42083,#42084,#42085,#42086,#42087,#42088,#42089,#42090,#42091,#42092,#42093,
#42094,#42095,#42096,#42097,#42098,#42099,#42100,#42101,#42102,#42103,#42104,
#42105,#42106,#42107,#42108,#42109,#42110,#42111,#42112,#42113,#42114,#42115,
#42116,#42117,#42118,#42119,#42120,#42121,#42122,#42123,#42124,#42125,#42126,
#42127,#42128,#42129,#42130,#42131,#42132,#42133,#42134,#42135,#42136,#42137,
#42138,#42139,#42140,#42141,#42142,#42143,#42144,#42145,#42146,#42147,#42148,
#42149,#42150,#42151,#42152,#42153,#42154,#42155,#42156,#42157,#42158,#42159,
#42160,#42161,#42162,#42163,#42164,#42165,#42166,#42167,#42168,#42169,#42170,
#42171,#42172,#42173,#42174,#42175,#42176,#42177,#42178,#42179,#42180,#42181,
#42182,#42183,#42184,#42185,#42186,#42187,#42188,#42189,#42190,#42191,#42192,
#42193,#42194,#42195,#42196,#42197,#42198,#42199,#42200,#42201,#42202,#42203,
#42204,#42205,#42206,#42207,#42208,#42209,#42210,#42211,#42212,#42213,#42214,
#42215,#42216,#42217,#42218,#42219,#42220,#42221,#42222,#42223,#42224,#42225,
#42226,#42227,#42228,#42229,#42230,#42231,#42232,#42233,#42234,#42235,#42236,
#42237,#42238,#42239,#42240,#42241,#42242,#42243,#42244,#42245,#42246,#42247,
#42248,#42249,#42250,#42251,#42252,#42253,#42254,#42255,#42256,#42257,#42258,
#42259,#42260,#42261,#42262,#42263,#42264,#42265,#42266,#42267,#42268,#42269,
#42270,#42271,#42272,#42273,#42274,#42275,#42276,#42277,#42278,#42279,#42280,
#42281,#42282,#42283,#42284,#42285,#42286,#42287,#42288,#42289,#42290,#42291,
#42292,#42293,#42294,#42295,#42296,#42297,#42298,#42299,#42300,#42301,#42302,
#42303,#42304,#42305,#42306,#42307,#42308,#42309,#42310,#42311,#42312,#42313,
#42314,#42315,#42316,#42317,#42318,#42319,#42320,#42321,#42322,#42323,#42324,
#42325,#42326,#42327,#42328,#42329,#42330,#42331,#42332,#42333,#42334,#42335,
#42336,#42337,#42338,#42339,#42340,#42341,#42342,#42343,#42344,#42345,#42346,
#42347,#42348,#42349,#42350,#42351,#42352,#42353,#42354,#42355,#42356,#42357,
#42358,#42359,#42360,#42361,#42362,#42363,#42364,#42365,#42366,#42367,#42368,
#42369,#42370,#42371,#42372,#42373,#42374,#42375,#42376,#42377,#42378,#42379,
#42380,#42381,#42382,#42383,#42384,#42385,#42386,#42387,#42388,#42389,#42390,
#42391,#42392,#42393,#42394,#42395,#42396,#42397,#42398,#42399,#42400,#42401,
#42402,#42403,#42404,#42405,#42406,#42407,#42408,#42409,#42410,#42411,#42412,
#42413,#42414,#42415,#42416,#42417,#42418,#42419,#42420,#42421,#42422,#42423,
#42424,#42425,#42426,#42427,#42428,#42429,#42430,#42431,#42432,#42433,#42434,
#42435,#42436,#42437,#42438,#42439,#42440,#42441,#42442,#42443,#42444,#42445,
#42446,#42447,#42448,#42449,#42450,#42451,#42452,#42453,#42454,#42455,#42456),
 .UNSPECIFIED.,.F.,.F.,(4,2,2,2,2,2,2,2,2,2,2,2,2,2,2,2,2,2,2,2,2,2,2,2,
2,2,2,2,2,2,2,2,2,2,2,2,2,2,2,2,2,2,2,2,2,2,2,2,2,2,2,2,2,2,2,2,2,2,2,2,
2,2,2,2,2,2,2,2,2,2,2,2,2,2,2,2,2,2,2,2,2,2,2,2,2,2,2,2,2,2,2,2,2,2,2,2,
2,2,2,2,2,2,2,2,2,2,2,2,2,2,2,2,2,2,2,2,2,2,2,2,2,2,2,2,2,2,2,2,2,2,2,2,
2,2,2,2,2,2,2,2,2,2,2,2,2,2,2,2,2,2,2,2,2,2,2,2,2,2,2,2,2,2,2,2,2,2,2,2,
2,2,2,2,2,2,2,2,2,2,2,2,2,2,2,2,2,2,2,2,2,2,2,2,2,2,2,2,2,2,2,2,2,2,2,2,
2,2,2,2,2,2,2,2,2,2,2,2,2,2,2,2,2,2,2,2,2,2,2,2,2,2,2,2,2,2,2,2,2,2,2,2,
2,2,2,2,2,2,2,2,2,2,2,2,2,2,2,2,2,2,2,2,2,2,2,2,2,2,2,2,2,2,2,2,2,2,2,2,
2,2,2,2,2,2,2,2,2,2,2,2,2,2,2,2,2,2,2,2,2,2,2,2,2,2,2,2,2,2,2,2,2,2,2,2,
2,2,2,2,2,2,2,2,2,2,2,2,2,2,4),(-0.393065589708965,-0.388966566095848,-0.383448746522827,
-0.376179753135169,-0.374191610189867,-0.374158237312468,-0.374135335710637,
-0.374114778741838,-0.374096326457447,-0.37407976325486,-0.374064895468,
-0.374052707000776,-0.374040843322002,-0.374029295564849,-0.374018055142535,
-0.37400711363893,-0.373996462896227,-0.373986094955537,-0.373976002159433,
-0.373966176968725,-0.373956612117498,-0.373947300479584,-0.373938235136589,
-0.373929409439409,-0.373920816821315,-0.373912450941929,-0.373904305666952,
-0.373896374972697,-0.373888653100104,-0.373881134329663,-0.373873813111811,
-0.373866684166782,-0.373860607584359,-0.373854573307737,-0.373848580835059,
-0.373842629926712,-0.373836720268857,-0.373830851509131,-0.373825023272392,
-0.373819235235161,-0.373813487086501,-0.373807778489716,-0.373802109135364,
-0.373796478691675,-0.373790886896402,-0.373785333367384,-0.373779817875267,
-0.373774340096372,-0.373768899680037,-0.373763496322769,-0.37375812978838,
-0.373752799775776,-0.373747505962267,-0.373742248096514,-0.373737025860778,
-0.373731838925717,-0.373726687062818,-0.373721569958284,-0.373716487431612,
-0.373711439097369,-0.373706424692151,-0.37370144397626,-0.373696496687196,
-0.373691582474535,-0.37368670118131,-0.373681852575176,-0.373677036273045,
-0.37367225212438,-0.373667499855715,-0.37366277918764,-0.373658089812767,
-0.373653431609658,-0.37364880421959,-0.373644207441387,-0.37363964110511,
-0.373635104865037,-0.373630598506484,-0.373626121825299,-0.373621674617905,
-0.373617256638368,-0.373612867642864,-0.373608507324453,-0.373604175512244,
-0.373599872088644,-0.373595596695155,-0.373591349100151,-0.373587129240475,
-0.373582936840201,-0.373578771687893,-0.373574633522961,-0.373570522099672,
-0.373566437263598,-0.373562378858738,-0.373558346621176,-0.37355434033864,
-0.373550359894408,-0.373546404978224,-0.373542475498692,-0.373538571202167,
-0.373534691880213,-0.373530837433716,-0.373527007687636,-0.373523202332135,
-0.373519421188301,-0.373515664008997,-0.371762372943665,-0.367585412427757,
-0.358613561453349,-0.352598337538184,-0.349970187718555,-0.349783763189994,
-0.349399873062088,-0.348443704439419,-0.348420198822344,-0.348398319008721,
-0.348377956190562,-0.346350426019905,-0.342846265948606,-0.33837561685244,
-0.323747138385486,-0.314628245737323,-0.303306470593153,-0.29761714021614,
-0.29751154058311,-0.297420043127292,-0.297340718720898,-0.297271910531709,
-0.297212194441151,-0.297160345241728,-0.297115307808145,-0.297005477530411,
-0.296899735717524,-0.296797879150421,-0.296699715967274,-0.296605065040454,
-0.296513755385228,-0.296425625561051,-0.296340523124463,-0.296258304111954,
-0.296178832569933,-0.296101980046967,-0.291688624157727,-0.287195888750989,
-0.280948704889126,-0.270198282438431,-0.267725595730619,-0.266255559945261,
-0.265102789113086,-0.263494144148679,-0.261728698969323,-0.258807088843284,
-0.25228863854667,-0.243580587869969,-0.240698578544022,-0.239321581938187,
-0.23823237340428,-0.237044660585399,-0.237040800982266,-0.237036934285919,
-0.23703306143964,-0.237029181853243,-0.237025295974021,-0.237021403755482,
-0.237017504634154,-0.237013599004515,-0.237009686534246,-0.237005767298947,
-0.237001841459152,-0.236997908635496,-0.236993968801003,-0.236990021739105,
-0.236986067654262,-0.236982106044023,-0.236978137342861,-0.236974161392018,
-0.23697017760217,-0.236966186281581,-0.23696218752544,-0.236958181222895,
-0.236954166974552,-0.23695014457853,-0.236946114306944,-0.236942076447991,
-0.236938030398093,-0.236933975907316,-0.236929912896609,-0.236925841365424,
-0.236921761508152,-0.236917673035839,-0.236913575943062,-0.236909470398506,
-0.236905355729577,-0.236901231847539,-0.236897099020933,-0.236892957094873,
-0.236888806195107,-0.236884645778026,-0.236880475992086,-0.236876296995416,
-0.236872107931012,-0.236867909171639,-0.236863701105506,-0.236859483371062,
-0.236855255499268,-0.236851017540101,-0.236846769356363,-0.236842511046265,
-0.236838242439205,-0.236833963293048,-0.23682967368968,-0.236825373304639,
-0.236821062388024,-0.236816740610951,-0.236812407982378,-0.236808064449367,
-0.236803709763215,-0.236799343749095,-0.236794966459936,-0.236790577909174,
-0.236786177609795,-0.236781765590968,-0.23677734198399,-0.236772906440799,
-0.236768459118643,-0.236763999450378,-0.236759527756641,-0.236755043949369,
-0.236750547798447,-0.236746039176336,-0.236741517915517,-0.23673698380523,
-0.23673243739724,-0.236727877973662,-0.236723305538348,-0.236718719816909,
-0.236714120437942,-0.236709507749938,-0.236704881494466,-0.23670024166752,
-0.236695588310455,-0.236690921045407,-0.236686240032755,-0.236681544736176,
-0.236676835247036,-0.235042424229185,-0.232085425740897,-0.221287541399645,
-0.219367323172205,-0.217301279783494,-0.210208222778234,-0.205932429359203,
-0.203111120439414,-0.199409758631995,-0.195007879852957,-0.189557019084433,
-0.187373499785273,-0.186489280858067,-0.186279454516391,-0.184275899608854,
-0.181927580489253,-0.177430693699789,-0.169025708425269,-0.162822605197181,
-0.159080604885825,-0.158224549345706,-0.158068265860158,-0.157746773017292,
-0.157485494790619,-0.157270578554057,-0.157091971577553,-0.156942232166822,
-0.156815749634271,-0.151620017481765,-0.146505313209591,-0.13770255809697,
-0.13360939923471,-0.129750206181053,-0.120875262469577,-0.114559186246218,
-0.113039759143288,-0.111359459678535,-0.111298677526727,-0.111244279657613,
-0.111195464270134,-0.111151549741104,-0.111111953849125,-0.111076177036546,
-0.111043788777336,-0.111014416324963,-0.110987735641776,-0.110963464046509,
-0.110941353812947,-0.110921187251175,-0.109180491091203,-0.107596966103121,
-0.102160409383009,-0.0942720035046282,-0.0912491998483847,-0.088868421435765,
-0.0853546399509588,-0.0811656674535144,-0.0703065043256505,-0.0680660783932548,
-0.0667589626736305,-0.0651824959318863,-0.062996302784368,-0.0575869508532417,
-0.0535188263621436,-0.051050432989073,-0.0487233765368177,-0.0471473950526166,
-0.0441655697277461,-0.0359017938579531,-0.0339314541286829,-0.0324758421304942,
-0.0308070834985168,-0.0290307014167538,-0.0262848070699855,-0.0228410082915044,
-0.0151658803392792,-0.0136856958442221,-0.0128656229705687,-0.0120507563698123,
-0.0112427406305335,-0.0102043876099121,-0.00839362727804128,-1.00000003522283E-6),
 .UNSPECIFIED.) ;
#3338=B_SPLINE_CURVE_WITH_KNOTS('',3,(#42457,#42458,#42459,#42460,#42461,
#42462,#42463,#42464,#42465,#42466,#42467,#42468,#42469,#42470,#42471,#42472,
#42473,#42474,#42475,#42476,#42477,#42478,#42479,#42480,#42481,#42482,#42483,
#42484,#42485,#42486,#42487,#42488,#42489,#42490,#42491,#42492,#42493,#42494,
#42495,#42496,#42497,#42498,#42499,#42500,#42501,#42502,#42503,#42504,#42505,
#42506,#42507,#42508,#42509,#42510,#42511,#42512,#42513,#42514,#42515,#42516,
#42517,#42518,#42519,#42520),.UNSPECIFIED.,.F.,.F.,(4,3,3,3,3,3,3,3,3,3,
3,3,3,3,3,3,3,3,3,3,3,4),(0.,0.194611379569939,0.413105731031986,0.631646549932974,
0.984685058974708,1.0681572847997,1.2854939556078,1.50413078441806,1.72074571686338,
1.93938203882708,1.96857224711482,2.15652830010514,2.37516406745792,2.59283702522495,
2.80932989456835,2.95242475684296,3.0277774580989,3.24484714263336,3.46348192766738,
3.68172528565085,3.89858695415034,3.93630690328113),.UNSPECIFIED.) ;
#3339=B_SPLINE_CURVE_WITH_KNOTS('',3,(#42524,#42525,#42526,#42527,#42528,
#42529,#42530,#42531,#42532,#42533,#42534,#42535,#42536),.UNSPECIFIED.,
 .F.,.F.,(4,3,2,2,2,4),(-0.00235052512319675,0.,0.0113491260853101,0.0226982521706202,
0.034046050040237,0.0453938479098539),.UNSPECIFIED.) ;
#3340=B_SPLINE_CURVE_WITH_KNOTS('',3,(#42538,#42539,#42540,#42541,#42542,
#42543,#42544,#42545,#42546,#42547,#42548,#42549,#42550,#42551,#42552,#42553,
#42554,#42555,#42556,#42557,#42558,#42559,#42560,#42561,#42562,#42563,#42564,
#42565,#42566,#42567,#42568,#42569,#42570,#42571,#42572,#42573,#42574,#42575,
#42576,#42577,#42578,#42579,#42580,#42581,#42582,#42583,#42584,#42585,#42586,
#42587,#42588,#42589,#42590,#42591,#42592,#42593,#42594,#42595,#42596,#42597,
#42598,#42599,#42600,#42601,#42602,#42603,#42604,#42605,#42606,#42607,#42608,
#42609,#42610,#42611,#42612,#42613,#42614,#42615,#42616,#42617,#42618,#42619,
#42620,#42621,#42622,#42623,#42624,#42625,#42626,#42627,#42628,#42629,#42630,
#42631,#42632,#42633,#42634,#42635,#42636,#42637,#42638,#42639,#42640,#42641,
#42642,#42643,#42644,#42645,#42646,#42647,#42648,#42649,#42650,#42651,#42652,
#42653,#42654,#42655,#42656,#42657,#42658,#42659,#42660,#42661,#42662,#42663,
#42664,#42665,#42666,#42667,#42668,#42669,#42670,#42671,#42672,#42673,#42674,
#42675,#42676,#42677,#42678,#42679,#42680,#42681,#42682,#42683,#42684,#42685,
#42686,#42687,#42688,#42689,#42690,#42691,#42692,#42693,#42694,#42695,#42696,
#42697,#42698,#42699,#42700,#42701,#42702,#42703,#42704,#42705,#42706,#42707,
#42708,#42709,#42710,#42711,#42712,#42713,#42714,#42715,#42716,#42717,#42718,
#42719,#42720,#42721,#42722,#42723,#42724,#42725,#42726,#42727,#42728,#42729,
#42730,#42731,#42732,#42733,#42734,#42735,#42736,#42737,#42738,#42739,#42740,
#42741,#42742,#42743,#42744,#42745,#42746,#42747,#42748,#42749,#42750,#42751,
#42752,#42753,#42754,#42755,#42756,#42757,#42758,#42759,#42760,#42761,#42762,
#42763,#42764,#42765,#42766,#42767,#42768,#42769,#42770,#42771,#42772,#42773,
#42774,#42775,#42776,#42777,#42778,#42779,#42780,#42781,#42782,#42783,#42784,
#42785,#42786,#42787,#42788,#42789,#42790,#42791,#42792,#42793,#42794,#42795,
#42796,#42797,#42798,#42799,#42800,#42801,#42802,#42803,#42804,#42805,#42806,
#42807,#42808,#42809,#42810,#42811,#42812,#42813,#42814,#42815,#42816,#42817,
#42818,#42819,#42820,#42821,#42822,#42823,#42824,#42825,#42826,#42827,#42828,
#42829,#42830,#42831,#42832,#42833,#42834,#42835,#42836,#42837,#42838,#42839,
#42840,#42841,#42842,#42843,#42844,#42845,#42846,#42847,#42848,#42849,#42850,
#42851,#42852,#42853,#42854,#42855,#42856,#42857,#42858,#42859,#42860,#42861,
#42862,#42863,#42864,#42865,#42866,#42867,#42868,#42869,#42870,#42871,#42872,
#42873,#42874,#42875,#42876,#42877,#42878,#42879,#42880,#42881,#42882,#42883,
#42884,#42885,#42886,#42887,#42888,#42889,#42890,#42891,#42892,#42893,#42894,
#42895,#42896,#42897,#42898,#42899,#42900,#42901,#42902,#42903,#42904,#42905,
#42906,#42907,#42908,#42909,#42910,#42911,#42912,#42913,#42914,#42915,#42916,
#42917,#42918,#42919,#42920,#42921,#42922,#42923,#42924,#42925,#42926,#42927,
#42928,#42929,#42930,#42931),.UNSPECIFIED.,.F.,.F.,(4,2,2,2,2,2,2,2,2,2,
2,2,2,2,2,2,2,2,2,2,2,2,2,2,2,2,2,2,2,2,2,2,2,2,2,2,2,2,2,2,2,2,2,2,2,2,
2,2,2,2,2,2,2,2,2,2,2,2,2,2,2,2,2,2,2,2,2,2,2,2,2,2,2,2,2,2,2,2,2,2,2,2,
2,2,2,2,2,2,2,2,2,2,2,2,2,2,2,2,2,2,2,2,2,2,2,2,2,2,2,2,2,2,2,2,2,2,2,2,
2,2,2,2,2,2,2,2,2,2,2,2,2,2,2,2,2,2,2,2,2,2,2,2,2,2,2,2,2,2,2,2,2,2,2,2,
2,2,2,2,2,2,2,2,2,2,2,2,2,2,2,2,2,2,2,2,2,2,2,2,2,2,2,2,2,2,2,2,2,2,2,2,
2,2,2,2,2,2,4),(-0.338631569254744,-0.336734654040014,-0.334665307627351,
-0.325963066244536,-0.324026710452822,-0.322380662939139,-0.320388042855082,
-0.314253169168998,-0.311839994745291,-0.310214874905825,-0.308693228330123,
-0.307237952438348,-0.305185045258803,-0.298034605265837,-0.293405752588105,
-0.290428016768423,-0.289077367253203,-0.28796560372676,-0.286852955957451,
-0.284806427012391,-0.274926628259733,-0.271422900114645,-0.269729797054094,
-0.268657672992355,-0.267816313919124,-0.266952036340973,-0.266079447166832,
-0.264447264494238,-0.257570040233546,-0.252592203538653,-0.250216384988825,
-0.248700949561993,-0.248632464842557,-0.248568481034681,-0.248508631189948,
-0.248452576601431,-0.24840000531737,-0.248350630439625,-0.248304188574536,
-0.248260438055414,-0.248219157208751,-0.248180142845309,-0.248143208779721,
-0.248108184287919,-0.248074912796556,-0.24804325071982,-0.248013066120397,
-0.247984237858192,-0.247956654237224,-0.247930212389863,-0.247904817474043,
-0.247880381581244,-0.24785682312758,-0.247834066309284,-0.24781204061228,
-0.247790679923397,-0.247769922152786,-0.247749708861411,-0.247729984556913,
-0.246507560424402,-0.24509133284851,-0.242593824359581,-0.235999289760559,
-0.232926352893635,-0.230688043389769,-0.228517290840238,-0.227039427442087,
-0.219388666888622,-0.217665456719758,-0.217019247371198,-0.216676122635613,
-0.216319358125661,-0.21470742327233,-0.213094110076598,-0.206648321242796,
-0.203826866646343,-0.202141702601408,-0.200788110338928,-0.199645563913887,
-0.197964777160737,-0.194655651619069,-0.186005871621098,-0.183252900996211,
-0.18169874370884,-0.180697396005963,-0.1806889464537,-0.180680594203109,
-0.180672336985844,-0.180664172571408,-0.180656098583319,-0.180648112706023,
-0.180640212914428,-0.180632396970588,-0.180624663069236,-0.180617008915489,
-0.180609432678236,-0.180601932391217,-0.180594505992267,-0.180587151886344,
-0.180579867992514,-0.180572652375439,-0.180565503195765,-0.180558418705696,
-0.180551397343621,-0.180544437198527,-0.180537536934857,-0.1805306943673,
-0.180523907902386,-0.18051717611988,-0.180510497480495,-0.180503870227966,
-0.180497293018481,-0.180490764023599,-0.180484281594919,-0.180477844687277,
-0.180471451615318,-0.180465100943189,-0.180458791043372,-0.180452520351895,
-0.180446287768797,-0.180440091869983,-0.180433931188036,-0.180427804187668,
-0.180421709398241,-0.180415645806202,-0.180409611787812,-0.180403605757985,
-0.180397626779217,-0.180391673454889,-0.180385744113069,-0.180379837431095,
-0.18037395189779,-0.180368086410412,-0.180362239526999,-0.180356409940254,
-0.179302518753018,-0.178256366520431,-0.176428224520422,-0.169274085184775,
-0.160721521229079,-0.15926326782659,-0.158400178395906,-0.157693395568019,
-0.156881584995432,-0.15590972122208,-0.154367141469796,-0.151240750842007,
-0.146109134458849,-0.139316786451658,-0.137868408683809,-0.137073205141669,
-0.136282115590371,-0.135380397820905,-0.133553731398204,-0.131159020760954,
-0.124761979671465,-0.123705062809495,-0.12237947135262,-0.117498075480047,
-0.116125649359041,-0.115350727199907,-0.11460597602389,-0.113633192853416,
-0.112559082792293,-0.110778577105945,-0.106872228035098,-0.0943360832791758,
-0.0919864445405689,-0.0905627277180745,-0.0893105960214068,-0.0878491374722877,
-0.0847657690986667,-0.0804642266826064,-0.0673398015862877,-0.0635702031269495,
-0.0616708223826233,-0.0604348086240259,-0.0593643263936798,-0.0570968745149313,
-0.0544573924190736,-0.0493100487068456,-0.0414061098843744,-0.0409465848615722,
-0.0358095315760844,-0.0335776201567591,-0.0318756311788981,-0.0302486677193898,
-0.0283707910132205,-0.0227320356787229,-0.014755322969727,-0.00882146644314774,
-0.00702341351978558,-0.00596810267110615,-0.00504964345917795,-0.00413109953237996,
-0.00245627375521964,-1.35388579686318E-6),.UNSPECIFIED.) ;
#3341=B_SPLINE_CURVE_WITH_KNOTS('',3,(#42933,#42934,#42935,#42936),
 .UNSPECIFIED.,.F.,.F.,(4,4),(0.597204295884584,0.669364392781264),
 .UNSPECIFIED.) ;
#3342=B_SPLINE_CURVE_WITH_KNOTS('',3,(#42938,#42939,#42940,#42941,#42942,
#42943,#42944,#42945,#42946,#42947,#42948,#42949,#42950,#42951,#42952,#42953,
#42954,#42955,#42956,#42957,#42958,#42959,#42960,#42961,#42962,#42963,#42964,
#42965,#42966,#42967,#42968,#42969,#42970,#42971,#42972,#42973,#42974,#42975,
#42976,#42977,#42978,#42979,#42980,#42981,#42982,#42983,#42984,#42985,#42986,
#42987,#42988,#42989,#42990,#42991,#42992,#42993,#42994,#42995,#42996,#42997,
#42998,#42999,#43000,#43001,#43002,#43003,#43004,#43005,#43006,#43007,#43008,
#43009,#43010,#43011,#43012,#43013,#43014,#43015,#43016,#43017,#43018,#43019,
#43020,#43021,#43022,#43023,#43024,#43025,#43026,#43027,#43028,#43029,#43030,
#43031,#43032,#43033,#43034,#43035,#43036,#43037,#43038,#43039,#43040,#43041,
#43042,#43043,#43044,#43045,#43046,#43047,#43048,#43049,#43050,#43051,#43052,
#43053,#43054,#43055,#43056,#43057,#43058,#43059,#43060,#43061,#43062,#43063,
#43064,#43065,#43066,#43067,#43068,#43069,#43070,#43071,#43072,#43073,#43074,
#43075,#43076,#43077,#43078,#43079,#43080,#43081,#43082,#43083,#43084,#43085,
#43086,#43087,#43088,#43089,#43090,#43091,#43092,#43093,#43094,#43095,#43096,
#43097,#43098,#43099,#43100,#43101,#43102,#43103,#43104,#43105,#43106,#43107,
#43108,#43109,#43110,#43111,#43112,#43113,#43114,#43115,#43116,#43117,#43118,
#43119,#43120,#43121,#43122,#43123,#43124,#43125,#43126,#43127,#43128,#43129,
#43130,#43131,#43132,#43133,#43134,#43135,#43136,#43137,#43138,#43139,#43140,
#43141,#43142,#43143,#43144,#43145,#43146,#43147,#43148,#43149,#43150,#43151,
#43152,#43153,#43154,#43155,#43156,#43157,#43158,#43159,#43160,#43161,#43162,
#43163,#43164,#43165,#43166,#43167,#43168,#43169,#43170,#43171,#43172,#43173,
#43174,#43175,#43176,#43177,#43178,#43179,#43180,#43181,#43182,#43183,#43184,
#43185,#43186,#43187,#43188,#43189,#43190,#43191,#43192,#43193,#43194,#43195,
#43196,#43197,#43198,#43199,#43200,#43201,#43202,#43203,#43204,#43205,#43206,
#43207,#43208,#43209,#43210,#43211,#43212,#43213,#43214,#43215),
 .UNSPECIFIED.,.F.,.F.,(4,2,2,2,2,2,2,2,2,2,2,2,2,2,2,2,2,2,2,2,2,2,2,2,
2,2,2,2,2,2,2,2,2,2,2,2,2,2,2,2,2,2,2,2,2,2,2,2,2,2,2,2,2,2,2,2,2,2,2,2,
2,2,2,2,2,2,2,2,2,2,2,2,2,2,2,2,2,2,2,2,2,2,2,2,2,2,2,2,2,2,2,2,2,2,2,2,
2,2,2,2,2,2,2,2,2,2,2,2,2,2,2,2,2,2,2,2,2,2,2,2,2,2,2,2,2,2,2,2,2,2,2,2,
2,2,2,2,2,2,4),(-0.255648930279346,-0.252997541914023,-0.250129508816139,
-0.244210307020476,-0.235916895314324,-0.234170956693684,-0.232581734776005,
-0.231043334138474,-0.228960848074572,-0.223018060278477,-0.217304903048903,
-0.215115149238904,-0.214045289292404,-0.213762778966205,-0.213544837882605,
-0.21267034927113,-0.211779906286584,-0.210886419354201,-0.209240569491487,
-0.200245314661032,-0.195659752547622,-0.193628747053223,-0.19199875282225,
-0.191155799364946,-0.190355763478676,-0.189321341453539,-0.187490259426295,
-0.178111063619884,-0.173947777970992,-0.172066662684669,-0.170719960522959,
-0.169907202828386,-0.169080407616088,-0.168125956034019,-0.166503868399372,
-0.159143686189377,-0.153892298833385,-0.151463180561509,-0.149957923478239,
-0.149923891593186,-0.149852516398666,-0.149787000180214,-0.149726927856389,
-0.149671902957905,-0.149621548601185,-0.149575508042802,-0.149533444910382,
-0.149495043241783,-0.149460007279618,-0.149428060969789,-0.149398947448583,
-0.149372428287741,-0.149348282727429,-0.149326306823944,-0.148216684864361,
-0.147036713161444,-0.145438572312611,-0.141547364205493,-0.133915278003247,
-0.131027999202793,-0.129244445564844,-0.127826135572844,-0.126440315731165,
-0.126372665632238,-0.126313570081502,-0.126260877382886,-0.126213119574936,
-0.12616924808184,-0.126128485907223,-0.126090239723491,-0.126054044534104,
-0.126019527514997,-0.125986383549398,-0.125954358172745,-0.12592323535276,
-0.125892828263452,-0.125862972666397,-0.125833521763597,-0.125804342006902,
-0.125775309964684,-0.125746309595708,-0.125717230067369,-0.125687963743893,
-0.125658404683168,-0.125628446977801,-0.125597983344769,-0.125566903782413,
-0.125535094159789,-0.12550243490758,-0.125468799508362,-0.125434053165129,
-0.125398051016836,-0.125360636381765,-0.125321638936169,-0.125280872491618,
-0.125238132559374,-0.125193193743492,-0.125145806626417,-0.125095694373013,
-0.12504254882899,-0.12498602602317,-0.123134106545598,-0.119878592254869,
-0.114023992805888,-0.111969741016468,-0.10916358533671,-0.10505083642492,
-0.100009585314172,-0.0968084810169616,-0.0931769772020695,-0.0889343467329334,
-0.0835736290368014,-0.0811284571804246,-0.0788395281498874,-0.076396123281033,
-0.0724625170395792,-0.0649643833672325,-0.0625961828505878,-0.060884501010045,
-0.058400734905096,-0.0550093093267712,-0.0499279043162481,-0.0484720480245992,
-0.0466014067838737,-0.0438229874809215,-0.0372914318420222,-0.03484561812626,
-0.032259227308613,-0.0307659861063578,-0.0287650324744632,-0.0222547659180821,
-0.0186956352932961,-0.0168281722189283,-0.0152082970564504,-0.0135169884610331,
-0.0111371344141474,-0.0062262270346876,-0.00219948967990509,-1.00011834170696E-6),
 .UNSPECIFIED.) ;
#3343=B_SPLINE_CURVE_WITH_KNOTS('',3,(#43219,#43220,#43221,#43222,#43223,
#43224,#43225,#43226,#43227,#43228),.UNSPECIFIED.,.F.,.F.,(4,2,2,2,4),(-0.0453938479098542,
-0.034046050040237,-0.0226982521706198,-0.0113491260853099,0.),
 .UNSPECIFIED.) ;
#3344=B_SPLINE_CURVE_WITH_KNOTS('',3,(#43230,#43231,#43232,#43233,#43234,
#43235,#43236,#43237,#43238,#43239),.UNSPECIFIED.,.F.,.F.,(4,2,2,2,4),(-0.0907876281662502,
-0.07943850588408,-0.0680893836019098,-0.056741615755882,-0.0453938479098542),
 .UNSPECIFIED.) ;
#3345=B_SPLINE_CURVE_WITH_KNOTS('',3,(#43242,#43243,#43244,#43245,#43246,
#43247,#43248,#43249,#43250,#43251),.UNSPECIFIED.,.F.,.F.,(4,2,2,2,4),(0.0453964590725441,
0.0567416157558807,0.0680893836019074,0.0794385058840781,0.0907876281662487),
 .UNSPECIFIED.) ;
#3346=B_SPLINE_CURVE_WITH_KNOTS('',3,(#50224,#50225,#50226,#50227,#50228,
#50229,#50230,#50231,#50232,#50233,#50234,#50235,#50236),.UNSPECIFIED.,
 .F.,.F.,(4,3,3,3,4),(0.00255363805101728,0.0798635693162218,0.156366831960307,
0.227369307234732,0.232870094604391),.UNSPECIFIED.) ;
#3347=B_SPLINE_CURVE_WITH_KNOTS('',3,(#50237,#50238,#50239,#50240,#50241,
#50242,#50243,#50244,#50245,#50246,#50247,#50248,#50249,#50250,#50251,#50252,
#50253,#50254,#50255,#50256,#50257,#50258,#50259,#50260,#50261,#50262,#50263,
#50264,#50265,#50266,#50267,#50268,#50269,#50270,#50271,#50272,#50273,#50274,
#50275,#50276,#50277,#50278,#50279,#50280,#50281,#50282,#50283,#50284,#50285,
#50286,#50287,#50288,#50289,#50290,#50291,#50292,#50293,#50294,#50295,#50296,
#50297,#50298,#50299,#50300,#50301,#50302,#50303),.UNSPECIFIED.,.F.,.F.,
(4,3,3,3,3,3,3,3,3,3,3,3,3,3,3,3,3,3,3,3,3,3,4),(0.827865437902793,0.969498981235656,
1.21799526332659,1.38410988280274,1.4652627416507,1.66145199561158,1.70762284974659,
1.8714343337634,1.94910512274864,2.16981834865978,2.18634162166884,2.3630091739159,
2.42204226640599,2.61858958173905,2.65392302673644,2.88181141853766,3.05474660487823,
3.10884255152698,3.28206710848474,3.33241715880223,3.53151885752025,3.55138058859422,
3.61157274718876),.UNSPECIFIED.) ;
#3348=B_SPLINE_CURVE_WITH_KNOTS('',3,(#57276,#57277,#57278,#57279,#57280,
#57281,#57282,#57283,#57284,#57285,#57286,#57287,#57288,#57289,#57290,#57291,
#57292,#57293,#57294,#57295,#57296,#57297,#57298,#57299,#57300,#57301,#57302,
#57303,#57304,#57305,#57306,#57307,#57308,#57309,#57310,#57311,#57312,#57313,
#57314,#57315,#57316,#57317,#57318,#57319),.UNSPECIFIED.,.F.,.F.,(4,2,2,
2,2,2,2,2,2,2,2,2,2,2,2,2,2,2,2,2,2,4),(0.,0.00971873963594822,0.0203964852574078,
0.0279299520213564,0.0332159680142414,0.0367507190487289,0.0382591314234756,
0.0385205125291013,0.0385320951859343,0.0385380775151796,0.0385445454156034,
0.0385477019368606,0.0385501373609749,0.0385527760503969,0.0385569787262409,
0.0385703376675416,0.0391296696114738,0.0414060512274473,0.0455043325938727,
0.051255059605876,0.0595245127263013,0.0750115373312587),.UNSPECIFIED.) ;
#3349=B_SPLINE_CURVE_WITH_KNOTS('',3,(#57321,#57322,#57323,#57324,#57325,
#57326,#57327,#57328,#57329,#57330,#57331,#57332,#57333,#57334,#57335,#57336,
#57337,#57338,#57339),.UNSPECIFIED.,.F.,.F.,(4,1,1,1,1,1,1,1,1,1,1,1,1,
1,1,1,4),(87.336489761411,87.4317045853384,87.8665778926469,88.3014512000977,
88.7363245076919,89.1711978154302,89.6060711233134,90.0409444313423,90.4758177395175,
90.9106910478396,91.345564356309,91.7804376649263,92.2153109736917,92.6501842826055,
93.085057591668,93.5199309008791,93.8817096841969),.UNSPECIFIED.) ;
#3350=B_SPLINE_CURVE_WITH_KNOTS('',3,(#57341,#57342,#57343,#57344,#57345,
#57346),.UNSPECIFIED.,.F.,.F.,(4,2,4),(-0.022111302478061,-0.0110566426887937,
-1.0000840920775E-6),.UNSPECIFIED.) ;
#3351=B_SPLINE_CURVE_WITH_KNOTS('',3,(#57347,#57348,#57349,#57350,#57351,
#57352),.UNSPECIFIED.,.F.,.F.,(4,2,4),(9.99929897944746E-7,0.014189921283727,
0.0275689001028884),.UNSPECIFIED.) ;
#3352=B_SPLINE_CURVE_WITH_KNOTS('',3,(#57353,#57354,#57355,#57356,#57357,
#57358,#57359,#57360,#57361,#57362,#57363,#57364,#57365,#57366,#57367,#57368,
#57369,#57370,#57371,#57372,#57373,#57374,#57375,#57376,#57377,#57378,#57379,
#57380,#57381,#57382,#57383,#57384,#57385,#57386,#57387,#57388,#57389,#57390,
#57391,#57392,#57393,#57394,#57395,#57396,#57397,#57398,#57399,#57400,#57401,
#57402,#57403,#57404,#57405,#57406,#57407,#57408,#57409,#57410,#57411,#57412,
#57413,#57414,#57415,#57416,#57417,#57418,#57419,#57420,#57421,#57422,#57423,
#57424,#57425,#57426,#57427,#57428,#57429,#57430,#57431,#57432,#57433,#57434,
#57435,#57436,#57437,#57438,#57439,#57440,#57441,#57442,#57443,#57444,#57445,
#57446,#57447,#57448,#57449,#57450,#57451,#57452,#57453,#57454,#57455,#57456,
#57457,#57458,#57459,#57460,#57461,#57462,#57463,#57464,#57465,#57466,#57467,
#57468,#57469,#57470,#57471,#57472,#57473,#57474,#57475,#57476,#57477,#57478,
#57479,#57480,#57481,#57482,#57483,#57484,#57485,#57486,#57487,#57488,#57489,
#57490,#57491,#57492,#57493,#57494,#57495,#57496,#57497,#57498,#57499,#57500,
#57501),.UNSPECIFIED.,.F.,.F.,(4,1,1,1,1,1,1,1,1,1,1,1,1,1,1,1,1,1,1,1,
1,1,1,1,1,1,1,1,1,1,1,1,1,1,1,1,1,1,1,1,1,1,1,1,1,1,1,1,1,1,1,1,1,1,1,1,
1,1,1,1,1,1,1,1,1,1,1,1,1,1,1,1,1,1,1,1,1,1,1,1,1,1,1,1,1,1,1,1,1,1,1,1,
1,1,1,1,1,1,1,1,1,1,1,1,1,1,1,1,1,1,1,1,1,1,1,1,1,1,1,1,1,1,1,1,1,1,1,1,
1,1,1,1,1,1,1,1,1,1,1,1,1,1,1,1,1,1,4),(94.7323961409497,94.8262562134414,
95.2611295230986,95.6960028329042,96.1308761428578,96.5657494529591,97.0006227632077,
97.4354960736028,97.870369384144,98.3052426948304,98.7401160056612,99.1749893166354,
99.6098626277522,100.04473593901,100.915335253024,101.351061255639,101.785934567313,
102.220807879124,102.655681191068,103.090554503145,103.525427815353,104.395174440154,
105.264921065453,105.699794378283,106.134667691232,106.569541004295,107.004414317471,
107.8750136343,108.745612951339,109.615359578629,110.485106206296,111.354852834309,
112.224599462639,113.094346091254,113.964092720119,114.834692038763,115.705291357499,
116.575037986826,117.444784616267,118.314531245777,119.184277875311,120.054024504821,
120.923771134261,121.794370453112,122.66496977189,123.534716400968,124.404463029834,
125.274209658448,126.143956286779,127.013702914792,127.883449542458,128.754048859798,
129.624648176939,130.494394803617,131.364141429857,132.233888055637,133.103634680937,
133.973381305737,134.843127930023,135.71372724472,136.584326559147,137.019199870684,
137.454073182083,137.888946493341,138.323819804458,139.193566426263,140.063313047491,
140.498186357887,140.933059668136,141.367932978237,141.802806288191,142.237679597997,
142.673405599673,143.109131601348,143.544004910857,143.978878220217,144.413751529429,
144.848624838491,145.283498147405,145.718371456171,146.153244764789,146.588118073258,
147.022991381581,147.457864689756,147.892737997785,148.327611305669,148.762484613407,
149.197357921002,149.633083921574,150.068809922147,150.503683229455,150.938556536623,
151.37342984365,151.808303150538,152.243176457288,152.678049763901,153.112923070379,
153.547796376722,153.982669682934,154.417542989014,154.852416294964,155.287289600787,
155.722162906483,156.157036212055,156.592762211626,157.028488211198,157.463361516526,
157.898234821735,158.333108126826,158.767981431803,159.202854736666,159.637728041419,
160.072601346062,160.507474650599,160.94234795503,161.37722125936,161.812094563589,
162.246967867721,162.681841171757,163.1167144757,163.552440474473,163.988166473247,
164.423039777011,164.85791308069,165.292786384286,165.727659687801,166.162532991238,
166.597406294601,167.03227959789,167.46715290111,167.902026204262,168.33689950735,
168.771772810376,169.206646113343,169.641519416254,170.076392719112,170.512118717363,
170.947844715614,171.382718018374,171.817591321089,172.252464623762,172.687337926397,
173.122211228996,173.557084531561,173.991957834097,174.426831136606,174.671174272867),
 .UNSPECIFIED.) ;
#3353=B_SPLINE_CURVE_WITH_KNOTS('',3,(#64473,#64474,#64475,#64476,#64477,
#64478,#64479,#64480,#64481,#64482,#64483,#64484,#64485),.UNSPECIFIED.,
 .F.,.F.,(4,3,3,3,4),(0.,0.0778109650715507,0.156406745035681,0.238225011997873,
0.302239126480066),.UNSPECIFIED.) ;
#3354=B_SPLINE_CURVE_WITH_KNOTS('',3,(#64486,#64487,#64488,#64489,#64490,
#64491,#64492,#64493,#64494,#64495,#64496,#64497,#64498,#64499,#64500,#64501,
#64502,#64503,#64504,#64505,#64506,#64507,#64508,#64509,#64510,#64511,#64512,
#64513,#64514,#64515,#64516,#64517,#64518,#64519,#64520,#64521,#64522,#64523,
#64524,#64525,#64526,#64527,#64528,#64529,#64530,#64531,#64532,#64533,#64534,
#64535,#64536,#64537,#64538,#64539,#64540,#64541,#64542,#64543,#64544,#64545,
#64546,#64547,#64548,#64549,#64550,#64551,#64552,#64553,#64554,#64555,#64556,
#64557,#64558),.UNSPECIFIED.,.F.,.F.,(4,3,3,3,3,3,3,3,3,3,3,3,3,3,3,3,3,
3,3,3,3,3,3,3,4),(0.730465481580952,0.828645125064031,1.05028297683293,
1.25837815006847,1.27510983870173,1.45572385054788,1.50312162767457,1.73316624271266,
1.90167574230222,1.96765453876246,2.20387853992392,2.44262970595966,2.62527594874715,
2.68580352301487,2.90417726726914,2.93079333089591,3.16390700345105,3.17732285394433,
3.35312908465868,3.42916468918551,3.68305064914715,3.93956813737864,4.1221204438191,
4.19992860565306,4.25678609882998),.UNSPECIFIED.) ;
#3355=B_SPLINE_CURVE_WITH_KNOTS('',3,(#71535,#71536,#71537,#71538,#71539,
#71540,#71541,#71542,#71543,#71544,#71545,#71546,#71547,#71548,#71549,#71550),
 .UNSPECIFIED.,.F.,.F.,(4,3,3,3,3,4),(0.0598809947678152,0.135924535410352,
0.211078185367313,0.230755660513956,0.309208503339108,0.36825634451708),
 .UNSPECIFIED.) ;
#3356=B_SPLINE_CURVE_WITH_KNOTS('',3,(#71552,#71553,#71554,#71555,#71556,
#71557,#71558,#71559,#71560,#71561,#71562,#71563,#71564,#71565,#71566,#71567,
#71568,#71569,#71570,#71571,#71572,#71573,#71574,#71575,#71576,#71577,#71578,
#71579,#71580,#71581,#71582,#71583,#71584,#71585,#71586,#71587,#71588,#71589,
#71590,#71591),.UNSPECIFIED.,.F.,.F.,(4,2,2,2,2,2,2,2,2,2,2,2,2,2,2,2,2,
2,2,4),(9.99997384787396E-7,0.0135018971911158,0.0220946867910526,0.027582782468828,
0.0313908326607115,0.0327527068279077,0.0343893874316741,0.0345526414539241,
0.0345596766530826,0.0345660072734853,0.0345689326430106,0.0345711188771073,
0.0345734204079688,0.0345769493878356,0.0345871620488376,0.0367578642760943,
0.040111326215381,0.0450373013211218,0.0525487888573377,0.0677449129025004),
 .UNSPECIFIED.) ;
#3357=B_SPLINE_CURVE_WITH_KNOTS('',3,(#71592,#71593,#71594,#71595,#71596,
#71597,#71598,#71599,#71600,#71601,#71602,#71603,#71604,#71605,#71606,#71607,
#71608,#71609,#71610,#71611,#71612,#71613,#71614,#71615,#71616,#71617,#71618,
#71619,#71620,#71621,#71622,#71623,#71624,#71625,#71626,#71627,#71628,#71629,
#71630,#71631,#71632,#71633,#71634,#71635,#71636,#71637,#71638,#71639,#71640,
#71641,#71642,#71643,#71644,#71645,#71646,#71647,#71648,#71649,#71650,#71651,
#71652,#71653,#71654,#71655,#71656,#71657,#71658,#71659,#71660,#71661,#71662,
#71663,#71664,#71665,#71666,#71667,#71668,#71669,#71670,#71671,#71672,#71673,
#71674,#71675,#71676,#71677,#71678,#71679,#71680,#71681,#71682,#71683,#71684,
#71685,#71686,#71687,#71688,#71689,#71690,#71691,#71692,#71693,#71694,#71695,
#71696,#71697,#71698,#71699,#71700,#71701,#71702,#71703,#71704,#71705,#71706,
#71707,#71708,#71709,#71710,#71711,#71712,#71713,#71714,#71715,#71716,#71717,
#71718,#71719,#71720,#71721,#71722,#71723,#71724,#71725,#71726,#71727,#71728,
#71729,#71730,#71731,#71732,#71733,#71734,#71735,#71736,#71737,#71738,#71739,
#71740,#71741,#71742,#71743,#71744,#71745,#71746,#71747,#71748,#71749,#71750,
#71751,#71752,#71753,#71754,#71755,#71756,#71757,#71758,#71759,#71760,#71761,
#71762,#71763,#71764,#71765,#71766,#71767,#71768,#71769,#71770,#71771,#71772,
#71773,#71774,#71775,#71776,#71777,#71778,#71779,#71780,#71781,#71782,#71783,
#71784,#71785,#71786,#71787,#71788,#71789,#71790,#71791,#71792,#71793,#71794,
#71795,#71796,#71797,#71798,#71799,#71800,#71801,#71802,#71803,#71804,#71805,
#71806,#71807,#71808,#71809,#71810,#71811,#71812,#71813,#71814,#71815,#71816,
#71817,#71818,#71819,#71820,#71821,#71822,#71823,#71824,#71825,#71826,#71827,
#71828,#71829,#71830,#71831,#71832,#71833,#71834,#71835,#71836,#71837,#71838,
#71839,#71840,#71841,#71842,#71843,#71844,#71845,#71846,#71847,#71848,#71849,
#71850,#71851,#71852,#71853,#71854,#71855,#71856,#71857,#71858,#71859,#71860,
#71861,#71862,#71863,#71864,#71865,#71866,#71867,#71868,#71869,#71870,#71871,
#71872,#71873,#71874,#71875,#71876,#71877,#71878,#71879,#71880,#71881,#71882,
#71883,#71884,#71885,#71886,#71887,#71888,#71889,#71890,#71891,#71892,#71893,
#71894,#71895,#71896,#71897,#71898,#71899,#71900,#71901,#71902,#71903,#71904,
#71905,#71906,#71907,#71908,#71909,#71910,#71911,#71912,#71913,#71914,#71915,
#71916,#71917,#71918,#71919,#71920,#71921,#71922,#71923,#71924,#71925,#71926,
#71927,#71928,#71929,#71930,#71931,#71932,#71933,#71934,#71935,#71936,#71937,
#71938,#71939,#71940,#71941,#71942,#71943,#71944,#71945,#71946,#71947,#71948,
#71949,#71950,#71951,#71952,#71953,#71954,#71955,#71956,#71957,#71958,#71959),
 .UNSPECIFIED.,.F.,.F.,(4,2,2,2,2,2,2,2,2,2,2,2,2,2,2,2,2,2,2,2,2,2,2,2,
2,2,2,2,2,2,2,2,2,2,2,2,2,2,2,2,2,2,2,2,2,2,2,2,2,2,2,2,2,2,2,2,2,2,2,2,
2,2,2,2,2,2,2,2,2,2,2,2,2,2,2,2,2,2,2,2,2,2,2,2,2,2,2,2,2,2,2,2,2,2,2,2,
2,2,2,2,2,2,2,2,2,2,2,2,2,2,2,2,2,2,2,2,2,2,2,2,2,2,2,2,2,2,2,2,2,2,2,2,
2,2,2,2,2,2,2,2,2,2,2,2,2,2,2,2,2,2,2,2,2,2,2,2,2,2,2,2,2,2,2,2,2,2,2,2,
2,2,2,2,2,2,2,2,2,2,2,2,2,2,2,4),(1.35400733413699E-6,0.00247712615579827,
0.00416327824388871,0.00508094205146327,0.00600249339869984,0.00706335045674913,
0.00883969038701396,0.0148099473822476,0.0223717149096194,0.0282144997247987,
0.0301112620467383,0.0317402129382764,0.0334276492258154,0.035620968207884,
0.04014858204514,0.041818613145435,0.0446047361014287,0.0527583621791066,
0.056170953193112,0.0582260663201588,0.0600962810291678,0.0613627721698091,
0.062890447110422,0.0656053777468073,0.0781892490459218,0.0837716676672865,
0.0863815797603843,0.0884353175008502,0.0896926063713129,0.0909040769289953,
0.0925010147903435,0.0957213105472747,0.107315595210945,0.110987479881035,
0.112703162161221,0.113752244471158,0.114706885863388,0.115459320656402,
0.116244504662199,0.117671271441775,0.124286961621675,0.129221268253395,
0.132637342200675,0.134292593949302,0.135648728949349,0.136457286584393,
0.137217119793651,0.138224392156069,0.140288657651391,0.15170269218118,
0.154607426891558,0.156079206690623,0.157023151154972,0.157823017364658,
0.158553592630756,0.15932922122094,0.160778639609794,0.169274631208156,
0.17634068036209,0.178159353561367,0.17920223816847,0.180252674718397,0.180259238384283,
0.180265816165773,0.180272408897723,0.180279016995136,0.180285641276059,
0.180292281883292,0.180298939237232,0.180305613920904,0.180312306657082,
0.180319018096007,0.180325748485621,0.180332498553139,0.180339268810392,
0.180346059541105,0.180352871422257,0.180359704913109,0.18036656035672,
0.180373438439803,0.180380339998498,0.180387264920328,0.18039421413319,
0.180401188293552,0.180408187593391,0.180415212537324,0.180422263678796,
0.180429341619825,0.180433899500866,0.180438500021273,0.180443144549349,
0.180447833609563,0.180452567793726,0.180457348925566,0.18046217785813,
0.180467055297385,0.18047198255009,0.180476960905836,0.180481991429058,
0.180487075020832,0.180492212776601,0.180497405893481,0.180502655702569,
0.180507963598798,0.180513330421916,0.180518757821487,0.180524247036456,
0.180529799495268,0.18053541611957,0.180541098419139,0.1812540104352,0.182637078659382,
0.184907612682179,0.190264930962229,0.19721030750339,0.199018921921987,
0.200342886349612,0.201754309915285,0.203268702276234,0.205528536271081,
0.211010514357248,0.213215625083288,0.214788461835044,0.216383819945492,
0.216677045527393,0.217059609681938,0.21736670252085,0.218221242950562,
0.222644625572557,0.227038488681671,0.228286630614335,0.230499490647744,
0.233501249236801,0.236831559789177,0.243983859626164,0.245565587400414,
0.246852731705488,0.248082986420242,0.248115535241426,0.248150077301255,
0.248186785422691,0.24822584879476,0.248267474505976,0.248311889112464,
0.248359340307674,0.248410098749749,0.248464459771102,0.24852274514359,
0.248585304912807,0.248652519012008,0.248724798736779,0.250293175307972,
0.252802035704825,0.258274709663911,0.258524204270529,0.258641428066646,
0.264406706682384,0.266093408532013,0.267063302604525,0.267797752698992,
0.268629450310478,0.269666667475709,0.27127109378087,0.274485218599025,
0.28441766485709,0.286615027587656,0.287893040214175,0.289005127074856,
0.290350347390146,0.293262005179613,0.297735907724777,0.305254160455839,
0.307305008735793,0.308761349714037,0.310272174180748,0.311899572851342,
0.314318074144669,0.320539171758634,0.322438859760375,0.324064743577309,
0.330918118892867,0.335527404899377,0.33711098117137,0.338630983095817),
 .UNSPECIFIED.) ;
#3358=B_SPLINE_CURVE_WITH_KNOTS('',3,(#71963,#71964,#71965,#71966,#71967,
#71968,#71969,#71970,#71971,#71972,#71973,#71974),.UNSPECIFIED.,.F.,.F.,
(4,2,2,2,2,4),(-0.0931391249568014,-0.0907876281662553,-0.0794385020809448,
-0.0680893759956343,-0.0567415781260163,-0.0453937802563982),
 .UNSPECIFIED.) ;
#3359=B_SPLINE_CURVE_WITH_KNOTS('',3,(#71975,#71976,#71977,#71978),
 .UNSPECIFIED.,.F.,.F.,(4,4),(0.282642643684195,0.354822145847901),
 .UNSPECIFIED.) ;
#3360=B_SPLINE_CURVE_WITH_KNOTS('',3,(#71980,#71981,#71982,#71983,#71984,
#71985,#71986,#71987,#71988,#71989),.UNSPECIFIED.,.F.,.F.,(4,2,2,2,4),(0.0907876281662566,
0.102136754251567,0.113485880336878,0.124833678206496,0.136181476076114),
 .UNSPECIFIED.) ;
#3361=B_SPLINE_CURVE_WITH_KNOTS('',3,(#71990,#71991,#71992,#71993,#71994,
#71995,#71996,#71997,#71998,#71999),.UNSPECIFIED.,.F.,.F.,(4,2,2,2,4),(0.136181476076114,
0.147529243922143,0.158877011768171,0.170226134050342,0.181575256332513),
 .UNSPECIFIED.) ;
#3362=B_SPLINE_CURVE_WITH_KNOTS('',3,(#72000,#72001,#72002,#72003,#72004,
#72005,#72006,#72007,#72008,#72009),.UNSPECIFIED.,.F.,.F.,(4,2,2,2,4),(-0.0453929098666937,
-0.0340453596051069,-0.02269780934352,-0.01134890467176,0.),
 .UNSPECIFIED.) ;
#3363=B_SPLINE_CURVE_WITH_KNOTS('',3,(#78980,#78981,#78982,#78983,#78984,
#78985,#78986,#78987,#78988,#78989,#78990,#78991,#78992,#78993,#78994,#78995),
 .UNSPECIFIED.,.F.,.F.,(4,3,3,3,3,4),(0.0598607559016046,0.135904671484349,
0.211058386868452,0.230755571039204,0.309208126739232,0.368256344517073),
 .UNSPECIFIED.) ;
#3364=B_SPLINE_CURVE_WITH_KNOTS('',3,(#78996,#78997,#78998,#78999,#79000,
#79001,#79002,#79003,#79004,#79005,#79006,#79007,#79008,#79009,#79010,#79011,
#79012,#79013,#79014,#79015,#79016,#79017,#79018,#79019,#79020,#79021,#79022,
#79023,#79024,#79025,#79026,#79027,#79028,#79029,#79030,#79031,#79032,#79033,
#79034,#79035),.UNSPECIFIED.,.F.,.F.,(4,2,2,2,2,2,2,2,2,2,2,2,2,2,2,2,2,
2,2,4),(8.8129793943429E-6,0.0135075679582764,0.0221000806739361,0.0275880663744416,
0.0313960477253353,0.0327588819471267,0.0343944713916458,0.0345576172666708,
0.0345645498592877,0.0345709399602103,0.0345738770438662,0.0345760653634415,
0.0345783628973854,0.0345818439872346,0.0345918197813435,0.0363912982801799,
0.0395253587707758,0.0441846088748481,0.051190397675679,0.0673693904034745),
 .UNSPECIFIED.) ;
#3365=B_SPLINE_CURVE_WITH_KNOTS('',3,(#79039,#79040,#79041,#79042,#79043,
#79044,#79045,#79046,#79047),.UNSPECIFIED.,.F.,.F.,(4,1,1,1,1,1,4),(0.,
0.520304865070705,0.709542561390409,0.804161409708611,0.898780258026813,
1.15893269056541,1.419085123104),.UNSPECIFIED.) ;
#3366=B_SPLINE_CURVE_WITH_KNOTS('',3,(#79049,#79050,#79051,#79052,#79053,
#79054,#79055,#79056,#79057,#79058),.UNSPECIFIED.,.F.,.F.,(4,1,1,1,1,1,
1,4),(1.419085123104,1.67923755563226,1.93938998816052,2.03400883639567,
2.12862768463082,2.31786538114359,2.57801781366682,2.83817024619004),
 .UNSPECIFIED.) ;
#3367=B_SPLINE_CURVE_WITH_KNOTS('',3,(#79096,#79097,#79098,#79099,#79100,
#79101,#79102,#79103,#79104,#79105),.UNSPECIFIED.,.F.,.F.,(4,1,1,1,1,1,
1,4),(1.41908512308802,1.67923755561058,1.93938998813313,2.03400883648099,
2.12862768482886,2.3178653810957,2.57801781365659,2.83817024621747),
 .UNSPECIFIED.) ;
#3368=B_SPLINE_CURVE_WITH_KNOTS('',3,(#79106,#79107,#79108,#79109,#79110,
#79111,#79112,#79113,#79114),.UNSPECIFIED.,.F.,.F.,(4,1,1,1,1,1,4),(0.,
0.520304865043955,0.70954256158844,0.804161409794499,0.898780258000557,
1.15893269054429,1.41908512308802),.UNSPECIFIED.) ;
#3369=B_SPLINE_CURVE_WITH_KNOTS('',3,(#79152,#79153,#79154,#79155,#79156,
#79157,#79158,#79159,#79160,#79161),.UNSPECIFIED.,.F.,.F.,(4,1,1,1,1,1,
1,4),(1.41908512299766,1.67923755554141,1.93938998808516,2.03400883629124,
2.12862768449733,2.31786538104175,2.57801781362961,2.83817024621746),
 .UNSPECIFIED.) ;
#3370=B_SPLINE_CURVE_WITH_KNOTS('',3,(#79162,#79163,#79164,#79165,#79166,
#79167,#79168,#79169,#79170),.UNSPECIFIED.,.F.,.F.,(4,1,1,1,1,1,4),(0.,
0.520304864990006,0.709542561256855,0.80416140961432,0.898780257971786,
1.15893269048473,1.41908512299766),.UNSPECIFIED.) ;
#3371=B_SPLINE_CURVE_WITH_KNOTS('',3,(#79174,#79175,#79176,#79177,#79178,
#79179,#79180,#79181,#79182),.UNSPECIFIED.,.F.,.F.,(4,1,1,1,1,1,4),(0.,
0.520304865114576,0.709542561608101,0.804161409843274,0.898780258078447,
1.1589326906067,1.41908512313495),.UNSPECIFIED.) ;
#3372=B_SPLINE_CURVE_WITH_KNOTS('',3,(#79184,#79185,#79186,#79187,#79188,
#79189,#79190,#79191,#79192,#79193),.UNSPECIFIED.,.F.,.F.,(4,1,1,1,1,1,
1,4),(1.41908512313495,1.67923755567353,1.9393899882121,2.03400883653032,
2.12862768484853,2.31786538116822,2.57801781373375,2.83817024629929),
 .UNSPECIFIED.) ;
#3463=VERTEX_POINT('',#12441) ;
#3464=VERTEX_POINT('',#12442) ;
#3465=VERTEX_POINT('',#12444) ;
#3466=VERTEX_POINT('',#12512) ;
#3467=VERTEX_POINT('',#12523) ;
#3468=VERTEX_POINT('',#12525) ;
#3469=VERTEX_POINT('',#12708) ;
#3470=VERTEX_POINT('',#12709) ;
#3471=VERTEX_POINT('',#12711) ;
#3472=VERTEX_POINT('',#12846) ;
#3473=VERTEX_POINT('',#12982) ;
#3474=VERTEX_POINT('',#12983) ;
#3475=VERTEX_POINT('',#12985) ;
#3476=VERTEX_POINT('',#13613) ;
#3477=VERTEX_POINT('',#13953) ;
#3478=VERTEX_POINT('',#13954) ;
#3479=VERTEX_POINT('',#13956) ;
#3480=VERTEX_POINT('',#14451) ;
#3481=VERTEX_POINT('',#15017) ;
#3482=VERTEX_POINT('',#15018) ;
#3483=VERTEX_POINT('',#15020) ;
#3484=VERTEX_POINT('',#15085) ;
#3485=VERTEX_POINT('',#15155) ;
#3486=VERTEX_POINT('',#15156) ;
#3487=VERTEX_POINT('',#15158) ;
#3488=VERTEX_POINT('',#15665) ;
#3489=VERTEX_POINT('',#15762) ;
#3490=VERTEX_POINT('',#15763) ;
#3491=VERTEX_POINT('',#16032) ;
#3492=VERTEX_POINT('',#16033) ;
#3493=VERTEX_POINT('',#16287) ;
#3494=VERTEX_POINT('',#16288) ;
#3495=VERTEX_POINT('',#17909) ;
#3496=VERTEX_POINT('',#17910) ;
#3497=VERTEX_POINT('',#17912) ;
#3498=VERTEX_POINT('',#18185) ;
#3499=VERTEX_POINT('',#18437) ;
#3500=VERTEX_POINT('',#18439) ;
#3501=VERTEX_POINT('',#18442) ;
#3502=VERTEX_POINT('',#18459) ;
#3503=VERTEX_POINT('',#18476) ;
#3504=VERTEX_POINT('',#18493) ;
#3505=VERTEX_POINT('',#18511) ;
#3506=VERTEX_POINT('',#18531) ;
#3507=VERTEX_POINT('',#18700) ;
#3508=VERTEX_POINT('',#18720) ;
#3509=VERTEX_POINT('',#18967) ;
#3510=VERTEX_POINT('',#18968) ;
#3511=VERTEX_POINT('',#18970) ;
#3512=VERTEX_POINT('',#18974) ;
#3513=VERTEX_POINT('',#18975) ;
#3514=VERTEX_POINT('',#18977) ;
#3515=VERTEX_POINT('',#25950) ;
#3516=VERTEX_POINT('',#25951) ;
#3517=VERTEX_POINT('',#25965) ;
#3518=VERTEX_POINT('',#33237) ;
#3519=VERTEX_POINT('',#33238) ;
#3520=VERTEX_POINT('',#33252) ;
#3521=VERTEX_POINT('',#33346) ;
#3522=VERTEX_POINT('',#33348) ;
#3523=VERTEX_POINT('',#33350) ;
#3524=VERTEX_POINT('',#41228) ;
#3525=VERTEX_POINT('',#41429) ;
#3526=VERTEX_POINT('',#41433) ;
#3527=VERTEX_POINT('',#41802) ;
#3528=VERTEX_POINT('',#42522) ;
#3529=VERTEX_POINT('',#42523) ;
#3530=VERTEX_POINT('',#42537) ;
#3531=VERTEX_POINT('',#42932) ;
#3532=VERTEX_POINT('',#42937) ;
#3533=VERTEX_POINT('',#43216) ;
#3534=VERTEX_POINT('',#43218) ;
#3535=VERTEX_POINT('',#43229) ;
#3536=VERTEX_POINT('',#43240) ;
#3537=VERTEX_POINT('',#50223) ;
#3538=VERTEX_POINT('',#57274) ;
#3539=VERTEX_POINT('',#57275) ;
#3540=VERTEX_POINT('',#57320) ;
#3541=VERTEX_POINT('',#57340) ;
#3542=VERTEX_POINT('',#64472) ;
#3543=VERTEX_POINT('',#71534) ;
#3544=VERTEX_POINT('',#71551) ;
#3545=VERTEX_POINT('',#71961) ;
#3546=VERTEX_POINT('',#71979) ;
#3547=VERTEX_POINT('',#79037) ;
#3548=VERTEX_POINT('',#79038) ;
#3549=VERTEX_POINT('',#79093) ;
#3550=VERTEX_POINT('',#79095) ;
#3551=VERTEX_POINT('',#79149) ;
#3552=VERTEX_POINT('',#79151) ;
#3553=VERTEX_POINT('',#79172) ;
#3554=VERTEX_POINT('',#79173) ;
#4317=EDGE_CURVE('',#3463,#3464,#1872,.T.) ;
#4318=EDGE_CURVE('',#3464,#3465,#3283,.T.) ;
#4319=EDGE_CURVE('',#3465,#3466,#3284,.T.) ;
#4320=EDGE_CURVE('',#3466,#3467,#614,.T.) ;
#4321=EDGE_CURVE('',#3467,#3468,#3285,.T.) ;
#4322=EDGE_CURVE('',#3468,#3463,#3286,.T.) ;
#4323=EDGE_CURVE('',#3469,#3470,#1873,.T.) ;
#4324=EDGE_CURVE('',#3470,#3471,#3287,.T.) ;
#4325=EDGE_CURVE('',#3471,#3464,#3288,.T.) ;
#4326=EDGE_CURVE('',#3463,#3472,#3289,.T.) ;
#4327=EDGE_CURVE('',#3472,#3469,#3290,.T.) ;
#4328=EDGE_CURVE('',#3473,#3474,#1874,.T.) ;
#4329=EDGE_CURVE('',#3474,#3475,#3291,.T.) ;
#4330=EDGE_CURVE('',#3475,#3470,#3292,.T.) ;
#4331=EDGE_CURVE('',#3469,#3476,#3293,.T.) ;
#4332=EDGE_CURVE('',#3476,#3473,#3294,.T.) ;
#4333=EDGE_CURVE('',#3477,#3478,#1875,.T.) ;
#4334=EDGE_CURVE('',#3478,#3479,#3295,.T.) ;
#4335=EDGE_CURVE('',#3479,#3474,#3296,.T.) ;
#4336=EDGE_CURVE('',#3473,#3480,#3297,.T.) ;
#4337=EDGE_CURVE('',#3480,#3477,#3298,.T.) ;
#4338=EDGE_CURVE('',#3481,#3482,#1876,.T.) ;
#4339=EDGE_CURVE('',#3481,#3483,#3299,.T.) ;
#4340=EDGE_CURVE('',#3484,#3483,#3300,.T.) ;
#4341=EDGE_CURVE('',#3484,#3482,#3301,.T.) ;
#4342=EDGE_CURVE('',#3485,#3486,#1877,.T.) ;
#4343=EDGE_CURVE('',#3487,#3486,#3302,.T.) ;
#4344=EDGE_CURVE('',#3487,#3488,#615,.T.) ;
#4345=EDGE_CURVE('',#3485,#3488,#3303,.T.) ;
#4346=EDGE_CURVE('',#3489,#3490,#1878,.T.) ;
#4347=EDGE_CURVE('',#3486,#3490,#3304,.T.) ;
#4348=EDGE_CURVE('',#3489,#3485,#3305,.T.) ;
#4349=EDGE_CURVE('',#3491,#3492,#1879,.T.) ;
#4350=EDGE_CURVE('',#3490,#3492,#3306,.T.) ;
#4351=EDGE_CURVE('',#3491,#3489,#3307,.T.) ;
#4352=EDGE_CURVE('',#3493,#3494,#1880,.T.) ;
#4353=EDGE_CURVE('',#3492,#3494,#3308,.T.) ;
#4354=EDGE_CURVE('',#3493,#3491,#3309,.T.) ;
#4355=EDGE_CURVE('',#3495,#3496,#1881,.T.) ;
#4356=EDGE_CURVE('',#3497,#3495,#3310,.T.) ;
#4357=EDGE_CURVE('',#3497,#3498,#3311,.T.) ;
#4358=EDGE_CURVE('',#3496,#3498,#3312,.T.) ;
#4359=EDGE_CURVE('',#3499,#3499,#616,.T.) ;
#4360=EDGE_CURVE('',#3499,#3500,#1882,.T.) ;
#4361=EDGE_CURVE('',#3500,#3500,#617,.T.) ;
#4362=EDGE_CURVE('',#3501,#3501,#3313,.T.) ;
#4363=EDGE_CURVE('',#3502,#3502,#3314,.T.) ;
#4364=EDGE_CURVE('',#3503,#3503,#3315,.T.) ;
#4365=EDGE_CURVE('',#3504,#3504,#3316,.T.) ;
#4366=EDGE_CURVE('',#3505,#3505,#3317,.T.) ;
#4367=EDGE_CURVE('',#3466,#3506,#3318,.T.) ;
#4368=EDGE_CURVE('',#3506,#3467,#3319,.T.) ;
#4369=EDGE_CURVE('',#3507,#3507,#3320,.T.) ;
#4370=EDGE_CURVE('',#3508,#3487,#3321,.T.) ;
#4371=EDGE_CURVE('',#3488,#3508,#3322,.T.) ;
#4372=EDGE_CURVE('',#3499,#3505,#1883,.T.) ;
#4373=EDGE_CURVE('',#3500,#3507,#1884,.T.) ;
#4374=EDGE_CURVE('',#3509,#3510,#1885,.T.) ;
#4375=EDGE_CURVE('',#3511,#3510,#618,.T.) ;
#4376=EDGE_CURVE('',#3510,#3511,#619,.T.) ;
#4377=EDGE_CURVE('',#3512,#3513,#620,.T.) ;
#4378=EDGE_CURVE('',#3513,#3514,#1886,.T.) ;
#4379=EDGE_CURVE('',#3513,#3512,#621,.T.) ;
#4380=EDGE_CURVE('',#3515,#3516,#3323,.T.) ;
#4381=EDGE_CURVE('',#3516,#3517,#3324,.T.) ;
#4382=EDGE_CURVE('',#3517,#3515,#3325,.T.) ;
#4383=EDGE_CURVE('',#3518,#3519,#3326,.T.) ;
#4384=EDGE_CURVE('',#3519,#3520,#3327,.T.) ;
#4385=EDGE_CURVE('',#3520,#3518,#3328,.T.) ;
#4386=EDGE_CURVE('',#3519,#3521,#1887,.T.) ;
#4387=EDGE_CURVE('',#3521,#3522,#622,.T.) ;
#4388=EDGE_CURVE('',#3522,#3523,#1888,.T.) ;
#4389=EDGE_CURVE('',#3520,#3523,#3329,.T.) ;
#4390=EDGE_CURVE('',#3494,#3496,#3330,.T.) ;
#4391=EDGE_CURVE('',#3495,#3493,#3331,.T.) ;
#4392=EDGE_CURVE('',#3524,#3518,#3332,.T.) ;
#4393=EDGE_CURVE('',#3523,#3497,#3333,.T.) ;
#4394=EDGE_CURVE('',#3524,#3508,#3334,.T.) ;
#4395=EDGE_CURVE('',#3516,#3525,#1889,.T.) ;
#4396=EDGE_CURVE('',#3525,#3517,#623,.T.) ;
#4397=EDGE_CURVE('',#3482,#3526,#3335,.T.) ;
#4398=EDGE_CURVE('',#3526,#3478,#3336,.T.) ;
#4399=EDGE_CURVE('',#3477,#3527,#3337,.T.) ;
#4400=EDGE_CURVE('',#3527,#3481,#3338,.T.) ;
#4401=EDGE_CURVE('',#3528,#3529,#3339,.T.) ;
#4402=EDGE_CURVE('',#3528,#3530,#3340,.T.) ;
#4403=EDGE_CURVE('',#3531,#3530,#3341,.T.) ;
#4404=EDGE_CURVE('',#3531,#3532,#3342,.T.) ;
#4405=EDGE_CURVE('',#3532,#3533,#624,.T.) ;
#4406=EDGE_CURVE('',#3534,#3533,#3343,.T.) ;
#4407=EDGE_CURVE('',#3535,#3534,#3344,.T.) ;
#4408=EDGE_CURVE('',#3535,#3536,#625,.T.) ;
#4409=EDGE_CURVE('',#3529,#3536,#3345,.T.) ;
#4410=EDGE_CURVE('',#3511,#3529,#1890,.T.) ;
#4411=EDGE_CURVE('',#3531,#3537,#3346,.T.) ;
#4412=EDGE_CURVE('',#3537,#3532,#3347,.T.) ;
#4413=EDGE_CURVE('',#3538,#3539,#3348,.T.) ;
#4414=EDGE_CURVE('',#3540,#3539,#3349,.T.) ;
#4415=EDGE_CURVE('',#3540,#3541,#3350,.T.) ;
#4416=EDGE_CURVE('',#3541,#3483,#3351,.T.) ;
#4417=EDGE_CURVE('',#3538,#3506,#3352,.T.) ;
#4418=EDGE_CURVE('',#3539,#3542,#3353,.T.) ;
#4419=EDGE_CURVE('',#3542,#3540,#3354,.T.) ;
#4420=EDGE_CURVE('',#3537,#3533,#1891,.T.) ;
#4421=EDGE_CURVE('',#3542,#3536,#1892,.T.) ;
#4422=EDGE_CURVE('',#3535,#3541,#1893,.T.) ;
#4423=EDGE_CURVE('',#3543,#3524,#3355,.T.) ;
#4424=EDGE_CURVE('',#3498,#3544,#3356,.T.) ;
#4425=EDGE_CURVE('',#3544,#3543,#3357,.T.) ;
#4426=EDGE_CURVE('',#3512,#3545,#1894,.T.) ;
#4427=EDGE_CURVE('',#3545,#3543,#3358,.F.) ;
#4428=EDGE_CURVE('',#3544,#3515,#3359,.T.) ;
#4429=EDGE_CURVE('',#3525,#3546,#3360,.T.) ;
#4430=EDGE_CURVE('',#3546,#3522,#3361,.T.) ;
#4431=EDGE_CURVE('',#3521,#3545,#3362,.F.) ;
#4432=EDGE_CURVE('',#3528,#3538,#3363,.T.) ;
#4433=EDGE_CURVE('',#3484,#3530,#3364,.T.) ;
#4434=EDGE_CURVE('',#3547,#3548,#3365,.T.) ;
#4435=EDGE_CURVE('',#3548,#3545,#1895,.T.) ;
#4436=EDGE_CURVE('',#3548,#3547,#3366,.T.) ;
#4437=EDGE_CURVE('',#3547,#3501,#1896,.T.) ;
#4438=EDGE_CURVE('',#3546,#3549,#1897,.T.) ;
#4439=EDGE_CURVE('',#3549,#3550,#3367,.T.) ;
#4440=EDGE_CURVE('',#3550,#3549,#3368,.T.) ;
#4441=EDGE_CURVE('',#3550,#3502,#1898,.T.) ;
#4442=EDGE_CURVE('',#3529,#3551,#1899,.T.) ;
#4443=EDGE_CURVE('',#3551,#3552,#3369,.T.) ;
#4444=EDGE_CURVE('',#3552,#3551,#3370,.T.) ;
#4445=EDGE_CURVE('',#3553,#3554,#3371,.T.) ;
#4446=EDGE_CURVE('',#3554,#3534,#1900,.T.) ;
#4447=EDGE_CURVE('',#3554,#3553,#3372,.T.) ;
#4448=EDGE_CURVE('',#3553,#3504,#1901,.T.) ;
#4449=EDGE_CURVE('',#3552,#3503,#1902,.T.) ;
#5618=ORIENTED_EDGE('',*,*,#4317,.T.) ;
#5619=ORIENTED_EDGE('',*,*,#4318,.T.) ;
#5620=ORIENTED_EDGE('',*,*,#4319,.T.) ;
#5621=ORIENTED_EDGE('',*,*,#4320,.T.) ;
#5622=ORIENTED_EDGE('',*,*,#4321,.T.) ;
#5623=ORIENTED_EDGE('',*,*,#4322,.T.) ;
#5624=ORIENTED_EDGE('',*,*,#4323,.T.) ;
#5625=ORIENTED_EDGE('',*,*,#4324,.T.) ;
#5626=ORIENTED_EDGE('',*,*,#4325,.T.) ;
#5627=ORIENTED_EDGE('',*,*,#4317,.F.) ;
#5628=ORIENTED_EDGE('',*,*,#4326,.T.) ;
#5629=ORIENTED_EDGE('',*,*,#4327,.T.) ;
#5630=ORIENTED_EDGE('',*,*,#4328,.T.) ;
#5631=ORIENTED_EDGE('',*,*,#4329,.T.) ;
#5632=ORIENTED_EDGE('',*,*,#4330,.T.) ;
#5633=ORIENTED_EDGE('',*,*,#4323,.F.) ;
#5634=ORIENTED_EDGE('',*,*,#4331,.T.) ;
#5635=ORIENTED_EDGE('',*,*,#4332,.T.) ;
#5636=ORIENTED_EDGE('',*,*,#4333,.T.) ;
#5637=ORIENTED_EDGE('',*,*,#4334,.T.) ;
#5638=ORIENTED_EDGE('',*,*,#4335,.T.) ;
#5639=ORIENTED_EDGE('',*,*,#4328,.F.) ;
#5640=ORIENTED_EDGE('',*,*,#4336,.T.) ;
#5641=ORIENTED_EDGE('',*,*,#4337,.T.) ;
#5642=ORIENTED_EDGE('',*,*,#4338,.F.) ;
#5643=ORIENTED_EDGE('',*,*,#4339,.T.) ;
#5644=ORIENTED_EDGE('',*,*,#4340,.F.) ;
#5645=ORIENTED_EDGE('',*,*,#4341,.T.) ;
#5646=ORIENTED_EDGE('',*,*,#4342,.T.) ;
#5647=ORIENTED_EDGE('',*,*,#4343,.F.) ;
#5648=ORIENTED_EDGE('',*,*,#4344,.T.) ;
#5649=ORIENTED_EDGE('',*,*,#4345,.F.) ;
#5650=ORIENTED_EDGE('',*,*,#4346,.T.) ;
#5651=ORIENTED_EDGE('',*,*,#4347,.F.) ;
#5652=ORIENTED_EDGE('',*,*,#4342,.F.) ;
#5653=ORIENTED_EDGE('',*,*,#4348,.F.) ;
#5654=ORIENTED_EDGE('',*,*,#4349,.T.) ;
#5655=ORIENTED_EDGE('',*,*,#4350,.F.) ;
#5656=ORIENTED_EDGE('',*,*,#4346,.F.) ;
#5657=ORIENTED_EDGE('',*,*,#4351,.F.) ;
#5658=ORIENTED_EDGE('',*,*,#4352,.T.) ;
#5659=ORIENTED_EDGE('',*,*,#4353,.F.) ;
#5660=ORIENTED_EDGE('',*,*,#4349,.F.) ;
#5661=ORIENTED_EDGE('',*,*,#4354,.F.) ;
#5662=ORIENTED_EDGE('',*,*,#4355,.F.) ;
#5663=ORIENTED_EDGE('',*,*,#4356,.F.) ;
#5664=ORIENTED_EDGE('',*,*,#4357,.T.) ;
#5665=ORIENTED_EDGE('',*,*,#4358,.F.) ;
#5666=ORIENTED_EDGE('',*,*,#4359,.T.) ;
#5667=ORIENTED_EDGE('',*,*,#4360,.T.) ;
#5668=ORIENTED_EDGE('',*,*,#4361,.F.) ;
#5669=ORIENTED_EDGE('',*,*,#4360,.F.) ;
#5670=ORIENTED_EDGE('',*,*,#4362,.F.) ;
#5671=ORIENTED_EDGE('',*,*,#4363,.F.) ;
#5672=ORIENTED_EDGE('',*,*,#4364,.F.) ;
#5673=ORIENTED_EDGE('',*,*,#4365,.F.) ;
#5674=ORIENTED_EDGE('',*,*,#4366,.F.) ;
#5675=ORIENTED_EDGE('',*,*,#4367,.T.) ;
#5676=ORIENTED_EDGE('',*,*,#4368,.T.) ;
#5677=ORIENTED_EDGE('',*,*,#4320,.F.) ;
#5678=ORIENTED_EDGE('',*,*,#4369,.T.) ;
#5679=ORIENTED_EDGE('',*,*,#4344,.F.) ;
#5680=ORIENTED_EDGE('',*,*,#4370,.F.) ;
#5681=ORIENTED_EDGE('',*,*,#4371,.F.) ;
#5682=ORIENTED_EDGE('',*,*,#4372,.T.) ;
#5683=ORIENTED_EDGE('',*,*,#4366,.T.) ;
#5684=ORIENTED_EDGE('',*,*,#4372,.F.) ;
#5685=ORIENTED_EDGE('',*,*,#4359,.F.) ;
#5686=ORIENTED_EDGE('',*,*,#4361,.T.) ;
#5687=ORIENTED_EDGE('',*,*,#4373,.T.) ;
#5688=ORIENTED_EDGE('',*,*,#4369,.F.) ;
#5689=ORIENTED_EDGE('',*,*,#4373,.F.) ;
#5690=ORIENTED_EDGE('',*,*,#4374,.T.) ;
#5691=ORIENTED_EDGE('',*,*,#4375,.F.) ;
#5692=ORIENTED_EDGE('',*,*,#4376,.F.) ;
#5693=ORIENTED_EDGE('',*,*,#4374,.F.) ;
#5694=ORIENTED_EDGE('',*,*,#4377,.T.) ;
#5695=ORIENTED_EDGE('',*,*,#4378,.T.) ;
#5696=ORIENTED_EDGE('',*,*,#4378,.F.) ;
#5697=ORIENTED_EDGE('',*,*,#4379,.T.) ;
#5698=ORIENTED_EDGE('',*,*,#4380,.T.) ;
#5699=ORIENTED_EDGE('',*,*,#4381,.T.) ;
#5700=ORIENTED_EDGE('',*,*,#4382,.T.) ;
#5701=ORIENTED_EDGE('',*,*,#4383,.T.) ;
#5702=ORIENTED_EDGE('',*,*,#4384,.T.) ;
#5703=ORIENTED_EDGE('',*,*,#4385,.T.) ;
#5704=ORIENTED_EDGE('',*,*,#4386,.T.) ;
#5705=ORIENTED_EDGE('',*,*,#4387,.T.) ;
#5706=ORIENTED_EDGE('',*,*,#4388,.T.) ;
#5707=ORIENTED_EDGE('',*,*,#4389,.F.) ;
#5708=ORIENTED_EDGE('',*,*,#4384,.F.) ;
#5709=ORIENTED_EDGE('',*,*,#4355,.T.) ;
#5710=ORIENTED_EDGE('',*,*,#4390,.F.) ;
#5711=ORIENTED_EDGE('',*,*,#4352,.F.) ;
#5712=ORIENTED_EDGE('',*,*,#4391,.F.) ;
#5713=ORIENTED_EDGE('',*,*,#4392,.T.) ;
#5714=ORIENTED_EDGE('',*,*,#4385,.F.) ;
#5715=ORIENTED_EDGE('',*,*,#4389,.T.) ;
#5716=ORIENTED_EDGE('',*,*,#4393,.T.) ;
#5717=ORIENTED_EDGE('',*,*,#4356,.T.) ;
#5718=ORIENTED_EDGE('',*,*,#4391,.T.) ;
#5719=ORIENTED_EDGE('',*,*,#4354,.T.) ;
#5720=ORIENTED_EDGE('',*,*,#4351,.T.) ;
#5721=ORIENTED_EDGE('',*,*,#4348,.T.) ;
#5722=ORIENTED_EDGE('',*,*,#4345,.T.) ;
#5723=ORIENTED_EDGE('',*,*,#4371,.T.) ;
#5724=ORIENTED_EDGE('',*,*,#4394,.F.) ;
#5725=ORIENTED_EDGE('',*,*,#4395,.T.) ;
#5726=ORIENTED_EDGE('',*,*,#4396,.T.) ;
#5727=ORIENTED_EDGE('',*,*,#4381,.F.) ;
#5728=ORIENTED_EDGE('',*,*,#4338,.T.) ;
#5729=ORIENTED_EDGE('',*,*,#4397,.T.) ;
#5730=ORIENTED_EDGE('',*,*,#4398,.T.) ;
#5731=ORIENTED_EDGE('',*,*,#4333,.F.) ;
#5732=ORIENTED_EDGE('',*,*,#4399,.T.) ;
#5733=ORIENTED_EDGE('',*,*,#4400,.T.) ;
#5734=ORIENTED_EDGE('',*,*,#4401,.F.) ;
#5735=ORIENTED_EDGE('',*,*,#4402,.T.) ;
#5736=ORIENTED_EDGE('',*,*,#4403,.F.) ;
#5737=ORIENTED_EDGE('',*,*,#4404,.T.) ;
#5738=ORIENTED_EDGE('',*,*,#4405,.T.) ;
#5739=ORIENTED_EDGE('',*,*,#4406,.F.) ;
#5740=ORIENTED_EDGE('',*,*,#4407,.F.) ;
#5741=ORIENTED_EDGE('',*,*,#4408,.T.) ;
#5742=ORIENTED_EDGE('',*,*,#4409,.F.) ;
#5743=ORIENTED_EDGE('',*,*,#4410,.F.) ;
#5744=ORIENTED_EDGE('',*,*,#4375,.T.) ;
#5745=ORIENTED_EDGE('',*,*,#4376,.T.) ;
#5746=ORIENTED_EDGE('',*,*,#4410,.T.) ;
#5747=ORIENTED_EDGE('',*,*,#4411,.T.) ;
#5748=ORIENTED_EDGE('',*,*,#4412,.T.) ;
#5749=ORIENTED_EDGE('',*,*,#4404,.F.) ;
#5750=ORIENTED_EDGE('',*,*,#4413,.T.) ;
#5751=ORIENTED_EDGE('',*,*,#4414,.F.) ;
#5752=ORIENTED_EDGE('',*,*,#4415,.T.) ;
#5753=ORIENTED_EDGE('',*,*,#4416,.T.) ;
#5754=ORIENTED_EDGE('',*,*,#4339,.F.) ;
#5755=ORIENTED_EDGE('',*,*,#4400,.F.) ;
#5756=ORIENTED_EDGE('',*,*,#4399,.F.) ;
#5757=ORIENTED_EDGE('',*,*,#4337,.F.) ;
#5758=ORIENTED_EDGE('',*,*,#4336,.F.) ;
#5759=ORIENTED_EDGE('',*,*,#4332,.F.) ;
#5760=ORIENTED_EDGE('',*,*,#4331,.F.) ;
#5761=ORIENTED_EDGE('',*,*,#4327,.F.) ;
#5762=ORIENTED_EDGE('',*,*,#4326,.F.) ;
#5763=ORIENTED_EDGE('',*,*,#4322,.F.) ;
#5764=ORIENTED_EDGE('',*,*,#4321,.F.) ;
#5765=ORIENTED_EDGE('',*,*,#4368,.F.) ;
#5766=ORIENTED_EDGE('',*,*,#4417,.F.) ;
#5767=ORIENTED_EDGE('',*,*,#4418,.T.) ;
#5768=ORIENTED_EDGE('',*,*,#4419,.T.) ;
#5769=ORIENTED_EDGE('',*,*,#4414,.T.) ;
#5770=ORIENTED_EDGE('',*,*,#4420,.T.) ;
#5771=ORIENTED_EDGE('',*,*,#4405,.F.) ;
#5772=ORIENTED_EDGE('',*,*,#4412,.F.) ;
#5773=ORIENTED_EDGE('',*,*,#4421,.T.) ;
#5774=ORIENTED_EDGE('',*,*,#4408,.F.) ;
#5775=ORIENTED_EDGE('',*,*,#4422,.T.) ;
#5776=ORIENTED_EDGE('',*,*,#4415,.F.) ;
#5777=ORIENTED_EDGE('',*,*,#4419,.F.) ;
#5778=ORIENTED_EDGE('',*,*,#4423,.T.) ;
#5779=ORIENTED_EDGE('',*,*,#4394,.T.) ;
#5780=ORIENTED_EDGE('',*,*,#4370,.T.) ;
#5781=ORIENTED_EDGE('',*,*,#4343,.T.) ;
#5782=ORIENTED_EDGE('',*,*,#4347,.T.) ;
#5783=ORIENTED_EDGE('',*,*,#4350,.T.) ;
#5784=ORIENTED_EDGE('',*,*,#4353,.T.) ;
#5785=ORIENTED_EDGE('',*,*,#4390,.T.) ;
#5786=ORIENTED_EDGE('',*,*,#4358,.T.) ;
#5787=ORIENTED_EDGE('',*,*,#4424,.T.) ;
#5788=ORIENTED_EDGE('',*,*,#4425,.T.) ;
#5789=ORIENTED_EDGE('',*,*,#4377,.F.) ;
#5790=ORIENTED_EDGE('',*,*,#4426,.T.) ;
#5791=ORIENTED_EDGE('',*,*,#4427,.T.) ;
#5792=ORIENTED_EDGE('',*,*,#4425,.F.) ;
#5793=ORIENTED_EDGE('',*,*,#4428,.T.) ;
#5794=ORIENTED_EDGE('',*,*,#4382,.F.) ;
#5795=ORIENTED_EDGE('',*,*,#4396,.F.) ;
#5796=ORIENTED_EDGE('',*,*,#4429,.T.) ;
#5797=ORIENTED_EDGE('',*,*,#4430,.T.) ;
#5798=ORIENTED_EDGE('',*,*,#4387,.F.) ;
#5799=ORIENTED_EDGE('',*,*,#4431,.T.) ;
#5800=ORIENTED_EDGE('',*,*,#4426,.F.) ;
#5801=ORIENTED_EDGE('',*,*,#4379,.F.) ;
#5802=ORIENTED_EDGE('',*,*,#4432,.T.) ;
#5803=ORIENTED_EDGE('',*,*,#4417,.T.) ;
#5804=ORIENTED_EDGE('',*,*,#4367,.F.) ;
#5805=ORIENTED_EDGE('',*,*,#4319,.F.) ;
#5806=ORIENTED_EDGE('',*,*,#4318,.F.) ;
#5807=ORIENTED_EDGE('',*,*,#4325,.F.) ;
#5808=ORIENTED_EDGE('',*,*,#4324,.F.) ;
#5809=ORIENTED_EDGE('',*,*,#4330,.F.) ;
#5810=ORIENTED_EDGE('',*,*,#4329,.F.) ;
#5811=ORIENTED_EDGE('',*,*,#4335,.F.) ;
#5812=ORIENTED_EDGE('',*,*,#4334,.F.) ;
#5813=ORIENTED_EDGE('',*,*,#4398,.F.) ;
#5814=ORIENTED_EDGE('',*,*,#4397,.F.) ;
#5815=ORIENTED_EDGE('',*,*,#4341,.F.) ;
#5816=ORIENTED_EDGE('',*,*,#4433,.T.) ;
#5817=ORIENTED_EDGE('',*,*,#4402,.F.) ;
#5818=ORIENTED_EDGE('',*,*,#4434,.T.) ;
#5819=ORIENTED_EDGE('',*,*,#4435,.T.) ;
#5820=ORIENTED_EDGE('',*,*,#4431,.F.) ;
#5821=ORIENTED_EDGE('',*,*,#4386,.F.) ;
#5822=ORIENTED_EDGE('',*,*,#4383,.F.) ;
#5823=ORIENTED_EDGE('',*,*,#4392,.F.) ;
#5824=ORIENTED_EDGE('',*,*,#4423,.F.) ;
#5825=ORIENTED_EDGE('',*,*,#4427,.F.) ;
#5826=ORIENTED_EDGE('',*,*,#4435,.F.) ;
#5827=ORIENTED_EDGE('',*,*,#4436,.T.) ;
#5828=ORIENTED_EDGE('',*,*,#4437,.T.) ;
#5829=ORIENTED_EDGE('',*,*,#4362,.T.) ;
#5830=ORIENTED_EDGE('',*,*,#4437,.F.) ;
#5831=ORIENTED_EDGE('',*,*,#4436,.F.) ;
#5832=ORIENTED_EDGE('',*,*,#4434,.F.) ;
#5833=ORIENTED_EDGE('',*,*,#4424,.F.) ;
#5834=ORIENTED_EDGE('',*,*,#4357,.F.) ;
#5835=ORIENTED_EDGE('',*,*,#4393,.F.) ;
#5836=ORIENTED_EDGE('',*,*,#4388,.F.) ;
#5837=ORIENTED_EDGE('',*,*,#4430,.F.) ;
#5838=ORIENTED_EDGE('',*,*,#4438,.T.) ;
#5839=ORIENTED_EDGE('',*,*,#4439,.T.) ;
#5840=ORIENTED_EDGE('',*,*,#4440,.T.) ;
#5841=ORIENTED_EDGE('',*,*,#4438,.F.) ;
#5842=ORIENTED_EDGE('',*,*,#4429,.F.) ;
#5843=ORIENTED_EDGE('',*,*,#4395,.F.) ;
#5844=ORIENTED_EDGE('',*,*,#4380,.F.) ;
#5845=ORIENTED_EDGE('',*,*,#4428,.F.) ;
#5846=ORIENTED_EDGE('',*,*,#4441,.T.) ;
#5847=ORIENTED_EDGE('',*,*,#4363,.T.) ;
#5848=ORIENTED_EDGE('',*,*,#4441,.F.) ;
#5849=ORIENTED_EDGE('',*,*,#4439,.F.) ;
#5850=ORIENTED_EDGE('',*,*,#4440,.F.) ;
#5851=ORIENTED_EDGE('',*,*,#4409,.T.) ;
#5852=ORIENTED_EDGE('',*,*,#4421,.F.) ;
#5853=ORIENTED_EDGE('',*,*,#4418,.F.) ;
#5854=ORIENTED_EDGE('',*,*,#4413,.F.) ;
#5855=ORIENTED_EDGE('',*,*,#4432,.F.) ;
#5856=ORIENTED_EDGE('',*,*,#4401,.T.) ;
#5857=ORIENTED_EDGE('',*,*,#4442,.T.) ;
#5858=ORIENTED_EDGE('',*,*,#4443,.T.) ;
#5859=ORIENTED_EDGE('',*,*,#4444,.T.) ;
#5860=ORIENTED_EDGE('',*,*,#4442,.F.) ;
#5861=ORIENTED_EDGE('',*,*,#4445,.T.) ;
#5862=ORIENTED_EDGE('',*,*,#4446,.T.) ;
#5863=ORIENTED_EDGE('',*,*,#4406,.T.) ;
#5864=ORIENTED_EDGE('',*,*,#4420,.F.) ;
#5865=ORIENTED_EDGE('',*,*,#4411,.F.) ;
#5866=ORIENTED_EDGE('',*,*,#4403,.T.) ;
#5867=ORIENTED_EDGE('',*,*,#4433,.F.) ;
#5868=ORIENTED_EDGE('',*,*,#4340,.T.) ;
#5869=ORIENTED_EDGE('',*,*,#4416,.F.) ;
#5870=ORIENTED_EDGE('',*,*,#4422,.F.) ;
#5871=ORIENTED_EDGE('',*,*,#4407,.T.) ;
#5872=ORIENTED_EDGE('',*,*,#4446,.F.) ;
#5873=ORIENTED_EDGE('',*,*,#4447,.T.) ;
#5874=ORIENTED_EDGE('',*,*,#4448,.T.) ;
#5875=ORIENTED_EDGE('',*,*,#4365,.T.) ;
#5876=ORIENTED_EDGE('',*,*,#4448,.F.) ;
#5877=ORIENTED_EDGE('',*,*,#4447,.F.) ;
#5878=ORIENTED_EDGE('',*,*,#4445,.F.) ;
#5879=ORIENTED_EDGE('',*,*,#4449,.T.) ;
#5880=ORIENTED_EDGE('',*,*,#4364,.T.) ;
#5881=ORIENTED_EDGE('',*,*,#4449,.F.) ;
#5882=ORIENTED_EDGE('',*,*,#4443,.F.) ;
#5883=ORIENTED_EDGE('',*,*,#4444,.F.) ;
#8123=CYLINDRICAL_SURFACE('',#8755,1.2500000000303) ;
#8124=CYLINDRICAL_SURFACE('',#8757,1.2500000000303) ;
#8125=CYLINDRICAL_SURFACE('',#8758,1.2500000000303) ;
#8126=CYLINDRICAL_SURFACE('',#8759,1.2500000000303) ;
#8127=CYLINDRICAL_SURFACE('',#8760,1.2500000000303) ;
#8128=CYLINDRICAL_SURFACE('',#8761,1.25000000003033) ;
#8129=CYLINDRICAL_SURFACE('',#8763,1.25000000003033) ;
#8130=CYLINDRICAL_SURFACE('',#8764,1.25000000003033) ;
#8131=CYLINDRICAL_SURFACE('',#8765,1.25000000003033) ;
#8132=CYLINDRICAL_SURFACE('',#8766,1.25000000003033) ;
#8133=CYLINDRICAL_SURFACE('',#8767,2.00000000000006) ;
#8134=CYLINDRICAL_SURFACE('',#8780,1.25000000003033) ;
#8135=CYLINDRICAL_SURFACE('',#8783,1.2500000000303) ;
#8136=CYLINDRICAL_SURFACE('',#8784,1.2500000000303) ;
#8137=CYLINDRICAL_SURFACE('',#8789,1.25000000003033) ;
#8138=CYLINDRICAL_SURFACE('',#8790,0.300000000000011) ;
#8139=CYLINDRICAL_SURFACE('',#8791,0.300000000000011) ;
#8140=CYLINDRICAL_SURFACE('',#8792,0.299999999999991) ;
#8141=CYLINDRICAL_SURFACE('',#8793,0.299999999999991) ;
#8253=ADVANCED_FACE('',(#870),#8123,.F.) ;
#8254=ADVANCED_FACE('',(#871),#8124,.F.) ;
#8255=ADVANCED_FACE('',(#872),#8125,.F.) ;
#8256=ADVANCED_FACE('',(#873),#8126,.F.) ;
#8257=ADVANCED_FACE('',(#874),#8127,.F.) ;
#8258=ADVANCED_FACE('',(#875),#8128,.F.) ;
#8259=ADVANCED_FACE('',(#876),#8129,.F.) ;
#8260=ADVANCED_FACE('',(#877),#8130,.F.) ;
#8261=ADVANCED_FACE('',(#878),#8131,.F.) ;
#8262=ADVANCED_FACE('',(#879),#8132,.F.) ;
#8263=ADVANCED_FACE('',(#880,#558,#559,#560,#561),#8133,.T.) ;
#8264=ADVANCED_FACE('',(#881,#562),#359,.T.) ;
#8265=ADVANCED_FACE('',(#882,#563),#360,.T.) ;
#8266=ADVANCED_FACE('',(#883),#817,.T.) ;
#8267=ADVANCED_FACE('',(#884),#818,.T.) ;
#8268=ADVANCED_FACE('',(#885),#311,.F.) ;
#8269=ADVANCED_FACE('',(#886),#312,.F.) ;
#8270=ADVANCED_FACE('',(#887),#819,.T.) ;
#8271=ADVANCED_FACE('',(#888),#820,.T.) ;
#8272=ADVANCED_FACE('',(#889),#361,.T.) ;
#8273=ADVANCED_FACE('',(#890),#8134,.F.) ;
#8274=ADVANCED_FACE('',(#891),#821,.T.) ;
#8275=ADVANCED_FACE('',(#892),#362,.T.) ;
#8276=ADVANCED_FACE('',(#893),#8135,.F.) ;
#8277=ADVANCED_FACE('',(#894),#8136,.F.) ;
#8278=ADVANCED_FACE('',(#895),#822,.T.) ;
#8279=ADVANCED_FACE('',(#896),#823,.T.) ;
#8280=ADVANCED_FACE('',(#897),#824,.T.) ;
#8281=ADVANCED_FACE('',(#898),#363,.T.) ;
#8282=ADVANCED_FACE('',(#899),#364,.T.) ;
#8283=ADVANCED_FACE('',(#900),#825,.T.) ;
#8284=ADVANCED_FACE('',(#901),#8137,.F.) ;
#8285=ADVANCED_FACE('',(#902),#826,.T.) ;
#8286=ADVANCED_FACE('',(#903),#8138,.F.) ;
#8287=ADVANCED_FACE('',(#904),#827,.T.) ;
#8288=ADVANCED_FACE('',(#905),#8139,.F.) ;
#8289=ADVANCED_FACE('',(#906),#828,.T.) ;
#8290=ADVANCED_FACE('',(#907),#8140,.F.) ;
#8291=ADVANCED_FACE('',(#908),#8141,.F.) ;
#8292=ADVANCED_FACE('',(#909),#829,.T.) ;
#8293=ADVANCED_FACE('',(#910),#830,.T.) ;
#8716=CLOSED_SHELL('',(#8253,#8254,#8255,#8256,#8257,#8258,#8259,#8260,
#8261,#8262,#8263,#8264,#8265,#8266,#8267,#8268,#8269,#8270,#8271,#8272,
#8273,#8274,#8275,#8276,#8277,#8278,#8279,#8280,#8281,#8282,#8283,#8284,
#8285,#8286,#8287,#8288,#8289,#8290,#8291,#8292,#8293)) ;
#8755=AXIS2_PLACEMENT_3D('',#12440,#9482,#9483) ;
#8756=AXIS2_PLACEMENT_3D('',#12524,#9485,#9486) ;
#8757=AXIS2_PLACEMENT_3D('',#12707,#9487,#9488) ;
#8758=AXIS2_PLACEMENT_3D('',#12981,#9490,#9491) ;
#8759=AXIS2_PLACEMENT_3D('',#13952,#9493,#9494) ;
#8760=AXIS2_PLACEMENT_3D('',#15016,#9496,#9497) ;
#8761=AXIS2_PLACEMENT_3D('',#15154,#9499,#9500) ;
#8762=AXIS2_PLACEMENT_3D('',#15666,#9502,#9503) ;
#8763=AXIS2_PLACEMENT_3D('',#15761,#9504,#9505) ;
#8764=AXIS2_PLACEMENT_3D('',#16031,#9507,#9508) ;
#8765=AXIS2_PLACEMENT_3D('',#16286,#9510,#9511) ;
#8766=AXIS2_PLACEMENT_3D('',#17908,#9513,#9514) ;
#8767=AXIS2_PLACEMENT_3D('',#18436,#9516,#9517) ;
#8768=AXIS2_PLACEMENT_3D('',#18438,#9518,#9519) ;
#8769=AXIS2_PLACEMENT_3D('',#18441,#9521,#9522) ;
#8770=AXIS2_PLACEMENT_3D('',#18510,#9523,#9524) ;
#8771=AXIS2_PLACEMENT_3D('',#18699,#9525,#9526) ;
#8772=AXIS2_PLACEMENT_3D('',#18966,#9529,#9530) ;
#8773=AXIS2_PLACEMENT_3D('',#18971,#9532,#9533) ;
#8774=AXIS2_PLACEMENT_3D('',#18972,#9534,#9535) ;
#8775=AXIS2_PLACEMENT_3D('',#18973,#9536,#9537) ;
#8776=AXIS2_PLACEMENT_3D('',#18976,#9538,#9539) ;
#8777=AXIS2_PLACEMENT_3D('',#18979,#9541,#9542) ;
#8778=AXIS2_PLACEMENT_3D('',#33345,#9543,#9544) ;
#8779=AXIS2_PLACEMENT_3D('',#33349,#9546,#9547) ;
#8780=AXIS2_PLACEMENT_3D('',#33358,#9549,#9550) ;
#8781=AXIS2_PLACEMENT_3D('',#41428,#9551,#9552) ;
#8782=AXIS2_PLACEMENT_3D('',#41431,#9554,#9555) ;
#8783=AXIS2_PLACEMENT_3D('',#41432,#9556,#9557) ;
#8784=AXIS2_PLACEMENT_3D('',#42521,#9558,#9559) ;
#8785=AXIS2_PLACEMENT_3D('',#43217,#9560,#9561) ;
#8786=AXIS2_PLACEMENT_3D('',#43241,#9562,#9563) ;
#8787=AXIS2_PLACEMENT_3D('',#64559,#9565,#9566) ;
#8788=AXIS2_PLACEMENT_3D('',#64561,#9568,#9569) ;
#8789=AXIS2_PLACEMENT_3D('',#71960,#9572,#9573) ;
#8790=AXIS2_PLACEMENT_3D('',#79036,#9575,#9576) ;
#8791=AXIS2_PLACEMENT_3D('',#79092,#9579,#9580) ;
#8792=AXIS2_PLACEMENT_3D('',#79148,#9583,#9584) ;
#8793=AXIS2_PLACEMENT_3D('',#79171,#9586,#9587) ;
#9482=DIRECTION('center_axis',(0.,1.,0.)) ;
#9483=DIRECTION('ref_axis',(-0.946103896364967,0.,-0.323863269425582)) ;
#9484=DIRECTION('',(0.,-1.,0.)) ;
#9485=DIRECTION('center_axis',(1.35769304206411E-14,-1.,2.27077106269489E-14)) ;
#9486=DIRECTION('ref_axis',(-0.0146228552552955,-2.30926389116428E-14,-0.999893080336184)) ;
#9487=DIRECTION('center_axis',(0.,1.,0.)) ;
#9488=DIRECTION('ref_axis',(-0.946103896364967,0.,-0.323863269425582)) ;
#9489=DIRECTION('',(0.,-1.,0.)) ;
#9490=DIRECTION('center_axis',(0.,1.,0.)) ;
#9491=DIRECTION('ref_axis',(-0.946103896364967,0.,-0.323863269425582)) ;
#9492=DIRECTION('',(0.,-1.,0.)) ;
#9493=DIRECTION('center_axis',(0.,1.,0.)) ;
#9494=DIRECTION('ref_axis',(-0.946103896364967,0.,-0.323863269425582)) ;
#9495=DIRECTION('',(0.,-1.,0.)) ;
#9496=DIRECTION('center_axis',(0.,1.,0.)) ;
#9497=DIRECTION('ref_axis',(-0.946103896364967,0.,-0.323863269425582)) ;
#9498=DIRECTION('',(0.,-1.,0.)) ;
#9499=DIRECTION('center_axis',(0.,-1.,0.)) ;
#9500=DIRECTION('ref_axis',(0.94610389636497,0.,0.323863269425573)) ;
#9501=DIRECTION('',(0.,1.,0.)) ;
#9502=DIRECTION('center_axis',(-1.2327844441336E-14,1.,4.81473066124874E-15)) ;
#9503=DIRECTION('ref_axis',(0.624375708152623,1.06581410361413E-14,-0.781124173911492)) ;
#9504=DIRECTION('center_axis',(0.,-1.,0.)) ;
#9505=DIRECTION('ref_axis',(0.94610389636497,0.,0.323863269425573)) ;
#9506=DIRECTION('',(0.,1.,0.)) ;
#9507=DIRECTION('center_axis',(0.,-1.,0.)) ;
#9508=DIRECTION('ref_axis',(0.94610389636497,0.,0.323863269425573)) ;
#9509=DIRECTION('',(0.,1.,0.)) ;
#9510=DIRECTION('center_axis',(0.,-1.,0.)) ;
#9511=DIRECTION('ref_axis',(0.94610389636497,0.,0.323863269425573)) ;
#9512=DIRECTION('',(0.,1.,0.)) ;
#9513=DIRECTION('center_axis',(0.,-1.,0.)) ;
#9514=DIRECTION('ref_axis',(0.94610389636497,0.,0.323863269425573)) ;
#9515=DIRECTION('',(0.,1.,0.)) ;
#9516=DIRECTION('center_axis',(0.,-1.,0.)) ;
#9517=DIRECTION('ref_axis',(-0.999901327181056,0.,0.014047629748903)) ;
#9518=DIRECTION('center_axis',(0.,1.,0.)) ;
#9519=DIRECTION('ref_axis',(0.821908931733379,0.,0.569618914658647)) ;
#9520=DIRECTION('',(0.,1.,0.)) ;
#9521=DIRECTION('center_axis',(-5.43957754046731E-16,1.,-1.6588297649198E-16)) ;
#9522=DIRECTION('ref_axis',(0.821908931733384,0.,0.569618914658641)) ;
#9523=DIRECTION('center_axis',(0.,-1.,0.)) ;
#9524=DIRECTION('ref_axis',(0.,0.,-1.)) ;
#9525=DIRECTION('center_axis',(0.,1.,0.)) ;
#9526=DIRECTION('ref_axis',(0.,0.,1.)) ;
#9527=DIRECTION('',(-0.707037008967148,-0.707106781186553,0.00993317425505793)) ;
#9528=DIRECTION('',(-0.707037008967142,0.707106781186558,0.00993317425505808)) ;
#9529=DIRECTION('center_axis',(-8.17256413651962E-16,-1.,-6.22886289721765E-15)) ;
#9530=DIRECTION('ref_axis',(-0.958163708642318,-9.99764261907128E-16,0.286220732024778)) ;
#9531=DIRECTION('',(0.878436458273725,-0.399365905228251,-0.262404768471792)) ;
#9532=DIRECTION('center_axis',(1.34449450164033E-15,1.,4.60237386928538E-16)) ;
#9533=DIRECTION('ref_axis',(-0.946103896364975,1.42108547148575E-15,-0.32386326942556)) ;
#9534=DIRECTION('center_axis',(1.34449450164033E-15,1.,4.60237386928538E-16)) ;
#9535=DIRECTION('ref_axis',(-0.946103896364975,1.42108547148575E-15,-0.32386326942556)) ;
#9536=DIRECTION('center_axis',(-2.00418059528623E-15,1.,-4.42697272393356E-15)) ;
#9537=DIRECTION('ref_axis',(-0.958163708642327,-6.53241738270602E-16,0.286220732024745)) ;
#9538=DIRECTION('center_axis',(-1.34449450164033E-15,1.,-4.60237386928538E-16)) ;
#9539=DIRECTION('ref_axis',(-0.946103896364975,-1.42108547148575E-15,-0.32386326942556)) ;
#9540=DIRECTION('',(-0.878436458273733,-0.399365905228253,0.262404768471762)) ;
#9541=DIRECTION('center_axis',(-1.34449450164033E-15,1.,-4.60237386928538E-16)) ;
#9542=DIRECTION('ref_axis',(-0.946103896364975,-1.42108547148575E-15,-0.32386326942556)) ;
#9543=DIRECTION('center_axis',(0.,1.,0.)) ;
#9544=DIRECTION('ref_axis',(0.,0.,1.)) ;
#9545=DIRECTION('',(0.946101641249305,0.,0.323869857234926)) ;
#9546=DIRECTION('center_axis',(-6.39729583226389E-16,-1.,-3.91154895135122E-16)) ;
#9547=DIRECTION('ref_axis',(0.996177335286308,-1.42108547148575E-15,0.0873539733605267)) ;
#9548=DIRECTION('',(0.946101641249524,1.83728335216313E-14,0.323869857234287)) ;
#9549=DIRECTION('center_axis',(0.,-1.,0.)) ;
#9550=DIRECTION('ref_axis',(0.94610389636497,0.,0.323863269425573)) ;
#9551=DIRECTION('center_axis',(0.,1.,0.)) ;
#9552=DIRECTION('ref_axis',(0.,0.,1.)) ;
#9553=DIRECTION('',(-0.946101641249542,0.,-0.323869857234233)) ;
#9554=DIRECTION('center_axis',(8.666064370551E-16,-1.,-2.17100603559229E-15)) ;
#9555=DIRECTION('ref_axis',(-0.85456353911045,-2.84217094297147E-15,0.51934685675666)) ;
#9556=DIRECTION('center_axis',(0.,1.,0.)) ;
#9557=DIRECTION('ref_axis',(-0.946103896364967,0.,-0.323863269425582)) ;
#9558=DIRECTION('center_axis',(0.,1.,0.)) ;
#9559=DIRECTION('ref_axis',(-0.946103896364967,0.,-0.323863269425582)) ;
#9560=DIRECTION('center_axis',(-8.0112472999825E-16,-1.,2.45282936024342E-15)) ;
#9561=DIRECTION('ref_axis',(-0.996179841145295,0.,-0.087325392044553)) ;
#9562=DIRECTION('center_axis',(4.89721590946324E-33,-1.,-1.43059439030947E-32)) ;
#9563=DIRECTION('ref_axis',(-0.840728824371145,0.,-0.541456409945908)) ;
#9564=DIRECTION('',(0.,-1.,0.)) ;
#9565=DIRECTION('center_axis',(0.,-1.,0.)) ;
#9566=DIRECTION('ref_axis',(0.,0.,-1.)) ;
#9567=DIRECTION('',(0.946101641249514,1.10210091516262E-14,0.323869857234315)) ;
#9568=DIRECTION('center_axis',(0.,-1.,0.)) ;
#9569=DIRECTION('ref_axis',(0.,0.,-1.)) ;
#9570=DIRECTION('',(-0.946101641249307,0.,-0.32386985723492)) ;
#9571=DIRECTION('',(-0.946101641249533,0.,-0.323869857234259)) ;
#9572=DIRECTION('center_axis',(0.,-1.,0.)) ;
#9573=DIRECTION('ref_axis',(0.94610389636497,0.,0.323863269425573)) ;
#9574=DIRECTION('',(0.,1.,0.)) ;
#9575=DIRECTION('center_axis',(-0.946101641249535,-2.18705461187032E-30,
-0.323869857234255)) ;
#9576=DIRECTION('ref_axis',(1.6950188065742E-15,1.,0.)) ;
#9577=DIRECTION('',(0.946101641249535,2.18705461187032E-30,0.323869857234254)) ;
#9578=DIRECTION('',(-0.668994874693665,0.707106793246477,-0.229010568704352)) ;
#9579=DIRECTION('center_axis',(-0.946101641249535,-2.18705461187032E-30,
-0.323869857234255)) ;
#9580=DIRECTION('ref_axis',(1.6950188065742E-15,1.,0.)) ;
#9581=DIRECTION('',(0.946101641249535,2.18705461187032E-30,0.323869857234254)) ;
#9582=DIRECTION('',(0.668994876573621,0.707106791113638,0.229010569798033)) ;
#9583=DIRECTION('center_axis',(-0.946101641249535,-1.74964368949631E-30,
-0.323869857234254)) ;
#9584=DIRECTION('ref_axis',(-1.69501880657431E-15,-1.,0.)) ;
#9585=DIRECTION('',(0.946101641249535,1.74964368949631E-30,0.323869857234254)) ;
#9586=DIRECTION('center_axis',(-0.946101641249535,-1.74964368949631E-30,
-0.323869857234254)) ;
#9587=DIRECTION('ref_axis',(-1.69501880657431E-15,-1.,0.)) ;
#9588=DIRECTION('',(0.946101641249535,1.74964368949631E-30,0.323869857234254)) ;
#9589=DIRECTION('',(-0.668994882500867,-0.707106785016779,-0.229010571308153)) ;
#9590=DIRECTION('',(0.668994877081364,-0.707106791113096,0.229010568316467)) ;
#12440=CARTESIAN_POINT('Origin',(-19.4092722359532,-13.9601742359176,123.411814366564)) ;
#12441=CARTESIAN_POINT('',(-18.2266423654683,-13.7497401139871,123.816643453356)) ;
#12442=CARTESIAN_POINT('',(-18.2266423654683,-13.8098218143905,123.816643453356)) ;
#12443=CARTESIAN_POINT('',(-18.2266423654683,-13.9601742359176,123.816643453356)) ;
#12444=CARTESIAN_POINT('',(-20.5919020986874,-13.9898268235108,123.006985257131)) ;
#12445=CARTESIAN_POINT('Ctrl Pts',(-18.2266423654683,-13.8098218143905,
123.816643453356)) ;
#12446=CARTESIAN_POINT('Ctrl Pts',(-18.237831871297,-13.8114016285963,123.849331430235)) ;
#12447=CARTESIAN_POINT('Ctrl Pts',(-18.2503723181934,-13.8129755447532,
123.881541832065)) ;
#12448=CARTESIAN_POINT('Ctrl Pts',(-18.2642254820877,-13.8145603623162,
123.913180431967)) ;
#12449=CARTESIAN_POINT('Ctrl Pts',(-18.293387889375,-13.8178965745782,123.979783104353)) ;
#12450=CARTESIAN_POINT('Ctrl Pts',(-18.3283004942603,-13.8212461938646,
124.043704483388)) ;
#12451=CARTESIAN_POINT('Ctrl Pts',(-18.368570392836,-13.8245506968226,124.104230190913)) ;
#12452=CARTESIAN_POINT('Ctrl Pts',(-18.4086263458682,-13.8278376436479,
124.16443433802)) ;
#12453=CARTESIAN_POINT('Ctrl Pts',(-18.4538295093184,-13.8311300264904,
124.221047239389)) ;
#12454=CARTESIAN_POINT('Ctrl Pts',(-18.5036720507278,-13.8344876377522,
124.27343394886)) ;
#12455=CARTESIAN_POINT('Ctrl Pts',(-18.5538218980809,-13.8378659504845,
124.326143650433)) ;
#12456=CARTESIAN_POINT('Ctrl Pts',(-18.6084761746544,-13.8412029173428,
124.374373283239)) ;
#12457=CARTESIAN_POINT('Ctrl Pts',(-18.6670195804605,-13.8444858761846,
124.417578253115)) ;
#12458=CARTESIAN_POINT('Ctrl Pts',(-18.7250431716585,-13.8477396852026,
124.460399600375)) ;
#12459=CARTESIAN_POINT('Ctrl Pts',(-18.7866588014402,-13.8510396003789,
124.498116602261)) ;
#12460=CARTESIAN_POINT('Ctrl Pts',(-18.8511838442244,-13.8543957488816,
124.530312174829)) ;
#12461=CARTESIAN_POINT('Ctrl Pts',(-18.8538780263867,-13.8545358816896,
124.531656470525)) ;
#12462=CARTESIAN_POINT('Ctrl Pts',(-18.8565786729133,-13.8546760972818,
124.532991824414)) ;
#12463=CARTESIAN_POINT('Ctrl Pts',(-18.8592826188426,-13.8548162117366,
124.534316669968)) ;
#12464=CARTESIAN_POINT('Ctrl Pts',(-18.9219079625751,-13.858061363866,124.565001051386)) ;
#12465=CARTESIAN_POINT('Ctrl Pts',(-18.9869884803353,-13.8612363658325,
124.590389744184)) ;
#12466=CARTESIAN_POINT('Ctrl Pts',(-19.053848666975,-13.8643940206219,124.610219175755)) ;
#12467=CARTESIAN_POINT('Ctrl Pts',(-19.1231784430325,-13.8676683085116,
124.630781039537)) ;
#12468=CARTESIAN_POINT('Ctrl Pts',(-19.1941569425128,-13.8709919984484,
124.645286729952)) ;
#12469=CARTESIAN_POINT('Ctrl Pts',(-19.2659898090002,-13.8743315341806,
124.653575271973)) ;
#12470=CARTESIAN_POINT('Ctrl Pts',(-19.3380668459781,-13.8776824214866,
124.66189198797)) ;
#12471=CARTESIAN_POINT('Ctrl Pts',(-19.4107314337425,-13.8809853979147,
124.663917527542)) ;
#12472=CARTESIAN_POINT('Ctrl Pts',(-19.4831611255667,-13.8843026555778,
124.659628628411)) ;
#12473=CARTESIAN_POINT('Ctrl Pts',(-19.5555009961429,-13.8876157994552,
124.655345048013)) ;
#12474=CARTESIAN_POINT('Ctrl Pts',(-19.6273312746973,-13.8909438819607,
124.64477956539)) ;
#12475=CARTESIAN_POINT('Ctrl Pts',(-19.6978504764238,-13.8942620357105,
124.628047320896)) ;
#12476=CARTESIAN_POINT('Ctrl Pts',(-19.7371131245775,-13.8961094687501,
124.618731386905)) ;
#12477=CARTESIAN_POINT('Ctrl Pts',(-19.7759127401105,-13.8979557647332,
124.607516713119)) ;
#12478=CARTESIAN_POINT('Ctrl Pts',(-19.8141025333163,-13.8998064971626,
124.594443822655)) ;
#12479=CARTESIAN_POINT('Ctrl Pts',(-19.8442734021559,-13.901268620958,124.58411592008)) ;
#12480=CARTESIAN_POINT('Ctrl Pts',(-19.8740391175611,-13.9027321500355,
124.572636509389)) ;
#12481=CARTESIAN_POINT('Ctrl Pts',(-19.9033228985707,-13.9041954603202,
124.560036445625)) ;
#12482=CARTESIAN_POINT('Ctrl Pts',(-19.9702090673073,-13.9075377615958,
124.531257033883)) ;
#12483=CARTESIAN_POINT('Ctrl Pts',(-20.0344429672726,-13.9108526467104,
124.496693112604)) ;
#12484=CARTESIAN_POINT('Ctrl Pts',(-20.0953021057173,-13.9142011387571,
124.456736860277)) ;
#12485=CARTESIAN_POINT('Ctrl Pts',(-20.1561612240545,-13.9175496296976,
124.416780621151)) ;
#12486=CARTESIAN_POINT('Ctrl Pts',(-20.2134131689817,-13.9209012130819,
124.371584177511)) ;
#12487=CARTESIAN_POINT('Ctrl Pts',(-20.2664070546696,-13.9242062414883,
124.321660453889)) ;
#12488=CARTESIAN_POINT('Ctrl Pts',(-20.3188879116673,-13.9274792742338,
124.272220037014)) ;
#12489=CARTESIAN_POINT('Ctrl Pts',(-20.3669908018908,-13.930769637394,124.218333654268)) ;
#12490=CARTESIAN_POINT('Ctrl Pts',(-20.4101800759874,-13.9341146887793,
124.16060238452)) ;
#12491=CARTESIAN_POINT('Ctrl Pts',(-20.4537632768795,-13.937490250179,124.1023445513)) ;
#12492=CARTESIAN_POINT('Ctrl Pts',(-20.4921765254999,-13.9408084513923,
124.040394209155)) ;
#12493=CARTESIAN_POINT('Ctrl Pts',(-20.5249854989838,-13.944113296651,123.975448924388)) ;
#12494=CARTESIAN_POINT('Ctrl Pts',(-20.5272755731685,-13.9443439756393,
123.970915728001)) ;
#12495=CARTESIAN_POINT('Ctrl Pts',(-20.5295394125655,-13.9445749823401,
123.966365762471)) ;
#12496=CARTESIAN_POINT('Ctrl Pts',(-20.5317741930428,-13.9448060533355,
123.961804690484)) ;
#12497=CARTESIAN_POINT('Ctrl Pts',(-20.5613319019382,-13.9478622502575,
123.901478927213)) ;
#12498=CARTESIAN_POINT('Ctrl Pts',(-20.5859770073022,-13.9509585031166,
123.838871618375)) ;
#12499=CARTESIAN_POINT('Ctrl Pts',(-20.6054716276694,-13.9540439669129,
123.774591178576)) ;
#12500=CARTESIAN_POINT('Ctrl Pts',(-20.6264743153418,-13.9573681164073,
123.705338124395)) ;
#12501=CARTESIAN_POINT('Ctrl Pts',(-20.6414226330833,-13.9606555846865,
123.634394702244)) ;
#12502=CARTESIAN_POINT('Ctrl Pts',(-20.650149436559,-13.9639885363328,123.562558431431)) ;
#12503=CARTESIAN_POINT('Ctrl Pts',(-20.6589235477942,-13.9673395558174,
123.490332738187)) ;
#12504=CARTESIAN_POINT('Ctrl Pts',(-20.6613751505953,-13.9706784023529,
123.41747960217)) ;
#12505=CARTESIAN_POINT('Ctrl Pts',(-20.65747594891,-13.9739866550751,123.344825628431)) ;
#12506=CARTESIAN_POINT('Ctrl Pts',(-20.6536031184412,-13.9772725333073,
123.272663030576)) ;
#12507=CARTESIAN_POINT('Ctrl Pts',(-20.6434804026981,-13.9805825593519,
123.200973456345)) ;
#12508=CARTESIAN_POINT('Ctrl Pts',(-20.6272177792161,-13.9839176336044,
123.13055176023)) ;
#12509=CARTESIAN_POINT('Ctrl Pts',(-20.6175741403921,-13.9858953127641,
123.088792114042)) ;
#12510=CARTESIAN_POINT('Ctrl Pts',(-20.6057862739718,-13.9878667772688,
123.047545187057)) ;
#12511=CARTESIAN_POINT('Ctrl Pts',(-20.5919020986876,-13.9898268235108,
123.006985257131)) ;
#12512=CARTESIAN_POINT('',(-20.5016202458523,-13.9999999999504,122.804133672988)) ;
#12513=CARTESIAN_POINT('Ctrl Pts',(-20.5919020986876,-13.9898268235109,
123.006985257131)) ;
#12514=CARTESIAN_POINT('Ctrl Pts',(-20.5829797836085,-13.9910863977926,
122.98092044111)) ;
#12515=CARTESIAN_POINT('Ctrl Pts',(-20.5732018900406,-13.9923407865095,
122.95516708369)) ;
#12516=CARTESIAN_POINT('Ctrl Pts',(-20.5589092931437,-13.9940330998902,
122.920973150037)) ;
#12517=CARTESIAN_POINT('Ctrl Pts',(-20.5551412455448,-13.9944678789148,
122.912239873399)) ;
#12518=CARTESIAN_POINT('Ctrl Pts',(-20.5468065244909,-13.9954058172095,
122.893512858021)) ;
#12519=CARTESIAN_POINT('Ctrl Pts',(-20.5422069987443,-13.9959090495036,
122.883534578517)) ;
#12520=CARTESIAN_POINT('Ctrl Pts',(-20.526250497057,-13.9976076684926,122.850085445758)) ;
#12521=CARTESIAN_POINT('Ctrl Pts',(-20.5142956053927,-13.9988037114221,
122.826918507055)) ;
#12522=CARTESIAN_POINT('Ctrl Pts',(-20.5016202458523,-13.9999999999504,
122.804133672988)) ;
#12523=CARTESIAN_POINT('',(-19.4275508050227,-13.9999999999504,122.161948016114)) ;
#12524=CARTESIAN_POINT('Origin',(-19.4092722359532,-13.9999999999504,123.411814366564)) ;
#12525=CARTESIAN_POINT('',(-20.5919020529002,-13.9297284766184,123.006985123376)) ;
#12526=CARTESIAN_POINT('Ctrl Pts',(-19.4275508050227,-13.9999999999504,
122.161948016114)) ;
#12527=CARTESIAN_POINT('Ctrl Pts',(-19.4313400989441,-13.9998265546944,
122.162003432335)) ;
#12528=CARTESIAN_POINT('Ctrl Pts',(-19.4351191276508,-13.999653443417,122.16207587392)) ;
#12529=CARTESIAN_POINT('Ctrl Pts',(-19.4429233390417,-13.9992956353971,
122.162260951395)) ;
#12530=CARTESIAN_POINT('Ctrl Pts',(-19.4469384386358,-13.9991113818313,
122.162375536062)) ;
#12531=CARTESIAN_POINT('Ctrl Pts',(-19.4568925373842,-13.9986541355976,
122.16270763557)) ;
#12532=CARTESIAN_POINT('Ctrl Pts',(-19.4628306599564,-13.9983809660134,
122.162948155404)) ;
#12533=CARTESIAN_POINT('Ctrl Pts',(-19.4831706784865,-13.9974438136556,
122.163917350673)) ;
#12534=CARTESIAN_POINT('Ctrl Pts',(-19.4975614785456,-13.9967782187756,
122.164852880824)) ;
#12535=CARTESIAN_POINT('Ctrl Pts',(-19.5339902925882,-13.9950870857167,
122.167854864106)) ;
#12536=CARTESIAN_POINT('Ctrl Pts',(-19.5559955461641,-13.9940591023316,
122.170258045284)) ;
#12537=CARTESIAN_POINT('Ctrl Pts',(-19.5928424694167,-13.9923365170248,
122.175275398734)) ;
#12538=CARTESIAN_POINT('Ctrl Pts',(-19.6077218672209,-13.991640719076,122.177575977864)) ;
#12539=CARTESIAN_POINT('Ctrl Pts',(-19.6261327352259,-13.9907806249149,
122.180764124246)) ;
#12540=CARTESIAN_POINT('Ctrl Pts',(-19.6297065625804,-13.9906137014449,
122.181399037088)) ;
#12541=CARTESIAN_POINT('Ctrl Pts',(-19.6362191814793,-13.990309578876,122.182585330092)) ;
#12542=CARTESIAN_POINT('Ctrl Pts',(-19.6391588541742,-13.9901723273278,
122.183131704924)) ;
#12543=CARTESIAN_POINT('Ctrl Pts',(-19.6449603074068,-13.9899015045205,
122.184231526615)) ;
#12544=CARTESIAN_POINT('Ctrl Pts',(-19.647822168119,-13.9897679284137,122.18478444603)) ;
#12545=CARTESIAN_POINT('Ctrl Pts',(-19.654434616522,-13.9894593362366,122.186085997644)) ;
#12546=CARTESIAN_POINT('Ctrl Pts',(-19.6581837571266,-13.9892844006816,
122.186841843616)) ;
#12547=CARTESIAN_POINT('Ctrl Pts',(-19.6690890614828,-13.9887756119914,
122.189092541385)) ;
#12548=CARTESIAN_POINT('Ctrl Pts',(-19.6762356664328,-13.988442258957,122.190632982731)) ;
#12549=CARTESIAN_POINT('Ctrl Pts',(-19.7082799404323,-13.9869472701456,
122.197834825916)) ;
#12550=CARTESIAN_POINT('Ctrl Pts',(-19.7330141597435,-13.9857932844965,
122.204195592942)) ;
#12551=CARTESIAN_POINT('Ctrl Pts',(-19.77189986965,-13.9839594567732,122.215476254775)) ;
#12552=CARTESIAN_POINT('Ctrl Pts',(-19.7861875528098,-13.9832812405568,
122.219900561472)) ;
#12553=CARTESIAN_POINT('Ctrl Pts',(-19.8073400288787,-13.9822683001325,
122.226868991719)) ;
#12554=CARTESIAN_POINT('Ctrl Pts',(-19.8142674640842,-13.9819351401419,
122.229218757883)) ;
#12555=CARTESIAN_POINT('Ctrl Pts',(-19.8256238694404,-13.9813864381683,
122.233182306854)) ;
#12556=CARTESIAN_POINT('Ctrl Pts',(-19.8300650540129,-13.9811712130438,
122.234760578939)) ;
#12557=CARTESIAN_POINT('Ctrl Pts',(-19.8380556278999,-13.9807827776198,
122.23765120823)) ;
#12558=CARTESIAN_POINT('Ctrl Pts',(-19.8416081886326,-13.9806096508407,
122.238954637732)) ;
#12559=CARTESIAN_POINT('Ctrl Pts',(-19.8481787379539,-13.9802886327113,
122.241399272334)) ;
#12560=CARTESIAN_POINT('Ctrl Pts',(-19.851198333927,-13.9801407832986,122.242536070278)) ;
#12561=CARTESIAN_POINT('Ctrl Pts',(-19.8578651656588,-13.9798136344481,
122.245075469938)) ;
#12562=CARTESIAN_POINT('Ctrl Pts',(-19.861510291863,-13.9796342864989,122.246483507899)) ;
#12563=CARTESIAN_POINT('Ctrl Pts',(-19.871770979672,-13.9791280781222,122.250502395653)) ;
#12564=CARTESIAN_POINT('Ctrl Pts',(-19.8783709302037,-13.9788008679235,
122.253152640202)) ;
#12565=CARTESIAN_POINT('Ctrl Pts',(-19.9053759425105,-13.9774554241485,
122.26426520365)) ;
#12566=CARTESIAN_POINT('Ctrl Pts',(-19.9255774279037,-13.976433158422,122.273211317236)) ;
#12567=CARTESIAN_POINT('Ctrl Pts',(-19.9625548125104,-13.9745363265479,
122.290773079595)) ;
#12568=CARTESIAN_POINT('Ctrl Pts',(-19.9793935891346,-13.9736625907819,
122.299242200312)) ;
#12569=CARTESIAN_POINT('Ctrl Pts',(-20.0030028643973,-13.9724270345094,
122.311793356447)) ;
#12570=CARTESIAN_POINT('Ctrl Pts',(-20.0099360213834,-13.9720628560408,
122.315563802345)) ;
#12571=CARTESIAN_POINT('Ctrl Pts',(-20.0173571119298,-13.9716716660796,
122.319691139405)) ;
#12572=CARTESIAN_POINT('Ctrl Pts',(-20.0178809821164,-13.9716440436766,
122.319982990487)) ;
#12573=CARTESIAN_POINT('Ctrl Pts',(-20.0186824307534,-13.9716017737803,
122.320430238153)) ;
#12574=CARTESIAN_POINT('Ctrl Pts',(-20.0189601601499,-13.9715871237066,
122.320585363851)) ;
#12575=CARTESIAN_POINT('Ctrl Pts',(-20.0197876471307,-13.9715434679437,
122.321047971057)) ;
#12576=CARTESIAN_POINT('Ctrl Pts',(-20.020337231717,-13.9715144652276,122.321355762212)) ;
#12577=CARTESIAN_POINT('Ctrl Pts',(-20.0213193983153,-13.9714626194997,
122.321906793688)) ;
#12578=CARTESIAN_POINT('Ctrl Pts',(-20.0217520684562,-13.9714397749691,
122.322149876391)) ;
#12579=CARTESIAN_POINT('Ctrl Pts',(-20.0225225239134,-13.9713990865927,
122.322583337473)) ;
#12580=CARTESIAN_POINT('Ctrl Pts',(-20.0228603655731,-13.9713812417699,
122.322773615441)) ;
#12581=CARTESIAN_POINT('Ctrl Pts',(-20.0234603996002,-13.9713495423621,
122.3231119323)) ;
#12582=CARTESIAN_POINT('Ctrl Pts',(-20.023722627053,-13.971335687167,122.323259908756)) ;
#12583=CARTESIAN_POINT('Ctrl Pts',(-20.0241874961885,-13.9713111217335,
122.323522458574)) ;
#12584=CARTESIAN_POINT('Ctrl Pts',(-20.0243901593995,-13.9713004111175,
122.323636993834)) ;
#12585=CARTESIAN_POINT('Ctrl Pts',(-20.0287511708992,-13.9710699102416,
122.326103230215)) ;
#12586=CARTESIAN_POINT('Ctrl Pts',(-20.0328960444638,-13.9708503582615,
122.328478699236)) ;
#12587=CARTESIAN_POINT('Ctrl Pts',(-20.0401386450013,-13.9704658746123,
122.332684846911)) ;
#12588=CARTESIAN_POINT('Ctrl Pts',(-20.0432422701575,-13.9703008392668,
122.334505245617)) ;
#12589=CARTESIAN_POINT('Ctrl Pts',(-20.0494089887849,-13.9699723614362,
122.338158146935)) ;
#12590=CARTESIAN_POINT('Ctrl Pts',(-20.0524721788521,-13.9698089183065,
122.339990419353)) ;
#12591=CARTESIAN_POINT('Ctrl Pts',(-20.0597411972348,-13.9694203765605,
122.344380826212)) ;
#12592=CARTESIAN_POINT('Ctrl Pts',(-20.0639398478046,-13.9691954007169,
122.346950736389)) ;
#12593=CARTESIAN_POINT('Ctrl Pts',(-20.0823086507002,-13.9682085640206,
122.358343617163)) ;
#12594=CARTESIAN_POINT('Ctrl Pts',(-20.0963164762467,-13.9674493441243,
122.367425142087)) ;
#12595=CARTESIAN_POINT('Ctrl Pts',(-20.1213689212244,-13.9660749163178,
122.384389298333)) ;
#12596=CARTESIAN_POINT('Ctrl Pts',(-20.132474838872,-13.9654594559669,122.392176223856)) ;
#12597=CARTESIAN_POINT('Ctrl Pts',(-20.1571536534888,-13.9640732867552,
122.410085864093)) ;
#12598=CARTESIAN_POINT('Ctrl Pts',(-20.1706519807994,-13.9633021838136,
122.420306676723)) ;
#12599=CARTESIAN_POINT('Ctrl Pts',(-20.1902573263851,-13.9621613987188,
122.435788183106)) ;
#12600=CARTESIAN_POINT('Ctrl Pts',(-20.1965276577979,-13.9617933117389,
122.440838711654)) ;
#12601=CARTESIAN_POINT('Ctrl Pts',(-20.2068064265991,-13.9611844404265,
122.449282916893)) ;
#12602=CARTESIAN_POINT('Ctrl Pts',(-20.2108430570657,-13.9609439064896,
122.452641913128)) ;
#12603=CARTESIAN_POINT('Ctrl Pts',(-20.2197349388992,-13.9604108763614,
122.46013643701)) ;
#12604=CARTESIAN_POINT('Ctrl Pts',(-20.2245799470123,-13.9601183077058,
122.464283886588)) ;
#12605=CARTESIAN_POINT('Ctrl Pts',(-20.2352820252772,-13.9594672759103,
122.473587996888)) ;
#12606=CARTESIAN_POINT('Ctrl Pts',(-20.2411229747021,-13.9591087169046,
122.478762791973)) ;
#12607=CARTESIAN_POINT('Ctrl Pts',(-20.2569437608605,-13.9581286420425,
122.493045878624)) ;
#12608=CARTESIAN_POINT('Ctrl Pts',(-20.2668249758572,-13.9575066710911,
122.502261814118)) ;
#12609=CARTESIAN_POINT('Ctrl Pts',(-20.2945935725675,-13.9557310272155,
122.529015648875)) ;
#12610=CARTESIAN_POINT('Ctrl Pts',(-20.3121059166192,-13.9545778178095,
122.546933565339)) ;
#12611=CARTESIAN_POINT('Ctrl Pts',(-20.3370085670051,-13.9528889187766,
122.573994098076)) ;
#12612=CARTESIAN_POINT('Ctrl Pts',(-20.3448272295371,-13.9523509602435,
122.582733937836)) ;
#12613=CARTESIAN_POINT('Ctrl Pts',(-20.3600652353632,-13.9512864797164,
122.600257326914)) ;
#12614=CARTESIAN_POINT('Ctrl Pts',(-20.3674886746231,-13.9507599910363,
122.609035808208)) ;
#12615=CARTESIAN_POINT('Ctrl Pts',(-20.3879539588389,-13.949284985644,122.633925116559)) ;
#12616=CARTESIAN_POINT('Ctrl Pts',(-20.4007177078815,-13.9483373362306,
122.650259722292)) ;
#12617=CARTESIAN_POINT('Ctrl Pts',(-20.4189775564808,-13.9469350335655,
122.674865618212)) ;
#12618=CARTESIAN_POINT('Ctrl Pts',(-20.4247907882943,-13.9464811282198,
122.682897113889)) ;
#12619=CARTESIAN_POINT('Ctrl Pts',(-20.4346542250202,-13.9456972002265,
122.696871376891)) ;
#12620=CARTESIAN_POINT('Ctrl Pts',(-20.4387498237064,-13.9453674144131,
122.702781505505)) ;
#12621=CARTESIAN_POINT('Ctrl Pts',(-20.4465129998918,-13.9447336976661,
122.714193186951)) ;
#12622=CARTESIAN_POINT('Ctrl Pts',(-20.4501883632713,-13.9444298562635,
122.71968914071)) ;
#12623=CARTESIAN_POINT('Ctrl Pts',(-20.463156107996,-13.9433443836467,122.739417396655)) ;
#12624=CARTESIAN_POINT('Ctrl Pts',(-20.4722016005217,-13.9425621315287,
122.753809756139)) ;
#12625=CARTESIAN_POINT('Ctrl Pts',(-20.4874546139563,-13.9411997355344,
122.779214648094)) ;
#12626=CARTESIAN_POINT('Ctrl Pts',(-20.4937938393718,-13.9406193020215,
122.79014521236)) ;
#12627=CARTESIAN_POINT('Ctrl Pts',(-20.5037522393955,-13.9396841060832,
122.807932272416)) ;
#12628=CARTESIAN_POINT('Ctrl Pts',(-20.5074752388329,-13.9393288726186,
122.814729593285)) ;
#12629=CARTESIAN_POINT('Ctrl Pts',(-20.5145480006963,-13.9386429369001,
122.827932758823)) ;
#12630=CARTESIAN_POINT('Ctrl Pts',(-20.5179058835757,-13.9383122056115,
122.834333904803)) ;
#12631=CARTESIAN_POINT('Ctrl Pts',(-20.5293114355171,-13.9371708050483,
122.856542520223)) ;
#12632=CARTESIAN_POINT('Ctrl Pts',(-20.5370780527677,-13.9363616963756,
122.872491944226)) ;
#12633=CARTESIAN_POINT('Ctrl Pts',(-20.5573951475415,-13.9341494952713,
122.916574527132)) ;
#12634=CARTESIAN_POINT('Ctrl Pts',(-20.5692492643665,-13.932747799697,122.945014618369)) ;
#12635=CARTESIAN_POINT('Ctrl Pts',(-20.5822750711628,-13.9310479712546,
122.979836339052)) ;
#12636=CARTESIAN_POINT('Ctrl Pts',(-20.5844636170084,-13.9307561760045,
122.985826238473)) ;
#12637=CARTESIAN_POINT('Ctrl Pts',(-20.58840503499,-13.9302189335495,122.996875207426)) ;
#12638=CARTESIAN_POINT('Ctrl Pts',(-20.5901681493033,-13.929974026106,123.001919861591)) ;
#12639=CARTESIAN_POINT('Ctrl Pts',(-20.5919020529013,-13.9297284766178,
123.006985123375)) ;
#12640=CARTESIAN_POINT('Ctrl Pts',(-20.5919020529002,-13.9297284766184,
123.006985123376)) ;
#12641=CARTESIAN_POINT('Ctrl Pts',(-20.6024246541309,-13.9282383012773,
123.037724867468)) ;
#12642=CARTESIAN_POINT('Ctrl Pts',(-20.6117446103661,-13.9267411197154,
123.068862757242)) ;
#12643=CARTESIAN_POINT('Ctrl Pts',(-20.6198408276881,-13.9252413439706,
123.100328115213)) ;
#12644=CARTESIAN_POINT('Ctrl Pts',(-20.6379709053181,-13.9218828557287,
123.170789339262)) ;
#12645=CARTESIAN_POINT('Ctrl Pts',(-20.6499146685378,-13.9185651787582,
123.242698766736)) ;
#12646=CARTESIAN_POINT('Ctrl Pts',(-20.6555359566546,-13.9152437317152,
123.31523932559)) ;
#12647=CARTESIAN_POINT('Ctrl Pts',(-20.6611343658999,-13.9119358030968,
123.387484641415)) ;
#12648=CARTESIAN_POINT('Ctrl Pts',(-20.6604401452033,-13.9086000938307,
123.460079826942)) ;
#12649=CARTESIAN_POINT('Ctrl Pts',(-20.6534612032785,-13.9052867540257,
123.53220462224)) ;
#12650=CARTESIAN_POINT('Ctrl Pts',(-20.6464800094602,-13.901972345106,123.604352690028)) ;
#12651=CARTESIAN_POINT('Ctrl Pts',(-20.6332366280487,-13.8986781273188,
123.675755651677)) ;
#12652=CARTESIAN_POINT('Ctrl Pts',(-20.6138811082396,-13.8953268861809,
123.745606914241)) ;
#12653=CARTESIAN_POINT('Ctrl Pts',(-20.5944401554272,-13.8919608530561,
123.815766492118)) ;
#12654=CARTESIAN_POINT('Ctrl Pts',(-20.5689075331187,-13.888617535704,123.884092649026)) ;
#12655=CARTESIAN_POINT('Ctrl Pts',(-20.5375717903147,-13.8853232938337,
123.949810756611)) ;
#12656=CARTESIAN_POINT('Ctrl Pts',(-20.5356609335309,-13.8851224106293,
123.953818253497)) ;
#12657=CARTESIAN_POINT('Ctrl Pts',(-20.5337286362003,-13.8849215188531,
123.957815753525)) ;
#12658=CARTESIAN_POINT('Ctrl Pts',(-20.5317752294988,-13.8847205822267,
123.961802575126)) ;
#12659=CARTESIAN_POINT('Ctrl Pts',(-20.5020529870819,-13.8816632121898,
124.022464432178)) ;
#12660=CARTESIAN_POINT('Ctrl Pts',(-20.4674642360604,-13.8785603363961,
124.080613672752)) ;
#12661=CARTESIAN_POINT('Ctrl Pts',(-20.4283471324293,-13.8754303943831,
124.135683384722)) ;
#12662=CARTESIAN_POINT('Ctrl Pts',(-20.3862144846183,-13.8720591646073,
124.194998430164)) ;
#12663=CARTESIAN_POINT('Ctrl Pts',(-20.3389839905469,-13.8687568953655,
124.250521590318)) ;
#12664=CARTESIAN_POINT('Ctrl Pts',(-20.2871913450968,-13.8654334148974,
124.301622232272)) ;
#12665=CARTESIAN_POINT('Ctrl Pts',(-20.2355216253904,-13.862117822447,124.352601590899)) ;
#12666=CARTESIAN_POINT('Ctrl Pts',(-20.1795096491898,-13.8587707311508,
124.398983559086)) ;
#12667=CARTESIAN_POINT('Ctrl Pts',(-20.1197902982936,-13.8554599676142,
124.440242333494)) ;
#12668=CARTESIAN_POINT('Ctrl Pts',(-20.060515588533,-13.8521738544067,124.481193915208)) ;
#12669=CARTESIAN_POINT('Ctrl Pts',(-19.9978127986901,-13.8488823096299,
124.51694345188)) ;
#12670=CARTESIAN_POINT('Ctrl Pts',(-19.9323811071369,-13.8455608652241,
124.547092794512)) ;
#12671=CARTESIAN_POINT('Ctrl Pts',(-19.893785334744,-13.8436016661073,124.564876793954)) ;
#12672=CARTESIAN_POINT('Ctrl Pts',(-19.8543076305284,-13.8416507393192,
124.580681111942)) ;
#12673=CARTESIAN_POINT('Ctrl Pts',(-19.814101322745,-13.8397085566956,124.594444237049)) ;
#12674=CARTESIAN_POINT('Ctrl Pts',(-19.785503854565,-13.8383271439561,124.604233510275)) ;
#12675=CARTESIAN_POINT('Ctrl Pts',(-19.7565607840212,-13.8369502231916,
124.612982255014)) ;
#12676=CARTESIAN_POINT('Ctrl Pts',(-19.7273292786425,-13.8355640133331,
124.620673215922)) ;
#12677=CARTESIAN_POINT('Ctrl Pts',(-19.6569681088544,-13.8322273618005,
124.639185605185)) ;
#12678=CARTESIAN_POINT('Ctrl Pts',(-19.5851249922426,-13.8288723975086,
124.651519743502)) ;
#12679=CARTESIAN_POINT('Ctrl Pts',(-19.5126168537562,-13.825567149945,124.657534997383)) ;
#12680=CARTESIAN_POINT('Ctrl Pts',(-19.440714796089,-13.8222895302752,124.663499970977)) ;
#12681=CARTESIAN_POINT('Ctrl Pts',(-19.3684348667034,-13.8190014895072,
124.663228499334)) ;
#12682=CARTESIAN_POINT('Ctrl Pts',(-19.2965827995173,-13.8156538984272,
124.65672444002)) ;
#12683=CARTESIAN_POINT('Ctrl Pts',(-19.2241237717474,-13.812278029026,124.650165438548)) ;
#12684=CARTESIAN_POINT('Ctrl Pts',(-19.1523768839061,-13.8089523611346,
124.637293312943)) ;
#12685=CARTESIAN_POINT('Ctrl Pts',(-19.0821535042039,-13.8056569319892,
124.618252651523)) ;
#12686=CARTESIAN_POINT('Ctrl Pts',(-19.012336785255,-13.8023805865408,124.599322253804)) ;
#12687=CARTESIAN_POINT('Ctrl Pts',(-18.9442978433093,-13.7990669066114,
124.574368048075)) ;
#12688=CARTESIAN_POINT('Ctrl Pts',(-18.878800215249,-13.7957175977018,124.54367099853)) ;
#12689=CARTESIAN_POINT('Ctrl Pts',(-18.8722681340602,-13.795383570984,124.540609580494)) ;
#12690=CARTESIAN_POINT('Ctrl Pts',(-18.8657617689437,-13.7950494529779,
124.537491232689)) ;
#12691=CARTESIAN_POINT('Ctrl Pts',(-18.8592840273916,-13.7947155573251,
124.53431736011)) ;
#12692=CARTESIAN_POINT('Ctrl Pts',(-18.8006996277619,-13.7916958202453,
124.505613001024)) ;
#12693=CARTESIAN_POINT('Ctrl Pts',(-18.7444522920878,-13.7887201278197,
124.472366521467)) ;
#12694=CARTESIAN_POINT('Ctrl Pts',(-18.691055332827,-13.7857602612236,124.434880581498)) ;
#12695=CARTESIAN_POINT('Ctrl Pts',(-18.6320350318466,-13.7824886850931,
124.393446921416)) ;
#12696=CARTESIAN_POINT('Ctrl Pts',(-18.5767130247363,-13.7791846808591,
124.346985418166)) ;
#12697=CARTESIAN_POINT('Ctrl Pts',(-18.525705839709,-13.7758516214606,124.296014809622)) ;
#12698=CARTESIAN_POINT('Ctrl Pts',(-18.4742416165445,-13.7724886969507,
124.244587490677)) ;
#12699=CARTESIAN_POINT('Ctrl Pts',(-18.42736553566,-13.7691782751684,124.188765347694)) ;
#12700=CARTESIAN_POINT('Ctrl Pts',(-18.385610641675,-13.7658541875205,124.12918243142)) ;
#12701=CARTESIAN_POINT('Ctrl Pts',(-18.3439058817256,-13.7625340910197,
124.069671054834)) ;
#12702=CARTESIAN_POINT('Ctrl Pts',(-18.3074701725757,-13.7591911677825,
124.006636261331)) ;
#12703=CARTESIAN_POINT('Ctrl Pts',(-18.2767175507807,-13.7558684310501,
123.940794408881)) ;
#12704=CARTESIAN_POINT('Ctrl Pts',(-18.2578201439997,-13.7538266178976,
123.900334760359)) ;
#12705=CARTESIAN_POINT('Ctrl Pts',(-18.2411044753891,-13.7517886023727,
123.858891710066)) ;
#12706=CARTESIAN_POINT('Ctrl Pts',(-18.2266423654683,-13.7497401139871,
123.816643453356)) ;
#12707=CARTESIAN_POINT('Origin',(-19.4092722359532,-13.9601742359176,123.411814366564)) ;
#12708=CARTESIAN_POINT('',(-18.2266423654683,-13.389762567023,123.816643453356)) ;
#12709=CARTESIAN_POINT('',(-18.2266423654683,-13.4498216097391,123.816643453356)) ;
#12710=CARTESIAN_POINT('',(-18.2266423654683,-13.9601742359176,123.816643453356)) ;
#12711=CARTESIAN_POINT('',(-20.5919018244023,-13.6298117104086,123.006984455878)) ;
#12712=CARTESIAN_POINT('Ctrl Pts',(-18.2266423654683,-13.4498216097391,
123.816643453356)) ;
#12713=CARTESIAN_POINT('Ctrl Pts',(-18.2411051331282,-13.451866762096,123.858893631524)) ;
#12714=CARTESIAN_POINT('Ctrl Pts',(-18.2578210120249,-13.4539192653427,
123.900335766088)) ;
#12715=CARTESIAN_POINT('Ctrl Pts',(-18.2767132755134,-13.4559701748973,
123.940785255369)) ;
#12716=CARTESIAN_POINT('Ctrl Pts',(-18.3074696069924,-13.4593090259637,
124.006636438382)) ;
#12717=CARTESIAN_POINT('Ctrl Pts',(-18.3439059816794,-13.4626146525442,
124.069671167035)) ;
#12718=CARTESIAN_POINT('Ctrl Pts',(-18.3856104692784,-13.4659567452903,
124.129182185416)) ;
#12719=CARTESIAN_POINT('Ctrl Pts',(-18.4273644851252,-13.4693028071056,
124.18876387908)) ;
#12720=CARTESIAN_POINT('Ctrl Pts',(-18.4742402852349,-13.4726487236205,
124.2445862188)) ;
#12721=CARTESIAN_POINT('Ctrl Pts',(-18.5257063424073,-13.4759548813671,
124.29601531196)) ;
#12722=CARTESIAN_POINT('Ctrl Pts',(-18.5767150680731,-13.4792316603312,
124.346987402078)) ;
#12723=CARTESIAN_POINT('Ctrl Pts',(-18.6320372107052,-13.4825256909799,
124.393448715711)) ;
#12724=CARTESIAN_POINT('Ctrl Pts',(-18.6910584062643,-13.4858646864138,
124.434882739118)) ;
#12725=CARTESIAN_POINT('Ctrl Pts',(-18.7444501579562,-13.4888852083368,
124.472364783803)) ;
#12726=CARTESIAN_POINT('Ctrl Pts',(-18.8006970773752,-13.4918805679309,
124.505611928027)) ;
#12727=CARTESIAN_POINT('Ctrl Pts',(-18.859286755982,-13.4948413716543,124.534318697022)) ;
#12728=CARTESIAN_POINT('Ctrl Pts',(-18.8657621299384,-13.4951686018384,
124.537491390041)) ;
#12729=CARTESIAN_POINT('Ctrl Pts',(-18.8722685020963,-13.4954958458738,
124.540609730944)) ;
#12730=CARTESIAN_POINT('Ctrl Pts',(-18.8787970831716,-13.4958229221628,
124.543669530601)) ;
#12731=CARTESIAN_POINT('Ctrl Pts',(-18.9443008042512,-13.4991046021717,
124.574369656864)) ;
#12732=CARTESIAN_POINT('Ctrl Pts',(-19.0123400187616,-13.5024091769527,
124.599323127993)) ;
#12733=CARTESIAN_POINT('Ctrl Pts',(-19.0821534630279,-13.5057638741365,
124.618252640358)) ;
#12734=CARTESIAN_POINT('Ctrl Pts',(-19.1523733052118,-13.5091380996785,
124.637292345173)) ;
#12735=CARTESIAN_POINT('Ctrl Pts',(-19.2241200758587,-13.5124685609189,
124.650165107281)) ;
#12736=CARTESIAN_POINT('Ctrl Pts',(-19.2965828555023,-13.5157624361232,
124.656724445088)) ;
#12737=CARTESIAN_POINT('Ctrl Pts',(-19.3684380285421,-13.5190286919022,
124.663228782286)) ;
#12738=CARTESIAN_POINT('Ctrl Pts',(-19.4407179870657,-13.5223421499354,
124.663499697653)) ;
#12739=CARTESIAN_POINT('Ctrl Pts',(-19.5126167057451,-13.525677463468,124.657535009662)) ;
#12740=CARTESIAN_POINT('Ctrl Pts',(-19.585123561392,-13.5290409878991,124.651519870879)) ;
#12741=CARTESIAN_POINT('Ctrl Pts',(-19.6569671415057,-13.5323424562459,
124.639186510576)) ;
#12742=CARTESIAN_POINT('Ctrl Pts',(-19.7273397362501,-13.5356766263208,
124.620670464423)) ;
#12743=CARTESIAN_POINT('Ctrl Pts',(-19.7565608213304,-13.5370610866747,
124.612981974864)) ;
#12744=CARTESIAN_POINT('Ctrl Pts',(-19.7855040203861,-13.538454324686,124.604233408267)) ;
#12745=CARTESIAN_POINT('Ctrl Pts',(-19.8140996478306,-13.5398436253275,
124.594444810392)) ;
#12746=CARTESIAN_POINT('Ctrl Pts',(-19.8543069293484,-13.5417970709064,
124.58068141558)) ;
#12747=CARTESIAN_POINT('Ctrl Pts',(-19.8937845784459,-13.5437386231534,
124.564876738282)) ;
#12748=CARTESIAN_POINT('Ctrl Pts',(-19.9323712999088,-13.5456743108948,
124.547097313395)) ;
#12749=CARTESIAN_POINT('Ctrl Pts',(-19.9978143159808,-13.5489572341173,
124.516943438059)) ;
#12750=CARTESIAN_POINT('Ctrl Pts',(-20.0605169122456,-13.5522582528221,
124.481192993183)) ;
#12751=CARTESIAN_POINT('Ctrl Pts',(-20.119790210187,-13.5555757593791,124.440242394365)) ;
#12752=CARTESIAN_POINT('Ctrl Pts',(-20.1795094803893,-13.5589182268535,
124.398983683265)) ;
#12753=CARTESIAN_POINT('Ctrl Pts',(-20.2355214723119,-13.5622118339914,
124.352601702896)) ;
#12754=CARTESIAN_POINT('Ctrl Pts',(-20.2871910044519,-13.5655509085027,
124.301622568366)) ;
#12755=CARTESIAN_POINT('Ctrl Pts',(-20.3389824289868,-13.5688978601473,
124.250523170142)) ;
#12756=CARTESIAN_POINT('Ctrl Pts',(-20.386213329745,-13.572251750231,124.195000415073)) ;
#12757=CARTESIAN_POINT('Ctrl Pts',(-20.4283492010573,-13.5755496368404,
124.135680472464)) ;
#12758=CARTESIAN_POINT('Ctrl Pts',(-20.4674660268464,-13.5786112290647,
124.080610818304)) ;
#12759=CARTESIAN_POINT('Ctrl Pts',(-20.5020545595273,-13.5816906805821,
124.022461487235)) ;
#12760=CARTESIAN_POINT('Ctrl Pts',(-20.5317761765119,-13.5848255321454,
123.961800642308)) ;
#12761=CARTESIAN_POINT('Ctrl Pts',(-20.5337286702634,-13.5850314690597,
123.957815666633)) ;
#12762=CARTESIAN_POINT('Ctrl Pts',(-20.5356609628748,-13.5852375713387,
123.953818171768)) ;
#12763=CARTESIAN_POINT('Ctrl Pts',(-20.5375707370962,-13.5854435438225,
123.949812965442)) ;
#12764=CARTESIAN_POINT('Ctrl Pts',(-20.568906233374,-13.5888231318001,123.884095706035)) ;
#12765=CARTESIAN_POINT('Ctrl Pts',(-20.5944392442653,-13.5921401332644,
123.815769648868)) ;
#12766=CARTESIAN_POINT('Ctrl Pts',(-20.6138809472479,-13.5954485434704,
123.745607495236)) ;
#12767=CARTESIAN_POINT('Ctrl Pts',(-20.633237100436,-13.5987423955991,123.675754077821)) ;
#12768=CARTESIAN_POINT('Ctrl Pts',(-20.6464801951646,-13.6020801028086,
123.604351035323)) ;
#12769=CARTESIAN_POINT('Ctrl Pts',(-20.653461245587,-13.6054094130713,123.532204184997)) ;
#12770=CARTESIAN_POINT('Ctrl Pts',(-20.6604401449323,-13.6087376974708,
123.460079565342)) ;
#12771=CARTESIAN_POINT('Ctrl Pts',(-20.6611343238489,-13.6120319361397,
123.387484385675)) ;
#12772=CARTESIAN_POINT('Ctrl Pts',(-20.655535986198,-13.6153669540374,123.315239706836)) ;
#12773=CARTESIAN_POINT('Ctrl Pts',(-20.6499148235769,-13.6187155691292,
123.242700479376)) ;
#12774=CARTESIAN_POINT('Ctrl Pts',(-20.6379719182571,-13.6220539984323,
123.170790628025)) ;
#12775=CARTESIAN_POINT('Ctrl Pts',(-20.6198380029924,-13.6253653991054,
123.100317137446)) ;
#12776=CARTESIAN_POINT('Ctrl Pts',(-20.6117442443413,-13.6268433853789,
123.068862516879)) ;
#12777=CARTESIAN_POINT('Ctrl Pts',(-20.6024245338594,-13.6283234680977,
123.037724446227)) ;
#12778=CARTESIAN_POINT('Ctrl Pts',(-20.5919018244078,-13.6298117104086,
123.006984455876)) ;
#12779=CARTESIAN_POINT('Ctrl Pts',(-20.5919018244078,-13.6298117104086,
123.006984455876)) ;
#12780=CARTESIAN_POINT('Ctrl Pts',(-20.5790310378141,-13.6316320449137,
122.969385027943)) ;
#12781=CARTESIAN_POINT('Ctrl Pts',(-20.5643742233044,-13.6334632796243,
122.932421164832)) ;
#12782=CARTESIAN_POINT('Ctrl Pts',(-20.5479870005735,-13.6352947183417,
122.896228597839)) ;
#12783=CARTESIAN_POINT('Ctrl Pts',(-20.5180638601431,-13.6386389334554,
122.830140812104)) ;
#12784=CARTESIAN_POINT('Ctrl Pts',(-20.4824491042485,-13.6419425094988,
122.766792714165)) ;
#12785=CARTESIAN_POINT('Ctrl Pts',(-20.4415430467989,-13.6452625229901,
122.706890985514)) ;
#12786=CARTESIAN_POINT('Ctrl Pts',(-20.4006930189139,-13.6485779890153,
122.647071305047)) ;
#12787=CARTESIAN_POINT('Ctrl Pts',(-20.3547207077085,-13.6519098165663,
122.590915838348)) ;
#12788=CARTESIAN_POINT('Ctrl Pts',(-20.3041444000383,-13.6552161178838,
122.539057922863)) ;
#12789=CARTESIAN_POINT('Ctrl Pts',(-20.2536686246012,-13.6585158471545,
122.487303087107)) ;
#12790=CARTESIAN_POINT('Ctrl Pts',(-20.1987988823212,-13.6618078080636,
122.440025296584)) ;
#12791=CARTESIAN_POINT('Ctrl Pts',(-20.1401511310019,-13.6651498353065,
122.397755176552)) ;
#12792=CARTESIAN_POINT('Ctrl Pts',(-20.0830181192173,-13.668405545501,122.356576798667)) ;
#12793=CARTESIAN_POINT('Ctrl Pts',(-20.0225069177832,-13.6716387672799,
122.320299907186)) ;
#12794=CARTESIAN_POINT('Ctrl Pts',(-19.9592592694379,-13.6748309727741,
122.289310797272)) ;
#12795=CARTESIAN_POINT('Ctrl Pts',(-19.9571731087758,-13.6749362644917,
122.288288652358)) ;
#12796=CARTESIAN_POINT('Ctrl Pts',(-19.9550828947529,-13.6750416109726,
122.287271738945)) ;
#12797=CARTESIAN_POINT('Ctrl Pts',(-19.9529911303783,-13.6751468959294,
122.286261274116)) ;
#12798=CARTESIAN_POINT('Ctrl Pts',(-19.8877979152717,-13.6784282716526,
122.254768505734)) ;
#12799=CARTESIAN_POINT('Ctrl Pts',(-19.8199962513967,-13.6817361681552,
122.229001185791)) ;
#12800=CARTESIAN_POINT('Ctrl Pts',(-19.7503470286679,-13.6850947732519,
122.209247118611)) ;
#12801=CARTESIAN_POINT('Ctrl Pts',(-19.6803520183055,-13.6884700528219,
122.189394978374)) ;
#12802=CARTESIAN_POINT('Ctrl Pts',(-19.6087586922491,-13.691794810947,122.175691770181)) ;
#12803=CARTESIAN_POINT('Ctrl Pts',(-19.5363764920953,-13.6950917400237,
122.168293354218)) ;
#12804=CARTESIAN_POINT('Ctrl Pts',(-19.4647038593956,-13.6983563490884,
122.160967465412)) ;
#12805=CARTESIAN_POINT('Ctrl Pts',(-19.3925347024683,-13.7016707095442,
122.159851859288)) ;
#12806=CARTESIAN_POINT('Ctrl Pts',(-19.320672411073,-13.7049909610782,122.164958291828)) ;
#12807=CARTESIAN_POINT('Ctrl Pts',(-19.2484184491182,-13.7083293089566,
122.170092555923)) ;
#12808=CARTESIAN_POINT('Ctrl Pts',(-19.1767469037732,-13.7116146814287,
122.181497090581)) ;
#12809=CARTESIAN_POINT('Ctrl Pts',(-19.1064574395215,-13.7149444349367,
122.199047612758)) ;
#12810=CARTESIAN_POINT('Ctrl Pts',(-19.0720477046613,-13.7165744933897,
122.207639352946)) ;
#12811=CARTESIAN_POINT('Ctrl Pts',(-19.0380083961707,-13.7182141781467,
122.217694693546)) ;
#12812=CARTESIAN_POINT('Ctrl Pts',(-19.0044432721584,-13.7198430895508,
122.229184453976)) ;
#12813=CARTESIAN_POINT('Ctrl Pts',(-18.9692063464723,-13.7215531332878,
122.241246492963)) ;
#12814=CARTESIAN_POINT('Ctrl Pts',(-18.9345261004571,-13.7232493727939,
122.254877696253)) ;
#12815=CARTESIAN_POINT('Ctrl Pts',(-18.9005158290295,-13.7249402776874,
122.270032023694)) ;
#12816=CARTESIAN_POINT('Ctrl Pts',(-18.8344701658612,-13.7282239014385,
122.299460709902)) ;
#12817=CARTESIAN_POINT('Ctrl Pts',(-18.7711147119131,-13.7315221600936,
122.334558126477)) ;
#12818=CARTESIAN_POINT('Ctrl Pts',(-18.7111486940344,-13.734874028962,122.374932733833)) ;
#12819=CARTESIAN_POINT('Ctrl Pts',(-18.650836934586,-13.7382452234492,122.415540126034)) ;
#12820=CARTESIAN_POINT('Ctrl Pts',(-18.5941839619728,-13.741568557929,122.461331315927)) ;
#12821=CARTESIAN_POINT('Ctrl Pts',(-18.5418304272057,-13.7448644969519,
122.511789528844)) ;
#12822=CARTESIAN_POINT('Ctrl Pts',(-18.4897993844536,-13.748140133353,122.561936924721)) ;
#12823=CARTESIAN_POINT('Ctrl Pts',(-18.4422167280386,-13.7514622574866,
122.616499809659)) ;
#12824=CARTESIAN_POINT('Ctrl Pts',(-18.3996148755258,-13.7547935670707,
122.674866597309)) ;
#12825=CARTESIAN_POINT('Ctrl Pts',(-18.3567697587302,-13.758143899035,122.733566669873)) ;
#12826=CARTESIAN_POINT('Ctrl Pts',(-18.3191252112809,-13.7614413358972,
122.795891495704)) ;
#12827=CARTESIAN_POINT('Ctrl Pts',(-18.287109025779,-13.7647793411791,122.8611332158)) ;
#12828=CARTESIAN_POINT('Ctrl Pts',(-18.2869957400592,-13.7647911523404,
122.861364066387)) ;
#12829=CARTESIAN_POINT('Ctrl Pts',(-18.2868824555566,-13.7648029714618,
122.861595094763)) ;
#12830=CARTESIAN_POINT('Ctrl Pts',(-18.2867693133322,-13.7648147838155,
122.861826013248)) ;
#12831=CARTESIAN_POINT('Ctrl Pts',(-18.2548919329702,-13.7681428684017,
122.92688639572)) ;
#12832=CARTESIAN_POINT('Ctrl Pts',(-18.2287311833278,-13.7714802152786,
122.994594787555)) ;
#12833=CARTESIAN_POINT('Ctrl Pts',(-18.2085821491953,-13.7747699914811,
123.064189114839)) ;
#12834=CARTESIAN_POINT('Ctrl Pts',(-18.1884929782487,-13.7780499936923,
123.133576675976)) ;
#12835=CARTESIAN_POINT('Ctrl Pts',(-18.1744570679719,-13.7813420328621,
123.204572243812)) ;
#12836=CARTESIAN_POINT('Ctrl Pts',(-18.1666307377936,-13.7846958763151,
123.276381330981)) ;
#12837=CARTESIAN_POINT('Ctrl Pts',(-18.1587479612325,-13.7880739089254,
123.3487083318)) ;
#12838=CARTESIAN_POINT('Ctrl Pts',(-18.1571945924796,-13.7914005465369,
123.421583595596)) ;
#12839=CARTESIAN_POINT('Ctrl Pts',(-18.1619891169103,-13.7946933269657,
123.494184391611)) ;
#12840=CARTESIAN_POINT('Ctrl Pts',(-18.1667385232767,-13.7979551212391,
123.56610199007)) ;
#12841=CARTESIAN_POINT('Ctrl Pts',(-18.177698121041,-13.801270000348,123.637471180153)) ;
#12842=CARTESIAN_POINT('Ctrl Pts',(-18.1947494013785,-13.8045976378414,
123.707507255171)) ;
#12843=CARTESIAN_POINT('Ctrl Pts',(-18.2037176269291,-13.8063478292054,
123.744343158692)) ;
#12844=CARTESIAN_POINT('Ctrl Pts',(-18.2143600602923,-13.8080877109819,
123.780763074565)) ;
#12845=CARTESIAN_POINT('Ctrl Pts',(-18.2266423654683,-13.8098218143905,
123.816643453356)) ;
#12846=CARTESIAN_POINT('',(-20.5919017786445,-13.5697518725948,123.006984322209)) ;
#12847=CARTESIAN_POINT('Ctrl Pts',(-18.2266423654683,-13.7497401139871,
123.816643453356)) ;
#12848=CARTESIAN_POINT('Ctrl Pts',(-18.217683602435,-13.7484711482467,123.790472160059)) ;
#12849=CARTESIAN_POINT('Ctrl Pts',(-18.209596088243,-13.747199545287,123.764010798093)) ;
#12850=CARTESIAN_POINT('Ctrl Pts',(-18.2023931563355,-13.7459265169278,
123.73730305647)) ;
#12851=CARTESIAN_POINT('Ctrl Pts',(-18.1834359019463,-13.7425760587033,
123.66701147818)) ;
#12852=CARTESIAN_POINT('Ctrl Pts',(-18.1706557494658,-13.7392571781483,
123.595198077764)) ;
#12853=CARTESIAN_POINT('Ctrl Pts',(-18.1641985295719,-13.7359220780221,
123.522681249598)) ;
#12854=CARTESIAN_POINT('Ctrl Pts',(-18.1577686536347,-13.7326011008212,
123.450471503589)) ;
#12855=CARTESIAN_POINT('Ctrl Pts',(-18.1576327530631,-13.7292616282286,
123.377839031082)) ;
#12856=CARTESIAN_POINT('Ctrl Pts',(-18.1637925927213,-13.7259597703705,
123.305604864303)) ;
#12857=CARTESIAN_POINT('Ctrl Pts',(-18.1699125413955,-13.7226792952701,
123.233838484373)) ;
#12858=CARTESIAN_POINT('Ctrl Pts',(-18.1822235644136,-13.7194010053182,
123.162738000472)) ;
#12859=CARTESIAN_POINT('Ctrl Pts',(-18.2005879905351,-13.7160618772626,
123.093094434721)) ;
#12860=CARTESIAN_POINT('Ctrl Pts',(-18.219138810058,-13.7126888580616,123.022744007727)) ;
#12861=CARTESIAN_POINT('Ctrl Pts',(-18.2437955606779,-13.7093580573816,
122.954148592409)) ;
#12862=CARTESIAN_POINT('Ctrl Pts',(-18.274280345546,-13.7060635466254,122.888084084085)) ;
#12863=CARTESIAN_POINT('Ctrl Pts',(-18.2783413762808,-13.7056246683622,
122.879283300352)) ;
#12864=CARTESIAN_POINT('Ctrl Pts',(-18.2825046241964,-13.7051855312,122.870530065893)) ;
#12865=CARTESIAN_POINT('Ctrl Pts',(-18.2867692424076,-13.7047457607437,
122.861826158003)) ;
#12866=CARTESIAN_POINT('Ctrl Pts',(-18.3143524068913,-13.7019013652481,
122.805530069791)) ;
#12867=CARTESIAN_POINT('Ctrl Pts',(-18.3461303693126,-13.6990184536646,
122.751390936298)) ;
#12868=CARTESIAN_POINT('Ctrl Pts',(-18.3818346967705,-13.6961143986274,
122.699864857713)) ;
#12869=CARTESIAN_POINT('Ctrl Pts',(-18.4232731976758,-13.6927439475965,
122.640063606545)) ;
#12870=CARTESIAN_POINT('Ctrl Pts',(-18.4698531456278,-13.689426373171,122.583994631975)) ;
#12871=CARTESIAN_POINT('Ctrl Pts',(-18.5210469159295,-13.6861158596704,
122.532294167282)) ;
#12872=CARTESIAN_POINT('Ctrl Pts',(-18.571913546219,-13.6828265011154,122.480924080496)) ;
#12873=CARTESIAN_POINT('Ctrl Pts',(-18.6271400827939,-13.6794977337672,
122.434064187781)) ;
#12874=CARTESIAN_POINT('Ctrl Pts',(-18.6861055940097,-13.6761809275718,
122.392240922395)) ;
#12875=CARTESIAN_POINT('Ctrl Pts',(-18.7451892734769,-13.67285747442,122.350333842215)) ;
#12876=CARTESIAN_POINT('Ctrl Pts',(-18.8078034512258,-13.6695704256265,
122.313642136408)) ;
#12877=CARTESIAN_POINT('Ctrl Pts',(-18.8732410608961,-13.6662262115031,
122.28257985618)) ;
#12878=CARTESIAN_POINT('Ctrl Pts',(-18.9159303161709,-13.6640445607501,
122.26231588846)) ;
#12879=CARTESIAN_POINT('Ctrl Pts',(-18.9597342782377,-13.6618533221964,
122.24448890521)) ;
#12880=CARTESIAN_POINT('Ctrl Pts',(-19.0044431491614,-13.6596962188292,
122.229184496079)) ;
#12881=CARTESIAN_POINT('Ctrl Pts',(-19.0285400460438,-13.6585335972659,
122.220935825043)) ;
#12882=CARTESIAN_POINT('Ctrl Pts',(-19.0528835163119,-13.657379728912,122.213425529107)) ;
#12883=CARTESIAN_POINT('Ctrl Pts',(-19.0774397388877,-13.6562275396947,
122.206664087982)) ;
#12884=CARTESIAN_POINT('Ctrl Pts',(-19.1469020155668,-13.6529683378388,
122.187537974723)) ;
#12885=CARTESIAN_POINT('Ctrl Pts',(-19.2178827654257,-13.6496744544506,
122.174454152537)) ;
#12886=CARTESIAN_POINT('Ctrl Pts',(-19.2895950549861,-13.6463266758792,
122.167556606921)) ;
#12887=CARTESIAN_POINT('Ctrl Pts',(-19.3620164691775,-13.6429457929088,
122.160590855151)) ;
#12888=CARTESIAN_POINT('Ctrl Pts',(-19.4349066876325,-13.6396283033778,
122.159961021446)) ;
#12889=CARTESIAN_POINT('Ctrl Pts',(-19.5074413065022,-13.636328050303,122.165675195499)) ;
#12890=CARTESIAN_POINT('Ctrl Pts',(-19.5797278270375,-13.6330390854559,
122.171369824718)) ;
#12891=CARTESIAN_POINT('Ctrl Pts',(-19.6513798255484,-13.629714992131,122.183343256875)) ;
#12892=CARTESIAN_POINT('Ctrl Pts',(-19.7215877702431,-13.6263635044537,
122.201459456996)) ;
#12893=CARTESIAN_POINT('Ctrl Pts',(-19.7917261706841,-13.6230153365818,
122.219557712172)) ;
#12894=CARTESIAN_POINT('Ctrl Pts',(-19.8601587554996,-13.61969725647,122.243718185573)) ;
#12895=CARTESIAN_POINT('Ctrl Pts',(-19.9261151842666,-13.6164089669526,
122.273669662735)) ;
#12896=CARTESIAN_POINT('Ctrl Pts',(-19.9372394666596,-13.615854360497,122.278721311168)) ;
#12897=CARTESIAN_POINT('Ctrl Pts',(-19.9482890748614,-13.6152998312536,
122.283935775826)) ;
#12898=CARTESIAN_POINT('Ctrl Pts',(-19.9592604445148,-13.6147444918876,
122.289311373019)) ;
#12899=CARTESIAN_POINT('Ctrl Pts',(-20.0129695493756,-13.6120258905479,
122.315627003833)) ;
#12900=CARTESIAN_POINT('Ctrl Pts',(-20.0647188293458,-13.6092767926613,
122.34576245919)) ;
#12901=CARTESIAN_POINT('Ctrl Pts',(-20.1141113952294,-13.6065083972215,
122.379486046878)) ;
#12902=CARTESIAN_POINT('Ctrl Pts',(-20.1741978731161,-13.6031406205451,
122.420511079079)) ;
#12903=CARTESIAN_POINT('Ctrl Pts',(-20.2305877405618,-13.599821667702,122.466703443609)) ;
#12904=CARTESIAN_POINT('Ctrl Pts',(-20.2826406945403,-13.596510155924,122.517539500753)) ;
#12905=CARTESIAN_POINT('Ctrl Pts',(-20.3346590645714,-13.5932008443122,
122.568341782456)) ;
#12906=CARTESIAN_POINT('Ctrl Pts',(-20.3821449392596,-13.5898716234696,
122.623585216385)) ;
#12907=CARTESIAN_POINT('Ctrl Pts',(-20.4245584780755,-13.5865186222975,
122.682640966999)) ;
#12908=CARTESIAN_POINT('Ctrl Pts',(-20.4669279463567,-13.5831691051203,
122.741635354696)) ;
#12909=CARTESIAN_POINT('Ctrl Pts',(-20.5040750609174,-13.5798384928574,
122.804210376071)) ;
#12910=CARTESIAN_POINT('Ctrl Pts',(-20.535578672954,-13.5765375789663,122.869657737861)) ;
#12911=CARTESIAN_POINT('Ctrl Pts',(-20.5570569928827,-13.5742871041785,
122.914277998338)) ;
#12912=CARTESIAN_POINT('Ctrl Pts',(-20.5758642994148,-13.5720326291569,
122.960134052569)) ;
#12913=CARTESIAN_POINT('Ctrl Pts',(-20.5919017786445,-13.5697518725948,
123.006984322209)) ;
#12914=CARTESIAN_POINT('Ctrl Pts',(-20.5919017786508,-13.5697518725948,
123.006984322206)) ;
#12915=CARTESIAN_POINT('Ctrl Pts',(-20.5992029839164,-13.5687135376991,
123.028313324747)) ;
#12916=CARTESIAN_POINT('Ctrl Pts',(-20.6059253602587,-13.5676717649293,
123.049835019345)) ;
#12917=CARTESIAN_POINT('Ctrl Pts',(-20.6120597630125,-13.5666314897859,
123.071517195218)) ;
#12918=CARTESIAN_POINT('Ctrl Pts',(-20.6318565136898,-13.563274346723,123.141489227888)) ;
#12919=CARTESIAN_POINT('Ctrl Pts',(-20.6455076403348,-13.5599739327008,
123.213046366258)) ;
#12920=CARTESIAN_POINT('Ctrl Pts',(-20.6528618564878,-13.5566399755896,
123.285383137137)) ;
#12921=CARTESIAN_POINT('Ctrl Pts',(-20.660220857568,-13.5533038492817,123.357766973017)) ;
#12922=CARTESIAN_POINT('Ctrl Pts',(-20.6612462363588,-13.5499476510624,
123.430654522817)) ;
#12923=CARTESIAN_POINT('Ctrl Pts',(-20.6559258644321,-13.5466424204047,
123.50321858242)) ;
#12924=CARTESIAN_POINT('Ctrl Pts',(-20.6506501065631,-13.5433649058076,
123.575174155024)) ;
#12925=CARTESIAN_POINT('Ctrl Pts',(-20.639154812979,-13.5400766780383,123.64653531386)) ;
#12926=CARTESIAN_POINT('Ctrl Pts',(-20.6215689686222,-13.5367288178819,
123.716505410141)) ;
#12927=CARTESIAN_POINT('Ctrl Pts',(-20.6038344301335,-13.5333526504602,
123.787067126734)) ;
#12928=CARTESIAN_POINT('Ctrl Pts',(-20.5799743244755,-13.530026994319,123.855944559216)) ;
#12929=CARTESIAN_POINT('Ctrl Pts',(-20.5502534132391,-13.5267312778305,
123.922365003774)) ;
#12930=CARTESIAN_POINT('Ctrl Pts',(-20.5443254392809,-13.5260739318507,
123.935612870318)) ;
#12931=CARTESIAN_POINT('Ctrl Pts',(-20.5381641641557,-13.5254154865591,
123.948762911758)) ;
#12932=CARTESIAN_POINT('Ctrl Pts',(-20.5317771332164,-13.5247555390931,
123.961798689701)) ;
#12933=CARTESIAN_POINT('Ctrl Pts',(-20.5063461686967,-13.5221278548448,
124.013702682259)) ;
#12934=CARTESIAN_POINT('Ctrl Pts',(-20.4773484677845,-13.519468252138,124.06377475595)) ;
#12935=CARTESIAN_POINT('Ctrl Pts',(-20.4449958583186,-13.5167925737403,
124.111654761333)) ;
#12936=CARTESIAN_POINT('Ctrl Pts',(-20.4044204134483,-13.5134368369663,
124.171704091229)) ;
#12937=CARTESIAN_POINT('Ctrl Pts',(-20.3587041928444,-13.5101223925437,
124.228105177321)) ;
#12938=CARTESIAN_POINT('Ctrl Pts',(-20.3083577719846,-13.506835085905,124.280229704392)) ;
#12939=CARTESIAN_POINT('Ctrl Pts',(-20.2582587553424,-13.5035639332156,
124.332098089565)) ;
#12940=CARTESIAN_POINT('Ctrl Pts',(-20.2037672884561,-13.5002613201806,
124.379531995468)) ;
#12941=CARTESIAN_POINT('Ctrl Pts',(-20.1454918425646,-13.4969268449828,
124.422002809834)) ;
#12942=CARTESIAN_POINT('Ctrl Pts',(-20.0866940195142,-13.4935624797746,
124.464854329711)) ;
#12943=CARTESIAN_POINT('Ctrl Pts',(-20.0242676357262,-13.4902466827157,
124.502491060534)) ;
#12944=CARTESIAN_POINT('Ctrl Pts',(-19.958913061696,-13.4869295538181,124.534487499205)) ;
#12945=CARTESIAN_POINT('Ctrl Pts',(-19.9119493347376,-13.4845458685422,
124.557480105792)) ;
#12946=CARTESIAN_POINT('Ctrl Pts',(-19.8635811255283,-13.482150708584,124.577506858947)) ;
#12947=CARTESIAN_POINT('Ctrl Pts',(-19.8140974496505,-13.4797495433924,
124.594445562851)) ;
#12948=CARTESIAN_POINT('Ctrl Pts',(-19.7947726882597,-13.4788118211322,
124.601060601152)) ;
#12949=CARTESIAN_POINT('Ctrl Pts',(-19.7752847959478,-13.4778732271369,
124.607202084085)) ;
#12950=CARTESIAN_POINT('Ctrl Pts',(-19.7556641998379,-13.4769335316329,
124.612860830042)) ;
#12951=CARTESIAN_POINT('Ctrl Pts',(-19.6860443921091,-13.4735992078467,
124.632939771746)) ;
#12952=CARTESIAN_POINT('Ctrl Pts',(-19.6148188662507,-13.4702746386561,
124.646925572577)) ;
#12953=CARTESIAN_POINT('Ctrl Pts',(-19.5427825802482,-13.4669784003535,
124.65466391017)) ;
#12954=CARTESIAN_POINT('Ctrl Pts',(-19.4711211737222,-13.463699315796,124.662361977171)) ;
#12955=CARTESIAN_POINT('Ctrl Pts',(-19.398930139708,-13.4604087499291,124.66384764412)) ;
#12956=CARTESIAN_POINT('Ctrl Pts',(-19.3270149562398,-13.4570754198169,
124.659104926141)) ;
#12957=CARTESIAN_POINT('Ctrl Pts',(-19.2544168698574,-13.4537104365719,
124.654317171554)) ;
#12958=CARTESIAN_POINT('Ctrl Pts',(-19.1823760896568,-13.4503926760514,
124.643200486903)) ;
#12959=CARTESIAN_POINT('Ctrl Pts',(-19.11171025158,-13.4470784684345,124.625880619094)) ;
#12960=CARTESIAN_POINT('Ctrl Pts',(-19.0412853620556,-13.4437755612359,
124.608619806653)) ;
#12961=CARTESIAN_POINT('Ctrl Pts',(-18.972496652837,-13.4404418428525,124.585264697601)) ;
#12962=CARTESIAN_POINT('Ctrl Pts',(-18.9061147649918,-13.4371150407692,
124.556075070902)) ;
#12963=CARTESIAN_POINT('Ctrl Pts',(-18.8903614558579,-13.4363255461744,
124.549147982387)) ;
#12964=CARTESIAN_POINT('Ctrl Pts',(-18.8747453259081,-13.4355365787144,
124.541892804038)) ;
#12965=CARTESIAN_POINT('Ctrl Pts',(-18.8592878554704,-13.4347481692111,
124.53431923573)) ;
#12966=CARTESIAN_POINT('Ctrl Pts',(-18.809762050661,-13.4322221016165,124.510053488806)) ;
#12967=CARTESIAN_POINT('Ctrl Pts',(-18.7619006318004,-13.4297044741409,
124.482538510267)) ;
#12968=CARTESIAN_POINT('Ctrl Pts',(-18.7160195400566,-13.4271691247233,
124.451958923685)) ;
#12969=CARTESIAN_POINT('Ctrl Pts',(-18.6556158482899,-13.4238312689983,
124.411700075169)) ;
#12970=CARTESIAN_POINT('Ctrl Pts',(-18.5988404405405,-13.4204997684909,
124.366261186538)) ;
#12971=CARTESIAN_POINT('Ctrl Pts',(-18.5463281077966,-13.4171952325858,
124.316152484613)) ;
#12972=CARTESIAN_POINT('Ctrl Pts',(-18.4940118329209,-13.4139030343589,
124.266230866459)) ;
#12973=CARTESIAN_POINT('Ctrl Pts',(-18.4461272458628,-13.410599070874,124.211864739455)) ;
#12974=CARTESIAN_POINT('Ctrl Pts',(-18.4032120923609,-13.4072587644132,
124.153665421393)) ;
#12975=CARTESIAN_POINT('Ctrl Pts',(-18.3600613169715,-13.4039001182927,
124.095146565079)) ;
#12976=CARTESIAN_POINT('Ctrl Pts',(-18.3220981235732,-13.4005793799823,
124.032974773141)) ;
#12977=CARTESIAN_POINT('Ctrl Pts',(-18.2897515266574,-13.3972674064958,
123.967847982035)) ;
#12978=CARTESIAN_POINT('Ctrl Pts',(-18.2654336498414,-13.3947774950077,
123.918886253923)) ;
#12979=CARTESIAN_POINT('Ctrl Pts',(-18.2443509121134,-13.392276521157,123.868375546994)) ;
#12980=CARTESIAN_POINT('Ctrl Pts',(-18.2266423654683,-13.389762567023,123.816643453356)) ;
#12981=CARTESIAN_POINT('Origin',(-19.4092722359532,-13.9601742359176,123.411814366564)) ;
#12982=CARTESIAN_POINT('',(-18.2266423654684,-13.0298305431221,123.816643453356)) ;
#12983=CARTESIAN_POINT('',(-18.2266423654688,-13.0898424649011,123.816643453357)) ;
#12984=CARTESIAN_POINT('',(-18.2266423654683,-13.9601742359176,123.816643453356)) ;
#12985=CARTESIAN_POINT('',(-20.5919015501437,-13.2698313022293,123.006983654703)) ;
#12986=CARTESIAN_POINT('Ctrl Pts',(-18.2266423654692,-13.0898424649011,
123.816643453359)) ;
#12987=CARTESIAN_POINT('Ctrl Pts',(-18.2310349193409,-13.0904621593805,
123.829475449838)) ;
#12988=CARTESIAN_POINT('Ctrl Pts',(-18.2356360431616,-13.0910823834473,
123.842235141906)) ;
#12989=CARTESIAN_POINT('Ctrl Pts',(-18.2440506239372,-13.0921691632372,
123.864431331654)) ;
#12990=CARTESIAN_POINT('Ctrl Pts',(-18.2477733535108,-13.0926353551193,
123.873900795199)) ;
#12991=CARTESIAN_POINT('Ctrl Pts',(-18.2516463086842,-13.0931062465292,
123.883409766478)) ;
#12992=CARTESIAN_POINT('Ctrl Pts',(-18.2516813587955,-13.0931105069494,
123.883495794889)) ;
#12993=CARTESIAN_POINT('Ctrl Pts',(-18.2517618579049,-13.0931202892023,
123.883693312144)) ;
#12994=CARTESIAN_POINT('Ctrl Pts',(-18.2518073133862,-13.0931258110546,
123.883804798245)) ;
#12995=CARTESIAN_POINT('Ctrl Pts',(-18.2518971976611,-13.0931367262883,
123.884025161276)) ;
#12996=CARTESIAN_POINT('Ctrl Pts',(-18.2519416257492,-13.0931421196713,
123.884134038596)) ;
#12997=CARTESIAN_POINT('Ctrl Pts',(-18.2520295016494,-13.0931527838599,
123.88434930409)) ;
#12998=CARTESIAN_POINT('Ctrl Pts',(-18.2520729487653,-13.0931580546624,
123.884455692533)) ;
#12999=CARTESIAN_POINT('Ctrl Pts',(-18.2521589063775,-13.0931684792276,
123.884666093028)) ;
#13000=CARTESIAN_POINT('Ctrl Pts',(-18.2522014162068,-13.0931736329853,
123.884770105289)) ;
#13001=CARTESIAN_POINT('Ctrl Pts',(-18.2522855402971,-13.0931838286635,
123.884975859327)) ;
#13002=CARTESIAN_POINT('Ctrl Pts',(-18.2523271539625,-13.0931888705825,
123.885077601367)) ;
#13003=CARTESIAN_POINT('Ctrl Pts',(-18.2524095244819,-13.0931988474895,
123.885278914824)) ;
#13004=CARTESIAN_POINT('Ctrl Pts',(-18.2524502807722,-13.0932037824754,
123.88537848647)) ;
#13005=CARTESIAN_POINT('Ctrl Pts',(-18.2525309731381,-13.0932135501443,
123.885575553321)) ;
#13006=CARTESIAN_POINT('Ctrl Pts',(-18.2525709086823,-13.0932183828248,
123.885673048732)) ;
#13007=CARTESIAN_POINT('Ctrl Pts',(-18.2526499940244,-13.0932279502384,
123.885866051727)) ;
#13008=CARTESIAN_POINT('Ctrl Pts',(-18.2526891433718,-13.0932326849749,
123.885961559622)) ;
#13009=CARTESIAN_POINT('Ctrl Pts',(-18.2527666891164,-13.0932420606393,
123.886150671782)) ;
#13010=CARTESIAN_POINT('Ctrl Pts',(-18.2528050850144,-13.0932467015614,
123.886244276152)) ;
#13011=CARTESIAN_POINT('Ctrl Pts',(-18.2528811547807,-13.0932558934961,
123.886429660569)) ;
#13012=CARTESIAN_POINT('Ctrl Pts',(-18.2529188281946,-13.0932604445051,
123.886521440752)) ;
#13013=CARTESIAN_POINT('Ctrl Pts',(-18.2529934823241,-13.0932694603092,
123.886703251942)) ;
#13014=CARTESIAN_POINT('Ctrl Pts',(-18.2530304626129,-13.0932739251008,
123.886793283077)) ;
#13015=CARTESIAN_POINT('Ctrl Pts',(-18.2531037582241,-13.0932827719612,
123.886971667157)) ;
#13016=CARTESIAN_POINT('Ctrl Pts',(-18.2531400731929,-13.0932871540326,
123.887060020339)) ;
#13017=CARTESIAN_POINT('Ctrl Pts',(-18.2532120645626,-13.0932958387727,
123.887235116003)) ;
#13018=CARTESIAN_POINT('Ctrl Pts',(-18.2532477406168,-13.0933001414421,
123.887321858677)) ;
#13019=CARTESIAN_POINT('Ctrl Pts',(-18.2533184792844,-13.0933086705353,
123.887493797491)) ;
#13020=CARTESIAN_POINT('Ctrl Pts',(-18.2533535415375,-13.0933128969558,
123.887578993732)) ;
#13021=CARTESIAN_POINT('Ctrl Pts',(-18.2534230763846,-13.0933212765373,
123.887747900365)) ;
#13022=CARTESIAN_POINT('Ctrl Pts',(-18.253457548674,-13.0933254296994,123.887831610938)) ;
#13023=CARTESIAN_POINT('Ctrl Pts',(-18.2535259262764,-13.0933336656095,
123.887997604052)) ;
#13024=CARTESIAN_POINT('Ctrl Pts',(-18.2535598312941,-13.0933377483577,
123.888079886745)) ;
#13025=CARTESIAN_POINT('Ctrl Pts',(-18.2536270959504,-13.093345846147,123.888243079094)) ;
#13026=CARTESIAN_POINT('Ctrl Pts',(-18.2536604552935,-13.0933498611864,
123.888323988855)) ;
#13027=CARTESIAN_POINT('Ctrl Pts',(-18.2537266492693,-13.0933578261462,
123.88848448791)) ;
#13028=CARTESIAN_POINT('Ctrl Pts',(-18.2537594835681,-13.0933617760584,
123.888564077171)) ;
#13029=CARTESIAN_POINT('Ctrl Pts',(-18.2538246470169,-13.0933696132122,
123.888721984952)) ;
#13030=CARTESIAN_POINT('Ctrl Pts',(-18.253856975902,-13.0933735004522,123.888800303564)) ;
#13031=CARTESIAN_POINT('Ctrl Pts',(-18.2539211471992,-13.0933812145971,
123.888955717474)) ;
#13032=CARTESIAN_POINT('Ctrl Pts',(-18.2539529893937,-13.0933850415045,
123.889032812941)) ;
#13033=CARTESIAN_POINT('Ctrl Pts',(-18.2540162052135,-13.0933926372212,
123.889185825978)) ;
#13034=CARTESIAN_POINT('Ctrl Pts',(-18.254047578617,-13.093396406031,123.889261743671)) ;
#13035=CARTESIAN_POINT('Ctrl Pts',(-18.2541098739552,-13.0934038876874,
123.8894124445)) ;
#13036=CARTESIAN_POINT('Ctrl Pts',(-18.2541407956692,-13.0934076005332,
123.889487227727)) ;
#13037=CARTESIAN_POINT('Ctrl Pts',(-18.2542022040059,-13.0934149723049,
123.889635701095)) ;
#13038=CARTESIAN_POINT('Ctrl Pts',(-18.2542326903996,-13.0934186312276,
123.889709391274)) ;
#13039=CARTESIAN_POINT('Ctrl Pts',(-18.2542932437135,-13.0934258971,123.889855718061)) ;
#13040=CARTESIAN_POINT('Ctrl Pts',(-18.2543233104349,-13.0934295040491,
123.889928354751)) ;
#13041=CARTESIAN_POINT('Ctrl Pts',(-18.2543830393939,-13.0934366678415,
123.890072612448)) ;
#13042=CARTESIAN_POINT('Ctrl Pts',(-18.2544127014494,-13.093440224685,123.89014423355)) ;
#13043=CARTESIAN_POINT('Ctrl Pts',(-18.254471635314,-13.0934472900391,123.890286496041)) ;
#13044=CARTESIAN_POINT('Ctrl Pts',(-18.2545009070083,-13.0934507985568,
123.890357137662)) ;
#13045=CARTESIAN_POINT('Ctrl Pts',(-18.2545590740688,-13.09345776899,123.890497476293)) ;
#13046=CARTESIAN_POINT('Ctrl Pts',(-18.2545879692201,-13.0934612308995,
123.890567173269)) ;
#13047=CARTESIAN_POINT('Ctrl Pts',(-18.2546453963592,-13.0934681097528,
123.890705655805)) ;
#13048=CARTESIAN_POINT('Ctrl Pts',(-18.2546739281699,-13.0934715266943,
123.890774441398)) ;
#13049=CARTESIAN_POINT('Ctrl Pts',(-18.2547306413153,-13.0934783171873,
123.890911133128)) ;
#13050=CARTESIAN_POINT('Ctrl Pts',(-18.2547588224857,-13.0934816907372,
123.890979039307)) ;
#13051=CARTESIAN_POINT('Ctrl Pts',(-18.2548148464286,-13.0934883959466,
123.891114002616)) ;
#13052=CARTESIAN_POINT('Ctrl Pts',(-18.2548426890988,-13.093491727611,123.891181059918)) ;
#13053=CARTESIAN_POINT('Ctrl Pts',(-18.2548980478379,-13.0934983505123,
123.891314355129)) ;
#13054=CARTESIAN_POINT('Ctrl Pts',(-18.2549255637414,-13.0935016417458,
123.891380593038)) ;
#13055=CARTESIAN_POINT('Ctrl Pts',(-18.2549802802188,-13.0935081851821,
123.891512277781)) ;
#13056=CARTESIAN_POINT('Ctrl Pts',(-18.2550074806312,-13.0935114373813,
123.891577724607)) ;
#13057=CARTESIAN_POINT('Ctrl Pts',(-18.2550615769081,-13.0935179040846,
123.891707854257)) ;
#13058=CARTESIAN_POINT('Ctrl Pts',(-18.2550884726559,-13.0935211185898,
123.891772537162)) ;
#13059=CARTESIAN_POINT('Ctrl Pts',(-18.2551419700071,-13.0935275111928,
123.89190116507)) ;
#13060=CARTESIAN_POINT('Ctrl Pts',(-18.2551685715089,-13.0935306892928,
123.891965110173)) ;
#13061=CARTESIAN_POINT('Ctrl Pts',(-18.2588710159056,-13.09397293733,123.900863018245)) ;
#13062=CARTESIAN_POINT('Ctrl Pts',(-18.2626481557355,-13.0944123725398,
123.909654470195)) ;
#13063=CARTESIAN_POINT('Ctrl Pts',(-18.2713158519632,-13.0953955404166,
123.929206832528)) ;
#13064=CARTESIAN_POINT('Ctrl Pts',(-18.2762588528341,-13.0959394388412,
123.939943487203)) ;
#13065=CARTESIAN_POINT('Ctrl Pts',(-18.2894723128965,-13.0973517592336,
123.967604727234)) ;
#13066=CARTESIAN_POINT('Ctrl Pts',(-18.2979743756871,-13.0982214800677,
123.984415321352)) ;
#13067=CARTESIAN_POINT('Ctrl Pts',(-18.3107049403825,-13.099467662679,124.008234247871)) ;
#13068=CARTESIAN_POINT('Ctrl Pts',(-18.314627450329,-13.0998445454559,124.015403275877)) ;
#13069=CARTESIAN_POINT('Ctrl Pts',(-18.3236841768078,-13.100698657994,124.031577227637)) ;
#13070=CARTESIAN_POINT('Ctrl Pts',(-18.3288606811316,-13.1011756304112,
124.040557805285)) ;
#13071=CARTESIAN_POINT('Ctrl Pts',(-18.3370102802456,-13.1019095112886,
124.054298431914)) ;
#13072=CARTESIAN_POINT('Ctrl Pts',(-18.3399047205286,-13.1021669917538,
124.059104558902)) ;
#13073=CARTESIAN_POINT('Ctrl Pts',(-18.345200664374,-13.102632451578,124.06776582654)) ;
#13074=CARTESIAN_POINT('Ctrl Pts',(-18.3475910075618,-13.1028405148632,
124.071627670998)) ;
#13075=CARTESIAN_POINT('Ctrl Pts',(-18.3527709573131,-13.1032871125696,
124.07989538022)) ;
#13076=CARTESIAN_POINT('Ctrl Pts',(-18.3555671953804,-13.1035255895825,
124.084296991062)) ;
#13077=CARTESIAN_POINT('Ctrl Pts',(-18.3620621274432,-13.1040736458535,
124.094380813642)) ;
#13078=CARTESIAN_POINT('Ctrl Pts',(-18.3657796736979,-13.1043830718856,
124.1000506915)) ;
#13079=CARTESIAN_POINT('Ctrl Pts',(-18.3764534158412,-13.1052598094217,
124.116044622508)) ;
#13080=CARTESIAN_POINT('Ctrl Pts',(-18.3835179685778,-13.105826351122,124.126295404085)) ;
#13081=CARTESIAN_POINT('Ctrl Pts',(-18.4082567007505,-13.1077673156245,
124.161068350903)) ;
#13082=CARTESIAN_POINT('Ctrl Pts',(-18.426666418208,-13.1091407114837,124.18505393761)) ;
#13083=CARTESIAN_POINT('Ctrl Pts',(-18.450842503503,-13.1108736009269,124.214292990531)) ;
#13084=CARTESIAN_POINT('Ctrl Pts',(-18.4558124867118,-13.1112262783963,
124.220191753671)) ;
#13085=CARTESIAN_POINT('Ctrl Pts',(-18.4645840571794,-13.1118427289033,
124.230409101703)) ;
#13086=CARTESIAN_POINT('Ctrl Pts',(-18.4683614606816,-13.1121063083581,
124.23474814777)) ;
#13087=CARTESIAN_POINT('Ctrl Pts',(-18.4721925190756,-13.1123717686401,
124.239087964348)) ;
#13088=CARTESIAN_POINT('Ctrl Pts',(-18.4722163631817,-13.112373420765,124.239114972558)) ;
#13089=CARTESIAN_POINT('Ctrl Pts',(-18.4722637217479,-13.1123767020309,
124.239168610915)) ;
#13090=CARTESIAN_POINT('Ctrl Pts',(-18.4722872362699,-13.1123783311782,
124.239195241196)) ;
#13091=CARTESIAN_POINT('Ctrl Pts',(-18.472333945564,-13.1123815671806,124.239248135096)) ;
#13092=CARTESIAN_POINT('Ctrl Pts',(-18.4723571399538,-13.112383174011,124.239274398343)) ;
#13093=CARTESIAN_POINT('Ctrl Pts',(-18.4724032156809,-13.1123863658493,
124.239326565945)) ;
#13094=CARTESIAN_POINT('Ctrl Pts',(-18.4724260977675,-13.1123879509109,
124.239352471208)) ;
#13095=CARTESIAN_POINT('Ctrl Pts',(-18.4724715588855,-13.1123910999094,
124.239403934336)) ;
#13096=CARTESIAN_POINT('Ctrl Pts',(-18.4724941374926,-13.1123926638187,
124.239429491778)) ;
#13097=CARTESIAN_POINT('Ctrl Pts',(-18.4725389991235,-13.1123957710355,
124.239480267896)) ;
#13098=CARTESIAN_POINT('Ctrl Pts',(-18.4725612821389,-13.1123973143441,
124.239505486616)) ;
#13099=CARTESIAN_POINT('Ctrl Pts',(-18.4757623563816,-13.1126190098441,
124.243127995727)) ;
#13100=CARTESIAN_POINT('Ctrl Pts',(-18.4789618382074,-13.1128393168581,
124.246706939893)) ;
#13101=CARTESIAN_POINT('Ctrl Pts',(-18.4821934827412,-13.1130605712647,
124.250280219011)) ;
#13102=CARTESIAN_POINT('Ctrl Pts',(-18.4822051132287,-13.1130613675291,
124.250293078482)) ;
#13103=CARTESIAN_POINT('Ctrl Pts',(-18.4867060902776,-13.1133695140606,
124.255269461835)) ;
#13104=CARTESIAN_POINT('Ctrl Pts',(-18.4912352182578,-13.1136771503203,
124.260196842037)) ;
#13105=CARTESIAN_POINT('Ctrl Pts',(-18.5029961979599,-13.1144697875344,
124.272787515896)) ;
#13106=CARTESIAN_POINT('Ctrl Pts',(-18.5102857583995,-13.114955144885,124.280396160682)) ;
#13107=CARTESIAN_POINT('Ctrl Pts',(-18.5391706341844,-13.1168551330375,
124.309792211026)) ;
#13108=CARTESIAN_POINT('Ctrl Pts',(-18.5614688750062,-13.1182719238249,
124.330873928998)) ;
#13109=CARTESIAN_POINT('Ctrl Pts',(-18.5912077229221,-13.1200931114176,
124.356986128304)) ;
#13110=CARTESIAN_POINT('Ctrl Pts',(-18.5979579289442,-13.1205022267812,
124.36278665988)) ;
#13111=CARTESIAN_POINT('Ctrl Pts',(-18.610123962439,-13.1212321034245,124.373017248742)) ;
#13112=CARTESIAN_POINT('Ctrl Pts',(-18.6155161200615,-13.1215530319699,
124.377474851738)) ;
#13113=CARTESIAN_POINT('Ctrl Pts',(-18.6265375378131,-13.1222039352963,
124.386431376386)) ;
#13114=CARTESIAN_POINT('Ctrl Pts',(-18.6321688506471,-13.1225338803142,
124.390927359243)) ;
#13115=CARTESIAN_POINT('Ctrl Pts',(-18.659317713252,-13.1241124725078,124.412220967454)) ;
#13116=CARTESIAN_POINT('Ctrl Pts',(-18.6813427454416,-13.125356647541,124.428359403571)) ;
#13117=CARTESIAN_POINT('Ctrl Pts',(-18.7141400913974,-13.1271703067843,
124.450778179022)) ;
#13118=CARTESIAN_POINT('Ctrl Pts',(-18.7245057083716,-13.1277383650305,
124.457639066536)) ;
#13119=CARTESIAN_POINT('Ctrl Pts',(-18.7452014217814,-13.1288631932976,
124.470897717983)) ;
#13120=CARTESIAN_POINT('Ctrl Pts',(-18.7555259128987,-13.1294197552475,
124.477301736512)) ;
#13121=CARTESIAN_POINT('Ctrl Pts',(-18.8034374491011,-13.1319815211123,
124.506061454043)) ;
#13122=CARTESIAN_POINT('Ctrl Pts',(-18.84208816418,-13.133989051426,124.526585513917)) ;
#13123=CARTESIAN_POINT('Ctrl Pts',(-18.8978516103161,-13.1368079660639,
124.55254439048)) ;
#13124=CARTESIAN_POINT('Ctrl Pts',(-18.9141267182019,-13.1376217468465,
124.559702410876)) ;
#13125=CARTESIAN_POINT('Ctrl Pts',(-18.9565876111898,-13.1397245216049,
124.577306185277)) ;
#13126=CARTESIAN_POINT('Ctrl Pts',(-18.9829839269009,-13.1410125449557,
124.587217626758)) ;
#13127=CARTESIAN_POINT('Ctrl Pts',(-19.0168268126724,-13.1426477650394,
124.598635026514)) ;
#13128=CARTESIAN_POINT('Ctrl Pts',(-19.0239825691278,-13.142992615301,124.600977333331)) ;
#13129=CARTESIAN_POINT('Ctrl Pts',(-19.0395993618215,-13.1437435089535,
124.605933447781)) ;
#13130=CARTESIAN_POINT('Ctrl Pts',(-19.0480678925587,-13.1441496124396,
124.60852228238)) ;
#13131=CARTESIAN_POINT('Ctrl Pts',(-19.0566656126265,-13.144560997464,124.611051032389)) ;
#13132=CARTESIAN_POINT('Ctrl Pts',(-19.0567680294082,-13.144565897787,124.611081140822)) ;
#13133=CARTESIAN_POINT('Ctrl Pts',(-19.0569720854165,-13.1445756609693,
124.611141100707)) ;
#13134=CARTESIAN_POINT('Ctrl Pts',(-19.0570737239492,-13.1445805237974,
124.611170952171)) ;
#13135=CARTESIAN_POINT('Ctrl Pts',(-19.0572762544782,-13.1445902134805,
124.611230407876)) ;
#13136=CARTESIAN_POINT('Ctrl Pts',(-19.0573771462216,-13.1445950403253,
124.61126001225)) ;
#13137=CARTESIAN_POINT('Ctrl Pts',(-19.0575782135723,-13.1446046595024,
124.61131898331)) ;
#13138=CARTESIAN_POINT('Ctrl Pts',(-19.0576783891745,-13.1446094518364,
124.611348350193)) ;
#13139=CARTESIAN_POINT('Ctrl Pts',(-19.057878054072,-13.1446190034247,124.611406855605)) ;
#13140=CARTESIAN_POINT('Ctrl Pts',(-19.0579775434136,-13.144623762683,124.611435994335)) ;
#13141=CARTESIAN_POINT('Ctrl Pts',(-19.0581758649481,-13.1446332495206,
124.611494052542)) ;
#13142=CARTESIAN_POINT('Ctrl Pts',(-19.0582746971249,-13.1446379771008,
124.611522972192)) ;
#13143=CARTESIAN_POINT('Ctrl Pts',(-19.0584717333316,-13.1446474019748,
124.611580601255)) ;
#13144=CARTESIAN_POINT('Ctrl Pts',(-19.0585699370761,-13.1446520992564,
124.611609310755)) ;
#13145=CARTESIAN_POINT('Ctrl Pts',(-19.0587657431968,-13.1446614648194,
124.611666527853)) ;
#13146=CARTESIAN_POINT('Ctrl Pts',(-19.0588633458189,-13.144666133114,124.611695035685)) ;
#13147=CARTESIAN_POINT('Ctrl Pts',(-19.059057978144,-13.1446754420682,124.611751858236)) ;
#13148=CARTESIAN_POINT('Ctrl Pts',(-19.0591550073154,-13.1446800827039,
124.611780172953)) ;
#13149=CARTESIAN_POINT('Ctrl Pts',(-19.0593485180305,-13.1446893375547,
124.611836617113)) ;
#13150=CARTESIAN_POINT('Ctrl Pts',(-19.0594449998465,-13.1446939517842,
124.611864746779)) ;
#13151=CARTESIAN_POINT('Ctrl Pts',(-19.0596374421591,-13.1447031550851,
124.611920828939)) ;
#13152=CARTESIAN_POINT('Ctrl Pts',(-19.0597334025954,-13.144707744155,124.611948781553)) ;
#13153=CARTESIAN_POINT('Ctrl Pts',(-19.0599248278039,-13.1447168983678,
124.612004517491)) ;
#13154=CARTESIAN_POINT('Ctrl Pts',(-19.060020292348,-13.144721463501,124.612032300878)) ;
#13155=CARTESIAN_POINT('Ctrl Pts',(-19.0602107502955,-13.1447305710172,
124.612087705889)) ;
#13156=CARTESIAN_POINT('Ctrl Pts',(-19.0603057437097,-13.1447351134018,
124.612115327638)) ;
#13157=CARTESIAN_POINT('Ctrl Pts',(-19.0604952835146,-13.1447441765778,
124.61217041675)) ;
#13158=CARTESIAN_POINT('Ctrl Pts',(-19.0605898300139,-13.1447486973754,
124.612197884261)) ;
#13159=CARTESIAN_POINT('Ctrl Pts',(-19.0607785001241,-13.144757718535,124.612252672255)) ;
#13160=CARTESIAN_POINT('Ctrl Pts',(-19.0608726236526,-13.1447622188941,
124.612279992824)) ;
#13161=CARTESIAN_POINT('Ctrl Pts',(-19.0610604710687,-13.1447712002914,
124.612334494007)) ;
#13162=CARTESIAN_POINT('Ctrl Pts',(-19.0611541950045,-13.1447756813329,
124.612361674739)) ;
#13163=CARTESIAN_POINT('Ctrl Pts',(-19.0613412658663,-13.1447846251805,
124.612415903118)) ;
#13164=CARTESIAN_POINT('Ctrl Pts',(-19.0614346129884,-13.1447890879967,
124.61244295092)) ;
#13165=CARTESIAN_POINT('Ctrl Pts',(-19.0616209532137,-13.1447979964959,
124.612496920388)) ;
#13166=CARTESIAN_POINT('Ctrl Pts',(-19.0617139461724,-13.1448024421727,
124.612523842105)) ;
#13167=CARTESIAN_POINT('Ctrl Pts',(-19.0701246441923,-13.1452045196795,
124.614957703267)) ;
#13168=CARTESIAN_POINT('Ctrl Pts',(-19.0784671134198,-13.1456025103169,
124.617278156111)) ;
#13169=CARTESIAN_POINT('Ctrl Pts',(-19.0966574785671,-13.1464688668204,
124.622134743199)) ;
#13170=CARTESIAN_POINT('Ctrl Pts',(-19.1065135525949,-13.1469373914084,
124.624637758299)) ;
#13171=CARTESIAN_POINT('Ctrl Pts',(-19.1380898301671,-13.1484361587805,
124.63224786319)) ;
#13172=CARTESIAN_POINT('Ctrl Pts',(-19.1599168044813,-13.1494678486818,
124.636893830941)) ;
#13173=CARTESIAN_POINT('Ctrl Pts',(-19.1903972640696,-13.1508961541302,
124.642533339211)) ;
#13174=CARTESIAN_POINT('Ctrl Pts',(-19.1989543551023,-13.1512958441314,
124.644024508106)) ;
#13175=CARTESIAN_POINT('Ctrl Pts',(-19.2123542771536,-13.1519196102268,
124.646215942286)) ;
#13176=CARTESIAN_POINT('Ctrl Pts',(-19.2171868347842,-13.1521441370725,
124.646977162109)) ;
#13177=CARTESIAN_POINT('Ctrl Pts',(-19.2242912449845,-13.1524735931526,
124.64805353947)) ;
#13178=CARTESIAN_POINT('Ctrl Pts',(-19.2265596862365,-13.1525786955101,
124.648390843715)) ;
#13179=CARTESIAN_POINT('Ctrl Pts',(-19.2330304688316,-13.1528782405571,
124.649334817798)) ;
#13180=CARTESIAN_POINT('Ctrl Pts',(-19.2372349950484,-13.1530725610995,
124.649926322557)) ;
#13181=CARTESIAN_POINT('Ctrl Pts',(-19.2462901288882,-13.1534904117656,
124.651153208099)) ;
#13182=CARTESIAN_POINT('Ctrl Pts',(-19.2511416191126,-13.153713883491,124.651781559505)) ;
#13183=CARTESIAN_POINT('Ctrl Pts',(-19.2634422001535,-13.1542795397735,
124.653301330934)) ;
#13184=CARTESIAN_POINT('Ctrl Pts',(-19.2708958641679,-13.1546214308535,
124.65415420025)) ;
#13185=CARTESIAN_POINT('Ctrl Pts',(-19.2948238210377,-13.1557166956165,
124.656674090119)) ;
#13186=CARTESIAN_POINT('Ctrl Pts',(-19.31132372631,-13.1564683854513,124.658080895838)) ;
#13187=CARTESIAN_POINT('Ctrl Pts',(-19.3329598836559,-13.1574531361168,
124.659493283953)) ;
#13188=CARTESIAN_POINT('Ctrl Pts',(-19.3380750562304,-13.157685892142,124.659795623455)) ;
#13189=CARTESIAN_POINT('Ctrl Pts',(-19.3615756453435,-13.1587553070828,
124.661039703747)) ;
#13190=CARTESIAN_POINT('Ctrl Pts',(-19.3799784943124,-13.1595930499558,
124.661606660638)) ;
#13191=CARTESIAN_POINT('Ctrl Pts',(-19.4044460601184,-13.1607103448831,
124.661819735427)) ;
#13192=CARTESIAN_POINT('Ctrl Pts',(-19.4105053340604,-13.1609873078717,
124.661828443805)) ;
#13193=CARTESIAN_POINT('Ctrl Pts',(-19.4214952121225,-13.1614902158258,
124.661764330555)) ;
#13194=CARTESIAN_POINT('Ctrl Pts',(-19.4264257824356,-13.1617160523299,
124.661706389616)) ;
#13195=CARTESIAN_POINT('Ctrl Pts',(-19.4330679733629,-13.1620205884781,
124.661589024318)) ;
#13196=CARTESIAN_POINT('Ctrl Pts',(-19.4347800097721,-13.1620991101471,
124.661555254008)) ;
#13197=CARTESIAN_POINT('Ctrl Pts',(-19.436523232661,-13.162179090023,124.661517284954)) ;
#13198=CARTESIAN_POINT('Ctrl Pts',(-19.4365544949973,-13.1621805243627,
124.661516602857)) ;
#13199=CARTESIAN_POINT('Ctrl Pts',(-19.4366168350662,-13.1621833845904,
124.66151524035)) ;
#13200=CARTESIAN_POINT('Ctrl Pts',(-19.4366479118928,-13.1621848104368,
124.661514559974)) ;
#13201=CARTESIAN_POINT('Ctrl Pts',(-19.4367098839824,-13.1621876538171,
124.661513200884)) ;
#13202=CARTESIAN_POINT('Ctrl Pts',(-19.4367407796487,-13.1621890713695,
124.661512522175)) ;
#13203=CARTESIAN_POINT('Ctrl Pts',(-19.4368023945972,-13.1621918983992,
124.661511166346)) ;
#13204=CARTESIAN_POINT('Ctrl Pts',(-19.4368331139683,-13.1621933078805,
124.661510489237)) ;
#13205=CARTESIAN_POINT('Ctrl Pts',(-19.4368943808986,-13.1621961189775,
124.661509136545)) ;
#13206=CARTESIAN_POINT('Ctrl Pts',(-19.4369249284788,-13.1621975205941,
124.661508460975)) ;
#13207=CARTESIAN_POINT('Ctrl Pts',(-19.4369858576715,-13.1622003162296,
124.66150711127)) ;
#13208=CARTESIAN_POINT('Ctrl Pts',(-19.4370162387357,-13.1622017102231,
124.66150643716)) ;
#13209=CARTESIAN_POINT('Ctrl Pts',(-19.4370768368356,-13.1622044907013,
124.661505090367)) ;
#13210=CARTESIAN_POINT('Ctrl Pts',(-19.4371070548759,-13.162205877232,124.661504417675)) ;
#13211=CARTESIAN_POINT('Ctrl Pts',(-19.4371673331625,-13.1622086430699,
124.661503073616)) ;
#13212=CARTESIAN_POINT('Ctrl Pts',(-19.437197393112,-13.1622100223635,124.661502402267)) ;
#13213=CARTESIAN_POINT('Ctrl Pts',(-19.4372573587044,-13.1622127738874,
124.66150106085)) ;
#13214=CARTESIAN_POINT('Ctrl Pts',(-19.4372872644325,-13.1622141461214,
124.661500390792)) ;
#13215=CARTESIAN_POINT('Ctrl Pts',(-19.4373469272122,-13.162216883784,124.661499051864)) ;
#13216=CARTESIAN_POINT('Ctrl Pts',(-19.4373766835954,-13.1622182491819,
124.66149838302)) ;
#13217=CARTESIAN_POINT('Ctrl Pts',(-19.4374360496195,-13.1622209732608,
124.661497046509)) ;
#13218=CARTESIAN_POINT('Ctrl Pts',(-19.4374656599422,-13.162222331973,124.661496378836)) ;
#13219=CARTESIAN_POINT('Ctrl Pts',(-19.4431424395461,-13.1624828207325,
124.661368173396)) ;
#13220=CARTESIAN_POINT('Ctrl Pts',(-19.4487886668811,-13.1627422070177,
124.661202360058)) ;
#13221=CARTESIAN_POINT('Ctrl Pts',(-19.4610445885615,-13.1633059021537,
124.660759275812)) ;
#13222=CARTESIAN_POINT('Ctrl Pts',(-19.4676535954587,-13.163610293137,124.660467792989)) ;
#13223=CARTESIAN_POINT('Ctrl Pts',(-19.4860926208311,-13.1644606623515,
124.659507846472)) ;
#13224=CARTESIAN_POINT('Ctrl Pts',(-19.4979158879045,-13.1650072329207,
124.658723622613)) ;
#13225=CARTESIAN_POINT('Ctrl Pts',(-19.5399823241736,-13.1669554952568,
124.655332061422)) ;
#13226=CARTESIAN_POINT('Ctrl Pts',(-19.570139811574,-13.168357632994,124.651791395006)) ;
#13227=CARTESIAN_POINT('Ctrl Pts',(-19.6089550128361,-13.1701642708499,
124.645794258631)) ;
#13228=CARTESIAN_POINT('Ctrl Pts',(-19.6177566470167,-13.1705741618161,
124.644337728013)) ;
#13229=CARTESIAN_POINT('Ctrl Pts',(-19.6272606473483,-13.1710170818383,
124.642660248542)) ;
#13230=CARTESIAN_POINT('Ctrl Pts',(-19.627979228012,-13.1710505722539,124.642532768275)) ;
#13231=CARTESIAN_POINT('Ctrl Pts',(-19.6295028986685,-13.1711215893653,
124.642261083915)) ;
#13232=CARTESIAN_POINT('Ctrl Pts',(-19.630307959614,-13.1711591152381,124.642116718796)) ;
#13233=CARTESIAN_POINT('Ctrl Pts',(-19.6321185686697,-13.1712435182342,
124.641790202252)) ;
#13234=CARTESIAN_POINT('Ctrl Pts',(-19.6331240363326,-13.1712903931164,
124.641607607661)) ;
#13235=CARTESIAN_POINT('Ctrl Pts',(-19.6355950408535,-13.1714056020495,
124.641155738341)) ;
#13236=CARTESIAN_POINT('Ctrl Pts',(-19.6370603226104,-13.1714739291314,
124.640885075661)) ;
#13237=CARTESIAN_POINT('Ctrl Pts',(-19.6437717659995,-13.1717869335608,
124.63963294272)) ;
#13238=CARTESIAN_POINT('Ctrl Pts',(-19.6490120984118,-13.1720314554083,
124.638620497968)) ;
#13239=CARTESIAN_POINT('Ctrl Pts',(-19.662602030648,-13.1726659916714,124.635904490251)) ;
#13240=CARTESIAN_POINT('Ctrl Pts',(-19.6709409870404,-13.1730557513577,
124.634149051108)) ;
#13241=CARTESIAN_POINT('Ctrl Pts',(-19.6908393878121,-13.1739871506946,
124.629747266883)) ;
#13242=CARTESIAN_POINT('Ctrl Pts',(-19.7023804036596,-13.1745284529203,
124.627021432699)) ;
#13243=CARTESIAN_POINT('Ctrl Pts',(-19.7460984587356,-13.1765853735677,
124.616036769641)) ;
#13244=CARTESIAN_POINT('Ctrl Pts',(-19.7779804360324,-13.1781007308305,
124.606660698948)) ;
#13245=CARTESIAN_POINT('Ctrl Pts',(-19.8283478969974,-13.1805330323252,
124.589640101509)) ;
#13246=CARTESIAN_POINT('Ctrl Pts',(-19.8470892114594,-13.1814462454693,
124.582802908141)) ;
#13247=CARTESIAN_POINT('Ctrl Pts',(-19.8797664604814,-13.1830549926636,
124.569987420011)) ;
#13248=CARTESIAN_POINT('Ctrl Pts',(-19.8937722886083,-13.1837499850763,
124.564198562149)) ;
#13249=CARTESIAN_POINT('Ctrl Pts',(-19.9190991042095,-13.1850180725259,
124.553187179286)) ;
#13250=CARTESIAN_POINT('Ctrl Pts',(-19.9304538572855,-13.185590834726,124.548047198927)) ;
#13251=CARTESIAN_POINT('Ctrl Pts',(-19.9605375507083,-13.1871210210911,
124.533883301463)) ;
#13252=CARTESIAN_POINT('Ctrl Pts',(-19.9791213745648,-13.1880805375218,
124.524560560187)) ;
#13253=CARTESIAN_POINT('Ctrl Pts',(-20.011706357743,-13.1897841325236,124.507183557057)) ;
#13254=CARTESIAN_POINT('Ctrl Pts',(-20.0258003924317,-13.1905280291399,
124.499313134937)) ;
#13255=CARTESIAN_POINT('Ctrl Pts',(-20.0451481404434,-13.1915580342455,
124.488011880329)) ;
#13256=CARTESIAN_POINT('Ctrl Pts',(-20.0505343489378,-13.1918457553199,
124.484811177997)) ;
#13257=CARTESIAN_POINT('Ctrl Pts',(-20.0595177192731,-13.1923272742818,
124.479381094275)) ;
#13258=CARTESIAN_POINT('Ctrl Pts',(-20.06312802651,-13.1925212411184,124.477173701232)) ;
#13259=CARTESIAN_POINT('Ctrl Pts',(-20.0707778154162,-13.1929332048542,
124.472442978393)) ;
#13260=CARTESIAN_POINT('Ctrl Pts',(-20.0748142264151,-13.1931511586604,
124.469914807443)) ;
#13261=CARTESIAN_POINT('Ctrl Pts',(-20.0835648084347,-13.1936249669841,
124.464364073129)) ;
#13262=CARTESIAN_POINT('Ctrl Pts',(-20.088273318736,-13.1938807445917,124.461332774182)) ;
#13263=CARTESIAN_POINT('Ctrl Pts',(-20.1002424181368,-13.1945331689814,
124.453512907989)) ;
#13264=CARTESIAN_POINT('Ctrl Pts',(-20.1074736957034,-13.1949294546799,
124.448680011807)) ;
#13265=CARTESIAN_POINT('Ctrl Pts',(-20.1314072437273,-13.1962489094192,
124.432320534887)) ;
#13266=CARTESIAN_POINT('Ctrl Pts',(-20.1478791658137,-13.1971697804674,
124.420462775931)) ;
#13267=CARTESIAN_POINT('Ctrl Pts',(-20.1789628313203,-13.1989415873577,
124.396916469971)) ;
#13268=CARTESIAN_POINT('Ctrl Pts',(-20.1936151270096,-13.1997923122615,
124.38529060656)) ;
#13269=CARTESIAN_POINT('Ctrl Pts',(-20.2124628006012,-13.2009109731273,
124.369634058183)) ;
#13270=CARTESIAN_POINT('Ctrl Pts',(-20.2168987312121,-13.2011760663774,
124.365896694586)) ;
#13271=CARTESIAN_POINT('Ctrl Pts',(-20.2248042548,-13.2016518552551,124.359141485154)) ;
#13272=CARTESIAN_POINT('Ctrl Pts',(-20.2282835151841,-13.2018624337127,
124.35613511065)) ;
#13273=CARTESIAN_POINT('Ctrl Pts',(-20.2350006148788,-13.2022713162564,
124.350265922449)) ;
#13274=CARTESIAN_POINT('Ctrl Pts',(-20.2382403519709,-13.2024695946763,
124.34740537817)) ;
#13275=CARTESIAN_POINT('Ctrl Pts',(-20.2415009548241,-13.2026702463444,
124.344496178256)) ;
#13276=CARTESIAN_POINT('Ctrl Pts',(-20.2415367247745,-13.2026724476971,
124.344464259622)) ;
#13277=CARTESIAN_POINT('Ctrl Pts',(-20.2416084121409,-13.2026768597465,
124.344400283358)) ;
#13278=CARTESIAN_POINT('Ctrl Pts',(-20.2416443297749,-13.2026790704577,
124.344368225502)) ;
#13279=CARTESIAN_POINT('Ctrl Pts',(-20.241716322823,-13.2026835018622,124.344303961493)) ;
#13280=CARTESIAN_POINT('Ctrl Pts',(-20.2417523976714,-13.2026857225219,
124.344271755811)) ;
#13281=CARTESIAN_POINT('Ctrl Pts',(-20.2418247136814,-13.2026901743526,
124.344207188429)) ;
#13282=CARTESIAN_POINT('Ctrl Pts',(-20.2418609547872,-13.2026924055213,
124.344174826744)) ;
#13283=CARTESIAN_POINT('Ctrl Pts',(-20.241933612165,-13.202696878919,124.344109939344)) ;
#13284=CARTESIAN_POINT('Ctrl Pts',(-20.2419700285834,-13.2026991211583,
124.344077413461)) ;
#13285=CARTESIAN_POINT('Ctrl Pts',(-20.2420430462514,-13.2027036172961,
124.344012188917)) ;
#13286=CARTESIAN_POINT('Ctrl Pts',(-20.242079647378,-13.2027058711886,124.343979490328)) ;
#13287=CARTESIAN_POINT('Ctrl Pts',(-20.2421530437522,-13.2027103912095,
124.343913911951)) ;
#13288=CARTESIAN_POINT('Ctrl Pts',(-20.2421898389658,-13.2027126573372,
124.343881032153)) ;
#13289=CARTESIAN_POINT('Ctrl Pts',(-20.2422636327911,-13.2027172024045,
124.343815082944)) ;
#13290=CARTESIAN_POINT('Ctrl Pts',(-20.2423006314859,-13.2027194813508,
124.343782013414)) ;
#13291=CARTESIAN_POINT('Ctrl Pts',(-20.2423748418137,-13.2027240526477,
124.343715676079)) ;
#13292=CARTESIAN_POINT('Ctrl Pts',(-20.2424120535201,-13.2027263450045,
124.343682408162)) ;
#13293=CARTESIAN_POINT('Ctrl Pts',(-20.242486699591,-13.2027309437264,124.343615665223)) ;
#13294=CARTESIAN_POINT('Ctrl Pts',(-20.2425241339824,-13.2027332500949,
124.343582190128)) ;
#13295=CARTESIAN_POINT('Ctrl Pts',(-20.2425992350049,-13.2027378774359,
124.343515024115)) ;
#13296=CARTESIAN_POINT('Ctrl Pts',(-20.2426369017402,-13.2027401984166,
124.343481333054)) ;
#13297=CARTESIAN_POINT('Ctrl Pts',(-20.2427124776084,-13.2027448556137,
124.343413725867)) ;
#13298=CARTESIAN_POINT('Ctrl Pts',(-20.2427503866397,-13.2027471918257,
124.343379809779)) ;
#13299=CARTESIAN_POINT('Ctrl Pts',(-20.2428264570372,-13.2027518801036,
124.343311743486)) ;
#13300=CARTESIAN_POINT('Ctrl Pts',(-20.2428646183768,-13.2027542321699,
124.343277593248)) ;
#13301=CARTESIAN_POINT('Ctrl Pts',(-20.2465276130872,-13.2029800148025,
124.339999207004)) ;
#13302=CARTESIAN_POINT('Ctrl Pts',(-20.2501334717912,-13.203203658973,124.336733847621)) ;
#13303=CARTESIAN_POINT('Ctrl Pts',(-20.2589724710791,-13.2037553160657,
124.328635099664)) ;
#13304=CARTESIAN_POINT('Ctrl Pts',(-20.2641835221125,-13.2040835582772,
124.323777873765)) ;
#13305=CARTESIAN_POINT('Ctrl Pts',(-20.279355708365,-13.2050481212444,124.309391534564)) ;
#13306=CARTESIAN_POINT('Ctrl Pts',(-20.2892010393449,-13.2056854730979,
124.299741908408)) ;
#13307=CARTESIAN_POINT('Ctrl Pts',(-20.3188834461116,-13.2076412136095,
124.269670930688)) ;
#13308=CARTESIAN_POINT('Ctrl Pts',(-20.3381843649342,-13.208960842666,124.24873295245)) ;
#13309=CARTESIAN_POINT('Ctrl Pts',(-20.3615161931857,-13.2106091507762,
124.221619749046)) ;
#13310=CARTESIAN_POINT('Ctrl Pts',(-20.3662301694618,-13.2109451172313,
124.216043703116)) ;
#13311=CARTESIAN_POINT('Ctrl Pts',(-20.3734020262741,-13.211460815155,124.207407946915)) ;
#13312=CARTESIAN_POINT('Ctrl Pts',(-20.375894791969,-13.211640925463,124.204377444177)) ;
#13313=CARTESIAN_POINT('Ctrl Pts',(-20.3801244114799,-13.2119480236235,
124.199185778373)) ;
#13314=CARTESIAN_POINT('Ctrl Pts',(-20.3818684178132,-13.2120750897628,
124.197030485814)) ;
#13315=CARTESIAN_POINT('Ctrl Pts',(-20.3836409275724,-13.2122046863192,
124.19482500258)) ;
#13316=CARTESIAN_POINT('Ctrl Pts',(-20.3836766105861,-13.2122072954613,
124.194780597009)) ;
#13317=CARTESIAN_POINT('Ctrl Pts',(-20.3837438250645,-13.2122122105394,
124.194696940534)) ;
#13318=CARTESIAN_POINT('Ctrl Pts',(-20.383775357339,-13.2122145164933,124.194657689982)) ;
#13319=CARTESIAN_POINT('Ctrl Pts',(-20.3838346878026,-13.2122188556048,
124.194583827831)) ;
#13320=CARTESIAN_POINT('Ctrl Pts',(-20.3838624865803,-13.2122208887727,
124.19454921658)) ;
#13321=CARTESIAN_POINT('Ctrl Pts',(-20.3839147403571,-13.212224710764,124.194484150196)) ;
#13322=CARTESIAN_POINT('Ctrl Pts',(-20.3839391955521,-13.2122264995759,
124.194453695673)) ;
#13323=CARTESIAN_POINT('Ctrl Pts',(-20.3839851232315,-13.2122298591915,
124.194396495561)) ;
#13324=CARTESIAN_POINT('Ctrl Pts',(-20.384006596013,-13.2122314299965,124.194369750273)) ;
#13325=CARTESIAN_POINT('Ctrl Pts',(-20.3840575440562,-13.212235157177,124.194306286905)) ;
#13326=CARTESIAN_POINT('Ctrl Pts',(-20.3840870182223,-13.2122373135327,
124.194269568197)) ;
#13327=CARTESIAN_POINT('Ctrl Pts',(-20.3841450951676,-13.2122415627468,
124.194197207973)) ;
#13328=CARTESIAN_POINT('Ctrl Pts',(-20.3841736982301,-13.2122436556185,
124.194161566351)) ;
#13329=CARTESIAN_POINT('Ctrl Pts',(-20.3842300466298,-13.212247778842,124.19409134401)) ;
#13330=CARTESIAN_POINT('Ctrl Pts',(-20.3842577921076,-13.2122498091969,
124.194056763352)) ;
#13331=CARTESIAN_POINT('Ctrl Pts',(-20.3843124396511,-13.2122538084129,
124.193988645799)) ;
#13332=CARTESIAN_POINT('Ctrl Pts',(-20.3843393416097,-13.2122557772594,
124.193955109264)) ;
#13333=CARTESIAN_POINT('Ctrl Pts',(-20.3843923164775,-13.2122596544895,
124.193889062722)) ;
#13334=CARTESIAN_POINT('Ctrl Pts',(-20.384418389635,-13.2122615628848,124.193856552621)) ;
#13335=CARTESIAN_POINT('Ctrl Pts',(-20.3844697217364,-13.212265320279,124.193792541086)) ;
#13336=CARTESIAN_POINT('Ctrl Pts',(-20.3844949808291,-13.2122671692827,
124.193761039671)) ;
#13337=CARTESIAN_POINT('Ctrl Pts',(-20.3845447001952,-13.2122708090022,
124.193699026918)) ;
#13338=CARTESIAN_POINT('Ctrl Pts',(-20.3845691604211,-13.2122725997086,
124.193668515833)) ;
#13339=CARTESIAN_POINT('Ctrl Pts',(-20.387271314347,-13.2124704312913,124.190297591266)) ;
#13340=CARTESIAN_POINT('Ctrl Pts',(-20.3899318356961,-13.2126662822313,
124.186943438435)) ;
#13341=CARTESIAN_POINT('Ctrl Pts',(-20.3956417030208,-13.2130889627621,
124.179668483476)) ;
#13342=CARTESIAN_POINT('Ctrl Pts',(-20.3986850183309,-13.2133157255107,
124.175743039087)) ;
#13343=CARTESIAN_POINT('Ctrl Pts',(-20.4066368105968,-13.2139122399235,
124.165359128652)) ;
#13344=CARTESIAN_POINT('Ctrl Pts',(-20.4115059607716,-13.2142815979078,
124.158870833534)) ;
#13345=CARTESIAN_POINT('Ctrl Pts',(-20.4279107743671,-13.2155408918573,
124.136561825865)) ;
#13346=CARTESIAN_POINT('Ctrl Pts',(-20.4391377325234,-13.2164282997163,
124.120517698698)) ;
#13347=CARTESIAN_POINT('Ctrl Pts',(-20.4604098068225,-13.2181707260936,
124.088544831266)) ;
#13348=CARTESIAN_POINT('Ctrl Pts',(-20.4704810381876,-13.2190255576639,
124.072639749763)) ;
#13349=CARTESIAN_POINT('Ctrl Pts',(-20.4846951720288,-13.2202814601768,
124.049028487326)) ;
#13350=CARTESIAN_POINT('Ctrl Pts',(-20.4891225103211,-13.2206801676099,
124.041496596796)) ;
#13351=CARTESIAN_POINT('Ctrl Pts',(-20.4959629754166,-13.2213085324731,
124.029575095466)) ;
#13352=CARTESIAN_POINT('Ctrl Pts',(-20.4984293048242,-13.221537713073,124.0252163233)) ;
#13353=CARTESIAN_POINT('Ctrl Pts',(-20.5028175879064,-13.2219503033097,
124.017350948677)) ;
#13354=CARTESIAN_POINT('Ctrl Pts',(-20.5047490376571,-13.2221336247457,
124.013849719241)) ;
#13355=CARTESIAN_POINT('Ctrl Pts',(-20.5067105899526,-13.2223215959497,
124.010253226312)) ;
#13356=CARTESIAN_POINT('Ctrl Pts',(-20.5067575187116,-13.2223260940893,
124.010167158665)) ;
#13357=CARTESIAN_POINT('Ctrl Pts',(-20.5068505934254,-13.2223350174414,
124.00999641125)) ;
#13358=CARTESIAN_POINT('Ctrl Pts',(-20.5068967396566,-13.2223394426462,
124.009911731753)) ;
#13359=CARTESIAN_POINT('Ctrl Pts',(-20.5069883325988,-13.2223482280149,
124.009743610095)) ;
#13360=CARTESIAN_POINT('Ctrl Pts',(-20.5070337796333,-13.2223525881798,
124.009660168022)) ;
#13361=CARTESIAN_POINT('Ctrl Pts',(-20.5071240516448,-13.2223612508123,
124.009494380994)) ;
#13362=CARTESIAN_POINT('Ctrl Pts',(-20.5071688768753,-13.2223655532779,
124.00941203617)) ;
#13363=CARTESIAN_POINT('Ctrl Pts',(-20.5072579776126,-13.2223741073777,
124.009248312512)) ;
#13364=CARTESIAN_POINT('Ctrl Pts',(-20.5073022532778,-13.2223783590042,
124.009166933908)) ;
#13365=CARTESIAN_POINT('Ctrl Pts',(-20.5073903223693,-13.222386817839,124.009005020179)) ;
#13366=CARTESIAN_POINT('Ctrl Pts',(-20.5074341160333,-13.2223910250504,
124.008924485067)) ;
#13367=CARTESIAN_POINT('Ctrl Pts',(-20.5075212847402,-13.2223994011089,
124.008764142647)) ;
#13368=CARTESIAN_POINT('Ctrl Pts',(-20.5075646599821,-13.2224035699582,
124.008684335357)) ;
#13369=CARTESIAN_POINT('Ctrl Pts',(-20.5076510520888,-13.2224118750332,
124.008525338863)) ;
#13370=CARTESIAN_POINT('Ctrl Pts',(-20.5076940690545,-13.2224160112544,
124.008446149797)) ;
#13371=CARTESIAN_POINT('Ctrl Pts',(-20.5077798015358,-13.2224242565055,
124.0082882859)) ;
#13372=CARTESIAN_POINT('Ctrl Pts',(-20.5078225172013,-13.2224283655379,
124.008209611062)) ;
#13373=CARTESIAN_POINT('Ctrl Pts',(-20.5079077016156,-13.2224365616231,
124.008052675961)) ;
#13374=CARTESIAN_POINT('Ctrl Pts',(-20.5079501703968,-13.2224406486693,
124.007974415855)) ;
#13375=CARTESIAN_POINT('Ctrl Pts',(-20.5080349130489,-13.2224488057597,
124.007818215007)) ;
#13376=CARTESIAN_POINT('Ctrl Pts',(-20.5080771869836,-13.2224528758026,
124.007740274315)) ;
#13377=CARTESIAN_POINT('Ctrl Pts',(-20.5081615899908,-13.2224610036838,
124.007584620499)) ;
#13378=CARTESIAN_POINT('Ctrl Pts',(-20.5082037191219,-13.2224650615225,
124.007506907386)) ;
#13379=CARTESIAN_POINT('Ctrl Pts',(-20.5082878809129,-13.2224731696416,
124.007351619802)) ;
#13380=CARTESIAN_POINT('Ctrl Pts',(-20.5083299136024,-13.2224772199216,
124.007274045351)) ;
#13381=CARTESIAN_POINT('Ctrl Pts',(-20.5084139292939,-13.2224853174226,
124.007118948949)) ;
#13382=CARTESIAN_POINT('Ctrl Pts',(-20.5084559123575,-13.2224893646482,
124.007041426915)) ;
#13383=CARTESIAN_POINT('Ctrl Pts',(-20.5085398747323,-13.2224974604656,
124.006886350601)) ;
#13384=CARTESIAN_POINT('Ctrl Pts',(-20.5085818539358,-13.2225015090477,
124.006808796508)) ;
#13385=CARTESIAN_POINT('Ctrl Pts',(-20.5086658531473,-13.2225096118778,
124.006653573701)) ;
#13386=CARTESIAN_POINT('Ctrl Pts',(-20.5087078731521,-13.2225136661279,
124.00657590494)) ;
#13387=CARTESIAN_POINT('Ctrl Pts',(-20.5087919977242,-13.2225217845244,
124.006420371736)) ;
#13388=CARTESIAN_POINT('Ctrl Pts',(-20.5088341023445,-13.2225258486801,
124.0063425071)) ;
#13389=CARTESIAN_POINT('Ctrl Pts',(-20.5089184396558,-13.2225339911008,
124.006186501382)) ;
#13390=CARTESIAN_POINT('Ctrl Pts',(-20.5089606722452,-13.2225380693621,
124.006108360351)) ;
#13391=CARTESIAN_POINT('Ctrl Pts',(-20.5090453082258,-13.2225462441396,
124.00595172235)) ;
#13392=CARTESIAN_POINT('Ctrl Pts',(-20.5090877115827,-13.2225503406603,
124.005873225265)) ;
#13393=CARTESIAN_POINT('Ctrl Pts',(-20.5091727318396,-13.2225585561104,
124.005715795483)) ;
#13394=CARTESIAN_POINT('Ctrl Pts',(-20.5092153485984,-13.2225626750358,
124.005636862826)) ;
#13395=CARTESIAN_POINT('Ctrl Pts',(-20.509300838192,-13.2225709394361,124.005478482443)) ;
#13396=CARTESIAN_POINT('Ctrl Pts',(-20.5093437108805,-13.2225750849084,
124.005399034726)) ;
#13397=CARTESIAN_POINT('Ctrl Pts',(-20.5094297547471,-13.2225834065394,
124.00523954482)) ;
#13398=CARTESIAN_POINT('Ctrl Pts',(-20.5094729258629,-13.2225875827056,
124.005159502441)) ;
#13399=CARTESIAN_POINT('Ctrl Pts',(-20.5095596094434,-13.2225959699116,
124.00499874281)) ;
#13400=CARTESIAN_POINT('Ctrl Pts',(-20.5096031217613,-13.2226001809528,
124.004918025482)) ;
#13401=CARTESIAN_POINT('Ctrl Pts',(-20.5096905308847,-13.2226086421313,
124.004755834856)) ;
#13402=CARTESIAN_POINT('Ctrl Pts',(-20.5097344275118,-13.2226128922687,
124.004674361496)) ;
#13403=CARTESIAN_POINT('Ctrl Pts',(-20.5098226488504,-13.2226214359145,
124.004510576681)) ;
#13404=CARTESIAN_POINT('Ctrl Pts',(-20.5098669733686,-13.2226257294237,
124.004428265143)) ;
#13405=CARTESIAN_POINT('Ctrl Pts',(-20.5099560947392,-13.222634364159,124.004262720447)) ;
#13406=CARTESIAN_POINT('Ctrl Pts',(-20.5100008913645,-13.2226387053849,
124.004179487218)) ;
#13407=CARTESIAN_POINT('Ctrl Pts',(-20.5100910019517,-13.2226474399816,
124.004012014019)) ;
#13408=CARTESIAN_POINT('Ctrl Pts',(-20.5101363156724,-13.222651833353,124.003927773953)) ;
#13409=CARTESIAN_POINT('Ctrl Pts',(-20.5102275062613,-13.2226606767558,
124.003758200254)) ;
#13410=CARTESIAN_POINT('Ctrl Pts',(-20.5102733829157,-13.222665126793,124.003672866418)) ;
#13411=CARTESIAN_POINT('Ctrl Pts',(-20.510365746308,-13.2226740881611,124.003501016047)) ;
#13412=CARTESIAN_POINT('Ctrl Pts',(-20.5104122327811,-13.2226785994953,
124.003414499346)) ;
#13413=CARTESIAN_POINT('Ctrl Pts',(-20.5127192806822,-13.2229025432853,
123.999119602498)) ;
#13414=CARTESIAN_POINT('Ctrl Pts',(-20.51495570431,-13.2231221882135,123.994898312744)) ;
#13415=CARTESIAN_POINT('Ctrl Pts',(-20.5203926287287,-13.2236625351034,
123.984492257007)) ;
#13416=CARTESIAN_POINT('Ctrl Pts',(-20.5235657444156,-13.2239834654429,
123.978293377557)) ;
#13417=CARTESIAN_POINT('Ctrl Pts',(-20.5324914662498,-13.2249024247406,
123.960491214424)) ;
#13418=CARTESIAN_POINT('Ctrl Pts',(-20.5381157482922,-13.2255014262097,
123.948824649928)) ;
#13419=CARTESIAN_POINT('Ctrl Pts',(-20.5497460249898,-13.2267836645162,
123.923709293786)) ;
#13420=CARTESIAN_POINT('Ctrl Pts',(-20.5556976834382,-13.2274672902103,
123.910237450697)) ;
#13421=CARTESIAN_POINT('Ctrl Pts',(-20.5687669555109,-13.2290298513582,
123.879181200905)) ;
#13422=CARTESIAN_POINT('Ctrl Pts',(-20.5757252103543,-13.2299077599351,
123.861533427979)) ;
#13423=CARTESIAN_POINT('Ctrl Pts',(-20.5840096247004,-13.2310117694385,
123.839034620967)) ;
#13424=CARTESIAN_POINT('Ctrl Pts',(-20.5857117523212,-13.2312420594871,
123.834324890587)) ;
#13425=CARTESIAN_POINT('Ctrl Pts',(-20.5883811745478,-13.231608824275,123.826797480329)) ;
#13426=CARTESIAN_POINT('Ctrl Pts',(-20.5893667745698,-13.2317455053305,
123.823986361942)) ;
#13427=CARTESIAN_POINT('Ctrl Pts',(-20.5913247343314,-13.2320195997308,
123.818337293829)) ;
#13428=CARTESIAN_POINT('Ctrl Pts',(-20.592296945304,-13.2321570105281,123.815499313575)) ;
#13429=CARTESIAN_POINT('Ctrl Pts',(-20.5932702436132,-13.232295919675,123.812624445251)) ;
#13430=CARTESIAN_POINT('Ctrl Pts',(-20.5932815534663,-13.2322975340031,
123.812591034251)) ;
#13431=CARTESIAN_POINT('Ctrl Pts',(-20.5933039539709,-13.2323007317392,
123.812524850581)) ;
#13432=CARTESIAN_POINT('Ctrl Pts',(-20.5933150446569,-13.2323023151451,
123.812492077986)) ;
#13433=CARTESIAN_POINT('Ctrl Pts',(-20.593337007394,-13.2323054510967,123.812427169979)) ;
#13434=CARTESIAN_POINT('Ctrl Pts',(-20.5933478795744,-13.2323070036539,
123.812395034357)) ;
#13435=CARTESIAN_POINT('Ctrl Pts',(-20.5933694060848,-13.2323100779995,
123.812331398497)) ;
#13436=CARTESIAN_POINT('Ctrl Pts',(-20.5933800603911,-13.2323115997778,
123.812299898496)) ;
#13437=CARTESIAN_POINT('Ctrl Pts',(-20.5934011519478,-13.232314612659,123.812237532032)) ;
#13438=CARTESIAN_POINT('Ctrl Pts',(-20.5934115892942,-13.232316103769,123.812206665449)) ;
#13439=CARTESIAN_POINT('Ctrl Pts',(-20.5934322479728,-13.2323190554426,
123.812145563235)) ;
#13440=CARTESIAN_POINT('Ctrl Pts',(-20.5934424691705,-13.2323205159807,
123.812115328163)) ;
#13441=CARTESIAN_POINT('Ctrl Pts',(-20.5934626964174,-13.2323234066149,
123.812055486888)) ;
#13442=CARTESIAN_POINT('Ctrl Pts',(-20.5934727027086,-13.2323248367394,
123.812025880128)) ;
#13443=CARTESIAN_POINT('Ctrl Pts',(-20.5934925013243,-13.2323276666968,
123.811967292451)) ;
#13444=CARTESIAN_POINT('Ctrl Pts',(-20.5935022936413,-13.2323290665225,
123.811938311711)) ;
#13445=CARTESIAN_POINT('Ctrl Pts',(-20.5935216656142,-13.2323318360507,
123.811880972668)) ;
#13446=CARTESIAN_POINT('Ctrl Pts',(-20.593531245312,-13.2323332057531,123.811852614391)) ;
#13447=CARTESIAN_POINT('Ctrl Pts',(-20.5935501933926,-13.2323359152095,
123.811796516736)) ;
#13448=CARTESIAN_POINT('Ctrl Pts',(-20.5935595618137,-13.232337254963,123.81176877739)) ;
#13449=CARTESIAN_POINT('Ctrl Pts',(-20.5949634967169,-13.2325380472751,
123.807611326579)) ;
#13450=CARTESIAN_POINT('Ctrl Pts',(-20.5963364569888,-13.2327372525458,
123.80347433993)) ;
#13451=CARTESIAN_POINT('Ctrl Pts',(-20.5992447333403,-13.233165478885,123.794555374446)) ;
#13452=CARTESIAN_POINT('Ctrl Pts',(-20.6007729250949,-13.2333944186272,
123.789771152056)) ;
#13453=CARTESIAN_POINT('Ctrl Pts',(-20.6050610497314,-13.2340483877114,
123.776062058956)) ;
#13454=CARTESIAN_POINT('Ctrl Pts',(-20.6077498272948,-13.2344726890735,
123.767115271395)) ;
#13455=CARTESIAN_POINT('Ctrl Pts',(-20.6198084755657,-13.2364464684551,
123.725295478689)) ;
#13456=CARTESIAN_POINT('Ctrl Pts',(-20.6279276550355,-13.2379883912266,
123.692077419293)) ;
#13457=CARTESIAN_POINT('Ctrl Pts',(-20.6362462453926,-13.2399072669868,
123.650766479905)) ;
#13458=CARTESIAN_POINT('Ctrl Pts',(-20.6377426628943,-13.2402702657409,
123.642950130762)) ;
#13459=CARTESIAN_POINT('Ctrl Pts',(-20.639956169466,-13.2408365305729,123.63075888611)) ;
#13460=CARTESIAN_POINT('Ctrl Pts',(-20.6407248013252,-13.2410393107784,
123.62639354988)) ;
#13461=CARTESIAN_POINT('Ctrl Pts',(-20.6420475115065,-13.2413995259455,
123.618640151511)) ;
#13462=CARTESIAN_POINT('Ctrl Pts',(-20.6426108818422,-13.2415568735001,
123.615253718243)) ;
#13463=CARTESIAN_POINT('Ctrl Pts',(-20.6432139852792,-13.2417297357313,
123.611533849585)) ;
#13464=CARTESIAN_POINT('Ctrl Pts',(-20.643267543516,-13.2417451260631,123.611202664968)) ;
#13465=CARTESIAN_POINT('Ctrl Pts',(-20.6433625295904,-13.2417724912093,
123.610613801525)) ;
#13466=CARTESIAN_POINT('Ctrl Pts',(-20.6434040100676,-13.241784465553,123.610356131217)) ;
#13467=CARTESIAN_POINT('Ctrl Pts',(-20.6434793526173,-13.2418062587071,
123.60988717903)) ;
#13468=CARTESIAN_POINT('Ctrl Pts',(-20.6435132411385,-13.2418160772806,
123.609675901436)) ;
#13469=CARTESIAN_POINT('Ctrl Pts',(-20.6435758635897,-13.2418342509642,
123.609284840375)) ;
#13470=CARTESIAN_POINT('Ctrl Pts',(-20.6436046125028,-13.2418426059436,
123.609105059261)) ;
#13471=CARTESIAN_POINT('Ctrl Pts',(-20.6436584482548,-13.2418582736923,
123.608767925417)) ;
#13472=CARTESIAN_POINT('Ctrl Pts',(-20.6436835442932,-13.241865586382,123.608610574118)) ;
#13473=CARTESIAN_POINT('Ctrl Pts',(-20.6437310470047,-13.2418794452309,
123.608312367153)) ;
#13474=CARTESIAN_POINT('Ctrl Pts',(-20.6437534596543,-13.241885991336,123.608171512468)) ;
#13475=CARTESIAN_POINT('Ctrl Pts',(-20.6437962658573,-13.2418985076946,
123.607902195314)) ;
#13476=CARTESIAN_POINT('Ctrl Pts',(-20.6438166634713,-13.2419044779131,
123.607773733471)) ;
#13477=CARTESIAN_POINT('Ctrl Pts',(-20.6438559229165,-13.2419159804863,
123.607526232546)) ;
#13478=CARTESIAN_POINT('Ctrl Pts',(-20.6438747875813,-13.2419215128154,
123.607407193926)) ;
#13479=CARTESIAN_POINT('Ctrl Pts',(-20.6439113434672,-13.2419322434317,
123.607176305273)) ;
#13480=CARTESIAN_POINT('Ctrl Pts',(-20.6439290367006,-13.2419374416993,
123.607064455597)) ;
#13481=CARTESIAN_POINT('Ctrl Pts',(-20.64396353105,-13.2419475851048,123.606846203688)) ;
#13482=CARTESIAN_POINT('Ctrl Pts',(-20.6439803336231,-13.2419525302333,
123.60673980161)) ;
#13483=CARTESIAN_POINT('Ctrl Pts',(-20.6440132725188,-13.2419622325864,
123.606531041336)) ;
#13484=CARTESIAN_POINT('Ctrl Pts',(-20.6440294098682,-13.241966989802,123.606428683301)) ;
#13485=CARTESIAN_POINT('Ctrl Pts',(-20.6440612056593,-13.2419763706723,
123.606226841756)) ;
#13486=CARTESIAN_POINT('Ctrl Pts',(-20.6440768647887,-13.2419809943155,
123.606127358472)) ;
#13487=CARTESIAN_POINT('Ctrl Pts',(-20.6441078645935,-13.241990154814,123.60593025999)) ;
#13488=CARTESIAN_POINT('Ctrl Pts',(-20.6441232057302,-13.2419946916694,
123.605832644777)) ;
#13489=CARTESIAN_POINT('Ctrl Pts',(-20.644153711724,-13.242003720262,123.605638385829)) ;
#13490=CARTESIAN_POINT('Ctrl Pts',(-20.644168876814,-13.242008211998,123.605541742112)) ;
#13491=CARTESIAN_POINT('Ctrl Pts',(-20.6441991609771,-13.242017188754,123.605348599886)) ;
#13492=CARTESIAN_POINT('Ctrl Pts',(-20.6442142800696,-13.242021673769,123.605252101481)) ;
#13493=CARTESIAN_POINT('Ctrl Pts',(-20.6442445955782,-13.2420306736674,
123.605058462736)) ;
#13494=CARTESIAN_POINT('Ctrl Pts',(-20.6442597918502,-13.242035188554,123.604961322332)) ;
#13495=CARTESIAN_POINT('Ctrl Pts',(-20.6442903824531,-13.2420442842324,
123.604765624249)) ;
#13496=CARTESIAN_POINT('Ctrl Pts',(-20.6443057764614,-13.2420488650311,
123.604667066432)) ;
#13497=CARTESIAN_POINT('Ctrl Pts',(-20.6443368845317,-13.2420581291745,
123.60446774522)) ;
#13498=CARTESIAN_POINT('Ctrl Pts',(-20.6443525980408,-13.2420628125177,
123.604366981871)) ;
#13499=CARTESIAN_POINT('Ctrl Pts',(-20.6443844718098,-13.2420723200347,
123.604162425944)) ;
#13500=CARTESIAN_POINT('Ctrl Pts',(-20.6444006313255,-13.2420771442172,
123.604058633201)) ;
#13501=CARTESIAN_POINT('Ctrl Pts',(-20.644433532294,-13.2420869745007,123.603847134545)) ;
#13502=CARTESIAN_POINT('Ctrl Pts',(-20.6444502727458,-13.2420919806114,
123.603739428455)) ;
#13503=CARTESIAN_POINT('Ctrl Pts',(-20.6444844831264,-13.2421022198438,
123.603519133043)) ;
#13504=CARTESIAN_POINT('Ctrl Pts',(-20.6445019517491,-13.2421074529765,
123.603406543524)) ;
#13505=CARTESIAN_POINT('Ctrl Pts',(-20.6449826564407,-13.2422515899396,
123.600305486515)) ;
#13506=CARTESIAN_POINT('Ctrl Pts',(-20.6454350606017,-13.2423905868134,
123.597315354453)) ;
#13507=CARTESIAN_POINT('Ctrl Pts',(-20.646710448646,-13.2427923297152,123.588673872152)) ;
#13508=CARTESIAN_POINT('Ctrl Pts',(-20.6475055582442,-13.2430553012139,
123.583018496788)) ;
#13509=CARTESIAN_POINT('Ctrl Pts',(-20.6496686256223,-13.243808176189,123.566829290923)) ;
#13510=CARTESIAN_POINT('Ctrl Pts',(-20.6509411030967,-13.2442987359153,
123.556283232296)) ;
#13511=CARTESIAN_POINT('Ctrl Pts',(-20.6547674229386,-13.2459499561538,
123.520770943318)) ;
#13512=CARTESIAN_POINT('Ctrl Pts',(-20.6567038410745,-13.2471120323295,
123.495744117968)) ;
#13513=CARTESIAN_POINT('Ctrl Pts',(-20.6583711143033,-13.2487443418533,
123.460376708612)) ;
#13514=CARTESIAN_POINT('Ctrl Pts',(-20.658729187192,-13.2492189084885,123.450071881699)) ;
#13515=CARTESIAN_POINT('Ctrl Pts',(-20.659081761401,-13.2499434469168,123.434307408055)) ;
#13516=CARTESIAN_POINT('Ctrl Pts',(-20.6591680572249,-13.2501939920321,
123.428850299373)) ;
#13517=CARTESIAN_POINT('Ctrl Pts',(-20.6592697800476,-13.2506976969608,
123.417868832571)) ;
#13518=CARTESIAN_POINT('Ctrl Pts',(-20.6592843302475,-13.2509508458169,
123.412344587542)) ;
#13519=CARTESIAN_POINT('Ctrl Pts',(-20.6592320658466,-13.2515498551347,
123.399262759844)) ;
#13520=CARTESIAN_POINT('Ctrl Pts',(-20.659133329772,-13.2518955266524,123.391705517948)) ;
#13521=CARTESIAN_POINT('Ctrl Pts',(-20.6587447242202,-13.2526979643449,
123.374151119848)) ;
#13522=CARTESIAN_POINT('Ctrl Pts',(-20.6584033994821,-13.2531544857217,
123.364155621625)) ;
#13523=CARTESIAN_POINT('Ctrl Pts',(-20.657046757164,-13.2544968066178,123.334770965737)) ;
#13524=CARTESIAN_POINT('Ctrl Pts',(-20.6556996299527,-13.2553818816995,
123.31540022368)) ;
#13525=CARTESIAN_POINT('Ctrl Pts',(-20.6535233190389,-13.2564573036706,
123.291998019709)) ;
#13526=CARTESIAN_POINT('Ctrl Pts',(-20.653124782946,-13.2566445191073,123.287929113048)) ;
#13527=CARTESIAN_POINT('Ctrl Pts',(-20.6523541012807,-13.256989643681,123.280439657227)) ;
#13528=CARTESIAN_POINT('Ctrl Pts',(-20.6519877812442,-13.2571474886067,
123.277018552164)) ;
#13529=CARTESIAN_POINT('Ctrl Pts',(-20.6510804613769,-13.2575241778776,
123.268863197068)) ;
#13530=CARTESIAN_POINT('Ctrl Pts',(-20.6505265065881,-13.2577431117644,
123.264130443661)) ;
#13531=CARTESIAN_POINT('Ctrl Pts',(-20.6493650304723,-13.2581810325394,
123.254675812322)) ;
#13532=CARTESIAN_POINT('Ctrl Pts',(-20.648757567283,-13.2584000157855,123.249954002097)) ;
#13533=CARTESIAN_POINT('Ctrl Pts',(-20.6455744831582,-13.2594990464321,
123.226281291259)) ;
#13534=CARTESIAN_POINT('Ctrl Pts',(-20.6425911423181,-13.260379790579,123.207387737494)) ;
#13535=CARTESIAN_POINT('Ctrl Pts',(-20.6377892840867,-13.2616155057429,
123.180933216226)) ;
#13536=CARTESIAN_POINT('Ctrl Pts',(-20.6363319886945,-13.2619719370507,
123.173309425696)) ;
#13537=CARTESIAN_POINT('Ctrl Pts',(-20.63359074007,-13.2626106272623,123.159659339202)) ;
#13538=CARTESIAN_POINT('Ctrl Pts',(-20.6323330578236,-13.262893015385,123.153628031461)) ;
#13539=CARTESIAN_POINT('Ctrl Pts',(-20.6298130798562,-13.2634389804049,
123.141975078206)) ;
#13540=CARTESIAN_POINT('Ctrl Pts',(-20.6285564052381,-13.2637025829745,
123.13635237654)) ;
#13541=CARTESIAN_POINT('Ctrl Pts',(-20.6257019214129,-13.26428290333,123.123983012898)) ;
#13542=CARTESIAN_POINT('Ctrl Pts',(-20.624086762122,-13.2645995092757,123.117240546905)) ;
#13543=CARTESIAN_POINT('Ctrl Pts',(-20.6137387177837,-13.2665581274631,
123.075575905445)) ;
#13544=CARTESIAN_POINT('Ctrl Pts',(-20.6035597890057,-13.2681895061261,
123.041040791705)) ;
#13545=CARTESIAN_POINT('Ctrl Pts',(-20.591901550154,-13.2698313022358,123.0069836547)) ;
#13546=CARTESIAN_POINT('Ctrl Pts',(-20.5919015501539,-13.2698313022293,
123.006983654699)) ;
#13547=CARTESIAN_POINT('Ctrl Pts',(-20.5758636698524,-13.2720898707903,
122.960132299735)) ;
#13548=CARTESIAN_POINT('Ctrl Pts',(-20.5570558803912,-13.2743709415705,
122.91427657311)) ;
#13549=CARTESIAN_POINT('Ctrl Pts',(-20.5355828802695,-13.2766593340433,
122.86966647846)) ;
#13550=CARTESIAN_POINT('Ctrl Pts',(-20.5040766219917,-13.2800169777764,
122.804212319476)) ;
#13551=CARTESIAN_POINT('Ctrl Pts',(-20.4669292256426,-13.2833316962248,
122.741637162349)) ;
#13552=CARTESIAN_POINT('Ctrl Pts',(-20.4245586326818,-13.2866403923901,
122.68264118227)) ;
#13553=CARTESIAN_POINT('Ctrl Pts',(-20.3821437711191,-13.289952545466,122.623583563461)) ;
#13554=CARTESIAN_POINT('Ctrl Pts',(-20.3346576217278,-13.2932753101363,
122.568340364587)) ;
#13555=CARTESIAN_POINT('Ctrl Pts',(-20.2826406174913,-13.2966313478395,
122.517539425506)) ;
#13556=CARTESIAN_POINT('Ctrl Pts',(-20.2305895807283,-13.2999895812562,
122.466705249518)) ;
#13557=CARTESIAN_POINT('Ctrl Pts',(-20.1742002693491,-13.3033270706483,
122.420512234535)) ;
#13558=CARTESIAN_POINT('Ctrl Pts',(-20.1141057638357,-13.3066289349038,
122.379482201974)) ;
#13559=CARTESIAN_POINT('Ctrl Pts',(-20.0647167286884,-13.3093425921404,
122.345761419966)) ;
#13560=CARTESIAN_POINT('Ctrl Pts',(-20.0129675752083,-13.3120689961557,
122.315625819962)) ;
#13561=CARTESIAN_POINT('Ctrl Pts',(-19.9592567940543,-13.3148330239689,
122.289309584425)) ;
#13562=CARTESIAN_POINT('Ctrl Pts',(-19.9482890254929,-13.3153974398404,
122.283935795875)) ;
#13563=CARTESIAN_POINT('Ctrl Pts',(-19.9372394078935,-13.315962787667,122.278721351692)) ;
#13564=CARTESIAN_POINT('Ctrl Pts',(-19.9261208864848,-13.3165278298207,
122.273672252187)) ;
#13565=CARTESIAN_POINT('Ctrl Pts',(-19.8601614086344,-13.319879883934,122.243718991793)) ;
#13566=CARTESIAN_POINT('Ctrl Pts',(-19.7917288273833,-13.3231893604028,
122.219558406364)) ;
#13567=CARTESIAN_POINT('Ctrl Pts',(-19.7215879104552,-13.3264812840528,
122.201459493175)) ;
#13568=CARTESIAN_POINT('Ctrl Pts',(-19.6513770194176,-13.3297764917976,
122.183342524116)) ;
#13569=CARTESIAN_POINT('Ctrl Pts',(-19.5797249492104,-13.3330861811419,
122.171369594936)) ;
#13570=CARTESIAN_POINT('Ctrl Pts',(-19.5074412538907,-13.3364442850282,
122.165675191354)) ;
#13571=CARTESIAN_POINT('Ctrl Pts',(-19.4349103776582,-13.3398138722674,
122.159961315223)) ;
#13572=CARTESIAN_POINT('Ctrl Pts',(-19.3620201718235,-13.343152644204,122.160590466159)) ;
#13573=CARTESIAN_POINT('Ctrl Pts',(-19.2895944956645,-13.3464412063207,
122.167556660719)) ;
#13574=CARTESIAN_POINT('Ctrl Pts',(-19.217878727295,-13.3496975343459,122.174454573476)) ;
#13575=CARTESIAN_POINT('Ctrl Pts',(-19.1468977227055,-13.3529957519314,
122.187538562837)) ;
#13576=CARTESIAN_POINT('Ctrl Pts',(-19.0774301610563,-13.3563408421583,
122.206666725234)) ;
#13577=CARTESIAN_POINT('Ctrl Pts',(-19.0528841036413,-13.3575228150794,
122.213425577298)) ;
#13578=CARTESIAN_POINT('Ctrl Pts',(-19.0285405414498,-13.3587029390482,
122.220935718747)) ;
#13579=CARTESIAN_POINT('Ctrl Pts',(-19.0044459295036,-13.3598747971121,
122.229183544337)) ;
#13580=CARTESIAN_POINT('Ctrl Pts',(-18.9597352574063,-13.3620493314751,
122.244488452601)) ;
#13581=CARTESIAN_POINT('Ctrl Pts',(-18.9159313512225,-13.3641865237851,
122.262315850384)) ;
#13582=CARTESIAN_POINT('Ctrl Pts',(-18.8732508465882,-13.3663367400634,
122.282575211106)) ;
#13583=CARTESIAN_POINT('Ctrl Pts',(-18.8078025555862,-13.3696339827251,
122.313641866655)) ;
#13584=CARTESIAN_POINT('Ctrl Pts',(-18.7451885059782,-13.3729744547292,
122.350334337807)) ;
#13585=CARTESIAN_POINT('Ctrl Pts',(-18.6861050339502,-13.3762902569431,
122.392241319636)) ;
#13586=CARTESIAN_POINT('Ctrl Pts',(-18.6271390302697,-13.3795994667584,
122.434064983005)) ;
#13587=CARTESIAN_POINT('Ctrl Pts',(-18.5719126530199,-13.3828853672828,
122.480925013947)) ;
#13588=CARTESIAN_POINT('Ctrl Pts',(-18.5210471848208,-13.3862235309958,
122.53229389573)) ;
#13589=CARTESIAN_POINT('Ctrl Pts',(-18.4698550783826,-13.3895831310969,
122.583992648478)) ;
#13590=CARTESIAN_POINT('Ctrl Pts',(-18.4232745350601,-13.3929217653088,
122.640061106466)) ;
#13591=CARTESIAN_POINT('Ctrl Pts',(-18.3818315198481,-13.3962207864909,
122.699869442455)) ;
#13592=CARTESIAN_POINT('Ctrl Pts',(-18.3461290173133,-13.3990628410931,
122.751393378547)) ;
#13593=CARTESIAN_POINT('Ctrl Pts',(-18.3143510291542,-13.4019183731984,
122.805532452684)) ;
#13594=CARTESIAN_POINT('Ctrl Pts',(-18.2867675863735,-13.4048208345985,
122.861829537912)) ;
#13595=CARTESIAN_POINT('Ctrl Pts',(-18.2825046326577,-13.4052694029193,
122.870530114942)) ;
#13596=CARTESIAN_POINT('Ctrl Pts',(-18.2783413961633,-13.4057187472834,
122.879283352965)) ;
#13597=CARTESIAN_POINT('Ctrl Pts',(-18.2742825127642,-13.4061681389656,
122.888079387466)) ;
#13598=CARTESIAN_POINT('Ctrl Pts',(-18.2437967985826,-13.4095434579958,
122.954145191128)) ;
#13599=CARTESIAN_POINT('Ctrl Pts',(-18.2191397332698,-13.4128687018052,
123.02274052249)) ;
#13600=CARTESIAN_POINT('Ctrl Pts',(-18.2005880082575,-13.4161655690401,
123.093094367513)) ;
#13601=CARTESIAN_POINT('Ctrl Pts',(-18.1822228833748,-13.4194292751619,
123.162740567474)) ;
#13602=CARTESIAN_POINT('Ctrl Pts',(-18.1699123138942,-13.4227413347909,
123.233841164989)) ;
#13603=CARTESIAN_POINT('Ctrl Pts',(-18.1637925943239,-13.4260626235858,
123.305604845509)) ;
#13604=CARTESIAN_POINT('Ctrl Pts',(-18.1576328251841,-13.4294056480477,
123.377838172471)) ;
#13605=CARTESIAN_POINT('Ctrl Pts',(-18.1577686102074,-13.4326992417446,
123.450470650516)) ;
#13606=CARTESIAN_POINT('Ctrl Pts',(-18.1641984800143,-13.4360244491812,
123.522680693047)) ;
#13607=CARTESIAN_POINT('Ctrl Pts',(-18.1706556540056,-13.4393637769779,
123.59519737263)) ;
#13608=CARTESIAN_POINT('Ctrl Pts',(-18.1834351267467,-13.4427053334337,
123.667011175704)) ;
#13609=CARTESIAN_POINT('Ctrl Pts',(-18.2023961502137,-13.4460291065788,
123.737314157264)) ;
#13610=CARTESIAN_POINT('Ctrl Pts',(-18.2095965795631,-13.4472913060453,
123.764011642907)) ;
#13611=CARTESIAN_POINT('Ctrl Pts',(-18.2176842050297,-13.4485548533778,
123.790473920422)) ;
#13612=CARTESIAN_POINT('Ctrl Pts',(-18.2266423654683,-13.4498216097391,
123.816643453356)) ;
#13613=CARTESIAN_POINT('',(-20.5919015043581,-13.2097350150005,123.006983520952)) ;
#13614=CARTESIAN_POINT('Ctrl Pts',(-18.2266423654683,-13.389762567023,123.816643453356)) ;
#13615=CARTESIAN_POINT('Ctrl Pts',(-18.2208517141787,-13.3889405101913,
123.799727185706)) ;
#13616=CARTESIAN_POINT('Ctrl Pts',(-18.2154234961749,-13.3881173609619,
123.782684538791)) ;
#13617=CARTESIAN_POINT('Ctrl Pts',(-18.2103653496133,-13.3872939371745,
123.765540642041)) ;
#13618=CARTESIAN_POINT('Ctrl Pts',(-18.1898368125956,-13.3839520637243,
123.695961970329)) ;
#13619=CARTESIAN_POINT('Ctrl Pts',(-18.1754061855548,-13.3806318060667,
123.624737071429)) ;
#13620=CARTESIAN_POINT('Ctrl Pts',(-18.1672328931745,-13.3773259277796,
123.552662764019)) ;
#13621=CARTESIAN_POINT('Ctrl Pts',(-18.1590901255551,-13.3740323959423,
123.480857632224)) ;
#13622=CARTESIAN_POINT('Ctrl Pts',(-18.1571895862557,-13.3707236336382,
123.408482713554)) ;
#13623=CARTESIAN_POINT('Ctrl Pts',(-18.1615522218905,-13.367395382414,123.336350689321)) ;
#13624=CARTESIAN_POINT('Ctrl Pts',(-18.1659397697021,-13.3640481257101,
123.263806765977)) ;
#13625=CARTESIAN_POINT('Ctrl Pts',(-18.1766465054669,-13.3607406977954,
123.191783782171)) ;
#13626=CARTESIAN_POINT('Ctrl Pts',(-18.1935445680407,-13.3574142163685,
123.121114800779)) ;
#13627=CARTESIAN_POINT('Ctrl Pts',(-18.2149719826111,-13.3531961057843,
123.031503725253)) ;
#13628=CARTESIAN_POINT('Ctrl Pts',(-18.2462351295285,-13.3489456270476,
122.944550720865)) ;
#13629=CARTESIAN_POINT('Ctrl Pts',(-18.2867794094466,-13.3447298622308,
122.861805407985)) ;
#13630=CARTESIAN_POINT('Ctrl Pts',(-18.3100370599979,-13.3423115485966,
122.814339734021)) ;
#13631=CARTESIAN_POINT('Ctrl Pts',(-18.3362958328213,-13.3399055899912,
122.768378902966)) ;
#13632=CARTESIAN_POINT('Ctrl Pts',(-18.3653355906569,-13.3374879499868,
122.724285253956)) ;
#13633=CARTESIAN_POINT('Ctrl Pts',(-18.415126928534,-13.333342683659,122.648682633973)) ;
#13634=CARTESIAN_POINT('Ctrl Pts',(-18.4728742233197,-13.3292130717818,
122.578872618133)) ;
#13635=CARTESIAN_POINT('Ctrl Pts',(-18.53750654097,-13.3250805809609,122.515977007929)) ;
#13636=CARTESIAN_POINT('Ctrl Pts',(-18.576278451038,-13.3226015647614,122.478246921323)) ;
#13637=CARTESIAN_POINT('Ctrl Pts',(-18.6175297786796,-13.320121512542,122.443004244074)) ;
#13638=CARTESIAN_POINT('Ctrl Pts',(-18.6610320384471,-13.3176364234057,
122.410496930927)) ;
#13639=CARTESIAN_POINT('Ctrl Pts',(-18.7189857342124,-13.314325788498,122.367190699334)) ;
#13640=CARTESIAN_POINT('Ctrl Pts',(-18.7806663699553,-13.3110019360265,
122.328946485067)) ;
#13641=CARTESIAN_POINT('Ctrl Pts',(-18.8453187237122,-13.307674266914,122.29626228974)) ;
#13642=CARTESIAN_POINT('Ctrl Pts',(-18.8967457914757,-13.3050273058213,
122.270263973667)) ;
#13643=CARTESIAN_POINT('Ctrl Pts',(-18.9499160737166,-13.3023886041235,
122.247849585121)) ;
#13644=CARTESIAN_POINT('Ctrl Pts',(-19.0044473239371,-13.2997505571177,
122.229183067009)) ;
#13645=CARTESIAN_POINT('Ctrl Pts',(-19.0187299939376,-13.2990596073471,
122.224293985663)) ;
#13646=CARTESIAN_POINT('Ctrl Pts',(-19.0331042467207,-13.298368351145,122.219662764486)) ;
#13647=CARTESIAN_POINT('Ctrl Pts',(-19.0475514893392,-13.2976762861676,
122.215295206022)) ;
#13648=CARTESIAN_POINT('Ctrl Pts',(-19.1172019067191,-13.2943398284228,
122.194239127852)) ;
#13649=CARTESIAN_POINT('Ctrl Pts',(-19.1885509316519,-13.2910006049844,
122.179306471)) ;
#13650=CARTESIAN_POINT('Ctrl Pts',(-19.2607930012224,-13.2876772541355,
122.170664127097)) ;
#13651=CARTESIAN_POINT('Ctrl Pts',(-19.3286989617926,-13.2845533772443,
122.162540513421)) ;
#13652=CARTESIAN_POINT('Ctrl Pts',(-19.397150832558,-13.2814420977885,122.160008543899)) ;
#13653=CARTESIAN_POINT('Ctrl Pts',(-19.4653809380022,-13.2783029805218,
122.163074276061)) ;
#13654=CARTESIAN_POINT('Ctrl Pts',(-19.4694620308998,-13.2781152184027,
122.163257648748)) ;
#13655=CARTESIAN_POINT('Ctrl Pts',(-19.4735423315437,-13.277927356689,122.163461032831)) ;
#13656=CARTESIAN_POINT('Ctrl Pts',(-19.4776216758803,-13.2777393867278,
122.163684423755)) ;
#13657=CARTESIAN_POINT('Ctrl Pts',(-19.5670120361899,-13.2736204153501,
122.16857957197)) ;
#13658=CARTESIAN_POINT('Ctrl Pts',(-19.6554229814129,-13.2695312352565,
122.183050310254)) ;
#13659=CARTESIAN_POINT('Ctrl Pts',(-19.7413880498576,-13.2654431054393,
122.206742133779)) ;
#13660=CARTESIAN_POINT('Ctrl Pts',(-19.7949433711462,-13.262896244141,122.22150188729)) ;
#13661=CARTESIAN_POINT('Ctrl Pts',(-19.8475511865818,-13.2603497904714,
122.239841482505)) ;
#13662=CARTESIAN_POINT('Ctrl Pts',(-19.8988539340659,-13.2577967950862,
122.261679695776)) ;
#13663=CARTESIAN_POINT('Ctrl Pts',(-19.9192020596477,-13.2567842046645,
122.27034135091)) ;
#13664=CARTESIAN_POINT('Ctrl Pts',(-19.9393590955496,-13.2557662128757,
122.27956102932)) ;
#13665=CARTESIAN_POINT('Ctrl Pts',(-19.9592313584971,-13.2547486978814,
122.289297122329)) ;
#13666=CARTESIAN_POINT('Ctrl Pts',(-20.0695534587163,-13.2490999002847,
122.343347646492)) ;
#13667=CARTESIAN_POINT('Ctrl Pts',(-20.1712738397568,-13.243529037934,122.413352172863)) ;
#13668=CARTESIAN_POINT('Ctrl Pts',(-20.2611234786059,-13.2378957449231,
122.497019602441)) ;
#13669=CARTESIAN_POINT('Ctrl Pts',(-20.3284914887736,-13.2336719801345,
122.559752278039)) ;
#13670=CARTESIAN_POINT('Ctrl Pts',(-20.3885923439257,-13.2294726355754,
122.629608515275)) ;
#13671=CARTESIAN_POINT('Ctrl Pts',(-20.4404392406267,-13.2252696171872,
122.705277312654)) ;
#13672=CARTESIAN_POINT('Ctrl Pts',(-20.4703608779298,-13.2228439909726,
122.748946933294)) ;
#13673=CARTESIAN_POINT('Ctrl Pts',(-20.4975339476738,-13.2204171411448,
122.794554140896)) ;
#13674=CARTESIAN_POINT('Ctrl Pts',(-20.5217638682247,-13.2179836675985,
122.84184737787)) ;
#13675=CARTESIAN_POINT('Ctrl Pts',(-20.5490412263194,-13.2152441320232,
122.895088764183)) ;
#13676=CARTESIAN_POINT('Ctrl Pts',(-20.5724985243224,-13.2124837581967,
122.950301743001)) ;
#13677=CARTESIAN_POINT('Ctrl Pts',(-20.591901504369,-13.2097350150005,123.006983520948)) ;
#13678=CARTESIAN_POINT('Ctrl Pts',(-20.5919015043689,-13.2097350149936,
123.006983520948)) ;
#13679=CARTESIAN_POINT('Ctrl Pts',(-20.5946210858209,-13.2093497426924,
123.014928213547)) ;
#13680=CARTESIAN_POINT('Ctrl Pts',(-20.5972574366855,-13.2089651469592,
123.022890624025)) ;
#13681=CARTESIAN_POINT('Ctrl Pts',(-20.602492077826,-13.2081779162429,123.039250951045)) ;
#13682=CARTESIAN_POINT('Ctrl Pts',(-20.6050795424771,-13.2077757810124,
123.047641364186)) ;
#13683=CARTESIAN_POINT('Ctrl Pts',(-20.613334929197,-13.2064479730121,123.075448288885)) ;
#13684=CARTESIAN_POINT('Ctrl Pts',(-20.6186199971734,-13.2055234737724,
123.09497512782)) ;
#13685=CARTESIAN_POINT('Ctrl Pts',(-20.6305962877421,-13.2032221981241,
123.143903285706)) ;
#13686=CARTESIAN_POINT('Ctrl Pts',(-20.6367020130782,-13.2018468734285,
123.173434582012)) ;
#13687=CARTESIAN_POINT('Ctrl Pts',(-20.6428457861355,-13.2001628545531,
123.209723679776)) ;
#13688=CARTESIAN_POINT('Ctrl Pts',(-20.6439049388441,-13.1998579709665,
123.216298540924)) ;
#13689=CARTESIAN_POINT('Ctrl Pts',(-20.6458110168909,-13.1992801267645,
123.228764478808)) ;
#13690=CARTESIAN_POINT('Ctrl Pts',(-20.6466685086863,-13.1990072266369,
123.234653755426)) ;
#13691=CARTESIAN_POINT('Ctrl Pts',(-20.6483603441677,-13.1984404431535,
123.246885355422)) ;
#13692=CARTESIAN_POINT('Ctrl Pts',(-20.6491881240791,-13.1981465201376,
123.253228400078)) ;
#13693=CARTESIAN_POINT('Ctrl Pts',(-20.653781363816,-13.1964113876931,123.290662238473)) ;
#13694=CARTESIAN_POINT('Ctrl Pts',(-20.6564259793383,-13.1949632529976,
123.321879200189)) ;
#13695=CARTESIAN_POINT('Ctrl Pts',(-20.6592114629349,-13.1922203625568,
123.381178413588)) ;
#13696=CARTESIAN_POINT('Ctrl Pts',(-20.6595841871457,-13.1909260926596,
123.409230991839)) ;
#13697=CARTESIAN_POINT('Ctrl Pts',(-20.6588665845069,-13.1893054903826,
123.444458217046)) ;
#13698=CARTESIAN_POINT('Ctrl Pts',(-20.6586582324099,-13.188975205851,123.451642612342)) ;
#13699=CARTESIAN_POINT('Ctrl Pts',(-20.6581484001321,-13.1883528058748,
123.465189374786)) ;
#13700=CARTESIAN_POINT('Ctrl Pts',(-20.6578602299974,-13.1880606346941,
123.471552012739)) ;
#13701=CARTESIAN_POINT('Ctrl Pts',(-20.6571614943111,-13.1874549642785,
123.484747572547)) ;
#13702=CARTESIAN_POINT('Ctrl Pts',(-20.6567434041897,-13.1871415129795,
123.491579888144)) ;
#13703=CARTESIAN_POINT('Ctrl Pts',(-20.6556804399702,-13.1864394819941,
123.506887092897)) ;
#13704=CARTESIAN_POINT('Ctrl Pts',(-20.6550052056448,-13.18605107047,123.515359541256)) ;
#13705=CARTESIAN_POINT('Ctrl Pts',(-20.6503822642157,-13.183695725344,123.566742675482)) ;
#13706=CARTESIAN_POINT('Ctrl Pts',(-20.6443042032766,-13.1817414224927,
123.6094325397)) ;
#13707=CARTESIAN_POINT('Ctrl Pts',(-20.63357903935,-13.1792008227938,123.664275109249)) ;
#13708=CARTESIAN_POINT('Ctrl Pts',(-20.6309318665241,-13.1786189595901,
123.67678855567)) ;
#13709=CARTESIAN_POINT('Ctrl Pts',(-20.6253580497198,-13.1774742231183,
123.701274453927)) ;
#13710=CARTESIAN_POINT('Ctrl Pts',(-20.6224454427361,-13.1769115250492,
123.713248633236)) ;
#13711=CARTESIAN_POINT('Ctrl Pts',(-20.616980561564,-13.1759148896647,123.734351818554)) ;
#13712=CARTESIAN_POINT('Ctrl Pts',(-20.6145005965985,-13.1754812589473,
123.743498562509)) ;
#13713=CARTESIAN_POINT('Ctrl Pts',(-20.5961905856121,-13.1724064222122,
123.808112170504)) ;
#13714=CARTESIAN_POINT('Ctrl Pts',(-20.5766418625237,-13.1697622421254,
123.862453108665)) ;
#13715=CARTESIAN_POINT('Ctrl Pts',(-20.5419059478119,-13.1658113150005,
123.941396178308)) ;
#13716=CARTESIAN_POINT('Ctrl Pts',(-20.5295081099116,-13.16450380464,123.967140942648)) ;
#13717=CARTESIAN_POINT('Ctrl Pts',(-20.5100001568819,-13.1625794616165,
124.004333106074)) ;
#13718=CARTESIAN_POINT('Ctrl Pts',(-20.5035698017111,-13.161963806948,124.016126578198)) ;
#13719=CARTESIAN_POINT('Ctrl Pts',(-20.491053121771,-13.1607984553304,124.038227435898)) ;
#13720=CARTESIAN_POINT('Ctrl Pts',(-20.4850063703509,-13.1602489441725,
124.048555514217)) ;
#13721=CARTESIAN_POINT('Ctrl Pts',(-20.4713014719199,-13.1590313997102,
124.071211423003)) ;
#13722=CARTESIAN_POINT('Ctrl Pts',(-20.463575087642,-13.1583630165779,124.083495891202)) ;
#13723=CARTESIAN_POINT('Ctrl Pts',(-20.4350794840134,-13.1559581988703,
124.127098600494)) ;
#13724=CARTESIAN_POINT('Ctrl Pts',(-20.413114441118,-13.1542165471007,124.157611174154)) ;
#13725=CARTESIAN_POINT('Ctrl Pts',(-20.3815599326205,-13.1518662655605,
124.197520101744)) ;
#13726=CARTESIAN_POINT('Ctrl Pts',(-20.3731455648034,-13.1512526701005,
124.207820067248)) ;
#13727=CARTESIAN_POINT('Ctrl Pts',(-20.3594754546815,-13.1502763347377,
124.224018899634)) ;
#13728=CARTESIAN_POINT('Ctrl Pts',(-20.3543254046035,-13.149912962448,124.230005584681)) ;
#13729=CARTESIAN_POINT('Ctrl Pts',(-20.3451672504657,-13.1492744825268,
124.240449658568)) ;
#13730=CARTESIAN_POINT('Ctrl Pts',(-20.3411831712019,-13.1489992156631,
124.244927764828)) ;
#13731=CARTESIAN_POINT('Ctrl Pts',(-20.3331605812835,-13.1484498174186,
124.253815600412)) ;
#13732=CARTESIAN_POINT('Ctrl Pts',(-20.3291223287344,-13.1481756919887,
124.258225353916)) ;
#13733=CARTESIAN_POINT('Ctrl Pts',(-20.3209595124054,-13.1476263432251,
124.267011696828)) ;
#13734=CARTESIAN_POINT('Ctrl Pts',(-20.3168346933931,-13.1473511297979,
124.271387836283)) ;
#13735=CARTESIAN_POINT('Ctrl Pts',(-20.3049913677881,-13.1465675658135,
124.283772475927)) ;
#13736=CARTESIAN_POINT('Ctrl Pts',(-20.2971973189354,-13.1460598190212,
124.291707971596)) ;
#13737=CARTESIAN_POINT('Ctrl Pts',(-20.2580438929012,-13.1435464495336,
124.330521878437)) ;
#13738=CARTESIAN_POINT('Ctrl Pts',(-20.2251749613224,-13.1415542245009,
124.359833128599)) ;
#13739=CARTESIAN_POINT('Ctrl Pts',(-20.1803738382925,-13.1389463361932,
124.395725837094)) ;
#13740=CARTESIAN_POINT('Ctrl Pts',(-20.1697850111937,-13.1383370517942,
124.403933200245)) ;
#13741=CARTESIAN_POINT('Ctrl Pts',(-20.1493832669874,-13.1371747867644,
124.419227945175)) ;
#13742=CARTESIAN_POINT('Ctrl Pts',(-20.1395953499515,-13.1366222814638,
124.426346083255)) ;
#13743=CARTESIAN_POINT('Ctrl Pts',(-20.1265156477306,-13.1358907642432,
124.435570746782)) ;
#13744=CARTESIAN_POINT('Ctrl Pts',(-20.1233151274146,-13.1357122956839,
124.437805588207)) ;
#13745=CARTESIAN_POINT('Ctrl Pts',(-20.1013867319363,-13.1344931300381,
124.452965320774)) ;
#13746=CARTESIAN_POINT('Ctrl Pts',(-20.0823194569265,-13.1334510254705,
124.465391710472)) ;
#13747=CARTESIAN_POINT('Ctrl Pts',(-20.0256225069944,-13.1304035066777,
124.500174317462)) ;
#13748=CARTESIAN_POINT('Ctrl Pts',(-19.9871453231867,-13.128399731876,124.521083377027)) ;
#13749=CARTESIAN_POINT('Ctrl Pts',(-19.9288247336841,-13.1254399836714,
124.548916102886)) ;
#13750=CARTESIAN_POINT('Ctrl Pts',(-19.9097764052515,-13.1244847172175,
124.557428058674)) ;
#13751=CARTESIAN_POINT('Ctrl Pts',(-19.8767869505092,-13.1228462004059,
124.571189861526)) ;
#13752=CARTESIAN_POINT('Ctrl Pts',(-19.8629486302767,-13.1221635391203,
124.576674561629)) ;
#13753=CARTESIAN_POINT('Ctrl Pts',(-19.8388027008165,-13.1209788264789,
124.585749039904)) ;
#13754=CARTESIAN_POINT('Ctrl Pts',(-19.828539909192,-13.1204772644073,124.589453383613)) ;
#13755=CARTESIAN_POINT('Ctrl Pts',(-19.8038969018518,-13.1192766497714,
124.597985279752)) ;
#13756=CARTESIAN_POINT('Ctrl Pts',(-19.789474816449,-13.1185769195871,124.602686339933)) ;
#13757=CARTESIAN_POINT('Ctrl Pts',(-19.7552307062143,-13.1169201861169,
124.613163141805)) ;
#13758=CARTESIAN_POINT('Ctrl Pts',(-19.7353441433544,-13.1159624063868,
124.618712560235)) ;
#13759=CARTESIAN_POINT('Ctrl Pts',(-19.6919784186862,-13.1138875783725,
124.629663804484)) ;
#13760=CARTESIAN_POINT('Ctrl Pts',(-19.6684618344387,-13.1127710659302,
124.634884602325)) ;
#13761=CARTESIAN_POINT('Ctrl Pts',(-19.6344197839601,-13.1111691733207,
124.641416128066)) ;
#13762=CARTESIAN_POINT('Ctrl Pts',(-19.6240056038621,-13.1106810061279,
124.643277517649)) ;
#13763=CARTESIAN_POINT('Ctrl Pts',(-19.6072053451249,-13.10989650755,124.646060732617)) ;
#13764=CARTESIAN_POINT('Ctrl Pts',(-19.6008335936111,-13.1095996685999,
124.647065699069)) ;
#13765=CARTESIAN_POINT('Ctrl Pts',(-19.5895980975686,-13.1090774373909,
124.64874876092)) ;
#13766=CARTESIAN_POINT('Ctrl Pts',(-19.5847376076761,-13.1088519115615,
124.649447598103)) ;
#13767=CARTESIAN_POINT('Ctrl Pts',(-19.5750788573241,-13.1084045034829,
124.650778282738)) ;
#13768=CARTESIAN_POINT('Ctrl Pts',(-19.5702807933502,-13.1081826194189,
124.651410940409)) ;
#13769=CARTESIAN_POINT('Ctrl Pts',(-19.5600063967649,-13.1077082457941,
124.652705030246)) ;
#13770=CARTESIAN_POINT('Ctrl Pts',(-19.5545291121831,-13.1074558186349,
124.653358109896)) ;
#13771=CARTESIAN_POINT('Ctrl Pts',(-19.5398903818906,-13.1067823384053,
124.655005348596)) ;
#13772=CARTESIAN_POINT('Ctrl Pts',(-19.5307219475339,-13.1063617454783,
124.655934492005)) ;
#13773=CARTESIAN_POINT('Ctrl Pts',(-19.4825436801578,-13.1041571812783,
124.66027930177)) ;
#13774=CARTESIAN_POINT('Ctrl Pts',(-19.443399469158,-13.1023862276664,124.661961864056)) ;
#13775=CARTESIAN_POINT('Ctrl Pts',(-19.3809520941096,-13.0995603406129,
124.661710497427)) ;
#13776=CARTESIAN_POINT('Ctrl Pts',(-19.3576708227804,-13.0985059328195,
124.6609659417)) ;
#13777=CARTESIAN_POINT('Ctrl Pts',(-19.317738254551,-13.0966872479062,124.658570534926)) ;
#13778=CARTESIAN_POINT('Ctrl Pts',(-19.3010744125512,-13.0959257543479,
124.657235034425)) ;
#13779=CARTESIAN_POINT('Ctrl Pts',(-19.2699653508192,-13.0944991984778,
124.654112756357)) ;
#13780=CARTESIAN_POINT('Ctrl Pts',(-19.2555147613564,-13.0938345314503,
124.65240710177)) ;
#13781=CARTESIAN_POINT('Ctrl Pts',(-19.2389782275323,-13.0930714487792,
124.650161863816)) ;
#13782=CARTESIAN_POINT('Ctrl Pts',(-19.2368599137098,-13.092973651853,124.649868712862)) ;
#13783=CARTESIAN_POINT('Ctrl Pts',(-19.2141324810124,-13.0919238780786,
124.646664028981)) ;
#13784=CARTESIAN_POINT('Ctrl Pts',(-19.1935984356369,-13.0909709543967,
124.643243626117)) ;
#13785=CARTESIAN_POINT('Ctrl Pts',(-19.144258780188,-13.0886686890323,124.633752998499)) ;
#13786=CARTESIAN_POINT('Ctrl Pts',(-19.1155635138413,-13.0873193296974,
124.627174943626)) ;
#13787=CARTESIAN_POINT('Ctrl Pts',(-19.0594368525581,-13.0846530206157,
124.612204517602)) ;
#13788=CARTESIAN_POINT('Ctrl Pts',(-19.0320086602249,-13.0833369254941,
124.603868684193)) ;
#13789=CARTESIAN_POINT('Ctrl Pts',(-18.953680150316,-13.0795281393135,124.577089007611)) ;
#13790=CARTESIAN_POINT('Ctrl Pts',(-18.9036603400733,-13.0770249750502,
124.556273038884)) ;
#13791=CARTESIAN_POINT('Ctrl Pts',(-18.8412132313845,-13.0738048888424,
124.525389976062)) ;
#13792=CARTESIAN_POINT('Ctrl Pts',(-18.8274081499145,-13.0730872103483,
124.518239176167)) ;
#13793=CARTESIAN_POINT('Ctrl Pts',(-18.8060922881046,-13.071970005057,124.506688611288)) ;
#13794=CARTESIAN_POINT('Ctrl Pts',(-18.7984880245361,-13.0715696063642,
124.502464772995)) ;
#13795=CARTESIAN_POINT('Ctrl Pts',(-18.7854343560365,-13.0708790061069,
124.495034687726)) ;
#13796=CARTESIAN_POINT('Ctrl Pts',(-18.7799640546951,-13.0705885959289,
124.491865836585)) ;
#13797=CARTESIAN_POINT('Ctrl Pts',(-18.7693926914893,-13.0700253691977,
124.485634446979)) ;
#13798=CARTESIAN_POINT('Ctrl Pts',(-18.7642889911474,-13.0697525308087,
124.482576716805)) ;
#13799=CARTESIAN_POINT('Ctrl Pts',(-18.7541541620249,-13.0692088333995,
124.47640598287)) ;
#13800=CARTESIAN_POINT('Ctrl Pts',(-18.7491229150831,-13.068937978748,124.473293464187)) ;
#13801=CARTESIAN_POINT('Ctrl Pts',(-18.7370780491303,-13.0682871807584,
124.465723296967)) ;
#13802=CARTESIAN_POINT('Ctrl Pts',(-18.7300864096677,-13.067907463319,124.46123119146)) ;
#13803=CARTESIAN_POINT('Ctrl Pts',(-18.694373230457,-13.0659571651033,124.437779178113)) ;
#13804=CARTESIAN_POINT('Ctrl Pts',(-18.6663987396338,-13.064394117346,124.417708678766)) ;
#13805=CARTESIAN_POINT('Ctrl Pts',(-18.6266587834868,-13.0621010006204,
124.386633943294)) ;
#13806=CARTESIAN_POINT('Ctrl Pts',(-18.6142207163909,-13.0613720753055,
124.37651644575)) ;
#13807=CARTESIAN_POINT('Ctrl Pts',(-18.5967015051739,-13.0603263955924,
124.361696791309)) ;
#13808=CARTESIAN_POINT('Ctrl Pts',(-18.5914594271576,-13.0600109980012,
124.357187320837)) ;
#13809=CARTESIAN_POINT('Ctrl Pts',(-18.5830978895291,-13.0595035800914,
124.349872757504)) ;
#13810=CARTESIAN_POINT('Ctrl Pts',(-18.5799546578483,-13.0593118338709,
124.347095046369)) ;
#13811=CARTESIAN_POINT('Ctrl Pts',(-18.5768123715238,-13.0591190969748,
124.344289875357)) ;
#13812=CARTESIAN_POINT('Ctrl Pts',(-18.5767992702655,-13.0591182933709,
124.344278179151)) ;
#13813=CARTESIAN_POINT('Ctrl Pts',(-18.5767732091918,-13.0591166948023,
124.344254912025)) ;
#13814=CARTESIAN_POINT('Ctrl Pts',(-18.5767602506733,-13.0591158999176,
124.344243342274)) ;
#13815=CARTESIAN_POINT('Ctrl Pts',(-18.5767344749876,-13.0591143187829,
124.344220328009)) ;
#13816=CARTESIAN_POINT('Ctrl Pts',(-18.5767216563103,-13.0591135324407,
124.344208882157)) ;
#13817=CARTESIAN_POINT('Ctrl Pts',(-18.5766961578895,-13.0591119682439,
124.344186113563)) ;
#13818=CARTESIAN_POINT('Ctrl Pts',(-18.5766834791831,-13.0591111904534,
124.344174791756)) ;
#13819=CARTESIAN_POINT('Ctrl Pts',(-18.576658259452,-13.0591096432842,124.344152270166)) ;
#13820=CARTESIAN_POINT('Ctrl Pts',(-18.576645717573,-13.0591088738536,124.344141069629)) ;
#13821=CARTESIAN_POINT('Ctrl Pts',(-18.5766207697322,-13.0591073432972,
124.344118789032)) ;
#13822=CARTESIAN_POINT('Ctrl Pts',(-18.5766083640755,-13.0591065821904,
124.344107709253)) ;
#13823=CARTESIAN_POINT('Ctrl Pts',(-18.5765836873645,-13.0591050682022,
124.344085669027)) ;
#13824=CARTESIAN_POINT('Ctrl Pts',(-18.5765714155829,-13.0591043152765,
124.34407470794)) ;
#13825=CARTESIAN_POINT('Ctrl Pts',(-18.5765470045118,-13.0591028175217,
124.344052903239)) ;
#13826=CARTESIAN_POINT('Ctrl Pts',(-18.5765348657958,-13.0591020727283,
124.344042060148)) ;
#13827=CARTESIAN_POINT('Ctrl Pts',(-18.5765107189499,-13.0591005911224,
124.344020489765)) ;
#13828=CARTESIAN_POINT('Ctrl Pts',(-18.5764987112384,-13.0590998543358,
124.344009762857)) ;
#13829=CARTESIAN_POINT('Ctrl Pts',(-18.5764748252108,-13.0590983886716,
124.343988423804)) ;
#13830=CARTESIAN_POINT('Ctrl Pts',(-18.5764629468541,-13.0590976597918,
124.343977811631)) ;
#13831=CARTESIAN_POINT('Ctrl Pts',(-18.5764393187023,-13.0590962098908,
124.343956701333)) ;
#13832=CARTESIAN_POINT('Ctrl Pts',(-18.5764275680372,-13.0590954888165,
124.343946202437)) ;
#13833=CARTESIAN_POINT('Ctrl Pts',(-18.5764041926353,-13.0590940543661,
124.343925316365)) ;
#13834=CARTESIAN_POINT('Ctrl Pts',(-18.576392569134,-13.059093341066,124.343914930301)) ;
#13835=CARTESIAN_POINT('Ctrl Pts',(-18.5763694473039,-13.0590919221184,
124.343894269241)) ;
#13836=CARTESIAN_POINT('Ctrl Pts',(-18.5763579480308,-13.0590912164133,
124.34388399341)) ;
#13837=CARTESIAN_POINT('Ctrl Pts',(-18.5763350733448,-13.059089812576,124.343863551669)) ;
#13838=CARTESIAN_POINT('Ctrl Pts',(-18.576323697843,-13.0590891144387,124.343853385688)) ;
#13839=CARTESIAN_POINT('Ctrl Pts',(-18.5763010687545,-13.0590877256186,
124.343833161932)) ;
#13840=CARTESIAN_POINT('Ctrl Pts',(-18.576289815373,-13.0590870349487,124.343823104349)) ;
#13841=CARTESIAN_POINT('Ctrl Pts',(-18.5762674290795,-13.0590856609755,
124.343803096123)) ;
#13842=CARTESIAN_POINT('Ctrl Pts',(-18.5762562962323,-13.0590849776765,
124.343793145545)) ;
#13843=CARTESIAN_POINT('Ctrl Pts',(-18.5762341500843,-13.0590836183894,
124.343773350525)) ;
#13844=CARTESIAN_POINT('Ctrl Pts',(-18.5762231361601,-13.0590829423633,
124.343763505535)) ;
#13845=CARTESIAN_POINT('Ctrl Pts',(-18.5762012266255,-13.0590815975472,
124.343743920612)) ;
#13846=CARTESIAN_POINT('Ctrl Pts',(-18.5761903304785,-13.0590809287245,
124.343734180207)) ;
#13847=CARTESIAN_POINT('Ctrl Pts',(-18.5761686531521,-13.0590795981106,
124.343714801487)) ;
#13848=CARTESIAN_POINT('Ctrl Pts',(-18.5761578743407,-13.059078936465,124.343705165295)) ;
#13849=CARTESIAN_POINT('Ctrl Pts',(-18.5761364315411,-13.0590776201972,
124.343685994895)) ;
#13850=CARTESIAN_POINT('Ctrl Pts',(-18.5761257665994,-13.0590769655168,
124.34367645984)) ;
#13851=CARTESIAN_POINT('Ctrl Pts',(-18.5761045512553,-13.0590756631627,
124.343657491479)) ;
#13852=CARTESIAN_POINT('Ctrl Pts',(-18.5760939999669,-13.0590750154349,
124.343648057388)) ;
#13853=CARTESIAN_POINT('Ctrl Pts',(-18.5760730092267,-13.059073726821,124.34362928856)) ;
#13854=CARTESIAN_POINT('Ctrl Pts',(-18.5760625709037,-13.0590730860044,
124.343619954839)) ;
#13855=CARTESIAN_POINT('Ctrl Pts',(-18.5760418048441,-13.0590718111368,
124.343601385653)) ;
#13856=CARTESIAN_POINT('Ctrl Pts',(-18.5760314771134,-13.0590711770864,
124.343592150199)) ;
#13857=CARTESIAN_POINT('Ctrl Pts',(-18.576010931704,-13.0590699157193,124.343573777091)) ;
#13858=CARTESIAN_POINT('Ctrl Pts',(-18.5760007134305,-13.0590692883663,
124.34356463891)) ;
#13859=CARTESIAN_POINT('Ctrl Pts',(-18.5759803855166,-13.0590680403073,
124.343546459097)) ;
#13860=CARTESIAN_POINT('Ctrl Pts',(-18.5759702757845,-13.059067419596,124.343537417389)) ;
#13861=CARTESIAN_POINT('Ctrl Pts',(-18.5759501627788,-13.0590661846879,
124.343519428596)) ;
#13862=CARTESIAN_POINT('Ctrl Pts',(-18.5759401605112,-13.0590655705529,
124.343510482417)) ;
#13863=CARTESIAN_POINT('Ctrl Pts',(-18.5759202621729,-13.0590643487821,
124.343492684466)) ;
#13864=CARTESIAN_POINT('Ctrl Pts',(-18.5759103650519,-13.0590637410819,
124.343483831761)) ;
#13865=CARTESIAN_POINT('Ctrl Pts',(-18.5758906753213,-13.0590625320777,
124.343466219268)) ;
#13866=CARTESIAN_POINT('Ctrl Pts',(-18.5758808833601,-13.0590619308138,
124.343457460067)) ;
#13867=CARTESIAN_POINT('Ctrl Pts',(-18.5758614032091,-13.0590607346372,
124.343440033938)) ;
#13868=CARTESIAN_POINT('Ctrl Pts',(-18.5758517140855,-13.0590601396675,
124.343431366181)) ;
#13869=CARTESIAN_POINT('Ctrl Pts',(-18.5758324379853,-13.0590589559804,
124.343414121504)) ;
#13870=CARTESIAN_POINT('Ctrl Pts',(-18.5758228514831,-13.0590583672923,
124.343405545015)) ;
#13871=CARTESIAN_POINT('Ctrl Pts',(-18.5758037792065,-13.059057196082,124.343388481622)) ;
#13872=CARTESIAN_POINT('Ctrl Pts',(-18.5757942935344,-13.0590566135662,
124.343379994815)) ;
#13873=CARTESIAN_POINT('Ctrl Pts',(-18.5757754224789,-13.059055454674,124.343363110411)) ;
#13874=CARTESIAN_POINT('Ctrl Pts',(-18.5757660362585,-13.0590548782464,
124.34335471207)) ;
#13875=CARTESIAN_POINT('Ctrl Pts',(-18.5757473631504,-13.0590537314726,
124.343338003758)) ;
#13876=CARTESIAN_POINT('Ctrl Pts',(-18.5757380755909,-13.0590531610852,
124.343329693191)) ;
#13877=CARTESIAN_POINT('Ctrl Pts',(-18.575719596903,-13.0590520262143,124.343313157847)) ;
#13878=CARTESIAN_POINT('Ctrl Pts',(-18.5757104076385,-13.0590514618454,
124.343304934742)) ;
#13879=CARTESIAN_POINT('Ctrl Pts',(-18.5756921253583,-13.0590503390006,
124.343288574176)) ;
#13880=CARTESIAN_POINT('Ctrl Pts',(-18.5756830314898,-13.0590497804725,
124.343280435955)) ;
#13881=CARTESIAN_POINT('Ctrl Pts',(-18.575664938979,-13.0590486692473,124.343264244256)) ;
#13882=CARTESIAN_POINT('Ctrl Pts',(-18.575655940697,-13.0590481165724,124.343256191106)) ;
#13883=CARTESIAN_POINT('Ctrl Pts',(-18.5756380379289,-13.0590470169662,
124.343240168281)) ;
#13884=CARTESIAN_POINT('Ctrl Pts',(-18.5756291336696,-13.059046470049,124.343232198814)) ;
#13885=CARTESIAN_POINT('Ctrl Pts',(-18.5756114182638,-13.0590453819167,
124.343216342762)) ;
#13886=CARTESIAN_POINT('Ctrl Pts',(-18.5756026067899,-13.0590448406817,
124.343208455888)) ;
#13887=CARTESIAN_POINT('Ctrl Pts',(-18.5755850758316,-13.0590437638453,
124.343192764027)) ;
#13888=CARTESIAN_POINT('Ctrl Pts',(-18.575576356355,-13.0590432282446,124.343184959053)) ;
#13889=CARTESIAN_POINT('Ctrl Pts',(-18.5755590078182,-13.0590421625808,
124.3431694296)) ;
#13890=CARTESIAN_POINT('Ctrl Pts',(-18.5755503793518,-13.0590416325543,
124.343161705657)) ;
#13891=CARTESIAN_POINT('Ctrl Pts',(-18.5755332122344,-13.0590405780024,
124.343146337741)) ;
#13892=CARTESIAN_POINT('Ctrl Pts',(-18.5755246731923,-13.0590400534532,
124.343138693422)) ;
#13893=CARTESIAN_POINT('Ctrl Pts',(-18.5755076844,-13.0590390098243,124.3431234843)) ;
#13894=CARTESIAN_POINT('Ctrl Pts',(-18.5754992339722,-13.0590384907031,
124.343115918894)) ;
#13895=CARTESIAN_POINT('Ctrl Pts',(-18.5754824207663,-13.0590374578298,
124.34310086614)) ;
#13896=CARTESIAN_POINT('Ctrl Pts',(-18.5754740583669,-13.0590369441011,
124.343093379135)) ;
#13897=CARTESIAN_POINT('Ctrl Pts',(-18.5754574204807,-13.059035921968,124.343078482537)) ;
#13898=CARTESIAN_POINT('Ctrl Pts',(-18.5754491444293,-13.059035413529,124.343071072441)) ;
#13899=CARTESIAN_POINT('Ctrl Pts',(-18.575432677479,-13.0590344018677,124.343056328097)) ;
#13900=CARTESIAN_POINT('Ctrl Pts',(-18.5754244876065,-13.0590338987086,
124.343048994772)) ;
#13901=CARTESIAN_POINT('Ctrl Pts',(-18.5754081929116,-13.0590328976011,
124.34303440389)) ;
#13902=CARTESIAN_POINT('Ctrl Pts',(-18.5754000869874,-13.0590323995852,
124.34302714535)) ;
#13903=CARTESIAN_POINT('Ctrl Pts',(-18.5753839586784,-13.0590314086717,
124.343012702696)) ;
#13904=CARTESIAN_POINT('Ctrl Pts',(-18.5753759370461,-13.0590309158206,
124.343005519261)) ;
#13905=CARTESIAN_POINT('Ctrl Pts',(-18.5753599752291,-13.0590299351086,
124.342991224955)) ;
#13906=CARTESIAN_POINT('Ctrl Pts',(-18.5753520365623,-13.0590294473412,
124.342984115449)) ;
#13907=CARTESIAN_POINT('Ctrl Pts',(-18.5753362416015,-13.0590284768539,
124.34296996984)) ;
#13908=CARTESIAN_POINT('Ctrl Pts',(-18.5753283835982,-13.0590279940291,
124.342962932211)) ;
#13909=CARTESIAN_POINT('Ctrl Pts',(-18.5753127493683,-13.059027033391,124.342948929836)) ;
#13910=CARTESIAN_POINT('Ctrl Pts',(-18.5753049725399,-13.0590265555408,
124.342941964555)) ;
#13911=CARTESIAN_POINT('Ctrl Pts',(-18.5752894984523,-13.0590256047165,
124.342928104908)) ;
#13912=CARTESIAN_POINT('Ctrl Pts',(-18.5752818019414,-13.0590251317886,
124.342921211217)) ;
#13913=CARTESIAN_POINT('Ctrl Pts',(-18.5752664864524,-13.059024190684,124.342907492938)) ;
#13914=CARTESIAN_POINT('Ctrl Pts',(-18.5752588692233,-13.0590237226151,
124.34290066992)) ;
#13915=CARTESIAN_POINT('Ctrl Pts',(-18.5752437133664,-13.0590227912946,
124.342887093954)) ;
#13916=CARTESIAN_POINT('Ctrl Pts',(-18.5752361730028,-13.0590223279366,
124.342880339456)) ;
#13917=CARTESIAN_POINT('Ctrl Pts',(-18.5752211686278,-13.0590214059001,
124.342866898524)) ;
#13918=CARTESIAN_POINT('Ctrl Pts',(-18.5752137066611,-13.0590209473474,
124.342860213927)) ;
#13919=CARTESIAN_POINT('Ctrl Pts',(-18.5751988595061,-13.0590200349483,
124.34284691319)) ;
#13920=CARTESIAN_POINT('Ctrl Pts',(-18.5751914724873,-13.0590195809894,
124.342840295414)) ;
#13921=CARTESIAN_POINT('Ctrl Pts',(-18.5751743963632,-13.0590185315866,
124.342824997135)) ;
#13922=CARTESIAN_POINT('Ctrl Pts',(-18.5751647058763,-13.0590179360534,
124.342816315281)) ;
#13923=CARTESIAN_POINT('Ctrl Pts',(-18.5727867012847,-13.0588717922316,
124.340685757895)) ;
#13924=CARTESIAN_POINT('Ctrl Pts',(-18.570426495529,-13.058726134459,124.338554856162)) ;
#13925=CARTESIAN_POINT('Ctrl Pts',(-18.5653873125959,-13.0584138015554,
124.333970228496)) ;
#13926=CARTESIAN_POINT('Ctrl Pts',(-18.5627108508765,-13.0582470915148,
124.33151378418)) ;
#13927=CARTESIAN_POINT('Ctrl Pts',(-18.5555039436618,-13.0577960020574,
124.324841202711)) ;
#13928=CARTESIAN_POINT('Ctrl Pts',(-18.5509940454421,-13.0575113625089,
124.320603037122)) ;
#13929=CARTESIAN_POINT('Ctrl Pts',(-18.5316298472319,-13.0562792074135,
124.302132867345)) ;
#13930=CARTESIAN_POINT('Ctrl Pts',(-18.5170967093551,-13.0553288007821,
124.287568908927)) ;
#13931=CARTESIAN_POINT('Ctrl Pts',(-18.4898906137748,-13.0535026066794,
124.258924699829)) ;
#13932=CARTESIAN_POINT('Ctrl Pts',(-18.4771651237092,-13.0526271265878,
124.244901887226)) ;
#13933=CARTESIAN_POINT('Ctrl Pts',(-18.4556659984273,-13.0511114655823,
124.220101459081)) ;
#13934=CARTESIAN_POINT('Ctrl Pts',(-18.4467444256926,-13.0504708434954,
124.209456577654)) ;
#13935=CARTESIAN_POINT('Ctrl Pts',(-18.4328952238659,-13.0494576288438,
124.192361448839)) ;
#13936=CARTESIAN_POINT('Ctrl Pts',(-18.4278498610943,-13.0490843801677,
124.186008102062)) ;
#13937=CARTESIAN_POINT('Ctrl Pts',(-18.419089738285,-13.0484289370592,124.174753703802)) ;
#13938=CARTESIAN_POINT('Ctrl Pts',(-18.415348631302,-13.0481465799679,124.169873519523)) ;
#13939=CARTESIAN_POINT('Ctrl Pts',(-18.4079182472009,-13.0475807947028,
124.160031193206)) ;
#13940=CARTESIAN_POINT('Ctrl Pts',(-18.4042294733846,-13.047297377047,124.155068882968)) ;
#13941=CARTESIAN_POINT('Ctrl Pts',(-18.3963653755716,-13.0466875849945,
124.144324133538)) ;
#13942=CARTESIAN_POINT('Ctrl Pts',(-18.3922024130721,-13.0463613052809,
124.138532910668)) ;
#13943=CARTESIAN_POINT('Ctrl Pts',(-18.3808185455468,-13.0454591844857,
124.122407038763)) ;
#13944=CARTESIAN_POINT('Ctrl Pts',(-18.3737040640521,-13.0448841010443,
124.111998272898)) ;
#13945=CARTESIAN_POINT('Ctrl Pts',(-18.3359168734013,-13.0417647713829,
124.054878062883)) ;
#13946=CARTESIAN_POINT('Ctrl Pts',(-18.308245391511,-13.0392411246978,124.006257445023)) ;
#13947=CARTESIAN_POINT('Ctrl Pts',(-18.2700598212074,-13.0352529346555,
123.927283913443)) ;
#13948=CARTESIAN_POINT('Ctrl Pts',(-18.2572999984862,-13.0338033535924,
123.898100013226)) ;
#13949=CARTESIAN_POINT('Ctrl Pts',(-18.2389457281613,-13.0315116611717,
123.851330589327)) ;
#13950=CARTESIAN_POINT('Ctrl Pts',(-18.2326021688887,-13.0306716162552,
123.834053866237)) ;
#13951=CARTESIAN_POINT('Ctrl Pts',(-18.2266423654684,-13.0298305431221,
123.816643453356)) ;
#13952=CARTESIAN_POINT('Origin',(-19.4092722359532,-13.9601742359176,123.411814366564)) ;
#13953=CARTESIAN_POINT('',(-18.2266423654694,-12.6697781342469,123.816643453359)) ;
#13954=CARTESIAN_POINT('',(-18.2266423654683,-12.7298216458232,123.816643453356)) ;
#13955=CARTESIAN_POINT('',(-18.2266423654683,-13.9601742359176,123.816643453356)) ;
#13956=CARTESIAN_POINT('',(-20.591901275917,-12.9098928303878,123.006982853621)) ;
#13957=CARTESIAN_POINT('Ctrl Pts',(-18.2266423654683,-12.7298216458232,
123.816643453356)) ;
#13958=CARTESIAN_POINT('Ctrl Pts',(-18.2326017142761,-12.7306672894293,
123.834052538174)) ;
#13959=CARTESIAN_POINT('Ctrl Pts',(-18.2389447360747,-12.7315136846607,
123.851327882605)) ;
#13960=CARTESIAN_POINT('Ctrl Pts',(-18.2572979468201,-12.7338268239059,
123.898095094483)) ;
#13961=CARTESIAN_POINT('Ctrl Pts',(-18.2700571991135,-12.735294271902,123.927278037118)) ;
#13962=CARTESIAN_POINT('Ctrl Pts',(-18.3082398863143,-12.7393454067758,
124.006246855078)) ;
#13963=CARTESIAN_POINT('Ctrl Pts',(-18.3359088431132,-12.7419370427707,
124.054864332949)) ;
#13964=CARTESIAN_POINT('Ctrl Pts',(-18.3736951240226,-12.7450944938988,
124.11198511765)) ;
#13965=CARTESIAN_POINT('Ctrl Pts',(-18.3808116436384,-12.7456749550272,
124.122397118766)) ;
#13966=CARTESIAN_POINT('Ctrl Pts',(-18.3921980634869,-12.7465821741772,
124.138526830088)) ;
#13967=CARTESIAN_POINT('Ctrl Pts',(-18.3963614188763,-12.7469095920066,
124.144318669634)) ;
#13968=CARTESIAN_POINT('Ctrl Pts',(-18.4042261169505,-12.7475202460246,
124.155064347167)) ;
#13969=CARTESIAN_POINT('Ctrl Pts',(-18.4079150871526,-12.747803554078,124.16002696724)) ;
#13970=CARTESIAN_POINT('Ctrl Pts',(-18.4153454927312,-12.7483681106648,
124.169869402047)) ;
#13971=CARTESIAN_POINT('Ctrl Pts',(-18.4190864161334,-12.7486493541137,
124.174749390141)) ;
#13972=CARTESIAN_POINT('Ctrl Pts',(-18.4278457554633,-12.7493011211007,
124.18600288753)) ;
#13973=CARTESIAN_POINT('Ctrl Pts',(-18.4328905146027,-12.7496714656466,
124.192355548919)) ;
#13974=CARTESIAN_POINT('Ctrl Pts',(-18.4467372532608,-12.7506748463988,
124.209447872826)) ;
#13975=CARTESIAN_POINT('Ctrl Pts',(-18.4556569326463,-12.7513071671426,
124.220090716886)) ;
#13976=CARTESIAN_POINT('Ctrl Pts',(-18.4771552127671,-12.7528005044379,
124.244890841725)) ;
#13977=CARTESIAN_POINT('Ctrl Pts',(-18.4898818553188,-12.7536608358596,
124.258915238493)) ;
#13978=CARTESIAN_POINT('Ctrl Pts',(-18.5170916260033,-12.7554572386405,
124.287563817407)) ;
#13979=CARTESIAN_POINT('Ctrl Pts',(-18.5316272030638,-12.7563931326534,
124.302130338426)) ;
#13980=CARTESIAN_POINT('Ctrl Pts',(-18.5509938955987,-12.7576151635076,
124.320602896252)) ;
#13981=CARTESIAN_POINT('Ctrl Pts',(-18.5555038384293,-12.7578980523225,
124.324841104505)) ;
#13982=CARTESIAN_POINT('Ctrl Pts',(-18.5627107845363,-12.7583476484,124.331513723214)) ;
#13983=CARTESIAN_POINT('Ctrl Pts',(-18.5653872543757,-12.758514085372,124.333970175208)) ;
#13984=CARTESIAN_POINT('Ctrl Pts',(-18.5704264469513,-12.7588265050528,
124.338554812247)) ;
#13985=CARTESIAN_POINT('Ctrl Pts',(-18.5727866565771,-12.7589724502519,
124.340685717616)) ;
#13986=CARTESIAN_POINT('Ctrl Pts',(-18.5751646562309,-12.7591191023728,
124.342816270802)) ;
#13987=CARTESIAN_POINT('Ctrl Pts',(-18.5751743458909,-12.7591196999312,
124.342824951917)) ;
#13988=CARTESIAN_POINT('Ctrl Pts',(-18.5751914208737,-12.7591207529287,
124.342840249175)) ;
#13989=CARTESIAN_POINT('Ctrl Pts',(-18.5751988058895,-12.7591212083516,
124.342846865157)) ;
#13990=CARTESIAN_POINT('Ctrl Pts',(-18.5752136547505,-12.7591221240511,
124.342860167424)) ;
#13991=CARTESIAN_POINT('Ctrl Pts',(-18.5752211171675,-12.7591225842395,
124.342866852425)) ;
#13992=CARTESIAN_POINT('Ctrl Pts',(-18.5752361163824,-12.7591235091955,
124.342880288736)) ;
#13993=CARTESIAN_POINT('Ctrl Pts',(-18.5752436552404,-12.7591239740899,
124.342887041887)) ;
#13994=CARTESIAN_POINT('Ctrl Pts',(-18.5752588107679,-12.7591249086693,
124.342900617559)) ;
#13995=CARTESIAN_POINT('Ctrl Pts',(-18.5752664274573,-12.7591253783553,
124.342907440094)) ;
#13996=CARTESIAN_POINT('Ctrl Pts',(-18.5752817405074,-12.7591263226322,
124.342921156191)) ;
#13997=CARTESIAN_POINT('Ctrl Pts',(-18.5752894363132,-12.7591267971888,
124.342928049251)) ;
#13998=CARTESIAN_POINT('Ctrl Pts',(-18.5753049082886,-12.7591277512493,
124.342941907008)) ;
#13999=CARTESIAN_POINT('Ctrl Pts',(-18.5753126844561,-12.7591282307529,
124.342948871698)) ;
#14000=CARTESIAN_POINT('Ctrl Pts',(-18.575328315123,-12.759129194582,124.342962870884)) ;
#14001=CARTESIAN_POINT('Ctrl Pts',(-18.5753361711164,-12.7591296789994,
124.342969906714)) ;
#14002=CARTESIAN_POINT('Ctrl Pts',(-18.5753519669284,-12.7591306529945,
124.342984053087)) ;
#14003=CARTESIAN_POINT('Ctrl Pts',(-18.5753599053588,-12.7591311424864,
124.342991162383)) ;
#14004=CARTESIAN_POINT('Ctrl Pts',(-18.5753758637796,-12.7591321264906,
124.34300545365)) ;
#14005=CARTESIAN_POINT('Ctrl Pts',(-18.5753838844763,-12.7591326210463,
124.343012636248)) ;
#14006=CARTESIAN_POINT('Ctrl Pts',(-18.5754000099134,-12.7591336153308,
124.343027076332)) ;
#14007=CARTESIAN_POINT('Ctrl Pts',(-18.5754081140767,-12.7591341150239,
124.343034333297)) ;
#14008=CARTESIAN_POINT('Ctrl Pts',(-18.5754244091464,-12.7591351197494,
124.343048924517)) ;
#14009=CARTESIAN_POINT('Ctrl Pts',(-18.5754325988824,-12.7591356247096,
124.343056257722)) ;
#14010=CARTESIAN_POINT('Ctrl Pts',(-18.5754490614152,-12.7591366397418,
124.343070998112)) ;
#14011=CARTESIAN_POINT('Ctrl Pts',(-18.5754573358176,-12.7591371499128,
124.343078406733)) ;
#14012=CARTESIAN_POINT('Ctrl Pts',(-18.5754739732433,-12.7591381757093,
124.343093302922)) ;
#14013=CARTESIAN_POINT('Ctrl Pts',(-18.5754823349523,-12.7591386912537,
124.34310078931)) ;
#14014=CARTESIAN_POINT('Ctrl Pts',(-18.5754991450576,-12.7591397276773,
124.343115839291)) ;
#14015=CARTESIAN_POINT('Ctrl Pts',(-18.575507594108,-12.7591402485969,124.343123403465)) ;
#14016=CARTESIAN_POINT('Ctrl Pts',(-18.5755245814094,-12.7591412959255,
124.343138611256)) ;
#14017=CARTESIAN_POINT('Ctrl Pts',(-18.5755331193561,-12.7591418223158,
124.343146254595)) ;
#14018=CARTESIAN_POINT('Ctrl Pts',(-18.5755502845499,-12.7591428805918,
124.343161620792)) ;
#14019=CARTESIAN_POINT('Ctrl Pts',(-18.5755589120634,-12.7591434124938,
124.343169343884)) ;
#14020=CARTESIAN_POINT('Ctrl Pts',(-18.5755762580752,-12.7591444818969,
124.34318487108)) ;
#14021=CARTESIAN_POINT('Ctrl Pts',(-18.5755849763239,-12.7591450193824,
124.343192674957)) ;
#14022=CARTESIAN_POINT('Ctrl Pts',(-18.5756025056162,-12.7591461000636,
124.343208365329)) ;
#14023=CARTESIAN_POINT('Ctrl Pts',(-18.5756113162067,-12.7591466432313,
124.343216251415)) ;
#14024=CARTESIAN_POINT('Ctrl Pts',(-18.5756290289732,-12.759147735202,124.343232105108)) ;
#14025=CARTESIAN_POINT('Ctrl Pts',(-18.575637932094,-12.7591482840631,124.343240073557)) ;
#14026=CARTESIAN_POINT('Ctrl Pts',(-18.5756558327912,-12.7591493875973,
124.343256094533)) ;
#14027=CARTESIAN_POINT('Ctrl Pts',(-18.5756648300303,-12.7591499422495,
124.343264146752)) ;
#14028=CARTESIAN_POINT('Ctrl Pts',(-18.5756829202618,-12.7591510574454,
124.343280336415)) ;
#14029=CARTESIAN_POINT('Ctrl Pts',(-18.575692013104,-12.7591516179798,124.343288473719)) ;
#14030=CARTESIAN_POINT('Ctrl Pts',(-18.5757102936334,-12.7591527448837,
124.343304832723)) ;
#14031=CARTESIAN_POINT('Ctrl Pts',(-18.5757194824738,-12.7591533113242,
124.343313055449)) ;
#14032=CARTESIAN_POINT('Ctrl Pts',(-18.575737956618,-12.7591544501399,124.343329586732)) ;
#14033=CARTESIAN_POINT('Ctrl Pts',(-18.5757472421849,-12.7591550225311,
124.343337895518)) ;
#14034=CARTESIAN_POINT('Ctrl Pts',(-18.5757659147772,-12.7591561735558,
124.343354603373)) ;
#14035=CARTESIAN_POINT('Ctrl Pts',(-18.5757752999546,-12.7591567520751,
124.343363000783)) ;
#14036=CARTESIAN_POINT('Ctrl Pts',(-18.5757941681839,-12.7591579151347,
124.343379882663)) ;
#14037=CARTESIAN_POINT('Ctrl Pts',(-18.5758036524342,-12.7591584997486,
124.3433883682)) ;
#14038=CARTESIAN_POINT('Ctrl Pts',(-18.5758227231047,-12.7591596752617,
124.343405430161)) ;
#14039=CARTESIAN_POINT('Ctrl Pts',(-18.5758323086862,-12.759160266109,124.343414005829)) ;
#14040=CARTESIAN_POINT('Ctrl Pts',(-18.5758515817138,-12.7591614540696,
124.343431247762)) ;
#14041=CARTESIAN_POINT('Ctrl Pts',(-18.5758612694762,-12.7591620512023,
124.343439914304)) ;
#14042=CARTESIAN_POINT('Ctrl Pts',(-18.575880747629,-12.7591632517802,124.34345733865)) ;
#14043=CARTESIAN_POINT('Ctrl Pts',(-18.5758905384708,-12.7591638552532,
124.343466096853)) ;
#14044=CARTESIAN_POINT('Ctrl Pts',(-18.5759102256245,-12.7591650686865,
124.343483707046)) ;
#14045=CARTESIAN_POINT('Ctrl Pts',(-18.5759201215757,-12.7591656786245,
124.343492558707)) ;
#14046=CARTESIAN_POINT('Ctrl Pts',(-18.5759400175723,-12.7591669049027,
124.343510354569)) ;
#14047=CARTESIAN_POINT('Ctrl Pts',(-18.5759500188267,-12.7591675213172,
124.343519299845)) ;
#14048=CARTESIAN_POINT('Ctrl Pts',(-18.5759701283546,-12.7591687607282,
124.343537285533)) ;
#14049=CARTESIAN_POINT('Ctrl Pts',(-18.5759802362928,-12.7591693837039,
124.343546325639)) ;
#14050=CARTESIAN_POINT('Ctrl Pts',(-18.5760005631137,-12.7591706364788,
124.34356450448)) ;
#14051=CARTESIAN_POINT('Ctrl Pts',(-18.5760107804656,-12.7591712661834,
124.34357364184)) ;
#14052=CARTESIAN_POINT('Ctrl Pts',(-18.5760313226115,-12.7591725321999,
124.343592012036)) ;
#14053=CARTESIAN_POINT('Ctrl Pts',(-18.5760416490364,-12.759173168612,124.343601246325)) ;
#14054=CARTESIAN_POINT('Ctrl Pts',(-18.5760624126772,-12.7591744482494,
124.343619813355)) ;
#14055=CARTESIAN_POINT('Ctrl Pts',(-18.5760728498013,-12.7591750914688,
124.343629146007)) ;
#14056=CARTESIAN_POINT('Ctrl Pts',(-18.5760938371435,-12.7591763848621,
124.343647911803)) ;
#14057=CARTESIAN_POINT('Ctrl Pts',(-18.5761043865159,-12.7591770349838,
124.343657344184)) ;
#14058=CARTESIAN_POINT('Ctrl Pts',(-18.5761256008144,-12.7591783423326,
124.343676311617)) ;
#14059=CARTESIAN_POINT('Ctrl Pts',(-18.5761362648107,-12.7591789995024,
124.34368584583)) ;
#14060=CARTESIAN_POINT('Ctrl Pts',(-18.5761577046036,-12.7591803207157,
124.34370501355)) ;
#14061=CARTESIAN_POINT('Ctrl Pts',(-18.5761684824747,-12.759180984887,124.343714648904)) ;
#14062=CARTESIAN_POINT('Ctrl Pts',(-18.5761901562053,-12.759182320484,124.343734024417)) ;
#14063=CARTESIAN_POINT('Ctrl Pts',(-18.5762010508702,-12.7591829918361,
124.3437437635)) ;
#14064=CARTESIAN_POINT('Ctrl Pts',(-18.5762229576896,-12.7591843417635,
124.343763346004)) ;
#14065=CARTESIAN_POINT('Ctrl Pts',(-18.5762339699876,-12.7591850203475,
124.343773189545)) ;
#14066=CARTESIAN_POINT('Ctrl Pts',(-18.5762561140326,-12.7591863848592,
124.343792982692)) ;
#14067=CARTESIAN_POINT('Ctrl Pts',(-18.5762672456259,-12.7591870707771,
124.343802932153)) ;
#14068=CARTESIAN_POINT('Ctrl Pts',(-18.5762896288272,-12.7591884499908,
124.343822937624)) ;
#14069=CARTESIAN_POINT('Ctrl Pts',(-18.5763008807322,-12.7591891433047,
124.343832993891)) ;
#14070=CARTESIAN_POINT('Ctrl Pts',(-18.5763235068996,-12.7591905374541,
124.343853215044)) ;
#14071=CARTESIAN_POINT('Ctrl Pts',(-18.576334880719,-12.7591912382621,124.343863379527)) ;
#14072=CARTESIAN_POINT('Ctrl Pts',(-18.5763577530773,-12.7591926475448,
124.343883819196)) ;
#14073=CARTESIAN_POINT('Ctrl Pts',(-18.5763692508888,-12.7591933559744,
124.343894093725)) ;
#14074=CARTESIAN_POINT('Ctrl Pts',(-18.5763923704753,-12.759194780453,124.343914752789)) ;
#14075=CARTESIAN_POINT('Ctrl Pts',(-18.5764039930901,-12.7591954965536,
124.343925138066)) ;
#14076=CARTESIAN_POINT('Ctrl Pts',(-18.5764273643471,-12.7591969365007,
124.343946020443)) ;
#14077=CARTESIAN_POINT('Ctrl Pts',(-18.5764391133914,-12.7591976603718,
124.343956517895)) ;
#14078=CARTESIAN_POINT('Ctrl Pts',(-18.5764627386005,-12.7591991159267,
124.343977625574)) ;
#14079=CARTESIAN_POINT('Ctrl Pts',(-18.576474615157,-12.7591998476345,124.343988236143)) ;
#14080=CARTESIAN_POINT('Ctrl Pts',(-18.5764984992101,-12.7592013190973,
124.344009573442)) ;
#14081=CARTESIAN_POINT('Ctrl Pts',(-18.576510505759,-12.7592020587938,124.344020299317)) ;
#14082=CARTESIAN_POINT('Ctrl Pts',(-18.5765346490174,-12.7592035461856,
124.344041866505)) ;
#14083=CARTESIAN_POINT('Ctrl Pts',(-18.5765467862843,-12.759204293915,124.344052708307)) ;
#14084=CARTESIAN_POINT('Ctrl Pts',(-18.5765711940765,-12.7592057975626,
124.344074510089)) ;
#14085=CARTESIAN_POINT('Ctrl Pts',(-18.5765834641956,-12.7592065534556,
124.344085469696)) ;
#14086=CARTESIAN_POINT('Ctrl Pts',(-18.5766081383778,-12.7592080734721,
124.344107507675)) ;
#14087=CARTESIAN_POINT('Ctrl Pts',(-18.5766205427388,-12.7592088376137,
124.344118586301)) ;
#14088=CARTESIAN_POINT('Ctrl Pts',(-18.5766454867075,-12.7592103742069,
124.344140863452)) ;
#14089=CARTESIAN_POINT('Ctrl Pts',(-18.5766580267301,-12.7592111466838,
124.344152062337)) ;
#14090=CARTESIAN_POINT('Ctrl Pts',(-18.5766832440137,-12.7592127000697,
124.344174581752)) ;
#14091=CARTESIAN_POINT('Ctrl Pts',(-18.576695921225,-12.7592134809753,124.344185902229)) ;
#14092=CARTESIAN_POINT('Ctrl Pts',(-18.5767214162173,-12.759215051423,124.344208667774)) ;
#14093=CARTESIAN_POINT('Ctrl Pts',(-18.5767342331826,-12.7592158409146,
124.344220112103)) ;
#14094=CARTESIAN_POINT('Ctrl Pts',(-18.5767600061612,-12.7592174284398,
124.344243123963)) ;
#14095=CARTESIAN_POINT('Ctrl Pts',(-18.5767729633222,-12.7592182265438,
124.344254692508)) ;
#14096=CARTESIAN_POINT('Ctrl Pts',(-18.5767990208619,-12.7592198315499,
124.344277956491)) ;
#14097=CARTESIAN_POINT('Ctrl Pts',(-18.5768121206846,-12.7592206384175,
124.344289651422)) ;
#14098=CARTESIAN_POINT('Ctrl Pts',(-18.5799543720719,-12.7594141786897,
124.347094792777)) ;
#14099=CARTESIAN_POINT('Ctrl Pts',(-18.583097558938,-12.7596070945764,124.349872466011)) ;
#14100=CARTESIAN_POINT('Ctrl Pts',(-18.5914589411826,-12.7601184272586,
124.357186899497)) ;
#14101=CARTESIAN_POINT('Ctrl Pts',(-18.5967008949658,-12.7604370990635,
124.361696267903)) ;
#14102=CARTESIAN_POINT('Ctrl Pts',(-18.6142194942362,-12.7614955712047,
124.37651542867)) ;
#14103=CARTESIAN_POINT('Ctrl Pts',(-18.6266570252239,-12.7622365207948,
124.386632519347)) ;
#14104=CARTESIAN_POINT('Ctrl Pts',(-18.6663971117434,-12.7645688214455,
124.417707511162)) ;
#14105=CARTESIAN_POINT('Ctrl Pts',(-18.6943727063018,-12.7661594369059,
124.437778868525)) ;
#14106=CARTESIAN_POINT('Ctrl Pts',(-18.73008714712,-12.7681254681389,124.461231667369)) ;
#14107=CARTESIAN_POINT('Ctrl Pts',(-18.7370786758153,-12.7685074288161,
124.465723695912)) ;
#14108=CARTESIAN_POINT('Ctrl Pts',(-18.7491234197455,-12.7691605635696,
124.473293777753)) ;
#14109=CARTESIAN_POINT('Ctrl Pts',(-18.7541546411038,-12.769431946238,124.47640627762)) ;
#14110=CARTESIAN_POINT('Ctrl Pts',(-18.7642894294835,-12.7699757842253,
124.482576980619)) ;
#14111=CARTESIAN_POINT('Ctrl Pts',(-18.7693931148766,-12.7702482299903,
124.485634699285)) ;
#14112=CARTESIAN_POINT('Ctrl Pts',(-18.7799644880319,-12.7708096955153,
124.491866089112)) ;
#14113=CARTESIAN_POINT('Ctrl Pts',(-18.7854348161993,-12.77109867739,124.495034953049)) ;
#14114=CARTESIAN_POINT('Ctrl Pts',(-18.798488578728,-12.7717846908643,124.502465083759)) ;
#14115=CARTESIAN_POINT('Ctrl Pts',(-18.8060929249016,-12.7721814802344,
124.506688963167)) ;
#14116=CARTESIAN_POINT('Ctrl Pts',(-18.827409080212,-12.7732862682195,124.518239668095)) ;
#14117=CARTESIAN_POINT('Ctrl Pts',(-18.8412144235751,-12.7739932454686,
124.525390589664)) ;
#14118=CARTESIAN_POINT('Ctrl Pts',(-18.9036640460803,-12.7771582774044,
124.556274788094)) ;
#14119=CARTESIAN_POINT('Ctrl Pts',(-18.9536853187154,-12.7796106807045,
124.577091089033)) ;
#14120=CARTESIAN_POINT('Ctrl Pts',(-19.0320157727976,-12.7833898013155,
124.603870949393)) ;
#14121=CARTESIAN_POINT('Ctrl Pts',(-19.0594444436341,-12.7846998776024,
124.612206737053)) ;
#14122=CARTESIAN_POINT('Ctrl Pts',(-19.1155718308537,-12.7873582674251,
124.627176961971)) ;
#14123=CARTESIAN_POINT('Ctrl Pts',(-19.1442673790073,-12.7887058255138,
124.633754866544)) ;
#14124=CARTESIAN_POINT('Ctrl Pts',(-19.1936065288727,-12.7910093160185,
124.643245031454)) ;
#14125=CARTESIAN_POINT('Ctrl Pts',(-19.2141398095654,-12.7919640533508,
124.646665172238)) ;
#14126=CARTESIAN_POINT('Ctrl Pts',(-19.236866182519,-12.7930183171429,124.649869585487)) ;
#14127=CARTESIAN_POINT('Ctrl Pts',(-19.2389842913548,-12.7931165519873,
124.650162697319)) ;
#14128=CARTESIAN_POINT('Ctrl Pts',(-19.2555154005346,-12.793883076883,124.652407119127)) ;
#14129=CARTESIAN_POINT('Ctrl Pts',(-19.2699606813584,-12.7945519057057,
124.654112169403)) ;
#14130=CARTESIAN_POINT('Ctrl Pts',(-19.3010638516899,-12.7959913443683,
124.657234110347)) ;
#14131=CARTESIAN_POINT('Ctrl Pts',(-19.3177270702512,-12.7967621004021,
124.658569703818)) ;
#14132=CARTESIAN_POINT('Ctrl Pts',(-19.3576560865813,-12.7986107176195,
124.660965280775)) ;
#14133=CARTESIAN_POINT('Ctrl Pts',(-19.3809344503295,-12.7996907717898,
124.661710037211)) ;
#14134=CARTESIAN_POINT('Ctrl Pts',(-19.4433867258348,-12.8025898172644,
124.661962466935)) ;
#14135=CARTESIAN_POINT('Ctrl Pts',(-19.4825398110413,-12.8044067169687,
124.660279821104)) ;
#14136=CARTESIAN_POINT('Ctrl Pts',(-19.5307263214418,-12.8066364472764,
124.655934057454)) ;
#14137=CARTESIAN_POINT('Ctrl Pts',(-19.5398937974138,-12.8070604300559,
124.655004983066)) ;
#14138=CARTESIAN_POINT('Ctrl Pts',(-19.5545314138148,-12.8077371332337,
124.65335783964)) ;
#14139=CARTESIAN_POINT('Ctrl Pts',(-19.5600085032303,-12.8079902825689,
124.652704773599)) ;
#14140=CARTESIAN_POINT('Ctrl Pts',(-19.5702826133265,-12.808465075288,124.651410703569)) ;
#14141=CARTESIAN_POINT('Ctrl Pts',(-19.5750805807026,-12.8086867715125,
124.650778051794)) ;
#14142=CARTESIAN_POINT('Ctrl Pts',(-19.5847393217084,-12.8091330395337,
124.649447355378)) ;
#14143=CARTESIAN_POINT('Ctrl Pts',(-19.5895998988103,-12.8093576018542,
124.648748498749)) ;
#14144=CARTESIAN_POINT('Ctrl Pts',(-19.6008357490794,-12.8098767241804,
124.647065366126)) ;
#14145=CARTESIAN_POINT('Ctrl Pts',(-19.6072077785756,-12.8101711394818,
124.646060344001)) ;
#14146=CARTESIAN_POINT('Ctrl Pts',(-19.6240090187073,-12.8109476139213,
124.643276928103)) ;
#14147=CARTESIAN_POINT('Ctrl Pts',(-19.6344239393097,-12.8114291270485,
124.64141537431)) ;
#14148=CARTESIAN_POINT('Ctrl Pts',(-19.6684697379865,-12.8130047941458,
124.63488298679)) ;
#14149=CARTESIAN_POINT('Ctrl Pts',(-19.6919893947084,-12.8140957545046,
124.629661323584)) ;
#14150=CARTESIAN_POINT('Ctrl Pts',(-19.7353618648572,-12.816121610241,124.618707835472)) ;
#14151=CARTESIAN_POINT('Ctrl Pts',(-19.7552517860486,-12.8170562573009,
124.613157130575)) ;
#14152=CARTESIAN_POINT('Ctrl Pts',(-19.7894947587977,-12.8186826313674,
124.602679916513)) ;
#14153=CARTESIAN_POINT('Ctrl Pts',(-19.8039124706347,-12.8193731537586,
124.597980039551)) ;
#14154=CARTESIAN_POINT('Ctrl Pts',(-19.8285507303693,-12.8205631056495,
124.589449529066)) ;
#14155=CARTESIAN_POINT('Ctrl Pts',(-19.8388132444028,-12.8210617156686,
124.585745179152)) ;
#14156=CARTESIAN_POINT('Ctrl Pts',(-19.8629615017187,-12.8222418478977,
124.576669585387)) ;
#14157=CARTESIAN_POINT('Ctrl Pts',(-19.8768023814789,-12.8229236901255,
124.571183674441)) ;
#14158=CARTESIAN_POINT('Ctrl Pts',(-19.9098018091956,-12.8245623797158,
124.5574171103)) ;
#14159=CARTESIAN_POINT('Ctrl Pts',(-19.9288574422983,-12.8255193692947,
124.548901307972)) ;
#14160=CARTESIAN_POINT('Ctrl Pts',(-19.9871965467417,-12.8284840258764,
124.521057219369)) ;
#14161=CARTESIAN_POINT('Ctrl Pts',(-20.0256844747708,-12.8304891715993,
124.500139763345)) ;
#14162=CARTESIAN_POINT('Ctrl Pts',(-20.0823781022484,-12.8335386363419,
124.465353929019)) ;
#14163=CARTESIAN_POINT('Ctrl Pts',(-20.1014324430568,-12.8345812962938,
124.452934609476)) ;
#14164=CARTESIAN_POINT('Ctrl Pts',(-20.1233438087625,-12.8358049379282,
124.437785606451)) ;
#14165=CARTESIAN_POINT('Ctrl Pts',(-20.1265398989144,-12.8359840554574,
124.435553735641)) ;
#14166=CARTESIAN_POINT('Ctrl Pts',(-20.1396143035031,-12.8367194523825,
124.426332428001)) ;
#14167=CARTESIAN_POINT('Ctrl Pts',(-20.1494012861676,-12.8372762312192,
124.419214694118)) ;
#14168=CARTESIAN_POINT('Ctrl Pts',(-20.1698041636898,-12.8384515108891,
124.403918556395)) ;
#14169=CARTESIAN_POINT('Ctrl Pts',(-20.1803949931304,-12.8390703489683,
124.395709293072)) ;
#14170=CARTESIAN_POINT('Ctrl Pts',(-20.225115556298,-12.8417202382887,124.359879394597)) ;
#14171=CARTESIAN_POINT('Ctrl Pts',(-20.2579095152776,-12.843754580663,124.330641028655)) ;
#14172=CARTESIAN_POINT('Ctrl Pts',(-20.2970342675946,-12.8462923176429,
124.291873131076)) ;
#14173=CARTESIAN_POINT('Ctrl Pts',(-20.3048656616391,-12.8468063913784,
124.283902247049)) ;
#14174=CARTESIAN_POINT('Ctrl Pts',(-20.3167518534326,-12.8475962996151,
124.271475353459)) ;
#14175=CARTESIAN_POINT('Ctrl Pts',(-20.3208830520861,-12.8478726939179,
124.26709326184)) ;
#14176=CARTESIAN_POINT('Ctrl Pts',(-20.3290565117171,-12.8484233004166,
124.258296917279)) ;
#14177=CARTESIAN_POINT('Ctrl Pts',(-20.3330990583362,-12.8486975084328,
124.253883143514)) ;
#14178=CARTESIAN_POINT('Ctrl Pts',(-20.3411230451982,-12.8492456339764,
124.24499498233)) ;
#14179=CARTESIAN_POINT('Ctrl Pts',(-20.3451043400114,-12.8495195440812,
124.240520673072)) ;
#14180=CARTESIAN_POINT('Ctrl Pts',(-20.3542499840372,-12.8501533840125,
124.230092541126)) ;
#14181=CARTESIAN_POINT('Ctrl Pts',(-20.3593904908652,-12.8505131343864,
124.224118138291)) ;
#14182=CARTESIAN_POINT('Ctrl Pts',(-20.3730234662391,-12.8514769485059,
124.207967141218)) ;
#14183=CARTESIAN_POINT('Ctrl Pts',(-20.3814111593863,-12.852080304637,124.197703410935)) ;
#14184=CARTESIAN_POINT('Ctrl Pts',(-20.4127129938379,-12.8543745585008,
124.158132337548)) ;
#14185=CARTESIAN_POINT('Ctrl Pts',(-20.4344779286586,-12.856059051023,124.127940852657)) ;
#14186=CARTESIAN_POINT('Ctrl Pts',(-20.462952793321,-12.858423421377,124.084477101685)) ;
#14187=CARTESIAN_POINT('Ctrl Pts',(-20.4708222736493,-12.859096559288,124.071988120083)) ;
#14188=CARTESIAN_POINT('Ctrl Pts',(-20.484652665494,-12.8603163932561,124.049152134433)) ;
#14189=CARTESIAN_POINT('Ctrl Pts',(-20.490690040506,-12.8608625217,124.038853463684)) ;
#14190=CARTESIAN_POINT('Ctrl Pts',(-20.5031559892708,-12.8620195826105,
124.016873105728)) ;
#14191=CARTESIAN_POINT('Ctrl Pts',(-20.509547054518,-12.8626305558189,124.005171818958)) ;
#14192=CARTESIAN_POINT('Ctrl Pts',(-20.5286655508952,-12.8645145864201,
123.968796683161)) ;
#14193=CARTESIAN_POINT('Ctrl Pts',(-20.5407591637519,-12.8657878954575,
123.943799353735)) ;
#14194=CARTESIAN_POINT('Ctrl Pts',(-20.5761903754447,-12.8697966497089,
123.86387804393)) ;
#14195=CARTESIAN_POINT('Ctrl Pts',(-20.596434399967,-12.8725233361498,123.807674804892)) ;
#14196=CARTESIAN_POINT('Ctrl Pts',(-20.6153990071595,-12.8757375971586,
123.740244066871)) ;
#14197=CARTESIAN_POINT('Ctrl Pts',(-20.6180860565241,-12.8762144539577,
123.730211921012)) ;
#14198=CARTESIAN_POINT('Ctrl Pts',(-20.6232668921773,-12.8771798972182,
123.709857514234)) ;
#14199=CARTESIAN_POINT('Ctrl Pts',(-20.6257547864346,-12.8776684675554,
123.699534623669)) ;
#14200=CARTESIAN_POINT('Ctrl Pts',(-20.6309517764012,-12.8787478359158,
123.676697396913)) ;
#14201=CARTESIAN_POINT('Ctrl Pts',(-20.633600725302,-12.879338944442,123.664170597919)) ;
#14202=CARTESIAN_POINT('Ctrl Pts',(-20.6443107105378,-12.8819184993699,
123.609377697487)) ;
#14203=CARTESIAN_POINT('Ctrl Pts',(-20.6503789088771,-12.8839083919632,
123.566751697832)) ;
#14204=CARTESIAN_POINT('Ctrl Pts',(-20.654999940553,-12.8862792553361,123.515423623374)) ;
#14205=CARTESIAN_POINT('Ctrl Pts',(-20.6556763172627,-12.8866702638371,
123.506941959054)) ;
#14206=CARTESIAN_POINT('Ctrl Pts',(-20.6567406270531,-12.887375169527,123.491623482111)) ;
#14207=CARTESIAN_POINT('Ctrl Pts',(-20.6571590758495,-12.8876892041029,
123.484789135382)) ;
#14208=CARTESIAN_POINT('Ctrl Pts',(-20.6578583610003,-12.8882948369598,
123.4715911087)) ;
#14209=CARTESIAN_POINT('Ctrl Pts',(-20.6581467493784,-12.8885864637149,
123.465228040448)) ;
#14210=CARTESIAN_POINT('Ctrl Pts',(-20.6586568763359,-12.8892064974777,
123.451684472268)) ;
#14211=CARTESIAN_POINT('Ctrl Pts',(-20.658865374892,-12.8895348294125,123.444503698921)) ;
#14212=CARTESIAN_POINT('Ctrl Pts',(-20.6595849924584,-12.8911453132697,
123.40924555664)) ;
#14213=CARTESIAN_POINT('Ctrl Pts',(-20.6592117538883,-12.8924228737751,
123.381158170071)) ;
#14214=CARTESIAN_POINT('Ctrl Pts',(-20.6564231569889,-12.89512259501,123.321848631689)) ;
#14215=CARTESIAN_POINT('Ctrl Pts',(-20.6537801752152,-12.8965435669904,
123.290656533896)) ;
#14216=CARTESIAN_POINT('Ctrl Pts',(-20.6491903713324,-12.8982651229884,
123.253245901899)) ;
#14217=CARTESIAN_POINT('Ctrl Pts',(-20.6483624559018,-12.8985577366996,
123.246901156957)) ;
#14218=CARTESIAN_POINT('Ctrl Pts',(-20.6466704796217,-12.8991231389022,
123.234667509143)) ;
#14219=CARTESIAN_POINT('Ctrl Pts',(-20.6458129994407,-12.8993958720515,
123.228777860617)) ;
#14220=CARTESIAN_POINT('Ctrl Pts',(-20.6439072145186,-12.8999741464242,
123.216312959949)) ;
#14221=CARTESIAN_POINT('Ctrl Pts',(-20.6428483703075,-12.9002797301754,
123.209739502278)) ;
#14222=CARTESIAN_POINT('Ctrl Pts',(-20.6367048048506,-12.901970069064,123.173448546114)) ;
#14223=CARTESIAN_POINT('Ctrl Pts',(-20.6305987330449,-12.9033575521151,
123.143914086722)) ;
#14224=CARTESIAN_POINT('Ctrl Pts',(-20.6186215546723,-12.9056739694174,
123.094980946943)) ;
#14225=CARTESIAN_POINT('Ctrl Pts',(-20.613336029205,-12.9066032901679,123.075452097576)) ;
#14226=CARTESIAN_POINT('Ctrl Pts',(-20.6050799446674,-12.9079343362961,
123.047642673982)) ;
#14227=CARTESIAN_POINT('Ctrl Pts',(-20.6024923489333,-12.908336974391,123.039251807705)) ;
#14228=CARTESIAN_POINT('Ctrl Pts',(-20.5972574559531,-12.9091242371297,
123.02289067531)) ;
#14229=CARTESIAN_POINT('Ctrl Pts',(-20.5946209881441,-12.909508404291,123.014927913574)) ;
#14230=CARTESIAN_POINT('Ctrl Pts',(-20.5919012759315,-12.9098928303969,
123.006982853616)) ;
#14231=CARTESIAN_POINT('Ctrl Pts',(-20.5919012759315,-12.9098928303969,
123.006982853616)) ;
#14232=CARTESIAN_POINT('Ctrl Pts',(-20.5775883978109,-12.9119159282728,
122.965170828688)) ;
#14233=CARTESIAN_POINT('Ctrl Pts',(-20.5610720915834,-12.913930083847,122.924156496481)) ;
#14234=CARTESIAN_POINT('Ctrl Pts',(-20.5390005048911,-12.9163204656711,
122.876763499143)) ;
#14235=CARTESIAN_POINT('Ctrl Pts',(-20.535515506082,-12.9166903884443,122.86946624177)) ;
#14236=CARTESIAN_POINT('Ctrl Pts',(-20.5292796758374,-12.9173397518683,
122.856728342592)) ;
#14237=CARTESIAN_POINT('Ctrl Pts',(-20.5265593912635,-12.9176190406129,
122.851273046282)) ;
#14238=CARTESIAN_POINT('Ctrl Pts',(-20.5205508334242,-12.9182275802382,
122.839440928627)) ;
#14239=CARTESIAN_POINT('Ctrl Pts',(-20.5172473473947,-12.9185569433274,
122.833072087567)) ;
#14240=CARTESIAN_POINT('Ctrl Pts',(-20.5020609149817,-12.9200477324229,
122.804400581149)) ;
#14241=CARTESIAN_POINT('Ctrl Pts',(-20.4895581579928,-12.9212119086459,
122.782432984259)) ;
#14242=CARTESIAN_POINT('Ctrl Pts',(-20.466223985624,-12.9232759343705,122.744180711674)) ;
#14243=CARTESIAN_POINT('Ctrl Pts',(-20.4556601246545,-12.924175579931,122.727742669082)) ;
#14244=CARTESIAN_POINT('Ctrl Pts',(-20.4364479105815,-12.9257529044473,
122.699334242229)) ;
#14245=CARTESIAN_POINT('Ctrl Pts',(-20.4279646375281,-12.926430934959,122.687256855252)) ;
#14246=CARTESIAN_POINT('Ctrl Pts',(-20.4133949963966,-12.9275656788204,
122.667276326277)) ;
#14247=CARTESIAN_POINT('Ctrl Pts',(-20.4074243176364,-12.9280227994365,
122.65929072306)) ;
#14248=CARTESIAN_POINT('Ctrl Pts',(-20.3941634429978,-12.9290213380387,
122.641990229912)) ;
#14249=CARTESIAN_POINT('Ctrl Pts',(-20.3868352717985,-12.929562547123,122.632705642966)) ;
#14250=CARTESIAN_POINT('Ctrl Pts',(-20.3610542716988,-12.9314315605306,
122.600978331977)) ;
#14251=CARTESIAN_POINT('Ctrl Pts',(-20.3419515233651,-12.9327561986542,
122.579075828085)) ;
#14252=CARTESIAN_POINT('Ctrl Pts',(-20.3106440615985,-12.9348459453513,
122.545609901931)) ;
#14253=CARTESIAN_POINT('Ctrl Pts',(-20.2989397911291,-12.935610738074,122.533592878431)) ;
#14254=CARTESIAN_POINT('Ctrl Pts',(-20.2814419447094,-12.9367329085392,
122.516336350602)) ;
#14255=CARTESIAN_POINT('Ctrl Pts',(-20.27583545528,-12.9370894005287,122.510909785357)) ;
#14256=CARTESIAN_POINT('Ctrl Pts',(-20.2659046674212,-12.9377158583434,
122.501476173242)) ;
#14257=CARTESIAN_POINT('Ctrl Pts',(-20.2616021434998,-12.9379856691212,
122.497446564531)) ;
#14258=CARTESIAN_POINT('Ctrl Pts',(-20.2519496753662,-12.938587562321,122.488533695003)) ;
#14259=CARTESIAN_POINT('Ctrl Pts',(-20.2465854743106,-12.9389197320638,
122.483666207131)) ;
#14260=CARTESIAN_POINT('Ctrl Pts',(-20.2270582676089,-12.9401204287918,
122.466254240205)) ;
#14261=CARTESIAN_POINT('Ctrl Pts',(-20.2126532360644,-12.9409902152709,
122.453985095874)) ;
#14262=CARTESIAN_POINT('Ctrl Pts',(-20.1764627723942,-12.9431355769463,
122.424551696291)) ;
#14263=CARTESIAN_POINT('Ctrl Pts',(-20.1543739584847,-12.9444108212181,
122.407776355452)) ;
#14264=CARTESIAN_POINT('Ctrl Pts',(-20.1214485345774,-12.9462637013913,
122.38445652436)) ;
#14265=CARTESIAN_POINT('Ctrl Pts',(-20.1110416642655,-12.9468427140955,
122.377319858696)) ;
#14266=CARTESIAN_POINT('Ctrl Pts',(-20.0893877105434,-12.948034356684,122.36294748405)) ;
#14267=CARTESIAN_POINT('Ctrl Pts',(-20.0781289530905,-12.9486468519291,
122.355732225217)) ;
#14268=CARTESIAN_POINT('Ctrl Pts',(-20.0404641982286,-12.950673807246,122.332438434902)) ;
#14269=CARTESIAN_POINT('Ctrl Pts',(-20.013577594316,-12.9520852288538,122.317158833203)) ;
#14270=CARTESIAN_POINT('Ctrl Pts',(-19.9722410487926,-12.9542132268343,
122.295654876225)) ;
#14271=CARTESIAN_POINT('Ctrl Pts',(-19.9581949553827,-12.9549293486662,
122.288680474729)) ;
#14272=CARTESIAN_POINT('Ctrl Pts',(-19.9367534984031,-12.9560139352812,
122.278532330691)) ;
#14273=CARTESIAN_POINT('Ctrl Pts',(-19.929452589261,-12.9563817676605,122.275162680817)) ;
#14274=CARTESIAN_POINT('Ctrl Pts',(-19.9165600417877,-12.9570290663708,
122.269362508569)) ;
#14275=CARTESIAN_POINT('Ctrl Pts',(-19.9109821796069,-12.9573083830753,
122.266902012721)) ;
#14276=CARTESIAN_POINT('Ctrl Pts',(-19.8991668995139,-12.9578986875235,
122.261793003398)) ;
#14277=CARTESIAN_POINT('Ctrl Pts',(-19.8929255038013,-12.9582097501578,
122.259154211467)) ;
#14278=CARTESIAN_POINT('Ctrl Pts',(-19.8700549107403,-12.9593467891548,
122.249703246257)) ;
#14279=CARTESIAN_POINT('Ctrl Pts',(-19.8533008261686,-12.9601742283784,
122.243199144594)) ;
#14280=CARTESIAN_POINT('Ctrl Pts',(-19.8150409010411,-12.9620496723781,
122.229287870074)) ;
#14281=CARTESIAN_POINT('Ctrl Pts',(-19.7934612941257,-12.9630975384539,
122.222101840424)) ;
#14282=CARTESIAN_POINT('Ctrl Pts',(-19.7608071561949,-12.964667639962,122.212209144376)) ;
#14283=CARTESIAN_POINT('Ctrl Pts',(-19.7498720628182,-12.9651908792965,
122.20905867726)) ;
#14284=CARTESIAN_POINT('Ctrl Pts',(-19.730578335943,-12.9661096961196,122.203784261632)) ;
#14285=CARTESIAN_POINT('Ctrl Pts',(-19.7222378945073,-12.9665054658401,
122.201596683093)) ;
#14286=CARTESIAN_POINT('Ctrl Pts',(-19.7059301429664,-12.9672766282725,
122.19749925101)) ;
#14287=CARTESIAN_POINT('Ctrl Pts',(-19.697965364666,-12.9676520343278,122.195581086492)) ;
#14288=CARTESIAN_POINT('Ctrl Pts',(-19.6793714499795,-12.9685257088492,
122.19129604052)) ;
#14289=CARTESIAN_POINT('Ctrl Pts',(-19.6687290844817,-12.9690237042166,
122.188989475399)) ;
#14290=CARTESIAN_POINT('Ctrl Pts',(-19.6314713285406,-12.9707606754512,
122.18142273586)) ;
#14291=CARTESIAN_POINT('Ctrl Pts',(-19.6047159181063,-12.9719964138408,
122.176890166614)) ;
#14292=CARTESIAN_POINT('Ctrl Pts',(-19.5534875532042,-12.9743496367233,
122.169918365052)) ;
#14293=CARTESIAN_POINT('Ctrl Pts',(-19.5290485731015,-12.9754668014679,
122.167323562315)) ;
#14294=CARTESIAN_POINT('Ctrl Pts',(-19.4953567298301,-12.9770065505603,
122.164748027889)) ;
#14295=CARTESIAN_POINT('Ctrl Pts',(-19.4861569061565,-12.9774269667192,
122.164147047146)) ;
#14296=CARTESIAN_POINT('Ctrl Pts',(-19.4692081758792,-12.9782020447752,
122.163228039796)) ;
#14297=CARTESIAN_POINT('Ctrl Pts',(-19.4614613306496,-12.9785565199066,
122.162880248932)) ;
#14298=CARTESIAN_POINT('Ctrl Pts',(-19.4457005712165,-12.9792781019746,
122.162319573871)) ;
#14299=CARTESIAN_POINT('Ctrl Pts',(-19.4376868317705,-12.9796452147584,
122.162111653568)) ;
#14300=CARTESIAN_POINT('Ctrl Pts',(-19.4231292281717,-12.9803124980177,
122.161874048511)) ;
#14301=CARTESIAN_POINT('Ctrl Pts',(-19.4165860636093,-12.9806125642582,
122.16181863751)) ;
#14302=CARTESIAN_POINT('Ctrl Pts',(-19.3894599254743,-12.9818571648361,
122.161801916126)) ;
#14303=CARTESIAN_POINT('Ctrl Pts',(-19.3688799470573,-12.9828028529772,
122.162297614695)) ;
#14304=CARTESIAN_POINT('Ctrl Pts',(-19.2997663948605,-12.9859843516414,
122.165671636333)) ;
#14305=CARTESIAN_POINT('Ctrl Pts',(-19.2513906353841,-12.9882209259606,
122.170872526433)) ;
#14306=CARTESIAN_POINT('Ctrl Pts',(-19.1906592259112,-12.9910469194208,
122.181011263803)) ;
#14307=CARTESIAN_POINT('Ctrl Pts',(-19.1779114292336,-12.9916411202217,
122.183343730252)) ;
#14308=CARTESIAN_POINT('Ctrl Pts',(-19.1387932554911,-12.9934685562291,
122.191131690272)) ;
#14309=CARTESIAN_POINT('Ctrl Pts',(-19.112561093433,-12.9946994898168,122.19724136478)) ;
#14310=CARTESIAN_POINT('Ctrl Pts',(-19.0766342740806,-12.9964005165196,
122.206842474578)) ;
#14311=CARTESIAN_POINT('Ctrl Pts',(-19.0667548191317,-12.9968699254867,
122.209613429599)) ;
#14312=CARTESIAN_POINT('Ctrl Pts',(-19.0475907638457,-12.9977845517515,
122.215243904706)) ;
#14313=CARTESIAN_POINT('Ctrl Pts',(-19.0383031769058,-12.9982297840111,
122.218090649035)) ;
#14314=CARTESIAN_POINT('Ctrl Pts',(-19.0092749852391,-12.9996275150051,
122.227359593344)) ;
#14315=CARTESIAN_POINT('Ctrl Pts',(-18.9896606004508,-13.0005806747561,
122.234165443737)) ;
#14316=CARTESIAN_POINT('Ctrl Pts',(-18.9553630060942,-13.0022616890983,
122.247031825415)) ;
#14317=CARTESIAN_POINT('Ctrl Pts',(-18.9406087125977,-13.00298965324,122.252889666438)) ;
#14318=CARTESIAN_POINT('Ctrl Pts',(-18.8899170461784,-13.0055084196402,
122.274141977281)) ;
#14319=CARTESIAN_POINT('Ctrl Pts',(-18.8545930053298,-13.0072943080635,
122.290940047591)) ;
#14320=CARTESIAN_POINT('Ctrl Pts',(-18.789226128513,-13.0106847478791,122.325872663727)) ;
#14321=CARTESIAN_POINT('Ctrl Pts',(-18.7590453480146,-13.0122863021443,
122.343670393544)) ;
#14322=CARTESIAN_POINT('Ctrl Pts',(-18.7164615896387,-13.0146092337777,
122.371256628846)) ;
#14323=CARTESIAN_POINT('Ctrl Pts',(-18.7034336533728,-13.0153289723965,
122.380049426649)) ;
#14324=CARTESIAN_POINT('Ctrl Pts',(-18.6805344091642,-13.0166118918159,
122.396141300326)) ;
#14325=CARTESIAN_POINT('Ctrl Pts',(-18.6705982792143,-13.0171747476147,
122.403344544381)) ;
#14326=CARTESIAN_POINT('Ctrl Pts',(-18.6469979013449,-13.0185277606215,
122.42098969531)) ;
#14327=CARTESIAN_POINT('Ctrl Pts',(-18.6334399184256,-13.0193183437501,
122.431569548518)) ;
#14328=CARTESIAN_POINT('Ctrl Pts',(-18.5984805170206,-13.0213918369986,
122.460029577977)) ;
#14329=CARTESIAN_POINT('Ctrl Pts',(-18.5774515410442,-13.0226746626617,
122.478352085696)) ;
#14330=CARTESIAN_POINT('Ctrl Pts',(-18.5429132329147,-13.0248445416171,
122.510539905779)) ;
#14331=CARTESIAN_POINT('Ctrl Pts',(-18.5290810402856,-13.0257320030397,
122.52404354139)) ;
#14332=CARTESIAN_POINT('Ctrl Pts',(-18.5047329145781,-13.0273293859359,
122.548941977604)) ;
#14333=CARTESIAN_POINT('Ctrl Pts',(-18.4941052648056,-13.028039496196,122.560221999166)) ;
#14334=CARTESIAN_POINT('Ctrl Pts',(-18.4589733246402,-13.0304330212014,
122.598927883898)) ;
#14335=CARTESIAN_POINT('Ctrl Pts',(-18.4354703127565,-13.0321124777807,
122.627236596445)) ;
#14336=CARTESIAN_POINT('Ctrl Pts',(-18.4047310311276,-13.0344379210765,
122.667774222138)) ;
#14337=CARTESIAN_POINT('Ctrl Pts',(-18.3964031040837,-13.0350824709017,
122.679151490865)) ;
#14338=CARTESIAN_POINT('Ctrl Pts',(-18.3833515378214,-13.0361177635829,
122.697629945667)) ;
#14339=CARTESIAN_POINT('Ctrl Pts',(-18.3785050054822,-13.0365080752328,
122.704642830045)) ;
#14340=CARTESIAN_POINT('Ctrl Pts',(-18.369132579751,-13.0372749482622,122.718505711784)) ;
#14341=CARTESIAN_POINT('Ctrl Pts',(-18.3646016899217,-13.0376514897607,
122.725351807494)) ;
#14342=CARTESIAN_POINT('Ctrl Pts',(-18.3488433516192,-13.0389822660292,
122.749679759746)) ;
#14343=CARTESIAN_POINT('Ctrl Pts',(-18.3379846614465,-13.0399379662251,
122.76739634588)) ;
#14344=CARTESIAN_POINT('Ctrl Pts',(-18.3171127031513,-13.041854177952,122.803436863907)) ;
#14345=CARTESIAN_POINT('Ctrl Pts',(-18.3071067891807,-13.0428143931389,
122.821757622706)) ;
#14346=CARTESIAN_POINT('Ctrl Pts',(-18.2941348880858,-13.0441183797035,
122.846991420965)) ;
#14347=CARTESIAN_POINT('Ctrl Pts',(-18.290765598599,-13.044462973073,122.853693262422)) ;
#14348=CARTESIAN_POINT('Ctrl Pts',(-18.2867069652352,-13.0448854653208,
122.861950653556)) ;
#14349=CARTESIAN_POINT('Ctrl Pts',(-18.28596021056,-13.0449635157868,122.863477806124)) ;
#14350=CARTESIAN_POINT('Ctrl Pts',(-18.2802327545433,-13.0455645893776,
122.875251556097)) ;
#14351=CARTESIAN_POINT('Ctrl Pts',(-18.2753892269254,-13.0460871962536,
122.885564309199)) ;
#14352=CARTESIAN_POINT('Ctrl Pts',(-18.2655112925735,-13.0471842395133,
122.907365948865)) ;
#14353=CARTESIAN_POINT('Ctrl Pts',(-18.2605074570837,-13.0477585241867,
122.918867325056)) ;
#14354=CARTESIAN_POINT('Ctrl Pts',(-18.2451817496326,-13.0495793052044,
122.955594936856)) ;
#14355=CARTESIAN_POINT('Ctrl Pts',(-18.2355113869129,-13.0508234540972,
122.981084399287)) ;
#14356=CARTESIAN_POINT('Ctrl Pts',(-18.2203367506623,-13.0529613368954,
123.02540001655)) ;
#14357=CARTESIAN_POINT('Ctrl Pts',(-18.2144279535755,-13.0538549217811,
123.04407699115)) ;
#14358=CARTESIAN_POINT('Ctrl Pts',(-18.2065168751264,-13.0551496405923,
123.071290985516)) ;
#14359=CARTESIAN_POINT('Ctrl Pts',(-18.2041616510312,-13.0555497707345,
123.079722348193)) ;
#14360=CARTESIAN_POINT('Ctrl Pts',(-18.2003504332994,-13.0562232653936,
123.093940691903)) ;
#14361=CARTESIAN_POINT('Ctrl Pts',(-18.1988469605123,-13.0564964154554,
123.099714622365)) ;
#14362=CARTESIAN_POINT('Ctrl Pts',(-18.1964149231448,-13.0569511588676,
123.109336588704)) ;
#14363=CARTESIAN_POINT('Ctrl Pts',(-18.1954631943831,-13.0571326213352,
123.113178672354)) ;
#14364=CARTESIAN_POINT('Ctrl Pts',(-18.1928193199878,-13.057646912745,123.124073328738)) ;
#14365=CARTESIAN_POINT('Ctrl Pts',(-18.1911702881845,-13.0579800440933,
123.131136177628)) ;
#14366=CARTESIAN_POINT('Ctrl Pts',(-18.1851915367861,-13.0592356437218,
123.157788890227)) ;
#14367=CARTESIAN_POINT('Ctrl Pts',(-18.1812721773872,-13.0601593967781,
123.177467705277)) ;
#14368=CARTESIAN_POINT('Ctrl Pts',(-18.1762450257569,-13.0615059729539,
123.206317538316)) ;
#14369=CARTESIAN_POINT('Ctrl Pts',(-18.1747624931863,-13.0619297561237,
123.215420010491)) ;
#14370=CARTESIAN_POINT('Ctrl Pts',(-18.1733279372883,-13.0623693498795,
123.22488706714)) ;
#14371=CARTESIAN_POINT('Ctrl Pts',(-18.1732752009602,-13.0623855546872,
123.225236087655)) ;
#14372=CARTESIAN_POINT('Ctrl Pts',(-18.1731739898418,-13.0624167411119,
123.225907850948)) ;
#14373=CARTESIAN_POINT('Ctrl Pts',(-18.1731254935991,-13.0624317228131,
123.226230590453)) ;
#14374=CARTESIAN_POINT('Ctrl Pts',(-18.1730322579247,-13.0624605999273,
123.22685272611)) ;
#14375=CARTESIAN_POINT('Ctrl Pts',(-18.1729875008424,-13.0624744954116,
123.227152119618)) ;
#14376=CARTESIAN_POINT('Ctrl Pts',(-18.1729013020541,-13.0625013214108,
123.227730165044)) ;
#14377=CARTESIAN_POINT('Ctrl Pts',(-18.1728598457825,-13.0625142519837,
123.228008814765)) ;
#14378=CARTESIAN_POINT('Ctrl Pts',(-18.1727798609613,-13.0625392560214,
123.228547686934)) ;
#14379=CARTESIAN_POINT('Ctrl Pts',(-18.1727413203504,-13.0625513295345,
123.228807907568)) ;
#14380=CARTESIAN_POINT('Ctrl Pts',(-18.172666825022,-13.0625747156766,123.229311987152)) ;
#14381=CARTESIAN_POINT('Ctrl Pts',(-18.172630860287,-13.0625860283463,123.229555844607)) ;
#14382=CARTESIAN_POINT('Ctrl Pts',(-18.1725612139819,-13.0626079789659,
123.230029048278)) ;
#14383=CARTESIAN_POINT('Ctrl Pts',(-18.1725275240742,-13.0626186169493,
123.230258393242)) ;
#14384=CARTESIAN_POINT('Ctrl Pts',(-18.1714248313732,-13.0629674569973,
123.237779552869)) ;
#14385=CARTESIAN_POINT('Ctrl Pts',(-18.1704202705523,-13.0633053813651,
123.245080681877)) ;
#14386=CARTESIAN_POINT('Ctrl Pts',(-18.168431666638,-13.06401971258,123.260545440612)) ;
#14387=CARTESIAN_POINT('Ctrl Pts',(-18.1674634882772,-13.0643960305851,
123.268710763728)) ;
#14388=CARTESIAN_POINT('Ctrl Pts',(-18.1635092236459,-13.0660711434776,
123.305129464474)) ;
#14389=CARTESIAN_POINT('Ctrl Pts',(-18.1614063174537,-13.0673653346237,
123.333470214096)) ;
#14390=CARTESIAN_POINT('Ctrl Pts',(-18.1597382240551,-13.0692691129838,
123.375175643557)) ;
#14391=CARTESIAN_POINT('Ctrl Pts',(-18.1594185947804,-13.0698773215834,
123.388500908696)) ;
#14392=CARTESIAN_POINT('Ctrl Pts',(-18.1592439251985,-13.0708763703781,
123.410365268362)) ;
#14393=CARTESIAN_POINT('Ctrl Pts',(-18.159263180604,-13.0712667198629,123.418902286574)) ;
#14394=CARTESIAN_POINT('Ctrl Pts',(-18.1594670905398,-13.0720133768512,
123.435214793494)) ;
#14395=CARTESIAN_POINT('Ctrl Pts',(-18.1596368666112,-13.0723696050656,
123.44299007411)) ;
#14396=CARTESIAN_POINT('Ctrl Pts',(-18.1601550285815,-13.0731320120191,
123.459611551135)) ;
#14397=CARTESIAN_POINT('Ctrl Pts',(-18.1605248558696,-13.073538264051,123.468456653791)) ;
#14398=CARTESIAN_POINT('Ctrl Pts',(-18.1618961037786,-13.0747406513569,
123.494596480354)) ;
#14399=CARTESIAN_POINT('Ctrl Pts',(-18.1631631162199,-13.0755378065521,
123.511875105038)) ;
#14400=CARTESIAN_POINT('Ctrl Pts',(-18.1668635155437,-13.0773543273082,
123.551131676553)) ;
#14401=CARTESIAN_POINT('Ctrl Pts',(-18.1695217492384,-13.0783739957619,
123.57308269195)) ;
#14402=CARTESIAN_POINT('Ctrl Pts',(-18.1737028013295,-13.0796881684279,
123.60131243919)) ;
#14403=CARTESIAN_POINT('Ctrl Pts',(-18.1746939543766,-13.0799841292373,
123.607665877077)) ;
#14404=CARTESIAN_POINT('Ctrl Pts',(-18.1769725583315,-13.08063206423,123.62156689713)) ;
#14405=CARTESIAN_POINT('Ctrl Pts',(-18.1782804218478,-13.0809839434711,
123.629110877309)) ;
#14406=CARTESIAN_POINT('Ctrl Pts',(-18.1796825750349,-13.0813418989933,
123.636779442194)) ;
#14407=CARTESIAN_POINT('Ctrl Pts',(-18.1797076591581,-13.0813482967574,
123.636916501118)) ;
#14408=CARTESIAN_POINT('Ctrl Pts',(-18.1797571007982,-13.08136089524,123.637186393973)) ;
#14409=CARTESIAN_POINT('Ctrl Pts',(-18.17978145692,-13.0813670959634,123.637319228122)) ;
#14410=CARTESIAN_POINT('Ctrl Pts',(-18.1798294756377,-13.0813793098524,
123.637580875011)) ;
#14411=CARTESIAN_POINT('Ctrl Pts',(-18.1798531369639,-13.0813853230271,
123.637709688049)) ;
#14412=CARTESIAN_POINT('Ctrl Pts',(-18.1798997978742,-13.0813971708785,
123.637963487097)) ;
#14413=CARTESIAN_POINT('Ctrl Pts',(-18.1799227962642,-13.081403005558,123.638088473264)) ;
#14414=CARTESIAN_POINT('Ctrl Pts',(-18.1799681618166,-13.0814145050659,
123.638334804078)) ;
#14415=CARTESIAN_POINT('Ctrl Pts',(-18.1799905278861,-13.0814201698995,
123.638456148926)) ;
#14416=CARTESIAN_POINT('Ctrl Pts',(-18.1800346581077,-13.0814313379743,
123.63869537427)) ;
#14417=CARTESIAN_POINT('Ctrl Pts',(-18.18005642125,-13.0814368412202,123.638813254951)) ;
#14418=CARTESIAN_POINT('Ctrl Pts',(-18.1800993737828,-13.0814476940123,
123.639045721263)) ;
#14419=CARTESIAN_POINT('Ctrl Pts',(-18.1801205622433,-13.0814530435636,
123.639160307084)) ;
#14420=CARTESIAN_POINT('Ctrl Pts',(-18.1801623924911,-13.0814635965141,
123.639386345569)) ;
#14421=CARTESIAN_POINT('Ctrl Pts',(-18.1801830334174,-13.0814687999178,
123.639497798402)) ;
#14422=CARTESIAN_POINT('Ctrl Pts',(-18.1802237946366,-13.0814790677941,
123.639717725786)) ;
#14423=CARTESIAN_POINT('Ctrl Pts',(-18.1802439141367,-13.0814841322717,
123.639826200512)) ;
#14424=CARTESIAN_POINT('Ctrl Pts',(-18.1802836575684,-13.0814941292115,
123.640040319999)) ;
#14425=CARTESIAN_POINT('Ctrl Pts',(-18.1803032807535,-13.081499061675,123.640145964852)) ;
#14426=CARTESIAN_POINT('Ctrl Pts',(-18.1803420556776,-13.0815088012103,
123.640354566639)) ;
#14427=CARTESIAN_POINT('Ctrl Pts',(-18.1803612067343,-13.0815136082854,
123.640457523704)) ;
#14428=CARTESIAN_POINT('Ctrl Pts',(-18.1803990606398,-13.0815231033946,
123.640660886096)) ;
#14429=CARTESIAN_POINT('Ctrl Pts',(-18.1804177628551,-13.0815277914313,
123.640761291535)) ;
#14430=CARTESIAN_POINT('Ctrl Pts',(-18.1804547414835,-13.0815370545586,
123.640959681367)) ;
#14431=CARTESIAN_POINT('Ctrl Pts',(-18.1804730173109,-13.0815416296518,
123.641057665866)) ;
#14432=CARTESIAN_POINT('Ctrl Pts',(-18.1805091647896,-13.0815506727483,
123.641251339383)) ;
#14433=CARTESIAN_POINT('Ctrl Pts',(-18.1805270358877,-13.0815551407512,
123.641347028439)) ;
#14434=CARTESIAN_POINT('Ctrl Pts',(-18.180562394769,-13.0815639752917,123.641536231661)) ;
#14435=CARTESIAN_POINT('Ctrl Pts',(-18.1805798820687,-13.0815683418361,
123.641629746015)) ;
#14436=CARTESIAN_POINT('Ctrl Pts',(-18.1806144935397,-13.0815769788782,
123.641814716)) ;
#14437=CARTESIAN_POINT('Ctrl Pts',(-18.1806316172486,-13.0815812493785,
123.641906171725)) ;
#14438=CARTESIAN_POINT('Ctrl Pts',(-18.1806655210745,-13.081589699554,123.642087136392)) ;
#14439=CARTESIAN_POINT('Ctrl Pts',(-18.1806823007714,-13.0815938792336,
123.642176645462)) ;
#14440=CARTESIAN_POINT('Ctrl Pts',(-18.1819650070658,-13.0819132007008,
123.649014945714)) ;
#14441=CARTESIAN_POINT('Ctrl Pts',(-18.1832865131806,-13.082228067896,123.655753204651)) ;
#14442=CARTESIAN_POINT('Ctrl Pts',(-18.1862418262234,-13.0829032804911,
123.670191157947)) ;
#14443=CARTESIAN_POINT('Ctrl Pts',(-18.1878929743441,-13.0832635260659,
123.677887005614)) ;
#14444=CARTESIAN_POINT('Ctrl Pts',(-18.1953906008683,-13.0848290950261,
123.711291358972)) ;
#14445=CARTESIAN_POINT('Ctrl Pts',(-18.2019769201654,-13.0860303966778,
123.736826857018)) ;
#14446=CARTESIAN_POINT('Ctrl Pts',(-18.214421298012,-13.0880550658993,123.779450919123)) ;
#14447=CARTESIAN_POINT('Ctrl Pts',(-18.2198510183822,-13.0888780516765,
123.796655324863)) ;
#14448=CARTESIAN_POINT('Ctrl Pts',(-18.225980363612,-13.0897489060499,123.814705658685)) ;
#14449=CARTESIAN_POINT('Ctrl Pts',(-18.2263107702426,-13.0897956839766,
123.815674762045)) ;
#14450=CARTESIAN_POINT('Ctrl Pts',(-18.2266423654692,-13.0898424649011,
123.816643453359)) ;
#14451=CARTESIAN_POINT('',(-20.5919012301245,-12.8497876110288,123.00698271985)) ;
#14452=CARTESIAN_POINT('Ctrl Pts',(-18.2266423654684,-13.0298305431221,
123.816643453356)) ;
#14453=CARTESIAN_POINT('Ctrl Pts',(-18.2266336269289,-13.0298293099018,
123.816617925403)) ;
#14454=CARTESIAN_POINT('Ctrl Pts',(-18.2266248892215,-13.0298280766837,
123.81659239716)) ;
#14455=CARTESIAN_POINT('Ctrl Pts',(-18.2220695400772,-13.0291850824373,
123.803282012787)) ;
#14456=CARTESIAN_POINT('Ctrl Pts',(-18.2177471039428,-13.0285428243449,
123.789921517234)) ;
#14457=CARTESIAN_POINT('Ctrl Pts',(-18.2110538843167,-13.0274922431459,
123.767977264901)) ;
#14458=CARTESIAN_POINT('Ctrl Pts',(-18.2085481026181,-13.0270843823758,
123.759435976209)) ;
#14459=CARTESIAN_POINT('Ctrl Pts',(-18.2034737365447,-13.0262264601579,
123.741429524127)) ;
#14460=CARTESIAN_POINT('Ctrl Pts',(-18.2009248867699,-13.025776357877,123.731959421547)) ;
#14461=CARTESIAN_POINT('Ctrl Pts',(-18.1960681444864,-13.0248784475954,
123.71302961412)) ;
#14462=CARTESIAN_POINT('Ctrl Pts',(-18.1937588160346,-13.0244306771055,
123.703570974076)) ;
#14463=CARTESIAN_POINT('Ctrl Pts',(-18.1888032044353,-13.0234201674437,
123.682192629131)) ;
#14464=CARTESIAN_POINT('Ctrl Pts',(-18.1862205901484,-13.0228571695493,
123.670259198915)) ;
#14465=CARTESIAN_POINT('Ctrl Pts',(-18.1801998711803,-13.0214465253905,
123.640324607423)) ;
#14466=CARTESIAN_POINT('Ctrl Pts',(-18.1769820460673,-13.0205977435113,
123.622282147979)) ;
#14467=CARTESIAN_POINT('Ctrl Pts',(-18.1684886776864,-13.018032102044,123.567748056236)) ;
#14468=CARTESIAN_POINT('Ctrl Pts',(-18.1644296947558,-13.0163037321195,
123.531087755827)) ;
#14469=CARTESIAN_POINT('Ctrl Pts',(-18.161852745762,-13.0144791238167,123.492122447006)) ;
#14470=CARTESIAN_POINT('Ctrl Pts',(-18.1617143016538,-13.0143770752841,
123.489942292877)) ;
#14471=CARTESIAN_POINT('Ctrl Pts',(-18.1613715988705,-13.0141136548413,
123.484312252165)) ;
#14472=CARTESIAN_POINT('Ctrl Pts',(-18.16117593067,-13.0139523234107,123.480861859157)) ;
#14473=CARTESIAN_POINT('Ctrl Pts',(-18.1595470511962,-13.0125040126246,
123.449864791374)) ;
#14474=CARTESIAN_POINT('Ctrl Pts',(-18.1590116944642,-13.0112227479266,
123.422278195262)) ;
#14475=CARTESIAN_POINT('Ctrl Pts',(-18.159474092363,-13.0096659130224,123.388516362409)) ;
#14476=CARTESIAN_POINT('Ctrl Pts',(-18.1596045604335,-13.0093814246662,
123.382337290293)) ;
#14477=CARTESIAN_POINT('Ctrl Pts',(-18.1598838429588,-13.0089314951013,
123.372550118525)) ;
#14478=CARTESIAN_POINT('Ctrl Pts',(-18.1600024749048,-13.0087657375565,
123.368941275192)) ;
#14479=CARTESIAN_POINT('Ctrl Pts',(-18.1602544879414,-13.0084549319154,
123.362168704233)) ;
#14480=CARTESIAN_POINT('Ctrl Pts',(-18.1603842569619,-13.0083098464332,
123.359004872697)) ;
#14481=CARTESIAN_POINT('Ctrl Pts',(-18.1605262519108,-13.0081646794803,
123.355836983321)) ;
#14482=CARTESIAN_POINT('Ctrl Pts',(-18.1605264572053,-13.0081644696259,
123.355832403791)) ;
#14483=CARTESIAN_POINT('Ctrl Pts',(-18.1605268679082,-13.0081640498524,
123.355823243313)) ;
#14484=CARTESIAN_POINT('Ctrl Pts',(-18.1605270732759,-13.0081638399751,
123.355818663275)) ;
#14485=CARTESIAN_POINT('Ctrl Pts',(-18.1605274840961,-13.008163420186,123.355809502436)) ;
#14486=CARTESIAN_POINT('Ctrl Pts',(-18.1605276895816,-13.0081632102403,
123.355804920897)) ;
#14487=CARTESIAN_POINT('Ctrl Pts',(-18.1605281006209,-13.0081627903314,
123.355795757425)) ;
#14488=CARTESIAN_POINT('Ctrl Pts',(-18.1605283061963,-13.008162580346,123.355791175009)) ;
#14489=CARTESIAN_POINT('Ctrl Pts',(-18.1605287174557,-13.0081621603164,
123.355782008884)) ;
#14490=CARTESIAN_POINT('Ctrl Pts',(-18.1605289231072,-13.0081619503053,
123.355777425898)) ;
#14491=CARTESIAN_POINT('Ctrl Pts',(-18.1605293344944,-13.0081615302493,
123.355768259179)) ;
#14492=CARTESIAN_POINT('Ctrl Pts',(-18.1605295402624,-13.0081613201714,
123.355763674725)) ;
#14493=CARTESIAN_POINT('Ctrl Pts',(-18.160529951926,-13.0081608999375,123.355754504102)) ;
#14494=CARTESIAN_POINT('Ctrl Pts',(-18.160530157757,-13.0081606898473,123.355749919372)) ;
#14495=CARTESIAN_POINT('Ctrl Pts',(-18.1605305695104,-13.0081602696258,
123.355740749002)) ;
#14496=CARTESIAN_POINT('Ctrl Pts',(-18.1605307754719,-13.0081600594547,
123.355736162494)) ;
#14497=CARTESIAN_POINT('Ctrl Pts',(-18.1605311874696,-13.0081596390882,
123.35572698894)) ;
#14498=CARTESIAN_POINT('Ctrl Pts',(-18.1605313935188,-13.0081594288795,
123.355722401605)) ;
#14499=CARTESIAN_POINT('Ctrl Pts',(-18.1605318057245,-13.0081590084051,
123.355713225676)) ;
#14500=CARTESIAN_POINT('Ctrl Pts',(-18.1605320118591,-13.0081587981614,
123.355708637567)) ;
#14501=CARTESIAN_POINT('Ctrl Pts',(-18.1605324242075,-13.0081583776457,
123.355699460718)) ;
#14502=CARTESIAN_POINT('Ctrl Pts',(-18.1605326304599,-13.0081581673341,
123.355694871117)) ;
#14503=CARTESIAN_POINT('Ctrl Pts',(-18.1605330430493,-13.0081577466768,
123.35568569116)) ;
#14504=CARTESIAN_POINT('Ctrl Pts',(-18.1605332493872,-13.0081575363302,
123.355681100786)) ;
#14505=CARTESIAN_POINT('Ctrl Pts',(-18.1605336622005,-13.008157115549,123.355671918105)) ;
#14506=CARTESIAN_POINT('Ctrl Pts',(-18.1605338686172,-13.0081569051743,
123.355667327108)) ;
#14507=CARTESIAN_POINT('Ctrl Pts',(-18.1605342815563,-13.0081564843692,
123.355658143886)) ;
#14508=CARTESIAN_POINT('Ctrl Pts',(-18.1605344880983,-13.0081562739189,
123.35565355123)) ;
#14509=CARTESIAN_POINT('Ctrl Pts',(-18.1605349012702,-13.008155852981,123.35564436509)) ;
#14510=CARTESIAN_POINT('Ctrl Pts',(-18.1605351079081,-13.0081556424851,
123.355639771429)) ;
#14511=CARTESIAN_POINT('Ctrl Pts',(-18.1605355212854,-13.0081552214423,
123.355630582984)) ;
#14512=CARTESIAN_POINT('Ctrl Pts',(-18.1605357280191,-13.0081550109011,
123.355625988324)) ;
#14513=CARTESIAN_POINT('Ctrl Pts',(-18.1605361415585,-13.0081545897976,
123.355616798532)) ;
#14514=CARTESIAN_POINT('Ctrl Pts',(-18.1605363484103,-13.0081543791883,
123.355612202376)) ;
#14515=CARTESIAN_POINT('Ctrl Pts',(-18.1605367622167,-13.0081539579174,
123.355603008913)) ;
#14516=CARTESIAN_POINT('Ctrl Pts',(-18.1605369691463,-13.0081537472812,
123.35559841216)) ;
#14517=CARTESIAN_POINT('Ctrl Pts',(-18.1605373831376,-13.0081533259264,
123.355589216849)) ;
#14518=CARTESIAN_POINT('Ctrl Pts',(-18.1605375901665,-13.0081531152414,
123.35558461902)) ;
#14519=CARTESIAN_POINT('Ctrl Pts',(-18.1605380043394,-13.0081526938064,
123.355575421938)) ;
#14520=CARTESIAN_POINT('Ctrl Pts',(-18.160538211481,-13.0081524830589,123.355570822737)) ;
#14521=CARTESIAN_POINT('Ctrl Pts',(-18.1605386258578,-13.0081520615208,
123.355561623386)) ;
#14522=CARTESIAN_POINT('Ctrl Pts',(-18.1605388331084,-13.0081518507147,
123.355557022897)) ;
#14523=CARTESIAN_POINT('Ctrl Pts',(-18.1605392477027,-13.00815142906,123.355547820981)) ;
#14524=CARTESIAN_POINT('Ctrl Pts',(-18.1605394550545,-13.0081512182032,
123.355543219377)) ;
#14525=CARTESIAN_POINT('Ctrl Pts',(-18.1605398698522,-13.0081507964462,
123.355534015209)) ;
#14526=CARTESIAN_POINT('Ctrl Pts',(-18.1605400773091,-13.0081505855348,
123.355529412403)) ;
#14527=CARTESIAN_POINT('Ctrl Pts',(-18.1605404923302,-13.0081501636553,
123.355520205542)) ;
#14528=CARTESIAN_POINT('Ctrl Pts',(-18.1605406998851,-13.0081499526966,
123.355515601694)) ;
#14529=CARTESIAN_POINT('Ctrl Pts',(-18.1605411150961,-13.0081495307287,
123.355506392886)) ;
#14530=CARTESIAN_POINT('Ctrl Pts',(-18.1605413227629,-13.0081493197085,
123.355501787686)) ;
#14531=CARTESIAN_POINT('Ctrl Pts',(-18.1605417382234,-13.0081488975917,
123.355492575609)) ;
#14532=CARTESIAN_POINT('Ctrl Pts',(-18.1605419459802,-13.0081486865325,
123.355487969547)) ;
#14533=CARTESIAN_POINT('Ctrl Pts',(-18.1605423616186,-13.0081482643396,
123.35547875579)) ;
#14534=CARTESIAN_POINT('Ctrl Pts',(-18.160542569491,-13.0081480532153,123.355474148299)) ;
#14535=CARTESIAN_POINT('Ctrl Pts',(-18.1605429853108,-13.0081476309429,
123.355464932787)) ;
#14536=CARTESIAN_POINT('Ctrl Pts',(-18.1605431933107,-13.0081474197415,
123.355460323603)) ;
#14537=CARTESIAN_POINT('Ctrl Pts',(-18.1607071371375,-13.0079809731343,
123.351827848802)) ;
#14538=CARTESIAN_POINT('Ctrl Pts',(-18.1608866822671,-13.0078149080799,
123.348200706442)) ;
#14539=CARTESIAN_POINT('Ctrl Pts',(-18.1613048012872,-13.0074598272328,
123.340439072758)) ;
#14540=CARTESIAN_POINT('Ctrl Pts',(-18.1615481206548,-13.0072708640559,
123.336304878289)) ;
#14541=CARTESIAN_POINT('Ctrl Pts',(-18.1622337413082,-13.0067804141476,
123.325565819221)) ;
#14542=CARTESIAN_POINT('Ctrl Pts',(-18.1627079720956,-13.0064792686464,
123.318963110444)) ;
#14543=CARTESIAN_POINT('Ctrl Pts',(-18.1642847940806,-13.0055791824351,
123.299206637341)) ;
#14544=CARTESIAN_POINT('Ctrl Pts',(-18.1655433124905,-13.0049818528825,
123.286066203533)) ;
#14545=CARTESIAN_POINT('Ctrl Pts',(-18.1715514625257,-13.0025412296005,
123.232318819475)) ;
#14546=CARTESIAN_POINT('Ctrl Pts',(-18.1780836579929,-13.0007151883165,
123.191937003724)) ;
#14547=CARTESIAN_POINT('Ctrl Pts',(-18.1968525805178,-12.9966613247086,
123.103627966524)) ;
#14548=CARTESIAN_POINT('Ctrl Pts',(-18.2099775134481,-12.9944296132711,
123.055960035106)) ;
#14549=CARTESIAN_POINT('Ctrl Pts',(-18.2300830433367,-12.9915874550878,
122.996865630726)) ;
#14550=CARTESIAN_POINT('Ctrl Pts',(-18.2344701859164,-12.990993435481,122.984602772603)) ;
#14551=CARTESIAN_POINT('Ctrl Pts',(-18.2416863646024,-12.9900553184883,
122.965384572863)) ;
#14552=CARTESIAN_POINT('Ctrl Pts',(-18.2443878243063,-12.9897119888688,
122.958382304742)) ;
#14553=CARTESIAN_POINT('Ctrl Pts',(-18.2494567369432,-12.9890817584299,
122.945587859146)) ;
#14554=CARTESIAN_POINT('Ctrl Pts',(-18.2518049374338,-12.9887949789871,
122.939788307398)) ;
#14555=CARTESIAN_POINT('Ctrl Pts',(-18.2565169420212,-12.9882294608902,
122.928397278077)) ;
#14556=CARTESIAN_POINT('Ctrl Pts',(-18.258878133078,-12.9879507448073,122.922804901488)) ;
#14557=CARTESIAN_POINT('Ctrl Pts',(-18.2642164911473,-12.9873307249975,
122.910413904723)) ;
#14558=CARTESIAN_POINT('Ctrl Pts',(-18.2672136599557,-12.9869893135365,
122.903624155769)) ;
#14559=CARTESIAN_POINT('Ctrl Pts',(-18.2748041407707,-12.9861408104745,
122.886835111482)) ;
#14560=CARTESIAN_POINT('Ctrl Pts',(-18.279469348912,-12.9856333172014,122.876869030968)) ;
#14561=CARTESIAN_POINT('Ctrl Pts',(-18.2928029426141,-12.9842201787856,
122.849337739322)) ;
#14562=CARTESIAN_POINT('Ctrl Pts',(-18.3017534746653,-12.9833129500962,
122.831912803098)) ;
#14563=CARTESIAN_POINT('Ctrl Pts',(-18.3320185935628,-12.98036955666,122.776251227436)) ;
#14564=CARTESIAN_POINT('Ctrl Pts',(-18.3549326776928,-12.978319937505,122.738922182948)) ;
#14565=CARTESIAN_POINT('Ctrl Pts',(-18.3805682746663,-12.9762021091121,
122.701694512618)) ;
#14566=CARTESIAN_POINT('Ctrl Pts',(-18.3813817150016,-12.9761350814685,
122.700517576275)) ;
#14567=CARTESIAN_POINT('Ctrl Pts',(-18.3829085278908,-12.9760095963076,
122.698316576487)) ;
#14568=CARTESIAN_POINT('Ctrl Pts',(-18.3836214170162,-12.975951137194,122.697292179863)) ;
#14569=CARTESIAN_POINT('Ctrl Pts',(-18.3856052009132,-12.9757888267649,
122.6944506383)) ;
#14570=CARTESIAN_POINT('Ctrl Pts',(-18.3868793990702,-12.9756849888592,
122.692635804345)) ;
#14571=CARTESIAN_POINT('Ctrl Pts',(-18.3885619414863,-12.9755484216114,
122.690252876268)) ;
#14572=CARTESIAN_POINT('Ctrl Pts',(-18.3889659424946,-12.9755156712703,
122.68968172152)) ;
#14573=CARTESIAN_POINT('Ctrl Pts',(-18.4095513146084,-12.9738490210497,
122.660630998101)) ;
#14574=CARTESIAN_POINT('Ctrl Pts',(-18.4309165761555,-12.9722230114565,
122.633008445789)) ;
#14575=CARTESIAN_POINT('Ctrl Pts',(-18.4574777499708,-12.9703218249028,
122.601489062063)) ;
#14576=CARTESIAN_POINT('Ctrl Pts',(-18.4615817755378,-12.9700311986185,
122.596693127422)) ;
#14577=CARTESIAN_POINT('Ctrl Pts',(-18.4680875489468,-12.9695753349817,
122.589206080453)) ;
#14578=CARTESIAN_POINT('Ctrl Pts',(-18.4704649068005,-12.969409749005,122.586493940138)) ;
#14579=CARTESIAN_POINT('Ctrl Pts',(-18.4747039860114,-12.96911624171,122.581699924995)) ;
#14580=CARTESIAN_POINT('Ctrl Pts',(-18.4765610072051,-12.9689882528876,
122.57961393174)) ;
#14581=CARTESIAN_POINT('Ctrl Pts',(-18.4807071325828,-12.9687037920801,
122.57498789679)) ;
#14582=CARTESIAN_POINT('Ctrl Pts',(-18.4829997009781,-12.9685473722279,
122.572450987117)) ;
#14583=CARTESIAN_POINT('Ctrl Pts',(-18.4891499840908,-12.9681300395952,
122.565701092549)) ;
#14584=CARTESIAN_POINT('Ctrl Pts',(-18.4930262244294,-12.9678694026981,
122.561505083046)) ;
#14585=CARTESIAN_POINT('Ctrl Pts',(-18.5018871512243,-12.9672788868826,
122.552044122779)) ;
#14586=CARTESIAN_POINT('Ctrl Pts',(-18.5068891610307,-12.966949267643,122.546795666759)) ;
#14587=CARTESIAN_POINT('Ctrl Pts',(-18.5226418805273,-12.9659224157567,
122.530552162321)) ;
#14588=CARTESIAN_POINT('Ctrl Pts',(-18.5335500387934,-12.9652274025998,
122.519711738178)) ;
#14589=CARTESIAN_POINT('Ctrl Pts',(-18.5685045394797,-12.9630457268317,
122.486233354646)) ;
#14590=CARTESIAN_POINT('Ctrl Pts',(-18.5932493131368,-12.9615673047214,
122.464345570966)) ;
#14591=CARTESIAN_POINT('Ctrl Pts',(-18.6206388709681,-12.9599777408857,
122.44198816693)) ;
#14592=CARTESIAN_POINT('Ctrl Pts',(-18.6224501432689,-12.9598728304576,
122.440518100581)) ;
#14593=CARTESIAN_POINT('Ctrl Pts',(-18.6499022235741,-12.9582857807891,
122.418364599517)) ;
#14594=CARTESIAN_POINT('Ctrl Pts',(-18.6763462679647,-12.9567933113416,
122.398698032973)) ;
#14595=CARTESIAN_POINT('Ctrl Pts',(-18.7133702272744,-12.9547495281684,
122.373372087445)) ;
#14596=CARTESIAN_POINT('Ctrl Pts',(-18.7233003775803,-12.9542057289873,
122.366785859565)) ;
#14597=CARTESIAN_POINT('Ctrl Pts',(-18.7409818158024,-12.9532450486145,
122.355419170495)) ;
#14598=CARTESIAN_POINT('Ctrl Pts',(-18.7486940463885,-12.9528285133464,
122.35057954299)) ;
#14599=CARTESIAN_POINT('Ctrl Pts',(-18.7622664335023,-12.9520997667497,
122.34226779189)) ;
#14600=CARTESIAN_POINT('Ctrl Pts',(-18.7681033879392,-12.951787726319,122.338758500398)) ;
#14601=CARTESIAN_POINT('Ctrl Pts',(-18.7829311162439,-12.9509984493496,
122.330007960016)) ;
#14602=CARTESIAN_POINT('Ctrl Pts',(-18.7919591987644,-12.9505210172755,
122.324830966065)) ;
#14603=CARTESIAN_POINT('Ctrl Pts',(-18.8137769629896,-12.949374552362,122.312679446884)) ;
#14604=CARTESIAN_POINT('Ctrl Pts',(-18.8266259755181,-12.9487053124731,
122.305814580976)) ;
#14605=CARTESIAN_POINT('Ctrl Pts',(-18.8637275526131,-12.9467890850053,
122.286818262751)) ;
#14606=CARTESIAN_POINT('Ctrl Pts',(-18.8882587671795,-12.9455415981957,
122.275249280256)) ;
#14607=CARTESIAN_POINT('Ctrl Pts',(-18.9655149318505,-12.9416657207147,
122.241842280331)) ;
#14608=CARTESIAN_POINT('Ctrl Pts',(-19.0193720611548,-12.9390347776241,
122.222809309062)) ;
#14609=CARTESIAN_POINT('Ctrl Pts',(-19.0998063954986,-12.9351796273224,
122.200439281251)) ;
#14610=CARTESIAN_POINT('Ctrl Pts',(-19.1254912117884,-12.9339608305303,
122.194166204317)) ;
#14611=CARTESIAN_POINT('Ctrl Pts',(-19.1611221700657,-12.9322863484592,
122.186652674809)) ;
#14612=CARTESIAN_POINT('Ctrl Pts',(-19.1709130152423,-12.9318278759446,
122.184710251597)) ;
#14613=CARTESIAN_POINT('Ctrl Pts',(-19.1880786543583,-12.9310267643606,
122.181517926934)) ;
#14614=CARTESIAN_POINT('Ctrl Pts',(-19.1954433497235,-12.9306839207001,
122.180216567884)) ;
#14615=CARTESIAN_POINT('Ctrl Pts',(-19.2106804647844,-12.9299762523928,
122.177664926839)) ;
#14616=CARTESIAN_POINT('Ctrl Pts',(-19.2185540627371,-12.929611481886,122.176423695558)) ;
#14617=CARTESIAN_POINT('Ctrl Pts',(-19.2267892434218,-12.9292308121882,
122.175206068492)) ;
#14618=CARTESIAN_POINT('Ctrl Pts',(-19.2271395021093,-12.9292146231502,
122.175154432433)) ;
#14619=CARTESIAN_POINT('Ctrl Pts',(-19.2278650919944,-12.9291810895227,
122.175047779008)) ;
#14620=CARTESIAN_POINT('Ctrl Pts',(-19.2282404264384,-12.9291637450193,
122.174992783667)) ;
#14621=CARTESIAN_POINT('Ctrl Pts',(-19.2290188956756,-12.9291277751127,
122.174879081532)) ;
#14622=CARTESIAN_POINT('Ctrl Pts',(-19.2294220342588,-12.9291091498134,
122.17482040094)) ;
#14623=CARTESIAN_POINT('Ctrl Pts',(-19.2302591420934,-12.9290704791468,
122.174698969938)) ;
#14624=CARTESIAN_POINT('Ctrl Pts',(-19.230693115835,-12.9290504339025,122.17463625077)) ;
#14625=CARTESIAN_POINT('Ctrl Pts',(-19.2315952603674,-12.9290087688394,
122.174506354742)) ;
#14626=CARTESIAN_POINT('Ctrl Pts',(-19.2320634365575,-12.9289871491633,
122.17443921521)) ;
#14627=CARTESIAN_POINT('Ctrl Pts',(-19.2326798965397,-12.9289586856092,
122.174351167854)) ;
#14628=CARTESIAN_POINT('Ctrl Pts',(-19.2328281457554,-12.9289518408366,
122.174330020993)) ;
#14629=CARTESIAN_POINT('Ctrl Pts',(-19.2432580248853,-12.9284703053083,
122.172844173597)) ;
#14630=CARTESIAN_POINT('Ctrl Pts',(-19.2535575246023,-12.927996125137,122.171507635619)) ;
#14631=CARTESIAN_POINT('Ctrl Pts',(-19.2833886519586,-12.9266258326528,
122.168013969547)) ;
#14632=CARTESIAN_POINT('Ctrl Pts',(-19.3029560120388,-12.9257308843601,
122.166188833968)) ;
#14633=CARTESIAN_POINT('Ctrl Pts',(-19.3494351787517,-12.9236089078578,
122.162956733505)) ;
#14634=CARTESIAN_POINT('Ctrl Pts',(-19.3763653699954,-12.9223825329253,
122.161957179838)) ;
#14635=CARTESIAN_POINT('Ctrl Pts',(-19.4095786774992,-12.920864405504,122.161798668492)) ;
#14636=CARTESIAN_POINT('Ctrl Pts',(-19.4158508302743,-12.9205774594865,
122.161815942134)) ;
#14637=CARTESIAN_POINT('Ctrl Pts',(-19.424764287832,-12.9201691529254,122.161907579719)) ;
#14638=CARTESIAN_POINT('Ctrl Pts',(-19.4274059076983,-12.9200480805764,
122.161943113438)) ;
#14639=CARTESIAN_POINT('Ctrl Pts',(-19.433577950039,-12.9197650267835,122.162045707723)) ;
#14640=CARTESIAN_POINT('Ctrl Pts',(-19.4371082377077,-12.919602993327,122.162119353658)) ;
#14641=CARTESIAN_POINT('Ctrl Pts',(-19.4444216276046,-12.9192670049565,
122.162302924444)) ;
#14642=CARTESIAN_POINT('Ctrl Pts',(-19.448204628969,-12.9190930270137,122.162415073944)) ;
#14643=CARTESIAN_POINT('Ctrl Pts',(-19.4647608464062,-12.9183307874337,
122.162981161356)) ;
#14644=CARTESIAN_POINT('Ctrl Pts',(-19.4775271204573,-12.9177409559588,
122.163613810563)) ;
#14645=CARTESIAN_POINT('Ctrl Pts',(-19.5167179285795,-12.9159257189815,
122.16615901209)) ;
#14646=CARTESIAN_POINT('Ctrl Pts',(-19.5430931910481,-12.9146979116109,
122.16871590326)) ;
#14647=CARTESIAN_POINT('Ctrl Pts',(-19.5943413384001,-12.9123067125982,
122.175334065345)) ;
#14648=CARTESIAN_POINT('Ctrl Pts',(-19.6192124398147,-12.9111436626271,
122.17931315571)) ;
#14649=CARTESIAN_POINT('Ctrl Pts',(-19.6510624441114,-12.9096515318053,
122.185400903659)) ;
#14650=CARTESIAN_POINT('Ctrl Pts',(-19.6581664503071,-12.9093185273144,
122.186822873812)) ;
#14651=CARTESIAN_POINT('Ctrl Pts',(-19.6703540734346,-12.9087468532339,
122.18937279983)) ;
#14652=CARTESIAN_POINT('Ctrl Pts',(-19.6754437342661,-12.9085080046585,
122.190470908064)) ;
#14653=CARTESIAN_POINT('Ctrl Pts',(-19.6856423385317,-12.9080291478141,
122.192738063472)) ;
#14654=CARTESIAN_POINT('Ctrl Pts',(-19.6907510886693,-12.9077891469546,
122.193907505581)) ;
#14655=CARTESIAN_POINT('Ctrl Pts',(-19.6959008113091,-12.9075470716328,
122.19512045997)) ;
#14656=CARTESIAN_POINT('Ctrl Pts',(-19.6959492799863,-12.9075447932305,
122.195131879232)) ;
#14657=CARTESIAN_POINT('Ctrl Pts',(-19.6960468120107,-12.9075402084448,
122.195154864015)) ;
#14658=CARTESIAN_POINT('Ctrl Pts',(-19.6960958755598,-12.9075379020515,
122.195166429657)) ;
#14659=CARTESIAN_POINT('Ctrl Pts',(-19.6961946333434,-12.9075332595898,
122.195189715919)) ;
#14660=CARTESIAN_POINT('Ctrl Pts',(-19.6962443272368,-12.9075309235369,
122.195201436538)) ;
#14661=CARTESIAN_POINT('Ctrl Pts',(-19.6963443822194,-12.9075262200386,
122.195225041611)) ;
#14662=CARTESIAN_POINT('Ctrl Pts',(-19.6963947433603,-12.9075238525903,
122.195236926163)) ;
#14663=CARTESIAN_POINT('Ctrl Pts',(-19.6964961705905,-12.9075190845251,
122.195260868275)) ;
#14664=CARTESIAN_POINT('Ctrl Pts',(-19.6965472363417,-12.9075166839237,
122.195272925848)) ;
#14665=CARTESIAN_POINT('Ctrl Pts',(-19.6966501111315,-12.9075118477487,
122.195297223336)) ;
#14666=CARTESIAN_POINT('Ctrl Pts',(-19.6967019206264,-12.9075094121531,
122.195309463459)) ;
#14667=CARTESIAN_POINT('Ctrl Pts',(-19.6968063228351,-12.9075045041113,
122.195334135785)) ;
#14668=CARTESIAN_POINT('Ctrl Pts',(-19.6968589155912,-12.9075020316625,
122.195346568104)) ;
#14669=CARTESIAN_POINT('Ctrl Pts',(-19.6969649258501,-12.9074970479603,
122.195371634962)) ;
#14670=CARTESIAN_POINT('Ctrl Pts',(-19.6970183430982,-12.9074945367184,
122.195384269554)) ;
#14671=CARTESIAN_POINT('Ctrl Pts',(-19.6971260448847,-12.9074894734284,
122.195409751368)) ;
#14672=CARTESIAN_POINT('Ctrl Pts',(-19.6971803293735,-12.9074869213822,
122.195422598699)) ;
#14673=CARTESIAN_POINT('Ctrl Pts',(-19.6972898096683,-12.9074817744119,
122.195448516779)) ;
#14674=CARTESIAN_POINT('Ctrl Pts',(-19.6973450053305,-12.907479179494,122.195461587624)) ;
#14675=CARTESIAN_POINT('Ctrl Pts',(-19.704265524275,-12.9071538223972,122.197100928202)) ;
#14676=CARTESIAN_POINT('Ctrl Pts',(-19.7111169724853,-12.9068314400042,
122.198785293131)) ;
#14677=CARTESIAN_POINT('Ctrl Pts',(-19.7263062321166,-12.9061159953381,
122.202656089544)) ;
#14678=CARTESIAN_POINT('Ctrl Pts',(-19.734636437213,-12.9057231274384,122.204870941649)) ;
#14679=CARTESIAN_POINT('Ctrl Pts',(-19.7584528572146,-12.9045980652846,
122.211467790609)) ;
#14680=CARTESIAN_POINT('Ctrl Pts',(-19.7738782638569,-12.9038671703928,
122.216062947165)) ;
#14681=CARTESIAN_POINT('Ctrl Pts',(-19.8516783300404,-12.9001633362013,
122.24088471048)) ;
#14682=CARTESIAN_POINT('Ctrl Pts',(-19.9124807820148,-12.8971994397584,
122.265698950611)) ;
#14683=CARTESIAN_POINT('Ctrl Pts',(-19.9933469057756,-12.8930709015398,
122.306382565535)) ;
#14684=CARTESIAN_POINT('Ctrl Pts',(-20.0152975841486,-12.8919314023757,
122.318262375764)) ;
#14685=CARTESIAN_POINT('Ctrl Pts',(-20.0508343508998,-12.8900519423772,
122.338893824642)) ;
#14686=CARTESIAN_POINT('Ctrl Pts',(-20.0646325832518,-12.8893132135106,
122.347265988289)) ;
#14687=CARTESIAN_POINT('Ctrl Pts',(-20.0889086065258,-12.8879962232401,
122.362646520013)) ;
#14688=CARTESIAN_POINT('Ctrl Pts',(-20.0994498145624,-12.8874183586131,
122.369550640215)) ;
#14689=CARTESIAN_POINT('Ctrl Pts',(-20.1199539244083,-12.8862817600257,
122.383427588994)) ;
#14690=CARTESIAN_POINT('Ctrl Pts',(-20.1299230498108,-12.8857231260621,
122.390388779537)) ;
#14691=CARTESIAN_POINT('Ctrl Pts',(-20.1510262187234,-12.8845268629432,
122.405587353481)) ;
#14692=CARTESIAN_POINT('Ctrl Pts',(-20.1621281300676,-12.883889129219,122.413866585721)) ;
#14693=CARTESIAN_POINT('Ctrl Pts',(-20.1880618963314,-12.8823780137799,
122.433885745853)) ;
#14694=CARTESIAN_POINT('Ctrl Pts',(-20.2027693373749,-12.8815039618097,
122.445781207129)) ;
#14695=CARTESIAN_POINT('Ctrl Pts',(-20.2422270825019,-12.8791075192343,
122.479204108083)) ;
#14696=CARTESIAN_POINT('Ctrl Pts',(-20.2664088268576,-12.8775784849994,
122.50137903495)) ;
#14697=CARTESIAN_POINT('Ctrl Pts',(-20.3143596103905,-12.8744327100056,
122.548956005798)) ;
#14698=CARTESIAN_POINT('Ctrl Pts',(-20.3379978085208,-12.8728190552624,
122.574451495325)) ;
#14699=CARTESIAN_POINT('Ctrl Pts',(-20.3651938259588,-12.8708871736827,
122.606354680304)) ;
#14700=CARTESIAN_POINT('Ctrl Pts',(-20.369797483671,-12.870557326814,122.611850216361)) ;
#14701=CARTESIAN_POINT('Ctrl Pts',(-20.3768479368778,-12.8700477093013,
122.620415183956)) ;
#14702=CARTESIAN_POINT('Ctrl Pts',(-20.379327966626,-12.869867575701,122.623457034667)) ;
#14703=CARTESIAN_POINT('Ctrl Pts',(-20.3842477556619,-12.8695084663496,
122.629549708395)) ;
#14704=CARTESIAN_POINT('Ctrl Pts',(-20.3866876218531,-12.8693294911164,
122.632600388911)) ;
#14705=CARTESIAN_POINT('Ctrl Pts',(-20.391486102151,-12.8689757270967,122.638658155829)) ;
#14706=CARTESIAN_POINT('Ctrl Pts',(-20.3938453055434,-12.8688009335381,
122.641664721437)) ;
#14707=CARTESIAN_POINT('Ctrl Pts',(-20.3991777528262,-12.8684038553865,
122.648524933948)) ;
#14708=CARTESIAN_POINT('Ctrl Pts',(-20.4021423534296,-12.8681816650298,
122.652385225493)) ;
#14709=CARTESIAN_POINT('Ctrl Pts',(-20.4179046597561,-12.8669924500009,
122.673159842202)) ;
#14710=CARTESIAN_POINT('Ctrl Pts',(-20.4302929158171,-12.8660298218524,
122.690380615241)) ;
#14711=CARTESIAN_POINT('Ctrl Pts',(-20.4558607530719,-12.8639748920025,
122.727900792871)) ;
#14712=CARTESIAN_POINT('Ctrl Pts',(-20.4689011499024,-12.8628838738838,
122.748284510883)) ;
#14713=CARTESIAN_POINT('Ctrl Pts',(-20.4960531297929,-12.8604999761191,
122.79357028138)) ;
#14714=CARTESIAN_POINT('Ctrl Pts',(-20.5099175272468,-12.8592058092289,
122.818604125775)) ;
#14715=CARTESIAN_POINT('Ctrl Pts',(-20.5278103056523,-12.857410504853,122.853702410417)) ;
#14716=CARTESIAN_POINT('Ctrl Pts',(-20.5325850941712,-12.8569179869799,
122.863376047395)) ;
#14717=CARTESIAN_POINT('Ctrl Pts',(-20.5411855853415,-12.8560055498111,
122.881384124822)) ;
#14718=CARTESIAN_POINT('Ctrl Pts',(-20.5450459528377,-12.8555858504352,
122.889701222488)) ;
#14719=CARTESIAN_POINT('Ctrl Pts',(-20.5527611804059,-12.8547258746532,
122.906814124024)) ;
#14720=CARTESIAN_POINT('Ctrl Pts',(-20.5566068930768,-12.8542855922374,
122.915613404169)) ;
#14721=CARTESIAN_POINT('Ctrl Pts',(-20.5718381409455,-12.8524934115106,
122.951587685943)) ;
#14722=CARTESIAN_POINT('Ctrl Pts',(-20.5823591340654,-12.8511406227468,
122.979107528826)) ;
#14723=CARTESIAN_POINT('Ctrl Pts',(-20.5919012301394,-12.8497876110192,
123.006982719845)) ;
#14724=CARTESIAN_POINT('Ctrl Pts',(-20.591897994858,-12.8497880697573,123.006973268786)) ;
#14725=CARTESIAN_POINT('Ctrl Pts',(-20.6111184683608,-12.8470627224272,
123.063121767626)) ;
#14726=CARTESIAN_POINT('Ctrl Pts',(-20.6263167775151,-12.8443459906656,
123.12056761031)) ;
#14727=CARTESIAN_POINT('Ctrl Pts',(-20.6404254348758,-12.8408729354201,
123.194951409159)) ;
#14728=CARTESIAN_POINT('Ctrl Pts',(-20.6431587032736,-12.8401219927567,
123.211085880344)) ;
#14729=CARTESIAN_POINT('Ctrl Pts',(-20.6485794869424,-12.8384343525263,
123.24740073539)) ;
#14730=CARTESIAN_POINT('Ctrl Pts',(-20.6510923700098,-12.8374973655753,
123.267602520437)) ;
#14731=CARTESIAN_POINT('Ctrl Pts',(-20.6551772941716,-12.8356010116792,
123.308592176691)) ;
#14732=CARTESIAN_POINT('Ctrl Pts',(-20.6567249160465,-12.8346419398219,
123.329376219405)) ;
#14733=CARTESIAN_POINT('Ctrl Pts',(-20.6583609785053,-12.8331162334971,
123.362521647017)) ;
#14734=CARTESIAN_POINT('Ctrl Pts',(-20.6587869472194,-12.8325489975594,
123.374862420184)) ;
#14735=CARTESIAN_POINT('Ctrl Pts',(-20.6592477243384,-12.8314746058903,
123.398264816964)) ;
#14736=CARTESIAN_POINT('Ctrl Pts',(-20.6593186805196,-12.830967401308,123.409324560519)) ;
#14737=CARTESIAN_POINT('Ctrl Pts',(-20.6591661534216,-12.8299478594391,
123.431572739217)) ;
#14738=CARTESIAN_POINT('Ctrl Pts',(-20.658939214423,-12.8294355778214,123.442760157749)) ;
#14739=CARTESIAN_POINT('Ctrl Pts',(-20.6575861303244,-12.827598841482,123.482884715425)) ;
#14740=CARTESIAN_POINT('Ctrl Pts',(-20.6556047333337,-12.8262772621163,
123.511783798392)) ;
#14741=CARTESIAN_POINT('Ctrl Pts',(-20.6507140711558,-12.8241107008861,
123.559004657467)) ;
#14742=CARTESIAN_POINT('Ctrl Pts',(-20.6483977097181,-12.8232659356874,
123.577376652466)) ;
#14743=CARTESIAN_POINT('Ctrl Pts',(-20.6448453939834,-12.8221626324877,
123.601262802907)) ;
#14744=CARTESIAN_POINT('Ctrl Pts',(-20.6439790072615,-12.8219051452136,
123.606829565049)) ;
#14745=CARTESIAN_POINT('Ctrl Pts',(-20.6418443054908,-12.8212967745573,
123.619960758218)) ;
#14746=CARTESIAN_POINT('Ctrl Pts',(-20.6405439435258,-12.8209457839077,
123.627519741223)) ;
#14747=CARTESIAN_POINT('Ctrl Pts',(-20.6381883339577,-12.8203415746451,
123.64049687)) ;
#14748=CARTESIAN_POINT('Ctrl Pts',(-20.6371666138787,-12.820088541863,123.645920880265)) ;
#14749=CARTESIAN_POINT('Ctrl Pts',(-20.6348819041793,-12.8195414167891,
123.657623135203)) ;
#14750=CARTESIAN_POINT('Ctrl Pts',(-20.6336065260582,-12.8192472270464,
123.663898787321)) ;
#14751=CARTESIAN_POINT('Ctrl Pts',(-20.6272779984606,-12.8178391551606,
123.693857594239)) ;
#14752=CARTESIAN_POINT('Ctrl Pts',(-20.6215855761488,-12.8167219894872,
123.717400325192)) ;
#14753=CARTESIAN_POINT('Ctrl Pts',(-20.609868590585,-12.8146679819657,123.760355363193)) ;
#14754=CARTESIAN_POINT('Ctrl Pts',(-20.60404755338,-12.81373140255,123.77981487948)) ;
#14755=CARTESIAN_POINT('Ctrl Pts',(-20.5944667169948,-12.8123076232002,
123.809214252221)) ;
#14756=CARTESIAN_POINT('Ctrl Pts',(-20.5910500584737,-12.8118194031044,
123.819262284889)) ;
#14757=CARTESIAN_POINT('Ctrl Pts',(-20.5848732477587,-12.8109694296603,
123.83669600002)) ;
#14758=CARTESIAN_POINT('Ctrl Pts',(-20.5821704069237,-12.8106074643119,
123.844101334191)) ;
#14759=CARTESIAN_POINT('Ctrl Pts',(-20.5765619710992,-12.8098759256259,
123.859027595902)) ;
#14760=CARTESIAN_POINT('Ctrl Pts',(-20.5736532958038,-12.8095063835442,
123.866546976148)) ;
#14761=CARTESIAN_POINT('Ctrl Pts',(-20.5671289983014,-12.808698354596,123.882940172802)) ;
#14762=CARTESIAN_POINT('Ctrl Pts',(-20.5634836714251,-12.8082600277093,
123.891801627255)) ;
#14763=CARTESIAN_POINT('Ctrl Pts',(-20.5442239905619,-12.8060090510775,
123.937131641893)) ;
#14764=CARTESIAN_POINT('Ctrl Pts',(-20.5269818522385,-12.8042053158095,
123.972883839771)) ;
#14765=CARTESIAN_POINT('Ctrl Pts',(-20.5037351473603,-12.8019843312899,
124.015746122103)) ;
#14766=CARTESIAN_POINT('Ctrl Pts',(-20.4993143935588,-12.8015701363743,
124.023689128243)) ;
#14767=CARTESIAN_POINT('Ctrl Pts',(-20.4895808701211,-12.8006747773791,
124.040737552588)) ;
#14768=CARTESIAN_POINT('Ctrl Pts',(-20.4842387633027,-12.8001935162605,
124.049825403061)) ;
#14769=CARTESIAN_POINT('Ctrl Pts',(-20.4759764565303,-12.7994633905796,
124.063482603025)) ;
#14770=CARTESIAN_POINT('Ctrl Pts',(-20.4731404129509,-12.7992151917061,
124.068102326436)) ;
#14771=CARTESIAN_POINT('Ctrl Pts',(-20.4667137767816,-12.7986581674899,
124.078419753693)) ;
#14772=CARTESIAN_POINT('Ctrl Pts',(-20.4631070056883,-12.7983492405114,
124.084107183854)) ;
#14773=CARTESIAN_POINT('Ctrl Pts',(-20.4490991301561,-12.7971635698918,
124.105806135454)) ;
#14774=CARTESIAN_POINT('Ctrl Pts',(-20.4383776607561,-12.7962853555577,
124.121607693117)) ;
#14775=CARTESIAN_POINT('Ctrl Pts',(-20.414170942734,-12.7943657812944,124.155582065262)) ;
#14776=CARTESIAN_POINT('Ctrl Pts',(-20.400545607209,-12.7933246556129,124.17364696391)) ;
#14777=CARTESIAN_POINT('Ctrl Pts',(-20.3785548314267,-12.7917035889498,
124.201213523587)) ;
#14778=CARTESIAN_POINT('Ctrl Pts',(-20.3705226732172,-12.7911229375677,
124.210974786593)) ;
#14779=CARTESIAN_POINT('Ctrl Pts',(-20.355315148532,-12.7900442150157,124.228895029304)) ;
#14780=CARTESIAN_POINT('Ctrl Pts',(-20.3481787790495,-12.7895460575861,
124.237085537754)) ;
#14781=CARTESIAN_POINT('Ctrl Pts',(-20.3332879201031,-12.7885225946496,
124.253732790805)) ;
#14782=CARTESIAN_POINT('Ctrl Pts',(-20.3255219236296,-12.7879973835778,
124.262177893759)) ;
#14783=CARTESIAN_POINT('Ctrl Pts',(-20.3003883323565,-12.7863236944491,
124.288765233842)) ;
#14784=CARTESIAN_POINT('Ctrl Pts',(-20.2825897784024,-12.785177190022,124.30649151298)) ;
#14785=CARTESIAN_POINT('Ctrl Pts',(-20.2510111217323,-12.7832012383649,
124.336101102422)) ;
#14786=CARTESIAN_POINT('Ctrl Pts',(-20.2374833845805,-12.7823719214179,
124.348241947181)) ;
#14787=CARTESIAN_POINT('Ctrl Pts',(-20.2173881470175,-12.7811616242106,
124.365500797064)) ;
#14788=CARTESIAN_POINT('Ctrl Pts',(-20.2110266432474,-12.7807815260881,
124.37085503483)) ;
#14789=CARTESIAN_POINT('Ctrl Pts',(-20.2044183990009,-12.7803895702814,
124.376305238775)) ;
#14790=CARTESIAN_POINT('Ctrl Pts',(-20.2042245444069,-12.7803780746881,
124.376465023782)) ;
#14791=CARTESIAN_POINT('Ctrl Pts',(-20.2038946797953,-12.7803585179886,
124.376736748338)) ;
#14792=CARTESIAN_POINT('Ctrl Pts',(-20.2037586943496,-12.780350457055,124.376848717523)) ;
#14793=CARTESIAN_POINT('Ctrl Pts',(-20.2031109720567,-12.7803120673327,
124.377381816493)) ;
#14794=CARTESIAN_POINT('Ctrl Pts',(-20.2025989239471,-12.7802817364031,
124.377802568054)) ;
#14795=CARTESIAN_POINT('Ctrl Pts',(-20.196974407164,-12.7799487620146,124.382416762939)) ;
#14796=CARTESIAN_POINT('Ctrl Pts',(-20.1918290918141,-12.7796458770426,
124.38656997156)) ;
#14797=CARTESIAN_POINT('Ctrl Pts',(-20.1796522912951,-12.7789329269418,
124.396240314173)) ;
#14798=CARTESIAN_POINT('Ctrl Pts',(-20.172594122113,-12.7785226886753,124.401723237862)) ;
#14799=CARTESIAN_POINT('Ctrl Pts',(-20.141547880952,-12.7767316008984,124.425311071857)) ;
#14800=CARTESIAN_POINT('Ctrl Pts',(-20.1169701138398,-12.7753483534963,
124.442623224899)) ;
#14801=CARTESIAN_POINT('Ctrl Pts',(-20.0785151148125,-12.7732373228449,
124.467686109091)) ;
#14802=CARTESIAN_POINT('Ctrl Pts',(-20.0650744502059,-12.7725088934285,
124.476086242062)) ;
#14803=CARTESIAN_POINT('Ctrl Pts',(-20.0410946360899,-12.7712253596146,
124.490446335023)) ;
#14804=CARTESIAN_POINT('Ctrl Pts',(-20.0306218191546,-12.7706700450617,
124.496513018329)) ;
#14805=CARTESIAN_POINT('Ctrl Pts',(-20.0087759546366,-12.7695220855161,
124.508747652244)) ;
#14806=CARTESIAN_POINT('Ctrl Pts',(-19.9973919037328,-12.7689295740919,
124.514893058028)) ;
#14807=CARTESIAN_POINT('Ctrl Pts',(-19.9660925518482,-12.7673150650081,
124.531166976599)) ;
#14808=CARTESIAN_POINT('Ctrl Pts',(-19.945997817985,-12.7662943500498,124.540940038853)) ;
#14809=CARTESIAN_POINT('Ctrl Pts',(-19.9047980069988,-12.7642284240287,
124.559629065831)) ;
#14810=CARTESIAN_POINT('Ctrl Pts',(-19.883688076969,-12.7631836307977,124.568513974081)) ;
#14811=CARTESIAN_POINT('Ctrl Pts',(-19.8535349855995,-12.7617054793112,
124.580240652778)) ;
#14812=CARTESIAN_POINT('Ctrl Pts',(-19.8446853390475,-12.7612733408557,
124.583567244159)) ;
#14813=CARTESIAN_POINT('Ctrl Pts',(-19.8353641904228,-12.76081963052,124.586950894893)) ;
#14814=CARTESIAN_POINT('Ctrl Pts',(-19.8349294694028,-12.7607984736074,
124.587108429124)) ;
#14815=CARTESIAN_POINT('Ctrl Pts',(-19.8341348059984,-12.7607598050446,
124.587395900569)) ;
#14816=CARTESIAN_POINT('Ctrl Pts',(-19.8337748911753,-12.7607422937099,
124.587525913768)) ;
#14817=CARTESIAN_POINT('Ctrl Pts',(-19.8331134295949,-12.760710114946,124.587764512348)) ;
#14818=CARTESIAN_POINT('Ctrl Pts',(-19.8328119006692,-12.7606954477249,
124.587873147072)) ;
#14819=CARTESIAN_POINT('Ctrl Pts',(-19.8322548081753,-12.7606683520074,
124.588073614102)) ;
#14820=CARTESIAN_POINT('Ctrl Pts',(-19.8319992563856,-12.7606559236504,
124.588165479123)) ;
#14821=CARTESIAN_POINT('Ctrl Pts',(-19.8315246761774,-12.7606328452277,
124.588335905231)) ;
#14822=CARTESIAN_POINT('Ctrl Pts',(-19.8313056556935,-12.7606221952567,
124.588414488459)) ;
#14823=CARTESIAN_POINT('Ctrl Pts',(-19.8308968899834,-12.7606023203299,
124.588561022311)) ;
#14824=CARTESIAN_POINT('Ctrl Pts',(-19.830707150122,-12.7605930954353,124.588628988251)) ;
#14825=CARTESIAN_POINT('Ctrl Pts',(-19.8303513303538,-12.7605757970804,
124.588756347906)) ;
#14826=CARTESIAN_POINT('Ctrl Pts',(-19.830185254445,-12.7605677236746,124.588815752311)) ;
#14827=CARTESIAN_POINT('Ctrl Pts',(-19.8298723718533,-12.7605525144503,
124.588927593938)) ;
#14828=CARTESIAN_POINT('Ctrl Pts',(-19.8297255678651,-12.7605453786632,
124.588980038873)) ;
#14829=CARTESIAN_POINT('Ctrl Pts',(-19.8294477615593,-12.76053187584,124.589079225083)) ;
#14830=CARTESIAN_POINT('Ctrl Pts',(-19.8293167612351,-12.7605255088285,
124.589125971961)) ;
#14831=CARTESIAN_POINT('Ctrl Pts',(-19.8290677964725,-12.7605134089227,
124.589214767077)) ;
#14832=CARTESIAN_POINT('Ctrl Pts',(-19.8289498335817,-12.7605076760504,
124.589256819429)) ;
#14833=CARTESIAN_POINT('Ctrl Pts',(-19.8284960393133,-12.7604856229994,
124.589418514769)) ;
#14834=CARTESIAN_POINT('Ctrl Pts',(-19.8281601627657,-12.7604693022374,
124.589538031922)) ;
#14835=CARTESIAN_POINT('Ctrl Pts',(-19.8215533261999,-12.7601483016356,
124.591885802008)) ;
#14836=CARTESIAN_POINT('Ctrl Pts',(-19.8152647384488,-12.7598433916911,
124.594064076999)) ;
#14837=CARTESIAN_POINT('Ctrl Pts',(-19.8000690057879,-12.7591079026105,
124.599192115322)) ;
#14838=CARTESIAN_POINT('Ctrl Pts',(-19.791145477876,-12.7586771055641,124.602092006426)) ;
#14839=CARTESIAN_POINT('Ctrl Pts',(-19.7531986697255,-12.7568503150416,
124.613952974159)) ;
#14840=CARTESIAN_POINT('Ctrl Pts',(-19.7238865152444,-12.7554521746053,
124.621955051919)) ;
#14841=CARTESIAN_POINT('Ctrl Pts',(-19.6808877986279,-12.7534217475114,
124.632025447434)) ;
#14842=CARTESIAN_POINT('Ctrl Pts',(-19.667412410108,-12.7527882655239,124.634947126119)) ;
#14843=CARTESIAN_POINT('Ctrl Pts',(-19.6415240070757,-12.7515764002764,
124.640113254841)) ;
#14844=CARTESIAN_POINT('Ctrl Pts',(-19.629119919105,-12.7509979946013,124.642393921712)) ;
#14845=CARTESIAN_POINT('Ctrl Pts',(-19.605274756875,-12.7498899647433,124.64640614307)) ;
#14846=CARTESIAN_POINT('Ctrl Pts',(-19.5938399686473,-12.7493603118689,
124.648167307998)) ;
#14847=CARTESIAN_POINT('Ctrl Pts',(-19.558082345876,-12.7477085470678,124.653167494658)) ;
#14848=CARTESIAN_POINT('Ctrl Pts',(-19.5336875014784,-12.7465882481635,
124.655849287354)) ;
#14849=CARTESIAN_POINT('Ctrl Pts',(-19.4945147079598,-12.744794221295,124.65899183605)) ;
#14850=CARTESIAN_POINT('Ctrl Pts',(-19.4797801406896,-12.7441204923527,
124.659911539982)) ;
#14851=CARTESIAN_POINT('Ctrl Pts',(-19.4580664522149,-12.7431277471803,
124.660881118485)) ;
#14852=CARTESIAN_POINT('Ctrl Pts',(-19.4510976689019,-12.7428091483195,
124.66113388505)) ;
#14853=CARTESIAN_POINT('Ctrl Pts',(-19.4395253783455,-12.7422799063551,
124.66145669146)) ;
#14854=CARTESIAN_POINT('Ctrl Pts',(-19.4349229434507,-12.7420693732442,
124.661559634178)) ;
#14855=CARTESIAN_POINT('Ctrl Pts',(-19.4300767291584,-12.7418476000308,
124.66164124752)) ;
#14856=CARTESIAN_POINT('Ctrl Pts',(-19.4298334076449,-12.7418364648781,
124.661645274134)) ;
#14857=CARTESIAN_POINT('Ctrl Pts',(-19.4293707042464,-12.7418152896658,
124.661652796038)) ;
#14858=CARTESIAN_POINT('Ctrl Pts',(-19.4291513226569,-12.7418052496651,
124.661656304622)) ;
#14859=CARTESIAN_POINT('Ctrl Pts',(-19.4287335909311,-12.7417861317869,
124.661662875421)) ;
#14860=CARTESIAN_POINT('Ctrl Pts',(-19.4285352409226,-12.7417770539518,
124.66166594818)) ;
#14861=CARTESIAN_POINT('Ctrl Pts',(-19.4281570631425,-12.7417597456665,
124.661671716714)) ;
#14862=CARTESIAN_POINT('Ctrl Pts',(-19.4279772354914,-12.7417515152514,
124.661674420896)) ;
#14863=CARTESIAN_POINT('Ctrl Pts',(-19.427633933676,-12.7417358026273,124.661679509234)) ;
#14864=CARTESIAN_POINT('Ctrl Pts',(-19.4274704595811,-12.7417283204457,
124.66168190013)) ;
#14865=CARTESIAN_POINT('Ctrl Pts',(-19.4271579868272,-12.7417140183976,
124.661686408894)) ;
#14866=CARTESIAN_POINT('Ctrl Pts',(-19.4270089881829,-12.7417071985514,
124.661688532191)) ;
#14867=CARTESIAN_POINT('Ctrl Pts',(-19.4267238362295,-12.7416941466172,
124.661692544734)) ;
#14868=CARTESIAN_POINT('Ctrl Pts',(-19.4265876831022,-12.7416879145538,
124.661694438374)) ;
#14869=CARTESIAN_POINT('Ctrl Pts',(-19.4263268050373,-12.741675973364,124.661698024073)) ;
#14870=CARTESIAN_POINT('Ctrl Pts',(-19.4262020801381,-12.7416702642528,
124.661699719711)) ;
#14871=CARTESIAN_POINT('Ctrl Pts',(-19.4259628233202,-12.7416593124649,
124.661702936593)) ;
#14872=CARTESIAN_POINT('Ctrl Pts',(-19.4258482914266,-12.7416540698004,
124.661704460765)) ;
#14873=CARTESIAN_POINT('Ctrl Pts',(-19.425628341563,-12.7416440015434,124.661707357584)) ;
#14874=CARTESIAN_POINT('Ctrl Pts',(-19.4255229236269,-12.7416391759616,
124.661708732637)) ;
#14875=CARTESIAN_POINT('Ctrl Pts',(-19.4253202574757,-12.7416298986742,
124.661711350535)) ;
#14876=CARTESIAN_POINT('Ctrl Pts',(-19.4252230090526,-12.7416254469667,
124.66171259537)) ;
#14877=CARTESIAN_POINT('Ctrl Pts',(-19.4250358524253,-12.7416168794777,
124.661714969235)) ;
#14878=CARTESIAN_POINT('Ctrl Pts',(-19.424945944365,-12.7416127637092,124.661716099912)) ;
#14879=CARTESIAN_POINT('Ctrl Pts',(-19.4247727398005,-12.7416048347597,
124.661718259428)) ;
#14880=CARTESIAN_POINT('Ctrl Pts',(-19.424689443183,-12.741601021579,124.661719289643)) ;
#14881=CARTESIAN_POINT('Ctrl Pts',(-19.4245288178724,-12.741593668356,124.661721260203)) ;
#14882=CARTESIAN_POINT('Ctrl Pts',(-19.4244514894822,-12.7415901283321,
124.661722201694)) ;
#14883=CARTESIAN_POINT('Ctrl Pts',(-19.4241944601864,-12.7415783616686,
124.66172530723)) ;
#14884=CARTESIAN_POINT('Ctrl Pts',(-19.4240147584981,-12.7415701348681,
124.661727439703)) ;
#14885=CARTESIAN_POINT('Ctrl Pts',(-19.4236605694096,-12.7415539196717,
124.661731566376)) ;
#14886=CARTESIAN_POINT('Ctrl Pts',(-19.4234860822174,-12.7415459312944,
124.661733562792)) ;
#14887=CARTESIAN_POINT('Ctrl Pts',(-19.4231419025592,-12.7415301737581,
124.661737428686)) ;
#14888=CARTESIAN_POINT('Ctrl Pts',(-19.4229722100233,-12.7415224046041,
124.661739300144)) ;
#14889=CARTESIAN_POINT('Ctrl Pts',(-19.4226372151494,-12.7415070670136,
124.661742926417)) ;
#14890=CARTESIAN_POINT('Ctrl Pts',(-19.4224719129676,-12.7414994985916,
124.661744682994)) ;
#14891=CARTESIAN_POINT('Ctrl Pts',(-19.4221453083585,-12.7414845446067,
124.661748088849)) ;
#14892=CARTESIAN_POINT('Ctrl Pts',(-19.4219840059091,-12.7414771590492,
124.661749739694)) ;
#14893=CARTESIAN_POINT('Ctrl Pts',(-19.4216650210744,-12.7414625534245,
124.661752942583)) ;
#14894=CARTESIAN_POINT('Ctrl Pts',(-19.4215073385547,-12.7414553333568,
124.661754496013)) ;
#14895=CARTESIAN_POINT('Ctrl Pts',(-19.4211952222683,-12.7414410417241,
124.661757511801)) ;
#14896=CARTESIAN_POINT('Ctrl Pts',(-19.4210407887336,-12.7414339701748,
124.661758975374)) ;
#14897=CARTESIAN_POINT('Ctrl Pts',(-19.4207348053506,-12.7414199588746,
124.661761818479)) ;
#14898=CARTESIAN_POINT('Ctrl Pts',(-19.4205832554236,-12.7414130191247,
124.66176319907)) ;
#14899=CARTESIAN_POINT('Ctrl Pts',(-19.4202826773881,-12.7413992548634,
124.66176588261)) ;
#14900=CARTESIAN_POINT('Ctrl Pts',(-19.4201336493401,-12.7413924303588,
124.661767186468)) ;
#14901=CARTESIAN_POINT('Ctrl Pts',(-19.4198377534698,-12.7413788800386,
124.661769722362)) ;
#14902=CARTESIAN_POINT('Ctrl Pts',(-19.4196908856624,-12.7413721542271,
124.661770955165)) ;
#14903=CARTESIAN_POINT('Ctrl Pts',(-19.4193989456822,-12.7413587846041,
124.661773354241)) ;
#14904=CARTESIAN_POINT('Ctrl Pts',(-19.4192538736498,-12.7413521408019,
124.661774521142)) ;
#14905=CARTESIAN_POINT('Ctrl Pts',(-19.4189651541696,-12.7413389182103,
124.661776793219)) ;
#14906=CARTESIAN_POINT('Ctrl Pts',(-19.4188215066021,-12.7413323394177,
124.661777898889)) ;
#14907=CARTESIAN_POINT('Ctrl Pts',(-19.4185352540363,-12.7413192293539,
124.661780052857)) ;
#14908=CARTESIAN_POINT('Ctrl Pts',(-19.4183926490306,-12.741312698084,124.661781101513)) ;
#14909=CARTESIAN_POINT('Ctrl Pts',(-19.4181080838835,-12.7412996648531,
124.661783145383)) ;
#14910=CARTESIAN_POINT('Ctrl Pts',(-19.4179661234659,-12.7412931628804,
124.661784140819)) ;
#14911=CARTESIAN_POINT('Ctrl Pts',(-19.4176824277518,-12.7412801690196,
124.66178608178)) ;
#14912=CARTESIAN_POINT('Ctrl Pts',(-19.4175406926215,-12.7412736771395,
124.661787027381)) ;
#14913=CARTESIAN_POINT('Ctrl Pts',(-19.4172569990523,-12.7412606829228,
124.661788871819)) ;
#14914=CARTESIAN_POINT('Ctrl Pts',(-19.4171150405906,-12.7412541805848,
124.66178977058)) ;
#14915=CARTESIAN_POINT('Ctrl Pts',(-19.4168304142005,-12.7412411431805,
124.661791524104)) ;
#14916=CARTESIAN_POINT('Ctrl Pts',(-19.4166877464522,-12.7412346081213,
124.661792378625)) ;
#14917=CARTESIAN_POINT('Ctrl Pts',(-19.4164011667507,-12.7412214807738,
124.661794046052)) ;
#14918=CARTESIAN_POINT('Ctrl Pts',(-19.4162572546592,-12.7412148884771,
124.661794858532)) ;
#14919=CARTESIAN_POINT('Ctrl Pts',(-19.4159675882246,-12.7412016192506,
124.661796443867)) ;
#14920=CARTESIAN_POINT('Ctrl Pts',(-19.4158218341684,-12.7411949423307,
124.66179721608)) ;
#14921=CARTESIAN_POINT('Ctrl Pts',(-19.415527804632,-12.7411814727326,124.661798722435)) ;
#14922=CARTESIAN_POINT('Ctrl Pts',(-19.4153795288802,-12.7411746800376,
124.661799455689)) ;
#14923=CARTESIAN_POINT('Ctrl Pts',(-19.4150796704779,-12.7411609428892,
124.661800885195)) ;
#14924=CARTESIAN_POINT('Ctrl Pts',(-19.4149280877281,-12.7411539984253,
124.661801580257)) ;
#14925=CARTESIAN_POINT('Ctrl Pts',(-19.4146764267807,-12.7411424688468,
124.661802688435)) ;
#14926=CARTESIAN_POINT('Ctrl Pts',(-19.4145763486713,-12.7411378838144,
124.661803117106)) ;
#14927=CARTESIAN_POINT('Ctrl Pts',(-19.4143577102211,-12.7411278668618,
124.661804027355)) ;
#14928=CARTESIAN_POINT('Ctrl Pts',(-19.4142391500948,-12.741122434927,124.661804504084)) ;
#14929=CARTESIAN_POINT('Ctrl Pts',(-19.4139767884034,-12.7411104144087,
124.661805521709)) ;
#14930=CARTESIAN_POINT('Ctrl Pts',(-19.4138329867694,-12.7411038257816,
124.661806054659)) ;
#14931=CARTESIAN_POINT('Ctrl Pts',(-19.4135090098818,-12.7410889816924,
124.661807199458)) ;
#14932=CARTESIAN_POINT('Ctrl Pts',(-19.4133288346815,-12.7410807261601,
124.661807797165)) ;
#14933=CARTESIAN_POINT('Ctrl Pts',(-19.4129116967387,-12.7410616126508,
124.661809090774)) ;
#14934=CARTESIAN_POINT('Ctrl Pts',(-19.4126747338643,-12.7410507545197,
124.66180975825)) ;
#14935=CARTESIAN_POINT('Ctrl Pts',(-19.4122186413849,-12.7410298547295,
124.661810913275)) ;
#14936=CARTESIAN_POINT('Ctrl Pts',(-19.4119995118601,-12.7410198131256,
124.661811410585)) ;
#14937=CARTESIAN_POINT('Ctrl Pts',(-19.4061760536978,-12.7407529451198,
124.661823095476)) ;
#14938=CARTESIAN_POINT('Ctrl Pts',(-19.4005717232996,-12.7404959171753,
124.661796650256)) ;
#14939=CARTESIAN_POINT('Ctrl Pts',(-19.3885371437218,-12.7399433916313,
124.661658922666)) ;
#14940=CARTESIAN_POINT('Ctrl Pts',(-19.3821072100128,-12.7396477965462,
124.661535703254)) ;
#14941=CARTESIAN_POINT('Ctrl Pts',(-19.3561057532977,-12.7384508484387,
124.660836662306)) ;
#14942=CARTESIAN_POINT('Ctrl Pts',(-19.3365481209036,-12.7375470829579,
124.659850651173)) ;
#14943=CARTESIAN_POINT('Ctrl Pts',(-19.2991144258305,-12.7358134425116,
124.657080477771)) ;
#14944=CARTESIAN_POINT('Ctrl Pts',(-19.2812376495889,-12.7349838439677,
124.655369583169)) ;
#14945=CARTESIAN_POINT('Ctrl Pts',(-19.2491038960038,-12.7334905955723,
124.651593950738)) ;
#14946=CARTESIAN_POINT('Ctrl Pts',(-19.2348339142787,-12.7328267349061,
124.64966677643)) ;
#14947=CARTESIAN_POINT('Ctrl Pts',(-19.21213017858,-12.7317693899077,124.64620021637)) ;
#14948=CARTESIAN_POINT('Ctrl Pts',(-19.2036734814637,-12.7313752928506,
124.644819869289)) ;
#14949=CARTESIAN_POINT('Ctrl Pts',(-19.1886329593461,-12.730673860828,124.642205835725)) ;
#14950=CARTESIAN_POINT('Ctrl Pts',(-19.1820436026388,-12.7303663803995,
124.641005973387)) ;
#14951=CARTESIAN_POINT('Ctrl Pts',(-19.1691632151487,-12.7297649357601,
124.638553458616)) ;
#14952=CARTESIAN_POINT('Ctrl Pts',(-19.1628715512888,-12.7294709590662,
124.637305225249)) ;
#14953=CARTESIAN_POINT('Ctrl Pts',(-19.148524178448,-12.7288000686123,124.634343824607)) ;
#14954=CARTESIAN_POINT('Ctrl Pts',(-19.1404752266585,-12.7284233258926,
124.63259935732)) ;
#14955=CARTESIAN_POINT('Ctrl Pts',(-19.1158282873605,-12.7272682641916,
124.627001995282)) ;
#14956=CARTESIAN_POINT('Ctrl Pts',(-19.0992913261169,-12.7264913056927,
124.622889163484)) ;
#14957=CARTESIAN_POINT('Ctrl Pts',(-19.0511034112341,-12.7242180712362,
124.60985287223)) ;
#14958=CARTESIAN_POINT('Ctrl Pts',(-19.019714466083,-12.7227259025544,124.600017173422)) ;
#14959=CARTESIAN_POINT('Ctrl Pts',(-18.9795197956115,-12.7207832260973,
124.58565801372)) ;
#14960=CARTESIAN_POINT('Ctrl Pts',(-18.9703287956385,-12.7203367556637,
124.582252200529)) ;
#14961=CARTESIAN_POINT('Ctrl Pts',(-18.9518947179989,-12.7194358270147,
124.575173601909)) ;
#14962=CARTESIAN_POINT('Ctrl Pts',(-18.9426535103517,-12.7189813740649,
124.571497887254)) ;
#14963=CARTESIAN_POINT('Ctrl Pts',(-18.9252874242451,-12.7181222055062,
124.564349293078)) ;
#14964=CARTESIAN_POINT('Ctrl Pts',(-18.9171535661215,-12.7177176241507,
124.560899772032)) ;
#14965=CARTESIAN_POINT('Ctrl Pts',(-18.8835970301816,-12.716039662397,124.54624699214)) ;
#14966=CARTESIAN_POINT('Ctrl Pts',(-18.8585148236061,-12.7147643904582,
124.534283997291)) ;
#14967=CARTESIAN_POINT('Ctrl Pts',(-18.8118708653506,-12.7123525971582,
124.5100969806)) ;
#14968=CARTESIAN_POINT('Ctrl Pts',(-18.7902330855619,-12.7112165713594,
124.498048057546)) ;
#14969=CARTESIAN_POINT('Ctrl Pts',(-18.7293221041502,-12.7079650224653,
124.461718506287)) ;
#14970=CARTESIAN_POINT('Ctrl Pts',(-18.6910169953789,-12.7058549056396,
124.435894588803)) ;
#14971=CARTESIAN_POINT('Ctrl Pts',(-18.6491946069308,-12.7034521432387,
124.404196293759)) ;
#14972=CARTESIAN_POINT('Ctrl Pts',(-18.6441900359713,-12.70316290484,124.400343131319)) ;
#14973=CARTESIAN_POINT('Ctrl Pts',(-18.6311498776929,-12.7024045372778,
124.390144793104)) ;
#14974=CARTESIAN_POINT('Ctrl Pts',(-18.6231626798287,-12.7019352791285,
124.383738536986)) ;
#14975=CARTESIAN_POINT('Ctrl Pts',(-18.6079519929447,-12.7010317731049,
124.371228396891)) ;
#14976=CARTESIAN_POINT('Ctrl Pts',(-18.6007172912797,-12.7005976199917,
124.365139239889)) ;
#14977=CARTESIAN_POINT('Ctrl Pts',(-18.5673897488739,-12.6985755979616,
124.336436483005)) ;
#14978=CARTESIAN_POINT('Ctrl Pts',(-18.5421720173711,-12.6969815299611,
124.312830112949)) ;
#14979=CARTESIAN_POINT('Ctrl Pts',(-18.506446813958,-12.694631909931,124.276497027065)) ;
#14980=CARTESIAN_POINT('Ctrl Pts',(-18.4951615683014,-12.6938750055421,
124.264557901108)) ;
#14981=CARTESIAN_POINT('Ctrl Pts',(-18.4774842918996,-12.6926653854845,
124.245102101226)) ;
#14982=CARTESIAN_POINT('Ctrl Pts',(-18.4709402613766,-12.6922120640712,
124.237726182475)) ;
#14983=CARTESIAN_POINT('Ctrl Pts',(-18.459214622211,-12.6913895174003,124.224190695924)) ;
#14984=CARTESIAN_POINT('Ctrl Pts',(-18.4540039325131,-12.691020166777,124.218057034019)) ;
#14985=CARTESIAN_POINT('Ctrl Pts',(-18.4451026932765,-12.6903824405403,
124.207371669837)) ;
#14986=CARTESIAN_POINT('Ctrl Pts',(-18.441384248471,-12.6901139305891,124.202843552928)) ;
#14987=CARTESIAN_POINT('Ctrl Pts',(-18.4313015562118,-12.6893799792537,
124.190387867465)) ;
#14988=CARTESIAN_POINT('Ctrl Pts',(-18.4250019569179,-12.6889148889622,
124.182408530454)) ;
#14989=CARTESIAN_POINT('Ctrl Pts',(-18.4041484103778,-12.6873524172539,
124.15532158167)) ;
#14990=CARTESIAN_POINT('Ctrl Pts',(-18.3900479733075,-12.686257440072,124.135871542147)) ;
#14991=CARTESIAN_POINT('Ctrl Pts',(-18.3619657477377,-12.6839864835463,
124.094687868424)) ;
#14992=CARTESIAN_POINT('Ctrl Pts',(-18.348079780465,-12.6828111822156,124.072902611342)) ;
#14993=CARTESIAN_POINT('Ctrl Pts',(-18.3294714797503,-12.6811501530786,
124.041609770132)) ;
#14994=CARTESIAN_POINT('Ctrl Pts',(-18.3241799145749,-12.6806670205677,
124.032448378074)) ;
#14995=CARTESIAN_POINT('Ctrl Pts',(-18.3170899769716,-12.6800038847141,
124.019805523438)) ;
#14996=CARTESIAN_POINT('Ctrl Pts',(-18.3151907173501,-12.679824621286,124.016381124012)) ;
#14997=CARTESIAN_POINT('Ctrl Pts',(-18.3132919922828,-12.6796437647429,
124.012919437755)) ;
#14998=CARTESIAN_POINT('Ctrl Pts',(-18.3132764027887,-12.6796422797065,
124.012891012935)) ;
#14999=CARTESIAN_POINT('Ctrl Pts',(-18.313245064012,-12.6796392941861,124.012833866677)) ;
#15000=CARTESIAN_POINT('Ctrl Pts',(-18.3132293149034,-12.6796377937163,
124.0128051455)) ;
#15001=CARTESIAN_POINT('Ctrl Pts',(-18.3131976531155,-12.6796347769618,
124.012747399463)) ;
#15002=CARTESIAN_POINT('Ctrl Pts',(-18.3131817403595,-12.6796332606672,
124.012718374406)) ;
#15003=CARTESIAN_POINT('Ctrl Pts',(-18.309928903321,-12.6793232803598,124.00678460178)) ;
#15004=CARTESIAN_POINT('Ctrl Pts',(-18.3067397500352,-12.6790145106252,
124.000853805789)) ;
#15005=CARTESIAN_POINT('Ctrl Pts',(-18.2965035192995,-12.6780075326363,
123.981443316685)) ;
#15006=CARTESIAN_POINT('Ctrl Pts',(-18.2896545366928,-12.6773084808496,
123.967860734372)) ;
#15007=CARTESIAN_POINT('Ctrl Pts',(-18.2727067620015,-12.6755123331438,
123.932667321939)) ;
#15008=CARTESIAN_POINT('Ctrl Pts',(-18.2629755326819,-12.6744151479685,
123.910886252887)) ;
#15009=CARTESIAN_POINT('Ctrl Pts',(-18.2488486181997,-12.6727140219334,
123.87666961053)) ;
#15010=CARTESIAN_POINT('Ctrl Pts',(-18.2440164172915,-12.6721093732509,
123.864420430033)) ;
#15011=CARTESIAN_POINT('Ctrl Pts',(-18.2352505607384,-12.6709674769033,
123.841128311431)) ;
#15012=CARTESIAN_POINT('Ctrl Pts',(-18.2312769522516,-12.6704301796671,
123.830101910755)) ;
#15013=CARTESIAN_POINT('Ctrl Pts',(-18.2271859813095,-12.6698549070907,
123.818228919656)) ;
#15014=CARTESIAN_POINT('Ctrl Pts',(-18.2269137742071,-12.6698165194887,
123.817436321487)) ;
#15015=CARTESIAN_POINT('Ctrl Pts',(-18.2266423654705,-12.6697781342469,
123.816643453362)) ;
#15016=CARTESIAN_POINT('Origin',(-19.4092722359532,-13.9601742359176,123.411814366564)) ;
#15017=CARTESIAN_POINT('',(-18.2266423654684,-12.3098085062257,123.816643453356)) ;
#15018=CARTESIAN_POINT('',(-18.2266423654683,-12.3699164408135,123.816643453356)) ;
#15019=CARTESIAN_POINT('',(-18.2266423654683,-13.9601742359176,123.816643453356)) ;
#15020=CARTESIAN_POINT('',(-20.4795958874297,-12.1420202715133,122.766130804778)) ;
#15021=CARTESIAN_POINT('Ctrl Pts',(-18.2266423654683,-12.3098085062256,
123.816643453356)) ;
#15022=CARTESIAN_POINT('Ctrl Pts',(-18.2071382676369,-12.307033814287,123.759666004243)) ;
#15023=CARTESIAN_POINT('Ctrl Pts',(-18.1917772261847,-12.3042925781088,
123.701353432471)) ;
#15024=CARTESIAN_POINT('Ctrl Pts',(-18.1806792743743,-12.3015413901064,
123.642160486207)) ;
#15025=CARTESIAN_POINT('Ctrl Pts',(-18.1672798095677,-12.2982196558401,
123.570692001408)) ;
#15026=CARTESIAN_POINT('Ctrl Pts',(-18.1601420106916,-12.2948828760311,
123.498190812995)) ;
#15027=CARTESIAN_POINT('Ctrl Pts',(-18.1593469593498,-12.2915492218341,
123.425481955367)) ;
#15028=CARTESIAN_POINT('Ctrl Pts',(-18.1585560485259,-12.2882329288491,
123.353151755455)) ;
#15029=CARTESIAN_POINT('Ctrl Pts',(-18.1640449721141,-12.2849230192802,
123.280889352721)) ;
#15030=CARTESIAN_POINT('Ctrl Pts',(-18.1757519544758,-12.2816088917125,
123.209508372437)) ;
#15031=CARTESIAN_POINT('Ctrl Pts',(-18.1874753869865,-12.2782901072751,
123.138027090665)) ;
#15032=CARTESIAN_POINT('Ctrl Pts',(-18.2053899848115,-12.2749858874049,
123.067700353702)) ;
#15033=CARTESIAN_POINT('Ctrl Pts',(-18.2292933016391,-12.271654511838,122.999322288276)) ;
#15034=CARTESIAN_POINT('Ctrl Pts',(-18.2457003206291,-12.2693678859867,
122.952388206866)) ;
#15035=CARTESIAN_POINT('Ctrl Pts',(-18.2648929858744,-12.2670763569669,
122.906474685123)) ;
#15036=CARTESIAN_POINT('Ctrl Pts',(-18.2867692424075,-12.2648035518453,
122.861826158003)) ;
#15037=CARTESIAN_POINT('Ctrl Pts',(-18.2967949115885,-12.2637619480304,
122.841364185377)) ;
#15038=CARTESIAN_POINT('Ctrl Pts',(-18.3073782405547,-12.2627238792631,
122.821180099074)) ;
#15039=CARTESIAN_POINT('Ctrl Pts',(-18.3185073894126,-12.2616864052147,
122.801296512913)) ;
#15040=CARTESIAN_POINT('Ctrl Pts',(-18.3538031655938,-12.2583960860471,
122.738236290088)) ;
#15041=CARTESIAN_POINT('Ctrl Pts',(-18.3944999698131,-12.2550939574768,
122.678357271757)) ;
#15042=CARTESIAN_POINT('Ctrl Pts',(-18.4401408613266,-12.251755308735,122.622330751288)) ;
#15043=CARTESIAN_POINT('Ctrl Pts',(-18.4860923063305,-12.2483939428861,
122.565923010581)) ;
#15044=CARTESIAN_POINT('Ctrl Pts',(-18.5368805148624,-12.2450746925093,
122.51363490565)) ;
#15045=CARTESIAN_POINT('Ctrl Pts',(-18.5919290849859,-12.2417567353599,
122.466060607046)) ;
#15046=CARTESIAN_POINT('Ctrl Pts',(-18.6467053236761,-12.2384551925155,
122.418721663818)) ;
#15047=CARTESIAN_POINT('Ctrl Pts',(-18.7054903794304,-12.2351249633638,
122.376231244306)) ;
#15048=CARTESIAN_POINT('Ctrl Pts',(-18.7676211251744,-12.2318073394179,
122.339068426412)) ;
#15049=CARTESIAN_POINT('Ctrl Pts',(-18.8296626744797,-12.2284944783352,
122.301958960381)) ;
#15050=CARTESIAN_POINT('Ctrl Pts',(-18.8948062425277,-12.2251977295908,
122.270301806749)) ;
#15051=CARTESIAN_POINT('Ctrl Pts',(-18.9623192834267,-12.2218722717631,
122.244452786631)) ;
#15052=CARTESIAN_POINT('Ctrl Pts',(-18.9762682192872,-12.2211851956467,
122.239112095131)) ;
#15053=CARTESIAN_POINT('Ctrl Pts',(-18.9903117626875,-12.2204976817919,
122.234021847498)) ;
#15054=CARTESIAN_POINT('Ctrl Pts',(-19.0044431491614,-12.2198107912305,
122.229184496079)) ;
#15055=CARTESIAN_POINT('Ctrl Pts',(-19.0591252903551,-12.2171528321739,
122.210466111033)) ;
#15056=CARTESIAN_POINT('Ctrl Pts',(-19.1150398834128,-12.2145206077749,
122.19556279089)) ;
#15057=CARTESIAN_POINT('Ctrl Pts',(-19.171784845047,-12.2118736008468,122.184581813526)) ;
#15058=CARTESIAN_POINT('Ctrl Pts',(-19.2429017173703,-12.2085561811443,
122.170819661915)) ;
#15059=CARTESIAN_POINT('Ctrl Pts',(-19.3150804375643,-12.2052211939969,
122.163265203702)) ;
#15060=CARTESIAN_POINT('Ctrl Pts',(-19.3875063718663,-12.2019188342252,
122.162003882036)) ;
#15061=CARTESIAN_POINT('Ctrl Pts',(-19.4595412383739,-12.1986343057257,
122.160749370946)) ;
#15062=CARTESIAN_POINT('Ctrl Pts',(-19.5315476603163,-12.1953483824408,
122.165724878648)) ;
#15063=CARTESIAN_POINT('Ctrl Pts',(-19.6027233506959,-12.1920179074264,
122.176874422162)) ;
#15064=CARTESIAN_POINT('Ctrl Pts',(-19.6746028384665,-12.1886545001058,
122.188134214267)) ;
#15065=CARTESIAN_POINT('Ctrl Pts',(-19.7453616842655,-12.1853369611187,
122.205647863526)) ;
#15066=CARTESIAN_POINT('Ctrl Pts',(-19.8141965675247,-12.1820193804115,
122.229217103851)) ;
#15067=CARTESIAN_POINT('Ctrl Pts',(-19.8637631275544,-12.1796304599181,
122.246188820953)) ;
#15068=CARTESIAN_POINT('Ctrl Pts',(-19.912213297844,-12.1772230759955,122.266259874658)) ;
#15069=CARTESIAN_POINT('Ctrl Pts',(-19.9592604445148,-12.1748180670287,
122.289311373019)) ;
#15070=CARTESIAN_POINT('Ctrl Pts',(-19.9773014805228,-12.1738958250558,
122.29815086577)) ;
#15071=CARTESIAN_POINT('Ctrl Pts',(-19.9951268470279,-12.1729744116093,
122.307424039078)) ;
#15072=CARTESIAN_POINT('Ctrl Pts',(-20.0127210039351,-12.1720549235839,
122.317122818914)) ;
#15073=CARTESIAN_POINT('Ctrl Pts',(-20.0761584828758,-12.1687396182497,
122.352092732213)) ;
#15074=CARTESIAN_POINT('Ctrl Pts',(-20.1364353178746,-12.1654485820723,
122.39251026949)) ;
#15075=CARTESIAN_POINT('Ctrl Pts',(-20.1928714724686,-12.1621004922349,
122.437918973512)) ;
#15076=CARTESIAN_POINT('Ctrl Pts',(-20.2495200548409,-12.1587398000631,
122.48349859758)) ;
#15077=CARTESIAN_POINT('Ctrl Pts',(-20.3020832139595,-12.1553990858244,
122.533933057542)) ;
#15078=CARTESIAN_POINT('Ctrl Pts',(-20.349966190867,-12.152108722025,122.588652849446)) ;
#15079=CARTESIAN_POINT('Ctrl Pts',(-20.3974426337882,-12.1488462939305,
122.642908061732)) ;
#15080=CARTESIAN_POINT('Ctrl Pts',(-20.4401335679279,-12.1455431186542,
122.701165344678)) ;
#15081=CARTESIAN_POINT('Ctrl Pts',(-20.4775654001596,-12.1422019500507,
122.762776836536)) ;
#15082=CARTESIAN_POINT('Ctrl Pts',(-20.4782440081759,-12.1421413774401,
122.76389380169)) ;
#15083=CARTESIAN_POINT('Ctrl Pts',(-20.4789208411427,-12.1420808251965,
122.765011792716)) ;
#15084=CARTESIAN_POINT('Ctrl Pts',(-20.4795958968043,-12.1420202930341,
122.766130805631)) ;
#15085=CARTESIAN_POINT('',(-20.5005106396601,-12.2002211326089,122.802143425663)) ;
#15086=CARTESIAN_POINT('Ctrl Pts',(-20.5005103834412,-12.2002204255305,
122.802142893111)) ;
#15087=CARTESIAN_POINT('Ctrl Pts',(-20.4926703724558,-12.1825726976742,
122.788110222342)) ;
#15088=CARTESIAN_POINT('Ctrl Pts',(-20.4855685242308,-12.1630483237294,
122.776031389631)) ;
#15089=CARTESIAN_POINT('Ctrl Pts',(-20.4795958968858,-12.1420202930341,
122.766130805581)) ;
#15090=CARTESIAN_POINT('Ctrl Pts',(-20.5005103834412,-12.2002204255305,
122.802142893111)) ;
#15091=CARTESIAN_POINT('Ctrl Pts',(-20.4980414512689,-12.2004500404988,
122.797723803343)) ;
#15092=CARTESIAN_POINT('Ctrl Pts',(-20.495545380739,-12.2006795489797,122.793319183576)) ;
#15093=CARTESIAN_POINT('Ctrl Pts',(-20.4930223283398,-12.2009089649636,
122.788929355244)) ;
#15094=CARTESIAN_POINT('Ctrl Pts',(-20.4570110484069,-12.2041833968457,
122.726273765135)) ;
#15095=CARTESIAN_POINT('Ctrl Pts',(-20.4156352266409,-12.207512021703,122.666860836852)) ;
#15096=CARTESIAN_POINT('Ctrl Pts',(-20.3693591437261,-12.210839025915,122.61135629171)) ;
#15097=CARTESIAN_POINT('Ctrl Pts',(-20.3230162773553,-12.2141708315023,
122.555771645032)) ;
#15098=CARTESIAN_POINT('Ctrl Pts',(-20.271932289558,-12.2174515742627,122.504317235034)) ;
#15099=CARTESIAN_POINT('Ctrl Pts',(-20.2167075184025,-12.2207696513077,
122.457587839616)) ;
#15100=CARTESIAN_POINT('Ctrl Pts',(-20.1381326067292,-12.2254906778559,
122.391100318877)) ;
#15101=CARTESIAN_POINT('Ctrl Pts',(-20.0516694314546,-12.2302432845576,
122.334585724807)) ;
#15102=CARTESIAN_POINT('Ctrl Pts',(-19.9592320193965,-12.2349405707703,
122.289297446126)) ;
#15103=CARTESIAN_POINT('Ctrl Pts',(-19.9214262417386,-12.2368617037207,
122.27077509077)) ;
#15104=CARTESIAN_POINT('Ctrl Pts',(-19.8826793167483,-12.2387770175723,
122.254163964086)) ;
#15105=CARTESIAN_POINT('Ctrl Pts',(-19.8432390345038,-12.2407017030626,
122.239563191333)) ;
#15106=CARTESIAN_POINT('Ctrl Pts',(-19.7572792109858,-12.244896541833,122.207740907675)) ;
#15107=CARTESIAN_POINT('Ctrl Pts',(-19.6682620386448,-12.2490797655514,
122.185533907236)) ;
#15108=CARTESIAN_POINT('Ctrl Pts',(-19.577774796042,-12.2532634090411,122.173223680615)) ;
#15109=CARTESIAN_POINT('Ctrl Pts',(-19.5248777586114,-12.2557090835903,
122.166027367637)) ;
#15110=CARTESIAN_POINT('Ctrl Pts',(-19.4714765234977,-12.2581549015896,
122.162213503222)) ;
#15111=CARTESIAN_POINT('Ctrl Pts',(-19.4178896361136,-12.260603267245,122.161844070721)) ;
#15112=CARTESIAN_POINT('Ctrl Pts',(-19.3453693064356,-12.2639166950848,
122.16134410948)) ;
#15113=CARTESIAN_POINT('Ctrl Pts',(-19.2728507009386,-12.2672457315864,
122.167160940948)) ;
#15114=CARTESIAN_POINT('Ctrl Pts',(-19.2012479947592,-12.2705914932778,
122.17924553881)) ;
#15115=CARTESIAN_POINT('Ctrl Pts',(-19.1344032274444,-12.2737149319533,
122.190527125432)) ;
#15116=CARTESIAN_POINT('Ctrl Pts',(-19.0685839173307,-12.2768197584562,
122.207228164016)) ;
#15117=CARTESIAN_POINT('Ctrl Pts',(-19.004440839025,-12.2799106019281,122.229185286871)) ;
#15118=CARTESIAN_POINT('Ctrl Pts',(-18.9997562439645,-12.2801363371195,
122.230788892934)) ;
#15119=CARTESIAN_POINT('Ctrl Pts',(-18.9950786111294,-12.2803622331698,
122.232421236984)) ;
#15120=CARTESIAN_POINT('Ctrl Pts',(-18.990413797334,-12.2805880872903,122.234080267341)) ;
#15121=CARTESIAN_POINT('Ctrl Pts',(-18.9223714524588,-12.2838824618636,
122.258279371666)) ;
#15122=CARTESIAN_POINT('Ctrl Pts',(-18.8565569035649,-12.2872058584351,
122.288328386266)) ;
#15123=CARTESIAN_POINT('Ctrl Pts',(-18.7937055044243,-12.2905106869698,
122.323890840249)) ;
#15124=CARTESIAN_POINT('Ctrl Pts',(-18.7346124431284,-12.2936178960031,
122.357326758967)) ;
#15125=CARTESIAN_POINT('Ctrl Pts',(-18.6783500331761,-12.2966797947069,
122.395522002636)) ;
#15126=CARTESIAN_POINT('Ctrl Pts',(-18.6255288196949,-12.299797885005,122.438034998562)) ;
#15127=CARTESIAN_POINT('Ctrl Pts',(-18.6220810332869,-12.3000014113657,
122.440809939156)) ;
#15128=CARTESIAN_POINT('Ctrl Pts',(-18.618647896259,-12.3002051771326,122.44360326177)) ;
#15129=CARTESIAN_POINT('Ctrl Pts',(-18.615229573615,-12.3004092105329,122.446414837632)) ;
#15130=CARTESIAN_POINT('Ctrl Pts',(-18.5444122897155,-12.3046361641429,
122.504662167325)) ;
#15131=CARTESIAN_POINT('Ctrl Pts',(-18.480371878575,-12.3088502666534,122.570394955275)) ;
#15132=CARTESIAN_POINT('Ctrl Pts',(-18.4241492754252,-12.3130415268771,
122.642377720234)) ;
#15133=CARTESIAN_POINT('Ctrl Pts',(-18.3909287184771,-12.3155180397233,
122.684910570167)) ;
#15134=CARTESIAN_POINT('Ctrl Pts',(-18.3604369532267,-12.3179865775546,
122.729627329799)) ;
#15135=CARTESIAN_POINT('Ctrl Pts',(-18.3328942108092,-12.3204450792431,
122.776274952316)) ;
#15136=CARTESIAN_POINT('Ctrl Pts',(-18.3164372882747,-12.3219140459576,
122.804147133617)) ;
#15137=CARTESIAN_POINT('Ctrl Pts',(-18.3010393318235,-12.323392818313,122.832703539378)) ;
#15138=CARTESIAN_POINT('Ctrl Pts',(-18.2867844628654,-12.3248738381016,
122.861795094771)) ;
#15139=CARTESIAN_POINT('Ctrl Pts',(-18.2372995361152,-12.3300151098995,
122.962784692914)) ;
#15140=CARTESIAN_POINT('Ctrl Pts',(-18.2016881138637,-12.335146203594,123.069957542943)) ;
#15141=CARTESIAN_POINT('Ctrl Pts',(-18.1808841676186,-12.3403323963515,
123.180378082354)) ;
#15142=CARTESIAN_POINT('Ctrl Pts',(-18.163574053859,-12.3446476154717,123.272254502149)) ;
#15143=CARTESIAN_POINT('Ctrl Pts',(-18.1566580150728,-12.3489087243486,
123.365595950155)) ;
#15144=CARTESIAN_POINT('Ctrl Pts',(-18.1601514393078,-12.3531688566601,
123.458689044843)) ;
#15145=CARTESIAN_POINT('Ctrl Pts',(-18.1620825709398,-12.3555238172117,
123.510150020602)) ;
#15146=CARTESIAN_POINT('Ctrl Pts',(-18.1671952521868,-12.3578784793472,
123.561536635825)) ;
#15147=CARTESIAN_POINT('Ctrl Pts',(-18.1754965725959,-12.3602418184192,
123.612557019189)) ;
#15148=CARTESIAN_POINT('Ctrl Pts',(-18.1861378683255,-12.3632713352592,
123.67795902283)) ;
#15149=CARTESIAN_POINT('Ctrl Pts',(-18.2019792791202,-12.3663301102207,
123.74248622446)) ;
#15150=CARTESIAN_POINT('Ctrl Pts',(-18.2228680686441,-12.3693743269832,
123.805445096903)) ;
#15151=CARTESIAN_POINT('Ctrl Pts',(-18.2241083997099,-12.3695550859792,
123.809183458347)) ;
#15152=CARTESIAN_POINT('Ctrl Pts',(-18.2253665112514,-12.3697357936469,
123.812916292051)) ;
#15153=CARTESIAN_POINT('Ctrl Pts',(-18.2266423654683,-12.3699164408135,
123.816643453356)) ;
#15154=CARTESIAN_POINT('Origin',(-19.4092722359532,16.5113612779716,123.411814366564)) ;
#15155=CARTESIAN_POINT('',(-20.591901915765,13.7497304410597,123.00698472277)) ;
#15156=CARTESIAN_POINT('',(-20.5919019615554,13.8098330347218,123.006984856535)) ;
#15157=CARTESIAN_POINT('',(-20.5919021064381,16.5113612779716,123.006985279772)) ;
#15158=CARTESIAN_POINT('',(-18.1736437367582,14.0000000000496,123.600817573026)) ;
#15159=CARTESIAN_POINT('Ctrl Pts',(-18.1736437367582,14.0000000000496,123.600817573026)) ;
#15160=CARTESIAN_POINT('Ctrl Pts',(-18.1774626726793,13.9988411071295,123.625784271471)) ;
#15161=CARTESIAN_POINT('Ctrl Pts',(-18.1820355296742,13.9976824688196,123.650619704676)) ;
#15162=CARTESIAN_POINT('Ctrl Pts',(-18.1896653961921,13.9960232543353,123.686001901941)) ;
#15163=CARTESIAN_POINT('Ctrl Pts',(-18.1921114177232,13.9955221581955,123.696663785581)) ;
#15164=CARTESIAN_POINT('Ctrl Pts',(-18.1974156151627,13.994495191266,123.718466931781)) ;
#15165=CARTESIAN_POINT('Ctrl Pts',(-18.200288262439,13.9939694764739,123.72960363417)) ;
#15166=CARTESIAN_POINT('Ctrl Pts',(-18.2090082034946,13.9924563586871,123.761578001962)) ;
#15167=CARTESIAN_POINT('Ctrl Pts',(-18.21524346533,13.9914701085433,123.782305451609)) ;
#15168=CARTESIAN_POINT('Ctrl Pts',(-18.2252105208952,13.9900148307282,123.812566509253)) ;
#15169=CARTESIAN_POINT('Ctrl Pts',(-18.2285262460103,13.9895476550969,123.822232849602)) ;
#15170=CARTESIAN_POINT('Ctrl Pts',(-18.2341064833042,13.9887874444646,123.837873343762)) ;
#15171=CARTESIAN_POINT('Ctrl Pts',(-18.2362989265072,13.988494807074,123.843872711341)) ;
#15172=CARTESIAN_POINT('Ctrl Pts',(-18.2410879283046,13.9878681419586,123.856672099124)) ;
#15173=CARTESIAN_POINT('Ctrl Pts',(-18.2436980934359,13.9875340483542,123.863466773523)) ;
#15174=CARTESIAN_POINT('Ctrl Pts',(-18.2515425072828,13.9865512760902,123.883366056176)) ;
#15175=CARTESIAN_POINT('Ctrl Pts',(-18.2569394701305,13.9859017227269,123.896405240024)) ;
#15176=CARTESIAN_POINT('Ctrl Pts',(-18.2723161968905,13.9841210133041,123.931845384347)) ;
#15177=CARTESIAN_POINT('Ctrl Pts',(-18.2827361925457,13.9829884709045,123.954048483007)) ;
#15178=CARTESIAN_POINT('Ctrl Pts',(-18.2982079472457,13.9814081723277,123.984641950125)) ;
#15179=CARTESIAN_POINT('Ctrl Pts',(-18.302715314106,13.9809585867847,123.993301317154)) ;
#15180=CARTESIAN_POINT('Ctrl Pts',(-18.3103412489143,13.9802155212036,124.007542111373)) ;
#15181=CARTESIAN_POINT('Ctrl Pts',(-18.3134020234888,13.9799217350464,124.013153986035)) ;
#15182=CARTESIAN_POINT('Ctrl Pts',(-18.3191921184688,13.9793741626028,124.023578985777)) ;
#15183=CARTESIAN_POINT('Ctrl Pts',(-18.3219106105217,13.9791203147805,124.028397943711)) ;
#15184=CARTESIAN_POINT('Ctrl Pts',(-18.3275946469856,13.9785961438282,124.03831929092)) ;
#15185=CARTESIAN_POINT('Ctrl Pts',(-18.3305645128967,13.978325856509,124.043419049256)) ;
#15186=CARTESIAN_POINT('Ctrl Pts',(-18.3372625960084,13.9777241008422,124.054735729306)) ;
#15187=CARTESIAN_POINT('Ctrl Pts',(-18.3410090060583,13.9773927667428,124.060941641393)) ;
#15188=CARTESIAN_POINT('Ctrl Pts',(-18.3609314387805,13.9756575029645,124.093303437313)) ;
#15189=CARTESIAN_POINT('Ctrl Pts',(-18.3780146280628,13.9742608468966,124.118888288694)) ;
#15190=CARTESIAN_POINT('Ctrl Pts',(-18.4026702478654,13.9723458718292,124.15301693434)) ;
#15191=CARTESIAN_POINT('Ctrl Pts',(-18.4094414481529,13.9718292772952,124.16212577085)) ;
#15192=CARTESIAN_POINT('Ctrl Pts',(-18.4202152258821,13.9710205269863,124.176214142201)) ;
#15193=CARTESIAN_POINT('Ctrl Pts',(-18.4241335282709,13.970729028581,124.18125735499)) ;
#15194=CARTESIAN_POINT('Ctrl Pts',(-18.4285455719007,13.970403619078,124.186847108107)) ;
#15195=CARTESIAN_POINT('Ctrl Pts',(-18.4290013534839,13.9703700361816,124.187423505905)) ;
#15196=CARTESIAN_POINT('Ctrl Pts',(-18.4296752113697,13.970320433815,124.188274148053)) ;
#15197=CARTESIAN_POINT('Ctrl Pts',(-18.4298928952509,13.9703044177141,124.18854870329)) ;
#15198=CARTESIAN_POINT('Ctrl Pts',(-18.4306537361755,13.9702484649923,124.189507490593)) ;
#15199=CARTESIAN_POINT('Ctrl Pts',(-18.4311974948828,13.9702085232008,124.190191244528)) ;
#15200=CARTESIAN_POINT('Ctrl Pts',(-18.4344159675732,13.9699723843594,124.194229642365)) ;
#15201=CARTESIAN_POINT('Ctrl Pts',(-18.4371072173425,13.9697760439941,124.197571061907)) ;
#15202=CARTESIAN_POINT('Ctrl Pts',(-18.4427506060693,13.9693666130753,124.204504441975)) ;
#15203=CARTESIAN_POINT('Ctrl Pts',(-18.4457056892622,13.9691534986071,124.208093919632)) ;
#15204=CARTESIAN_POINT('Ctrl Pts',(-18.4527626088121,13.9686475595177,124.216569003977)) ;
#15205=CARTESIAN_POINT('Ctrl Pts',(-18.4568819487203,13.9683545842259,124.221439856322)) ;
#15206=CARTESIAN_POINT('Ctrl Pts',(-18.4736304101306,13.967172829716,124.240939117987)) ;
#15207=CARTESIAN_POINT('Ctrl Pts',(-18.486560665668,13.9662815712753,124.255305226442)) ;
#15208=CARTESIAN_POINT('Ctrl Pts',(-18.5068019288656,13.9649205685167,124.276771566171)) ;
#15209=CARTESIAN_POINT('Ctrl Pts',(-18.5138753587099,13.9644510609814,124.284091871219)) ;
#15210=CARTESIAN_POINT('Ctrl Pts',(-18.5264829401535,13.9636258235447,124.296824512246)) ;
#15211=CARTESIAN_POINT('Ctrl Pts',(-18.5319794341126,13.9632698229375,124.302273371309)) ;
#15212=CARTESIAN_POINT('Ctrl Pts',(-18.5435767368815,13.9625262213588,124.313558552678)) ;
#15213=CARTESIAN_POINT('Ctrl Pts',(-18.5496867891908,13.9621387063724,124.319384823664)) ;
#15214=CARTESIAN_POINT('Ctrl Pts',(-18.5627686055446,13.9613175721196,124.331608432353)) ;
#15215=CARTESIAN_POINT('Ctrl Pts',(-18.5697549345301,13.9608840605959,124.337989415325)) ;
#15216=CARTESIAN_POINT('Ctrl Pts',(-18.5781440697749,13.9603690900883,124.345478736162)) ;
#15217=CARTESIAN_POINT('Ctrl Pts',(-18.5794776389229,13.9602873938489,124.346664146161)) ;
#15218=CARTESIAN_POINT('Ctrl Pts',(-18.5992498898033,13.9590785366069,124.364164064333)) ;
#15219=CARTESIAN_POINT('Ctrl Pts',(-18.6181641013105,13.9579531970331,124.379933196125)) ;
#15220=CARTESIAN_POINT('Ctrl Pts',(-18.6452463333279,13.9563775433393,124.401188207421)) ;
#15221=CARTESIAN_POINT('Ctrl Pts',(-18.6530320199043,13.9559285191457,124.407151953503)) ;
#15222=CARTESIAN_POINT('Ctrl Pts',(-18.6677935907847,13.955083954693,124.418185953165)) ;
#15223=CARTESIAN_POINT('Ctrl Pts',(-18.6747533357469,13.9546885262551,124.42327684053)) ;
#15224=CARTESIAN_POINT('Ctrl Pts',(-18.6915483860493,13.9537403635067,124.435297250517)) ;
#15225=CARTESIAN_POINT('Ctrl Pts',(-18.7014321324551,13.9531871694207,124.442157573656)) ;
#15226=CARTESIAN_POINT('Ctrl Pts',(-18.7177546985943,13.9522819741949,124.453141365083)) ;
#15227=CARTESIAN_POINT('Ctrl Pts',(-18.7241350703599,13.9519301945439,124.457350347097)) ;
#15228=CARTESIAN_POINT('Ctrl Pts',(-18.7412113938347,13.9509943661721,124.468391759775)) ;
#15229=CARTESIAN_POINT('Ctrl Pts',(-18.7519734952643,13.9504104232339,124.475120269405)) ;
#15230=CARTESIAN_POINT('Ctrl Pts',(-18.7691506254861,13.9494879987677,124.48549902805)) ;
#15231=CARTESIAN_POINT('Ctrl Pts',(-18.7754987105456,13.9491491296948,124.489258354591)) ;
#15232=CARTESIAN_POINT('Ctrl Pts',(-18.7872212334678,13.9485271211577,124.496060966905)) ;
#15233=CARTESIAN_POINT('Ctrl Pts',(-18.7925856602834,13.9482439039994,124.49912104257)) ;
#15234=CARTESIAN_POINT('Ctrl Pts',(-18.8036283754401,13.9476638170881,124.505312221034)) ;
#15235=CARTESIAN_POINT('Ctrl Pts',(-18.8093087962845,13.9473669804819,124.508439149661)) ;
#15236=CARTESIAN_POINT('Ctrl Pts',(-18.8218670007401,13.9467141488494,124.515225341474)) ;
#15237=CARTESIAN_POINT('Ctrl Pts',(-18.8287551906648,13.9463582978248,124.518864794803)) ;
#15238=CARTESIAN_POINT('Ctrl Pts',(-18.8600968988099,13.9447490311704,124.535051582596)) ;
#15239=CARTESIAN_POINT('Ctrl Pts',(-18.8849257999716,13.943503381499,124.546854542897)) ;
#15240=CARTESIAN_POINT('Ctrl Pts',(-18.9202000696658,13.9417573700227,124.562218299917)) ;
#15241=CARTESIAN_POINT('Ctrl Pts',(-18.9303338072544,13.9412581327668,124.566473958707)) ;
#15242=CARTESIAN_POINT('Ctrl Pts',(-18.945672474652,13.9405047369784,124.572678753916)) ;
#15243=CARTESIAN_POINT('Ctrl Pts',(-18.9508364482386,13.9402514834011,124.574727730801)) ;
#15244=CARTESIAN_POINT('Ctrl Pts',(-18.9595707122399,13.9398236601065,124.578126119822)) ;
#15245=CARTESIAN_POINT('Ctrl Pts',(-18.9631338388344,13.9396492776055,124.579493730395)) ;
#15246=CARTESIAN_POINT('Ctrl Pts',(-18.966745181488,13.9394726659897,124.580860904629)) ;
#15247=CARTESIAN_POINT('Ctrl Pts',(-18.9667871975745,13.9394706112237,124.580876808397)) ;
#15248=CARTESIAN_POINT('Ctrl Pts',(-18.9668706198766,13.9394665315524,124.580908379947)) ;
#15249=CARTESIAN_POINT('Ctrl Pts',(-18.9669120265165,13.9394645066259,124.580924047964)) ;
#15250=CARTESIAN_POINT('Ctrl Pts',(-18.9669942433454,13.9394604859759,124.580955153311)) ;
#15251=CARTESIAN_POINT('Ctrl Pts',(-18.9670350533953,13.9394584902587,124.58097059066)) ;
#15252=CARTESIAN_POINT('Ctrl Pts',(-18.9671160898843,13.9394545273977,124.581001239745)) ;
#15253=CARTESIAN_POINT('Ctrl Pts',(-18.9671563160248,13.9394525602681,124.581016451437)) ;
#15254=CARTESIAN_POINT('Ctrl Pts',(-18.9672361962167,13.9394486540174,124.581046653771)) ;
#15255=CARTESIAN_POINT('Ctrl Pts',(-18.9672758504303,13.939446714888,124.581061644542)) ;
#15256=CARTESIAN_POINT('Ctrl Pts',(-18.9673545995492,13.9394428640114,124.581091410065)) ;
#15257=CARTESIAN_POINT('Ctrl Pts',(-18.9673936942426,13.9394409522741,124.581106184802)) ;
#15258=CARTESIAN_POINT('Ctrl Pts',(-18.9674713347892,13.9394371556684,124.581135522408)) ;
#15259=CARTESIAN_POINT('Ctrl Pts',(-18.967509881168,13.9394352707739,124.581150085538)) ;
#15260=CARTESIAN_POINT('Ctrl Pts',(-18.9675864383075,13.9394315272059,124.581179005111)) ;
#15261=CARTESIAN_POINT('Ctrl Pts',(-18.9676244485248,13.9394296685586,124.58119336141)) ;
#15262=CARTESIAN_POINT('Ctrl Pts',(-18.9676999440553,13.9394259769598,124.581221871547)) ;
#15263=CARTESIAN_POINT('Ctrl Pts',(-18.9677374293982,13.9394241440066,124.581236025454)) ;
#15264=CARTESIAN_POINT('Ctrl Pts',(-18.9678118860851,13.9394205032614,124.581264135101)) ;
#15265=CARTESIAN_POINT('Ctrl Pts',(-18.9678488576418,13.9394186954588,124.581278090977)) ;
#15266=CARTESIAN_POINT('Ctrl Pts',(-18.9679222976972,13.9394151044788,124.581305808857)) ;
#15267=CARTESIAN_POINT('Ctrl Pts',(-18.967958766328,13.9394133212946,124.581319570966)) ;
#15268=CARTESIAN_POINT('Ctrl Pts',(-18.9680312123382,13.939409778973,124.581346905929)) ;
#15269=CARTESIAN_POINT('Ctrl Pts',(-18.9680671892768,13.9394080198568,124.58136047867)) ;
#15270=CARTESIAN_POINT('Ctrl Pts',(-18.9681386615179,13.9394045252001,124.581387438681)) ;
#15271=CARTESIAN_POINT('Ctrl Pts',(-18.9681741570821,13.9394027896464,124.581400826101)) ;
#15272=CARTESIAN_POINT('Ctrl Pts',(-18.9682446774375,13.9393993415823,124.581427419718)) ;
#15273=CARTESIAN_POINT('Ctrl Pts',(-18.9682797022772,13.9393976290692,124.581440625982)) ;
#15274=CARTESIAN_POINT('Ctrl Pts',(-18.9683492904791,13.939394226631,124.581466860938)) ;
#15275=CARTESIAN_POINT('Ctrl Pts',(-18.96838385427,13.9393925366845,124.581479889839)) ;
#15276=CARTESIAN_POINT('Ctrl Pts',(-18.9684525326365,13.9393891787789,124.581505774831)) ;
#15277=CARTESIAN_POINT('Ctrl Pts',(-18.9684866462715,13.9393875108655,124.581518630613)) ;
#15278=CARTESIAN_POINT('Ctrl Pts',(-18.9685544328501,13.9393841966083,124.581544172715)) ;
#15279=CARTESIAN_POINT('Ctrl Pts',(-18.9685881058439,13.9393825502617,124.581556859099)) ;
#15280=CARTESIAN_POINT('Ctrl Pts',(-18.9686550213212,13.9393792786396,124.581582066369)) ;
#15281=CARTESIAN_POINT('Ctrl Pts',(-18.9686882636257,13.9393776533724,124.581594587232)) ;
#15282=CARTESIAN_POINT('Ctrl Pts',(-18.9687543270124,13.9393744234541,124.581619467087)) ;
#15283=CARTESIAN_POINT('Ctrl Pts',(-18.9687871482268,13.9393728187962,124.581631826169)) ;
#15284=CARTESIAN_POINT('Ctrl Pts',(-18.9688523781887,13.9393696296675,124.581656385882)) ;
#15285=CARTESIAN_POINT('Ctrl Pts',(-18.9688847873888,13.9393680451743,124.581668586722)) ;
#15286=CARTESIAN_POINT('Ctrl Pts',(-18.9689492037355,13.9393648958649,124.581692833989)) ;
#15287=CARTESIAN_POINT('Ctrl Pts',(-18.9689812105766,13.9393633310635,124.581704880338)) ;
#15288=CARTESIAN_POINT('Ctrl Pts',(-18.9690448309592,13.9393602207091,124.581728822031)) ;
#15289=CARTESIAN_POINT('Ctrl Pts',(-18.9690764444664,13.9393586751575,124.581740717397)) ;
#15290=CARTESIAN_POINT('Ctrl Pts',(-18.9691392875197,13.9393556028453,124.581764360749)) ;
#15291=CARTESIAN_POINT('Ctrl Pts',(-18.969170516958,13.9393540760898,124.581776108728)) ;
#15292=CARTESIAN_POINT('Ctrl Pts',(-18.9692325994227,13.939351041,124.581799460249)) ;
#15293=CARTESIAN_POINT('Ctrl Pts',(-18.969263453047,13.9393495326363,124.58181106405)) ;
#15294=CARTESIAN_POINT('Ctrl Pts',(-18.9693247941971,13.9393465338253,124.581834131196)) ;
#15295=CARTESIAN_POINT('Ctrl Pts',(-18.9693552812066,13.939345043403,124.58184559438)) ;
#15296=CARTESIAN_POINT('Ctrl Pts',(-18.9694158972986,13.9393420800745,124.581868383461)) ;
#15297=CARTESIAN_POINT('Ctrl Pts',(-18.9694460261724,13.9393406071784,124.581879709313)) ;
#15298=CARTESIAN_POINT('Ctrl Pts',(-18.9695059349098,13.9393376784658,124.581902227177)) ;
#15299=CARTESIAN_POINT('Ctrl Pts',(-18.9695357145272,13.9393362226611,124.581913419129)) ;
#15300=CARTESIAN_POINT('Ctrl Pts',(-18.9695949312375,13.9393333278137,124.581935671721)) ;
#15301=CARTESIAN_POINT('Ctrl Pts',(-18.9696243692418,13.9393318887263,124.581946732735)) ;
#15302=CARTESIAN_POINT('Ctrl Pts',(-18.9696829119197,13.9393290268632,124.581968726996)) ;
#15303=CARTESIAN_POINT('Ctrl Pts',(-18.9697120166187,13.9393276040862,124.581979660282)) ;
#15304=CARTESIAN_POINT('Ctrl Pts',(-18.9697699017845,13.9393247743987,124.582001402589)) ;
#15305=CARTESIAN_POINT('Ctrl Pts',(-18.9697986816223,13.9393233675188,124.582012211403)) ;
#15306=CARTESIAN_POINT('Ctrl Pts',(-18.9698559250561,13.9393205692343,124.582033707849)) ;
#15307=CARTESIAN_POINT('Ctrl Pts',(-18.9698843883754,13.9393191778431,124.582044395405)) ;
#15308=CARTESIAN_POINT('Ctrl Pts',(-18.9699410043546,13.9393164102626,124.582065651512)) ;
#15309=CARTESIAN_POINT('Ctrl Pts',(-18.9699691581441,13.9393150340179,124.582076220513)) ;
#15310=CARTESIAN_POINT('Ctrl Pts',(-18.9700251644834,13.9393122962695,124.582097243123)) ;
#15311=CARTESIAN_POINT('Ctrl Pts',(-18.9700530168869,13.9393109347728,124.582107696701)) ;
#15312=CARTESIAN_POINT('Ctrl Pts',(-18.9701084286675,13.9393082261182,124.582128491623)) ;
#15313=CARTESIAN_POINT('Ctrl Pts',(-18.9701359877231,13.939306878976,124.582138832869)) ;
#15314=CARTESIAN_POINT('Ctrl Pts',(-18.9701908187779,13.9393041987381,124.582159405438)) ;
#15315=CARTESIAN_POINT('Ctrl Pts',(-18.9702180913467,13.9393028656145,124.582169636996)) ;
#15316=CARTESIAN_POINT('Ctrl Pts',(-18.9732080926408,13.9391567107115,124.583291244657)) ;
#15317=CARTESIAN_POINT('Ctrl Pts',(-18.9761750241519,13.9390117688047,124.584391365336)) ;
#15318=CARTESIAN_POINT('Ctrl Pts',(-18.9820807847831,13.9387234143468,124.586555713941)) ;
#15319=CARTESIAN_POINT('Ctrl Pts',(-18.9850194915413,13.9385800058607,124.587620208521)) ;
#15320=CARTESIAN_POINT('Ctrl Pts',(-18.9928479852357,13.9381981699311,124.590422772352)) ;
#15321=CARTESIAN_POINT('Ctrl Pts',(-18.9977446446959,13.9379595339167,124.592141428061)) ;
#15322=CARTESIAN_POINT('Ctrl Pts',(-19.0207307657352,13.9368402336773,124.600048793045)) ;
#15323=CARTESIAN_POINT('Ctrl Pts',(-19.038949793513,13.9359554506044,124.605852390117)) ;
#15324=CARTESIAN_POINT('Ctrl Pts',(-19.0774247613116,13.9340960678331,124.61714310735)) ;
#15325=CARTESIAN_POINT('Ctrl Pts',(-19.0977005875379,13.9331220884634,124.622542757756)) ;
#15326=CARTESIAN_POINT('Ctrl Pts',(-19.1263403553744,13.9317600742956,124.629402680527)) ;
#15327=CARTESIAN_POINT('Ctrl Pts',(-19.1345978289103,13.9313689069911,124.631292009863)) ;
#15328=CARTESIAN_POINT('Ctrl Pts',(-19.147787481875,13.9307466536259,124.634169067745)) ;
#15329=CARTESIAN_POINT('Ctrl Pts',(-19.1527074981449,13.9305151027838,124.635211206382)) ;
#15330=CARTESIAN_POINT('Ctrl Pts',(-19.16130417932,13.9301114985128,124.636977981991)) ;
#15331=CARTESIAN_POINT('Ctrl Pts',(-19.1649780563968,13.9299393258473,124.637715829006)) ;
#15332=CARTESIAN_POINT('Ctrl Pts',(-19.1721756599988,13.9296026186865,124.639127726821)) ;
#15333=CARTESIAN_POINT('Ctrl Pts',(-19.1756990796923,13.9294380729136,124.639803149641)) ;
#15334=CARTESIAN_POINT('Ctrl Pts',(-19.1827392516312,13.9291098407486,124.641121320646)) ;
#15335=CARTESIAN_POINT('Ctrl Pts',(-19.186255950468,13.9289461549195,124.641764169133)) ;
#15336=CARTESIAN_POINT('Ctrl Pts',(-19.1947302003395,13.9285523503711,124.643275712488)) ;
#15337=CARTESIAN_POINT('Ctrl Pts',(-19.1996903387403,13.9283223694788,124.64412956981)) ;
#15338=CARTESIAN_POINT('Ctrl Pts',(-19.2245417840649,13.927172527981,124.648253209569)) ;
#15339=CARTESIAN_POINT('Ctrl Pts',(-19.2445050504352,13.9262568255469,124.65107145639)) ;
#15340=CARTESIAN_POINT('Ctrl Pts',(-19.2654189592725,13.9253013542152,124.653509594785)) ;
#15341=CARTESIAN_POINT('Ctrl Pts',(-19.2663102099474,13.9252606433657,124.653612524124)) ;
#15342=CARTESIAN_POINT('Ctrl Pts',(-19.2677614680521,13.9251943624866,124.653778544885)) ;
#15343=CARTESIAN_POINT('Ctrl Pts',(-19.2683214086561,13.9251687917241,124.653842217278)) ;
#15344=CARTESIAN_POINT('Ctrl Pts',(-19.2707238703482,13.9250590887249,124.654113762265)) ;
#15345=CARTESIAN_POINT('Ctrl Pts',(-19.2725668096922,13.9249749603644,124.654317913683)) ;
#15346=CARTESIAN_POINT('Ctrl Pts',(-19.2750571409665,13.9248613069928,124.654588172138)) ;
#15347=CARTESIAN_POINT('Ctrl Pts',(-19.275704140049,13.9248317818754,124.654657875337)) ;
#15348=CARTESIAN_POINT('Ctrl Pts',(-19.2926060973418,13.924060539582,124.656465424471)) ;
#15349=CARTESIAN_POINT('Ctrl Pts',(-19.3088934680056,13.9233185683605,124.657884727485)) ;
#15350=CARTESIAN_POINT('Ctrl Pts',(-19.3332750460147,13.9222063384977,124.659528222146)) ;
#15351=CARTESIAN_POINT('Ctrl Pts',(-19.3413511852334,13.9218377068823,124.659993908311)) ;
#15352=CARTESIAN_POINT('Ctrl Pts',(-19.3549040558307,13.9212184829742,124.66064346673)) ;
#15353=CARTESIAN_POINT('Ctrl Pts',(-19.3603785104605,13.9209681926304,124.660869779183)) ;
#15354=CARTESIAN_POINT('Ctrl Pts',(-19.3659434873133,13.9207135668985,124.661063191894)) ;
#15355=CARTESIAN_POINT('Ctrl Pts',(-19.3660327097756,13.9207094844702,124.661066283282)) ;
#15356=CARTESIAN_POINT('Ctrl Pts',(-19.3662045149436,13.9207016233211,124.661072217574)) ;
#15357=CARTESIAN_POINT('Ctrl Pts',(-19.3662870975194,13.9206978446137,124.661075061847)) ;
#15358=CARTESIAN_POINT('Ctrl Pts',(-19.366446161289,13.9206905662934,124.661080524459)) ;
#15359=CARTESIAN_POINT('Ctrl Pts',(-19.3665226419754,13.92068706671,124.661083143948)) ;
#15360=CARTESIAN_POINT('Ctrl Pts',(-19.3666699907485,13.9206803242905,124.661088177147)) ;
#15361=CARTESIAN_POINT('Ctrl Pts',(-19.3667408592481,13.9206770814408,124.661090591864)) ;
#15362=CARTESIAN_POINT('Ctrl Pts',(-19.3668774321641,13.9206708319806,124.661095233707)) ;
#15363=CARTESIAN_POINT('Ctrl Pts',(-19.3669431362677,13.9206678253889,124.66109746167)) ;
#15364=CARTESIAN_POINT('Ctrl Pts',(-19.3670697879421,13.9206620298087,124.661101746304)) ;
#15365=CARTESIAN_POINT('Ctrl Pts',(-19.3671307358306,13.9206592408094,124.661103803709)) ;
#15366=CARTESIAN_POINT('Ctrl Pts',(-19.3672482479186,13.920653863364,124.661107761932)) ;
#15367=CARTESIAN_POINT('Ctrl Pts',(-19.3673048124465,13.9206512749061,124.661109663379)) ;
#15368=CARTESIAN_POINT('Ctrl Pts',(-19.3674138995754,13.9206462829134,124.661113322985)) ;
#15369=CARTESIAN_POINT('Ctrl Pts',(-19.3674664219875,13.9206438793902,124.661115081667)) ;
#15370=CARTESIAN_POINT('Ctrl Pts',(-19.3675677362742,13.9206392430257,124.66111846772)) ;
#15371=CARTESIAN_POINT('Ctrl Pts',(-19.3676165281633,13.9206370101861,124.661120095546)) ;
#15372=CARTESIAN_POINT('Ctrl Pts',(-19.3677106680637,13.9206327020776,124.66112323078)) ;
#15373=CARTESIAN_POINT('Ctrl Pts',(-19.367756015428,13.9206306268404,124.661124738557)) ;
#15374=CARTESIAN_POINT('Ctrl Pts',(-19.3679269435706,13.9206228045837,124.661130412512)) ;
#15375=CARTESIAN_POINT('Ctrl Pts',(-19.3680525250163,13.9206170574446,124.661134562228)) ;
#15376=CARTESIAN_POINT('Ctrl Pts',(-19.3683006178882,13.9206057034606,124.661142722768)) ;
#15377=CARTESIAN_POINT('Ctrl Pts',(-19.3684231293397,13.9206000966194,124.661146734507)) ;
#15378=CARTESIAN_POINT('Ctrl Pts',(-19.3686652174968,13.9205890170547,124.661154626238)) ;
#15379=CARTESIAN_POINT('Ctrl Pts',(-19.3687847942475,13.9205835443338,124.661158507085)) ;
#15380=CARTESIAN_POINT('Ctrl Pts',(-19.3690211441822,13.920572727019,124.661166143822)) ;
#15381=CARTESIAN_POINT('Ctrl Pts',(-19.3691379173936,13.9205673824282,124.661169900509)) ;
#15382=CARTESIAN_POINT('Ctrl Pts',(-19.3693687878214,13.9205568155477,124.661177295394)) ;
#15383=CARTESIAN_POINT('Ctrl Pts',(-19.3694828849103,13.9205515932677,124.66118093433)) ;
#15384=CARTESIAN_POINT('Ctrl Pts',(-19.3697085263931,13.9205412653768,124.661188099847)) ;
#15385=CARTESIAN_POINT('Ctrl Pts',(-19.3698200708131,13.9205361597685,124.661191627121)) ;
#15386=CARTESIAN_POINT('Ctrl Pts',(-19.3700407278998,13.920526059696,124.661198575192)) ;
#15387=CARTESIAN_POINT('Ctrl Pts',(-19.3701498401933,13.9205210652524,124.661201996623)) ;
#15388=CARTESIAN_POINT('Ctrl Pts',(-19.3703657490253,13.9205111822102,124.661208738557)) ;
#15389=CARTESIAN_POINT('Ctrl Pts',(-19.3704725458167,13.9205062936031,124.66121205967)) ;
#15390=CARTESIAN_POINT('Ctrl Pts',(-19.3706839380596,13.920496617006,124.661218606309)) ;
#15391=CARTESIAN_POINT('Ctrl Pts',(-19.370788533413,13.9204918290235,124.661221832392)) ;
#15392=CARTESIAN_POINT('Ctrl Pts',(-19.370995634061,13.9204823485902,124.661228194061)) ;
#15393=CARTESIAN_POINT('Ctrl Pts',(-19.3710981392099,13.920477656149,124.661231330164)) ;
#15394=CARTESIAN_POINT('Ctrl Pts',(-19.3713011679266,13.9204683618408,124.661237516735)) ;
#15395=CARTESIAN_POINT('Ctrl Pts',(-19.3714016914962,13.9204637599763,124.661240567687)) ;
#15396=CARTESIAN_POINT('Ctrl Pts',(-19.3764233886142,13.9202338685576,124.661392372686)) ;
#15397=CARTESIAN_POINT('Ctrl Pts',(-19.3813453883059,13.920008379841,124.661512062472)) ;
#15398=CARTESIAN_POINT('Ctrl Pts',(-19.3913102620274,13.919551522313,124.661695481316)) ;
#15399=CARTESIAN_POINT('Ctrl Pts',(-19.3963530721949,13.9193201480641,124.661757776703)) ;
#15400=CARTESIAN_POINT('Ctrl Pts',(-19.4114053570885,13.9186289925624,124.661852621509)) ;
#15401=CARTESIAN_POINT('Ctrl Pts',(-19.4214149662524,13.9181686774593,124.661795463211)) ;
#15402=CARTESIAN_POINT('Ctrl Pts',(-19.4506181858273,13.9168239996106,124.661277888179)) ;
#15403=CARTESIAN_POINT('Ctrl Pts',(-19.4698031946768,13.9159383507741,124.660495502817)) ;
#15404=CARTESIAN_POINT('Ctrl Pts',(-19.4953775834862,13.914757901529,124.658861755587)) ;
#15405=CARTESIAN_POINT('Ctrl Pts',(-19.50178942799,13.9144619770801,124.658402466501)) ;
#15406=CARTESIAN_POINT('Ctrl Pts',(-19.5148496310689,13.9138595559828,124.657365627663)) ;
#15407=CARTESIAN_POINT('Ctrl Pts',(-19.5214974836442,13.9135530864495,124.656784255579)) ;
#15408=CARTESIAN_POINT('Ctrl Pts',(-19.5374234120754,13.9128189560705,124.655262892759)) ;
#15409=CARTESIAN_POINT('Ctrl Pts',(-19.5466962535454,13.9123915595447,124.654272253695)) ;
#15410=CARTESIAN_POINT('Ctrl Pts',(-19.5668074263285,13.9114639489423,124.651895830038)) ;
#15411=CARTESIAN_POINT('Ctrl Pts',(-19.5776404313177,13.9109638642758,124.650471511811)) ;
#15412=CARTESIAN_POINT('Ctrl Pts',(-19.6080326443963,13.909558338681,124.646069482035)) ;
#15413=CARTESIAN_POINT('Ctrl Pts',(-19.6275418109054,13.9086530916704,124.64276919171)) ;
#15414=CARTESIAN_POINT('Ctrl Pts',(-19.6671877083547,13.9068032839008,124.635090269406)) ;
#15415=CARTESIAN_POINT('Ctrl Pts',(-19.6873110655574,13.905858910027,124.63067396429)) ;
#15416=CARTESIAN_POINT('Ctrl Pts',(-19.7301892752595,13.9038330797831,124.620146678596)) ;
#15417=CARTESIAN_POINT('Ctrl Pts',(-19.7528995079878,13.9027520150845,124.613885509814)) ;
#15418=CARTESIAN_POINT('Ctrl Pts',(-19.8012734673872,13.9004308672457,124.599065902957)) ;
#15419=CARTESIAN_POINT('Ctrl Pts',(-19.8268639143808,13.8991915779605,124.590308478354)) ;
#15420=CARTESIAN_POINT('Ctrl Pts',(-19.879223751613,13.8966271417408,124.570470385132)) ;
#15421=CARTESIAN_POINT('Ctrl Pts',(-19.9059327736428,13.8953029119353,124.559275262651)) ;
#15422=CARTESIAN_POINT('Ctrl Pts',(-19.956855287508,13.8927364115002,124.535819672403)) ;
#15423=CARTESIAN_POINT('Ctrl Pts',(-19.9811060066009,13.8914945859408,124.5236782338)) ;
#15424=CARTESIAN_POINT('Ctrl Pts',(-20.0281006258142,13.8890432369325,124.498205310685)) ;
#15425=CARTESIAN_POINT('Ctrl Pts',(-20.0508560573835,13.8878344303593,124.484923894662)) ;
#15426=CARTESIAN_POINT('Ctrl Pts',(-20.080460114139,13.8862323867493,124.466366765715)) ;
#15427=CARTESIAN_POINT('Ctrl Pts',(-20.0876980866373,13.8858383092675,124.461724979836)) ;
#15428=CARTESIAN_POINT('Ctrl Pts',(-20.1018009566885,13.8850658649542,124.452473932091)) ;
#15429=CARTESIAN_POINT('Ctrl Pts',(-20.1086691645535,13.884687494958,124.447870493019)) ;
#15430=CARTESIAN_POINT('Ctrl Pts',(-20.1219453760699,13.883951980122,124.438779888109)) ;
#15431=CARTESIAN_POINT('Ctrl Pts',(-20.1283579311245,13.8835948071044,124.434300039068)) ;
#15432=CARTESIAN_POINT('Ctrl Pts',(-20.1562744967525,13.8820301564728,124.414404842634)) ;
#15433=CARTESIAN_POINT('Ctrl Pts',(-20.1773279440905,13.8808242007162,124.398369213678)) ;
#15434=CARTESIAN_POINT('Ctrl Pts',(-20.2033402422412,13.8792903909254,124.377218919719)) ;
#15435=CARTESIAN_POINT('Ctrl Pts',(-20.2087859377444,13.878966786266,124.372713835882)) ;
#15436=CARTESIAN_POINT('Ctrl Pts',(-20.2186624930317,13.8783751243418,124.364401127657)) ;
#15437=CARTESIAN_POINT('Ctrl Pts',(-20.2231054293776,13.8781071752414,124.360608158024)) ;
#15438=CARTESIAN_POINT('Ctrl Pts',(-20.2276995668302,13.877828195985,124.356630094399)) ;
#15439=CARTESIAN_POINT('Ctrl Pts',(-20.2278774832658,13.8778173889995,124.356475948594)) ;
#15440=CARTESIAN_POINT('Ctrl Pts',(-20.2282365229829,13.877795574178,124.356164700991)) ;
#15441=CARTESIAN_POINT('Ctrl Pts',(-20.2284176446522,13.8777845663278,124.356007597301)) ;
#15442=CARTESIAN_POINT('Ctrl Pts',(-20.2287839208127,13.8777622992213,124.355689707162)) ;
#15443=CARTESIAN_POINT('Ctrl Pts',(-20.228969073219,13.8777510399482,124.355528918315)) ;
#15444=CARTESIAN_POINT('Ctrl Pts',(-20.2293442523262,13.8777282183736,124.355202914006)) ;
#15445=CARTESIAN_POINT('Ctrl Pts',(-20.2295342763912,13.8777166560548,124.355037695632)) ;
#15446=CARTESIAN_POINT('Ctrl Pts',(-20.2299200672067,13.8776931749944,124.354702061097)) ;
#15447=CARTESIAN_POINT('Ctrl Pts',(-20.2301158308275,13.877681256228,124.354531641359)) ;
#15448=CARTESIAN_POINT('Ctrl Pts',(-20.2353433106641,13.8773628912432,124.34997805692)) ;
#15449=CARTESIAN_POINT('Ctrl Pts',(-20.2403398901878,13.8770561624978,124.345554739535)) ;
#15450=CARTESIAN_POINT('Ctrl Pts',(-20.2537736939653,13.8762248039489,124.333468956207)) ;
#15451=CARTESIAN_POINT('Ctrl Pts',(-20.2621419114022,13.875699665424,124.325730779803)) ;
#15452=CARTESIAN_POINT('Ctrl Pts',(-20.2890188048205,13.8739891719933,124.300186778883)) ;
#15453=CARTESIAN_POINT('Ctrl Pts',(-20.3070847995225,13.8728014336502,124.281924801571)) ;
#15454=CARTESIAN_POINT('Ctrl Pts',(-20.3327228911498,13.871065222241,124.254359324485)) ;
#15455=CARTESIAN_POINT('Ctrl Pts',(-20.3407442207031,13.8705142530263,124.245482803349)) ;
#15456=CARTESIAN_POINT('Ctrl Pts',(-20.3522514987485,13.8697126148666,124.232375227732)) ;
#15457=CARTESIAN_POINT('Ctrl Pts',(-20.3558389721217,13.8694610543272,124.228234253128)) ;
#15458=CARTESIAN_POINT('Ctrl Pts',(-20.3609359035609,13.8691012787815,124.22227217366)) ;
#15459=CARTESIAN_POINT('Ctrl Pts',(-20.3624675910696,13.8689928512087,124.22047016994)) ;
#15460=CARTESIAN_POINT('Ctrl Pts',(-20.36628960837,13.8687215102603,124.215947686043)) ;
#15461=CARTESIAN_POINT('Ctrl Pts',(-20.3685734618813,13.8685586616537,124.21322175648)) ;
#15462=CARTESIAN_POINT('Ctrl Pts',(-20.3736850283819,13.868192576821,124.207067605549)) ;
#15463=CARTESIAN_POINT('Ctrl Pts',(-20.3765061568603,13.867989408835,124.203633973995)) ;
#15464=CARTESIAN_POINT('Ctrl Pts',(-20.3830296711849,13.8675169572769,124.195607235035)) ;
#15465=CARTESIAN_POINT('Ctrl Pts',(-20.3867179739935,13.8672478203455,124.191002811594)) ;
#15466=CARTESIAN_POINT('Ctrl Pts',(-20.3964126849496,13.8665348986633,124.178722914163)) ;
#15467=CARTESIAN_POINT('Ctrl Pts',(-20.4023621678777,13.8660916906057,124.171002995942)) ;
#15468=CARTESIAN_POINT('Ctrl Pts',(-20.4219847678086,13.8646097237938,124.144915731517)) ;
#15469=CARTESIAN_POINT('Ctrl Pts',(-20.4352432116931,13.8635757257447,124.12624269323)) ;
#15470=CARTESIAN_POINT('Ctrl Pts',(-20.4569931975374,13.8618053092372,124.093755122169)) ;
#15471=CARTESIAN_POINT('Ctrl Pts',(-20.4657424565696,13.8610701433617,124.080120489348)) ;
#15472=CARTESIAN_POINT('Ctrl Pts',(-20.4766311972598,13.8601215799561,124.062403314976)) ;
#15473=CARTESIAN_POINT('Ctrl Pts',(-20.4790165525729,13.8599116168089,124.05847365003)) ;
#15474=CARTESIAN_POINT('Ctrl Pts',(-20.4827617245927,13.8595784489231,124.052226372633)) ;
#15475=CARTESIAN_POINT('Ctrl Pts',(-20.4841358418109,13.8594554445667,124.049917374306)) ;
#15476=CARTESIAN_POINT('Ctrl Pts',(-20.4868163538934,13.8592139829952,124.045379948361)) ;
#15477=CARTESIAN_POINT('Ctrl Pts',(-20.4881233071963,13.8590955343428,124.043151866303)) ;
#15478=CARTESIAN_POINT('Ctrl Pts',(-20.4894303910201,13.8589763455646,124.040907650835)) ;
#15479=CARTESIAN_POINT('Ctrl Pts',(-20.4894374392435,13.8589757028383,124.040895548824)) ;
#15480=CARTESIAN_POINT('Ctrl Pts',(-20.4894515373059,13.8589744171956,124.040871341091)) ;
#15481=CARTESIAN_POINT('Ctrl Pts',(-20.4894585869626,13.8589737742958,124.040859235683)) ;
#15482=CARTESIAN_POINT('Ctrl Pts',(-20.489472687908,13.8589724883046,124.040835021129)) ;
#15483=CARTESIAN_POINT('Ctrl Pts',(-20.4894797397975,13.8589718451583,124.04082291095)) ;
#15484=CARTESIAN_POINT('Ctrl Pts',(-20.4894938476967,13.8589705584471,124.040798682581)) ;
#15485=CARTESIAN_POINT('Ctrl Pts',(-20.4895009034205,13.8589699149082,124.04078656488)) ;
#15486=CARTESIAN_POINT('Ctrl Pts',(-20.4895150206131,13.8589686272635,124.040762318674)) ;
#15487=CARTESIAN_POINT('Ctrl Pts',(-20.4895220816866,13.8589679831937,124.040750190847)) ;
#15488=CARTESIAN_POINT('Ctrl Pts',(-20.4895362104088,13.8589666944114,124.040725922959)) ;
#15489=CARTESIAN_POINT('Ctrl Pts',(-20.4895432780922,13.8589660496956,124.040713782838)) ;
#15490=CARTESIAN_POINT('Ctrl Pts',(-20.4895574210412,13.8589647595293,124.04068948863)) ;
#15491=CARTESIAN_POINT('Ctrl Pts',(-20.4895644965789,13.8589641140539,124.040677334074)) ;
#15492=CARTESIAN_POINT('Ctrl Pts',(-20.4895786563188,13.8589628222694,124.040653009136)) ;
#15493=CARTESIAN_POINT('Ctrl Pts',(-20.4895857408142,13.8589621759336,124.040640838247)) ;
#15494=CARTESIAN_POINT('Ctrl Pts',(-20.4895999205315,13.8589608822399,124.040616477096)) ;
#15495=CARTESIAN_POINT('Ctrl Pts',(-20.4896070154501,13.8589602349097,124.040604287352)) ;
#15496=CARTESIAN_POINT('Ctrl Pts',(-20.4896212177068,13.8589589390727,124.040579885577)) ;
#15497=CARTESIAN_POINT('Ctrl Pts',(-20.4896283246326,13.8589582906034,124.040567674252)) ;
#15498=CARTESIAN_POINT('Ctrl Pts',(-20.4896425511479,13.8589569924657,124.040543228891)) ;
#15499=CARTESIAN_POINT('Ctrl Pts',(-20.4896496710771,13.8589563427662,124.040530994268)) ;
#15500=CARTESIAN_POINT('Ctrl Pts',(-20.4896639249594,13.8589550420437,124.040506499968)) ;
#15501=CARTESIAN_POINT('Ctrl Pts',(-20.4896710591065,13.8589543910029,124.040494239955)) ;
#15502=CARTESIAN_POINT('Ctrl Pts',(-20.4896853432603,13.85895308743,124.040469691712)) ;
#15503=CARTESIAN_POINT('Ctrl Pts',(-20.4896924930939,13.8589524349136,124.040457403779)) ;
#15504=CARTESIAN_POINT('Ctrl Pts',(-20.4897068096879,13.8589511282918,124.040432797854)) ;
#15505=CARTESIAN_POINT('Ctrl Pts',(-20.4897139764488,13.8589504741863,124.040420479861)) ;
#15506=CARTESIAN_POINT('Ctrl Pts',(-20.4897283281319,13.8589491642732,124.040395811688)) ;
#15507=CARTESIAN_POINT('Ctrl Pts',(-20.4897355130865,13.8589485084626,124.040383461451)) ;
#15508=CARTESIAN_POINT('Ctrl Pts',(-20.4897499024844,13.8589471950179,124.040358726501)) ;
#15509=CARTESIAN_POINT('Ctrl Pts',(-20.4897571069399,13.8589465373825,124.040346341765)) ;
#15510=CARTESIAN_POINT('Ctrl Pts',(-20.4897715364221,13.8589452201891,124.040321535949)) ;
#15511=CARTESIAN_POINT('Ctrl Pts',(-20.489778761504,13.8589445606258,124.040309114772)) ;
#15512=CARTESIAN_POINT('Ctrl Pts',(-20.489793234226,13.8589432393949,124.040284232648)) ;
#15513=CARTESIAN_POINT('Ctrl Pts',(-20.4898004814714,13.8589425777631,124.040271772377)) ;
#15514=CARTESIAN_POINT('Ctrl Pts',(-20.4898149995318,13.8589412523022,124.040246810319)) ;
#15515=CARTESIAN_POINT('Ctrl Pts',(-20.4898222702575,13.8589405884811,124.040234308681)) ;
#15516=CARTESIAN_POINT('Ctrl Pts',(-20.4898368358522,13.8589392585889,124.040209262893)) ;
#15517=CARTESIAN_POINT('Ctrl Pts',(-20.4898441310091,13.8589385924913,124.040196718243)) ;
#15518=CARTESIAN_POINT('Ctrl Pts',(-20.4898587477926,13.8589372578331,124.040171582421)) ;
#15519=CARTESIAN_POINT('Ctrl Pts',(-20.4898660690434,13.8589365893067,124.04015899189)) ;
#15520=CARTESIAN_POINT('Ctrl Pts',(-20.4898807390652,13.8589352496944,124.040133762486)) ;
#15521=CARTESIAN_POINT('Ctrl Pts',(-20.4898880878917,13.8589345786033,124.040121123514)) ;
#15522=CARTESIAN_POINT('Ctrl Pts',(-20.4899028125276,13.8589332339102,124.040095798141)) ;
#15523=CARTESIAN_POINT('Ctrl Pts',(-20.4899101893572,13.8589325602149,124.040083109981)) ;
#15524=CARTESIAN_POINT('Ctrl Pts',(-20.4899249737321,13.858931209972,124.040057679799)) ;
#15525=CARTESIAN_POINT('Ctrl Pts',(-20.4899323805983,13.8589305334861,124.040044938941)) ;
#15526=CARTESIAN_POINT('Ctrl Pts',(-20.4899472258219,13.8589291775908,124.040019402016)) ;
#15527=CARTESIAN_POINT('Ctrl Pts',(-20.4899546639547,13.8589284982015,124.040006606331)) ;
#15528=CARTESIAN_POINT('Ctrl Pts',(-20.4899695730428,13.858927136377,124.039980957449)) ;
#15529=CARTESIAN_POINT('Ctrl Pts',(-20.4899770439415,13.8589264539467,124.039968104345)) ;
#15530=CARTESIAN_POINT('Ctrl Pts',(-20.4899920187781,13.8589250860198,124.039942340237)) ;
#15531=CARTESIAN_POINT('Ctrl Pts',(-20.4899995233242,13.8589244004673,124.039929428182)) ;
#15532=CARTESIAN_POINT('Ctrl Pts',(-20.490014567712,13.8589230260892,124.039903542275)) ;
#15533=CARTESIAN_POINT('Ctrl Pts',(-20.4900221074345,13.8589223372742,124.039890568624)) ;
#15534=CARTESIAN_POINT('Ctrl Pts',(-20.4900372239377,13.8589209562093,124.039864556478)) ;
#15535=CARTESIAN_POINT('Ctrl Pts',(-20.4900448004046,13.8589202639877,124.039851518516)) ;
#15536=CARTESIAN_POINT('Ctrl Pts',(-20.4900599912619,13.85891887603,124.039825376245)) ;
#15537=CARTESIAN_POINT('Ctrl Pts',(-20.4900676057556,13.858918180284,124.039812271751)) ;
#15538=CARTESIAN_POINT('Ctrl Pts',(-20.4900828737317,13.8589167851793,124.039785994564)) ;
#15539=CARTESIAN_POINT('Ctrl Pts',(-20.4900905274526,13.8589160857985,124.039772821455)) ;
#15540=CARTESIAN_POINT('Ctrl Pts',(-20.4901058758524,13.8589146832433,124.039746403629)) ;
#15541=CARTESIAN_POINT('Ctrl Pts',(-20.4901135703395,13.8589139800862,124.039733159238)) ;
#15542=CARTESIAN_POINT('Ctrl Pts',(-20.4901290017798,13.8589125698397,124.039706596234)) ;
#15543=CARTESIAN_POINT('Ctrl Pts',(-20.490136738525,13.8589118627691,124.039693277974)) ;
#15544=CARTESIAN_POINT('Ctrl Pts',(-20.4901522556526,13.8589104445877,124.039666565199)) ;
#15545=CARTESIAN_POINT('Ctrl Pts',(-20.4901600360511,13.8589097334752,124.03965317065)) ;
#15546=CARTESIAN_POINT('Ctrl Pts',(-20.4901756416255,13.858908307105,124.039626303313)) ;
#15547=CARTESIAN_POINT('Ctrl Pts',(-20.4901834669257,13.8589075918356,124.039612830306)) ;
#15548=CARTESIAN_POINT('Ctrl Pts',(-20.4901991644811,13.8589061569517,124.039585802283)) ;
#15549=CARTESIAN_POINT('Ctrl Pts',(-20.4902070363817,13.8589054373692,124.039572247872)) ;
#15550=CARTESIAN_POINT('Ctrl Pts',(-20.4902228285179,13.8589039937319,124.039545054645)) ;
#15551=CARTESIAN_POINT('Ctrl Pts',(-20.4902307486361,13.8589032696875,124.039531416024)) ;
#15552=CARTESIAN_POINT('Ctrl Pts',(-20.4902466377406,13.8589018170766,124.039504053438)) ;
#15553=CARTESIAN_POINT('Ctrl Pts',(-20.490254607265,13.8589010884606,124.039490328539)) ;
#15554=CARTESIAN_POINT('Ctrl Pts',(-20.4902705968986,13.8588996265486,124.039462790417)) ;
#15555=CARTESIAN_POINT('Ctrl Pts',(-20.4902786172617,13.858898893229,124.039448976749)) ;
#15556=CARTESIAN_POINT('Ctrl Pts',(-20.4902947108765,13.858897421698,124.039421257098)) ;
#15557=CARTESIAN_POINT('Ctrl Pts',(-20.4903027838594,13.8588966835109,124.03940735157)) ;
#15558=CARTESIAN_POINT('Ctrl Pts',(-20.490318984017,13.8588952021245,124.039379445929)) ;
#15559=CARTESIAN_POINT('Ctrl Pts',(-20.4903271111362,13.85889445893,124.039365445904)) ;
#15560=CARTESIAN_POINT('Ctrl Pts',(-20.4903434209091,13.858892967405,124.039337348932)) ;
#15561=CARTESIAN_POINT('Ctrl Pts',(-20.4903516036067,13.8588922190701,124.0393232519)) ;
#15562=CARTESIAN_POINT('Ctrl Pts',(-20.490368026599,13.8588907170744,124.039294957334)) ;
#15563=CARTESIAN_POINT('Ctrl Pts',(-20.4903762666247,13.8588899634379,124.039280760255)) ;
#15564=CARTESIAN_POINT('Ctrl Pts',(-20.4903928059815,13.8588884506815,124.039252262623)) ;
#15565=CARTESIAN_POINT('Ctrl Pts',(-20.4904011051923,13.8588876915722,124.039237962269)) ;
#15566=CARTESIAN_POINT('Ctrl Pts',(-20.4904177630321,13.8588861678587,124.039209257865)) ;
#15567=CARTESIAN_POINT('Ctrl Pts',(-20.49042612239,13.8588854031874,124.03919485255)) ;
#15568=CARTESIAN_POINT('Ctrl Pts',(-20.4904429039086,13.8588838680388,124.039165932363)) ;
#15569=CARTESIAN_POINT('Ctrl Pts',(-20.4904513255905,13.858883097605,124.039151418306)) ;
#15570=CARTESIAN_POINT('Ctrl Pts',(-20.4904682332062,13.8588815507975,124.039122278108)) ;
#15571=CARTESIAN_POINT('Ctrl Pts',(-20.4904767189753,13.8588807744384,124.039107652241)) ;
#15572=CARTESIAN_POINT('Ctrl Pts',(-20.4904937556984,13.8588792156936,124.039078286781)) ;
#15573=CARTESIAN_POINT('Ctrl Pts',(-20.4905023070026,13.8588784332754,124.039063546575)) ;
#15574=CARTESIAN_POINT('Ctrl Pts',(-20.4905194768878,13.8588768622195,124.039033948802)) ;
#15575=CARTESIAN_POINT('Ctrl Pts',(-20.4905280955026,13.8588760735782,124.039019091165)) ;
#15576=CARTESIAN_POINT('Ctrl Pts',(-20.4905454021255,13.8588744898809,124.038989254846)) ;
#15577=CARTESIAN_POINT('Ctrl Pts',(-20.4905540899291,13.8588736948431,124.038974276506)) ;
#15578=CARTESIAN_POINT('Ctrl Pts',(-20.4905715368505,13.8588720981754,124.038944195435)) ;
#15579=CARTESIAN_POINT('Ctrl Pts',(-20.4905802958176,13.8588712965588,124.038929092952)) ;
#15580=CARTESIAN_POINT('Ctrl Pts',(-20.4905978858839,13.8588696866569,124.038898762151)) ;
#15581=CARTESIAN_POINT('Ctrl Pts',(-20.4906067173874,13.8588688783342,124.038883533122)) ;
#15582=CARTESIAN_POINT('Ctrl Pts',(-20.4906244559245,13.8588672547074,124.038852943332)) ;
#15583=CARTESIAN_POINT('Ctrl Pts',(-20.4906333625065,13.8588664394441,124.038837583336)) ;
#15584=CARTESIAN_POINT('Ctrl Pts',(-20.4925060872012,13.8586950124741,124.035607785913)) ;
#15585=CARTESIAN_POINT('Ctrl Pts',(-20.4943555594237,13.8585242006034,124.032385061572)) ;
#15586=CARTESIAN_POINT('Ctrl Pts',(-20.4984073425928,13.8581466155113,124.025251295366)) ;
#15587=CARTESIAN_POINT('Ctrl Pts',(-20.5006030102197,13.8579397538586,124.021336545848)) ;
#15588=CARTESIAN_POINT('Ctrl Pts',(-20.5067339656082,13.8573557488863,124.010266070541)) ;
#15589=CARTESIAN_POINT('Ctrl Pts',(-20.5106202659879,13.8569779812798,124.003083514696)) ;
#15590=CARTESIAN_POINT('Ctrl Pts',(-20.5250084049492,13.855550733782,123.97585763689)) ;
#15591=CARTESIAN_POINT('Ctrl Pts',(-20.5350356906742,13.8544962881016,123.95556857681)) ;
#15592=CARTESIAN_POINT('Ctrl Pts',(-20.5462215008487,13.853253601279,123.931297912025)) ;
#15593=CARTESIAN_POINT('Ctrl Pts',(-20.5479180270713,13.8530631769229,123.927568714486)) ;
#15594=CARTESIAN_POINT('Ctrl Pts',(-20.5564722995342,13.8520931399368,123.908517307534)) ;
#15595=CARTESIAN_POINT('Ctrl Pts',(-20.5630392767027,13.8513157188205,123.893066300478)) ;
#15596=CARTESIAN_POINT('Ctrl Pts',(-20.5710773663457,13.8503216087064,123.873042918714)) ;
#15597=CARTESIAN_POINT('Ctrl Pts',(-20.5728360442873,13.8501012649038,123.868588055111)) ;
#15598=CARTESIAN_POINT('Ctrl Pts',(-20.5755554935889,13.8497560278985,123.861581855792)) ;
#15599=CARTESIAN_POINT('Ctrl Pts',(-20.5765335913721,13.8496309104058,123.859037308292)) ;
#15600=CARTESIAN_POINT('Ctrl Pts',(-20.5784730666476,13.8493809012957,123.853942004285)) ;
#15601=CARTESIAN_POINT('Ctrl Pts',(-20.5794344397893,13.8492560103599,123.851391262342)) ;
#15602=CARTESIAN_POINT('Ctrl Pts',(-20.5813437051298,13.8490060249524,123.846274896412)) ;
#15603=CARTESIAN_POINT('Ctrl Pts',(-20.5822915354826,13.8488809319206,123.843709265631)) ;
#15604=CARTESIAN_POINT('Ctrl Pts',(-20.5844466743752,13.8485941973408,123.837816207583)) ;
#15605=CARTESIAN_POINT('Ctrl Pts',(-20.5856482861597,13.8484326303224,123.834486719443)) ;
#15606=CARTESIAN_POINT('Ctrl Pts',(-20.5887268310778,13.8480142128925,123.825841703016)) ;
#15607=CARTESIAN_POINT('Ctrl Pts',(-20.59058198091,13.8477576376177,123.820518494502)) ;
#15608=CARTESIAN_POINT('Ctrl Pts',(-20.5961275571019,13.8469766745545,123.80425264692)) ;
#15609=CARTESIAN_POINT('Ctrl Pts',(-20.599702417897,13.8464536308975,123.793271234192)) ;
#15610=CARTESIAN_POINT('Ctrl Pts',(-20.6078865899836,13.8452052115143,123.76689442607)) ;
#15611=CARTESIAN_POINT('Ctrl Pts',(-20.6123521773435,13.8444809736554,123.751456638938)) ;
#15612=CARTESIAN_POINT('Ctrl Pts',(-20.6221057458753,13.8427831404181,123.715127918939)) ;
#15613=CARTESIAN_POINT('Ctrl Pts',(-20.6271535931931,13.8418083464274,123.69417799717)) ;
#15614=CARTESIAN_POINT('Ctrl Pts',(-20.632662572683,13.8406070400145,123.668405883066)) ;
#15615=CARTESIAN_POINT('Ctrl Pts',(-20.6336405850954,13.8403875204966,123.663697807199)) ;
#15616=CARTESIAN_POINT('Ctrl Pts',(-20.6351215793787,13.8400450546363,123.656355930081)) ;
#15617=CARTESIAN_POINT('Ctrl Pts',(-20.6356432956637,13.8399223495409,123.653725947344)) ;
#15618=CARTESIAN_POINT('Ctrl Pts',(-20.6366693634811,13.8396768262338,123.648464885835)) ;
#15619=CARTESIAN_POINT('Ctrl Pts',(-20.6371737264599,13.8395540088683,123.645833824075)) ;
#15620=CARTESIAN_POINT('Ctrl Pts',(-20.6382647529297,13.8392835638612,123.640041730175)) ;
#15621=CARTESIAN_POINT('Ctrl Pts',(-20.6388476866218,13.8391358901061,123.636880017672)) ;
#15622=CARTESIAN_POINT('Ctrl Pts',(-20.6404368331247,13.8387242872355,123.628070341032)) ;
#15623=CARTESIAN_POINT('Ctrl Pts',(-20.6414163682009,13.8384600341338,123.622417663562)) ;
#15624=CARTESIAN_POINT('Ctrl Pts',(-20.6436865203896,13.8378211990229,123.608758865712)) ;
#15625=CARTESIAN_POINT('Ctrl Pts',(-20.6449382045098,13.8374461951142,123.600746561701)) ;
#15626=CARTESIAN_POINT('Ctrl Pts',(-20.6496729280767,13.8359307419014,123.568376055449)) ;
#15627=CARTESIAN_POINT('Ctrl Pts',(-20.6525143594187,13.8347851345806,123.543929710565)) ;
#15628=CARTESIAN_POINT('Ctrl Pts',(-20.6560731010156,13.8328688437911,123.50274127297)) ;
#15629=CARTESIAN_POINT('Ctrl Pts',(-20.6571787555777,13.8320952927126,123.486039873176)) ;
#15630=CARTESIAN_POINT('Ctrl Pts',(-20.6582002209345,13.8310728765529,123.463860245269)) ;
#15631=CARTESIAN_POINT('Ctrl Pts',(-20.6584158938758,13.8308214518473,123.458397704149)) ;
#15632=CARTESIAN_POINT('Ctrl Pts',(-20.6587240404368,13.8303911552722,123.449035373961)) ;
#15633=CARTESIAN_POINT('Ctrl Pts',(-20.6588341060291,13.8302121351201,123.445136252507)) ;
#15634=CARTESIAN_POINT('Ctrl Pts',(-20.6590191586386,13.8298516231369,123.437276512479)) ;
#15635=CARTESIAN_POINT('Ctrl Pts',(-20.6590935730801,13.8296701382022,123.433315924923)) ;
#15636=CARTESIAN_POINT('Ctrl Pts',(-20.6592073956233,13.8292988307163,123.425205395734)) ;
#15637=CARTESIAN_POINT('Ctrl Pts',(-20.6592449656735,13.8291090253997,123.421055476931)) ;
#15638=CARTESIAN_POINT('Ctrl Pts',(-20.6592848914349,13.8286610542947,123.411252675077)) ;
#15639=CARTESIAN_POINT('Ctrl Pts',(-20.6592695695077,13.828403027617,123.40559980729)) ;
#15640=CARTESIAN_POINT('Ctrl Pts',(-20.6591212732369,13.8276907096031,123.389980040162)) ;
#15641=CARTESIAN_POINT('Ctrl Pts',(-20.6589074274615,13.8272369760471,123.380014318608)) ;
#15642=CARTESIAN_POINT('Ctrl Pts',(-20.6576959315526,13.825587946215,123.343772802066)) ;
#15643=CARTESIAN_POINT('Ctrl Pts',(-20.6559884885777,13.824395522853,123.317527758314)) ;
#15644=CARTESIAN_POINT('Ctrl Pts',(-20.6523816219189,13.8226905337696,123.280273378837)) ;
#15645=CARTESIAN_POINT('Ctrl Pts',(-20.6511606008671,13.8221825655415,123.269205585923)) ;
#15646=CARTESIAN_POINT('Ctrl Pts',(-20.6489900538264,13.8213755280736,123.251682299429)) ;
#15647=CARTESIAN_POINT('Ctrl Pts',(-20.6481375719521,13.8210770925249,123.245215369656)) ;
#15648=CARTESIAN_POINT('Ctrl Pts',(-20.6464332518936,13.8205132799827,123.233023662662)) ;
#15649=CARTESIAN_POINT('Ctrl Pts',(-20.6455921939868,13.8202479758133,123.227297548119)) ;
#15650=CARTESIAN_POINT('Ctrl Pts',(-20.6433621649221,13.819575707691,123.212815259956)) ;
#15651=CARTESIAN_POINT('Ctrl Pts',(-20.6419197522443,13.8191684611513,123.204067652846)) ;
#15652=CARTESIAN_POINT('Ctrl Pts',(-20.6382952721087,13.8182061765109,123.183455224921)) ;
#15653=CARTESIAN_POINT('Ctrl Pts',(-20.6360342618968,13.8176508528775,123.171605183326)) ;
#15654=CARTESIAN_POINT('Ctrl Pts',(-20.6304391192508,13.8163731021567,123.144424107673)) ;
#15655=CARTESIAN_POINT('Ctrl Pts',(-20.6269871583983,13.8156506840672,123.129119341833)) ;
#15656=CARTESIAN_POINT('Ctrl Pts',(-20.6222365092715,13.814735199601,123.109761915679)) ;
#15657=CARTESIAN_POINT('Ctrl Pts',(-20.6212039949632,13.8145404259391,123.105645421179)) ;
#15658=CARTESIAN_POINT('Ctrl Pts',(-20.6190653056221,13.8141453570206,123.097299116212)) ;
#15659=CARTESIAN_POINT('Ctrl Pts',(-20.6179578661426,13.8139450614029,123.093069701326)) ;
#15660=CARTESIAN_POINT('Ctrl Pts',(-20.6152923470607,13.8134727285282,123.083103507354)) ;
#15661=CARTESIAN_POINT('Ctrl Pts',(-20.6137154874376,13.8132008056718,123.077371858019)) ;
#15662=CARTESIAN_POINT('Ctrl Pts',(-20.6059504255896,13.8118962166956,123.049914365113)) ;
#15663=CARTESIAN_POINT('Ctrl Pts',(-20.5992179952884,13.8108659483098,123.028357208965)) ;
#15664=CARTESIAN_POINT('Ctrl Pts',(-20.5919019615583,13.8098330347236,123.006984856534)) ;
#15665=CARTESIAN_POINT('',(-18.6288026007436,14.0000000000496,122.435409149151)) ;
#15666=CARTESIAN_POINT('Origin',(-19.4092722359534,14.0000000000496,123.411814366564)) ;
#15667=CARTESIAN_POINT('Ctrl Pts',(-20.591901915765,13.7497304410597,123.00698472277)) ;
#15668=CARTESIAN_POINT('Ctrl Pts',(-20.6063625370814,13.7517786882633,123.049228630798)) ;
#15669=CARTESIAN_POINT('Ctrl Pts',(-20.618549234163,13.75381645875,123.09221653556)) ;
#15670=CARTESIAN_POINT('Ctrl Pts',(-20.628409768268,13.7558580462895,123.135764230942)) ;
#15671=CARTESIAN_POINT('Ctrl Pts',(-20.6444583543449,13.7591808473683,123.206640608462)) ;
#15672=CARTESIAN_POINT('Ctrl Pts',(-20.6542956538904,13.7625238879391,123.278781574249)) ;
#15673=CARTESIAN_POINT('Ctrl Pts',(-20.6578098406935,13.7658441537945,123.351367285367)) ;
#15674=CARTESIAN_POINT('Ctrl Pts',(-20.6613282498486,13.7691684090029,123.424040209387)) ;
#15675=CARTESIAN_POINT('Ctrl Pts',(-20.6584949399899,13.7724790496621,123.496879685578)) ;
#15676=CARTESIAN_POINT('Ctrl Pts',(-20.6493425744953,13.7758422437701,123.569057985016)) ;
#15677=CARTESIAN_POINT('Ctrl Pts',(-20.6402714976604,13.779175566962,123.640595217702)) ;
#15678=CARTESIAN_POINT('Ctrl Pts',(-20.6250273305645,13.7824798826356,123.71121346105)) ;
#15679=CARTESIAN_POINT('Ctrl Pts',(-20.6037793807761,13.7857518148978,123.780124943446)) ;
#15680=CARTESIAN_POINT('Ctrl Pts',(-20.5845554178812,13.7887120771833,123.842472219009)) ;
#15681=CARTESIAN_POINT('Ctrl Pts',(-20.5604806409632,13.791688203282,123.903216027636)) ;
#15682=CARTESIAN_POINT('Ctrl Pts',(-20.5317752294988,13.79470840778,123.961802575126)) ;
#15683=CARTESIAN_POINT('Ctrl Pts',(-20.5286018957133,13.7950422861842,123.968279217022)) ;
#15684=CARTESIAN_POINT('Ctrl Pts',(-20.5253721137233,13.7953763684717,123.974729168241)) ;
#15685=CARTESIAN_POINT('Ctrl Pts',(-20.522087337898,13.7957103411746,123.981149548122)) ;
#15686=CARTESIAN_POINT('Ctrl Pts',(-20.4891410878708,13.799060082149,124.04554585766)) ;
#15687=CARTESIAN_POINT('Ctrl Pts',(-20.4506672093765,13.8023742322835,124.106961354719)) ;
#15688=CARTESIAN_POINT('Ctrl Pts',(-20.4070969000589,13.8056510812251,124.164706085059)) ;
#15689=CARTESIAN_POINT('Ctrl Pts',(-20.3632728925256,13.8089470103785,124.222787047464)) ;
#15690=CARTESIAN_POINT('Ctrl Pts',(-20.3144647152299,13.8122732103732,124.276927063412)) ;
#15691=CARTESIAN_POINT('Ctrl Pts',(-20.2612249334786,13.8156496387038,124.32651464603)) ;
#15692=CARTESIAN_POINT('Ctrl Pts',(-20.208431235917,13.8189977766988,124.375686745416)) ;
#15693=CARTESIAN_POINT('Ctrl Pts',(-20.1514799540918,13.8222863880002,124.420195860513)) ;
#15694=CARTESIAN_POINT('Ctrl Pts',(-20.0910054456041,13.825564595863,124.459545167359)) ;
#15695=CARTESIAN_POINT('Ctrl Pts',(-20.030021323317,13.8288704289188,124.499226067637)) ;
#15696=CARTESIAN_POINT('Ctrl Pts',(-19.9656903848931,13.8322259945227,124.533506066526)) ;
#15697=CARTESIAN_POINT('Ctrl Pts',(-19.8987443715233,13.8355632563884,124.561995669045)) ;
#15698=CARTESIAN_POINT('Ctrl Pts',(-19.8709317381632,13.8369497174489,124.573831637007)) ;
#15699=CARTESIAN_POINT('Ctrl Pts',(-19.8426988053596,13.8383268906909,124.584654958882)) ;
#15700=CARTESIAN_POINT('Ctrl Pts',(-19.814101322745,13.8397085566956,124.594444237049)) ;
#15701=CARTESIAN_POINT('Ctrl Pts',(-19.7738950433856,13.8416510930409,124.608207352427)) ;
#15702=CARTESIAN_POINT('Ctrl Pts',(-19.7330136490518,13.8436023746858,124.619910968345)) ;
#15703=CARTESIAN_POINT('Ctrl Pts',(-19.6916159984558,13.8455619284086,124.629509730706)) ;
#15704=CARTESIAN_POINT('Ctrl Pts',(-19.621434395943,13.8488839676667,124.6457825509)) ;
#15705=CARTESIAN_POINT('Ctrl Pts',(-19.5499773540891,13.8521761049423,124.655957672648)) ;
#15706=CARTESIAN_POINT('Ctrl Pts',(-19.4780413667292,13.8554628014865,124.659921255708)) ;
#15707=CARTESIAN_POINT('Ctrl Pts',(-19.405565930974,13.8587741449875,124.6639145617)) ;
#15708=CARTESIAN_POINT('Ctrl Pts',(-19.3328805747897,13.8621218045964,124.661587512882)) ;
#15709=CARTESIAN_POINT('Ctrl Pts',(-19.2608092074874,13.8654379472561,124.652966544685)) ;
#15710=CARTESIAN_POINT('Ctrl Pts',(-19.1885665372109,13.868761971896,124.644325085723)) ;
#15711=CARTESIAN_POINT('Ctrl Pts',(-19.1172187765043,13.8720647651682,124.629393167417)) ;
#15712=CARTESIAN_POINT('Ctrl Pts',(-19.0475756931357,13.8754364916762,124.60834084391)) ;
#15713=CARTESIAN_POINT('Ctrl Pts',(-18.9829156430693,13.8785669677303,124.588794835518)) ;
#15714=CARTESIAN_POINT('Ctrl Pts',(-18.9199468679241,13.881670349849,124.564040084399)) ;
#15715=CARTESIAN_POINT('Ctrl Pts',(-18.8592840273916,13.884728198393,124.53431736011)) ;
#15716=CARTESIAN_POINT('Ctrl Pts',(-18.855298686588,13.8849290885668,124.532364678949)) ;
#15717=CARTESIAN_POINT('Ctrl Pts',(-18.8513235602125,13.8851299295488,124.530390680638)) ;
#15718=CARTESIAN_POINT('Ctrl Pts',(-18.8473593255089,13.8853307575762,124.528395703123)) ;
#15719=CARTESIAN_POINT('Ctrl Pts',(-18.7823244508309,13.8886254226425,124.495667289604)) ;
#15720=CARTESIAN_POINT('Ctrl Pts',(-18.7202769990253,13.8919691269502,124.457321787188)) ;
#15721=CARTESIAN_POINT('Ctrl Pts',(-18.6619196785191,13.895335505774,124.413794483619)) ;
#15722=CARTESIAN_POINT('Ctrl Pts',(-18.6038188900024,13.8986870863883,124.37045852101)) ;
#15723=CARTESIAN_POINT('Ctrl Pts',(-18.5495970331295,13.9019816026392,124.322150842453)) ;
#15724=CARTESIAN_POINT('Ctrl Pts',(-18.4998669553414,13.9052962640052,124.269416859373)) ;
#15725=CARTESIAN_POINT('Ctrl Pts',(-18.4501529716476,13.9086098526508,124.216699942537)) ;
#15726=CARTESIAN_POINT('Ctrl Pts',(-18.4051169093404,13.9119457639183,124.159759999861)) ;
#15727=CARTESIAN_POINT('Ctrl Pts',(-18.365267674092,13.9152538452324,124.099240344317)) ;
#15728=CARTESIAN_POINT('Ctrl Pts',(-18.3252556152,13.9185754433392,124.038473405963)) ;
#15729=CARTESIAN_POINT('Ctrl Pts',(-18.2906263158313,13.9218932210603,123.974330716603)) ;
#15730=CARTESIAN_POINT('Ctrl Pts',(-18.2617728896448,13.9252517568863,123.907541358262)) ;
#15731=CARTESIAN_POINT('Ctrl Pts',(-18.2488857250803,13.9267518215097,123.87771039654)) ;
#15732=CARTESIAN_POINT('Ctrl Pts',(-18.237166646834,13.928249280156,123.847388105641)) ;
#15733=CARTESIAN_POINT('Ctrl Pts',(-18.2266423654683,13.9297397117846,123.816643453356)) ;
#15734=CARTESIAN_POINT('Ctrl Pts',(-18.2137737426247,13.9315621452446,123.779050260911)) ;
#15735=CARTESIAN_POINT('Ctrl Pts',(-18.2027048827386,13.9333715008147,123.740864689436)) ;
#15736=CARTESIAN_POINT('Ctrl Pts',(-18.1934735105708,13.9351820521686,123.702216603874)) ;
#15737=CARTESIAN_POINT('Ctrl Pts',(-18.176621872162,13.9384871682643,123.631665492809)) ;
#15738=CARTESIAN_POINT('Ctrl Pts',(-18.1659433494583,13.9418197322647,123.559782448994)) ;
#15739=CARTESIAN_POINT('Ctrl Pts',(-18.161558421319,13.9451493424424,123.487380475678)) ;
#15740=CARTESIAN_POINT('Ctrl Pts',(-18.1571794512759,13.9484744284551,123.415076879786)) ;
#15741=CARTESIAN_POINT('Ctrl Pts',(-18.1590936196939,13.9517699060233,123.342529732206)) ;
#15742=CARTESIAN_POINT('Ctrl Pts',(-18.1672792240671,13.9551028655101,123.270558009178)) ;
#15743=CARTESIAN_POINT('Ctrl Pts',(-18.1754485141975,13.958429182273,123.198729728726)) ;
#15744=CARTESIAN_POINT('Ctrl Pts',(-18.1898334630847,13.9617514594568,123.127745020702)) ;
#15745=CARTESIAN_POINT('Ctrl Pts',(-18.2102729618659,13.9650365151445,123.058401377536)) ;
#15746=CARTESIAN_POINT('Ctrl Pts',(-18.2301882885713,13.9682373253976,122.990836055931)) ;
#15747=CARTESIAN_POINT('Ctrl Pts',(-18.2557778940949,13.9714482125329,122.925078207253)) ;
#15748=CARTESIAN_POINT('Ctrl Pts',(-18.2867692424076,13.9747119452089,122.861826158003)) ;
#15749=CARTESIAN_POINT('Ctrl Pts',(-18.2877875997057,13.9748191895262,122.859747733233)) ;
#15750=CARTESIAN_POINT('Ctrl Pts',(-18.2888117423678,13.9749264410021,122.857672111156)) ;
#15751=CARTESIAN_POINT('Ctrl Pts',(-18.2898416231274,13.9750336881797,122.855599387312)) ;
#15752=CARTESIAN_POINT('Ctrl Pts',(-18.3220556999662,13.9783883181092,122.790765779584)) ;
#15753=CARTESIAN_POINT('Ctrl Pts',(-18.3598411869483,13.9817039828769,122.728853071035)) ;
#15754=CARTESIAN_POINT('Ctrl Pts',(-18.4027743783516,13.9849814727061,122.67055728382)) ;
#15755=CARTESIAN_POINT('Ctrl Pts',(-18.445920839689,13.9882752434131,122.611971913224)) ;
#15756=CARTESIAN_POINT('Ctrl Pts',(-18.494096845034,13.9916059899517,122.557269259677)) ;
#15757=CARTESIAN_POINT('Ctrl Pts',(-18.5467569764074,13.9949784443263,122.507067204576)) ;
#15758=CARTESIAN_POINT('Ctrl Pts',(-18.5730635066385,13.9966631642585,122.481988613889)) ;
#15759=CARTESIAN_POINT('Ctrl Pts',(-18.6004389456167,13.9983320474216,122.458081011944)) ;
#15760=CARTESIAN_POINT('Ctrl Pts',(-18.6288026007436,14.0000000000496,122.435409149151)) ;
#15761=CARTESIAN_POINT('Origin',(-19.4092722359532,16.5113612779716,123.411814366564)) ;
#15762=CARTESIAN_POINT('',(-20.5919016415084,13.3897528569022,123.006983921601)) ;
#15763=CARTESIAN_POINT('',(-20.5919016872816,13.4498327922206,123.006984055316)) ;
#15764=CARTESIAN_POINT('',(-20.5919021064381,16.5113612779716,123.006985279772)) ;
#15765=CARTESIAN_POINT('Ctrl Pts',(-20.5919019615583,13.8098330347217,123.006984856534)) ;
#15766=CARTESIAN_POINT('Ctrl Pts',(-20.5796177619238,13.8080986910531,122.971098985364)) ;
#15767=CARTESIAN_POINT('Ctrl Pts',(-20.5657063569306,13.8063585292808,122.935791351964)) ;
#15768=CARTESIAN_POINT('Ctrl Pts',(-20.5502165472103,13.8046080448643,122.901181348942)) ;
#15769=CARTESIAN_POINT('Ctrl Pts',(-20.520770181677,13.8012803471765,122.835387203082)) ;
#15770=CARTESIAN_POINT('Ctrl Pts',(-20.4856929834176,13.7979653615935,122.77227295707)) ;
#15771=CARTESIAN_POINT('Ctrl Pts',(-20.4453721849218,13.7947034100367,122.712531236621)) ;
#15772=CARTESIAN_POINT('Ctrl Pts',(-20.4046683728878,13.7914104726945,122.652222020274)) ;
#15773=CARTESIAN_POINT('Ctrl Pts',(-20.3587800304366,13.7880836260627,122.595586200155)) ;
#15774=CARTESIAN_POINT('Ctrl Pts',(-20.3082259775898,13.7847053333764,122.543262600419)) ;
#15775=CARTESIAN_POINT('Ctrl Pts',(-20.2580339768125,13.7813512349492,122.491313725686)) ;
#15776=CARTESIAN_POINT('Ctrl Pts',(-20.2034335311599,13.7780588930693,122.443813244608)) ;
#15777=CARTESIAN_POINT('Ctrl Pts',(-20.1450350735511,13.7747785422853,122.401293190692)) ;
#15778=CARTESIAN_POINT('Ctrl Pts',(-20.0864707072361,13.7714888720984,122.358652338258)) ;
#15779=CARTESIAN_POINT('Ctrl Pts',(-20.0243124708696,13.7681516077852,122.321184637964)) ;
#15780=CARTESIAN_POINT('Ctrl Pts',(-19.959260294232,13.7648235341903,122.289311299385)) ;
#15781=CARTESIAN_POINT('Ctrl Pts',(-19.9590204835755,13.7648112654615,122.289193800377)) ;
#15782=CARTESIAN_POINT('Ctrl Pts',(-19.9587804848829,13.7647989897311,122.289076304615)) ;
#15783=CARTESIAN_POINT('Ctrl Pts',(-19.9585405969292,13.7647867222929,122.288958958372)) ;
#15784=CARTESIAN_POINT('Ctrl Pts',(-19.8932580416504,13.7614482898999,122.257024622146)) ;
#15785=CARTESIAN_POINT('Ctrl Pts',(-19.8253154321585,13.7581503872716,122.230844614302)) ;
#15786=CARTESIAN_POINT('Ctrl Pts',(-19.7554846306214,13.7547995544403,122.210716128345)) ;
#15787=CARTESIAN_POINT('Ctrl Pts',(-19.6860504463898,13.7514677533008,122.190701965948)) ;
#15788=CARTESIAN_POINT('Ctrl Pts',(-19.6150115325245,13.7481451053711,122.176746188182)) ;
#15789=CARTESIAN_POINT('Ctrl Pts',(-19.5431634314469,13.7448689186883,122.169005794078)) ;
#15790=CARTESIAN_POINT('Ctrl Pts',(-19.4708701670743,13.7415724330966,122.161217441304)) ;
#15791=CARTESIAN_POINT('Ctrl Pts',(-19.3980395735329,13.738248527013,122.159751929489)) ;
#15792=CARTESIAN_POINT('Ctrl Pts',(-19.3254946073445,13.7348767418505,122.164625002826)) ;
#15793=CARTESIAN_POINT('Ctrl Pts',(-19.253365677566,13.7315242934589,122.169470129691)) ;
#15794=CARTESIAN_POINT('Ctrl Pts',(-19.1817924542661,13.7282254390405,122.180562543553)) ;
#15795=CARTESIAN_POINT('Ctrl Pts',(-19.1115674292446,13.7249412096492,122.197783128029)) ;
#15796=CARTESIAN_POINT('Ctrl Pts',(-19.0754163348061,13.7232505233612,122.206648101385)) ;
#15797=CARTESIAN_POINT('Ctrl Pts',(-19.0396689861174,13.7215545046655,122.217126244833)) ;
#15798=CARTESIAN_POINT('Ctrl Pts',(-19.004443029643,13.7198446883909,122.229184536992)) ;
#15799=CARTESIAN_POINT('Ctrl Pts',(-18.9708669395833,13.7182149542128,122.240678058929)) ;
#15800=CARTESIAN_POINT('Ctrl Pts',(-18.9377955116159,13.7165744351769,122.253596611336)) ;
#15801=CARTESIAN_POINT('Ctrl Pts',(-18.9053287039429,13.7149435467734,122.267899633457)) ;
#15802=CARTESIAN_POINT('Ctrl Pts',(-18.8390299193649,13.7116131941244,122.297107093332)) ;
#15803=CARTESIAN_POINT('Ctrl Pts',(-18.7754054879488,13.7083272240729,122.332018128119)) ;
#15804=CARTESIAN_POINT('Ctrl Pts',(-18.7151634716232,13.7049882872184,122.372240885104)) ;
#15805=CARTESIAN_POINT('Ctrl Pts',(-18.6552481525976,13.701667457687,122.412245510842)) ;
#15806=CARTESIAN_POINT('Ctrl Pts',(-18.5989034145165,13.6983525297203,122.45735485489)) ;
#15807=CARTESIAN_POINT('Ctrl Pts',(-18.5467568890626,13.6950873699958,122.507067287843)) ;
#15808=CARTESIAN_POINT('Ctrl Pts',(-18.49409422378,13.6917898921261,122.557271768281)) ;
#15809=CARTESIAN_POINT('Ctrl Pts',(-18.445918683257,13.6884646048685,122.611974839834)) ;
#15810=CARTESIAN_POINT('Ctrl Pts',(-18.4027743696019,13.6850888225092,122.6705572957)) ;
#15811=CARTESIAN_POINT('Ctrl Pts',(-18.3598432833932,13.6817297239117,122.728850225869)) ;
#15812=CARTESIAN_POINT('Ctrl Pts',(-18.3220572040567,13.6784213609289,122.790762571335)) ;
#15813=CARTESIAN_POINT('Ctrl Pts',(-18.2898410039093,13.6751395513273,122.855600633544)) ;
#15814=CARTESIAN_POINT('Ctrl Pts',(-18.2888117333323,13.6750347012815,122.85767213513)) ;
#15815=CARTESIAN_POINT('Ctrl Pts',(-18.2877875931879,13.6749297900114,122.859747751965)) ;
#15816=CARTESIAN_POINT('Ctrl Pts',(-18.2867698102722,13.6748249334085,122.861824999016)) ;
#15817=CARTESIAN_POINT('Ctrl Pts',(-18.2557765411956,13.6716318665394,122.925080803166)) ;
#15818=CARTESIAN_POINT('Ctrl Pts',(-18.2301875245126,13.6683978244689,122.990838860913)) ;
#15819=CARTESIAN_POINT('Ctrl Pts',(-18.2102732637651,13.6651413129147,123.058400353306)) ;
#15820=CARTESIAN_POINT('Ctrl Pts',(-18.189833938375,13.6617989393195,123.127743189796)) ;
#15821=CARTESIAN_POINT('Ctrl Pts',(-18.1754487613198,13.6585066721384,123.198727822783)) ;
#15822=CARTESIAN_POINT('Ctrl Pts',(-18.1672792829945,13.6552066817733,123.270557491061)) ;
#15823=CARTESIAN_POINT('Ctrl Pts',(-18.1590935425314,13.6519001224578,123.342530143251)) ;
#15824=CARTESIAN_POINT('Ctrl Pts',(-18.1571794535857,13.6485680833321,123.415077287784)) ;
#15825=CARTESIAN_POINT('Ctrl Pts',(-18.1615584446444,13.645252454877,123.487380860816)) ;
#15826=CARTESIAN_POINT('Ctrl Pts',(-18.1659434387934,13.6419322810787,123.559783553686)) ;
#15827=CARTESIAN_POINT('Ctrl Pts',(-18.1766215634281,13.6386285943287,123.631666966055)) ;
#15828=CARTESIAN_POINT('Ctrl Pts',(-18.1934760829817,13.6352843211117,123.702227373324)) ;
#15829=CARTESIAN_POINT('Ctrl Pts',(-18.2027050724799,13.6334531053182,123.740863969023)) ;
#15830=CARTESIAN_POINT('Ctrl Pts',(-18.2137735295612,13.6316221081851,123.779049754104)) ;
#15831=CARTESIAN_POINT('Ctrl Pts',(-18.2266427469473,13.6298019695379,123.816644567771)) ;
#15832=CARTESIAN_POINT('Ctrl Pts',(-18.2371665378509,13.6283135528017,123.84738769272)) ;
#15833=CARTESIAN_POINT('Ctrl Pts',(-18.2488858666179,13.626833215586,123.877709981225)) ;
#15834=CARTESIAN_POINT('Ctrl Pts',(-18.2617683941932,13.6253549862017,123.907530952147)) ;
#15835=CARTESIAN_POINT('Ctrl Pts',(-18.2906263032546,13.6220436322074,123.974332351326)) ;
#15836=CARTESIAN_POINT('Ctrl Pts',(-18.3252565395882,13.6187053027923,124.038474850358)) ;
#15837=CARTESIAN_POINT('Ctrl Pts',(-18.3652678845994,13.6153568405027,124.099240664017)) ;
#15838=CARTESIAN_POINT('Ctrl Pts',(-18.4051167833731,13.6120219729847,124.159759768204)) ;
#15839=CARTESIAN_POINT('Ctrl Pts',(-18.4501528084057,13.6087279356488,124.216699732329)) ;
#15840=CARTESIAN_POINT('Ctrl Pts',(-18.4998666540437,13.6053999030847,124.269416539875)) ;
#15841=CARTESIAN_POINT('Ctrl Pts',(-18.5495958694593,13.6020708416096,124.322149645609)) ;
#15842=CARTESIAN_POINT('Ctrl Pts',(-18.6038175488692,13.5987334322945,124.37045756425)) ;
#15843=CARTESIAN_POINT('Ctrl Pts',(-18.6619201611746,13.5954399239144,124.413794843619)) ;
#15844=CARTESIAN_POINT('Ctrl Pts',(-18.7202796504269,13.5921318546333,124.457323721052)) ;
#15845=CARTESIAN_POINT('Ctrl Pts',(-18.7823273457249,13.5888152394048,124.495668911736)) ;
#15846=CARTESIAN_POINT('Ctrl Pts',(-18.8473615900167,13.5854360760084,124.52839684272)) ;
#15847=CARTESIAN_POINT('Ctrl Pts',(-18.8513236554735,13.5852302080581,124.530390718504)) ;
#15848=CARTESIAN_POINT('Ctrl Pts',(-18.8552987755696,13.5850242107854,124.532364714391)) ;
#15849=CARTESIAN_POINT('Ctrl Pts',(-18.8592821745989,13.5848183791732,124.534316452303)) ;
#15850=CARTESIAN_POINT('Ctrl Pts',(-18.9199438203079,13.5816838490294,124.564038715334)) ;
#15851=CARTESIAN_POINT('Ctrl Pts',(-18.9829124758655,13.5786047482829,124.588793676453)) ;
#15852=CARTESIAN_POINT('Ctrl Pts',(-19.0475722740586,13.5755435395108,124.608339810356)) ;
#15853=CARTESIAN_POINT('Ctrl Pts',(-19.117220902973,13.5722461429869,124.629394027427)) ;
#15854=CARTESIAN_POINT('Ctrl Pts',(-19.1885687370152,13.5688927764746,124.644325376909)) ;
#15855=CARTESIAN_POINT('Ctrl Pts',(-19.2608096826416,13.5655463761473,124.652966601522)) ;
#15856=CARTESIAN_POINT('Ctrl Pts',(-19.3328807626323,13.5622078444659,124.661587507365)) ;
#15857=CARTESIAN_POINT('Ctrl Pts',(-19.4055661388187,13.5589148053625,124.663914556485)) ;
#15858=CARTESIAN_POINT('Ctrl Pts',(-19.4780414738124,13.5555729255004,124.659921249808)) ;
#15859=CARTESIAN_POINT('Ctrl Pts',(-19.5499757422459,13.5522559945321,124.655957755269)) ;
#15860=CARTESIAN_POINT('Ctrl Pts',(-19.6214331874791,13.5489555682235,124.645783470017)) ;
#15861=CARTESIAN_POINT('Ctrl Pts',(-19.6916265174306,13.5456732478082,124.629507291651)) ;
#15862=CARTESIAN_POINT('Ctrl Pts',(-19.7330142124773,13.543737911837,124.61991046091)) ;
#15863=CARTESIAN_POINT('Ctrl Pts',(-19.7738957834929,13.5417967144381,124.608207162694)) ;
#15864=CARTESIAN_POINT('Ctrl Pts',(-19.8141029976705,13.5398436253417,124.5944436637)) ;
#15865=CARTESIAN_POINT('Ctrl Pts',(-19.8426986118306,13.5384545765513,124.584654979883)) ;
#15866=CARTESIAN_POINT('Ctrl Pts',(-19.8709315370337,13.5370615910196,124.573831438472)) ;
#15867=CARTESIAN_POINT('Ctrl Pts',(-19.8987344214074,13.5356773831792,124.561999903374)) ;
#15868=CARTESIAN_POINT('Ctrl Pts',(-19.9656917047657,13.5323438155049,124.533506188929)) ;
#15869=CARTESIAN_POINT('Ctrl Pts',(-20.03002253282,13.529042948606,124.499225290944)) ;
#15870=CARTESIAN_POINT('Ctrl Pts',(-20.0910055699437,13.5256800175593,124.459545086455)) ;
#15871=CARTESIAN_POINT('Ctrl Pts',(-20.1514772664395,13.5223452845715,124.420197599088)) ;
#15872=CARTESIAN_POINT('Ctrl Pts',(-20.2084289118012,13.5190323972408,124.375688905688)) ;
#15873=CARTESIAN_POINT('Ctrl Pts',(-20.2612248925498,13.5157666958334,124.326514684151)) ;
#15874=CARTESIAN_POINT('Ctrl Pts',(-20.3144674343984,13.5124733723383,124.276924535225)) ;
#15875=CARTESIAN_POINT('Ctrl Pts',(-20.3632751289368,13.509143443657,124.222784087567)) ;
#15876=CARTESIAN_POINT('Ctrl Pts',(-20.4070969254272,13.5057697249261,124.164706051438)) ;
#15877=CARTESIAN_POINT('Ctrl Pts',(-20.4506651917908,13.5024155247774,124.106964024625)) ;
#15878=CARTESIAN_POINT('Ctrl Pts',(-20.4891397541629,13.4991114205771,124.045548950693)) ;
#15879=CARTESIAN_POINT('Ctrl Pts',(-20.5220890806921,13.4958301620486,123.981146141667)) ;
#15880=CARTESIAN_POINT('Ctrl Pts',(-20.5253722816855,13.495503204493,123.974728791485)) ;
#15881=CARTESIAN_POINT('Ctrl Pts',(-20.5286020647114,13.4951760805788,123.968278837046)) ;
#15882=CARTESIAN_POINT('Ctrl Pts',(-20.5317740529339,13.4948489720632,123.961804976439)) ;
#15883=CARTESIAN_POINT('Ctrl Pts',(-20.5604819830401,13.4918884918396,123.903213605737)) ;
#15884=CARTESIAN_POINT('Ctrl Pts',(-20.5845560403659,13.4888934110731,123.842469535021)) ;
#15885=CARTESIAN_POINT('Ctrl Pts',(-20.6037782743388,13.4858731327153,123.780128531831)) ;
#15886=CARTESIAN_POINT('Ctrl Pts',(-20.6250267095882,13.4825344890795,123.711216210218)) ;
#15887=CARTESIAN_POINT('Ctrl Pts',(-20.6402710993088,13.4792407703463,123.640598033625)) ;
#15888=CARTESIAN_POINT('Ctrl Pts',(-20.6493424851837,13.4759642590232,123.569058689353)) ;
#15889=CARTESIAN_POINT('Ctrl Pts',(-20.6584952131101,13.4726583676079,123.496877860185)) ;
#15890=CARTESIAN_POINT('Ctrl Pts',(-20.6613281797614,13.4693126707748,123.424038400504)) ;
#15891=CARTESIAN_POINT('Ctrl Pts',(-20.6578098261807,13.4659667790302,123.351366985605)) ;
#15892=CARTESIAN_POINT('Ctrl Pts',(-20.6542956434512,13.462624853691,123.278781719428)) ;
#15893=CARTESIAN_POINT('Ctrl Pts',(-20.6444589385975,13.4593193451983,123.206640390291)) ;
#15894=CARTESIAN_POINT('Ctrl Pts',(-20.6284074207966,13.4559805354722,123.135753863861)) ;
#15895=CARTESIAN_POINT('Ctrl Pts',(-20.6185489584221,13.4539299175512,123.092217036856)) ;
#15896=CARTESIAN_POINT('Ctrl Pts',(-20.6063626760676,13.4518776618907,123.049228894074)) ;
#15897=CARTESIAN_POINT('Ctrl Pts',(-20.5919016872896,13.4498327922206,123.006984055313)) ;
#15898=CARTESIAN_POINT('Ctrl Pts',(-20.5919016415084,13.3897528569022,123.006983921601)) ;
#15899=CARTESIAN_POINT('Ctrl Pts',(-20.6096080658287,13.392266476473,123.058709815247)) ;
#15900=CARTESIAN_POINT('Ctrl Pts',(-20.6239017189868,13.3947672797745,123.111540715973)) ;
#15901=CARTESIAN_POINT('Ctrl Pts',(-20.6346907958086,13.3972573925309,123.165137749842)) ;
#15902=CARTESIAN_POINT('Ctrl Pts',(-20.6490396665439,13.4005691036854,123.236418817118)) ;
#15903=CARTESIAN_POINT('Ctrl Pts',(-20.6571413877915,13.403889973363,123.30881366061)) ;
#15904=CARTESIAN_POINT('Ctrl Pts',(-20.6589046230443,13.4072487960544,123.381501049216)) ;
#15905=CARTESIAN_POINT('Ctrl Pts',(-20.6606582369518,13.4105892908493,123.453791808687)) ;
#15906=CARTESIAN_POINT('Ctrl Pts',(-20.6561356733065,13.4138934854337,123.526098736805)) ;
#15907=CARTESIAN_POINT('Ctrl Pts',(-20.6453871553045,13.4171859802309,123.597609700824)) ;
#15908=CARTESIAN_POINT('Ctrl Pts',(-20.6345984778003,13.4204907767195,123.669387850024)) ;
#15909=CARTESIAN_POINT('Ctrl Pts',(-20.6175786325927,13.4238226028832,123.740088534419)) ;
#15910=CARTESIAN_POINT('Ctrl Pts',(-20.5945206605617,13.4271604423045,123.808911548673)) ;
#15911=CARTESIAN_POINT('Ctrl Pts',(-20.5770011918516,13.4296965358179,123.861203339258)) ;
#15912=CARTESIAN_POINT('Ctrl Pts',(-20.5560402721388,13.4322145441203,123.912278635198)) ;
#15913=CARTESIAN_POINT('Ctrl Pts',(-20.5317752294988,13.4347408220453,123.961802575126)) ;
#15914=CARTESIAN_POINT('Ctrl Pts',(-20.5242004077163,13.4355294505814,123.977262470437)) ;
#15915=CARTESIAN_POINT('Ctrl Pts',(-20.5163070208699,13.4363184440496,123.992564200258)) ;
#15916=CARTESIAN_POINT('Ctrl Pts',(-20.5081001234656,13.4371083476146,124.007697974076)) ;
#15917=CARTESIAN_POINT('Ctrl Pts',(-20.4735348526787,13.4404352115042,124.071437407417)) ;
#15918=CARTESIAN_POINT('Ctrl Pts',(-20.433488919695,13.4437694104166,124.132048922023)) ;
#15919=CARTESIAN_POINT('Ctrl Pts',(-20.3884151303904,13.4470728117549,124.188846664702)) ;
#15920=CARTESIAN_POINT('Ctrl Pts',(-20.3431867001421,13.4503875465335,124.245839271329)) ;
#15921=CARTESIAN_POINT('Ctrl Pts',(-20.2930704869686,13.4537058462015,124.298772133185)) ;
#15922=CARTESIAN_POINT('Ctrl Pts',(-20.238635611067,13.4570713797941,124.347045029072)) ;
#15923=CARTESIAN_POINT('Ctrl Pts',(-20.1847124380153,13.4604052764426,124.394864146422)) ;
#15924=CARTESIAN_POINT('Ctrl Pts',(-20.1267546075334,13.4636964169222,124.43793023851)) ;
#15925=CARTESIAN_POINT('Ctrl Pts',(-20.0654077536679,13.4669761165231,124.47576275933)) ;
#15926=CARTESIAN_POINT('Ctrl Pts',(-20.003741022508,13.4702729172688,124.51379254804)) ;
#15927=CARTESIAN_POINT('Ctrl Pts',(-19.9388859742016,13.4735980873333,124.54638833385)) ;
#15928=CARTESIAN_POINT('Ctrl Pts',(-19.8715743626068,13.4769325967039,124.573182845458)) ;
#15929=CARTESIAN_POINT('Ctrl Pts',(-19.8525933543406,13.4778728854361,124.580738552924)) ;
#15930=CARTESIAN_POINT('Ctrl Pts',(-19.8334299159491,13.4788116501096,124.587827816366)) ;
#15931=CARTESIAN_POINT('Ctrl Pts',(-19.814101322745,13.4797497313322,124.594444237049)) ;
#15932=CARTESIAN_POINT('Ctrl Pts',(-19.7646216857739,13.4821511434707,124.611381739432)) ;
#15933=CARTESIAN_POINT('Ctrl Pts',(-19.7141274172429,13.4845467399973,124.625197452426)) ;
#15934=CARTESIAN_POINT('Ctrl Pts',(-19.6629163446019,13.4869312681577,124.635809736745)) ;
#15935=CARTESIAN_POINT('Ctrl Pts',(-19.5916722453883,13.4902485890432,124.650573392296)) ;
#15936=CARTESIAN_POINT('Ctrl Pts',(-19.5192774247709,13.4935649815752,124.65908828476)) ;
#15937=CARTESIAN_POINT('Ctrl Pts',(-19.4465542531183,13.4969299197589,124.661258263373)) ;
#15938=CARTESIAN_POINT('Ctrl Pts',(-19.3744768420486,13.5002649782716,124.663408973207)) ;
#15939=CARTESIAN_POINT('Ctrl Pts',(-19.3023484006358,13.5035681505303,124.659318872779)) ;
#15940=CARTESIAN_POINT('Ctrl Pts',(-19.2309733580835,13.5068398475563,124.649032823518)) ;
#15941=CARTESIAN_POINT('Ctrl Pts',(-19.1592461784923,13.5101276858784,124.638696026841)) ;
#15942=CARTESIAN_POINT('Ctrl Pts',(-19.0885571371086,13.5134426445569,124.622142011887)) ;
#15943=CARTESIAN_POINT('Ctrl Pts',(-19.0197012273749,13.5167985406652,124.599557785553)) ;
#15944=CARTESIAN_POINT('Ctrl Pts',(-18.9647857648684,13.5194750079085,124.581545922239)) ;
#15945=CARTESIAN_POINT('Ctrl Pts',(-18.911185101128,13.5221350524653,124.559747117296)) ;
#15946=CARTESIAN_POINT('Ctrl Pts',(-18.8592840273916,13.5247629594564,124.53431736011)) ;
#15947=CARTESIAN_POINT('Ctrl Pts',(-18.8462460429093,13.5254231117058,124.527929192087)) ;
#15948=CARTESIAN_POINT('Ctrl Pts',(-18.8333202942993,13.5260815641942,124.521314326895)) ;
#15949=CARTESIAN_POINT('Ctrl Pts',(-18.8205126727063,13.5267392402366,124.514475772782)) ;
#15950=CARTESIAN_POINT('Ctrl Pts',(-18.7563299793194,13.5300350449625,124.480205801679)) ;
#15951=CARTESIAN_POINT('Ctrl Pts',(-18.6952661557814,13.5333610765098,124.440400107414)) ;
#15952=CARTESIAN_POINT('Ctrl Pts',(-18.6380110606181,13.5367375625947,124.395509542671)) ;
#15953=CARTESIAN_POINT('Ctrl Pts',(-18.5812356069805,13.5400857629362,124.350995038416)) ;
#15954=CARTESIAN_POINT('Ctrl Pts',(-18.5284206806311,13.5433742750728,124.301649181655)) ;
#15955=CARTESIAN_POINT('Ctrl Pts',(-18.4801555612243,13.5466520760842,124.248021401225)) ;
#15956=CARTESIAN_POINT('Ctrl Pts',(-18.4314837544484,13.5499574962186,124.193941747036)) ;
#15957=CARTESIAN_POINT('Ctrl Pts',(-18.3876273377621,13.5533138836049,124.135717018223)) ;
#15958=CARTESIAN_POINT('Ctrl Pts',(-18.3490847229093,13.5566501206704,124.074009532102)) ;
#15959=CARTESIAN_POINT('Ctrl Pts',(-18.3105665437652,13.5599842425884,124.012341168032)) ;
#15960=CARTESIAN_POINT('Ctrl Pts',(-18.2775029179448,13.563284743103,123.947430551321)) ;
#15961=CARTESIAN_POINT('Ctrl Pts',(-18.2502692690622,13.5666414760701,123.880015309337)) ;
#15962=CARTESIAN_POINT('Ctrl Pts',(-18.2418235197772,13.5676824722722,123.85910837049)) ;
#15963=CARTESIAN_POINT('Ctrl Pts',(-18.2339450036271,13.5687245182647,123.837976698179)) ;
#15964=CARTESIAN_POINT('Ctrl Pts',(-18.2266423654683,13.56976307206,123.816643453356)) ;
#15965=CARTESIAN_POINT('Ctrl Pts',(-18.2106069186927,13.5720435731261,123.769798997357)) ;
#15966=CARTESIAN_POINT('Ctrl Pts',(-18.1973688323647,13.5742977726772,123.722043018589)) ;
#15967=CARTESIAN_POINT('Ctrl Pts',(-18.1869980402704,13.5765479499922,123.673626877044)) ;
#15968=CARTESIAN_POINT('Ctrl Pts',(-18.1717848592061,13.5798487928408,123.602603996529)) ;
#15969=CARTESIAN_POINT('Ctrl Pts',(-18.1627913440007,13.5831792810849,123.530392408845)) ;
#15970=CARTESIAN_POINT('Ctrl Pts',(-18.160118757509,13.5865286217716,123.457809881199)) ;
#15971=CARTESIAN_POINT('Ctrl Pts',(-18.1574433894047,13.5898814484327,123.385151810077)) ;
#15972=CARTESIAN_POINT('Ctrl Pts',(-18.1611123933561,13.5932104436744,123.312397800328)) ;
#15973=CARTESIAN_POINT('Ctrl Pts',(-18.1710845532211,13.596519480288,123.240375565803)) ;
#15974=CARTESIAN_POINT('Ctrl Pts',(-18.1810633531557,13.5998307202592,123.168305374501)) ;
#15975=CARTESIAN_POINT('Ctrl Pts',(-18.1973148957516,13.6031493528183,123.097246856212)) ;
#15976=CARTESIAN_POINT('Ctrl Pts',(-18.2196541162406,13.6065167629075,123.028006173156)) ;
#15977=CARTESIAN_POINT('Ctrl Pts',(-18.2380205748496,13.6092853195836,122.971079113412)) ;
#15978=CARTESIAN_POINT('Ctrl Pts',(-18.2604495238595,13.6120345366518,122.915543605758)) ;
#15979=CARTESIAN_POINT('Ctrl Pts',(-18.2867692424076,13.6147532278699,122.861826158003)) ;
#15980=CARTESIAN_POINT('Ctrl Pts',(-18.292140428932,13.6153080437433,122.85086379034)) ;
#15981=CARTESIAN_POINT('Ctrl Pts',(-18.297671923081,13.6158620502894,122.839980677052)) ;
#15982=CARTESIAN_POINT('Ctrl Pts',(-18.30336194444,13.6164161328298,122.829180324304)) ;
#15983=CARTESIAN_POINT('Ctrl Pts',(-18.3371257771952,13.6197039852025,122.765092462256)) ;
#15984=CARTESIAN_POINT('Ctrl Pts',(-18.3763951344284,13.6230215899451,122.704063178082)) ;
#15985=CARTESIAN_POINT('Ctrl Pts',(-18.4207275060417,13.6263692488929,122.646778866055)) ;
#15986=CARTESIAN_POINT('Ctrl Pts',(-18.4651039227243,13.6297202338046,122.589437640955)) ;
#15987=CARTESIAN_POINT('Ctrl Pts',(-18.5143858945347,13.6330437932077,122.536065466233)) ;
#15988=CARTESIAN_POINT('Ctrl Pts',(-18.5680171014335,13.6363321986858,122.48726593694)) ;
#15989=CARTESIAN_POINT('Ctrl Pts',(-18.6218324962497,13.6396318976735,122.438298813364)) ;
#15990=CARTESIAN_POINT('Ctrl Pts',(-18.6798167018632,13.6429488094819,122.394126811195)) ;
#15991=CARTESIAN_POINT('Ctrl Pts',(-18.7413133163744,13.6463290970248,122.355248759595)) ;
#15992=CARTESIAN_POINT('Ctrl Pts',(-18.8022079204943,13.6496762938318,122.316751297906)) ;
#15993=CARTESIAN_POINT('Ctrl Pts',(-18.8663156296209,13.6529695807162,122.283590577323)) ;
#15994=CARTESIAN_POINT('Ctrl Pts',(-18.9329263684835,13.6562281778483,122.256135079469)) ;
#15995=CARTESIAN_POINT('Ctrl Pts',(-18.9564852890182,13.6573806801655,122.246424604804)) ;
#15996=CARTESIAN_POINT('Ctrl Pts',(-18.9803352804135,13.6585348629319,122.237436922923)) ;
#15997=CARTESIAN_POINT('Ctrl Pts',(-19.0044431491614,13.6596978079258,122.229184496079)) ;
#15998=CARTESIAN_POINT('Ctrl Pts',(-19.0491410660855,13.6618540009626,122.213883836641)) ;
#15999=CARTESIAN_POINT('Ctrl Pts',(-19.0946693789181,13.6640443093058,122.201129870366)) ;
#16000=CARTESIAN_POINT('Ctrl Pts',(-19.1408100100882,13.666225029951,122.190983488285)) ;
#16001=CARTESIAN_POINT('Ctrl Pts',(-19.2115557014482,13.6695686467546,122.17542642292)) ;
#16002=CARTESIAN_POINT('Ctrl Pts',(-19.2835202288677,13.67285510112,122.166048117887)) ;
#16003=CARTESIAN_POINT('Ctrl Pts',(-19.3558911093926,13.6761779698804,122.162954704551)) ;
#16004=CARTESIAN_POINT('Ctrl Pts',(-19.4281174154066,13.6794942005824,122.159867470894)) ;
#16005=CARTESIAN_POINT('Ctrl Pts',(-19.5004757896116,13.6828224045214,122.163051673021)) ;
#16006=CARTESIAN_POINT('Ctrl Pts',(-19.572152935276,13.6861112181146,122.172471848184)) ;
#16007=CARTESIAN_POINT('Ctrl Pts',(-19.6442912188223,13.6894211904262,122.181952628435)) ;
#16008=CARTESIAN_POINT('Ctrl Pts',(-19.7154607876134,13.6927382445772,122.197713058344)) ;
#16009=CARTESIAN_POINT('Ctrl Pts',(-19.7848547858062,13.6961082030634,122.219573724612)) ;
#16010=CARTESIAN_POINT('Ctrl Pts',(-19.8446557588647,13.6990122985457,122.238412372747)) ;
#16011=CARTESIAN_POINT('Ctrl Pts',(-19.9029549380021,13.7018952591033,122.261723593888)) ;
#16012=CARTESIAN_POINT('Ctrl Pts',(-19.9592604445148,13.7047397236552,122.289311373019)) ;
#16013=CARTESIAN_POINT('Ctrl Pts',(-19.9679555433876,13.7051789862079,122.293571675111)) ;
#16014=CARTESIAN_POINT('Ctrl Pts',(-19.9766008662182,13.7056176176954,122.297932873291)) ;
#16015=CARTESIAN_POINT('Ctrl Pts',(-19.9851946599321,13.7060559914406,122.30239408478)) ;
#16016=CARTESIAN_POINT('Ctrl Pts',(-20.0497714252281,13.709350084759,122.335917184919)) ;
#16017=CARTESIAN_POINT('Ctrl Pts',(-20.111293772392,13.712680504547,122.375011977987)) ;
#16018=CARTESIAN_POINT('Ctrl Pts',(-20.16906659148,13.7160531847087,122.419235635488)) ;
#16019=CARTESIAN_POINT('Ctrl Pts',(-20.2262590038304,13.7193919816997,122.463015006053)) ;
#16020=CARTESIAN_POINT('Ctrl Pts',(-20.2795606967903,13.7226699814663,122.511655498151)) ;
#16021=CARTESIAN_POINT('Ctrl Pts',(-20.3283780924974,13.7259502118371,122.5646163823)) ;
#16022=CARTESIAN_POINT('Ctrl Pts',(-20.3775137405789,13.7292518268207,122.617922531223)) ;
#16023=CARTESIAN_POINT('Ctrl Pts',(-20.4219183778006,13.7325911038699,122.675401764479)) ;
#16024=CARTESIAN_POINT('Ctrl Pts',(-20.4610902269716,13.7359119352449,122.736404184641)) ;
#16025=CARTESIAN_POINT('Ctrl Pts',(-20.5004286853823,13.7392468910794,122.797666065795)) ;
#16026=CARTESIAN_POINT('Ctrl Pts',(-20.5343394352926,13.7425656777551,122.862247058436)) ;
#16027=CARTESIAN_POINT('Ctrl Pts',(-20.5624361654185,13.7459160952872,122.929411058267)) ;
#16028=CARTESIAN_POINT('Ctrl Pts',(-20.5731138668484,13.7471893665154,122.954935634751)) ;
#16029=CARTESIAN_POINT('Ctrl Pts',(-20.5829411995565,13.748461219154,122.980807763874)) ;
#16030=CARTESIAN_POINT('Ctrl Pts',(-20.591901915765,13.7497304410597,123.00698472277)) ;
#16031=CARTESIAN_POINT('Origin',(-19.4092722359532,16.5113612779716,123.411814366564)) ;
#16032=CARTESIAN_POINT('',(-20.5919013672866,13.0298207905601,123.006983120533)) ;
#16033=CARTESIAN_POINT('',(-20.5919014130239,13.0898536069789,123.006983254143)) ;
#16034=CARTESIAN_POINT('',(-20.5919021064381,16.5113612779716,123.006985279772)) ;
#16035=CARTESIAN_POINT('Ctrl Pts',(-20.5919016872895,13.4498327922206,123.006984055313)) ;
#16036=CARTESIAN_POINT('Ctrl Pts',(-20.5829410927979,13.44856571106,122.980807500216)) ;
#16037=CARTESIAN_POINT('Ctrl Pts',(-20.5731135903211,13.4473019494881,122.954935597809)) ;
#16038=CARTESIAN_POINT('Ctrl Pts',(-20.5624403655201,13.4460395001892,122.929421098548)) ;
#16039=CARTESIAN_POINT('Ctrl Pts',(-20.5343398276492,13.4427157152044,122.862246353698)) ;
#16040=CARTESIAN_POINT('Ctrl Pts',(-20.5004283260913,13.4393740656987,122.797665446055)) ;
#16041=CARTESIAN_POINT('Ctrl Pts',(-20.4610899251354,13.4360345919639,122.736403714591)) ;
#16042=CARTESIAN_POINT('Ctrl Pts',(-20.4219178868664,13.4327092409135,122.675401059906)) ;
#16043=CARTESIAN_POINT('Ctrl Pts',(-20.3775131542739,13.4294154523931,122.617921893582)) ;
#16044=CARTESIAN_POINT('Ctrl Pts',(-20.3283780800447,13.4260721821416,122.56461636879)) ;
#16045=CARTESIAN_POINT('Ctrl Pts',(-20.2795625165461,13.4227506521792,122.511657473925)) ;
#16046=CARTESIAN_POINT('Ctrl Pts',(-20.2262611118225,13.4194383028478,122.463016614552)) ;
#16047=CARTESIAN_POINT('Ctrl Pts',(-20.1690665354927,13.4161742615484,122.419235592631)) ;
#16048=CARTESIAN_POINT('Ctrl Pts',(-20.1112909038241,13.4128770599609,122.375009787338)) ;
#16049=CARTESIAN_POINT('Ctrl Pts',(-20.0497683592175,13.4095514359962,122.335915254354)) ;
#16050=CARTESIAN_POINT('Ctrl Pts',(-19.9851900730519,13.4061756943286,122.30239170365)) ;
#16051=CARTESIAN_POINT('Ctrl Pts',(-19.976600882643,13.4057267061365,122.297932926911)) ;
#16052=CARTESIAN_POINT('Ctrl Pts',(-19.9679555666344,13.4052777640964,122.293571718947)) ;
#16053=CARTESIAN_POINT('Ctrl Pts',(-19.9592638229184,13.4048295958068,122.289313028327)) ;
#16054=CARTESIAN_POINT('Ctrl Pts',(-19.9029574856406,13.4019262986443,122.261724632002)) ;
#16055=CARTESIAN_POINT('Ctrl Pts',(-19.8446583224451,13.3990699102258,122.238413473407)) ;
#16056=CARTESIAN_POINT('Ctrl Pts',(-19.7848601012782,13.3962269818687,122.219575399118)) ;
#16057=CARTESIAN_POINT('Ctrl Pts',(-19.7154581960279,13.3929274749498,122.197711901821)) ;
#16058=CARTESIAN_POINT('Ctrl Pts',(-19.6442884736089,13.3895883209325,122.181952245224)) ;
#16059=CARTESIAN_POINT('Ctrl Pts',(-19.5721525566041,13.3862281725593,122.172471798418)) ;
#16060=CARTESIAN_POINT('Ctrl Pts',(-19.5004770657968,13.3828894712046,122.163051863021)) ;
#16061=CARTESIAN_POINT('Ctrl Pts',(-19.4281187326612,13.3796030075022,122.159867454332)) ;
#16062=CARTESIAN_POINT('Ctrl Pts',(-19.3558917953174,13.3762932146361,122.162954675232)) ;
#16063=CARTESIAN_POINT('Ctrl Pts',(-19.2835211381005,13.3729768358199,122.166048039201)) ;
#16064=CARTESIAN_POINT('Ctrl Pts',(-19.211556242851,13.3696357695286,122.175425660969)) ;
#16065=CARTESIAN_POINT('Ctrl Pts',(-19.1407994285092,13.3663379214254,122.190985815236)) ;
#16066=CARTESIAN_POINT('Ctrl Pts',(-19.0946685383492,13.3641878434431,122.201130474433)) ;
#16067=CARTESIAN_POINT('Ctrl Pts',(-19.0491400157151,13.3620507828497,122.213884078904)) ;
#16068=CARTESIAN_POINT('Ctrl Pts',(-19.00444037134,13.3598763993695,122.229185446966)) ;
#16069=CARTESIAN_POINT('Ctrl Pts',(-18.9803348232941,13.3587038015516,122.23743714266)) ;
#16070=CARTESIAN_POINT('Ctrl Pts',(-18.9564848539747,13.3575229288198,122.246425003157)) ;
#16071=CARTESIAN_POINT('Ctrl Pts',(-18.9329355549791,13.3563402041787,122.256131293038)) ;
#16072=CARTESIAN_POINT('Ctrl Pts',(-18.8663193831009,13.352994516989,122.283588410771)) ;
#16073=CARTESIAN_POINT('Ctrl Pts',(-18.8022113698638,13.3496957028308,122.316749155544)) ;
#16074=CARTESIAN_POINT('Ctrl Pts',(-18.7413137914152,13.3464387851846,122.355248459275)) ;
#16075=CARTESIAN_POINT('Ctrl Pts',(-18.6798135387548,13.3431496353819,122.394128772204)) ;
#16076=CARTESIAN_POINT('Ctrl Pts',(-18.6218297616564,13.3398102854306,122.438301305722)) ;
#16077=CARTESIAN_POINT('Ctrl Pts',(-18.5680171402105,13.3364401366298,122.487265901657)) ;
#16078=CARTESIAN_POINT('Ctrl Pts',(-18.5143880295376,13.333081480646,122.536063519463)) ;
#16079=CARTESIAN_POINT('Ctrl Pts',(-18.4651056924899,13.3297712570681,122.589435340438)) ;
#16080=CARTESIAN_POINT('Ctrl Pts',(-18.4207274175418,13.3264755396218,122.64677898041)) ;
#16081=CARTESIAN_POINT('Ctrl Pts',(-18.3763934622691,13.3231831135411,122.704065352463)) ;
#16082=CARTESIAN_POINT('Ctrl Pts',(-18.3371241763958,13.3198731611861,122.765094722657)) ;
#16083=CARTESIAN_POINT('Ctrl Pts',(-18.3033590273297,13.3165206640947,122.829185861367)) ;
#16084=CARTESIAN_POINT('Ctrl Pts',(-18.2976719942798,13.3159560060883,122.839980673004)) ;
#16085=CARTESIAN_POINT('Ctrl Pts',(-18.2921404801968,13.3153910434634,122.8508637759)) ;
#16086=CARTESIAN_POINT('Ctrl Pts',(-18.2867710305383,13.3148270119737,122.861822508517)) ;
#16087=CARTESIAN_POINT('Ctrl Pts',(-18.2604503598235,13.3120621686366,122.915541457575)) ;
#16088=CARTESIAN_POINT('Ctrl Pts',(-18.2380215987695,13.3093349778737,122.971077001873)) ;
#16089=CARTESIAN_POINT('Ctrl Pts',(-18.219656208807,13.3066205690874,123.027999687282)) ;
#16090=CARTESIAN_POINT('Ctrl Pts',(-18.1973137117869,13.3033183429792,123.097249233941)) ;
#16091=CARTESIAN_POINT('Ctrl Pts',(-18.1810630063032,13.2999805325553,123.168307925099)) ;
#16092=CARTESIAN_POINT('Ctrl Pts',(-18.1710845679303,13.2966220234551,123.240375459568)) ;
#16093=CARTESIAN_POINT('Ctrl Pts',(-18.1611126652386,13.2932657141124,123.312395791219)) ;
#16094=CARTESIAN_POINT('Ctrl Pts',(-18.1574432993759,13.2899427231762,123.385149783515)) ;
#16095=CARTESIAN_POINT('Ctrl Pts',(-18.1601187672495,13.28663039293,123.457810145731)) ;
#16096=CARTESIAN_POINT('Ctrl Pts',(-18.1627914406836,13.2833215223053,123.530394616556)) ;
#16097=CARTESIAN_POINT('Ctrl Pts',(-18.1717848155254,13.2800066790244,123.602606484272)) ;
#16098=CARTESIAN_POINT('Ctrl Pts',(-18.1870000723738,13.2766489629358,123.673636363758)) ;
#16099=CARTESIAN_POINT('Ctrl Pts',(-18.1973688869123,13.274360763943,123.72204143864)) ;
#16100=CARTESIAN_POINT('Ctrl Pts',(-18.2106063125809,13.2720799068548,123.769797668518)) ;
#16101=CARTESIAN_POINT('Ctrl Pts',(-18.2266435352718,13.2698214087154,123.816646870694)) ;
#16102=CARTESIAN_POINT('Ctrl Pts',(-18.2339450354743,13.2687931493378,123.837976590046)) ;
#16103=CARTESIAN_POINT('Ctrl Pts',(-18.24182366522,13.2677686676792,123.859108252036)) ;
#16104=CARTESIAN_POINT('Ctrl Pts',(-18.2502655468571,13.2667432995336,123.88000609514)) ;
#16105=CARTESIAN_POINT('Ctrl Pts',(-18.2775027042839,13.2634350188916,123.947431565781)) ;
#16106=CARTESIAN_POINT('Ctrl Pts',(-18.3105670637979,13.2600836373738,124.01234206466)) ;
#16107=CARTESIAN_POINT('Ctrl Pts',(-18.3490850319139,13.2567516262153,124.074010026824)) ;
#16108=CARTESIAN_POINT('Ctrl Pts',(-18.387628084856,13.2534174450847,124.135718150248)) ;
#16109=CARTESIAN_POINT('Ctrl Pts',(-18.4314846764746,13.2501174792409,124.193942781695)) ;
#16110=CARTESIAN_POINT('Ctrl Pts',(-18.4801556395518,13.2467541682034,124.248021488256)) ;
#16111=CARTESIAN_POINT('Ctrl Pts',(-18.5284185147809,13.2434190572728,124.301646765059)) ;
#16112=CARTESIAN_POINT('Ctrl Pts',(-18.5812330789978,13.2401060534054,124.350993050291)) ;
#16113=CARTESIAN_POINT('Ctrl Pts',(-18.6380109954579,13.2368404025748,124.395509491583)) ;
#16114=CARTESIAN_POINT('Ctrl Pts',(-18.6952690635548,13.2335471352395,124.440402393363)) ;
#16115=CARTESIAN_POINT('Ctrl Pts',(-18.7563330368345,13.2302170351911,124.480207906015)) ;
#16116=CARTESIAN_POINT('Ctrl Pts',(-18.8205189799835,13.226842865693,124.514479140492)) ;
#16117=CARTESIAN_POINT('Ctrl Pts',(-18.833320226369,13.2261699212292,124.521314196502)) ;
#16118=CARTESIAN_POINT('Ctrl Pts',(-18.8462459585297,13.2254975236865,124.527929095792)) ;
#16119=CARTESIAN_POINT('Ctrl Pts',(-18.8592802116798,13.2248269260802,124.534315490533)) ;
#16120=CARTESIAN_POINT('Ctrl Pts',(-18.9111830063035,13.2221565859056,124.559746309684)) ;
#16121=CARTESIAN_POINT('Ctrl Pts',(-18.9647837095672,13.2195252081346,124.5815448943)) ;
#16122=CARTESIAN_POINT('Ctrl Pts',(-19.019694317989,13.2169040953244,124.599555519304)) ;
#16123=CARTESIAN_POINT('Ctrl Pts',(-19.0885599989045,13.213616848586,124.622143394219)) ;
#16124=CARTESIAN_POINT('Ctrl Pts',(-19.1592492674356,13.2103016820336,124.638696482181)) ;
#16125=CARTESIAN_POINT('Ctrl Pts',(-19.2309735301825,13.2069465475215,124.649032848319)) ;
#16126=CARTESIAN_POINT('Ctrl Pts',(-19.3023454913827,13.2036078930544,124.659318443384)) ;
#16127=CARTESIAN_POINT('Ctrl Pts',(-19.3744738881038,13.200313127969,124.663409024748)) ;
#16128=CARTESIAN_POINT('Ctrl Pts',(-19.4465536192155,13.1970382089384,124.661258282287)) ;
#16129=CARTESIAN_POINT('Ctrl Pts',(-19.5192796330319,13.1937339262643,124.659088255798)) ;
#16130=CARTESIAN_POINT('Ctrl Pts',(-19.5916746647344,13.1903937844111,124.6505734399)) ;
#16131=CARTESIAN_POINT('Ctrl Pts',(-19.6629253872211,13.18704088229,124.635807862841)) ;
#16132=CARTESIAN_POINT('Ctrl Pts',(-19.7141264295642,13.1846314739713,124.625197262557)) ;
#16133=CARTESIAN_POINT('Ctrl Pts',(-19.7646209257032,13.1822377967368,124.611382178439)) ;
#16134=CARTESIAN_POINT('Ctrl Pts',(-19.8141051483714,13.1798450308754,124.594442927482)) ;
#16135=CARTESIAN_POINT('Ctrl Pts',(-19.8334298206514,13.1789106034232,124.587827779143)) ;
#16136=CARTESIAN_POINT('Ctrl Pts',(-19.8525932488088,13.1779769401818,124.580738434888)) ;
#16137=CARTESIAN_POINT('Ctrl Pts',(-19.8715659077101,13.1770448707288,124.573186211035)) ;
#16138=CARTESIAN_POINT('Ctrl Pts',(-19.9388875606489,13.1737375611655,124.546388270071)) ;
#16139=CARTESIAN_POINT('Ctrl Pts',(-20.0037424838628,13.1704339176419,124.513791655081)) ;
#16140=CARTESIAN_POINT('Ctrl Pts',(-20.0654078568684,13.1670897087974,124.475762695686)) ;
#16141=CARTESIAN_POINT('Ctrl Pts',(-20.1267524640324,13.1637628955821,124.437931552191)) ;
#16142=CARTESIAN_POINT('Ctrl Pts',(-20.1847105512711,13.160459384278,124.394865788352)) ;
#16143=CARTESIAN_POINT('Ctrl Pts',(-20.2386353078162,13.1571865872795,124.347045297996)) ;
#16144=CARTESIAN_POINT('Ctrl Pts',(-20.2930722512412,13.1538827046759,124.298770600159)) ;
#16145=CARTESIAN_POINT('Ctrl Pts',(-20.3431881478507,13.150544876991,124.24583746345)) ;
#16146=CARTESIAN_POINT('Ctrl Pts',(-20.3884152391871,13.1471896049157,124.188846527606)) ;
#16147=CARTESIAN_POINT('Ctrl Pts',(-20.4334882142278,13.1438457662996,124.132049794654)) ;
#16148=CARTESIAN_POINT('Ctrl Pts',(-20.4735347227404,13.1405458478673,124.071438635973)) ;
#16149=CARTESIAN_POINT('Ctrl Pts',(-20.5081039974958,13.1372261673073,124.007690830188)) ;
#16150=CARTESIAN_POINT('Ctrl Pts',(-20.5163069447483,13.1364384399187,123.992564105893)) ;
#16151=CARTESIAN_POINT('Ctrl Pts',(-20.5242003769134,13.1356495875477,123.977262397619)) ;
#16152=CARTESIAN_POINT('Ctrl Pts',(-20.5317733220291,13.1348603689426,123.961806468175)) ;
#16153=CARTESIAN_POINT('Ctrl Pts',(-20.5560402481142,13.1323313780068,123.912279118952)) ;
#16154=CARTESIAN_POINT('Ctrl Pts',(-20.5770007045201,13.1297993711523,123.861203677247)) ;
#16155=CARTESIAN_POINT('Ctrl Pts',(-20.5945181062435,13.127280121411,123.808919172674)) ;
#16156=CARTESIAN_POINT('Ctrl Pts',(-20.6175795522041,13.1239635598178,123.740087259368)) ;
#16157=CARTESIAN_POINT('Ctrl Pts',(-20.6345986982784,13.120654726801,123.669386379736)) ;
#16158=CARTESIAN_POINT('Ctrl Pts',(-20.6453871540013,13.117306267284,123.597609709495)) ;
#16159=CARTESIAN_POINT('Ctrl Pts',(-20.6561353420231,13.113970305827,123.52610094428)) ;
#16160=CARTESIAN_POINT('Ctrl Pts',(-20.660658278922,13.1106580562661,123.453794034973)) ;
#16161=CARTESIAN_POINT('Ctrl Pts',(-20.6589046280877,13.1073697954084,123.38150125712)) ;
#16162=CARTESIAN_POINT('Ctrl Pts',(-20.6571413476508,13.104063478137,123.308811507018)) ;
#16163=CARTESIAN_POINT('Ctrl Pts',(-20.6490396908371,13.1007322821932,123.23641645862)) ;
#16164=CARTESIAN_POINT('Ctrl Pts',(-20.6346891360308,13.0973782862631,123.165129504685)) ;
#16165=CARTESIAN_POINT('Ctrl Pts',(-20.6239016001173,13.0948570352009,123.111541989351)) ;
#16166=CARTESIAN_POINT('Ctrl Pts',(-20.6096085084526,13.0923516502569,123.058710819136)) ;
#16167=CARTESIAN_POINT('Ctrl Pts',(-20.5919014130363,13.0898536069789,123.006983254139)) ;
#16168=CARTESIAN_POINT('Ctrl Pts',(-20.5919013672997,13.0298207905601,123.006983120529)) ;
#16169=CARTESIAN_POINT('Ctrl Pts',(-20.6128415365065,13.0327758983278,123.068155409876)) ;
#16170=CARTESIAN_POINT('Ctrl Pts',(-20.6289991091982,13.0357170266271,123.130860810711)) ;
#16171=CARTESIAN_POINT('Ctrl Pts',(-20.6402267339071,13.0386471338238,123.194441359862)) ;
#16172=CARTESIAN_POINT('Ctrl Pts',(-20.6564173041211,13.0428724359275,123.286126410971)) ;
#16173=CARTESIAN_POINT('Ctrl Pts',(-20.6622820922898,13.04712862656,123.379134979086)) ;
#16174=CARTESIAN_POINT('Ctrl Pts',(-20.657833380239,13.0513934496921,123.47177326128)) ;
#16175=CARTESIAN_POINT('Ctrl Pts',(-20.6553317958422,13.0537916303073,123.523865300199)) ;
#16176=CARTESIAN_POINT('Ctrl Pts',(-20.6495684445029,13.056192540518,123.575841899756)) ;
#16177=CARTESIAN_POINT('Ctrl Pts',(-20.6405410520404,13.0585922231034,123.627399854497)) ;
#16178=CARTESIAN_POINT('Ctrl Pts',(-20.6202302906749,13.0639912772098,123.743400274284)) ;
#16179=CARTESIAN_POINT('Ctrl Pts',(-20.5836175232734,13.069281839856,123.856001963048)) ;
#16180=CARTESIAN_POINT('Ctrl Pts',(-20.5317601409036,13.0747309735579,123.96183336925)) ;
#16181=CARTESIAN_POINT('Ctrl Pts',(-20.5197068854819,13.0759975203316,123.986431852867)) ;
#16182=CARTESIAN_POINT('Ctrl Pts',(-20.5068314945853,13.077267794894,124.010657329884)) ;
#16183=CARTESIAN_POINT('Ctrl Pts',(-20.4931985752011,13.0785324723927,124.034392627637)) ;
#16184=CARTESIAN_POINT('Ctrl Pts',(-20.4451665262531,13.0829882349343,124.118017781675)) ;
#16185=CARTESIAN_POINT('Ctrl Pts',(-20.3877135875372,13.0874031785866,124.195641337355)) ;
#16186=CARTESIAN_POINT('Ctrl Pts',(-20.3220694358251,13.0917957573214,124.265805743559)) ;
#16187=CARTESIAN_POINT('Ctrl Pts',(-20.2890474332361,13.0940054247871,124.301101640344)) ;
#16188=CARTESIAN_POINT('Ctrl Pts',(-20.2539515931778,13.0962094327011,124.334510747036)) ;
#16189=CARTESIAN_POINT('Ctrl Pts',(-20.216938518417,13.0984101302198,124.365845380865)) ;
#16190=CARTESIAN_POINT('Ctrl Pts',(-20.105950262194,13.1050091923529,124.459806133667)) ;
#16191=CARTESIAN_POINT('Ctrl Pts',(-19.9794225674485,13.1116356102903,124.533679037231)) ;
#16192=CARTESIAN_POINT('Ctrl Pts',(-19.8430228892276,13.1183574025859,124.584145536012)) ;
#16193=CARTESIAN_POINT('Ctrl Pts',(-19.833439869117,13.1188296549518,124.587691156347)) ;
#16194=CARTESIAN_POINT('Ctrl Pts',(-19.8237911871676,13.1193020977122,124.591127097987)) ;
#16195=CARTESIAN_POINT('Ctrl Pts',(-19.8141206275482,13.1197729541245,124.594437628596)) ;
#16196=CARTESIAN_POINT('Ctrl Pts',(-19.6865529013262,13.1259841853512,124.638107992979)) ;
#16197=CARTESIAN_POINT('Ctrl Pts',(-19.5527786571738,13.1321239816196,124.66084402754)) ;
#16198=CARTESIAN_POINT('Ctrl Pts',(-19.4179888083276,13.1382623043066,124.661783974771)) ;
#16199=CARTESIAN_POINT('Ctrl Pts',(-19.3220565319828,13.1426310551683,124.66245295154)) ;
#16200=CARTESIAN_POINT('Ctrl Pts',(-19.2265435863915,13.1469968366946,124.652077540438)) ;
#16201=CARTESIAN_POINT('Ctrl Pts',(-19.1332868126833,13.1513888479219,124.630966549935)) ;
#16202=CARTESIAN_POINT('Ctrl Pts',(-19.0852591382136,13.1536507542383,124.620094291125)) ;
#16203=CARTESIAN_POINT('Ctrl Pts',(-19.0378287111207,13.1559196174534,124.606373923211)) ;
#16204=CARTESIAN_POINT('Ctrl Pts',(-18.9912494073237,13.1581994259979,124.589845314723)) ;
#16205=CARTESIAN_POINT('Ctrl Pts',(-18.94628666701,13.16040011238,124.573890341793)) ;
#16206=CARTESIAN_POINT('Ctrl Pts',(-18.9022002374828,13.1625869461434,124.555343671711)) ;
#16207=CARTESIAN_POINT('Ctrl Pts',(-18.8593086838134,13.1647748278629,124.53432944058)) ;
#16208=CARTESIAN_POINT('Ctrl Pts',(-18.772080200369,13.1692243193834,124.49159283266)) ;
#16209=CARTESIAN_POINT('Ctrl Pts',(-18.690158054208,13.1736772079637,124.438843783208)) ;
#16210=CARTESIAN_POINT('Ctrl Pts',(-18.6152211808927,13.1781001339968,124.377206992408)) ;
#16211=CARTESIAN_POINT('Ctrl Pts',(-18.5450664514027,13.1822408082161,124.31950359228)) ;
#16212=CARTESIAN_POINT('Ctrl Pts',(-18.4815599704335,13.1863804049238,124.254452152417)) ;
#16213=CARTESIAN_POINT('Ctrl Pts',(-18.4257140315598,13.1905344974001,124.183250208774)) ;
#16214=CARTESIAN_POINT('Ctrl Pts',(-18.3920578426148,13.1930380083822,124.140339549256)) ;
#16215=CARTESIAN_POINT('Ctrl Pts',(-18.3611833015205,13.1955467842376,124.095193139965)) ;
#16216=CARTESIAN_POINT('Ctrl Pts',(-18.3333180481067,13.1980642337553,124.04807106455)) ;
#16217=CARTESIAN_POINT('Ctrl Pts',(-18.2923218608707,13.201767980147,123.978743669676)) ;
#16218=CARTESIAN_POINT('Ctrl Pts',(-18.2580892369449,13.2054233460874,123.905552327292)) ;
#16219=CARTESIAN_POINT('Ctrl Pts',(-18.2311459975247,13.2091185082985,123.829568560322)) ;
#16220=CARTESIAN_POINT('Ctrl Pts',(-18.2296197656979,13.2093278251547,123.825264369513)) ;
#16221=CARTESIAN_POINT('Ctrl Pts',(-18.2281169132799,13.2095372697089,123.820951227691)) ;
#16222=CARTESIAN_POINT('Ctrl Pts',(-18.2266375321997,13.2097468579884,123.816629333622)) ;
#16223=CARTESIAN_POINT('Ctrl Pts',(-18.2072420008511,13.2124946801017,123.759966832634)) ;
#16224=CARTESIAN_POINT('Ctrl Pts',(-18.1919435736847,13.2152547785462,123.701967615488)) ;
#16225=CARTESIAN_POINT('Ctrl Pts',(-18.1808718008391,13.217994004838,123.643185002314)) ;
#16226=CARTESIAN_POINT('Ctrl Pts',(-18.1641841076027,13.2221226451832,123.554586163632)) ;
#16227=CARTESIAN_POINT('Ctrl Pts',(-18.1571640677684,13.2262321383058,123.464633492152)) ;
#16228=CARTESIAN_POINT('Ctrl Pts',(-18.1598183418223,13.230348860005,123.3748689133)) ;
#16229=CARTESIAN_POINT('Ctrl Pts',(-18.1614392540987,13.232862859918,123.320051473618)) ;
#16230=CARTESIAN_POINT('Ctrl Pts',(-18.1666685394986,13.2353795555852,123.265302296028)) ;
#16231=CARTESIAN_POINT('Ctrl Pts',(-18.1755124084081,13.2379049538576,123.210974410351)) ;
#16232=CARTESIAN_POINT('Ctrl Pts',(-18.1952399603618,13.2435382265954,123.089788061005)) ;
#16233=CARTESIAN_POINT('Ctrl Pts',(-18.2327234730855,13.2491089318735,122.972124085933)) ;
#16234=CARTESIAN_POINT('Ctrl Pts',(-18.2867834910586,13.2547574492201,122.861797078053)) ;
#16235=CARTESIAN_POINT('Ctrl Pts',(-18.2965161638263,13.2557743776825,122.841934401247)) ;
#16236=CARTESIAN_POINT('Ctrl Pts',(-18.3067898552594,13.2567917787257,122.822305058631)) ;
#16237=CARTESIAN_POINT('Ctrl Pts',(-18.3175560614831,13.2578037787098,122.802999292444)) ;
#16238=CARTESIAN_POINT('Ctrl Pts',(-18.3596833735975,13.2617636544824,122.72745735865)) ;
#16239=CARTESIAN_POINT('Ctrl Pts',(-18.4094498495815,13.2657077366537,122.656644641517)) ;
#16240=CARTESIAN_POINT('Ctrl Pts',(-18.4659943370288,13.2696619762082,122.591615119139)) ;
#16241=CARTESIAN_POINT('Ctrl Pts',(-18.5044087373086,13.272348351979,122.547436274916)) ;
#16242=CARTESIAN_POINT('Ctrl Pts',(-18.5459532309635,13.2750394157692,122.505925244562)) ;
#16243=CARTESIAN_POINT('Ctrl Pts',(-18.590360693387,13.2777433045955,122.467418323832)) ;
#16244=CARTESIAN_POINT('Ctrl Pts',(-18.6419648825726,13.2808853888964,122.422670925223)) ;
#16245=CARTESIAN_POINT('Ctrl Pts',(-18.6972101956397,13.2839971960161,122.382181921752)) ;
#16246=CARTESIAN_POINT('Ctrl Pts',(-18.7554884296589,13.287119167613,122.346419259243)) ;
#16247=CARTESIAN_POINT('Ctrl Pts',(-18.7589739169019,13.2873058855594,122.344280376588)) ;
#16248=CARTESIAN_POINT('Ctrl Pts',(-18.7624702419052,13.2874926398637,122.34215838877)) ;
#16249=CARTESIAN_POINT('Ctrl Pts',(-18.7659772702078,13.2876794391776,122.340053391756)) ;
#16250=CARTESIAN_POINT('Ctrl Pts',(-18.8283598045692,13.291002199536,122.302609996028)) ;
#16251=CARTESIAN_POINT('Ctrl Pts',(-18.8938915827265,13.2943408185553,122.270684529986)) ;
#16252=CARTESIAN_POINT('Ctrl Pts',(-18.9618337722691,13.2976766648834,122.244638792243)) ;
#16253=CARTESIAN_POINT('Ctrl Pts',(-18.9759375383491,13.2983691358886,122.239232092886)) ;
#16254=CARTESIAN_POINT('Ctrl Pts',(-18.9901453618968,13.2990607962286,122.234078864962)) ;
#16255=CARTESIAN_POINT('Ctrl Pts',(-19.0044389742765,13.2997521504947,122.229185925203)) ;
#16256=CARTESIAN_POINT('Ctrl Pts',(-19.058959152331,13.3023891856044,122.210522767159)) ;
#16257=CARTESIAN_POINT('Ctrl Pts',(-19.1147001378851,13.3050268795537,122.195653767887)) ;
#16258=CARTESIAN_POINT('Ctrl Pts',(-19.1712596402296,13.3076728273998,122.184683564916)) ;
#16259=CARTESIAN_POINT('Ctrl Pts',(-19.2423788180773,13.3109999011477,122.170889387391)) ;
#16260=CARTESIAN_POINT('Ctrl Pts',(-19.3145571156168,13.3143231624351,122.163310005777)) ;
#16261=CARTESIAN_POINT('Ctrl Pts',(-19.3868925501702,13.317633218063,122.162014722725)) ;
#16262=CARTESIAN_POINT('Ctrl Pts',(-19.4772904561789,13.3217698089244,122.160396001883)) ;
#16263=CARTESIAN_POINT('Ctrl Pts',(-19.5674021360052,13.3258924613772,122.168589834439)) ;
#16264=CARTESIAN_POINT('Ctrl Pts',(-19.6557028168064,13.3300196499126,122.186346305415)) ;
#16265=CARTESIAN_POINT('Ctrl Pts',(-19.7088544483455,13.3325039660281,122.197034619414)) ;
#16266=CARTESIAN_POINT('Ctrl Pts',(-19.7613515886273,13.3349899257055,122.211188766597)) ;
#16267=CARTESIAN_POINT('Ctrl Pts',(-19.8128584910012,13.3374815582495,122.228759788444)) ;
#16268=CARTESIAN_POINT('Ctrl Pts',(-19.8628380221861,13.3398993046232,122.245809764153)) ;
#16269=CARTESIAN_POINT('Ctrl Pts',(-19.9117638198388,13.3423053796767,122.266040733864)) ;
#16270=CARTESIAN_POINT('Ctrl Pts',(-19.9592397024072,13.344723836538,122.28930121033)) ;
#16271=CARTESIAN_POINT('Ctrl Pts',(-20.0419784854064,13.3489386118432,122.329838498122)) ;
#16272=CARTESIAN_POINT('Ctrl Pts',(-20.1199625744019,13.3531881524558,122.379386706394)) ;
#16273=CARTESIAN_POINT('Ctrl Pts',(-20.1918044690641,13.3574053919986,122.437061421343)) ;
#16274=CARTESIAN_POINT('Ctrl Pts',(-20.2484665510601,13.3607315511136,122.482549773827)) ;
#16275=CARTESIAN_POINT('Ctrl Pts',(-20.3010658368689,13.3640386988681,122.532902439704)) ;
#16276=CARTESIAN_POINT('Ctrl Pts',(-20.3489907498894,13.3673857229415,122.587539464216)) ;
#16277=CARTESIAN_POINT('Ctrl Pts',(-20.3966435956241,13.37071374613,122.641866317127)) ;
#16278=CARTESIAN_POINT('Ctrl Pts',(-20.439495919874,13.374022327351,122.700223486028)) ;
#16279=CARTESIAN_POINT('Ctrl Pts',(-20.4770662197135,13.3773157278759,122.761955914037)) ;
#16280=CARTESIAN_POINT('Ctrl Pts',(-20.5147773812097,13.3806214762888,122.82391979434)) ;
#16281=CARTESIAN_POINT('Ctrl Pts',(-20.5470231453038,13.3839416549025,122.889047248779)) ;
#16282=CARTESIAN_POINT('Ctrl Pts',(-20.5734409337567,13.3872834493149,122.956609749793)) ;
#16283=CARTESIAN_POINT('Ctrl Pts',(-20.5799521068342,13.3881070989495,122.973261830205)) ;
#16284=CARTESIAN_POINT('Ctrl Pts',(-20.5861082466563,13.3889304241705,122.990059702568)) ;
#16285=CARTESIAN_POINT('Ctrl Pts',(-20.5919016415172,13.3897528569022,123.006983921598)) ;
#16286=CARTESIAN_POINT('Origin',(-19.4092722359532,16.5113612779716,123.411814366564)) ;
#16287=CARTESIAN_POINT('',(-20.5919010929731,12.6697683433189,123.006982319198)) ;
#16288=CARTESIAN_POINT('',(-20.5919043739536,12.7298332115048,123.006991903941)) ;
#16289=CARTESIAN_POINT('',(-20.5919021064381,16.5113612779716,123.006985279772)) ;
#16290=CARTESIAN_POINT('Ctrl Pts',(-20.5919014130362,13.0898536069868,123.006983254138)) ;
#16291=CARTESIAN_POINT('Ctrl Pts',(-20.5791790206653,13.0880587850324,122.969817453491)) ;
#16292=CARTESIAN_POINT('Ctrl Pts',(-20.5647155841445,13.0862721300352,122.933281380902)) ;
#16293=CARTESIAN_POINT('Ctrl Pts',(-20.5452931183874,13.0841163519632,122.890259692648)) ;
#16294=CARTESIAN_POINT('Ctrl Pts',(-20.5419658468915,13.0837543841713,122.883072551962)) ;
#16295=CARTESIAN_POINT('Ctrl Pts',(-20.5357135669482,13.0830872032147,122.86989708902)) ;
#16296=CARTESIAN_POINT('Ctrl Pts',(-20.5328085362647,13.0827821035447,122.863899601794)) ;
#16297=CARTESIAN_POINT('Ctrl Pts',(-20.5266929064853,13.0821496688658,122.851526947794)) ;
#16298=CARTESIAN_POINT('Ctrl Pts',(-20.5234753799025,13.0818223066021,122.845155474289)) ;
#16299=CARTESIAN_POINT('Ctrl Pts',(-20.5150841630547,13.080981988997,122.828886669669)) ;
#16300=CARTESIAN_POINT('Ctrl Pts',(-20.5098320947547,13.0804686351631,122.819030498871)) ;
#16301=CARTESIAN_POINT('Ctrl Pts',(-20.4908842883934,13.078659771017,122.784592592427)) ;
#16302=CARTESIAN_POINT('Ctrl Pts',(-20.4764913302073,13.0773615396779,122.760404213382)) ;
#16303=CARTESIAN_POINT('Ctrl Pts',(-20.4527297071399,13.0753350760544,122.723375557597)) ;
#16304=CARTESIAN_POINT('Ctrl Pts',(-20.4439117842298,13.074605487379,122.710193032768)) ;
#16305=CARTESIAN_POINT('Ctrl Pts',(-20.4304362998422,13.0735228553301,122.690854289597)) ;
#16306=CARTESIAN_POINT('Ctrl Pts',(-20.4259687220333,13.0731689209277,122.684567686564)) ;
#16307=CARTESIAN_POINT('Ctrl Pts',(-20.4166292464149,13.0724390993785,122.671679812802)) ;
#16308=CARTESIAN_POINT('Ctrl Pts',(-20.4117499578622,13.0720632693731,122.665084347226)) ;
#16309=CARTESIAN_POINT('Ctrl Pts',(-20.4004511138357,13.0712050694164,122.650121750988)) ;
#16310=CARTESIAN_POINT('Ctrl Pts',(-20.393989886461,13.0707229458926,122.641786861669)) ;
#16311=CARTESIAN_POINT('Ctrl Pts',(-20.3705899742046,13.0690061987055,122.612377555842)) ;
#16312=CARTESIAN_POINT('Ctrl Pts',(-20.3530739992861,13.0677746166432,122.591772147451)) ;
#16313=CARTESIAN_POINT('Ctrl Pts',(-20.3280211934725,13.0660737435465,122.564167488205)) ;
#16314=CARTESIAN_POINT('Ctrl Pts',(-20.3210458281659,13.0656062078695,122.556668885868)) ;
#16315=CARTESIAN_POINT('Ctrl Pts',(-20.3083267464374,13.0647637665576,122.543328278811)) ;
#16316=CARTESIAN_POINT('Ctrl Pts',(-20.3026162469189,13.0643890731206,122.537455415673)) ;
#16317=CARTESIAN_POINT('Ctrl Pts',(-20.2956550140089,13.0639364010447,122.530435649181)) ;
#16318=CARTESIAN_POINT('Ctrl Pts',(-20.2944591356239,13.0638587797494,122.52923461077)) ;
#16319=CARTESIAN_POINT('Ctrl Pts',(-20.2925818801849,13.0637371557354,122.527356908787)) ;
#16320=CARTESIAN_POINT('Ctrl Pts',(-20.2919021595124,13.0636931635908,122.526678591529)) ;
#16321=CARTESIAN_POINT('Ctrl Pts',(-20.2855535475068,13.0632827007654,122.520357671943)) ;
#16322=CARTESIAN_POINT('Ctrl Pts',(-20.2798314133098,13.0629158959593,122.5147688306)) ;
#16323=CARTESIAN_POINT('Ctrl Pts',(-20.2620038089164,13.0617826277711,122.49768775231)) ;
#16324=CARTESIAN_POINT('Ctrl Pts',(-20.2497215250182,13.0610151242612,122.486382796024)) ;
#16325=CARTESIAN_POINT('Ctrl Pts',(-20.2275007691805,13.0596504182977,122.466737519096)) ;
#16326=CARTESIAN_POINT('Ctrl Pts',(-20.2176518666741,13.059053514139,122.45829952495)) ;
#16327=CARTESIAN_POINT('Ctrl Pts',(-20.2032180846653,13.0581909897426,122.446317852719)) ;
#16328=CARTESIAN_POINT('Ctrl Pts',(-20.1987370681398,13.0579248875879,122.442650392889)) ;
#16329=CARTESIAN_POINT('Ctrl Pts',(-20.1935525025875,13.0576190062421,122.438466934799)) ;
#16330=CARTESIAN_POINT('Ctrl Pts',(-20.1928737080088,13.0575789976055,122.437920382319)) ;
#16331=CARTESIAN_POINT('Ctrl Pts',(-20.1915087192564,13.0574986234605,122.4368236703)) ;
#16332=CARTESIAN_POINT('Ctrl Pts',(-20.1908225152045,13.057458258173,122.436273524459)) ;
#16333=CARTESIAN_POINT('Ctrl Pts',(-20.1875199419223,13.0572641797235,122.433631495324)) ;
#16334=CARTESIAN_POINT('Ctrl Pts',(-20.1848957489494,13.057110545949,122.431549408724)) ;
#16335=CARTESIAN_POINT('Ctrl Pts',(-20.1817827671608,13.0569289610988,122.429099833748)) ;
#16336=CARTESIAN_POINT('Ctrl Pts',(-20.1813020415568,13.0569009383371,122.428722126184)) ;
#16337=CARTESIAN_POINT('Ctrl Pts',(-20.1749755695237,13.0565323959611,122.423758900124)) ;
#16338=CARTESIAN_POINT('Ctrl Pts',(-20.1690893191057,13.0561922396103,122.419225226801)) ;
#16339=CARTESIAN_POINT('Ctrl Pts',(-20.1464151149356,13.0548917623543,122.402081122969)) ;
#16340=CARTESIAN_POINT('Ctrl Pts',(-20.1293507949056,13.0539333670138,122.38984190088)) ;
#16341=CARTESIAN_POINT('Ctrl Pts',(-20.0935184368185,13.0519557092244,122.365484690616)) ;
#16342=CARTESIAN_POINT('Ctrl Pts',(-20.0747175367803,13.0509367931673,122.353428234847)) ;
#16343=CARTESIAN_POINT('Ctrl Pts',(-20.0446747203537,13.0493330165717,122.335279780015)) ;
#16344=CARTESIAN_POINT('Ctrl Pts',(-20.0336451243973,13.0487492306961,122.328845517366)) ;
#16345=CARTESIAN_POINT('Ctrl Pts',(-20.0148661944338,13.0477629679816,122.318272833221)) ;
#16346=CARTESIAN_POINT('Ctrl Pts',(-20.0071682925871,13.0473608151302,122.314045068055)) ;
#16347=CARTESIAN_POINT('Ctrl Pts',(-19.9885573709466,13.0463934044849,122.304077594401)) ;
#16348=CARTESIAN_POINT('Ctrl Pts',(-19.9776027396486,13.0458279314908,122.298417554343)) ;
#16349=CARTESIAN_POINT('Ctrl Pts',(-19.9450826159544,13.0441602047694,122.28222006754)) ;
#16350=CARTESIAN_POINT('Ctrl Pts',(-19.9232953680866,13.0430567814907,122.272140616113)) ;
#16351=CARTESIAN_POINT('Ctrl Pts',(-19.8827606791136,13.041028033727,122.254786968767)) ;
#16352=CARTESIAN_POINT('Ctrl Pts',(-19.8641018238544,13.0401032834668,122.247325744044)) ;
#16353=CARTESIAN_POINT('Ctrl Pts',(-19.8370544133023,13.0387763300771,122.237259439374)) ;
#16354=CARTESIAN_POINT('Ctrl Pts',(-19.8288056227823,13.0383734293611,122.234287888713)) ;
#16355=CARTESIAN_POINT('Ctrl Pts',(-19.819577315835,13.0379247506337,122.231072755854)) ;
#16356=CARTESIAN_POINT('Ctrl Pts',(-19.8186279901786,13.0378786188541,122.2307432949)) ;
#16357=CARTESIAN_POINT('Ctrl Pts',(-19.8168267041893,13.037791132955,122.23012059603)) ;
#16358=CARTESIAN_POINT('Ctrl Pts',(-19.8159748220509,13.0377497778537,122.229827133824)) ;
#16359=CARTESIAN_POINT('Ctrl Pts',(-19.8140710536562,13.0376574023267,122.229173612418)) ;
#16360=CARTESIAN_POINT('Ctrl Pts',(-19.8130190027272,13.0376063842296,122.228814034991)) ;
#16361=CARTESIAN_POINT('Ctrl Pts',(-19.8055448821177,13.0372441481705,122.226270608562)) ;
#16362=CARTESIAN_POINT('Ctrl Pts',(-19.7991056000856,13.0369331808838,122.224137659408)) ;
#16363=CARTESIAN_POINT('Ctrl Pts',(-19.7900598760826,13.0364977577974,122.22122284369)) ;
#16364=CARTESIAN_POINT('Ctrl Pts',(-19.7874677668294,13.0363731466514,122.220396915938)) ;
#16365=CARTESIAN_POINT('Ctrl Pts',(-19.7617315938096,13.0351374677625,122.212289012309)) ;
#16366=CARTESIAN_POINT('Ctrl Pts',(-19.7383827968355,13.0340287048108,122.205673861513)) ;
#16367=CARTESIAN_POINT('Ctrl Pts',(-19.6942375807687,13.0319476481019,122.194544098501)) ;
#16368=CARTESIAN_POINT('Ctrl Pts',(-19.673489620474,13.0309757755871,122.189872745543)) ;
#16369=CARTESIAN_POINT('Ctrl Pts',(-19.6364815259975,13.0292493797788,122.182527144479)) ;
#16370=CARTESIAN_POINT('Ctrl Pts',(-19.6202686646467,13.0284954717176,122.179640823168)) ;
#16371=CARTESIAN_POINT('Ctrl Pts',(-19.6022976823653,13.027661616081,122.176806609706)) ;
#16372=CARTESIAN_POINT('Ctrl Pts',(-19.6005912530173,13.0275824556779,122.176541110896)) ;
#16373=CARTESIAN_POINT('Ctrl Pts',(-19.5976149459336,13.0274444165535,122.176084350409)) ;
#16374=CARTESIAN_POINT('Ctrl Pts',(-19.596345313313,13.0273855414425,122.175891507743)) ;
#16375=CARTESIAN_POINT('Ctrl Pts',(-19.593487886595,13.0272530584297,122.175462001246)) ;
#16376=CARTESIAN_POINT('Ctrl Pts',(-19.591899929316,13.0271794481916,122.175226438924)) ;
#16377=CARTESIAN_POINT('Ctrl Pts',(-19.5714744332639,13.0262327976296,122.172236661951)) ;
#16378=CARTESIAN_POINT('Ctrl Pts',(-19.5525768533619,13.025358891184,122.169910094061)) ;
#16379=CARTESIAN_POINT('Ctrl Pts',(-19.4970543984554,13.0227947785655,122.164358674257)) ;
#16380=CARTESIAN_POINT('Ctrl Pts',(-19.4603317164738,13.0211029801371,122.162316733384)) ;
#16381=CARTESIAN_POINT('Ctrl Pts',(-19.4119781567302,13.0188790327024,122.161763516417)) ;
#16382=CARTESIAN_POINT('Ctrl Pts',(-19.4003823613712,13.0183460185202,122.161792198416)) ;
#16383=CARTESIAN_POINT('Ctrl Pts',(-19.3882597526607,13.0177891852922,122.161990876862)) ;
#16384=CARTESIAN_POINT('Ctrl Pts',(-19.3877308783924,13.0177648930705,122.161999880419)) ;
#16385=CARTESIAN_POINT('Ctrl Pts',(-19.3865241254111,13.0177094664024,122.162021190389)) ;
#16386=CARTESIAN_POINT('Ctrl Pts',(-19.3858462506889,13.0176783326659,122.162033712625)) ;
#16387=CARTESIAN_POINT('Ctrl Pts',(-19.3841699374231,13.0176013452949,122.162066043118)) ;
#16388=CARTESIAN_POINT('Ctrl Pts',(-19.383171511717,13.0175554937149,122.162086496369)) ;
#16389=CARTESIAN_POINT('Ctrl Pts',(-19.3805211783401,13.017433786664,122.162143967248)) ;
#16390=CARTESIAN_POINT('Ctrl Pts',(-19.3788693174578,13.0173579376186,122.162183063823)) ;
#16391=CARTESIAN_POINT('Ctrl Pts',(-19.3759793380935,13.0172252472493,122.162257198133)) ;
#16392=CARTESIAN_POINT('Ctrl Pts',(-19.3747411853149,13.0171684019035,122.162290801053)) ;
#16393=CARTESIAN_POINT('Ctrl Pts',(-19.3719442822547,13.0170399981373,122.16237086812)) ;
#16394=CARTESIAN_POINT('Ctrl Pts',(-19.3703855647219,13.0169684427767,122.162418409018)) ;
#16395=CARTESIAN_POINT('Ctrl Pts',(-19.3615548536221,13.0165630737479,122.162704287283)) ;
#16396=CARTESIAN_POINT('Ctrl Pts',(-19.3542849546739,13.0162294236945,122.16300319676)) ;
#16397=CARTESIAN_POINT('Ctrl Pts',(-19.3120330825369,13.014290162207,122.165110095221)) ;
#16398=CARTESIAN_POINT('Ctrl Pts',(-19.2771367987849,13.0126877295686,122.168324427429)) ;
#16399=CARTESIAN_POINT('Ctrl Pts',(-19.1956810388155,13.0089264329111,122.179295353745)) ;
#16400=CARTESIAN_POINT('Ctrl Pts',(-19.1493341988922,13.0067723538331,122.188230890597)) ;
#16401=CARTESIAN_POINT('Ctrl Pts',(-19.0901293426453,13.0039758566922,122.203161846975)) ;
#16402=CARTESIAN_POINT('Ctrl Pts',(-19.0767128216625,13.0033389811045,122.20678435273)) ;
#16403=CARTESIAN_POINT('Ctrl Pts',(-19.0626349751978,13.0026670308939,122.210838439235)) ;
#16404=CARTESIAN_POINT('Ctrl Pts',(-19.0619106250721,13.0026324466501,122.211047744837)) ;
#16405=CARTESIAN_POINT('Ctrl Pts',(-19.027951217023,13.0010105651996,122.220893833009)) ;
#16406=CARTESIAN_POINT('Ctrl Pts',(-18.9951304778569,12.999420487923,122.231905879089)) ;
#16407=CARTESIAN_POINT('Ctrl Pts',(-18.9457163206155,12.9969958633874,122.250801535115)) ;
#16408=CARTESIAN_POINT('Ctrl Pts',(-18.928769184131,12.9961588816672,122.257712247526)) ;
#16409=CARTESIAN_POINT('Ctrl Pts',(-18.8926559513687,12.9943582312864,122.273371903399)) ;
#16410=CARTESIAN_POINT('Ctrl Pts',(-18.8735469465325,12.9933947708513,122.282238322564)) ;
#16411=CARTESIAN_POINT('Ctrl Pts',(-18.843319986932,12.9918494458271,122.297203007569)) ;
#16412=CARTESIAN_POINT('Ctrl Pts',(-18.8320549271127,12.9912686851965,122.302994901097)) ;
#16413=CARTESIAN_POINT('Ctrl Pts',(-18.7779523075682,12.9884543504816,122.331859529778)) ;
#16414=CARTESIAN_POINT('Ctrl Pts',(-18.7363986331257,12.9862155933072,122.35724886596)) ;
#16415=CARTESIAN_POINT('Ctrl Pts',(-18.6832536210952,12.9832401877453,122.394143349128)) ;
#16416=CARTESIAN_POINT('Ctrl Pts',(-18.670253570575,12.982502785968,122.40354419319)) ;
#16417=CARTESIAN_POINT('Ctrl Pts',(-18.6568542700139,12.9817324570081,122.413632149447)) ;
#16418=CARTESIAN_POINT('Ctrl Pts',(-18.6562708796068,12.9816988970731,122.414072169713)) ;
#16419=CARTESIAN_POINT('Ctrl Pts',(-18.6552280583346,12.9816388710275,122.414860149748)) ;
#16420=CARTESIAN_POINT('Ctrl Pts',(-18.6547684816316,12.9816124043525,122.415207916182)) ;
#16421=CARTESIAN_POINT('Ctrl Pts',(-18.6539431552673,12.9815648512559,122.415833347259)) ;
#16422=CARTESIAN_POINT('Ctrl Pts',(-18.6535773177867,12.9815437644863,122.416110895844)) ;
#16423=CARTESIAN_POINT('Ctrl Pts',(-18.652917595774,12.981505723505,122.416611977756)) ;
#16424=CARTESIAN_POINT('Ctrl Pts',(-18.6526236571881,12.9814887690753,122.416835439821)) ;
#16425=CARTESIAN_POINT('Ctrl Pts',(-18.6520916392232,12.9814580725791,122.417240269984)) ;
#16426=CARTESIAN_POINT('Ctrl Pts',(-18.6518535258812,12.9814443303732,122.417421593418)) ;
#16427=CARTESIAN_POINT('Ctrl Pts',(-18.6514211573751,12.9814193708071,122.417751087661)) ;
#16428=CARTESIAN_POINT('Ctrl Pts',(-18.651226880506,12.9814081533581,122.41789922992)) ;
#16429=CARTESIAN_POINT('Ctrl Pts',(-18.6505383182002,12.9813683878704,122.418424599783)) ;
#16430=CARTESIAN_POINT('Ctrl Pts',(-18.6500442707932,12.981339840836,122.418802139241)) ;
#16431=CARTESIAN_POINT('Ctrl Pts',(-18.6490926691779,12.9812848263507,122.419530456217)) ;
#16432=CARTESIAN_POINT('Ctrl Pts',(-18.6486350755503,12.9812583587371,122.419881181974)) ;
#16433=CARTESIAN_POINT('Ctrl Pts',(-18.647750956529,12.9812071954238,122.420559792556)) ;
#16434=CARTESIAN_POINT('Ctrl Pts',(-18.6473243998143,12.9811824995908,122.420887636422)) ;
#16435=CARTESIAN_POINT('Ctrl Pts',(-18.6464975854278,12.9811346085761,122.421523960694)) ;
#16436=CARTESIAN_POINT('Ctrl Pts',(-18.6460973028754,12.9811114132861,122.421832408666)) ;
#16437=CARTESIAN_POINT('Ctrl Pts',(-18.6453187930819,12.9810662812955,122.422433062091)) ;
#16438=CARTESIAN_POINT('Ctrl Pts',(-18.644940546199,12.9810443445111,122.422725241888)) ;
#16439=CARTESIAN_POINT('Ctrl Pts',(-18.6442022752297,12.9810015103051,122.423296201526)) ;
#16440=CARTESIAN_POINT('Ctrl Pts',(-18.6438422357157,12.9809806128162,122.423574961285)) ;
#16441=CARTESIAN_POINT('Ctrl Pts',(-18.6431368540126,12.9809396549576,122.424121718167)) ;
#16442=CARTESIAN_POINT('Ctrl Pts',(-18.6427914999497,12.9809195945366,122.42438969982)) ;
#16443=CARTESIAN_POINT('Ctrl Pts',(-18.6421121710587,12.9808801199055,122.424917404414)) ;
#16444=CARTESIAN_POINT('Ctrl Pts',(-18.6417781874006,12.9808607056574,122.425177115845)) ;
#16445=CARTESIAN_POINT('Ctrl Pts',(-18.6411183874357,12.9808223380162,122.425690725379)) ;
#16446=CARTESIAN_POINT('Ctrl Pts',(-18.6407925649553,12.9808033845936,122.425944615553)) ;
#16447=CARTESIAN_POINT('Ctrl Pts',(-18.640145871009,12.9807657524226,122.426449053314)) ;
#16448=CARTESIAN_POINT('Ctrl Pts',(-18.6398249960202,12.9807470736617,122.426699596211)) ;
#16449=CARTESIAN_POINT('Ctrl Pts',(-18.6391848458334,12.9807097962395,122.42719993645)) ;
#16450=CARTESIAN_POINT('Ctrl Pts',(-18.6388655696197,12.9806911975741,122.427449732458)) ;
#16451=CARTESIAN_POINT('Ctrl Pts',(-18.6382249639607,12.9806538676342,122.42795143346)) ;
#16452=CARTESIAN_POINT('Ctrl Pts',(-18.6379036362931,12.9806351363697,122.428203340679)) ;
#16453=CARTESIAN_POINT('Ctrl Pts',(-18.6372547426427,12.9805972969007,122.428712559218)) ;
#16454=CARTESIAN_POINT('Ctrl Pts',(-18.6369271817776,12.9805781887261,122.428969876894)) ;
#16455=CARTESIAN_POINT('Ctrl Pts',(-18.6362607636861,12.9805392994611,122.429493925064)) ;
#16456=CARTESIAN_POINT('Ctrl Pts',(-18.6359219157202,12.9805195184189,122.429760667299)) ;
#16457=CARTESIAN_POINT('Ctrl Pts',(-18.635226450761,12.9804789039328,122.430308722763)) ;
#16458=CARTESIAN_POINT('Ctrl Pts',(-18.6348698489277,12.9804580705699,122.430590055126)) ;
#16459=CARTESIAN_POINT('Ctrl Pts',(-18.6343297402126,12.9804265040148,122.431016638618)) ;
#16460=CARTESIAN_POINT('Ctrl Pts',(-18.6341461206411,12.9804157702345,122.431161747025)) ;
#16461=CARTESIAN_POINT('Ctrl Pts',(-18.6336578666299,12.9803872227858,122.431547820649)) ;
#16462=CARTESIAN_POINT('Ctrl Pts',(-18.6333533036907,12.9803694094925,122.431788876335)) ;
#16463=CARTESIAN_POINT('Ctrl Pts',(-18.6320800479274,12.9802949142445,122.432797599279)) ;
#16464=CARTESIAN_POINT('Ctrl Pts',(-18.6311123814247,12.9802382377696,122.433566561274)) ;
#16465=CARTESIAN_POINT('Ctrl Pts',(-18.6234797433569,12.979790713378,122.439650374163)) ;
#16466=CARTESIAN_POINT('Ctrl Pts',(-18.6168681460405,12.9794001674855,122.44503185309)) ;
#16467=CARTESIAN_POINT('Ctrl Pts',(-18.6041453408943,12.9786429798368,122.455605718184)) ;
#16468=CARTESIAN_POINT('Ctrl Pts',(-18.5980280233729,12.9782763130836,122.460790116357)) ;
#16469=CARTESIAN_POINT('Ctrl Pts',(-18.5675857788878,12.9764385012305,122.487097241842)) ;
#16470=CARTESIAN_POINT('Ctrl Pts',(-18.5440338962702,12.9749740577999,122.509095980903)) ;
#16471=CARTESIAN_POINT('Ctrl Pts',(-18.5075320730355,12.9726134887217,122.545933009054)) ;
#16472=CARTESIAN_POINT('Ctrl Pts',(-18.4940368669183,12.9717190257007,122.56020996154)) ;
#16473=CARTESIAN_POINT('Ctrl Pts',(-18.4735195841935,12.9703212760591,122.58296702056)) ;
#16474=CARTESIAN_POINT('Ctrl Pts',(-18.4662635579141,12.9698191604314,122.591231902454)) ;
#16475=CARTESIAN_POINT('Ctrl Pts',(-18.4526278932898,12.9688599725934,122.607183176556)) ;
#16476=CARTESIAN_POINT('Ctrl Pts',(-18.4462294645572,12.9684030344231,122.614852403913)) ;
#16477=CARTESIAN_POINT('Ctrl Pts',(-18.4365858263844,12.9677034888554,122.626697116171)) ;
#16478=CARTESIAN_POINT('Ctrl Pts',(-18.4332740517988,12.9674612371538,122.630817892419)) ;
#16479=CARTESIAN_POINT('Ctrl Pts',(-18.4236239785505,12.966749325402,122.642982532909)) ;
#16480=CARTESIAN_POINT('Ctrl Pts',(-18.417358283924,12.9662793296657,122.651083411056)) ;
#16481=CARTESIAN_POINT('Ctrl Pts',(-18.3971954033054,12.9647408224713,122.677824555117)) ;
#16482=CARTESIAN_POINT('Ctrl Pts',(-18.3837186616704,12.9636706487908,122.696775613893)) ;
#16483=CARTESIAN_POINT('Ctrl Pts',(-18.3566449155309,12.9614295702289,122.737188136417)) ;
#16484=CARTESIAN_POINT('Ctrl Pts',(-18.3431576106487,12.9602589686713,122.75871067245)) ;
#16485=CARTESIAN_POINT('Ctrl Pts',(-18.3270206646114,12.9587889819773,122.786294883082)) ;
#16486=CARTESIAN_POINT('Ctrl Pts',(-18.323750793524,12.9584872474056,122.791986740363)) ;
#16487=CARTESIAN_POINT('Ctrl Pts',(-18.320511645787,12.9581844576396,122.797729373897)) ;
#16488=CARTESIAN_POINT('Ctrl Pts',(-18.3204973895175,12.9581831249122,122.797754650668)) ;
#16489=CARTESIAN_POINT('Ctrl Pts',(-18.3204691408688,12.9581804839746,122.7978047404)) ;
#16490=CARTESIAN_POINT('Ctrl Pts',(-18.3204551484335,12.9581791757621,122.797829553387)) ;
#16491=CARTESIAN_POINT('Ctrl Pts',(-18.3204274204869,12.9581765832113,122.797878727682)) ;
#16492=CARTESIAN_POINT('Ctrl Pts',(-18.3204136850449,12.9581752988823,122.797903088795)) ;
#16493=CARTESIAN_POINT('Ctrl Pts',(-18.3203864645046,12.9581727534913,122.797951370802)) ;
#16494=CARTESIAN_POINT('Ctrl Pts',(-18.3203729794039,12.9581714924316,122.79797529163)) ;
#16495=CARTESIAN_POINT('Ctrl Pts',(-18.3203462532489,12.9581689929981,122.798022704032)) ;
#16496=CARTESIAN_POINT('Ctrl Pts',(-18.3203330120995,12.9581677546178,122.798046195708)) ;
#16497=CARTESIAN_POINT('Ctrl Pts',(-18.3203067676139,12.9581652999673,122.79809276067)) ;
#16498=CARTESIAN_POINT('Ctrl Pts',(-18.3202937642996,12.9581640837015,122.798115833853)) ;
#16499=CARTESIAN_POINT('Ctrl Pts',(-18.3202679893627,12.9581616727145,122.798161572502)) ;
#16500=CARTESIAN_POINT('Ctrl Pts',(-18.3202552178929,12.9581604780098,122.798184237637)) ;
#16501=CARTESIAN_POINT('Ctrl Pts',(-18.3202299010075,12.9581581096243,122.798229170014)) ;
#16502=CARTESIAN_POINT('Ctrl Pts',(-18.320217355408,12.9581569359284,122.798251437526)) ;
#16503=CARTESIAN_POINT('Ctrl Pts',(-18.3201924845428,12.9581546090318,122.79829558464)) ;
#16504=CARTESIAN_POINT('Ctrl Pts',(-18.3201801593888,12.9581534558435,122.798317463988)) ;
#16505=CARTESIAN_POINT('Ctrl Pts',(-18.3201557240377,12.9581511694652,122.798360844154)) ;
#16506=CARTESIAN_POINT('Ctrl Pts',(-18.3201436136676,12.958150036261,122.798382345226)) ;
#16507=CARTESIAN_POINT('Ctrl Pts',(-18.320119602475,12.9581477893504,122.798424978287)) ;
#16508=CARTESIAN_POINT('Ctrl Pts',(-18.3201077017835,12.9581466756582,122.798446109992)) ;
#16509=CARTESIAN_POINT('Ctrl Pts',(-18.3200841050796,12.9581444673218,122.798488012811)) ;
#16510=CARTESIAN_POINT('Ctrl Pts',(-18.3200724086253,12.958143372638,122.798508784662)) ;
#16511=CARTESIAN_POINT('Ctrl Pts',(-18.3200408206558,12.9581404161459,122.798564885807)) ;
#16512=CARTESIAN_POINT('Ctrl Pts',(-18.3200209304437,12.9581385543615,122.798600215418)) ;
#16513=CARTESIAN_POINT('Ctrl Pts',(-18.3199812996294,12.9581348444979,122.798670616911)) ;
#16514=CARTESIAN_POINT('Ctrl Pts',(-18.3199615590029,12.9581329964186,122.798705688777)) ;
#16515=CARTESIAN_POINT('Ctrl Pts',(-18.3199222249075,12.9581293137423,122.79877557896)) ;
#16516=CARTESIAN_POINT('Ctrl Pts',(-18.3199026313337,12.9581274791376,122.798810397407)) ;
#16517=CARTESIAN_POINT('Ctrl Pts',(-18.3198635887295,12.9581238231721,122.798879785223)) ;
#16518=CARTESIAN_POINT('Ctrl Pts',(-18.3198441397624,12.9581220018193,122.798914354426)) ;
#16519=CARTESIAN_POINT('Ctrl Pts',(-18.3198053839813,12.95811837214,122.798983247836)) ;
#16520=CARTESIAN_POINT('Ctrl Pts',(-18.3197860769893,12.9581165637989,122.799017572306)) ;
#16521=CARTESIAN_POINT('Ctrl Pts',(-18.3197476025284,12.9581129599028,122.799085980764)) ;
#16522=CARTESIAN_POINT('Ctrl Pts',(-18.3197284352537,12.958111164368,122.799120064353)) ;
#16523=CARTESIAN_POINT('Ctrl Pts',(-18.3196902379257,12.9581075858748,122.799187994982)) ;
#16524=CARTESIAN_POINT('Ctrl Pts',(-18.3196712076845,12.9581058029009,122.799221842304)) ;
#16525=CARTESIAN_POINT('Ctrl Pts',(-18.3196332820241,12.9581022493103,122.799289304511)) ;
#16526=CARTESIAN_POINT('Ctrl Pts',(-18.319614386617,12.9581004786969,122.799322919324)) ;
#16527=CARTESIAN_POINT('Ctrl Pts',(-18.319576728093,12.9580969495959,122.799389920864)) ;
#16528=CARTESIAN_POINT('Ctrl Pts',(-18.319557965132,12.9580951911248,122.799423307264)) ;
#16529=CARTESIAN_POINT('Ctrl Pts',(-18.3195205692749,12.9580916861055,122.79948985579)) ;
#16530=CARTESIAN_POINT('Ctrl Pts',(-18.3195019362965,12.9580899395515,122.799523018014)) ;
#16531=CARTESIAN_POINT('Ctrl Pts',(-18.3194647981766,12.9580864581629,122.799589122009)) ;
#16532=CARTESIAN_POINT('Ctrl Pts',(-18.3194462929502,12.9580847233222,122.799622063884)) ;
#16533=CARTESIAN_POINT('Ctrl Pts',(-18.319409408017,12.9580812651482,122.799687731163)) ;
#16534=CARTESIAN_POINT('Ctrl Pts',(-18.319391028292,12.9580795418151,122.799720456554)) ;
#16535=CARTESIAN_POINT('Ctrl Pts',(-18.3193543920568,12.9580761064453,122.799785694832)) ;
#16536=CARTESIAN_POINT('Ctrl Pts',(-18.3193361355751,12.9580743944131,122.799818207623)) ;
#16537=CARTESIAN_POINT('Ctrl Pts',(-18.3192997436849,12.9580709814495,122.799883024381)) ;
#16538=CARTESIAN_POINT('Ctrl Pts',(-18.31928160816,12.9580692805088,122.79991532851)) ;
#16539=CARTESIAN_POINT('Ctrl Pts',(-18.3192454558336,12.9580658895128,122.799979732)) ;
#16540=CARTESIAN_POINT('Ctrl Pts',(-18.3192274392185,12.9580641994765,122.800011830984)) ;
#16541=CARTESIAN_POINT('Ctrl Pts',(-18.3191915225708,12.9580608300932,122.800075827869)) ;
#16542=CARTESIAN_POINT('Ctrl Pts',(-18.3191736225289,12.9580591507469,122.800107725744)) ;
#16543=CARTESIAN_POINT('Ctrl Pts',(-18.3191379370034,12.9580558025584,122.800171323891)) ;
#16544=CARTESIAN_POINT('Ctrl Pts',(-18.3191201514281,12.9580541337091,122.800203024287)) ;
#16545=CARTESIAN_POINT('Ctrl Pts',(-18.3190846927604,12.9580508063243,122.800266231052)) ;
#16546=CARTESIAN_POINT('Ctrl Pts',(-18.3190670195495,12.9580491477793,122.800297737594)) ;
#16547=CARTESIAN_POINT('Ctrl Pts',(-18.3190317834253,12.9580458408024,122.80036056043)) ;
#16548=CARTESIAN_POINT('Ctrl Pts',(-18.3190142205457,12.9580441923752,122.800391876624)) ;
#16549=CARTESIAN_POINT('Ctrl Pts',(-18.318979203096,12.9580409054517,122.800454322194)) ;
#16550=CARTESIAN_POINT('Ctrl Pts',(-18.3189617483507,12.9580392669405,122.800485451844)) ;
#16551=CARTESIAN_POINT('Ctrl Pts',(-18.3189269448545,12.9580359996359,122.800547528339)) ;
#16552=CARTESIAN_POINT('Ctrl Pts',(-18.3189095964382,12.9580343708753,122.800578474552)) ;
#16553=CARTESIAN_POINT('Ctrl Pts',(-18.3188750037851,12.9580311229058,122.8006401873)) ;
#16554=CARTESIAN_POINT('Ctrl Pts',(-18.3188577592977,12.9580295036747,122.800670954246)) ;
#16555=CARTESIAN_POINT('Ctrl Pts',(-18.3188233724603,12.9580262745764,122.800732311998)) ;
#16556=CARTESIAN_POINT('Ctrl Pts',(-18.3188062302139,12.9580246647203,122.800762902584)) ;
#16557=CARTESIAN_POINT('Ctrl Pts',(-18.3187720458929,12.9580214541912,122.800823911017)) ;
#16558=CARTESIAN_POINT('Ctrl Pts',(-18.3187550037101,12.9580198535094,122.800854329023)) ;
#16559=CARTESIAN_POINT('Ctrl Pts',(-18.3187210176789,12.9580166611602,122.800914995474)) ;
#16560=CARTESIAN_POINT('Ctrl Pts',(-18.3187040736376,12.9580150694761,122.80094524423)) ;
#16561=CARTESIAN_POINT('Ctrl Pts',(-18.3186702818322,12.9580118949326,122.801005575753)) ;
#16562=CARTESIAN_POINT('Ctrl Pts',(-18.3186534340845,12.9580103120762,122.801035658459)) ;
#16563=CARTESIAN_POINT('Ctrl Pts',(-18.3186198328771,12.958007155005,122.801095661336)) ;
#16564=CARTESIAN_POINT('Ctrl Pts',(-18.3186030794223,12.9580055807919,122.801125581467)) ;
#16565=CARTESIAN_POINT('Ctrl Pts',(-18.3185696648586,12.9580024408285,122.801185262568)) ;
#16566=CARTESIAN_POINT('Ctrl Pts',(-18.3185530038092,12.9580008750849,122.801215023402)) ;
#16567=CARTESIAN_POINT('Ctrl Pts',(-18.3185197722134,12.9579977518908,122.801274389108)) ;
#16568=CARTESIAN_POINT('Ctrl Pts',(-18.3185032016251,12.9579961944375,122.801303994025)) ;
#16569=CARTESIAN_POINT('Ctrl Pts',(-18.3184701490802,12.9579930876513,122.801363051152)) ;
#16570=CARTESIAN_POINT('Ctrl Pts',(-18.3184536671329,12.9579915383205,122.801392503316)) ;
#16571=CARTESIAN_POINT('Ctrl Pts',(-18.3184207900036,12.9579884476071,122.801451258183)) ;
#16572=CARTESIAN_POINT('Ctrl Pts',(-18.3184043948167,12.9579869062252,122.801480560867)) ;
#16573=CARTESIAN_POINT('Ctrl Pts',(-18.3183716893758,12.9579838312407,122.801539019963)) ;
#16574=CARTESIAN_POINT('Ctrl Pts',(-18.3183553791066,12.9579822976377,122.801568176376)) ;
#16575=CARTESIAN_POINT('Ctrl Pts',(-18.3183228416279,12.957979238038,122.801626346195)) ;
#16576=CARTESIAN_POINT('Ctrl Pts',(-18.3183066144865,12.9579777120487,122.801655359453)) ;
#16577=CARTESIAN_POINT('Ctrl Pts',(-18.3182742414877,12.9579746675123,122.801713246059)) ;
#16578=CARTESIAN_POINT('Ctrl Pts',(-18.3182580955985,12.9579731489632,122.801742119436)) ;
#16579=CARTESIAN_POINT('Ctrl Pts',(-18.3182258833002,12.9579701191407,122.801799729426)) ;
#16580=CARTESIAN_POINT('Ctrl Pts',(-18.3182098169197,12.9579686078709,122.801828465963)) ;
#16581=CARTESIAN_POINT('Ctrl Pts',(-18.318177761933,12.9579655924493,122.801885805246)) ;
#16582=CARTESIAN_POINT('Ctrl Pts',(-18.3181617732108,12.9579640882874,122.801914408175)) ;
#16583=CARTESIAN_POINT('Ctrl Pts',(-18.3181298717196,12.9579610869133,122.801971483426)) ;
#16584=CARTESIAN_POINT('Ctrl Pts',(-18.3181139589831,12.9579595897049,122.801999955666)) ;
#16585=CARTESIAN_POINT('Ctrl Pts',(-18.3180822072798,12.9579566020348,122.802056773373)) ;
#16586=CARTESIAN_POINT('Ctrl Pts',(-18.3180663683915,12.9579551115814,122.802085118677)) ;
#16587=CARTESIAN_POINT('Ctrl Pts',(-18.3180347599055,12.9579521370024,122.802141690458)) ;
#16588=CARTESIAN_POINT('Ctrl Pts',(-18.3180189903425,12.9579506528809,122.802169916852)) ;
#16589=CARTESIAN_POINT('Ctrl Pts',(-18.317987515633,12.9579476905094,122.802226259472)) ;
#16590=CARTESIAN_POINT('Ctrl Pts',(-18.3179718104936,12.9579462122609,122.802254375665)) ;
#16591=CARTESIAN_POINT('Ctrl Pts',(-18.3179404598983,12.9579432611921,122.802310506299)) ;
#16592=CARTESIAN_POINT('Ctrl Pts',(-18.3179248142511,12.9579417883546,122.802338521063)) ;
#16593=CARTESIAN_POINT('Ctrl Pts',(-18.3178935777475,12.9579388476493,122.802394457543)) ;
#16594=CARTESIAN_POINT('Ctrl Pts',(-18.3178779868653,12.9579373797797,122.802422379288)) ;
#16595=CARTESIAN_POINT('Ctrl Pts',(-18.3178468549704,12.9579344485489,122.802478138494)) ;
#16596=CARTESIAN_POINT('Ctrl Pts',(-18.3178313139951,12.9579329851917,122.802505975872)) ;
#16597=CARTESIAN_POINT('Ctrl Pts',(-18.3178002771128,12.9579300625354,122.802561574899)) ;
#16598=CARTESIAN_POINT('Ctrl Pts',(-18.3177847811949,12.9579286032356,122.802589336553)) ;
#16599=CARTESIAN_POINT('Ctrl Pts',(-18.3177538295913,12.9579256882402,122.802644792755)) ;
#16600=CARTESIAN_POINT('Ctrl Pts',(-18.3177383739782,12.9579242325517,122.80267248716)) ;
#16601=CARTESIAN_POINT('Ctrl Pts',(-18.3177074983048,12.9579213243395,122.802727817214)) ;
#16602=CARTESIAN_POINT('Ctrl Pts',(-18.3176920781,12.9579198718025,122.80275545311)) ;
#16603=CARTESIAN_POINT('Ctrl Pts',(-18.3176612684483,12.9579169694427,122.802810674706)) ;
#16604=CARTESIAN_POINT('Ctrl Pts',(-18.3176458789701,12.9579155196172,122.802838260454)) ;
#16605=CARTESIAN_POINT('Ctrl Pts',(-18.3176151259614,12.9579126222283,122.802893390349)) ;
#16606=CARTESIAN_POINT('Ctrl Pts',(-18.3175997623536,12.9579111746578,122.802920934628)) ;
#16607=CARTESIAN_POINT('Ctrl Pts',(-18.3175689857566,12.9579082746817,122.802976116626)) ;
#16608=CARTESIAN_POINT('Ctrl Pts',(-18.3175535730068,12.957906822298,122.803003753934)) ;
#16609=CARTESIAN_POINT('Ctrl Pts',(-18.3175226870624,12.9579039116511,122.803059141879)) ;
#16610=CARTESIAN_POINT('Ctrl Pts',(-18.3175072138764,12.9579024533879,122.803086892521)) ;
#16611=CARTESIAN_POINT('Ctrl Pts',(-18.3174762059163,12.9578995308718,122.803142509248)) ;
#16612=CARTESIAN_POINT('Ctrl Pts',(-18.3174606711264,12.9578980666167,122.803170375381)) ;
#16613=CARTESIAN_POINT('Ctrl Pts',(-18.3174295382349,12.957895131952,122.803226226241)) ;
#16614=CARTESIAN_POINT('Ctrl Pts',(-18.3174139403413,12.9578936615613,122.803254210618)) ;
#16615=CARTESIAN_POINT('Ctrl Pts',(-18.3173826802084,12.9578907145256,122.803310299884)) ;
#16616=CARTESIAN_POINT('Ctrl Pts',(-18.3173670179411,12.9578892378772,122.803338404846)) ;
#16617=CARTESIAN_POINT('Ctrl Pts',(-18.3173356275022,12.9578862781766,122.803394738146)) ;
#16618=CARTESIAN_POINT('Ctrl Pts',(-18.3173198993763,12.957884795128,122.803422966424)) ;
#16619=CARTESIAN_POINT('Ctrl Pts',(-18.317288376136,12.9578818225223,122.80347954837)) ;
#16620=CARTESIAN_POINT('Ctrl Pts',(-18.3172725808613,12.9578803329492,122.803507902347)) ;
#16621=CARTESIAN_POINT('Ctrl Pts',(-18.3172409216345,12.9578773471329,122.803564738791)) ;
#16622=CARTESIAN_POINT('Ctrl Pts',(-18.3172250577093,12.9578758508913,122.803593221233)) ;
#16623=CARTESIAN_POINT('Ctrl Pts',(-18.3171932596826,12.9578728515937,122.803650317367)) ;
#16624=CARTESIAN_POINT('Ctrl Pts',(-18.3171773256136,12.9578713485399,122.803678931025)) ;
#16625=CARTESIAN_POINT('Ctrl Pts',(-18.3171453859397,12.9578683354871,122.803736292105)) ;
#16626=CARTESIAN_POINT('Ctrl Pts',(-18.3171293802991,12.9578668254838,122.803765039616)) ;
#16627=CARTESIAN_POINT('Ctrl Pts',(-18.3170972958036,12.9578637983708,122.803822671491)) ;
#16628=CARTESIAN_POINT('Ctrl Pts',(-18.3170812170452,12.9578622812693,122.803851555707)) ;
#16629=CARTESIAN_POINT('Ctrl Pts',(-18.3170489846219,12.9578592397973,122.803909464108)) ;
#16630=CARTESIAN_POINT('Ctrl Pts',(-18.317032831108,12.9578577154401,122.803938488047)) ;
#16631=CARTESIAN_POINT('Ctrl Pts',(-18.3170004478664,12.9578546593306,122.803996678322)) ;
#16632=CARTESIAN_POINT('Ctrl Pts',(-18.3169842180737,12.9578531275711,122.804025844801)) ;
#16633=CARTESIAN_POINT('Ctrl Pts',(-18.3169516808187,12.9578500565165,122.804084322851)) ;
#16634=CARTESIAN_POINT('Ctrl Pts',(-18.3169353732382,12.9578485172092,122.804113634662)) ;
#16635=CARTESIAN_POINT('Ctrl Pts',(-18.316902678415,12.9578454308678,122.804172407039)) ;
#16636=CARTESIAN_POINT('Ctrl Pts',(-18.3168862912965,12.9578438838444,122.80420186741)) ;
#16637=CARTESIAN_POINT('Ctrl Pts',(-18.3168534359091,12.9578407819271,122.804260939667)) ;
#16638=CARTESIAN_POINT('Ctrl Pts',(-18.3168369676573,12.9578392270338,122.804290551552)) ;
#16639=CARTESIAN_POINT('Ctrl Pts',(-18.316803948079,12.9578361091918,122.804349930383)) ;
#16640=CARTESIAN_POINT('Ctrl Pts',(-18.3167873968819,12.9578345462542,122.804379697126)) ;
#16641=CARTESIAN_POINT('Ctrl Pts',(-18.3167542100353,12.9578314121902,122.804439388242)) ;
#16642=CARTESIAN_POINT('Ctrl Pts',(-18.3167375742817,12.9578298410529,122.804469312831)) ;
#16643=CARTESIAN_POINT('Ctrl Pts',(-18.3167042163813,12.9578266904026,122.80452932322)) ;
#16644=CARTESIAN_POINT('Ctrl Pts',(-18.3166874942634,12.9578251108913,122.804559408999)) ;
#16645=CARTESIAN_POINT('Ctrl Pts',(-18.3166539617726,12.9578219433137,122.804619745211)) ;
#16646=CARTESIAN_POINT('Ctrl Pts',(-18.3166371514269,12.9578203552488,122.804649995627)) ;
#16647=CARTESIAN_POINT('Ctrl Pts',(-18.316603440968,12.9578171704177,122.80471066393)) ;
#16648=CARTESIAN_POINT('Ctrl Pts',(-18.3165865406907,12.9578155736347,122.804741082145)) ;
#16649=CARTESIAN_POINT('Ctrl Pts',(-18.316552648186,12.9578123711574,122.804802090074)) ;
#16650=CARTESIAN_POINT('Ctrl Pts',(-18.3165356559975,12.9578107654655,122.804832679751)) ;
#16651=CARTESIAN_POINT('Ctrl Pts',(-18.3165015779855,12.9578075450074,122.804894033737)) ;
#16652=CARTESIAN_POINT('Ctrl Pts',(-18.3164844920787,12.957805930232,122.804924798231)) ;
#16653=CARTESIAN_POINT('Ctrl Pts',(-18.3164502243585,12.9578026913883,122.804986506045)) ;
#16654=CARTESIAN_POINT('Ctrl Pts',(-18.3164330426506,12.9578010673286,122.80501744921)) ;
#16655=CARTESIAN_POINT('Ctrl Pts',(-18.3163985817227,12.9577978097606,122.805079517366)) ;
#16656=CARTESIAN_POINT('Ctrl Pts',(-18.3163813023888,12.9577961762401,122.805110642597)) ;
#16657=CARTESIAN_POINT('Ctrl Pts',(-18.3163466437754,12.9577928995163,122.805173079376)) ;
#16658=CARTESIAN_POINT('Ctrl Pts',(-18.3163292646603,12.9577912563271,122.805204390666)) ;
#16659=CARTESIAN_POINT('Ctrl Pts',(-18.3162944045629,12.95778796008,122.805267203136)) ;
#16660=CARTESIAN_POINT('Ctrl Pts',(-18.3162769236473,12.9577863070269,122.805298704235)) ;
#16661=CARTESIAN_POINT('Ctrl Pts',(-18.3162418576804,12.9577829908332,122.805361900527)) ;
#16662=CARTESIAN_POINT('Ctrl Pts',(-18.3162242727583,12.9577813277032,122.805393595527)) ;
#16663=CARTESIAN_POINT('Ctrl Pts',(-18.316188996903,12.9577779911739,122.805457183121)) ;
#16664=CARTESIAN_POINT('Ctrl Pts',(-18.3161713058894,12.9577763177654,122.8054890759)) ;
#16665=CARTESIAN_POINT('Ctrl Pts',(-18.31613581567,12.957772960468,122.805553063104)) ;
#16666=CARTESIAN_POINT('Ctrl Pts',(-18.3161180164072,12.9577712765722,122.805585157674)) ;
#16667=CARTESIAN_POINT('Ctrl Pts',(-18.3160823071395,12.9577678980544,122.805649553184)) ;
#16668=CARTESIAN_POINT('Ctrl Pts',(-18.316064397259,12.9577662034425,122.805681853942)) ;
#16669=CARTESIAN_POINT('Ctrl Pts',(-18.3160324290167,12.95776317842,122.805739515208)) ;
#16670=CARTESIAN_POINT('Ctrl Pts',(-18.3160183700517,12.9577618480006,122.805764875509)) ;
#16671=CARTESIAN_POINT('Ctrl Pts',(-18.3159899011619,12.9577591537927,122.805816233405)) ;
#16672=CARTESIAN_POINT('Ctrl Pts',(-18.3159754912136,12.957757789998,122.805842231148)) ;
#16673=CARTESIAN_POINT('Ctrl Pts',(-18.3159463075245,12.957755027813,122.8058948874)) ;
#16674=CARTESIAN_POINT('Ctrl Pts',(-18.3159315339375,12.9577536294331,122.805921545745)) ;
#16675=CARTESIAN_POINT('Ctrl Pts',(-18.3159016099104,12.9577507968285,122.805975547108)) ;
#16676=CARTESIAN_POINT('Ctrl Pts',(-18.3158864595222,12.9577493626044,122.806002890153)) ;
#16677=CARTESIAN_POINT('Ctrl Pts',(-18.3158557680647,12.9577464569889,122.806058286236)) ;
#16678=CARTESIAN_POINT('Ctrl Pts',(-18.3158402270104,12.9577449855942,122.806086339374)) ;
#16679=CARTESIAN_POINT('Ctrl Pts',(-18.3158087398723,12.9577420042647,122.806143181929)) ;
#16680=CARTESIAN_POINT('Ctrl Pts',(-18.3157927937014,12.9577404943166,122.806171971638)) ;
#16681=CARTESIAN_POINT('Ctrl Pts',(-18.3157604808174,12.9577374343961,122.806230315753)) ;
#16682=CARTESIAN_POINT('Ctrl Pts',(-18.3157441142046,12.9577358844277,122.806259870121)) ;
#16683=CARTESIAN_POINT('Ctrl Pts',(-18.3157109441543,12.9577327429083,122.806319773394)) ;
#16684=CARTESIAN_POINT('Ctrl Pts',(-18.3156941409143,12.9577311513702,122.806350122095)) ;
#16685=CARTESIAN_POINT('Ctrl Pts',(-18.3156600808917,12.9577279251104,122.806411644695)) ;
#16686=CARTESIAN_POINT('Ctrl Pts',(-18.3156428241278,12.9577262903843,122.806442818723)) ;
#16687=CARTESIAN_POINT('Ctrl Pts',(-18.3156078393083,12.9577229760484,122.806506024537)) ;
#16688=CARTESIAN_POINT('Ctrl Pts',(-18.3155901112489,12.9577212964318,122.806538056505)) ;
#16689=CARTESIAN_POINT('Ctrl Pts',(-18.3155541645785,12.9577178904702,122.806603013531)) ;
#16690=CARTESIAN_POINT('Ctrl Pts',(-18.315535946212,12.9577161641414,122.806635938334)) ;
#16691=CARTESIAN_POINT('Ctrl Pts',(-18.3154989995035,12.9577126628936,122.806702716702)) ;
#16692=CARTESIAN_POINT('Ctrl Pts',(-18.3154802711214,12.9577108879633,122.80673657054)) ;
#16693=CARTESIAN_POINT('Ctrl Pts',(-18.3154422829925,12.9577072874628,122.806805246248)) ;
#16694=CARTESIAN_POINT('Ctrl Pts',(-18.3154230234525,12.957705461904,122.806840067961)) ;
#16695=CARTESIAN_POINT('Ctrl Pts',(-18.315383951108,12.9577017580462,122.806910719666)) ;
#16696=CARTESIAN_POINT('Ctrl Pts',(-18.3153641383384,12.9576998797418,122.806946549827)) ;
#16697=CARTESIAN_POINT('Ctrl Pts',(-18.3153239356422,12.9576960681015,122.807019262336)) ;
#16698=CARTESIAN_POINT('Ctrl Pts',(-18.3153035459935,12.9576941347826,122.807056144429)) ;
#16699=CARTESIAN_POINT('Ctrl Pts',(-18.3152621649308,12.9576902107518,122.807131006068)) ;
#16700=CARTESIAN_POINT('Ctrl Pts',(-18.3152411735959,12.9576882200374,122.807168985737)) ;
#16701=CARTESIAN_POINT('Ctrl Pts',(-18.3151985626186,12.9576841786682,122.807246091354)) ;
#16702=CARTESIAN_POINT('Ctrl Pts',(-18.3151769431235,12.9576821280167,122.807285217323)) ;
#16703=CARTESIAN_POINT('Ctrl Pts',(-18.3151330481096,12.9576779641117,122.80736466657)) ;
#16704=CARTESIAN_POINT('Ctrl Pts',(-18.3151107725755,12.9576758508452,122.807404990183)) ;
#16705=CARTESIAN_POINT('Ctrl Pts',(-18.3150655353323,12.957671558815,122.807486890234)) ;
#16706=CARTESIAN_POINT('Ctrl Pts',(-18.3150425738581,12.957669380061,122.807528466577)) ;
#16707=CARTESIAN_POINT('Ctrl Pts',(-18.3149959333314,12.9576649540381,122.807612929959)) ;
#16708=CARTESIAN_POINT('Ctrl Pts',(-18.314972254352,12.9576627067626,122.807655817222)) ;
#16709=CARTESIAN_POINT('Ctrl Pts',(-18.3149241449129,12.9576581404384,122.807742964933)) ;
#16710=CARTESIAN_POINT('Ctrl Pts',(-18.314899714647,12.9576558213935,122.807787225418)) ;
#16711=CARTESIAN_POINT('Ctrl Pts',(-18.3148500668834,12.9576511080926,122.807877185519)) ;
#16712=CARTESIAN_POINT('Ctrl Pts',(-18.3148248494684,12.9576487138287,122.807922885405)) ;
#16713=CARTESIAN_POINT('Ctrl Pts',(-18.3147735889681,12.9576438463923,122.808015795242)) ;
#16714=CARTESIAN_POINT('Ctrl Pts',(-18.3147475460057,12.9576413732145,122.808063005424)) ;
#16715=CARTESIAN_POINT('Ctrl Pts',(-18.314694593362,12.9576363440003,122.808159011647)) ;
#16716=CARTESIAN_POINT('Ctrl Pts',(-18.3146676839348,12.9576337879696,122.808207807719)) ;
#16717=CARTESIAN_POINT('Ctrl Pts',(-18.3146129545306,12.95762858883,122.808307066698)) ;
#16718=CARTESIAN_POINT('Ctrl Pts',(-18.3145851347164,12.9576259457165,122.808357529846)) ;
#16719=CARTESIAN_POINT('Ctrl Pts',(-18.3145285375267,12.9576205678836,122.808460209882)) ;
#16720=CARTESIAN_POINT('Ctrl Pts',(-18.3144997604089,12.9576178331669,122.808512426885)) ;
#16721=CARTESIAN_POINT('Ctrl Pts',(-18.3144411981411,12.9576122672647,122.808618707985)) ;
#16722=CARTESIAN_POINT('Ctrl Pts',(-18.3144114132964,12.9576094360844,122.808672772163)) ;
#16723=CARTESIAN_POINT('Ctrl Pts',(-18.3143507814169,12.9576036720343,122.808782847852)) ;
#16724=CARTESIAN_POINT('Ctrl Pts',(-18.3143199346509,12.9576007391641,122.808838859568)) ;
#16725=CARTESIAN_POINT('Ctrl Pts',(-18.3142571205621,12.9575947661053,122.808952938428)) ;
#16726=CARTESIAN_POINT('Ctrl Pts',(-18.3142251536367,12.9575917259261,122.809011005608)) ;
#16727=CARTESIAN_POINT('Ctrl Pts',(-18.3141600363797,12.9575855321851,122.809129311873)) ;
#16728=CARTESIAN_POINT('Ctrl Pts',(-18.3141268863937,12.9575823786251,122.809189551159)) ;
#16729=CARTESIAN_POINT('Ctrl Pts',(-18.3140593351694,12.957575951573,122.809312327458)) ;
#16730=CARTESIAN_POINT('Ctrl Pts',(-18.3140249342908,12.9575726780808,122.809374864729)) ;
#16731=CARTESIAN_POINT('Ctrl Pts',(-18.3104970887637,12.9572369292352,122.815789427175)) ;
#16732=CARTESIAN_POINT('Ctrl Pts',(-18.3070589554122,12.956904803191,122.822171731532)) ;
#16733=CARTESIAN_POINT('Ctrl Pts',(-18.2961610813973,12.9558355002876,122.842830179727)) ;
#16734=CARTESIAN_POINT('Ctrl Pts',(-18.2889216865892,12.9550993590262,122.857220735031)) ;
#16735=CARTESIAN_POINT('Ctrl Pts',(-18.27147266284,12.9532542762629,122.893642974524)) ;
#16736=CARTESIAN_POINT('Ctrl Pts',(-18.2616230735756,12.9521459955161,122.915839710725)) ;
#16737=CARTESIAN_POINT('Ctrl Pts',(-18.2459725991599,12.950257428141,122.95407622725)) ;
#16738=CARTESIAN_POINT('Ctrl Pts',(-18.2398420577145,12.9494781401921,122.969973552403)) ;
#16739=CARTESIAN_POINT('Ctrl Pts',(-18.2295216232024,12.948090626654,122.998457026655)) ;
#16740=CARTESIAN_POINT('Ctrl Pts',(-18.2252034973743,12.947482880953,123.010993933247)) ;
#16741=CARTESIAN_POINT('Ctrl Pts',(-18.2142783325241,12.9458689441818,123.044431744035)) ;
#16742=CARTESIAN_POINT('Ctrl Pts',(-18.2080202126451,12.9448619942941,123.0654417458)) ;
#16743=CARTESIAN_POINT('Ctrl Pts',(-18.1943463949412,12.9424452373669,123.116189647364)) ;
#16744=CARTESIAN_POINT('Ctrl Pts',(-18.1874654466672,12.941035227401,123.146057058026)) ;
#16745=CARTESIAN_POINT('Ctrl Pts',(-18.1816683493887,12.9396231975372,123.176253950506)) ;
#16746=CARTESIAN_POINT('Ctrl Pts',(-18.1816478436446,12.9396181994907,123.176360839662)) ;
#16747=CARTESIAN_POINT('Ctrl Pts',(-18.1816080473459,12.9396084930705,123.176568430149)) ;
#16748=CARTESIAN_POINT('Ctrl Pts',(-18.1815887552277,12.9396037846932,123.176669131141)) ;
#16749=CARTESIAN_POINT('Ctrl Pts',(-18.1815512981532,12.9395946372377,123.176864779826)) ;
#16750=CARTESIAN_POINT('Ctrl Pts',(-18.1815331318249,12.9395901981559,123.176959727234)) ;
#16751=CARTESIAN_POINT('Ctrl Pts',(-18.1814978459639,12.9395815706274,123.177144266888)) ;
#16752=CARTESIAN_POINT('Ctrl Pts',(-18.1814807252205,12.939577382176,123.177233858916)) ;
#16753=CARTESIAN_POINT('Ctrl Pts',(-18.181447457043,12.9395692387868,123.177408053108)) ;
#16754=CARTESIAN_POINT('Ctrl Pts',(-18.1814313085426,12.9395652838446,123.177492655087)) ;
#16755=CARTESIAN_POINT('Ctrl Pts',(-18.1813999175518,12.9395575917456,123.177657204805)) ;
#16756=CARTESIAN_POINT('Ctrl Pts',(-18.1813846741313,12.9395538545871,123.177737152332)) ;
#16757=CARTESIAN_POINT('Ctrl Pts',(-18.1813550316109,12.9395465835969,123.17789270173)) ;
#16758=CARTESIAN_POINT('Ctrl Pts',(-18.1813406316666,12.9395430497578,123.177968303538)) ;
#16759=CARTESIAN_POINT('Ctrl Pts',(-18.1813126194362,12.9395361720888,123.178115445765)) ;
#16760=CARTESIAN_POINT('Ctrl Pts',(-18.1812990064273,12.9395328282582,123.178186986005)) ;
#16761=CARTESIAN_POINT('Ctrl Pts',(-18.1812725159887,12.9395263183341,123.178326267087)) ;
#16762=CARTESIAN_POINT('Ctrl Pts',(-18.1812596379002,12.9395231522354,123.178394007869)) ;
#16763=CARTESIAN_POINT('Ctrl Pts',(-18.1812345693507,12.9395169864471,123.178525931897)) ;
#16764=CARTESIAN_POINT('Ctrl Pts',(-18.1812223783251,12.9395139867577,123.178590114987)) ;
#16765=CARTESIAN_POINT('Ctrl Pts',(-18.1811986397071,12.9395081433232,123.1787151471)) ;
#16766=CARTESIAN_POINT('Ctrl Pts',(-18.1811870916137,12.9395052995784,123.178775995981)) ;
#16767=CARTESIAN_POINT('Ctrl Pts',(-18.1811645981009,12.9394997583599,123.178894566255)) ;
#16768=CARTESIAN_POINT('Ctrl Pts',(-18.1811536522131,12.9394970608809,123.178952287643)) ;
#16769=CARTESIAN_POINT('Ctrl Pts',(-18.1811323254288,12.9394918032316,123.179064794358)) ;
#16770=CARTESIAN_POINT('Ctrl Pts',(-18.181121944146,12.9394892430643,123.179119579517)) ;
#16771=CARTESIAN_POINT('Ctrl Pts',(-18.1810892024377,12.939481165697,123.17929243061)) ;
#16772=CARTESIAN_POINT('Ctrl Pts',(-18.1810668553675,12.9394756485441,123.179410499093)) ;
#16773=CARTESIAN_POINT('Ctrl Pts',(-18.181022666351,12.9394647307492,123.179644151669)) ;
#16774=CARTESIAN_POINT('Ctrl Pts',(-18.181000823699,12.9394593301059,123.179759735601)) ;
#16775=CARTESIAN_POINT('Ctrl Pts',(-18.1809576226227,12.9394486406781,123.179988518082)) ;
#16776=CARTESIAN_POINT('Ctrl Pts',(-18.1809362635275,12.9394433518906,123.180101716519)) ;
#16777=CARTESIAN_POINT('Ctrl Pts',(-18.1808940096477,12.9394328817271,123.180325822676)) ;
#16778=CARTESIAN_POINT('Ctrl Pts',(-18.1808731141226,12.9394277003212,123.180436730871)) ;
#16779=CARTESIAN_POINT('Ctrl Pts',(-18.1794581206302,12.9390765796052,123.187952755114)) ;
#16780=CARTESIAN_POINT('Ctrl Pts',(-18.1781309923844,12.9387308918906,123.195370336562)) ;
#16781=CARTESIAN_POINT('Ctrl Pts',(-18.1757657578108,12.9380826164572,123.209316318956)) ;
#16782=CARTESIAN_POINT('Ctrl Pts',(-18.1747122112557,12.9377799831221,123.21584182609)) ;
#16783=CARTESIAN_POINT('Ctrl Pts',(-18.1717069603954,12.9368728810166,123.235442720272)) ;
#16784=CARTESIAN_POINT('Ctrl Pts',(-18.1699108725588,12.9362692023525,123.248541032574)) ;
#16785=CARTESIAN_POINT('Ctrl Pts',(-18.1649658156275,12.9343905396532,123.289410877513)) ;
#16786=CARTESIAN_POINT('Ctrl Pts',(-18.1625402001211,12.9331172882892,123.317261138592)) ;
#16787=CARTESIAN_POINT('Ctrl Pts',(-18.1603588706949,12.9312498209466,123.358116088442)) ;
#16788=CARTESIAN_POINT('Ctrl Pts',(-18.1598690864403,12.930657652216,123.37107289146)) ;
#16789=CARTESIAN_POINT('Ctrl Pts',(-18.1593242379878,12.9295366741171,123.395583561866)) ;
#16790=CARTESIAN_POINT('Ctrl Pts',(-18.1592276205016,12.9290080527271,123.40713516286)) ;
#16791=CARTESIAN_POINT('Ctrl Pts',(-18.1593138238008,12.9282897303717,123.422814981604)) ;
#16792=CARTESIAN_POINT('Ctrl Pts',(-18.1593569757214,12.92810052608,123.426943405856)) ;
#16793=CARTESIAN_POINT('Ctrl Pts',(-18.1595960598034,12.9273890608911,123.442460723563)) ;
#16794=CARTESIAN_POINT('Ctrl Pts',(-18.159927205597,12.9268663684156,123.453846955133)) ;
#16795=CARTESIAN_POINT('Ctrl Pts',(-18.161235129003,12.9254604078605,123.48442791674)) ;
#16796=CARTESIAN_POINT('Ctrl Pts',(-18.1624990362419,12.9245763576782,123.503607245375)) ;
#16797=CARTESIAN_POINT('Ctrl Pts',(-18.1664096371934,12.9225474469302,123.547497327835)) ;
#16798=CARTESIAN_POINT('Ctrl Pts',(-18.1693519972108,12.9214024106477,123.572173672582)) ;
#16799=CARTESIAN_POINT('Ctrl Pts',(-18.1739785388711,12.9199629074833,123.603101533229)) ;
#16800=CARTESIAN_POINT('Ctrl Pts',(-18.1749782874093,12.9196672107574,123.60944975546)) ;
#16801=CARTESIAN_POINT('Ctrl Pts',(-18.1774139353592,12.9189808291118,123.624175786378)) ;
#16802=CARTESIAN_POINT('Ctrl Pts',(-18.1788864237521,12.9185902941876,123.632547234821)) ;
#16803=CARTESIAN_POINT('Ctrl Pts',(-18.1804477772138,12.9181993395347,123.640922310696)) ;
#16804=CARTESIAN_POINT('Ctrl Pts',(-18.1804513722318,12.9181984394775,123.640941591798)) ;
#16805=CARTESIAN_POINT('Ctrl Pts',(-18.1804585570762,12.918196640895,123.640980121126)) ;
#16806=CARTESIAN_POINT('Ctrl Pts',(-18.1804621468857,12.9181957423737,123.640999369269)) ;
#16807=CARTESIAN_POINT('Ctrl Pts',(-18.1804693213972,12.9181939468408,123.641037833157)) ;
#16808=CARTESIAN_POINT('Ctrl Pts',(-18.1804729061151,12.9181930498249,123.641057048993)) ;
#16809=CARTESIAN_POINT('Ctrl Pts',(-18.1804800705661,12.9181912572712,123.64109544895)) ;
#16810=CARTESIAN_POINT('Ctrl Pts',(-18.1804836502603,12.9181903617427,123.641114632869)) ;
#16811=CARTESIAN_POINT('Ctrl Pts',(-18.1804908047521,12.9181885721404,123.641152969487)) ;
#16812=CARTESIAN_POINT('Ctrl Pts',(-18.1804943795522,12.9181876780656,123.641172122208)) ;
#16813=CARTESIAN_POINT('Ctrl Pts',(-18.1805015243192,12.9181858913539,123.641210396793)) ;
#16814=CARTESIAN_POINT('Ctrl Pts',(-18.1805050943191,12.9181849987084,123.641229518842)) ;
#16815=CARTESIAN_POINT('Ctrl Pts',(-18.1805122296001,12.9181832148254,123.64126773272)) ;
#16816=CARTESIAN_POINT('Ctrl Pts',(-18.1805157948734,12.9181823235896,123.641286824515)) ;
#16817=CARTESIAN_POINT('Ctrl Pts',(-18.1805229208078,12.9181805424983,123.641324978479)) ;
#16818=CARTESIAN_POINT('Ctrl Pts',(-18.1805264814681,12.9181796526427,123.641344040652)) ;
#16819=CARTESIAN_POINT('Ctrl Pts',(-18.1805335982779,12.9181778742855,123.641382135936)) ;
#16820=CARTESIAN_POINT('Ctrl Pts',(-18.180537154418,12.918176985786,123.641401169006)) ;
#16821=CARTESIAN_POINT('Ctrl Pts',(-18.1805442622957,12.9181752101128,123.641439206686)) ;
#16822=CARTESIAN_POINT('Ctrl Pts',(-18.1805478140121,12.9181743229441,123.641458211191)) ;
#16823=CARTESIAN_POINT('Ctrl Pts',(-18.1805549131316,12.9181725499094,123.641496192242)) ;
#16824=CARTESIAN_POINT('Ctrl Pts',(-18.1805584605333,12.9181716640434,123.641515168787)) ;
#16825=CARTESIAN_POINT('Ctrl Pts',(-18.1805655510948,12.9181698935952,123.641553094322)) ;
#16826=CARTESIAN_POINT('Ctrl Pts',(-18.1805690942831,12.9181690090056,123.641572043471)) ;
#16827=CARTESIAN_POINT('Ctrl Pts',(-18.1805761765045,12.9181672410876,123.641609914697)) ;
#16828=CARTESIAN_POINT('Ctrl Pts',(-18.1805797155685,12.9181663577511,123.641628836947)) ;
#16829=CARTESIAN_POINT('Ctrl Pts',(-18.1805867897101,12.9181645922965,123.641666655297)) ;
#16830=CARTESIAN_POINT('Ctrl Pts',(-18.1805903247121,12.9181637101967,123.641685551001)) ;
#16831=CARTESIAN_POINT('Ctrl Pts',(-18.1805973908086,12.9181619471949,123.641723316701)) ;
#16832=CARTESIAN_POINT('Ctrl Pts',(-18.1806009219106,12.9181610662905,123.641742186745)) ;
#16833=CARTESIAN_POINT('Ctrl Pts',(-18.1806079802736,12.9181593056619,123.641779901501)) ;
#16834=CARTESIAN_POINT('Ctrl Pts',(-18.180611507549,12.9181584259337,123.641798746296)) ;
#16835=CARTESIAN_POINT('Ctrl Pts',(-18.180618558347,12.9181566676345,123.641836411045)) ;
#16836=CARTESIAN_POINT('Ctrl Pts',(-18.1806220818969,12.9181557890565,123.641855231151)) ;
#16837=CARTESIAN_POINT('Ctrl Pts',(-18.1806291253781,12.9181540330231,123.641892847257)) ;
#16838=CARTESIAN_POINT('Ctrl Pts',(-18.1806326452775,12.9181531555755,123.641911643092)) ;
#16839=CARTESIAN_POINT('Ctrl Pts',(-18.1809539616441,12.9180730672334,123.643627215908)) ;
#16840=CARTESIAN_POINT('Ctrl Pts',(-18.1812752722338,12.9179938774841,123.645323332608)) ;
#16841=CARTESIAN_POINT('Ctrl Pts',(-18.1816065659832,12.9179131305516,123.647052552315)) ;
#16842=CARTESIAN_POINT('Ctrl Pts',(-18.1816130377265,12.9179115535273,123.647086324663)) ;
#16843=CARTESIAN_POINT('Ctrl Pts',(-18.182969480035,12.9175810906054,123.654163245793)) ;
#16844=CARTESIAN_POINT('Ctrl Pts',(-18.1843800374522,12.9172525519745,123.661194660238)) ;
#16845=CARTESIAN_POINT('Ctrl Pts',(-18.1890235626927,12.9162161904394,123.683351466648)) ;
#16846=CARTESIAN_POINT('Ctrl Pts',(-18.1924767942197,12.9155093084493,123.698429223739)) ;
#16847=CARTESIAN_POINT('Ctrl Pts',(-18.2018417324611,12.9137361373218,123.736092797363)) ;
#16848=CARTESIAN_POINT('Ctrl Pts',(-18.2081079994041,12.9126704373141,123.758584315276)) ;
#16849=CARTESIAN_POINT('Ctrl Pts',(-18.2189372055151,12.9109937672517,123.793626229474)) ;
#16850=CARTESIAN_POINT('Ctrl Pts',(-18.2230776127245,12.9103838947887,123.806301499499)) ;
#16851=CARTESIAN_POINT('Ctrl Pts',(-18.2316673068012,12.9091763649064,123.831238630323)) ;
#16852=CARTESIAN_POINT('Ctrl Pts',(-18.2361073175613,12.9085788070171,123.843501933227)) ;
#16853=CARTESIAN_POINT('Ctrl Pts',(-18.2452420675944,12.9073990018184,123.867549616553)) ;
#16854=CARTESIAN_POINT('Ctrl Pts',(-18.2499259084114,12.9068168544759,123.879336497236)) ;
#16855=CARTESIAN_POINT('Ctrl Pts',(-18.2620303679774,12.9053665360661,123.908496272049)) ;
#16856=CARTESIAN_POINT('Ctrl Pts',(-18.2696669653528,12.9044979794044,123.925776081124)) ;
#16857=CARTESIAN_POINT('Ctrl Pts',(-18.2788860231544,12.903499878364,123.945419938184)) ;
#16858=CARTESIAN_POINT('Ctrl Pts',(-18.2800884222473,12.9033706262114,123.947959692957)) ;
#16859=CARTESIAN_POINT('Ctrl Pts',(-18.2851283176188,12.9028326886442,123.958512998435)) ;
#16860=CARTESIAN_POINT('Ctrl Pts',(-18.2890426365442,12.9024240169746,123.966489575971)) ;
#16861=CARTESIAN_POINT('Ctrl Pts',(-18.2994759865159,12.9013581159805,123.987189593902)) ;
#16862=CARTESIAN_POINT('Ctrl Pts',(-18.3061288452239,12.900701145255,123.999844152114)) ;
#16863=CARTESIAN_POINT('Ctrl Pts',(-18.3162308743147,12.8997362908999,124.018284380569)) ;
#16864=CARTESIAN_POINT('Ctrl Pts',(-18.3195120663737,12.8994276798789,124.024160730369)) ;
#16865=CARTESIAN_POINT('Ctrl Pts',(-18.3228570573256,12.899117844315,124.030039293946)) ;
#16866=CARTESIAN_POINT('Ctrl Pts',(-18.3228735541318,12.8991163163849,124.030068283111)) ;
#16867=CARTESIAN_POINT('Ctrl Pts',(-18.32290637926,12.8991132763587,124.03012596)) ;
#16868=CARTESIAN_POINT('Ctrl Pts',(-18.3229227074044,12.8991117642766,124.030154647467)) ;
#16869=CARTESIAN_POINT('Ctrl Pts',(-18.3229551986617,12.8991087556196,124.030211727194)) ;
#16870=CARTESIAN_POINT('Ctrl Pts',(-18.3229713620229,12.8991072590194,124.030240119942)) ;
#16871=CARTESIAN_POINT('Ctrl Pts',(-18.3230035273146,12.8991042809858,124.030296616717)) ;
#16872=CARTESIAN_POINT('Ctrl Pts',(-18.323019529296,12.8991027995455,124.030324720885)) ;
#16873=CARTESIAN_POINT('Ctrl Pts',(-18.323051375567,12.8990998514791,124.030380647219)) ;
#16874=CARTESIAN_POINT('Ctrl Pts',(-18.3230672196567,12.8990983848692,124.030408469085)) ;
#16875=CARTESIAN_POINT('Ctrl Pts',(-18.3230987535156,12.8990954661453,124.030463836887)) ;
#16876=CARTESIAN_POINT('Ctrl Pts',(-18.323114443261,12.8990940140312,124.030491382829)) ;
#16877=CARTESIAN_POINT('Ctrl Pts',(-18.3231456716406,12.8990911239955,124.030546204565)) ;
#16878=CARTESIAN_POINT('Ctrl Pts',(-18.3231612103119,12.8990896860685,124.03057348047)) ;
#16879=CARTESIAN_POINT('Ctrl Pts',(-18.3231921396949,12.899086824109,124.030627767804)) ;
#16880=CARTESIAN_POINT('Ctrl Pts',(-18.3232075305103,12.8990854000651,124.03065477946)) ;
#16881=CARTESIAN_POINT('Ctrl Pts',(-18.3245493294304,12.8989612580724,124.033009499938)) ;
#16882=CARTESIAN_POINT('Ctrl Pts',(-18.3258832176993,12.8988385899037,124.035332941119)) ;
#16883=CARTESIAN_POINT('Ctrl Pts',(-18.3298950327256,12.8984718678071,124.042269204339)) ;
#16884=CARTESIAN_POINT('Ctrl Pts',(-18.3325950296598,12.8982279842675,124.046869201278)) ;
#16885=CARTESIAN_POINT('Ctrl Pts',(-18.3388262284224,12.8976717668316,124.057331350921)) ;
#16886=CARTESIAN_POINT('Ctrl Pts',(-18.3423762941214,12.8973595810617,124.063182067527)) ;
#16887=CARTESIAN_POINT('Ctrl Pts',(-18.354025380079,12.8963497021812,124.08202969001)) ;
#16888=CARTESIAN_POINT('Ctrl Pts',(-18.3623152447091,12.8956531781392,124.094907015862)) ;
#16889=CARTESIAN_POINT('Ctrl Pts',(-18.3914065642736,12.8932768979946,124.138322865386)) ;
#16890=CARTESIAN_POINT('Ctrl Pts',(-18.4133241694576,12.8915987489053,124.168089815719)) ;
#16891=CARTESIAN_POINT('Ctrl Pts',(-18.4418758265974,12.8895228903143,124.203468773847)) ;
#16892=CARTESIAN_POINT('Ctrl Pts',(-18.4472912978354,12.8891336910807,124.210040642423)) ;
#16893=CARTESIAN_POINT('Ctrl Pts',(-18.4572290045737,12.8884273879469,124.221852379309)) ;
#16894=CARTESIAN_POINT('Ctrl Pts',(-18.4617284192692,12.8881104450006,124.227111006818)) ;
#16895=CARTESIAN_POINT('Ctrl Pts',(-18.4666832069913,12.887764441578,124.232805424004)) ;
#16896=CARTESIAN_POINT('Ctrl Pts',(-18.467095506948,12.8877356723225,124.233278550346)) ;
#16897=CARTESIAN_POINT('Ctrl Pts',(-18.4675648714596,12.8877029468146,124.233816341727)) ;
#16898=CARTESIAN_POINT('Ctrl Pts',(-18.4676215866458,12.8876989928851,124.233881311632)) ;
#16899=CARTESIAN_POINT('Ctrl Pts',(-18.4677318916404,12.8876913037381,124.234007644781)) ;
#16900=CARTESIAN_POINT('Ctrl Pts',(-18.4677854810087,12.8876875685056,124.234069008982)) ;
#16901=CARTESIAN_POINT('Ctrl Pts',(-18.4678889337335,12.8876803584776,124.234187447423)) ;
#16902=CARTESIAN_POINT('Ctrl Pts',(-18.4679387961866,12.887676883694,124.234244522259)) ;
#16903=CARTESIAN_POINT('Ctrl Pts',(-18.4680349418722,12.8876701841842,124.234354554794)) ;
#16904=CARTESIAN_POINT('Ctrl Pts',(-18.4680812244232,12.8876669594601,124.234407513167)) ;
#16905=CARTESIAN_POINT('Ctrl Pts',(-18.4681703672058,12.8876607490035,124.234509496583)) ;
#16906=CARTESIAN_POINT('Ctrl Pts',(-18.4682132266936,12.8876577632826,124.234558522063)) ;
#16907=CARTESIAN_POINT('Ctrl Pts',(-18.468295687275,12.8876520192948,124.234652830986)) ;
#16908=CARTESIAN_POINT('Ctrl Pts',(-18.4683352878139,12.8876492610311,124.234698114928)) ;
#16909=CARTESIAN_POINT('Ctrl Pts',(-18.468411399551,12.8876439600789,124.234785137415)) ;
#16910=CARTESIAN_POINT('Ctrl Pts',(-18.4684479103416,12.8876414173877,124.234826876486)) ;
#16911=CARTESIAN_POINT('Ctrl Pts',(-18.4685180147853,12.8876365354972,124.234907009001)) ;
#16912=CARTESIAN_POINT('Ctrl Pts',(-18.4685516080128,12.8876341963005,124.234945402819)) ;
#16913=CARTESIAN_POINT('Ctrl Pts',(-18.4686160507956,12.8876297092412,124.235019045605)) ;
#16914=CARTESIAN_POINT('Ctrl Pts',(-18.4686468998015,12.8876275613936,124.235054294689)) ;
#16915=CARTESIAN_POINT('Ctrl Pts',(-18.4687060259814,12.8876234450001,124.235121846536)) ;
#16916=CARTESIAN_POINT('Ctrl Pts',(-18.4687343029867,12.8876214764459,124.235154149746)) ;
#16917=CARTESIAN_POINT('Ctrl Pts',(-18.468790884058,12.8876175376635,124.235218780361)) ;
#16918=CARTESIAN_POINT('Ctrl Pts',(-18.4688191884352,12.8876155674136,124.235251108115)) ;
#16919=CARTESIAN_POINT('Ctrl Pts',(-18.4688752008435,12.8876116686328,124.235315075854)) ;
#16920=CARTESIAN_POINT('Ctrl Pts',(-18.4689029109598,12.8876097399525,124.235346718361)) ;
#16921=CARTESIAN_POINT('Ctrl Pts',(-18.4689577443706,12.8876059236345,124.2354093269)) ;
#16922=CARTESIAN_POINT('Ctrl Pts',(-18.4689848653394,12.8876040361545,124.235440290412)) ;
#16923=CARTESIAN_POINT('Ctrl Pts',(-18.4690385145869,12.8876003026333,124.23550153467)) ;
#16924=CARTESIAN_POINT('Ctrl Pts',(-18.4690650454101,12.8875984564108,124.235531818454)) ;
#16925=CARTESIAN_POINT('Ctrl Pts',(-18.4691175258074,12.8875948045957,124.235591716712)) ;
#16926=CARTESIAN_POINT('Ctrl Pts',(-18.4691434722948,12.8875929992139,124.235621327792)) ;
#16927=CARTESIAN_POINT('Ctrl Pts',(-18.4699224641026,12.8875387988499,124.236510257003)) ;
#16928=CARTESIAN_POINT('Ctrl Pts',(-18.4706766859725,12.8874863960561,124.237368543549)) ;
#16929=CARTESIAN_POINT('Ctrl Pts',(-18.4757060554748,12.8871374506776,124.243076045287)) ;
#16930=CARTESIAN_POINT('Ctrl Pts',(-18.4800175818452,12.8868406696014,124.247893058657)) ;
#16931=CARTESIAN_POINT('Ctrl Pts',(-18.4898500289464,12.8861690840557,124.258708256137)) ;
#16932=CARTESIAN_POINT('Ctrl Pts',(-18.4953926474036,12.8857941488287,124.264686310065)) ;
#16933=CARTESIAN_POINT('Ctrl Pts',(-18.5101231320875,12.8848070781492,124.280265561429)) ;
#16934=CARTESIAN_POINT('Ctrl Pts',(-18.5194062998423,12.8841944007577,124.289775187233)) ;
#16935=CARTESIAN_POINT('Ctrl Pts',(-18.5550983049626,12.8818736011182,124.32519014002)) ;
#16936=CARTESIAN_POINT('Ctrl Pts',(-18.5825009328651,12.880161273313,124.350066794169)) ;
#16937=CARTESIAN_POINT('Ctrl Pts',(-18.6212524488809,12.8778392074262,124.382228452977)) ;
#16938=CARTESIAN_POINT('Ctrl Pts',(-18.6316748627251,12.877224095369,124.390599843998)) ;
#16939=CARTESIAN_POINT('Ctrl Pts',(-18.6524795894873,12.8760131830291,124.406768339183)) ;
#16940=CARTESIAN_POINT('Ctrl Pts',(-18.6628530867348,12.8754173924744,124.414574044891)) ;
#16941=CARTESIAN_POINT('Ctrl Pts',(-18.7467658024364,12.8706560174457,124.475691817207)) ;
#16942=CARTESIAN_POINT('Ctrl Pts',(-18.8257959080712,12.866506260928,124.521005702758)) ;
#16943=CARTESIAN_POINT('Ctrl Pts',(-18.9215326984024,12.8617196442192,124.562812243808)) ;
#16944=CARTESIAN_POINT('Ctrl Pts',(-18.9341186520534,12.8610952313076,124.56806479059)) ;
#16945=CARTESIAN_POINT('Ctrl Pts',(-18.9585064594863,12.8598946991652,124.577777194201)) ;
#16946=CARTESIAN_POINT('Ctrl Pts',(-18.9702948770285,12.8593185422153,124.582266407866)) ;
#16947=CARTESIAN_POINT('Ctrl Pts',(-18.9933300089094,12.8582009555687,124.590641579749)) ;
#16948=CARTESIAN_POINT('Ctrl Pts',(-19.0045682200008,12.8576596143712,124.594546878756)) ;
#16949=CARTESIAN_POINT('Ctrl Pts',(-19.0547419910352,12.8552571323346,124.611183486482)) ;
#16950=CARTESIAN_POINT('Ctrl Pts',(-19.0942336129539,12.8534025960457,124.622156733051)) ;
#16951=CARTESIAN_POINT('Ctrl Pts',(-19.147482036072,12.8509166562023,124.634169261791)) ;
#16952=CARTESIAN_POINT('Ctrl Pts',(-19.1608195927546,12.8502952981591,124.636949820319)) ;
#16953=CARTESIAN_POINT('Ctrl Pts',(-19.1812816780191,12.8493431719853,124.640867781224)) ;
#16954=CARTESIAN_POINT('Ctrl Pts',(-19.1883750582263,12.8490133199613,124.642162458373)) ;
#16955=CARTESIAN_POINT('Ctrl Pts',(-19.1993763911068,12.8485019728867,124.644072204825)) ;
#16956=CARTESIAN_POINT('Ctrl Pts',(-19.203276739423,12.8483207277948,124.644730219724)) ;
#16957=CARTESIAN_POINT('Ctrl Pts',(-19.2073727034653,12.848130430802,124.645401257275)) ;
#16958=CARTESIAN_POINT('Ctrl Pts',(-19.2075652738395,12.8481214841415,124.64543275958)) ;
#16959=CARTESIAN_POINT('Ctrl Pts',(-19.2078963833416,12.8481061012184,124.645486845695)) ;
#16960=CARTESIAN_POINT('Ctrl Pts',(-19.2080349189704,12.848099665076,124.645509451272)) ;
#16961=CARTESIAN_POINT('Ctrl Pts',(-19.2082911550508,12.8480877608434,124.645551218334)) ;
#16962=CARTESIAN_POINT('Ctrl Pts',(-19.2084088545248,12.8480822927861,124.645570386326)) ;
#16963=CARTESIAN_POINT('Ctrl Pts',(-19.2086254579747,12.8480722299281,124.645605629543)) ;
#16964=CARTESIAN_POINT('Ctrl Pts',(-19.2087243611196,12.8480676351566,124.645621709716)) ;
#16965=CARTESIAN_POINT('Ctrl Pts',(-19.2089055418012,12.8480592180358,124.645651144626)) ;
#16966=CARTESIAN_POINT('Ctrl Pts',(-19.2089878186411,12.8480553957119,124.645664503009)) ;
#16967=CARTESIAN_POINT('Ctrl Pts',(-19.2091379278608,12.8480484221368,124.645688859178)) ;
#16968=CARTESIAN_POINT('Ctrl Pts',(-19.2092057599288,12.8480452708951,124.645699859618)) ;
#16969=CARTESIAN_POINT('Ctrl Pts',(-19.2093290753509,12.8480395421093,124.645719847451)) ;
#16970=CARTESIAN_POINT('Ctrl Pts',(-19.2093845585461,12.848036964569,124.645728836718)) ;
#16971=CARTESIAN_POINT('Ctrl Pts',(-19.209510775576,12.8480311010172,124.645749277391)) ;
#16972=CARTESIAN_POINT('Ctrl Pts',(-19.2095815099182,12.8480278149865,124.645760726479)) ;
#16973=CARTESIAN_POINT('Ctrl Pts',(-19.2097196683629,12.8480213967277,124.645783076665)) ;
#16974=CARTESIAN_POINT('Ctrl Pts',(-19.2097870922423,12.848018264509,124.6457939783)) ;
#16975=CARTESIAN_POINT('Ctrl Pts',(-19.2099186765971,12.8480121516952,124.645815242849)) ;
#16976=CARTESIAN_POINT('Ctrl Pts',(-19.2099828370863,12.8480091710985,124.645825606302)) ;
#16977=CARTESIAN_POINT('Ctrl Pts',(-19.2101079518054,12.8480033588711,124.645845805308)) ;
#16978=CARTESIAN_POINT('Ctrl Pts',(-19.2101689056141,12.8480005272591,124.645855641294)) ;
#16979=CARTESIAN_POINT('Ctrl Pts',(-19.2102876702736,12.8479950100576,124.645874797064)) ;
#16980=CARTESIAN_POINT('Ctrl Pts',(-19.2103454815312,12.8479923244485,124.645884117381)) ;
#16981=CARTESIAN_POINT('Ctrl Pts',(-19.2161162292188,12.8477242463938,124.64681405981)) ;
#16982=CARTESIAN_POINT('Ctrl Pts',(-19.2218354778886,12.8474586336503,124.647695002688)) ;
#16983=CARTESIAN_POINT('Ctrl Pts',(-19.2345582346726,12.8468678811711,124.649564358063)) ;
#16984=CARTESIAN_POINT('Ctrl Pts',(-19.2415644276858,12.8465426422506,124.650533105558)) ;
#16985=CARTESIAN_POINT('Ctrl Pts',(-19.259456908882,12.845712178287,124.652852519616)) ;
#16986=CARTESIAN_POINT('Ctrl Pts',(-19.2703534272261,12.8452065484907,124.654119438914)) ;
#16987=CARTESIAN_POINT('Ctrl Pts',(-19.3050349554443,12.8435975211568,124.657689793635)) ;
#16988=CARTESIAN_POINT('Ctrl Pts',(-19.3288699377701,12.8424920380273,124.659454720743)) ;
#16989=CARTESIAN_POINT('Ctrl Pts',(-19.3745494290596,12.8403758739273,124.661522700791)) ;
#16990=CARTESIAN_POINT('Ctrl Pts',(-19.3963803122365,12.8393656325211,124.661938519652)) ;
#16991=CARTESIAN_POINT('Ctrl Pts',(-19.432945950675,12.837678722305,124.66167703405)) ;
#16992=CARTESIAN_POINT('Ctrl Pts',(-19.4476780266782,12.837000512866,124.661311117628)) ;
#16993=CARTESIAN_POINT('Ctrl Pts',(-19.477091111899,12.8356472640861,124.660059860304)) ;
#16994=CARTESIAN_POINT('Ctrl Pts',(-19.4917698531057,12.8349723267023,124.659175724632)) ;
#16995=CARTESIAN_POINT('Ctrl Pts',(-19.5267989942869,12.8333605140487,124.656444791742)) ;
#16996=CARTESIAN_POINT('Ctrl Pts',(-19.5471264172699,12.8324242243262,124.654357589391)) ;
#16997=CARTESIAN_POINT('Ctrl Pts',(-19.6182032101922,12.8291402385589,124.645293775542)) ;
#16998=CARTESIAN_POINT('Ctrl Pts',(-19.6685666298544,12.8267934440379,124.635697538319)) ;
#16999=CARTESIAN_POINT('Ctrl Pts',(-19.7237530651233,12.824182748023,124.62162206394)) ;
#17000=CARTESIAN_POINT('Ctrl Pts',(-19.729297502019,12.8239200336279,124.620167247834)) ;
#17001=CARTESIAN_POINT('Ctrl Pts',(-19.7453102774323,12.8231600512955,124.615847681961)) ;
#17002=CARTESIAN_POINT('Ctrl Pts',(-19.7557515722823,12.8226629523962,124.612884664246)) ;
#17003=CARTESIAN_POINT('Ctrl Pts',(-19.7776792348842,12.8216157457921,124.606352322668)) ;
#17004=CARTESIAN_POINT('Ctrl Pts',(-19.7891553756961,12.8210657723521,124.60275241991)) ;
#17005=CARTESIAN_POINT('Ctrl Pts',(-19.8160271673877,12.8197736585971,124.593895176047)) ;
#17006=CARTESIAN_POINT('Ctrl Pts',(-19.831375760289,12.8190322555227,124.588501766008)) ;
#17007=CARTESIAN_POINT('Ctrl Pts',(-19.8892021343457,12.8162272661075,124.566904820949)) ;
#17008=CARTESIAN_POINT('Ctrl Pts',(-19.930890129217,12.8141775002152,124.548687916848)) ;
#17009=CARTESIAN_POINT('Ctrl Pts',(-19.9862120828362,12.8113637638717,124.520828344151)) ;
#17010=CARTESIAN_POINT('Ctrl Pts',(-20.0007829108018,12.8106136312639,124.513125723737)) ;
#17011=CARTESIAN_POINT('Ctrl Pts',(-20.0206311839269,12.8095776576652,124.502125714621)) ;
#17012=CARTESIAN_POINT('Ctrl Pts',(-20.0260427212809,12.8092937326215,124.499073658109)) ;
#17013=CARTESIAN_POINT('Ctrl Pts',(-20.035858034968,12.8087759827119,124.493441051767)) ;
#17014=CARTESIAN_POINT('Ctrl Pts',(-20.0402691930536,12.8085422657929,124.490873627959)) ;
#17015=CARTESIAN_POINT('Ctrl Pts',(-20.0485942994345,12.8080991758376,124.485959665455)) ;
#17016=CARTESIAN_POINT('Ctrl Pts',(-20.052511365692,12.8078898494702,124.483618567812)) ;
#17017=CARTESIAN_POINT('Ctrl Pts',(-20.0608231855,12.8074438352094,124.478588898318)) ;
#17018=CARTESIAN_POINT('Ctrl Pts',(-20.0652143134094,12.8072071044632,124.475894500893)) ;
#17019=CARTESIAN_POINT('Ctrl Pts',(-20.0756650115014,12.8066410225639,124.469392676705)) ;
#17020=CARTESIAN_POINT('Ctrl Pts',(-20.0817087801683,12.8063114827346,124.465560212044)) ;
#17021=CARTESIAN_POINT('Ctrl Pts',(-20.0981953601386,12.8054065086142,124.45490616916)) ;
#17022=CARTESIAN_POINT('Ctrl Pts',(-20.108569470628,12.8048303290835,124.447979872099)) ;
#17023=CARTESIAN_POINT('Ctrl Pts',(-20.1460575515924,12.8027234604015,124.422131413952)) ;
#17024=CARTESIAN_POINT('Ctrl Pts',(-20.1725215412225,12.8011874577774,124.40229082695)) ;
#17025=CARTESIAN_POINT('Ctrl Pts',(-20.2212601773955,12.7982733269864,124.362636042478)) ;
#17026=CARTESIAN_POINT('Ctrl Pts',(-20.2436741976618,12.7968980591233,124.343028447747)) ;
#17027=CARTESIAN_POINT('Ctrl Pts',(-20.278705135832,12.7946837528688,124.310102465427)) ;
#17028=CARTESIAN_POINT('Ctrl Pts',(-20.2917663602418,12.7938421796276,124.297274247366)) ;
#17029=CARTESIAN_POINT('Ctrl Pts',(-20.3177657482889,12.7921310504403,124.270591769246)) ;
#17030=CARTESIAN_POINT('Ctrl Pts',(-20.3306800159469,12.7912617719045,124.256720748975)) ;
#17031=CARTESIAN_POINT('Ctrl Pts',(-20.3630764839494,12.7890269111174,124.220297683454)) ;
#17032=CARTESIAN_POINT('Ctrl Pts',(-20.3820766671837,12.7876626907649,124.197332897656)) ;
#17033=CARTESIAN_POINT('Ctrl Pts',(-20.4182038309825,12.7849502876743,124.150343874601)) ;
#17034=CARTESIAN_POINT('Ctrl Pts',(-20.4353375002655,12.7836029411305,124.126348396332)) ;
#17035=CARTESIAN_POINT('Ctrl Pts',(-20.4697376095668,12.7807578157418,124.074379195959)) ;
#17036=CARTESIAN_POINT('Ctrl Pts',(-20.4867817015409,12.779262053449,124.046284493577)) ;
#17037=CARTESIAN_POINT('Ctrl Pts',(-20.5230877319292,12.7758603065869,123.980747753984)) ;
#17038=CARTESIAN_POINT('Ctrl Pts',(-20.541604763314,12.7739546870016,123.94293882141)) ;
#17039=CARTESIAN_POINT('Ctrl Pts',(-20.5621348410788,12.7715779299649,123.895041629938)) ;
#17040=CARTESIAN_POINT('Ctrl Pts',(-20.5659783913867,12.7711194890167,123.885767574364)) ;
#17041=CARTESIAN_POINT('Ctrl Pts',(-20.571910552757,12.7703895793769,123.870951817134)) ;
#17042=CARTESIAN_POINT('Ctrl Pts',(-20.5740722190011,12.7701185660944,123.865439821601)) ;
#17043=CARTESIAN_POINT('Ctrl Pts',(-20.5783397596512,12.7695731654723,123.854326437396)) ;
#17044=CARTESIAN_POINT('Ctrl Pts',(-20.5804447348212,12.7692987800961,123.848724867049)) ;
#17045=CARTESIAN_POINT('Ctrl Pts',(-20.5847002094871,12.7687327577329,123.837148817864)) ;
#17046=CARTESIAN_POINT('Ctrl Pts',(-20.5868455715947,12.7684410990576,123.831172632627)) ;
#17047=CARTESIAN_POINT('Ctrl Pts',(-20.5918500775142,12.7677453575245,123.816890662744)) ;
#17048=CARTESIAN_POINT('Ctrl Pts',(-20.5946673850309,12.7673410620299,123.808570585047)) ;
#17049=CARTESIAN_POINT('Ctrl Pts',(-20.6023936864466,12.7661953980693,123.784936087112)) ;
#17050=CARTESIAN_POINT('Ctrl Pts',(-20.6070951589504,12.7654531286899,123.76955569206)) ;
#17051=CARTESIAN_POINT('Ctrl Pts',(-20.6205219745194,12.7631875501231,123.722394515124)) ;
#17052=CARTESIAN_POINT('Ctrl Pts',(-20.6282885327783,12.7616623429431,123.690355627853)) ;
#17053=CARTESIAN_POINT('Ctrl Pts',(-20.6360870201024,12.7598387539018,123.651542354722)) ;
#17054=CARTESIAN_POINT('Ctrl Pts',(-20.6373422095278,12.7595334695377,123.645027066479)) ;
#17055=CARTESIAN_POINT('Ctrl Pts',(-20.6392240234138,12.7590567365784,123.634822439879)) ;
#17056=CARTESIAN_POINT('Ctrl Pts',(-20.639886053901,12.7588849807024,123.63113976734)) ;
#17057=CARTESIAN_POINT('Ctrl Pts',(-20.6409475265519,12.7586028129954,123.625078974985)) ;
#17058=CARTESIAN_POINT('Ctrl Pts',(-20.6413566394029,12.7584923035238,123.622702577425)) ;
#17059=CARTESIAN_POINT('Ctrl Pts',(-20.6423489989286,12.7582198229145,123.616836834334)) ;
#17060=CARTESIAN_POINT('Ctrl Pts',(-20.6429243141292,12.7580579273651,123.61334616499)) ;
#17061=CARTESIAN_POINT('Ctrl Pts',(-20.6450986418836,12.7574303499593,123.599795367796)) ;
#17062=CARTESIAN_POINT('Ctrl Pts',(-20.6465894837429,12.7569655719389,123.58971825148)) ;
#17063=CARTESIAN_POINT('Ctrl Pts',(-20.6520137578833,12.7551243987104,123.549679039718)) ;
#17064=CARTESIAN_POINT('Ctrl Pts',(-20.654983329489,12.7537530258065,123.519596740252)) ;
#17065=CARTESIAN_POINT('Ctrl Pts',(-20.6582655644916,12.7513491962733,123.466842689343)) ;
#17066=CARTESIAN_POINT('Ctrl Pts',(-20.6590572717309,12.750318552095,123.444215089052)) ;
#17067=CARTESIAN_POINT('Ctrl Pts',(-20.6592991453929,12.7489043762898,123.413251758331)) ;
#17068=CARTESIAN_POINT('Ctrl Pts',(-20.6592809837611,12.7485236808201,123.404924505231)) ;
#17069=CARTESIAN_POINT('Ctrl Pts',(-20.6591047730988,12.7478611164033,123.390450084068)) ;
#17070=CARTESIAN_POINT('Ctrl Pts',(-20.6589845682959,12.7475794597131,123.384302740036)) ;
#17071=CARTESIAN_POINT('Ctrl Pts',(-20.6586615394446,12.7470294081541,123.372310292645)) ;
#17072=CARTESIAN_POINT('Ctrl Pts',(-20.6584630376171,12.7467610437371,123.366465228349)) ;
#17073=CARTESIAN_POINT('Ctrl Pts',(-20.6579435639546,12.7461785126314,123.353791570327)) ;
#17074=CARTESIAN_POINT('Ctrl Pts',(-20.6576075802162,12.745864273721,123.346963783305)) ;
#17075=CARTESIAN_POINT('Ctrl Pts',(-20.6566344107474,12.7450833683746,123.330019855304)) ;
#17076=CARTESIAN_POINT('Ctrl Pts',(-20.6559301558479,12.7446163757512,123.319908072816)) ;
#17077=CARTESIAN_POINT('Ctrl Pts',(-20.6516201662555,12.7421801010544,123.267270058961)) ;
#17078=CARTESIAN_POINT('Ctrl Pts',(-20.6459611978017,12.7402017054295,123.224940545904)) ;
#17079=CARTESIAN_POINT('Ctrl Pts',(-20.6316045218902,12.7365752730097,123.14784170075)) ;
#17080=CARTESIAN_POINT('Ctrl Pts',(-20.6235562276742,12.7349267210823,123.112996372846)) ;
#17081=CARTESIAN_POINT('Ctrl Pts',(-20.6073664514362,12.7321292633185,123.054471273078)) ;
#17082=CARTESIAN_POINT('Ctrl Pts',(-20.5999902727943,12.73098059351,123.030613108942)) ;
#17083=CARTESIAN_POINT('Ctrl Pts',(-20.5919011387506,12.7298327524269,123.006982452872)) ;
#17084=CARTESIAN_POINT('Ctrl Pts',(-20.5919010929902,12.6697683433082,123.006982319192)) ;
#17085=CARTESIAN_POINT('Ctrl Pts',(-20.5960841911158,12.670359945217,123.019202331386)) ;
#17086=CARTESIAN_POINT('Ctrl Pts',(-20.6000745876603,12.670951590307,123.03147690456)) ;
#17087=CARTESIAN_POINT('Ctrl Pts',(-20.6095371759573,12.6724264498721,123.062194962408)) ;
#17088=CARTESIAN_POINT('Ctrl Pts',(-20.6147726348497,12.6733097112788,123.080697409861)) ;
#17089=CARTESIAN_POINT('Ctrl Pts',(-20.6262171461193,12.6754144557165,123.125021633689)) ;
#17090=CARTESIAN_POINT('Ctrl Pts',(-20.6320342620921,12.6766361409836,123.150935055497)) ;
#17091=CARTESIAN_POINT('Ctrl Pts',(-20.6383947320466,12.6781917078399,123.184193370554)) ;
#17092=CARTESIAN_POINT('Ctrl Pts',(-20.6397047453997,12.6785273148293,123.1913846312)) ;
#17093=CARTESIAN_POINT('Ctrl Pts',(-20.6419465529887,12.6791302266929,123.204334131621)) ;
#17094=CARTESIAN_POINT('Ctrl Pts',(-20.6429012601135,12.6793976240357,123.210088188933)) ;
#17095=CARTESIAN_POINT('Ctrl Pts',(-20.6448184532083,12.6799577788107,123.222166113018)) ;
#17096=CARTESIAN_POINT('Ctrl Pts',(-20.6457727400574,12.6802504575829,123.2284911037)) ;
#17097=CARTESIAN_POINT('Ctrl Pts',(-20.6509979349282,12.681937339407,123.265022233269)) ;
#17098=CARTESIAN_POINT('Ctrl Pts',(-20.6542104815208,12.6833254213589,123.295369434085)) ;
#17099=CARTESIAN_POINT('Ctrl Pts',(-20.6575714221632,12.6855504427503,123.344098551755)) ;
#17100=CARTESIAN_POINT('Ctrl Pts',(-20.6584304990138,12.6863860329828,123.362418808225)) ;
#17101=CARTESIAN_POINT('Ctrl Pts',(-20.6591438126329,12.6876960563132,123.391114177311)) ;
#17102=CARTESIAN_POINT('Ctrl Pts',(-20.6592724971882,12.6881695188179,123.401479855197)) ;
#17103=CARTESIAN_POINT('Ctrl Pts',(-20.6592720305176,12.6890150091815,123.419971766697)) ;
#17104=CARTESIAN_POINT('Ctrl Pts',(-20.6591925900471,12.6893868245354,123.428097411713)) ;
#17105=CARTESIAN_POINT('Ctrl Pts',(-20.6588800036677,12.6901199812654,123.444103201659)) ;
#17106=CARTESIAN_POINT('Ctrl Pts',(-20.6586515286575,12.6904812870742,123.451983067533)) ;
#17107=CARTESIAN_POINT('Ctrl Pts',(-20.6579463760958,12.6913228529623,123.47031532929)) ;
#17108=CARTESIAN_POINT('Ctrl Pts',(-20.657412968387,12.6918033144494,123.480764942856)) ;
#17109=CARTESIAN_POINT('Ctrl Pts',(-20.6545300396442,12.6938898653405,123.526063893808)) ;
#17110=CARTESIAN_POINT('Ctrl Pts',(-20.6508516386006,12.6955006384372,123.5608127491)) ;
#17111=CARTESIAN_POINT('Ctrl Pts',(-20.6434453671924,12.6978273649608,123.610704464615)) ;
#17112=CARTESIAN_POINT('Ctrl Pts',(-20.6408823918687,12.6985426801364,123.626003569198)) ;
#17113=CARTESIAN_POINT('Ctrl Pts',(-20.6360773279863,12.699748176064,123.65173740467)) ;
#17114=CARTESIAN_POINT('Ctrl Pts',(-20.6339851356085,12.7002387717928,123.662198297223)) ;
#17115=CARTESIAN_POINT('Ctrl Pts',(-20.6295931646807,12.7012055395411,123.682784116522)) ;
#17116=CARTESIAN_POINT('Ctrl Pts',(-20.6273006372482,12.7016817804223,123.692909704444)) ;
#17117=CARTESIAN_POINT('Ctrl Pts',(-20.6192555467027,12.7032649767667,123.72649482735)) ;
#17118=CARTESIAN_POINT('Ctrl Pts',(-20.6129492002108,12.7043702405481,123.74981610374)) ;
#17119=CARTESIAN_POINT('Ctrl Pts',(-20.5987616512748,12.7066181825287,123.796830832246)) ;
#17120=CARTESIAN_POINT('Ctrl Pts',(-20.5908383556585,12.7077603904967,123.820500370868)) ;
#17121=CARTESIAN_POINT('Ctrl Pts',(-20.5691859489112,12.7106306795419,123.879275708034)) ;
#17122=CARTESIAN_POINT('Ctrl Pts',(-20.554567805643,12.7123593141006,123.914027442314)) ;
#17123=CARTESIAN_POINT('Ctrl Pts',(-20.5312799784474,12.714851400869,123.963062274047)) ;
#17124=CARTESIAN_POINT('Ctrl Pts',(-20.5238595910577,12.7156134915765,123.977915645908)) ;
#17125=CARTESIAN_POINT('Ctrl Pts',(-20.5115265343122,12.7168310374864,124.001419561266)) ;
#17126=CARTESIAN_POINT('Ctrl Pts',(-20.5068026689408,12.7172867938634,124.010166915736)) ;
#17127=CARTESIAN_POINT('Ctrl Pts',(-20.4978981798395,12.7181267113076,124.026195377235)) ;
#17128=CARTESIAN_POINT('Ctrl Pts',(-20.4937475718544,12.7185109603369,124.033492513457)) ;
#17129=CARTESIAN_POINT('Ctrl Pts',(-20.484074561646,12.7193900331888,124.050106819316)) ;
#17130=CARTESIAN_POINT('Ctrl Pts',(-20.4785039340141,12.7198845012148,124.059395150944)) ;
#17131=CARTESIAN_POINT('Ctrl Pts',(-20.4577249953554,12.7216871083823,124.093042230999)) ;
#17132=CARTESIAN_POINT('Ctrl Pts',(-20.4417992473004,12.7229909559485,124.116947384176)) ;
#17133=CARTESIAN_POINT('Ctrl Pts',(-20.4153099550804,12.7250583774299,124.153884621786)) ;
#17134=CARTESIAN_POINT('Ctrl Pts',(-20.4052833669348,12.725820179281,124.167289038643)) ;
#17135=CARTESIAN_POINT('Ctrl Pts',(-20.3892704711107,12.7270075392837,124.187823378824)) ;
#17136=CARTESIAN_POINT('Ctrl Pts',(-20.3834685953634,12.7274320816729,124.195094636064)) ;
#17137=CARTESIAN_POINT('Ctrl Pts',(-20.3732279861567,12.728172005311,124.20763897346)) ;
#17138=CARTESIAN_POINT('Ctrl Pts',(-20.3688257917484,12.728487152105,124.212941364308)) ;
#17139=CARTESIAN_POINT('Ctrl Pts',(-20.3600054097702,12.7291129549736,124.223388402231)) ;
#17140=CARTESIAN_POINT('Ctrl Pts',(-20.3555887555784,12.7294235916436,124.228534041554)) ;
#17141=CARTESIAN_POINT('Ctrl Pts',(-20.3459834859214,12.7300934440423,124.239542172173)) ;
#17142=CARTESIAN_POINT('Ctrl Pts',(-20.3407812242484,12.7304527372553,124.245392371438)) ;
#17143=CARTESIAN_POINT('Ctrl Pts',(-20.3258658971748,12.7314731713045,124.2618513899)) ;
#17144=CARTESIAN_POINT('Ctrl Pts',(-20.3160242279232,12.7321350948293,124.272341939088)) ;
#17145=CARTESIAN_POINT('Ctrl Pts',(-20.2812999062747,12.734432249313,124.308098429861)) ;
#17146=CARTESIAN_POINT('Ctrl Pts',(-20.2555248551346,12.7360719711633,124.332473842558)) ;
#17147=CARTESIAN_POINT('Ctrl Pts',(-20.2211458861119,12.7381733695348,124.362320833883)) ;
#17148=CARTESIAN_POINT('Ctrl Pts',(-20.2134636698923,12.7386377109107,124.368829260275)) ;
#17149=CARTESIAN_POINT('Ctrl Pts',(-20.2015341545535,12.7393504866588,124.378690944663)) ;
#17150=CARTESIAN_POINT('Ctrl Pts',(-20.1973423201663,12.7395994024534,124.382110613887)) ;
#17151=CARTESIAN_POINT('Ctrl Pts',(-20.1890785660805,12.7400870287261,124.388763248654)) ;
#17152=CARTESIAN_POINT('Ctrl Pts',(-20.1850084127581,12.7403257569446,124.391998234485)) ;
#17153=CARTESIAN_POINT('Ctrl Pts',(-20.176100047614,12.7408452668696,124.398988421823)) ;
#17154=CARTESIAN_POINT('Ctrl Pts',(-20.1712541781852,12.7411259647486,124.402733650917)) ;
#17155=CARTESIAN_POINT('Ctrl Pts',(-20.1571358542692,12.7419385723428,124.413480481145)) ;
#17156=CARTESIAN_POINT('Ctrl Pts',(-20.1477930444285,12.7424698975658,124.420388614398)) ;
#17157=CARTESIAN_POINT('Ctrl Pts',(-20.1151790775322,12.7443047457421,124.443807399264)) ;
#17158=CARTESIAN_POINT('Ctrl Pts',(-20.0914398751812,12.7456060970084,124.459650900859)) ;
#17159=CARTESIAN_POINT('Ctrl Pts',(-20.0556172272129,12.7475308243228,124.481825141139)) ;
#17160=CARTESIAN_POINT('Ctrl Pts',(-20.0439390903719,12.7481523714528,124.488792958826)) ;
#17161=CARTESIAN_POINT('Ctrl Pts',(-20.0222919202932,12.7492947459734,124.501234460079)) ;
#17162=CARTESIAN_POINT('Ctrl Pts',(-20.0123573959929,12.7498153332996,124.506765307206)) ;
#17163=CARTESIAN_POINT('Ctrl Pts',(-19.9921044066942,12.7508697151045,124.517681491241)) ;
#17164=CARTESIAN_POINT('Ctrl Pts',(-19.9817834003166,12.7514034805954,124.523059795089)) ;
#17165=CARTESIAN_POINT('Ctrl Pts',(-19.9403110568032,12.7535349213214,124.54393998708)) ;
#17166=CARTESIAN_POINT('Ctrl Pts',(-19.9085936151727,12.7551357689768,124.558282332323)) ;
#17167=CARTESIAN_POINT('Ctrl Pts',(-19.8649452523373,12.7573006602749,124.575864393316)) ;
#17168=CARTESIAN_POINT('Ctrl Pts',(-19.8535042902745,12.7578646144217,124.580278420503)) ;
#17169=CARTESIAN_POINT('Ctrl Pts',(-19.8354973285712,12.7587465139232,124.586922964131)) ;
#17170=CARTESIAN_POINT('Ctrl Pts',(-19.8289745737445,12.7590648080492,124.589268396916)) ;
#17171=CARTESIAN_POINT('Ctrl Pts',(-19.8160890946309,12.7596912209761,124.593781041037)) ;
#17172=CARTESIAN_POINT('Ctrl Pts',(-19.8097277340896,12.7599993211959,124.59595142382)) ;
#17173=CARTESIAN_POINT('Ctrl Pts',(-19.7924203720171,12.7608346137997,124.601700968439)) ;
#17174=CARTESIAN_POINT('Ctrl Pts',(-19.7814419096567,12.761361320123,124.605180343383)) ;
#17175=CARTESIAN_POINT('Ctrl Pts',(-19.7415587011706,12.7632654326589,124.617216518696)) ;
#17176=CARTESIAN_POINT('Ctrl Pts',(-19.7123948864096,12.7646403719188,124.624878793787)) ;
#17177=CARTESIAN_POINT('Ctrl Pts',(-19.6690142600122,12.7666717374937,124.634614032808)) ;
#17178=CARTESIAN_POINT('Ctrl Pts',(-19.654993057669,12.767326163707,124.637508545113)) ;
#17179=CARTESIAN_POINT('Ctrl Pts',(-19.6289971539258,12.7685366841072,124.642411091961)) ;
#17180=CARTESIAN_POINT('Ctrl Pts',(-19.6170369337289,12.7690925279948,124.644486735641)) ;
#17181=CARTESIAN_POINT('Ctrl Pts',(-19.5938211084317,12.7701699042363,124.648168254323)) ;
#17182=CARTESIAN_POINT('Ctrl Pts',(-19.5825700660305,12.7706913232976,124.649795417854)) ;
#17183=CARTESIAN_POINT('Ctrl Pts',(-19.5340414165973,12.772938014668,124.656139266378)) ;
#17184=CARTESIAN_POINT('Ctrl Pts',(-19.4965838483847,12.7746668440938,124.659327280877)) ;
#17185=CARTESIAN_POINT('Ctrl Pts',(-19.4466341005257,12.7769666458711,124.661317563188)) ;
#17186=CARTESIAN_POINT('Ctrl Pts',(-19.4342216473971,12.7775376245486,124.661627022527)) ;
#17187=CARTESIAN_POINT('Ctrl Pts',(-19.4200629558388,12.7781881799603,124.661769006205)) ;
#17188=CARTESIAN_POINT('Ctrl Pts',(-19.4183192425384,12.7782682859684,124.661782843155)) ;
#17189=CARTESIAN_POINT('Ctrl Pts',(-19.4155790323222,12.7783941494927,124.661798853423)) ;
#17190=CARTESIAN_POINT('Ctrl Pts',(-19.4145825523688,12.7784399154207,124.66180348396)) ;
#17191=CARTESIAN_POINT('Ctrl Pts',(-19.4130294681036,12.7785112377391,124.661808843788)) ;
#17192=CARTESIAN_POINT('Ctrl Pts',(-19.4124728671917,12.7785367971106,124.661810392895)) ;
#17193=CARTESIAN_POINT('Ctrl Pts',(-19.4111369635157,12.7785981389672,124.661813218636)) ;
#17194=CARTESIAN_POINT('Ctrl Pts',(-19.4103576601202,12.7786339200973,124.661814138262)) ;
#17195=CARTESIAN_POINT('Ctrl Pts',(-19.4033948987358,12.7789535843599,124.661815843416)) ;
#17196=CARTESIAN_POINT('Ctrl Pts',(-19.3972115053518,12.7792372867439,124.661771475524)) ;
#17197=CARTESIAN_POINT('Ctrl Pts',(-19.3837819763669,12.7798529971387,124.661575452831)) ;
#17198=CARTESIAN_POINT('Ctrl Pts',(-19.3765363228649,12.7801848822632,124.661406654615)) ;
#17199=CARTESIAN_POINT('Ctrl Pts',(-19.3497108423677,12.7814129872106,124.660548235554)) ;
#17200=CARTESIAN_POINT('Ctrl Pts',(-19.3301465385876,12.7823074962193,124.659461337073)) ;
#17201=CARTESIAN_POINT('Ctrl Pts',(-19.2880638559818,12.784234764284,124.65612956335)) ;
#17202=CARTESIAN_POINT('Ctrl Pts',(-19.2655645192677,12.7852671702212,124.653732186074)) ;
#17203=CARTESIAN_POINT('Ctrl Pts',(-19.2311176840881,12.7868556544937,124.649113100317)) ;
#17204=CARTESIAN_POINT('Ctrl Pts',(-19.2191168125422,12.787410521221,124.64732564328)) ;
#17205=CARTESIAN_POINT('Ctrl Pts',(-19.1955740162531,12.7885025974153,124.643467940859)) ;
#17206=CARTESIAN_POINT('Ctrl Pts',(-19.1840314116677,12.7890397178046,124.641409432529)) ;
#17207=CARTESIAN_POINT('Ctrl Pts',(-19.1586869820179,12.7902233490391,124.636520653156)) ;
#17208=CARTESIAN_POINT('Ctrl Pts',(-19.1449005902117,12.790870004571,124.633618806386)) ;
#17209=CARTESIAN_POINT('Ctrl Pts',(-19.0983886574912,12.7930620641666,124.623004574635)) ;
#17210=CARTESIAN_POINT('Ctrl Pts',(-19.0659262492723,12.7946099096908,124.614205253279)) ;
#17211=CARTESIAN_POINT('Ctrl Pts',(-19.0237681370969,12.7966434077663,124.600931052706)) ;
#17212=CARTESIAN_POINT('Ctrl Pts',(-19.0137187708793,12.7971298798037,124.597626054994)) ;
#17213=CARTESIAN_POINT('Ctrl Pts',(-18.9976052074849,12.7979125334102,124.592099055018)) ;
#17214=CARTESIAN_POINT('Ctrl Pts',(-18.9915141721302,12.7982089905183,124.58995692521)) ;
#17215=CARTESIAN_POINT('Ctrl Pts',(-18.9803258451703,12.7987545965281,124.585924474665)) ;
#17216=CARTESIAN_POINT('Ctrl Pts',(-18.9752237614047,12.7990038112658,124.584047907311)) ;
#17217=CARTESIAN_POINT('Ctrl Pts',(-18.9644313744561,12.7995317874279,124.579998302248)) ;
#17218=CARTESIAN_POINT('Ctrl Pts',(-18.9587443938632,12.799810463628,124.577816838011)) ;
#17219=CARTESIAN_POINT('Ctrl Pts',(-18.9256333390202,12.8014360006373,124.564837386973)) ;
#17220=CARTESIAN_POINT('Ctrl Pts',(-18.8985820134551,12.8027767993694,124.553113705154)) ;
#17221=CARTESIAN_POINT('Ctrl Pts',(-18.8558699778635,12.8049312152057,124.532779982081)) ;
#17222=CARTESIAN_POINT('Ctrl Pts',(-18.839935527488,12.8057435595496,124.524771544718)) ;
#17223=CARTESIAN_POINT('Ctrl Pts',(-18.8153499744578,12.8070130804467,124.511748975838)) ;
#17224=CARTESIAN_POINT('Ctrl Pts',(-18.8065784404411,12.807469289257,124.506967317279)) ;
#17225=CARTESIAN_POINT('Ctrl Pts',(-18.7911142894719,12.8082798229713,124.498295227069)) ;
#17226=CARTESIAN_POINT('Ctrl Pts',(-18.7843987140776,12.8086339352717,124.494446801091)) ;
#17227=CARTESIAN_POINT('Ctrl Pts',(-18.7713762521518,12.8093249321281,124.486822617535)) ;
#17228=CARTESIAN_POINT('Ctrl Pts',(-18.7650660677071,12.8096617727325,124.483053106636)) ;
#17229=CARTESIAN_POINT('Ctrl Pts',(-18.7504283843418,12.8104479788474,124.474132892003)) ;
#17230=CARTESIAN_POINT('Ctrl Pts',(-18.742127435643,12.8108975360351,124.468939564859)) ;
#17231=CARTESIAN_POINT('Ctrl Pts',(-18.7027397971061,12.8130489198317,124.443648737006)) ;
#17232=CARTESIAN_POINT('Ctrl Pts',(-18.6724951513233,12.8147566502298,124.422274537197)) ;
#17233=CARTESIAN_POINT('Ctrl Pts',(-18.6326722836895,12.8170813965894,124.391391564076)) ;
#17234=CARTESIAN_POINT('Ctrl Pts',(-18.6222329658112,12.8176982802149,124.38302400425)) ;
#17235=CARTESIAN_POINT('Ctrl Pts',(-18.6069019144491,12.8186149139447,124.370325968801)) ;
#17236=CARTESIAN_POINT('Ctrl Pts',(-18.6019065631736,12.8189153133053,124.366122123626)) ;
#17237=CARTESIAN_POINT('Ctrl Pts',(-18.5930292678969,12.8194521687923,124.358531827554)) ;
#17238=CARTESIAN_POINT('Ctrl Pts',(-18.5891348980241,12.8196887243887,124.355160157333)) ;
#17239=CARTESIAN_POINT('Ctrl Pts',(-18.5807880113737,12.8201980365719,124.347842828215)) ;
#17240=CARTESIAN_POINT('Ctrl Pts',(-18.5763426001166,12.82047073064,124.343889263449)) ;
#17241=CARTESIAN_POINT('Ctrl Pts',(-18.564347902368,12.8212106848589,124.333067335709)) ;
#17242=CARTESIAN_POINT('Ctrl Pts',(-18.5568542285001,12.8216775159828,124.326137998624)) ;
#17243=CARTESIAN_POINT('Ctrl Pts',(-18.5425264467297,12.8225797307972,124.312559959872)) ;
#17244=CARTESIAN_POINT('Ctrl Pts',(-18.5356818918536,12.8230151294021,124.305923307416)) ;
#17245=CARTESIAN_POINT('Ctrl Pts',(-18.5242856482261,12.8237480503756,124.294617426755)) ;
#17246=CARTESIAN_POINT('Ctrl Pts',(-18.5196933662955,12.8240456319155,124.289989712524)) ;
#17247=CARTESIAN_POINT('Ctrl Pts',(-18.4996292911165,12.8253561124514,124.269451942769)) ;
#17248=CARTESIAN_POINT('Ctrl Pts',(-18.4845465990051,12.8263686717888,124.253167439685)) ;
#17249=CARTESIAN_POINT('Ctrl Pts',(-18.4615839543545,12.8279589485158,124.227011285135)) ;
#17250=CARTESIAN_POINT('Ctrl Pts',(-18.4534064174256,12.828535602789,124.217407086905)) ;
#17251=CARTESIAN_POINT('Ctrl Pts',(-18.4383242250919,12.8296196212799,124.19914061251)) ;
#17252=CARTESIAN_POINT('Ctrl Pts',(-18.4313866247621,12.8301268102426,124.190507109525)) ;
#17253=CARTESIAN_POINT('Ctrl Pts',(-18.4173167616063,12.8311737882064,124.17251324898)) ;
#17254=CARTESIAN_POINT('Ctrl Pts',(-18.4102000964298,12.8317135837244,124.163142065915)) ;
#17255=CARTESIAN_POINT('Ctrl Pts',(-18.3785915210041,12.8341590400966,124.120276717119)) ;
#17256=CARTESIAN_POINT('Ctrl Pts',(-18.3556443403483,12.8360695219318,124.085676277074)) ;
#17257=CARTESIAN_POINT('Ctrl Pts',(-18.3275920554326,12.8385982385192,124.038431452916)) ;
#17258=CARTESIAN_POINT('Ctrl Pts',(-18.320910784028,12.8392169989039,124.026753662401)) ;
#17259=CARTESIAN_POINT('Ctrl Pts',(-18.2999386576922,12.8412137193077,123.988684908242)) ;
#17260=CARTESIAN_POINT('Ctrl Pts',(-18.2864092655001,12.8425889950063,123.961886513872)) ;
#17261=CARTESIAN_POINT('Ctrl Pts',(-18.2561390929588,12.8459075576379,123.896147498959)) ;
#17262=CARTESIAN_POINT('Ctrl Pts',(-18.2403883533361,12.8478499286865,123.856791991268)) ;
#17263=CARTESIAN_POINT('Ctrl Pts',(-18.2159181794863,12.8513191239244,123.785320842823)) ;
#17264=CARTESIAN_POINT('Ctrl Pts',(-18.2064243658445,12.8528431832765,123.753513062738)) ;
#17265=CARTESIAN_POINT('Ctrl Pts',(-18.1965692307665,12.8546680305787,123.714956539527)) ;
#17266=CARTESIAN_POINT('Ctrl Pts',(-18.1949820290037,12.8549712114887,123.708534856787)) ;
#17267=CARTESIAN_POINT('Ctrl Pts',(-18.1914072689346,12.8556763185502,123.693562450381)) ;
#17268=CARTESIAN_POINT('Ctrl Pts',(-18.189458661781,12.8560780887129,123.68500277319)) ;
#17269=CARTESIAN_POINT('Ctrl Pts',(-18.1852034382759,12.8569970743002,123.665356847336)) ;
#17270=CARTESIAN_POINT('Ctrl Pts',(-18.1829569675309,12.8575139552109,123.654258329805)) ;
#17271=CARTESIAN_POINT('Ctrl Pts',(-18.1796945423303,12.8583170926136,123.636933153194)) ;
#17272=CARTESIAN_POINT('Ctrl Pts',(-18.1785744105169,12.8586040579667,123.630726759156)) ;
#17273=CARTESIAN_POINT('Ctrl Pts',(-18.1748597197803,12.8595960697717,123.609214318925)) ;
#17274=CARTESIAN_POINT('Ctrl Pts',(-18.1725033720112,12.8602986929342,123.593868700848)) ;
#17275=CARTESIAN_POINT('Ctrl Pts',(-18.1639997962845,12.8631805185092,123.530662102417)) ;
#17276=CARTESIAN_POINT('Ctrl Pts',(-18.1603405148723,12.865351269217,123.482509207639)) ;
#17277=CARTESIAN_POINT('Ctrl Pts',(-18.1593282957932,12.8679179022969,123.426161558769)) ;
#17278=CARTESIAN_POINT('Ctrl Pts',(-18.1592615433982,12.8682876430093,123.418056403349)) ;
#17279=CARTESIAN_POINT('Ctrl Pts',(-18.1592804871582,12.8688684674536,123.40534702554)) ;
#17280=CARTESIAN_POINT('Ctrl Pts',(-18.1593127879161,12.8690790917927,123.400742933181)) ;
#17281=CARTESIAN_POINT('Ctrl Pts',(-18.1594151706232,12.8694529712368,123.392579205984)) ;
#17282=CARTESIAN_POINT('Ctrl Pts',(-18.1594750249168,12.8696161365814,123.389019490853)) ;
#17283=CARTESIAN_POINT('Ctrl Pts',(-18.159632765082,12.869959302323,123.381539439266)) ;
#17284=CARTESIAN_POINT('Ctrl Pts',(-18.1597338933685,12.8701393287889,123.377619210777)) ;
#17285=CARTESIAN_POINT('Ctrl Pts',(-18.1600664474139,12.8706404508407,123.36671796321)) ;
#17286=CARTESIAN_POINT('Ctrl Pts',(-18.1603379409469,12.8709618823952,123.359738327528)) ;
#17287=CARTESIAN_POINT('Ctrl Pts',(-18.1610858282145,12.8716915036932,123.343925157774)) ;
#17288=CARTESIAN_POINT('Ctrl Pts',(-18.1615975234618,12.8720999681551,123.335093680034)) ;
#17289=CARTESIAN_POINT('Ctrl Pts',(-18.1635094233256,12.8733921735138,123.307222442001)) ;
#17290=CARTESIAN_POINT('Ctrl Pts',(-18.1652520719457,12.8742783891576,123.288209034038)) ;
#17291=CARTESIAN_POINT('Ctrl Pts',(-18.1742895560144,12.8779645148339,123.209489550242)) ;
#17292=CARTESIAN_POINT('Ctrl Pts',(-18.1854536468484,12.880764858379,123.150307440896)) ;
#17293=CARTESIAN_POINT('Ctrl Pts',(-18.2051839412113,12.8843217173769,123.075718257719)) ;
#17294=CARTESIAN_POINT('Ctrl Pts',(-18.2098679568054,12.885104230482,123.059367781973)) ;
#17295=CARTESIAN_POINT('Ctrl Pts',(-18.2188151390036,12.8864981714979,123.030383482486)) ;
#17296=CARTESIAN_POINT('Ctrl Pts',(-18.2229495608453,12.8871098980653,123.017712690547)) ;
#17297=CARTESIAN_POINT('Ctrl Pts',(-18.2312369557602,12.8882780263911,122.993627386663)) ;
#17298=CARTESIAN_POINT('Ctrl Pts',(-18.2353552290918,12.8888344541128,122.982202526046)) ;
#17299=CARTESIAN_POINT('Ctrl Pts',(-18.2447155077819,12.8900493585435,122.957375511653)) ;
#17300=CARTESIAN_POINT('Ctrl Pts',(-18.2500238013672,12.8907075928925,122.944000178725)) ;
#17301=CARTESIAN_POINT('Ctrl Pts',(-18.2628071722129,12.8922258766517,122.913344464763)) ;
#17302=CARTESIAN_POINT('Ctrl Pts',(-18.2704441053724,12.8930853963541,122.896135321457)) ;
#17303=CARTESIAN_POINT('Ctrl Pts',(-18.289582210683,12.8951337624835,122.8555100139)) ;
#17304=CARTESIAN_POINT('Ctrl Pts',(-18.3014334469546,12.89632135519,122.832268412208)) ;
#17305=CARTESIAN_POINT('Ctrl Pts',(-18.3327522209393,12.8992749106568,122.775325356876)) ;
#17306=CARTESIAN_POINT('Ctrl Pts',(-18.3530825246731,12.9010333462363,122.742130189385)) ;
#17307=CARTESIAN_POINT('Ctrl Pts',(-18.3894936180088,12.9039728161439,122.688471779208)) ;
#17308=CARTESIAN_POINT('Ctrl Pts',(-18.4047240157505,12.9051508716758,122.667465130711)) ;
#17309=CARTESIAN_POINT('Ctrl Pts',(-18.4257461752842,12.9067181083841,122.640291647039)) ;
#17310=CARTESIAN_POINT('Ctrl Pts',(-18.4309625618981,12.9071024941052,122.63368777043)) ;
#17311=CARTESIAN_POINT('Ctrl Pts',(-18.4394885333965,12.9077237505213,122.623115270299)) ;
#17312=CARTESIAN_POINT('Ctrl Pts',(-18.4427567443871,12.907960276725,122.619113604254)) ;
#17313=CARTESIAN_POINT('Ctrl Pts',(-18.4492906270678,12.9084299999391,122.611213861411)) ;
#17314=CARTESIAN_POINT('Ctrl Pts',(-18.4525554640106,12.9086631861876,122.607315220292)) ;
#17315=CARTESIAN_POINT('Ctrl Pts',(-18.4558540804007,12.9088972815569,122.603424719808)) ;
#17316=CARTESIAN_POINT('Ctrl Pts',(-18.4558641674244,12.9088979973962,122.603412823281)) ;
#17317=CARTESIAN_POINT('Ctrl Pts',(-18.4558843566946,12.9088994301272,122.603389013175)) ;
#17318=CARTESIAN_POINT('Ctrl Pts',(-18.4558944592937,12.9089001470437,122.603377099183)) ;
#17319=CARTESIAN_POINT('Ctrl Pts',(-18.4559146813778,12.9089015820471,122.60335325219)) ;
#17320=CARTESIAN_POINT('Ctrl Pts',(-18.4559248003457,12.9089023000971,122.603341319802)) ;
#17321=CARTESIAN_POINT('Ctrl Pts',(-18.455945056138,12.9089037374361,122.603317434877)) ;
#17322=CARTESIAN_POINT('Ctrl Pts',(-18.455955192484,12.908904456691,122.603305482907)) ;
#17323=CARTESIAN_POINT('Ctrl Pts',(-18.4559754810373,12.9089058962981,122.603281561176)) ;
#17324=CARTESIAN_POINT('Ctrl Pts',(-18.4559856343577,12.9089066167292,122.603269590104)) ;
#17325=CARTESIAN_POINT('Ctrl Pts',(-18.4560059588853,12.9089080588321,122.603245627787)) ;
#17326=CARTESIAN_POINT('Ctrl Pts',(-18.4560161301038,12.9089087805047,122.603233636529)) ;
#17327=CARTESIAN_POINT('Ctrl Pts',(-18.4560364903646,12.9089102250861,122.603209633919)) ;
#17328=CARTESIAN_POINT('Ctrl Pts',(-18.4560466796096,12.9089109480092,122.603197622329)) ;
#17329=CARTESIAN_POINT('Ctrl Pts',(-18.4560670777304,12.9089123952197,122.603173576929)) ;
#17330=CARTESIAN_POINT('Ctrl Pts',(-18.4560772858882,12.908913119456,122.603161543966)) ;
#17331=CARTESIAN_POINT('Ctrl Pts',(-18.4560977223255,12.9089145693275,122.603137455248)) ;
#17332=CARTESIAN_POINT('Ctrl Pts',(-18.4561079501488,12.9089152949304,122.603125400031)) ;
#17333=CARTESIAN_POINT('Ctrl Pts',(-18.456128425055,12.9089167474735,122.603101267825)) ;
#17334=CARTESIAN_POINT('Ctrl Pts',(-18.4561386727124,12.9089174744546,122.60308919016)) ;
#17335=CARTESIAN_POINT('Ctrl Pts',(-18.456159187164,12.9089189297455,122.603065013207)) ;
#17336=CARTESIAN_POINT('Ctrl Pts',(-18.4561694545687,12.9089196580985,122.603052913202)) ;
#17337=CARTESIAN_POINT('Ctrl Pts',(-18.4561900120466,12.9089211163836,122.603028687412)) ;
#17338=CARTESIAN_POINT('Ctrl Pts',(-18.4562003009971,12.908921846236,122.603016562952)) ;
#17339=CARTESIAN_POINT('Ctrl Pts',(-18.4562208987565,12.9089233073204,122.60299229157)) ;
#17340=CARTESIAN_POINT('Ctrl Pts',(-18.4562312086243,12.9089240386274,122.602980143403)) ;
#17341=CARTESIAN_POINT('Ctrl Pts',(-18.4562518503084,12.908925502769,122.602955822147)) ;
#17342=CARTESIAN_POINT('Ctrl Pts',(-18.4562621819516,12.9089262355913,122.602943649266)) ;
#17343=CARTESIAN_POINT('Ctrl Pts',(-18.4562828682643,12.9089277028398,122.60291927732)) ;
#17344=CARTESIAN_POINT('Ctrl Pts',(-18.4562932226001,12.9089284372423,122.60290707865)) ;
#17345=CARTESIAN_POINT('Ctrl Pts',(-18.4563139528768,12.9089299075501,122.602882656808)) ;
#17346=CARTESIAN_POINT('Ctrl Pts',(-18.4563243295604,12.9089306435081,122.602870432763)) ;
#17347=CARTESIAN_POINT('Ctrl Pts',(-18.4563451072982,12.908932117123,122.602845956917)) ;
#17348=CARTESIAN_POINT('Ctrl Pts',(-18.456355507598,12.9089328547263,122.602833706007)) ;
#17349=CARTESIAN_POINT('Ctrl Pts',(-18.4563763318937,12.9089343315837,122.602809177235)) ;
#17350=CARTESIAN_POINT('Ctrl Pts',(-18.4563867559345,12.9089350708409,122.602796899321)) ;
#17351=CARTESIAN_POINT('Ctrl Pts',(-18.4564076289155,12.9089365510913,122.602772315129)) ;
#17352=CARTESIAN_POINT('Ctrl Pts',(-18.4564180775277,12.9089372920612,122.602760009239)) ;
#17353=CARTESIAN_POINT('Ctrl Pts',(-18.4564389991234,12.9089387756992,122.602735369723)) ;
#17354=CARTESIAN_POINT('Ctrl Pts',(-18.4564494723635,12.9089395183855,122.602723035797)) ;
#17355=CARTESIAN_POINT('Ctrl Pts',(-18.4564704452369,12.9089410055996,122.602698337835)) ;
#17356=CARTESIAN_POINT('Ctrl Pts',(-18.4564809443246,12.9089417500887,122.602685974444)) ;
#17357=CARTESIAN_POINT('Ctrl Pts',(-18.4565019674821,12.9089432408079,122.60266121922)) ;
#17358=CARTESIAN_POINT('Ctrl Pts',(-18.4565124923333,12.9089439870934,122.602648826469)) ;
#17359=CARTESIAN_POINT('Ctrl Pts',(-18.4565335679513,12.9089454814717,122.602624011434)) ;
#17360=CARTESIAN_POINT('Ctrl Pts',(-18.4565441189964,12.9089462295841,122.602611588825)) ;
#17361=CARTESIAN_POINT('Ctrl Pts',(-18.4565652487466,12.9089477277395,122.602586712025)) ;
#17362=CARTESIAN_POINT('Ctrl Pts',(-18.4565758269448,12.9089484777465,122.602574258435)) ;
#17363=CARTESIAN_POINT('Ctrl Pts',(-18.4565970109862,12.9089499796898,122.602549319699)) ;
#17364=CARTESIAN_POINT('Ctrl Pts',(-18.4566076168602,12.9089507316283,122.602536834519)) ;
#17365=CARTESIAN_POINT('Ctrl Pts',(-18.4566288557991,12.9089522374021,122.602511833148)) ;
#17366=CARTESIAN_POINT('Ctrl Pts',(-18.4566394894094,12.908952991276,122.602499316316)) ;
#17367=CARTESIAN_POINT('Ctrl Pts',(-18.456660785507,12.9089545010401,122.602474249663)) ;
#17368=CARTESIAN_POINT('Ctrl Pts',(-18.4566714476506,12.9089552569058,122.602461700249)) ;
#17369=CARTESIAN_POINT('Ctrl Pts',(-18.456692801756,12.9089567707199,122.60243656733)) ;
#17370=CARTESIAN_POINT('Ctrl Pts',(-18.456703493267,12.9089575286362,122.602423984359)) ;
#17371=CARTESIAN_POINT('Ctrl Pts',(-18.4567249053252,12.9089590464959,122.602398785257)) ;
#17372=CARTESIAN_POINT('Ctrl Pts',(-18.4567356262341,12.9089598064648,122.602386168702)) ;
#17373=CARTESIAN_POINT('Ctrl Pts',(-18.4567570988112,12.9089613285514,122.602360900411)) ;
#17374=CARTESIAN_POINT('Ctrl Pts',(-18.4567678501102,12.9089620906429,122.602348249113)) ;
#17375=CARTESIAN_POINT('Ctrl Pts',(-18.4567893831584,12.9089636169527,122.602322911708)) ;
#17376=CARTESIAN_POINT('Ctrl Pts',(-18.456800165178,12.90896438119,122.602310225286)) ;
#17377=CARTESIAN_POINT('Ctrl Pts',(-18.4568217602641,12.9089659118333,122.60228481694)) ;
#17378=CARTESIAN_POINT('Ctrl Pts',(-18.4568325735926,12.9089666782578,122.602272094711)) ;
#17379=CARTESIAN_POINT('Ctrl Pts',(-18.4568542313575,12.9089682132796,122.602246614688)) ;
#17380=CARTESIAN_POINT('Ctrl Pts',(-18.4568650761759,12.9089689819039,122.602233856447)) ;
#17381=CARTESIAN_POINT('Ctrl Pts',(-18.4568867992335,12.9089705214889,122.602208301689)) ;
#17382=CARTESIAN_POINT('Ctrl Pts',(-18.4568976768567,12.9089712924059,122.6021955059)) ;
#17383=CARTESIAN_POINT('Ctrl Pts',(-18.4569194638754,12.9089728364592,122.602169877992)) ;
#17384=CARTESIAN_POINT('Ctrl Pts',(-18.4569303739604,12.9089736096443,122.602157045066)) ;
#17385=CARTESIAN_POINT('Ctrl Pts',(-18.456952228497,12.9089751584173,122.602131339843)) ;
#17386=CARTESIAN_POINT('Ctrl Pts',(-18.4569631722283,12.9089759339541,122.602118468397)) ;
#17387=CARTESIAN_POINT('Ctrl Pts',(-18.4569850941584,12.9089774874374,122.602092686025)) ;
#17388=CARTESIAN_POINT('Ctrl Pts',(-18.4569960721004,12.9089782653657,122.602079775404)) ;
#17389=CARTESIAN_POINT('Ctrl Pts',(-18.4570180622743,12.908979823619,122.602053914902)) ;
#17390=CARTESIAN_POINT('Ctrl Pts',(-18.4570290747303,12.9089806039599,122.60204096476)) ;
#17391=CARTESIAN_POINT('Ctrl Pts',(-18.4570511350328,12.9089821671162,122.602015023931)) ;
#17392=CARTESIAN_POINT('Ctrl Pts',(-18.4570621827805,12.9089829499245,122.602002033364)) ;
#17393=CARTESIAN_POINT('Ctrl Pts',(-18.4570843139133,12.9089845180328,122.601976011403)) ;
#17394=CARTESIAN_POINT('Ctrl Pts',(-18.4570953975003,12.908985303347,122.601962979776)) ;
#17395=CARTESIAN_POINT('Ctrl Pts',(-18.45711760032,12.9089868764674,122.601936875698)) ;
#17396=CARTESIAN_POINT('Ctrl Pts',(-18.4571287199829,12.908987664304,122.601923802743)) ;
#17397=CARTESIAN_POINT('Ctrl Pts',(-18.4571509967091,12.9089892425931,122.601897613958)) ;
#17398=CARTESIAN_POINT('Ctrl Pts',(-18.4571621533885,12.9089900330183,122.601884498581)) ;
#17399=CARTESIAN_POINT('Ctrl Pts',(-18.4571845043054,12.9089916164956,122.601858224776)) ;
#17400=CARTESIAN_POINT('Ctrl Pts',(-18.4571956984338,12.9089924095398,122.60184506648)) ;
#17401=CARTESIAN_POINT('Ctrl Pts',(-18.4572181253768,12.9089939983346,122.60181870552)) ;
#17402=CARTESIAN_POINT('Ctrl Pts',(-18.4572293578823,12.9089947940632,122.601805503223)) ;
#17403=CARTESIAN_POINT('Ctrl Pts',(-18.4572518608785,12.9089963881768,122.601779055099)) ;
#17404=CARTESIAN_POINT('Ctrl Pts',(-18.4572631318871,12.9089971865984,122.601765808666)) ;
#17405=CARTESIAN_POINT('Ctrl Pts',(-18.4572857132798,12.908998786196,122.601739270645)) ;
#17406=CARTESIAN_POINT('Ctrl Pts',(-18.4572970235877,12.9089995873666,122.601725979151)) ;
#17407=CARTESIAN_POINT('Ctrl Pts',(-18.4573196841441,12.9090011925019,122.601699350356)) ;
#17408=CARTESIAN_POINT('Ctrl Pts',(-18.4573310343277,12.909001996462,122.601686013135)) ;
#17409=CARTESIAN_POINT('Ctrl Pts',(-18.45735377563,12.9090036072463,122.601659291729)) ;
#17410=CARTESIAN_POINT('Ctrl Pts',(-18.4573651665971,12.9090044140598,122.601645907727)) ;
#17411=CARTESIAN_POINT('Ctrl Pts',(-18.4573879885289,12.9090060304842,122.601619093872)) ;
#17412=CARTESIAN_POINT('Ctrl Pts',(-18.4573994201699,12.9090068401429,122.601605663229)) ;
#17413=CARTESIAN_POINT('Ctrl Pts',(-18.4574223260808,12.9090084624439,122.601578753014)) ;
#17414=CARTESIAN_POINT('Ctrl Pts',(-18.457433799672,12.9090092750379,122.601565274243)) ;
#17415=CARTESIAN_POINT('Ctrl Pts',(-18.4574567891932,12.9090109031885,122.601538268126)) ;
#17416=CARTESIAN_POINT('Ctrl Pts',(-18.4574683050772,12.9090117187417,122.601524740838)) ;
#17417=CARTESIAN_POINT('Ctrl Pts',(-18.4574913803924,12.9090133528958,122.601497636278)) ;
#17418=CARTESIAN_POINT('Ctrl Pts',(-18.4575029395734,12.9090141714789,122.601484059305)) ;
#17419=CARTESIAN_POINT('Ctrl Pts',(-18.4575261006358,12.9090158116324,122.601456856385)) ;
#17420=CARTESIAN_POINT('Ctrl Pts',(-18.4575377031876,12.9090166332502,122.601443229654)) ;
#17421=CARTESIAN_POINT('Ctrl Pts',(-18.4575609527486,12.9090182795971,122.601415925167)) ;
#17422=CARTESIAN_POINT('Ctrl Pts',(-18.4575725996707,12.90901910432,122.601402247517)) ;
#17423=CARTESIAN_POINT('Ctrl Pts',(-18.4575959378497,12.9090207568679,122.60137484135)) ;
#17424=CARTESIAN_POINT('Ctrl Pts',(-18.4576076293573,12.9090215847107,122.601361112543)) ;
#17425=CARTESIAN_POINT('Ctrl Pts',(-18.4576310589047,12.9090232436536,122.601333601494)) ;
#17426=CARTESIAN_POINT('Ctrl Pts',(-18.4576427962344,12.9090240747034,122.60131982009)) ;
#17427=CARTESIAN_POINT('Ctrl Pts',(-18.4576663171573,12.9090257400409,122.601292204178)) ;
#17428=CARTESIAN_POINT('Ctrl Pts',(-18.4576781008623,12.9090265743365,122.601278369543)) ;
#17429=CARTESIAN_POINT('Ctrl Pts',(-18.4577017142152,12.9090282461424,122.601250647559)) ;
#17430=CARTESIAN_POINT('Ctrl Pts',(-18.4577135445022,12.9090290836979,122.601236759464)) ;
#17431=CARTESIAN_POINT('Ctrl Pts',(-18.4577372527087,12.9090307621429,122.60120892859)) ;
#17432=CARTESIAN_POINT('Ctrl Pts',(-18.4577491304199,12.9090316030176,122.601194986061)) ;
#17433=CARTESIAN_POINT('Ctrl Pts',(-18.4577729347397,12.9090332881899,122.601167044849)) ;
#17434=CARTESIAN_POINT('Ctrl Pts',(-18.4577848608323,12.909034132451,122.601153046777)) ;
#17435=CARTESIAN_POINT('Ctrl Pts',(-18.457808761954,12.9090358243986,122.601124994448)) ;
#17436=CARTESIAN_POINT('Ctrl Pts',(-18.4578207370233,12.9090366720878,122.601110940149)) ;
#17437=CARTESIAN_POINT('Ctrl Pts',(-18.4578447362279,12.9090383709002,122.601082775231)) ;
#17438=CARTESIAN_POINT('Ctrl Pts',(-18.4578567607262,12.9090392220491,122.60106866419)) ;
#17439=CARTESIAN_POINT('Ctrl Pts',(-18.457880859675,12.9090409278431,122.601040384763)) ;
#17440=CARTESIAN_POINT('Ctrl Pts',(-18.4578929341062,12.9090417824868,122.601026216404)) ;
#17441=CARTESIAN_POINT('Ctrl Pts',(-18.457917135395,12.9090434954452,122.600997819454)) ;
#17442=CARTESIAN_POINT('Ctrl Pts',(-18.4579292613029,12.9090443536925,122.600983591983)) ;
#17443=CARTESIAN_POINT('Ctrl Pts',(-18.4579535637288,12.9090460737291,122.600955078953)) ;
#17444=CARTESIAN_POINT('Ctrl Pts',(-18.4579657409352,12.9090469355669,122.600940792593)) ;
#17445=CARTESIAN_POINT('Ctrl Pts',(-18.4579901481554,12.9090486629395,122.600912159226)) ;
#17446=CARTESIAN_POINT('Ctrl Pts',(-18.4580023778348,12.9090495284504,122.600897812616)) ;
#17447=CARTESIAN_POINT('Ctrl Pts',(-18.4580268902977,12.9090512631897,122.600869058419)) ;
#17448=CARTESIAN_POINT('Ctrl Pts',(-18.4580391731387,12.909052132422,122.600854650769)) ;
#17449=CARTESIAN_POINT('Ctrl Pts',(-18.4580637922039,12.9090538746233,122.60082577418)) ;
#17450=CARTESIAN_POINT('Ctrl Pts',(-18.4580761288096,12.909054747619,122.600811304799)) ;
#17451=CARTESIAN_POINT('Ctrl Pts',(-18.4581008560335,12.9090564973912,122.600782304028)) ;
#17452=CARTESIAN_POINT('Ctrl Pts',(-18.4581132470015,12.9090573741923,122.600767772233)) ;
#17453=CARTESIAN_POINT('Ctrl Pts',(-18.458138084327,12.9090591316718,122.600738645035)) ;
#17454=CARTESIAN_POINT('Ctrl Pts',(-18.4581505306124,12.9090600123451,122.600724049723)) ;
#17455=CARTESIAN_POINT('Ctrl Pts',(-18.4581754788481,12.9090617775882,122.600694795187)) ;
#17456=CARTESIAN_POINT('Ctrl Pts',(-18.4581879809698,12.90906266217,122.600680135768)) ;
#17457=CARTESIAN_POINT('Ctrl Pts',(-18.4582130421042,12.9090644353161,122.600650751598)) ;
#17458=CARTESIAN_POINT('Ctrl Pts',(-18.4582256008775,12.9090653238634,122.600636027134)) ;
#17459=CARTESIAN_POINT('Ctrl Pts',(-18.4582507766476,12.9090671050344,122.60060651133)) ;
#17460=CARTESIAN_POINT('Ctrl Pts',(-18.4582633931829,12.9090679976252,122.600591720538)) ;
#17461=CARTESIAN_POINT('Ctrl Pts',(-18.4582886840692,12.9090697868538,122.600562072575)) ;
#17462=CARTESIAN_POINT('Ctrl Pts',(-18.4583013588228,12.9090706835199,122.600547214938)) ;
#17463=CARTESIAN_POINT('Ctrl Pts',(-18.4583267667073,12.9090724809382,122.600517432648)) ;
#17464=CARTESIAN_POINT('Ctrl Pts',(-18.4583395001851,12.9090733817147,122.600502507594)) ;
#17465=CARTESIAN_POINT('Ctrl Pts',(-18.4583650277375,12.9090751875102,122.600472587887)) ;
#17466=CARTESIAN_POINT('Ctrl Pts',(-18.4583778212882,12.9090760924919,122.600457593854)) ;
#17467=CARTESIAN_POINT('Ctrl Pts',(-18.4584034682777,12.9090779066471,122.600427537039)) ;
#17468=CARTESIAN_POINT('Ctrl Pts',(-18.4584163220759,12.9090788158458,122.600412473842)) ;
#17469=CARTESIAN_POINT('Ctrl Pts',(-18.4584420920024,12.9090806386071,122.600382275859)) ;
#17470=CARTESIAN_POINT('Ctrl Pts',(-18.4584550075113,12.9090815521256,122.600367141805)) ;
#17471=CARTESIAN_POINT('Ctrl Pts',(-18.4584808999983,12.909083383465,122.600336803135)) ;
#17472=CARTESIAN_POINT('Ctrl Pts',(-18.4584938774174,12.9090843013168,122.60032159801)) ;
#17473=CARTESIAN_POINT('Ctrl Pts',(-18.4585198958153,12.90908614147,122.600291114771)) ;
#17474=CARTESIAN_POINT('Ctrl Pts',(-18.4585329364719,12.9090870637484,122.600275837041)) ;
#17475=CARTESIAN_POINT('Ctrl Pts',(-18.4585590810185,12.9090889127309,122.600245208995)) ;
#17476=CARTESIAN_POINT('Ctrl Pts',(-18.4585721853996,12.9090898394696,122.600229858111)) ;
#17477=CARTESIAN_POINT('Ctrl Pts',(-18.4585984582777,12.9090916974344,122.600199082746)) ;
#17478=CARTESIAN_POINT('Ctrl Pts',(-18.4586116270783,12.9090926286819,122.600183657916)) ;
#17479=CARTESIAN_POINT('Ctrl Pts',(-18.4586380302734,12.9090944957681,122.600152732949)) ;
#17480=CARTESIAN_POINT('Ctrl Pts',(-18.4586512643879,12.9090954315869,122.600137233148)) ;
#17481=CARTESIAN_POINT('Ctrl Pts',(-18.4586778000525,12.9090973079453,122.600106156103)) ;
#17482=CARTESIAN_POINT('Ctrl Pts',(-18.4586911009341,12.9090982484375,122.600090579651)) ;
#17483=CARTESIAN_POINT('Ctrl Pts',(-18.4587177686679,12.9091001340384,122.600059351043)) ;
#17484=CARTESIAN_POINT('Ctrl Pts',(-18.4587311362994,12.9091010792021,122.600043697983)) ;
#17485=CARTESIAN_POINT('Ctrl Pts',(-18.4587579402238,12.9091029743355,122.600012313033)) ;
#17486=CARTESIAN_POINT('Ctrl Pts',(-18.4587713761281,12.9091039242776,122.599996581605)) ;
#17487=CARTESIAN_POINT('Ctrl Pts',(-18.4587983161713,12.9091058289369,122.599965040444)) ;
#17488=CARTESIAN_POINT('Ctrl Pts',(-18.4588118207581,12.9091067836856,122.599949230193)) ;
#17489=CARTESIAN_POINT('Ctrl Pts',(-18.4588388997442,12.9091086980691,122.599917529561)) ;
#17490=CARTESIAN_POINT('Ctrl Pts',(-18.4588524740382,12.9091096576961,122.599901639312)) ;
#17491=CARTESIAN_POINT('Ctrl Pts',(-18.4588796934132,12.9091115819044,122.599869777567)) ;
#17492=CARTESIAN_POINT('Ctrl Pts',(-18.4588933382743,12.9091125464698,122.599853806338)) ;
#17493=CARTESIAN_POINT('Ctrl Pts',(-18.4589207003143,12.9091144806623,122.599821780865)) ;
#17494=CARTESIAN_POINT('Ctrl Pts',(-18.458934417088,12.9091154502604,122.599805727105)) ;
#17495=CARTESIAN_POINT('Ctrl Pts',(-18.4589619220333,12.9091173944524,122.599773537675)) ;
#17496=CARTESIAN_POINT('Ctrl Pts',(-18.4589757109707,12.9091183691002,122.599757401116)) ;
#17497=CARTESIAN_POINT('Ctrl Pts',(-18.4590033621648,12.9091203235266,122.599725043866)) ;
#17498=CARTESIAN_POINT('Ctrl Pts',(-18.4590172243706,12.9091213033013,122.599708823243)) ;
#17499=CARTESIAN_POINT('Ctrl Pts',(-18.4590450235525,12.9091232680833,122.599676296191)) ;
#17500=CARTESIAN_POINT('Ctrl Pts',(-18.4590589602244,12.9091242530688,122.599659990128)) ;
#17501=CARTESIAN_POINT('Ctrl Pts',(-18.4590869084532,12.9091262282796,122.599627292089)) ;
#17502=CARTESIAN_POINT('Ctrl Pts',(-18.4591009202929,12.9091272185246,122.599610899792)) ;
#17503=CARTESIAN_POINT('Ctrl Pts',(-18.4591290198551,12.9091292043242,122.599578028145)) ;
#17504=CARTESIAN_POINT('Ctrl Pts',(-18.4591431077237,12.9091301998887,122.599561548634)) ;
#17505=CARTESIAN_POINT('Ctrl Pts',(-18.4591713608469,12.9091321964327,122.599528500829)) ;
#17506=CARTESIAN_POINT('Ctrl Pts',(-18.4591855258646,12.9091331973951,122.599511932822)) ;
#17507=CARTESIAN_POINT('Ctrl Pts',(-18.4592139342817,12.9091352048042,122.599478706888)) ;
#17508=CARTESIAN_POINT('Ctrl Pts',(-18.4592281775396,12.9091362112407,122.599462049137)) ;
#17509=CARTESIAN_POINT('Ctrl Pts',(-18.459256742632,12.9091382296108,122.599428643517)) ;
#17510=CARTESIAN_POINT('Ctrl Pts',(-18.4592710648103,12.9091392415685,122.599411895256)) ;
#17511=CARTESIAN_POINT('Ctrl Pts',(-18.4592997893301,12.9091412710922,122.599378306789)) ;
#17512=CARTESIAN_POINT('Ctrl Pts',(-18.459314191593,12.9091422886525,122.599361466685)) ;
#17513=CARTESIAN_POINT('Ctrl Pts',(-18.4593430770686,12.909144329436,122.599327693644)) ;
#17514=CARTESIAN_POINT('Ctrl Pts',(-18.4593575603095,12.909145352661,122.599310760684)) ;
#17515=CARTESIAN_POINT('Ctrl Pts',(-18.4593866090798,12.9091474048677,122.599276800394)) ;
#17516=CARTESIAN_POINT('Ctrl Pts',(-18.4594011744278,12.9091484338363,122.599259773288)) ;
#17517=CARTESIAN_POINT('Ctrl Pts',(-18.4594303883272,12.9091504975939,122.599225623668)) ;
#17518=CARTESIAN_POINT('Ctrl Pts',(-18.459445036834,12.9091515323793,122.599208501217)) ;
#17519=CARTESIAN_POINT('Ctrl Pts',(-18.4594744175564,12.9091536078055,122.599174160349)) ;
#17520=CARTESIAN_POINT('Ctrl Pts',(-18.4594891499515,12.9091546484584,122.599156941732)) ;
#17521=CARTESIAN_POINT('Ctrl Pts',(-18.4595187004174,12.9091567357574,122.599122406267)) ;
#17522=CARTESIAN_POINT('Ctrl Pts',(-18.4595335179825,12.9091577823674,122.599105090019)) ;
#17523=CARTESIAN_POINT('Ctrl Pts',(-18.45956324037,12.9091598816911,122.599070357476)) ;
#17524=CARTESIAN_POINT('Ctrl Pts',(-18.4595781446964,12.9091609343695,122.59905294177)) ;
#17525=CARTESIAN_POINT('Ctrl Pts',(-18.4596080389952,12.9091630457151,122.599018012227)) ;
#17526=CARTESIAN_POINT('Ctrl Pts',(-18.4596230301123,12.9091641044629,122.599000497063)) ;
#17527=CARTESIAN_POINT('Ctrl Pts',(-18.4596531011768,12.9091662281713,122.598965364916)) ;
#17528=CARTESIAN_POINT('Ctrl Pts',(-18.4596681807437,12.9091672931047,122.598947748389)) ;
#17529=CARTESIAN_POINT('Ctrl Pts',(-18.4596984295507,12.9091694292426,122.598912412566)) ;
#17530=CARTESIAN_POINT('Ctrl Pts',(-18.4597135986353,12.9091705004358,122.598894693463)) ;
#17531=CARTESIAN_POINT('Ctrl Pts',(-18.459744027297,12.9091726491504,122.598859151566)) ;
#17532=CARTESIAN_POINT('Ctrl Pts',(-18.4597592868648,12.9091737266706,122.598841328795)) ;
#17533=CARTESIAN_POINT('Ctrl Pts',(-18.4597898983033,12.9091758881658,122.598805577483)) ;
#17534=CARTESIAN_POINT('Ctrl Pts',(-18.459805249875,12.9091769721193,122.598787649303)) ;
#17535=CARTESIAN_POINT('Ctrl Pts',(-18.459836044968,12.909179146455,122.598751687623)) ;
#17536=CARTESIAN_POINT('Ctrl Pts',(-18.4598514891151,12.9091802368809,122.598733653404)) ;
#17537=CARTESIAN_POINT('Ctrl Pts',(-18.4598824715749,12.9091824243169,122.598697477095)) ;
#17538=CARTESIAN_POINT('Ctrl Pts',(-18.4598980097247,12.9091835213149,122.598679335208)) ;
#17539=CARTESIAN_POINT('Ctrl Pts',(-18.4599291813399,12.9091857219751,122.598642942256)) ;
#17540=CARTESIAN_POINT('Ctrl Pts',(-18.4599448147177,12.9091868256306,122.598624691308)) ;
#17541=CARTESIAN_POINT('Ctrl Pts',(-18.4599761776266,12.9091890396635,122.598588079295)) ;
#17542=CARTESIAN_POINT('Ctrl Pts',(-18.4599919073227,12.9091901500522,122.598569718051)) ;
#17543=CARTESIAN_POINT('Ctrl Pts',(-18.4600234638922,12.9091923776227,122.598532884291)) ;
#17544=CARTESIAN_POINT('Ctrl Pts',(-18.4600392909431,12.9091934948166,122.598514411581)) ;
#17545=CARTESIAN_POINT('Ctrl Pts',(-18.4600710442307,12.9091957361379,122.598477352586)) ;
#17546=CARTESIAN_POINT('Ctrl Pts',(-18.4600869701876,12.9091968602452,122.59845876664)) ;
#17547=CARTESIAN_POINT('Ctrl Pts',(-18.4601189216041,12.9091991154144,122.598421480843)) ;
#17548=CARTESIAN_POINT('Ctrl Pts',(-18.4601349473819,12.9092002464985,122.598402780634)) ;
#17549=CARTESIAN_POINT('Ctrl Pts',(-18.4601670999788,12.9092025157285,122.598365264557)) ;
#17550=CARTESIAN_POINT('Ctrl Pts',(-18.4601832268061,12.9092036538747,122.598346448693)) ;
#17551=CARTESIAN_POINT('Ctrl Pts',(-18.460215583374,12.9092059373599,122.598308699164)) ;
#17552=CARTESIAN_POINT('Ctrl Pts',(-18.4602318127925,12.9092070826757,122.598289765889)) ;
#17553=CARTESIAN_POINT('Ctrl Pts',(-18.4602643749783,12.9092093805296,122.598251781072)) ;
#17554=CARTESIAN_POINT('Ctrl Pts',(-18.4602807079974,12.909210533085,122.598232729251)) ;
#17555=CARTESIAN_POINT('Ctrl Pts',(-18.4603134788421,12.9092128455195,122.598194505686)) ;
#17556=CARTESIAN_POINT('Ctrl Pts',(-18.4603299167182,12.9092140054018,122.598175333898)) ;
#17557=CARTESIAN_POINT('Ctrl Pts',(-18.4603628989903,12.9092163326095,122.598136868444)) ;
#17558=CARTESIAN_POINT('Ctrl Pts',(-18.4603794431861,12.9092174999204,122.598117575028)) ;
#17559=CARTESIAN_POINT('Ctrl Pts',(-18.4604126391193,12.9092198420563,122.598078865172)) ;
#17560=CARTESIAN_POINT('Ctrl Pts',(-18.4604292909056,12.9092210168841,122.598059448691)) ;
#17561=CARTESIAN_POINT('Ctrl Pts',(-18.4604627030195,12.9092233741229,122.598020491586)) ;
#17562=CARTESIAN_POINT('Ctrl Pts',(-18.4604794635528,12.9092245565479,122.598000950738)) ;
#17563=CARTESIAN_POINT('Ctrl Pts',(-18.4605130950949,12.9092269291159,122.597961742691)) ;
#17564=CARTESIAN_POINT('Ctrl Pts',(-18.4605299659331,12.9092281192464,122.597942075708)) ;
#17565=CARTESIAN_POINT('Ctrl Pts',(-18.4605638189522,12.9092305072852,122.597902614427)) ;
#17566=CARTESIAN_POINT('Ctrl Pts',(-18.4605808012713,12.9092317052027,122.597882819985)) ;
#17567=CARTESIAN_POINT('Ctrl Pts',(-18.4606148789107,12.909234108931,122.597843101903)) ;
#17568=CARTESIAN_POINT('Ctrl Pts',(-18.4606319741094,12.9092353147327,122.597823178422)) ;
#17569=CARTESIAN_POINT('Ctrl Pts',(-18.4606662793476,12.9092377343575,122.597783200167)) ;
#17570=CARTESIAN_POINT('Ctrl Pts',(-18.460683489093,12.9092389481594,122.597763145753)) ;
#17571=CARTESIAN_POINT('Ctrl Pts',(-18.4607180237009,12.9092413838026,122.597722905362)) ;
#17572=CARTESIAN_POINT('Ctrl Pts',(-18.4607353489293,12.9092426056691,122.597702718976)) ;
#17573=CARTESIAN_POINT('Ctrl Pts',(-18.4607701171478,12.9092450576265,122.597662211611)) ;
#17574=CARTESIAN_POINT('Ctrl Pts',(-18.4607875597353,12.9092462876885,122.597641891119)) ;
#17575=CARTESIAN_POINT('Ctrl Pts',(-18.4608225632399,12.909248756075,122.597601114933)) ;
#17576=CARTESIAN_POINT('Ctrl Pts',(-18.4608401243544,12.9092499944131,122.597580659026)) ;
#17577=CARTESIAN_POINT('Ctrl Pts',(-18.4608753667552,12.9092524794801,122.59753960992)) ;
#17578=CARTESIAN_POINT('Ctrl Pts',(-18.4608930480052,12.909253726206,122.59751901678)) ;
#17579=CARTESIAN_POINT('Ctrl Pts',(-18.460928531824,12.9092562281279,122.597477691926)) ;
#17580=CARTESIAN_POINT('Ctrl Pts',(-18.4609463345614,12.9092574833353,122.597456960033)) ;
#17581=CARTESIAN_POINT('Ctrl Pts',(-18.4609820631147,12.9092600023425,122.597415355679)) ;
#17582=CARTESIAN_POINT('Ctrl Pts',(-18.4609999889301,12.9092612661418,122.597394483237)) ;
#17583=CARTESIAN_POINT('Ctrl Pts',(-18.4610359650053,12.9092638024274,122.597352596251)) ;
#17584=CARTESIAN_POINT('Ctrl Pts',(-18.4610540153673,12.9092650749203,122.597331581607)) ;
#17585=CARTESIAN_POINT('Ctrl Pts',(-18.4610902420817,12.9092676287005,122.597289408474)) ;
#17586=CARTESIAN_POINT('Ctrl Pts',(-18.4611084184928,12.9092689099912,122.597268249937)) ;
#17587=CARTESIAN_POINT('Ctrl Pts',(-18.4611448989465,12.9092714814809,122.597225787166)) ;
#17588=CARTESIAN_POINT('Ctrl Pts',(-18.4611632029019,12.909272771673,122.597204483055)) ;
#17589=CARTESIAN_POINT('Ctrl Pts',(-18.4611999407044,12.9092753611229,122.597161726565)) ;
#17590=CARTESIAN_POINT('Ctrl Pts',(-18.461218374137,12.9092766603507,122.59714027469)) ;
#17591=CARTESIAN_POINT('Ctrl Pts',(-18.4612553713637,12.9092792679033,122.597097222188)) ;
#17592=CARTESIAN_POINT('Ctrl Pts',(-18.4612739354962,12.9092805762512,122.597075621188)) ;
#17593=CARTESIAN_POINT('Ctrl Pts',(-18.4613111963032,12.9092832021956,122.597032267961)) ;
#17594=CARTESIAN_POINT('Ctrl Pts',(-18.4613298929496,12.9092845197895,122.597010515788)) ;
#17595=CARTESIAN_POINT('Ctrl Pts',(-18.4613674200902,12.9092871643158,122.59696685876)) ;
#17596=CARTESIAN_POINT('Ctrl Pts',(-18.4613862507815,12.9092884912615,122.596944953698)) ;
#17597=CARTESIAN_POINT('Ctrl Pts',(-18.4614240476814,12.9092911546072,122.596900989013)) ;
#17598=CARTESIAN_POINT('Ctrl Pts',(-18.4614430139965,12.909292491014,122.596878929289)) ;
#17599=CARTESIAN_POINT('Ctrl Pts',(-18.4614810843628,12.9092951734362,122.596834652767)) ;
#17600=CARTESIAN_POINT('Ctrl Pts',(-18.4615001881808,12.9092965194344,122.596812436262)) ;
#17601=CARTESIAN_POINT('Ctrl Pts',(-18.4615385348547,12.9092992211292,122.596767844733)) ;
#17602=CARTESIAN_POINT('Ctrl Pts',(-18.4615577777627,12.9093005768286,122.596745469671)) ;
#17603=CARTESIAN_POINT('Ctrl Pts',(-18.4615964045957,12.9093032980631,122.596700558792)) ;
#17604=CARTESIAN_POINT('Ctrl Pts',(-18.4616157885023,12.909304663596,122.596678023022)) ;
#17605=CARTESIAN_POINT('Ctrl Pts',(-18.4616546980943,12.909307404549,122.596632789911)) ;
#17606=CARTESIAN_POINT('Ctrl Pts',(-18.4616742242616,12.9093087800022,122.596610092035)) ;
#17607=CARTESIAN_POINT('Ctrl Pts',(-18.4617134215183,12.9093115410149,122.596564531132)) ;
#17608=CARTESIAN_POINT('Ctrl Pts',(-18.4617330921166,12.9093129265391,122.5965416687)) ;
#17609=CARTESIAN_POINT('Ctrl Pts',(-18.4674875411176,12.9097182335068,122.589853968253)) ;
#17610=CARTESIAN_POINT('Ctrl Pts',(-18.473292462641,12.9101227053002,122.583249842278)) ;
#17611=CARTESIAN_POINT('Ctrl Pts',(-18.4872082049094,12.9110821196766,122.567751093745)) ;
#17612=CARTESIAN_POINT('Ctrl Pts',(-18.495378772698,12.9116374674313,122.558911311203)) ;
#17613=CARTESIAN_POINT('Ctrl Pts',(-18.5255320502739,12.9136583732359,122.527219155736)) ;
#17614=CARTESIAN_POINT('Ctrl Pts',(-18.5482545240481,12.9151279126444,122.505087344132)) ;
#17615=CARTESIAN_POINT('Ctrl Pts',(-18.5834615782862,12.9173213746547,122.473313552973)) ;
#17616=CARTESIAN_POINT('Ctrl Pts',(-18.5953270213179,12.9180472819376,122.463004474182)) ;
#17617=CARTESIAN_POINT('Ctrl Pts',(-18.6111133294123,12.9189944941176,122.449802933513)) ;
#17618=CARTESIAN_POINT('Ctrl Pts',(-18.6148610700442,12.9192180186811,122.44670580419)) ;
#17619=CARTESIAN_POINT('Ctrl Pts',(-18.6199527977924,12.9195198879582,122.442547759573)) ;
#17620=CARTESIAN_POINT('Ctrl Pts',(-18.6212810162356,12.9195984690759,122.441467640624)) ;
#17621=CARTESIAN_POINT('Ctrl Pts',(-18.623556650964,12.9197328262149,122.439624828017)) ;
#17622=CARTESIAN_POINT('Ctrl Pts',(-18.6245029685735,12.9197886170874,122.43886078271)) ;
#17623=CARTESIAN_POINT('Ctrl Pts',(-18.6276810450864,12.9199757136843,122.436302495557)) ;
#17624=CARTESIAN_POINT('Ctrl Pts',(-18.6299178563148,12.9201069525261,122.434514539952)) ;
#17625=CARTESIAN_POINT('Ctrl Pts',(-18.6356317807976,12.9204411004961,122.429979307164)) ;
#17626=CARTESIAN_POINT('Ctrl Pts',(-18.6391173987332,12.9206439058288,122.427242802604)) ;
#17627=CARTESIAN_POINT('Ctrl Pts',(-18.6544951624273,12.9215342969607,122.415301588195)) ;
#17628=CARTESIAN_POINT('Ctrl Pts',(-18.6665383447217,12.9222202964339,122.406293348238)) ;
#17629=CARTESIAN_POINT('Ctrl Pts',(-18.7059019576485,12.9244311582386,122.377942697902)) ;
#17630=CARTESIAN_POINT('Ctrl Pts',(-18.7338374985042,12.9259529893569,122.359479681101)) ;
#17631=CARTESIAN_POINT('Ctrl Pts',(-18.7750620373161,12.9281503928211,122.334552279372)) ;
#17632=CARTESIAN_POINT('Ctrl Pts',(-18.7877770182112,12.9288217515954,122.327167017206)) ;
#17633=CARTESIAN_POINT('Ctrl Pts',(-18.8072714322977,12.9298425449056,122.316299402806)) ;
#17634=CARTESIAN_POINT('Ctrl Pts',(-18.8139573259136,12.930191145774,122.312651884988)) ;
#17635=CARTESIAN_POINT('Ctrl Pts',(-18.8259528867814,12.9308140718044,122.30624921072)) ;
#17636=CARTESIAN_POINT('Ctrl Pts',(-18.8312497904658,12.9310882719835,122.303470634121)) ;
#17637=CARTESIAN_POINT('Ctrl Pts',(-18.8366485738281,12.9313669002543,122.300687843529)) ;
#17638=CARTESIAN_POINT('Ctrl Pts',(-18.8367307270997,12.9313711399417,122.300645509344)) ;
#17639=CARTESIAN_POINT('Ctrl Pts',(-18.8368947521112,12.931379604392,122.300561009068)) ;
#17640=CARTESIAN_POINT('Ctrl Pts',(-18.8369766237777,12.9313838291524,122.300518842934)) ;
#17641=CARTESIAN_POINT('Ctrl Pts',(-18.837140121316,12.9313922655971,122.300434660116)) ;
#17642=CARTESIAN_POINT('Ctrl Pts',(-18.8372217471904,12.9313964772827,122.30039264336)) ;
#17643=CARTESIAN_POINT('Ctrl Pts',(-18.8373847881378,12.9314048893872,122.300308741077)) ;
#17644=CARTESIAN_POINT('Ctrl Pts',(-18.837466203088,12.9314090898007,122.300266855552)) ;
#17645=CARTESIAN_POINT('Ctrl Pts',(-18.8376288558034,12.9314174810986,122.300183198257)) ;
#17646=CARTESIAN_POINT('Ctrl Pts',(-18.8377100935985,12.9314216719854,122.300141426421)) ;
#17647=CARTESIAN_POINT('Ctrl Pts',(-18.8378724244463,12.9314300459062,122.300057979671)) ;
#17648=CARTESIAN_POINT('Ctrl Pts',(-18.8379535176861,12.9314342289506,122.300016304618)) ;
#17649=CARTESIAN_POINT('Ctrl Pts',(-18.8381155922966,12.9314425888847,122.29993303442)) ;
#17650=CARTESIAN_POINT('Ctrl Pts',(-18.838196573277,12.9314467657548,122.299891439441)) ;
#17651=CARTESIAN_POINT('Ctrl Pts',(-18.8383584540782,12.931455114926,122.299808313518)) ;
#17652=CARTESIAN_POINT('Ctrl Pts',(-18.8384393538655,12.9314592872258,122.299766782567)) ;
#17653=CARTESIAN_POINT('Ctrl Pts',(-18.838601103016,12.931467628843,122.299683768853)) ;
#17654=CARTESIAN_POINT('Ctrl Pts',(-18.8386819522676,12.9314717981549,122.29964228613)) ;
#17655=CARTESIAN_POINT('Ctrl Pts',(-18.8388436296266,12.9314801353072,122.299559353803)) ;
#17656=CARTESIAN_POINT('Ctrl Pts',(-18.8389244580086,12.9314843031619,122.29951790405)) ;
#17657=CARTESIAN_POINT('Ctrl Pts',(-18.8390861230783,12.9314926389188,122.29943502254)) ;
#17658=CARTESIAN_POINT('Ctrl Pts',(-18.8391669598491,12.9314968068253,122.29939359074)) ;
#17659=CARTESIAN_POINT('Ctrl Pts',(-18.8393286708288,12.9315051441881,122.299310730208)) ;
#17660=CARTESIAN_POINT('Ctrl Pts',(-18.83940954489,12.9315093136366,122.299269301559)) ;
#17661=CARTESIAN_POINT('Ctrl Pts',(-18.8395713582431,12.931517655516,122.29918643312)) ;
#17662=CARTESIAN_POINT('Ctrl Pts',(-18.8396522976801,12.931521827954,122.29914499327)) ;
#17663=CARTESIAN_POINT('Ctrl Pts',(-18.8398142699771,12.931530177265,122.299062088046)) ;
#17664=CARTESIAN_POINT('Ctrl Pts',(-18.8398953027382,12.9315343541325,122.299020622745)) ;
#17665=CARTESIAN_POINT('Ctrl Pts',(-18.8400574889383,12.9315427137062,122.298937652743)) ;
#17666=CARTESIAN_POINT('Ctrl Pts',(-18.8401386424167,12.9315468964139,122.298896148054)) ;
#17667=CARTESIAN_POINT('Ctrl Pts',(-18.8403010971093,12.9315552690612,122.298813085534)) ;
#17668=CARTESIAN_POINT('Ctrl Pts',(-18.8403823983439,12.9315594590012,122.298771527731)) ;
#17669=CARTESIAN_POINT('Ctrl Pts',(-18.8405451757876,12.931567847515,122.29868834518)) ;
#17670=CARTESIAN_POINT('Ctrl Pts',(-18.8406266518086,12.9315720460783,122.298646720574)) ;
#17671=CARTESIAN_POINT('Ctrl Pts',(-18.8407898045557,12.9315804531624,122.298563391411)) ;
#17672=CARTESIAN_POINT('Ctrl Pts',(-18.8408714815939,12.9315846616984,122.298521686749)) ;
#17673=CARTESIAN_POINT('Ctrl Pts',(-18.8410350633922,12.9315930901173,122.298438183843)) ;
#17674=CARTESIAN_POINT('Ctrl Pts',(-18.841116967973,12.93159730999,122.298396385751)) ;
#17675=CARTESIAN_POINT('Ctrl Pts',(-18.8412810308414,12.9316057624182,122.298312682912)) ;
#17676=CARTESIAN_POINT('Ctrl Pts',(-18.8413631890634,12.9316099949692,122.298270778265)) ;
#17677=CARTESIAN_POINT('Ctrl Pts',(-18.8415277853316,12.931618474096,122.298186849202)) ;
#17678=CARTESIAN_POINT('Ctrl Pts',(-18.8416102233135,12.9316227206673,122.298144824894)) ;
#17679=CARTESIAN_POINT('Ctrl Pts',(-18.8417754043808,12.9316312291333,122.298060643852)) ;
#17680=CARTESIAN_POINT('Ctrl Pts',(-18.841858147757,12.9316354910416,122.298018487053)) ;
#17681=CARTESIAN_POINT('Ctrl Pts',(-18.8420239660036,12.9316440315367,122.297934027836)) ;
#17682=CARTESIAN_POINT('Ctrl Pts',(-18.8421070407767,12.931648310117,122.297891725558)) ;
#17683=CARTESIAN_POINT('Ctrl Pts',(-18.8422735472217,12.9316568852601,122.297806962722)) ;
#17684=CARTESIAN_POINT('Ctrl Pts',(-18.8423569790373,12.9316611818287,122.297764502188)) ;
#17685=CARTESIAN_POINT('Ctrl Pts',(-18.8425242254762,12.9316697942777,122.297679409955)) ;
#17686=CARTESIAN_POINT('Ctrl Pts',(-18.8426080401333,12.9316741101582,122.297636778343)) ;
#17687=CARTESIAN_POINT('Ctrl Pts',(-18.8427760776543,12.9316827625335,122.297551331354)) ;
#17688=CARTESIAN_POINT('Ctrl Pts',(-18.8428603007136,12.9316870990366,122.297508515991)) ;
#17689=CARTESIAN_POINT('Ctrl Pts',(-18.8430291814528,12.9316957940116,122.297422688417)) ;
#17690=CARTESIAN_POINT('Ctrl Pts',(-18.8431138389162,12.9317001524703,122.297379676438)) ;
#17691=CARTESIAN_POINT('Ctrl Pts',(-18.8432836139418,12.9317088926623,122.297293443054)) ;
#17692=CARTESIAN_POINT('Ctrl Pts',(-18.8433687315986,12.9317132743982,122.297250221731)) ;
#17693=CARTESIAN_POINT('Ctrl Pts',(-18.8435394526221,12.9317220624565,122.297163557048)) ;
#17694=CARTESIAN_POINT('Ctrl Pts',(-18.843625056254,12.9317264687902,122.297120113691)) ;
#17695=CARTESIAN_POINT('Ctrl Pts',(-18.8437967757305,12.9317353074015,122.297032991906)) ;
#17696=CARTESIAN_POINT('Ctrl Pts',(-18.8438828915313,12.9317397396743,122.296989313646)) ;
#17697=CARTESIAN_POINT('Ctrl Pts',(-18.8440556613335,12.931748631494,122.296901709317)) ;
#17698=CARTESIAN_POINT('Ctrl Pts',(-18.8441423154511,12.9317530910443,122.296857783343)) ;
#17699=CARTESIAN_POINT('Ctrl Pts',(-18.84431618814,12.9317620387624,122.296769670745)) ;
#17700=CARTESIAN_POINT('Ctrl Pts',(-18.8444034068392,12.9317665269339,122.296725484219)) ;
#17701=CARTESIAN_POINT('Ctrl Pts',(-18.8445784358176,12.9317755332823,122.296636837266)) ;
#17702=CARTESIAN_POINT('Ctrl Pts',(-18.8446662459436,12.9317800514484,122.296592377089)) ;
#17703=CARTESIAN_POINT('Ctrl Pts',(-18.8448424835274,12.9317891191021,122.296503170317)) ;
#17704=CARTESIAN_POINT('Ctrl Pts',(-18.844930911437,12.93179366861,122.296458423674)) ;
#17705=CARTESIAN_POINT('Ctrl Pts',(-18.8451084126807,12.9318028003837,122.2963686303)) ;
#17706=CARTESIAN_POINT('Ctrl Pts',(-18.8451974857573,12.9318073826331,122.29632358389)) ;
#17707=CARTESIAN_POINT('Ctrl Pts',(-18.8453283074218,12.9318141122521,122.296257443886)) ;
#17708=CARTESIAN_POINT('Ctrl Pts',(-18.8453700518626,12.9318162595851,122.296236341932)) ;
#17709=CARTESIAN_POINT('Ctrl Pts',(-18.845454195118,12.9318205878119,122.296193813167)) ;
#17710=CARTESIAN_POINT('Ctrl Pts',(-18.8454965939828,12.9318227687067,122.296172386423)) ;
#17711=CARTESIAN_POINT('Ctrl Pts',(-18.845582071843,12.9318271653772,122.29612919534)) ;
#17712=CARTESIAN_POINT('Ctrl Pts',(-18.8456251512476,12.9318293811723,122.296107430891)) ;
#17713=CARTESIAN_POINT('Ctrl Pts',(-18.8457120188534,12.9318338491129,122.296063550215)) ;
#17714=CARTESIAN_POINT('Ctrl Pts',(-18.8457558066999,12.9318361012385,122.296041434268)) ;
#17715=CARTESIAN_POINT('Ctrl Pts',(-18.8458441192737,12.9318406432791,122.295996836724)) ;
#17716=CARTESIAN_POINT('Ctrl Pts',(-18.8458886440798,12.9318429331964,122.295974355195)) ;
#17717=CARTESIAN_POINT('Ctrl Pts',(-18.8459784598595,12.9318475523212,122.29592901203)) ;
#17718=CARTESIAN_POINT('Ctrl Pts',(-18.8460237511192,12.9318498815415,122.295906150365)) ;
#17719=CARTESIAN_POINT('Ctrl Pts',(-18.8461151315823,12.9318545809005,122.295860031236)) ;
#17720=CARTESIAN_POINT('Ctrl Pts',(-18.8461612205627,12.9318569510258,122.295836774008)) ;
#17721=CARTESIAN_POINT('Ctrl Pts',(-18.8462542277535,12.9318617337975,122.295789848339)) ;
#17722=CARTESIAN_POINT('Ctrl Pts',(-18.8463011462655,12.9318641464572,122.295766179875)) ;
#17723=CARTESIAN_POINT('Ctrl Pts',(-18.8463958472504,12.9318690160772,122.295718414605)) ;
#17724=CARTESIAN_POINT('Ctrl Pts',(-18.8464436293148,12.9318714730142,122.295694318142)) ;
#17725=CARTESIAN_POINT('Ctrl Pts',(-18.846540091158,12.9318764329172,122.295645680271)) ;
#17726=CARTESIAN_POINT('Ctrl Pts',(-18.8465887713337,12.9318789359012,122.295621138807)) ;
#17727=CARTESIAN_POINT('Ctrl Pts',(-18.8466870664997,12.9318839897986,122.295571592669)) ;
#17728=CARTESIAN_POINT('Ctrl Pts',(-18.8467366814487,12.9318865407072,122.29554658817)) ;
#17729=CARTESIAN_POINT('Ctrl Pts',(-18.8468368836946,12.9318916923757,122.295496097515)) ;
#17730=CARTESIAN_POINT('Ctrl Pts',(-18.8468874712014,12.9318942931435,122.295470611416)) ;
#17731=CARTESIAN_POINT('Ctrl Pts',(-18.8469896591545,12.931899546609,122.295419137605)) ;
#17732=CARTESIAN_POINT('Ctrl Pts',(-18.8470412593468,12.9319021992906,122.295393150196)) ;
#17733=CARTESIAN_POINT('Ctrl Pts',(-18.847145512571,12.931907558626,122.295340654195)) ;
#17734=CARTESIAN_POINT('Ctrl Pts',(-18.8471981662542,12.9319102653101,122.295314145461)) ;
#17735=CARTESIAN_POINT('Ctrl Pts',(-18.8473045713181,12.9319157349471,122.295260584787)) ;
#17736=CARTESIAN_POINT('Ctrl Pts',(-18.8473583223143,12.9319184978769,122.295233533236)) ;
#17737=CARTESIAN_POINT('Ctrl Pts',(-18.847466966332,12.9319240822737,122.295178865213)) ;
#17738=CARTESIAN_POINT('Ctrl Pts',(-18.847521859613,12.9319269037506,122.295151248819)) ;
#17739=CARTESIAN_POINT('Ctrl Pts',(-18.8476328359797,12.931932607687,122.295095427702)) ;
#17740=CARTESIAN_POINT('Ctrl Pts',(-18.8476889190898,12.931935490144,122.295067223189)) ;
#17741=CARTESIAN_POINT('Ctrl Pts',(-18.8478023237632,12.9319413185296,122.295010202041)) ;
#17742=CARTESIAN_POINT('Ctrl Pts',(-18.8478596458301,12.9319442644802,122.294981385388)) ;
#17743=CARTESIAN_POINT('Ctrl Pts',(-18.8479755811761,12.9319502225524,122.294923114152)) ;
#17744=CARTESIAN_POINT('Ctrl Pts',(-18.8480341942732,12.9319532346606,122.294893659911)) ;
#17745=CARTESIAN_POINT('Ctrl Pts',(-18.8481527658151,12.9319593278172,122.294834087056)) ;
#17746=CARTESIAN_POINT('Ctrl Pts',(-18.8482127241924,12.9319624088578,122.294803968743)) ;
#17747=CARTESIAN_POINT('Ctrl Pts',(-18.8483340431089,12.9319686427852,122.294743040015)) ;
#17748=CARTESIAN_POINT('Ctrl Pts',(-18.8483954036568,12.9319717956678,122.29471222988)) ;
#17749=CARTESIAN_POINT('Ctrl Pts',(-18.8485195862066,12.9319781763113,122.294649888603)) ;
#17750=CARTESIAN_POINT('Ctrl Pts',(-18.8485824084158,12.9319814040778,122.294618357659)) ;
#17751=CARTESIAN_POINT('Ctrl Pts',(-18.8487095769781,12.9319879376948,122.294554544222)) ;
#17752=CARTESIAN_POINT('Ctrl Pts',(-18.848773923437,12.9319912435453,122.294522261999)) ;
#17753=CARTESIAN_POINT('Ctrl Pts',(-18.8489042056603,12.9319979366616,122.294456914295)) ;
#17754=CARTESIAN_POINT('Ctrl Pts',(-18.8489701417443,12.9320013239379,122.294423849)) ;
#17755=CARTESIAN_POINT('Ctrl Pts',(-18.8491036725522,12.9320081834502,122.294356901436)) ;
#17756=CARTESIAN_POINT('Ctrl Pts',(-18.8491712672356,12.9320116556778,122.294323019558)) ;
#17757=CARTESIAN_POINT('Ctrl Pts',(-18.8493081872479,12.9320186887725,122.294254403857)) ;
#17758=CARTESIAN_POINT('Ctrl Pts',(-18.8493775127453,12.9320222496417,122.294219670347)) ;
#17759=CARTESIAN_POINT('Ctrl Pts',(-18.8495179701918,12.9320294638932,122.294149314607)) ;
#17760=CARTESIAN_POINT('Ctrl Pts',(-18.8495891023662,12.93203311728,122.294113692688)) ;
#17761=CARTESIAN_POINT('Ctrl Pts',(-18.849733252841,12.9320405206374,122.294041521519)) ;
#17762=CARTESIAN_POINT('Ctrl Pts',(-18.84980627137,12.9320442706121,122.294004972608)) ;
#17763=CARTESIAN_POINT('Ctrl Pts',(-18.8499542789408,12.9320518714562,122.293930906596)) ;
#17764=CARTESIAN_POINT('Ctrl Pts',(-18.8500292679488,12.9320557223156,122.293893389999)) ;
#17765=CARTESIAN_POINT('Ctrl Pts',(-18.8501813037246,12.9320635293847,122.293817346445)) ;
#17766=CARTESIAN_POINT('Ctrl Pts',(-18.8502583510448,12.932067485614,122.293778819734)) ;
#17767=CARTESIAN_POINT('Ctrl Pts',(-18.8504145971473,12.9320755082078,122.293700710685)) ;
#17768=CARTESIAN_POINT('Ctrl Pts',(-18.8504937958913,12.9320795745609,122.293661128928)) ;
#17769=CARTESIAN_POINT('Ctrl Pts',(-18.8506544420563,12.9320878223653,122.293580862905)) ;
#17770=CARTESIAN_POINT('Ctrl Pts',(-18.8507358897974,12.9320920038229,122.293540179083)) ;
#17771=CARTESIAN_POINT('Ctrl Pts',(-18.8509011369854,12.9321004870952,122.293457659299)) ;
#17772=CARTESIAN_POINT('Ctrl Pts',(-18.8509849366996,12.9321047889128,122.293415823852)) ;
#17773=CARTESIAN_POINT('Ctrl Pts',(-18.8511549958087,12.9321135184149,122.293330948885)) ;
#17774=CARTESIAN_POINT('Ctrl Pts',(-18.8512412556717,12.9321179461119,122.29328790983)) ;
#17775=CARTESIAN_POINT('Ctrl Pts',(-18.8514163501207,12.9321269332427,122.293200572365)) ;
#17776=CARTESIAN_POINT('Ctrl Pts',(-18.8515051846889,12.932131492663,122.293156274718)) ;
#17777=CARTESIAN_POINT('Ctrl Pts',(-18.8516855484862,12.9321407493585,122.293066362546)) ;
#17778=CARTESIAN_POINT('Ctrl Pts',(-18.8517770781079,12.9321454466401,122.293020748638)) ;
#17779=CARTESIAN_POINT('Ctrl Pts',(-18.851962958982,12.9321549855332,122.292928143131)) ;
#17780=CARTESIAN_POINT('Ctrl Pts',(-18.8520573107043,12.9321598271542,122.292881152174)) ;
#17781=CARTESIAN_POINT('Ctrl Pts',(-18.8522489698198,12.93216966156,122.292785728469)) ;
#17782=CARTESIAN_POINT('Ctrl Pts',(-18.8523462776524,12.9321746543516,122.292737296447)) ;
#17783=CARTESIAN_POINT('Ctrl Pts',(-18.8525439910054,12.9321847983378,122.292638922798)) ;
#17784=CARTESIAN_POINT('Ctrl Pts',(-18.8526443967264,12.9321899495258,122.292588982091)) ;
#17785=CARTESIAN_POINT('Ctrl Pts',(-18.8528484545785,12.9322004178831,122.292487520199)) ;
#17786=CARTESIAN_POINT('Ctrl Pts',(-18.8529521074033,12.9322057350698,122.292435999771)) ;
#17787=CARTESIAN_POINT('Ctrl Pts',(-18.853162817694,12.932216543486,122.292331303142)) ;
#17788=CARTESIAN_POINT('Ctrl Pts',(-18.8532698755792,12.9322220347172,122.292278127926)) ;
#17789=CARTESIAN_POINT('Ctrl Pts',(-18.8534875630272,12.9322331997299,122.292170042383)) ;
#17790=CARTESIAN_POINT('Ctrl Pts',(-18.8535981929083,12.9322388735062,122.292115133191)) ;
#17791=CARTESIAN_POINT('Ctrl Pts',(-18.8538232005821,12.9322504125824,122.292003496157)) ;
#17792=CARTESIAN_POINT('Ctrl Pts',(-18.8539375788908,12.9322562778855,122.291946769461)) ;
#17793=CARTESIAN_POINT('Ctrl Pts',(-18.8541702693955,12.9322682094813,122.291831409446)) ;
#17794=CARTESIAN_POINT('Ctrl Pts',(-18.8542885824548,12.9322742757931,122.29177277722)) ;
#17795=CARTESIAN_POINT('Ctrl Pts',(-18.8545293401758,12.9322866194675,122.29165351279)) ;
#17796=CARTESIAN_POINT('Ctrl Pts',(-18.8546517854035,12.9322928968316,122.291592881956)) ;
#17797=CARTESIAN_POINT('Ctrl Pts',(-18.8549010162086,12.9323056732292,122.291469521972)) ;
#17798=CARTESIAN_POINT('Ctrl Pts',(-18.8550278024044,12.9323121722647,122.29140679431)) ;
#17799=CARTESIAN_POINT('Ctrl Pts',(-18.8552859360825,12.9323254032399,122.291279136819)) ;
#17800=CARTESIAN_POINT('Ctrl Pts',(-18.8554172842975,12.9323321351848,122.291214208582)) ;
#17801=CARTESIAN_POINT('Ctrl Pts',(-18.8556847757652,12.9323458438613,122.291082040335)) ;
#17802=CARTESIAN_POINT('Ctrl Pts',(-18.8558209199634,12.932352820606,122.291014801985)) ;
#17803=CARTESIAN_POINT('Ctrl Pts',(-18.8560982512303,12.9323670314755,122.290877897584)) ;
#17804=CARTESIAN_POINT('Ctrl Pts',(-18.8562394392617,12.9323742656111,122.290808233376)) ;
#17805=CARTESIAN_POINT('Ctrl Pts',(-18.8565271208855,12.9323890046059,122.290666354694)) ;
#17806=CARTESIAN_POINT('Ctrl Pts',(-18.856673615425,12.9323965094716,122.290594142281)) ;
#17807=CARTESIAN_POINT('Ctrl Pts',(-18.8569721882283,12.93241180405,122.290447037766)) ;
#17808=CARTESIAN_POINT('Ctrl Pts',(-18.8571242675855,12.9324195937729,122.290372147883)) ;
#17809=CARTESIAN_POINT('Ctrl Pts',(-18.8574343049127,12.9324354730321,122.290219551611)) ;
#17810=CARTESIAN_POINT('Ctrl Pts',(-18.857592264099,12.9324435625807,122.290141847635)) ;
#17811=CARTESIAN_POINT('Ctrl Pts',(-18.8579143741494,12.9324600573732,122.289983478348)) ;
#17812=CARTESIAN_POINT('Ctrl Pts',(-18.8580785261881,12.9324684626227,122.289902815753)) ;
#17813=CARTESIAN_POINT('Ctrl Pts',(-18.8584133532803,12.9324856056179,122.289738376444)) ;
#17814=CARTESIAN_POINT('Ctrl Pts',(-18.858584029907,12.9324943433845,122.289654602562)) ;
#17815=CARTESIAN_POINT('Ctrl Pts',(-18.8589322584015,12.9325121692658,122.289483778775)) ;
#17816=CARTESIAN_POINT('Ctrl Pts',(-18.8591098118056,12.9325212573938,122.289396732065)) ;
#17817=CARTESIAN_POINT('Ctrl Pts',(-18.8594721673803,12.9325398029194,122.289219191528)) ;
#17818=CARTESIAN_POINT('Ctrl Pts',(-18.8596569712518,12.9325492603327,122.289128701196)) ;
#17819=CARTESIAN_POINT('Ctrl Pts',(-18.8600342243982,12.9325685645106,122.288944092386)) ;
#17820=CARTESIAN_POINT('Ctrl Pts',(-18.8602266754899,12.93257841129,122.288849977767)) ;
#17821=CARTESIAN_POINT('Ctrl Pts',(-18.8606196441781,12.9325985155088,122.288657928924)) ;
#17822=CARTESIAN_POINT('Ctrl Pts',(-18.8608201637914,12.9326087729655,122.288559998927)) ;
#17823=CARTESIAN_POINT('Ctrl Pts',(-18.8704120783376,12.933099389029,122.283878669612)) ;
#17824=CARTESIAN_POINT('Ctrl Pts',(-18.8798605336001,12.9335802702349,122.279413176892)) ;
#17825=CARTESIAN_POINT('Ctrl Pts',(-18.9068396207035,12.9349468081373,122.267073891715)) ;
#17826=CARTESIAN_POINT('Ctrl Pts',(-18.9244973367847,12.9358334611394,122.259485168479)) ;
#17827=CARTESIAN_POINT('Ctrl Pts',(-19.0120424708204,12.9401914228891,122.22422957043)) ;
#17828=CARTESIAN_POINT('Ctrl Pts',(-19.084152996879,12.9436502135292,122.202497728059)) ;
#17829=CARTESIAN_POINT('Ctrl Pts',(-19.1798876361204,12.9481446493443,122.182834225966)) ;
#17830=CARTESIAN_POINT('Ctrl Pts',(-19.2021167447081,12.9491817115664,122.178892597979)) ;
#17831=CARTESIAN_POINT('Ctrl Pts',(-19.2357943629815,12.9507444199954,122.173857492605)) ;
#17832=CARTESIAN_POINT('Ctrl Pts',(-19.2471711954837,12.951270874863,122.172316465083)) ;
#17833=CARTESIAN_POINT('Ctrl Pts',(-19.2684751569415,12.9522541226503,122.169729108203)) ;
#17834=CARTESIAN_POINT('Ctrl Pts',(-19.2783967332762,12.9527109950239,122.168644543059)) ;
#17835=CARTESIAN_POINT('Ctrl Pts',(-19.3008372961763,12.9537420636157,122.166463103544)) ;
#17836=CARTESIAN_POINT('Ctrl Pts',(-19.313362005199,12.9543159331095,122.165435959296)) ;
#17837=CARTESIAN_POINT('Ctrl Pts',(-19.3537240736603,12.9561602188178,122.162737893979)) ;
#17838=CARTESIAN_POINT('Ctrl Pts',(-19.3816027879756,12.9574264055357,122.161809539956)) ;
#17839=CARTESIAN_POINT('Ctrl Pts',(-19.4512552245047,12.9605698802966,122.161821642425)) ;
#17840=CARTESIAN_POINT('Ctrl Pts',(-19.4929943814269,12.962434938441,122.16392214131)) ;
#17841=CARTESIAN_POINT('Ctrl Pts',(-19.5589099914151,12.9654189939075,122.170561787472)) ;
#17842=CARTESIAN_POINT('Ctrl Pts',(-19.5831921538476,12.9665262986323,122.173730662339)) ;
#17843=CARTESIAN_POINT('Ctrl Pts',(-19.6132613713239,12.9679136321864,122.178556854359)) ;
#17844=CARTESIAN_POINT('Ctrl Pts',(-19.6191505208534,12.968186107096,122.17954541711)) ;
#17845=CARTESIAN_POINT('Ctrl Pts',(-19.628474040098,12.9686187602559,122.181179254851)) ;
#17846=CARTESIAN_POINT('Ctrl Pts',(-19.6319131883064,12.9687786286577,122.181796799472)) ;
#17847=CARTESIAN_POINT('Ctrl Pts',(-19.6383363147696,12.9690777377784,122.18297797818)) ;
#17848=CARTESIAN_POINT('Ctrl Pts',(-19.6413209177538,12.9692169380229,122.183538082161)) ;
#17849=CARTESIAN_POINT('Ctrl Pts',(-19.6480727531287,12.9695323353698,122.184830649697)) ;
#17850=CARTESIAN_POINT('Ctrl Pts',(-19.6518387094439,12.9697086037091,122.185569597253)) ;
#17851=CARTESIAN_POINT('Ctrl Pts',(-19.6628268223413,12.9702239522019,122.187778259695)) ;
#17852=CARTESIAN_POINT('Ctrl Pts',(-19.670039430323,12.9705635458441,122.189294514544)) ;
#17853=CARTESIAN_POINT('Ctrl Pts',(-19.7000703661138,12.9719831286628,122.195885557967)) ;
#17854=CARTESIAN_POINT('Ctrl Pts',(-19.7227571849713,12.9730693314094,122.20153605961)) ;
#17855=CARTESIAN_POINT('Ctrl Pts',(-19.8094878681108,12.9772723613184,122.225740049305)) ;
#17856=CARTESIAN_POINT('Ctrl Pts',(-19.872169205209,12.9804045347924,122.248770262787)) ;
#17857=CARTESIAN_POINT('Ctrl Pts',(-19.9534618610653,12.9845532872059,122.286256883173)) ;
#17858=CARTESIAN_POINT('Ctrl Pts',(-19.9739433774441,12.9856084637886,122.296391346827)) ;
#17859=CARTESIAN_POINT('Ctrl Pts',(-20.0017133809356,12.9870552141847,122.311093237271)) ;
#17860=CARTESIAN_POINT('Ctrl Pts',(-20.0092495684584,12.987449501757,122.315182835022)) ;
#17861=CARTESIAN_POINT('Ctrl Pts',(-20.0221058496954,12.9881251632742,122.322331639189)) ;
#17862=CARTESIAN_POINT('Ctrl Pts',(-20.0274465779288,12.9884067549695,122.325353076606)) ;
#17863=CARTESIAN_POINT('Ctrl Pts',(-20.0379365902499,12.9889617089518,122.331390035552)) ;
#17864=CARTESIAN_POINT('Ctrl Pts',(-20.0430869601818,12.9892350770928,122.33440334889)) ;
#17865=CARTESIAN_POINT('Ctrl Pts',(-20.0535780213267,12.9897938183034,122.340642586843)) ;
#17866=CARTESIAN_POINT('Ctrl Pts',(-20.0589165353511,12.9900791625694,122.343871853466)) ;
#17867=CARTESIAN_POINT('Ctrl Pts',(-20.0710288206462,12.9907289793603,122.351323005343)) ;
#17868=CARTESIAN_POINT('Ctrl Pts',(-20.0777867885088,12.9910932811806,122.35557007748)) ;
#17869=CARTESIAN_POINT('Ctrl Pts',(-20.0948774979195,12.9920192198657,122.366540534747)) ;
#17870=CARTESIAN_POINT('Ctrl Pts',(-20.1051523315045,12.9925802556669,122.373352593796)) ;
#17871=CARTESIAN_POINT('Ctrl Pts',(-20.134259171672,12.9941829003336,122.393275988063)) ;
#17872=CARTESIAN_POINT('Ctrl Pts',(-20.1528332651535,12.9952219042424,122.406755415464)) ;
#17873=CARTESIAN_POINT('Ctrl Pts',(-20.1953433956368,12.997642355661,122.439429249522)) ;
#17874=CARTESIAN_POINT('Ctrl Pts',(-20.2189647590874,12.9990191712639,122.459008656394)) ;
#17875=CARTESIAN_POINT('Ctrl Pts',(-20.2489818399481,13.0008229873648,122.48581253063)) ;
#17876=CARTESIAN_POINT('Ctrl Pts',(-20.2560479852833,13.0012519697605,122.492269669813)) ;
#17877=CARTESIAN_POINT('Ctrl Pts',(-20.2909306306717,13.0033940407219,122.524888971852)) ;
#17878=CARTESIAN_POINT('Ctrl Pts',(-20.3176116774352,13.0051122985087,122.552234490449)) ;
#17879=CARTESIAN_POINT('Ctrl Pts',(-20.3472930089684,13.007145055823,122.585582712459)) ;
#17880=CARTESIAN_POINT('Ctrl Pts',(-20.351549669853,13.0074396586775,122.590440545582)) ;
#17881=CARTESIAN_POINT('Ctrl Pts',(-20.3581920643393,13.007904352087,122.598140644171)) ;
#17882=CARTESIAN_POINT('Ctrl Pts',(-20.3606031275432,13.0080740787272,122.600960926167)) ;
#17883=CARTESIAN_POINT('Ctrl Pts',(-20.3648611428621,13.0083757119404,122.605986769328)) ;
#17884=CARTESIAN_POINT('Ctrl Pts',(-20.3667131074318,13.0085075465504,122.608188052261)) ;
#17885=CARTESIAN_POINT('Ctrl Pts',(-20.3704947100324,13.008778075814,122.612714569607)) ;
#17886=CARTESIAN_POINT('Ctrl Pts',(-20.3724235485874,13.0089167805941,122.615040446887)) ;
#17887=CARTESIAN_POINT('Ctrl Pts',(-20.3766866224998,13.0092249519798,122.620219146849)) ;
#17888=CARTESIAN_POINT('Ctrl Pts',(-20.3790167089273,13.0093944741667,122.623075344965)) ;
#17889=CARTESIAN_POINT('Ctrl Pts',(-20.3884700562282,13.0100866988123,122.634768384046)) ;
#17890=CARTESIAN_POINT('Ctrl Pts',(-20.3954853887506,13.0106108313071,122.643691691344)) ;
#17891=CARTESIAN_POINT('Ctrl Pts',(-20.4084567331962,13.0115999618398,122.660661566689)) ;
#17892=CARTESIAN_POINT('Ctrl Pts',(-20.4144395185823,13.0120645938256,122.66868657116)) ;
#17893=CARTESIAN_POINT('Ctrl Pts',(-20.4410931707525,13.0141729511637,122.705349275846)) ;
#17894=CARTESIAN_POINT('Ctrl Pts',(-20.4606409254937,13.0158274690159,122.734783197618)) ;
#17895=CARTESIAN_POINT('Ctrl Pts',(-20.491024875738,13.0185720224918,122.785029832403)) ;
#17896=CARTESIAN_POINT('Ctrl Pts',(-20.5025692118449,13.0196619659135,122.805390942654)) ;
#17897=CARTESIAN_POINT('Ctrl Pts',(-20.5240951216122,13.0217916569603,122.845971852595)) ;
#17898=CARTESIAN_POINT('Ctrl Pts',(-20.5341147387331,13.0228321625972,122.866161385836)) ;
#17899=CARTESIAN_POINT('Ctrl Pts',(-20.5486990264017,13.0244307390882,122.897659873808)) ;
#17900=CARTESIAN_POINT('Ctrl Pts',(-20.5536532004924,13.0249906160355,122.908783092264)) ;
#17901=CARTESIAN_POINT('Ctrl Pts',(-20.5625761816843,13.0260321613578,122.929631523645)) ;
#17902=CARTESIAN_POINT('Ctrl Pts',(-20.566586452295,13.026513955654,122.939337816036)) ;
#17903=CARTESIAN_POINT('Ctrl Pts',(-20.5740330793367,13.027436072693,122.95802518626)) ;
#17904=CARTESIAN_POINT('Ctrl Pts',(-20.5774890521294,13.0278764301476,122.966997647652)) ;
#17905=CARTESIAN_POINT('Ctrl Pts',(-20.5846647335729,13.0288184617986,122.986287927234)) ;
#17906=CARTESIAN_POINT('Ctrl Pts',(-20.5883495459185,13.0293195521975,122.996607223224)) ;
#17907=CARTESIAN_POINT('Ctrl Pts',(-20.5919013672999,13.0298207905518,123.006983120529)) ;
#17908=CARTESIAN_POINT('Origin',(-19.4092722359532,16.5113612779716,123.411814366564)) ;
#17909=CARTESIAN_POINT('',(-20.5919008187226,12.3097986802463,123.006981518046)) ;
#17910=CARTESIAN_POINT('',(-20.591900864533,12.3699275081008,123.006981651869)) ;
#17911=CARTESIAN_POINT('',(-20.5919021064381,16.5113612779716,123.006985279772)) ;
#17912=CARTESIAN_POINT('',(-18.1677926225402,12.1420303928368,123.557513887265)) ;
#17913=CARTESIAN_POINT('Ctrl Pts',(-18.1677926148176,12.1420303769689,123.557513887431)) ;
#17914=CARTESIAN_POINT('Ctrl Pts',(-18.1645228320525,12.1433302273642,123.529652651895)) ;
#17915=CARTESIAN_POINT('Ctrl Pts',(-18.1621918274906,12.1446319180994,123.501688885341)) ;
#17916=CARTESIAN_POINT('Ctrl Pts',(-18.1605900595685,12.1461231432797,123.46935956271)) ;
#17917=CARTESIAN_POINT('Ctrl Pts',(-18.1603988140212,12.1463217701979,123.465047846456)) ;
#17918=CARTESIAN_POINT('Ctrl Pts',(-18.1601009307609,12.1466716722533,123.457442320227)) ;
#17919=CARTESIAN_POINT('Ctrl Pts',(-18.1599849810047,12.1468230373754,123.454148921874)) ;
#17920=CARTESIAN_POINT('Ctrl Pts',(-18.1597798801821,12.1471244037961,123.447585239556)) ;
#17921=CARTESIAN_POINT('Ctrl Pts',(-18.1596905410702,12.1472744058144,123.444314987744)) ;
#17922=CARTESIAN_POINT('Ctrl Pts',(-18.1595265963476,12.1475955886168,123.437305938292)) ;
#17923=CARTESIAN_POINT('Ctrl Pts',(-18.1594559280288,12.147766727388,123.433567079176)) ;
#17924=CARTESIAN_POINT('Ctrl Pts',(-18.1593105106464,12.1482280747479,123.423477313111)) ;
#17925=CARTESIAN_POINT('Ctrl Pts',(-18.1592673857191,12.1485179544301,123.417126051257)) ;
#17926=CARTESIAN_POINT('Ctrl Pts',(-18.1592916562,12.1498477125098,123.387945093611)) ;
#17927=CARTESIAN_POINT('Ctrl Pts',(-18.1599360703523,12.1508814866486,123.36512017961)) ;
#17928=CARTESIAN_POINT('Ctrl Pts',(-18.161259740427,12.1519589376578,123.341346121815)) ;
#17929=CARTESIAN_POINT('Ctrl Pts',(-18.1613154302979,12.1520033290725,123.340366667329)) ;
#17930=CARTESIAN_POINT('Ctrl Pts',(-18.1623541770848,12.1528145355369,123.322469329078)) ;
#17931=CARTESIAN_POINT('Ctrl Pts',(-18.1636800155036,12.1535813892693,123.305573137795)) ;
#17932=CARTESIAN_POINT('Ctrl Pts',(-18.1660691461184,12.1546833930302,123.281432032133)) ;
#17933=CARTESIAN_POINT('Ctrl Pts',(-18.1668531734841,12.155016086958,123.274161367388)) ;
#17934=CARTESIAN_POINT('Ctrl Pts',(-18.1683731377733,12.1556136837441,123.261139067942)) ;
#17935=CARTESIAN_POINT('Ctrl Pts',(-18.1690853820572,12.1558783464076,123.255384879309)) ;
#17936=CARTESIAN_POINT('Ctrl Pts',(-18.1698791912853,12.1561580650851,123.249318263516)) ;
#17937=CARTESIAN_POINT('Ctrl Pts',(-18.1699208718392,12.1561727105025,123.249000672589)) ;
#17938=CARTESIAN_POINT('Ctrl Pts',(-18.1703951832096,12.1563388981152,123.245397325292)) ;
#17939=CARTESIAN_POINT('Ctrl Pts',(-18.1708407567144,12.1564905715711,123.242113292349)) ;
#17940=CARTESIAN_POINT('Ctrl Pts',(-18.1717536802671,12.156792752142,123.235579860305)) ;
#17941=CARTESIAN_POINT('Ctrl Pts',(-18.1722207812292,12.1569432555277,123.232330453215)) ;
#17942=CARTESIAN_POINT('Ctrl Pts',(-18.1733413883875,12.1572949972217,123.224747133327)) ;
#17943=CARTESIAN_POINT('Ctrl Pts',(-18.1740048982661,12.1574963338795,123.220414748016)) ;
#17944=CARTESIAN_POINT('Ctrl Pts',(-18.176220707127,12.1581470900796,123.206438261038)) ;
#17945=CARTESIAN_POINT('Ctrl Pts',(-18.1778632635612,12.1585973562675,123.196808881856)) ;
#17946=CARTESIAN_POINT('Ctrl Pts',(-18.1803766629264,12.1592432274774,123.18304926372)) ;
#17947=CARTESIAN_POINT('Ctrl Pts',(-18.1811558254033,12.159438190199,123.178902615624)) ;
#17948=CARTESIAN_POINT('Ctrl Pts',(-18.185495245598,12.160496098832,123.156435866658)) ;
#17949=CARTESIAN_POINT('Ctrl Pts',(-18.1894444480382,12.161361062067,123.138193336859)) ;
#17950=CARTESIAN_POINT('Ctrl Pts',(-18.1960672856455,12.1626720506994,123.110603393496)) ;
#17951=CARTESIAN_POINT('Ctrl Pts',(-18.1984439196893,12.1631199756946,123.101187433458)) ;
#17952=CARTESIAN_POINT('Ctrl Pts',(-18.2032493208257,12.1639844506056,123.083042714816)) ;
#17953=CARTESIAN_POINT('Ctrl Pts',(-18.2056637430767,12.1644010634853,123.074310784912)) ;
#17954=CARTESIAN_POINT('Ctrl Pts',(-18.2097924770936,12.1650857327849,123.059986990096)) ;
#17955=CARTESIAN_POINT('Ctrl Pts',(-18.2114514850232,12.1653540857128,123.054379556268)) ;
#17956=CARTESIAN_POINT('Ctrl Pts',(-18.214057171405,12.165765521525,123.045794269898)) ;
#17957=CARTESIAN_POINT('Ctrl Pts',(-18.2149757674291,12.165908741072,123.042807988586)) ;
#17958=CARTESIAN_POINT('Ctrl Pts',(-18.2168873050962,12.1662030805942,123.036675645351)) ;
#17959=CARTESIAN_POINT('Ctrl Pts',(-18.2178815247523,12.1663541935308,123.033530006875)) ;
#17960=CARTESIAN_POINT('Ctrl Pts',(-18.2277045729832,12.167828260825,123.002873473018)) ;
#17961=CARTESIAN_POINT('Ctrl Pts',(-18.2374722997836,12.1691466736145,122.975672517264)) ;
#17962=CARTESIAN_POINT('Ctrl Pts',(-18.2517635928554,12.1709094370337,122.939831656671)) ;
#17963=CARTESIAN_POINT('Ctrl Pts',(-18.2554579799746,12.1713523598241,122.930870919293)) ;
#17964=CARTESIAN_POINT('Ctrl Pts',(-18.2595555461703,12.1718306571154,122.921251305588)) ;
#17965=CARTESIAN_POINT('Ctrl Pts',(-18.2598555385629,12.1718656017964,122.920548817884)) ;
#17966=CARTESIAN_POINT('Ctrl Pts',(-18.2605742227398,12.1719491452172,122.918870147864)) ;
#17967=CARTESIAN_POINT('Ctrl Pts',(-18.2609935151812,12.1719977464906,122.917894223493)) ;
#17968=CARTESIAN_POINT('Ctrl Pts',(-18.2641936761055,12.1723676321057,122.910471786482)) ;
#17969=CARTESIAN_POINT('Ctrl Pts',(-18.2670275633275,12.1726891559544,122.904048280276)) ;
#17970=CARTESIAN_POINT('Ctrl Pts',(-18.2766027056258,12.1737558853549,122.882830391168)) ;
#17971=CARTESIAN_POINT('Ctrl Pts',(-18.283578450434,12.1745018651069,122.868143684651)) ;
#17972=CARTESIAN_POINT('Ctrl Pts',(-18.3008589420707,12.1762783256065,122.833520807817)) ;
#17973=CARTESIAN_POINT('Ctrl Pts',(-18.3114179902996,12.1773088320195,122.813717779776)) ;
#17974=CARTESIAN_POINT('Ctrl Pts',(-18.327646145792,12.1788154804924,122.785161909371)) ;
#17975=CARTESIAN_POINT('Ctrl Pts',(-18.3329007623534,12.1792925311924,122.776178659087)) ;
#17976=CARTESIAN_POINT('Ctrl Pts',(-18.3428180928227,12.1801732727208,122.759699758564)) ;
#17977=CARTESIAN_POINT('Ctrl Pts',(-18.3474492136124,12.1805770762111,122.752185856506)) ;
#17978=CARTESIAN_POINT('Ctrl Pts',(-18.3646853118381,12.1820529446047,122.724872565516)) ;
#17979=CARTESIAN_POINT('Ctrl Pts',(-18.3777675134087,12.1831202428263,122.705380445828)) ;
#17980=CARTESIAN_POINT('Ctrl Pts',(-18.3973055966241,12.1846527491358,122.677970131367)) ;
#17981=CARTESIAN_POINT('Ctrl Pts',(-18.4033216118026,12.185116969702,122.669744840478)) ;
#17982=CARTESIAN_POINT('Ctrl Pts',(-18.4129162732998,12.1858463967867,122.656957829174)) ;
#17983=CARTESIAN_POINT('Ctrl Pts',(-18.4164272301395,12.1861110921839,122.652345874445)) ;
#17984=CARTESIAN_POINT('Ctrl Pts',(-18.420041004912,12.1863813662252,122.647666746629)) ;
#17985=CARTESIAN_POINT('Ctrl Pts',(-18.420111891752,12.186386667003,122.647574988503)) ;
#17986=CARTESIAN_POINT('Ctrl Pts',(-18.4202521364862,12.1863971525557,122.647393503566)) ;
#17987=CARTESIAN_POINT('Ctrl Pts',(-18.4203214938545,12.1864023373279,122.647303776291)) ;
#17988=CARTESIAN_POINT('Ctrl Pts',(-18.4204587764218,12.1864125982132,122.647126224475)) ;
#17989=CARTESIAN_POINT('Ctrl Pts',(-18.420526701111,12.1864176743217,122.647038399543)) ;
#17990=CARTESIAN_POINT('Ctrl Pts',(-18.4206612104076,12.1864277248613,122.646864530246)) ;
#17991=CARTESIAN_POINT('Ctrl Pts',(-18.4207277944761,12.186432699283,122.646778485616)) ;
#17992=CARTESIAN_POINT('Ctrl Pts',(-18.4208597100436,12.1864425530785,122.646608060991)) ;
#17993=CARTESIAN_POINT('Ctrl Pts',(-18.4209250410815,12.1864474324461,122.646523680711)) ;
#17994=CARTESIAN_POINT('Ctrl Pts',(-18.4210545342517,12.1864571024661,122.646356474126)) ;
#17995=CARTESIAN_POINT('Ctrl Pts',(-18.4211186959259,12.18646189311,122.646273647605)) ;
#17996=CARTESIAN_POINT('Ctrl Pts',(-18.4212459298864,12.1864713916966,122.646109443506)) ;
#17997=CARTESIAN_POINT('Ctrl Pts',(-18.4213090019489,12.1864760996461,122.646028065478)) ;
#17998=CARTESIAN_POINT('Ctrl Pts',(-18.4214341334466,12.186485438644,122.645866657143)) ;
#17999=CARTESIAN_POINT('Ctrl Pts',(-18.4214961924914,12.1864900696847,122.645786626665)) ;
#18000=CARTESIAN_POINT('Ctrl Pts',(-18.4216193713305,12.1864992604048,122.645627816813)) ;
#18001=CARTESIAN_POINT('Ctrl Pts',(-18.421680490808,12.1865038200801,122.645549037231)) ;
#18002=CARTESIAN_POINT('Ctrl Pts',(-18.4218018609868,12.1865128733855,122.645392636513)) ;
#18003=CARTESIAN_POINT('Ctrl Pts',(-18.421862111496,12.1865173670192,122.645315015064)) ;
#18004=CARTESIAN_POINT('Ctrl Pts',(-18.4247301928209,12.1867312470328,122.641620931058)) ;
#18005=CARTESIAN_POINT('Ctrl Pts',(-18.4275578574986,12.1869408064192,122.638019922427)) ;
#18006=CARTESIAN_POINT('Ctrl Pts',(-18.432909717685,12.1873350404602,122.631280926748)) ;
#18007=CARTESIAN_POINT('Ctrl Pts',(-18.4354294184834,12.1875196702613,122.62813944384)) ;
#18008=CARTESIAN_POINT('Ctrl Pts',(-18.4415875171941,12.1879685633477,122.620537284786)) ;
#18009=CARTESIAN_POINT('Ctrl Pts',(-18.4452416263481,12.1882329747225,122.616089465293)) ;
#18010=CARTESIAN_POINT('Ctrl Pts',(-18.4554550410091,12.1889666793585,122.603831208705)) ;
#18011=CARTESIAN_POINT('Ctrl Pts',(-18.4620793939813,12.1894365720639,122.596075595045)) ;
#18012=CARTESIAN_POINT('Ctrl Pts',(-18.4834781031392,12.190935347645,122.571634699625)) ;
#18013=CARTESIAN_POINT('Ctrl Pts',(-18.4986040563497,12.1919666004084,122.555263075848)) ;
#18014=CARTESIAN_POINT('Ctrl Pts',(-18.5219361861099,12.1935103138716,122.531326512936)) ;
#18015=CARTESIAN_POINT('Ctrl Pts',(-18.5298191447238,12.1940242968596,122.523452735519)) ;
#18016=CARTESIAN_POINT('Ctrl Pts',(-18.5441774619311,12.1949467881151,122.509489585183)) ;
#18017=CARTESIAN_POINT('Ctrl Pts',(-18.5506145026092,12.195355573551,122.503361903832)) ;
#18018=CARTESIAN_POINT('Ctrl Pts',(-18.5612083052461,12.1960206591927,122.493490430241)) ;
#18019=CARTESIAN_POINT('Ctrl Pts',(-18.5653258024633,12.1962773126799,122.489704991146)) ;
#18020=CARTESIAN_POINT('Ctrl Pts',(-18.5710013053714,12.1966285987161,122.484557051096)) ;
#18021=CARTESIAN_POINT('Ctrl Pts',(-18.5725374861609,12.1967234345237,122.483170602438)) ;
#18022=CARTESIAN_POINT('Ctrl Pts',(-18.5748995165934,12.1968688794334,122.481049419282)) ;
#18023=CARTESIAN_POINT('Ctrl Pts',(-18.5757229089568,12.1969195113214,122.480311955742)) ;
#18024=CARTESIAN_POINT('Ctrl Pts',(-18.5817032191462,12.197286749831,122.474970026566)) ;
#18025=CARTESIAN_POINT('Ctrl Pts',(-18.5868972891204,12.1976030028579,122.470407312092)) ;
#18026=CARTESIAN_POINT('Ctrl Pts',(-18.6097881440936,12.1989853968337,122.450632932986)) ;
#18027=CARTESIAN_POINT('Ctrl Pts',(-18.6278710570068,12.2000477396646,122.435875452628)) ;
#18028=CARTESIAN_POINT('Ctrl Pts',(-18.6565981779941,12.2016995526509,122.413741762877)) ;
#18029=CARTESIAN_POINT('Ctrl Pts',(-18.6669616198807,12.2022887508295,122.406010157)) ;
#18030=CARTESIAN_POINT('Ctrl Pts',(-18.6847886219544,12.2032925103567,122.393136012444)) ;
#18031=CARTESIAN_POINT('Ctrl Pts',(-18.6921915544269,12.2037064914759,122.387911347904)) ;
#18032=CARTESIAN_POINT('Ctrl Pts',(-18.69990698398,12.2041351326502,122.3825908552)) ;
#18033=CARTESIAN_POINT('Ctrl Pts',(-18.7001634145111,12.2041493758014,122.382414164308)) ;
#18034=CARTESIAN_POINT('Ctrl Pts',(-18.70067945401,12.2041780322253,122.382058876777)) ;
#18035=CARTESIAN_POINT('Ctrl Pts',(-18.7009390645633,12.2041924455099,122.381880282422)) ;
#18036=CARTESIAN_POINT('Ctrl Pts',(-18.7014625314209,12.2042215012206,122.381520464463)) ;
#18037=CARTESIAN_POINT('Ctrl Pts',(-18.7017263897835,12.2042361436569,122.381339244057)) ;
#18038=CARTESIAN_POINT('Ctrl Pts',(-18.7022594983657,12.2042657209516,122.380973401359)) ;
#18039=CARTESIAN_POINT('Ctrl Pts',(-18.70252875142,12.2042806558321,122.380788783115)) ;
#18040=CARTESIAN_POINT('Ctrl Pts',(-18.7093338711574,12.2046580327664,122.376126647569)) ;
#18041=CARTESIAN_POINT('Ctrl Pts',(-18.7159120750066,12.2050207724632,122.371711269472)) ;
#18042=CARTESIAN_POINT('Ctrl Pts',(-18.7306319494098,12.205828002473,122.362032798999)) ;
#18043=CARTESIAN_POINT('Ctrl Pts',(-18.738793770146,12.2062726075636,122.356801284005)) ;
#18044=CARTESIAN_POINT('Ctrl Pts',(-18.7664242306082,12.2077678053906,122.339541018082)) ;
#18045=CARTESIAN_POINT('Ctrl Pts',(-18.7861621285198,12.208819668736,122.327952067438)) ;
#18046=CARTESIAN_POINT('Ctrl Pts',(-18.8153085662974,12.2103479166225,122.311898401772)) ;
#18047=CARTESIAN_POINT('Ctrl Pts',(-18.8244723425432,12.2108248883029,122.306998972057)) ;
#18048=CARTESIAN_POINT('Ctrl Pts',(-18.8389253835496,12.2115713244619,122.29950183374)) ;
#18049=CARTESIAN_POINT('Ctrl Pts',(-18.8441737320509,12.2118411751851,122.296826302062)) ;
#18050=CARTESIAN_POINT('Ctrl Pts',(-18.8627668017161,12.2127928880342,122.287512827957)) ;
#18051=CARTESIAN_POINT('Ctrl Pts',(-18.8762111380298,12.2134735730895,122.281076551096)) ;
#18052=CARTESIAN_POINT('Ctrl Pts',(-18.9008902714506,12.2147131183202,122.269799774599)) ;
#18053=CARTESIAN_POINT('Ctrl Pts',(-18.9120871344803,12.2152718330016,122.264880835652)) ;
#18054=CARTESIAN_POINT('Ctrl Pts',(-18.9237710317051,12.2158518287665,122.259951186637)) ;
#18055=CARTESIAN_POINT('Ctrl Pts',(-18.9241878009281,12.2158725134481,122.259775610491)) ;
#18056=CARTESIAN_POINT('Ctrl Pts',(-18.9249915696815,12.2159123976629,122.259437513042)) ;
#18057=CARTESIAN_POINT('Ctrl Pts',(-18.9253785559055,12.2159315970852,122.259274960441)) ;
#18058=CARTESIAN_POINT('Ctrl Pts',(-18.9261280064668,12.2159687727633,122.258960599595)) ;
#18059=CARTESIAN_POINT('Ctrl Pts',(-18.9264904607414,12.2159867489388,122.258808767261)) ;
#18060=CARTESIAN_POINT('Ctrl Pts',(-18.9271952010047,12.2160216952847,122.258513941671)) ;
#18061=CARTESIAN_POINT('Ctrl Pts',(-18.9275374791285,12.2160386653868,122.258370929828)) ;
#18062=CARTESIAN_POINT('Ctrl Pts',(-18.9282055447689,12.2160717828812,122.258092145542)) ;
#18063=CARTESIAN_POINT('Ctrl Pts',(-18.9285313261947,12.2160879302194,122.257956358692)) ;
#18064=CARTESIAN_POINT('Ctrl Pts',(-18.929169564206,12.2161195598355,122.257690656053)) ;
#18065=CARTESIAN_POINT('Ctrl Pts',(-18.9294820160998,12.2161350420713,122.257560729136)) ;
#18066=CARTESIAN_POINT('Ctrl Pts',(-18.9300963749889,12.2161654797999,122.257305552748)) ;
#18067=CARTESIAN_POINT('Ctrl Pts',(-18.9303982784671,12.2161804352628,122.257180294768)) ;
#18068=CARTESIAN_POINT('Ctrl Pts',(-18.9309940349823,12.2162099434465,122.256933392741)) ;
#18069=CARTESIAN_POINT('Ctrl Pts',(-18.9312878854123,12.2162244961448,122.256811742385)) ;
#18070=CARTESIAN_POINT('Ctrl Pts',(-18.9318698271665,12.2162533125961,122.256571085987)) ;
#18071=CARTESIAN_POINT('Ctrl Pts',(-18.932157916626,12.2162675763311,122.256452075537)) ;
#18072=CARTESIAN_POINT('Ctrl Pts',(-18.9327304953461,12.216295921971,122.256215792568)) ;
#18073=CARTESIAN_POINT('Ctrl Pts',(-18.9330149834148,12.2163100038627,122.256098517332)) ;
#18074=CARTESIAN_POINT('Ctrl Pts',(-18.9335824493013,12.2163380894059,122.255864834544)) ;
#18075=CARTESIAN_POINT('Ctrl Pts',(-18.9338654267041,12.2163520930564,122.255748425788)) ;
#18076=CARTESIAN_POINT('Ctrl Pts',(-18.93443195383,12.2163801252376,122.255515616025)) ;
#18077=CARTESIAN_POINT('Ctrl Pts',(-18.9347155036718,12.2163941537683,122.255399215387)) ;
#18078=CARTESIAN_POINT('Ctrl Pts',(-18.9352853123423,12.2164223414045,122.255165546906)) ;
#18079=CARTESIAN_POINT('Ctrl Pts',(-18.9355715719559,12.216436500517,122.255048281005)) ;
#18080=CARTESIAN_POINT('Ctrl Pts',(-18.9433240163868,12.2168199085375,122.251875861885)) ;
#18081=CARTESIAN_POINT('Ctrl Pts',(-18.9508195454011,12.217189431199,122.248892955615)) ;
#18082=CARTESIAN_POINT('Ctrl Pts',(-18.9594342632914,12.2176128970995,122.245560892225)) ;
#18083=CARTESIAN_POINT('Ctrl Pts',(-18.9605257069928,12.2176665255784,122.245140495766)) ;
#18084=CARTESIAN_POINT('Ctrl Pts',(-18.9621261687957,12.2177451319789,122.244526616593)) ;
#18085=CARTESIAN_POINT('Ctrl Pts',(-18.9626347260644,12.217770104821,122.244331933562)) ;
#18086=CARTESIAN_POINT('Ctrl Pts',(-18.9673729995085,12.2180027339373,122.242521603515)) ;
#18087=CARTESIAN_POINT('Ctrl Pts',(-18.9716113334257,12.2182104841213,122.240928618418)) ;
#18088=CARTESIAN_POINT('Ctrl Pts',(-18.9942224841391,12.2193170749833,122.232570102365)) ;
#18089=CARTESIAN_POINT('Ctrl Pts',(-19.0127436520792,12.220217578565,122.226213924235)) ;
#18090=CARTESIAN_POINT('Ctrl Pts',(-19.0515907926042,12.2220924950652,122.213894348849)) ;
#18091=CARTESIAN_POINT('Ctrl Pts',(-19.071934638872,12.2230659205256,122.208007183392)) ;
#18092=CARTESIAN_POINT('Ctrl Pts',(-19.1057136292822,12.2246688135965,122.199155685149)) ;
#18093=CARTESIAN_POINT('Ctrl Pts',(-19.1190655972305,12.2252990883806,122.195891254894)) ;
#18094=CARTESIAN_POINT('Ctrl Pts',(-19.1677225864566,12.2275854979155,122.184842202695)) ;
#18095=CARTESIAN_POINT('Ctrl Pts',(-19.2033071707242,12.2292373528706,122.178369873062)) ;
#18096=CARTESIAN_POINT('Ctrl Pts',(-19.2443297510396,12.2311329501925,122.172733413564)) ;
#18097=CARTESIAN_POINT('Ctrl Pts',(-19.2495418353335,12.2313736456963,122.17205074778)) ;
#18098=CARTESIAN_POINT('Ctrl Pts',(-19.269469403528,12.232293533661,122.1695684369)) ;
#18099=CARTESIAN_POINT('Ctrl Pts',(-19.2842121442157,12.2329734011545,122.167997759009)) ;
#18100=CARTESIAN_POINT('Ctrl Pts',(-19.3261818803678,12.2349069048186,122.16428008652)) ;
#18101=CARTESIAN_POINT('Ctrl Pts',(-19.3534561389592,12.236161044958,122.162762585656)) ;
#18102=CARTESIAN_POINT('Ctrl Pts',(-19.3854043401168,12.2376270461804,122.162033617022)) ;
#18103=CARTESIAN_POINT('Ctrl Pts',(-19.3900510857168,12.2378401950327,122.161953515986)) ;
#18104=CARTESIAN_POINT('Ctrl Pts',(-19.4042099196831,12.238489435588,122.161788423365)) ;
#18105=CARTESIAN_POINT('Ctrl Pts',(-19.4137226380546,12.238925311864,122.161786094804)) ;
#18106=CARTESIAN_POINT('Ctrl Pts',(-19.4236828948241,12.2393813517582,122.16189735568)) ;
#18107=CARTESIAN_POINT('Ctrl Pts',(-19.4241313187826,12.2394018825517,122.161902606141)) ;
#18108=CARTESIAN_POINT('Ctrl Pts',(-19.43481762074,12.2398911304649,122.162033480441)) ;
#18109=CARTESIAN_POINT('Ctrl Pts',(-19.4450535984701,12.2403593816135,122.162284644999)) ;
#18110=CARTESIAN_POINT('Ctrl Pts',(-19.4650656910383,12.2412741002838,122.163021799644)) ;
#18111=CARTESIAN_POINT('Ctrl Pts',(-19.4748414735195,12.2417205339493,122.1634969145)) ;
#18112=CARTESIAN_POINT('Ctrl Pts',(-19.5101735512852,12.2433332668824,122.165630284742)) ;
#18113=CARTESIAN_POINT('Ctrl Pts',(-19.5356828364579,12.2444975683689,122.16795898834)) ;
#18114=CARTESIAN_POINT('Ctrl Pts',(-19.5670788919768,12.245942413207,122.171800935203)) ;
#18115=CARTESIAN_POINT('Ctrl Pts',(-19.5730497812065,12.2462176921639,122.17257542027)) ;
#18116=CARTESIAN_POINT('Ctrl Pts',(-19.5830888528739,12.2466814763301,122.173951412425)) ;
#18117=CARTESIAN_POINT('Ctrl Pts',(-19.5871600885699,12.2468698213672,122.174529912069)) ;
#18118=CARTESIAN_POINT('Ctrl Pts',(-19.5960297390353,12.2472807554412,122.175834922107)) ;
#18119=CARTESIAN_POINT('Ctrl Pts',(-19.6008269242351,12.2475033964753,122.176569308568)) ;
#18120=CARTESIAN_POINT('Ctrl Pts',(-19.6118824274516,12.2480174128346,122.178327713083)) ;
#18121=CARTESIAN_POINT('Ctrl Pts',(-19.6181374656133,12.2483089197332,122.179371455317)) ;
#18122=CARTESIAN_POINT('Ctrl Pts',(-19.6326959910645,12.2489890051571,122.181914769569)) ;
#18123=CARTESIAN_POINT('Ctrl Pts',(-19.6409927663036,12.2493778053678,122.183450907276)) ;
#18124=CARTESIAN_POINT('Ctrl Pts',(-19.6695561075008,12.2507203181433,122.189039062843)) ;
#18125=CARTESIAN_POINT('Ctrl Pts',(-19.6897373188593,12.2516758609037,122.193509612739)) ;
#18126=CARTESIAN_POINT('Ctrl Pts',(-19.7266671776703,12.2534321971237,122.202656616647)) ;
#18127=CARTESIAN_POINT('Ctrl Pts',(-19.7434470677064,12.2542333066548,122.207186125052)) ;
#18128=CARTESIAN_POINT('Ctrl Pts',(-19.7673306764107,12.2553776010228,122.214170645652)) ;
#18129=CARTESIAN_POINT('Ctrl Pts',(-19.774515124887,12.2557223579459,122.216342091005)) ;
#18130=CARTESIAN_POINT('Ctrl Pts',(-19.786802523401,12.256312972159,122.220176970858)) ;
#18131=CARTESIAN_POINT('Ctrl Pts',(-19.7919151072575,12.2565590119332,122.221808806064)) ;
#18132=CARTESIAN_POINT('Ctrl Pts',(-19.803032729246,12.2570947320051,122.225436384868)) ;
#18133=CARTESIAN_POINT('Ctrl Pts',(-19.8090334453629,12.2573843278035,122.227444906771)) ;
#18134=CARTESIAN_POINT('Ctrl Pts',(-19.8152179863916,12.2576833057436,122.22956731447)) ;
#18135=CARTESIAN_POINT('Ctrl Pts',(-19.8154172922062,12.2576929412929,122.229635768481)) ;
#18136=CARTESIAN_POINT('Ctrl Pts',(-19.8158264704854,12.2577127243783,122.229776421438)) ;
#18137=CARTESIAN_POINT('Ctrl Pts',(-19.8160363409848,12.2577228718798,122.229848625862)) ;
#18138=CARTESIAN_POINT('Ctrl Pts',(-19.8164678811901,12.257743738657,122.229997222692)) ;
#18139=CARTESIAN_POINT('Ctrl Pts',(-19.8166895486924,12.2577544578976,122.230073621591)) ;
#18140=CARTESIAN_POINT('Ctrl Pts',(-19.8171460621064,12.257776535075,122.230231105113)) ;
#18141=CARTESIAN_POINT('Ctrl Pts',(-19.817380905454,12.2577878929727,122.230312197425)) ;
#18142=CARTESIAN_POINT('Ctrl Pts',(-19.8178653185846,12.2578113226024,122.230479628803)) ;
#18143=CARTESIAN_POINT('Ctrl Pts',(-19.8181148853065,12.2578233942877,122.230565976984)) ;
#18144=CARTESIAN_POINT('Ctrl Pts',(-19.8257395270663,12.2581922296512,122.233206750634)) ;
#18145=CARTESIAN_POINT('Ctrl Pts',(-19.833090557614,12.2585486001865,122.235830120235)) ;
#18146=CARTESIAN_POINT('Ctrl Pts',(-19.8539029521174,12.2595601497174,122.243477955619)) ;
#18147=CARTESIAN_POINT('Ctrl Pts',(-19.8673029248661,12.2602145014084,122.248665909766)) ;
#18148=CARTESIAN_POINT('Ctrl Pts',(-19.9060376920783,12.2621184626908,122.264435707635)) ;
#18149=CARTESIAN_POINT('Ctrl Pts',(-19.931116818952,12.2633675442307,122.275622512465)) ;
#18150=CARTESIAN_POINT('Ctrl Pts',(-19.9631384724602,12.2649943851343,122.291190146319)) ;
#18151=CARTESIAN_POINT('Ctrl Pts',(-19.9704346873014,12.2653672269055,122.294825936211)) ;
#18152=CARTESIAN_POINT('Ctrl Pts',(-19.9834768149942,12.2660377602939,122.301485024137)) ;
#18153=CARTESIAN_POINT('Ctrl Pts',(-19.9892357318739,12.2663352864247,122.304482216601)) ;
#18154=CARTESIAN_POINT('Ctrl Pts',(-20.0017259720429,12.2669837836874,122.311106850548)) ;
#18155=CARTESIAN_POINT('Ctrl Pts',(-20.0084478865366,12.267334839778,122.31475146749)) ;
#18156=CARTESIAN_POINT('Ctrl Pts',(-20.0239105945599,12.2681471562515,122.323319844205)) ;
#18157=CARTESIAN_POINT('Ctrl Pts',(-20.0326263957985,12.2686086028019,122.328287612043)) ;
#18158=CARTESIAN_POINT('Ctrl Pts',(-20.058118491202,12.2699685184745,122.343226802386)) ;
#18159=CARTESIAN_POINT('Ctrl Pts',(-20.0747221784813,12.270867654615,122.353486808107)) ;
#18160=CARTESIAN_POINT('Ctrl Pts',(-20.1010857275969,12.272313816415,122.370643564332)) ;
#18161=CARTESIAN_POINT('Ctrl Pts',(-20.1109988064159,12.2728619851654,122.377298843122)) ;
#18162=CARTESIAN_POINT('Ctrl Pts',(-20.1445612175643,12.2747347802739,122.400535823734)) ;
#18163=CARTESIAN_POINT('Ctrl Pts',(-20.1677305109691,12.2760569511258,122.417794633536)) ;
#18164=CARTESIAN_POINT('Ctrl Pts',(-20.2727534369062,12.2822167198327,122.501837704674)) ;
#18165=CARTESIAN_POINT('Ctrl Pts',(-20.3465286166676,12.2870386308518,122.578023182883)) ;
#18166=CARTESIAN_POINT('Ctrl Pts',(-20.4323847470827,12.293605133144,122.692679227499)) ;
#18167=CARTESIAN_POINT('Ctrl Pts',(-20.4535580323012,12.2953292495682,122.723786946419)) ;
#18168=CARTESIAN_POINT('Ctrl Pts',(-20.4833812613681,12.2979356525796,122.772158942524)) ;
#18169=CARTESIAN_POINT('Ctrl Pts',(-20.4930875715225,12.2988167664969,122.78874648869)) ;
#18170=CARTESIAN_POINT('Ctrl Pts',(-20.5068966632968,12.3001207856383,122.81364525862)) ;
#18171=CARTESIAN_POINT('Ctrl Pts',(-20.5112956719335,12.3005444128992,122.821788932931)) ;
#18172=CARTESIAN_POINT('Ctrl Pts',(-20.5246851473785,12.3018597350152,122.847248443507)) ;
#18173=CARTESIAN_POINT('Ctrl Pts',(-20.5333609025052,12.3027491591494,122.864726334894)) ;
#18174=CARTESIAN_POINT('Ctrl Pts',(-20.5484219081126,12.3043714020717,122.89693997333)) ;
#18175=CARTESIAN_POINT('Ctrl Pts',(-20.5549390719354,12.305103978519,122.911609293826)) ;
#18176=CARTESIAN_POINT('Ctrl Pts',(-20.5639447883878,12.3061647490169,122.932980070922)) ;
#18177=CARTESIAN_POINT('Ctrl Pts',(-20.5666612096697,12.306491641395,122.939583756425)) ;
#18178=CARTESIAN_POINT('Ctrl Pts',(-20.571603098209,12.3070996427502,122.951896431715)) ;
#18179=CARTESIAN_POINT('Ctrl Pts',(-20.5738434595775,12.3073806560075,122.957599213814)) ;
#18180=CARTESIAN_POINT('Ctrl Pts',(-20.5784317875143,12.307967686466,122.969535819076)) ;
#18181=CARTESIAN_POINT('Ctrl Pts',(-20.5807720339025,12.3082737386583,122.97577240339)) ;
#18182=CARTESIAN_POINT('Ctrl Pts',(-20.586097636059,12.3089860108875,122.990317141197)) ;
#18183=CARTESIAN_POINT('Ctrl Pts',(-20.5890417450682,12.3093919517987,122.998629374036)) ;
#18184=CARTESIAN_POINT('Ctrl Pts',(-20.591900818743,12.3097986802335,123.00698151804)) ;
#18185=CARTESIAN_POINT('',(-18.1733329886729,12.2002114096132,123.598774520568)) ;
#18186=CARTESIAN_POINT('Ctrl Pts',(-18.1677926155534,12.1420304143771,123.5575138937)) ;
#18187=CARTESIAN_POINT('Ctrl Pts',(-18.169135727965,12.1629836299978,123.568958314418)) ;
#18188=CARTESIAN_POINT('Ctrl Pts',(-18.1709219229379,12.182512173169,123.58283582176)) ;
#18189=CARTESIAN_POINT('Ctrl Pts',(-18.1733328671508,12.200210692235,123.598773925614)) ;
#18190=CARTESIAN_POINT('Ctrl Pts',(-20.5919008645526,12.3699275081133,123.006981651862)) ;
#18191=CARTESIAN_POINT('Ctrl Pts',(-20.588467048387,12.3694413279222,122.99695052257)) ;
#18192=CARTESIAN_POINT('Ctrl Pts',(-20.5849091447236,12.3689552610106,122.986972898729)) ;
#18193=CARTESIAN_POINT('Ctrl Pts',(-20.5698738748206,12.3669703159962,122.946445527993)) ;
#18194=CARTESIAN_POINT('Ctrl Pts',(-20.5573333724681,12.3654693923714,122.916314680899)) ;
#18195=CARTESIAN_POINT('Ctrl Pts',(-20.5391761439346,12.3634817537078,122.877090607563)) ;
#18196=CARTESIAN_POINT('Ctrl Pts',(-20.5346014928025,12.3629945400929,122.867529143557)) ;
#18197=CARTESIAN_POINT('Ctrl Pts',(-20.5269913366345,12.3622056239413,122.852129376477)) ;
#18198=CARTESIAN_POINT('Ctrl Pts',(-20.5240303683542,12.3619036716072,122.84625483596)) ;
#18199=CARTESIAN_POINT('Ctrl Pts',(-20.5183841361507,12.3613371956875,122.835269380443)) ;
#18200=CARTESIAN_POINT('Ctrl Pts',(-20.5157095679168,12.3610726226028,122.830153160319)) ;
#18201=CARTESIAN_POINT('Ctrl Pts',(-20.5101047504447,12.360525924615,122.819610171444)) ;
#18202=CARTESIAN_POINT('Ctrl Pts',(-20.507169587209,12.3602438538138,122.814186187643)) ;
#18203=CARTESIAN_POINT('Ctrl Pts',(-20.4945872284831,12.3590523216907,122.79134039582)) ;
#18204=CARTESIAN_POINT('Ctrl Pts',(-20.4845645338713,12.3581457997232,122.774128658132)) ;
#18205=CARTESIAN_POINT('Ctrl Pts',(-20.4532563116821,12.3554263223768,122.723202330166)) ;
#18206=CARTESIAN_POINT('Ctrl Pts',(-20.4307651059345,12.3536159843102,122.690259388991)) ;
#18207=CARTESIAN_POINT('Ctrl Pts',(-20.4021529489442,12.3514481267618,122.652376565067)) ;
#18208=CARTESIAN_POINT('Ctrl Pts',(-20.3975122219132,12.3511004161684,122.646347440896)) ;
#18209=CARTESIAN_POINT('Ctrl Pts',(-20.3887647950201,12.3504520301483,122.635195134209)) ;
#18210=CARTESIAN_POINT('Ctrl Pts',(-20.3846722088182,12.3501514498756,122.63006120989)) ;
#18211=CARTESIAN_POINT('Ctrl Pts',(-20.376131643927,12.3495297687297,122.619519020634)) ;
#18212=CARTESIAN_POINT('Ctrl Pts',(-20.3716782842844,12.3492086436625,122.614115408473)) ;
#18213=CARTESIAN_POINT('Ctrl Pts',(-20.3617186080977,12.3484970327808,122.602235360749)) ;
#18214=CARTESIAN_POINT('Ctrl Pts',(-20.3561911563641,12.3481064272172,122.595777102711)) ;
#18215=CARTESIAN_POINT('Ctrl Pts',(-20.3333834307839,12.3465118842596,122.569672411961)) ;
#18216=CARTESIAN_POINT('Ctrl Pts',(-20.3155542965339,12.3453047223799,122.550514543849)) ;
#18217=CARTESIAN_POINT('Ctrl Pts',(-20.2782081435285,12.3428528304214,122.512829639854)) ;
#18218=CARTESIAN_POINT('Ctrl Pts',(-20.2586676016641,12.3416086114623,122.494344658606)) ;
#18219=CARTESIAN_POINT('Ctrl Pts',(-20.2183254075472,12.3391198137629,122.458576062302)) ;
#18220=CARTESIAN_POINT('Ctrl Pts',(-20.1975285548273,12.3378761032523,122.441308165068)) ;
#18221=CARTESIAN_POINT('Ctrl Pts',(-20.1460043562943,12.3348761268626,122.401276478576)) ;
#18222=CARTESIAN_POINT('Ctrl Pts',(-20.1147605172763,12.3331224335785,122.379221833841)) ;
#18223=CARTESIAN_POINT('Ctrl Pts',(-20.0620911182597,12.3302543283572,122.34555105895)) ;
#18224=CARTESIAN_POINT('Ctrl Pts',(-20.0412499364868,12.329140632997,122.333067814715)) ;
#18225=CARTESIAN_POINT('Ctrl Pts',(-20.0032253422425,12.327143406379,122.31177258232)) ;
#18226=CARTESIAN_POINT('Ctrl Pts',(-19.9861763379106,12.3262599298032,122.302736425427)) ;
#18227=CARTESIAN_POINT('Ctrl Pts',(-19.9538417565517,12.3246057809125,122.286546140861)) ;
#18228=CARTESIAN_POINT('Ctrl Pts',(-19.9386071313741,12.3238350590984,122.279299857031)) ;
#18229=CARTESIAN_POINT('Ctrl Pts',(-19.8922897410144,12.3215172354616,122.258408023563)) ;
#18230=CARTESIAN_POINT('Ctrl Pts',(-19.8607933567466,12.319977302789,122.245717969921)) ;
#18231=CARTESIAN_POINT('Ctrl Pts',(-19.8058604983243,12.317337094044,122.226145029492)) ;
#18232=CARTESIAN_POINT('Ctrl Pts',(-19.7826674169025,12.3162341222542,122.218637909037)) ;
#18233=CARTESIAN_POINT('Ctrl Pts',(-19.7495244487148,12.3146656782143,122.208971283558)) ;
#18234=CARTESIAN_POINT('Ctrl Pts',(-19.7397448889059,12.3142038406693,122.206247746719)) ;
#18235=CARTESIAN_POINT('Ctrl Pts',(-19.7241202988396,12.3134670066372,122.202100818508)) ;
#18236=CARTESIAN_POINT('Ctrl Pts',(-19.7182962793939,12.3131925825627,122.200599971301)) ;
#18237=CARTESIAN_POINT('Ctrl Pts',(-19.7095960001252,12.3127828935473,122.198424749774)) ;
#18238=CARTESIAN_POINT('Ctrl Pts',(-19.7067278040873,12.3126478750999,122.197718443499)) ;
#18239=CARTESIAN_POINT('Ctrl Pts',(-19.7037467265872,12.312507581474,122.196995537541)) ;
#18240=CARTESIAN_POINT('Ctrl Pts',(-19.7036363146429,12.3125023853904,122.19696877878)) ;
#18241=CARTESIAN_POINT('Ctrl Pts',(-19.7034191767295,12.3124921667962,122.196916185906)) ;
#18242=CARTESIAN_POINT('Ctrl Pts',(-19.703312451234,12.3124871443043,122.196890350861)) ;
#18243=CARTESIAN_POINT('Ctrl Pts',(-19.7031025646948,12.3124772671633,122.196839572895)) ;
#18244=CARTESIAN_POINT('Ctrl Pts',(-19.70299940392,12.3124724125236,122.196814629059)) ;
#18245=CARTESIAN_POINT('Ctrl Pts',(-19.7027965279017,12.3124628654805,122.196765601849)) ;
#18246=CARTESIAN_POINT('Ctrl Pts',(-19.7026968130805,12.3124581730937,122.196741517663)) ;
#18247=CARTESIAN_POINT('Ctrl Pts',(-19.7025007143907,12.312448945155,122.196694179365)) ;
#18248=CARTESIAN_POINT('Ctrl Pts',(-19.7024043305009,12.3124444095992,122.196670924393)) ;
#18249=CARTESIAN_POINT('Ctrl Pts',(-19.702214780929,12.3124354900077,122.196625214785)) ;
#18250=CARTESIAN_POINT('Ctrl Pts',(-19.7021216155958,12.3124311059859,122.196602759434)) ;
#18251=CARTESIAN_POINT('Ctrl Pts',(-19.7019383943474,12.312422484335,122.196558620482)) ;
#18252=CARTESIAN_POINT('Ctrl Pts',(-19.7018483385442,12.3124182467087,122.19653693616)) ;
#18253=CARTESIAN_POINT('Ctrl Pts',(-19.7016712305259,12.3124099128612,122.196494311572)) ;
#18254=CARTESIAN_POINT('Ctrl Pts',(-19.7015841783424,12.3124058166393,122.196473370617)) ;
#18255=CARTESIAN_POINT('Ctrl Pts',(-19.701412973721,12.312397760707,122.196432205718)) ;
#18256=CARTESIAN_POINT('Ctrl Pts',(-19.7013288217064,12.3123938010145,122.196411981227)) ;
#18257=CARTESIAN_POINT('Ctrl Pts',(-19.7011633180545,12.3123860134588,122.196372223447)) ;
#18258=CARTESIAN_POINT('Ctrl Pts',(-19.7010819663145,12.3123821855888,122.196352689529)) ;
#18259=CARTESIAN_POINT('Ctrl Pts',(-19.700921965019,12.3123746570517,122.196314287521)) ;
#18260=CARTESIAN_POINT('Ctrl Pts',(-19.7008433158003,12.3123709563986,122.196295418948)) ;
#18261=CARTESIAN_POINT('Ctrl Pts',(-19.7006886257722,12.3123636778772,122.196258323457)) ;
#18262=CARTESIAN_POINT('Ctrl Pts',(-19.7006125847527,12.3123600999972,122.196240095961)) ;
#18263=CARTESIAN_POINT('Ctrl Pts',(-19.7004630188019,12.3123530626729,122.196204258933)) ;
#18264=CARTESIAN_POINT('Ctrl Pts',(-19.7003894940058,12.3123496032333,122.19618664894)) ;
#18265=CARTESIAN_POINT('Ctrl Pts',(-19.7002448708444,12.3123427985663,122.196152023985)) ;
#18266=CARTESIAN_POINT('Ctrl Pts',(-19.7001737727723,12.3123394533511,122.196135008634)) ;
#18267=CARTESIAN_POINT('Ctrl Pts',(-19.7000339175844,12.3123328731067,122.196101551147)) ;
#18268=CARTESIAN_POINT('Ctrl Pts',(-19.6999651600884,12.3123296380582,122.196085108493)) ;
#18269=CARTESIAN_POINT('Ctrl Pts',(-19.699829901114,12.3123232741464,122.196052774817)) ;
#18270=CARTESIAN_POINT('Ctrl Pts',(-19.6997633999366,12.3123201452961,122.19603688347)) ;
#18271=CARTESIAN_POINT('Ctrl Pts',(-19.6996325719889,12.3123139899369,122.196005631727)) ;
#18272=CARTESIAN_POINT('Ctrl Pts',(-19.6995682454869,12.3123109634396,122.195990271023)) ;
#18273=CARTESIAN_POINT('Ctrl Pts',(-19.6994416886969,12.3123050091039,122.195960060793)) ;
#18274=CARTESIAN_POINT('Ctrl Pts',(-19.6993794581854,12.312302081254,122.195945210866)) ;
#18275=CARTESIAN_POINT('Ctrl Pts',(-19.6992570161039,12.3122963205741,122.195916002724)) ;
#18276=CARTESIAN_POINT('Ctrl Pts',(-19.6991968047329,12.3122934877525,122.195901644234)) ;
#18277=CARTESIAN_POINT('Ctrl Pts',(-19.695037932913,12.3120978224063,122.194910212487)) ;
#18278=CARTESIAN_POINT('Ctrl Pts',(-19.6909343665839,12.3119048291196,122.19395386642)) ;
#18279=CARTESIAN_POINT('Ctrl Pts',(-19.6827682213374,12.3115208845478,122.192094207692)) ;
#18280=CARTESIAN_POINT('Ctrl Pts',(-19.6787058098706,12.3113299397366,122.191190399446)) ;
#18281=CARTESIAN_POINT('Ctrl Pts',(-19.669033246936,12.3108754120162,122.189089080806)) ;
#18282=CARTESIAN_POINT('Ctrl Pts',(-19.6634192234708,12.3106116884295,122.187909870423)) ;
#18283=CARTESIAN_POINT('Ctrl Pts',(-19.6420652691515,12.3096088300584,122.183577790628)) ;
#18284=CARTESIAN_POINT('Ctrl Pts',(-19.6262733308779,12.3088676866191,122.18068959581)) ;
#18285=CARTESIAN_POINT('Ctrl Pts',(-19.6086221891221,12.3080397782311,122.177811549611)) ;
#18286=CARTESIAN_POINT('Ctrl Pts',(-19.606813481942,12.3079549489677,122.177520717467)) ;
#18287=CARTESIAN_POINT('Ctrl Pts',(-19.5651027493367,12.3059988467742,122.170907846769)) ;
#18288=CARTESIAN_POINT('Ctrl Pts',(-19.5249184829976,12.3041158481762,122.166520003657)) ;
#18289=CARTESIAN_POINT('Ctrl Pts',(-19.4745760993058,12.3017763554151,122.163481037315)) ;
#18290=CARTESIAN_POINT('Ctrl Pts',(-19.4645526576686,12.3013116081471,122.162997017124)) ;
#18291=CARTESIAN_POINT('Ctrl Pts',(-19.4494450108058,12.30061333689,122.162449734982)) ;
#18292=CARTESIAN_POINT('Ctrl Pts',(-19.4443645042219,12.3003789067837,122.162296712571)) ;
#18293=CARTESIAN_POINT('Ctrl Pts',(-19.4354623917786,12.2999688480163,122.162082922384)) ;
#18294=CARTESIAN_POINT('Ctrl Pts',(-19.4316412048991,12.299793051477,122.16200868719)) ;
#18295=CARTESIAN_POINT('Ctrl Pts',(-19.4242244275214,12.2994522061578,122.16189862497)) ;
#18296=CARTESIAN_POINT('Ctrl Pts',(-19.4206289054718,12.2992871386862,122.161860785317)) ;
#18297=CARTESIAN_POINT('Ctrl Pts',(-19.4129827002951,12.2989364149981,122.161813310474)) ;
#18298=CARTESIAN_POINT('Ctrl Pts',(-19.4089320310557,12.2987507982878,122.161807849719)) ;
#18299=CARTESIAN_POINT('Ctrl Pts',(-19.3996007625189,12.2983235503752,122.161840627581)) ;
#18300=CARTESIAN_POINT('Ctrl Pts',(-19.3943202852577,12.2980820295986,122.161892639038)) ;
#18301=CARTESIAN_POINT('Ctrl Pts',(-19.3637500698311,12.2966848516152,122.162387499916)) ;
#18302=CARTESIAN_POINT('Ctrl Pts',(-19.3384780035975,12.2955339128568,122.163564411745)) ;
#18303=CARTESIAN_POINT('Ctrl Pts',(-19.2906845727353,12.2933512318317,122.167246330981)) ;
#18304=CARTESIAN_POINT('Ctrl Pts',(-19.2681616561263,12.2923200618826,122.16959843275)) ;
#18305=CARTESIAN_POINT('Ctrl Pts',(-19.2401756423187,12.2910301254465,122.173292036207)) ;
#18306=CARTESIAN_POINT('Ctrl Pts',(-19.2346411055983,12.2907746070115,122.174060275935)) ;
#18307=CARTESIAN_POINT('Ctrl Pts',(-19.2223537945282,12.2902062672279,122.175849910196)) ;
#18308=CARTESIAN_POINT('Ctrl Pts',(-19.2156038663577,12.2898933420975,122.176889590148)) ;
#18309=CARTESIAN_POINT('Ctrl Pts',(-19.1904972080944,12.2887270000533,122.180967632988)) ;
#18310=CARTESIAN_POINT('Ctrl Pts',(-19.1722005295293,12.2878722713777,122.184360417084)) ;
#18311=CARTESIAN_POINT('Ctrl Pts',(-19.1403098492094,12.2863757976791,122.191013635334)) ;
#18312=CARTESIAN_POINT('Ctrl Pts',(-19.1266825098048,12.2857341492844,122.194095921746)) ;
#18313=CARTESIAN_POINT('Ctrl Pts',(-19.110813865766,12.2849845803541,122.197965870317)) ;
#18314=CARTESIAN_POINT('Ctrl Pts',(-19.1085168015902,12.284876020602,122.198532961923)) ;
#18315=CARTESIAN_POINT('Ctrl Pts',(-19.1015386210917,12.2845460392018,122.200276781587)) ;
#18316=CARTESIAN_POINT('Ctrl Pts',(-19.096862691438,12.2843246784062,122.201474094536)) ;
#18317=CARTESIAN_POINT('Ctrl Pts',(-19.0827599510133,12.2836562933839,122.205172395672)) ;
#18318=CARTESIAN_POINT('Ctrl Pts',(-19.0733553516249,12.2832095543121,122.20775665796)) ;
#18319=CARTESIAN_POINT('Ctrl Pts',(-19.0523916685137,12.2822113184325,122.213781941223)) ;
#18320=CARTESIAN_POINT('Ctrl Pts',(-19.0408501819625,12.281660090464,122.217280724036)) ;
#18321=CARTESIAN_POINT('Ctrl Pts',(-19.0153625143223,12.2804385890047,122.225411806087)) ;
#18322=CARTESIAN_POINT('Ctrl Pts',(-19.0014437770044,12.2797688841339,122.230124114127)) ;
#18323=CARTESIAN_POINT('Ctrl Pts',(-18.9712843919364,12.2783081133726,122.240931176282)) ;
#18324=CARTESIAN_POINT('Ctrl Pts',(-18.9550810446259,12.2775169566702,122.247120777925)) ;
#18325=CARTESIAN_POINT('Ctrl Pts',(-18.9323864157559,12.2763968647427,122.25633565762)) ;
#18326=CARTESIAN_POINT('Ctrl Pts',(-18.9257842783509,12.2760695777695,122.259082599512)) ;
#18327=CARTESIAN_POINT('Ctrl Pts',(-18.918638433755,12.2757136824681,122.262127951505)) ;
#18328=CARTESIAN_POINT('Ctrl Pts',(-18.9180709595142,12.2756854083269,122.262370289258)) ;
#18329=CARTESIAN_POINT('Ctrl Pts',(-18.9117455598407,12.2753701210517,122.265077067178)) ;
#18330=CARTESIAN_POINT('Ctrl Pts',(-18.9060060664993,12.2750828608151,122.267584324291)) ;
#18331=CARTESIAN_POINT('Ctrl Pts',(-18.9002450930505,12.2747933090545,122.270152696087)) ;
#18332=CARTESIAN_POINT('Ctrl Pts',(-18.9002045177652,12.2747912696429,122.270170788056)) ;
#18333=CARTESIAN_POINT('Ctrl Pts',(-18.9001238435967,12.2747872146438,122.270206764731)) ;
#18334=CARTESIAN_POINT('Ctrl Pts',(-18.9000837447658,12.2747851990603,122.270224649351)) ;
#18335=CARTESIAN_POINT('Ctrl Pts',(-18.9000039974015,12.2747811904094,122.270260222792)) ;
#18336=CARTESIAN_POINT('Ctrl Pts',(-18.8999643486846,12.2747791973341,122.270277911637)) ;
#18337=CARTESIAN_POINT('Ctrl Pts',(-18.8998854756348,12.2747752324008,122.270313104921)) ;
#18338=CARTESIAN_POINT('Ctrl Pts',(-18.8998462514276,12.2747732605504,122.270330609251)) ;
#18339=CARTESIAN_POINT('Ctrl Pts',(-18.8997682031301,12.2747693368507,122.270365444176)) ;
#18340=CARTESIAN_POINT('Ctrl Pts',(-18.8997293789889,12.274767385,122.270382774746)) ;
#18341=CARTESIAN_POINT('Ctrl Pts',(-18.8996521075579,12.2747635001334,122.270417272393)) ;
#18342=CARTESIAN_POINT('Ctrl Pts',(-18.8996136600522,12.2747615671078,122.27043443952)) ;
#18343=CARTESIAN_POINT('Ctrl Pts',(-18.8901227457624,12.2742843787962,122.274672785936)) ;
#18344=CARTESIAN_POINT('Ctrl Pts',(-18.8807231096184,12.2738084572363,122.279011211801)) ;
#18345=CARTESIAN_POINT('Ctrl Pts',(-18.8584552144583,12.2726730772487,122.289626515565)) ;
#18346=CARTESIAN_POINT('Ctrl Pts',(-18.8456387735708,12.2720131872733,122.296008701345)) ;
#18347=CARTESIAN_POINT('Ctrl Pts',(-18.8034859099685,12.2698233381113,122.317911124905)) ;
#18348=CARTESIAN_POINT('Ctrl Pts',(-18.7746579481472,12.268296215917,122.334379405317)) ;
#18349=CARTESIAN_POINT('Ctrl Pts',(-18.729774918897,12.2658636237062,122.36244626291)) ;
#18350=CARTESIAN_POINT('Ctrl Pts',(-18.7132808206666,12.2649570395387,122.373312573618)) ;
#18351=CARTESIAN_POINT('Ctrl Pts',(-18.6858255325879,12.2634248487849,122.392348106488)) ;
#18352=CARTESIAN_POINT('Ctrl Pts',(-18.6747282917063,12.2627989047404,122.400314597226)) ;
#18353=CARTESIAN_POINT('Ctrl Pts',(-18.6588867192605,12.2618953578861,122.412085156003)) ;
#18354=CARTESIAN_POINT('Ctrl Pts',(-18.6540360857326,12.2616173103472,122.41574445152)) ;
#18355=CARTESIAN_POINT('Ctrl Pts',(-18.6196057881474,12.2596336692377,122.442114602542)) ;
#18356=CARTESIAN_POINT('Ctrl Pts',(-18.5910288274408,12.25793525988,122.46610380482)) ;
#18357=CARTESIAN_POINT('Ctrl Pts',(-18.5446811999161,12.2550642157518,122.508686412553)) ;
#18358=CARTESIAN_POINT('Ctrl Pts',(-18.5263338269143,12.2538936811264,122.526615225297)) ;
#18359=CARTESIAN_POINT('Ctrl Pts',(-18.5004252806398,12.2521846431382,122.553540196993)) ;
#18360=CARTESIAN_POINT('Ctrl Pts',(-18.4924186937888,12.2516482177633,122.562098579029)) ;
#18361=CARTESIAN_POINT('Ctrl Pts',(-18.4765275394243,12.2505661431255,122.579571061819)) ;
#18362=CARTESIAN_POINT('Ctrl Pts',(-18.4686475438167,12.2500205336862,122.588487715261)) ;
#18363=CARTESIAN_POINT('Ctrl Pts',(-18.4596648071987,12.2493877277592,122.598949492375)) ;
#18364=CARTESIAN_POINT('Ctrl Pts',(-18.4584367967134,12.2493009783825,122.600386279844)) ;
#18365=CARTESIAN_POINT('Ctrl Pts',(-18.4540964245262,12.2489935107512,122.605487951596)) ;
#18366=CARTESIAN_POINT('Ctrl Pts',(-18.4510019563454,12.248772737706,122.609168000239)) ;
#18367=CARTESIAN_POINT('Ctrl Pts',(-18.4364374526138,12.2477261432029,122.626692895836)) ;
#18368=CARTESIAN_POINT('Ctrl Pts',(-18.4252457743225,12.2468996133807,122.640766274439)) ;
#18369=CARTESIAN_POINT('Ctrl Pts',(-18.3970626550235,12.2447585189469,122.677819622791)) ;
#18370=CARTESIAN_POINT('Ctrl Pts',(-18.3805486588605,12.2434439300822,122.7011496581)) ;
#18371=CARTESIAN_POINT('Ctrl Pts',(-18.3641079048297,12.2420706366636,122.72615166601)) ;
#18372=CARTESIAN_POINT('Ctrl Pts',(-18.363368930255,12.2420087663343,122.727279419964)) ;
#18373=CARTESIAN_POINT('Ctrl Pts',(-18.3618263016116,12.2418793090405,122.729641965138)) ;
#18374=CARTESIAN_POINT('Ctrl Pts',(-18.3610230029253,12.241811723894,122.730876986113)) ;
#18375=CARTESIAN_POINT('Ctrl Pts',(-18.3592869206189,12.2416652856262,122.733556455323)) ;
#18376=CARTESIAN_POINT('Ctrl Pts',(-18.3583549299985,12.2415864367627,122.735001414096)) ;
#18377=CARTESIAN_POINT('Ctrl Pts',(-18.35578853018,12.2413686612092,122.738998443687)) ;
#18378=CARTESIAN_POINT('Ctrl Pts',(-18.3541604150833,12.2412297703263,122.741554543885)) ;
#18379=CARTESIAN_POINT('Ctrl Pts',(-18.34901876643,12.2407888109909,122.749691963831)) ;
#18380=CARTESIAN_POINT('Ctrl Pts',(-18.3455401023303,12.2404869920065,122.755295178696)) ;
#18381=CARTESIAN_POINT('Ctrl Pts',(-18.3379625151143,12.2398216208448,122.767719032272)) ;
#18382=CARTESIAN_POINT('Ctrl Pts',(-18.3338840517041,12.2394581818918,122.774551805886)) ;
#18383=CARTESIAN_POINT('Ctrl Pts',(-18.3203920329754,12.2382369966701,122.797653806684)) ;
#18384=CARTESIAN_POINT('Ctrl Pts',(-18.311280246106,12.2373803772665,122.814096304466)) ;
#18385=CARTESIAN_POINT('Ctrl Pts',(-18.2911935706694,12.2354100982693,122.85235378503)) ;
#18386=CARTESIAN_POINT('Ctrl Pts',(-18.2804801919914,12.2342965057199,122.874297335255)) ;
#18387=CARTESIAN_POINT('Ctrl Pts',(-18.2662453165183,12.2327174067882,122.905759187717)) ;
#18388=CARTESIAN_POINT('Ctrl Pts',(-18.2621864058117,12.2322543060521,122.915028215334)) ;
#18389=CARTESIAN_POINT('Ctrl Pts',(-18.2550235982066,12.2314127743658,122.931941333661)) ;
#18390=CARTESIAN_POINT('Ctrl Pts',(-18.251881982541,12.2310345295728,122.939568830559)) ;
#18391=CARTESIAN_POINT('Ctrl Pts',(-18.2479664032967,12.2305510393385,122.949349243928)) ;
#18392=CARTESIAN_POINT('Ctrl Pts',(-18.2471225296527,12.2304460958085,122.951473963436)) ;
#18393=CARTESIAN_POINT('Ctrl Pts',(-18.2454472212734,12.2302362570263,122.955726050333)) ;
#18394=CARTESIAN_POINT('Ctrl Pts',(-18.2446157789638,12.2301313622132,122.957853405489)) ;
#18395=CARTESIAN_POINT('Ctrl Pts',(-18.2430841197492,12.2299367181332,122.961804263218)) ;
#18396=CARTESIAN_POINT('Ctrl Pts',(-18.2423823371754,12.2298469755033,122.963627151649)) ;
#18397=CARTESIAN_POINT('Ctrl Pts',(-18.233728298671,12.2287333183734,122.986264228168)) ;
#18398=CARTESIAN_POINT('Ctrl Pts',(-18.2263297036955,12.2277073069662,123.007285718844)) ;
#18399=CARTESIAN_POINT('Ctrl Pts',(-18.214337801579,12.2259042432553,123.044506945988)) ;
#18400=CARTESIAN_POINT('Ctrl Pts',(-18.2095024578894,12.2251279733657,123.060622791061)) ;
#18401=CARTESIAN_POINT('Ctrl Pts',(-18.1998067486145,12.2234591172079,123.095479277654)) ;
#18402=CARTESIAN_POINT('Ctrl Pts',(-18.1950534336388,12.2225668174507,123.114245284689)) ;
#18403=CARTESIAN_POINT('Ctrl Pts',(-18.1893717760513,12.2213952032092,123.139086654396)) ;
#18404=CARTESIAN_POINT('Ctrl Pts',(-18.1880496822321,12.2211137745665,123.145069147926)) ;
#18405=CARTESIAN_POINT('Ctrl Pts',(-18.1857893972217,12.2206166445939,123.155666139424)) ;
#18406=CARTESIAN_POINT('Ctrl Pts',(-18.1848331988293,12.220400819434,123.160276664812)) ;
#18407=CARTESIAN_POINT('Ctrl Pts',(-18.1824333868243,12.2198443859124,123.172185919867)) ;
#18408=CARTESIAN_POINT('Ctrl Pts',(-18.1810288431811,12.2195040264401,123.17949234274)) ;
#18409=CARTESIAN_POINT('Ctrl Pts',(-18.1766059563161,12.2183807461962,123.20366221221)) ;
#18410=CARTESIAN_POINT('Ctrl Pts',(-18.1738690426115,12.2175989178843,123.22057517632)) ;
#18411=CARTESIAN_POINT('Ctrl Pts',(-18.1691061808155,12.21603901677,123.254403436511)) ;
#18412=CARTESIAN_POINT('Ctrl Pts',(-18.1670766631612,12.2152611132664,123.27131453819)) ;
#18413=CARTESIAN_POINT('Ctrl Pts',(-18.1646428192148,12.2141343776665,123.295817523801)) ;
#18414=CARTESIAN_POINT('Ctrl Pts',(-18.1639611801692,12.2137866922403,123.303379932456)) ;
#18415=CARTESIAN_POINT('Ctrl Pts',(-18.1628689072857,12.2131663096348,123.316871938782)) ;
#18416=CARTESIAN_POINT('Ctrl Pts',(-18.1624315836002,12.2128937404882,123.322799144614)) ;
#18417=CARTESIAN_POINT('Ctrl Pts',(-18.1614290089668,12.2122014674298,123.337849332735)) ;
#18418=CARTESIAN_POINT('Ctrl Pts',(-18.1609215222235,12.2117815076055,123.346975797005)) ;
#18419=CARTESIAN_POINT('Ctrl Pts',(-18.1602635259034,12.2111023445527,123.361725694803)) ;
#18420=CARTESIAN_POINT('Ctrl Pts',(-18.1600507988238,12.2108434482576,123.36734602186)) ;
#18421=CARTESIAN_POINT('Ctrl Pts',(-18.15929935674,12.2097297218122,123.391514022561)) ;
#18422=CARTESIAN_POINT('Ctrl Pts',(-18.1591357380438,12.2088736550973,123.410070988659)) ;
#18423=CARTESIAN_POINT('Ctrl Pts',(-18.1595676857259,12.2073935829303,123.442187280998)) ;
#18424=CARTESIAN_POINT('Ctrl Pts',(-18.1599708359102,12.2067691775243,123.455746029733)) ;
#18425=CARTESIAN_POINT('Ctrl Pts',(-18.1608769099055,12.2058638878957,123.475428887471)) ;
#18426=CARTESIAN_POINT('Ctrl Pts',(-18.1612044345401,12.205582049248,123.481560052821)) ;
#18427=CARTESIAN_POINT('Ctrl Pts',(-18.1618840520735,12.2050686225412,123.492735860338)) ;
#18428=CARTESIAN_POINT('Ctrl Pts',(-18.1622216097911,12.2048369459569,123.497781252151)) ;
#18429=CARTESIAN_POINT('Ctrl Pts',(-18.1629363815045,12.2043875693017,123.507572400197)) ;
#18430=CARTESIAN_POINT('Ctrl Pts',(-18.1633101105923,12.2041698487456,123.512318323823)) ;
#18431=CARTESIAN_POINT('Ctrl Pts',(-18.1642130828346,12.2036798223058,123.5230046184)) ;
#18432=CARTESIAN_POINT('Ctrl Pts',(-18.1647577459922,12.2034076348197,123.528943575076)) ;
#18433=CARTESIAN_POINT('Ctrl Pts',(-18.1674587481127,12.2021569478018,123.556245214178)) ;
#18434=CARTESIAN_POINT('Ctrl Pts',(-18.1701214789119,12.2011833699327,123.577544331091)) ;
#18435=CARTESIAN_POINT('Ctrl Pts',(-18.1733329056176,12.2002114875201,123.598774179907)) ;
#18436=CARTESIAN_POINT('Origin',(-19.409269639048,-13.9999999999504,123.411833654989)) ;
#18437=CARTESIAN_POINT('',(-17.409466984686,-13.6999999999504,123.383738395492)) ;
#18438=CARTESIAN_POINT('Origin',(-19.4092696390481,-13.6999999999504,123.411833654989)) ;
#18439=CARTESIAN_POINT('',(-17.409466984686,13.7000000000496,123.383738395492)) ;
#18440=CARTESIAN_POINT('',(-17.4094669846859,-13.9999999999504,123.383738395492)) ;
#18441=CARTESIAN_POINT('Origin',(-19.4092696390481,13.7000000000496,123.411833654989)) ;
#18442=CARTESIAN_POINT('',(-21.3014729215226,12.450000004364,122.764093940449)) ;
#18443=CARTESIAN_POINT('Ctrl Pts',(-21.3014729215226,12.4500000043639,122.764093940449)) ;
#18444=CARTESIAN_POINT('Ctrl Pts',(-21.2417386817332,12.4533908072994,122.58468313231)) ;
#18445=CARTESIAN_POINT('Ctrl Pts',(-21.1183669661588,12.3003323944147,122.368106075024)) ;
#18446=CARTESIAN_POINT('Ctrl Pts',(-21.0828841600767,12.0313004597594,122.317703938634)) ;
#18447=CARTESIAN_POINT('Ctrl Pts',(-21.0912110587446,11.9055147635765,122.329236338449)) ;
#18448=CARTESIAN_POINT('Ctrl Pts',(-21.1188098709144,11.7623911882616,122.373395814998)) ;
#18449=CARTESIAN_POINT('Ctrl Pts',(-21.1966797848952,11.6016650881281,122.503047298049)) ;
#18450=CARTESIAN_POINT('Ctrl Pts',(-21.3085421953233,11.5240330679577,122.761739092861)) ;
#18451=CARTESIAN_POINT('Ctrl Pts',(-21.3785516269951,11.6016367477315,123.03446770917)) ;
#18452=CARTESIAN_POINT('Ctrl Pts',(-21.3966874043036,11.7624517905451,123.184919968199)) ;
#18453=CARTESIAN_POINT('Ctrl Pts',(-21.4016453124917,11.905416630659,123.236367319138)) ;
#18454=CARTESIAN_POINT('Ctrl Pts',(-21.4027247828246,12.0315229430405,123.251325161369)) ;
#18455=CARTESIAN_POINT('Ctrl Pts',(-21.3995856881047,12.2128162203883,123.208193040234)) ;
#18456=CARTESIAN_POINT('Ctrl Pts',(-21.3783532801531,12.3983256286576,123.034306001354)) ;
#18457=CARTESIAN_POINT('Ctrl Pts',(-21.3321155076486,12.450187696004,122.852788427119)) ;
#18458=CARTESIAN_POINT('Ctrl Pts',(-21.3014729215226,12.4500000043639,122.764093940449)) ;
#18459=CARTESIAN_POINT('',(-17.5170663566028,12.4500000035941,124.059573369615)) ;
#18460=CARTESIAN_POINT('Ctrl Pts',(-17.5170663566028,12.4500000035941,124.059573369615)) ;
#18461=CARTESIAN_POINT('Ctrl Pts',(-17.5768010750503,12.4533889497169,124.238978500622)) ;
#18462=CARTESIAN_POINT('Ctrl Pts',(-17.7001719976827,12.3003338187364,124.455565035223)) ;
#18463=CARTESIAN_POINT('Ctrl Pts',(-17.735655182611,12.0313017495778,124.505966784337)) ;
#18464=CARTESIAN_POINT('Ctrl Pts',(-17.727328311671,11.9055139654912,124.494427918119)) ;
#18465=CARTESIAN_POINT('Ctrl Pts',(-17.6997289374594,11.7623915473154,124.450272614137)) ;
#18466=CARTESIAN_POINT('Ctrl Pts',(-17.6218598761679,11.6016648611214,124.320619335508)) ;
#18467=CARTESIAN_POINT('Ctrl Pts',(-17.5099968647986,11.5240331921794,124.061928577266)) ;
#18468=CARTESIAN_POINT('Ctrl Pts',(-17.4399877214087,11.6016367193622,123.789199422435)) ;
#18469=CARTESIAN_POINT('Ctrl Pts',(-17.4218519288077,11.7624517529768,123.638747342328)) ;
#18470=CARTESIAN_POINT('Ctrl Pts',(-17.4168941310285,11.9054163828466,123.587299846138)) ;
#18471=CARTESIAN_POINT('Ctrl Pts',(-17.415814460062,12.0315228305656,123.572342418142)) ;
#18472=CARTESIAN_POINT('Ctrl Pts',(-17.4189536889037,12.2128158889338,123.615474365746)) ;
#18473=CARTESIAN_POINT('Ctrl Pts',(-17.4401858916256,12.3983259401867,123.789361234211)) ;
#18474=CARTESIAN_POINT('Ctrl Pts',(-17.486423826463,12.4501875413069,123.970878916215)) ;
#18475=CARTESIAN_POINT('Ctrl Pts',(-17.5170663566028,12.4500000035941,124.059573369615)) ;
#18476=CARTESIAN_POINT('',(-17.5170663564952,-12.4500000035939,124.059573369301)) ;
#18477=CARTESIAN_POINT('Ctrl Pts',(-17.5170663564952,-12.4500000035939,
124.059573369301)) ;
#18478=CARTESIAN_POINT('Ctrl Pts',(-17.4543214499664,-12.4533908062079,
123.881193173708)) ;
#18479=CARTESIAN_POINT('Ctrl Pts',(-17.4190874317839,-12.3003323949396,
123.634444787988)) ;
#18480=CARTESIAN_POINT('Ctrl Pts',(-17.4162387146148,-12.0313004596384,
123.572871338394)) ;
#18481=CARTESIAN_POINT('Ctrl Pts',(-17.4167260337872,-11.905514763682,123.587087385896)) ;
#18482=CARTESIAN_POINT('Ctrl Pts',(-17.4219791397424,-11.76239118819,123.638896252699)) ;
#18483=CARTESIAN_POINT('Ctrl Pts',(-17.4398990467708,-11.6016650883087,
123.789069843982)) ;
#18484=CARTESIAN_POINT('Ctrl Pts',(-17.5100369831582,-11.5240330679591,
124.062044775725)) ;
#18485=CARTESIAN_POINT('Ctrl Pts',(-17.6218499912451,-11.6016367475424,
124.320463176737)) ;
#18486=CARTESIAN_POINT('Ctrl Pts',(-17.6997200962288,-11.7624517905878,
124.450467158943)) ;
#18487=CARTESIAN_POINT('Ctrl Pts',(-17.7273306316869,-11.9054166305896,
124.494160054312)) ;
#18488=CARTESIAN_POINT('Ctrl Pts',(-17.7356441949461,-12.0315229428807,
124.50664151924)) ;
#18489=CARTESIAN_POINT('Ctrl Pts',(-17.7116922052291,-12.2128162206925,
124.470634075889)) ;
#18490=CARTESIAN_POINT('Ctrl Pts',(-17.6219076292031,-12.3983256278298,
124.320213840095)) ;
#18491=CARTESIAN_POINT('Ctrl Pts',(-17.5472065053376,-12.4501876978419,
124.148439850519)) ;
#18492=CARTESIAN_POINT('Ctrl Pts',(-17.5170663564952,-12.4500000035939,
124.059573369301)) ;
#18493=CARTESIAN_POINT('',(-21.3014729215271,-12.4500000013844,122.764093940462)) ;
#18494=CARTESIAN_POINT('Ctrl Pts',(-21.3014729215271,-12.4500000013844,
122.764093940462)) ;
#18495=CARTESIAN_POINT('Ctrl Pts',(-21.3642139707748,-12.4533889553457,
122.942469943529)) ;
#18496=CARTESIAN_POINT('Ctrl Pts',(-21.3994544235377,-12.3003338159049,
123.189225332334)) ;
#18497=CARTESIAN_POINT('Ctrl Pts',(-21.4023026040227,-12.031301750527,123.250798708205)) ;
#18498=CARTESIAN_POINT('Ctrl Pts',(-21.4018113001397,-11.9055139651401,
123.236577567789)) ;
#18499=CARTESIAN_POINT('Ctrl Pts',(-21.3965611953891,-11.7623915476468,
123.184771653818)) ;
#18500=CARTESIAN_POINT('Ctrl Pts',(-21.3786395141694,-11.6016648610055,
123.034597166172)) ;
#18501=CARTESIAN_POINT('Ctrl Pts',(-21.3085026878959,-11.5240331923606,
122.761622685277)) ;
#18502=CARTESIAN_POINT('Ctrl Pts',(-21.1966891219787,-11.6016367190622,
122.503204035368)) ;
#18503=CARTESIAN_POINT('Ctrl Pts',(-21.118819138729,-11.7624517530713,122.373200185185)) ;
#18504=CARTESIAN_POINT('Ctrl Pts',(-21.0912084270103,-11.9054163827587,
122.329507242695)) ;
#18505=CARTESIAN_POINT('Ctrl Pts',(-21.0828952761476,-12.0315228306677,
122.317025982144)) ;
#18506=CARTESIAN_POINT('Ctrl Pts',(-21.1068470535444,-12.212815888551,122.353033370586)) ;
#18507=CARTESIAN_POINT('Ctrl Pts',(-21.1966316872743,-12.3983259410573,
122.503453345861)) ;
#18508=CARTESIAN_POINT('Ctrl Pts',(-21.2713327489301,-12.450187539844,122.675227520146)) ;
#18509=CARTESIAN_POINT('Ctrl Pts',(-21.3014729215271,-12.4500000013844,
122.764093940462)) ;
#18510=CARTESIAN_POINT('Origin',(-17.409466984686,-13.9999999999504,123.383738395492)) ;
#18511=CARTESIAN_POINT('',(-17.7094373828403,-13.9999999999504,123.387952684416)) ;
#18512=CARTESIAN_POINT('Ctrl Pts',(-17.7094373828403,-13.9999999999504,
123.387952684416)) ;
#18513=CARTESIAN_POINT('Ctrl Pts',(-17.7124365161054,-13.9999999999504,
123.165469985201)) ;
#18514=CARTESIAN_POINT('Ctrl Pts',(-17.8073115029348,-13.9999999999504,
122.721754746081)) ;
#18515=CARTESIAN_POINT('Ctrl Pts',(-18.1932733581975,-13.9999999999504,
122.161208794752)) ;
#18516=CARTESIAN_POINT('Ctrl Pts',(-18.7644631958589,-13.9999999999504,
121.791079731755)) ;
#18517=CARTESIAN_POINT('Ctrl Pts',(-19.4337624984685,-13.9999999999504,
121.66769040749)) ;
#18518=CARTESIAN_POINT('Ctrl Pts',(-20.0993607034912,-13.9999999999504,
121.809828608283)) ;
#18519=CARTESIAN_POINT('Ctrl Pts',(-20.659887032884,-13.9999999999504,122.195860778204)) ;
#18520=CARTESIAN_POINT('Ctrl Pts',(-21.0300277648269,-13.9999999999504,
122.767014628009)) ;
#18521=CARTESIAN_POINT('Ctrl Pts',(-21.153410552117,-13.9999999999504,123.436333440585)) ;
#18522=CARTESIAN_POINT('Ctrl Pts',(-21.0112760309154,-13.9999999999504,
124.101920740338)) ;
#18523=CARTESIAN_POINT('Ctrl Pts',(-20.6252417466303,-13.9999999999504,
124.66245330923)) ;
#18524=CARTESIAN_POINT('Ctrl Pts',(-20.0540890803186,-13.9999999999504,
125.032590535832)) ;
#18525=CARTESIAN_POINT('Ctrl Pts',(-19.3847696171533,-13.9999999999504,
125.155975257797)) ;
#18526=CARTESIAN_POINT('Ctrl Pts',(-18.7191817607919,-13.9999999999504,
125.013838725625)) ;
#18527=CARTESIAN_POINT('Ctrl Pts',(-18.1586286713331,-13.9999999999504,
124.627806965402)) ;
#18528=CARTESIAN_POINT('Ctrl Pts',(-17.7885531153341,-13.9999999999504,
124.056641767528)) ;
#18529=CARTESIAN_POINT('Ctrl Pts',(-17.7061836816795,-13.9999999999504,
123.610445192173)) ;
#18530=CARTESIAN_POINT('Ctrl Pts',(-17.7094373828403,-13.9999999999504,
123.387952684416)) ;
#18531=CARTESIAN_POINT('',(-18.6398461652381,-13.9999999999504,124.699448408814)) ;
#18532=CARTESIAN_POINT('Ctrl Pts',(-20.5016202458523,-13.9999999999504,
122.804133672988)) ;
#18533=CARTESIAN_POINT('Ctrl Pts',(-20.5261753546306,-13.9999999972095,
122.841288201641)) ;
#18534=CARTESIAN_POINT('Ctrl Pts',(-20.5488739735137,-13.9999999999504,
122.87995874555)) ;
#18535=CARTESIAN_POINT('Ctrl Pts',(-20.569533497391,-13.9999999999504,122.92000295199)) ;
#18536=CARTESIAN_POINT('Ctrl Pts',(-20.5959199140017,-13.9999999999504,
122.971147553399)) ;
#18537=CARTESIAN_POINT('Ctrl Pts',(-20.6189710732946,-14.0000000058558,
123.02451774586)) ;
#18538=CARTESIAN_POINT('Ctrl Pts',(-20.6383380498207,-14.000000002076,123.079380090936)) ;
#18539=CARTESIAN_POINT('Ctrl Pts',(-20.6436137949561,-14.0000000010463,
123.094325105702)) ;
#18540=CARTESIAN_POINT('Ctrl Pts',(-20.6486160641444,-13.9999999999504,
123.109380562199)) ;
#18541=CARTESIAN_POINT('Ctrl Pts',(-20.6533376246053,-13.9999999999504,
123.124530986896)) ;
#18542=CARTESIAN_POINT('Ctrl Pts',(-20.6753389534758,-13.9999999999504,
123.195128298747)) ;
#18543=CARTESIAN_POINT('Ctrl Pts',(-20.6912550483959,-13.9999999999504,
123.267816352402)) ;
#18544=CARTESIAN_POINT('Ctrl Pts',(-20.7007692461713,-13.9999999999504,
123.342502211065)) ;
#18545=CARTESIAN_POINT('Ctrl Pts',(-20.7075651409922,-13.9999999999504,
123.395849561211)) ;
#18546=CARTESIAN_POINT('Ctrl Pts',(-20.7110948242437,-14.0000000154151,
123.450221687122)) ;
#18547=CARTESIAN_POINT('Ctrl Pts',(-20.7112100367005,-14.0000000076297,
123.504837175163)) ;
#18548=CARTESIAN_POINT('Ctrl Pts',(-20.7112556701211,-14.000000004546,123.526469311179)) ;
#18549=CARTESIAN_POINT('Ctrl Pts',(-20.7107656107305,-13.9999999999504,
123.548139053146)) ;
#18550=CARTESIAN_POINT('Ctrl Pts',(-20.7097305817929,-13.9999999999504,
123.569795580814)) ;
#18551=CARTESIAN_POINT('Ctrl Pts',(-20.7060894144257,-13.9999999999504,
123.645981896936)) ;
#18552=CARTESIAN_POINT('Ctrl Pts',(-20.6957047852943,-13.9999999999504,
123.721939102819)) ;
#18553=CARTESIAN_POINT('Ctrl Pts',(-20.6787691492058,-13.9999999999504,
123.796817076466)) ;
#18554=CARTESIAN_POINT('Ctrl Pts',(-20.6618718109643,-13.9999999999504,
123.871525722834)) ;
#18555=CARTESIAN_POINT('Ctrl Pts',(-20.6384362784418,-13.9999999999504,
123.945249174943)) ;
#18556=CARTESIAN_POINT('Ctrl Pts',(-20.6081226092438,-13.9999999999504,
124.017450827467)) ;
#18557=CARTESIAN_POINT('Ctrl Pts',(-20.5874065939798,-13.9999999999504,
124.06679261206)) ;
#18558=CARTESIAN_POINT('Ctrl Pts',(-20.5634867253231,-14.0000000147266,
124.115399835518)) ;
#18559=CARTESIAN_POINT('Ctrl Pts',(-20.5367348692554,-14.000000008255,124.162498288013)) ;
#18560=CARTESIAN_POINT('Ctrl Pts',(-20.5244438287527,-14.0000000052816,
124.184137496364)) ;
#18561=CARTESIAN_POINT('Ctrl Pts',(-20.511555350795,-13.9999999999504,124.205457596068)) ;
#18562=CARTESIAN_POINT('Ctrl Pts',(-20.4981075052899,-13.9999999999504,
124.226380393993)) ;
#18563=CARTESIAN_POINT('Ctrl Pts',(-20.4617166845242,-13.9999999999504,
124.282998964521)) ;
#18564=CARTESIAN_POINT('Ctrl Pts',(-20.421232808245,-13.9999999879782,124.33670346053)) ;
#18565=CARTESIAN_POINT('Ctrl Pts',(-20.376464367816,-13.9999999971152,124.38762656574)) ;
#18566=CARTESIAN_POINT('Ctrl Pts',(-20.3687787652624,-13.9999999986838,
124.396368767695)) ;
#18567=CARTESIAN_POINT('Ctrl Pts',(-20.3609668115105,-13.9999999999504,
124.405029094405)) ;
#18568=CARTESIAN_POINT('Ctrl Pts',(-20.3530274377726,-13.9999999999504,
124.413608334624)) ;
#18569=CARTESIAN_POINT('Ctrl Pts',(-20.3133866407383,-13.9999999999504,
124.456443945021)) ;
#18570=CARTESIAN_POINT('Ctrl Pts',(-20.2705399280199,-14.0000000149581,
124.497290243693)) ;
#18571=CARTESIAN_POINT('Ctrl Pts',(-20.224931493167,-14.0000000069191,124.535470774106)) ;
#18572=CARTESIAN_POINT('Ctrl Pts',(-20.2082439815189,-14.0000000039777,
124.549440515625)) ;
#18573=CARTESIAN_POINT('Ctrl Pts',(-20.1911870824665,-13.9999999999504,
124.563053006214)) ;
#18574=CARTESIAN_POINT('Ctrl Pts',(-20.1737837366749,-13.9999999999504,
124.576273823417)) ;
#18575=CARTESIAN_POINT('Ctrl Pts',(-20.1180757041767,-13.9999999999504,
124.618593600501)) ;
#18576=CARTESIAN_POINT('Ctrl Pts',(-20.0588712508305,-14.0000000011967,
124.656857916382)) ;
#18577=CARTESIAN_POINT('Ctrl Pts',(-19.9969857205583,-14.0000000002329,
124.690555964017)) ;
#18578=CARTESIAN_POINT('Ctrl Pts',(-19.9868756103298,-14.0000000000754,
124.696061143896)) ;
#18579=CARTESIAN_POINT('Ctrl Pts',(-19.9766940496221,-13.9999999999504,
124.70144441283)) ;
#18580=CARTESIAN_POINT('Ctrl Pts',(-19.9664447168996,-13.9999999999504,
124.706703495921)) ;
#18581=CARTESIAN_POINT('Ctrl Pts',(-19.8937152512031,-13.9999999999504,
124.744022052514)) ;
#18582=CARTESIAN_POINT('Ctrl Pts',(-19.8175500316,-13.9999999999504,124.77509885579)) ;
#18583=CARTESIAN_POINT('Ctrl Pts',(-19.7385237038216,-13.9999999999504,
124.799520306937)) ;
#18584=CARTESIAN_POINT('Ctrl Pts',(-19.6697538216838,-13.9999999999504,
124.820772215817)) ;
#18585=CARTESIAN_POINT('Ctrl Pts',(-19.5987827926167,-14.0000000007161,
124.83699506817)) ;
#18586=CARTESIAN_POINT('Ctrl Pts',(-19.5264286897744,-14.0000000001071,
124.84774949464)) ;
#18587=CARTESIAN_POINT('Ctrl Pts',(-19.5158346133764,-14.000000000018,124.849324156078)) ;
#18588=CARTESIAN_POINT('Ctrl Pts',(-19.5052109717312,-13.9999999999504,
124.850781551346)) ;
#18589=CARTESIAN_POINT('Ctrl Pts',(-19.4945604218811,-13.9999999999504,
124.852120270616)) ;
#18590=CARTESIAN_POINT('Ctrl Pts',(-19.4278676945074,-13.9999999999504,
124.860503203003)) ;
#18591=CARTESIAN_POINT('Ctrl Pts',(-19.3601518171623,-14.0000000039356,
124.864227805718)) ;
#18592=CARTESIAN_POINT('Ctrl Pts',(-19.2923487645647,-14.0000000012686,
124.863241788224)) ;
#18593=CARTESIAN_POINT('Ctrl Pts',(-19.2755599993829,-14.0000000006082,
124.862997639686)) ;
#18594=CARTESIAN_POINT('Ctrl Pts',(-19.2587661385357,-13.9999999999504,
124.86246469874)) ;
#18595=CARTESIAN_POINT('Ctrl Pts',(-19.2419818835215,-13.9999999999504,
124.861642219978)) ;
#18596=CARTESIAN_POINT('Ctrl Pts',(-19.1575942447879,-13.9999999999504,
124.857506972949)) ;
#18597=CARTESIAN_POINT('Ctrl Pts',(-19.0734016471759,-13.9999999999504,
124.846051708994)) ;
#18598=CARTESIAN_POINT('Ctrl Pts',(-18.9895877266166,-13.9999999999504,
124.826900874729)) ;
#18599=CARTESIAN_POINT('Ctrl Pts',(-18.93283525063,-13.9999999999504,124.813933371784)) ;
#18600=CARTESIAN_POINT('Ctrl Pts',(-18.8762727270043,-14.0000000137146,
124.797440124957)) ;
#18601=CARTESIAN_POINT('Ctrl Pts',(-18.8208080269445,-14.000000007885,124.777687193927)) ;
#18602=CARTESIAN_POINT('Ctrl Pts',(-18.7945365568883,-14.0000000051237,
124.768330999166)) ;
#18603=CARTESIAN_POINT('Ctrl Pts',(-18.7685120965147,-13.9999999999504,
124.758243741055)) ;
#18604=CARTESIAN_POINT('Ctrl Pts',(-18.7428349004259,-13.9999999999504,
124.747455264173)) ;
#18605=CARTESIAN_POINT('Ctrl Pts',(-18.7078593253204,-13.9999999999504,
124.732759999854)) ;
#18606=CARTESIAN_POINT('Ctrl Pts',(-18.6735444651903,-13.9999999999504,
124.716770596899)) ;
#18607=CARTESIAN_POINT('Ctrl Pts',(-18.6398461652381,-13.9999999999504,
124.699448408814)) ;
#18608=CARTESIAN_POINT('Ctrl Pts',(-18.6398461652382,-13.9999999999504,
124.699448408814)) ;
#18609=CARTESIAN_POINT('Ctrl Pts',(-18.5997926981249,-13.9999999999504,
124.671930427777)) ;
#18610=CARTESIAN_POINT('Ctrl Pts',(-18.561258889765,-13.9999999999504,124.642528114611)) ;
#18611=CARTESIAN_POINT('Ctrl Pts',(-18.524128777116,-13.9999999999504,124.611194750015)) ;
#18612=CARTESIAN_POINT('Ctrl Pts',(-18.4794937216306,-13.9999999999504,
124.573528113221)) ;
#18613=CARTESIAN_POINT('Ctrl Pts',(-18.4369157182474,-13.9999999853488,
124.533094940628)) ;
#18614=CARTESIAN_POINT('Ctrl Pts',(-18.3970571422208,-13.999999991476,124.490600337269)) ;
#18615=CARTESIAN_POINT('Ctrl Pts',(-18.3778529676017,-13.9999999944282,
124.470126104001)) ;
#18616=CARTESIAN_POINT('Ctrl Pts',(-18.3592794755442,-13.9999999999504,
124.449172836299)) ;
#18617=CARTESIAN_POINT('Ctrl Pts',(-18.3414075317087,-13.9999999999504,
124.427816522051)) ;
#18618=CARTESIAN_POINT('Ctrl Pts',(-18.2894331035833,-13.9999999999504,
124.365708995856)) ;
#18619=CARTESIAN_POINT('Ctrl Pts',(-18.2434081158356,-14.0000000065016,
124.300213424349)) ;
#18620=CARTESIAN_POINT('Ctrl Pts',(-18.2030563822716,-14.0000000005206,
124.231473841747)) ;
#18621=CARTESIAN_POINT('Ctrl Pts',(-18.2006458781398,-14.0000000001633,
124.227367523796)) ;
#18622=CARTESIAN_POINT('Ctrl Pts',(-18.1982556304668,-13.9999999999504,
124.223249639981)) ;
#18623=CARTESIAN_POINT('Ctrl Pts',(-18.1958855844258,-13.9999999999504,
124.219120225186)) ;
#18624=CARTESIAN_POINT('Ctrl Pts',(-18.1630908596863,-13.9999999999504,
124.161980819791)) ;
#18625=CARTESIAN_POINT('Ctrl Pts',(-18.1341509923775,-13.9999999953418,
124.102610264843)) ;
#18626=CARTESIAN_POINT('Ctrl Pts',(-18.1094883112385,-13.9999999982308,
124.041868197465)) ;
#18627=CARTESIAN_POINT('Ctrl Pts',(-18.1024710551584,-13.9999999990528,
124.02458529788)) ;
#18628=CARTESIAN_POINT('Ctrl Pts',(-18.0957998868859,-13.9999999999504,
124.007191095672)) ;
#18629=CARTESIAN_POINT('Ctrl Pts',(-18.0894841182542,-13.9999999999504,
123.989704744565)) ;
#18630=CARTESIAN_POINT('Ctrl Pts',(-18.0670051782666,-13.9999999999504,
123.927467721639)) ;
#18631=CARTESIAN_POINT('Ctrl Pts',(-18.0490499339531,-13.99999999282,123.864126752265)) ;
#18632=CARTESIAN_POINT('Ctrl Pts',(-18.0355492695492,-13.9999999973936,
123.800543037458)) ;
#18633=CARTESIAN_POINT('Ctrl Pts',(-18.0318820335418,-13.9999999986359,
123.783271555)) ;
#18634=CARTESIAN_POINT('Ctrl Pts',(-18.0285434563634,-13.9999999999504,
123.765981864865)) ;
#18635=CARTESIAN_POINT('Ctrl Pts',(-18.0255321109708,-13.9999999999504,
123.748690566905)) ;
#18636=CARTESIAN_POINT('Ctrl Pts',(-18.0129887910751,-13.9999999999504,
123.676666187951)) ;
#18637=CARTESIAN_POINT('Ctrl Pts',(-18.0061094945016,-14.0000000069732,
123.604532181164)) ;
#18638=CARTESIAN_POINT('Ctrl Pts',(-18.0048778853208,-14.0000000012078,
123.532119117361)) ;
#18639=CARTESIAN_POINT('Ctrl Pts',(-18.0047217791523,-14.000000000477,123.52294077888)) ;
#18640=CARTESIAN_POINT('Ctrl Pts',(-18.0046564044181,-13.9999999999504,
123.513758025963)) ;
#18641=CARTESIAN_POINT('Ctrl Pts',(-18.0046817237998,-13.9999999999504,
123.504570573996)) ;
#18642=CARTESIAN_POINT('Ctrl Pts',(-18.0048326442755,-13.9999999999504,
123.44980720584)) ;
#18643=CARTESIAN_POINT('Ctrl Pts',(-18.0082057180376,-13.9999999818479,
123.394893776504)) ;
#18644=CARTESIAN_POINT('Ctrl Pts',(-18.0146634978623,-13.9999999892263,
123.340725835409)) ;
#18645=CARTESIAN_POINT('Ctrl Pts',(-18.0178533092883,-13.9999999928708,
123.313969655713)) ;
#18646=CARTESIAN_POINT('Ctrl Pts',(-18.0217957519895,-13.9999999999504,
123.287394556249)) ;
#18647=CARTESIAN_POINT('Ctrl Pts',(-18.0264744991499,-13.9999999999504,
123.261103782795)) ;
#18648=CARTESIAN_POINT('Ctrl Pts',(-18.0390326664452,-13.9999999999504,
123.190537043442)) ;
#18649=CARTESIAN_POINT('Ctrl Pts',(-18.0568929261115,-14.0000000132377,
123.122029372471)) ;
#18650=CARTESIAN_POINT('Ctrl Pts',(-18.0798718963981,-14.0000000023747,
123.05536761155)) ;
#18651=CARTESIAN_POINT('Ctrl Pts',(-18.0828457572662,-14.0000000009689,
123.046740471181)) ;
#18652=CARTESIAN_POINT('Ctrl Pts',(-18.0859053428976,-13.9999999999504,
123.038144318446)) ;
#18653=CARTESIAN_POINT('Ctrl Pts',(-18.0890502468538,-13.9999999999504,
123.029578754099)) ;
#18654=CARTESIAN_POINT('Ctrl Pts',(-18.1100272574254,-13.9999999999504,
122.972445074865)) ;
#18655=CARTESIAN_POINT('Ctrl Pts',(-18.1348094756135,-13.9999999944962,
122.916647791952)) ;
#18656=CARTESIAN_POINT('Ctrl Pts',(-18.1630319807289,-13.9999999977526,
122.863018295295)) ;
#18657=CARTESIAN_POINT('Ctrl Pts',(-18.1718071281557,-13.9999999987651,
122.846343420487)) ;
#18658=CARTESIAN_POINT('Ctrl Pts',(-18.1809149717527,-13.9999999999504,
122.829877752249)) ;
#18659=CARTESIAN_POINT('Ctrl Pts',(-18.1903448428654,-13.9999999999504,
122.813645300798)) ;
#18660=CARTESIAN_POINT('Ctrl Pts',(-18.2223967198354,-13.9999999999504,
122.758471637171)) ;
#18661=CARTESIAN_POINT('Ctrl Pts',(-18.2581335738048,-13.9999999944644,
122.706050735912)) ;
#18662=CARTESIAN_POINT('Ctrl Pts',(-18.2968706910898,-13.9999999981482,
122.656851834518)) ;
#18663=CARTESIAN_POINT('Ctrl Pts',(-18.3064010001469,-13.9999999990546,
122.644747662385)) ;
#18664=CARTESIAN_POINT('Ctrl Pts',(-18.3161130895013,-13.9999999999504,
122.632838342075)) ;
#18665=CARTESIAN_POINT('Ctrl Pts',(-18.3259971142104,-13.9999999999504,
122.621130531685)) ;
#18666=CARTESIAN_POINT('Ctrl Pts',(-18.3734383381901,-13.9999999999504,
122.564935522933)) ;
#18667=CARTESIAN_POINT('Ctrl Pts',(-18.4248932987606,-14.0000000041903,
122.513321647355)) ;
#18668=CARTESIAN_POINT('Ctrl Pts',(-18.4803670960102,-14.0000000003093,
122.466234561986)) ;
#18669=CARTESIAN_POINT('Ctrl Pts',(-18.4835871984864,-14.0000000000841,
122.463501285237)) ;
#18670=CARTESIAN_POINT('Ctrl Pts',(-18.4868208307239,-13.9999999999504,
122.460783270347)) ;
#18671=CARTESIAN_POINT('Ctrl Pts',(-18.4900679892232,-13.9999999999504,
122.458080509819)) ;
#18672=CARTESIAN_POINT('Ctrl Pts',(-18.5307483671629,-13.9999999999504,
122.424220345685)) ;
#18673=CARTESIAN_POINT('Ctrl Pts',(-18.5735407603444,-13.9999999831684,
122.392763309753)) ;
#18674=CARTESIAN_POINT('Ctrl Pts',(-18.6177141173049,-13.9999999906428,
122.364139246752)) ;
#18675=CARTESIAN_POINT('Ctrl Pts',(-18.637808728866,-13.999999994043,122.351118062335)) ;
#18676=CARTESIAN_POINT('Ctrl Pts',(-18.6581896700084,-13.9999999999504,
122.338682672565)) ;
#18677=CARTESIAN_POINT('Ctrl Pts',(-18.6787909658031,-13.9999999999504,
122.326871390036)) ;
#18678=CARTESIAN_POINT('Ctrl Pts',(-18.7400451319779,-13.9999999999504,
122.291752712553)) ;
#18679=CARTESIAN_POINT('Ctrl Pts',(-18.8032442560716,-14.0000000082293,
122.262152793656)) ;
#18680=CARTESIAN_POINT('Ctrl Pts',(-18.8683619735397,-14.0000000008848,
122.237841302782)) ;
#18681=CARTESIAN_POINT('Ctrl Pts',(-18.8734510451838,-14.0000000003108,
122.235941314213)) ;
#18682=CARTESIAN_POINT('Ctrl Pts',(-18.8785518127922,-13.9999999999504,
122.234073639899)) ;
#18683=CARTESIAN_POINT('Ctrl Pts',(-18.8836642521681,-13.9999999999504,
122.232238176495)) ;
#18684=CARTESIAN_POINT('Ctrl Pts',(-18.9362326297888,-13.9999999999504,
122.213365124662)) ;
#18685=CARTESIAN_POINT('Ctrl Pts',(-18.9900459354094,-13.9999999915247,
122.197893969736)) ;
#18686=CARTESIAN_POINT('Ctrl Pts',(-19.0442918567496,-13.999999996242,122.186032108559)) ;
#18687=CARTESIAN_POINT('Ctrl Pts',(-19.062980568766,-13.9999999978671,122.18194548044)) ;
#18688=CARTESIAN_POINT('Ctrl Pts',(-19.081721049772,-13.9999999999504,122.17828707369)) ;
#18689=CARTESIAN_POINT('Ctrl Pts',(-19.1004814153796,-13.9999999999504,
122.1750648481)) ;
#18690=CARTESIAN_POINT('Ctrl Pts',(-19.1614800110122,-13.9999999999504,
122.164587907514)) ;
#18691=CARTESIAN_POINT('Ctrl Pts',(-19.2226231882264,-13.9999999970496,
122.158731956407)) ;
#18692=CARTESIAN_POINT('Ctrl Pts',(-19.283163479914,-13.9999999991458,122.157230987035)) ;
#18693=CARTESIAN_POINT('Ctrl Pts',(-19.2955014863585,-13.999999999573,122.156925092081)) ;
#18694=CARTESIAN_POINT('Ctrl Pts',(-19.3078146229717,-13.9999999999504,
122.156800106915)) ;
#18695=CARTESIAN_POINT('Ctrl Pts',(-19.3200968225337,-13.9999999999504,
122.156853828668)) ;
#18696=CARTESIAN_POINT('Ctrl Pts',(-19.3561519827403,-13.9999999999504,
122.157011532215)) ;
#18697=CARTESIAN_POINT('Ctrl Pts',(-19.3919648957125,-14.0000000079266,
122.158709422108)) ;
#18698=CARTESIAN_POINT('Ctrl Pts',(-19.4275508050227,-13.9999999999504,
122.161948016114)) ;
#18699=CARTESIAN_POINT('Origin',(-17.409466984686,14.0000000000496,123.383738395492)) ;
#18700=CARTESIAN_POINT('',(-17.7094373828403,14.0000000000496,123.387952684416)) ;
#18701=CARTESIAN_POINT('Ctrl Pts',(-17.7094373828403,14.0000000000496,123.387952684416)) ;
#18702=CARTESIAN_POINT('Ctrl Pts',(-17.7124365161055,14.0000000000496,123.165469985201)) ;
#18703=CARTESIAN_POINT('Ctrl Pts',(-17.8073115029348,14.0000000000496,122.721754746081)) ;
#18704=CARTESIAN_POINT('Ctrl Pts',(-18.1932733581975,14.0000000000496,122.161208794752)) ;
#18705=CARTESIAN_POINT('Ctrl Pts',(-18.7644631958589,14.0000000000496,121.791079731755)) ;
#18706=CARTESIAN_POINT('Ctrl Pts',(-19.4337624984685,14.0000000000496,121.66769040749)) ;
#18707=CARTESIAN_POINT('Ctrl Pts',(-20.0993607034912,14.0000000000496,121.809828608283)) ;
#18708=CARTESIAN_POINT('Ctrl Pts',(-20.659887032884,14.0000000000496,122.195860778204)) ;
#18709=CARTESIAN_POINT('Ctrl Pts',(-21.0300277648268,14.0000000000496,122.767014628009)) ;
#18710=CARTESIAN_POINT('Ctrl Pts',(-21.153410552117,14.0000000000496,123.436333440585)) ;
#18711=CARTESIAN_POINT('Ctrl Pts',(-21.0112760309154,14.0000000000496,124.101920740338)) ;
#18712=CARTESIAN_POINT('Ctrl Pts',(-20.6252417466303,14.0000000000496,124.66245330923)) ;
#18713=CARTESIAN_POINT('Ctrl Pts',(-20.0540890803185,14.0000000000496,125.032590535832)) ;
#18714=CARTESIAN_POINT('Ctrl Pts',(-19.3847696171534,14.0000000000496,125.155975257797)) ;
#18715=CARTESIAN_POINT('Ctrl Pts',(-18.7191817607918,14.0000000000496,125.013838725625)) ;
#18716=CARTESIAN_POINT('Ctrl Pts',(-18.1586286713331,14.0000000000496,124.627806965402)) ;
#18717=CARTESIAN_POINT('Ctrl Pts',(-17.7885531153341,14.0000000000496,124.056641767528)) ;
#18718=CARTESIAN_POINT('Ctrl Pts',(-17.7061836816795,14.0000000000496,123.610445192173)) ;
#18719=CARTESIAN_POINT('Ctrl Pts',(-17.7094373828403,14.0000000000496,123.387952684416)) ;
#18720=CARTESIAN_POINT('',(-20.8063667317783,14.0000000000496,123.957804304199)) ;
#18721=CARTESIAN_POINT('Ctrl Pts',(-20.8063667317783,14.0000000000496,123.957804304199)) ;
#18722=CARTESIAN_POINT('Ctrl Pts',(-20.7903532895648,14.0000000000496,123.992143834147)) ;
#18723=CARTESIAN_POINT('Ctrl Pts',(-20.7730358647268,14.0000000000496,124.025808018184)) ;
#18724=CARTESIAN_POINT('Ctrl Pts',(-20.7544032477939,14.0000000000496,124.058854457495)) ;
#18725=CARTESIAN_POINT('Ctrl Pts',(-20.7255238457092,14.0000000000496,124.11007439143)) ;
#18726=CARTESIAN_POINT('Ctrl Pts',(-20.6935075653374,14.0000000137776,124.159770107137)) ;
#18727=CARTESIAN_POINT('Ctrl Pts',(-20.6589212017235,14.0000000079079,124.207153625976)) ;
#18728=CARTESIAN_POINT('Ctrl Pts',(-20.6425389066613,14.0000000051277,124.229597465269)) ;
#18729=CARTESIAN_POINT('Ctrl Pts',(-20.6255796316115,14.0000000000496,124.251523215916)) ;
#18730=CARTESIAN_POINT('Ctrl Pts',(-20.6081015241412,14.0000000000496,124.272850644239)) ;
#18731=CARTESIAN_POINT('Ctrl Pts',(-20.5536065311287,14.0000000000496,124.339347435121)) ;
#18732=CARTESIAN_POINT('Ctrl Pts',(-20.4940962390615,14.0000000000496,124.399995126451)) ;
#18733=CARTESIAN_POINT('Ctrl Pts',(-20.4299459192023,14.0000000000496,124.454977940252)) ;
#18734=CARTESIAN_POINT('Ctrl Pts',(-20.3784169085553,14.0000000000496,124.499143113613)) ;
#18735=CARTESIAN_POINT('Ctrl Pts',(-20.3238730196464,14.0000000040184,124.539669744578)) ;
#18736=CARTESIAN_POINT('Ctrl Pts',(-20.2670953919153,14.0000000013602,124.576016790401)) ;
#18737=CARTESIAN_POINT('Ctrl Pts',(-20.2530365163627,14.000000000702,124.58501678942)) ;
#18738=CARTESIAN_POINT('Ctrl Pts',(-20.238840502438,14.0000000000496,124.593760699861)) ;
#18739=CARTESIAN_POINT('Ctrl Pts',(-20.2245188440556,14.0000000000496,124.602240638756)) ;
#18740=CARTESIAN_POINT('Ctrl Pts',(-20.1614355826137,14.0000000000496,124.63959261211)) ;
#18741=CARTESIAN_POINT('Ctrl Pts',(-20.095955824469,14.0000000008143,124.671799735807)) ;
#18742=CARTESIAN_POINT('Ctrl Pts',(-20.0290025115168,14.0000000002061,124.698705425819)) ;
#18743=CARTESIAN_POINT('Ctrl Pts',(-20.0191991796927,14.000000000117,124.702644968098)) ;
#18744=CARTESIAN_POINT('Ctrl Pts',(-20.0093641701037,14.0000000000496,124.70647088242)) ;
#18745=CARTESIAN_POINT('Ctrl Pts',(-19.9995002913839,14.0000000000496,124.710182706931)) ;
#18746=CARTESIAN_POINT('Ctrl Pts',(-19.9220862328323,14.0000000000496,124.739313985635)) ;
#18747=CARTESIAN_POINT('Ctrl Pts',(-19.8428544874908,14.0000000000496,124.761432727835)) ;
#18748=CARTESIAN_POINT('Ctrl Pts',(-19.7625126120531,14.0000000000496,124.776513608246)) ;
#18749=CARTESIAN_POINT('Ctrl Pts',(-19.693208445859,14.0000000000496,124.789522613036)) ;
#18750=CARTESIAN_POINT('Ctrl Pts',(-19.6230634255686,14.0000000012919,124.797297340209)) ;
#18751=CARTESIAN_POINT('Ctrl Pts',(-19.5530430596108,14.000000000331,124.799739393028)) ;
#18752=CARTESIAN_POINT('Ctrl Pts',(-19.5416037822131,14.000000000174,124.800138352948)) ;
#18753=CARTESIAN_POINT('Ctrl Pts',(-19.5301677234554,14.0000000000496,124.80039501536)) ;
#18754=CARTESIAN_POINT('Ctrl Pts',(-19.5187389662347,14.0000000000496,124.800508987162)) ;
#18755=CARTESIAN_POINT('Ctrl Pts',(-19.4590087648072,14.0000000000496,124.801104638865)) ;
#18756=CARTESIAN_POINT('Ctrl Pts',(-19.3995343315883,14.0000000150306,124.797803035015)) ;
#18757=CARTESIAN_POINT('Ctrl Pts',(-19.3411000014312,14.0000000069942,124.790869863461)) ;
#18758=CARTESIAN_POINT('Ctrl Pts',(-19.3197195910949,14.0000000040538,124.788333100357)) ;
#18759=CARTESIAN_POINT('Ctrl Pts',(-19.2984779242726,14.0000000000496,124.785310081673)) ;
#18760=CARTESIAN_POINT('Ctrl Pts',(-19.2774117103375,14.0000000000496,124.78181350101)) ;
#18761=CARTESIAN_POINT('Ctrl Pts',(-19.2102415471371,14.0000000000496,124.770664563925)) ;
#18762=CARTESIAN_POINT('Ctrl Pts',(-19.1447976238525,13.9999999879324,124.75469117092)) ;
#18763=CARTESIAN_POINT('Ctrl Pts',(-19.0808386295641,13.9999999971719,124.733903584227)) ;
#18764=CARTESIAN_POINT('Ctrl Pts',(-19.0698584181317,13.9999999987581,124.730334858677)) ;
#18765=CARTESIAN_POINT('Ctrl Pts',(-19.0589220915987,14.0000000000496,124.72662427763)) ;
#18766=CARTESIAN_POINT('Ctrl Pts',(-19.0480285772954,14.0000000000496,124.722771939096)) ;
#18767=CARTESIAN_POINT('Ctrl Pts',(-18.9969916069748,14.0000000000496,124.704723430421)) ;
#18768=CARTESIAN_POINT('Ctrl Pts',(-18.9468984566506,14.0000000147882,124.683564801094)) ;
#18769=CARTESIAN_POINT('Ctrl Pts',(-18.8985399742721,14.000000008286,124.65968813236)) ;
#18770=CARTESIAN_POINT('Ctrl Pts',(-18.87632175014,14.0000000052986,124.648718036705)) ;
#18771=CARTESIAN_POINT('Ctrl Pts',(-18.8544690109434,14.0000000000496,124.637173952294)) ;
#18772=CARTESIAN_POINT('Ctrl Pts',(-18.8330550061689,14.0000000000496,124.625092613764)) ;
#18773=CARTESIAN_POINT('Ctrl Pts',(-18.7648534752608,14.0000000000496,124.586614720823)) ;
#18774=CARTESIAN_POINT('Ctrl Pts',(-18.7011545569484,14.0000000000496,124.542719161019)) ;
#18775=CARTESIAN_POINT('Ctrl Pts',(-18.6420184816923,14.0000000000496,124.494038304341)) ;
#18776=CARTESIAN_POINT('Ctrl Pts',(-18.5827483683475,14.0000000000496,124.445247107418)) ;
#18777=CARTESIAN_POINT('Ctrl Pts',(-18.5279935908249,14.0000000000496,124.391588448733)) ;
#18778=CARTESIAN_POINT('Ctrl Pts',(-18.4784272028069,14.0000000000496,124.33361616347)) ;
#18779=CARTESIAN_POINT('Ctrl Pts',(-18.4428545923722,14.0000000000496,124.292010841756)) ;
#18780=CARTESIAN_POINT('Ctrl Pts',(-18.4099776244296,14.0000000154805,124.248213063441)) ;
#18781=CARTESIAN_POINT('Ctrl Pts',(-18.3801700432554,14.0000000076918,124.202947967025)) ;
#18782=CARTESIAN_POINT('Ctrl Pts',(-18.3683638559556,14.0000000046068,124.185019366804)) ;
#18783=CARTESIAN_POINT('Ctrl Pts',(-18.3570388483513,14.0000000000496,124.166860110623)) ;
#18784=CARTESIAN_POINT('Ctrl Pts',(-18.3462169473724,14.0000000000496,124.148513408658)) ;
#18785=CARTESIAN_POINT('Ctrl Pts',(-18.307965669138,14.0000000000496,124.083664838807)) ;
#18786=CARTESIAN_POINT('Ctrl Pts',(-18.2759975850554,14.0000000000496,124.016471705333)) ;
#18787=CARTESIAN_POINT('Ctrl Pts',(-18.2501194198681,14.0000000000496,123.947201515044)) ;
#18788=CARTESIAN_POINT('Ctrl Pts',(-18.2297326885799,14.0000000000496,123.892630692673)) ;
#18789=CARTESIAN_POINT('Ctrl Pts',(-18.2131210008505,14.0000000059345,123.836756700599)) ;
#18790=CARTESIAN_POINT('Ctrl Pts',(-18.2004633524007,14.0000000021642,123.78038614397)) ;
#18791=CARTESIAN_POINT('Ctrl Pts',(-18.1970152704689,14.0000000011371,123.765030187564)) ;
#18792=CARTESIAN_POINT('Ctrl Pts',(-18.1938604966817,14.0000000000496,123.749637105053)) ;
#18793=CARTESIAN_POINT('Ctrl Pts',(-18.1910024087544,14.0000000000496,123.734222577563)) ;
#18794=CARTESIAN_POINT('Ctrl Pts',(-18.1827738973621,14.0000000000496,123.689843741683)) ;
#18795=CARTESIAN_POINT('Ctrl Pts',(-18.1770067892692,13.999999997305,123.645300232667)) ;
#18796=CARTESIAN_POINT('Ctrl Pts',(-18.1736437367582,14.0000000000496,123.600817573026)) ;
#18797=CARTESIAN_POINT('Ctrl Pts',(-18.6288026007436,14.0000000000496,122.435409149151)) ;
#18798=CARTESIAN_POINT('Ctrl Pts',(-18.6549557016393,14.0000000080335,122.411022804977)) ;
#18799=CARTESIAN_POINT('Ctrl Pts',(-18.6822339839383,14.0000000000496,122.387716398644)) ;
#18800=CARTESIAN_POINT('Ctrl Pts',(-18.7106491980473,14.0000000000496,122.36548016086)) ;
#18801=CARTESIAN_POINT('Ctrl Pts',(-18.7581113526755,14.0000000000496,122.328338798771)) ;
#18802=CARTESIAN_POINT('Ctrl Pts',(-18.8088016844457,13.9999999971444,122.294137942038)) ;
#18803=CARTESIAN_POINT('Ctrl Pts',(-18.8622996253852,13.9999999992434,122.263537949972)) ;
#18804=CARTESIAN_POINT('Ctrl Pts',(-18.8732022252909,13.9999999996712,122.257301832006)) ;
#18805=CARTESIAN_POINT('Ctrl Pts',(-18.8842213165307,14.0000000000496,122.251215395131)) ;
#18806=CARTESIAN_POINT('Ctrl Pts',(-18.8953531606705,14.0000000000496,122.24528442688)) ;
#18807=CARTESIAN_POINT('Ctrl Pts',(-18.9441153362962,14.0000000000496,122.219304282725)) ;
#18808=CARTESIAN_POINT('Ctrl Pts',(-18.995000848613,13.9999999915908,122.19632965352)) ;
#18809=CARTESIAN_POINT('Ctrl Pts',(-19.0472579864155,13.9999999963147,122.176689567072)) ;
#18810=CARTESIAN_POINT('Ctrl Pts',(-19.0652613628245,13.9999999979422,122.169923259465)) ;
#18811=CARTESIAN_POINT('Ctrl Pts',(-19.0834271029694,14.0000000000496,122.163552860095)) ;
#18812=CARTESIAN_POINT('Ctrl Pts',(-19.1017230829542,14.0000000000496,122.157592198567)) ;
#18813=CARTESIAN_POINT('Ctrl Pts',(-19.1678091301422,14.0000000000496,122.13606197393)) ;
#18814=CARTESIAN_POINT('Ctrl Pts',(-19.2356127427886,14.0000000082481,122.119870825476)) ;
#18815=CARTESIAN_POINT('Ctrl Pts',(-19.3052501799436,14.0000000009742,122.109217226808)) ;
#18816=CARTESIAN_POINT('Ctrl Pts',(-19.3106926051813,14.0000000004057,122.108384608369)) ;
#18817=CARTESIAN_POINT('Ctrl Pts',(-19.3161462578174,14.0000000000496,122.107585811876)) ;
#18818=CARTESIAN_POINT('Ctrl Pts',(-19.3216112068833,14.0000000000496,122.106820931957)) ;
#18819=CARTESIAN_POINT('Ctrl Pts',(-19.3733096004345,14.0000000000496,122.099585171368)) ;
#18820=CARTESIAN_POINT('Ctrl Pts',(-19.4260182147184,13.9999999832307,122.095385120388)) ;
#18821=CARTESIAN_POINT('Ctrl Pts',(-19.4789196753301,13.999999990678,122.094329066821)) ;
#18822=CARTESIAN_POINT('Ctrl Pts',(-19.5029846994337,13.9999999940658,122.093848665065)) ;
#18823=CARTESIAN_POINT('Ctrl Pts',(-19.5270889190625,14.0000000000496,122.094018890807)) ;
#18824=CARTESIAN_POINT('Ctrl Pts',(-19.5511518125165,14.0000000000496,122.094849910452)) ;
#18825=CARTESIAN_POINT('Ctrl Pts',(-19.6238904012892,14.0000000000496,122.097361960648)) ;
#18826=CARTESIAN_POINT('Ctrl Pts',(-19.6962268249112,14.0000000042239,122.105911687139)) ;
#18827=CARTESIAN_POINT('Ctrl Pts',(-19.7681953794014,14.0000000004026,122.120538847728)) ;
#18828=CARTESIAN_POINT('Ctrl Pts',(-19.7723731078155,14.0000000001808,122.121387945016)) ;
#18829=CARTESIAN_POINT('Ctrl Pts',(-19.776549611116,14.0000000000496,122.122257522262)) ;
#18830=CARTESIAN_POINT('Ctrl Pts',(-19.7807249013257,14.0000000000496,122.123147587728)) ;
#18831=CARTESIAN_POINT('Ctrl Pts',(-19.8416350175698,14.0000000000496,122.136132072222)) ;
#18832=CARTESIAN_POINT('Ctrl Pts',(-19.9023447220298,13.9999999945544,122.153488502169)) ;
#18833=CARTESIAN_POINT('Ctrl Pts',(-19.9620381343026,13.9999999982432,122.175266965352)) ;
#18834=CARTESIAN_POINT('Ctrl Pts',(-19.9767240413107,13.9999999991507,122.18062495165)) ;
#18835=CARTESIAN_POINT('Ctrl Pts',(-19.9913481896679,14.0000000000496,122.186250566072)) ;
#18836=CARTESIAN_POINT('Ctrl Pts',(-20.0058979474292,14.0000000000496,122.192144503185)) ;
#18837=CARTESIAN_POINT('Ctrl Pts',(-20.0618576588578,14.0000000000496,122.21481312939)) ;
#18838=CARTESIAN_POINT('Ctrl Pts',(-20.1166667194942,13.9999999945662,122.24143163317)) ;
#18839=CARTESIAN_POINT('Ctrl Pts',(-20.1695404077726,13.9999999978326,122.271576161658)) ;
#18840=CARTESIAN_POINT('Ctrl Pts',(-20.1859800181873,13.9999999988481,122.280948768726)) ;
#18841=CARTESIAN_POINT('Ctrl Pts',(-20.2022322213107,14.0000000000496,122.290662026939)) ;
#18842=CARTESIAN_POINT('Ctrl Pts',(-20.2182726032679,14.0000000000496,122.300702584319)) ;
#18843=CARTESIAN_POINT('Ctrl Pts',(-20.278035635958,14.0000000000496,122.338111553788)) ;
#18844=CARTESIAN_POINT('Ctrl Pts',(-20.3348894843774,14.0000000132225,122.380082458679)) ;
#18845=CARTESIAN_POINT('Ctrl Pts',(-20.388815293428,14.0000000024498,122.426891168377)) ;
#18846=CARTESIAN_POINT('Ctrl Pts',(-20.395794502225,14.0000000010555,122.43294926494)) ;
#18847=CARTESIAN_POINT('Ctrl Pts',(-20.40272471404,14.0000000000496,122.439088448526)) ;
#18848=CARTESIAN_POINT('Ctrl Pts',(-20.4096059290759,14.0000000000496,122.445309366784)) ;
#18849=CARTESIAN_POINT('Ctrl Pts',(-20.4497091790637,14.0000000000496,122.481564452365)) ;
#18850=CARTESIAN_POINT('Ctrl Pts',(-20.4881440190304,13.9999999819172,122.520592261045)) ;
#18851=CARTESIAN_POINT('Ctrl Pts',(-20.5242696457146,13.9999999892437,122.5617890429)) ;
#18852=CARTESIAN_POINT('Ctrl Pts',(-20.5421138243492,13.9999999928626,122.58213810815)) ;
#18853=CARTESIAN_POINT('Ctrl Pts',(-20.559394056096,14.0000000000496,122.603015774859)) ;
#18854=CARTESIAN_POINT('Ctrl Pts',(-20.5760301136045,14.0000000000496,122.624345659934)) ;
#18855=CARTESIAN_POINT('Ctrl Pts',(-20.6206086507397,14.0000000000496,122.681501934697)) ;
#18856=CARTESIAN_POINT('Ctrl Pts',(-20.6605441251487,14.0000000069509,122.741883401912)) ;
#18857=CARTESIAN_POINT('Ctrl Pts',(-20.6959233360179,14.0000000012818,122.805628776949)) ;
#18858=CARTESIAN_POINT('Ctrl Pts',(-20.700407733753,14.0000000005632,122.813708652346)) ;
#18859=CARTESIAN_POINT('Ctrl Pts',(-20.7048189720407,14.0000000000496,122.821842626814)) ;
#18860=CARTESIAN_POINT('Ctrl Pts',(-20.7091572619482,14.0000000000496,122.830031031177)) ;
#18861=CARTESIAN_POINT('Ctrl Pts',(-20.7394075255629,14.0000000000496,122.887127582083)) ;
#18862=CARTESIAN_POINT('Ctrl Pts',(-20.7661421097676,13.9999999929068,122.94692809065)) ;
#18863=CARTESIAN_POINT('Ctrl Pts',(-20.788786499386,13.9999999974862,123.00880613829)) ;
#18864=CARTESIAN_POINT('Ctrl Pts',(-20.7949374004377,13.9999999987301,123.025614087398)) ;
#18865=CARTESIAN_POINT('Ctrl Pts',(-20.8007863489826,14.0000000000496,123.042575077714)) ;
#18866=CARTESIAN_POINT('Ctrl Pts',(-20.8063214639271,14.0000000000496,123.059675998263)) ;
#18867=CARTESIAN_POINT('Ctrl Pts',(-20.8264435056946,14.0000000000496,123.121843711311)) ;
#18868=CARTESIAN_POINT('Ctrl Pts',(-20.8423993087311,13.9999999954176,123.185806239041)) ;
#18869=CARTESIAN_POINT('Ctrl Pts',(-20.8539969353865,13.9999999983166,123.250640258058)) ;
#18870=CARTESIAN_POINT('Ctrl Pts',(-20.8572967547092,13.9999999991414,123.269087183025)) ;
#18871=CARTESIAN_POINT('Ctrl Pts',(-20.8602437320734,14.0000000000496,123.287604337263)) ;
#18872=CARTESIAN_POINT('Ctrl Pts',(-20.8628333957635,14.0000000000496,123.306169682356)) ;
#18873=CARTESIAN_POINT('Ctrl Pts',(-20.8738443370904,14.0000000000496,123.385107316734)) ;
#18874=CARTESIAN_POINT('Ctrl Pts',(-20.8784022994741,14.0000000065374,123.464956496997)) ;
#18875=CARTESIAN_POINT('Ctrl Pts',(-20.8762013391412,14.000000000614,123.545769604119)) ;
#18876=CARTESIAN_POINT('Ctrl Pts',(-20.8760698399773,14.0000000002601,123.5505978856)) ;
#18877=CARTESIAN_POINT('Ctrl Pts',(-20.8759142108493,14.0000000000496,123.555429623132)) ;
#18878=CARTESIAN_POINT('Ctrl Pts',(-20.8757343850132,14.0000000000496,123.560264833683)) ;
#18879=CARTESIAN_POINT('Ctrl Pts',(-20.8735862885529,14.0000000000496,123.618023490037)) ;
#18880=CARTESIAN_POINT('Ctrl Pts',(-20.8679855063018,13.9999999854137,123.676265453797)) ;
#18881=CARTESIAN_POINT('Ctrl Pts',(-20.8590185588221,13.9999999914957,123.734052299697)) ;
#18882=CARTESIAN_POINT('Ctrl Pts',(-20.8546982311164,13.9999999944261,123.761894339803)) ;
#18883=CARTESIAN_POINT('Ctrl Pts',(-20.8495966167066,14.0000000000496,123.789629967368)) ;
#18884=CARTESIAN_POINT('Ctrl Pts',(-20.8437242586452,14.0000000000496,123.817149982747)) ;
#18885=CARTESIAN_POINT('Ctrl Pts',(-20.8335853768039,14.0000000000496,123.86466448736)) ;
#18886=CARTESIAN_POINT('Ctrl Pts',(-20.8211538688771,14.0000000000496,123.911513268694)) ;
#18887=CARTESIAN_POINT('Ctrl Pts',(-20.8063667317783,14.0000000000496,123.957804304199)) ;
#18888=CARTESIAN_POINT('Ctrl Pts',(-17.409466984686,-13.6999999999504,123.383738395492)) ;
#18889=CARTESIAN_POINT('Ctrl Pts',(-17.4129953764185,-13.6999999999504,
123.121994043902)) ;
#18890=CARTESIAN_POINT('Ctrl Pts',(-17.524613009103,-13.6999999999504,122.599976114327)) ;
#18891=CARTESIAN_POINT('Ctrl Pts',(-17.9786857788369,-13.6999999999504,
121.940510290626)) ;
#18892=CARTESIAN_POINT('Ctrl Pts',(-18.6506738232679,-13.6999999999504,
121.505064333141)) ;
#18893=CARTESIAN_POINT('Ctrl Pts',(-19.4380847682357,-13.6999999999504,
121.359900422812)) ;
#18894=CARTESIAN_POINT('Ctrl Pts',(-20.2211414796235,-13.6999999999504,
121.527121835554)) ;
#18895=CARTESIAN_POINT('Ctrl Pts',(-20.8805842197971,-13.6999999999504,
121.98127732928)) ;
#18896=CARTESIAN_POINT('Ctrl Pts',(-21.3160439046833,-13.6999999999504,
122.653223034764)) ;
#18897=CARTESIAN_POINT('Ctrl Pts',(-21.4612001247882,-13.6999999999504,
123.440656932859)) ;
#18898=CARTESIAN_POINT('Ctrl Pts',(-21.2939830415348,-13.6999999999504,
124.223700813763)) ;
#18899=CARTESIAN_POINT('Ctrl Pts',(-20.8398250592352,-13.6999999999504,
124.883150895787)) ;
#18900=CARTESIAN_POINT('Ctrl Pts',(-20.1678807467438,-13.6999999999504,
125.318606455482)) ;
#18901=CARTESIAN_POINT('Ctrl Pts',(-19.3804460839353,-13.6999999999504,
125.463764952492)) ;
#18902=CARTESIAN_POINT('Ctrl Pts',(-18.5974015471293,-13.6999999999504,
125.296545502889)) ;
#18903=CARTESIAN_POINT('Ctrl Pts',(-17.937927323658,-13.6999999999504,124.842390490217)) ;
#18904=CARTESIAN_POINT('Ctrl Pts',(-17.5025443176974,-13.6999999999504,
124.17043143519)) ;
#18905=CARTESIAN_POINT('Ctrl Pts',(-17.4056391005857,-13.6999999999504,
123.645494286554)) ;
#18906=CARTESIAN_POINT('Ctrl Pts',(-17.409466984686,-13.6999999999504,123.383738395492)) ;
#18907=CARTESIAN_POINT('Ctrl Pts',(-17.7094373828403,-13.9999999999504,
123.387952684416)) ;
#18908=CARTESIAN_POINT('Ctrl Pts',(-17.7124365161054,-13.9999999999504,
123.165469985201)) ;
#18909=CARTESIAN_POINT('Ctrl Pts',(-17.8073115029348,-13.9999999999504,
122.721754746081)) ;
#18910=CARTESIAN_POINT('Ctrl Pts',(-18.1932733581975,-13.9999999999504,
122.161208794752)) ;
#18911=CARTESIAN_POINT('Ctrl Pts',(-18.7644631958589,-13.9999999999504,
121.791079731755)) ;
#18912=CARTESIAN_POINT('Ctrl Pts',(-19.4337624984685,-13.9999999999504,
121.66769040749)) ;
#18913=CARTESIAN_POINT('Ctrl Pts',(-20.0993607034912,-13.9999999999504,
121.809828608283)) ;
#18914=CARTESIAN_POINT('Ctrl Pts',(-20.659887032884,-13.9999999999504,122.195860778204)) ;
#18915=CARTESIAN_POINT('Ctrl Pts',(-21.0300277648269,-13.9999999999504,
122.767014628009)) ;
#18916=CARTESIAN_POINT('Ctrl Pts',(-21.153410552117,-13.9999999999504,123.436333440585)) ;
#18917=CARTESIAN_POINT('Ctrl Pts',(-21.0112760309154,-13.9999999999504,
124.101920740338)) ;
#18918=CARTESIAN_POINT('Ctrl Pts',(-20.6252417466303,-13.9999999999504,
124.66245330923)) ;
#18919=CARTESIAN_POINT('Ctrl Pts',(-20.0540890803186,-13.9999999999504,
125.032590535832)) ;
#18920=CARTESIAN_POINT('Ctrl Pts',(-19.3847696171533,-13.9999999999504,
125.155975257797)) ;
#18921=CARTESIAN_POINT('Ctrl Pts',(-18.7191817607919,-13.9999999999504,
125.013838725625)) ;
#18922=CARTESIAN_POINT('Ctrl Pts',(-18.1586286713331,-13.9999999999504,
124.627806965402)) ;
#18923=CARTESIAN_POINT('Ctrl Pts',(-17.7885531153341,-13.9999999999504,
124.056641767528)) ;
#18924=CARTESIAN_POINT('Ctrl Pts',(-17.7061836816795,-13.9999999999504,
123.610445192173)) ;
#18925=CARTESIAN_POINT('Ctrl Pts',(-17.7094373828403,-13.9999999999504,
123.387952684416)) ;
#18926=CARTESIAN_POINT('',(-17.409466984686,-13.6999999999504,123.383738395492)) ;
#18927=CARTESIAN_POINT('Ctrl Pts',(-17.409466984686,13.7000000000496,123.383738395492)) ;
#18928=CARTESIAN_POINT('Ctrl Pts',(-17.7094373828403,14.0000000000496,123.387952684416)) ;
#18929=CARTESIAN_POINT('Ctrl Pts',(-17.4129953764185,13.7000000000496,123.121994043903)) ;
#18930=CARTESIAN_POINT('Ctrl Pts',(-17.7124365161055,14.0000000000496,123.165469985201)) ;
#18931=CARTESIAN_POINT('Ctrl Pts',(-17.524613009103,13.7000000000496,122.599976114327)) ;
#18932=CARTESIAN_POINT('Ctrl Pts',(-17.8073115029348,14.0000000000496,122.721754746081)) ;
#18933=CARTESIAN_POINT('Ctrl Pts',(-17.9786857788369,13.7000000000496,121.940510290626)) ;
#18934=CARTESIAN_POINT('Ctrl Pts',(-18.1932733581975,14.0000000000496,122.161208794752)) ;
#18935=CARTESIAN_POINT('Ctrl Pts',(-18.6506738232679,13.7000000000496,121.505064333141)) ;
#18936=CARTESIAN_POINT('Ctrl Pts',(-18.7644631958589,14.0000000000496,121.791079731755)) ;
#18937=CARTESIAN_POINT('Ctrl Pts',(-19.4380847682357,13.7000000000496,121.359900422812)) ;
#18938=CARTESIAN_POINT('Ctrl Pts',(-19.4337624984685,14.0000000000496,121.66769040749)) ;
#18939=CARTESIAN_POINT('Ctrl Pts',(-20.2211414796236,13.7000000000496,121.527121835554)) ;
#18940=CARTESIAN_POINT('Ctrl Pts',(-20.0993607034912,14.0000000000496,121.809828608283)) ;
#18941=CARTESIAN_POINT('Ctrl Pts',(-20.8805842197971,13.7000000000496,121.98127732928)) ;
#18942=CARTESIAN_POINT('Ctrl Pts',(-20.659887032884,14.0000000000496,122.195860778204)) ;
#18943=CARTESIAN_POINT('Ctrl Pts',(-21.3160439046833,13.7000000000496,122.653223034764)) ;
#18944=CARTESIAN_POINT('Ctrl Pts',(-21.0300277648268,14.0000000000496,122.767014628009)) ;
#18945=CARTESIAN_POINT('Ctrl Pts',(-21.4612001247882,13.7000000000496,123.440656932859)) ;
#18946=CARTESIAN_POINT('Ctrl Pts',(-21.153410552117,14.0000000000496,123.436333440585)) ;
#18947=CARTESIAN_POINT('Ctrl Pts',(-21.2939830415349,13.7000000000496,124.223700813763)) ;
#18948=CARTESIAN_POINT('Ctrl Pts',(-21.0112760309154,14.0000000000496,124.101920740338)) ;
#18949=CARTESIAN_POINT('Ctrl Pts',(-20.8398250592352,13.7000000000496,124.883150895787)) ;
#18950=CARTESIAN_POINT('Ctrl Pts',(-20.6252417466303,14.0000000000496,124.66245330923)) ;
#18951=CARTESIAN_POINT('Ctrl Pts',(-20.1678807467438,13.7000000000496,125.318606455482)) ;
#18952=CARTESIAN_POINT('Ctrl Pts',(-20.0540890803185,14.0000000000496,125.032590535832)) ;
#18953=CARTESIAN_POINT('Ctrl Pts',(-19.3804460839353,13.7000000000496,125.463764952492)) ;
#18954=CARTESIAN_POINT('Ctrl Pts',(-19.3847696171534,14.0000000000496,125.155975257797)) ;
#18955=CARTESIAN_POINT('Ctrl Pts',(-18.5974015471293,13.7000000000496,125.296545502889)) ;
#18956=CARTESIAN_POINT('Ctrl Pts',(-18.7191817607918,14.0000000000496,125.013838725625)) ;
#18957=CARTESIAN_POINT('Ctrl Pts',(-17.937927323658,13.7000000000496,124.842390490218)) ;
#18958=CARTESIAN_POINT('Ctrl Pts',(-18.1586286713331,14.0000000000496,124.627806965402)) ;
#18959=CARTESIAN_POINT('Ctrl Pts',(-17.5025443176974,13.7000000000496,124.17043143519)) ;
#18960=CARTESIAN_POINT('Ctrl Pts',(-17.7885531153341,14.0000000000496,124.056641767528)) ;
#18961=CARTESIAN_POINT('Ctrl Pts',(-17.4056391005857,13.7000000000496,123.645494286554)) ;
#18962=CARTESIAN_POINT('Ctrl Pts',(-17.7061836816795,14.0000000000496,123.610445192173)) ;
#18963=CARTESIAN_POINT('Ctrl Pts',(-17.409466984686,13.7000000000496,123.383738395492)) ;
#18964=CARTESIAN_POINT('Ctrl Pts',(-17.7094373828403,14.0000000000496,123.387952684416)) ;
#18965=CARTESIAN_POINT('',(-17.409466984686,13.7000000000496,123.383738395492)) ;
#18966=CARTESIAN_POINT('Origin',(-19.4092722359532,-11.3545356292023,123.411814366564)) ;
#18967=CARTESIAN_POINT('',(-19.4092722359532,-10.8644715472508,123.411814366564)) ;
#18968=CARTESIAN_POINT('',(-18.2115676001213,-11.4089871938635,123.054038451525)) ;
#18969=CARTESIAN_POINT('',(-18.3313380637045,-11.3545356292023,123.089816043029)) ;
#18970=CARTESIAN_POINT('',(-18.2266423654683,-11.4089871938635,123.816643453356)) ;
#18971=CARTESIAN_POINT('Origin',(-19.4092722359532,-11.4089871938635,123.411814366564)) ;
#18972=CARTESIAN_POINT('Origin',(-19.4092722359532,-11.4089871938635,123.411814366564)) ;
#18973=CARTESIAN_POINT('Origin',(-19.4092722359532,11.3545356292023,123.411814366564)) ;
#18974=CARTESIAN_POINT('',(-20.5919021064381,11.4089871938635,123.006985279772)) ;
#18975=CARTESIAN_POINT('',(-18.2115676001212,11.4089871938635,123.054038451525)) ;
#18976=CARTESIAN_POINT('Origin',(-19.4092722359532,11.4089871938635,123.411814366564)) ;
#18977=CARTESIAN_POINT('',(-19.4092722359532,10.8644715472508,123.411814366564)) ;
#18978=CARTESIAN_POINT('',(-18.3313380637044,11.3545356292023,123.089816043029)) ;
#18979=CARTESIAN_POINT('Origin',(-19.4092722359532,11.4089871938635,123.411814366564)) ;
#18980=CARTESIAN_POINT('Ctrl Pts',(-20.5445170967909,10.1799890803629,123.023196933748)) ;
#18981=CARTESIAN_POINT('Ctrl Pts',(-20.8283303706881,10.,122.926041870813)) ;
#18982=CARTESIAN_POINT('Ctrl Pts',(-20.5894888412031,10.186615931181,123.154521494311)) ;
#18983=CARTESIAN_POINT('Ctrl Pts',(-20.8845408159969,10.0066268508181,123.090165629856)) ;
#18984=CARTESIAN_POINT('Ctrl Pts',(-20.6334208464893,10.199846557662,123.432353270138)) ;
#18985=CARTESIAN_POINT('Ctrl Pts',(-20.9394617690737,10.0198574772991,123.437507823531)) ;
#18986=CARTESIAN_POINT('Ctrl Pts',(-20.5528814488852,10.2198221789206,123.849407494597)) ;
#18987=CARTESIAN_POINT('Ctrl Pts',(-20.8387858493119,10.0398330985578,123.958797508285)) ;
#18988=CARTESIAN_POINT('Ctrl Pts',(-20.3351890798294,10.2397395138226,124.21264452173)) ;
#18989=CARTESIAN_POINT('Ctrl Pts',(-20.5666727975867,10.0597504334597,124.412849839357)) ;
#18990=CARTESIAN_POINT('Ctrl Pts',(-20.0078940908122,10.2596127905386,124.479989674566)) ;
#18991=CARTESIAN_POINT('Ctrl Pts',(-20.157556275784,10.0796237101757,124.747029739186)) ;
#18992=CARTESIAN_POINT('Ctrl Pts',(-19.6059540280892,10.2796372807025,124.620350189469)) ;
#18993=CARTESIAN_POINT('Ctrl Pts',(-19.6551315118144,10.0996482003397,124.922482691163)) ;
#18994=CARTESIAN_POINT('Ctrl Pts',(-19.1834791470516,10.2995051218533,124.615075219233)) ;
#18995=CARTESIAN_POINT('Ctrl Pts',(-19.1270395366036,10.1195160414904,124.915890798164)) ;
#18996=CARTESIAN_POINT('Ctrl Pts',(-18.7864839057826,10.3194507727328,124.466021113069)) ;
#18997=CARTESIAN_POINT('Ctrl Pts',(-18.6307952228403,10.1394616923699,124.72957580943)) ;
#18998=CARTESIAN_POINT('Ctrl Pts',(-18.4649063701951,10.3393561733498,124.190844404071)) ;
#18999=CARTESIAN_POINT('Ctrl Pts',(-18.2288224078826,10.1593670929869,124.385607616877)) ;
#19000=CARTESIAN_POINT('Ctrl Pts',(-18.2561330011468,10.3592304011661,123.82343533093)) ;
#19001=CARTESIAN_POINT('Ctrl Pts',(-17.9678535157127,10.1792413208033,123.926349000794)) ;
#19002=CARTESIAN_POINT('Ctrl Pts',(-18.1848402354332,10.3792161920437,123.40449567957)) ;
#19003=CARTESIAN_POINT('Ctrl Pts',(-17.878734209588,10.1992271116809,123.402675114316)) ;
#19004=CARTESIAN_POINT('Ctrl Pts',(-18.2606699010585,10.3991104347035,122.98837126667)) ;
#19005=CARTESIAN_POINT('Ctrl Pts',(-17.973517700436,10.2191213543406,122.882519965019)) ;
#19006=CARTESIAN_POINT('Ctrl Pts',(-18.4728612596363,10.4189891507756,122.622758653604)) ;
#19007=CARTESIAN_POINT('Ctrl Pts',(-18.2387528910803,10.2390000704127,122.425502981447)) ;
#19008=CARTESIAN_POINT('Ctrl Pts',(-18.7999520439114,10.4390286006202,122.349765919269)) ;
#19009=CARTESIAN_POINT('Ctrl Pts',(-18.647614090005,10.2590395202573,122.084258749108)) ;
#19010=CARTESIAN_POINT('Ctrl Pts',(-19.1972003355021,10.458891762158,122.205978453982)) ;
#19011=CARTESIAN_POINT('Ctrl Pts',(-19.1441721121047,10.2789026817952,121.90452088182)) ;
#19012=CARTESIAN_POINT('Ctrl Pts',(-19.6218813508038,10.4788711301723,122.206142579944)) ;
#19013=CARTESIAN_POINT('Ctrl Pts',(-19.6750232066901,10.2988820498094,121.904721686728)) ;
#19014=CARTESIAN_POINT('Ctrl Pts',(-20.0180063674985,10.4986817106951,122.349636080019)) ;
#19015=CARTESIAN_POINT('Ctrl Pts',(-20.1701799765179,10.3186926303322,122.084083785786)) ;
#19016=CARTESIAN_POINT('Ctrl Pts',(-20.3444408594761,10.5186626389807,122.621421727286)) ;
#19017=CARTESIAN_POINT('Ctrl Pts',(-20.578226084171,10.3386735586178,122.423812224567)) ;
#19018=CARTESIAN_POINT('Ctrl Pts',(-20.5574140360782,10.5385553108501,122.986919561501)) ;
#19019=CARTESIAN_POINT('Ctrl Pts',(-20.8444469588477,10.3585662304872,122.880680954098)) ;
#19020=CARTESIAN_POINT('Ctrl Pts',(-20.6337210602673,10.5584816411372,123.403677138751)) ;
#19021=CARTESIAN_POINT('Ctrl Pts',(-20.9398341757817,10.3784925607743,123.40162915944)) ;
#19022=CARTESIAN_POINT('Ctrl Pts',(-20.5626906544988,10.5784521952295,123.822322212015)) ;
#19023=CARTESIAN_POINT('Ctrl Pts',(-20.8510572230715,10.3984631148666,123.924927290891)) ;
#19024=CARTESIAN_POINT('Ctrl Pts',(-20.3894921739839,10.5949840343171,124.128174611121)) ;
#19025=CARTESIAN_POINT('Ctrl Pts',(-20.6345446351863,10.4149949539542,124.307272603886)) ;
#19026=CARTESIAN_POINT('Ctrl Pts',(-20.1931290904253,10.6083237731447,124.328455789616)) ;
#19027=CARTESIAN_POINT('Ctrl Pts',(-20.3891097552813,10.4283346927818,124.557601822174)) ;
#19028=CARTESIAN_POINT('Ctrl Pts',(-20.0213870270135,10.6183560153633,124.45086066554)) ;
#19029=CARTESIAN_POINT('Ctrl Pts',(-20.1744300570267,10.4383669350004,124.710615084593)) ;
#19030=CARTESIAN_POINT('Ctrl Pts',(-19.8344327780229,10.6282137160067,124.54030505442)) ;
#19031=CARTESIAN_POINT('Ctrl Pts',(-19.9407404802418,10.4482246356439,124.822421617883)) ;
#19032=CARTESIAN_POINT('Ctrl Pts',(-19.6321963819504,10.638205580646,124.597047913329)) ;
#19033=CARTESIAN_POINT('Ctrl Pts',(-19.6879423525307,10.4582165002831,124.893352629427)) ;
#19034=CARTESIAN_POINT('Ctrl Pts',(-19.424609722569,10.6481281304061,124.617626313307)) ;
#19035=CARTESIAN_POINT('Ctrl Pts',(-19.4284710425139,10.4681390500432,124.919080315321)) ;
#19036=CARTESIAN_POINT('Ctrl Pts',(-19.1462074516632,10.6614059038996,124.597234583046)) ;
#19037=CARTESIAN_POINT('Ctrl Pts',(-19.0804105140851,10.4814168235367,124.893583985624)) ;
#19038=CARTESIAN_POINT('Ctrl Pts',(-18.8783190629616,10.6747532428402,124.503658368855)) ;
#19039=CARTESIAN_POINT('Ctrl Pts',(-18.7455859092888,10.4947641624773,124.776616835755)) ;
#19040=CARTESIAN_POINT('Ctrl Pts',(-18.6486031256444,10.6879604746334,124.347593152274)) ;
#19041=CARTESIAN_POINT('Ctrl Pts',(-18.4584522382473,10.5079713942705,124.581549246914)) ;
#19042=CARTESIAN_POINT('Ctrl Pts',(-18.4978121198163,10.6979475907231,124.201545393376)) ;
#19043=CARTESIAN_POINT('Ctrl Pts',(-18.269958838059,10.5179585103602,124.398989341533)) ;
#19044=CARTESIAN_POINT('Ctrl Pts',(-18.3749610360081,10.7078984963028,124.032167626381)) ;
#19045=CARTESIAN_POINT('Ctrl Pts',(-18.1163933969716,10.52790941594,124.187269395838)) ;
#19046=CARTESIAN_POINT('Ctrl Pts',(-18.2826761324805,10.7179535983103,123.842018510299)) ;
#19047=CARTESIAN_POINT('Ctrl Pts',(-18.0010345813923,10.5379645179474,123.949583784548)) ;
#19048=CARTESIAN_POINT('Ctrl Pts',(-18.2257894495901,10.7277752716314,123.643501818388)) ;
#19049=CARTESIAN_POINT('Ctrl Pts',(-17.9299233421522,10.5477861912685,123.701439503961)) ;
#19050=CARTESIAN_POINT('Ctrl Pts',(-18.2033755349775,10.7378337427063,123.433255143292)) ;
#19051=CARTESIAN_POINT('Ctrl Pts',(-17.9019040586336,10.5578446623434,123.43862866708)) ;
#19052=CARTESIAN_POINT('Ctrl Pts',(-18.2179011335089,10.7477583538828,123.225094347349)) ;
#19053=CARTESIAN_POINT('Ctrl Pts',(-17.9200547531203,10.5677692735199,123.178437417212)) ;
#19054=CARTESIAN_POINT('Ctrl Pts',(-18.2846726130989,10.7610356927832,122.954084571752)) ;
#19055=CARTESIAN_POINT('Ctrl Pts',(-18.0035329037317,10.5810466124203,122.839624585047)) ;
#19056=CARTESIAN_POINT('Ctrl Pts',(-18.4211117191118,10.7743345720208,122.706442666777)) ;
#19057=CARTESIAN_POINT('Ctrl Pts',(-18.174078890485,10.5943454916579,122.53009645584)) ;
#19058=CARTESIAN_POINT('Ctrl Pts',(-18.6137282560997,10.7875734441915,122.505480302123)) ;
#19059=CARTESIAN_POINT('Ctrl Pts',(-18.4148290889509,10.6075843638286,122.278909287836)) ;
#19060=CARTESIAN_POINT('Ctrl Pts',(-18.7832424185157,10.7975800623281,122.380894161506)) ;
#19061=CARTESIAN_POINT('Ctrl Pts',(-18.6267237904145,10.6175909819652,122.123170592624)) ;
#19062=CARTESIAN_POINT('Ctrl Pts',(-18.9724474720446,10.8076110073896,122.287775791708)) ;
#19063=CARTESIAN_POINT('Ctrl Pts',(-18.8632279358434,10.6276219270267,122.006771081612)) ;
#19064=CARTESIAN_POINT('Ctrl Pts',(-19.1713300500782,10.8174671807414,122.229578165669)) ;
#19065=CARTESIAN_POINT('Ctrl Pts',(-19.1118308518252,10.6374781003785,121.93402103227)) ;
#19066=CARTESIAN_POINT('Ctrl Pts',(-19.3802073449411,10.8274664517043,122.206207727251)) ;
#19067=CARTESIAN_POINT('Ctrl Pts',(-19.3729271808616,10.6474773713414,121.904805274484)) ;
#19068=CARTESIAN_POINT('Ctrl Pts',(-19.5878599933699,10.8373609034616,122.219083370884)) ;
#19069=CARTESIAN_POINT('Ctrl Pts',(-19.63249343999,10.6573718230987,121.920897070182)) ;
#19070=CARTESIAN_POINT('Ctrl Pts',(-19.7934840277289,10.847424219271,122.268698552168)) ;
#19071=CARTESIAN_POINT('Ctrl Pts',(-19.8895240952696,10.6674351389081,121.982913347126)) ;
#19072=CARTESIAN_POINT('Ctrl Pts',(-19.9832086160557,10.8572630760106,122.351185619817)) ;
#19073=CARTESIAN_POINT('Ctrl Pts',(-20.1266813029374,10.6772739956477,122.086019825898)) ;
#19074=CARTESIAN_POINT('Ctrl Pts',(-20.1597838606521,10.8673291978282,122.467764324916)) ;
#19075=CARTESIAN_POINT('Ctrl Pts',(-20.3474018172676,10.6873401174653,122.231740902041)) ;
#19076=CARTESIAN_POINT('Ctrl Pts',(-20.3106209535211,10.8772124255524,122.610700532014)) ;
#19077=CARTESIAN_POINT('Ctrl Pts',(-20.5359503275351,10.6972233451896,122.410409425907)) ;
#19078=CARTESIAN_POINT('Ctrl Pts',(-20.4360184408181,10.8872018868312,122.779136894016)) ;
#19079=CARTESIAN_POINT('Ctrl Pts',(-20.6926994160287,10.7072128064683,122.620953380555)) ;
#19080=CARTESIAN_POINT('Ctrl Pts',(-20.5299682723289,10.8971655972577,122.966365986146)) ;
#19081=CARTESIAN_POINT('Ctrl Pts',(-20.8101391925705,10.7171765168948,122.854988704109)) ;
#19082=CARTESIAN_POINT('Ctrl Pts',(-20.5903840833054,10.9071605999886,123.167636072351)) ;
#19083=CARTESIAN_POINT('Ctrl Pts',(-20.8856615342042,10.7271715196257,123.106575647569)) ;
#19084=CARTESIAN_POINT('Ctrl Pts',(-20.6147046372521,10.9171969309989,123.377214474421)) ;
#19085=CARTESIAN_POINT('Ctrl Pts',(-20.9160649147156,10.737207850636,123.368548316933)) ;
#19086=CARTESIAN_POINT('Ctrl Pts',(-20.602840741777,10.9270431603412,123.583885830223)) ;
#19087=CARTESIAN_POINT('Ctrl Pts',(-20.901237668564,10.7470540799783,123.626888226543)) ;
#19088=CARTESIAN_POINT('Ctrl Pts',(-20.5549910593693,10.9370286586164,123.788252345139)) ;
#19089=CARTESIAN_POINT('Ctrl Pts',(-20.8414280631531,10.7570395782535,123.88234711985)) ;
#19090=CARTESIAN_POINT('Ctrl Pts',(-20.4729131510359,10.9469635615994,123.98035400042)) ;
#19091=CARTESIAN_POINT('Ctrl Pts',(-20.7388329136923,10.7669744812365,124.122475498249)) ;
#19092=CARTESIAN_POINT('Ctrl Pts',(-20.3571965408839,10.9570210646946,124.157283328264)) ;
#19093=CARTESIAN_POINT('Ctrl Pts',(-20.5941893977946,10.7770319843317,124.343638489499)) ;
#19094=CARTESIAN_POINT('Ctrl Pts',(-20.2161055904513,10.9668427210651,124.308072643193)) ;
#19095=CARTESIAN_POINT('Ctrl Pts',(-20.4178270374552,10.7868536407023,124.532127444505)) ;
#19096=CARTESIAN_POINT('Ctrl Pts',(-20.0473038580147,10.9768987837303,124.435324360385)) ;
#19097=CARTESIAN_POINT('Ctrl Pts',(-20.2068264505713,10.7969097033674,124.691194003415)) ;
#19098=CARTESIAN_POINT('Ctrl Pts',(-19.8609387437001,10.9868394484335,124.529907956578)) ;
#19099=CARTESIAN_POINT('Ctrl Pts',(-19.9738709151238,10.8068503680706,124.809425923824)) ;
#19100=CARTESIAN_POINT('Ctrl Pts',(-19.6619073820417,10.996743852382,124.591096321842)) ;
#19101=CARTESIAN_POINT('Ctrl Pts',(-19.7250819168071,10.8167547720191,124.885913848072)) ;
#19102=CARTESIAN_POINT('Ctrl Pts',(-19.4523135812511,11.0067903373756,124.6170333815)) ;
#19103=CARTESIAN_POINT('Ctrl Pts',(-19.4630900672441,10.8268012570127,124.918337587752)) ;
#19104=CARTESIAN_POINT('Ctrl Pts',(-19.2444994497963,11.0166865651873,124.606521749711)) ;
#19105=CARTESIAN_POINT('Ctrl Pts',(-19.2033217042056,10.8366974848244,124.905200421478)) ;
#19106=CARTESIAN_POINT('Ctrl Pts',(-19.038362504801,11.0267461487508,124.559366648931)) ;
#19107=CARTESIAN_POINT('Ctrl Pts',(-18.9456501548748,10.8467570683879,124.846258925075)) ;
#19108=CARTESIAN_POINT('Ctrl Pts',(-18.8475263552642,11.0365981584196,124.478841690953)) ;
#19109=CARTESIAN_POINT('Ctrl Pts',(-18.7071032762899,10.8566090780567,124.745604613553)) ;
#19110=CARTESIAN_POINT('Ctrl Pts',(-18.6712543899711,11.0465606898592,124.365745599051)) ;
#19111=CARTESIAN_POINT('Ctrl Pts',(-18.4867618466311,10.8665716094963,124.604236201826)) ;
#19112=CARTESIAN_POINT('Ctrl Pts',(-18.5164393691186,11.0565922380985,124.222526123336)) ;
#19113=CARTESIAN_POINT('Ctrl Pts',(-18.2932415519936,10.8766031577357,124.425213596724)) ;
#19114=CARTESIAN_POINT('Ctrl Pts',(-18.3904718457185,11.0664836493116,124.057073079274)) ;
#19115=CARTESIAN_POINT('Ctrl Pts',(-18.1357799386366,10.8864945689487,124.218398117847)) ;
#19116=CARTESIAN_POINT('Ctrl Pts',(-18.2936007393847,11.0764999030196,123.870096289376)) ;
#19117=CARTESIAN_POINT('Ctrl Pts',(-18.0146891209222,10.8965108226567,123.984678099418)) ;
#19118=CARTESIAN_POINT('Ctrl Pts',(-18.2310191009212,11.0865300058643,123.668736110514)) ;
#19119=CARTESIAN_POINT('Ctrl Pts',(-17.9364599064937,10.9065409255014,123.732978598351)) ;
#19120=CARTESIAN_POINT('Ctrl Pts',(-18.2044167485645,11.096386454818,123.463224365483)) ;
#19121=CARTESIAN_POINT('Ctrl Pts',(-17.9032046926023,10.9163973744551,123.476088297528)) ;
#19122=CARTESIAN_POINT('Ctrl Pts',(-18.2137726552221,11.1063854655903,123.253255515666)) ;
#19123=CARTESIAN_POINT('Ctrl Pts',(-17.9148974747618,10.9263963852274,123.213627004979)) ;
#19124=CARTESIAN_POINT('Ctrl Pts',(-18.2587594656026,11.1162806825083,123.050114933331)) ;
#19125=CARTESIAN_POINT('Ctrl Pts',(-17.9711291549323,10.9362916021454,122.959700121601)) ;
#19126=CARTESIAN_POINT('Ctrl Pts',(-18.3396629587075,11.1263411978656,122.85472528768)) ;
#19127=CARTESIAN_POINT('Ctrl Pts',(-18.0722565351528,10.9463521175027,122.715462501341)) ;
#19128=CARTESIAN_POINT('Ctrl Pts',(-18.4508021074728,11.1361904912527,122.67999776762)) ;
#19129=CARTESIAN_POINT('Ctrl Pts',(-18.2111793287984,10.9562014108898,122.497051143162)) ;
#19130=CARTESIAN_POINT('Ctrl Pts',(-18.5927075074045,11.1462176669327,122.524117766382)) ;
#19131=CARTESIAN_POINT('Ctrl Pts',(-18.388559678523,10.9662285865698,122.302199917963)) ;
#19132=CARTESIAN_POINT('Ctrl Pts',(-18.7598974171996,11.1562462425598,122.39565716601)) ;
#19133=CARTESIAN_POINT('Ctrl Pts',(-18.5975457775489,10.976257162197,122.141622604304)) ;
#19134=CARTESIAN_POINT('Ctrl Pts',(-18.9432305176374,11.1660913361057,122.299619707887)) ;
#19135=CARTESIAN_POINT('Ctrl Pts',(-18.8267122580128,10.9861022557429,122.021573575598)) ;
#19136=CARTESIAN_POINT('Ctrl Pts',(-19.1432259259205,11.1760825775375,122.235411488495)) ;
#19137=CARTESIAN_POINT('Ctrl Pts',(-19.0767061726053,10.9960934971746,121.941311591283)) ;
#19138=CARTESIAN_POINT('Ctrl Pts',(-19.3523221570473,11.1861183586808,122.207211675339)) ;
#19139=CARTESIAN_POINT('Ctrl Pts',(-19.3380760888337,11.0061292783179,121.906059986019)) ;
#19140=CARTESIAN_POINT('Ctrl Pts',(-19.5592805247249,11.1959705644105,122.215313540189)) ;
#19141=CARTESIAN_POINT('Ctrl Pts',(-19.5967752495355,11.0159814840476,121.916185579079)) ;
#19142=CARTESIAN_POINT('Ctrl Pts',(-19.7640786083089,11.2059326585275,122.259120874168)) ;
#19143=CARTESIAN_POINT('Ctrl Pts',(-19.8527735772293,11.0259435781646,121.970943280899)) ;
#19144=CARTESIAN_POINT('Ctrl Pts',(-19.9592440107104,11.2159552193546,122.338540115345)) ;
#19145=CARTESIAN_POINT('Ctrl Pts',(-20.0967309229679,11.0359661389917,122.070215768955)) ;
#19146=CARTESIAN_POINT('Ctrl Pts',(-20.1360936806095,11.2258829910061,122.449415578369)) ;
#19147=CARTESIAN_POINT('Ctrl Pts',(-20.3177943873502,11.0458939106433,122.208809071659)) ;
#19148=CARTESIAN_POINT('Ctrl Pts',(-20.2927527732055,11.235925375131,122.59092205436)) ;
#19149=CARTESIAN_POINT('Ctrl Pts',(-20.513619210783,11.0559362947681,122.385690857822)) ;
#19150=CARTESIAN_POINT('Ctrl Pts',(-20.4205680894076,11.2458145992016,122.754908938647)) ;
#19151=CARTESIAN_POINT('Ctrl Pts',(-20.6733901753496,11.0658255188387,122.590674219405)) ;
#19152=CARTESIAN_POINT('Ctrl Pts',(-20.5192928454941,11.2558038473689,122.940253974445)) ;
#19153=CARTESIAN_POINT('Ctrl Pts',(-20.7967974985103,11.075814767006,122.822355021181)) ;
#19154=CARTESIAN_POINT('Ctrl Pts',(-20.5839847168731,11.2657624244109,123.139363117153)) ;
#19155=CARTESIAN_POINT('Ctrl Pts',(-20.8776639039544,11.085773344048,123.07124139589)) ;
#19156=CARTESIAN_POINT('Ctrl Pts',(-20.6134608095792,11.2756619935022,123.345397790749)) ;
#19157=CARTESIAN_POINT('Ctrl Pts',(-20.9145104547189,11.0956729131393,123.328785419539)) ;
#19158=CARTESIAN_POINT('Ctrl Pts',(-20.6065401284065,11.2857099055862,123.556501597487)) ;
#19159=CARTESIAN_POINT('Ctrl Pts',(-20.9058609614056,11.1057208252233,123.592665004876)) ;
#19160=CARTESIAN_POINT('Ctrl Pts',(-20.5638788823548,11.2956052598934,123.760144762529)) ;
#19161=CARTESIAN_POINT('Ctrl Pts',(-20.8525354819136,11.1156161795305,123.847220118537)) ;
#19162=CARTESIAN_POINT('Ctrl Pts',(-20.4852553344784,11.3056669103846,123.956492429052)) ;
#19163=CARTESIAN_POINT('Ctrl Pts',(-20.7542573598821,11.1256778300217,124.092654877015)) ;
#19164=CARTESIAN_POINT('Ctrl Pts',(-20.3761505871013,11.315511525847,124.132371029593)) ;
#19165=CARTESIAN_POINT('Ctrl Pts',(-20.6178768119318,11.1355224454842,124.31250491989)) ;
#19166=CARTESIAN_POINT('Ctrl Pts',(-20.237114111558,11.3254716047484,124.288935623539)) ;
#19167=CARTESIAN_POINT('Ctrl Pts',(-20.4440816600714,11.1454825243856,124.508211665868)) ;
#19168=CARTESIAN_POINT('Ctrl Pts',(-20.0714663398208,11.3355097991068,124.419675506507)) ;
#19169=CARTESIAN_POINT('Ctrl Pts',(-20.2370227832588,11.1555207187439,124.671637321506)) ;
#19170=CARTESIAN_POINT('Ctrl Pts',(-19.8888323535182,11.3453835145064,124.518385640457)) ;
#19171=CARTESIAN_POINT('Ctrl Pts',(-20.0087297938616,11.1653944341435,124.795026404838)) ;
#19172=CARTESIAN_POINT('Ctrl Pts',(-19.6879284940433,11.3554552240407,124.585159910392)) ;
#19173=CARTESIAN_POINT('Ctrl Pts',(-19.7576006730884,11.1754661436778,124.87849507525)) ;
#19174=CARTESIAN_POINT('Ctrl Pts',(-19.4834310386215,11.3652876644932,124.615427060217)) ;
#19175=CARTESIAN_POINT('Ctrl Pts',(-19.5019775459593,11.1852985841303,124.916330182897)) ;
#19176=CARTESIAN_POINT('Ctrl Pts',(-19.2726002542326,11.3753194854186,124.610200309681)) ;
#19177=CARTESIAN_POINT('Ctrl Pts',(-19.2384391664689,11.1953304050557,124.909797495667)) ;
#19178=CARTESIAN_POINT('Ctrl Pts',(-19.0662276962164,11.3853398553042,124.567903119432)) ;
#19179=CARTESIAN_POINT('Ctrl Pts',(-18.9804733109709,11.2053507749413,124.856926970494)) ;
#19180=CARTESIAN_POINT('Ctrl Pts',(-18.8731273416045,11.3952066264379,124.492104200881)) ;
#19181=CARTESIAN_POINT('Ctrl Pts',(-18.7390964607104,11.215217546075,124.762178595596)) ;
#19182=CARTESIAN_POINT('Ctrl Pts',(-18.6924952829997,11.4052773976273,124.381703676241)) ;
#19183=CARTESIAN_POINT('Ctrl Pts',(-18.5133063352698,11.2252883172644,124.624178813688)) ;
#19184=CARTESIAN_POINT('Ctrl Pts',(-18.5373237843845,11.4151205581489,124.244779697978)) ;
#19185=CARTESIAN_POINT('Ctrl Pts',(-18.3193404016488,11.235131477786,124.453023478491)) ;
#19186=CARTESIAN_POINT('Ctrl Pts',(-18.4059602071296,11.4251007913353,124.081184277243)) ;
#19187=CARTESIAN_POINT('Ctrl Pts',(-18.1551353492722,11.2451117109724,124.248529269541)) ;
#19188=CARTESIAN_POINT('Ctrl Pts',(-18.3049653385912,11.4351193113705,123.896363057127)) ;
#19189=CARTESIAN_POINT('Ctrl Pts',(-18.028891195577,11.2551302310076,124.017503067163)) ;
#19190=CARTESIAN_POINT('Ctrl Pts',(-18.2380760069019,11.4450026197542,123.69961958379)) ;
#19191=CARTESIAN_POINT('Ctrl Pts',(-17.94527872475,11.2650135393913,123.771572840937)) ;
#19192=CARTESIAN_POINT('Ctrl Pts',(-18.2058712454328,11.455070903925,123.490451765677)) ;
#19193=CARTESIAN_POINT('Ctrl Pts',(-17.9050223248742,11.2750818235621,123.510113552435)) ;
#19194=CARTESIAN_POINT('Ctrl Pts',(-18.2101233464429,11.4649010305926,123.283800583045)) ;
#19195=CARTESIAN_POINT('Ctrl Pts',(-17.9103370638304,11.2849119502298,123.251798025967)) ;
#19196=CARTESIAN_POINT('Ctrl Pts',(-18.250874219467,11.4749676027992,123.076164349147)) ;
#19197=CARTESIAN_POINT('Ctrl Pts',(-17.9612752714376,11.2949785224363,122.992253063296)) ;
#19198=CARTESIAN_POINT('Ctrl Pts',(-18.3258631651741,11.4848577590399,122.882207935105)) ;
#19199=CARTESIAN_POINT('Ctrl Pts',(-18.0550114914209,11.304868678677,122.749806436418)) ;
#19200=CARTESIAN_POINT('Ctrl Pts',(-18.4340938733603,11.4948502866163,122.702175775169)) ;
#19201=CARTESIAN_POINT('Ctrl Pts',(-18.1902998279982,11.3148612062534,122.524765958901)) ;
#19202=CARTESIAN_POINT('Ctrl Pts',(-18.5716561470465,11.5048117764906,122.544271291541)) ;
#19203=CARTESIAN_POINT('Ctrl Pts',(-18.362252777776,11.3248226961277,122.327384835979)) ;
#19204=CARTESIAN_POINT('Ctrl Pts',(-18.733397668661,11.5147209983778,122.412963329841)) ;
#19205=CARTESIAN_POINT('Ctrl Pts',(-18.5644303505552,11.3347319180149,122.163249256382)) ;
#19206=CARTESIAN_POINT('Ctrl Pts',(-18.9180612846803,11.5247695781881,122.310386430444)) ;
#19207=CARTESIAN_POINT('Ctrl Pts',(-18.7952595963488,11.3447804978252,122.035028175252)) ;
#19208=CARTESIAN_POINT('Ctrl Pts',(-19.1144372305553,11.5346525526582,122.242490101265)) ;
#19209=CARTESIAN_POINT('Ctrl Pts',(-19.0407305551564,11.3546634722953,121.950157334317)) ;
#19210=CARTESIAN_POINT('Ctrl Pts',(-19.3218535876862,11.5446474638009,122.208905343626)) ;
#19211=CARTESIAN_POINT('Ctrl Pts',(-19.3000011957523,11.364658383438,121.908176471057)) ;
#19212=CARTESIAN_POINT('Ctrl Pts',(-19.5325030834212,11.5546678503745,122.212142964224)) ;
#19213=CARTESIAN_POINT('Ctrl Pts',(-19.5633130308643,11.3746787700116,121.912223489131)) ;
#19214=CARTESIAN_POINT('Ctrl Pts',(-19.7371085501306,11.5645779542315,122.251347857035)) ;
#19215=CARTESIAN_POINT('Ctrl Pts',(-19.8190707586081,11.3845888738687,121.961229817149)) ;
#19216=CARTESIAN_POINT('Ctrl Pts',(-19.9323591296137,11.5745056664414,122.325110819767)) ;
#19217=CARTESIAN_POINT('Ctrl Pts',(-20.0631345837218,11.3945165860786,122.053434027889)) ;
#19218=CARTESIAN_POINT('Ctrl Pts',(-20.1138182396832,11.5845487762087,122.433038429192)) ;
#19219=CARTESIAN_POINT('Ctrl Pts',(-20.2899581915959,11.4045596958458,122.18834359306)) ;
#19220=CARTESIAN_POINT('Ctrl Pts',(-20.2713872169236,11.5944351966642,122.568595596171)) ;
#19221=CARTESIAN_POINT('Ctrl Pts',(-20.4869200798739,11.4144461163014,122.357790944953)) ;
#19222=CARTESIAN_POINT('Ctrl Pts',(-20.4047088338096,11.6044283742699,122.730945445389)) ;
#19223=CARTESIAN_POINT('Ctrl Pts',(-20.653571934063,11.424439293907,122.560728657171)) ;
#19224=CARTESIAN_POINT('Ctrl Pts',(-20.5072617933259,11.6143740371738,122.913157719128)) ;
#19225=CARTESIAN_POINT('Ctrl Pts',(-20.7817631202176,11.4343849568109,122.788494689918)) ;
#19226=CARTESIAN_POINT('Ctrl Pts',(-20.5770363442089,11.624321333379,123.110307996559)) ;
#19227=CARTESIAN_POINT('Ctrl Pts',(-20.8689810112581,11.4443322530161,123.034933251578)) ;
#19228=CARTESIAN_POINT('Ctrl Pts',(-20.6116338746559,11.6343690989569,123.318685651132)) ;
#19229=CARTESIAN_POINT('Ctrl Pts',(-20.9122274632139,11.454380018594,123.295405142899)) ;
#19230=CARTESIAN_POINT('Ctrl Pts',(-20.6097306714455,11.6442173121745,123.525714223304)) ;
#19231=CARTESIAN_POINT('Ctrl Pts',(-20.909847955661,11.4642282318116,123.554192250672)) ;
#19232=CARTESIAN_POINT('Ctrl Pts',(-20.5721619278645,11.6541768849686,123.731697031123)) ;
#19233=CARTESIAN_POINT('Ctrl Pts',(-20.8628861917845,11.4741878046057,123.811671085768)) ;
#19234=CARTESIAN_POINT('Ctrl Pts',(-20.4984904473743,11.6642135060011,123.92941246265)) ;
#19235=CARTESIAN_POINT('Ctrl Pts',(-20.7707963194684,11.4842244256382,124.058815012756)) ;
#19236=CARTESIAN_POINT('Ctrl Pts',(-20.3935356094815,11.6740940208114,124.108691624986)) ;
#19237=CARTESIAN_POINT('Ctrl Pts',(-20.6396015638057,11.4941049404486,124.282914554949)) ;
#19238=CARTESIAN_POINT('Ctrl Pts',(-20.2567978653035,11.6841466721185,124.269794367337)) ;
#19239=CARTESIAN_POINT('Ctrl Pts',(-20.4686789714687,11.5041575917556,124.484292270277)) ;
#19240=CARTESIAN_POINT('Ctrl Pts',(-20.0967123068534,11.6940420703985,124.40270437159)) ;
#19241=CARTESIAN_POINT('Ctrl Pts',(-20.2685707709031,11.5140529900356,124.650429772369)) ;
#19242=CARTESIAN_POINT('Ctrl Pts',(-19.9132571297185,11.7040921921046,124.507462775467)) ;
#19243=CARTESIAN_POINT('Ctrl Pts',(-20.0392516106828,11.5241031117417,124.781376915193)) ;
#19244=CARTESIAN_POINT('Ctrl Pts',(-19.7176472157066,11.7139764716465,124.577647205215)) ;
#19245=CARTESIAN_POINT('Ctrl Pts',(-19.794737934636,11.5339873912836,124.869107009898)) ;
#19246=CARTESIAN_POINT('Ctrl Pts',(-19.5106395256385,11.7239712529384,124.613575520575)) ;
#19247=CARTESIAN_POINT('Ctrl Pts',(-19.5359779545354,11.5439821725755,124.914016452958)) ;
#19248=CARTESIAN_POINT('Ctrl Pts',(-19.3014914963835,11.7339190981252,124.612936959039)) ;
#19249=CARTESIAN_POINT('Ctrl Pts',(-19.2745423776044,11.5539300177623,124.913217278818)) ;
#19250=CARTESIAN_POINT('Ctrl Pts',(-19.0958351736706,11.7438560615126,124.576338079464)) ;
#19251=CARTESIAN_POINT('Ctrl Pts',(-19.0174715357979,11.5638669811497,124.867467500935)) ;
#19252=CARTESIAN_POINT('Ctrl Pts',(-18.8986161272856,11.7538390262498,124.504485391709)) ;
#19253=CARTESIAN_POINT('Ctrl Pts',(-18.7709478903475,11.5738499458869,124.77765044511)) ;
#19254=CARTESIAN_POINT('Ctrl Pts',(-18.7159988224537,11.7638828776654,124.398530286436)) ;
#19255=CARTESIAN_POINT('Ctrl Pts',(-18.5426769439724,11.5838937973026,124.645205762056)) ;
#19256=CARTESIAN_POINT('Ctrl Pts',(-18.5576631664198,11.7737110790002,124.265735860728)) ;
#19257=CARTESIAN_POINT('Ctrl Pts',(-18.3447570490132,11.5937219986373,124.479210868658)) ;
#19258=CARTESIAN_POINT('Ctrl Pts',(-18.4214033173466,11.7837876515982,124.103588886124)) ;
#19259=CARTESIAN_POINT('Ctrl Pts',(-18.1744334770806,11.6037985712354,124.27652667465)) ;
#19260=CARTESIAN_POINT('Ctrl Pts',(-18.3175955543511,11.7936397316058,123.92430715972)) ;
#19261=CARTESIAN_POINT('Ctrl Pts',(-18.0446742700679,11.6136506512429,124.052422800966)) ;
#19262=CARTESIAN_POINT('Ctrl Pts',(-18.2447567569921,11.8037130166099,123.725492716322)) ;
#19263=CARTESIAN_POINT('Ctrl Pts',(-17.9536271837052,11.623723936247,123.80390465869)) ;
#19264=CARTESIAN_POINT('Ctrl Pts',(-18.2084461708989,11.8135543683204,123.521791919159)) ;
#19265=CARTESIAN_POINT('Ctrl Pts',(-17.9082400349615,11.6335652879575,123.549277141686)) ;
#19266=CARTESIAN_POINT('Ctrl Pts',(-18.2072783331998,11.8235158677169,123.312385813251)) ;
#19267=CARTESIAN_POINT('Ctrl Pts',(-17.9067818389188,11.643526787354,123.287519099378)) ;
#19268=CARTESIAN_POINT('Ctrl Pts',(-18.2431187666664,11.8335516438469,123.104460989179)) ;
#19269=CARTESIAN_POINT('Ctrl Pts',(-17.951583816689,11.653562563484,123.027613430416)) ;
#19270=CARTESIAN_POINT('Ctrl Pts',(-18.313260700151,11.8434400704844,122.908768536338)) ;
#19271=CARTESIAN_POINT('Ctrl Pts',(-18.0392630064654,11.6634509901216,122.782997517006)) ;
#19272=CARTESIAN_POINT('Ctrl Pts',(-18.4172968730816,11.8534553925594,122.725703223709)) ;
#19273=CARTESIAN_POINT('Ctrl Pts',(-18.169309686562,11.6734663121965,122.55416670281)) ;
#19274=CARTESIAN_POINT('Ctrl Pts',(-18.5521138610027,11.8634857414596,122.563558399555)) ;
#19275=CARTESIAN_POINT('Ctrl Pts',(-18.337832034103,11.6834966610967,122.351486710983)) ;
#19276=CARTESIAN_POINT('Ctrl Pts',(-18.7097629865951,11.8733291170662,122.429511598476)) ;
#19277=CARTESIAN_POINT('Ctrl Pts',(-18.5348954406339,11.6933400367034,122.18392868398)) ;
#19278=CARTESIAN_POINT('Ctrl Pts',(-18.8914357075047,11.8833585539634,122.322486366911)) ;
#19279=CARTESIAN_POINT('Ctrl Pts',(-18.7619871989816,11.7033694736005,122.05014873987)) ;
#19280=CARTESIAN_POINT('Ctrl Pts',(-19.0891853403317,11.8933904318963,122.249153011441)) ;
#19281=CARTESIAN_POINT('Ctrl Pts',(-19.0091747229,11.7134013515334,121.958483598159)) ;
#19282=CARTESIAN_POINT('Ctrl Pts',(-19.2923854095674,11.9032200550018,122.211622723258)) ;
#19283=CARTESIAN_POINT('Ctrl Pts',(-19.2631763810942,11.7232309746389,121.91157223852)) ;
#19284=CARTESIAN_POINT('Ctrl Pts',(-19.5023882087078,11.9132095261549,122.209287327401)) ;
#19285=CARTESIAN_POINT('Ctrl Pts',(-19.5256800788775,11.733220445792,121.908654949481)) ;
#19286=CARTESIAN_POINT('Ctrl Pts',(-19.7106392401679,11.9232533749173,122.244164803758)) ;
#19287=CARTESIAN_POINT('Ctrl Pts',(-19.7859934259949,11.7432642945544,121.95225353693)) ;
#19288=CARTESIAN_POINT('Ctrl Pts',(-19.9054125620073,11.933075080449,122.312709524051)) ;
#19289=CARTESIAN_POINT('Ctrl Pts',(-20.0294606191008,11.7530860000861,122.037936667196)) ;
#19290=CARTESIAN_POINT('Ctrl Pts',(-20.0894867289459,11.9431101202768,122.415781902165)) ;
#19291=CARTESIAN_POINT('Ctrl Pts',(-20.2595522204667,11.7631210399139,122.166778899388)) ;
#19292=CARTESIAN_POINT('Ctrl Pts',(-20.2523369083129,11.9531348271682,122.54956886486)) ;
#19293=CARTESIAN_POINT('Ctrl Pts',(-20.4631137171743,11.7731457468054,122.334014058184)) ;
#19294=CARTESIAN_POINT('Ctrl Pts',(-20.3874578810136,11.962987531509,122.706561960871)) ;
#19295=CARTESIAN_POINT('Ctrl Pts',(-20.6320140503155,11.7829984511461,122.530257519376)) ;
#19296=CARTESIAN_POINT('Ctrl Pts',(-20.4950292100305,11.9729756537167,122.88687951836)) ;
#19297=CARTESIAN_POINT('Ctrl Pts',(-20.7664764699797,11.7929865733538,122.755655719711)) ;
#19298=CARTESIAN_POINT('Ctrl Pts',(-20.5692290588118,11.982904123824,123.081978843733)) ;
#19299=CARTESIAN_POINT('Ctrl Pts',(-20.8592244692304,11.8029150434611,122.999531121806)) ;
#19300=CARTESIAN_POINT('Ctrl Pts',(-20.6090083992339,11.9928931009912,123.28818688241)) ;
#19301=CARTESIAN_POINT('Ctrl Pts',(-20.9089464870837,11.8129040206283,123.257291767332)) ;
#19302=CARTESIAN_POINT('Ctrl Pts',(-20.6120343021104,12.0029309082709,123.499185950342)) ;
#19303=CARTESIAN_POINT('Ctrl Pts',(-20.912726728438,11.822941827908,123.521040547069)) ;
#19304=CARTESIAN_POINT('Ctrl Pts',(-20.5793530027892,12.0127772091342,123.703591668076)) ;
#19305=CARTESIAN_POINT('Ctrl Pts',(-20.8718727620384,11.8327881287713,123.776548267499)) ;
#19306=CARTESIAN_POINT('Ctrl Pts',(-20.5108877173329,12.0228029525135,123.902937612404)) ;
#19307=CARTESIAN_POINT('Ctrl Pts',(-20.7862889531826,11.8428138721506,124.025729898005)) ;
#19308=CARTESIAN_POINT('Ctrl Pts',(-20.4083149981522,12.0328338189525,124.087198060114)) ;
#19309=CARTESIAN_POINT('Ctrl Pts',(-20.6580711492051,11.8528447385896,124.256054351195)) ;
#19310=CARTESIAN_POINT('Ctrl Pts',(-20.278204027201,12.0426711777513,124.247942559337)) ;
#19311=CARTESIAN_POINT('Ctrl Pts',(-20.4954300469777,11.8626820973884,124.456984258248)) ;
#19312=CARTESIAN_POINT('Ctrl Pts',(-20.1200700787013,12.052663138685,124.386216766339)) ;
#19313=CARTESIAN_POINT('Ctrl Pts',(-20.2977609080492,11.8726740583222,124.62982526479)) ;
#19314=CARTESIAN_POINT('Ctrl Pts',(-19.9393758024445,12.0626955012416,124.495014747097)) ;
#19315=CARTESIAN_POINT('Ctrl Pts',(-20.0718918884167,11.8827064208787,124.765820716401)) ;
#19316=CARTESIAN_POINT('Ctrl Pts',(-19.7459234684514,12.072560661816,124.569749829319)) ;
#19317=CARTESIAN_POINT('Ctrl Pts',(-19.830074922632,11.8925715814531,124.859237594725)) ;
#19318=CARTESIAN_POINT('Ctrl Pts',(-19.5405372405183,12.0825225663937,124.610739722099)) ;
#19319=CARTESIAN_POINT('Ctrl Pts',(-19.5733413955139,11.9025334860308,124.910472534242)) ;
#19320=CARTESIAN_POINT('Ctrl Pts',(-19.3296285023073,12.0925574964694,124.615133939641)) ;
#19321=CARTESIAN_POINT('Ctrl Pts',(-19.3097054567228,11.9125684161065,124.915962853087)) ;
#19322=CARTESIAN_POINT('Ctrl Pts',(-19.12418262518,12.102442443323,124.58366381539)) ;
#19323=CARTESIAN_POINT('Ctrl Pts',(-19.0528979312036,11.9224533629601,124.876622619197)) ;
#19324=CARTESIAN_POINT('Ctrl Pts',(-18.9237994034088,12.1125081196345,124.515756077525)) ;
#19325=CARTESIAN_POINT('Ctrl Pts',(-18.8024198540435,11.9325190392716,124.791735612442)) ;
#19326=CARTESIAN_POINT('Ctrl Pts',(-18.7422682640068,12.1223470392694,124.416531181598)) ;
#19327=CARTESIAN_POINT('Ctrl Pts',(-18.5755065294971,11.9423579589065,124.667701912514)) ;
#19328=CARTESIAN_POINT('Ctrl Pts',(-18.5769155643104,12.1324105490038,124.284598448374)) ;
#19329=CARTESIAN_POINT('Ctrl Pts',(-18.3688173844643,11.9524214686409,124.502784044984)) ;
#19330=CARTESIAN_POINT('Ctrl Pts',(-18.4394382528722,12.1423041621656,124.128483209612)) ;
#19331=CARTESIAN_POINT('Ctrl Pts',(-18.1969723593472,11.9623150818027,124.307637940785)) ;
#19332=CARTESIAN_POINT('Ctrl Pts',(-18.330159277488,12.152248168979,123.950297968068)) ;
#19333=CARTESIAN_POINT('Ctrl Pts',(-18.0603757685369,11.9722590886161,124.08490476088)) ;
#19334=CARTESIAN_POINT('Ctrl Pts',(-18.2529261348415,12.1622491233333,123.754711085262)) ;
#19335=CARTESIAN_POINT('Ctrl Pts',(-17.9638367967476,11.9822600429704,123.840420099808)) ;
#19336=CARTESIAN_POINT('Ctrl Pts',(-18.2110463667562,12.1722878810256,123.547880865785)) ;
#19337=CARTESIAN_POINT('Ctrl Pts',(-17.9114896578375,11.9922988006627,123.58188181945)) ;
#19338=CARTESIAN_POINT('Ctrl Pts',(-18.2053758043967,12.1821120651956,123.341406321408)) ;
#19339=CARTESIAN_POINT('Ctrl Pts',(-17.9044041219212,12.0021229848327,123.323787975382)) ;
#19340=CARTESIAN_POINT('Ctrl Pts',(-18.2360503167514,12.192170130795,123.132209463155)) ;
#19341=CARTESIAN_POINT('Ctrl Pts',(-17.9427499485555,12.0121810504321,123.062292370625)) ;
#19342=CARTESIAN_POINT('Ctrl Pts',(-18.302006424845,12.2021001775697,122.934128152636)) ;
#19343=CARTESIAN_POINT('Ctrl Pts',(-18.0251977237691,12.0221110972068,122.814691316201)) ;
#19344=CARTESIAN_POINT('Ctrl Pts',(-18.4010777311963,12.2120516199068,122.749859407281)) ;
#19345=CARTESIAN_POINT('Ctrl Pts',(-18.1490393731302,12.0320625395439,122.584356522223)) ;
#19346=CARTESIAN_POINT('Ctrl Pts',(-18.5321045118858,12.2220984170861,122.584200624693)) ;
#19347=CARTESIAN_POINT('Ctrl Pts',(-18.3128249788135,12.0421093367232,122.377284739554)) ;
#19348=CARTESIAN_POINT('Ctrl Pts',(-18.6866546754837,12.2319463577662,122.446441479111)) ;
#19349=CARTESIAN_POINT('Ctrl Pts',(-18.5060148098008,12.0519572774033,122.205087588693)) ;
#19350=CARTESIAN_POINT('Ctrl Pts',(-18.8644598958187,12.2419079891088,122.335805361285)) ;
#19351=CARTESIAN_POINT('Ctrl Pts',(-18.7282729224672,12.0619189087459,122.066794754727)) ;
#19352=CARTESIAN_POINT('Ctrl Pts',(-19.0602009714326,12.2519366484847,122.257435573529)) ;
#19353=CARTESIAN_POINT('Ctrl Pts',(-18.9729503385559,12.0719475681218,121.968835081685)) ;
#19354=CARTESIAN_POINT('Ctrl Pts',(-19.2641055065429,12.2618469513729,122.214691358915)) ;
#19355=CARTESIAN_POINT('Ctrl Pts',(-19.227831787757,12.08185787101,121.915407496624)) ;
#19356=CARTESIAN_POINT('Ctrl Pts',(-19.472848854405,12.2717818459351,122.20743693277)) ;
#19357=CARTESIAN_POINT('Ctrl Pts',(-19.4887612039821,12.0917927655722,121.906342273827)) ;
#19358=CARTESIAN_POINT('Ctrl Pts',(-19.6818517454895,12.281822944602,122.237040740592)) ;
#19359=CARTESIAN_POINT('Ctrl Pts',(-19.7500144690061,12.1018338642391,121.943349818059)) ;
#19360=CARTESIAN_POINT('Ctrl Pts',(-19.8795274393584,12.2917102271064,122.301350610276)) ;
#19361=CARTESIAN_POINT('Ctrl Pts',(-19.9971083719985,12.1117211467435,122.023739879768)) ;
#19362=CARTESIAN_POINT('Ctrl Pts',(-20.0651177529335,12.3017019676169,122.399712129327)) ;
#19363=CARTESIAN_POINT('Ctrl Pts',(-20.2290950029525,12.121712887254,122.146694306298)) ;
#19364=CARTESIAN_POINT('Ctrl Pts',(-20.2301016245503,12.3116525168523,122.52834286884)) ;
#19365=CARTESIAN_POINT('Ctrl Pts',(-20.4353231818005,12.1316634364894,122.307485013012)) ;
#19366=CARTESIAN_POINT('Ctrl Pts',(-20.3702511436106,12.3215881944871,122.68320837822)) ;
#19367=CARTESIAN_POINT('Ctrl Pts',(-20.6105080303125,12.1415991141242,122.501068844292)) ;
#19368=CARTESIAN_POINT('Ctrl Pts',(-20.4821440049613,12.3315736122799,122.86084640938)) ;
#19369=CARTESIAN_POINT('Ctrl Pts',(-20.750371753253,12.151584531917,122.723117938316)) ;
#19370=CARTESIAN_POINT('Ctrl Pts',(-20.561588894867,12.3416024051504,123.056141240279)) ;
#19371=CARTESIAN_POINT('Ctrl Pts',(-20.8496752814087,12.1616133247875,122.967237619846)) ;
#19372=CARTESIAN_POINT('Ctrl Pts',(-20.605473389762,12.3514819163783,123.25914772635)) ;
#19373=CARTESIAN_POINT('Ctrl Pts',(-20.9045281450594,12.1714928360155,123.220996340645)) ;
#19374=CARTESIAN_POINT('Ctrl Pts',(-20.6140174461044,12.3614754530513,123.469077690765)) ;
#19375=CARTESIAN_POINT('Ctrl Pts',(-20.9152054113298,12.1814863726884,123.483408955597)) ;
#19376=CARTESIAN_POINT('Ctrl Pts',(-20.5854395929456,12.3715077213151,123.67803354945)) ;
#19377=CARTESIAN_POINT('Ctrl Pts',(-20.8794802827671,12.1915186409522,123.744603500789)) ;
#19378=CARTESIAN_POINT('Ctrl Pts',(-20.5225086633852,12.381371683321,123.875648773567)) ;
#19379=CARTESIAN_POINT('Ctrl Pts',(-20.8008139737887,12.2013826029581,123.991621606298)) ;
#19380=CARTESIAN_POINT('Ctrl Pts',(-20.4242612791623,12.3914417446659,124.063150375643)) ;
#19381=CARTESIAN_POINT('Ctrl Pts',(-20.678002189668,12.211452664303,124.225997440401)) ;
#19382=CARTESIAN_POINT('Ctrl Pts',(-20.2978479151584,12.4012841090146,124.22697472228)) ;
#19383=CARTESIAN_POINT('Ctrl Pts',(-20.5199833626838,12.2212950286517,124.430776031763)) ;
#19384=CARTESIAN_POINT('Ctrl Pts',(-20.1436024751154,12.4112447815171,124.368597953825)) ;
#19385=CARTESIAN_POINT('Ctrl Pts',(-20.327174746647,12.2312557011542,124.607803018266)) ;
#19386=CARTESIAN_POINT('Ctrl Pts',(-19.9655160234336,12.4212828525849,124.481805478694)) ;
#19387=CARTESIAN_POINT('Ctrl Pts',(-20.1045650508631,12.241293772222,124.749310160051)) ;
#19388=CARTESIAN_POINT('Ctrl Pts',(-19.7737887271615,12.4311564675453,124.561434581507)) ;
#19389=CARTESIAN_POINT('Ctrl Pts',(-19.8649051459857,12.2511673871824,124.84884392232)) ;
#19390=CARTESIAN_POINT('Ctrl Pts',(-19.5671291833791,12.4412287021266,124.607402354197)) ;
#19391=CARTESIAN_POINT('Ctrl Pts',(-19.6065797304044,12.2612396217637,124.906300997495)) ;
#19392=CARTESIAN_POINT('Ctrl Pts',(-19.3607684693909,12.4510527205754,124.616796315158)) ;
#19393=CARTESIAN_POINT('Ctrl Pts',(-19.3486297183306,12.2710636402125,124.918040759663)) ;
#19394=CARTESIAN_POINT('Ctrl Pts',(-19.1509428265166,12.4611176415514,124.589849021404)) ;
#19395=CARTESIAN_POINT('Ctrl Pts',(-19.0863456687476,12.2811285611885,124.884353810211)) ;
#19396=CARTESIAN_POINT('Ctrl Pts',(-18.8857365452566,12.4743279398461,124.507174456424)) ;
#19397=CARTESIAN_POINT('Ctrl Pts',(-18.7548496615759,12.2943388594833,124.781008020348)) ;
#19398=CARTESIAN_POINT('Ctrl Pts',(-18.6462382926402,12.4876433865781,124.356312359537)) ;
#19399=CARTESIAN_POINT('Ctrl Pts',(-18.4555083325038,12.3076543062152,124.592460114452)) ;
#19400=CARTESIAN_POINT('Ctrl Pts',(-18.4564387488717,12.5009336318454,124.15121232202)) ;
#19401=CARTESIAN_POINT('Ctrl Pts',(-18.2182158984291,12.3209445514825,124.336043204847)) ;
#19402=CARTESIAN_POINT('Ctrl Pts',(-18.3421528810108,12.5109843814525,123.973529884011)) ;
#19403=CARTESIAN_POINT('Ctrl Pts',(-18.0753697674858,12.3309953010896,124.113946532571)) ;
#19404=CARTESIAN_POINT('Ctrl Pts',(-18.261991671417,12.5207969884347,123.783417454446)) ;
#19405=CARTESIAN_POINT('Ctrl Pts',(-17.9751686262583,12.3408079080718,123.876303265546)) ;
#19406=CARTESIAN_POINT('Ctrl Pts',(-18.2145854633708,12.530868086429,123.5770937702)) ;
#19407=CARTESIAN_POINT('Ctrl Pts',(-17.9159132713503,12.3508790060661,123.61839959421)) ;
#19408=CARTESIAN_POINT('Ctrl Pts',(-18.2041287449214,12.5407576592038,123.369434972959)) ;
#19409=CARTESIAN_POINT('Ctrl Pts',(-17.9028470180164,12.360768578841,123.358821518713)) ;
#19410=CARTESIAN_POINT('Ctrl Pts',(-18.2378495819674,12.5540277660071,123.092473664091)) ;
#19411=CARTESIAN_POINT('Ctrl Pts',(-17.9449900324593,12.3740386856443,123.012644489447)) ;
#19412=CARTESIAN_POINT('Ctrl Pts',(-18.3698646515677,12.5706444529296,122.764802678493)) ;
#19413=CARTESIAN_POINT('Ctrl Pts',(-18.1100382420715,12.3906553725668,122.603018959482)) ;
#19414=CARTESIAN_POINT('Ctrl Pts',(-18.6050396672439,12.5872184962459,122.502279793378)) ;
#19415=CARTESIAN_POINT('Ctrl Pts',(-18.403953809166,12.407229415883,122.274921978595)) ;
#19416=CARTESIAN_POINT('Ctrl Pts',(-18.8388843969827,12.6005150636777,122.349174786392)) ;
#19417=CARTESIAN_POINT('Ctrl Pts',(-18.6963080999561,12.4205259833148,122.083501484983)) ;
#19418=CARTESIAN_POINT('Ctrl Pts',(-19.032708382408,12.6105451272551,122.266104245232)) ;
#19419=CARTESIAN_POINT('Ctrl Pts',(-18.9385791929077,12.4305560468922,121.979673523522)) ;
#19420=CARTESIAN_POINT('Ctrl Pts',(-19.2351868358827,12.6204390191043,122.218590201878)) ;
#19421=CARTESIAN_POINT('Ctrl Pts',(-19.1916818709481,12.4404499387414,121.920281628208)) ;
#19422=CARTESIAN_POINT('Ctrl Pts',(-19.5133724231769,12.6336917748899,122.2020040059)) ;
#19423=CARTESIAN_POINT('Ctrl Pts',(-19.5394009792638,12.453702694527,121.899549493621)) ;
#19424=CARTESIAN_POINT('Ctrl Pts',(-19.8616244702295,12.6504198798823,122.274010765671)) ;
#19425=CARTESIAN_POINT('Ctrl Pts',(-19.9747293753154,12.4704307995194,121.989564308867)) ;
#19426=CARTESIAN_POINT('Ctrl Pts',(-20.2206924205023,12.6702507163608,122.495213042442)) ;
#19427=CARTESIAN_POINT('Ctrl Pts',(-20.423556659189,12.4902616359979,122.266069036656)) ;
#19428=CARTESIAN_POINT('Ctrl Pts',(-20.4846749217705,12.690176108251,122.826464817505)) ;
#19429=CARTESIAN_POINT('Ctrl Pts',(-20.7535327226879,12.5101870278881,122.680135635484)) ;
#19430=CARTESIAN_POINT('Ctrl Pts',(-20.6197750422256,12.710101321603,123.228081726851)) ;
#19431=CARTESIAN_POINT('Ctrl Pts',(-20.9224041261077,12.5301122412401,123.18215712058)) ;
#19432=CARTESIAN_POINT('Ctrl Pts',(-20.6098235900098,12.7300263350881,123.651575664266)) ;
#19433=CARTESIAN_POINT('Ctrl Pts',(-20.9099617273115,12.5500372547252,123.711523704258)) ;
#19434=CARTESIAN_POINT('Ctrl Pts',(-20.4568446708067,12.7499028067881,124.045572962216)) ;
#19435=CARTESIAN_POINT('Ctrl Pts',(-20.7187360422604,12.5699137264252,124.204018044716)) ;
#19436=CARTESIAN_POINT('Ctrl Pts',(-20.1773211945259,12.7698821246969,124.36546202135)) ;
#19437=CARTESIAN_POINT('Ctrl Pts',(-20.3693300643289,12.5898930443341,124.603877601687)) ;
#19438=CARTESIAN_POINT('Ctrl Pts',(-19.8060899945786,12.7898151282729,124.57002813045)) ;
#19439=CARTESIAN_POINT('Ctrl Pts',(-19.9052905888142,12.6098260479101,124.859582769263)) ;
#19440=CARTESIAN_POINT('Ctrl Pts',(-19.3882558614324,12.8097103983006,124.635945221289)) ;
#19441=CARTESIAN_POINT('Ctrl Pts',(-19.3829989743676,12.6297213179378,124.941977004567)) ;
#19442=CARTESIAN_POINT('Ctrl Pts',(-18.9723404365734,12.8296317362065,124.55563458962)) ;
#19443=CARTESIAN_POINT('Ctrl Pts',(-18.8631060156455,12.6496426558436,124.841587523865)) ;
#19444=CARTESIAN_POINT('Ctrl Pts',(-18.6081781423476,12.8495893594727,124.337737107174)) ;
#19445=CARTESIAN_POINT('Ctrl Pts',(-18.4079042835162,12.6696002791098,124.569214868981)) ;
#19446=CARTESIAN_POINT('Ctrl Pts',(-18.3412557610278,12.8694691914299,124.010060659351)) ;
#19447=CARTESIAN_POINT('Ctrl Pts',(-18.0742532724176,12.689480111067,124.15962015315)) ;
#19448=CARTESIAN_POINT('Ctrl Pts',(-18.2010112247405,12.8893510427268,123.611173077498)) ;
#19449=CARTESIAN_POINT('Ctrl Pts',(-17.8989480657597,12.7093619623639,123.661012507451)) ;
#19450=CARTESIAN_POINT('Ctrl Pts',(-18.2061520734863,12.9094220598306,123.184494838161)) ;
#19451=CARTESIAN_POINT('Ctrl Pts',(-17.9053743363839,12.7294329794677,123.127663535506)) ;
#19452=CARTESIAN_POINT('Ctrl Pts',(-18.3545914950356,12.9292292835837,122.790282514626)) ;
#19453=CARTESIAN_POINT('Ctrl Pts',(-18.0909224032866,12.7492402032208,122.634900991628)) ;
#19454=CARTESIAN_POINT('Ctrl Pts',(-18.6302173582225,12.9492104191524,122.467021464749)) ;
#19455=CARTESIAN_POINT('Ctrl Pts',(-18.4354537167374,12.7692213387896,122.230824135122)) ;
#19456=CARTESIAN_POINT('Ctrl Pts',(-18.9990267978771,12.9691379124917,122.258503177642)) ;
#19457=CARTESIAN_POINT('Ctrl Pts',(-18.8964641846084,12.7891488321288,121.970176160961)) ;
#19458=CARTESIAN_POINT('Ctrl Pts',(-19.414525111865,12.9889585738495,122.187284802443)) ;
#19459=CARTESIAN_POINT('Ctrl Pts',(-19.415834432645,12.8089694934866,121.881151656097)) ;
#19460=CARTESIAN_POINT('Ctrl Pts',(-19.8347816721657,13.0090557630713,122.26378936849)) ;
#19461=CARTESIAN_POINT('Ctrl Pts',(-19.9411566590933,12.8290666827084,121.976780870031)) ;
#19462=CARTESIAN_POINT('Ctrl Pts',(-20.1980367737812,13.0288194420796,122.475474924502)) ;
#19463=CARTESIAN_POINT('Ctrl Pts',(-20.3952240684518,12.8488303617167,122.241384544964)) ;
#19464=CARTESIAN_POINT('Ctrl Pts',(-20.47137453339,13.0488767207527,122.802591270838)) ;
#19465=CARTESIAN_POINT('Ctrl Pts',(-20.7368987004041,12.8688876403898,122.650278783027)) ;
#19466=CARTESIAN_POINT('Ctrl Pts',(-20.6146542104524,13.0686721445001,123.198479778478)) ;
#19467=CARTESIAN_POINT('Ctrl Pts',(-20.915999998585,12.8886830641372,123.145136393717)) ;
#19468=CARTESIAN_POINT('Ctrl Pts',(-20.6155493708649,13.0886357892277,123.622911309277)) ;
#19469=CARTESIAN_POINT('Ctrl Pts',(-20.9171224626081,12.9086467088648,123.675675466344)) ;
#19470=CARTESIAN_POINT('Ctrl Pts',(-20.4704208826885,13.1086192805018,124.022266658295)) ;
#19471=CARTESIAN_POINT('Ctrl Pts',(-20.7357148689362,12.9286302001389,124.174870580485)) ;
#19472=CARTESIAN_POINT('Ctrl Pts',(-20.2007675400314,13.1284267756511,124.345835412524)) ;
#19473=CARTESIAN_POINT('Ctrl Pts',(-20.3986521463145,12.9484376952882,124.579332558867)) ;
#19474=CARTESIAN_POINT('Ctrl Pts',(-19.834022972994,13.1484093663712,124.560193591737)) ;
#19475=CARTESIAN_POINT('Ctrl Pts',(-19.9402235763069,12.9684202860083,124.847283742868)) ;
#19476=CARTESIAN_POINT('Ctrl Pts',(-19.4180361300331,13.1682920203624,124.636116448361)) ;
#19477=CARTESIAN_POINT('Ctrl Pts',(-19.4202416053834,12.9883029399995,124.942191223807)) ;
#19478=CARTESIAN_POINT('Ctrl Pts',(-18.9996554886756,13.1882502652255,124.565604893307)) ;
#19479=CARTESIAN_POINT('Ctrl Pts',(-18.8972653738817,13.0082611848626,124.854056149815)) ;
#19480=CARTESIAN_POINT('Ctrl Pts',(-18.6317218676168,13.2081258522671,124.357573974673)) ;
#19481=CARTESIAN_POINT('Ctrl Pts',(-18.4373467193133,13.0281367719042,124.594021898923)) ;
#19482=CARTESIAN_POINT('Ctrl Pts',(-18.3552399068354,13.2281067404023,124.035038294504)) ;
#19483=CARTESIAN_POINT('Ctrl Pts',(-18.0917408140289,13.0481176600395,124.190855292359)) ;
#19484=CARTESIAN_POINT('Ctrl Pts',(-18.206044297576,13.2480418815133,123.638227388492)) ;
#19485=CARTESIAN_POINT('Ctrl Pts',(-17.9052414355018,13.0680528011505,123.694844185524)) ;
#19486=CARTESIAN_POINT('Ctrl Pts',(-18.2009152531286,13.2679538995244,123.214915566106)) ;
#19487=CARTESIAN_POINT('Ctrl Pts',(-17.8988271166947,13.0879648191615,123.165702838927)) ;
#19488=CARTESIAN_POINT('Ctrl Pts',(-18.3399734278226,13.287842117768,122.815536644445)) ;
#19489=CARTESIAN_POINT('Ctrl Pts',(-18.072637630343,13.1078530374051,122.666485551976)) ;
#19490=CARTESIAN_POINT('Ctrl Pts',(-18.5625167302271,13.3044404216149,122.541702141202)) ;
#19491=CARTESIAN_POINT('Ctrl Pts',(-18.3508356377982,13.124451341252,122.324166060085)) ;
#19492=CARTESIAN_POINT('Ctrl Pts',(-18.7884633242958,13.3177130115177,122.377888779236)) ;
#19493=CARTESIAN_POINT('Ctrl Pts',(-18.6332461345771,13.1377239311548,122.119417599801)) ;
#19494=CARTESIAN_POINT('Ctrl Pts',(-18.9775497688346,13.3277204264686,122.285661961006)) ;
#19495=CARTESIAN_POINT('Ctrl Pts',(-18.8696106143661,13.1477313461057,122.004127651261)) ;
#19496=CARTESIAN_POINT('Ctrl Pts',(-19.1798541137618,13.3377277732012,122.227841226343)) ;
#19497=CARTESIAN_POINT('Ctrl Pts',(-19.1224757065835,13.1577386928383,121.931849416177)) ;
#19498=CARTESIAN_POINT('Ctrl Pts',(-19.4571882805755,13.3509941330028,122.198742528533)) ;
#19499=CARTESIAN_POINT('Ctrl Pts',(-19.4692111889447,13.1710050526399,121.895476582139)) ;
#19500=CARTESIAN_POINT('Ctrl Pts',(-19.8041191619441,13.3675087906257,122.253086418136)) ;
#19501=CARTESIAN_POINT('Ctrl Pts',(-19.9027886653172,13.1875197102629,121.963391453896)) ;
#19502=CARTESIAN_POINT('Ctrl Pts',(-20.1135332813589,13.3841062238684,122.422657976203)) ;
#19503=CARTESIAN_POINT('Ctrl Pts',(-20.2896179416635,13.2041171435055,122.175375538865)) ;
#19504=CARTESIAN_POINT('Ctrl Pts',(-20.3161488488574,13.3974542210134,122.616898131359)) ;
#19505=CARTESIAN_POINT('Ctrl Pts',(-20.5428541366256,13.2174651406505,122.418153018463)) ;
#19506=CARTESIAN_POINT('Ctrl Pts',(-20.4392682471211,13.407349975365,122.78458790923)) ;
#19507=CARTESIAN_POINT('Ctrl Pts',(-20.6967627804406,13.2273608950021,122.62776755716)) ;
#19508=CARTESIAN_POINT('Ctrl Pts',(-20.5324892710804,13.4173379292963,122.972722988984)) ;
#19509=CARTESIAN_POINT('Ctrl Pts',(-20.8132896637095,13.2373488489335,122.862934128972)) ;
#19510=CARTESIAN_POINT('Ctrl Pts',(-20.5915443850433,13.4272951530011,123.173577963998)) ;
#19511=CARTESIAN_POINT('Ctrl Pts',(-20.887111769064,13.2473060726382,123.114002366625)) ;
#19512=CARTESIAN_POINT('Ctrl Pts',(-20.6149084211195,13.4373306995577,123.383244466026)) ;
#19513=CARTESIAN_POINT('Ctrl Pts',(-20.9163194697392,13.2573416191949,123.376085199788)) ;
#19514=CARTESIAN_POINT('Ctrl Pts',(-20.6018663431854,13.4472178108339,123.590706984687)) ;
#19515=CARTESIAN_POINT('Ctrl Pts',(-20.9000197111728,13.267228730471,123.635413520908)) ;
#19516=CARTESIAN_POINT('Ctrl Pts',(-20.5528158490788,13.4572092159347,123.794940084393)) ;
#19517=CARTESIAN_POINT('Ctrl Pts',(-20.8387093067046,13.2772201355718,123.890705618829)) ;
#19518=CARTESIAN_POINT('Ctrl Pts',(-20.4693700177335,13.4671548371495,123.986654821614)) ;
#19519=CARTESIAN_POINT('Ctrl Pts',(-20.7344045824693,13.2871657567866,124.130350209159)) ;
#19520=CARTESIAN_POINT('Ctrl Pts',(-20.3542090233936,13.4771040854178,124.161276470942)) ;
#19521=CARTESIAN_POINT('Ctrl Pts',(-20.5904556480587,13.2971150050549,124.348628887742)) ;
#19522=CARTESIAN_POINT('Ctrl Pts',(-20.2089077397589,13.4871505805864,124.314549867347)) ;
#19523=CARTESIAN_POINT('Ctrl Pts',(-20.4088310489179,13.3071615002235,124.540222615066)) ;
#19524=CARTESIAN_POINT('Ctrl Pts',(-20.0426037732206,13.4970019233779,124.438001198331)) ;
#19525=CARTESIAN_POINT('Ctrl Pts',(-20.2009526790891,13.3170128430151,124.69453910851)) ;
#19526=CARTESIAN_POINT('Ctrl Pts',(-19.8553954660048,13.5069737035053,124.532292944024)) ;
#19527=CARTESIAN_POINT('Ctrl Pts',(-19.9669434550335,13.3269846231424,124.812406349802)) ;
#19528=CARTESIAN_POINT('Ctrl Pts',(-19.6541253092378,13.516968903483,124.592783946963)) ;
#19529=CARTESIAN_POINT('Ctrl Pts',(-19.7153564891379,13.3369798231201,124.888022808457)) ;
#19530=CARTESIAN_POINT('Ctrl Pts',(-19.444620176713,13.527002895179,124.617242515377)) ;
#19531=CARTESIAN_POINT('Ctrl Pts',(-19.4534753611638,13.3470138148161,124.918598821052)) ;
#19532=CARTESIAN_POINT('Ctrl Pts',(-19.2377415370854,13.5368583001515,124.605497638602)) ;
#19533=CARTESIAN_POINT('Ctrl Pts',(-19.1948766730221,13.3568692197886,124.903920505576)) ;
#19534=CARTESIAN_POINT('Ctrl Pts',(-19.0330890851524,13.5468575979973,124.557608984223)) ;
#19535=CARTESIAN_POINT('Ctrl Pts',(-18.9390603846793,13.3668685176344,124.844062381727)) ;
#19536=CARTESIAN_POINT('Ctrl Pts',(-18.8417203854023,13.5567527106025,124.475953276878)) ;
#19537=CARTESIAN_POINT('Ctrl Pts',(-18.6998481883594,13.3767636302396,124.741995186928)) ;
#19538=CARTESIAN_POINT('Ctrl Pts',(-18.6645864621206,13.5668133561375,124.360423798942)) ;
#19539=CARTESIAN_POINT('Ctrl Pts',(-18.4784292945889,13.3868242757746,124.597585675323)) ;
#19540=CARTESIAN_POINT('Ctrl Pts',(-18.5133398637062,13.5766622331267,124.218993175225)) ;
#19541=CARTESIAN_POINT('Ctrl Pts',(-18.2893688821215,13.3966731527638,124.420799145494)) ;
#19542=CARTESIAN_POINT('Ctrl Pts',(-18.3862631485546,13.5866909442203,124.050762009217)) ;
#19543=CARTESIAN_POINT('Ctrl Pts',(-18.1305208053495,13.4067018638574,124.210511784196)) ;
#19544=CARTESIAN_POINT('Ctrl Pts',(-18.2908283109245,13.5967203454764,123.862742118593)) ;
#19545=CARTESIAN_POINT('Ctrl Pts',(-18.0112247910287,13.4167312651135,123.975488167396)) ;
#19546=CARTESIAN_POINT('Ctrl Pts',(-18.2302062670491,13.6065605372724,123.664948493123)) ;
#19547=CARTESIAN_POINT('Ctrl Pts',(-17.9354445009214,13.4265714569095,123.72824647118)) ;
#19548=CARTESIAN_POINT('Ctrl Pts',(-18.2040444170886,13.6165639664654,123.456299673931)) ;
#19549=CARTESIAN_POINT('Ctrl Pts',(-17.9027395319079,13.4365748861025,123.467435684465)) ;
#19550=CARTESIAN_POINT('Ctrl Pts',(-18.2145600866286,13.6265494789316,123.246600447077)) ;
#19551=CARTESIAN_POINT('Ctrl Pts',(-17.9158814573718,13.4465603985687,123.205311390375)) ;
#19552=CARTESIAN_POINT('Ctrl Pts',(-18.2617823017495,13.6365905753156,123.040875922897)) ;
#19553=CARTESIAN_POINT('Ctrl Pts',(-17.9749065837832,13.4566014949527,122.948155155583)) ;
#19554=CARTESIAN_POINT('Ctrl Pts',(-18.3421364497269,13.6464337712666,122.850159429394)) ;
#19555=CARTESIAN_POINT('Ctrl Pts',(-18.0753470360815,13.4664446909037,122.709757985454)) ;
#19556=CARTESIAN_POINT('Ctrl Pts',(-18.4556351281271,13.656420082321,122.67358245955)) ;
#19557=CARTESIAN_POINT('Ctrl Pts',(-18.217218281521,13.4764310019581,122.489035231126)) ;
#19558=CARTESIAN_POINT('Ctrl Pts',(-18.5972804388859,13.6663547675787,122.520040996224)) ;
#19559=CARTESIAN_POINT('Ctrl Pts',(-18.3942732512551,13.4863656872158,122.297106419642)) ;
#19560=CARTESIAN_POINT('Ctrl Pts',(-18.7655457253041,13.6764123287957,122.392050964971)) ;
#19561=CARTESIAN_POINT('Ctrl Pts',(-18.6046031877743,13.4964232484328,122.137116873894)) ;
#19562=CARTESIAN_POINT('Ctrl Pts',(-18.948971596639,13.6862339704043,122.297188134367)) ;
#19563=CARTESIAN_POINT('Ctrl Pts',(-18.8338850495127,13.5062448900414,122.018535713195)) ;
#19564=CARTESIAN_POINT('Ctrl Pts',(-19.150630895694,13.6962900339953,122.233780317479)) ;
#19565=CARTESIAN_POINT('Ctrl Pts',(-19.0859583258846,13.5163009536324,121.939273611562)) ;
#19566=CARTESIAN_POINT('Ctrl Pts',(-19.3579055678042,13.7062307097571,122.207035465086)) ;
#19567=CARTESIAN_POINT('Ctrl Pts',(-19.3450516698222,13.5262416293942,121.905839973782)) ;
#19568=CARTESIAN_POINT('Ctrl Pts',(-19.5659365047634,13.7161350685454,122.215998316577)) ;
#19569=CARTESIAN_POINT('Ctrl Pts',(-19.6050909750196,13.5361459881825,121.917041144644)) ;
#19570=CARTESIAN_POINT('Ctrl Pts',(-19.7721240618805,13.7261817231212,122.26171766678)) ;
#19571=CARTESIAN_POINT('Ctrl Pts',(-19.862825851585,13.5461926427583,121.97418792217)) ;
#19572=CARTESIAN_POINT('Ctrl Pts',(-19.9644220298839,13.7360773177641,122.341175721282)) ;
#19573=CARTESIAN_POINT('Ctrl Pts',(-20.1031997643857,13.5560882374012,122.073508487898)) ;
#19574=CARTESIAN_POINT('Ctrl Pts',(-20.1429187786372,13.7461392644209,122.454645564807)) ;
#19575=CARTESIAN_POINT('Ctrl Pts',(-20.3263218440362,13.5661501840581,122.215343672236)) ;
#19576=CARTESIAN_POINT('Ctrl Pts',(-20.2957594945872,13.7559888883531,122.594367289572)) ;
#19577=CARTESIAN_POINT('Ctrl Pts',(-20.5173749645332,13.5759998079902,122.38999462014)) ;
#19578=CARTESIAN_POINT('Ctrl Pts',(-20.4240087228008,13.7659521273829,122.75995684231)) ;
#19579=CARTESIAN_POINT('Ctrl Pts',(-20.6776884554839,13.5859630470201,122.596980439567)) ;
#19580=CARTESIAN_POINT('Ctrl Pts',(-20.5219126757159,13.7759767021588,122.946597688754)) ;
#19581=CARTESIAN_POINT('Ctrl Pts',(-20.8000704181908,13.5959876217959,122.830280403309)) ;
#19582=CARTESIAN_POINT('Ctrl Pts',(-20.5853680857787,13.7858952648465,123.145221491814)) ;
#19583=CARTESIAN_POINT('Ctrl Pts',(-20.8793920083737,13.6059061844836,123.07855998187)) ;
#19584=CARTESIAN_POINT('Ctrl Pts',(-20.6139486861192,13.7958874515705,123.353347867714)) ;
#19585=CARTESIAN_POINT('Ctrl Pts',(-20.9151199375489,13.6158983712076,123.338717822216)) ;
#19586=CARTESIAN_POINT('Ctrl Pts',(-20.6055443985715,13.8059222501547,123.564135174219)) ;
#19587=CARTESIAN_POINT('Ctrl Pts',(-20.9046168525977,13.6259331697918,123.6022019633)) ;
#19588=CARTESIAN_POINT('Ctrl Pts',(-20.5618138969041,13.8157774408283,123.766670893346)) ;
#19589=CARTESIAN_POINT('Ctrl Pts',(-20.8499556627768,13.6357883604655,123.855372966742)) ;
#19590=CARTESIAN_POINT('Ctrl Pts',(-20.4827162908005,13.8257767889813,123.961402445332)) ;
#19591=CARTESIAN_POINT('Ctrl Pts',(-20.7510855573927,13.6457877086185,124.098788324435)) ;
#19592=CARTESIAN_POINT('Ctrl Pts',(-20.3723265103831,13.8356719146565,124.137764210175)) ;
#19593=CARTESIAN_POINT('Ctrl Pts',(-20.6130996723433,13.6556828342936,124.319242233489)) ;
#19594=CARTESIAN_POINT('Ctrl Pts',(-20.2306869988819,13.8457324576046,124.294801970209)) ;
#19595=CARTESIAN_POINT('Ctrl Pts',(-20.4360519660016,13.6657433772417,124.515540628893)) ;
#19596=CARTESIAN_POINT('Ctrl Pts',(-20.0674724058813,13.8555817318715,124.422248257044)) ;
#19597=CARTESIAN_POINT('Ctrl Pts',(-20.2320341456861,13.6755926515086,124.674850714962)) ;
#19598=CARTESIAN_POINT('Ctrl Pts',(-19.8815742262112,13.8656089564414,124.521635316517)) ;
#19599=CARTESIAN_POINT('Ctrl Pts',(-19.9996623311131,13.6856198760785,124.799086161189)) ;
#19600=CARTESIAN_POINT('Ctrl Pts',(-19.6810321497663,13.8756373556292,124.586723666077)) ;
#19601=CARTESIAN_POINT('Ctrl Pts',(-19.7489854254844,13.6956482752663,124.880448501815)) ;
#19602=CARTESIAN_POINT('Ctrl Pts',(-19.4761166290859,13.8854831060427,124.615846164903)) ;
#19603=CARTESIAN_POINT('Ctrl Pts',(-19.4928401900497,13.7054940256798,124.916853671087)) ;
#19604=CARTESIAN_POINT('Ctrl Pts',(-19.2662085926654,13.8954718964434,124.609433443135)) ;
#19605=CARTESIAN_POINT('Ctrl Pts',(-19.230454887784,13.7154828160805,124.908839488335)) ;
#19606=CARTESIAN_POINT('Ctrl Pts',(-19.0595750845739,13.9055168248431,124.565911416118)) ;
#19607=CARTESIAN_POINT('Ctrl Pts',(-18.9721627761797,13.7255277444802,124.854438840815)) ;
#19608=CARTESIAN_POINT('Ctrl Pts',(-18.8677390185657,13.9153413096321,124.489339185228)) ;
#19609=CARTESIAN_POINT('Ctrl Pts',(-18.7323658376547,13.7353522292692,124.758724681303)) ;
#19610=CARTESIAN_POINT('Ctrl Pts',(-18.6878125716597,13.9253987071733,124.378319657156)) ;
#19611=CARTESIAN_POINT('Ctrl Pts',(-18.507457139982,13.7454096268104,124.619951807237)) ;
#19612=CARTESIAN_POINT('Ctrl Pts',(-18.5321161135312,13.9353247987595,124.239354765055)) ;
#19613=CARTESIAN_POINT('Ctrl Pts',(-18.3128349524813,13.7553357183966,124.44624656969)) ;
#19614=CARTESIAN_POINT('Ctrl Pts',(-18.4021255349772,13.945279583904,124.075342585797)) ;
#19615=CARTESIAN_POINT('Ctrl Pts',(-18.1503452309715,13.7652905035412,124.241231958245)) ;
#19616=CARTESIAN_POINT('Ctrl Pts',(-18.3019676622171,13.9553169535617,123.889610890228)) ;
#19617=CARTESIAN_POINT('Ctrl Pts',(-18.0251465109341,13.7753278731988,124.009068223143)) ;
#19618=CARTESIAN_POINT('Ctrl Pts',(-18.2364086645203,13.9652057636833,123.692318961985)) ;
#19619=CARTESIAN_POINT('Ctrl Pts',(-17.9431959784106,13.7852166833204,123.762452941019)) ;
#19620=CARTESIAN_POINT('Ctrl Pts',(-18.2054221774035,13.9751951227343,123.484614442852)) ;
#19621=CARTESIAN_POINT('Ctrl Pts',(-17.9044614031139,13.7952060423715,123.502822293364)) ;
#19622=CARTESIAN_POINT('Ctrl Pts',(-18.2111097202979,13.9851536701904,123.275338157667)) ;
#19623=CARTESIAN_POINT('Ctrl Pts',(-17.9115693386521,13.8051645898276,123.241226463732)) ;
#19624=CARTESIAN_POINT('Ctrl Pts',(-18.2523005245241,13.9950532467415,123.071321965387)) ;
#19625=CARTESIAN_POINT('Ctrl Pts',(-17.9630567197968,13.8150641663786,122.986205100608)) ;
#19626=CARTESIAN_POINT('Ctrl Pts',(-18.3294851382835,14.0051011585722,122.874712691268)) ;
#19627=CARTESIAN_POINT('Ctrl Pts',(-18.0595361492998,13.8251120782093,122.740443216478)) ;
#19628=CARTESIAN_POINT('Ctrl Pts',(-18.4378511245041,14.0149965064327,122.697097031468)) ;
#19629=CARTESIAN_POINT('Ctrl Pts',(-18.1949930036132,13.8350074260699,122.518422190268)) ;
#19630=CARTESIAN_POINT('Ctrl Pts',(-18.5776635026499,14.0250581829639,122.538393890947)) ;
#19631=CARTESIAN_POINT('Ctrl Pts',(-18.3697572977927,13.845069102601,122.320042659935)) ;
#19632=CARTESIAN_POINT('Ctrl Pts',(-18.7393445312316,14.0349027007131,122.409181627727)) ;
#19633=CARTESIAN_POINT('Ctrl Pts',(-18.5718588198519,13.8549136203502,122.158525512922)) ;
#19634=CARTESIAN_POINT('Ctrl Pts',(-18.9227751263348,14.0448631444279,122.308189876658)) ;
#19635=CARTESIAN_POINT('Ctrl Pts',(-18.8011469810602,13.864874064065,122.032284729829)) ;
#19636=CARTESIAN_POINT('Ctrl Pts',(-19.1226020522299,14.0548999772461,122.240434925921)) ;
#19637=CARTESIAN_POINT('Ctrl Pts',(-19.0509301231226,13.8749108968832,121.947590007007)) ;
#19638=CARTESIAN_POINT('Ctrl Pts',(-19.3278464181783,14.0647787739929,122.208569582796)) ;
#19639=CARTESIAN_POINT('Ctrl Pts',(-19.3074865101994,13.88478969363,121.907757156992)) ;
#19640=CARTESIAN_POINT('Ctrl Pts',(-19.5392604494556,14.0748380901212,122.212835075085)) ;
#19641=CARTESIAN_POINT('Ctrl Pts',(-19.5717537455678,13.8948490097584,121.91308802529)) ;
#19642=CARTESIAN_POINT('Ctrl Pts',(-19.7428603551298,14.0847085368744,122.252978784912)) ;
#19643=CARTESIAN_POINT('Ctrl Pts',(-19.8262549511952,13.9047194565116,121.963266910915)) ;
#19644=CARTESIAN_POINT('Ctrl Pts',(-19.9389874347738,14.0947011751325,122.328256871601)) ;
#19645=CARTESIAN_POINT('Ctrl Pts',(-20.0714142577279,13.9147120947696,122.057363864517)) ;
#19646=CARTESIAN_POINT('Ctrl Pts',(-20.1195329190691,14.1047331906804,122.437257388524)) ;
#19647=CARTESIAN_POINT('Ctrl Pts',(-20.2970965036502,13.9247441103175,122.193613633218)) ;
#19648=CARTESIAN_POINT('Ctrl Pts',(-20.2760952863307,14.114599046987,122.573331296322)) ;
#19649=CARTESIAN_POINT('Ctrl Pts',(-20.4928009018349,13.9346099666241,122.363706237578)) ;
#19650=CARTESIAN_POINT('Ctrl Pts',(-20.4093323895338,14.1246683364561,122.737799807902)) ;
#19651=CARTESIAN_POINT('Ctrl Pts',(-20.6593476164435,13.9446792560932,122.569291069351)) ;
#19652=CARTESIAN_POINT('Ctrl Pts',(-20.5097252080318,14.1345118940074,122.918773104725)) ;
#19653=CARTESIAN_POINT('Ctrl Pts',(-20.7848399902421,13.9545228136445,122.795508554596)) ;
#19654=CARTESIAN_POINT('Ctrl Pts',(-20.5787488120301,14.1444920207952,123.116900923629)) ;
#19655=CARTESIAN_POINT('Ctrl Pts',(-20.871120064522,13.9645029404324,123.043168459414)) ;
#19656=CARTESIAN_POINT('Ctrl Pts',(-20.6120524726319,14.1545105693952,123.324867150909)) ;
#19657=CARTESIAN_POINT('Ctrl Pts',(-20.9127502836893,13.9745214890323,123.303126129535)) ;
#19658=CARTESIAN_POINT('Ctrl Pts',(-20.6092267809851,14.1643938699184,123.532651027033)) ;
#19659=CARTESIAN_POINT('Ctrl Pts',(-20.9092186327094,13.9844047895555,123.562857078074)) ;
#19660=CARTESIAN_POINT('Ctrl Pts',(-20.5695586363973,14.1744621569665,123.740532636129)) ;
#19661=CARTESIAN_POINT('Ctrl Pts',(-20.8596340362664,13.9944730766036,123.822708783211)) ;
#19662=CARTESIAN_POINT('Ctrl Pts',(-20.4963791598284,14.1842922799851,123.933839607261)) ;
#19663=CARTESIAN_POINT('Ctrl Pts',(-20.7681595371697,14.0043031996223,124.064344085627)) ;
#19664=CARTESIAN_POINT('Ctrl Pts',(-20.3884763220446,14.1943588639105,124.115856989045)) ;
#19665=CARTESIAN_POINT('Ctrl Pts',(-20.6332814623007,14.0143697835476,124.291865630646)) ;
#19666=CARTESIAN_POINT('Ctrl Pts',(-20.2528909010088,14.2042489769249,124.273525084078)) ;
#19667=CARTESIAN_POINT('Ctrl Pts',(-20.4637992773007,14.0242598965621,124.488951781943)) ;
#19668=CARTESIAN_POINT('Ctrl Pts',(-20.0906371997248,14.2142416656876,124.406937747112)) ;
#19669=CARTESIAN_POINT('Ctrl Pts',(-20.2609821100153,14.0342525853247,124.655717889191)) ;
#19670=CARTESIAN_POINT('Ctrl Pts',(-19.9081695184652,14.2242025540433,124.509708404688)) ;
#19671=CARTESIAN_POINT('Ctrl Pts',(-20.0328972096088,14.0442134736805,124.784181661414)) ;
#19672=CARTESIAN_POINT('Ctrl Pts',(-19.7116219047513,14.2341204989233,124.579266374256)) ;
#19673=CARTESIAN_POINT('Ctrl Pts',(-19.7872119388903,14.0541314185605,124.87112949854)) ;
#19674=CARTESIAN_POINT('Ctrl Pts',(-19.5041267455453,14.2441282520195,124.61419846985)) ;
#19675=CARTESIAN_POINT('Ctrl Pts',(-19.527842932523,14.0641391716567,124.914794637581)) ;
#19676=CARTESIAN_POINT('Ctrl Pts',(-19.2932629141695,14.2541593459786,124.612140808349)) ;
#19677=CARTESIAN_POINT('Ctrl Pts',(-19.2642632651857,14.0741702656157,124.912222739613)) ;
#19678=CARTESIAN_POINT('Ctrl Pts',(-19.0896342106667,14.2640073140066,124.57465995118)) ;
#19679=CARTESIAN_POINT('Ctrl Pts',(-19.0097259981526,14.0840182336437,124.865371406458)) ;
#19680=CARTESIAN_POINT('Ctrl Pts',(-18.8913548972053,14.2740692701324,124.501004306892)) ;
#19681=CARTESIAN_POINT('Ctrl Pts',(-18.7618772164016,14.0940801897696,124.773301901415)) ;
#19682=CARTESIAN_POINT('Ctrl Pts',(-18.7119419266118,14.2839664817336,124.395611023166)) ;
#19683=CARTESIAN_POINT('Ctrl Pts',(-18.5376101429091,14.1039774013707,124.641559789166)) ;
#19684=CARTESIAN_POINT('Ctrl Pts',(-18.5525741212308,14.2938976483982,124.260736428545)) ;
#19685=CARTESIAN_POINT('Ctrl Pts',(-18.3384000135968,14.1139085680353,124.472965869001)) ;
#19686=CARTESIAN_POINT('Ctrl Pts',(-18.4177287010278,14.3039398326024,124.098297375406)) ;
#19687=CARTESIAN_POINT('Ctrl Pts',(-18.169843513441,14.1239507522395,124.269917095288)) ;
#19688=CARTESIAN_POINT('Ctrl Pts',(-18.3146195122506,14.3138265008555,123.917815954086)) ;
#19689=CARTESIAN_POINT('Ctrl Pts',(-18.0409566998773,14.1338374204927,124.044314253981)) ;
#19690=CARTESIAN_POINT('Ctrl Pts',(-18.2433338154398,14.3238196128338,123.720204704618)) ;
#19691=CARTESIAN_POINT('Ctrl Pts',(-17.9518498698231,14.1438305324709,123.797299870393)) ;
#19692=CARTESIAN_POINT('Ctrl Pts',(-18.2076886193533,14.3337652904496,123.514175880864)) ;
#19693=CARTESIAN_POINT('Ctrl Pts',(-17.9072936184703,14.1537762100867,123.539763194409)) ;
#19694=CARTESIAN_POINT('Ctrl Pts',(-18.2079318857893,14.3437125934346,123.305042620039)) ;
#19695=CARTESIAN_POINT('Ctrl Pts',(-17.9075982211722,14.1637235130717,123.278346044345)) ;
#19696=CARTESIAN_POINT('Ctrl Pts',(-18.2450800860336,14.3537603171813,123.09710524755)) ;
#19697=CARTESIAN_POINT('Ctrl Pts',(-17.9540338467725,14.1737712368185,123.018424649771)) ;
#19698=CARTESIAN_POINT('Ctrl Pts',(-18.3161751561514,14.3636086909439,122.902654315691)) ;
#19699=CARTESIAN_POINT('Ctrl Pts',(-18.0429036250617,14.183619610581,122.775359841272)) ;
#19700=CARTESIAN_POINT('Ctrl Pts',(-18.420516020689,14.3735676633896,122.72113759086)) ;
#19701=CARTESIAN_POINT('Ctrl Pts',(-18.1733306008267,14.1935785830267,122.54846390798)) ;
#19702=CARTESIAN_POINT('Ctrl Pts',(-18.5561553946168,14.3836065252707,122.559457330409)) ;
#19703=CARTESIAN_POINT('Ctrl Pts',(-18.3428801887918,14.2036174449079,122.346364098552)) ;
#19704=CARTESIAN_POINT('Ctrl Pts',(-18.7150352575607,14.3934851294425,122.425678518084)) ;
#19705=CARTESIAN_POINT('Ctrl Pts',(-18.5414813532127,14.2134960490797,122.179140432255)) ;
#19706=CARTESIAN_POINT('Ctrl Pts',(-18.8977873014348,14.4035366706458,122.319642116266)) ;
#19707=CARTESIAN_POINT('Ctrl Pts',(-18.7699215575239,14.223547590283,122.046595739492)) ;
#19708=CARTESIAN_POINT('Ctrl Pts',(-19.0931303673642,14.4134320686262,122.247993391467)) ;
#19709=CARTESIAN_POINT('Ctrl Pts',(-19.0141015690712,14.2334429882633,121.957035255779)) ;
#19710=CARTESIAN_POINT('Ctrl Pts',(-19.3010884804579,14.4234833011715,122.21067275502)) ;
#19711=CARTESIAN_POINT('Ctrl Pts',(-19.2740491001981,14.2434942208086,121.910385335695)) ;
#19712=CARTESIAN_POINT('Ctrl Pts',(-19.5089481133767,14.4333694917958,122.210014197756)) ;
#19713=CARTESIAN_POINT('Ctrl Pts',(-19.5338747027506,14.2533804114329,121.909562985904)) ;
#19714=CARTESIAN_POINT('Ctrl Pts',(-19.7159932801428,14.4433620311115,122.245450565557)) ;
#19715=CARTESIAN_POINT('Ctrl Pts',(-19.7926811889532,14.2633729507487,121.953859464746)) ;
#19716=CARTESIAN_POINT('Ctrl Pts',(-19.9128752055225,14.4533104770063,122.316060788436)) ;
#19717=CARTESIAN_POINT('Ctrl Pts',(-20.0387837794866,14.2733213966434,122.042123340413)) ;
#19718=CARTESIAN_POINT('Ctrl Pts',(-20.0944137100652,14.4632472795382,122.419388130175)) ;
#19719=CARTESIAN_POINT('Ctrl Pts',(-20.2657069288235,14.2832581991753,122.171283774759)) ;
#19720=CARTESIAN_POINT('Ctrl Pts',(-20.2562053966534,14.4732302869895,122.553111371439)) ;
#19721=CARTESIAN_POINT('Ctrl Pts',(-20.4679459835233,14.2932412066266,122.338438899069)) ;
#19722=CARTESIAN_POINT('Ctrl Pts',(-20.3928213225405,14.4832741284043,122.714082144546)) ;
#19723=CARTESIAN_POINT('Ctrl Pts',(-20.6387149774407,14.3032850480414,122.539652891498)) ;
#19724=CARTESIAN_POINT('Ctrl Pts',(-20.4975727490238,14.4931023270282,122.892216003962)) ;
#19725=CARTESIAN_POINT('Ctrl Pts',(-20.7696539436816,14.3131132466653,122.762322078436)) ;
#19726=CARTESIAN_POINT('Ctrl Pts',(-20.5716961928806,14.5031789204704,123.09062015157)) ;
#19727=CARTESIAN_POINT('Ctrl Pts',(-20.8623069213888,14.3231898401075,123.010327296333)) ;
#19728=CARTESIAN_POINT('Ctrl Pts',(-20.6095053348988,14.513030919812,123.29430613063)) ;
#19729=CARTESIAN_POINT('Ctrl Pts',(-20.909567306365,14.3330418394491,123.264936220785)) ;
#19730=CARTESIAN_POINT('Ctrl Pts',(-20.6115890759441,14.5231045066358,123.506038201766)) ;
#19731=CARTESIAN_POINT('Ctrl Pts',(-20.9121706248892,14.343115426273,123.529600919858)) ;
#19732=CARTESIAN_POINT('Ctrl Pts',(-20.5776337189286,14.5329447317333,123.710123522401)) ;
#19733=CARTESIAN_POINT('Ctrl Pts',(-20.8697248958235,14.3529556513705,123.784708643342)) ;
#19734=CARTESIAN_POINT('Ctrl Pts',(-20.5085876603415,14.542910435762,123.907911470471)) ;
#19735=CARTESIAN_POINT('Ctrl Pts',(-20.7834156858806,14.3629213553991,124.031943418832)) ;
#19736=CARTESIAN_POINT('Ctrl Pts',(-20.4053409396209,14.5529370690686,124.091700513601)) ;
#19737=CARTESIAN_POINT('Ctrl Pts',(-20.6543560175008,14.3729479887057,124.26167893838)) ;
#19738=CARTESIAN_POINT('Ctrl Pts',(-20.2733679541214,14.5628513647804,124.253019570529)) ;
#19739=CARTESIAN_POINT('Ctrl Pts',(-20.4893881315526,14.3828622844175,124.463327357308)) ;
#19740=CARTESIAN_POINT('Ctrl Pts',(-20.1144447570708,14.5728396534728,124.390287718717)) ;
#19741=CARTESIAN_POINT('Ctrl Pts',(-20.29073289972,14.39285057311,124.634911409917)) ;
#19742=CARTESIAN_POINT('Ctrl Pts',(-19.93300982332,14.5828783866312,124.498080446046)) ;
#19743=CARTESIAN_POINT('Ctrl Pts',(-20.0639385669575,14.4028893062683,124.769650931547)) ;
#19744=CARTESIAN_POINT('Ctrl Pts',(-19.739575472665,14.5927217184587,124.571609128069)) ;
#19745=CARTESIAN_POINT('Ctrl Pts',(-19.8221438934761,14.4127326380959,124.861560677325)) ;
#19746=CARTESIAN_POINT('Ctrl Pts',(-19.5325945345893,14.6027494443383,124.611640004367)) ;
#19747=CARTESIAN_POINT('Ctrl Pts',(-19.5634174500474,14.4227603639755,124.911597480083)) ;
#19748=CARTESIAN_POINT('Ctrl Pts',(-19.3216956220107,14.6127817807269,124.614552263941)) ;
#19749=CARTESIAN_POINT('Ctrl Pts',(-19.2997938732283,14.432792700364,124.915236180486)) ;
#19750=CARTESIAN_POINT('Ctrl Pts',(-19.1176575039999,14.6226112810275,124.581899390616)) ;
#19751=CARTESIAN_POINT('Ctrl Pts',(-19.0447452472327,14.4426222006646,124.874418148553)) ;
#19752=CARTESIAN_POINT('Ctrl Pts',(-18.9189866148987,14.6326007849443,124.513805611947)) ;
#19753=CARTESIAN_POINT('Ctrl Pts',(-18.796407103076,14.4526117045814,124.789299015739)) ;
#19754=CARTESIAN_POINT('Ctrl Pts',(-18.7344236623876,14.6426446254567,124.411231786097)) ;
#19755=CARTESIAN_POINT('Ctrl Pts',(-18.5657044122553,14.4626555450938,124.661080239922)) ;
#19756=CARTESIAN_POINT('Ctrl Pts',(-18.5738301995033,14.6524663312247,124.281444401144)) ;
#19757=CARTESIAN_POINT('Ctrl Pts',(-18.3649628204512,14.4724772508619,124.498843726449)) ;
#19758=CARTESIAN_POINT('Ctrl Pts',(-18.4348762560386,14.6625013783571,124.122702247143)) ;
#19759=CARTESIAN_POINT('Ctrl Pts',(-18.1912720235427,14.4825122979942,124.300414746533)) ;
#19760=CARTESIAN_POINT('Ctrl Pts',(-18.3262031256769,14.672526055794,123.942122520734)) ;
#19761=CARTESIAN_POINT('Ctrl Pts',(-18.055432254409,14.4925369754311,124.074689127998)) ;
#19762=CARTESIAN_POINT('Ctrl Pts',(-18.2514273159942,14.6823788706484,123.748954040769)) ;
#19763=CARTESIAN_POINT('Ctrl Pts',(-17.9619640242889,14.5023897902856,123.833226852752)) ;
#19764=CARTESIAN_POINT('Ctrl Pts',(-18.2104197904952,14.692366580256,123.543040108188)) ;
#19765=CARTESIAN_POINT('Ctrl Pts',(-17.9107066774369,14.5123774998931,123.575833839664)) ;
#19766=CARTESIAN_POINT('Ctrl Pts',(-18.2058049225117,14.7022965902501,123.334323737137)) ;
#19767=CARTESIAN_POINT('Ctrl Pts',(-17.9049402191342,14.5223075098872,123.314937805648)) ;
#19768=CARTESIAN_POINT('Ctrl Pts',(-18.2373702335,14.7122863454692,123.126689249675)) ;
#19769=CARTESIAN_POINT('Ctrl Pts',(-17.9443990827381,14.5322972651064,123.055394867544)) ;
#19770=CARTESIAN_POINT('Ctrl Pts',(-18.3050137193924,14.7223129541521,122.927042802694)) ;
#19771=CARTESIAN_POINT('Ctrl Pts',(-18.0289554645481,14.5423238737893,122.80583753216)) ;
#19772=CARTESIAN_POINT('Ctrl Pts',(-18.4046749189677,14.732196894174,122.744715504703)) ;
#19773=CARTESIAN_POINT('Ctrl Pts',(-18.1535342537274,14.5522078138111,122.577928818094)) ;
#19774=CARTESIAN_POINT('Ctrl Pts',(-18.5354880156566,14.7421861217125,122.580419937995)) ;
#19775=CARTESIAN_POINT('Ctrl Pts',(-18.3170525414426,14.5621970413496,122.372560685954)) ;
#19776=CARTESIAN_POINT('Ctrl Pts',(-18.6939694465223,14.7522289922362,122.44092045882)) ;
#19777=CARTESIAN_POINT('Ctrl Pts',(-18.5151557257719,14.5722399118733,122.198188061704)) ;
#19778=CARTESIAN_POINT('Ctrl Pts',(-18.8703137137284,14.7620613789916,122.333079749863)) ;
#19779=CARTESIAN_POINT('Ctrl Pts',(-18.7355880780577,14.5820722986287,122.063388638443)) ;
#19780=CARTESIAN_POINT('Ctrl Pts',(-19.0656282841589,14.7720546721632,122.255693489157)) ;
#19781=CARTESIAN_POINT('Ctrl Pts',(-18.9797323076057,14.5920655918003,121.966658037112)) ;
#19782=CARTESIAN_POINT('Ctrl Pts',(-19.2723122403626,14.7820866778116,122.213661473494)) ;
#19783=CARTESIAN_POINT('Ctrl Pts',(-19.2380876823601,14.6020975974487,121.914120317295)) ;
#19784=CARTESIAN_POINT('Ctrl Pts',(-19.4796224788741,14.7919519337806,122.207990741201)) ;
#19785=CARTESIAN_POINT('Ctrl Pts',(-19.4972262784199,14.6119628534177,121.907034280981)) ;
#19786=CARTESIAN_POINT('Ctrl Pts',(-19.686880956539,14.8019138136881,122.238115152982)) ;
#19787=CARTESIAN_POINT('Ctrl Pts',(-19.7562992627137,14.6219247333252,121.944692330567)) ;
#19788=CARTESIAN_POINT('Ctrl Pts',(-19.8870940592205,14.81194874705,122.304572113576)) ;
#19789=CARTESIAN_POINT('Ctrl Pts',(-20.0065648350329,14.6319596666871,122.027765848265)) ;
#19790=CARTESIAN_POINT('Ctrl Pts',(-20.0701544259768,14.8218337054293,122.402996415654)) ;
#19791=CARTESIAN_POINT('Ctrl Pts',(-20.2353895991265,14.6418446250664,122.150798715635)) ;
#19792=CARTESIAN_POINT('Ctrl Pts',(-20.2362472111695,14.8318993323519,122.534060407699)) ;
#19793=CARTESIAN_POINT('Ctrl Pts',(-20.4430039039663,14.6519102519891,122.314630587451)) ;
#19794=CARTESIAN_POINT('Ctrl Pts',(-20.3740932209751,14.8417384380163,122.688329422969)) ;
#19795=CARTESIAN_POINT('Ctrl Pts',(-20.6153099874822,14.6617493576534,122.507469086936)) ;
#19796=CARTESIAN_POINT('Ctrl Pts',(-20.4857432775784,14.8518012530216,122.867986014556)) ;
#19797=CARTESIAN_POINT('Ctrl Pts',(-20.7548702754188,14.6718121726588,122.732041086105)) ;
#19798=CARTESIAN_POINT('Ctrl Pts',(-20.5630404308717,14.8616974590703,123.061166562861)) ;
#19799=CARTESIAN_POINT('Ctrl Pts',(-20.8514895076296,14.6817083787074,122.973518167656)) ;
#19800=CARTESIAN_POINT('Ctrl Pts',(-20.6063727048954,14.8716382820956,123.265587679795)) ;
#19801=CARTESIAN_POINT('Ctrl Pts',(-20.905652298732,14.6916492017327,123.229045388477)) ;
#19802=CARTESIAN_POINT('Ctrl Pts',(-20.6136516344617,14.8816428650742,123.47581329813)) ;
#19803=CARTESIAN_POINT('Ctrl Pts',(-20.9147482972179,14.7016537847114,123.49182757385)) ;
#19804=CARTESIAN_POINT('Ctrl Pts',(-20.5840199308421,14.891663759519,123.684384900853)) ;
#19805=CARTESIAN_POINT('Ctrl Pts',(-20.8777060565819,14.7116746791561,123.752541737872)) ;
#19806=CARTESIAN_POINT('Ctrl Pts',(-20.5197082244626,14.9015556801084,123.882155751433)) ;
#19807=CARTESIAN_POINT('Ctrl Pts',(-20.7973137583484,14.7215665997455,123.999754867603)) ;
#19808=CARTESIAN_POINT('Ctrl Pts',(-20.4213024996246,14.9115491124538,124.067769431274)) ;
#19809=CARTESIAN_POINT('Ctrl Pts',(-20.6743041569518,14.7315600320909,124.231770792966)) ;
#19810=CARTESIAN_POINT('Ctrl Pts',(-20.2927239230316,14.9214947173536,124.232648085746)) ;
#19811=CARTESIAN_POINT('Ctrl Pts',(-20.5135786631871,14.7415056369908,124.437867633095)) ;
#19812=CARTESIAN_POINT('Ctrl Pts',(-20.1377200748608,14.9314419908352,124.373043867283)) ;
#19813=CARTESIAN_POINT('Ctrl Pts',(-20.3198218573511,14.7514529104723,124.613360457444)) ;
#19814=CARTESIAN_POINT('Ctrl Pts',(-19.9587916673367,14.9414899053115,124.485309172283)) ;
#19815=CARTESIAN_POINT('Ctrl Pts',(-20.0961599099383,14.7615008249487,124.753689774848)) ;
#19816=CARTESIAN_POINT('Ctrl Pts',(-19.7670469759163,14.9513375456589,124.563382819774)) ;
#19817=CARTESIAN_POINT('Ctrl Pts',(-19.8564776376663,14.771348465296,124.851279444888)) ;
#19818=CARTESIAN_POINT('Ctrl Pts',(-19.5624646344758,14.9612992610355,124.608121127697)) ;
#19819=CARTESIAN_POINT('Ctrl Pts',(-19.6007489896213,14.7813101806726,124.907199618394)) ;
#19820=CARTESIAN_POINT('Ctrl Pts',(-19.3517826029045,14.9713278846083,124.61644912002)) ;
#19821=CARTESIAN_POINT('Ctrl Pts',(-19.3373962978428,14.7913388042454,124.917606836282)) ;
#19822=CARTESIAN_POINT('Ctrl Pts',(-19.145332332827,14.9812382466747,124.588473295284)) ;
#19823=CARTESIAN_POINT('Ctrl Pts',(-19.0793336231031,14.8012491663118,124.882634265756)) ;
#19824=CARTESIAN_POINT('Ctrl Pts',(-18.9462038692032,14.9911729403271,124.525440044832)) ;
#19825=CARTESIAN_POINT('Ctrl Pts',(-18.8304237660988,14.8111838599642,124.803839977348)) ;
#19826=CARTESIAN_POINT('Ctrl Pts',(-18.7591614865791,15.001214783455,124.427569567412)) ;
#19827=CARTESIAN_POINT('Ctrl Pts',(-18.5966220485025,14.8212257030921,124.681499373881)) ;
#19828=CARTESIAN_POINT('Ctrl Pts',(-18.5944360678556,15.0110992890254,124.300855256588)) ;
#19829=CARTESIAN_POINT('Ctrl Pts',(-18.390716860511,14.8311102086625,124.523104155642)) ;
#19830=CARTESIAN_POINT('Ctrl Pts',(-18.4524001316479,15.0211013928106,124.145842998901)) ;
#19831=CARTESIAN_POINT('Ctrl Pts',(-18.2131739736385,14.8411123124477,124.329336878928)) ;
#19832=CARTESIAN_POINT('Ctrl Pts',(-18.3402023620306,15.0310197442256,123.970045804479)) ;
#19833=CARTESIAN_POINT('Ctrl Pts',(-18.0729290956816,14.8510306638627,124.109588770675)) ;
#19834=CARTESIAN_POINT('Ctrl Pts',(-18.2592672869496,15.0410674002465,123.774968507367)) ;
#19835=CARTESIAN_POINT('Ctrl Pts',(-17.9717628132547,14.8610783198836,123.865741080711)) ;
#19836=CARTESIAN_POINT('Ctrl Pts',(-18.2139943917343,15.0509385932747,123.572398931231)) ;
#19837=CARTESIAN_POINT('Ctrl Pts',(-17.9151745106479,14.8709495129118,123.612528140335)) ;
#19838=CARTESIAN_POINT('Ctrl Pts',(-18.2043671465967,15.0610043064182,123.361053655738)) ;
#19839=CARTESIAN_POINT('Ctrl Pts',(-17.9031429831484,14.8810152260553,123.34834743098)) ;
#19840=CARTESIAN_POINT('Ctrl Pts',(-18.2307795956915,15.0708567669908,123.155558216153)) ;
#19841=CARTESIAN_POINT('Ctrl Pts',(-17.9361624249687,14.890867686628,123.091474379834)) ;
#19842=CARTESIAN_POINT('Ctrl Pts',(-18.314927021648,15.0842852297134,122.886155404172)) ;
#19843=CARTESIAN_POINT('Ctrl Pts',(-18.0413449335706,14.9042961493505,122.754742299802)) ;
#19844=CARTESIAN_POINT('Ctrl Pts',(-18.4633001207492,15.0973661772305,122.650732206668)) ;
#19845=CARTESIAN_POINT('Ctrl Pts',(-18.2267874470069,14.9173770968676,122.460483907588)) ;
#19846=CARTESIAN_POINT('Ctrl Pts',(-18.6709215131284,15.110840675465,122.458175069999)) ;
#19847=CARTESIAN_POINT('Ctrl Pts',(-18.4863543902938,14.9308515951022,122.219747666857)) ;
#19848=CARTESIAN_POINT('Ctrl Pts',(-18.8447665738617,15.1206727790745,122.346277793249)) ;
#19849=CARTESIAN_POINT('Ctrl Pts',(-18.7036544341988,14.9406836987116,122.079886991967)) ;
#19850=CARTESIAN_POINT('Ctrl Pts',(-19.0375991766532,15.1306386822012,122.264426190155)) ;
#19851=CARTESIAN_POINT('Ctrl Pts',(-18.9446987351203,14.9506496018383,121.977572951031)) ;
#19852=CARTESIAN_POINT('Ctrl Pts',(-19.2431027809361,15.1406660915114,122.217314375215)) ;
#19853=CARTESIAN_POINT('Ctrl Pts',(-19.2015765911018,14.9606770111485,121.918685704724)) ;
#19854=CARTESIAN_POINT('Ctrl Pts',(-19.4511603917055,15.150577122878,122.206669239406)) ;
#19855=CARTESIAN_POINT('Ctrl Pts',(-19.4616556588049,14.9705880425151,121.905384721623)) ;
#19856=CARTESIAN_POINT('Ctrl Pts',(-19.7276733496542,15.163821430499,122.240072867962)) ;
#19857=CARTESIAN_POINT('Ctrl Pts',(-19.8072618039374,14.9838323501362,121.947128778354)) ;
#19858=CARTESIAN_POINT('Ctrl Pts',(-20.0569080569754,15.1805219131702,122.372778838028)) ;
#19859=CARTESIAN_POINT('Ctrl Pts',(-20.2188550941679,15.0005328328073,122.113045312188)) ;
#19860=CARTESIAN_POINT('Ctrl Pts',(-20.3183298277955,15.197028742326,122.607156814012)) ;
#19861=CARTESIAN_POINT('Ctrl Pts',(-20.5455679441702,15.0170396619631,122.405960959497)) ;
#19862=CARTESIAN_POINT('Ctrl Pts',(-20.4717021929632,15.2103393705636,122.841112767138)) ;
#19863=CARTESIAN_POINT('Ctrl Pts',(-20.7373262391937,15.0303502902007,122.698457845509)) ;
#19864=CARTESIAN_POINT('Ctrl Pts',(-20.5546889086436,15.2203319341037,123.034149268203)) ;
#19865=CARTESIAN_POINT('Ctrl Pts',(-20.8410482037776,15.0403428537408,122.939743261889)) ;
#19866=CARTESIAN_POINT('Ctrl Pts',(-20.6028117634593,15.2303620171052,123.239415681091)) ;
#19867=CARTESIAN_POINT('Ctrl Pts',(-20.9012011780977,15.0503729367423,123.196334518998)) ;
#19868=CARTESIAN_POINT('Ctrl Pts',(-20.6188231290724,15.243535621103,123.51597584994)) ;
#19869=CARTESIAN_POINT('Ctrl Pts',(-20.9212136813736,15.0635465407401,123.542009444152)) ;
#19870=CARTESIAN_POINT('Ctrl Pts',(-20.5476924046879,15.2601733263344,123.862358698214)) ;
#19871=CARTESIAN_POINT('Ctrl Pts',(-20.8322977307926,15.0801842459715,123.97501211203)) ;
#19872=CARTESIAN_POINT('Ctrl Pts',(-20.3266298052787,15.2800550889018,124.222868771879)) ;
#19873=CARTESIAN_POINT('Ctrl Pts',(-20.5559470864143,15.1000660085389,124.425649304088)) ;
#19874=CARTESIAN_POINT('Ctrl Pts',(-20.0488038588937,15.2967514411183,124.443780899376)) ;
#19875=CARTESIAN_POINT('Ctrl Pts',(-20.2087222530336,15.1167623607554,124.70175262575)) ;
#19876=CARTESIAN_POINT('Ctrl Pts',(-19.7952370287234,15.3099084689074,124.554316113986)) ;
#19877=CARTESIAN_POINT('Ctrl Pts',(-19.8917080630513,15.1299193885445,124.839949683673)) ;
#19878=CARTESIAN_POINT('Ctrl Pts',(-19.5219729563658,15.3232858235509,124.620769738121)) ;
#19879=CARTESIAN_POINT('Ctrl Pts',(-19.5501536847632,15.1432967431881,124.92300774244)) ;
#19880=CARTESIAN_POINT('Ctrl Pts',(-19.1705511769297,15.3398166578097,124.612563673835)) ;
#19881=CARTESIAN_POINT('Ctrl Pts',(-19.1108554066313,15.1598275774469,124.912748434119)) ;
#19882=CARTESIAN_POINT('Ctrl Pts',(-18.7747945960682,15.3597813475528,124.459104510139)) ;
#19883=CARTESIAN_POINT('Ctrl Pts',(-18.616168502824,15.17979226719,124.720920100906)) ;
#19884=CARTESIAN_POINT('Ctrl Pts',(-18.4561643055464,15.3796978409765,124.180149863833)) ;
#19885=CARTESIAN_POINT('Ctrl Pts',(-18.2178819295255,15.1997087606136,124.372224270615)) ;
#19886=CARTESIAN_POINT('Ctrl Pts',(-18.2513709239315,15.399587560326,123.810085056575)) ;
#19887=CARTESIAN_POINT('Ctrl Pts',(-17.9618943674429,15.2195984799632,123.909642300137)) ;
#19888=CARTESIAN_POINT('Ctrl Pts',(-18.185122044345,15.4195942899739,123.38994096914)) ;
#19889=CARTESIAN_POINT('Ctrl Pts',(-17.8790867340295,15.239605209611,123.384461553137)) ;
#19890=CARTESIAN_POINT('Ctrl Pts',(-18.2652543652805,15.4394323436208,122.975722101847)) ;
#19891=CARTESIAN_POINT('Ctrl Pts',(-17.9792551414852,15.2594432632579,122.866690154571)) ;
#19892=CARTESIAN_POINT('Ctrl Pts',(-18.4831677244092,15.4594256818344,122.610800320768)) ;
#19893=CARTESIAN_POINT('Ctrl Pts',(-18.2516493430185,15.2794366014715,122.410539526417)) ;
#19894=CARTESIAN_POINT('Ctrl Pts',(-18.8109961180814,15.479308481241,122.343735818946)) ;
#19895=CARTESIAN_POINT('Ctrl Pts',(-18.661435692982,15.2993194008781,122.076711965965)) ;
#19896=CARTESIAN_POINT('Ctrl Pts',(-19.2100433870964,15.4992006621597,122.203893854528)) ;
#19897=CARTESIAN_POINT('Ctrl Pts',(-19.1602442446391,15.3192115817968,121.901912195536)) ;
#19898=CARTESIAN_POINT('Ctrl Pts',(-19.6333249972784,15.5191028406548,122.207913004512)) ;
#19899=CARTESIAN_POINT('Ctrl Pts',(-19.6893450348153,15.3391137602919,121.906937811211)) ;
#19900=CARTESIAN_POINT('Ctrl Pts',(-20.0320344555378,15.5391401518585,122.357748545318)) ;
#19901=CARTESIAN_POINT('Ctrl Pts',(-20.1877316480936,15.3591510714956,122.094234259217)) ;
#19902=CARTESIAN_POINT('Ctrl Pts',(-20.3526586672201,15.5589525933994,122.631285692703)) ;
#19903=CARTESIAN_POINT('Ctrl Pts',(-20.5885091138174,15.3789635130365,122.4361550605)) ;
#19904=CARTESIAN_POINT('Ctrl Pts',(-20.5630361294496,15.5790178341343,123.002216406184)) ;
#19905=CARTESIAN_POINT('Ctrl Pts',(-20.8514802727897,15.3990287537714,122.899819819407)) ;
#19906=CARTESIAN_POINT('Ctrl Pts',(-20.633508538707,15.5987750389901,123.416561760013)) ;
#19907=CARTESIAN_POINT('Ctrl Pts',(-20.939569466923,15.4187859586272,123.417748054594)) ;
#19908=CARTESIAN_POINT('Ctrl Pts',(-20.5580007528934,15.6188083116358,123.835558911533)) ;
#19909=CARTESIAN_POINT('Ctrl Pts',(-20.8451846342489,15.4388192312729,123.941494843128)) ;
#19910=CARTESIAN_POINT('Ctrl Pts',(-20.3461462838386,15.6386212200896,124.199911351364)) ;
#19911=CARTESIAN_POINT('Ctrl Pts',(-20.5803681949361,15.4586321397268,124.396932991369)) ;
#19912=CARTESIAN_POINT('Ctrl Pts',(-20.0203388845668,15.6586173662171,124.472784286855)) ;
#19913=CARTESIAN_POINT('Ctrl Pts',(-20.1731096405733,15.4786282858542,124.738024765008)) ;
#19914=CARTESIAN_POINT('Ctrl Pts',(-19.6233743789427,15.6784791194396,124.617449122825)) ;
#19915=CARTESIAN_POINT('Ctrl Pts',(-19.6769061894164,15.4984900390767,124.918856330261)) ;
#19916=CARTESIAN_POINT('Ctrl Pts',(-19.1967590474696,15.6985476365677,124.617705022532)) ;
#19917=CARTESIAN_POINT('Ctrl Pts',(-19.1436360482035,15.5185585562048,124.919177517765)) ;
#19918=CARTESIAN_POINT('Ctrl Pts',(-18.8003320264179,15.7183785095645,124.473760456347)) ;
#19919=CARTESIAN_POINT('Ctrl Pts',(-18.6481039856445,15.5383894292016,124.739248841471)) ;
#19920=CARTESIAN_POINT('Ctrl Pts',(-18.4747503929125,15.7383004203812,124.20293742243)) ;
#19921=CARTESIAN_POINT('Ctrl Pts',(-18.2411262734598,15.5583113400183,124.400722475563)) ;
#19922=CARTESIAN_POINT('Ctrl Pts',(-18.2610720953533,15.7582298638165,123.836921398904)) ;
#19923=CARTESIAN_POINT('Ctrl Pts',(-17.9740267390617,15.5782407834536,123.943204335233)) ;
#19924=CARTESIAN_POINT('Ctrl Pts',(-18.185068198707,15.7781395339329,123.420531358687)) ;
#19925=CARTESIAN_POINT('Ctrl Pts',(-17.8790194223619,15.59815045357,123.422718308582)) ;
#19926=CARTESIAN_POINT('Ctrl Pts',(-18.2548638512684,15.7980128911957,123.003722761479)) ;
#19927=CARTESIAN_POINT('Ctrl Pts',(-17.9662605748662,15.6180238108329,122.901708304058)) ;
#19928=CARTESIAN_POINT('Ctrl Pts',(-18.4639568410273,15.8180044258137,122.633696412297)) ;
#19929=CARTESIAN_POINT('Ctrl Pts',(-18.2276238439571,15.6380153454508,122.439173769157)) ;
#19930=CARTESIAN_POINT('Ctrl Pts',(-18.7847146040937,15.8378700432244,122.358763046612)) ;
#19931=CARTESIAN_POINT('Ctrl Pts',(-18.6285678009232,15.6578809628615,122.095505124988)) ;
#19932=CARTESIAN_POINT('Ctrl Pts',(-19.182109206407,15.8578509730526,122.208558793697)) ;
#19933=CARTESIAN_POINT('Ctrl Pts',(-19.1253095706751,15.6778618926898,121.907746174012)) ;
#19934=CARTESIAN_POINT('Ctrl Pts',(-19.606033490729,15.8777894351358,122.203463863361)) ;
#19935=CARTESIAN_POINT('Ctrl Pts',(-19.6552143908038,15.6978003547729,121.901373660419)) ;
#19936=CARTESIAN_POINT('Ctrl Pts',(-20.0055761170638,15.8976816283575,122.342403399768)) ;
#19937=CARTESIAN_POINT('Ctrl Pts',(-20.1546433032014,15.7176925479946,122.075043824401)) ;
#19938=CARTESIAN_POINT('Ctrl Pts',(-20.3347791009066,15.9176523433929,122.61046686242)) ;
#19939=CARTESIAN_POINT('Ctrl Pts',(-20.5661496331982,15.73766326303,122.410119645807)) ;
#19940=CARTESIAN_POINT('Ctrl Pts',(-20.551706715397,15.937462015059,122.971635608473)) ;
#19941=CARTESIAN_POINT('Ctrl Pts',(-20.8373123753955,15.7574729346961,122.861577302707)) ;
#19942=CARTESIAN_POINT('Ctrl Pts',(-20.6333723481961,15.9574552317502,123.388667733852)) ;
#19943=CARTESIAN_POINT('Ctrl Pts',(-20.9393997364478,15.7774661513873,123.382866096592)) ;
#19944=CARTESIAN_POINT('Ctrl Pts',(-20.5685874573327,15.9773061439465,123.805925874308)) ;
#19945=CARTESIAN_POINT('Ctrl Pts',(-20.8584216081124,15.7973170635836,123.904440437728)) ;
#19946=CARTESIAN_POINT('Ctrl Pts',(-20.3629339575336,15.9973807502655,124.179831486359)) ;
#19947=CARTESIAN_POINT('Ctrl Pts',(-20.6013666268889,15.8173916699027,124.371819409561)) ;
#19948=CARTESIAN_POINT('Ctrl Pts',(-20.0986057487275,16.0138973821489,124.411216269807)) ;
#19949=CARTESIAN_POINT('Ctrl Pts',(-20.2709357008999,15.833908301786,124.661071335312)) ;
#19950=CARTESIAN_POINT('Ctrl Pts',(-19.8472305510429,16.027236089843,124.535405517903)) ;
#19951=CARTESIAN_POINT('Ctrl Pts',(-19.9567400193657,15.8472470094801,124.816295036982)) ;
#19952=CARTESIAN_POINT('Ctrl Pts',(-19.648689899929,16.0370784641513,124.593781061793)) ;
#19953=CARTESIAN_POINT('Ctrl Pts',(-19.7085577801769,15.8570893837884,124.889269258747)) ;
#19954=CARTESIAN_POINT('Ctrl Pts',(-19.4386553018546,16.047133484134,124.61748484339)) ;
#19955=CARTESIAN_POINT('Ctrl Pts',(-19.4460289923727,15.8671444037711,124.918903925048)) ;
#19956=CARTESIAN_POINT('Ctrl Pts',(-19.1610280376061,16.0603656407916,124.600218445625)) ;
#19957=CARTESIAN_POINT('Ctrl Pts',(-19.0989283678214,15.8803765604287,124.897309206157)) ;
#19958=CARTESIAN_POINT('Ctrl Pts',(-18.825889100884,16.0769806081367,124.488333617129)) ;
#19959=CARTESIAN_POINT('Ctrl Pts',(-18.680086550223,15.8969915277738,124.757481852894)) ;
#19960=CARTESIAN_POINT('Ctrl Pts',(-18.5495711916303,16.0935751951479,124.269005818189)) ;
#19961=CARTESIAN_POINT('Ctrl Pts',(-18.3346327392559,15.913586114785,124.48329340641)) ;
#19962=CARTESIAN_POINT('Ctrl Pts',(-18.383354158807,16.1068087635033,124.045842736508)) ;
#19963=CARTESIAN_POINT('Ctrl Pts',(-18.1268897362054,15.9268196831404,124.204366870051)) ;
#19964=CARTESIAN_POINT('Ctrl Pts',(-18.2885245171761,16.1168523813119,123.857213437139)) ;
#19965=CARTESIAN_POINT('Ctrl Pts',(-18.0083439444997,15.9368633009491,123.968576154149)) ;
#19966=CARTESIAN_POINT('Ctrl Pts',(-18.2287506235429,16.1267393055468,123.658118953478)) ;
#19967=CARTESIAN_POINT('Ctrl Pts',(-17.9336253681816,15.9467502251839,123.719711066793)) ;
#19968=CARTESIAN_POINT('Ctrl Pts',(-18.2038316638123,16.1367299599936,123.449583936804)) ;
#19969=CARTESIAN_POINT('Ctrl Pts',(-17.9024744065932,15.9567408796307,123.459039355824)) ;
#19970=CARTESIAN_POINT('Ctrl Pts',(-18.2155127325471,16.1466917184475,123.240472594879)) ;
#19971=CARTESIAN_POINT('Ctrl Pts',(-17.9170694041595,15.9667026380847,123.197660756749)) ;
#19972=CARTESIAN_POINT('Ctrl Pts',(-18.2792368886857,16.1600315835148,122.967353209043)) ;
#19973=CARTESIAN_POINT('Ctrl Pts',(-17.9967391763496,15.9800425031519,122.856207482281)) ;
#19974=CARTESIAN_POINT('Ctrl Pts',(-18.41302923077,16.1733403664281,122.718017566954)) ;
#19975=CARTESIAN_POINT('Ctrl Pts',(-18.1639736695918,15.9933512860652,122.544568270991)) ;
#19976=CARTESIAN_POINT('Ctrl Pts',(-18.6026009651151,16.1865361238721,122.515452306746)) ;
#19977=CARTESIAN_POINT('Ctrl Pts',(-18.4009205226991,16.0065470435093,122.291373958012)) ;
#19978=CARTESIAN_POINT('Ctrl Pts',(-18.7697316480871,16.1964980075486,122.389244608376)) ;
#19979=CARTESIAN_POINT('Ctrl Pts',(-18.6098352782094,16.0165089271858,122.133609050801)) ;
#19980=CARTESIAN_POINT('Ctrl Pts',(-18.9579132109796,16.2065411170633,122.293505577334)) ;
#19981=CARTESIAN_POINT('Ctrl Pts',(-18.8450601920169,16.0265520367004,122.013933523829)) ;
#19982=CARTESIAN_POINT('Ctrl Pts',(-19.1559583596013,16.2163933670625,122.232828073835)) ;
#19983=CARTESIAN_POINT('Ctrl Pts',(-19.0926161288735,16.0364042866996,121.938083702946)) ;
#19984=CARTESIAN_POINT('Ctrl Pts',(-19.3639266023041,16.226364904013,122.20664426832)) ;
#19985=CARTESIAN_POINT('Ctrl Pts',(-19.3525761374353,16.0463758236501,121.90535120371)) ;
#19986=CARTESIAN_POINT('Ctrl Pts',(-19.5738352772956,16.2363601694905,122.217013254614)) ;
#19987=CARTESIAN_POINT('Ctrl Pts',(-19.6149622143192,16.0563710891276,121.918309627861)) ;
#19988=CARTESIAN_POINT('Ctrl Pts',(-19.7794415898056,16.2463941423641,122.264093918599)) ;
#19989=CARTESIAN_POINT('Ctrl Pts',(-19.8719707676213,16.0664050620013,121.977157725234)) ;
#19990=CARTESIAN_POINT('Ctrl Pts',(-19.9704548769762,16.2562495571265,122.344410165683)) ;
#19991=CARTESIAN_POINT('Ctrl Pts',(-20.1107386746183,16.0762604767636,122.077550542983)) ;
#19992=CARTESIAN_POINT('Ctrl Pts',(-20.1472714092236,16.2662488346353,122.458039635008)) ;
#19993=CARTESIAN_POINT('Ctrl Pts',(-20.3317609231274,16.0862597542724,122.219585083318)) ;
#19994=CARTESIAN_POINT('Ctrl Pts',(-20.3002692337498,16.2761440187983,122.599043469478)) ;
#19995=CARTESIAN_POINT('Ctrl Pts',(-20.5230102658078,16.0961549384354,122.395838020282)) ;
#19996=CARTESIAN_POINT('Ctrl Pts',(-20.4285086882037,16.2862043984391,122.767195696691)) ;
#19997=CARTESIAN_POINT('Ctrl Pts',(-20.6833117694189,16.1062153180762,122.606026601043)) ;
#19998=CARTESIAN_POINT('Ctrl Pts',(-20.5237070485476,16.2960542674472,122.951113827602)) ;
#19999=CARTESIAN_POINT('Ctrl Pts',(-20.8023123453152,16.1160651870843,122.835923343469)) ;
#20000=CARTESIAN_POINT('Ctrl Pts',(-20.5871150710927,16.3060858286551,123.152237015231)) ;
#20001=CARTESIAN_POINT('Ctrl Pts',(-20.8815749658397,16.1260967482922,123.087326542233)) ;
#20002=CARTESIAN_POINT('Ctrl Pts',(-20.6141638262457,16.3160962775374,123.360962196681)) ;
#20003=CARTESIAN_POINT('Ctrl Pts',(-20.9153886455586,16.1361071971745,123.3482327168)) ;
#20004=CARTESIAN_POINT('Ctrl Pts',(-20.6048907446535,16.3260030169544,123.569019571295)) ;
#20005=CARTESIAN_POINT('Ctrl Pts',(-20.9038000062041,16.1460139365915,123.608304860459)) ;
#20006=CARTESIAN_POINT('Ctrl Pts',(-20.5598881669259,16.3359410330228,123.773031366739)) ;
#20007=CARTESIAN_POINT('Ctrl Pts',(-20.8475493442764,16.1559519526599,123.863320444448)) ;
#20008=CARTESIAN_POINT('Ctrl Pts',(-20.4797215293116,16.3459462794739,123.967521538131)) ;
#20009=CARTESIAN_POINT('Ctrl Pts',(-20.7473434745622,16.1659571991111,124.106434248665)) ;
#20010=CARTESIAN_POINT('Ctrl Pts',(-20.3663921716625,16.3559803405302,124.145428527425)) ;
#20011=CARTESIAN_POINT('Ctrl Pts',(-20.6056840713685,16.1759912601674,124.328819428175)) ;
#20012=CARTESIAN_POINT('Ctrl Pts',(-20.2268261020098,16.3658254215884,124.29828451982)) ;
#20013=CARTESIAN_POINT('Ctrl Pts',(-20.4312280688443,16.1858363412255,124.519891626386)) ;
#20014=CARTESIAN_POINT('Ctrl Pts',(-20.0607710857715,16.3758112275419,124.42667346357)) ;
#20015=CARTESIAN_POINT('Ctrl Pts',(-20.2236607634961,16.195822147179,124.680379963816)) ;
#20016=CARTESIAN_POINT('Ctrl Pts',(-19.8759009892187,16.3857460480961,124.523947203319)) ;
#20017=CARTESIAN_POINT('Ctrl Pts',(-19.9925740517516,16.2057569677332,124.801974564811)) ;
#20018=CARTESIAN_POINT('Ctrl Pts',(-19.6745001645774,16.3958035732283,124.588229437951)) ;
#20019=CARTESIAN_POINT('Ctrl Pts',(-19.7408239243177,16.2158144928654,124.88232980859)) ;
#20020=CARTESIAN_POINT('Ctrl Pts',(-19.4699018787836,16.4056252238796,124.616221674398)) ;
#20021=CARTESIAN_POINT('Ctrl Pts',(-19.4850756391553,16.2256361435168,124.917322735119)) ;
#20022=CARTESIAN_POINT('Ctrl Pts',(-19.2586509012011,16.4156812873844,124.608469860798)) ;
#20023=CARTESIAN_POINT('Ctrl Pts',(-19.2210119356238,16.2356922070215,124.90763544783)) ;
#20024=CARTESIAN_POINT('Ctrl Pts',(-19.0543812444969,16.4256219544483,124.56429049855)) ;
#20025=CARTESIAN_POINT('Ctrl Pts',(-18.965674000184,16.2456328740854,124.852413667813)) ;
#20026=CARTESIAN_POINT('Ctrl Pts',(-18.861349537296,16.4355263481143,124.486210004502)) ;
#20027=CARTESIAN_POINT('Ctrl Pts',(-18.7243829673979,16.2555372677514,124.754815092852)) ;
#20028=CARTESIAN_POINT('Ctrl Pts',(-18.6823656137702,16.4455728718773,124.374110855955)) ;
#20029=CARTESIAN_POINT('Ctrl Pts',(-18.5006518515227,16.2655837915144,124.614693286642)) ;
#20030=CARTESIAN_POINT('Ctrl Pts',(-18.5277366886048,16.4554689548937,124.234866899934)) ;
#20031=CARTESIAN_POINT('Ctrl Pts',(-18.3073636533246,16.2754798745308,124.440639733717)) ;
#20032=CARTESIAN_POINT('Ctrl Pts',(-18.397512504775,16.4655356541237,124.068090149014)) ;
#20033=CARTESIAN_POINT('Ctrl Pts',(-18.1445816442607,16.2855465737608,124.232170442766)) ;
#20034=CARTESIAN_POINT('Ctrl Pts',(-18.3003784994557,16.4753592645248,123.885799724295)) ;
#20035=CARTESIAN_POINT('Ctrl Pts',(-18.0231616074987,16.2953701841619,124.004307681981)) ;
#20036=CARTESIAN_POINT('Ctrl Pts',(-18.2345231615704,16.4854151247023,123.684941160413)) ;
#20037=CARTESIAN_POINT('Ctrl Pts',(-17.9408403240638,16.3054260443394,123.753235338654)) ;
#20038=CARTESIAN_POINT('Ctrl Pts',(-18.2051689662618,16.4953482710072,123.478162940321)) ;
#20039=CARTESIAN_POINT('Ctrl Pts',(-17.904145201317,16.3153591906443,123.494762458891)) ;
#20040=CARTESIAN_POINT('Ctrl Pts',(-18.2117436428783,16.5052935267778,123.269210161589)) ;
#20041=CARTESIAN_POINT('Ctrl Pts',(-17.9123613233359,16.3253044464149,123.233570994404)) ;
#20042=CARTESIAN_POINT('Ctrl Pts',(-18.2545082390918,16.5152768252163,123.063705916951)) ;
#20043=CARTESIAN_POINT('Ctrl Pts',(-17.9658149650056,16.3352877448534,122.976690048544)) ;
#20044=CARTESIAN_POINT('Ctrl Pts',(-18.3329769113409,16.5253140053629,122.867842390834)) ;
#20045=CARTESIAN_POINT('Ctrl Pts',(-18.0638986666255,16.345324925,122.731859880856)) ;
#20046=CARTESIAN_POINT('Ctrl Pts',(-18.4419820599427,16.5351685580724,122.691641388023)) ;
#20047=CARTESIAN_POINT('Ctrl Pts',(-18.2001537297579,16.3551794777095,122.511606700127)) ;
#20048=CARTESIAN_POINT('Ctrl Pts',(-18.581699061968,16.5451680765197,122.534616193338)) ;
#20049=CARTESIAN_POINT('Ctrl Pts',(-18.3747984971053,16.3651789961568,122.315323705892)) ;
#20050=CARTESIAN_POINT('Ctrl Pts',(-18.7447549291817,16.5550631589818,122.405380089369)) ;
#20051=CARTESIAN_POINT('Ctrl Pts',(-18.5786176379803,16.3750740786189,122.153776522294)) ;
#20052=CARTESIAN_POINT('Ctrl Pts',(-18.9307890892371,16.5651237044879,122.304812169695)) ;
#20053=CARTESIAN_POINT('Ctrl Pts',(-18.8111591522696,16.385134624125,122.028064933009)) ;
#20054=CARTESIAN_POINT('Ctrl Pts',(-19.1272493004739,16.5749730117359,122.239351514005)) ;
#20055=CARTESIAN_POINT('Ctrl Pts',(-19.0567347651697,16.394983931373,121.946236873333)) ;
#20056=CARTESIAN_POINT('Ctrl Pts',(-19.3356895472675,16.5850001018232,122.207921910754)) ;
#20057=CARTESIAN_POINT('Ctrl Pts',(-19.3172847594668,16.4050110214604,121.906948036796)) ;
#20058=CARTESIAN_POINT('Ctrl Pts',(-19.5464580747962,16.5950290059602,122.213723078869)) ;
#20059=CARTESIAN_POINT('Ctrl Pts',(-19.5807454043777,16.4150399255973,121.91419747043)) ;
#20060=CARTESIAN_POINT('Ctrl Pts',(-19.7492714933066,16.6048728710595,122.254846303391)) ;
#20061=CARTESIAN_POINT('Ctrl Pts',(-19.8342636546748,16.4248837906966,121.965599859095)) ;
#20062=CARTESIAN_POINT('Ctrl Pts',(-19.9450340387056,16.6148686977679,122.331249053741)) ;
#20063=CARTESIAN_POINT('Ctrl Pts',(-20.0789676317228,16.434879617405,122.0611017389)) ;
#20064=CARTESIAN_POINT('Ctrl Pts',(-20.1248865780728,16.6248939144169,122.441136839792)) ;
#20065=CARTESIAN_POINT('Ctrl Pts',(-20.3037842341569,16.444904834054,122.198459857618)) ;
#20066=CARTESIAN_POINT('Ctrl Pts',(-20.28097718897,16.6347837465745,122.57849001676)) ;
#20067=CARTESIAN_POINT('Ctrl Pts',(-20.4988993121104,16.4547946662116,122.370150559373)) ;
#20068=CARTESIAN_POINT('Ctrl Pts',(-20.4123923595961,16.6447746026592,122.742330187419)) ;
#20069=CARTESIAN_POINT('Ctrl Pts',(-20.6631697043296,16.4647855222963,122.574949866266)) ;
#20070=CARTESIAN_POINT('Ctrl Pts',(-20.5128694027826,16.6547196972521,122.925680754585)) ;
#20071=CARTESIAN_POINT('Ctrl Pts',(-20.7887677400445,16.4747306168892,122.804137700936)) ;
#20072=CARTESIAN_POINT('Ctrl Pts',(-20.5804045472884,16.6646716010202,123.12370981409)) ;
#20073=CARTESIAN_POINT('Ctrl Pts',(-20.8731883104183,16.4846825206573,123.051673973059)) ;
#20074=CARTESIAN_POINT('Ctrl Pts',(-20.6126176827345,16.6747080004896,123.332227708226)) ;
#20075=CARTESIAN_POINT('Ctrl Pts',(-20.9134563188917,16.4947189201267,123.312320962728)) ;
#20076=CARTESIAN_POINT('Ctrl Pts',(-20.6083540179915,16.6845970705783,123.540090086078)) ;
#20077=CARTESIAN_POINT('Ctrl Pts',(-20.9081282976239,16.5046079902154,123.572149884728)) ;
#20078=CARTESIAN_POINT('Ctrl Pts',(-20.5680279223368,16.6945863599492,123.746183169029)) ;
#20079=CARTESIAN_POINT('Ctrl Pts',(-20.8577220598271,16.5145972795863,123.829766727629)) ;
#20080=CARTESIAN_POINT('Ctrl Pts',(-20.4926169706463,16.7045449261589,123.941483709514)) ;
#20081=CARTESIAN_POINT('Ctrl Pts',(-20.76345961891,16.524555845796,124.073893348995)) ;
#20082=CARTESIAN_POINT('Ctrl Pts',(-20.3855116246943,16.7144444973757,124.119942910735)) ;
#20083=CARTESIAN_POINT('Ctrl Pts',(-20.6295786198911,16.5344554170128,124.296968784774)) ;
#20084=CARTESIAN_POINT('Ctrl Pts',(-20.2469681262543,16.7244924117899,124.279374314369)) ;
#20085=CARTESIAN_POINT('Ctrl Pts',(-20.4564004098396,16.5445033314271,124.49625876178)) ;
#20086=CARTESIAN_POINT('Ctrl Pts',(-20.0853998211911,16.7343877546505,124.410470530884)) ;
#20087=CARTESIAN_POINT('Ctrl Pts',(-20.254440134761,16.5543986742876,124.660130610446)) ;
#20088=CARTESIAN_POINT('Ctrl Pts',(-19.9005296097113,16.7444494485979,124.513218405503)) ;
#20089=CARTESIAN_POINT('Ctrl Pts',(-20.0233532789183,16.5644603682351,124.788566418278)) ;
#20090=CARTESIAN_POINT('Ctrl Pts',(-19.7049244472247,16.7542939016821,124.580859195891)) ;
#20091=CARTESIAN_POINT('Ctrl Pts',(-19.7788459931032,16.5743048213192,124.873119039239)) ;
#20092=CARTESIAN_POINT('Ctrl Pts',(-19.4982683090675,16.7642545866405,124.614617061562)) ;
#20093=CARTESIAN_POINT('Ctrl Pts',(-19.5205255375102,16.5842655062777,124.915317433973)) ;
#20094=CARTESIAN_POINT('Ctrl Pts',(-19.2872959543148,16.7742905191491,124.611604709264)) ;
#20095=CARTESIAN_POINT('Ctrl Pts',(-19.2568102129339,16.5943014387862,124.911553126493)) ;
#20096=CARTESIAN_POINT('Ctrl Pts',(-19.083065641411,16.7841791348371,124.572793885594)) ;
#20097=CARTESIAN_POINT('Ctrl Pts',(-19.0015211293968,16.6041900544743,124.863040443295)) ;
#20098=CARTESIAN_POINT('Ctrl Pts',(-18.8860375470221,16.7941935439796,124.498559615146)) ;
#20099=CARTESIAN_POINT('Ctrl Pts',(-18.7552356821971,16.6142044636167,124.770248444018)) ;
#20100=CARTESIAN_POINT('Ctrl Pts',(-18.7048442029777,16.8042273529374,124.390576815252)) ;
#20101=CARTESIAN_POINT('Ctrl Pts',(-18.5287435554736,16.6242382725745,124.635270964711)) ;
#20102=CARTESIAN_POINT('Ctrl Pts',(-18.5479851568458,16.8140578071936,124.255979370359)) ;
#20103=CARTESIAN_POINT('Ctrl Pts',(-18.3326680459431,16.6340687268307,124.467023867572)) ;
#20104=CARTESIAN_POINT('Ctrl Pts',(-18.4135706987232,16.8241354747718,124.092266151809)) ;
#20105=CARTESIAN_POINT('Ctrl Pts',(-18.164649593129,16.6441463944089,124.262383242805)) ;
#20106=CARTESIAN_POINT('Ctrl Pts',(-18.3118178527469,16.833987342894,123.911815748702)) ;
#20107=CARTESIAN_POINT('Ctrl Pts',(-18.037457177748,16.6539982625311,124.03681949593)) ;
#20108=CARTESIAN_POINT('Ctrl Pts',(-18.2412580423385,16.8440603804594,123.712187854895)) ;
#20109=CARTESIAN_POINT('Ctrl Pts',(-17.949256848314,16.6640713000965,123.787285292001)) ;
#20110=CARTESIAN_POINT('Ctrl Pts',(-18.2072505630093,16.8539029338102,123.508062557237)) ;
#20111=CARTESIAN_POINT('Ctrl Pts',(-17.9067465102641,16.6739138534474,123.53212739955)) ;
#20112=CARTESIAN_POINT('Ctrl Pts',(-18.2085239591176,16.8638833293037,123.298256187537)) ;
#20113=CARTESIAN_POINT('Ctrl Pts',(-17.908337764321,16.6838942489408,123.269869124294)) ;
#20114=CARTESIAN_POINT('Ctrl Pts',(-18.2467556082462,16.8739018072815,123.091139951509)) ;
#20115=CARTESIAN_POINT('Ctrl Pts',(-17.9561266808866,16.6939127269186,123.010973721011)) ;
#20116=CARTESIAN_POINT('Ctrl Pts',(-18.3189697446899,16.8837851215876,122.896288022926)) ;
#20117=CARTESIAN_POINT('Ctrl Pts',(-18.046394284067,16.7037960412247,122.767407615452)) ;
#20118=CARTESIAN_POINT('Ctrl Pts',(-18.425934681268,16.8938534241263,122.713676624745)) ;
#20119=CARTESIAN_POINT('Ctrl Pts',(-18.1800998015951,16.7138643437634,122.539143460683)) ;
#20120=CARTESIAN_POINT('Ctrl Pts',(-18.5595970562926,16.9036834713997,122.556016451482)) ;
#20121=CARTESIAN_POINT('Ctrl Pts',(-18.3471784469217,16.7236943910368,122.342066798614)) ;
#20122=CARTESIAN_POINT('Ctrl Pts',(-18.722208363347,16.9137503428152,122.42061719112)) ;
#20123=CARTESIAN_POINT('Ctrl Pts',(-18.5504420735912,16.7337612624523,122.172817736648)) ;
#20124=CARTESIAN_POINT('Ctrl Pts',(-18.9027264908965,16.9236393816143,122.317430530049)) ;
#20125=CARTESIAN_POINT('Ctrl Pts',(-18.7760904676618,16.7436503012514,122.043833574538)) ;
#20126=CARTESIAN_POINT('Ctrl Pts',(-19.1003612730022,16.9336360797484,122.246020456028)) ;
#20127=CARTESIAN_POINT('Ctrl Pts',(-19.0231340623094,16.7536469993855,121.95457073187)) ;
#20128=CARTESIAN_POINT('Ctrl Pts',(-19.3065267658046,16.9435885054603,122.210251377386)) ;
#20129=CARTESIAN_POINT('Ctrl Pts',(-19.2808414151497,16.7635994250975,121.909859064209)) ;
#20130=CARTESIAN_POINT('Ctrl Pts',(-19.5155081682475,16.9535298076933,122.210531944557)) ;
#20131=CARTESIAN_POINT('Ctrl Pts',(-19.5420687997964,16.7735407273304,121.910209653822)) ;
#20132=CARTESIAN_POINT('Ctrl Pts',(-19.7222133629213,16.9635130467772,122.24703377313)) ;
#20133=CARTESIAN_POINT('Ctrl Pts',(-19.8004505578449,16.7835239664143,121.955836958364)) ;
#20134=CARTESIAN_POINT('Ctrl Pts',(-19.9203861587656,16.9735518483458,122.319565863544)) ;
#20135=CARTESIAN_POINT('Ctrl Pts',(-20.0481664431086,16.7935627679829,122.04650185724)) ;
#20136=CARTESIAN_POINT('Ctrl Pts',(-20.0997203161893,16.9833999544674,122.423063092642)) ;
#20137=CARTESIAN_POINT('Ctrl Pts',(-20.27233537467,16.8034108741046,122.175874106053)) ;
#20138=CARTESIAN_POINT('Ctrl Pts',(-20.2618757976447,16.9934601500428,122.558817396899)) ;
#20139=CARTESIAN_POINT('Ctrl Pts',(-20.4750293998556,16.8134710696799,122.345566817946)) ;
#20140=CARTESIAN_POINT('Ctrl Pts',(-20.3956688355369,17.0033578333542,122.718192247894)) ;
#20141=CARTESIAN_POINT('Ctrl Pts',(-20.6422713390571,16.8233687529913,122.544786148084)) ;
#20142=CARTESIAN_POINT('Ctrl Pts',(-20.5006942150535,17.0132888737282,122.898630233536)) ;
#20143=CARTESIAN_POINT('Ctrl Pts',(-20.7735531876702,16.8332997933653,122.770334392659)) ;
#20144=CARTESIAN_POINT('Ctrl Pts',(-20.5733879414346,17.0233310913848,123.096836226167)) ;
#20145=CARTESIAN_POINT('Ctrl Pts',(-20.864420100794,16.8433420110219,123.018091751125)) ;
#20146=CARTESIAN_POINT('Ctrl Pts',(-20.61013604455,17.0332177521188,123.301420117355)) ;
#20147=CARTESIAN_POINT('Ctrl Pts',(-20.9103551819919,16.8532286717559,123.273822728003)) ;
#20148=CARTESIAN_POINT('Ctrl Pts',(-20.6111628873651,17.0432108607212,123.511493426387)) ;
#20149=CARTESIAN_POINT('Ctrl Pts',(-20.9116383536201,16.8632217803584,123.536414570098)) ;
#20150=CARTESIAN_POINT('Ctrl Pts',(-20.5757869989794,17.0531565593595,123.717568908306)) ;
#20151=CARTESIAN_POINT('Ctrl Pts',(-20.8674180471858,16.8731674789966,123.794009449891)) ;
#20152=CARTESIAN_POINT('Ctrl Pts',(-20.5055557491606,17.0631037816305,123.91455588214)) ;
#20153=CARTESIAN_POINT('Ctrl Pts',(-20.7796283027966,16.8831147012677,124.04024353424)) ;
#20154=CARTESIAN_POINT('Ctrl Pts',(-20.400941475518,17.0731518072107,124.098065903988)) ;
#20155=CARTESIAN_POINT('Ctrl Pts',(-20.6488602156385,16.8931627268478,124.269630633099)) ;
#20156=CARTESIAN_POINT('Ctrl Pts',(-20.2688802244909,17.0829990543536,124.257492396339)) ;
#20157=CARTESIAN_POINT('Ctrl Pts',(-20.4837823786232,16.9030099739907,124.468914512535)) ;
#20158=CARTESIAN_POINT('Ctrl Pts',(-20.1097187274717,17.0929622314443,124.39364708618)) ;
#20159=CARTESIAN_POINT('Ctrl Pts',(-20.2848296697992,16.9129731510814,124.639107596571)) ;
#20160=CARTESIAN_POINT('Ctrl Pts',(-19.9279652479733,17.1029919524777,124.500535991782)) ;
#20161=CARTESIAN_POINT('Ctrl Pts',(-20.0576375877666,16.9230028721148,124.772718133945)) ;
#20162=CARTESIAN_POINT('Ctrl Pts',(-19.7329501884367,17.1128964200106,124.573568512816)) ;
#20163=CARTESIAN_POINT('Ctrl Pts',(-19.8138676646833,16.9329073396477,124.864008421836)) ;
#20164=CARTESIAN_POINT('Ctrl Pts',(-19.5257911753333,17.1229209058404,124.612154491612)) ;
#20165=CARTESIAN_POINT('Ctrl Pts',(-19.5549188176407,16.9429318254775,124.912240141092)) ;
#20166=CARTESIAN_POINT('Ctrl Pts',(-19.31756391383,17.1328247409643,124.61433347866)) ;
#20167=CARTESIAN_POINT('Ctrl Pts',(-19.2946338276999,16.9528356606014,124.914963066489)) ;
#20168=CARTESIAN_POINT('Ctrl Pts',(-19.1091090081414,17.1428759316743,124.579872920246)) ;
#20169=CARTESIAN_POINT('Ctrl Pts',(-19.0340655773043,16.9628868513114,124.871886584455)) ;
#20170=CARTESIAN_POINT('Ctrl Pts',(-18.9130563367156,17.1527603743326,124.510927123554)) ;
#20171=CARTESIAN_POINT('Ctrl Pts',(-18.7889990253017,16.9727712939697,124.785703184415)) ;
#20172=CARTESIAN_POINT('Ctrl Pts',(-18.7298067492815,17.1627533821844,124.408227429551)) ;
#20173=CARTESIAN_POINT('Ctrl Pts',(-18.5599373549121,16.9827643018216,124.657327597577)) ;
#20174=CARTESIAN_POINT('Ctrl Pts',(-18.5679203831117,17.1727017019007,124.275788607794)) ;
#20175=CARTESIAN_POINT('Ctrl Pts',(-18.3575795915092,16.9927126215379,124.491777975001)) ;
#20176=CARTESIAN_POINT('Ctrl Pts',(-18.4314404984795,17.1826385406102,124.117654900574)) ;
#20177=CARTESIAN_POINT('Ctrl Pts',(-18.186980138861,17.0026494602473,124.294109650112)) ;
#20178=CARTESIAN_POINT('Ctrl Pts',(-18.3237434951537,17.1926215295298,123.937489058372)) ;
#20179=CARTESIAN_POINT('Ctrl Pts',(-18.0523597654586,17.0126324491669,124.06890152174)) ;
#20180=CARTESIAN_POINT('Ctrl Pts',(-18.2488910018654,17.2026654088939,123.740073906393)) ;
#20181=CARTESIAN_POINT('Ctrl Pts',(-17.9587951854769,17.022676328531,123.82213239202)) ;
#20182=CARTESIAN_POINT('Ctrl Pts',(-18.2098074279025,17.2124934742523,123.537154265796)) ;
#20183=CARTESIAN_POINT('Ctrl Pts',(-17.9099416408422,17.0325043938894,123.568481191394)) ;
#20184=CARTESIAN_POINT('Ctrl Pts',(-18.2063795196312,17.2225705628072,123.325376725486)) ;
#20185=CARTESIAN_POINT('Ctrl Pts',(-17.9056580144789,17.0425814824443,123.303759681484)) ;
#20186=CARTESIAN_POINT('Ctrl Pts',(-18.2389039387934,17.2324207149635,123.120811528731)) ;
#20187=CARTESIAN_POINT('Ctrl Pts',(-17.9463150166963,17.0524316346006,123.048052157451)) ;
#20188=CARTESIAN_POINT('Ctrl Pts',(-18.3079172661289,17.2425011954158,122.920496194751)) ;
#20189=CARTESIAN_POINT('Ctrl Pts',(-18.032582786432,17.062512115053,122.797658849589)) ;
#20190=CARTESIAN_POINT('Ctrl Pts',(-18.4078418322244,17.2523156931847,122.739922505072)) ;
#20191=CARTESIAN_POINT('Ctrl Pts',(-18.1574904407852,17.0723266128218,122.571941098829)) ;
#20192=CARTESIAN_POINT('Ctrl Pts',(-18.5406376489348,17.2623839892048,122.575157598147)) ;
#20193=CARTESIAN_POINT('Ctrl Pts',(-18.3234861663821,17.0823949088419,122.36598619016)) ;
#20194=CARTESIAN_POINT('Ctrl Pts',(-18.6974563857139,17.2722828216876,122.43827365892)) ;
#20195=CARTESIAN_POINT('Ctrl Pts',(-18.5195111943069,17.0922937413247,122.194881832912)) ;
#20196=CARTESIAN_POINT('Ctrl Pts',(-18.878314400253,17.2823357017021,122.329011502217)) ;
#20197=CARTESIAN_POINT('Ctrl Pts',(-18.7455842875903,17.1023466213392,122.058305557914)) ;
#20198=CARTESIAN_POINT('Ctrl Pts',(-19.0718160918219,17.2922055171983,122.253987097039)) ;
#20199=CARTESIAN_POINT('Ctrl Pts',(-18.9874629412991,17.1122164368354,121.964526142813)) ;
#20200=CARTESIAN_POINT('Ctrl Pts',(-19.2795008716947,17.3022781982811,122.212830255507)) ;
#20201=CARTESIAN_POINT('Ctrl Pts',(-19.2470688770235,17.1222891179182,121.913081725806)) ;
#20202=CARTESIAN_POINT('Ctrl Pts',(-19.4861827851385,17.312110676852,122.208383210554)) ;
#20203=CARTESIAN_POINT('Ctrl Pts',(-19.505422587486,17.1321215964892,121.907524515032)) ;
#20204=CARTESIAN_POINT('Ctrl Pts',(-19.6946785789896,17.3221413108381,122.23992020577)) ;
#20205=CARTESIAN_POINT('Ctrl Pts',(-19.7660419704814,17.1421522304753,121.946947546496)) ;
#20206=CARTESIAN_POINT('Ctrl Pts',(-19.8943714717527,17.3321728680573,122.307777090262)) ;
#20207=CARTESIAN_POINT('Ctrl Pts',(-20.0156574864725,17.1521837876944,122.031770159067)) ;
#20208=CARTESIAN_POINT('Ctrl Pts',(-20.0757133418564,17.342002576929,122.406842625941)) ;
#20209=CARTESIAN_POINT('Ctrl Pts',(-20.2423350956265,17.1620134965661,122.155604235088)) ;
#20210=CARTESIAN_POINT('Ctrl Pts',(-20.2401293619726,17.3519920257311,122.53751027012)) ;
#20211=CARTESIAN_POINT('Ctrl Pts',(-20.4478540416198,17.1720029453682,122.318940433098)) ;
#20212=CARTESIAN_POINT('Ctrl Pts',(-20.3797110879383,17.3620358781311,122.695945873639)) ;
#20213=CARTESIAN_POINT('Ctrl Pts',(-20.6223297569369,17.1820467977682,122.516986010216)) ;
#20214=CARTESIAN_POINT('Ctrl Pts',(-20.4875963394876,17.3718575914632,122.872002282074)) ;
#20215=CARTESIAN_POINT('Ctrl Pts',(-20.7571853342976,17.1918685111003,122.737058592109)) ;
#20216=CARTESIAN_POINT('Ctrl Pts',(-20.565398754166,17.3818925964519,123.068098579527)) ;
#20217=CARTESIAN_POINT('Ctrl Pts',(-20.8544363834582,17.201903516089,122.982179630652)) ;
#20218=CARTESIAN_POINT('Ctrl Pts',(-20.6073560537494,17.3919174348995,123.274640875661)) ;
#20219=CARTESIAN_POINT('Ctrl Pts',(-20.9068811373926,17.2119283545366,123.240357855693)) ;
#20220=CARTESIAN_POINT('Ctrl Pts',(-20.6131626095599,17.4017696478547,123.481683897343)) ;
#20221=CARTESIAN_POINT('Ctrl Pts',(-20.9141373279082,17.2217805674918,123.499162698651)) ;
#20222=CARTESIAN_POINT('Ctrl Pts',(-20.5828638631299,17.4117596040485,123.689490947812)) ;
#20223=CARTESIAN_POINT('Ctrl Pts',(-20.8762617532287,17.2317705236856,123.758921385039)) ;
#20224=CARTESIAN_POINT('Ctrl Pts',(-20.5173607069601,17.4216877143317,123.887673199299)) ;
#20225=CARTESIAN_POINT('Ctrl Pts',(-20.7943806135892,17.2416986339689,124.006649024893)) ;
#20226=CARTESIAN_POINT('Ctrl Pts',(-20.4181341555085,17.4316763144113,124.072748693797)) ;
#20227=CARTESIAN_POINT('Ctrl Pts',(-20.670345385213,17.2516872340484,124.237992487124)) ;
#20228=CARTESIAN_POINT('Ctrl Pts',(-20.2875580116088,17.4417029063388,124.238230031649)) ;
#20229=CARTESIAN_POINT('Ctrl Pts',(-20.5071235397933,17.2617138259759,124.444842800166)) ;
#20230=CARTESIAN_POINT('Ctrl Pts',(-20.1326042864627,17.451588034403,124.376702910318)) ;
#20231=CARTESIAN_POINT('Ctrl Pts',(-20.3134293623449,17.2715989540401,124.617932746978)) ;
#20232=CARTESIAN_POINT('Ctrl Pts',(-19.9543077801982,17.4615791518765,124.487754355148)) ;
#20233=CARTESIAN_POINT('Ctrl Pts',(-20.0905573668405,17.2815900715136,124.756745161351)) ;
#20234=CARTESIAN_POINT('Ctrl Pts',(-19.7583141539382,17.4716197677283,124.566132788164)) ;
#20235=CARTESIAN_POINT('Ctrl Pts',(-19.8455645964301,17.2916306873654,124.854716110604)) ;
#20236=CARTESIAN_POINT('Ctrl Pts',(-19.5560340189507,17.481452758582,124.608731196182)) ;
#20237=CARTESIAN_POINT('Ctrl Pts',(-19.5927130154484,17.3014636782191,124.907962066392)) ;
#20238=CARTESIAN_POINT('Ctrl Pts',(-19.3460857373288,17.4914458900323,124.61627350105)) ;
#20239=CARTESIAN_POINT('Ctrl Pts',(-19.330277450202,17.3114568096694,124.917387511024)) ;
#20240=CARTESIAN_POINT('Ctrl Pts',(-19.1372544365684,17.5014779384677,124.586697623401)) ;
#20241=CARTESIAN_POINT('Ctrl Pts',(-19.0692386893252,17.3214888581048,124.88041535309)) ;
#20242=CARTESIAN_POINT('Ctrl Pts',(-18.9400052555549,17.5113431850101,124.522647715946)) ;
#20243=CARTESIAN_POINT('Ctrl Pts',(-18.822677257513,17.3313541046472,124.800350459875)) ;
#20244=CARTESIAN_POINT('Ctrl Pts',(-18.7547863337693,17.5213050598369,124.424885268183)) ;
#20245=CARTESIAN_POINT('Ctrl Pts',(-18.5911545600622,17.341315979474,124.678145049276)) ;
#20246=CARTESIAN_POINT('Ctrl Pts',(-18.5883681930039,17.5313400229482,124.295243637519)) ;
#20247=CARTESIAN_POINT('Ctrl Pts',(-18.38313341919,17.3513509425853,124.516091097511)) ;
#20248=CARTESIAN_POINT('Ctrl Pts',(-18.4488134106994,17.5412248674106,124.141223324118)) ;
#20249=CARTESIAN_POINT('Ctrl Pts',(-18.2086914290502,17.3612357870477,124.323563591818)) ;
#20250=CARTESIAN_POINT('Ctrl Pts',(-18.3361743130609,17.5512909202513,123.962114608032)) ;
#20251=CARTESIAN_POINT('Ctrl Pts',(-18.0678947666769,17.3713018398884,124.099676485538)) ;
#20252=CARTESIAN_POINT('Ctrl Pts',(-18.2579149300862,17.5611284361603,123.770636276305)) ;
#20253=CARTESIAN_POINT('Ctrl Pts',(-17.9700726313909,17.3811393557974,123.860326944384)) ;
#20254=CARTESIAN_POINT('Ctrl Pts',(-18.2128572603931,17.5711971842692,123.563847910291)) ;
#20255=CARTESIAN_POINT('Ctrl Pts',(-17.9137531151006,17.3912081039063,123.601841075206)) ;
#20256=CARTESIAN_POINT('Ctrl Pts',(-18.2046218359309,17.5810777013002,123.356259866829)) ;
#20257=CARTESIAN_POINT('Ctrl Pts',(-17.9034613928053,17.4010886209373,123.342355402501)) ;
#20258=CARTESIAN_POINT('Ctrl Pts',(-18.2324382002903,17.5910688882346,123.148094680984)) ;
#20259=CARTESIAN_POINT('Ctrl Pts',(-17.9382344928248,17.4110798078718,123.082149155382)) ;
#20260=CARTESIAN_POINT('Ctrl Pts',(-18.2957212303086,17.6010219545096,122.948615518676)) ;
#20261=CARTESIAN_POINT('Ctrl Pts',(-18.0173408799565,17.4210328741467,122.832800782693)) ;
#20262=CARTESIAN_POINT('Ctrl Pts',(-18.3935237813903,17.6110577920422,122.761687553403)) ;
#20263=CARTESIAN_POINT('Ctrl Pts',(-18.1395964065383,17.4310687116793,122.599142062341)) ;
#20264=CARTESIAN_POINT('Ctrl Pts',(-18.5203340583895,17.6209479182536,122.596896263532)) ;
#20265=CARTESIAN_POINT('Ctrl Pts',(-18.2981116221672,17.4409588378907,122.393154239559)) ;
#20266=CARTESIAN_POINT('Ctrl Pts',(-18.6751694912199,17.6309401001616,122.454946682161)) ;
#20267=CARTESIAN_POINT('Ctrl Pts',(-18.4916578231572,17.4509510197987,122.215719190812)) ;
#20268=CARTESIAN_POINT('Ctrl Pts',(-18.8515274887847,17.6408860401002,122.342614062486)) ;
#20269=CARTESIAN_POINT('Ctrl Pts',(-18.7121069676179,17.4608969597373,122.075305569039)) ;
#20270=CARTESIAN_POINT('Ctrl Pts',(-19.0445828832562,17.6508332238642,122.262203190812)) ;
#20271=CARTESIAN_POINT('Ctrl Pts',(-18.9534274542707,17.4708441435014,121.974794440461)) ;
#20272=CARTESIAN_POINT('Ctrl Pts',(-19.2507687647506,17.6608811621717,122.21630679009)) ;
#20273=CARTESIAN_POINT('Ctrl Pts',(-19.211160386698,17.4808920818088,121.917426601221)) ;
#20274=CARTESIAN_POINT('Ctrl Pts',(-19.4575859789318,17.670728796912,122.206920104581)) ;
#20275=CARTESIAN_POINT('Ctrl Pts',(-19.4696824314095,17.4907397165491,121.905695967141)) ;
#20276=CARTESIAN_POINT('Ctrl Pts',(-19.6653420100825,17.6806905108858,122.233242738369)) ;
#20277=CARTESIAN_POINT('Ctrl Pts',(-19.7293772423961,17.5007014305229,121.938602055784)) ;
#20278=CARTESIAN_POINT('Ctrl Pts',(-19.8666582474384,17.6907191456766,122.295917378937)) ;
#20279=CARTESIAN_POINT('Ctrl Pts',(-19.9810217545707,17.5107300653138,122.016948020053)) ;
#20280=CARTESIAN_POINT('Ctrl Pts',(-20.0518343532791,17.7006294642738,122.391384008924)) ;
#20281=CARTESIAN_POINT('Ctrl Pts',(-20.2124907996332,17.5206403839109,122.136283881726)) ;
#20282=CARTESIAN_POINT('Ctrl Pts',(-20.2183778744694,17.7105643205853,122.517438880118)) ;
#20283=CARTESIAN_POINT('Ctrl Pts',(-20.4206686080383,17.5305752402224,122.293854796919)) ;
#20284=CARTESIAN_POINT('Ctrl Pts',(-20.3618650760254,17.720605556546,122.672260820024)) ;
#20285=CARTESIAN_POINT('Ctrl Pts',(-20.6000255828736,17.5406164761831,122.487384162176)) ;
#20286=CARTESIAN_POINT('Ctrl Pts',(-20.4746913192289,17.730492328126,122.846848178747)) ;
#20287=CARTESIAN_POINT('Ctrl Pts',(-20.7410561133952,17.5505032477631,122.70562002418)) ;
#20288=CARTESIAN_POINT('Ctrl Pts',(-20.5566303036143,17.7404925068322,123.040424795211)) ;
#20289=CARTESIAN_POINT('Ctrl Pts',(-20.8434772707178,17.5605034264693,122.947591960567)) ;
#20290=CARTESIAN_POINT('Ctrl Pts',(-20.6035135712802,17.7504097850418,123.243613328282)) ;
#20291=CARTESIAN_POINT('Ctrl Pts',(-20.9020786278622,17.5704207046789,123.201578349681)) ;
#20292=CARTESIAN_POINT('Ctrl Pts',(-20.6144792344301,17.7604570314554,123.454524019583)) ;
#20293=CARTESIAN_POINT('Ctrl Pts',(-20.91578288945,17.5804679510926,123.465216930615)) ;
#20294=CARTESIAN_POINT('Ctrl Pts',(-20.5893156501157,17.7703309204367,123.660606188454)) ;
#20295=CARTESIAN_POINT('Ctrl Pts',(-20.8843256015444,17.5903418400739,123.722819361991)) ;
#20296=CARTESIAN_POINT('Ctrl Pts',(-20.5277259008089,17.7803929380173,123.862949653921)) ;
#20297=CARTESIAN_POINT('Ctrl Pts',(-20.8073356878369,17.6004038576544,123.975747950634)) ;
#20298=CARTESIAN_POINT('Ctrl Pts',(-20.4337117630159,17.7902639997516,124.047969554099)) ;
#20299=CARTESIAN_POINT('Ctrl Pts',(-20.6898154915697,17.6102749193887,124.207021563565)) ;
#20300=CARTESIAN_POINT('Ctrl Pts',(-20.3079243206762,17.8002580631119,124.216261726582)) ;
#20301=CARTESIAN_POINT('Ctrl Pts',(-20.5325789116341,17.620268982749,124.417385133982)) ;
#20302=CARTESIAN_POINT('Ctrl Pts',(-20.1539268427788,17.8102902211453,124.360359874933)) ;
#20303=CARTESIAN_POINT('Ctrl Pts',(-20.3400800616733,17.6303011407824,124.597505830153)) ;
#20304=CARTESIAN_POINT('Ctrl Pts',(-19.9804372227752,17.8201540973854,124.473993821074)) ;
#20305=CARTESIAN_POINT('Ctrl Pts',(-20.1232165512678,17.6401650170226,124.739545873156)) ;
#20306=CARTESIAN_POINT('Ctrl Pts',(-19.7859124945591,17.8302246120237,124.557495151561)) ;
#20307=CARTESIAN_POINT('Ctrl Pts',(-19.8800594521067,17.6502355316608,124.843920027478)) ;
#20308=CARTESIAN_POINT('Ctrl Pts',(-19.5845131324371,17.8400652489647,124.604874841152)) ;
#20309=CARTESIAN_POINT('Ctrl Pts',(-19.6283095577294,17.6600761686018,124.90314183829)) ;
#20310=CARTESIAN_POINT('Ctrl Pts',(-19.3753651784529,17.8500323778049,124.617404469325)) ;
#20311=CARTESIAN_POINT('Ctrl Pts',(-19.366875274711,17.670043297442,124.918801259543)) ;
#20312=CARTESIAN_POINT('Ctrl Pts',(-19.1662372548247,17.8600463509294,124.593093186389)) ;
#20313=CARTESIAN_POINT('Ctrl Pts',(-19.1054626465016,17.6800572705665,124.888408905222)) ;
#20314=CARTESIAN_POINT('Ctrl Pts',(-18.8985829814894,17.8733310847927,124.513236748648)) ;
#20315=CARTESIAN_POINT('Ctrl Pts',(-18.7709105569482,17.6933420044298,124.788587304081)) ;
#20316=CARTESIAN_POINT('Ctrl Pts',(-18.6588816082281,17.8865563495074,124.366233166193)) ;
#20317=CARTESIAN_POINT('Ctrl Pts',(-18.4713115759659,17.7065672691446,124.604860086354)) ;
#20318=CARTESIAN_POINT('Ctrl Pts',(-18.4660643936239,17.8998668720623,124.16345986531)) ;
#20319=CARTESIAN_POINT('Ctrl Pts',(-18.23024753484,17.7198777916994,124.351352544017)) ;
#20320=CARTESIAN_POINT('Ctrl Pts',(-18.3496539207817,17.9098955169645,123.987675168725)) ;
#20321=CARTESIAN_POINT('Ctrl Pts',(-18.0847456433107,17.7299064366016,124.131627885447)) ;
#20322=CARTESIAN_POINT('Ctrl Pts',(-18.2666046768902,17.9197765493184,123.797265561307)) ;
#20323=CARTESIAN_POINT('Ctrl Pts',(-17.9809344252587,17.7397874689555,123.893612632043)) ;
#20324=CARTESIAN_POINT('Ctrl Pts',(-18.2169614950972,17.9297575219985,123.593391497918)) ;
#20325=CARTESIAN_POINT('Ctrl Pts',(-17.9188829813947,17.7497684416356,123.638771587196)) ;
#20326=CARTESIAN_POINT('Ctrl Pts',(-18.203650414156,17.9397386495845,123.383995886292)) ;
#20327=CARTESIAN_POINT('Ctrl Pts',(-17.9022490540845,17.7597495692216,123.377020959202)) ;
#20328=CARTESIAN_POINT('Ctrl Pts',(-18.2339270986067,17.9529818398459,123.107154473442)) ;
#20329=CARTESIAN_POINT('Ctrl Pts',(-17.940086062115,17.772992759483,123.030998917188)) ;
#20330=CARTESIAN_POINT('Ctrl Pts',(-18.3623848961341,17.9696498352067,122.77698011445)) ;
#20331=CARTESIAN_POINT('Ctrl Pts',(-18.1006895820262,17.7896607548438,122.618237447441)) ;
#20332=CARTESIAN_POINT('Ctrl Pts',(-18.5937018814127,17.9861703352187,122.512467682985)) ;
#20333=CARTESIAN_POINT('Ctrl Pts',(-18.3897812209932,17.8061812548558,122.28765824502)) ;
#20334=CARTESIAN_POINT('Ctrl Pts',(-18.8258934089198,17.9994833515347,122.356347563406)) ;
#20335=CARTESIAN_POINT('Ctrl Pts',(-18.6800705190158,17.8194942711718,122.092466331838)) ;
#20336=CARTESIAN_POINT('Ctrl Pts',(-19.0164028181987,18.0093999097677,122.271568361071)) ;
#20337=CARTESIAN_POINT('Ctrl Pts',(-18.9181973224567,17.8294108294048,121.986503440751)) ;
#20338=CARTESIAN_POINT('Ctrl Pts',(-19.2209294726659,18.0194275780706,122.220690420935)) ;
#20339=CARTESIAN_POINT('Ctrl Pts',(-19.1738622433935,17.8394384977077,121.92290647105)) ;
#20340=CARTESIAN_POINT('Ctrl Pts',(-19.4974318665862,18.0326081678152,122.200829010894)) ;
#20341=CARTESIAN_POINT('Ctrl Pts',(-19.5194723945054,17.8526190874524,121.898080551952)) ;
#20342=CARTESIAN_POINT('Ctrl Pts',(-19.8468976293333,18.0493563069346,122.268323420744)) ;
#20343=CARTESIAN_POINT('Ctrl Pts',(-19.9563231936178,17.8693672265717,121.982455382444)) ;
#20344=CARTESIAN_POINT('Ctrl Pts',(-20.208402785875,18.0691510494452,122.484267090907)) ;
#20345=CARTESIAN_POINT('Ctrl Pts',(-20.4081951552472,17.8891619690823,122.252387033747)) ;
#20346=CARTESIAN_POINT('Ctrl Pts',(-20.4779851808533,18.089195442254,122.814181391248)) ;
#20347=CARTESIAN_POINT('Ctrl Pts',(-20.7451718132866,17.9092063618911,122.66478304066)) ;
#20348=CARTESIAN_POINT('Ctrl Pts',(-20.6171002054309,18.1090346245527,123.212537767396)) ;
#20349=CARTESIAN_POINT('Ctrl Pts',(-20.9190608630453,17.9290455441898,123.162728597956)) ;
#20350=CARTESIAN_POINT('Ctrl Pts',(-20.6129501344917,18.1289599482456,123.636081201346)) ;
#20351=CARTESIAN_POINT('Ctrl Pts',(-20.9138698455996,17.9489708678827,123.692157121899)) ;
#20352=CARTESIAN_POINT('Ctrl Pts',(-20.4644170209885,18.1488835862971,124.032892736758)) ;
#20353=CARTESIAN_POINT('Ctrl Pts',(-20.7282004987486,17.9688945059342,124.188169695646)) ;
#20354=CARTESIAN_POINT('Ctrl Pts',(-20.1895488356295,18.1688084597626,124.355214759084)) ;
#20355=CARTESIAN_POINT('Ctrl Pts',(-20.3846133570625,17.9888193793997,124.591069561661)) ;
#20356=CARTESIAN_POINT('Ctrl Pts',(-19.8222522044971,18.1886870668415,124.564420794737)) ;
#20357=CARTESIAN_POINT('Ctrl Pts',(-19.9254924402877,18.0086979864787,124.852574068712)) ;
#20358=CARTESIAN_POINT('Ctrl Pts',(-19.4036094051165,18.2086645096735,124.636282835696)) ;
#20359=CARTESIAN_POINT('Ctrl Pts',(-19.4021887856867,18.0286754293106,124.94239921452)) ;
#20360=CARTESIAN_POINT('Ctrl Pts',(-18.9865333106449,18.2285963577582,124.560840820189)) ;
#20361=CARTESIAN_POINT('Ctrl Pts',(-18.8808448567372,18.0486072773953,124.848094480769)) ;
#20362=CARTESIAN_POINT('Ctrl Pts',(-18.6207574150074,18.2484916261008,124.348382771225)) ;
#20363=CARTESIAN_POINT('Ctrl Pts',(-18.4236271458194,18.0685025457379,124.582520931676)) ;
#20364=CARTESIAN_POINT('Ctrl Pts',(-18.3486814493143,18.2684141245129,124.02368906418)) ;
#20365=CARTESIAN_POINT('Ctrl Pts',(-18.083533966346,18.08842504415,124.176653707817)) ;
#20366=CARTESIAN_POINT('Ctrl Pts',(-18.2035687666535,18.2883736063889,123.62485045441)) ;
#20367=CARTESIAN_POINT('Ctrl Pts',(-17.9021445000866,18.108384526026,123.678105539859)) ;
#20368=CARTESIAN_POINT('Ctrl Pts',(-18.203194006856,18.3082513588482,123.202260983975)) ;
#20369=CARTESIAN_POINT('Ctrl Pts',(-17.901677043034,18.1282622784854,123.149870596743)) ;
#20370=CARTESIAN_POINT('Ctrl Pts',(-18.3459964134725,18.3281331495828,122.804281369069)) ;
#20371=CARTESIAN_POINT('Ctrl Pts',(-18.0801792550787,18.1481440692199,122.65239779122)) ;
#20372=CARTESIAN_POINT('Ctrl Pts',(-18.6191997385848,18.3482064884338,122.476442912359)) ;
#20373=CARTESIAN_POINT('Ctrl Pts',(-18.4216843162061,18.1682174080709,122.242598944837)) ;
#20374=CARTESIAN_POINT('Ctrl Pts',(-18.9830102331295,18.3680109556696,122.264221298364)) ;
#20375=CARTESIAN_POINT('Ctrl Pts',(-18.8764446818162,18.1880218753067,121.977323375824)) ;
#20376=CARTESIAN_POINT('Ctrl Pts',(-19.4008308381281,18.3879942960774,122.187305861743)) ;
#20377=CARTESIAN_POINT('Ctrl Pts',(-19.3987200282656,18.2080052157145,121.881178045719)) ;
#20378=CARTESIAN_POINT('Ctrl Pts',(-19.8183304642668,18.4079092606754,122.258027106077)) ;
#20379=CARTESIAN_POINT('Ctrl Pts',(-19.9205934708167,18.2279201803125,121.969578565073)) ;
#20380=CARTESIAN_POINT('Ctrl Pts',(-20.1864288478707,18.4277777953917,122.465496330421)) ;
#20381=CARTESIAN_POINT('Ctrl Pts',(-20.3807158505364,18.2477887150289,122.228912632756)) ;
#20382=CARTESIAN_POINT('Ctrl Pts',(-20.4635196115804,18.4478301796035,122.789385037709)) ;
#20383=CARTESIAN_POINT('Ctrl Pts',(-20.7270809482803,18.2678410992406,122.6337729235)) ;
#20384=CARTESIAN_POINT('Ctrl Pts',(-20.6120028434724,18.4676041433927,123.182923094544)) ;
#20385=CARTESIAN_POINT('Ctrl Pts',(-20.9126860426018,18.2876150630298,123.125692137824)) ;
#20386=CARTESIAN_POINT('Ctrl Pts',(-20.6176815723447,18.487658522414,123.609124769732)) ;
#20387=CARTESIAN_POINT('Ctrl Pts',(-20.919787056096,18.3076694420512,123.658444810698)) ;
#20388=CARTESIAN_POINT('Ctrl Pts',(-20.4791262983683,18.5074552599873,124.006731982983)) ;
#20389=CARTESIAN_POINT('Ctrl Pts',(-20.7465962162573,18.3274661796244,124.155452562203)) ;
#20390=CARTESIAN_POINT('Ctrl Pts',(-20.2119627746794,18.5274230723387,124.33658343425)) ;
#20391=CARTESIAN_POINT('Ctrl Pts',(-20.4126446942546,18.3474339919759,124.567768827108)) ;
#20392=CARTESIAN_POINT('Ctrl Pts',(-19.8479424439338,18.5473820484038,124.554891666292)) ;
#20393=CARTESIAN_POINT('Ctrl Pts',(-19.9576212451287,18.3673929680409,124.840656736435)) ;
#20394=CARTESIAN_POINT('Ctrl Pts',(-19.4327602934189,18.5672769666812,124.635860460392)) ;
#20395=CARTESIAN_POINT('Ctrl Pts',(-19.4386451944303,18.3872878863183,124.941871042673)) ;
#20396=CARTESIAN_POINT('Ctrl Pts',(-19.0147820526511,18.5871732791315,124.570804620221)) ;
#20397=CARTESIAN_POINT('Ctrl Pts',(-18.9161726453232,18.4071841987686,124.860555263088)) ;
#20398=CARTESIAN_POINT('Ctrl Pts',(-18.6435903312615,18.6070812125056,124.367280330836)) ;
#20399=CARTESIAN_POINT('Ctrl Pts',(-18.4521815633956,18.4270921321427,124.606153931591)) ;
#20400=CARTESIAN_POINT('Ctrl Pts',(-18.3636220458617,18.6270311027941,124.048654042255)) ;
#20401=CARTESIAN_POINT('Ctrl Pts',(-18.1022181077,18.4470420224312,124.207874213592)) ;
#20402=CARTESIAN_POINT('Ctrl Pts',(-18.2093224184274,18.6469083332954,123.655139111936)) ;
#20403=CARTESIAN_POINT('Ctrl Pts',(-17.9093397630461,18.4669192529325,123.715982843254)) ;
#20404=CARTESIAN_POINT('Ctrl Pts',(-18.1982991555925,18.6668910021664,123.230417623875)) ;
#20405=CARTESIAN_POINT('Ctrl Pts',(-17.8955552161801,18.4869019218035,123.185081472576)) ;
#20406=CARTESIAN_POINT('Ctrl Pts',(-18.3328317480087,18.6868238887468,122.828454448446)) ;
#20407=CARTESIAN_POINT('Ctrl Pts',(-18.0637189576036,18.5068348083839,122.682625101242)) ;
#20408=CARTESIAN_POINT('Ctrl Pts',(-18.5959241687473,18.7067366347647,122.496751886595)) ;
#20409=CARTESIAN_POINT('Ctrl Pts',(-18.3925705510188,18.5267475544018,122.267998602716)) ;
#20410=CARTESIAN_POINT('Ctrl Pts',(-18.8956709172905,18.7233063561065,122.311665038351)) ;
#20411=CARTESIAN_POINT('Ctrl Pts',(-18.767281881698,18.5433172757436,122.036622749478)) ;
#20412=CARTESIAN_POINT('Ctrl Pts',(-19.1634796639719,18.7366063674115,122.231169175464)) ;
#20413=CARTESIAN_POINT('Ctrl Pts',(-19.1020056145289,18.5566172870486,121.936011376313)) ;
#20414=CARTESIAN_POINT('Ctrl Pts',(-19.44044901437,18.7498765551614,122.198083479457)) ;
#20415=CARTESIAN_POINT('Ctrl Pts',(-19.4482877506077,18.5698874747985,121.89465138511)) ;
#20416=CARTESIAN_POINT('Ctrl Pts',(-19.7904919604174,18.7665039375268,122.248222801517)) ;
#20417=CARTESIAN_POINT('Ctrl Pts',(-19.8857560482088,18.5865148571639,121.957313792384)) ;
#20418=CARTESIAN_POINT('Ctrl Pts',(-20.1021440207609,18.783126227272,122.414835522395)) ;
#20419=CARTESIAN_POINT('Ctrl Pts',(-20.2753787251303,18.6031371469091,122.165595250357)) ;
#20420=CARTESIAN_POINT('Ctrl Pts',(-20.3055329334675,18.7963714416665,122.605057021473)) ;
#20421=CARTESIAN_POINT('Ctrl Pts',(-20.5295847929134,18.6163823613036,122.403352527217)) ;
#20422=CARTESIAN_POINT('Ctrl Pts',(-20.4311881436849,18.8062834066272,122.771300615763)) ;
#20423=CARTESIAN_POINT('Ctrl Pts',(-20.6866624263127,18.6262943262643,122.611158628173)) ;
#20424=CARTESIAN_POINT('Ctrl Pts',(-20.5272430540412,18.8163420297916,122.959664946299)) ;
#20425=CARTESIAN_POINT('Ctrl Pts',(-20.8067318368115,18.6363529494288,122.846612050245)) ;
#20426=CARTESIAN_POINT('Ctrl Pts',(-20.5880949584386,18.8261821439075,123.157414828597)) ;
#20427=CARTESIAN_POINT('Ctrl Pts',(-20.882799746978,18.6461930635446,123.093798587262)) ;
#20428=CARTESIAN_POINT('Ctrl Pts',(-20.6144765414881,18.8362479288651,123.367346989237)) ;
#20429=CARTESIAN_POINT('Ctrl Pts',(-20.9157793856879,18.6562588485022,123.356213554678)) ;
#20430=CARTESIAN_POINT('Ctrl Pts',(-20.6041033810044,18.846131246653,123.574893561351)) ;
#20431=CARTESIAN_POINT('Ctrl Pts',(-20.9028157443252,18.6661421662901,123.615646798569)) ;
#20432=CARTESIAN_POINT('Ctrl Pts',(-20.557811278042,18.8561206845115,123.779716355101)) ;
#20433=CARTESIAN_POINT('Ctrl Pts',(-20.8449533316139,18.6761316041487,123.871675964814)) ;
#20434=CARTESIAN_POINT('Ctrl Pts',(-20.4767860972541,18.8660843985643,123.972890703501)) ;
#20435=CARTESIAN_POINT('Ctrl Pts',(-20.7436744284095,18.6860953182014,124.113145006398)) ;
#20436=CARTESIAN_POINT('Ctrl Pts',(-20.3632771377155,18.8760794102235,124.149739579038)) ;
#20437=CARTESIAN_POINT('Ctrl Pts',(-20.6017905558508,18.6960903298606,124.334207674781)) ;
#20438=CARTESIAN_POINT('Ctrl Pts',(-20.2199721057436,18.8861157019177,124.304588195844)) ;
#20439=CARTESIAN_POINT('Ctrl Pts',(-20.4226612590053,18.7061266215549,124.527770408748)) ;
#20440=CARTESIAN_POINT('Ctrl Pts',(-20.0553231898177,18.8959620796112,124.430069749636)) ;
#20441=CARTESIAN_POINT('Ctrl Pts',(-20.2168518529892,18.7159729992483,124.684624557531)) ;
#20442=CARTESIAN_POINT('Ctrl Pts',(-19.8690215673185,18.9059470237619,124.526730415756)) ;
#20443=CARTESIAN_POINT('Ctrl Pts',(-19.9839760536042,18.725957943399,124.805452933041)) ;
#20444=CARTESIAN_POINT('Ctrl Pts',(-19.6697047219603,18.9158839948918,124.589408387716)) ;
#20445=CARTESIAN_POINT('Ctrl Pts',(-19.7348307743134,18.735894914529,124.883803103654)) ;
#20446=CARTESIAN_POINT('Ctrl Pts',(-19.4602197023148,18.9259337795236,124.616715999974)) ;
#20447=CARTESIAN_POINT('Ctrl Pts',(-19.4729748038764,18.7459446991607,124.917940423187)) ;
#20448=CARTESIAN_POINT('Ctrl Pts',(-19.2533184450846,18.9357842416011,124.607579273782)) ;
#20449=CARTESIAN_POINT('Ctrl Pts',(-19.21434799551,18.7557951612382,124.906522324717)) ;
#20450=CARTESIAN_POINT('Ctrl Pts',(-19.0485745773188,18.9457562551215,124.562644959168)) ;
#20451=CARTESIAN_POINT('Ctrl Pts',(-18.9584174462669,18.7657671747586,124.850357148989)) ;
#20452=CARTESIAN_POINT('Ctrl Pts',(-18.8542477972193,18.9557514022409,124.482609220366)) ;
#20453=CARTESIAN_POINT('Ctrl Pts',(-18.7155078312172,18.775762321878,124.750315034863)) ;
#20454=CARTESIAN_POINT('Ctrl Pts',(-18.6762610468344,18.965785371977,124.369422704143)) ;
#20455=CARTESIAN_POINT('Ctrl Pts',(-18.493022848757,18.7857962916141,124.608834245128)) ;
#20456=CARTESIAN_POINT('Ctrl Pts',(-18.5231511574649,18.9756409176476,124.229798349696)) ;
#20457=CARTESIAN_POINT('Ctrl Pts',(-18.3016334315015,18.7956518372847,124.434305714712)) ;
#20458=CARTESIAN_POINT('Ctrl Pts',(-18.3945701733205,18.9856396746608,124.063548623651)) ;
#20459=CARTESIAN_POINT('Ctrl Pts',(-18.140904940295,18.8056505942979,124.226495189743)) ;
#20460=CARTESIAN_POINT('Ctrl Pts',(-18.2975958365009,18.995536809898,123.879424723443)) ;
#20461=CARTESIAN_POINT('Ctrl Pts',(-18.019684455447,18.8155477295351,123.99634137885)) ;
#20462=CARTESIAN_POINT('Ctrl Pts',(-18.2330434105871,19.0055899057376,123.678199215092)) ;
#20463=CARTESIAN_POINT('Ctrl Pts',(-17.93899129175,18.8256008253747,123.744810345997)) ;
#20464=CARTESIAN_POINT('Ctrl Pts',(-18.2048687725473,19.0154734144682,123.472321453931)) ;
#20465=CARTESIAN_POINT('Ctrl Pts',(-17.9037702162779,18.8354843341053,123.487463211661)) ;
#20466=CARTESIAN_POINT('Ctrl Pts',(-18.2124671547143,19.0254682871143,123.262341510424)) ;
#20467=CARTESIAN_POINT('Ctrl Pts',(-17.9132654845491,18.8454792067514,123.224988077224)) ;
#20468=CARTESIAN_POINT('Ctrl Pts',(-18.2568443718026,19.03548824875,123.056405743036)) ;
#20469=CARTESIAN_POINT('Ctrl Pts',(-17.9687343278623,18.8554991683871,122.967567757792)) ;
#20470=CARTESIAN_POINT('Ctrl Pts',(-18.3352281082984,19.0453936125498,122.863482475236)) ;
#20471=CARTESIAN_POINT('Ctrl Pts',(-18.0667115840973,18.865404532187,122.726412358638)) ;
#20472=CARTESIAN_POINT('Ctrl Pts',(-18.4459450487129,19.0553342001574,122.686255011705)) ;
#20473=CARTESIAN_POINT('Ctrl Pts',(-18.2051056278125,18.8753451197945,122.504876382137)) ;
#20474=CARTESIAN_POINT('Ctrl Pts',(-18.5865641592456,19.065337018258,122.529862565855)) ;
#20475=CARTESIAN_POINT('Ctrl Pts',(-18.3808775940096,18.8853479378952,122.309383985207)) ;
#20476=CARTESIAN_POINT('Ctrl Pts',(-18.7529137805727,19.0753717299822,122.400141597635)) ;
#20477=CARTESIAN_POINT('Ctrl Pts',(-18.5888129419843,18.8953826496193,122.147230647452)) ;
#20478=CARTESIAN_POINT('Ctrl Pts',(-18.9355927334257,19.0852166367195,122.302823707512)) ;
#20479=CARTESIAN_POINT('Ctrl Pts',(-18.8171608789422,18.9052275563566,122.025580674038)) ;
#20480=CARTESIAN_POINT('Ctrl Pts',(-19.135044952863,19.0952024892885,122.237424139112)) ;
#20481=CARTESIAN_POINT('Ctrl Pts',(-19.066475495053,18.9152134089256,121.943828689904)) ;
#20482=CARTESIAN_POINT('Ctrl Pts',(-19.3418110241518,19.1051372977015,122.207643930743)) ;
#20483=CARTESIAN_POINT('Ctrl Pts',(-19.3249330398174,18.9251482173387,121.906600838846)) ;
#20484=CARTESIAN_POINT('Ctrl Pts',(-19.5531110415552,19.1151948247826,122.214485106709)) ;
#20485=CARTESIAN_POINT('Ctrl Pts',(-19.5890580305708,18.9352057444197,121.915149697282)) ;
#20486=CARTESIAN_POINT('Ctrl Pts',(-19.7552767450465,19.1250164797797,122.256593308277)) ;
#20487=CARTESIAN_POINT('Ctrl Pts',(-19.8417664438443,18.9450273994168,121.967782613312)) ;
#20488=CARTESIAN_POINT('Ctrl Pts',(-19.9517461949997,19.1350725239527,122.334610066435)) ;
#20489=CARTESIAN_POINT('Ctrl Pts',(-20.0873540689241,18.9550834435898,122.065301218056)) ;
#20490=CARTESIAN_POINT('Ctrl Pts',(-20.1294455067056,19.1450132639979,122.44461757867)) ;
#20491=CARTESIAN_POINT('Ctrl Pts',(-20.3094798342934,18.965024183635,122.20280861514)) ;
#20492=CARTESIAN_POINT('Ctrl Pts',(-20.2852002013898,19.1549173850707,122.582803466189)) ;
#20493=CARTESIAN_POINT('Ctrl Pts',(-20.5041752042223,18.9749283047079,122.375539516404)) ;
#20494=CARTESIAN_POINT('Ctrl Pts',(-20.4163570695297,19.164964926225,122.748363557703)) ;
#20495=CARTESIAN_POINT('Ctrl Pts',(-20.6681231446912,18.9849758458621,122.58248803559)) ;
#20496=CARTESIAN_POINT('Ctrl Pts',(-20.5154426781397,19.1748636778254,122.931394298921)) ;
#20497=CARTESIAN_POINT('Ctrl Pts',(-20.7919825435621,18.9948745974625,122.811275811282)) ;
#20498=CARTESIAN_POINT('Ctrl Pts',(-20.5823095621663,19.1849121567912,123.13175874193)) ;
#20499=CARTESIAN_POINT('Ctrl Pts',(-20.8755683816824,19.0049230764283,123.061730492506)) ;
#20500=CARTESIAN_POINT('Ctrl Pts',(-20.6128955919429,19.1947996538749,123.337384367782)) ;
#20501=CARTESIAN_POINT('Ctrl Pts',(-20.9138033739238,19.014810573512,123.318762800787)) ;
#20502=CARTESIAN_POINT('Ctrl Pts',(-20.6076449007628,19.204792744173,123.547386563793)) ;
#20503=CARTESIAN_POINT('Ctrl Pts',(-20.9072423074913,19.0248036638101,123.581265757207)) ;
#20504=CARTESIAN_POINT('Ctrl Pts',(-20.5661040890578,19.2147449142333,123.752459949604)) ;
#20505=CARTESIAN_POINT('Ctrl Pts',(-20.8553184944048,19.0347558338704,123.837608299615)) ;
#20506=CARTESIAN_POINT('Ctrl Pts',(-20.4899691627066,19.2246833341478,123.947015816567)) ;
#20507=CARTESIAN_POINT('Ctrl Pts',(-20.7601517684657,19.0446942537849,124.080804362951)) ;
#20508=CARTESIAN_POINT('Ctrl Pts',(-20.3808817205689,19.2346684642334,124.126388705012)) ;
#20509=CARTESIAN_POINT('Ctrl Pts',(-20.6237942335491,19.0546793838705,124.305021774752)) ;
#20510=CARTESIAN_POINT('Ctrl Pts',(-20.241378136144,19.2447051536475,124.284677346866)) ;
#20511=CARTESIAN_POINT('Ctrl Pts',(-20.4494165139908,19.0647160732846,124.502884010772)) ;
#20512=CARTESIAN_POINT('Ctrl Pts',(-20.0796809670724,19.25455983764,124.414229163885)) ;
#20513=CARTESIAN_POINT('Ctrl Pts',(-20.2472957009717,19.0745707572771,124.664826057112)) ;
#20514=CARTESIAN_POINT('Ctrl Pts',(-19.8954624316429,19.2645593216878,124.515427636075)) ;
#20515=CARTESIAN_POINT('Ctrl Pts',(-20.0170234288064,19.0845702413249,124.791326058903)) ;
#20516=CARTESIAN_POINT('Ctrl Pts',(-19.6985533037412,19.2744544104647,124.582628798739)) ;
#20517=CARTESIAN_POINT('Ctrl Pts',(-19.7708869846679,19.0944653301018,124.875329679388)) ;
#20518=CARTESIAN_POINT('Ctrl Pts',(-19.4895873463579,19.2845149651109,124.615123526839)) ;
#20519=CARTESIAN_POINT('Ctrl Pts',(-19.5096800897201,19.104525884748,124.915950078661)) ;
#20520=CARTESIAN_POINT('Ctrl Pts',(-19.2825491814808,19.2943642294838,124.611047104812)) ;
#20521=CARTESIAN_POINT('Ctrl Pts',(-19.2508813050788,19.1143751491209,124.910856545189)) ;
#20522=CARTESIAN_POINT('Ctrl Pts',(-19.0756100518396,19.3043914819316,124.570889809376)) ;
#20523=CARTESIAN_POINT('Ctrl Pts',(-18.99220707569,19.1244024015687,124.86066175785)) ;
#20524=CARTESIAN_POINT('Ctrl Pts',(-18.8789515708921,19.3144197795018,124.494880706852)) ;
#20525=CARTESIAN_POINT('Ctrl Pts',(-18.7463833099064,19.1344306991389,124.765652294078)) ;
#20526=CARTESIAN_POINT('Ctrl Pts',(-18.701566831824,19.3242659085078,124.388210448307)) ;
#20527=CARTESIAN_POINT('Ctrl Pts',(-18.5246504442198,19.1442768281449,124.632315524006)) ;
#20528=CARTESIAN_POINT('Ctrl Pts',(-18.5427028733491,19.3342598138698,124.250713710067)) ;
#20529=CARTESIAN_POINT('Ctrl Pts',(-18.3260692253604,19.154270733507,124.460445802928)) ;
#20530=CARTESIAN_POINT('Ctrl Pts',(-18.4100146534908,19.3442839115529,124.086985981103)) ;
#20531=CARTESIAN_POINT('Ctrl Pts',(-18.1602075359614,19.16429483119,124.255787351941)) ;
#20532=CARTESIAN_POINT('Ctrl Pts',(-18.3089126305251,19.3541737394069,123.90530352091)) ;
#20533=CARTESIAN_POINT('Ctrl Pts',(-18.0338280399953,19.174184659044,124.028684394348)) ;
#20534=CARTESIAN_POINT('Ctrl Pts',(-18.2399042502461,19.3641657208373,123.706908085251)) ;
#20535=CARTESIAN_POINT('Ctrl Pts',(-17.947565914458,19.1841766404745,123.780690475578)) ;
#20536=CARTESIAN_POINT('Ctrl Pts',(-18.2065905895425,19.3741127256032,123.50046117222)) ;
#20537=CARTESIAN_POINT('Ctrl Pts',(-17.9059220811503,19.1941236452403,123.522631607328)) ;
#20538=CARTESIAN_POINT('Ctrl Pts',(-18.2092454060776,19.384062376993,123.291296502426)) ;
#20539=CARTESIAN_POINT('Ctrl Pts',(-17.9092390395663,19.2040732966301,123.261175270493)) ;
#20540=CARTESIAN_POINT('Ctrl Pts',(-18.2486861191594,19.3940993799704,123.084011953046)) ;
#20541=CARTESIAN_POINT('Ctrl Pts',(-17.958538306793,19.2141102996075,123.002069408009)) ;
#20542=CARTESIAN_POINT('Ctrl Pts',(-18.3222825230277,19.4039882884054,122.889570998935)) ;
#20543=CARTESIAN_POINT('Ctrl Pts',(-18.0505326598567,19.2239992080425,122.759016798404)) ;
#20544=CARTESIAN_POINT('Ctrl Pts',(-18.4292681158825,19.4139776208829,122.708864244681)) ;
#20545=CARTESIAN_POINT('Ctrl Pts',(-18.1842635126106,19.23398854052,122.533132432072)) ;
#20546=CARTESIAN_POINT('Ctrl Pts',(-18.5657022346844,19.42393617632,122.550072619534)) ;
#20547=CARTESIAN_POINT('Ctrl Pts',(-18.3548053010277,19.2439470959571,122.334641591459)) ;
#20548=CARTESIAN_POINT('Ctrl Pts',(-18.7263649466662,19.4338357475205,122.417759602104)) ;
#20549=CARTESIAN_POINT('Ctrl Pts',(-18.5556335270977,19.2538466671576,122.169248739393)) ;
#20550=CARTESIAN_POINT('Ctrl Pts',(-18.9102833479291,19.4438836727725,122.313900274746)) ;
#20551=CARTESIAN_POINT('Ctrl Pts',(-18.7855306745994,19.2638945924096,122.039423510114)) ;
#20552=CARTESIAN_POINT('Ctrl Pts',(-19.1064125465237,19.4537789722985,122.244448286497)) ;
#20553=CARTESIAN_POINT('Ctrl Pts',(-19.0306926009335,19.2737898919356,121.952607002251)) ;
#20554=CARTESIAN_POINT('Ctrl Pts',(-19.3150144344435,19.4638408287464,122.209510718595)) ;
#20555=CARTESIAN_POINT('Ctrl Pts',(-19.2914444276105,19.2838517483836,121.908933829335)) ;
#20556=CARTESIAN_POINT('Ctrl Pts',(-19.521965316198,19.4736846751631,122.211242753843)) ;
#20557=CARTESIAN_POINT('Ctrl Pts',(-19.5501343610573,19.2936955948002,121.911097613413)) ;
#20558=CARTESIAN_POINT('Ctrl Pts',(-19.7280448443102,19.4836476242911,122.248623144845)) ;
#20559=CARTESIAN_POINT('Ctrl Pts',(-19.8077343935755,19.3036585439283,121.957822195286)) ;
#20560=CARTESIAN_POINT('Ctrl Pts',(-19.9258004100159,19.4936816607191,122.322067326375)) ;
#20561=CARTESIAN_POINT('Ctrl Pts',(-20.0549291177178,19.3136925803563,122.049626315006)) ;
#20562=CARTESIAN_POINT('Ctrl Pts',(-20.1052428274456,19.5035690876772,122.426981156448)) ;
#20563=CARTESIAN_POINT('Ctrl Pts',(-20.2792335465816,19.3235800073143,122.18076820435)) ;
#20564=CARTESIAN_POINT('Ctrl Pts',(-20.2660510972554,19.5135835220135,122.562891810069)) ;
#20565=CARTESIAN_POINT('Ctrl Pts',(-20.4802444747173,19.3335944416507,122.350655841088)) ;
#20566=CARTESIAN_POINT('Ctrl Pts',(-20.4006689400157,19.5236184666485,122.725307394749)) ;
#20567=CARTESIAN_POINT('Ctrl Pts',(-20.6485175407954,19.3436293862856,122.553674509814)) ;
#20568=CARTESIAN_POINT('Ctrl Pts',(-20.5034449260328,19.5334508166795,122.90468153521)) ;
#20569=CARTESIAN_POINT('Ctrl Pts',(-20.7769890298325,19.3534617363166,122.777893029322)) ;
#20570=CARTESIAN_POINT('Ctrl Pts',(-20.5752821949681,19.5435262557967,123.10390261523)) ;
#20571=CARTESIAN_POINT('Ctrl Pts',(-20.8667862746344,19.3635371754338,123.026918659849)) ;
#20572=CARTESIAN_POINT('Ctrl Pts',(-20.6107689996992,19.5533787210313,123.308014325579)) ;
#20573=CARTESIAN_POINT('Ctrl Pts',(-20.9111458115105,19.3733896406684,123.282059452494)) ;
#20574=CARTESIAN_POINT('Ctrl Pts',(-20.6104349718264,19.5634515986082,123.519742050673)) ;
#20575=CARTESIAN_POINT('Ctrl Pts',(-20.9107290324318,19.3834625182453,123.546718673386)) ;
#20576=CARTESIAN_POINT('Ctrl Pts',(-20.5741538852815,19.5732941948007,123.723476229926)) ;
#20577=CARTESIAN_POINT('Ctrl Pts',(-20.8653781808651,19.3933051144378,123.801387925564)) ;
#20578=CARTESIAN_POINT('Ctrl Pts',(-20.5027249485285,19.583274578916,123.920753137784)) ;
#20579=CARTESIAN_POINT('Ctrl Pts',(-20.7760923678515,19.4032854985531,124.047984519831)) ;
#20580=CARTESIAN_POINT('Ctrl Pts',(-20.3973703972249,19.5932930595648,124.10312422854)) ;
#20581=CARTESIAN_POINT('Ctrl Pts',(-20.6443997501556,19.4133039792019,124.275948701137)) ;
#20582=CARTESIAN_POINT('Ctrl Pts',(-20.2640988385909,19.6031763745651,124.262563519958)) ;
#20583=CARTESIAN_POINT('Ctrl Pts',(-20.4778099653252,19.4231872942023,124.475248963833)) ;
#20584=CARTESIAN_POINT('Ctrl Pts',(-20.1021786910339,19.6132446716556,124.398835786557)) ;
#20585=CARTESIAN_POINT('Ctrl Pts',(-20.2754104277972,19.4332555912927,124.645589428262)) ;
#20586=CARTESIAN_POINT('Ctrl Pts',(-19.923452222074,19.6230747400279,124.502661288851)) ;
#20587=CARTESIAN_POINT('Ctrl Pts',(-20.0520012191522,19.443085659665,124.775372441285)) ;
#20588=CARTESIAN_POINT('Ctrl Pts',(-19.7249017076277,19.6331415324963,124.575813941918)) ;
#20589=CARTESIAN_POINT('Ctrl Pts',(-19.8038135625138,19.4531524521334,124.86681341649)) ;
#20590=CARTESIAN_POINT('Ctrl Pts',(-19.5202469349877,19.6430308659848,124.612640504371)) ;
#20591=CARTESIAN_POINT('Ctrl Pts',(-19.5479941097252,19.4630417856219,124.912847154411)) ;
#20592=CARTESIAN_POINT('Ctrl Pts',(-19.3100107554735,19.6530329974009,124.613711705916)) ;
#20593=CARTESIAN_POINT('Ctrl Pts',(-19.2851987471319,19.473043917038,124.914186378401)) ;
#20594=CARTESIAN_POINT('Ctrl Pts',(-19.1043078669417,19.6629568670219,124.578660210897)) ;
#20595=CARTESIAN_POINT('Ctrl Pts',(-19.0280693627692,19.482967786659,124.870372052193)) ;
#20596=CARTESIAN_POINT('Ctrl Pts',(-18.9055323179189,19.6730003825391,124.507541988361)) ;
#20597=CARTESIAN_POINT('Ctrl Pts',(-18.7796000674895,19.4930113021762,124.781474531052)) ;
#20598=CARTESIAN_POINT('Ctrl Pts',(-18.7248906132605,19.6828825954274,124.404844874836)) ;
#20599=CARTESIAN_POINT('Ctrl Pts',(-18.5537969176444,19.5028935150645,124.653102676941)) ;
#20600=CARTESIAN_POINT('Ctrl Pts',(-18.5618762979718,19.6929506726468,124.269896713313)) ;
#20601=CARTESIAN_POINT('Ctrl Pts',(-18.3500292628219,19.5129615922839,124.484417808806)) ;
#20602=CARTESIAN_POINT('Ctrl Pts',(-18.42770753592,19.702789177381,124.112435729889)) ;
#20603=CARTESIAN_POINT('Ctrl Pts',(-18.1823173295114,19.5228000970181,124.287590469283)) ;
#20604=CARTESIAN_POINT('Ctrl Pts',(-18.3203002755283,19.7128519458104,123.930208646522)) ;
#20605=CARTESIAN_POINT('Ctrl Pts',(-18.04805852035,19.5328628654475,124.059806889975)) ;
#20606=CARTESIAN_POINT('Ctrl Pts',(-18.2475857905658,19.7227489390931,123.735249596216)) ;
#20607=CARTESIAN_POINT('Ctrl Pts',(-17.9571650618813,19.5427598587302,123.816107138229)) ;
#20608=CARTESIAN_POINT('Ctrl Pts',(-18.2090139650098,19.7326801667279,123.530063285988)) ;
#20609=CARTESIAN_POINT('Ctrl Pts',(-17.9089504191746,19.552691086365,123.559623490826)) ;
#20610=CARTESIAN_POINT('Ctrl Pts',(-18.206860266534,19.74272232537,123.318958748455)) ;
#20611=CARTESIAN_POINT('Ctrl Pts',(-17.9062584823097,19.5627332450072,123.295743025407)) ;
#20612=CARTESIAN_POINT('Ctrl Pts',(-18.2407132566598,19.7526090349011,123.113875533513)) ;
#20613=CARTESIAN_POINT('Ctrl Pts',(-17.9485751372052,19.5726199545382,123.039387974114)) ;
#20614=CARTESIAN_POINT('Ctrl Pts',(-18.3100612563688,19.7626020073297,122.915577612345)) ;
#20615=CARTESIAN_POINT('Ctrl Pts',(-18.035260566707,19.5826129269668,122.791515506251)) ;
#20616=CARTESIAN_POINT('Ctrl Pts',(-18.4123864646547,19.7725482018663,122.733228885072)) ;
#20617=CARTESIAN_POINT('Ctrl Pts',(-18.1631676695922,19.5925591215034,122.563579250553)) ;
#20618=CARTESIAN_POINT('Ctrl Pts',(-18.544466725532,19.7824935767178,122.571123242096)) ;
#20619=CARTESIAN_POINT('Ctrl Pts',(-18.3282687771438,19.6025044963549,122.360947075224)) ;
#20620=CARTESIAN_POINT('Ctrl Pts',(-18.7046124165122,19.7925484960777,122.433182725376)) ;
#20621=CARTESIAN_POINT('Ctrl Pts',(-18.5284509193618,19.6125594157148,122.188521930226)) ;
#20622=CARTESIAN_POINT('Ctrl Pts',(-18.8818996060472,19.8023700155212,122.327286077013)) ;
#20623=CARTESIAN_POINT('Ctrl Pts',(-18.750061582201,19.6223809351583,122.056150769602)) ;
#20624=CARTESIAN_POINT('Ctrl Pts',(-19.0795285112847,19.8124357842881,122.251735177665)) ;
#20625=CARTESIAN_POINT('Ctrl Pts',(-18.9970975872,19.6324467039252,121.961712899097)) ;
#20626=CARTESIAN_POINT('Ctrl Pts',(-19.2839777888797,19.8223377059431,122.212355081407)) ;
#20627=CARTESIAN_POINT('Ctrl Pts',(-19.2526602063055,19.6423486255803,121.912488218236)) ;
#20628=CARTESIAN_POINT('Ctrl Pts',(-19.4950664842811,19.8323807647642,122.208839746125)) ;
#20629=CARTESIAN_POINT('Ctrl Pts',(-19.5165208729935,19.6523916844013,121.908094752818)) ;
#20630=CARTESIAN_POINT('Ctrl Pts',(-19.7007200879061,19.8422867588069,122.241689755879)) ;
#20631=CARTESIAN_POINT('Ctrl Pts',(-19.7735886685139,19.662297678444,121.949158051718)) ;
#20632=CARTESIAN_POINT('Ctrl Pts',(-19.8983711923909,19.8522245318887,122.309384254829)) ;
#20633=CARTESIAN_POINT('Ctrl Pts',(-20.0206528799151,19.6722354515258,122.033777229908)) ;
#20634=CARTESIAN_POINT('Ctrl Pts',(-20.0830422576944,19.862264895621,122.41160883403)) ;
#20635=CARTESIAN_POINT('Ctrl Pts',(-20.2514911587077,19.6822758152581,122.161558568198)) ;
#20636=CARTESIAN_POINT('Ctrl Pts',(-20.2447669194783,19.8721522393445,122.542209039445)) ;
#20637=CARTESIAN_POINT('Ctrl Pts',(-20.4536472526372,19.6921631589816,122.324810150255)) ;
#20638=CARTESIAN_POINT('Ctrl Pts',(-20.383052541564,19.8821444699132,122.700322050731)) ;
#20639=CARTESIAN_POINT('Ctrl Pts',(-20.6265036649569,19.7021553895503,122.522452222942)) ;
#20640=CARTESIAN_POINT('Ctrl Pts',(-20.4912730530166,19.8920929976968,122.879309922931)) ;
#20641=CARTESIAN_POINT('Ctrl Pts',(-20.7617787531808,19.7121039173339,122.746188030278)) ;
#20642=CARTESIAN_POINT('Ctrl Pts',(-20.5669463250774,19.9020297814201,123.074005487427)) ;
#20643=CARTESIAN_POINT('Ctrl Pts',(-20.856369565108,19.7220407010572,122.989558473137)) ;
#20644=CARTESIAN_POINT('Ctrl Pts',(-20.6081237683006,19.912012782217,123.279827787106)) ;
#20645=CARTESIAN_POINT('Ctrl Pts',(-20.9078402627332,19.7320237018542,123.246836830907)) ;
#20646=CARTESIAN_POINT('Ctrl Pts',(-20.6125768739177,19.9220566690578,123.490910400367)) ;
#20647=CARTESIAN_POINT('Ctrl Pts',(-20.9134056044351,19.7420675886949,123.510689929292)) ;
#20648=CARTESIAN_POINT('Ctrl Pts',(-20.5814828811847,19.9318846926323,123.695206220071)) ;
#20649=CARTESIAN_POINT('Ctrl Pts',(-20.8745366916682,19.7518956122695,123.766060949729)) ;
#20650=CARTESIAN_POINT('Ctrl Pts',(-20.5138218279158,19.941961940846,123.895916711096)) ;
#20651=CARTESIAN_POINT('Ctrl Pts',(-20.7899593277774,19.7619728604831,124.016948250578)) ;
#20652=CARTESIAN_POINT('Ctrl Pts',(-20.4147085608249,19.9518114961513,124.077785912975)) ;
#20653=CARTESIAN_POINT('Ctrl Pts',(-20.6660660069028,19.7718224157884,124.244285226899)) ;
#20654=CARTESIAN_POINT('Ctrl Pts',(-20.2825893140887,19.961894204349,124.243476019033)) ;
#20655=CARTESIAN_POINT('Ctrl Pts',(-20.5009161893016,19.7819051239861,124.451396677659)) ;
#20656=CARTESIAN_POINT('Ctrl Pts',(-20.1280154651316,19.9717067972754,124.38015779365)) ;
#20657=CARTESIAN_POINT('Ctrl Pts',(-20.307696830118,19.7917177169126,124.622248846254)) ;
#20658=CARTESIAN_POINT('Ctrl Pts',(-19.9477519695599,19.9817739895334,124.49096411443)) ;
#20659=CARTESIAN_POINT('Ctrl Pts',(-20.0823669714035,19.8017849091705,124.760755273323)) ;
#20660=CARTESIAN_POINT('Ctrl Pts',(-19.7541568951815,19.991672818996,124.56745105753)) ;
#20661=CARTESIAN_POINT('Ctrl Pts',(-19.8403718039497,19.8116837386331,124.856362880226)) ;
#20662=CARTESIAN_POINT('Ctrl Pts',(-19.5471389116745,20.0017268101862,124.609885515152)) ;
#20663=CARTESIAN_POINT('Ctrl Pts',(-19.581599257843,19.8217377298233,124.90940442077)) ;
#20664=CARTESIAN_POINT('Ctrl Pts',(-19.3396458322229,20.0115985349694,124.615811551427)) ;
#20665=CARTESIAN_POINT('Ctrl Pts',(-19.3222318233483,19.8316094546065,124.916810422138)) ;
#20666=CARTESIAN_POINT('Ctrl Pts',(-19.1302124053593,20.0216689770996,124.585074256382)) ;
#20667=CARTESIAN_POINT('Ctrl Pts',(-19.0604406240858,19.8416798967367,124.878387276188)) ;
#20668=CARTESIAN_POINT('Ctrl Pts',(-18.9339520390974,20.0315020555299,124.520082076835)) ;
#20669=CARTESIAN_POINT('Ctrl Pts',(-18.8151144576531,19.851512975167,124.797145106877)) ;
#20670=CARTESIAN_POINT('Ctrl Pts',(-18.7480434856124,20.0415325290313,124.420574067109)) ;
#20671=CARTESIAN_POINT('Ctrl Pts',(-18.5827297027157,19.8615434486684,124.672758530689)) ;
#20672=CARTESIAN_POINT('Ctrl Pts',(-18.5825831311572,20.0515641283299,124.289788081662)) ;
#20673=CARTESIAN_POINT('Ctrl Pts',(-18.3759053294246,19.8715750479671,124.509274829673)) ;
#20674=CARTESIAN_POINT('Ctrl Pts',(-18.4448629357415,20.0613938293681,124.13573633142)) ;
#20675=CARTESIAN_POINT('Ctrl Pts',(-18.2037555511074,19.8814047490052,124.31670801897)) ;
#20676=CARTESIAN_POINT('Ctrl Pts',(-18.3336698872255,20.0713832674246,123.957571401983)) ;
#20677=CARTESIAN_POINT('Ctrl Pts',(-18.0647658072952,19.8913941870617,124.094000670336)) ;
#20678=CARTESIAN_POINT('Ctrl Pts',(-18.2551742977455,20.0814271706407,123.761552123901)) ;
#20679=CARTESIAN_POINT('Ctrl Pts',(-17.9666480383149,19.9014380902778,123.848976044792)) ;
#20680=CARTESIAN_POINT('Ctrl Pts',(-18.2124417079699,20.0912486914542,123.559542282254)) ;
#20681=CARTESIAN_POINT('Ctrl Pts',(-17.9132339251412,19.9112596110913,123.596462120658)) ;
#20682=CARTESIAN_POINT('Ctrl Pts',(-18.2047766515983,20.1012844157013,123.348703573776)) ;
#20683=CARTESIAN_POINT('Ctrl Pts',(-17.9036546813369,19.9212953353384,123.332913768264)) ;
#20684=CARTESIAN_POINT('Ctrl Pts',(-18.2343404621047,20.1113065696338,123.140074801071)) ;
#20685=CARTESIAN_POINT('Ctrl Pts',(-17.9406113337571,19.9313174892709,123.072128085455)) ;
#20686=CARTESIAN_POINT('Ctrl Pts',(-18.2983054280949,20.1211688013911,122.942870332528)) ;
#20687=CARTESIAN_POINT('Ctrl Pts',(-18.0205697573143,19.9411797210282,122.825622198603)) ;
#20688=CARTESIAN_POINT('Ctrl Pts',(-18.3959846631864,20.131127871849,122.757674344572)) ;
#20689=CARTESIAN_POINT('Ctrl Pts',(-18.1426708877126,19.9511387914861,122.594127929803)) ;
#20690=CARTESIAN_POINT('Ctrl Pts',(-18.525566423674,20.1411630442251,122.591200036149)) ;
#20691=CARTESIAN_POINT('Ctrl Pts',(-18.3046496822276,19.9611739638623,122.386036391047)) ;
#20692=CARTESIAN_POINT('Ctrl Pts',(-18.6794843882295,20.1510434293834,122.45168426529)) ;
#20693=CARTESIAN_POINT('Ctrl Pts',(-18.4970491714254,19.9710543490205,122.211642765681)) ;
#20694=CARTESIAN_POINT('Ctrl Pts',(-18.8583463704345,20.1611001439773,122.33899114382)) ;
#20695=CARTESIAN_POINT('Ctrl Pts',(-18.720627652709,19.9811110636145,122.070778322321)) ;
#20696=CARTESIAN_POINT('Ctrl Pts',(-19.0506399135892,20.1709794125494,122.260478579803)) ;
#20697=CARTESIAN_POINT('Ctrl Pts',(-18.960996130641,19.9909903321865,121.972639347132)) ;
#20698=CARTESIAN_POINT('Ctrl Pts',(-19.2558093771799,20.1809703700351,122.21550063428)) ;
#20699=CARTESIAN_POINT('Ctrl Pts',(-19.2174586026876,20.0009812896722,121.916419162101)) ;
#20700=CARTESIAN_POINT('Ctrl Pts',(-19.466736361105,20.1910110286703,122.20725269721)) ;
#20701=CARTESIAN_POINT('Ctrl Pts',(-19.4811173295918,20.0110219483074,121.906111456795)) ;
#20702=CARTESIAN_POINT('Ctrl Pts',(-19.6716056707991,20.2008440083783,122.234820237226)) ;
#20703=CARTESIAN_POINT('Ctrl Pts',(-19.7372046092749,20.0208549280154,121.940573290861)) ;
#20704=CARTESIAN_POINT('Ctrl Pts',(-19.8719676861379,20.210837141628,122.297989647427)) ;
#20705=CARTESIAN_POINT('Ctrl Pts',(-19.9876565139675,20.0308480612651,122.019537420732)) ;
#20706=CARTESIAN_POINT('Ctrl Pts',(-20.0588521291231,20.2208691940113,122.395761902795)) ;
#20707=CARTESIAN_POINT('Ctrl Pts',(-20.2212609501245,20.0408801136485,122.141754795336)) ;
#20708=CARTESIAN_POINT('Ctrl Pts',(-20.2232832799828,20.2307344229627,122.522142243572)) ;
#20709=CARTESIAN_POINT('Ctrl Pts',(-20.4267990069944,20.0507453425998,122.29973257063)) ;
#20710=CARTESIAN_POINT('Ctrl Pts',(-20.3650928807111,20.2406963642059,122.676265084852)) ;
#20711=CARTESIAN_POINT('Ctrl Pts',(-20.6040593213488,20.060707283843,122.492388017739)) ;
#20712=CARTESIAN_POINT('Ctrl Pts',(-20.4785174817246,20.2507310792426,122.854128710168)) ;
#20713=CARTESIAN_POINT('Ctrl Pts',(-20.7458379853386,20.0707419988798,122.71471883926)) ;
#20714=CARTESIAN_POINT('Ctrl Pts',(-20.5584598459099,20.2606168495867,123.045995752101)) ;
#20715=CARTESIAN_POINT('Ctrl Pts',(-20.8457638320152,20.0806277692238,122.954554133205)) ;
#20716=CARTESIAN_POINT('Ctrl Pts',(-20.6046719527906,20.2706794469754,123.252408259714)) ;
#20717=CARTESIAN_POINT('Ctrl Pts',(-20.9035264743855,20.0906903666126,123.212570178599)) ;
#20718=CARTESIAN_POINT('Ctrl Pts',(-20.6142327360248,20.2805298588107,123.459290301903)) ;
#20719=CARTESIAN_POINT('Ctrl Pts',(-20.9154749497781,20.1005407784478,123.471173528851)) ;
#20720=CARTESIAN_POINT('Ctrl Pts',(-20.5877918422668,20.2905570280966,123.668422397058)) ;
#20721=CARTESIAN_POINT('Ctrl Pts',(-20.8824212203225,20.1105679477337,123.732588303383)) ;
#20722=CARTESIAN_POINT('Ctrl Pts',(-20.5249072417576,20.3005845088108,123.869644711752)) ;
#20723=CARTESIAN_POINT('Ctrl Pts',(-20.8038130480593,20.1205954284479,123.984115444725)) ;
#20724=CARTESIAN_POINT('Ctrl Pts',(-20.4301831206918,20.3104275613901,124.053614638865)) ;
#20725=CARTESIAN_POINT('Ctrl Pts',(-20.6854052876472,20.1304384810272,124.214077225316)) ;
#20726=CARTESIAN_POINT('Ctrl Pts',(-20.3034580062551,20.3204214648287,124.221197227413)) ;
#20727=CARTESIAN_POINT('Ctrl Pts',(-20.5269966913248,20.1404323844658,124.423553915828)) ;
#20728=CARTESIAN_POINT('Ctrl Pts',(-20.1487806009657,20.3304485876051,124.364425720184)) ;
#20729=CARTESIAN_POINT('Ctrl Pts',(-20.3336481312429,20.1504595072422,124.602587618317)) ;
#20730=CARTESIAN_POINT('Ctrl Pts',(-19.9741372933805,20.3403392924971,124.477286085174)) ;
#20731=CARTESIAN_POINT('Ctrl Pts',(-20.1153421998912,20.1603502121343,124.743661057522)) ;
#20732=CARTESIAN_POINT('Ctrl Pts',(-19.7807153610016,20.3503313193475,124.559212631353)) ;
#20733=CARTESIAN_POINT('Ctrl Pts',(-19.873563628878,20.1703422389846,124.846066786522)) ;
#20734=CARTESIAN_POINT('Ctrl Pts',(-19.5769304517105,20.360277300836,124.606034161387)) ;
#20735=CARTESIAN_POINT('Ctrl Pts',(-19.618831660715,20.1802882204731,124.904591118333)) ;
#20736=CARTESIAN_POINT('Ctrl Pts',(-19.3680954416651,20.3702244734579,124.617184177661)) ;
#20737=CARTESIAN_POINT('Ctrl Pts',(-19.3577875500338,20.190235393095,124.918525903528)) ;
#20738=CARTESIAN_POINT('Ctrl Pts',(-19.1584407875054,20.3802724147841,124.591416106205)) ;
#20739=CARTESIAN_POINT('Ctrl Pts',(-19.0957195762214,20.2002833344212,124.886313111744)) ;
#20740=CARTESIAN_POINT('Ctrl Pts',(-18.9604121411015,20.3901200485918,124.531032969309)) ;
#20741=CARTESIAN_POINT('Ctrl Pts',(-18.8481841830687,20.210130968229,124.810831448379)) ;
#20742=CARTESIAN_POINT('Ctrl Pts',(-18.7734517586268,20.4000817632769,124.436686230099)) ;
#20743=CARTESIAN_POINT('Ctrl Pts',(-18.6144848557031,20.220092682914,124.692895466025)) ;
#20744=CARTESIAN_POINT('Ctrl Pts',(-18.604728389867,20.4101103961554,124.310240172556)) ;
#20745=CARTESIAN_POINT('Ctrl Pts',(-18.4035822760522,20.2301213157925,124.534835645106)) ;
#20746=CARTESIAN_POINT('Ctrl Pts',(-18.4621885899076,20.4200207216905,124.158296132863)) ;
#20747=CARTESIAN_POINT('Ctrl Pts',(-18.2254094105789,20.2400316413277,124.34490354003)) ;
#20748=CARTESIAN_POINT('Ctrl Pts',(-18.3474529168086,20.4299555521623,123.983766306947)) ;
#20749=CARTESIAN_POINT('Ctrl Pts',(-18.0819921054121,20.2499664717994,124.126739575367)) ;
#20750=CARTESIAN_POINT('Ctrl Pts',(-18.2640446601778,20.4399968845442,123.789842819283)) ;
#20751=CARTESIAN_POINT('Ctrl Pts',(-17.9777343205273,20.2600078041814,123.884334153632)) ;
#20752=CARTESIAN_POINT('Ctrl Pts',(-18.21621844815,20.4498897579831,123.587439108983)) ;
#20753=CARTESIAN_POINT('Ctrl Pts',(-17.9179543452334,20.2699006776202,123.631328380915)) ;
#20754=CARTESIAN_POINT('Ctrl Pts',(-18.203638204828,20.459858923801,123.378224162259)) ;
#20755=CARTESIAN_POINT('Ctrl Pts',(-17.9022315156781,20.2798698434381,123.369810686241)) ;
#20756=CARTESIAN_POINT('Ctrl Pts',(-18.2280625767773,20.4698876575175,123.168828358653)) ;
#20757=CARTESIAN_POINT('Ctrl Pts',(-17.9327660607719,20.2898985771546,123.108061591331)) ;
#20758=CARTESIAN_POINT('Ctrl Pts',(-18.3069889150334,20.4830801762886,122.902870280924)) ;
#20759=CARTESIAN_POINT('Ctrl Pts',(-18.0314212956118,20.3030910959258,122.775637805959)) ;
#20760=CARTESIAN_POINT('Ctrl Pts',(-18.4552942626579,20.4964400443313,122.660681326423)) ;
#20761=CARTESIAN_POINT('Ctrl Pts',(-18.2167817772954,20.3164509639684,122.472918789065)) ;
#20762=CARTESIAN_POINT('Ctrl Pts',(-18.657015951964,20.5096653814802,122.469309191778)) ;
#20763=CARTESIAN_POINT('Ctrl Pts',(-18.4689719567282,20.3296763011173,122.233665328807)) ;
#20764=CARTESIAN_POINT('Ctrl Pts',(-18.8316741273677,20.5196466073208,122.353005072726)) ;
#20765=CARTESIAN_POINT('Ctrl Pts',(-18.6872891439649,20.3396575269579,122.0882957323)) ;
#20766=CARTESIAN_POINT('Ctrl Pts',(-19.0250769115555,20.5296821743037,122.268720045023)) ;
#20767=CARTESIAN_POINT('Ctrl Pts',(-18.9290457583576,20.3496930939408,121.982939786469)) ;
#20768=CARTESIAN_POINT('Ctrl Pts',(-19.2265825671295,20.5395452522658,122.219728041552)) ;
#20769=CARTESIAN_POINT('Ctrl Pts',(-19.1809279027677,20.3595561719029,121.921703115503)) ;
#20770=CARTESIAN_POINT('Ctrl Pts',(-19.4378331047405,20.5496155510669,122.206147359895)) ;
#20771=CARTESIAN_POINT('Ctrl Pts',(-19.4449915418395,20.369626470704,121.904729894139)) ;
#20772=CARTESIAN_POINT('Ctrl Pts',(-19.6434998813334,20.5594578496347,122.228940856017)) ;
#20773=CARTESIAN_POINT('Ctrl Pts',(-19.7020745055463,20.3794687692718,121.933224576347)) ;
#20774=CARTESIAN_POINT('Ctrl Pts',(-19.8446762990893,20.5694185478045,122.287051453372)) ;
#20775=CARTESIAN_POINT('Ctrl Pts',(-19.9535442296739,20.3894294674416,122.005865433082)) ;
#20776=CARTESIAN_POINT('Ctrl Pts',(-20.0339789138857,20.579456581984,122.380301038949)) ;
#20777=CARTESIAN_POINT('Ctrl Pts',(-20.1901714045228,20.3994675016211,122.122429978516)) ;
#20778=CARTESIAN_POINT('Ctrl Pts',(-20.2016869726508,20.5893303188304,122.50266789996)) ;
#20779=CARTESIAN_POINT('Ctrl Pts',(-20.3998046709007,20.4093412384676,122.275390622965)) ;
#20780=CARTESIAN_POINT('Ctrl Pts',(-20.3484287632797,20.5994021027557,122.65527287763)) ;
#20781=CARTESIAN_POINT('Ctrl Pts',(-20.5832300951106,20.4194130223928,122.466148916955)) ;
#20782=CARTESIAN_POINT('Ctrl Pts',(-20.4637684790007,20.6092342239569,122.82682741127)) ;
#20783=CARTESIAN_POINT('Ctrl Pts',(-20.7274022481108,20.429245143594,122.680593266604)) ;
#20784=CARTESIAN_POINT('Ctrl Pts',(-20.549786388294,20.6192672479823,123.019405571818)) ;
#20785=CARTESIAN_POINT('Ctrl Pts',(-20.83492227229,20.4392781676194,122.921317142792)) ;
#20786=CARTESIAN_POINT('Ctrl Pts',(-20.600454739304,20.629283128179,123.223797814881)) ;
#20787=CARTESIAN_POINT('Ctrl Pts',(-20.8982551027824,20.4492940478161,123.176808341218)) ;
#20788=CARTESIAN_POINT('Ctrl Pts',(-20.6150583626326,20.6391666472732,123.431067002261)) ;
#20789=CARTESIAN_POINT('Ctrl Pts',(-20.9165069215087,20.4591775669103,123.435894221683)) ;
#20790=CARTESIAN_POINT('Ctrl Pts',(-20.5934884418527,20.6491570596368,123.639971139436)) ;
#20791=CARTESIAN_POINT('Ctrl Pts',(-20.8895420040221,20.469167979274,123.697025786576)) ;
#20792=CARTESIAN_POINT('Ctrl Pts',(-20.5172126026985,20.6624202228403,123.908195883155)) ;
#20793=CARTESIAN_POINT('Ctrl Pts',(-20.7941934591565,20.4824311424774,124.032297261989)) ;
#20794=CARTESIAN_POINT('Ctrl Pts',(-20.3727499039758,20.6756977930915,124.150760947289)) ;
#20795=CARTESIAN_POINT('Ctrl Pts',(-20.61364497499,20.4957087127286,124.335469275498)) ;
#20796=CARTESIAN_POINT('Ctrl Pts',(-20.1718067412588,20.6890280955981,124.346077378148)) ;
#20797=CARTESIAN_POINT('Ctrl Pts',(-20.3624251620307,20.5090390152352,124.579659196355)) ;
#20798=CARTESIAN_POINT('Ctrl Pts',(-19.9998354457734,20.6989267774145,124.463273965374)) ;
#20799=CARTESIAN_POINT('Ctrl Pts',(-20.1474678125217,20.5189376970516,124.726143222167)) ;
#20800=CARTESIAN_POINT('Ctrl Pts',(-19.8085029004183,20.708916292462,124.549834225346)) ;
#20801=CARTESIAN_POINT('Ctrl Pts',(-19.9082988338251,20.5289272120991,124.834343756603)) ;
#20802=CARTESIAN_POINT('Ctrl Pts',(-19.6058699471084,20.718864344237,124.601638834298)) ;
#20803=CARTESIAN_POINT('Ctrl Pts',(-19.6550087594271,20.5388752638742,124.899096739163)) ;
#20804=CARTESIAN_POINT('Ctrl Pts',(-19.3975069469639,20.7288057475155,124.617723893743)) ;
#20805=CARTESIAN_POINT('Ctrl Pts',(-19.3945515389815,20.5488166671527,124.919199688652)) ;
#20806=CARTESIAN_POINT('Ctrl Pts',(-19.1194310874959,20.7420924122965,124.5908661902)) ;
#20807=CARTESIAN_POINT('Ctrl Pts',(-19.0469745337114,20.5621033319336,124.885630332357)) ;
#20808=CARTESIAN_POINT('Ctrl Pts',(-18.7886547609525,20.7587028339513,124.467201444823)) ;
#20809=CARTESIAN_POINT('Ctrl Pts',(-18.6334863377988,20.5787137535884,124.731039345078)) ;
#20810=CARTESIAN_POINT('Ctrl Pts',(-18.4662665698674,20.7786140962021,124.192751228819)) ;
#20811=CARTESIAN_POINT('Ctrl Pts',(-18.2305106418667,20.5986250158392,124.387975748647)) ;
#20812=CARTESIAN_POINT('Ctrl Pts',(-18.2563995968813,20.7985582253669,123.82423191738)) ;
#20813=CARTESIAN_POINT('Ctrl Pts',(-17.9681790722083,20.6185691450041,123.927324296484)) ;
#20814=CARTESIAN_POINT('Ctrl Pts',(-18.1850241779996,20.8184813879721,123.406707624286)) ;
#20815=CARTESIAN_POINT('Ctrl Pts',(-17.8789643904274,20.6384923076093,123.405418987404)) ;
#20816=CARTESIAN_POINT('Ctrl Pts',(-18.2596109544151,20.8383715103787,122.990352378829)) ;
#20817=CARTESIAN_POINT('Ctrl Pts',(-17.9722011638597,20.6583824300158,122.884976490813)) ;
#20818=CARTESIAN_POINT('Ctrl Pts',(-18.4732404987063,20.8583764639788,122.622607393527)) ;
#20819=CARTESIAN_POINT('Ctrl Pts',(-18.2392413285999,20.6783873836159,122.425297035635)) ;
#20820=CARTESIAN_POINT('Ctrl Pts',(-18.7967167999957,20.8782147209944,122.351758323974)) ;
#20821=CARTESIAN_POINT('Ctrl Pts',(-18.6435876221089,20.6982256406315,122.086739272797)) ;
#20822=CARTESIAN_POINT('Ctrl Pts',(-19.1960471170997,20.8982090217809,122.206055805286)) ;
#20823=CARTESIAN_POINT('Ctrl Pts',(-19.1427514572152,20.718219941418,121.904613931299)) ;
#20824=CARTESIAN_POINT('Ctrl Pts',(-19.6188717893715,20.9180942638254,122.205753928318)) ;
#20825=CARTESIAN_POINT('Ctrl Pts',(-19.6712810445263,20.7381051834625,121.904239572849)) ;
#20826=CARTESIAN_POINT('Ctrl Pts',(-20.0166066720332,20.9379692103013,122.348559948617)) ;
#20827=CARTESIAN_POINT('Ctrl Pts',(-20.168447470455,20.7579801299384,122.082748587511)) ;
#20828=CARTESIAN_POINT('Ctrl Pts',(-20.3441382460836,20.9580022802424,122.620951616946)) ;
#20829=CARTESIAN_POINT('Ctrl Pts',(-20.5778609764888,20.7780131998795,122.423240113376)) ;
#20830=CARTESIAN_POINT('Ctrl Pts',(-20.5570102326951,20.9778907871428,122.986308371611)) ;
#20831=CARTESIAN_POINT('Ctrl Pts',(-20.8439482662448,20.7979017067799,122.879935963145)) ;
#20832=CARTESIAN_POINT('Ctrl Pts',(-20.6337603887322,20.9977456469241,123.401507209435)) ;
#20833=CARTESIAN_POINT('Ctrl Pts',(-20.9398845189848,20.8177565665612,123.398932664504)) ;
#20834=CARTESIAN_POINT('Ctrl Pts',(-20.5628715307167,21.0177964807118,123.821804823539)) ;
#20835=CARTESIAN_POINT('Ctrl Pts',(-20.8512719992327,20.8378074003489,123.924305207163)) ;
#20836=CARTESIAN_POINT('Ctrl Pts',(-20.356096985501,21.037562422601,124.187831810963)) ;
#20837=CARTESIAN_POINT('Ctrl Pts',(-20.5928049104702,20.8575733422382,124.381835472892)) ;
#20838=CARTESIAN_POINT('Ctrl Pts',(-20.0335794669859,21.0575751540604,124.465226345288)) ;
#20839=CARTESIAN_POINT('Ctrl Pts',(-20.1896580437569,20.8775860736975,124.728578782344)) ;
#20840=CARTESIAN_POINT('Ctrl Pts',(-19.637720643514,21.0774679890039,124.614558860712)) ;
#20841=CARTESIAN_POINT('Ctrl Pts',(-19.6948360554275,20.8974789086411,124.915243821142)) ;
#20842=CARTESIAN_POINT('Ctrl Pts',(-19.214589507988,21.0973750123435,124.620545648609)) ;
#20843=CARTESIAN_POINT('Ctrl Pts',(-19.1659236264529,20.9173859319806,124.922728039924)) ;
#20844=CARTESIAN_POINT('Ctrl Pts',(-18.8142996405734,21.1172902772442,124.482107958723)) ;
#20845=CARTESIAN_POINT('Ctrl Pts',(-18.6655619227043,20.9373011968813,124.749682544139)) ;
#20846=CARTESIAN_POINT('Ctrl Pts',(-18.4838027384896,21.1373219694039,124.213487981599)) ;
#20847=CARTESIAN_POINT('Ctrl Pts',(-18.2524397020174,20.957332889041,124.413908184194)) ;
#20848=CARTESIAN_POINT('Ctrl Pts',(-18.2668088815555,21.1571650159769,123.851596586135)) ;
#20849=CARTESIAN_POINT('Ctrl Pts',(-17.9811972981208,20.977175935614,123.961546540794)) ;
#20850=CARTESIAN_POINT('Ctrl Pts',(-18.1851023806558,21.1770815638767,123.436137199122)) ;
#20851=CARTESIAN_POINT('Ctrl Pts',(-17.8790621516814,20.9970924835138,123.442223784006)) ;
#20852=CARTESIAN_POINT('Ctrl Pts',(-18.2502145798426,21.197013806868,123.017317548737)) ;
#20853=CARTESIAN_POINT('Ctrl Pts',(-17.9604499278885,21.0170247265051,122.918699625149)) ;
#20854=CARTESIAN_POINT('Ctrl Pts',(-18.453820244144,21.2169176416773,122.646330539081)) ;
#20855=CARTESIAN_POINT('Ctrl Pts',(-18.2149540834011,21.0369285613144,122.454965536719)) ;
#20856=CARTESIAN_POINT('Ctrl Pts',(-18.771411200767,21.2368180418648,122.366728476114)) ;
#20857=CARTESIAN_POINT('Ctrl Pts',(-18.6119399166127,21.0568289615019,122.105461255144)) ;
#20858=CARTESIAN_POINT('Ctrl Pts',(-19.1662802143597,21.2567677182441,122.211733257638)) ;
#20859=CARTESIAN_POINT('Ctrl Pts',(-19.1055245267092,21.0767786378812,121.91171422936)) ;
#20860=CARTESIAN_POINT('Ctrl Pts',(-19.5899666832492,21.2767002424645,122.200890341999)) ;
#20861=CARTESIAN_POINT('Ctrl Pts',(-19.6351319246211,21.0967111621016,121.898157078062)) ;
#20862=CARTESIAN_POINT('Ctrl Pts',(-19.9918071979918,21.2966202514507,122.334860446379)) ;
#20863=CARTESIAN_POINT('Ctrl Pts',(-20.1374331359232,21.1166311710878,122.065615887878)) ;
#20864=CARTESIAN_POINT('Ctrl Pts',(-20.3243261883736,21.3165771576268,122.598408286184)) ;
#20865=CARTESIAN_POINT('Ctrl Pts',(-20.5530840765956,21.136588077264,122.395047352195)) ;
#20866=CARTESIAN_POINT('Ctrl Pts',(-20.5465500206849,21.3364629971283,122.958223520543)) ;
#20867=CARTESIAN_POINT('Ctrl Pts',(-20.8308668599276,21.1564739167655,122.844813593085)) ;
#20868=CARTESIAN_POINT('Ctrl Pts',(-20.6329313729834,21.3564341692642,123.373889795751)) ;
#20869=CARTESIAN_POINT('Ctrl Pts',(-20.9388483133597,21.1764450889013,123.364394953387)) ;
#20870=CARTESIAN_POINT('Ctrl Pts',(-20.5733172895036,21.3762483662486,123.791020354018)) ;
#20871=CARTESIAN_POINT('Ctrl Pts',(-20.8643333248033,21.1962592858857,123.885809151916)) ;
#20872=CARTESIAN_POINT('Ctrl Pts',(-20.3738339937494,21.3962295522168,124.166047638378)) ;
#20873=CARTESIAN_POINT('Ctrl Pts',(-20.6149914724651,21.2162404718539,124.35458992427)) ;
#20874=CARTESIAN_POINT('Ctrl Pts',(-20.1119197884198,21.4128050576061,124.401919568806)) ;
#20875=CARTESIAN_POINT('Ctrl Pts',(-20.2875771231592,21.2328159772432,124.649450004713)) ;
#20876=CARTESIAN_POINT('Ctrl Pts',(-19.8627851378671,21.4261145054697,124.529357888635)) ;
#20877=CARTESIAN_POINT('Ctrl Pts',(-19.976190695121,21.2461254251068,124.808734121278)) ;
#20878=CARTESIAN_POINT('Ctrl Pts',(-19.5941578117551,21.4394822032463,124.611771760159)) ;
#20879=CARTESIAN_POINT('Ctrl Pts',(-19.6403422561752,21.2594931228834,124.911767929916)) ;
#20880=CARTESIAN_POINT('Ctrl Pts',(-19.2437108626746,21.4559727749122,124.6246956008)) ;
#20881=CARTESIAN_POINT('Ctrl Pts',(-19.2023540010426,21.2759836945493,124.927912591737)) ;
#20882=CARTESIAN_POINT('Ctrl Pts',(-18.8402511753296,21.475893047245,124.495996346843)) ;
#20883=CARTESIAN_POINT('Ctrl Pts',(-18.6980130161789,21.2959039668821,124.76705541604)) ;
#20884=CARTESIAN_POINT('Ctrl Pts',(-18.5605799960303,21.492510082966,124.28007609183)) ;
#20885=CARTESIAN_POINT('Ctrl Pts',(-18.3484015779916,21.3125210026031,124.497134075246)) ;
#20886=CARTESIAN_POINT('Ctrl Pts',(-18.3909714744252,21.5058009332471,124.057970104108)) ;
#20887=CARTESIAN_POINT('Ctrl Pts',(-18.1364098503999,21.3258118528842,124.219524949621)) ;
#20888=CARTESIAN_POINT('Ctrl Pts',(-18.2945586514006,21.5157699784016,123.871912739408)) ;
#20889=CARTESIAN_POINT('Ctrl Pts',(-18.0158871388316,21.3357808980387,123.986950081581)) ;
#20890=CARTESIAN_POINT('Ctrl Pts',(-18.2319181244892,21.5256733690351,123.673331471138)) ;
#20891=CARTESIAN_POINT('Ctrl Pts',(-17.9375848219816,21.3456842886722,123.7387264045)) ;
#20892=CARTESIAN_POINT('Ctrl Pts',(-18.2044053248853,21.5357311551478,123.46370878248)) ;
#20893=CARTESIAN_POINT('Ctrl Pts',(-17.9031917373362,21.355742074785,123.476694986446)) ;
#20894=CARTESIAN_POINT('Ctrl Pts',(-18.213339943562,21.5455831917976,123.256751493961)) ;
#20895=CARTESIAN_POINT('Ctrl Pts',(-17.9143537185253,21.3655941114347,123.218009520766)) ;
#20896=CARTESIAN_POINT('Ctrl Pts',(-18.2735424653214,21.5589483159408,122.982353800711)) ;
#20897=CARTESIAN_POINT('Ctrl Pts',(-17.9896212280947,21.3789592355779,122.874956968011)) ;
#20898=CARTESIAN_POINT('Ctrl Pts',(-18.4029674767116,21.5721743789038,122.732632420697)) ;
#20899=CARTESIAN_POINT('Ctrl Pts',(-18.1513956643206,21.3921852985409,122.562838107837)) ;
#20900=CARTESIAN_POINT('Ctrl Pts',(-18.5911529593693,21.5854780271861,122.525730956398)) ;
#20901=CARTESIAN_POINT('Ctrl Pts',(-18.3866109363659,21.4054889468232,122.304222180962)) ;
#20902=CARTESIAN_POINT('Ctrl Pts',(-18.7572783870989,21.5954695583491,122.397143887496)) ;
#20903=CARTESIAN_POINT('Ctrl Pts',(-18.5942688365872,21.4154804779862,122.143483381919)) ;
#20904=CARTESIAN_POINT('Ctrl Pts',(-18.9441977840221,21.6055090061484,122.299154895599)) ;
#20905=CARTESIAN_POINT('Ctrl Pts',(-18.8279161165822,21.4255199257855,122.020995347853)) ;
#20906=CARTESIAN_POINT('Ctrl Pts',(-19.1413056725189,21.6153527816622,122.236053528025)) ;
#20907=CARTESIAN_POINT('Ctrl Pts',(-19.0743002770801,21.4353637012994,121.942115783865)) ;
#20908=CARTESIAN_POINT('Ctrl Pts',(-19.3492278326637,21.6253384230499,122.207322375982)) ;
#20909=CARTESIAN_POINT('Ctrl Pts',(-19.3342026170286,21.445349342687,121.90619908811)) ;
#20910=CARTESIAN_POINT('Ctrl Pts',(-19.5580238062598,21.6352752074117,122.21497981521)) ;
#20911=CARTESIAN_POINT('Ctrl Pts',(-19.5951977714836,21.4552861270488,121.915768063468)) ;
#20912=CARTESIAN_POINT('Ctrl Pts',(-19.7645659584739,21.645325041879,122.259368244298)) ;
#20913=CARTESIAN_POINT('Ctrl Pts',(-19.8533761099886,21.4653359615162,121.971250859302)) ;
#20914=CARTESIAN_POINT('Ctrl Pts',(-19.9564732011589,21.6551754913822,122.337234509043)) ;
#20915=CARTESIAN_POINT('Ctrl Pts',(-20.0932613278945,21.4751864110193,122.068581121297)) ;
#20916=CARTESIAN_POINT('Ctrl Pts',(-20.1343652145138,21.6651475053643,122.448110905834)) ;
#20917=CARTESIAN_POINT('Ctrl Pts',(-20.3156279272745,21.4851584250014,122.207174295959)) ;
#20918=CARTESIAN_POINT('Ctrl Pts',(-20.2906914128935,21.6751426632114,122.588577277018)) ;
#20919=CARTESIAN_POINT('Ctrl Pts',(-20.5110376061981,21.4951535828485,122.382755229701)) ;
#20920=CARTESIAN_POINT('Ctrl Pts',(-20.4205236147211,21.6851765895751,122.754811362263)) ;
#20921=CARTESIAN_POINT('Ctrl Pts',(-20.6733301023097,21.5051875092122,122.590546133602)) ;
#20922=CARTESIAN_POINT('Ctrl Pts',(-20.5180643029118,21.6950322980075,122.937635457501)) ;
#20923=CARTESIAN_POINT('Ctrl Pts',(-20.7952585397872,21.5150432176446,122.819075138393)) ;
#20924=CARTESIAN_POINT('Ctrl Pts',(-20.5835791686227,21.7050304473461,123.137322140165)) ;
#20925=CARTESIAN_POINT('Ctrl Pts',(-20.8771547988309,21.5250413669833,123.068682710145)) ;
#20926=CARTESIAN_POINT('Ctrl Pts',(-20.6133259213828,21.7149298505197,123.343332794389)) ;
#20927=CARTESIAN_POINT('Ctrl Pts',(-20.9143410126104,21.5349407701568,123.326195883179)) ;
#20928=CARTESIAN_POINT('Ctrl Pts',(-20.6067986597741,21.7249810474082,123.554517472211)) ;
#20929=CARTESIAN_POINT('Ctrl Pts',(-20.9061846999684,21.5449919670453,123.590176807784)) ;
#20930=CARTESIAN_POINT('Ctrl Pts',(-20.5644486467122,21.734863371221,123.757928803125)) ;
#20931=CARTESIAN_POINT('Ctrl Pts',(-20.853249823519,21.5548742908582,123.844441837906)) ;
#20932=CARTESIAN_POINT('Ctrl Pts',(-20.4869932248377,21.7448582668776,123.953249465948)) ;
#20933=CARTESIAN_POINT('Ctrl Pts',(-20.7564330306425,21.5648691865148,124.088593766656)) ;
#20934=CARTESIAN_POINT('Ctrl Pts',(-20.376239486151,21.7548793662602,124.132475484503)) ;
#20935=CARTESIAN_POINT('Ctrl Pts',(-20.6179931768872,21.5748902858973,124.312627761359)) ;
#20936=CARTESIAN_POINT('Ctrl Pts',(-20.2377724390061,21.7647866341222,124.288062190397)) ;
#20937=CARTESIAN_POINT('Ctrl Pts',(-20.4449112034606,21.5847975537594,124.507113190861)) ;
#20938=CARTESIAN_POINT('Ctrl Pts',(-20.0741502835799,21.7747249779475,124.417970243514)) ;
#20939=CARTESIAN_POINT('Ctrl Pts',(-20.2403849662515,21.5947358975846,124.669500522451)) ;
#20940=CARTESIAN_POINT('Ctrl Pts',(-19.8892850130631,21.784728397248,124.518280702167)) ;
#20941=CARTESIAN_POINT('Ctrl Pts',(-20.0093045735368,21.6047393168851,124.79489097273)) ;
#20942=CARTESIAN_POINT('Ctrl Pts',(-19.6891120590807,21.7947629479551,124.584833460336)) ;
#20943=CARTESIAN_POINT('Ctrl Pts',(-19.7590892507398,21.6147738675922,124.878084487071)) ;
#20944=CARTESIAN_POINT('Ctrl Pts',(-19.484395225653,21.8046078975607,124.615389634734)) ;
#20945=CARTESIAN_POINT('Ctrl Pts',(-19.5031930456652,21.6246188171978,124.916282417656)) ;
#20946=CARTESIAN_POINT('Ctrl Pts',(-19.2745575619711,21.8145937396736,124.610253310873)) ;
#20947=CARTESIAN_POINT('Ctrl Pts',(-19.2408957415365,21.6346046593107,124.909864611199)) ;
#20948=CARTESIAN_POINT('Ctrl Pts',(-19.0697507053397,21.8245285470427,124.569104542372)) ;
#20949=CARTESIAN_POINT('Ctrl Pts',(-18.9848863453834,21.6445394666798,124.858431106566)) ;
#20950=CARTESIAN_POINT('Ctrl Pts',(-18.8729297754626,21.834586088756,124.491928841901)) ;
#20951=CARTESIAN_POINT('Ctrl Pts',(-18.738859338082,21.6545970083931,124.761963952245)) ;
#20952=CARTESIAN_POINT('Ctrl Pts',(-18.6965214907536,21.8444076862681,124.384579575107)) ;
#20953=CARTESIAN_POINT('Ctrl Pts',(-18.5183469904694,21.6644186059052,124.627779140097)) ;
#20954=CARTESIAN_POINT('Ctrl Pts',(-18.5374995717357,21.8544639457486,124.245294446865)) ;
#20955=CARTESIAN_POINT('Ctrl Pts',(-18.3195680415686,21.6744748653857,124.453674665829)) ;
#20956=CARTESIAN_POINT('Ctrl Pts',(-18.4068771812102,21.864403882049,124.082167341671)) ;
#20957=CARTESIAN_POINT('Ctrl Pts',(-18.1562878546674,21.6844148016861,124.249767117428)) ;
#20958=CARTESIAN_POINT('Ctrl Pts',(-18.3063513222259,21.8743110027934,123.899756894152)) ;
#20959=CARTESIAN_POINT('Ctrl Pts',(-18.0306281552504,21.6943219224305,124.021754765608)) ;
#20960=CARTESIAN_POINT('Ctrl Pts',(-18.2381764644266,21.8843539087187,123.699938324222)) ;
#20961=CARTESIAN_POINT('Ctrl Pts',(-17.9454073048491,21.7043648283558,123.771982422679)) ;
#20962=CARTESIAN_POINT('Ctrl Pts',(-18.2061259507257,21.8942616898179,123.494118034549)) ;
#20963=CARTESIAN_POINT('Ctrl Pts',(-17.9053416812303,21.714272609455,123.51470692144)) ;
#20964=CARTESIAN_POINT('Ctrl Pts',(-18.2099726092004,21.9042720588203,123.283696769241)) ;
#20965=CARTESIAN_POINT('Ctrl Pts',(-17.9101476585179,21.7242829784574,123.251680239082)) ;
#20966=CARTESIAN_POINT('Ctrl Pts',(-18.250799150117,21.9143028973891,123.076808306462)) ;
#20967=CARTESIAN_POINT('Ctrl Pts',(-17.9611784249865,21.7343138170262,122.993069233019)) ;
#20968=CARTESIAN_POINT('Ctrl Pts',(-18.3252324167252,21.9241557370288,122.88350173726)) ;
#20969=CARTESIAN_POINT('Ctrl Pts',(-18.0542181019441,21.7441666566659,122.751434398998)) ;
#20970=CARTESIAN_POINT('Ctrl Pts',(-18.4332250657028,21.9341437381937,122.703441071799)) ;
#20971=CARTESIAN_POINT('Ctrl Pts',(-18.1892070598107,21.7541546578309,122.526357242308)) ;
#20972=CARTESIAN_POINT('Ctrl Pts',(-18.5700375225545,21.9440725571729,122.545786789656)) ;
#20973=CARTESIAN_POINT('Ctrl Pts',(-18.3602212353183,21.76408347681,122.32928753721)) ;
#20974=CARTESIAN_POINT('Ctrl Pts',(-18.732888520769,21.9540602598952,122.413224493809)) ;
#20975=CARTESIAN_POINT('Ctrl Pts',(-18.5637837492857,21.7740711795323,122.163582862095)) ;
#20976=CARTESIAN_POINT('Ctrl Pts',(-18.9173249515201,21.9640962596979,122.31077716545)) ;
#20977=CARTESIAN_POINT('Ctrl Pts',(-18.7943281092038,21.784107179335,122.035521757821)) ;
#20978=CARTESIAN_POINT('Ctrl Pts',(-19.1130605451374,21.9739511294993,122.242820238378)) ;
#20979=CARTESIAN_POINT('Ctrl Pts',(-19.038997751584,21.7939620491364,121.950573239043)) ;
#20980=CARTESIAN_POINT('Ctrl Pts',(-19.3205261715052,21.9839505599228,122.209124296924)) ;
#20981=CARTESIAN_POINT('Ctrl Pts',(-19.2983295791008,21.80396147956,121.908451210414)) ;
#20982=CARTESIAN_POINT('Ctrl Pts',(-19.5285708919945,21.9938456773881,122.211711498228)) ;
#20983=CARTESIAN_POINT('Ctrl Pts',(-19.5583862373949,21.8138565970253,121.911683181411)) ;
#20984=CARTESIAN_POINT('Ctrl Pts',(-19.7363587174108,22.0039061709051,122.251037909545)) ;
#20985=CARTESIAN_POINT('Ctrl Pts',(-19.8181211650492,21.8239170905422,121.96083913654)) ;
#20986=CARTESIAN_POINT('Ctrl Pts',(-19.9300913010617,22.0137556511063,122.324185172849)) ;
#20987=CARTESIAN_POINT('Ctrl Pts',(-20.0602885784198,21.8337665707434,122.052271697296)) ;
#20988=CARTESIAN_POINT('Ctrl Pts',(-20.1116425157324,22.0237821013701,122.431281071649)) ;
#20989=CARTESIAN_POINT('Ctrl Pts',(-20.2872285089844,21.8437930210072,122.186139952124)) ;
#20990=CARTESIAN_POINT('Ctrl Pts',(-20.2715450400608,22.0338133918482,122.568785511319)) ;
#20991=CARTESIAN_POINT('Ctrl Pts',(-20.4871079315352,21.8538243114853,122.35801891506)) ;
#20992=CARTESIAN_POINT('Ctrl Pts',(-20.4029602797824,22.0436547795,122.728588268752)) ;
#20993=CARTESIAN_POINT('Ctrl Pts',(-20.6513791646752,21.8636656991371,122.557772038563)) ;
#20994=CARTESIAN_POINT('Ctrl Pts',(-20.5066507219347,22.0536581803912,122.911527607421)) ;
#20995=CARTESIAN_POINT('Ctrl Pts',(-20.7809938111829,21.8736691000283,122.786445434062)) ;
#20996=CARTESIAN_POINT('Ctrl Pts',(-20.5768052643418,22.0636425631824,123.109399042822)) ;
#20997=CARTESIAN_POINT('Ctrl Pts',(-20.8686887483206,21.8836534828195,123.033784325657)) ;
#20998=CARTESIAN_POINT('Ctrl Pts',(-20.6115199861339,22.0736816531958,123.317556791633)) ;
#20999=CARTESIAN_POINT('Ctrl Pts',(-20.9120839655183,21.8936925728329,123.293981074003)) ;
#21000=CARTESIAN_POINT('Ctrl Pts',(-20.6098913500393,22.0835274621049,123.524555130428)) ;
#21001=CARTESIAN_POINT('Ctrl Pts',(-20.9100499298834,21.9035383817421,123.552730180815)) ;
#21002=CARTESIAN_POINT('Ctrl Pts',(-20.5722452970051,22.0935118849239,123.731024894997)) ;
#21003=CARTESIAN_POINT('Ctrl Pts',(-20.8629939222876,21.9135228045611,123.810817924676)) ;
#21004=CARTESIAN_POINT('Ctrl Pts',(-20.4997117600218,22.1034515101651,123.927025671405)) ;
#21005=CARTESIAN_POINT('Ctrl Pts',(-20.7723283116897,21.9234624298023,124.05581995963)) ;
#21006=CARTESIAN_POINT('Ctrl Pts',(-20.3931662714284,22.1134911996838,124.109206689079)) ;
#21007=CARTESIAN_POINT('Ctrl Pts',(-20.6391479210158,21.9335021193209,124.283546922036)) ;
#21008=CARTESIAN_POINT('Ctrl Pts',(-20.2587285375417,22.1233793881024,124.267780927574)) ;
#21009=CARTESIAN_POINT('Ctrl Pts',(-20.4711013650952,21.9433903077395,124.481766445994)) ;
#21010=CARTESIAN_POINT('Ctrl Pts',(-20.0974265999504,22.1333689141044,124.402255862019)) ;
#21011=CARTESIAN_POINT('Ctrl Pts',(-20.2694747065142,21.9533798337416,124.649861363959)) ;
#21012=CARTESIAN_POINT('Ctrl Pts',(-19.9157102403435,22.1433274154596,124.506217438115)) ;
#21013=CARTESIAN_POINT('Ctrl Pts',(-20.0423296292845,21.9633383350968,124.779814856002)) ;
#21014=CARTESIAN_POINT('Ctrl Pts',(-19.7200260725257,22.1532270094633,124.577119056446)) ;
#21015=CARTESIAN_POINT('Ctrl Pts',(-19.7977240449736,21.9732379291004,124.868443422786)) ;
#21016=CARTESIAN_POINT('Ctrl Pts',(-19.5119529377031,22.1632748975846,124.61342395275)) ;
#21017=CARTESIAN_POINT('Ctrl Pts',(-19.5376330731142,21.9832858172217,124.913825837491)) ;
#21018=CARTESIAN_POINT('Ctrl Pts',(-19.3038874510347,22.1731703228301,124.613217769104)) ;
#21019=CARTESIAN_POINT('Ctrl Pts',(-19.2775503015537,21.9931812424672,124.913569399124)) ;
#21020=CARTESIAN_POINT('Ctrl Pts',(-19.0956337768571,22.1832317135307,124.576318144067)) ;
#21021=CARTESIAN_POINT('Ctrl Pts',(-19.017233305932,22.0032426331678,124.86744619023)) ;
#21022=CARTESIAN_POINT('Ctrl Pts',(-18.9011658613922,22.1930772972174,124.505398277424)) ;
#21023=CARTESIAN_POINT('Ctrl Pts',(-18.7741467328486,22.0130882168545,124.778797095436)) ;
#21024=CARTESIAN_POINT('Ctrl Pts',(-18.7194990589113,22.2030402705266,124.401179624215)) ;
#21025=CARTESIAN_POINT('Ctrl Pts',(-18.5470623486079,22.0230511901637,124.648524437436)) ;
#21026=CARTESIAN_POINT('Ctrl Pts',(-18.5578335683124,22.2130659373523,124.265923043721)) ;
#21027=CARTESIAN_POINT('Ctrl Pts',(-18.3449798305692,22.0330768569895,124.479454619294)) ;
#21028=CARTESIAN_POINT('Ctrl Pts',(-18.4235409053948,22.2229804152186,124.106527257626)) ;
#21029=CARTESIAN_POINT('Ctrl Pts',(-18.1771126653133,22.0429913348558,124.28020996493)) ;
#21030=CARTESIAN_POINT('Ctrl Pts',(-18.3178094286118,22.2329689298936,123.925078039381)) ;
#21031=CARTESIAN_POINT('Ctrl Pts',(-18.0449474119808,22.0529798495308,124.053398711337)) ;
#21032=CARTESIAN_POINT('Ctrl Pts',(-18.2452217442394,22.2430130408091,123.726808026642)) ;
#21033=CARTESIAN_POINT('Ctrl Pts',(-17.954211848732,22.0630239604462,123.805561752125)) ;
#21034=CARTESIAN_POINT('Ctrl Pts',(-18.2084565806548,22.2528411784036,123.523457249866)) ;
#21035=CARTESIAN_POINT('Ctrl Pts',(-17.9082542485454,22.0728520980408,123.551371969022)) ;
#21036=CARTESIAN_POINT('Ctrl Pts',(-18.2074383421507,22.2629177464626,123.311661356134)) ;
#21037=CARTESIAN_POINT('Ctrl Pts',(-17.9069805912369,22.0829286660997,123.286627562761)) ;
#21038=CARTESIAN_POINT('Ctrl Pts',(-18.2423241793869,22.2727699083667,123.107451203336)) ;
#21039=CARTESIAN_POINT('Ctrl Pts',(-17.9505873022016,22.0927808280039,123.031363437666)) ;
#21040=CARTESIAN_POINT('Ctrl Pts',(-18.3135102543039,22.2828428703236,122.908047647564)) ;
#21041=CARTESIAN_POINT('Ctrl Pts',(-18.0395690380517,22.1028537899607,122.782109150564)) ;
#21042=CARTESIAN_POINT('Ctrl Pts',(-18.4158946807527,22.2926854323265,122.728210968454)) ;
#21043=CARTESIAN_POINT('Ctrl Pts',(-18.1675496052933,22.1126963519636,122.557311692099)) ;
#21044=CARTESIAN_POINT('Ctrl Pts',(-18.549238880053,22.3026658688203,122.566223969324)) ;
#21045=CARTESIAN_POINT('Ctrl Pts',(-18.3342296705409,22.1226767884574,122.354827390352)) ;
#21046=CARTESIAN_POINT('Ctrl Pts',(-18.7095577945463,22.3126841741447,122.429637874185)) ;
#21047=CARTESIAN_POINT('Ctrl Pts',(-18.5346278830778,22.1326950937818,122.184094281001)) ;
#21048=CARTESIAN_POINT('Ctrl Pts',(-18.8885239198384,22.3225681380641,122.324009756949)) ;
#21049=CARTESIAN_POINT('Ctrl Pts',(-18.7583362356547,22.1425790577013,122.052058163512)) ;
#21050=CARTESIAN_POINT('Ctrl Pts',(-19.0866690738758,22.3326340148027,122.249785568809)) ;
#21051=CARTESIAN_POINT('Ctrl Pts',(-19.0060171333251,22.1526449344398,121.959277593487)) ;
#21052=CARTESIAN_POINT('Ctrl Pts',(-19.2900221608687,22.3424731156636,122.211822747741)) ;
#21053=CARTESIAN_POINT('Ctrl Pts',(-19.2602098520566,22.1624840353007,121.911823353389)) ;
#21054=CARTESIAN_POINT('Ctrl Pts',(-19.5009224073841,22.3525061985293,122.209172430537)) ;
#21055=CARTESIAN_POINT('Ctrl Pts',(-19.5238350449174,22.1725171181664,121.908510218283)) ;
#21056=CARTESIAN_POINT('Ctrl Pts',(-19.7087834710141,22.3625278838048,122.243664453097)) ;
#21057=CARTESIAN_POINT('Ctrl Pts',(-19.7836614016497,22.1825388034419,121.951624796669)) ;
#21058=CARTESIAN_POINT('Ctrl Pts',(-19.9045062463924,22.3723945789033,122.312314874088)) ;
#21059=CARTESIAN_POINT('Ctrl Pts',(-20.0283161574298,22.1924054985404,122.037437936202)) ;
#21060=CARTESIAN_POINT('Ctrl Pts',(-20.0873367852254,22.3823544686378,122.414394213939)) ;
#21061=CARTESIAN_POINT('Ctrl Pts',(-20.2568547840646,22.2023653882749,122.165037255751)) ;
#21062=CARTESIAN_POINT('Ctrl Pts',(-20.2506677841391,22.3923894564633,122.547902606798)) ;
#21063=CARTESIAN_POINT('Ctrl Pts',(-20.4610185638516,22.2124003761004,122.331922477437)) ;
#21064=CARTESIAN_POINT('Ctrl Pts',(-20.3865916163423,22.4022761605376,122.705186554573)) ;
#21065=CARTESIAN_POINT('Ctrl Pts',(-20.6309241388541,22.2222870801747,122.528528183517)) ;
#21066=CARTESIAN_POINT('Ctrl Pts',(-20.4949858769458,22.4123413047705,122.886876646557)) ;
#21067=CARTESIAN_POINT('Ctrl Pts',(-20.766416856272,22.2323522244076,122.755640405164)) ;
#21068=CARTESIAN_POINT('Ctrl Pts',(-20.5687197159867,22.422180595499,123.080175375466)) ;
#21069=CARTESIAN_POINT('Ctrl Pts',(-20.8585847061565,22.2421915151362,122.997265190441)) ;
#21070=CARTESIAN_POINT('Ctrl Pts',(-20.6089305970685,22.4322431529375,123.287840199753)) ;
#21071=CARTESIAN_POINT('Ctrl Pts',(-20.9088481489483,22.2522540725746,123.256845872699)) ;
#21072=CARTESIAN_POINT('Ctrl Pts',(-20.6121922591228,22.4421402041896,123.495893346216)) ;
#21073=CARTESIAN_POINT('Ctrl Pts',(-20.9129252441028,22.2621511238267,123.516913308371)) ;
#21074=CARTESIAN_POINT('Ctrl Pts',(-20.5798565032163,22.4520714109378,123.702154164007)) ;
#21075=CARTESIAN_POINT('Ctrl Pts',(-20.8725051637196,22.272082330575,123.774739999813)) ;
#21076=CARTESIAN_POINT('Ctrl Pts',(-20.5112221625243,22.4621135951567,123.901801813168)) ;
#21077=CARTESIAN_POINT('Ctrl Pts',(-20.786712131682,22.2821245147938,124.024299304319)) ;
#21078=CARTESIAN_POINT('Ctrl Pts',(-20.4106758088328,22.4720002232676,124.083722626987)) ;
#21079=CARTESIAN_POINT('Ctrl Pts',(-20.6610284500015,22.2920111429047,124.25170115506)) ;
#21080=CARTESIAN_POINT('Ctrl Pts',(-20.278945382695,22.4819934958,124.2473690502)) ;
#21081=CARTESIAN_POINT('Ctrl Pts',(-20.4963649928319,22.3020044154371,124.45625910245)) ;
#21082=CARTESIAN_POINT('Ctrl Pts',(-20.1215083587096,22.4919385713414,124.384944915974)) ;
#21083=CARTESIAN_POINT('Ctrl Pts',(-20.2995680280399,22.3119494909786,124.628229064092)) ;
#21084=CARTESIAN_POINT('Ctrl Pts',(-19.9426983959548,22.5018881220697,124.493496277981)) ;
#21085=CARTESIAN_POINT('Ctrl Pts',(-20.0760548364874,22.3218990417068,124.763918115327)) ;
#21086=CARTESIAN_POINT('Ctrl Pts',(-19.7459427076918,22.5119274569177,124.569841858884)) ;
#21087=CARTESIAN_POINT('Ctrl Pts',(-19.8301102215282,22.3319383765548,124.859349625922)) ;
#21088=CARTESIAN_POINT('Ctrl Pts',(-19.5420901927288,22.5218135958616,124.610431047829)) ;
#21089=CARTESIAN_POINT('Ctrl Pts',(-19.5752934234394,22.3418245154987,124.910085821145)) ;
#21090=CARTESIAN_POINT('Ctrl Pts',(-19.331980404051,22.5318117088353,124.615326987992)) ;
#21091=CARTESIAN_POINT('Ctrl Pts',(-19.3126560173104,22.3518226284724,124.916205138615)) ;
#21092=CARTESIAN_POINT('Ctrl Pts',(-19.1257731714612,22.5417314711877,124.584031987848)) ;
#21093=CARTESIAN_POINT('Ctrl Pts',(-19.0548963059002,22.3617423908249,124.877085616116)) ;
#21094=CARTESIAN_POINT('Ctrl Pts',(-18.925760197074,22.5517708668004,124.51667777525)) ;
#21095=CARTESIAN_POINT('Ctrl Pts',(-18.8048804750818,22.3717817864375,124.792892259255)) ;
#21096=CARTESIAN_POINT('Ctrl Pts',(-18.7429037014523,22.5616800525887,124.416866967638)) ;
#21097=CARTESIAN_POINT('Ctrl Pts',(-18.5763093840162,22.3816909722258,124.668127742339)) ;
#21098=CARTESIAN_POINT('Ctrl Pts',(-18.579362600272,22.5716152367462,124.286939430316)) ;
#21099=CARTESIAN_POINT('Ctrl Pts',(-18.3718830460784,22.3916261563833,124.505717216813)) ;
#21100=CARTESIAN_POINT('Ctrl Pts',(-18.4395493540934,22.5816562941321,124.128790649976)) ;
#21101=CARTESIAN_POINT('Ctrl Pts',(-18.1971172156532,22.4016672137692,124.308030847448)) ;
#21102=CARTESIAN_POINT('Ctrl Pts',(-18.3308735820911,22.5915434521654,123.951591507098)) ;
#21103=CARTESIAN_POINT('Ctrl Pts',(-18.0612726927552,22.4115543718025,124.086530580778)) ;
#21104=CARTESIAN_POINT('Ctrl Pts',(-18.253489695394,22.6015357318413,123.756310473585)) ;
#21105=CARTESIAN_POINT('Ctrl Pts',(-17.9645436848904,22.4215466514784,123.842428732897)) ;
#21106=CARTESIAN_POINT('Ctrl Pts',(-18.2114252982926,22.6114842488863,123.551423040072)) ;
#21107=CARTESIAN_POINT('Ctrl Pts',(-17.9119640315032,22.4314951685235,123.586318714181)) ;
#21108=CARTESIAN_POINT('Ctrl Pts',(-18.2052879099196,22.6214210264567,123.342628586766)) ;
#21109=CARTESIAN_POINT('Ctrl Pts',(-17.9042933598069,22.4414319460939,123.325324977717)) ;
#21110=CARTESIAN_POINT('Ctrl Pts',(-18.2353818524349,22.6314040626037,123.134895795784)) ;
#21111=CARTESIAN_POINT('Ctrl Pts',(-17.9419119920911,22.4514149822408,123.065658904093)) ;
#21112=CARTESIAN_POINT('Ctrl Pts',(-18.3018390798526,22.6414478141974,122.934500268376)) ;
#21113=CARTESIAN_POINT('Ctrl Pts',(-18.0249844510094,22.4614587338345,122.815165001349)) ;
#21114=CARTESIAN_POINT('Ctrl Pts',(-18.3995334670519,22.65127634341,122.752393803793)) ;
#21115=CARTESIAN_POINT('Ctrl Pts',(-18.1471041894676,22.4712872630471,122.587531223368)) ;
#21116=CARTESIAN_POINT('Ctrl Pts',(-18.5304390769983,22.6613517043187,122.585924560108)) ;
#21117=CARTESIAN_POINT('Ctrl Pts',(-18.310736925562,22.4813626239558,122.379445782567)) ;
#21118=CARTESIAN_POINT('Ctrl Pts',(-18.6848484847896,22.6712083032059,122.447668513297)) ;
#21119=CARTESIAN_POINT('Ctrl Pts',(-18.5037504475988,22.491219222843,122.2066258693)) ;
#21120=CARTESIAN_POINT('Ctrl Pts',(-18.8644168488015,22.6812712972238,122.335891874011)) ;
#21121=CARTESIAN_POINT('Ctrl Pts',(-18.7282113464719,22.5012822168609,122.066906399844)) ;
#21122=CARTESIAN_POINT('Ctrl Pts',(-19.0571331275604,22.6911492315132,122.25842835509)) ;
#21123=CARTESIAN_POINT('Ctrl Pts',(-18.9691081441337,22.5111601511503,121.970077874885)) ;
#21124=CARTESIAN_POINT('Ctrl Pts',(-19.2627566660564,22.7011498790713,122.214769477626)) ;
#21125=CARTESIAN_POINT('Ctrl Pts',(-19.2261379991879,22.5211607987084,121.915505689096)) ;
#21126=CARTESIAN_POINT('Ctrl Pts',(-19.4711669419206,22.7110677255094,122.207377365738)) ;
#21127=CARTESIAN_POINT('Ctrl Pts',(-19.4866516087189,22.5310786451465,121.906267040837)) ;
#21128=CARTESIAN_POINT('Ctrl Pts',(-19.6803914078797,22.721118842515,122.236721719079)) ;
#21129=CARTESIAN_POINT('Ctrl Pts',(-19.7481817747748,22.5411297621521,121.942948938101)) ;
#21130=CARTESIAN_POINT('Ctrl Pts',(-19.8778768048327,22.7309895778256,122.300577463833)) ;
#21131=CARTESIAN_POINT('Ctrl Pts',(-19.9950390178656,22.5510004974627,122.022770439589)) ;
#21132=CARTESIAN_POINT('Ctrl Pts',(-20.0649458105329,22.7410602850686,122.39964958428)) ;
#21133=CARTESIAN_POINT('Ctrl Pts',(-20.2288742155722,22.5610712047057,122.146611832965)) ;
#21134=CARTESIAN_POINT('Ctrl Pts',(-20.2281280729297,22.7508932925205,122.526586135203)) ;
#21135=CARTESIAN_POINT('Ctrl Pts',(-20.432852059648,22.5709042121576,122.305284591667)) ;
#21136=CARTESIAN_POINT('Ctrl Pts',(-20.3700041193385,22.7609237848228,122.682583660361)) ;
#21137=CARTESIAN_POINT('Ctrl Pts',(-20.6101957114275,22.5809347044599,122.50028265826)) ;
#21138=CARTESIAN_POINT('Ctrl Pts',(-20.4821412733727,22.7709553798962,122.861209839806)) ;
#21139=CARTESIAN_POINT('Ctrl Pts',(-20.7503657377508,22.5909662995333,122.723566173364)) ;
#21140=CARTESIAN_POINT('Ctrl Pts',(-20.5603509074772,22.7807850790344,123.052474175343)) ;
#21141=CARTESIAN_POINT('Ctrl Pts',(-20.848126630718,22.6007959986715,122.962648437251)) ;
#21142=CARTESIAN_POINT('Ctrl Pts',(-20.6054919636736,22.790774528916,123.257581426922)) ;
#21143=CARTESIAN_POINT('Ctrl Pts',(-20.904551077241,22.6107854485531,123.219033095629)) ;
#21144=CARTESIAN_POINT('Ctrl Pts',(-20.6138461179592,22.8008183867317,123.468567262756)) ;
#21145=CARTESIAN_POINT('Ctrl Pts',(-20.9149919746047,22.6208293063688,123.482765312887)) ;
#21146=CARTESIAN_POINT('Ctrl Pts',(-20.5864922399839,22.8106400773219,123.673230555573)) ;
#21147=CARTESIAN_POINT('Ctrl Pts',(-20.8807975538298,22.630650996959,123.738595413769)) ;
#21148=CARTESIAN_POINT('Ctrl Pts',(-20.5231490604348,22.8206751678623,123.874462180045)) ;
#21149=CARTESIAN_POINT('Ctrl Pts',(-20.8016166335874,22.6406860874994,123.990134218036)) ;
#21150=CARTESIAN_POINT('Ctrl Pts',(-20.4254247657349,22.830699686845,124.061198211658)) ;
#21151=CARTESIAN_POINT('Ctrl Pts',(-20.6794595798729,22.6507106064821,124.223553358068)) ;
#21152=CARTESIAN_POINT('Ctrl Pts',(-20.2991731667971,22.8405595322552,124.225579994862)) ;
#21153=CARTESIAN_POINT('Ctrl Pts',(-20.5216428899484,22.6605704518923,124.429030130044)) ;
#21154=CARTESIAN_POINT('Ctrl Pts',(-20.1451242577046,22.8505193085708,124.367400091411)) ;
#21155=CARTESIAN_POINT('Ctrl Pts',(-20.3290800370369,22.670530228208,124.606303874563)) ;
#21156=CARTESIAN_POINT('Ctrl Pts',(-19.9674278032907,22.8605475058855,124.480844125221)) ;
#21157=CARTESIAN_POINT('Ctrl Pts',(-20.1069583810948,22.6805584255226,124.748107125882)) ;
#21158=CARTESIAN_POINT('Ctrl Pts',(-19.7751521418593,22.8704550481758,124.56097363697)) ;
#21159=CARTESIAN_POINT('Ctrl Pts',(-19.8666123895492,22.6904659678129,124.848267265594)) ;
#21160=CARTESIAN_POINT('Ctrl Pts',(-19.5693646949917,22.8804876987396,124.607138562997)) ;
#21161=CARTESIAN_POINT('Ctrl Pts',(-19.6093776535577,22.7004986183768,124.905971284957)) ;
#21162=CARTESIAN_POINT('Ctrl Pts',(-19.3617911177059,22.8903716551663,124.616789062193)) ;
#21163=CARTESIAN_POINT('Ctrl Pts',(-19.349909838197,22.7103825748034,124.918032249207)) ;
#21164=CARTESIAN_POINT('Ctrl Pts',(-19.1534263144048,22.9003613565281,124.590486564837)) ;
#21165=CARTESIAN_POINT('Ctrl Pts',(-19.0894539708058,22.7203722761653,124.88515179817)) ;
#21166=CARTESIAN_POINT('Ctrl Pts',(-18.9518995245256,22.9104023518042,124.527657154102)) ;
#21167=CARTESIAN_POINT('Ctrl Pts',(-18.8375462307077,22.7304132714413,124.806612946757)) ;
#21168=CARTESIAN_POINT('Ctrl Pts',(-18.768077928406,22.9202352410725,124.433102961583)) ;
#21169=CARTESIAN_POINT('Ctrl Pts',(-18.6077694357356,22.7402461607097,124.68841772116)) ;
#21170=CARTESIAN_POINT('Ctrl Pts',(-18.6004184578311,22.93022839944,124.306510185862)) ;
#21171=CARTESIAN_POINT('Ctrl Pts',(-18.3981964690907,22.7502393190771,124.530174726569)) ;
#21172=CARTESIAN_POINT('Ctrl Pts',(-18.4570423276391,22.9402604417921,124.151821923113)) ;
#21173=CARTESIAN_POINT('Ctrl Pts',(-18.2189780474116,22.7602713614292,124.336812835409)) ;
#21174=CARTESIAN_POINT('Ctrl Pts',(-18.3444002375447,22.9501256857505,123.977691444909)) ;
#21175=CARTESIAN_POINT('Ctrl Pts',(-18.078177052041,22.7701366053876,124.11914781899)) ;
#21176=CARTESIAN_POINT('Ctrl Pts',(-18.2623606113742,22.9600875769965,123.78499218241)) ;
#21177=CARTESIAN_POINT('Ctrl Pts',(-17.9756297430813,22.7800984966336,123.878272519234)) ;
#21178=CARTESIAN_POINT('Ctrl Pts',(-18.2150170839736,22.970122477015,123.579418516963)) ;
#21179=CARTESIAN_POINT('Ctrl Pts',(-17.9164527324428,22.7901333966521,123.621304920688)) ;
#21180=CARTESIAN_POINT('Ctrl Pts',(-18.2039051887294,22.9800075574296,123.371873650446)) ;
#21181=CARTESIAN_POINT('Ctrl Pts',(-17.9025653496462,22.8000184770667,123.361873137659)) ;
#21182=CARTESIAN_POINT('Ctrl Pts',(-18.2294709369507,22.9900727295544,123.161850154122)) ;
#21183=CARTESIAN_POINT('Ctrl Pts',(-17.9345250196897,22.8100836491915,123.099344214703)) ;
#21184=CARTESIAN_POINT('Ctrl Pts',(-18.2896793781521,22.9999199642779,122.963757686704)) ;
#21185=CARTESIAN_POINT('Ctrl Pts',(-18.0097882001565,22.819930883915,122.851728714304)) ;
#21186=CARTESIAN_POINT('Ctrl Pts',(-18.3846575460078,23.0099507755956,122.775493829682)) ;
#21187=CARTESIAN_POINT('Ctrl Pts',(-18.1285132437623,22.8299616952328,122.616400101498)) ;
#21188=CARTESIAN_POINT('Ctrl Pts',(-18.5109834152174,23.0199603915091,122.607165887845)) ;
#21189=CARTESIAN_POINT('Ctrl Pts',(-18.2864226563192,22.8399713111463,122.40599165732)) ;
#21190=CARTESIAN_POINT('Ctrl Pts',(-18.6629287718639,23.0298711709128,122.464629523893)) ;
#21191=CARTESIAN_POINT('Ctrl Pts',(-18.4763564295643,22.84988209055,122.227822802769)) ;
#21192=CARTESIAN_POINT('Ctrl Pts',(-18.8373784129168,23.0398004367019,122.349974057845)) ;
#21193=CARTESIAN_POINT('Ctrl Pts',(-18.6944202111758,22.859811356339,122.084505529354)) ;
#21194=CARTESIAN_POINT('Ctrl Pts',(-19.0313295538799,23.0498431300145,122.266578270263)) ;
#21195=CARTESIAN_POINT('Ctrl Pts',(-18.9368601501301,22.8698540496516,121.980263237278)) ;
#21196=CARTESIAN_POINT('Ctrl Pts',(-19.2336083459502,23.0597296627092,122.218742068884)) ;
#21197=CARTESIAN_POINT('Ctrl Pts',(-19.1897096706424,22.8797405823464,121.920470478153)) ;
#21198=CARTESIAN_POINT('Ctrl Pts',(-19.4433140464625,23.0697228078125,122.206271347254)) ;
#21199=CARTESIAN_POINT('Ctrl Pts',(-19.4518420605083,22.8897337274496,121.904884777647)) ;
#21200=CARTESIAN_POINT('Ctrl Pts',(-19.6510110881743,23.0796684884866,122.230368010918)) ;
#21201=CARTESIAN_POINT('Ctrl Pts',(-19.7114632832621,22.8996794081237,121.935008316747)) ;
#21202=CARTESIAN_POINT('Ctrl Pts',(-19.8515326787835,23.0896157461133,122.289763971548)) ;
#21203=CARTESIAN_POINT('Ctrl Pts',(-19.9621146837926,22.9096266657504,122.009255961602)) ;
#21204=CARTESIAN_POINT('Ctrl Pts',(-20.0404673828271,23.0996636482348,122.38422357924)) ;
#21205=CARTESIAN_POINT('Ctrl Pts',(-20.1982818352397,22.9196745678719,122.127332902665)) ;
#21206=CARTESIAN_POINT('Ctrl Pts',(-20.2068601688876,23.1095113538565,122.507411205616)) ;
#21207=CARTESIAN_POINT('Ctrl Pts',(-20.4062715090379,22.9295222734936,122.281319880695)) ;
#21208=CARTESIAN_POINT('Ctrl Pts',(-20.3514553093839,23.1194728204906,122.658891921361)) ;
#21209=CARTESIAN_POINT('Ctrl Pts',(-20.5870134936696,22.9394837401277,122.470672801482)) ;
#21210=CARTESIAN_POINT('Ctrl Pts',(-20.4681173020612,23.1295023737588,122.83453984717)) ;
#21211=CARTESIAN_POINT('Ctrl Pts',(-20.7328386955894,22.9495132933959,122.690234279952)) ;
#21212=CARTESIAN_POINT('Ctrl Pts',(-20.5515843547797,23.1394092657862,123.025360354087)) ;
#21213=CARTESIAN_POINT('Ctrl Pts',(-20.8371700436695,22.9594201854233,122.928761227148)) ;
#21214=CARTESIAN_POINT('Ctrl Pts',(-20.6012418234421,23.1493569098992,123.228492863603)) ;
#21215=CARTESIAN_POINT('Ctrl Pts',(-20.8992391770811,22.9693678295363,123.182677656175)) ;
#21216=CARTESIAN_POINT('Ctrl Pts',(-20.6150800343719,23.1593569529281,123.438296909276)) ;
#21217=CARTESIAN_POINT('Ctrl Pts',(-20.9165341377211,22.9793678725652,123.444932969306)) ;
#21218=CARTESIAN_POINT('Ctrl Pts',(-20.5918224314329,23.1693957189221,123.648041713659)) ;
#21219=CARTESIAN_POINT('Ctrl Pts',(-20.8874593437994,22.9894066385592,123.707113721901)) ;
#21220=CARTESIAN_POINT('Ctrl Pts',(-20.5341745069886,23.1792207809443,123.846402561714)) ;
#21221=CARTESIAN_POINT('Ctrl Pts',(-20.8153966815368,22.9992317005814,123.955064177239)) ;
#21222=CARTESIAN_POINT('Ctrl Pts',(-20.4411557623912,23.1892753282707,124.036199337756)) ;
#21223=CARTESIAN_POINT('Ctrl Pts',(-20.6991206973961,23.0092862479078,124.192308936938)) ;
#21224=CARTESIAN_POINT('Ctrl Pts',(-20.3176702770705,23.1992185717199,124.204874255302)) ;
#21225=CARTESIAN_POINT('Ctrl Pts',(-20.5447615013441,23.019229491357,124.403151003466)) ;
#21226=CARTESIAN_POINT('Ctrl Pts',(-20.1678477489804,23.2091207433278,124.349412148835)) ;
#21227=CARTESIAN_POINT('Ctrl Pts',(-20.357481348229,23.0291316629649,124.583821375332)) ;
#21228=CARTESIAN_POINT('Ctrl Pts',(-19.9925143602655,23.219173578938,124.467395725293)) ;
#21229=CARTESIAN_POINT('Ctrl Pts',(-20.1383129462667,23.0391844985751,124.731298547748)) ;
#21230=CARTESIAN_POINT('Ctrl Pts',(-19.8028310164097,23.2290466366235,124.551692861004)) ;
#21231=CARTESIAN_POINT('Ctrl Pts',(-19.9012076725115,23.0490575562606,124.836667408501)) ;
#21232=CARTESIAN_POINT('Ctrl Pts',(-19.599035620592,23.2390418981492,124.602895730111)) ;
#21233=CARTESIAN_POINT('Ctrl Pts',(-19.6464624451115,23.0590528177863,124.90066823185)) ;
#21234=CARTESIAN_POINT('Ctrl Pts',(-19.3887803257811,23.2490672675697,124.617604462307)) ;
#21235=CARTESIAN_POINT('Ctrl Pts',(-19.3836439744441,23.0690781872068,124.919051527796)) ;
#21236=CARTESIAN_POINT('Ctrl Pts',(-19.1819671042923,23.2589571000963,124.596152765897)) ;
#21237=CARTESIAN_POINT('Ctrl Pts',(-19.1251242692714,23.0789680197334,124.892233416081)) ;
#21238=CARTESIAN_POINT('Ctrl Pts',(-18.9130557461595,23.2722550709057,124.5197923832)) ;
#21239=CARTESIAN_POINT('Ctrl Pts',(-18.7890035337137,23.0922659905428,124.796782825436)) ;
#21240=CARTESIAN_POINT('Ctrl Pts',(-18.6717587243513,23.2854534660148,124.376385706573)) ;
#21241=CARTESIAN_POINT('Ctrl Pts',(-18.4874072190834,23.105464385652,124.617549791502)) ;
#21242=CARTESIAN_POINT('Ctrl Pts',(-18.4752682237642,23.2988489082943,124.174730150354)) ;
#21243=CARTESIAN_POINT('Ctrl Pts',(-18.2417519026231,23.1188598279314,124.365440342986)) ;
#21244=CARTESIAN_POINT('Ctrl Pts',(-18.358218981122,23.3087247465333,124.00319866305)) ;
#21245=CARTESIAN_POINT('Ctrl Pts',(-18.0954516814504,23.1287356661704,124.151032241541)) ;
#21246=CARTESIAN_POINT('Ctrl Pts',(-18.2710692283596,23.318786149131,123.810502936059)) ;
#21247=CARTESIAN_POINT('Ctrl Pts',(-17.9865146772214,23.1387970687681,123.910158781384)) ;
#21248=CARTESIAN_POINT('Ctrl Pts',(-18.2196477196924,23.3286512060661,123.609550825009)) ;
#21249=CARTESIAN_POINT('Ctrl Pts',(-17.922240462111,23.1486621257033,123.658970587668)) ;
#21250=CARTESIAN_POINT('Ctrl Pts',(-18.2032931252815,23.3386633020149,123.399733102314)) ;
#21251=CARTESIAN_POINT('Ctrl Pts',(-17.9018022904604,23.1586742216521,123.396691351192)) ;
#21252=CARTESIAN_POINT('Ctrl Pts',(-18.2303090879066,23.3519406111604,123.121854743172)) ;
#21253=CARTESIAN_POINT('Ctrl Pts',(-17.9355630207714,23.1719515307975,123.049376976604)) ;
#21254=CARTESIAN_POINT('Ctrl Pts',(-18.3537865412185,23.3685396366677,122.791280328664)) ;
#21255=CARTESIAN_POINT('Ctrl Pts',(-18.0899419028751,23.1885505563048,122.636110521846)) ;
#21256=CARTESIAN_POINT('Ctrl Pts',(-18.5826974213556,23.3851386847007,122.522589585536)) ;
#21257=CARTESIAN_POINT('Ctrl Pts',(-18.3760258329839,23.2051496043378,122.300311520429)) ;
#21258=CARTESIAN_POINT('Ctrl Pts',(-18.8116870577227,23.3983820967316,122.364269542791)) ;
#21259=CARTESIAN_POINT('Ctrl Pts',(-18.6623130734036,23.2183930163688,122.102367993719)) ;
#21260=CARTESIAN_POINT('Ctrl Pts',(-19.0034183423248,23.4084195244201,122.276133501985)) ;
#21261=CARTESIAN_POINT('Ctrl Pts',(-18.9019676656497,23.2284304440572,121.992209381467)) ;
#21262=CARTESIAN_POINT('Ctrl Pts',(-19.2048395995662,23.4183238263757,122.223371608911)) ;
#21263=CARTESIAN_POINT('Ctrl Pts',(-19.1537511180854,23.2383347460128,121.926257438649)) ;
#21264=CARTESIAN_POINT('Ctrl Pts',(-19.4827891473364,23.4315906663508,122.19988920511)) ;
#21265=CARTESIAN_POINT('Ctrl Pts',(-19.5011668383559,23.251601585988,121.896906683047)) ;
#21266=CARTESIAN_POINT('Ctrl Pts',(-19.8307318849537,23.4482168644408,122.262263108639)) ;
#21267=CARTESIAN_POINT('Ctrl Pts',(-19.9361152832958,23.2682277840779,121.974875772965)) ;
#21268=CARTESIAN_POINT('Ctrl Pts',(-20.1971528166808,23.4681359798242,122.474678281948)) ;
#21269=CARTESIAN_POINT('Ctrl Pts',(-20.394142712814,23.2881468994613,122.240416456631)) ;
#21270=CARTESIAN_POINT('Ctrl Pts',(-20.4241051193176,23.4847424029584,122.745236826327)) ;
#21271=CARTESIAN_POINT('Ctrl Pts',(-20.6777956763041,23.3047533225956,122.578559316856)) ;
#21272=CARTESIAN_POINT('Ctrl Pts',(-20.5421768965827,23.4980386234541,122.998554900509)) ;
#21273=CARTESIAN_POINT('Ctrl Pts',(-20.8254141685684,23.3180495430913,122.895260367424)) ;
#21274=CARTESIAN_POINT('Ctrl Pts',(-20.614959986531,23.5113074557956,123.267928258052)) ;
#21275=CARTESIAN_POINT('Ctrl Pts',(-20.9163840285696,23.3313183754327,123.231954203337)) ;
#21276=CARTESIAN_POINT('Ctrl Pts',(-20.6152647113257,23.5279987038287,123.622730942973)) ;
#21277=CARTESIAN_POINT('Ctrl Pts',(-20.9167633041339,23.3480096234658,123.675476169135)) ;
#21278=CARTESIAN_POINT('Ctrl Pts',(-20.4722994274042,23.5478084355015,124.018996186989)) ;
#21279=CARTESIAN_POINT('Ctrl Pts',(-20.7380527826187,23.3678193551386,124.170798980292)) ;
#21280=CARTESIAN_POINT('Ctrl Pts',(-20.2010981674225,23.56778604283,124.345907252259)) ;
#21281=CARTESIAN_POINT('Ctrl Pts',(-20.3990487800684,23.3877969624672,124.579436972735)) ;
#21282=CARTESIAN_POINT('Ctrl Pts',(-19.8351962742171,23.5877123518879,124.559408382312)) ;
#21283=CARTESIAN_POINT('Ctrl Pts',(-19.9416700356385,23.407723271525,124.846309372867)) ;
#21284=CARTESIAN_POINT('Ctrl Pts',(-19.4207969533748,23.6075292120526,124.636299831341)) ;
#21285=CARTESIAN_POINT('Ctrl Pts',(-19.423672280542,23.4275401316897,124.942420637845)) ;
#21286=CARTESIAN_POINT('Ctrl Pts',(-18.9994637731957,23.6276290276466,124.565563992342)) ;
#21287=CARTESIAN_POINT('Ctrl Pts',(-18.897005210854,23.4476399472837,124.853997620555)) ;
#21288=CARTESIAN_POINT('Ctrl Pts',(-18.6335253229913,23.6473859915291,124.358902751464)) ;
#21289=CARTESIAN_POINT('Ctrl Pts',(-18.4395858732156,23.4673969111663,124.595670036021)) ;
#21290=CARTESIAN_POINT('Ctrl Pts',(-18.3557767431134,23.6674229175986,124.036039149984)) ;
#21291=CARTESIAN_POINT('Ctrl Pts',(-18.0924014778527,23.4874338372357,124.192088863914)) ;
#21292=CARTESIAN_POINT('Ctrl Pts',(-18.2066700929233,23.6872924999801,123.640628669761)) ;
#21293=CARTESIAN_POINT('Ctrl Pts',(-17.9060208621862,23.5073034196172,123.697826439083)) ;
#21294=CARTESIAN_POINT('Ctrl Pts',(-18.20037309154,23.7071970717333,123.217532309015)) ;
#21295=CARTESIAN_POINT('Ctrl Pts',(-17.8981510516399,23.5272079913704,123.168957382108)) ;
#21296=CARTESIAN_POINT('Ctrl Pts',(-18.3392583799834,23.7271496739318,122.816587599737)) ;
#21297=CARTESIAN_POINT('Ctrl Pts',(-18.0717585757874,23.5471605935689,122.667777463739)) ;
#21298=CARTESIAN_POINT('Ctrl Pts',(-18.6060586541103,23.747059164902,122.488027614891)) ;
#21299=CARTESIAN_POINT('Ctrl Pts',(-18.4052588840874,23.5670700845392,122.257079257931)) ;
#21300=CARTESIAN_POINT('Ctrl Pts',(-18.9674540788008,23.7669105336015,122.269754789477)) ;
#21301=CARTESIAN_POINT('Ctrl Pts',(-18.8570010753677,23.5869214532386,121.984239388305)) ;
#21302=CARTESIAN_POINT('Ctrl Pts',(-19.3863467957852,23.7869907297375,122.187619791407)) ;
#21303=CARTESIAN_POINT('Ctrl Pts',(-19.3806182677798,23.6070016493746,121.881570519937)) ;
#21304=CARTESIAN_POINT('Ctrl Pts',(-19.8024562321169,23.8067916733129,122.25247266476)) ;
#21305=CARTESIAN_POINT('Ctrl Pts',(-19.9007519851589,23.62680259295,121.962636023239)) ;
#21306=CARTESIAN_POINT('Ctrl Pts',(-20.1751703809712,23.8267756498224,122.456380190659)) ;
#21307=CARTESIAN_POINT('Ctrl Pts',(-20.366645013507,23.6467865694595,122.217519363045)) ;
#21308=CARTESIAN_POINT('Ctrl Pts',(-20.4545225997992,23.846691612798,122.774634398599)) ;
#21309=CARTESIAN_POINT('Ctrl Pts',(-20.7158350928187,23.6667025324351,122.615335633075)) ;
#21310=CARTESIAN_POINT('Ctrl Pts',(-20.6092694572912,23.8665620476199,123.167863522626)) ;
#21311=CARTESIAN_POINT('Ctrl Pts',(-20.909269753505,23.686572967257,123.106869748193)) ;
#21312=CARTESIAN_POINT('Ctrl Pts',(-20.6199224875745,23.886612332853,123.593929804403)) ;
#21313=CARTESIAN_POINT('Ctrl Pts',(-20.922587690353,23.7066232524901,123.639453176953)) ;
#21314=CARTESIAN_POINT('Ctrl Pts',(-20.4868864023955,23.9063863016123,123.992954670448)) ;
#21315=CARTESIAN_POINT('Ctrl Pts',(-20.7562955195823,23.7263972212494,124.138232320058)) ;
#21316=CARTESIAN_POINT('Ctrl Pts',(-20.2223831801166,23.9264427597318,124.327253105703)) ;
#21317=CARTESIAN_POINT('Ctrl Pts',(-20.4256681461167,23.746453679369,124.556107455173)) ;
#21318=CARTESIAN_POINT('Ctrl Pts',(-19.8640850949148,23.9462376427228,124.548331334748)) ;
#21319=CARTESIAN_POINT('Ctrl Pts',(-19.9777988611578,23.76624856236,124.832456311627)) ;
#21320=CARTESIAN_POINT('Ctrl Pts',(-19.448727810941,23.9662042980252,124.63574281183)) ;
#21321=CARTESIAN_POINT('Ctrl Pts',(-19.4586032621524,23.7862152176623,124.941723989977)) ;
#21322=CARTESIAN_POINT('Ctrl Pts',(-19.0285651397822,23.9861632681017,124.575472295223)) ;
#21323=CARTESIAN_POINT('Ctrl Pts',(-18.9333997951415,23.8061741877388,124.86638911577)) ;
#21324=CARTESIAN_POINT('Ctrl Pts',(-18.6553168032142,24.0060593556918,124.376389568719)) ;
#21325=CARTESIAN_POINT('Ctrl Pts',(-18.466838553606,23.8260702753289,124.617539311619)) ;
#21326=CARTESIAN_POINT('Ctrl Pts',(-18.3720148561307,24.0259575256034,124.062201487962)) ;
#21327=CARTESIAN_POINT('Ctrl Pts',(-18.1127087822637,23.8459684452405,124.224807490326)) ;
#21328=CARTESIAN_POINT('Ctrl Pts',(-18.2124303919169,24.0458633609705,123.67015401321)) ;
#21329=CARTESIAN_POINT('Ctrl Pts',(-17.9132245363324,23.8658742806076,123.734750368409)) ;
#21330=CARTESIAN_POINT('Ctrl Pts',(-18.1961880168038,24.0658132859084,123.246313641307)) ;
#21331=CARTESIAN_POINT('Ctrl Pts',(-17.8929172316979,23.8858242055455,123.204950398228)) ;
#21332=CARTESIAN_POINT('Ctrl Pts',(-18.3247423088814,24.0856924758188,122.84360479257)) ;
#21333=CARTESIAN_POINT('Ctrl Pts',(-18.0536055022471,23.9057033954559,122.701563671004)) ;
#21334=CARTESIAN_POINT('Ctrl Pts',(-18.5841033382921,24.1056738000994,122.507146079178)) ;
#21335=CARTESIAN_POINT('Ctrl Pts',(-18.3778029519875,23.9256847197365,122.280987362701)) ;
#21336=CARTESIAN_POINT('Ctrl Pts',(-18.942010615732,24.1256035843077,122.280096072877)) ;
#21337=CARTESIAN_POINT('Ctrl Pts',(-18.8251843464588,23.9456145039448,121.997171158723)) ;
#21338=CARTESIAN_POINT('Ctrl Pts',(-19.3555068623215,24.1455235736985,122.188809483554)) ;
#21339=CARTESIAN_POINT('Ctrl Pts',(-19.3420527237489,23.9655344933356,121.8830575886)) ;
#21340=CARTESIAN_POINT('Ctrl Pts',(-19.7742904831662,24.1653787690525,122.2430041829)) ;
#21341=CARTESIAN_POINT('Ctrl Pts',(-19.8655341729859,23.9853896886896,121.950798016933)) ;
#21342=CARTESIAN_POINT('Ctrl Pts',(-20.1526808934445,24.1854247707119,122.438992855019)) ;
#21343=CARTESIAN_POINT('Ctrl Pts',(-20.3385180584329,24.005435690349,122.195770834828)) ;
#21344=CARTESIAN_POINT('Ctrl Pts',(-20.3906070125325,24.2019245179217,122.696923893817)) ;
#21345=CARTESIAN_POINT('Ctrl Pts',(-20.6359495242104,24.0219354375588,122.518207743344)) ;
#21346=CARTESIAN_POINT('Ctrl Pts',(-20.5216768074671,24.2153131223698,122.945999721875)) ;
#21347=CARTESIAN_POINT('Ctrl Pts',(-20.7997715920691,24.0353240420069,122.829526935845)) ;
#21348=CARTESIAN_POINT('Ctrl Pts',(-20.5848955736062,24.2251749507047,123.143455647205)) ;
#21349=CARTESIAN_POINT('Ctrl Pts',(-20.8788004514205,24.0451858703418,123.076353832387)) ;
#21350=CARTESIAN_POINT('Ctrl Pts',(-20.6138199274551,24.2351410934622,123.350985731134)) ;
#21351=CARTESIAN_POINT('Ctrl Pts',(-20.9149604443776,24.0551520130994,123.335751428972)) ;
#21352=CARTESIAN_POINT('Ctrl Pts',(-20.6032002789081,24.2485028395872,123.631591883731)) ;
#21353=CARTESIAN_POINT('Ctrl Pts',(-20.9016757192965,24.0685137592243,123.68657640661)) ;
#21354=CARTESIAN_POINT('Ctrl Pts',(-20.5008787541352,24.2649571685423,123.966355059804)) ;
#21355=CARTESIAN_POINT('Ctrl Pts',(-20.7738010339285,24.0849680881794,124.104947280262)) ;
#21356=CARTESIAN_POINT('Ctrl Pts',(-20.2867198767303,24.2817244135906,124.2511417434)) ;
#21357=CARTESIAN_POINT('Ctrl Pts',(-20.506074005893,24.1017353332277,124.460989068715)) ;
#21358=CARTESIAN_POINT('Ctrl Pts',(-20.068100156107,24.2949109788646,124.421823870107)) ;
#21359=CARTESIAN_POINT('Ctrl Pts',(-20.2328267963323,24.1149218985017,124.674311881725)) ;
#21360=CARTESIAN_POINT('Ctrl Pts',(-19.8829901974809,24.3049004376092,124.520886533694)) ;
#21361=CARTESIAN_POINT('Ctrl Pts',(-20.0014355866622,24.1249113572463,124.798149275947)) ;
#21362=CARTESIAN_POINT('Ctrl Pts',(-19.6841183586994,24.3148542100903,124.586142139234)) ;
#21363=CARTESIAN_POINT('Ctrl Pts',(-19.7528479925732,24.1348651297274,124.879719694348)) ;
#21364=CARTESIAN_POINT('Ctrl Pts',(-19.4750256631218,24.324902026623,124.61598118881)) ;
#21365=CARTESIAN_POINT('Ctrl Pts',(-19.4914820582763,24.1449129462601,124.917021763208)) ;
#21366=CARTESIAN_POINT('Ctrl Pts',(-19.2682080171776,24.3347435597455,124.609445253002)) ;
#21367=CARTESIAN_POINT('Ctrl Pts',(-19.2329600579686,24.1547544793826,124.90885452434)) ;
#21368=CARTESIAN_POINT('Ctrl Pts',(-19.0626517418926,24.3447298019652,124.566925901012)) ;
#21369=CARTESIAN_POINT('Ctrl Pts',(-18.9760140363379,24.1647407216023,124.855708116863)) ;
#21370=CARTESIAN_POINT('Ctrl Pts',(-18.8684666859137,24.3546664253901,124.489818172107)) ;
#21371=CARTESIAN_POINT('Ctrl Pts',(-18.7332816198796,24.1746773450272,124.759326036302)) ;
#21372=CARTESIAN_POINT('Ctrl Pts',(-18.688696650813,24.3647163027731,124.378854486706)) ;
#21373=CARTESIAN_POINT('Ctrl Pts',(-18.5085675410313,24.1847272224102,124.620623799681)) ;
#21374=CARTESIAN_POINT('Ctrl Pts',(-18.5339244507054,24.3745667415506,124.241242493615)) ;
#21375=CARTESIAN_POINT('Ctrl Pts',(-18.3151003354371,24.1945776611878,124.448610838)) ;
#21376=CARTESIAN_POINT('Ctrl Pts',(-18.4034080881523,24.3845387555194,124.077216087896)) ;
#21377=CARTESIAN_POINT('Ctrl Pts',(-18.1519526133633,24.2045496751565,124.243579488805)) ;
#21378=CARTESIAN_POINT('Ctrl Pts',(-18.3031188994434,24.3945339241455,123.892525344681)) ;
#21379=CARTESIAN_POINT('Ctrl Pts',(-18.0265886284109,24.2145448437826,124.012717326557)) ;
#21380=CARTESIAN_POINT('Ctrl Pts',(-18.2364182379383,24.4045678074067,123.692421879584)) ;
#21381=CARTESIAN_POINT('Ctrl Pts',(-17.9432101173695,24.2245787270438,123.762588848226)) ;
#21382=CARTESIAN_POINT('Ctrl Pts',(-18.2057083821517,24.41442367747,123.487493870639)) ;
#21383=CARTESIAN_POINT('Ctrl Pts',(-17.9048199953682,24.2344345971071,123.506429025599)) ;
#21384=CARTESIAN_POINT('Ctrl Pts',(-18.2107882331578,24.4244212233872,123.277398137475)) ;
#21385=CARTESIAN_POINT('Ctrl Pts',(-17.9111670277577,24.2444321430243,123.243809194865)) ;
#21386=CARTESIAN_POINT('Ctrl Pts',(-18.2518400342972,24.4343293502864,123.073174907185)) ;
#21387=CARTESIAN_POINT('Ctrl Pts',(-17.9624791058961,24.2543402699236,122.988529382377)) ;
#21388=CARTESIAN_POINT('Ctrl Pts',(-18.3281714579042,24.4443397218086,122.877045008902)) ;
#21389=CARTESIAN_POINT('Ctrl Pts',(-18.0578908532251,24.2643506414457,122.743365948088)) ;
#21390=CARTESIAN_POINT('Ctrl Pts',(-18.438010301051,24.454370164556,122.69704745568)) ;
#21391=CARTESIAN_POINT('Ctrl Pts',(-18.1951870356825,24.2743810841931,122.518367543358)) ;
#21392=CARTESIAN_POINT('Ctrl Pts',(-18.5745495647584,24.4642181171093,122.541397741827)) ;
#21393=CARTESIAN_POINT('Ctrl Pts',(-18.3658593160879,24.2842290367464,122.323803295538)) ;
#21394=CARTESIAN_POINT('Ctrl Pts',(-18.7394306699372,24.4742807861303,122.408888682602)) ;
#21395=CARTESIAN_POINT('Ctrl Pts',(-18.5719589574334,24.2942917057674,122.158164871478)) ;
#21396=CARTESIAN_POINT('Ctrl Pts',(-18.9218207597135,24.4841751615942,122.308835807993)) ;
#21397=CARTESIAN_POINT('Ctrl Pts',(-18.7999455381362,24.3041860812313,122.033096218261)) ;
#21398=CARTESIAN_POINT('Ctrl Pts',(-19.119533784816,24.4941169599123,122.241135188269)) ;
#21399=CARTESIAN_POINT('Ctrl Pts',(-19.0470862012802,24.3141278795495,121.948467825779)) ;
#21400=CARTESIAN_POINT('Ctrl Pts',(-19.327299776132,24.5041194536396,122.208506614829)) ;
#21401=CARTESIAN_POINT('Ctrl Pts',(-19.306793360523,24.3241303732768,121.9076794678)) ;
#21402=CARTESIAN_POINT('Ctrl Pts',(-19.5382060178291,24.5141542521466,122.212793291372)) ;
#21403=CARTESIAN_POINT('Ctrl Pts',(-19.5704262020177,24.3341651717837,121.913035104117)) ;
#21404=CARTESIAN_POINT('Ctrl Pts',(-19.741340693941,24.5239991361259,122.252526138907)) ;
#21405=CARTESIAN_POINT('Ctrl Pts',(-19.8243456090835,24.3440100557631,121.962698662003)) ;
#21406=CARTESIAN_POINT('Ctrl Pts',(-19.9373544726432,24.533984992944,122.327605162214)) ;
#21407=CARTESIAN_POINT('Ctrl Pts',(-20.069363913774,24.3539959125811,122.056545067836)) ;
#21408=CARTESIAN_POINT('Ctrl Pts',(-20.1165728966918,24.5439198071187,122.434935896096)) ;
#21409=CARTESIAN_POINT('Ctrl Pts',(-20.2933885436929,24.3639307267559,122.190706447143)) ;
#21410=CARTESIAN_POINT('Ctrl Pts',(-20.2762066027916,24.5539773069041,122.573540909043)) ;
#21411=CARTESIAN_POINT('Ctrl Pts',(-20.4929322997301,24.3739882265412,122.363960667453)) ;
#21412=CARTESIAN_POINT('Ctrl Pts',(-20.4065058320593,24.5637990653224,122.733750397852)) ;
#21413=CARTESIAN_POINT('Ctrl Pts',(-20.6558088061112,24.3838099849595,122.564221525997)) ;
#21414=CARTESIAN_POINT('Ctrl Pts',(-20.5097290699146,24.5738547231064,122.918217818253)) ;
#21415=CARTESIAN_POINT('Ctrl Pts',(-20.7848399620391,24.3938656427435,122.794804496023)) ;
#21416=CARTESIAN_POINT('Ctrl Pts',(-20.5782202375852,24.5837969052864,123.115704900593)) ;
#21417=CARTESIAN_POINT('Ctrl Pts',(-20.8704564403244,24.4038078249235,123.041662828752)) ;
#21418=CARTESIAN_POINT('Ctrl Pts',(-20.6118814894185,24.5937021139811,123.32120168517)) ;
#21419=CARTESIAN_POINT('Ctrl Pts',(-20.9125354801232,24.4137130336182,123.298533938)) ;
#21420=CARTESIAN_POINT('Ctrl Pts',(-20.6092481539705,24.6037439049435,123.532291786237)) ;
#21421=CARTESIAN_POINT('Ctrl Pts',(-20.909246248355,24.4237548245807,123.562396507273)) ;
#21422=CARTESIAN_POINT('Ctrl Pts',(-20.5705464706402,24.6136516794158,123.73696556278)) ;
#21423=CARTESIAN_POINT('Ctrl Pts',(-20.8608714359243,24.4336625990529,123.818239689833)) ;
#21424=CARTESIAN_POINT('Ctrl Pts',(-20.4964883343986,24.6236631796434,123.933985160015)) ;
#21425=CARTESIAN_POINT('Ctrl Pts',(-20.7683009426795,24.4436740992805,124.064515066611)) ;
#21426=CARTESIAN_POINT('Ctrl Pts',(-20.388743463947,24.6336959400361,124.115308071487)) ;
#21427=CARTESIAN_POINT('Ctrl Pts',(-20.6336219825576,24.4537068596732,124.291169915681)) ;
#21428=CARTESIAN_POINT('Ctrl Pts',(-20.2539226961547,24.643546509171,124.272507133189)) ;
#21429=CARTESIAN_POINT('Ctrl Pts',(-20.4650972755638,24.4635574288081,124.487670909562)) ;
#21430=CARTESIAN_POINT('Ctrl Pts',(-20.0918811514129,24.6535351187009,124.406043156148)) ;
#21431=CARTESIAN_POINT('Ctrl Pts',(-20.262546647733,24.473546038338,124.654592807145)) ;
#21432=CARTESIAN_POINT('Ctrl Pts',(-19.9101907899771,24.663463774725,124.50880446125)) ;
#21433=CARTESIAN_POINT('Ctrl Pts',(-20.035434390892,24.4834746943621,124.783046651201)) ;
#21434=CARTESIAN_POINT('Ctrl Pts',(-19.7123608153397,24.6734515209028,124.579209070927)) ;
#21435=CARTESIAN_POINT('Ctrl Pts',(-19.788147480938,24.4934624405399,124.871054527459)) ;
#21436=CARTESIAN_POINT('Ctrl Pts',(-19.504271624768,24.6834875098385,124.614009588062)) ;
#21437=CARTESIAN_POINT('Ctrl Pts',(-19.5280364525962,24.5034984294756,124.914557400059)) ;
#21438=CARTESIAN_POINT('Ctrl Pts',(-19.2970799984549,24.6933423796521,124.612527488624)) ;
#21439=CARTESIAN_POINT('Ctrl Pts',(-19.2690459880752,24.5133532992892,124.912706949231)) ;
#21440=CARTESIAN_POINT('Ctrl Pts',(-19.090303135345,24.7033418208939,124.574834044645)) ;
#21441=CARTESIAN_POINT('Ctrl Pts',(-19.0105743992336,24.523352740531,124.865592193593)) ;
#21442=CARTESIAN_POINT('Ctrl Pts',(-18.8951262772354,24.713236895074,124.502757695016)) ;
#21443=CARTESIAN_POINT('Ctrl Pts',(-18.7666019329129,24.5332478147111,124.775498416424)) ;
#21444=CARTESIAN_POINT('Ctrl Pts',(-18.7124871130711,24.7232975509137,124.396143715782)) ;
#21445=CARTESIAN_POINT('Ctrl Pts',(-18.5383021509909,24.5433084705508,124.642232833805)) ;
#21446=CARTESIAN_POINT('Ctrl Pts',(-18.5544214010454,24.7331464251093,124.262378682155)) ;
#21447=CARTESIAN_POINT('Ctrl Pts',(-18.3407179161461,24.5531573447464,124.475027408876)) ;
#21448=CARTESIAN_POINT('Ctrl Pts',(-18.4191678408928,24.7431751370725,124.100648450517)) ;
#21449=CARTESIAN_POINT('Ctrl Pts',(-18.1716495641239,24.5631860567097,124.272865839476)) ;
#21450=CARTESIAN_POINT('Ctrl Pts',(-18.3145372263734,24.7532045376556,123.917586468341)) ;
#21451=CARTESIAN_POINT('Ctrl Pts',(-18.0408595712216,24.5732154572928,124.044039432676)) ;
#21452=CARTESIAN_POINT('Ctrl Pts',(-18.2441926662311,24.7630447312725,123.723038994785)) ;
#21453=CARTESIAN_POINT('Ctrl Pts',(-17.9529267054046,24.5830556509096,123.80085466428)) ;
#21454=CARTESIAN_POINT('Ctrl Pts',(-18.2077279525062,24.7730481538477,123.515942344631)) ;
#21455=CARTESIAN_POINT('Ctrl Pts',(-17.9073440510645,24.5930590734848,123.541984051105)) ;
#21456=CARTESIAN_POINT('Ctrl Pts',(-18.2078442834315,24.7830336909408,123.305979629472)) ;
#21457=CARTESIAN_POINT('Ctrl Pts',(-17.9074876720707,24.6030446105779,123.279530447817)) ;
#21458=CARTESIAN_POINT('Ctrl Pts',(-18.244816810972,24.7930746954276,123.098169474309)) ;
#21459=CARTESIAN_POINT('Ctrl Pts',(-17.953701474388,24.6130856150647,123.019767558698)) ;
#21460=CARTESIAN_POINT('Ctrl Pts',(-18.3156319158811,24.8029182343688,122.903704450163)) ;
#21461=CARTESIAN_POINT('Ctrl Pts',(-18.0422190940517,24.6229291540059,122.776684574555)) ;
#21462=CARTESIAN_POINT('Ctrl Pts',(-18.4202205854455,24.8129032653596,122.721733922501)) ;
#21463=CARTESIAN_POINT('Ctrl Pts',(-18.1729536422505,24.6329141849967,122.549220386111)) ;
#21464=CARTESIAN_POINT('Ctrl Pts',(-18.5541770056788,24.8228427278816,122.561322433432)) ;
#21465=CARTESIAN_POINT('Ctrl Pts',(-18.3403982888488,24.6428536475187,122.348704583029)) ;
#21466=CARTESIAN_POINT('Ctrl Pts',(-18.715558190906,24.8328824601054,122.425314061368)) ;
#21467=CARTESIAN_POINT('Ctrl Pts',(-18.5421236161833,24.6528933797425,122.178692975382)) ;
#21468=CARTESIAN_POINT('Ctrl Pts',(-18.8953205226514,24.8427706404226,122.320888321674)) ;
#21469=CARTESIAN_POINT('Ctrl Pts',(-18.766826532383,24.6627815600597,122.048158969798)) ;
#21470=CARTESIAN_POINT('Ctrl Pts',(-19.0923303882549,24.8527601561251,122.248163396936)) ;
#21471=CARTESIAN_POINT('Ctrl Pts',(-19.0130885634454,24.6727710757622,121.957251380598)) ;
#21472=CARTESIAN_POINT('Ctrl Pts',(-19.298364039197,24.8627187067798,122.211026101757)) ;
#21473=CARTESIAN_POINT('Ctrl Pts',(-19.2706307855915,24.6827296264169,121.910828202634)) ;
#21474=CARTESIAN_POINT('Ctrl Pts',(-19.5064905058478,24.8726181138848,122.209713205834)) ;
#21475=CARTESIAN_POINT('Ctrl Pts',(-19.5307897392351,24.6926290335219,121.909185754216)) ;
#21476=CARTESIAN_POINT('Ctrl Pts',(-19.7147219092595,24.8826667003011,122.245162774326)) ;
#21477=CARTESIAN_POINT('Ctrl Pts',(-19.7910790035536,24.7026776199382,121.953496342207)) ;
#21478=CARTESIAN_POINT('Ctrl Pts',(-19.9106826139148,24.8925595192655,122.314960468538)) ;
#21479=CARTESIAN_POINT('Ctrl Pts',(-20.0360311856884,24.7125704389027,122.040742561825)) ;
#21480=CARTESIAN_POINT('Ctrl Pts',(-20.0946951962707,24.9026306367953,122.41960013013)) ;
#21481=CARTESIAN_POINT('Ctrl Pts',(-20.2660472328048,24.7226415564325,122.171540812148)) ;
#21482=CARTESIAN_POINT('Ctrl Pts',(-20.2538475997201,24.9124463307614,122.551014009269)) ;
#21483=CARTESIAN_POINT('Ctrl Pts',(-20.4649896868534,24.7324572503985,122.33580820644)) ;
#21484=CARTESIAN_POINT('Ctrl Pts',(-20.3913621573758,24.9225127082587,122.711814363181)) ;
#21485=CARTESIAN_POINT('Ctrl Pts',(-20.6368834830163,24.7425236278958,122.536807653796)) ;
#21486=CARTESIAN_POINT('Ctrl Pts',(-20.4970748886783,24.9324116943406,122.891133137665)) ;
#21487=CARTESIAN_POINT('Ctrl Pts',(-20.7690258159267,24.7524226139777,122.760956322212)) ;
#21488=CARTESIAN_POINT('Ctrl Pts',(-20.571232101278,24.9424658743341,123.089018879175)) ;
#21489=CARTESIAN_POINT('Ctrl Pts',(-20.8617232642626,24.7624767939712,123.008312860307)) ;
#21490=CARTESIAN_POINT('Ctrl Pts',(-20.6094160911567,24.9523366872668,123.293040667745)) ;
#21491=CARTESIAN_POINT('Ctrl Pts',(-20.9094544648808,24.7723476069039,123.263341038962)) ;
#21492=CARTESIAN_POINT('Ctrl Pts',(-20.6116329545151,24.9624105881206,123.504764653356)) ;
#21493=CARTESIAN_POINT('Ctrl Pts',(-20.9122265609454,24.7824215077577,123.527995577717)) ;
#21494=CARTESIAN_POINT('Ctrl Pts',(-20.5781600299015,24.9722307435072,123.708532107742)) ;
#21495=CARTESIAN_POINT('Ctrl Pts',(-20.8703860648763,24.7922416631444,123.782706579754)) ;
#21496=CARTESIAN_POINT('Ctrl Pts',(-20.508237892881,24.9823094504595,123.908493710654)) ;
#21497=CARTESIAN_POINT('Ctrl Pts',(-20.7829843523247,24.8023203700966,124.032658419494)) ;
#21498=CARTESIAN_POINT('Ctrl Pts',(-20.4070053264551,24.9921610389983,124.089234851178)) ;
#21499=CARTESIAN_POINT('Ctrl Pts',(-20.6564437174401,24.8121719586354,124.258586397133)) ;
#21500=CARTESIAN_POINT('Ctrl Pts',(-20.2731799394624,25.0022341555233,124.253310305418)) ;
#21501=CARTESIAN_POINT('Ctrl Pts',(-20.4891628443996,24.8222450751604,124.463680852311)) ;
#21502=CARTESIAN_POINT('Ctrl Pts',(-20.1165044718704,25.0120766726191,124.388500704501)) ;
#21503=CARTESIAN_POINT('Ctrl Pts',(-20.2933179390205,24.8320875922562,124.632670356776)) ;
#21504=CARTESIAN_POINT('Ctrl Pts',(-19.936630039934,25.022057134173,124.496508778481)) ;
#21505=CARTESIAN_POINT('Ctrl Pts',(-20.0684748873038,24.8420680538102,124.767681031673)) ;
#21506=CARTESIAN_POINT('Ctrl Pts',(-19.7398406206067,25.0320753841638,124.571552225653)) ;
#21507=CARTESIAN_POINT('Ctrl Pts',(-19.8224883546883,24.8520863038009,124.861485946865)) ;
#21508=CARTESIAN_POINT('Ctrl Pts',(-19.5358376882034,25.0419595443576,124.611179719753)) ;
#21509=CARTESIAN_POINT('Ctrl Pts',(-19.5674837085229,24.8619704639947,124.911020996683)) ;
#21510=CARTESIAN_POINT('Ctrl Pts',(-19.3242913071813,25.0520246913326,124.614802833866)) ;
#21511=CARTESIAN_POINT('Ctrl Pts',(-19.3030511330044,24.8720356109697,124.915550386411)) ;
#21512=CARTESIAN_POINT('Ctrl Pts',(-19.1199106240367,25.0618665149734,124.582483950528)) ;
#21513=CARTESIAN_POINT('Ctrl Pts',(-19.0475737608601,24.8818774346105,124.875152002711)) ;
#21514=CARTESIAN_POINT('Ctrl Pts',(-18.9203492375791,25.0718959874342,124.514427752027)) ;
#21515=CARTESIAN_POINT('Ctrl Pts',(-18.7981220481967,24.8919069070713,124.790082006543)) ;
#21516=CARTESIAN_POINT('Ctrl Pts',(-18.7359613362089,25.0819228426962,124.412260699821)) ;
#21517=CARTESIAN_POINT('Ctrl Pts',(-18.5676370265376,24.9019337623334,124.662373648599)) ;
#21518=CARTESIAN_POINT('Ctrl Pts',(-18.5748042640139,25.0917660928068,124.282445342146)) ;
#21519=CARTESIAN_POINT('Ctrl Pts',(-18.3661893963596,24.9117770124439,124.500103756191)) ;
#21520=CARTESIAN_POINT('Ctrl Pts',(-18.4355859909014,25.1018145323899,124.123567079919)) ;
#21521=CARTESIAN_POINT('Ctrl Pts',(-18.1921666070184,24.9218254520271,124.30150622892)) ;
#21522=CARTESIAN_POINT('Ctrl Pts',(-18.3274272880711,25.1117640266378,123.944530772977)) ;
#21523=CARTESIAN_POINT('Ctrl Pts',(-18.056967678217,24.931774946275,124.077710500125)) ;
#21524=CARTESIAN_POINT('Ctrl Pts',(-18.2517272644222,25.1216718823638,123.750467023187)) ;
#21525=CARTESIAN_POINT('Ctrl Pts',(-17.9623422828139,24.941682802001,123.835129981)) ;
#21526=CARTESIAN_POINT('Ctrl Pts',(-18.2104743970335,25.1317313590138,123.543070104516)) ;
#21527=CARTESIAN_POINT('Ctrl Pts',(-17.9107761380726,24.9517422786509,123.575884197323)) ;
#21528=CARTESIAN_POINT('Ctrl Pts',(-18.2056782190192,25.1415721684225,123.336215569633)) ;
#21529=CARTESIAN_POINT('Ctrl Pts',(-17.9047808645182,24.9615830880596,123.317314560702)) ;
#21530=CARTESIAN_POINT('Ctrl Pts',(-18.2373040930332,25.1516343187233,123.127077183961)) ;
#21531=CARTESIAN_POINT('Ctrl Pts',(-17.9443132377084,24.9716452383604,123.055891956674)) ;
#21532=CARTESIAN_POINT('Ctrl Pts',(-18.3038712513499,25.1615314798458,122.929932299027)) ;
#21533=CARTESIAN_POINT('Ctrl Pts',(-18.027522505227,24.981542399483,122.809459900675)) ;
#21534=CARTESIAN_POINT('Ctrl Pts',(-18.4033840340755,25.1714626542499,122.746394261675)) ;
#21535=CARTESIAN_POINT('Ctrl Pts',(-18.15191407074,24.991473573887,122.580036852208)) ;
#21536=CARTESIAN_POINT('Ctrl Pts',(-18.534887670248,25.1815048579749,122.581237562845)) ;
#21537=CARTESIAN_POINT('Ctrl Pts',(-18.3162936300384,25.001515777612,122.373591256392)) ;
#21538=CARTESIAN_POINT('Ctrl Pts',(-18.690527647173,25.1913914404053,122.443467269935)) ;
#21539=CARTESIAN_POINT('Ctrl Pts',(-18.5108445770742,25.0114023600425,122.201377852405)) ;
#21540=CARTESIAN_POINT('Ctrl Pts',(-18.8694400895696,25.2013848761537,122.333355299341)) ;
#21541=CARTESIAN_POINT('Ctrl Pts',(-18.7344855027603,25.0213957957908,122.063738108185)) ;
#21542=CARTESIAN_POINT('Ctrl Pts',(-19.0638333349581,25.2113293445118,122.256415312659)) ;
#21543=CARTESIAN_POINT('Ctrl Pts',(-18.9774777481212,25.031340264149,121.967563232072)) ;
#21544=CARTESIAN_POINT('Ctrl Pts',(-19.2687117383254,25.2212811607574,122.213977770171)) ;
#21545=CARTESIAN_POINT('Ctrl Pts',(-19.2335763972328,25.0412920803945,121.914516693683)) ;
#21546=CARTESIAN_POINT('Ctrl Pts',(-19.4796320217027,25.2313185968719,122.207898426795)) ;
#21547=CARTESIAN_POINT('Ctrl Pts',(-19.4972265998584,25.051329516509,121.906917954592)) ;
#21548=CARTESIAN_POINT('Ctrl Pts',(-19.6852897576632,25.2412035560482,122.237873411144)) ;
#21549=CARTESIAN_POINT('Ctrl Pts',(-19.7542997604475,25.0612144756854,121.944387345544)) ;
#21550=CARTESIAN_POINT('Ctrl Pts',(-19.8849152260127,25.2512016742602,122.303598681316)) ;
#21551=CARTESIAN_POINT('Ctrl Pts',(-20.0038315528282,25.0712125938973,122.026544562977)) ;
#21552=CARTESIAN_POINT('Ctrl Pts',(-20.0687767747122,25.2611226067721,122.402114690331)) ;
#21553=CARTESIAN_POINT('Ctrl Pts',(-20.2336588620757,25.0811335264093,122.149690526495)) ;
#21554=CARTESIAN_POINT('Ctrl Pts',(-20.2347377539777,25.2711639069942,122.532559750854)) ;
#21555=CARTESIAN_POINT('Ctrl Pts',(-20.4411095234431,25.0911748266313,122.31274727971)) ;
#21556=CARTESIAN_POINT('Ctrl Pts',(-20.3735985016344,25.2810708253842,122.687791031638)) ;
#21557=CARTESIAN_POINT('Ctrl Pts',(-20.6146855652456,25.1010817450213,122.506787487702)) ;
#21558=CARTESIAN_POINT('Ctrl Pts',(-20.4842246461165,25.2910066170932,122.864973861521)) ;
#21559=CARTESIAN_POINT('Ctrl Pts',(-20.7529678400047,25.1110175367304,122.728267052382)) ;
#21560=CARTESIAN_POINT('Ctrl Pts',(-20.5630324165797,25.3010475116711,123.060797396838)) ;
#21561=CARTESIAN_POINT('Ctrl Pts',(-20.8514767358832,25.1210584313083,122.973046599286)) ;
#21562=CARTESIAN_POINT('Ctrl Pts',(-20.6061255781903,25.310934713385,123.264152339049)) ;
#21563=CARTESIAN_POINT('Ctrl Pts',(-20.9053425589782,25.1309456330221,123.227241473632)) ;
#21564=CARTESIAN_POINT('Ctrl Pts',(-20.6136784836377,25.3209269811466,123.474070984614)) ;
#21565=CARTESIAN_POINT('Ctrl Pts',(-20.9147827032288,25.1409379007837,123.489640019812)) ;
#21566=CARTESIAN_POINT('Ctrl Pts',(-20.5847340091675,25.3308755021684,123.681219469277)) ;
#21567=CARTESIAN_POINT('Ctrl Pts',(-20.8786010725189,25.1508864218055,123.748576028363)) ;
#21568=CARTESIAN_POINT('Ctrl Pts',(-20.5206272668833,25.3408122757461,123.880023760585)) ;
#21569=CARTESIAN_POINT('Ctrl Pts',(-20.7984664179347,25.1608231953832,123.997081667606)) ;
#21570=CARTESIAN_POINT('Ctrl Pts',(-20.4227342551937,25.3507953238871,124.065699360491)) ;
#21571=CARTESIAN_POINT('Ctrl Pts',(-20.6760989906385,25.1708062435242,124.229175844446)) ;
#21572=CARTESIAN_POINT('Ctrl Pts',(-20.2930330978776,25.3608390314972,124.232290893968)) ;
#21573=CARTESIAN_POINT('Ctrl Pts',(-20.5139718407011,25.1808499511343,124.437414474404)) ;
#21574=CARTESIAN_POINT('Ctrl Pts',(-20.1400132496701,25.3706677246505,124.3711852769)) ;
#21575=CARTESIAN_POINT('Ctrl Pts',(-20.3226951495202,25.1906786442876,124.611032523133)) ;
#21576=CARTESIAN_POINT('Ctrl Pts',(-19.9609525577094,25.3807424737799,124.484253952446)) ;
#21577=CARTESIAN_POINT('Ctrl Pts',(-20.098868954127,25.200753393417,124.752367074633)) ;
#21578=CARTESIAN_POINT('Ctrl Pts',(-19.7689867735879,25.3906077995755,124.56282261199)) ;
#21579=CARTESIAN_POINT('Ctrl Pts',(-19.858910190644,25.2106187192126,124.850577176108)) ;
#21580=CARTESIAN_POINT('Ctrl Pts',(-19.5632165090055,25.4006299739324,124.608087313352)) ;
#21581=CARTESIAN_POINT('Ctrl Pts',(-19.6016970937392,25.2206408935695,124.907156637884)) ;
#21582=CARTESIAN_POINT('Ctrl Pts',(-19.3525876909076,25.4106560271393,124.616422421431)) ;
#21583=CARTESIAN_POINT('Ctrl Pts',(-19.33841109203,25.2306669467765,124.91757426496)) ;
#21584=CARTESIAN_POINT('Ctrl Pts',(-19.147287360646,25.4205097239856,124.588883432483)) ;
#21585=CARTESIAN_POINT('Ctrl Pts',(-19.0817846505437,25.2405206436227,124.883149004069)) ;
#21586=CARTESIAN_POINT('Ctrl Pts',(-18.9475566685195,25.4304691287386,124.526036690547)) ;
#21587=CARTESIAN_POINT('Ctrl Pts',(-18.8321213569949,25.2504800483757,124.804588928289)) ;
#21588=CARTESIAN_POINT('Ctrl Pts',(-18.7604916580374,25.4405073744435,124.428375640314)) ;
#21589=CARTESIAN_POINT('Ctrl Pts',(-18.5982908950502,25.2605182940806,124.68251138002)) ;
#21590=CARTESIAN_POINT('Ctrl Pts',(-18.5957013870381,25.4503815586055,124.302092265061)) ;
#21591=CARTESIAN_POINT('Ctrl Pts',(-18.3923032184799,25.2703924782426,124.52465527997)) ;
#21592=CARTESIAN_POINT('Ctrl Pts',(-18.4526055536538,25.4604513417434,124.146119088409)) ;
#21593=CARTESIAN_POINT('Ctrl Pts',(-18.2134348354326,25.2804622613806,124.32968799242)) ;
#21594=CARTESIAN_POINT('Ctrl Pts',(-18.3413212778129,25.4702845967642,123.971882300025)) ;
#21595=CARTESIAN_POINT('Ctrl Pts',(-18.0743301698985,25.2902955164013,124.111890050986)) ;
#21596=CARTESIAN_POINT('Ctrl Pts',(-18.2598482943526,25.4803150228959,123.777393425404)) ;
#21597=CARTESIAN_POINT('Ctrl Pts',(-17.9724906536207,25.300325942533,123.868778335182)) ;
#21598=CARTESIAN_POINT('Ctrl Pts',(-18.2139714522043,25.4903466350829,123.571535696539)) ;
#21599=CARTESIAN_POINT('Ctrl Pts',(-17.9151462002579,25.31035755472,123.611455902983)) ;
#21600=CARTESIAN_POINT('Ctrl Pts',(-18.2042958256806,25.5001763319375,123.365125390913)) ;
#21601=CARTESIAN_POINT('Ctrl Pts',(-17.9030533678709,25.3201872515746,123.353441667699)) ;
#21602=CARTESIAN_POINT('Ctrl Pts',(-18.2304147172978,25.51016577384,123.156740327135)) ;
#21603=CARTESIAN_POINT('Ctrl Pts',(-17.935703946638,25.3301766934771,123.092960405583)) ;
#21604=CARTESIAN_POINT('Ctrl Pts',(-18.2931661314917,25.5202096658556,122.955127632222)) ;
#21605=CARTESIAN_POINT('Ctrl Pts',(-18.01414488107,25.3402205854928,122.840945210804)) ;
#21606=CARTESIAN_POINT('Ctrl Pts',(-18.3874495319765,25.5300312276249,122.771432509652)) ;
#21607=CARTESIAN_POINT('Ctrl Pts',(-18.1320014123289,25.350042147262,122.611326074322)) ;
#21608=CARTESIAN_POINT('Ctrl Pts',(-18.5144967250623,25.5400667992491,122.60299121237)) ;
#21609=CARTESIAN_POINT('Ctrl Pts',(-18.290812004256,25.3600777188862,122.400775785575)) ;
#21610=CARTESIAN_POINT('Ctrl Pts',(-18.669193308683,25.5500960735309,122.459723633636)) ;
#21611=CARTESIAN_POINT('Ctrl Pts',(-18.4841839838092,25.370106993168,122.221692735608)) ;
#21612=CARTESIAN_POINT('Ctrl Pts',(-18.8426660315161,25.5599299106495,122.34725013946)) ;
#21613=CARTESIAN_POINT('Ctrl Pts',(-18.7010269361118,25.3799408302867,122.081101987193)) ;
#21614=CARTESIAN_POINT('Ctrl Pts',(-19.0371487210636,25.5699823067377,122.26458450001)) ;
#21615=CARTESIAN_POINT('Ctrl Pts',(-18.9441309444256,25.3899932263748,121.977771975232)) ;
#21616=CARTESIAN_POINT('Ctrl Pts',(-19.2407432881081,25.5799190736882,122.217749926032)) ;
#21617=CARTESIAN_POINT('Ctrl Pts',(-19.1986250893084,25.3999299933253,121.919230643914)) ;
#21618=CARTESIAN_POINT('Ctrl Pts',(-19.4492836308601,25.5898533086675,122.206441411571)) ;
#21619=CARTESIAN_POINT('Ctrl Pts',(-19.459301128586,25.4098642283046,121.905097168243)) ;
#21620=CARTESIAN_POINT('Ctrl Pts',(-19.6584731388207,25.5998770719943,122.231868584206)) ;
#21621=CARTESIAN_POINT('Ctrl Pts',(-19.72078773703,25.4198879916314,121.936883279556)) ;
#21622=CARTESIAN_POINT('Ctrl Pts',(-19.8573510139272,25.6097634133789,122.292244191361)) ;
#21623=CARTESIAN_POINT('Ctrl Pts',(-19.9693851432808,25.429774333016,122.012355109386)) ;
#21624=CARTESIAN_POINT('Ctrl Pts',(-20.0448786077411,25.6197524621459,122.386778679778)) ;
#21625=CARTESIAN_POINT('Ctrl Pts',(-20.2037937296493,25.439763381783,122.130525368287)) ;
#21626=CARTESIAN_POINT('Ctrl Pts',(-20.2137531182518,25.6297936828433,122.513441376923)) ;
#21627=CARTESIAN_POINT('Ctrl Pts',(-20.4148854638875,25.4498046024804,122.288855457116)) ;
#21628=CARTESIAN_POINT('Ctrl Pts',(-20.3553169833918,25.6396263230212,122.664067992544)) ;
#21629=CARTESIAN_POINT('Ctrl Pts',(-20.5918392755866,25.4596372426583,122.477141002139)) ;
#21630=CARTESIAN_POINT('Ctrl Pts',(-20.4709395710573,25.6496202523291,122.839494815761)) ;
#21631=CARTESIAN_POINT('Ctrl Pts',(-20.7363655379612,25.4696311719663,122.696425976588)) ;
#21632=CARTESIAN_POINT('Ctrl Pts',(-20.5542313166204,25.6596494600097,123.033193067616)) ;
#21633=CARTESIAN_POINT('Ctrl Pts',(-20.8404780632738,25.4796603796468,122.93854969465)) ;
#21634=CARTESIAN_POINT('Ctrl Pts',(-20.6022166705038,25.6695252717138,123.235204192602)) ;
#21635=CARTESIAN_POINT('Ctrl Pts',(-20.9004575630717,25.4895361913509,123.191064817286)) ;
#21636=CARTESIAN_POINT('Ctrl Pts',(-20.6147777399099,25.6795244986852,123.445015641522)) ;
#21637=CARTESIAN_POINT('Ctrl Pts',(-20.9161564441938,25.4995354183223,123.453329386861)) ;
#21638=CARTESIAN_POINT('Ctrl Pts',(-20.5911250967984,25.6894339798409,123.652027739966)) ;
#21639=CARTESIAN_POINT('Ctrl Pts',(-20.8865881009697,25.509444899478,123.712094698215)) ;
#21640=CARTESIAN_POINT('Ctrl Pts',(-20.531017224915,25.6994872101418,123.854627589131)) ;
#21641=CARTESIAN_POINT('Ctrl Pts',(-20.81145089258,25.5194981297789,123.965343699702)) ;
#21642=CARTESIAN_POINT('Ctrl Pts',(-20.4384325667578,25.7093578266928,124.040355450809)) ;
#21643=CARTESIAN_POINT('Ctrl Pts',(-20.6957175422055,25.52936874633,124.197502953534)) ;
#21644=CARTESIAN_POINT('Ctrl Pts',(-20.3135029459365,25.7193794884249,124.210003208649)) ;
#21645=CARTESIAN_POINT('Ctrl Pts',(-20.5395534186836,25.539390408062,124.409561109384)) ;
#21646=CARTESIAN_POINT('Ctrl Pts',(-20.1606542811385,25.729402301606,124.355058412312)) ;
#21647=CARTESIAN_POINT('Ctrl Pts',(-20.3484908449209,25.5494132212431,124.590878299816)) ;
#21648=CARTESIAN_POINT('Ctrl Pts',(-19.9878788008662,25.7392694660659,124.469843004655)) ;
#21649=CARTESIAN_POINT('Ctrl Pts',(-20.1325195803171,25.5592803857031,124.734357216796)) ;
#21650=CARTESIAN_POINT('Ctrl Pts',(-19.7955437673314,25.7492629082859,124.554394992238)) ;
#21651=CARTESIAN_POINT('Ctrl Pts',(-19.8920996177146,25.569273827923,124.840044812153)) ;
#21652=CARTESIAN_POINT('Ctrl Pts',(-19.5905777687678,25.7592945818862,124.604056660559)) ;
#21653=CARTESIAN_POINT('Ctrl Pts',(-19.6358915111173,25.5793055015233,124.902119378316)) ;
#21654=CARTESIAN_POINT('Ctrl Pts',(-19.3835799225067,25.7691610169992,124.617474520566)) ;
#21655=CARTESIAN_POINT('Ctrl Pts',(-19.377143513442,25.5891719366363,124.918889100785)) ;
#21656=CARTESIAN_POINT('Ctrl Pts',(-19.1748644935385,25.7791484675323,124.594811648332)) ;
#21657=CARTESIAN_POINT('Ctrl Pts',(-19.1162493958071,25.5991593871694,124.890557819024)) ;
#21658=CARTESIAN_POINT('Ctrl Pts',(-18.9740276761385,25.7890933973602,124.536594188768)) ;
#21659=CARTESIAN_POINT('Ctrl Pts',(-18.8652039002789,25.6091043169973,124.817783333034)) ;
#21660=CARTESIAN_POINT('Ctrl Pts',(-18.7845612887665,25.7991382924153,124.443378041818)) ;
#21661=CARTESIAN_POINT('Ctrl Pts',(-18.6283721225821,25.6191492120525,124.701260743701)) ;
#21662=CARTESIAN_POINT('Ctrl Pts',(-18.6171242290503,25.8090003541012,124.321077049524)) ;
#21663=CARTESIAN_POINT('Ctrl Pts',(-18.419077049514,25.6290112737383,124.548382059341)) ;
#21664=CARTESIAN_POINT('Ctrl Pts',(-18.4712964694787,25.818992076888,124.169910090686)) ;
#21665=CARTESIAN_POINT('Ctrl Pts',(-18.2367942709095,25.6390029965252,124.359421375143)) ;
#21666=CARTESIAN_POINT('Ctrl Pts',(-18.3546829235641,25.828924291128,123.996697923502)) ;
#21667=CARTESIAN_POINT('Ctrl Pts',(-18.091029495205,25.6489352107651,124.142904444548)) ;
#21668=CARTESIAN_POINT('Ctrl Pts',(-18.269414013462,25.8388636096937,123.805925409421)) ;
#21669=CARTESIAN_POINT('Ctrl Pts',(-17.9844458363519,25.6588745293309,123.904437503963)) ;
#21670=CARTESIAN_POINT('Ctrl Pts',(-18.2182183799845,25.8489077844696,123.601068446955)) ;
#21671=CARTESIAN_POINT('Ctrl Pts',(-17.9204539831751,25.6689187041067,123.648365609469)) ;
#21672=CARTESIAN_POINT('Ctrl Pts',(-18.2035144290787,25.8587783385346,123.394080423168)) ;
#21673=CARTESIAN_POINT('Ctrl Pts',(-17.9020768058315,25.6787892581717,123.389630116784)) ;
#21674=CARTESIAN_POINT('Ctrl Pts',(-18.2245755858917,25.8687433208888,123.185646036697)) ;
#21675=CARTESIAN_POINT('Ctrl Pts',(-17.9284060681277,25.6887542405259,123.1290873224)) ;
#21676=CARTESIAN_POINT('Ctrl Pts',(-18.2821927216553,25.8787740237786,122.982799143705)) ;
#21677=CARTESIAN_POINT('Ctrl Pts',(-18.000430199717,25.6987849434157,122.875529417126)) ;
#21678=CARTESIAN_POINT('Ctrl Pts',(-18.3726282398812,25.8886663638038,122.795495732635)) ;
#21679=CARTESIAN_POINT('Ctrl Pts',(-18.1134771988756,25.7086772834409,122.641401239108)) ;
#21680=CARTESIAN_POINT('Ctrl Pts',(-18.4961390189177,25.8987195969637,122.624026714153)) ;
#21681=CARTESIAN_POINT('Ctrl Pts',(-18.2678679863379,25.7187305166009,122.427066576845)) ;
#21682=CARTESIAN_POINT('Ctrl Pts',(-18.6449144456404,25.9086008414405,122.478993547401)) ;
#21683=CARTESIAN_POINT('Ctrl Pts',(-18.4538393268546,25.7286117610776,122.245777047898)) ;
#21684=CARTESIAN_POINT('Ctrl Pts',(-18.8191018734821,25.9186339623115,122.36011093306)) ;
#21685=CARTESIAN_POINT('Ctrl Pts',(-18.6715752593228,25.7386448819486,122.097176077592)) ;
#21686=CARTESIAN_POINT('Ctrl Pts',(-19.0083693285525,25.9285151725866,122.274392628594)) ;
#21687=CARTESIAN_POINT('Ctrl Pts',(-18.9081608033064,25.7485260922237,121.990030737852)) ;
#21688=CARTESIAN_POINT('Ctrl Pts',(-19.2132442732851,25.9385772483559,122.221858172896)) ;
#21689=CARTESIAN_POINT('Ctrl Pts',(-19.1642552672847,25.758588167993,121.924365385186)) ;
#21690=CARTESIAN_POINT('Ctrl Pts',(-19.41988850403,25.9484343067377,122.205946244502)) ;
#21691=CARTESIAN_POINT('Ctrl Pts',(-19.4225607860531,25.7684452263748,121.904478285387)) ;
#21692=CARTESIAN_POINT('Ctrl Pts',(-19.6290114818218,25.9584288620267,122.226010291668)) ;
#21693=CARTESIAN_POINT('Ctrl Pts',(-19.6839642883553,25.7784397816638,121.929561151871)) ;
#21694=CARTESIAN_POINT('Ctrl Pts',(-19.8301627349406,25.9683547495622,122.281640275295)) ;
#21695=CARTESIAN_POINT('Ctrl Pts',(-19.9354025958823,25.7883656691993,121.999101330404)) ;
#21696=CARTESIAN_POINT('Ctrl Pts',(-20.0204672700362,25.9783797695574,122.372173587935)) ;
#21697=CARTESIAN_POINT('Ctrl Pts',(-20.1732821454297,25.7983906891946,122.112270545144)) ;
#21698=CARTESIAN_POINT('Ctrl Pts',(-20.1900359400144,25.9882771466611,122.492771224812)) ;
#21699=CARTESIAN_POINT('Ctrl Pts',(-20.3852412939983,25.8082880662982,122.26301982624)) ;
#21700=CARTESIAN_POINT('Ctrl Pts',(-20.3377857345997,25.998267383742,122.642047679255)) ;
#21701=CARTESIAN_POINT('Ctrl Pts',(-20.5699265939808,25.8182783033791,122.449617357553)) ;
#21702=CARTESIAN_POINT('Ctrl Pts',(-20.4575881124741,26.0083039965508,122.815736066675)) ;
#21703=CARTESIAN_POINT('Ctrl Pts',(-20.7196773404664,25.8283149161879,122.666729559919)) ;
#21704=CARTESIAN_POINT('Ctrl Pts',(-20.5440893195705,26.0181538799688,123.003887825492)) ;
#21705=CARTESIAN_POINT('Ctrl Pts',(-20.8278012350198,25.8381647996059,122.901920140004)) ;
#21706=CARTESIAN_POINT('Ctrl Pts',(-20.5978286138219,26.0281574968712,123.207191914562)) ;
#21707=CARTESIAN_POINT('Ctrl Pts',(-20.8949727103039,25.8481684165084,123.156051177432)) ;
#21708=CARTESIAN_POINT('Ctrl Pts',(-20.6153163617937,26.0381469086364,123.416505710601)) ;
#21709=CARTESIAN_POINT('Ctrl Pts',(-20.9168297433397,25.8581578282735,123.417692998704)) ;
#21710=CARTESIAN_POINT('Ctrl Pts',(-20.5960135788333,26.0481656699812,123.626222930686)) ;
#21711=CARTESIAN_POINT('Ctrl Pts',(-20.8926982525151,25.8681765896183,123.67984195633)) ;
#21712=CARTESIAN_POINT('Ctrl Pts',(-20.5232631932467,26.0613843453623,123.894483327193)) ;
#21713=CARTESIAN_POINT('Ctrl Pts',(-20.8017581311539,25.8813952649994,124.015153473732)) ;
#21714=CARTESIAN_POINT('Ctrl Pts',(-20.3813483402664,26.074694652607,124.13929149955)) ;
#21715=CARTESIAN_POINT('Ctrl Pts',(-20.6243920028856,25.8947055722441,124.321133430442)) ;
#21716=CARTESIAN_POINT('Ctrl Pts',(-20.1842168943985,26.087932318833,124.335713981098)) ;
#21717=CARTESIAN_POINT('Ctrl Pts',(-20.3779377392562,25.9079432384701,124.566705392269)) ;
#21718=CARTESIAN_POINT('Ctrl Pts',(-20.0135494311699,26.0978520142437,124.455575991443)) ;
#21719=CARTESIAN_POINT('Ctrl Pts',(-20.1646098417396,25.9178629338808,124.716521317829)) ;
#21720=CARTESIAN_POINT('Ctrl Pts',(-19.8220452045287,26.1079048812422,124.544939686849)) ;
#21721=CARTESIAN_POINT('Ctrl Pts',(-19.9252257840937,25.9279158008794,124.828226044214)) ;
#21722=CARTESIAN_POINT('Ctrl Pts',(-19.6219710853917,26.1177602895715,124.598853822715)) ;
#21723=CARTESIAN_POINT('Ctrl Pts',(-19.6751350635831,25.9377712092086,124.895616007158)) ;
#21724=CARTESIAN_POINT('Ctrl Pts',(-19.4118059045154,26.1277989212481,124.617896062361)) ;
#21725=CARTESIAN_POINT('Ctrl Pts',(-19.4124225556355,25.9478098408852,124.919414322609)) ;
#21726=CARTESIAN_POINT('Ctrl Pts',(-19.1331380537758,26.1411011035151,124.594040851199)) ;
#21727=CARTESIAN_POINT('Ctrl Pts',(-19.0641152659986,25.9611120231522,124.889602889987)) ;
#21728=CARTESIAN_POINT('Ctrl Pts',(-18.8021064780862,26.157646116598,124.475037573678)) ;
#21729=CARTESIAN_POINT('Ctrl Pts',(-18.6502847526992,25.9776570362351,124.740819809691)) ;
#21730=CARTESIAN_POINT('Ctrl Pts',(-18.5297345481408,26.1742981326742,124.248799717429)) ;
#21731=CARTESIAN_POINT('Ctrl Pts',(-18.3098802866931,25.9943090523113,124.458074394266)) ;
#21732=CARTESIAN_POINT('Ctrl Pts',(-18.369098727454,26.1875212235794,124.021942776296)) ;
#21733=CARTESIAN_POINT('Ctrl Pts',(-18.1090436808664,26.0075321432166,124.174455573223)) ;
#21734=CARTESIAN_POINT('Ctrl Pts',(-18.2790691456165,26.1974821831388,123.832864887124)) ;
#21735=CARTESIAN_POINT('Ctrl Pts',(-17.9965176539852,26.0174931027759,123.938117510176)) ;
#21736=CARTESIAN_POINT('Ctrl Pts',(-18.2231373596907,26.2075069798899,123.629678729636)) ;
#21737=CARTESIAN_POINT('Ctrl Pts',(-17.9266031351628,26.027517899527,123.684128674994)) ;
#21738=CARTESIAN_POINT('Ctrl Pts',(-18.19662185451,26.2207314272857,123.352884992182)) ;
#21739=CARTESIAN_POINT('Ctrl Pts',(-17.8934600554389,26.0407423469228,123.338151922398)) ;
#21740=CARTESIAN_POINT('Ctrl Pts',(-18.2547370627252,26.2373652119848,123.004073948381)) ;
#21741=CARTESIAN_POINT('Ctrl Pts',(-17.9661098980233,26.0573761316219,122.902122581917)) ;
#21742=CARTESIAN_POINT('Ctrl Pts',(-18.4626485183739,26.2572678787097,122.635440004849)) ;
#21743=CARTESIAN_POINT('Ctrl Pts',(-18.2260016702492,26.0772787983468,122.441338078492)) ;
#21744=CARTESIAN_POINT('Ctrl Pts',(-18.7834207710504,26.2771681064916,122.359539756273)) ;
#21745=CARTESIAN_POINT('Ctrl Pts',(-18.6269689740633,26.0971790261287,122.096464789941)) ;
#21746=CARTESIAN_POINT('Ctrl Pts',(-19.1793519772945,26.2970855940231,122.209249706673)) ;
#21747=CARTESIAN_POINT('Ctrl Pts',(-19.1218834344603,26.1170965136602,121.908606135804)) ;
#21748=CARTESIAN_POINT('Ctrl Pts',(-19.60307943523,26.31701511984,122.202825724999)) ;
#21749=CARTESIAN_POINT('Ctrl Pts',(-19.6515421009118,26.1370260394771,121.900579250022)) ;
#21750=CARTESIAN_POINT('Ctrl Pts',(-20.004197714649,26.3369773877262,122.341686788595)) ;
#21751=CARTESIAN_POINT('Ctrl Pts',(-20.1529386123422,26.1569883073634,122.074158377623)) ;
#21752=CARTESIAN_POINT('Ctrl Pts',(-20.3326211942537,26.3568675826784,122.608053388485)) ;
#21753=CARTESIAN_POINT('Ctrl Pts',(-20.5634651727886,26.1768785023156,122.407118082729)) ;
#21754=CARTESIAN_POINT('Ctrl Pts',(-20.5514266364284,26.3767578274247,122.970081973903)) ;
#21755=CARTESIAN_POINT('Ctrl Pts',(-20.8369695350651,26.1967687470618,122.859653772299)) ;
#21756=CARTESIAN_POINT('Ctrl Pts',(-20.6334217410706,26.3968321999872,123.388909430167)) ;
#21757=CARTESIAN_POINT('Ctrl Pts',(-20.9394612388346,26.2168431196243,123.383189522101)) ;
#21758=CARTESIAN_POINT('Ctrl Pts',(-20.5686369856693,26.4166175773475,123.804638740479)) ;
#21759=CARTESIAN_POINT('Ctrl Pts',(-20.858478621002,26.2366284969846,123.902848054689)) ;
#21760=CARTESIAN_POINT('Ctrl Pts',(-20.3652722304398,26.4365794514146,124.177147234351)) ;
#21761=CARTESIAN_POINT('Ctrl Pts',(-20.604272042101,26.2565903710517,124.368482650199)) ;
#21762=CARTESIAN_POINT('Ctrl Pts',(-20.0459994667024,26.4565594269051,124.457421972499)) ;
#21763=CARTESIAN_POINT('Ctrl Pts',(-20.2051802401964,26.2765703465422,124.718824795122)) ;
#21764=CARTESIAN_POINT('Ctrl Pts',(-19.6538522670745,26.476371856783,124.611397902099)) ;
#21765=CARTESIAN_POINT('Ctrl Pts',(-19.7149987089246,26.2963827764202,124.911292999828)) ;
#21766=CARTESIAN_POINT('Ctrl Pts',(-19.2292568239862,26.4963519648733,124.622952036836)) ;
#21767=CARTESIAN_POINT('Ctrl Pts',(-19.1842547999823,26.3163628845105,124.925735636618)) ;
#21768=CARTESIAN_POINT('Ctrl Pts',(-18.8278291774401,26.5162463484706,124.489264756815)) ;
#21769=CARTESIAN_POINT('Ctrl Pts',(-18.6824717518944,26.3362572681077,124.758627144309)) ;
#21770=CARTESIAN_POINT('Ctrl Pts',(-18.4954865718006,26.5361732764478,124.226604674122)) ;
#21771=CARTESIAN_POINT('Ctrl Pts',(-18.2670439988586,26.3561841960849,124.430303289928)) ;
#21772=CARTESIAN_POINT('Ctrl Pts',(-18.2725029600721,26.556068133749,123.867014296754)) ;
#21773=CARTESIAN_POINT('Ctrl Pts',(-17.9883141683562,26.3760790533862,123.980817223551)) ;
#21774=CARTESIAN_POINT('Ctrl Pts',(-18.1854325985899,26.5761073273527,123.449960855483)) ;
#21775=CARTESIAN_POINT('Ctrl Pts',(-17.8794749235701,26.3961182469898,123.459500138785)) ;
#21776=CARTESIAN_POINT('Ctrl Pts',(-18.2454084367871,26.5959472952634,123.032350538864)) ;
#21777=CARTESIAN_POINT('Ctrl Pts',(-17.9544430376458,26.4159582149006,122.937489228161)) ;
#21778=CARTESIAN_POINT('Ctrl Pts',(-18.4440381416904,26.6158621122275,122.658424632547)) ;
#21779=CARTESIAN_POINT('Ctrl Pts',(-18.2027276437108,26.4358730318646,122.470081707864)) ;
#21780=CARTESIAN_POINT('Ctrl Pts',(-18.75897849637,26.6358043576238,122.374552553596)) ;
#21781=CARTESIAN_POINT('Ctrl Pts',(-18.596400995126,26.4558152772609,122.115240379138)) ;
#21782=CARTESIAN_POINT('Ctrl Pts',(-19.1503485290493,26.6556764057383,122.215041816388)) ;
#21783=CARTESIAN_POINT('Ctrl Pts',(-19.0856111707764,26.4756873253754,121.915849802114)) ;
#21784=CARTESIAN_POINT('Ctrl Pts',(-19.5753925439647,26.6756874706924,122.198865355149)) ;
#21785=CARTESIAN_POINT('Ctrl Pts',(-19.6169161682822,26.4956983903295,121.895626311636)) ;
#21786=CARTESIAN_POINT('Ctrl Pts',(-19.9769190829482,26.695498994996,122.326876472295)) ;
#21787=CARTESIAN_POINT('Ctrl Pts',(-20.118823655691,26.5155099146331,122.055636433992)) ;
#21788=CARTESIAN_POINT('Ctrl Pts',(-20.3149929284387,26.7155942069594,122.58789233349)) ;
#21789=CARTESIAN_POINT('Ctrl Pts',(-20.5414187886625,26.5356051265965,122.381904092641)) ;
#21790=CARTESIAN_POINT('Ctrl Pts',(-20.5402392709743,26.7353749308792,122.943283604957)) ;
#21791=CARTESIAN_POINT('Ctrl Pts',(-20.8229786362358,26.5553858505163,122.826139617815)) ;
#21792=CARTESIAN_POINT('Ctrl Pts',(-20.6325355714334,26.755366006522,123.358044401428)) ;
#21793=CARTESIAN_POINT('Ctrl Pts',(-20.9383530388371,26.5753769261591,123.344589665565)) ;
#21794=CARTESIAN_POINT('Ctrl Pts',(-20.5777323731222,26.775247945565,123.777341421288)) ;
#21795=CARTESIAN_POINT('Ctrl Pts',(-20.86985320622,26.5952588652021,123.868710610695)) ;
#21796=CARTESIAN_POINT('Ctrl Pts',(-20.3829509016501,26.7952005500682,124.154152656679)) ;
#21797=CARTESIAN_POINT('Ctrl Pts',(-20.6263804833536,26.6152114697054,124.339726432393)) ;
#21798=CARTESIAN_POINT('Ctrl Pts',(-20.0720296957647,26.8150994187989,124.441175273159)) ;
#21799=CARTESIAN_POINT('Ctrl Pts',(-20.2377323609478,26.635110338436,124.698507478413)) ;
#21800=CARTESIAN_POINT('Ctrl Pts',(-19.682246570693,26.8349928186085,124.605258451714)) ;
#21801=CARTESIAN_POINT('Ctrl Pts',(-19.750506384729,26.6550037382456,124.903616092832)) ;
#21802=CARTESIAN_POINT('Ctrl Pts',(-19.2594063736317,26.8549019494485,124.627157490124)) ;
#21803=CARTESIAN_POINT('Ctrl Pts',(-19.2219548120851,26.6749128690856,124.930993209538)) ;
#21804=CARTESIAN_POINT('Ctrl Pts',(-18.8522665349481,26.8749340492121,124.502164719981)) ;
#21805=CARTESIAN_POINT('Ctrl Pts',(-18.7130356342311,26.6949449688492,124.774763267432)) ;
#21806=CARTESIAN_POINT('Ctrl Pts',(-18.5715001351461,26.8914661223815,124.290581364288)) ;
#21807=CARTESIAN_POINT('Ctrl Pts',(-18.3620528555376,26.7114770420187,124.510268121194)) ;
#21808=CARTESIAN_POINT('Ctrl Pts',(-18.3986933822299,26.9048014629875,124.069844703011)) ;
#21809=CARTESIAN_POINT('Ctrl Pts',(-18.1460617747501,26.7248123826246,124.234367496516)) ;
#21810=CARTESIAN_POINT('Ctrl Pts',(-18.3010328118348,26.9146440215272,123.887397849221)) ;
#21811=CARTESIAN_POINT('Ctrl Pts',(-18.0239800547126,26.7346549411643,124.006303612785)) ;
#21812=CARTESIAN_POINT('Ctrl Pts',(-18.234968179349,26.9246959283771,123.68668524791)) ;
#21813=CARTESIAN_POINT('Ctrl Pts',(-17.9413973813911,26.7447068480142,123.755428033597)) ;
#21814=CARTESIAN_POINT('Ctrl Pts',(-18.1952008801186,26.937944442768,123.411026766241)) ;
#21815=CARTESIAN_POINT('Ctrl Pts',(-17.891686149238,26.7579553624051,123.410787353362)) ;
#21816=CARTESIAN_POINT('Ctrl Pts',(-18.2364062598888,26.9545436177157,123.060472721167)) ;
#21817=CARTESIAN_POINT('Ctrl Pts',(-17.9431815127596,26.7745545373529,122.972680824458)) ;
#21818=CARTESIAN_POINT('Ctrl Pts',(-18.3945264788303,26.9711324035108,122.745229733751)) ;
#21819=CARTESIAN_POINT('Ctrl Pts',(-18.1408483242503,26.7911433231479,122.578566000262)) ;
#21820=CARTESIAN_POINT('Ctrl Pts',(-18.5797786495349,26.9844082198528,122.536429267407)) ;
#21821=CARTESIAN_POINT('Ctrl Pts',(-18.3723926843041,26.8044191394899,122.317598644227)) ;
#21822=CARTESIAN_POINT('Ctrl Pts',(-18.7438802886562,26.9943820706466,122.405894110244)) ;
#21823=CARTESIAN_POINT('Ctrl Pts',(-18.5775216542846,26.8143929902837,122.15442033865)) ;
#21824=CARTESIAN_POINT('Ctrl Pts',(-18.929271898675,27.004411102739,122.305482739616)) ;
#21825=CARTESIAN_POINT('Ctrl Pts',(-18.8092589677791,26.8244220223761,122.028905565457)) ;
#21826=CARTESIAN_POINT('Ctrl Pts',(-19.1264590553554,27.0143012282409,122.239497823847)) ;
#21827=CARTESIAN_POINT('Ctrl Pts',(-19.0557421895212,26.834312147878,121.946421302957)) ;
#21828=CARTESIAN_POINT('Ctrl Pts',(-19.3341576766828,27.0242937065124,122.208161049022)) ;
#21829=CARTESIAN_POINT('Ctrl Pts',(-19.3153650354541,26.8443046261495,121.907247691411)) ;
#21830=CARTESIAN_POINT('Ctrl Pts',(-19.5433352481452,27.0342449216098,122.213230891029)) ;
#21831=CARTESIAN_POINT('Ctrl Pts',(-19.5768371046668,26.8542558412469,121.913582155201)) ;
#21832=CARTESIAN_POINT('Ctrl Pts',(-19.7503716423327,27.0442934233648,122.255105192578)) ;
#21833=CARTESIAN_POINT('Ctrl Pts',(-19.8356332457282,26.8643043430019,121.965922317603)) ;
#21834=CARTESIAN_POINT('Ctrl Pts',(-19.9430662208723,27.0541347729816,122.330491998155)) ;
#21835=CARTESIAN_POINT('Ctrl Pts',(-20.0765024472187,26.8741456926187,122.060153190044)) ;
#21836=CARTESIAN_POINT('Ctrl Pts',(-20.1225333341149,27.0641210640018,122.439364927213)) ;
#21837=CARTESIAN_POINT('Ctrl Pts',(-20.3008378724975,26.8841319836389,122.196241980051)) ;
#21838=CARTESIAN_POINT('Ctrl Pts',(-20.2797057557656,27.0740576757304,122.57702448676)) ;
#21839=CARTESIAN_POINT('Ctrl Pts',(-20.4973053062689,26.8940685953675,122.368314358404)) ;
#21840=CARTESIAN_POINT('Ctrl Pts',(-20.4119625359954,27.084107551098,122.74176172172)) ;
#21841=CARTESIAN_POINT('Ctrl Pts',(-20.662628518743,26.9041184707351,122.574234184223)) ;
#21842=CARTESIAN_POINT('Ctrl Pts',(-20.5117431177263,27.0939580096334,122.92324291587)) ;
#21843=CARTESIAN_POINT('Ctrl Pts',(-20.7873567686691,26.9139689292705,122.801084418396)) ;
#21844=CARTESIAN_POINT('Ctrl Pts',(-20.579826322129,27.1039299465862,123.121493753205)) ;
#21845=CARTESIAN_POINT('Ctrl Pts',(-20.8724634669083,26.9239408662233,123.048897162386)) ;
#21846=CARTESIAN_POINT('Ctrl Pts',(-20.6125055315077,27.1139254035183,123.329105646214)) ;
#21847=CARTESIAN_POINT('Ctrl Pts',(-20.9133152577875,26.9339363231554,123.308411671272)) ;
#21848=CARTESIAN_POINT('Ctrl Pts',(-20.6083877682446,27.1239582105714,123.539972730989)) ;
#21849=CARTESIAN_POINT('Ctrl Pts',(-20.9081708679061,26.9439691302085,123.571995622508)) ;
#21850=CARTESIAN_POINT('Ctrl Pts',(-20.5686916631752,27.1338180971613,123.743433100123)) ;
#21851=CARTESIAN_POINT('Ctrl Pts',(-20.8585534427238,26.9538290167985,123.826321841959)) ;
#21852=CARTESIAN_POINT('Ctrl Pts',(-20.4936737353725,27.1438071777266,123.939559222509)) ;
#21853=CARTESIAN_POINT('Ctrl Pts',(-20.7647835915375,26.9638180973637,124.071480590036)) ;
#21854=CARTESIAN_POINT('Ctrl Pts',(-20.3863494619409,27.1537386569357,124.118661541936)) ;
#21855=CARTESIAN_POINT('Ctrl Pts',(-20.6306305349959,26.9737495765729,124.29536007837)) ;
#21856=CARTESIAN_POINT('Ctrl Pts',(-20.2490645865285,27.1637245163817,124.277504970353)) ;
#21857=CARTESIAN_POINT('Ctrl Pts',(-20.4590264458182,26.9837354360188,124.493916247248)) ;
#21858=CARTESIAN_POINT('Ctrl Pts',(-20.0852193557923,27.1737626670289,124.410486117788)) ;
#21859=CARTESIAN_POINT('Ctrl Pts',(-20.254221659418,26.993773586666,124.66014484481)) ;
#21860=CARTESIAN_POINT('Ctrl Pts',(-19.9044415797665,27.1836107575333,124.511442323854)) ;
#21861=CARTESIAN_POINT('Ctrl Pts',(-20.0282504284219,27.0036216771704,124.786342691733)) ;
#21862=CARTESIAN_POINT('Ctrl Pts',(-19.7047523070118,27.1936716660512,124.581101591854)) ;
#21863=CARTESIAN_POINT('Ctrl Pts',(-19.7786397745395,27.0136825856884,124.873419336829)) ;
#21864=CARTESIAN_POINT('Ctrl Pts',(-19.4993833052846,27.2035665132092,124.614334962714)) ;
#21865=CARTESIAN_POINT('Ctrl Pts',(-19.5219286374244,27.0235774328464,124.914963808306)) ;
#21866=CARTESIAN_POINT('Ctrl Pts',(-19.2904166566976,27.2135081852543,124.611948250234)) ;
#21867=CARTESIAN_POINT('Ctrl Pts',(-19.2607200330095,27.0335191048914,124.911983091372)) ;
#21868=CARTESIAN_POINT('Ctrl Pts',(-19.0837134685083,27.2235107123797,124.573148992734)) ;
#21869=CARTESIAN_POINT('Ctrl Pts',(-19.002340474553,27.0435216320169,124.863486618766)) ;
#21870=CARTESIAN_POINT('Ctrl Pts',(-18.886408762246,27.2335455035672,124.49851245076)) ;
#21871=CARTESIAN_POINT('Ctrl Pts',(-18.755708647713,27.0535564232043,124.770193481186)) ;
#21872=CARTESIAN_POINT('Ctrl Pts',(-18.7082920067272,27.2433903834263,124.393076161983)) ;
#21873=CARTESIAN_POINT('Ctrl Pts',(-18.53306086531,27.0634013030634,124.63840012197)) ;
#21874=CARTESIAN_POINT('Ctrl Pts',(-18.548717036597,27.2533762640448,124.256715634161)) ;
#21875=CARTESIAN_POINT('Ctrl Pts',(-18.3335903392706,27.0733871836819,124.467951336687)) ;
#21876=CARTESIAN_POINT('Ctrl Pts',(-18.415763782662,27.263310987138,124.095588178805)) ;
#21877=CARTESIAN_POINT('Ctrl Pts',(-18.1673965821684,27.0833219067751,124.266543402248)) ;
#21878=CARTESIAN_POINT('Ctrl Pts',(-18.3117355785266,27.2733688274492,123.911537425513)) ;
#21879=CARTESIAN_POINT('Ctrl Pts',(-18.0373591121067,27.0933797470863,124.03648134582)) ;
#21880=CARTESIAN_POINT('Ctrl Pts',(-18.2425753593927,27.2831893148457,123.716980331988)) ;
#21881=CARTESIAN_POINT('Ctrl Pts',(-17.9509061764655,27.1032002344828,123.793285094069)) ;
#21882=CARTESIAN_POINT('Ctrl Pts',(-18.2070714729757,27.2932497161908,123.508505960271)) ;
#21883=CARTESIAN_POINT('Ctrl Pts',(-17.9065238901742,27.1132606358279,123.532692664086)) ;
#21884=CARTESIAN_POINT('Ctrl Pts',(-18.2085717097183,27.3031806817437,123.299707474007)) ;
#21885=CARTESIAN_POINT('Ctrl Pts',(-17.9083966530251,27.1231916013808,123.271694164607)) ;
#21886=CARTESIAN_POINT('Ctrl Pts',(-18.2458677394489,27.3131195440802,123.094139009505)) ;
#21887=CARTESIAN_POINT('Ctrl Pts',(-17.9550143490479,27.1331304637173,123.014732779571)) ;
#21888=CARTESIAN_POINT('Ctrl Pts',(-18.3185162099704,27.3231052750064,122.897153471792)) ;
#21889=CARTESIAN_POINT('Ctrl Pts',(-18.0458227293772,27.1431161946435,122.768499870868)) ;
#21890=CARTESIAN_POINT('Ctrl Pts',(-18.4248467767158,27.3331296604338,122.715218646708)) ;
#21891=CARTESIAN_POINT('Ctrl Pts',(-18.1787338062467,27.1531405800709,122.54108010085)) ;
#21892=CARTESIAN_POINT('Ctrl Pts',(-18.5592899800235,27.3430329447871,122.556213400873)) ;
#21893=CARTESIAN_POINT('Ctrl Pts',(-18.3467863406668,27.1630438644242,122.342321573022)) ;
#21894=CARTESIAN_POINT('Ctrl Pts',(-18.7218362744338,27.3530929493651,122.42094597078)) ;
#21895=CARTESIAN_POINT('Ctrl Pts',(-18.5499675318017,27.1731038690022,122.173235543931)) ;
#21896=CARTESIAN_POINT('Ctrl Pts',(-18.9014128659292,27.3629362184342,122.3180699415)) ;
#21897=CARTESIAN_POINT('Ctrl Pts',(-18.7744378365037,27.1829471380713,122.044638016558)) ;
#21898=CARTESIAN_POINT('Ctrl Pts',(-19.0988286897178,27.3729267840419,122.246443873207)) ;
#21899=CARTESIAN_POINT('Ctrl Pts',(-19.0212070083882,27.192937703679,121.955103241881)) ;
#21900=CARTESIAN_POINT('Ctrl Pts',(-19.3044292359815,27.3828549158207,122.210437107956)) ;
#21901=CARTESIAN_POINT('Ctrl Pts',(-19.2782077784814,27.2028658354578,121.910092465526)) ;
#21902=CARTESIAN_POINT('Ctrl Pts',(-19.5144154098307,27.3928428029016,122.21031147887)) ;
#21903=CARTESIAN_POINT('Ctrl Pts',(-19.5406906769413,27.2128537225387,121.909933250644)) ;
#21904=CARTESIAN_POINT('Ctrl Pts',(-19.7221490194526,27.4028787524703,122.247173181467)) ;
#21905=CARTESIAN_POINT('Ctrl Pts',(-19.8003580009036,27.2228896721074,121.956008127035)) ;
#21906=CARTESIAN_POINT('Ctrl Pts',(-19.916892573696,27.4127336388491,122.317923368138)) ;
#21907=CARTESIAN_POINT('Ctrl Pts',(-20.0437890490973,27.2327445584862,122.044444124203)) ;
#21908=CARTESIAN_POINT('Ctrl Pts',(-20.0991236220355,27.422733053197,122.422656802109)) ;
#21909=CARTESIAN_POINT('Ctrl Pts',(-20.2715790260407,27.2427439728341,122.175359156114)) ;
#21910=CARTESIAN_POINT('Ctrl Pts',(-20.2589164113812,27.4326282183875,122.555908904654)) ;
#21911=CARTESIAN_POINT('Ctrl Pts',(-20.47132188163,27.2526391380246,122.341923187153)) ;
#21912=CARTESIAN_POINT('Ctrl Pts',(-20.3953279566597,27.4426885370794,122.71750152297)) ;
#21913=CARTESIAN_POINT('Ctrl Pts',(-20.6418377253297,27.2626994567166,122.543912452748)) ;
#21914=CARTESIAN_POINT('Ctrl Pts',(-20.4995174983559,27.4525386688555,122.896483303571)) ;
#21915=CARTESIAN_POINT('Ctrl Pts',(-20.7720769168341,27.2725495884926,122.767639569015)) ;
#21916=CARTESIAN_POINT('Ctrl Pts',(-20.5728149864719,27.4625692393058,123.094198738288)) ;
#21917=CARTESIAN_POINT('Ctrl Pts',(-20.8637005068752,27.2825801589429,123.014783157539)) ;
#21918=CARTESIAN_POINT('Ctrl Pts',(-20.6101494969086,27.4725833899786,123.301402871192)) ;
#21919=CARTESIAN_POINT('Ctrl Pts',(-20.9103706252309,27.2925943096157,123.273787983254)) ;
#21920=CARTESIAN_POINT('Ctrl Pts',(-20.6112662653975,27.482476323524,123.509383815082)) ;
#21921=CARTESIAN_POINT('Ctrl Pts',(-20.911768495837,27.3024872431611,123.533764947733)) ;
#21922=CARTESIAN_POINT('Ctrl Pts',(-20.5761521288518,27.4924658375142,123.716418000998)) ;
#21923=CARTESIAN_POINT('Ctrl Pts',(-20.8678776029836,27.3124767571514,123.792558185261)) ;
#21924=CARTESIAN_POINT('Ctrl Pts',(-20.5059891635455,27.5024196081667,123.913596204343)) ;
#21925=CARTESIAN_POINT('Ctrl Pts',(-20.7801754400193,27.3224305278038,124.03903194835)) ;
#21926=CARTESIAN_POINT('Ctrl Pts',(-20.4015400398466,27.5124673768272,124.097177756809)) ;
#21927=CARTESIAN_POINT('Ctrl Pts',(-20.6496157399914,27.3324782964644,124.26850963764)) ;
#21928=CARTESIAN_POINT('Ctrl Pts',(-20.2697294375057,27.522309103267,124.256684479157)) ;
#21929=CARTESIAN_POINT('Ctrl Pts',(-20.4848531000536,27.3423200229042,124.467895083723)) ;
#21930=CARTESIAN_POINT('Ctrl Pts',(-20.1102592973178,27.5322946200898,124.393158289807)) ;
#21931=CARTESIAN_POINT('Ctrl Pts',(-20.2855162962699,27.3523055397269,124.638488743857)) ;
#21932=CARTESIAN_POINT('Ctrl Pts',(-19.9303364745535,27.5422339517853,124.499474121132)) ;
#21933=CARTESIAN_POINT('Ctrl Pts',(-20.0606131128351,27.3622448714225,124.771385186807)) ;
#21934=CARTESIAN_POINT('Ctrl Pts',(-19.7327382041188,27.5522737214829,124.573617862549)) ;
#21935=CARTESIAN_POINT('Ctrl Pts',(-19.8136159800649,27.37228464112,124.864066326302)) ;
#21936=CARTESIAN_POINT('Ctrl Pts',(-19.5283912957834,27.5621618827317,124.611847447798)) ;
#21937=CARTESIAN_POINT('Ctrl Pts',(-19.5581817302825,27.3821728023688,124.911855032732)) ;
#21938=CARTESIAN_POINT('Ctrl Pts',(-19.3184025008245,27.5721514372341,124.614431043553)) ;
#21939=CARTESIAN_POINT('Ctrl Pts',(-19.2956955404914,27.3921623568712,124.915085978907)) ;
#21940=CARTESIAN_POINT('Ctrl Pts',(-19.1118246407992,27.5821098517577,124.580462400769)) ;
#21941=CARTESIAN_POINT('Ctrl Pts',(-19.0374725439821,27.4021207713948,124.872626590807)) ;
#21942=CARTESIAN_POINT('Ctrl Pts',(-18.9152594132557,27.5920097645871,124.512023957247)) ;
#21943=CARTESIAN_POINT('Ctrl Pts',(-18.7917647458714,27.4120206842242,124.787079499337)) ;
#21944=CARTESIAN_POINT('Ctrl Pts',(-18.7309264013132,27.602056464237,124.408951439022)) ;
#21945=CARTESIAN_POINT('Ctrl Pts',(-18.5613480077617,27.4220673838741,124.658240132733)) ;
#21946=CARTESIAN_POINT('Ctrl Pts',(-18.5695583676357,27.6119563245426,124.277459812412)) ;
#21947=CARTESIAN_POINT('Ctrl Pts',(-18.3596364546277,27.4319672441797,124.493876043428)) ;
#21948=CARTESIAN_POINT('Ctrl Pts',(-18.4313772500186,27.622007728748,124.117627545932)) ;
#21949=CARTESIAN_POINT('Ctrl Pts',(-18.186909253097,27.4420186483852,124.294086730336)) ;
#21950=CARTESIAN_POINT('Ctrl Pts',(-18.3247881894919,27.6318887656692,123.939292964072)) ;
#21951=CARTESIAN_POINT('Ctrl Pts',(-18.0536713291326,27.4518996853063,124.071168267617)) ;
#21952=CARTESIAN_POINT('Ctrl Pts',(-18.2496492643862,27.6418885978467,123.742988738701)) ;
#21953=CARTESIAN_POINT('Ctrl Pts',(-17.9597465513536,27.4618995174838,123.825788262627)) ;
#21954=CARTESIAN_POINT('Ctrl Pts',(-18.2098807597813,27.6518066008316,123.538271728212)) ;
#21955=CARTESIAN_POINT('Ctrl Pts',(-17.9100347106082,27.4718175204687,123.56989145949)) ;
#21956=CARTESIAN_POINT('Ctrl Pts',(-18.2062837040758,27.6618579067061,123.327027887074)) ;
#21957=CARTESIAN_POINT('Ctrl Pts',(-17.9055372820663,27.4818688263432,123.305836914717)) ;
#21958=CARTESIAN_POINT('Ctrl Pts',(-18.2385839581239,27.6717277300977,123.122017781039)) ;
#21959=CARTESIAN_POINT('Ctrl Pts',(-17.9459117765369,27.4917386497348,123.049572996332)) ;
#21960=CARTESIAN_POINT('Ctrl Pts',(-18.307368702007,27.681801896148,122.921759006394)) ;
#21961=CARTESIAN_POINT('Ctrl Pts',(-18.0318915985893,27.5018128157851,122.799249602971)) ;
#21962=CARTESIAN_POINT('Ctrl Pts',(-18.4071173488075,27.6916219802896,122.74095235675)) ;
#21963=CARTESIAN_POINT('Ctrl Pts',(-18.1565773494833,27.5116328999267,122.573239483822)) ;
#21964=CARTESIAN_POINT('Ctrl Pts',(-18.5399396605626,27.7017007070255,122.575930572394)) ;
#21965=CARTESIAN_POINT('Ctrl Pts',(-18.3226042808018,27.5217116266626,122.366962086733)) ;
#21966=CARTESIAN_POINT('Ctrl Pts',(-18.6958321778564,27.711552287675,122.439501623981)) ;
#21967=CARTESIAN_POINT('Ctrl Pts',(-18.5174703780383,27.5315632073121,122.196424414338)) ;
#21968=CARTESIAN_POINT('Ctrl Pts',(-18.8768591143373,27.7216254159734,122.329686829936)) ;
#21969=CARTESIAN_POINT('Ctrl Pts',(-18.7437532834736,27.5416363356105,122.05915550415)) ;
#21970=CARTESIAN_POINT('Ctrl Pts',(-19.069748360102,27.7314678938648,122.254738925638)) ;
#21971=CARTESIAN_POINT('Ctrl Pts',(-18.9848658829686,27.5514788135019,121.965469396346)) ;
#21972=CARTESIAN_POINT('Ctrl Pts',(-19.275402729767,27.7414485004629,122.213172865234)) ;
#21973=CARTESIAN_POINT('Ctrl Pts',(-19.2419340497948,27.5614594201,121.913511275121)) ;
#21974=CARTESIAN_POINT('Ctrl Pts',(-19.4859500150315,27.7514662094817,122.208323768403)) ;
#21975=CARTESIAN_POINT('Ctrl Pts',(-19.505118136635,27.5714771291188,121.907449255122)) ;
#21976=CARTESIAN_POINT('Ctrl Pts',(-19.6914845982736,27.7613523885191,122.23929217762)) ;
#21977=CARTESIAN_POINT('Ctrl Pts',(-19.7620374996728,27.5813633081562,121.946159440311)) ;
#21978=CARTESIAN_POINT('Ctrl Pts',(-19.8919086335487,27.7714100010914,122.306601119756)) ;
#21979=CARTESIAN_POINT('Ctrl Pts',(-20.0125674013974,27.5914209207286,122.030295059284)) ;
#21980=CARTESIAN_POINT('Ctrl Pts',(-20.0742918881656,27.7812863944636,122.405862590949)) ;
#21981=CARTESIAN_POINT('Ctrl Pts',(-20.2405477178494,27.6012973141007,122.154372035112)) ;
#21982=CARTESIAN_POINT('Ctrl Pts',(-20.2389323043103,27.791281422614,122.536416615308)) ;
#21983=CARTESIAN_POINT('Ctrl Pts',(-20.4463485472987,27.6112923422511,122.317564461287)) ;
#21984=CARTESIAN_POINT('Ctrl Pts',(-20.3785025030073,27.80130216946,122.694229664895)) ;
#21985=CARTESIAN_POINT('Ctrl Pts',(-20.6208115759906,27.6213130890971,122.51483046535)) ;
#21986=CARTESIAN_POINT('Ctrl Pts',(-20.4874494476852,27.8112042381264,122.871614573746)) ;
#21987=CARTESIAN_POINT('Ctrl Pts',(-20.7569960330264,27.6312151577635,122.736562250952)) ;
#21988=CARTESIAN_POINT('Ctrl Pts',(-20.5649160847513,27.8211949779461,123.066844849364)) ;
#21989=CARTESIAN_POINT('Ctrl Pts',(-20.8538296011518,27.6412058975832,122.980600241119)) ;
#21990=CARTESIAN_POINT('Ctrl Pts',(-20.6070370985664,27.8311581741564,123.272013328294)) ;
#21991=CARTESIAN_POINT('Ctrl Pts',(-20.9064812123952,27.6511690937935,123.237061229662)) ;
#21992=CARTESIAN_POINT('Ctrl Pts',(-20.6133758883929,27.8410623584565,123.480152818403)) ;
#21993=CARTESIAN_POINT('Ctrl Pts',(-20.9144047817725,27.6610732780936,123.497236530681)) ;
#21994=CARTESIAN_POINT('Ctrl Pts',(-20.5828360532262,27.8511228188474,123.689412748153)) ;
#21995=CARTESIAN_POINT('Ctrl Pts',(-20.8762301626549,27.6711337384845,123.758811110914)) ;
#21996=CARTESIAN_POINT('Ctrl Pts',(-20.5181122383662,27.8609633647182,123.885935058997)) ;
#21997=CARTESIAN_POINT('Ctrl Pts',(-20.7953249519176,27.6809742843553,124.004465402187)) ;
#21998=CARTESIAN_POINT('Ctrl Pts',(-20.4183061486459,27.8710255854299,124.072424108861)) ;
#21999=CARTESIAN_POINT('Ctrl Pts',(-20.6705674371017,27.6910365050671,124.237576347375)) ;
#22000=CARTESIAN_POINT('Ctrl Pts',(-20.2895881644942,27.8809227284465,124.235913842461)) ;
#22001=CARTESIAN_POINT('Ctrl Pts',(-20.5096693378974,27.7009336480836,124.441939302609)) ;
#22002=CARTESIAN_POINT('Ctrl Pts',(-20.1343799700791,27.8908539048637,124.375554329111)) ;
#22003=CARTESIAN_POINT('Ctrl Pts',(-20.315658373556,27.7108648245008,124.61649018712)) ;
#22004=CARTESIAN_POINT('Ctrl Pts',(-19.9551790503614,27.9008961186423,124.487164722517)) ;
#22005=CARTESIAN_POINT('Ctrl Pts',(-20.091657303987,27.7209070382794,124.756002912722)) ;
#22006=CARTESIAN_POINT('Ctrl Pts',(-19.762401523415,27.910782658845,124.564891732212)) ;
#22007=CARTESIAN_POINT('Ctrl Pts',(-19.8506842942627,27.7307935784821,124.85316185408)) ;
#22008=CARTESIAN_POINT('Ctrl Pts',(-19.5569511425706,27.9207762534504,124.608757066638)) ;
#22009=CARTESIAN_POINT('Ctrl Pts',(-19.5938710456304,27.7407871730876,124.907993194414)) ;
#22010=CARTESIAN_POINT('Ctrl Pts',(-19.3480204997779,27.930720128608,124.616215006894)) ;
#22011=CARTESIAN_POINT('Ctrl Pts',(-19.3327071093546,27.7507310482451,124.917315275339)) ;
#22012=CARTESIAN_POINT('Ctrl Pts',(-19.1406090152874,27.9406806647228,124.587509478741)) ;
#22013=CARTESIAN_POINT('Ctrl Pts',(-19.0734423500519,27.7606915843599,124.881432829596)) ;
#22014=CARTESIAN_POINT('Ctrl Pts',(-18.9405381225761,27.9506772680455,124.523103824295)) ;
#22015=CARTESIAN_POINT('Ctrl Pts',(-18.823353749831,27.7706881876827,124.800925220385)) ;
#22016=CARTESIAN_POINT('Ctrl Pts',(-18.7541744874109,27.960710351,124.424327030337)) ;
#22017=CARTESIAN_POINT('Ctrl Pts',(-18.5903995182117,27.7807212706372,124.677453935382)) ;
#22018=CARTESIAN_POINT('Ctrl Pts',(-18.5906478671095,27.9705615197016,124.297248746626)) ;
#22019=CARTESIAN_POINT('Ctrl Pts',(-18.3859904696139,27.7905724393387,124.518604840361)) ;
#22020=CARTESIAN_POINT('Ctrl Pts',(-18.4496441002172,27.9805240104005,124.142390521308)) ;
#22021=CARTESIAN_POINT('Ctrl Pts',(-18.2097360022858,27.8005349300376,124.325031213336)) ;
#22022=CARTESIAN_POINT('Ctrl Pts',(-18.3371397750335,27.9905524388182,123.964073852674)) ;
#22023=CARTESIAN_POINT('Ctrl Pts',(-18.0691061956658,27.8105633584554,124.102135115778)) ;
#22024=CARTESIAN_POINT('Ctrl Pts',(-18.2581916508595,28.0004628061828,123.771274447575)) ;
#22025=CARTESIAN_POINT('Ctrl Pts',(-17.9704213296521,27.8204737258199,123.861134793012)) ;
#22026=CARTESIAN_POINT('Ctrl Pts',(-18.2132715984884,28.0103976737979,123.567293786419)) ;
#22027=CARTESIAN_POINT('Ctrl Pts',(-17.9142719852206,27.830408593435,123.606158130962)) ;
#22028=CARTESIAN_POINT('Ctrl Pts',(-18.2045541391692,28.0204388157769,123.356384171661)) ;
#22029=CARTESIAN_POINT('Ctrl Pts',(-17.9033759753097,27.840449735414,123.342521266579)) ;
#22030=CARTESIAN_POINT('Ctrl Pts',(-18.2320173963766,28.0303259519801,123.150336225817)) ;
#22031=CARTESIAN_POINT('Ctrl Pts',(-17.9377060396121,27.8503368716172,123.084960416994)) ;
#22032=CARTESIAN_POINT('Ctrl Pts',(-18.2951662826154,28.0403182343835,122.949998669832)) ;
#22033=CARTESIAN_POINT('Ctrl Pts',(-18.0166431581778,27.8603291540206,122.834538577221)) ;
#22034=CARTESIAN_POINT('Ctrl Pts',(-18.3917805672602,28.0502667623487,122.764488512371)) ;
#22035=CARTESIAN_POINT('Ctrl Pts',(-18.137412126526,27.8702776819858,122.602650848213)) ;
#22036=CARTESIAN_POINT('Ctrl Pts',(-18.5187344195011,28.0602034935108,122.598611319051)) ;
#22037=CARTESIAN_POINT('Ctrl Pts',(-18.2961056898845,27.8802144131479,122.395304507949)) ;
#22038=CARTESIAN_POINT('Ctrl Pts',(-18.6731352153546,28.0701867043708,122.456413854557)) ;
#22039=CARTESIAN_POINT('Ctrl Pts',(-18.4891076721817,27.8901976240079,122.217558370946)) ;
#22040=CARTESIAN_POINT('Ctrl Pts',(-18.8511053323271,28.0802298035207,122.342850389306)) ;
#22041=CARTESIAN_POINT('Ctrl Pts',(-18.7115707177152,27.9002407231578,122.075605016214)) ;
#22042=CARTESIAN_POINT('Ctrl Pts',(-19.0418370727349,28.0900607677956,122.26317827219)) ;
#22043=CARTESIAN_POINT('Ctrl Pts',(-18.9499871891245,27.9100716874327,121.976015433695)) ;
#22044=CARTESIAN_POINT('Ctrl Pts',(-19.2483766387023,28.1001336201815,122.216578929442)) ;
#22045=CARTESIAN_POINT('Ctrl Pts',(-19.2081615249894,27.9201445398186,121.917767583989)) ;
#22046=CARTESIAN_POINT('Ctrl Pts',(-19.4555437861215,28.1099977478933,122.206790899523)) ;
#22047=CARTESIAN_POINT('Ctrl Pts',(-19.4671216625185,27.9300086675304,121.905533740892)) ;
#22048=CARTESIAN_POINT('Ctrl Pts',(-19.6645948451265,28.1200199500282,122.233024086339)) ;
#22049=CARTESIAN_POINT('Ctrl Pts',(-19.7284352632182,27.9400308696653,121.938326646805)) ;
#22050=CARTESIAN_POINT('Ctrl Pts',(-19.8658877748029,28.1300471429966,122.295670934239)) ;
#22051=CARTESIAN_POINT('Ctrl Pts',(-19.980050984628,27.9500580626337,122.016636385366)) ;
#22052=CARTESIAN_POINT('Ctrl Pts',(-20.0501626714237,28.1399027369636,122.39036087509)) ;
#22053=CARTESIAN_POINT('Ctrl Pts',(-20.2103950643466,27.9599136566007,122.135000592785)) ;
#22054=CARTESIAN_POINT('Ctrl Pts',(-20.2172929353047,28.1498599088289,122.516416762394)) ;
#22055=CARTESIAN_POINT('Ctrl Pts',(-20.4193072748828,27.969870828466,122.29257198083)) ;
#22056=CARTESIAN_POINT('Ctrl Pts',(-20.36088775291,28.1598987528273,122.67106650366)) ;
#22057=CARTESIAN_POINT('Ctrl Pts',(-20.5987996284151,27.9799096724644,122.485885053549)) ;
#22058=CARTESIAN_POINT('Ctrl Pts',(-20.4738977645388,28.1697727767028,122.845224021032)) ;
#22059=CARTESIAN_POINT('Ctrl Pts',(-20.7400613604965,27.98978369634,122.703583668428)) ;
#22060=CARTESIAN_POINT('Ctrl Pts',(-20.5565305050554,28.1798426026932,123.040098786974)) ;
#22061=CARTESIAN_POINT('Ctrl Pts',(-20.8433506853364,27.9998535223304,122.947177423952)) ;
#22062=CARTESIAN_POINT('Ctrl Pts',(-20.603072347858,28.1896758465905,123.241534739974)) ;
#22063=CARTESIAN_POINT('Ctrl Pts',(-20.9015266940339,28.0096867662276,123.198973980949)) ;
#22064=CARTESIAN_POINT('Ctrl Pts',(-20.614743890259,28.1997062743635,123.452075818359)) ;
#22065=CARTESIAN_POINT('Ctrl Pts',(-20.9161142994382,28.0197171940007,123.462150342134)) ;
#22066=CARTESIAN_POINT('Ctrl Pts',(-20.5890670250738,28.2097378911087,123.661414868918)) ;
#22067=CARTESIAN_POINT('Ctrl Pts',(-20.8840166201033,28.0297488107458,123.72382387547)) ;
#22068=CARTESIAN_POINT('Ctrl Pts',(-20.5290926772713,28.2195675680894,123.859156375962)) ;
#22069=CARTESIAN_POINT('Ctrl Pts',(-20.80904662986,28.0395784877265,123.971001465148)) ;
#22070=CARTESIAN_POINT('Ctrl Pts',(-20.4347263329766,28.2295570849293,124.046779224324)) ;
#22071=CARTESIAN_POINT('Ctrl Pts',(-20.6910868706554,28.0495680045665,124.205529304447)) ;
#22072=CARTESIAN_POINT('Ctrl Pts',(-20.308112533224,28.2396006970691,124.215750588149)) ;
#22073=CARTESIAN_POINT('Ctrl Pts',(-20.5328182779669,28.0596116167062,124.416742316167)) ;
#22074=CARTESIAN_POINT('Ctrl Pts',(-20.1577648900733,28.2494233034044,124.357312030463)) ;
#22075=CARTESIAN_POINT('Ctrl Pts',(-20.3448814894554,28.0694342230415,124.593693576125)) ;
#22076=CARTESIAN_POINT('Ctrl Pts',(-19.9816030750299,28.2594615333036,124.473500882314)) ;
#22077=CARTESIAN_POINT('Ctrl Pts',(-20.124678185504,28.0794724529408,124.73892784558)) ;
#22078=CARTESIAN_POINT('Ctrl Pts',(-19.7882531660864,28.2694725680956,124.556669707045)) ;
#22079=CARTESIAN_POINT('Ctrl Pts',(-19.8829899980489,28.0894834877327,124.842887131756)) ;
#22080=CARTESIAN_POINT('Ctrl Pts',(-19.5858129110288,28.2793702990627,124.604775415822)) ;
#22081=CARTESIAN_POINT('Ctrl Pts',(-19.6299384968335,28.0993812186998,124.903017471924)) ;
#22082=CARTESIAN_POINT('Ctrl Pts',(-19.376180880844,28.2893599269132,124.617388122946)) ;
#22083=CARTESIAN_POINT('Ctrl Pts',(-19.3678981582499,28.1093708465503,124.918781274721)) ;
#22084=CARTESIAN_POINT('Ctrl Pts',(-19.1682588404928,28.2993157173592,124.593418733339)) ;
#22085=CARTESIAN_POINT('Ctrl Pts',(-19.1079954571358,28.1193266369963,124.888817431813)) ;
#22086=CARTESIAN_POINT('Ctrl Pts',(-18.96810534998,28.3092431159212,124.534261318973)) ;
#22087=CARTESIAN_POINT('Ctrl Pts',(-18.8578037171305,28.1292540355584,124.814868421456)) ;
#22088=CARTESIAN_POINT('Ctrl Pts',(-18.7794564522439,28.3192687110311,124.440280835038)) ;
#22089=CARTESIAN_POINT('Ctrl Pts',(-18.6219935808609,28.1392796306682,124.697390886151)) ;
#22090=CARTESIAN_POINT('Ctrl Pts',(-18.6122710106145,28.3291545617007,124.31681671948)) ;
#22091=CARTESIAN_POINT('Ctrl Pts',(-18.413012495007,28.1491654813378,124.543058534145)) ;
#22092=CARTESIAN_POINT('Ctrl Pts',(-18.4672022044828,28.3391437415449,124.164964313106)) ;
#22093=CARTESIAN_POINT('Ctrl Pts',(-18.2316780606301,28.159154661182,124.353241304876)) ;
#22094=CARTESIAN_POINT('Ctrl Pts',(-18.350468282265,28.3491849286484,123.98908060691)) ;
#22095=CARTESIAN_POINT('Ctrl Pts',(-18.085762555499,28.1691958482856,124.133385523761)) ;
#22096=CARTESIAN_POINT('Ctrl Pts',(-18.267489993905,28.3590175721244,123.799757295272)) ;
#22097=CARTESIAN_POINT('Ctrl Pts',(-17.9820414176768,28.1790284917615,123.896729581303)) ;
#22098=CARTESIAN_POINT('Ctrl Pts',(-18.2172586034104,28.3690115218339,123.595747330936)) ;
#22099=CARTESIAN_POINT('Ctrl Pts',(-17.9192545217861,28.189022441471,123.641716424028)) ;
#22100=CARTESIAN_POINT('Ctrl Pts',(-18.2036074114145,28.3790406446104,123.385343767415)) ;
#22101=CARTESIAN_POINT('Ctrl Pts',(-17.9021928664862,28.1990515642475,123.378711840277)) ;
#22102=CARTESIAN_POINT('Ctrl Pts',(-18.2260142937554,28.3889167755291,123.178918899559)) ;
#22103=CARTESIAN_POINT('Ctrl Pts',(-17.9302039422221,28.2089276951662,123.120680343544)) ;
#22104=CARTESIAN_POINT('Ctrl Pts',(-18.2843913723889,28.3989148105461,122.977024252762)) ;
#22105=CARTESIAN_POINT('Ctrl Pts',(-18.0031776926144,28.2189257301832,122.86831261201)) ;
#22106=CARTESIAN_POINT('Ctrl Pts',(-18.3760366799018,28.4088287403048,122.789803762381)) ;
#22107=CARTESIAN_POINT('Ctrl Pts',(-18.117736776842,28.2288396599419,122.634287677194)) ;
#22108=CARTESIAN_POINT('Ctrl Pts',(-18.500337734295,28.4188719280426,122.619151689602)) ;
#22109=CARTESIAN_POINT('Ctrl Pts',(-18.2731150794606,28.2388828476797,122.420974122389)) ;
#22110=CARTESIAN_POINT('Ctrl Pts',(-18.6502217855382,28.428771770183,122.474737172695)) ;
#22111=CARTESIAN_POINT('Ctrl Pts',(-18.4604722427515,28.2487826898201,122.24045743561)) ;
#22112=CARTESIAN_POINT('Ctrl Pts',(-18.8242413063613,28.438763036991,122.357101788211)) ;
#22113=CARTESIAN_POINT('Ctrl Pts',(-18.6779981948743,28.2587739566281,122.093415286291)) ;
#22114=CARTESIAN_POINT('Ctrl Pts',(-19.0169763775656,28.4487951391229,122.271451770785)) ;
#22115=CARTESIAN_POINT('Ctrl Pts',(-18.918918044841,28.2688060587601,121.986355077235)) ;
#22116=CARTESIAN_POINT('Ctrl Pts',(-19.2182110681717,28.4586620200777,122.221141613254)) ;
#22117=CARTESIAN_POINT('Ctrl Pts',(-19.1704626082505,28.2786729397148,121.923469734543)) ;
#22118=CARTESIAN_POINT('Ctrl Pts',(-19.4277169110003,28.4686538113658,122.205851400272)) ;
#22119=CARTESIAN_POINT('Ctrl Pts',(-19.432345213223,28.288664731003,121.904359612356)) ;
#22120=CARTESIAN_POINT('Ctrl Pts',(-19.6374921877922,28.4786859272774,122.227662227062)) ;
#22121=CARTESIAN_POINT('Ctrl Pts',(-19.694564039776,28.2986968469145,121.93162572317)) ;
#22122=CARTESIAN_POINT('Ctrl Pts',(-19.8370378148064,28.4885522440774,122.284307432454)) ;
#22123=CARTESIAN_POINT('Ctrl Pts',(-19.943995852301,28.3085631637145,122.002434913296)) ;
#22124=CARTESIAN_POINT('Ctrl Pts',(-20.0261278855234,28.498539725551,122.375526578932)) ;
#22125=CARTESIAN_POINT('Ctrl Pts',(-20.1803573809643,28.3185506451881,122.116461326157)) ;
#22126=CARTESIAN_POINT('Ctrl Pts',(-20.1958916606712,28.5084846499299,122.497612228053)) ;
#22127=CARTESIAN_POINT('Ctrl Pts',(-20.3925607131235,28.328495569567,122.269070719418)) ;
#22128=CARTESIAN_POINT('Ctrl Pts',(-20.3432261236584,28.5185295358406,122.64887127178)) ;
#22129=CARTESIAN_POINT('Ctrl Pts',(-20.5767268496923,28.3385404554777,122.458146387094)) ;
#22130=CARTESIAN_POINT('Ctrl Pts',(-20.4600658639641,28.5283916395532,122.820164450749)) ;
#22131=CARTESIAN_POINT('Ctrl Pts',(-20.7227745276264,28.3484025591903,122.672264744843)) ;
#22132=CARTESIAN_POINT('Ctrl Pts',(-20.546882409536,28.5383832033776,123.011421338606)) ;
#22133=CARTESIAN_POINT('Ctrl Pts',(-20.8312927348308,28.3583941230148,122.911337082898)) ;
#22134=CARTESIAN_POINT('Ctrl Pts',(-20.5987837541194,28.5483160114405,123.213686812683)) ;
#22135=CARTESIAN_POINT('Ctrl Pts',(-20.8961668071842,28.3683269310777,123.164169825498)) ;
#22136=CARTESIAN_POINT('Ctrl Pts',(-20.6152968104347,28.5582531136769,123.42195527368)) ;
#22137=CARTESIAN_POINT('Ctrl Pts',(-20.9168053566465,28.378264033314,123.424505796562)) ;
#22138=CARTESIAN_POINT('Ctrl Pts',(-20.5948899082448,28.5683055599473,123.632285532663)) ;
#22139=CARTESIAN_POINT('Ctrl Pts',(-20.8912939664117,28.3883164795844,123.687418366482)) ;
#22140=CARTESIAN_POINT('Ctrl Pts',(-20.5397117951602,28.5781516755289,123.831810652888)) ;
#22141=CARTESIAN_POINT('Ctrl Pts',(-20.8223185569164,28.398162595166,123.936824298385)) ;
#22142=CARTESIAN_POINT('Ctrl Pts',(-20.4492135047243,28.5881996952438,124.022668210418)) ;
#22143=CARTESIAN_POINT('Ctrl Pts',(-20.709193147176,28.4082106148809,124.175395051952)) ;
#22144=CARTESIAN_POINT('Ctrl Pts',(-20.3279884165152,28.5981416468727,124.192947955947)) ;
#22145=CARTESIAN_POINT('Ctrl Pts',(-20.5576594223878,28.4181525665098,124.388243230741)) ;
#22146=CARTESIAN_POINT('Ctrl Pts',(-20.1794561705445,28.6080804278718,124.339907298682)) ;
#22147=CARTESIAN_POINT('Ctrl Pts',(-20.3719920554206,28.4280913475089,124.571940487482)) ;
#22148=CARTESIAN_POINT('Ctrl Pts',(-20.0060768723233,28.6181064765979,124.459748019633)) ;
#22149=CARTESIAN_POINT('Ctrl Pts',(-20.155266255181,28.438117396235,124.721739105602)) ;
#22150=CARTESIAN_POINT('Ctrl Pts',(-19.8172567237363,28.6279933370061,124.546699844584)) ;
#22151=CARTESIAN_POINT('Ctrl Pts',(-19.9192398618305,28.4480042566432,124.830426395165)) ;
#22152=CARTESIAN_POINT('Ctrl Pts',(-19.6133539599856,28.6380246121379,124.600393761194)) ;
#22153=CARTESIAN_POINT('Ctrl Pts',(-19.6643603212813,28.458035531775,124.897541005947)) ;
#22154=CARTESIAN_POINT('Ctrl Pts',(-19.4062711547036,28.6479075894383,124.617827169365)) ;
#22155=CARTESIAN_POINT('Ctrl Pts',(-19.405507635062,28.4679185090754,124.919330220156)) ;
#22156=CARTESIAN_POINT('Ctrl Pts',(-19.1957631832706,28.6579644428455,124.598722627596)) ;
#22157=CARTESIAN_POINT('Ctrl Pts',(-19.14236864725,28.4779753624826,124.895445755536)) ;
#22158=CARTESIAN_POINT('Ctrl Pts',(-18.9283731228152,28.6711326839214,124.526630695589)) ;
#22159=CARTESIAN_POINT('Ctrl Pts',(-18.8081529113529,28.4911436035585,124.80533200887)) ;
#22160=CARTESIAN_POINT('Ctrl Pts',(-18.6817983350219,28.6845337131479,124.384021538888)) ;
#22161=CARTESIAN_POINT('Ctrl Pts',(-18.4999549682012,28.504544632785,124.627092881207)) ;
#22162=CARTESIAN_POINT('Ctrl Pts',(-18.4857344421306,28.6977466298788,124.187192207811)) ;
#22163=CARTESIAN_POINT('Ctrl Pts',(-18.2548346129752,28.5177575495159,124.381018273064)) ;
#22164=CARTESIAN_POINT('Ctrl Pts',(-18.3657858162467,28.707675024332,124.016416499208)) ;
#22165=CARTESIAN_POINT('Ctrl Pts',(-18.1049098192041,28.5276859439691,124.167554176501)) ;
#22166=CARTESIAN_POINT('Ctrl Pts',(-18.2766712212058,28.7176565244601,123.826404589139)) ;
#22167=CARTESIAN_POINT('Ctrl Pts',(-17.9935167509591,28.5376674440972,123.930036177092)) ;
#22168=CARTESIAN_POINT('Ctrl Pts',(-18.2218707889986,28.7276970677302,123.622569483315)) ;
#22169=CARTESIAN_POINT('Ctrl Pts',(-17.9250194853092,28.5477079873673,123.675241990111)) ;
#22170=CARTESIAN_POINT('Ctrl Pts',(-18.2033757282844,28.7375463995133,123.416330418717)) ;
#22171=CARTESIAN_POINT('Ctrl Pts',(-17.9019033242933,28.5575573191504,123.417442838969)) ;
#22172=CARTESIAN_POINT('Ctrl Pts',(-18.2206940069242,28.747541803985,123.206912125949)) ;
#22173=CARTESIAN_POINT('Ctrl Pts',(-17.9235537436292,28.5675527236221,123.155670875178)) ;
#22174=CARTESIAN_POINT('Ctrl Pts',(-18.2745872662887,28.7575581314336,123.003350839589)) ;
#22175=CARTESIAN_POINT('Ctrl Pts',(-17.990923682755,28.5775690510707,122.901217359065)) ;
#22176=CARTESIAN_POINT('Ctrl Pts',(-18.3909335432918,28.7707817886001,122.750824717369)) ;
#22177=CARTESIAN_POINT('Ctrl Pts',(-18.1363563321866,28.5907927082372,122.585573838039)) ;
#22178=CARTESIAN_POINT('Ctrl Pts',(-18.5712652888683,28.7840760799895,122.533196711622)) ;
#22179=CARTESIAN_POINT('Ctrl Pts',(-18.361738888197,28.6040869996266,122.313564150216)) ;
#22180=CARTESIAN_POINT('Ctrl Pts',(-18.799057046922,28.797360430921,122.371600064136)) ;
#22181=CARTESIAN_POINT('Ctrl Pts',(-18.6465253994931,28.6173713505581,122.111531614028)) ;
#22182=CARTESIAN_POINT('Ctrl Pts',(-18.9884277129976,28.8073328119828,122.281692967666)) ;
#22183=CARTESIAN_POINT('Ctrl Pts',(-18.8832307222806,28.6273437316199,121.999158080089)) ;
#22184=CARTESIAN_POINT('Ctrl Pts',(-19.1891836686621,28.8172411916084,122.226029840972)) ;
#22185=CARTESIAN_POINT('Ctrl Pts',(-19.1341788049863,28.6372521112455,121.929579826141)) ;
#22186=CARTESIAN_POINT('Ctrl Pts',(-19.3995659070131,28.8272951903564,122.205875393867)) ;
#22187=CARTESIAN_POINT('Ctrl Pts',(-19.3971551455222,28.6473061099936,121.904389073441)) ;
#22188=CARTESIAN_POINT('Ctrl Pts',(-19.6062836932465,28.8371573874727,122.222079550303)) ;
#22189=CARTESIAN_POINT('Ctrl Pts',(-19.6555567772795,28.6571683071099,121.924649710965)) ;
#22190=CARTESIAN_POINT('Ctrl Pts',(-19.8780826757267,28.8505045138469,122.29182043757)) ;
#22191=CARTESIAN_POINT('Ctrl Pts',(-19.9952798306344,28.670515433484,122.011813758423)) ;
#22192=CARTESIAN_POINT('Ctrl Pts',(-20.1845000475927,28.8670414794883,122.464288153073)) ;
#22193=CARTESIAN_POINT('Ctrl Pts',(-20.3783371558031,28.6870523991254,122.227433848027)) ;
#22194=CARTESIAN_POINT('Ctrl Pts',(-20.4154369591003,28.8836760836622,122.732174044355)) ;
#22195=CARTESIAN_POINT('Ctrl Pts',(-20.6669572705968,28.7036870032994,122.562229846375)) ;
#22196=CARTESIAN_POINT('Ctrl Pts',(-20.5367399369156,28.8969658769049,122.98386445411)) ;
#22197=CARTESIAN_POINT('Ctrl Pts',(-20.818619503667,28.716976796542,122.876897221786)) ;
#22198=CARTESIAN_POINT('Ctrl Pts',(-20.5937434976173,28.9069185081643,123.1851719771)) ;
#22199=CARTESIAN_POINT('Ctrl Pts',(-20.8898646071741,28.7269294278014,123.12852052043)) ;
#22200=CARTESIAN_POINT('Ctrl Pts',(-20.6151704596498,28.916870475469,123.393312690541)) ;
#22201=CARTESIAN_POINT('Ctrl Pts',(-20.916646989976,28.7368813951061,123.388702342932)) ;
#22202=CARTESIAN_POINT('Ctrl Pts',(-20.5948058201253,28.9302377339328,123.673577606172)) ;
#22203=CARTESIAN_POINT('Ctrl Pts',(-20.891192739327,28.7502486535699,123.739016958567)) ;
#22204=CARTESIAN_POINT('Ctrl Pts',(-20.4800520817175,28.9467545458819,124.005580786161)) ;
#22205=CARTESIAN_POINT('Ctrl Pts',(-20.7477418810432,28.7667654655191,124.154036877155)) ;
#22206=CARTESIAN_POINT('Ctrl Pts',(-20.2120144615373,28.9667804408883,124.336293100921)) ;
#22207=CARTESIAN_POINT('Ctrl Pts',(-20.4126932064644,28.7867913605254,124.567418944492)) ;
#22208=CARTESIAN_POINT('Ctrl Pts',(-19.8510301281953,28.9865911710184,124.553536596618)) ;
#22209=CARTESIAN_POINT('Ctrl Pts',(-19.9614615275447,28.8066020906556,124.838970603354)) ;
#22210=CARTESIAN_POINT('Ctrl Pts',(-19.4344012108349,29.0065683871483,124.636109825588)) ;
#22211=CARTESIAN_POINT('Ctrl Pts',(-19.4406750274565,28.8265793067854,124.942183198345)) ;
#22212=CARTESIAN_POINT('Ctrl Pts',(-19.0157681070412,29.0264952625436,124.57095034557)) ;
#22213=CARTESIAN_POINT('Ctrl Pts',(-18.9173848458449,28.8465061821807,124.860730356123)) ;
#22214=CARTESIAN_POINT('Ctrl Pts',(-18.6457374117665,29.0463167240198,124.369076668043)) ;
#22215=CARTESIAN_POINT('Ctrl Pts',(-18.4548495376105,28.866327643657,124.608386572972)) ;
#22216=CARTESIAN_POINT('Ctrl Pts',(-18.3635430708779,29.0663910418292,124.048922971134)) ;
#22217=CARTESIAN_POINT('Ctrl Pts',(-18.1021082199431,28.8864019614663,124.20819190284)) ;
#22218=CARTESIAN_POINT('Ctrl Pts',(-18.2096162661091,29.0862390108371,123.655849066001)) ;
#22219=CARTESIAN_POINT('Ctrl Pts',(-17.9097030414757,28.9062499304742,123.716849978485)) ;
#22220=CARTESIAN_POINT('Ctrl Pts',(-18.1981447189495,29.1061860449003,123.231968651957)) ;
#22221=CARTESIAN_POINT('Ctrl Pts',(-17.8953659112392,28.9261969645374,123.187000088179)) ;
#22222=CARTESIAN_POINT('Ctrl Pts',(-18.3318077694759,29.1260819958724,122.830562780161)) ;
#22223=CARTESIAN_POINT('Ctrl Pts',(-18.0624463345147,28.9460929155096,122.685244684184)) ;
#22224=CARTESIAN_POINT('Ctrl Pts',(-18.5938358537856,29.1459774754907,122.498483434728)) ;
#22225=CARTESIAN_POINT('Ctrl Pts',(-18.3899816868081,28.9659883951278,122.270147568337)) ;
#22226=CARTESIAN_POINT('Ctrl Pts',(-18.9545509966917,29.1659335864555,122.274963150452)) ;
#22227=CARTESIAN_POINT('Ctrl Pts',(-18.8408757372252,28.9859445060926,121.990748528834)) ;
#22228=CARTESIAN_POINT('Ctrl Pts',(-19.3687523473574,29.1858381344955,122.188317116435)) ;
#22229=CARTESIAN_POINT('Ctrl Pts',(-19.3586261760562,29.0058490541326,121.882442313881)) ;
#22230=CARTESIAN_POINT('Ctrl Pts',(-19.7873033294093,29.2057122588146,122.247090838418)) ;
#22231=CARTESIAN_POINT('Ctrl Pts',(-19.8818129365437,29.0257231784517,121.95590917428)) ;
#22232=CARTESIAN_POINT('Ctrl Pts',(-20.1636458920224,29.2257667888136,122.447434307739)) ;
#22233=CARTESIAN_POINT('Ctrl Pts',(-20.3522418344828,29.0457777084507,122.206339109689)) ;
#22234=CARTESIAN_POINT('Ctrl Pts',(-20.4457143490153,29.2455743025736,122.760308780651)) ;
#22235=CARTESIAN_POINT('Ctrl Pts',(-20.7048254925126,29.0655852222107,122.597429836113)) ;
#22236=CARTESIAN_POINT('Ctrl Pts',(-20.6062625022629,29.2655576583413,123.153645694702)) ;
#22237=CARTESIAN_POINT('Ctrl Pts',(-20.9055115949536,29.0855685779784,123.089100356984)) ;
#22238=CARTESIAN_POINT('Ctrl Pts',(-20.6222571826096,29.2854759609252,123.57685578804)) ;
#22239=CARTESIAN_POINT('Ctrl Pts',(-20.9255057422183,29.1054868805624,123.618111697477)) ;
#22240=CARTESIAN_POINT('Ctrl Pts',(-20.4942524999631,29.305344176371,123.97953847386)) ;
#22241=CARTESIAN_POINT('Ctrl Pts',(-20.7655021762044,29.1253550960081,124.121463964361)) ;
#22242=CARTESIAN_POINT('Ctrl Pts',(-20.2337505644514,29.3253944931673,124.316857983923)) ;
#22243=CARTESIAN_POINT('Ctrl Pts',(-20.4398756731327,29.1454054128044,124.543114839599)) ;
#22244=CARTESIAN_POINT('Ctrl Pts',(-19.8787560188095,29.3451705550497,124.542547094781)) ;
#22245=CARTESIAN_POINT('Ctrl Pts',(-19.9961359923068,29.1651814746869,124.82522657557)) ;
#22246=CARTESIAN_POINT('Ctrl Pts',(-19.4626770517434,29.3652251607422,124.635063105545)) ;
#22247=CARTESIAN_POINT('Ctrl Pts',(-19.4760372478541,29.1852360803793,124.9408742549)) ;
#22248=CARTESIAN_POINT('Ctrl Pts',(-19.0452208405963,29.3850188498981,124.580591047788)) ;
#22249=CARTESIAN_POINT('Ctrl Pts',(-18.9542188864203,29.2050297695352,124.872787108227)) ;
#22250=CARTESIAN_POINT('Ctrl Pts',(-18.6678065643519,29.4049855414925,124.386372516553)) ;
#22251=CARTESIAN_POINT('Ctrl Pts',(-18.4824497195716,29.2249964611296,124.630017164074)) ;
#22252=CARTESIAN_POINT('Ctrl Pts',(-18.379791129464,29.4249455872434,124.074550900543)) ;
#22253=CARTESIAN_POINT('Ctrl Pts',(-18.1224282621344,29.2449565068806,124.240242601981)) ;
#22254=CARTESIAN_POINT('Ctrl Pts',(-18.2157634731263,29.4448438473937,123.684577273612)) ;
#22255=CARTESIAN_POINT('Ctrl Pts',(-17.9173907834527,29.2648547670308,123.752777846934)) ;
#22256=CARTESIAN_POINT('Ctrl Pts',(-18.1941500603982,29.4647387629429,123.262128718319)) ;
#22257=CARTESIAN_POINT('Ctrl Pts',(-17.8903701259974,29.28474968258,123.224718223152)) ;
#22258=CARTESIAN_POINT('Ctrl Pts',(-18.3177155519128,29.4846489433565,122.85722218228)) ;
#22259=CARTESIAN_POINT('Ctrl Pts',(-18.0448227791641,29.3046598629936,122.718584462674)) ;
#22260=CARTESIAN_POINT('Ctrl Pts',(-18.5722210885648,29.5045847424707,122.518222965031)) ;
#22261=CARTESIAN_POINT('Ctrl Pts',(-18.3629508949474,29.3245956621079,122.294833096222)) ;
#22262=CARTESIAN_POINT('Ctrl Pts',(-18.9271398359767,29.5245226041249,122.286384499788)) ;
#22263=CARTESIAN_POINT('Ctrl Pts',(-18.8065966645385,29.344533523762,122.005031573975)) ;
#22264=CARTESIAN_POINT('Ctrl Pts',(-19.3394465637527,29.5444416507625,122.189407632929)) ;
#22265=CARTESIAN_POINT('Ctrl Pts',(-19.3219781329333,29.3644525703997,121.88380547982)) ;
#22266=CARTESIAN_POINT('Ctrl Pts',(-19.7607048779396,29.5643905488167,122.23896191623)) ;
#22267=CARTESIAN_POINT('Ctrl Pts',(-19.8485530096058,29.3844014684538,121.945745518254)) ;
#22268=CARTESIAN_POINT('Ctrl Pts',(-20.1390238650554,29.5842963762597,122.428800132525)) ;
#22269=CARTESIAN_POINT('Ctrl Pts',(-20.3214474198052,29.4043072958969,122.18303123303)) ;
#22270=CARTESIAN_POINT('Ctrl Pts',(-20.381503088585,29.600879071625,122.684669772167)) ;
#22271=CARTESIAN_POINT('Ctrl Pts',(-20.6245684184595,29.4208899912622,122.502888255951)) ;
#22272=CARTESIAN_POINT('Ctrl Pts',(-20.5148467807965,29.6141532853487,122.929890317395)) ;
#22273=CARTESIAN_POINT('Ctrl Pts',(-20.791234180934,29.4341642049858,122.809390920718)) ;
#22274=CARTESIAN_POINT('Ctrl Pts',(-20.5818729164079,29.624200004548,123.130156956782)) ;
#22275=CARTESIAN_POINT('Ctrl Pts',(-20.8750220852076,29.4442109241851,123.05973121324)) ;
#22276=CARTESIAN_POINT('Ctrl Pts',(-20.6127109296286,29.6340440391937,123.334823989138)) ;
#22277=CARTESIAN_POINT('Ctrl Pts',(-20.9135737768039,29.4540549588308,123.315549607641)) ;
#22278=CARTESIAN_POINT('Ctrl Pts',(-20.6063479572666,29.6473784240982,123.615020683285)) ;
#22279=CARTESIAN_POINT('Ctrl Pts',(-20.9056110532671,29.4673893437353,123.665862635849)) ;
#22280=CARTESIAN_POINT('Ctrl Pts',(-20.5072137738658,29.663965641398,123.953603105851)) ;
#22281=CARTESIAN_POINT('Ctrl Pts',(-20.7817183691016,29.4839765610351,124.089008121444)) ;
#22282=CARTESIAN_POINT('Ctrl Pts',(-20.2982490380892,29.6805988534359,124.238824540592)) ;
#22283=CARTESIAN_POINT('Ctrl Pts',(-20.5204871039959,29.500609773073,124.445591168462)) ;
#22284=CARTESIAN_POINT('Ctrl Pts',(-20.0804621860381,29.6938812957081,124.413688383922)) ;
#22285=CARTESIAN_POINT('Ctrl Pts',(-20.2482786094575,29.5138922153452,124.664142759317)) ;
#22286=CARTESIAN_POINT('Ctrl Pts',(-19.8981216436981,29.7037871836223,124.514250466141)) ;
#22287=CARTESIAN_POINT('Ctrl Pts',(-20.0203496111071,29.5237981032594,124.789853895898)) ;
#22288=CARTESIAN_POINT('Ctrl Pts',(-19.6995040700482,29.7137756017274,124.582447696612)) ;
#22289=CARTESIAN_POINT('Ctrl Pts',(-19.7720804977814,29.5337865213645,124.875101645455)) ;
#22290=CARTESIAN_POINT('Ctrl Pts',(-19.491307008318,29.7237990289661,124.615012952645)) ;
#22291=CARTESIAN_POINT('Ctrl Pts',(-19.5118312861888,29.5438099486033,124.9158105401)) ;
#22292=CARTESIAN_POINT('Ctrl Pts',(-19.2831262713956,29.7337034600831,124.611097510971)) ;
#22293=CARTESIAN_POINT('Ctrl Pts',(-19.2516162816116,29.5537143797203,124.910922144998)) ;
#22294=CARTESIAN_POINT('Ctrl Pts',(-19.0093558420609,29.7469666126936,124.55825582872)) ;
#22295=CARTESIAN_POINT('Ctrl Pts',(-18.9093488133413,29.5669775323307,124.844857601197)) ;
#22296=CARTESIAN_POINT('Ctrl Pts',(-18.7545952522591,29.7602915105975,124.434343951779)) ;
#22297=CARTESIAN_POINT('Ctrl Pts',(-18.5909285364746,29.5803024302346,124.689972489664)) ;
#22298=CARTESIAN_POINT('Ctrl Pts',(-18.5439553830956,29.7735472542131,124.251793494169)) ;
#22299=CARTESIAN_POINT('Ctrl Pts',(-18.3276416499704,29.5935581738502,124.461801734779)) ;
#22300=CARTESIAN_POINT('Ctrl Pts',(-18.4117225992589,29.7835066276604,124.089495823393)) ;
#22301=CARTESIAN_POINT('Ctrl Pts',(-18.1623453454126,29.6035175472975,124.258928464813)) ;
#22302=CARTESIAN_POINT('Ctrl Pts',(-18.3095785405791,29.7934504515873,123.907068143892)) ;
#22303=CARTESIAN_POINT('Ctrl Pts',(-18.0346636089127,29.6134613712245,124.030895956569)) ;
#22304=CARTESIAN_POINT('Ctrl Pts',(-18.2401254145393,29.8034983957346,123.707589819514)) ;
#22305=CARTESIAN_POINT('Ctrl Pts',(-17.9478442966657,29.6235093153718,123.781548712612)) ;
#22306=CARTESIAN_POINT('Ctrl Pts',(-18.2068401315693,29.8133493669528,123.503171166359)) ;
#22307=CARTESIAN_POINT('Ctrl Pts',(-17.906234953778,29.6333602865899,123.526025793516)) ;
#22308=CARTESIAN_POINT('Ctrl Pts',(-18.20904682234,29.8233211843949,123.293567779389)) ;
#22309=CARTESIAN_POINT('Ctrl Pts',(-17.9089904954044,29.643332104032,123.264021399714)) ;
#22310=CARTESIAN_POINT('Ctrl Pts',(-18.2477491639959,29.833316606687,123.086997661394)) ;
#22311=CARTESIAN_POINT('Ctrl Pts',(-17.9573656877064,29.6533275263241,123.005808163303)) ;
#22312=CARTESIAN_POINT('Ctrl Pts',(-18.3222034367972,29.8433496718107,122.889655956978)) ;
#22313=CARTESIAN_POINT('Ctrl Pts',(-18.0504309097234,29.6633605914478,122.75912999775)) ;
#22314=CARTESIAN_POINT('Ctrl Pts',(-18.427820698995,29.8532150044759,122.711168026723)) ;
#22315=CARTESIAN_POINT('Ctrl Pts',(-18.1824501820335,29.673225924113,122.536018472183)) ;
#22316=CARTESIAN_POINT('Ctrl Pts',(-18.5636657279792,29.8631755470735,122.551802567031)) ;
#22317=CARTESIAN_POINT('Ctrl Pts',(-18.352254460823,29.6831864667106,122.336809734032)) ;
#22318=CARTESIAN_POINT('Ctrl Pts',(-18.7265192984171,29.8732092325752,122.41775022895)) ;
#22319=CARTESIAN_POINT('Ctrl Pts',(-18.5558196647205,29.6932201522123,122.169242143868)) ;
#22320=CARTESIAN_POINT('Ctrl Pts',(-18.9073064956514,29.8830940645654,122.315216883983)) ;
#22321=CARTESIAN_POINT('Ctrl Pts',(-18.7818025397086,29.7031049842026,122.041072921772)) ;
#22322=CARTESIAN_POINT('Ctrl Pts',(-19.1067239041188,29.8931614913253,122.244413082228)) ;
#22323=CARTESIAN_POINT('Ctrl Pts',(-19.0310733364163,29.7131724109624,121.952565569517)) ;
#22324=CARTESIAN_POINT('Ctrl Pts',(-19.3106948006957,29.9029999804841,122.209895700099)) ;
#22325=CARTESIAN_POINT('Ctrl Pts',(-19.286036901977,29.7230109001213,121.909416064618)) ;
#22326=CARTESIAN_POINT('Ctrl Pts',(-19.5222278617027,29.9130634616742,122.211069618084)) ;
#22327=CARTESIAN_POINT('Ctrl Pts',(-19.550453199473,29.7330743813114,121.910880737687)) ;
#22328=CARTESIAN_POINT('Ctrl Pts',(-19.7268617704073,29.9229576194894,122.24850430312)) ;
#22329=CARTESIAN_POINT('Ctrl Pts',(-19.8062464008285,29.7429685391265,121.957671456219)) ;
#22330=CARTESIAN_POINT('Ctrl Pts',(-19.9229782407006,29.9328994762337,122.320699146715)) ;
#22331=CARTESIAN_POINT('Ctrl Pts',(-20.0513931602021,29.7529103958708,122.047912589705)) ;
#22332=CARTESIAN_POINT('Ctrl Pts',(-20.1047692037057,29.9429019539051,122.426450883275)) ;
#22333=CARTESIAN_POINT('Ctrl Pts',(-20.27863327422,29.7629128735422,122.180100002924)) ;
#22334=CARTESIAN_POINT('Ctrl Pts',(-20.2657090613012,29.9529367582094,122.562825912537)) ;
#22335=CARTESIAN_POINT('Ctrl Pts',(-20.4798098359431,29.7729476778465,122.350566712122)) ;
#22336=CARTESIAN_POINT('Ctrl Pts',(-20.3982580149733,29.962781635055,122.72180138389)) ;
#22337=CARTESIAN_POINT('Ctrl Pts',(-20.64549843004,29.7827925546922,122.549284780308)) ;
#22338=CARTESIAN_POINT('Ctrl Pts',(-20.5029831129388,29.9727675146106,122.903710362573)) ;
#22339=CARTESIAN_POINT('Ctrl Pts',(-20.7764071388104,29.7927784342477,122.776669844146)) ;
#22340=CARTESIAN_POINT('Ctrl Pts',(-20.5743335334042,29.9827022449691,123.100047335692)) ;
#22341=CARTESIAN_POINT('Ctrl Pts',(-20.8655976909384,29.8027131646062,123.022090489185)) ;
#22342=CARTESIAN_POINT('Ctrl Pts',(-20.6107482776223,29.992760057282,123.308299706397)) ;
#22343=CARTESIAN_POINT('Ctrl Pts',(-20.911118673284,29.8127709769191,123.2824053866)) ;
#22344=CARTESIAN_POINT('Ctrl Pts',(-20.6108122645727,30.0025806494063,123.514793587701)) ;
#22345=CARTESIAN_POINT('Ctrl Pts',(-20.9112011989042,29.8225915690435,123.540523528446)) ;
#22346=CARTESIAN_POINT('Ctrl Pts',(-20.5743946708493,30.0126472350161,123.723224917904)) ;
#22347=CARTESIAN_POINT('Ctrl Pts',(-20.8656816934186,29.8326581546532,123.801062971402)) ;
#22348=CARTESIAN_POINT('Ctrl Pts',(-20.5034684423452,30.0225468155979,123.918938589695)) ;
#22349=CARTESIAN_POINT('Ctrl Pts',(-20.7770260888292,29.8425577352351,124.045706385067)) ;
#22350=CARTESIAN_POINT('Ctrl Pts',(-20.398156180313,30.0325984152762,124.102097749828)) ;
#22351=CARTESIAN_POINT('Ctrl Pts',(-20.6453879764234,29.8526093349133,124.274656477308)) ;
#22352=CARTESIAN_POINT('Ctrl Pts',(-20.2651035498594,30.0424726016932,124.261488906871)) ;
#22353=CARTESIAN_POINT('Ctrl Pts',(-20.4790736605817,29.8624835213303,124.473897491922)) ;
#22354=CARTESIAN_POINT('Ctrl Pts',(-20.1036145885846,30.0525290775741,124.397880998235)) ;
#22355=CARTESIAN_POINT('Ctrl Pts',(-20.2772141277769,29.8725399972112,124.644389380226)) ;
#22356=CARTESIAN_POINT('Ctrl Pts',(-19.9238362938821,30.0624220088767,124.502541628328)) ;
#22357=CARTESIAN_POINT('Ctrl Pts',(-20.0524919644059,29.8824329285138,124.775217544899)) ;
#22358=CARTESIAN_POINT('Ctrl Pts',(-19.7253526604774,30.0724847875893,124.575641997785)) ;
#22359=CARTESIAN_POINT('Ctrl Pts',(-19.8043884253136,29.8924957072264,124.866595201475)) ;
#22360=CARTESIAN_POINT('Ctrl Pts',(-19.5217089265332,30.0823273131705,124.612461273804)) ;
#22361=CARTESIAN_POINT('Ctrl Pts',(-19.5498333322758,29.9023382328076,124.91262179111)) ;
#22362=CARTESIAN_POINT('Ctrl Pts',(-19.3117032501177,30.0923180785953,124.613877366419)) ;
#22363=CARTESIAN_POINT('Ctrl Pts',(-19.2873260771025,29.9123289982325,124.914394172825)) ;
#22364=CARTESIAN_POINT('Ctrl Pts',(-19.1059111788541,30.1022461545934,124.578985148832)) ;
#22365=CARTESIAN_POINT('Ctrl Pts',(-19.0300851291776,29.9222570742305,124.870781057726)) ;
#22366=CARTESIAN_POINT('Ctrl Pts',(-18.9079961280173,30.1122340649804,124.508814514259)) ;
#22367=CARTESIAN_POINT('Ctrl Pts',(-18.7826904157509,29.9322449846175,124.783069756764)) ;
#22368=CARTESIAN_POINT('Ctrl Pts',(-18.7245848851423,30.1222699771053,124.404544827108)) ;
#22369=CARTESIAN_POINT('Ctrl Pts',(-18.5534253143983,29.9422808967425,124.652734665094)) ;
#22370=CARTESIAN_POINT('Ctrl Pts',(-18.5647574103382,30.132124989953,124.272686477183)) ;
#22371=CARTESIAN_POINT('Ctrl Pts',(-18.3536388771245,29.9521359095901,124.487912827377)) ;
#22372=CARTESIAN_POINT('Ctrl Pts',(-18.4280975268948,30.1421239358693,124.11300608856)) ;
#22373=CARTESIAN_POINT('Ctrl Pts',(-18.1828123336801,29.9621348555064,124.288313606199)) ;
#22374=CARTESIAN_POINT('Ctrl Pts',(-18.3221216583478,30.1520208483173,123.933916262018)) ;
#22375=CARTESIAN_POINT('Ctrl Pts',(-18.0503403718914,29.9720317679544,124.064451745925)) ;
#22376=CARTESIAN_POINT('Ctrl Pts',(-18.2476869675524,30.1620746464108,123.736121592027)) ;
#22377=CARTESIAN_POINT('Ctrl Pts',(-17.9572951648542,29.9820855660479,123.817209301492)) ;
#22378=CARTESIAN_POINT('Ctrl Pts',(-18.209328142363,30.1719555672375,123.531942530913)) ;
#22379=CARTESIAN_POINT('Ctrl Pts',(-17.9093444927588,29.9919664868746,123.56198502385)) ;
#22380=CARTESIAN_POINT('Ctrl Pts',(-18.2065963316718,30.1819600932352,123.321657997475)) ;
#22381=CARTESIAN_POINT('Ctrl Pts',(-17.9059278138796,30.0019710128723,123.299129283876)) ;
#22382=CARTESIAN_POINT('Ctrl Pts',(-18.2404207061427,30.1919440568527,123.114471153255)) ;
#22383=CARTESIAN_POINT('Ctrl Pts',(-17.9482064112771,30.0119549764898,123.040145215749)) ;
#22384=CARTESIAN_POINT('Ctrl Pts',(-18.31026366629,30.201983697404,122.915313410186)) ;
#22385=CARTESIAN_POINT('Ctrl Pts',(-18.035508186737,30.0219946170411,122.791197498885)) ;
#22386=CARTESIAN_POINT('Ctrl Pts',(-18.4113981835528,30.2118277230187,122.734755075974)) ;
#22387=CARTESIAN_POINT('Ctrl Pts',(-18.161925212928,30.0318386426558,122.565497657734)) ;
#22388=CARTESIAN_POINT('Ctrl Pts',(-18.5438338536838,30.221818728836,122.571724660386)) ;
#22389=CARTESIAN_POINT('Ctrl Pts',(-18.3274685805744,30.0418296484732,122.361708399386)) ;
#22390=CARTESIAN_POINT('Ctrl Pts',(-18.7036229588605,30.2318565203682,122.433886669261)) ;
#22391=CARTESIAN_POINT('Ctrl Pts',(-18.5272036340267,30.0518674400053,122.189409573137)) ;
#22392=CARTESIAN_POINT('Ctrl Pts',(-18.8812446957364,30.2417009201566,122.327651393259)) ;
#22393=CARTESIAN_POINT('Ctrl Pts',(-18.749230903998,30.0617118397937,122.056613364073)) ;
#22394=CARTESIAN_POINT('Ctrl Pts',(-19.0771915548651,30.2516857207133,122.252443734513)) ;
#22395=CARTESIAN_POINT('Ctrl Pts',(-18.994164126273,30.0716966403505,121.962602178295)) ;
#22396=CARTESIAN_POINT('Ctrl Pts',(-19.2823241886974,30.2616252441245,122.212483119528)) ;
#22397=CARTESIAN_POINT('Ctrl Pts',(-19.2505801464928,30.0816361637616,121.912649736868)) ;
#22398=CARTESIAN_POINT('Ctrl Pts',(-19.4933414984696,30.2716649632255,122.20875992218)) ;
#22399=CARTESIAN_POINT('Ctrl Pts',(-19.5143516088782,30.0916758828626,121.907994125418)) ;
#22400=CARTESIAN_POINT('Ctrl Pts',(-19.698697204164,30.2815531351448,122.241136729093)) ;
#22401=CARTESIAN_POINT('Ctrl Pts',(-19.7710473972636,30.1015640547819,121.948463714533)) ;
#22402=CARTESIAN_POINT('Ctrl Pts',(-19.8974368961156,30.2915426975618,122.308992544338)) ;
#22403=CARTESIAN_POINT('Ctrl Pts',(-20.0194726827981,30.1115536171989,122.033282181041)) ;
#22404=CARTESIAN_POINT('Ctrl Pts',(-20.0807289084001,30.3015010697565,122.410148468044)) ;
#22405=CARTESIAN_POINT('Ctrl Pts',(-20.2485888048623,30.1215119893936,122.159725978258)) ;
#22406=CARTESIAN_POINT('Ctrl Pts',(-20.2430415790186,30.3114011439872,122.540440637745)) ;
#22407=CARTESIAN_POINT('Ctrl Pts',(-20.451481155513,30.1314120636243,122.322590700227)) ;
#22408=CARTESIAN_POINT('Ctrl Pts',(-20.3822575057102,30.3214472403608,122.699250508298)) ;
#22409=CARTESIAN_POINT('Ctrl Pts',(-20.6255019413428,30.1414581599979,122.521102011054)) ;
#22410=CARTESIAN_POINT('Ctrl Pts',(-20.4903053212277,30.3313558243579,122.877358635903)) ;
#22411=CARTESIAN_POINT('Ctrl Pts',(-20.7605632740528,30.151366743995,122.743737177707)) ;
#22412=CARTESIAN_POINT('Ctrl Pts',(-20.56692385887,30.3413664029488,123.073373311009)) ;
#22413=CARTESIAN_POINT('Ctrl Pts',(-20.8563375787038,30.1613773225859,122.988755129718)) ;
#22414=CARTESIAN_POINT('Ctrl Pts',(-20.6080032804155,30.3513955610616,123.280185120993)) ;
#22415=CARTESIAN_POINT('Ctrl Pts',(-20.9076881587369,30.1714064806987,123.247269528944)) ;
#22416=CARTESIAN_POINT('Ctrl Pts',(-20.6127668223826,30.3612484428997,123.487255373469)) ;
#22417=CARTESIAN_POINT('Ctrl Pts',(-20.913643859901,30.1812593625368,123.506108579083)) ;
#22418=CARTESIAN_POINT('Ctrl Pts',(-20.5818009833245,30.3712080040507,123.694340585296)) ;
#22419=CARTESIAN_POINT('Ctrl Pts',(-20.8749374874299,30.1912189236878,123.764965708006)) ;
#22420=CARTESIAN_POINT('Ctrl Pts',(-20.5144631349101,30.3812464386398,123.894334448527)) ;
#22421=CARTESIAN_POINT('Ctrl Pts',(-20.7907663164554,30.2012573582769,124.014958246547)) ;
#22422=CARTESIAN_POINT('Ctrl Pts',(-20.4154074111559,30.3911197108669,124.076778134823)) ;
#22423=CARTESIAN_POINT('Ctrl Pts',(-20.6669470046296,30.211130630504,124.243014320118)) ;
#22424=CARTESIAN_POINT('Ctrl Pts',(-20.283556385648,30.4011929528604,124.24244097245)) ;
#22425=CARTESIAN_POINT('Ctrl Pts',(-20.5021342923516,30.2212038724976,124.450093173102)) ;
#22426=CARTESIAN_POINT('Ctrl Pts',(-20.1290404897392,30.4110132843935,124.379433616432)) ;
#22427=CARTESIAN_POINT('Ctrl Pts',(-20.3089888716899,30.2310242040306,124.621335698669)) ;
#22428=CARTESIAN_POINT('Ctrl Pts',(-19.9486420914419,30.4210919456203,124.490474607517)) ;
#22429=CARTESIAN_POINT('Ctrl Pts',(-20.0834917211719,30.2411028652574,124.760137415769)) ;
#22430=CARTESIAN_POINT('Ctrl Pts',(-19.7560754413222,30.4309435409145,124.566851656652)) ;
#22431=CARTESIAN_POINT('Ctrl Pts',(-19.8427824861803,30.2509544605516,124.855609977345)) ;
#22432=CARTESIAN_POINT('Ctrl Pts',(-19.5487326187181,30.4410166761433,124.609735878305)) ;
#22433=CARTESIAN_POINT('Ctrl Pts',(-19.5836045391597,30.2610275957804,124.909215904106)) ;
#22434=CARTESIAN_POINT('Ctrl Pts',(-19.3418837703433,30.4508591116683,124.615794712703)) ;
#22435=CARTESIAN_POINT('Ctrl Pts',(-19.3250420856673,30.2708700313055,124.916790254833)) ;
#22436=CARTESIAN_POINT('Ctrl Pts',(-19.1341767024053,30.4608398808017,124.586121780913)) ;
#22437=CARTESIAN_POINT('Ctrl Pts',(-19.0654078751379,30.2808508004389,124.879699535808)) ;
#22438=CARTESIAN_POINT('Ctrl Pts',(-18.9341621364853,30.4708569820456,124.520222155215)) ;
#22439=CARTESIAN_POINT('Ctrl Pts',(-18.8153894691253,30.2908679016827,124.797325621791)) ;
#22440=CARTESIAN_POINT('Ctrl Pts',(-18.7508125062853,30.4807454296474,124.422211803213)) ;
#22441=CARTESIAN_POINT('Ctrl Pts',(-18.5862012535222,30.3007563492846,124.674812609811)) ;
#22442=CARTESIAN_POINT('Ctrl Pts',(-18.5845129446099,30.4908011438283,124.291721984471)) ;
#22443=CARTESIAN_POINT('Ctrl Pts',(-18.378326748722,30.3108120634654,124.511700910524)) ;
#22444=CARTESIAN_POINT('Ctrl Pts',(-18.44588508889,30.5006763502421,124.137161226805)) ;
#22445=CARTESIAN_POINT('Ctrl Pts',(-18.2050407985295,30.3206872698793,124.31849941652)) ;
#22446=CARTESIAN_POINT('Ctrl Pts',(-18.3344500450704,30.5106714027149,123.959022928956)) ;
#22447=CARTESIAN_POINT('Ctrl Pts',(-18.065746667546,30.330682322352,124.095826539079)) ;
#22448=CARTESIAN_POINT('Ctrl Pts',(-18.2557384460612,30.520693286677,123.763577906026)) ;
#22449=CARTESIAN_POINT('Ctrl Pts',(-17.9673568014916,30.3407042063141,123.851520456621)) ;
#22450=CARTESIAN_POINT('Ctrl Pts',(-18.2124447067718,30.5305972592063,123.559917806185)) ;
#22451=CARTESIAN_POINT('Ctrl Pts',(-17.9132391133063,30.3506081788434,123.596944459868)) ;
#22452=CARTESIAN_POINT('Ctrl Pts',(-18.204806352772,30.5405857558672,123.350065475818)) ;
#22453=CARTESIAN_POINT('Ctrl Pts',(-17.9036909635563,30.3605966755043,123.334628818861)) ;
#22454=CARTESIAN_POINT('Ctrl Pts',(-18.2337889801412,30.5505495531152,123.142620805064)) ;
#22455=CARTESIAN_POINT('Ctrl Pts',(-17.9399190541115,30.3705604727523,123.075322497842)) ;
#22456=CARTESIAN_POINT('Ctrl Pts',(-18.2974874686317,30.5604535764232,122.944369701572)) ;
#22457=CARTESIAN_POINT('Ctrl Pts',(-18.019542401481,30.3804644960603,122.827507706759)) ;
#22458=CARTESIAN_POINT('Ctrl Pts',(-18.3963113380305,30.5705140797448,122.757403023843)) ;
#22459=CARTESIAN_POINT('Ctrl Pts',(-18.1430719623568,30.3905249993819,122.593799613876)) ;
#22460=CARTESIAN_POINT('Ctrl Pts',(-18.5230838015688,30.5803546148847,122.593882778984)) ;
#22461=CARTESIAN_POINT('Ctrl Pts',(-18.3015384279696,30.4003655345218,122.38939813401)) ;
#22462=CARTESIAN_POINT('Ctrl Pts',(-18.6795561688118,30.5904168355893,122.451559837919)) ;
#22463=CARTESIAN_POINT('Ctrl Pts',(-18.4971286724099,30.4104277552264,122.211494771059)) ;
#22464=CARTESIAN_POINT('Ctrl Pts',(-18.8555743115362,30.6003139893655,122.340587366803)) ;
#22465=CARTESIAN_POINT('Ctrl Pts',(-18.7171521979687,30.4203249090026,122.072778646605)) ;
#22466=CARTESIAN_POINT('Ctrl Pts',(-19.0485703229917,30.610245122751,122.260955111829)) ;
#22467=CARTESIAN_POINT('Ctrl Pts',(-18.9583979844501,30.4302560423881,121.973238309069)) ;
#22468=CARTESIAN_POINT('Ctrl Pts',(-19.2547965608815,30.6202874978967,122.215768412004)) ;
#22469=CARTESIAN_POINT('Ctrl Pts',(-19.216180617271,30.4402984175338,121.916755158295)) ;
#22470=CARTESIAN_POINT('Ctrl Pts',(-19.4624589820246,30.6301734356628,122.207050198295)) ;
#22471=CARTESIAN_POINT('Ctrl Pts',(-19.4757597411927,30.4501843553,121.905857590778)) ;
#22472=CARTESIAN_POINT('Ctrl Pts',(-19.6707860504758,30.6401692786477,122.234500227154)) ;
#22473=CARTESIAN_POINT('Ctrl Pts',(-19.7361687240311,30.4601801982848,121.940170527014)) ;
#22474=CARTESIAN_POINT('Ctrl Pts',(-19.8701217771489,30.6501112565263,122.297396578507)) ;
#22475=CARTESIAN_POINT('Ctrl Pts',(-19.9853388632678,30.4701221761634,122.018791502423)) ;
#22476=CARTESIAN_POINT('Ctrl Pts',(-20.0559439542631,30.6600706310073,122.393853881732)) ;
#22477=CARTESIAN_POINT('Ctrl Pts',(-20.2176167858868,30.4800815506444,122.139363771227)) ;
#22478=CARTESIAN_POINT('Ctrl Pts',(-20.2229095752647,30.6700672468411,122.521521564149)) ;
#22479=CARTESIAN_POINT('Ctrl Pts',(-20.4263236161457,30.4900781664782,122.298948878856)) ;
#22480=CARTESIAN_POINT('Ctrl Pts',(-20.3654814517331,30.6801014654146,122.676991794271)) ;
#22481=CARTESIAN_POINT('Ctrl Pts',(-20.6045380695498,30.5001123850517,122.493286837832)) ;
#22482=CARTESIAN_POINT('Ctrl Pts',(-20.4770590422529,30.6899545326252,122.851511404317)) ;
#22483=CARTESIAN_POINT('Ctrl Pts',(-20.7440103711108,30.5099654522623,122.711437778196)) ;
#22484=CARTESIAN_POINT('Ctrl Pts',(-20.5580675426808,30.6999147905028,123.044595067161)) ;
#22485=CARTESIAN_POINT('Ctrl Pts',(-20.8452704862501,30.5199257101399,122.952793072304)) ;
#22486=CARTESIAN_POINT('Ctrl Pts',(-20.6044003781511,30.7099438172084,123.250294695878)) ;
#22487=CARTESIAN_POINT('Ctrl Pts',(-20.9031858777252,30.5299547368455,123.209917654151)) ;
#22488=CARTESIAN_POINT('Ctrl Pts',(-20.6142563398137,30.7198540242428,123.458395760156)) ;
#22489=CARTESIAN_POINT('Ctrl Pts',(-20.9155052003231,30.5398649438799,123.470044892547)) ;
#22490=CARTESIAN_POINT('Ctrl Pts',(-20.5883067682827,30.7297889348904,123.665646410074)) ;
#22491=CARTESIAN_POINT('Ctrl Pts',(-20.8830672767706,30.5497998545275,123.729108750999)) ;
#22492=CARTESIAN_POINT('Ctrl Pts',(-20.525923055177,30.7398300650696,123.867307187014)) ;
#22493=CARTESIAN_POINT('Ctrl Pts',(-20.8050869196827,30.5598409847068,123.981184304442)) ;
#22494=CARTESIAN_POINT('Ctrl Pts',(-20.4310732674177,30.7497172054396,124.052276123954)) ;
#22495=CARTESIAN_POINT('Ctrl Pts',(-20.6865234424483,30.5697281250767,124.212396007676)) ;
#22496=CARTESIAN_POINT('Ctrl Pts',(-20.3045079136013,30.7597094829755,124.219919068454)) ;
#22497=CARTESIAN_POINT('Ctrl Pts',(-20.5283158328247,30.5797204026127,124.421949250781)) ;
#22498=CARTESIAN_POINT('Ctrl Pts',(-20.1513705963158,30.7696580262439,124.36238740214)) ;
#22499=CARTESIAN_POINT('Ctrl Pts',(-20.336893127493,30.589668945881,124.600034325977)) ;
#22500=CARTESIAN_POINT('Ctrl Pts',(-19.97621673164,30.7795947010611,124.476202086606)) ;
#22501=CARTESIAN_POINT('Ctrl Pts',(-20.117949669728,30.5996056206982,124.742302120517)) ;
#22502=CARTESIAN_POINT('Ctrl Pts',(-19.7831216512904,30.7895781219974,124.558506793433)) ;
#22503=CARTESIAN_POINT('Ctrl Pts',(-19.8765801266705,30.6095890416346,124.845182022236)) ;
#22504=CARTESIAN_POINT('Ctrl Pts',(-19.577416346165,30.7996204371867,124.605973059919)) ;
#22505=CARTESIAN_POINT('Ctrl Pts',(-19.619448424608,30.6196313568238,124.904513792509)) ;
#22506=CARTESIAN_POINT('Ctrl Pts',(-19.3708401231471,30.8094607546259,124.617114838702)) ;
#22507=CARTESIAN_POINT('Ctrl Pts',(-19.3612267210301,30.629471674263,124.918439915204)) ;
#22508=CARTESIAN_POINT('Ctrl Pts',(-19.1614550331297,30.8194904586834,124.592230575313)) ;
#22509=CARTESIAN_POINT('Ctrl Pts',(-19.0994956244019,30.6395013783205,124.887333257162)) ;
#22510=CARTESIAN_POINT('Ctrl Pts',(-18.9599146448353,30.8295114154059,124.530878822072)) ;
#22511=CARTESIAN_POINT('Ctrl Pts',(-18.84757050077,30.649522335043,124.810642476183)) ;
#22512=CARTESIAN_POINT('Ctrl Pts',(-18.7747291699173,30.8393779577095,124.437402415365)) ;
#22513=CARTESIAN_POINT('Ctrl Pts',(-18.6160882477537,30.6593888773466,124.69379526334)) ;
#22514=CARTESIAN_POINT('Ctrl Pts',(-18.6051688450948,30.8494490576546,124.310638457262)) ;
#22515=CARTESIAN_POINT('Ctrl Pts',(-18.4041389450964,30.6694599772918,124.535339469786)) ;
#22516=CARTESIAN_POINT('Ctrl Pts',(-18.4634769424933,30.8592911318322,124.159844576277)) ;
#22517=CARTESIAN_POINT('Ctrl Pts',(-18.2270241518516,30.6793020514693,124.346845255088)) ;
#22518=CARTESIAN_POINT('Ctrl Pts',(-18.3481138935015,30.8692519264192,123.98508540905)) ;
#22519=CARTESIAN_POINT('Ctrl Pts',(-18.0828214570917,30.6892628460564,124.128395071014)) ;
#22520=CARTESIAN_POINT('Ctrl Pts',(-18.2645872120616,30.8792897993201,123.791299482673)) ;
#22521=CARTESIAN_POINT('Ctrl Pts',(-17.9784145006715,30.6993007189572,123.886162207482)) ;
#22522=CARTESIAN_POINT('Ctrl Pts',(-18.2163875155882,30.8891640848642,123.589358215528)) ;
#22523=CARTESIAN_POINT('Ctrl Pts',(-17.9181661940265,30.7091750045013,123.63373426702)) ;
#22524=CARTESIAN_POINT('Ctrl Pts',(-18.203753574643,30.8992338352781,123.378065938577)) ;
#22525=CARTESIAN_POINT('Ctrl Pts',(-17.9023753757216,30.7192447549152,123.369619175597)) ;
#22526=CARTESIAN_POINT('Ctrl Pts',(-18.2273236827773,30.9090671198127,123.172670784879)) ;
#22527=CARTESIAN_POINT('Ctrl Pts',(-17.9318397718058,30.7290780394499,123.112874144442)) ;
#22528=CARTESIAN_POINT('Ctrl Pts',(-18.2867987026179,30.9190974606128,122.970368878916)) ;
#22529=CARTESIAN_POINT('Ctrl Pts',(-18.0061852690051,30.7391083802499,122.859997359419)) ;
#22530=CARTESIAN_POINT('Ctrl Pts',(-18.3810728614528,30.9291293846124,122.781698599394)) ;
#22531=CARTESIAN_POINT('Ctrl Pts',(-18.1240293775023,30.7491403042495,122.624160309324)) ;
#22532=CARTESIAN_POINT('Ctrl Pts',(-18.50375518637,30.9389579195483,122.6154474201)) ;
#22533=CARTESIAN_POINT('Ctrl Pts',(-18.2773844645063,30.7589688391854,122.416346355351)) ;
#22534=CARTESIAN_POINT('Ctrl Pts',(-18.6555659033438,30.948951697313,122.470205569998)) ;
#22535=CARTESIAN_POINT('Ctrl Pts',(-18.4671493140597,30.7689626169501,122.234795344671)) ;
#22536=CARTESIAN_POINT('Ctrl Pts',(-18.8311197714127,30.9589794077985,122.353474256892)) ;
#22537=CARTESIAN_POINT('Ctrl Pts',(-18.6865926220814,30.7789903274356,122.088882738916)) ;
#22538=CARTESIAN_POINT('Ctrl Pts',(-19.021483587405,30.9688678186325,122.269936336135)) ;
#22539=CARTESIAN_POINT('Ctrl Pts',(-18.924548918543,30.7888787382696,121.984461740876)) ;
#22540=CARTESIAN_POINT('Ctrl Pts',(-19.2251633873121,30.978844669168,122.219928658385)) ;
#22541=CARTESIAN_POINT('Ctrl Pts',(-19.1791493957345,30.7988555888051,121.921954029357)) ;
#22542=CARTESIAN_POINT('Ctrl Pts',(-19.4347905985392,30.9888364657185,122.206004671817)) ;
#22543=CARTESIAN_POINT('Ctrl Pts',(-19.4411836962534,30.8088473853556,121.904551040875)) ;
#22544=CARTESIAN_POINT('Ctrl Pts',(-19.6445006365015,30.9988724718122,122.229041741586)) ;
#22545=CARTESIAN_POINT('Ctrl Pts',(-19.7033209422536,30.8188833914493,121.933349289194)) ;
#22546=CARTESIAN_POINT('Ctrl Pts',(-19.8434060708219,31.008723206075,122.286751984525)) ;
#22547=CARTESIAN_POINT('Ctrl Pts',(-19.9519531581678,30.8287341257121,122.005489324719)) ;
#22548=CARTESIAN_POINT('Ctrl Pts',(-20.0320403039582,31.0187144646032,122.379080702505)) ;
#22549=CARTESIAN_POINT('Ctrl Pts',(-20.1877451626918,30.8387253842403,122.12090221111)) ;
#22550=CARTESIAN_POINT('Ctrl Pts',(-20.2006501988176,31.0286323595064,122.501784715894)) ;
#22551=CARTESIAN_POINT('Ctrl Pts',(-20.3985067246429,30.8486432791435,122.274284311981)) ;
#22552=CARTESIAN_POINT('Ctrl Pts',(-20.3470107237814,31.0386605011694,122.65350091565)) ;
#22553=CARTESIAN_POINT('Ctrl Pts',(-20.5814557895788,30.8586714208065,122.463931047394)) ;
#22554=CARTESIAN_POINT('Ctrl Pts',(-20.4632104004851,31.0485456692853,122.825802329779)) ;
#22555=CARTESIAN_POINT('Ctrl Pts',(-20.726703975958,30.8685565889224,122.679309656422)) ;
#22556=CARTESIAN_POINT('Ctrl Pts',(-20.5490845959354,31.0585350327913,123.017454794976)) ;
#22557=CARTESIAN_POINT('Ctrl Pts',(-20.8340446604117,30.8785459524284,122.918876333056)) ;
#22558=CARTESIAN_POINT('Ctrl Pts',(-20.6002096975552,31.0685761678013,123.22226668955)) ;
#22559=CARTESIAN_POINT('Ctrl Pts',(-20.8979488651774,30.8885870874385,123.174891648262)) ;
#22560=CARTESIAN_POINT('Ctrl Pts',(-20.615028805326,31.0784088359894,123.42844428818)) ;
#22561=CARTESIAN_POINT('Ctrl Pts',(-20.916470523059,30.8984197556265,123.432614768819)) ;
#22562=CARTESIAN_POINT('Ctrl Pts',(-20.5940744638475,31.0884027389439,123.637499008543)) ;
#22563=CARTESIAN_POINT('Ctrl Pts',(-20.8902751541959,30.908413658581,123.693933046635)) ;
#22564=CARTESIAN_POINT('Ctrl Pts',(-20.5365069814263,31.0984320240284,123.840336990073)) ;
#22565=CARTESIAN_POINT('Ctrl Pts',(-20.8183135578191,30.9184429436655,123.947479863912)) ;
#22566=CARTESIAN_POINT('Ctrl Pts',(-20.446304755453,31.1083075524703,124.027344707869)) ;
#22567=CARTESIAN_POINT('Ctrl Pts',(-20.705558307434,30.9283184721074,124.181239071671)) ;
#22568=CARTESIAN_POINT('Ctrl Pts',(-20.3236808566818,31.1183078350863,124.198085320137)) ;
#22569=CARTESIAN_POINT('Ctrl Pts',(-20.55227636311,30.9383187547235,124.394663488926)) ;
#22570=CARTESIAN_POINT('Ctrl Pts',(-20.1746825112907,31.1282198511434,124.343800205569)) ;
#22571=CARTESIAN_POINT('Ctrl Pts',(-20.3660263502005,30.9482307707805,124.576805636963)) ;
#22572=CARTESIAN_POINT('Ctrl Pts',(-20.0004530429304,31.1382619264824,124.46299621068)) ;
#22573=CARTESIAN_POINT('Ctrl Pts',(-20.148238159027,30.9582728461195,124.725798531691)) ;
#22574=CARTESIAN_POINT('Ctrl Pts',(-19.8108716546696,31.1481617591385,124.548900830841)) ;
#22575=CARTESIAN_POINT('Ctrl Pts',(-19.9112599341149,30.9681726787756,124.833177229003)) ;
#22576=CARTESIAN_POINT('Ctrl Pts',(-19.6074951368638,31.1581541597165,124.601515467069)) ;
#22577=CARTESIAN_POINT('Ctrl Pts',(-19.6570385216495,30.9781650793536,124.898943043692)) ;
#22578=CARTESIAN_POINT('Ctrl Pts',(-19.3971675954827,31.1681881814759,124.617712800031)) ;
#22579=CARTESIAN_POINT('Ctrl Pts',(-19.3941289164041,30.988199101113,124.91918719167)) ;
#22580=CARTESIAN_POINT('Ctrl Pts',(-19.1907487982186,31.1780527923171,124.59775750716)) ;
#22581=CARTESIAN_POINT('Ctrl Pts',(-19.1361050769742,30.9980637119542,124.894240456014)) ;
#22582=CARTESIAN_POINT('Ctrl Pts',(-18.9881977091377,31.1880451917782,124.542038359077)) ;
#22583=CARTESIAN_POINT('Ctrl Pts',(-18.8829168166101,31.0080561114154,124.824588928341)) ;
#22584=CARTESIAN_POINT('Ctrl Pts',(-18.7978278631162,31.1980771451111,124.451266994197)) ;
#22585=CARTESIAN_POINT('Ctrl Pts',(-18.6449556256928,31.0180880647483,124.711122383822)) ;
#22586=CARTESIAN_POINT('Ctrl Pts',(-18.6287533564004,31.2079435040528,124.331095273272)) ;
#22587=CARTESIAN_POINT('Ctrl Pts',(-18.433613598993,31.0279544236899,124.56090527812)) ;
#22588=CARTESIAN_POINT('Ctrl Pts',(-18.4811055178957,31.2179309795386,124.181843664757)) ;
#22589=CARTESIAN_POINT('Ctrl Pts',(-18.2490556295149,31.0379418991757,124.374338785496)) ;
#22590=CARTESIAN_POINT('Ctrl Pts',(-18.3620004505735,31.2278758857271,124.009975732587)) ;
#22591=CARTESIAN_POINT('Ctrl Pts',(-18.1001763827017,31.0478868053642,124.159502137119)) ;
#22592=CARTESIAN_POINT('Ctrl Pts',(-18.2737974644408,31.2379208503873,123.81812345337)) ;
#22593=CARTESIAN_POINT('Ctrl Pts',(-17.9899251037199,31.0579317700244,123.919685682728)) ;
#22594=CARTESIAN_POINT('Ctrl Pts',(-18.2210312867946,31.2477826572922,123.617606509006)) ;
#22595=CARTESIAN_POINT('Ctrl Pts',(-17.9239698947395,31.0677935769293,123.669038395262)) ;
#22596=CARTESIAN_POINT('Ctrl Pts',(-18.2032568478729,31.2577753295979,123.408304026805)) ;
#22597=CARTESIAN_POINT('Ctrl Pts',(-17.9017545884407,31.0777862492351,123.407409964502)) ;
#22598=CARTESIAN_POINT('Ctrl Pts',(-18.222001276921,31.2677040005433,123.200401767921)) ;
#22599=CARTESIAN_POINT('Ctrl Pts',(-17.9251878868137,31.0877149201804,123.147532162219)) ;
#22600=CARTESIAN_POINT('Ctrl Pts',(-18.2763524420486,31.2776565427686,122.998365459932)) ;
#22601=CARTESIAN_POINT('Ctrl Pts',(-17.9931295756622,31.0976674624057,122.894987346514)) ;
#22602=CARTESIAN_POINT('Ctrl Pts',(-18.3653072061262,31.2876578987645,122.807825356539)) ;
#22603=CARTESIAN_POINT('Ctrl Pts',(-18.1043255909368,31.1076688184016,122.656813330348)) ;
#22604=CARTESIAN_POINT('Ctrl Pts',(-18.4865417491966,31.2976865110392,122.635347065935)) ;
#22605=CARTESIAN_POINT('Ctrl Pts',(-18.2558710625769,31.1176974306763,122.441217023634)) ;
#22606=CARTESIAN_POINT('Ctrl Pts',(-18.6332380965549,31.3075508455887,122.488744885021)) ;
#22607=CARTESIAN_POINT('Ctrl Pts',(-18.4392436560099,31.1275617652258,122.257966085798)) ;
#22608=CARTESIAN_POINT('Ctrl Pts',(-18.8051439882642,31.3175431696653,122.36805505233)) ;
#22609=CARTESIAN_POINT('Ctrl Pts',(-18.6541277020736,31.1375540893024,122.107106052772)) ;
#22610=CARTESIAN_POINT('Ctrl Pts',(-18.9941591698767,31.3274706620311,122.279486435379)) ;
#22611=CARTESIAN_POINT('Ctrl Pts',(-18.8903979931826,31.1474815816683,121.99639777191)) ;
#22612=CARTESIAN_POINT('Ctrl Pts',(-19.1976565576999,31.337498020582,122.224557944539)) ;
#22613=CARTESIAN_POINT('Ctrl Pts',(-19.1447705223875,31.1575089402191,121.927739862365)) ;
#22614=CARTESIAN_POINT('Ctrl Pts',(-19.4046860684407,31.3473844386331,122.205835676361)) ;
#22615=CARTESIAN_POINT('Ctrl Pts',(-19.403557785468,31.1673953582702,121.904339822956)) ;
#22616=CARTESIAN_POINT('Ctrl Pts',(-19.6148093834641,31.3574161733685,122.223490530873)) ;
#22617=CARTESIAN_POINT('Ctrl Pts',(-19.6662117593913,31.1774270930056,121.926411212978)) ;
#22618=CARTESIAN_POINT('Ctrl Pts',(-19.8157458443054,31.3672977546117,122.27637611023)) ;
#22619=CARTESIAN_POINT('Ctrl Pts',(-19.9173816828502,31.1873086742489,121.992520931665)) ;
#22620=CARTESIAN_POINT('Ctrl Pts',(-20.0078493459752,31.3773597326441,122.364859285606)) ;
#22621=CARTESIAN_POINT('Ctrl Pts',(-20.1575099536661,31.1973706522812,122.103127502672)) ;
#22622=CARTESIAN_POINT('Ctrl Pts',(-20.1782249889718,31.3872168110058,122.482873113296)) ;
#22623=CARTESIAN_POINT('Ctrl Pts',(-20.3704779128565,31.2072277306429,122.250647114545)) ;
#22624=CARTESIAN_POINT('Ctrl Pts',(-20.3278279199944,31.3972113841118,122.630365681166)) ;
#22625=CARTESIAN_POINT('Ctrl Pts',(-20.557479635411,31.2172223037489,122.435014859895)) ;
#22626=CARTESIAN_POINT('Ctrl Pts',(-20.4488094488748,31.4071371803994,122.800422727047)) ;
#22627=CARTESIAN_POINT('Ctrl Pts',(-20.7087042530508,31.2271481000365,122.647587798087)) ;
#22628=CARTESIAN_POINT('Ctrl Pts',(-20.5393550256187,31.4171625475691,122.990728200173)) ;
#22629=CARTESIAN_POINT('Ctrl Pts',(-20.8218837391766,31.2371734672062,122.885470873075)) ;
#22630=CARTESIAN_POINT('Ctrl Pts',(-20.5948502492867,31.427058627223,123.191245455736)) ;
#22631=CARTESIAN_POINT('Ctrl Pts',(-20.8912500206041,31.2470695468601,123.136118325641)) ;
#22632=CARTESIAN_POINT('Ctrl Pts',(-20.6153065851422,31.4370537069285,123.400378513475)) ;
#22633=CARTESIAN_POINT('Ctrl Pts',(-20.916817797818,31.2570646265657,123.397534145115)) ;
#22634=CARTESIAN_POINT('Ctrl Pts',(-20.5987327650594,31.4470787947444,123.610482201889)) ;
#22635=CARTESIAN_POINT('Ctrl Pts',(-20.8960973227342,31.2670897143815,123.660166672547)) ;
#22636=CARTESIAN_POINT('Ctrl Pts',(-20.5297708945593,31.4602626171116,123.878943016611)) ;
#22637=CARTESIAN_POINT('Ctrl Pts',(-20.809893476644,31.2802735367488,123.995726533553)) ;
#22638=CARTESIAN_POINT('Ctrl Pts',(-20.3913865952829,31.4735847352576,124.126114166337)) ;
#22639=CARTESIAN_POINT('Ctrl Pts',(-20.6369390480152,31.2935956548947,124.30466223955)) ;
#22640=CARTESIAN_POINT('Ctrl Pts',(-20.1945187909929,31.4869639448852,124.327003652239)) ;
#22641=CARTESIAN_POINT('Ctrl Pts',(-20.3908148582284,31.3069748645223,124.555818133117)) ;
#22642=CARTESIAN_POINT('Ctrl Pts',(-20.0266170027822,31.4968021821294,124.447815006563)) ;
#22643=CARTESIAN_POINT('Ctrl Pts',(-20.1809438414753,31.3168131017665,124.706820601801)) ;
#22644=CARTESIAN_POINT('Ctrl Pts',(-19.8359227028424,31.5068751053881,124.539840727089)) ;
#22645=CARTESIAN_POINT('Ctrl Pts',(-19.9425721439745,31.3268860250252,124.821852782534)) ;
#22646=CARTESIAN_POINT('Ctrl Pts',(-19.6364695609574,31.5167317468432,124.596111822066)) ;
#22647=CARTESIAN_POINT('Ctrl Pts',(-19.6932575438715,31.3367426664803,124.89218888602)) ;
#22648=CARTESIAN_POINT('Ctrl Pts',(-19.4276732492853,31.5267171223493,124.617725780505)) ;
#22649=CARTESIAN_POINT('Ctrl Pts',(-19.4322556852193,31.3467280419864,124.919201640466)) ;
#22650=CARTESIAN_POINT('Ctrl Pts',(-19.1491517758467,31.5400011538097,124.597557778909)) ;
#22651=CARTESIAN_POINT('Ctrl Pts',(-19.0841345592013,31.3600120734468,124.893999424143)) ;
#22652=CARTESIAN_POINT('Ctrl Pts',(-18.8168268265356,31.55651994568,124.4835998274)) ;
#22653=CARTESIAN_POINT('Ctrl Pts',(-18.6686831095259,31.3765308653172,124.751522351196)) ;
#22654=CARTESIAN_POINT('Ctrl Pts',(-18.5395236647983,31.5733056626867,124.258964597931)) ;
#22655=CARTESIAN_POINT('Ctrl Pts',(-18.3221176258635,31.3933165823238,124.470780414967)) ;
#22656=CARTESIAN_POINT('Ctrl Pts',(-18.3774782260285,31.5864188111957,124.035919217362)) ;
#22657=CARTESIAN_POINT('Ctrl Pts',(-18.1195171640873,31.4064297308328,124.19192546978)) ;
#22658=CARTESIAN_POINT('Ctrl Pts',(-18.2842368170373,31.5964543602758,123.846684019974)) ;
#22659=CARTESIAN_POINT('Ctrl Pts',(-18.0029767278721,31.416465279913,123.955390640417)) ;
#22660=CARTESIAN_POINT('Ctrl Pts',(-18.2259601248409,31.6064704164553,123.644318949324)) ;
#22661=CARTESIAN_POINT('Ctrl Pts',(-17.930131161295,31.4264813360924,123.702427282653)) ;
#22662=CARTESIAN_POINT('Ctrl Pts',(-18.1960923933868,31.6196484523213,123.368912551157)) ;
#22663=CARTESIAN_POINT('Ctrl Pts',(-17.8927981854828,31.4396593719584,123.358188928687)) ;
#22664=CARTESIAN_POINT('Ctrl Pts',(-18.2490034102453,31.6362503295084,123.019854463279)) ;
#22665=CARTESIAN_POINT('Ctrl Pts',(-17.9589427761027,31.4562612491455,122.921846253614)) ;
#22666=CARTESIAN_POINT('Ctrl Pts',(-18.4541225555357,31.6563134741243,122.64582032832)) ;
#22667=CARTESIAN_POINT('Ctrl Pts',(-18.2153452936868,31.4763243937614,122.454312103361)) ;
#22668=CARTESIAN_POINT('Ctrl Pts',(-18.7702542503997,31.676114364208,122.367683074125)) ;
#22669=CARTESIAN_POINT('Ctrl Pts',(-18.6105119795525,31.4961252838451,122.106643007625)) ;
#22670=CARTESIAN_POINT('Ctrl Pts',(-19.1646379113021,31.6960574894867,122.212071616699)) ;
#22671=CARTESIAN_POINT('Ctrl Pts',(-19.1034924936999,31.5160684091238,121.912133008607)) ;
#22672=CARTESIAN_POINT('Ctrl Pts',(-19.5875617432602,31.7159555346063,122.200691268626)) ;
#22673=CARTESIAN_POINT('Ctrl Pts',(-19.6321465341764,31.5359664542434,121.89791137193)) ;
#22674=CARTESIAN_POINT('Ctrl Pts',(-19.9891315337937,31.735841294233,122.333252820407)) ;
#22675=CARTESIAN_POINT('Ctrl Pts',(-20.1341066883384,31.5558522138702,122.063616102464)) ;
#22676=CARTESIAN_POINT('Ctrl Pts',(-20.3238700828937,31.7559064694129,122.597717645849)) ;
#22677=CARTESIAN_POINT('Ctrl Pts',(-20.5525283110554,31.57591738905,122.394200252169)) ;
#22678=CARTESIAN_POINT('Ctrl Pts',(-20.5455304831707,31.7757331125157,122.956392108189)) ;
#22679=CARTESIAN_POINT('Ctrl Pts',(-20.8296000415882,31.5957440321528,122.84254361497)) ;
#22680=CARTESIAN_POINT('Ctrl Pts',(-20.6329476537698,31.7956418219641,123.370466525032)) ;
#22681=CARTESIAN_POINT('Ctrl Pts',(-20.9388687495492,31.6156527416012,123.360136077141)) ;
#22682=CARTESIAN_POINT('Ctrl Pts',(-20.5737577153688,31.8155936589959,123.790666742913)) ;
#22683=CARTESIAN_POINT('Ctrl Pts',(-20.8648791195812,31.635604578633,123.885385533411)) ;
#22684=CARTESIAN_POINT('Ctrl Pts',(-20.3736372597136,31.835602133699,124.166043131573)) ;
#22685=CARTESIAN_POINT('Ctrl Pts',(-20.6147262487971,31.6556130533361,124.354604940983)) ;
#22686=CARTESIAN_POINT('Ctrl Pts',(-20.0609970576513,31.8554035924605,124.448061776785)) ;
#22687=CARTESIAN_POINT('Ctrl Pts',(-20.2239265792252,31.6754145120976,124.70712499995)) ;
#22688=CARTESIAN_POINT('Ctrl Pts',(-19.6682512234286,31.8753604806964,124.608723454266)) ;
#22689=CARTESIAN_POINT('Ctrl Pts',(-19.7329944592127,31.6953714003336,124.907950846951)) ;
#22690=CARTESIAN_POINT('Ctrl Pts',(-19.2436603324159,31.8953443181105,124.624778169694)) ;
#22691=CARTESIAN_POINT('Ctrl Pts',(-19.2022559885623,31.7153552377477,124.928017723692)) ;
#22692=CARTESIAN_POINT('Ctrl Pts',(-18.8422996219988,31.9151527573315,124.496909348728)) ;
#22693=CARTESIAN_POINT('Ctrl Pts',(-18.7005580952729,31.7351636769686,124.768181953029)) ;
#22694=CARTESIAN_POINT('Ctrl Pts',(-18.5055590914568,31.9351384667117,124.237910045326)) ;
#22695=CARTESIAN_POINT('Ctrl Pts',(-18.2796327533169,31.7551493863488,124.444432947283)) ;
#22696=CARTESIAN_POINT('Ctrl Pts',(-18.2784623208037,31.955007989727,123.881451590909)) ;
#22697=CARTESIAN_POINT('Ctrl Pts',(-17.9957625956122,31.7750189093641,123.998861683797)) ;
#22698=CARTESIAN_POINT('Ctrl Pts',(-18.1861815675504,31.9750287288442,123.466043557042)) ;
#22699=CARTESIAN_POINT('Ctrl Pts',(-17.8804111930879,31.7950396484813,123.479601508631)) ;
#22700=CARTESIAN_POINT('Ctrl Pts',(-18.2401047055373,31.9948327938211,123.04826047757)) ;
#22701=CARTESIAN_POINT('Ctrl Pts',(-17.947813732566,31.8148437134583,122.957375358431)) ;
#22702=CARTESIAN_POINT('Ctrl Pts',(-18.4356159524676,32.0148947575519,122.669266623573)) ;
#22703=CARTESIAN_POINT('Ctrl Pts',(-18.1922019497661,31.834905677189,122.483631625261)) ;
#22704=CARTESIAN_POINT('Ctrl Pts',(-18.7455928392011,32.0347279378404,122.383198650126)) ;
#22705=CARTESIAN_POINT('Ctrl Pts',(-18.579670503548,31.8547388574775,122.126047237428)) ;
#22706=CARTESIAN_POINT('Ctrl Pts',(-19.1356511664417,32.0546471351664,122.218343920433)) ;
#22707=CARTESIAN_POINT('Ctrl Pts',(-19.0672415407129,31.8746580548036,121.919977102834)) ;
#22708=CARTESIAN_POINT('Ctrl Pts',(-19.5590376558123,32.0745851602798,122.196738769831)) ;
#22709=CARTESIAN_POINT('Ctrl Pts',(-19.596473798273,31.8945960799169,121.892968380712)) ;
#22710=CARTESIAN_POINT('Ctrl Pts',(-19.9633771695477,32.0944632063358,122.319975235754)) ;
#22711=CARTESIAN_POINT('Ctrl Pts',(-20.1018977424829,31.914474125973,122.047010861552)) ;
#22712=CARTESIAN_POINT('Ctrl Pts',(-20.3031500801308,32.1144479406239,122.575069386705)) ;
#22713=CARTESIAN_POINT('Ctrl Pts',(-20.5266155989396,31.934458860261,122.365876034326)) ;
#22714=CARTESIAN_POINT('Ctrl Pts',(-20.5347790537855,32.1343587573024,122.929588130013)) ;
#22715=CARTESIAN_POINT('Ctrl Pts',(-20.8161540516341,31.9543696769395,122.809022005469)) ;
#22716=CARTESIAN_POINT('Ctrl Pts',(-20.6316344190319,32.1543577328211,123.343539091195)) ;
#22717=CARTESIAN_POINT('Ctrl Pts',(-20.9372264313366,31.9743686524582,123.326459903439)) ;
#22718=CARTESIAN_POINT('Ctrl Pts',(-20.5824108030896,32.1741626534663,123.761844882659)) ;
#22719=CARTESIAN_POINT('Ctrl Pts',(-20.8757007542274,31.9941735731034,123.849340834267)) ;
#22720=CARTESIAN_POINT('Ctrl Pts',(-20.3923321685515,32.1941466137575,124.141760103579)) ;
#22721=CARTESIAN_POINT('Ctrl Pts',(-20.6381061492539,32.0141575333947,124.324236585198)) ;
#22722=CARTESIAN_POINT('Ctrl Pts',(-20.0852664590449,32.2140328174815,124.432569654713)) ;
#22723=CARTESIAN_POINT('Ctrl Pts',(-20.254277484515,32.0340437371186,124.687750970673)) ;
#22724=CARTESIAN_POINT('Ctrl Pts',(-19.6964684402798,32.2339819958047,124.602063783456)) ;
#22725=CARTESIAN_POINT('Ctrl Pts',(-19.7682819396191,32.0539929154418,124.89962239012)) ;
#22726=CARTESIAN_POINT('Ctrl Pts',(-19.2741435561821,32.2538837950442,124.628548088097)) ;
#22727=CARTESIAN_POINT('Ctrl Pts',(-19.2403770539516,32.0738947146813,124.932732853793)) ;
#22728=CARTESIAN_POINT('Ctrl Pts',(-18.8683229480946,32.2737624000966,124.51031319366)) ;
#22729=CARTESIAN_POINT('Ctrl Pts',(-18.7330993587673,32.0937733197337,124.784941725984)) ;
#22730=CARTESIAN_POINT('Ctrl Pts',(-18.5246822894204,32.2937947598223,124.258593479938)) ;
#22731=CARTESIAN_POINT('Ctrl Pts',(-18.3035498467669,32.1138056794594,124.470304693559)) ;
#22732=CARTESIAN_POINT('Ctrl Pts',(-18.3288903417923,32.3103764857783,123.965395680415)) ;
#22733=CARTESIAN_POINT('Ctrl Pts',(-18.0587930611329,32.1303874054155,124.103782576889)) ;
#22734=CARTESIAN_POINT('Ctrl Pts',(-18.2389994739994,32.3235706560763,123.702969811419)) ;
#22735=CARTESIAN_POINT('Ctrl Pts',(-17.9464384610694,32.1435815757134,123.775785395635)) ;
#22736=CARTESIAN_POINT('Ctrl Pts',(-18.1952099825185,32.3368828341695,123.426608876342)) ;
#22737=CARTESIAN_POINT('Ctrl Pts',(-17.8916962164165,32.1568937538066,123.430264324837)) ;
#22738=CARTESIAN_POINT('Ctrl Pts',(-18.2318513898389,32.3534490137628,123.076189005305)) ;
#22739=CARTESIAN_POINT('Ctrl Pts',(-17.9374894753685,32.1734599333999,122.99232521224)) ;
#22740=CARTESIAN_POINT('Ctrl Pts',(-18.3860665926035,32.370077208623,122.758138167499)) ;
#22741=CARTESIAN_POINT('Ctrl Pts',(-18.1302718088824,32.1900881282601,122.594703559392)) ;
#22742=CARTESIAN_POINT('Ctrl Pts',(-18.5689151454784,32.3833657903327,122.546824011485)) ;
#22743=CARTESIAN_POINT('Ctrl Pts',(-18.3588141057148,32.2033767099699,122.330591540781)) ;
#22744=CARTESIAN_POINT('Ctrl Pts',(-18.7313456924468,32.3933340384363,122.414447869079)) ;
#22745=CARTESIAN_POINT('Ctrl Pts',(-18.5618539277949,32.2133449580735,122.165112713871)) ;
#22746=CARTESIAN_POINT('Ctrl Pts',(-18.9132084253142,32.4032487946925,122.312590576436)) ;
#22747=CARTESIAN_POINT('Ctrl Pts',(-18.7891790717996,32.2232597143296,122.037790376024)) ;
#22748=CARTESIAN_POINT('Ctrl Pts',(-19.1118736333332,32.4132619453437,122.242954847394)) ;
#22749=CARTESIAN_POINT('Ctrl Pts',(-19.037513591275,32.2332728649808,121.95074327932)) ;
#22750=CARTESIAN_POINT('Ctrl Pts',(-19.3196522724763,32.4232746525457,122.209207410282)) ;
#22751=CARTESIAN_POINT('Ctrl Pts',(-19.2972230251791,32.2432855721828,121.908553873528)) ;
#22752=CARTESIAN_POINT('Ctrl Pts',(-19.5975327146755,32.436493941237,122.212420867369)) ;
#22753=CARTESIAN_POINT('Ctrl Pts',(-19.6446403660395,32.2565048608741,121.9125795524)) ;
#22754=CARTESIAN_POINT('Ctrl Pts',(-19.9378232247677,32.453112622235,122.307507172536)) ;
#22755=CARTESIAN_POINT('Ctrl Pts',(-20.0699198327109,32.2731235418722,122.031411460383)) ;
#22756=CARTESIAN_POINT('Ctrl Pts',(-20.2246076543759,32.4696775300085,122.512015826499)) ;
#22757=CARTESIAN_POINT('Ctrl Pts',(-20.4284615240151,32.2896884496456,122.28707638829)) ;
#22758=CARTESIAN_POINT('Ctrl Pts',(-20.4036500534061,32.4830760016193,122.729503286316)) ;
#22759=CARTESIAN_POINT('Ctrl Pts',(-20.6522321703216,32.3030869212564,122.55890721292)) ;
#22760=CARTESIAN_POINT('Ctrl Pts',(-20.5055910328036,32.4929172571063,122.909552354167)) ;
#22761=CARTESIAN_POINT('Ctrl Pts',(-20.7796679108865,32.3129281767434,122.783972393412)) ;
#22762=CARTESIAN_POINT('Ctrl Pts',(-20.5761633681093,32.5029035726945,123.10724493237)) ;
#22763=CARTESIAN_POINT('Ctrl Pts',(-20.8678841148157,32.3229144923316,123.031085830974)) ;
#22764=CARTESIAN_POINT('Ctrl Pts',(-20.6112720105989,32.5128401802809,123.313207381497)) ;
#22765=CARTESIAN_POINT('Ctrl Pts',(-20.9117732133019,32.332851099918,123.288538866815)) ;
#22766=CARTESIAN_POINT('Ctrl Pts',(-20.6099679457665,32.5228900476492,123.524461765722)) ;
#22767=CARTESIAN_POINT('Ctrl Pts',(-20.910145815352,32.3429009672863,123.552606824038)) ;
#22768=CARTESIAN_POINT('Ctrl Pts',(-20.5729021146074,32.532740542324,123.728221890654)) ;
#22769=CARTESIAN_POINT('Ctrl Pts',(-20.8638163142715,32.3527514619611,123.807307622436)) ;
#22770=CARTESIAN_POINT('Ctrl Pts',(-20.5006629810764,32.5427123427185,123.924992058864)) ;
#22771=CARTESIAN_POINT('Ctrl Pts',(-20.773519983493,32.3627232623556,124.053271401024)) ;
#22772=CARTESIAN_POINT('Ctrl Pts',(-20.3950484487511,32.5527083097443,124.106711975887)) ;
#22773=CARTESIAN_POINT('Ctrl Pts',(-20.6415042015941,32.3727192293814,124.280422776241)) ;
#22774=CARTESIAN_POINT('Ctrl Pts',(-20.2587392018978,32.5627457691255,124.267771847846)) ;
#22775=CARTESIAN_POINT('Ctrl Pts',(-20.4711197706811,32.3827566887626,124.481749462152)) ;
#22776=CARTESIAN_POINT('Ctrl Pts',(-20.0999386935785,32.5725864700262,124.400395451585)) ;
#22777=CARTESIAN_POINT('Ctrl Pts',(-20.2726207381904,32.3925973896634,124.6475312724)) ;
#22778=CARTESIAN_POINT('Ctrl Pts',(-19.9169195431235,32.5826344912936,124.505860717618)) ;
#22779=CARTESIAN_POINT('Ctrl Pts',(-20.0438481628859,32.4026454109307,124.779365277945)) ;
#22780=CARTESIAN_POINT('Ctrl Pts',(-19.7202317170747,32.5925818843763,124.576913026863)) ;
#22781=CARTESIAN_POINT('Ctrl Pts',(-19.7979892008617,32.4125928040134,124.868183348147)) ;
#22782=CARTESIAN_POINT('Ctrl Pts',(-19.5150675447947,32.6024920304227,124.613229581171)) ;
#22783=CARTESIAN_POINT('Ctrl Pts',(-19.5415342218403,32.4225029500598,124.913581797367)) ;
#22784=CARTESIAN_POINT('Ctrl Pts',(-19.3036192781191,32.6125509442723,124.613134139564)) ;
#22785=CARTESIAN_POINT('Ctrl Pts',(-19.277223918375,32.4325618639094,124.913465271175)) ;
#22786=CARTESIAN_POINT('Ctrl Pts',(-19.0998162930448,32.6223917145616,124.5774017769)) ;
#22787=CARTESIAN_POINT('Ctrl Pts',(-19.022469311543,32.4424026341987,124.868802452506)) ;
#22788=CARTESIAN_POINT('Ctrl Pts',(-18.9008906926549,32.6324545841402,124.505484176666)) ;
#22789=CARTESIAN_POINT('Ctrl Pts',(-18.7738114256327,32.4524655037773,124.778908029314)) ;
#22790=CARTESIAN_POINT('Ctrl Pts',(-18.7205888208704,32.6423489072707,124.401712674565)) ;
#22791=CARTESIAN_POINT('Ctrl Pts',(-18.5484324346786,32.4623598269078,124.649195864268)) ;
#22792=CARTESIAN_POINT('Ctrl Pts',(-18.5599523550071,32.6522907143652,124.268035857057)) ;
#22793=CARTESIAN_POINT('Ctrl Pts',(-18.3476349380033,32.4723016340023,124.482101731582)) ;
#22794=CARTESIAN_POINT('Ctrl Pts',(-18.4240467284614,32.6622932253205,124.107533030312)) ;
#22795=CARTESIAN_POINT('Ctrl Pts',(-18.1777508202333,32.4823041449576,124.281474853431)) ;
#22796=CARTESIAN_POINT('Ctrl Pts',(-18.3180393506076,32.6723279461389,123.925154810979)) ;
#22797=CARTESIAN_POINT('Ctrl Pts',(-18.0452392633268,32.492338865776,124.053503454134)) ;
#22798=CARTESIAN_POINT('Ctrl Pts',(-18.2463535071879,32.6821731236446,123.730976061633)) ;
#22799=CARTESIAN_POINT('Ctrl Pts',(-17.9556292696089,32.5021840432817,123.810780412352)) ;
#22800=CARTESIAN_POINT('Ctrl Pts',(-18.2085503842841,32.6921578840457,123.524527153024)) ;
#22801=CARTESIAN_POINT('Ctrl Pts',(-17.9083727783839,32.5121688036828,123.552719582534)) ;
#22802=CARTESIAN_POINT('Ctrl Pts',(-18.2070734509099,32.7020967903621,123.315553842166)) ;
#22803=CARTESIAN_POINT('Ctrl Pts',(-17.9065240318847,32.5221077099992,123.291502653985)) ;
#22804=CARTESIAN_POINT('Ctrl Pts',(-18.2423288903742,32.7121390179978,123.107420822376)) ;
#22805=CARTESIAN_POINT('Ctrl Pts',(-17.9505907657664,32.5321499376349,123.031335993592)) ;
#22806=CARTESIAN_POINT('Ctrl Pts',(-18.3119535046348,32.7220242295822,122.91158798625)) ;
#22807=CARTESIAN_POINT('Ctrl Pts',(-18.0376192936705,32.5420351492193,122.786543593569)) ;
#22808=CARTESIAN_POINT('Ctrl Pts',(-18.4154411859655,32.7320231597841,122.728653020651)) ;
#22809=CARTESIAN_POINT('Ctrl Pts',(-18.1669767556182,32.5520340794212,122.557873550048)) ;
#22810=CARTESIAN_POINT('Ctrl Pts',(-18.5479494903237,32.7419405826945,122.567636304584)) ;
#22811=CARTESIAN_POINT('Ctrl Pts',(-18.3326104946629,32.5619515023317,122.356600741746)) ;
#22812=CARTESIAN_POINT('Ctrl Pts',(-18.7084645463627,32.7519885147733,122.430363552934)) ;
#22813=CARTESIAN_POINT('Ctrl Pts',(-18.5332526173871,32.5719994344104,122.185007966984)) ;
#22814=CARTESIAN_POINT('Ctrl Pts',(-18.8872415852668,32.7618658905827,122.324659315536)) ;
#22815=CARTESIAN_POINT('Ctrl Pts',(-18.7567232187338,32.5818768102198,122.052875232647)) ;
#22816=CARTESIAN_POINT('Ctrl Pts',(-19.0850258483024,32.7719197837506,122.25022120339)) ;
#22817=CARTESIAN_POINT('Ctrl Pts',(-19.0039525695959,32.5919307033877,121.95982536141)) ;
#22818=CARTESIAN_POINT('Ctrl Pts',(-19.2894783129814,32.7818134070039,122.211767437767)) ;
#22819=CARTESIAN_POINT('Ctrl Pts',(-19.2595182815849,32.601824326641,121.911755678648)) ;
#22820=CARTESIAN_POINT('Ctrl Pts',(-19.5009779859704,32.7918760006269,122.209324968633)) ;
#22821=CARTESIAN_POINT('Ctrl Pts',(-19.5238926627054,32.611886920264,121.908700188409)) ;
#22822=CARTESIAN_POINT('Ctrl Pts',(-19.7051996408792,32.8017185746159,122.242795102334)) ;
#22823=CARTESIAN_POINT('Ctrl Pts',(-19.7791709674073,32.6217294942531,121.950535647314)) ;
#22824=CARTESIAN_POINT('Ctrl Pts',(-19.9035645751163,32.8117093314989,122.311756543246)) ;
#22825=CARTESIAN_POINT('Ctrl Pts',(-20.0271280441419,32.631720251136,122.036735366636)) ;
#22826=CARTESIAN_POINT('Ctrl Pts',(-20.0858058022882,32.8216373932568,122.41352070292)) ;
#22827=CARTESIAN_POINT('Ctrl Pts',(-20.2549311093635,32.6416483128939,122.163938821337)) ;
#22828=CARTESIAN_POINT('Ctrl Pts',(-20.2488151784822,32.831625369146,122.545893277075)) ;
#22829=CARTESIAN_POINT('Ctrl Pts',(-20.4586943445291,32.6516362887831,122.329402962598)) ;
#22830=CARTESIAN_POINT('Ctrl Pts',(-20.3867446811956,32.8416610335024,122.705536508051)) ;
#22831=CARTESIAN_POINT('Ctrl Pts',(-20.6311078851739,32.6616719531395,122.528955452347)) ;
#22832=CARTESIAN_POINT('Ctrl Pts',(-20.4932113035389,32.8515169719221,122.883306696087)) ;
#22833=CARTESIAN_POINT('Ctrl Pts',(-20.76419350534,32.6715278915592,122.751167847475)) ;
#22834=CARTESIAN_POINT('Ctrl Pts',(-20.5685516723176,32.861512463319,123.079449372689)) ;
#22835=CARTESIAN_POINT('Ctrl Pts',(-20.8583709770248,32.6815233829561,122.99634558384)) ;
#22836=CARTESIAN_POINT('Ctrl Pts',(-20.6084146945894,32.8714222682724,123.283945522481)) ;
#22837=CARTESIAN_POINT('Ctrl Pts',(-20.9082019158921,32.6914331879096,123.251966021349)) ;
#22838=CARTESIAN_POINT('Ctrl Pts',(-20.6125455527865,32.8814344905392,123.494398317047)) ;
#22839=CARTESIAN_POINT('Ctrl Pts',(-20.913367466307,32.7014454101763,123.515032024856)) ;
#22840=CARTESIAN_POINT('Ctrl Pts',(-20.5796147863066,32.891462371232,123.702629937833)) ;
#22841=CARTESIAN_POINT('Ctrl Pts',(-20.8722060909322,32.7114732908691,123.775321815842)) ;
#22842=CARTESIAN_POINT('Ctrl Pts',(-20.512536676068,32.9013187672146,123.898683038546)) ;
#22843=CARTESIAN_POINT('Ctrl Pts',(-20.7883600167789,32.7213296868517,124.02038977865)) ;
#22844=CARTESIAN_POINT('Ctrl Pts',(-20.4111096637263,32.9113435643946,124.083427639594)) ;
#22845=CARTESIAN_POINT('Ctrl Pts',(-20.6615779007813,32.7313544840317,124.25132140461)) ;
#22846=CARTESIAN_POINT('Ctrl Pts',(-20.2786586384408,32.9213744943784,124.247533456191)) ;
#22847=CARTESIAN_POINT('Ctrl Pts',(-20.4960157375153,32.7413854140155,124.456454889738)) ;
#22848=CARTESIAN_POINT('Ctrl Pts',(-20.1229354505894,32.931219096887,124.38384374608)) ;
#22849=CARTESIAN_POINT('Ctrl Pts',(-20.3013621684409,32.7512300165242,124.626844922445)) ;
#22850=CARTESIAN_POINT('Ctrl Pts',(-19.9435638207466,32.9412099481111,124.493133513568)) ;
#22851=CARTESIAN_POINT('Ctrl Pts',(-20.0771483650704,32.7612208677483,124.763458712167)) ;
#22852=CARTESIAN_POINT('Ctrl Pts',(-19.7468547735515,32.9512477811224,124.569535084003)) ;
#22853=CARTESIAN_POINT('Ctrl Pts',(-19.8312628601083,32.7712587007595,124.858962378708)) ;
#22854=CARTESIAN_POINT('Ctrl Pts',(-19.5439187927745,32.9610921695878,124.610185963789)) ;
#22855=CARTESIAN_POINT('Ctrl Pts',(-19.5775920832475,32.7811030892249,124.909777937782)) ;
#22856=CARTESIAN_POINT('Ctrl Pts',(-19.3341011134292,32.9710769739574,124.615465585142)) ;
#22857=CARTESIAN_POINT('Ctrl Pts',(-19.3153197757331,32.7910878935945,124.916379101424)) ;
#22858=CARTESIAN_POINT('Ctrl Pts',(-19.1274257911367,32.9810164934402,124.584456615172)) ;
#22859=CARTESIAN_POINT('Ctrl Pts',(-19.0569748481772,32.8010274130773,124.877619388893)) ;
#22860=CARTESIAN_POINT('Ctrl Pts',(-18.927334989013,32.9910562244416,124.517330597724)) ;
#22861=CARTESIAN_POINT('Ctrl Pts',(-18.8068609697535,32.8110671440787,124.793713447214)) ;
#22862=CARTESIAN_POINT('Ctrl Pts',(-18.7446634407344,33.0009443526879,124.418083254216)) ;
#22863=CARTESIAN_POINT('Ctrl Pts',(-18.5785199696836,32.820955272325,124.669655218426)) ;
#22864=CARTESIAN_POINT('Ctrl Pts',(-18.5801005857967,33.0109340778964,124.28761411625)) ;
#22865=CARTESIAN_POINT('Ctrl Pts',(-18.3728153330768,32.8309449975335,124.506569798915)) ;
#22866=CARTESIAN_POINT('Ctrl Pts',(-18.4412469443852,33.0208918425979,124.130951753119)) ;
#22867=CARTESIAN_POINT('Ctrl Pts',(-18.1992468678326,32.840902762235,124.310742518053)) ;
#22868=CARTESIAN_POINT('Ctrl Pts',(-18.3318926647563,33.0307941840099,123.9538000731)) ;
#22869=CARTESIAN_POINT('Ctrl Pts',(-18.0625524288157,32.850805103647,124.089302873787)) ;
#22870=CARTESIAN_POINT('Ctrl Pts',(-18.2538818671851,33.0408383797163,123.757588934328)) ;
#22871=CARTESIAN_POINT('Ctrl Pts',(-17.9650377613778,32.8608492993534,123.844039624706)) ;
#22872=CARTESIAN_POINT('Ctrl Pts',(-18.2116804220347,33.0507457804755,123.553613209322)) ;
#22873=CARTESIAN_POINT('Ctrl Pts',(-17.9122844842802,32.8707567001127,123.58906943826)) ;
#22874=CARTESIAN_POINT('Ctrl Pts',(-18.2051029806548,33.0607563803499,123.343258587515)) ;
#22875=CARTESIAN_POINT('Ctrl Pts',(-17.9040614841339,32.880767299987,123.326126151249)) ;
#22876=CARTESIAN_POINT('Ctrl Pts',(-18.2356129749223,33.0707866762621,123.134602723717)) ;
#22877=CARTESIAN_POINT('Ctrl Pts',(-17.9421976273555,32.8907975958992,123.065306227518)) ;
#22878=CARTESIAN_POINT('Ctrl Pts',(-18.300450441629,33.0806414559118,122.937844780199)) ;
#22879=CARTESIAN_POINT('Ctrl Pts',(-18.0232436735507,32.9006523755489,122.819357208247)) ;
#22880=CARTESIAN_POINT('Ctrl Pts',(-18.3989330999902,33.0905987841293,122.753115564655)) ;
#22881=CARTESIAN_POINT('Ctrl Pts',(-18.1463463293519,32.9106097037664,122.588444800357)) ;
#22882=CARTESIAN_POINT('Ctrl Pts',(-18.5293347628917,33.1006378170362,122.587186806717)) ;
#22883=CARTESIAN_POINT('Ctrl Pts',(-18.3093474042476,32.9206487366733,122.381033273986)) ;
#22884=CARTESIAN_POINT('Ctrl Pts',(-18.6837449458525,33.1105109289255,122.44842798728)) ;
#22885=CARTESIAN_POINT('Ctrl Pts',(-18.5023603004912,32.9305218485626,122.207583253798)) ;
#22886=CARTESIAN_POINT('Ctrl Pts',(-18.8634428506156,33.1205842139526,122.336455552253)) ;
#22887=CARTESIAN_POINT('Ctrl Pts',(-18.7269817759468,32.9405951335897,122.067617063673)) ;
#22888=CARTESIAN_POINT('Ctrl Pts',(-19.0549009830223,33.1304045336893,122.259087158195)) ;
#22889=CARTESIAN_POINT('Ctrl Pts',(-18.9663055363985,32.9504154533265,121.970905134139)) ;
#22890=CARTESIAN_POINT('Ctrl Pts',(-19.2620617743464,33.1404831990678,122.214836805238)) ;
#22891=CARTESIAN_POINT('Ctrl Pts',(-19.2252558871534,32.9604941187049,121.915591458617)) ;
#22892=CARTESIAN_POINT('Ctrl Pts',(-19.4690858066591,33.1503347895516,122.207323763932)) ;
#22893=CARTESIAN_POINT('Ctrl Pts',(-19.4840372151867,32.9703457091887,121.906199287805)) ;
#22894=CARTESIAN_POINT('Ctrl Pts',(-19.6788221961635,33.1604079398705,122.236318117315)) ;
#22895=CARTESIAN_POINT('Ctrl Pts',(-19.7462073716882,32.9804188595076,121.942441422299)) ;
#22896=CARTESIAN_POINT('Ctrl Pts',(-19.8757676666468,33.1702503198455,122.29984587334)) ;
#22897=CARTESIAN_POINT('Ctrl Pts',(-19.9923907933803,32.9902612394826,122.021850824201)) ;
#22898=CARTESIAN_POINT('Ctrl Pts',(-20.0615568423931,33.1802312960886,122.397340048121)) ;
#22899=CARTESIAN_POINT('Ctrl Pts',(-20.2246277641436,33.0002422157257,122.143718242006)) ;
#22900=CARTESIAN_POINT('Ctrl Pts',(-20.2279876372291,33.1902476244439,122.526364012805)) ;
#22901=CARTESIAN_POINT('Ctrl Pts',(-20.4326666594073,33.010258544081,122.304997705767)) ;
#22902=CARTESIAN_POINT('Ctrl Pts',(-20.3679958704936,33.200145421435,122.680288715959)) ;
#22903=CARTESIAN_POINT('Ctrl Pts',(-20.6076780088902,33.0201563410721,122.497403957948)) ;
#22904=CARTESIAN_POINT('Ctrl Pts',(-20.4807568430483,33.2101579781671,122.858052147058)) ;
#22905=CARTESIAN_POINT('Ctrl Pts',(-20.7486295700232,33.0301688978042,122.719608055138)) ;
#22906=CARTESIAN_POINT('Ctrl Pts',(-20.5606237614743,33.2201900130135,123.053239269694)) ;
#22907=CARTESIAN_POINT('Ctrl Pts',(-20.8484637130917,33.0402009326507,122.96359161389)) ;
#22908=CARTESIAN_POINT('Ctrl Pts',(-20.6050359521563,33.230029413829,123.255287016282)) ;
#22909=CARTESIAN_POINT('Ctrl Pts',(-20.9039796443904,33.0500403334661,123.216152649294)) ;
#22910=CARTESIAN_POINT('Ctrl Pts',(-20.614049092095,33.2400951994806,123.466685199039)) ;
#22911=CARTESIAN_POINT('Ctrl Pts',(-20.9152463774755,33.0601061191177,123.480399984258)) ;
#22912=CARTESIAN_POINT('Ctrl Pts',(-20.5866016199623,33.2499856545952,123.672815882505)) ;
#22913=CARTESIAN_POINT('Ctrl Pts',(-20.8809372575507,33.0699965742323,123.738064421165)) ;
#22914=CARTESIAN_POINT('Ctrl Pts',(-20.5235744358789,33.2599777732309,123.873192435292)) ;
#22915=CARTESIAN_POINT('Ctrl Pts',(-20.8021533889854,33.0799886928681,123.98853537261)) ;
#22916=CARTESIAN_POINT('Ctrl Pts',(-20.4268201921986,33.269940599994,124.058949341531)) ;
#22917=CARTESIAN_POINT('Ctrl Pts',(-20.6812106073249,33.0899515196311,124.220732031348)) ;
#22918=CARTESIAN_POINT('Ctrl Pts',(-20.3004366840512,33.2798448832669,124.224447351388)) ;
#22919=CARTESIAN_POINT('Ctrl Pts',(-20.5232306933288,33.099855802904,124.427605321835)) ;
#22920=CARTESIAN_POINT('Ctrl Pts',(-20.1447295418141,33.289905317214,124.36754765931)) ;
#22921=CARTESIAN_POINT('Ctrl Pts',(-20.3285971107455,33.1099162368511,124.606480559927)) ;
#22922=CARTESIAN_POINT('Ctrl Pts',(-19.9705348461401,33.2997458698872,124.479200573106)) ;
#22923=CARTESIAN_POINT('Ctrl Pts',(-20.1108525131507,33.1197567895243,124.746047511506)) ;
#22924=CARTESIAN_POINT('Ctrl Pts',(-19.7754486620415,33.3098080898329,124.560937015525)) ;
#22925=CARTESIAN_POINT('Ctrl Pts',(-19.8669950901314,33.12981900947,124.84821784105)) ;
#22926=CARTESIAN_POINT('Ctrl Pts',(-19.57243885132,33.3197052291114,124.606588971433)) ;
#22927=CARTESIAN_POINT('Ctrl Pts',(-19.6132318493154,33.1397161487486,124.905283007203)) ;
#22928=CARTESIAN_POINT('Ctrl Pts',(-19.3639189425878,33.3296364212465,124.61702574814)) ;
#22929=CARTESIAN_POINT('Ctrl Pts',(-19.3525812289575,33.1496473408836,124.918328736674)) ;
#22930=CARTESIAN_POINT('Ctrl Pts',(-19.1544701914488,33.3396785758916,124.5905747195)) ;
#22931=CARTESIAN_POINT('Ctrl Pts',(-19.090770522027,33.1596894955287,124.885264797401)) ;
#22932=CARTESIAN_POINT('Ctrl Pts',(-18.9558448503062,33.3495653369109,124.529280922673)) ;
#22933=CARTESIAN_POINT('Ctrl Pts',(-18.842487870914,33.169576256548,124.808646986439)) ;
#22934=CARTESIAN_POINT('Ctrl Pts',(-18.7686911463768,33.3595646386281,124.433610207421)) ;
#22935=CARTESIAN_POINT('Ctrl Pts',(-18.6085457635101,33.1795755582652,124.689058201042)) ;
#22936=CARTESIAN_POINT('Ctrl Pts',(-18.6021783660485,33.3694854367949,124.307970432937)) ;
#22937=CARTESIAN_POINT('Ctrl Pts',(-18.4004044124469,33.189496356432,124.532007686267)) ;
#22938=CARTESIAN_POINT('Ctrl Pts',(-18.4584063019832,33.3795194903916,124.153637802788)) ;
#22939=CARTESIAN_POINT('Ctrl Pts',(-18.2206897370185,33.1995304100287,124.339091714962)) ;
#22940=CARTESIAN_POINT('Ctrl Pts',(-18.3447487639094,33.389442607958,123.978664957015)) ;
#22941=CARTESIAN_POINT('Ctrl Pts',(-18.0786177880743,33.2094535275951,124.120374761366)) ;
#22942=CARTESIAN_POINT('Ctrl Pts',(-18.262168874499,33.3994987314571,123.784072019688)) ;
#22943=CARTESIAN_POINT('Ctrl Pts',(-17.9753934550452,33.2195096510942,123.87713368977)) ;
#22944=CARTESIAN_POINT('Ctrl Pts',(-18.2155327305873,33.4093441731119,123.582403847225)) ;
#22945=CARTESIAN_POINT('Ctrl Pts',(-17.9170984303965,33.2293550927491,123.625046988953)) ;
#22946=CARTESIAN_POINT('Ctrl Pts',(-18.203805100798,33.4193064742361,123.373306871914)) ;
#22947=CARTESIAN_POINT('Ctrl Pts',(-17.9024396209619,33.2393173938732,123.363675275733)) ;
#22948=CARTESIAN_POINT('Ctrl Pts',(-18.2290055597389,33.4293349535112,123.163973793253)) ;
#22949=CARTESIAN_POINT('Ctrl Pts',(-17.9339408232565,33.2493458731483,123.102009100134)) ;
#22950=CARTESIAN_POINT('Ctrl Pts',(-18.289374518782,33.4392453070209,122.96457571185)) ;
#22951=CARTESIAN_POINT('Ctrl Pts',(-18.009402919707,33.259256226658,122.852760854094)) ;
#22952=CARTESIAN_POINT('Ctrl Pts',(-18.3832010117499,33.4491801791981,122.777967476055)) ;
#22953=CARTESIAN_POINT('Ctrl Pts',(-18.1266871223674,33.2691910988352,122.61950036567)) ;
#22954=CARTESIAN_POINT('Ctrl Pts',(-18.5094881208649,33.4592213167838,122.60882144455)) ;
#22955=CARTESIAN_POINT('Ctrl Pts',(-18.2845465433898,33.2792322364209,122.40806845954)) ;
#22956=CARTESIAN_POINT('Ctrl Pts',(-18.6607816210844,33.4691084659983,122.466272054033)) ;
#22957=CARTESIAN_POINT('Ctrl Pts',(-18.4736647676083,33.2891193856355,122.229881635933)) ;
#22958=CARTESIAN_POINT('Ctrl Pts',(-18.8361603645087,33.4791007007494,122.350665197575)) ;
#22959=CARTESIAN_POINT('Ctrl Pts',(-18.6928889148738,33.2991116203865,122.085373784708)) ;
#22960=CARTESIAN_POINT('Ctrl Pts',(-19.0281558133508,33.4890494063124,122.267675696057)) ;
#22961=CARTESIAN_POINT('Ctrl Pts',(-18.9328841091275,33.3090603259495,121.981637584403)) ;
#22962=CARTESIAN_POINT('Ctrl Pts',(-19.2312903333038,33.4989854747361,122.219054749115)) ;
#22963=CARTESIAN_POINT('Ctrl Pts',(-19.1868031331839,33.3189963943732,121.920862306553)) ;
#22964=CARTESIAN_POINT('Ctrl Pts',(-19.4408438884127,33.5089711589519,122.206138288306)) ;
#22965=CARTESIAN_POINT('Ctrl Pts',(-19.4487454010854,33.328982078589,121.90471788781)) ;
#22966=CARTESIAN_POINT('Ctrl Pts',(-19.6505310611523,33.5190115855205,122.230262302281)) ;
#22967=CARTESIAN_POINT('Ctrl Pts',(-19.7108540776556,33.3390225051576,121.934873930191)) ;
#22968=CARTESIAN_POINT('Ctrl Pts',(-19.8489000133317,33.5288506989843,122.288894555747)) ;
#22969=CARTESIAN_POINT('Ctrl Pts',(-19.9588162424853,33.3488616186214,122.008165761205)) ;
#22970=CARTESIAN_POINT('Ctrl Pts',(-20.0378734404374,33.5388804331601,122.382439401842)) ;
#22971=CARTESIAN_POINT('Ctrl Pts',(-20.1950323307625,33.3588913527972,122.125097981869)) ;
#22972=CARTESIAN_POINT('Ctrl Pts',(-20.2072755150805,33.548902532666,122.50771918548)) ;
#22973=CARTESIAN_POINT('Ctrl Pts',(-20.406784218548,33.3689134523031,122.281698617158)) ;
#22974=CARTESIAN_POINT('Ctrl Pts',(-20.3505163323491,33.5587709725594,122.657820476515)) ;
#22975=CARTESIAN_POINT('Ctrl Pts',(-20.5858350552601,33.3787818921965,122.469326974363)) ;
#22976=CARTESIAN_POINT('Ctrl Pts',(-20.467830910548,33.568839837245,122.833994863383)) ;
#22977=CARTESIAN_POINT('Ctrl Pts',(-20.732476955186,33.3888507568821,122.68954538537)) ;
#22978=CARTESIAN_POINT('Ctrl Pts',(-20.5508822742983,33.5786825103436,123.023527927505)) ;
#22979=CARTESIAN_POINT('Ctrl Pts',(-20.8362904559934,33.3986934299808,122.926463443138)) ;
#22980=CARTESIAN_POINT('Ctrl Pts',(-20.6010906324588,33.5886431445061,123.226819066084)) ;
#22981=CARTESIAN_POINT('Ctrl Pts',(-20.8990494415645,33.4086540641432,123.180578146984)) ;
#22982=CARTESIAN_POINT('Ctrl Pts',(-20.6149332523502,33.5986810601842,123.437385843915)) ;
#22983=CARTESIAN_POINT('Ctrl Pts',(-20.916351249052,33.4186919798213,123.443786581483)) ;
#22984=CARTESIAN_POINT('Ctrl Pts',(-20.5927561143563,33.6085553350436,123.64381161214)) ;
#22985=CARTESIAN_POINT('Ctrl Pts',(-20.8886281343362,33.4285662546808,123.701819630219)) ;
#22986=CARTESIAN_POINT('Ctrl Pts',(-20.5339350999099,33.6186250854188,123.847144174352)) ;
#22987=CARTESIAN_POINT('Ctrl Pts',(-20.8151004364326,33.4386360050559,123.95598455471)) ;
#22988=CARTESIAN_POINT('Ctrl Pts',(-20.4429721196494,33.6284583807933,124.032801166583)) ;
#22989=CARTESIAN_POINT('Ctrl Pts',(-20.7013946872375,33.4484693004304,124.188056231771)) ;
#22990=CARTESIAN_POINT('Ctrl Pts',(-20.3192120120837,33.6384886782729,124.203524561785)) ;
#22991=CARTESIAN_POINT('Ctrl Pts',(-20.5466931297227,33.45849959791,124.401459336272)) ;
#22992=CARTESIAN_POINT('Ctrl Pts',(-20.1672189301495,33.6485207647143,124.34975537749)) ;
#22993=CARTESIAN_POINT('Ctrl Pts',(-20.3567007162318,33.4685316843515,124.58424663072)) ;
#22994=CARTESIAN_POINT('Ctrl Pts',(-19.9959765672418,33.6583486932033,124.465347265226)) ;
#22995=CARTESIAN_POINT('Ctrl Pts',(-20.1426457143214,33.4783596128404,124.728735741513)) ;
#22996=CARTESIAN_POINT('Ctrl Pts',(-19.8042599262361,33.668344734314,124.551406477392)) ;
#22997=CARTESIAN_POINT('Ctrl Pts',(-19.9029989792466,33.4883556539512,124.836308043002)) ;
#22998=CARTESIAN_POINT('Ctrl Pts',(-19.5997986838968,33.6783705464153,124.602630095532)) ;
#22999=CARTESIAN_POINT('Ctrl Pts',(-19.6474220237301,33.4983814660524,124.900335793291)) ;
#23000=CARTESIAN_POINT('Ctrl Pts',(-19.3924774849365,33.6882577813101,124.617636375072)) ;
#23001=CARTESIAN_POINT('Ctrl Pts',(-19.3882695560054,33.5082687009472,124.919091810044)) ;
#23002=CARTESIAN_POINT('Ctrl Pts',(-19.1838086719246,33.6982346475211,124.59657238943)) ;
#23003=CARTESIAN_POINT('Ctrl Pts',(-19.1274334857693,33.5182455671582,124.892759807624)) ;
#23004=CARTESIAN_POINT('Ctrl Pts',(-18.9815887866603,33.7082275913929,124.539527650244)) ;
#23005=CARTESIAN_POINT('Ctrl Pts',(-18.8746590268341,33.52823851103,124.821451907867)) ;
#23006=CARTESIAN_POINT('Ctrl Pts',(-18.7916507877663,33.7182655140643,124.447604623788)) ;
#23007=CARTESIAN_POINT('Ctrl Pts',(-18.6372374521722,33.5382764337014,124.706546424498)) ;
#23008=CARTESIAN_POINT('Ctrl Pts',(-18.6235800416685,33.728113978326,124.326664479328)) ;
#23009=CARTESIAN_POINT('Ctrl Pts',(-18.4271493677989,33.5481248979631,124.555368999614)) ;
#23010=CARTESIAN_POINT('Ctrl Pts',(-18.4767212967357,33.73810584507,124.17651438228)) ;
#23011=CARTESIAN_POINT('Ctrl Pts',(-18.2435773439465,33.5581167647071,124.367679767415)) ;
#23012=CARTESIAN_POINT('Ctrl Pts',(-18.3589139649517,33.7480235771112,124.004451145981)) ;
#23013=CARTESIAN_POINT('Ctrl Pts',(-18.096319636919,33.5680344967483,124.152599028164)) ;
#23014=CARTESIAN_POINT('Ctrl Pts',(-18.2717798858509,33.7580517620064,123.812495005014)) ;
#23015=CARTESIAN_POINT('Ctrl Pts',(-17.9874040348388,33.5780626816436,123.912652984584)) ;
#23016=CARTESIAN_POINT('Ctrl Pts',(-18.2199583948153,33.7679369200553,123.611237430731)) ;
#23017=CARTESIAN_POINT('Ctrl Pts',(-17.9226291155959,33.5879478396924,123.661079753393)) ;
#23018=CARTESIAN_POINT('Ctrl Pts',(-18.2031899992664,33.777926280597,123.401895935145)) ;
#23019=CARTESIAN_POINT('Ctrl Pts',(-17.9016709287819,33.5979372002341,123.399402541443)) ;
#23020=CARTESIAN_POINT('Ctrl Pts',(-18.2235716353926,33.7879674375313,123.191785549963)) ;
#23021=CARTESIAN_POINT('Ctrl Pts',(-17.9271501704679,33.6079783571685,123.1367648659)) ;
#23022=CARTESIAN_POINT('Ctrl Pts',(-18.2786200114163,33.7978000209865,122.992541931651)) ;
#23023=CARTESIAN_POINT('Ctrl Pts',(-17.9959631146861,33.6178109406236,122.887710030823)) ;
#23024=CARTESIAN_POINT('Ctrl Pts',(-18.3683487595105,33.8077942409485,122.802558224902)) ;
#23025=CARTESIAN_POINT('Ctrl Pts',(-18.1081263093149,33.6278051605856,122.650231330554)) ;
#23026=CARTESIAN_POINT('Ctrl Pts',(-18.4904696258343,33.8178223427358,122.63070110739)) ;
#23027=CARTESIAN_POINT('Ctrl Pts',(-18.2607792875272,33.6378332623729,122.435411305488)) ;
#23028=CARTESIAN_POINT('Ctrl Pts',(-18.6381482308556,33.8277022873588,122.484636845884)) ;
#23029=CARTESIAN_POINT('Ctrl Pts',(-18.4453797141511,33.647713206996,122.252832221367)) ;
#23030=CARTESIAN_POINT('Ctrl Pts',(-18.8106558657306,33.8376926139159,122.364855145629)) ;
#23031=CARTESIAN_POINT('Ctrl Pts',(-18.6610157891126,33.657703533553,122.10310705135)) ;
#23032=CARTESIAN_POINT('Ctrl Pts',(-19.0004133748142,33.8476335455702,122.277272733612)) ;
#23033=CARTESIAN_POINT('Ctrl Pts',(-18.8982140305105,33.6676444652073,121.993631136502)) ;
#23034=CARTESIAN_POINT('Ctrl Pts',(-19.2033679275045,33.8576206640731,122.223428561579)) ;
#23035=CARTESIAN_POINT('Ctrl Pts',(-19.1519080089799,33.6776315837102,121.92632833614)) ;
#23036=CARTESIAN_POINT('Ctrl Pts',(-19.413555239702,33.8676539969703,122.205893497392)) ;
#23037=CARTESIAN_POINT('Ctrl Pts',(-19.4146423301779,33.6876649166074,121.904411969349)) ;
#23038=CARTESIAN_POINT('Ctrl Pts',(-19.6201683892138,33.877520101415,122.224398460952)) ;
#23039=CARTESIAN_POINT('Ctrl Pts',(-19.6729091690056,33.6975310210521,121.927545767156)) ;
#23040=CARTESIAN_POINT('Ctrl Pts',(-19.824456202544,33.8875862152953,122.279533485596)) ;
#23041=CARTESIAN_POINT('Ctrl Pts',(-19.9282681240009,33.7075971349325,121.996466980296)) ;
#23042=CARTESIAN_POINT('Ctrl Pts',(-20.0121077833752,33.8974422270637,122.367434002635)) ;
#23043=CARTESIAN_POINT('Ctrl Pts',(-20.1628320829574,33.7174531467009,122.10634520991)) ;
#23044=CARTESIAN_POINT('Ctrl Pts',(-20.1843716366312,33.9074369306951,122.487738822849)) ;
#23045=CARTESIAN_POINT('Ctrl Pts',(-20.3781604555604,33.7274478503322,122.256728476995)) ;
#23046=CARTESIAN_POINT('Ctrl Pts',(-20.3333627134761,33.9174682664199,122.63699684848)) ;
#23047=CARTESIAN_POINT('Ctrl Pts',(-20.5643974693118,33.7374791860571,122.443302838799)) ;
#23048=CARTESIAN_POINT('Ctrl Pts',(-20.4524620397036,33.9273347916236,122.806830884017)) ;
#23049=CARTESIAN_POINT('Ctrl Pts',(-20.713269761922,33.7473457112607,122.655597325724)) ;
#23050=CARTESIAN_POINT('Ctrl Pts',(-20.5416324218957,33.9373222196694,122.996895065908)) ;
#23051=CARTESIAN_POINT('Ctrl Pts',(-20.8247303532555,33.7573331393065,122.893178808627)) ;
#23052=CARTESIAN_POINT('Ctrl Pts',(-20.5963371639424,33.9472671493558,123.198716985131)) ;
#23053=CARTESIAN_POINT('Ctrl Pts',(-20.8931087336896,33.767278068993,123.145457142139)) ;
#23054=CARTESIAN_POINT('Ctrl Pts',(-20.615233404167,33.9573120674643,123.409025558996)) ;
#23055=CARTESIAN_POINT('Ctrl Pts',(-20.9167263518425,33.7773229871015,123.408343079754)) ;
#23056=CARTESIAN_POINT('Ctrl Pts',(-20.5978343581406,33.9671740370782,123.615640699636)) ;
#23057=CARTESIAN_POINT('Ctrl Pts',(-20.8949748056446,33.7871849567154,123.666612207482)) ;
#23058=CARTESIAN_POINT('Ctrl Pts',(-20.5445304522243,33.9771661050995,123.818808413641)) ;
#23059=CARTESIAN_POINT('Ctrl Pts',(-20.8283422293108,33.7971770247366,123.920571241178)) ;
#23060=CARTESIAN_POINT('Ctrl Pts',(-20.4572488945019,33.987097030474,124.008482314326)) ;
#23061=CARTESIAN_POINT('Ctrl Pts',(-20.7192376865205,33.8071079501112,124.157662672187)) ;
#23062=CARTESIAN_POINT('Ctrl Pts',(-20.3384279441806,33.9970476586975,124.180637038288)) ;
#23063=CARTESIAN_POINT('Ctrl Pts',(-20.5707091129721,33.8170585783346,124.372854625881)) ;
#23064=CARTESIAN_POINT('Ctrl Pts',(-20.1908473350017,34.0070478977566,124.330400148074)) ;
#23065=CARTESIAN_POINT('Ctrl Pts',(-20.3862313186414,33.8270588173937,124.560056609312)) ;
#23066=CARTESIAN_POINT('Ctrl Pts',(-20.0188703479351,34.0170763531258,124.452341161375)) ;
#23067=CARTESIAN_POINT('Ctrl Pts',(-20.1712584195521,33.8370872727629,124.71248063517)) ;
#23068=CARTESIAN_POINT('Ctrl Pts',(-19.8315368351169,34.026942387709,124.541398156012)) ;
#23069=CARTESIAN_POINT('Ctrl Pts',(-19.9370901885251,33.8469533073462,124.823799494521)) ;
#23070=CARTESIAN_POINT('Ctrl Pts',(-19.6291473919891,34.0369347094565,124.597606613349)) ;
#23071=CARTESIAN_POINT('Ctrl Pts',(-19.6841021964421,33.8569456290936,124.894057284954)) ;
#23072=CARTESIAN_POINT('Ctrl Pts',(-19.4212948778569,34.0468669991335,124.617735601843)) ;
#23073=CARTESIAN_POINT('Ctrl Pts',(-19.424287490384,33.8668779187706,124.9192160717)) ;
#23074=CARTESIAN_POINT('Ctrl Pts',(-19.2116608547725,34.0568686441042,124.601562538898)) ;
#23075=CARTESIAN_POINT('Ctrl Pts',(-19.1622401128872,33.8768795637414,124.898995670993)) ;
#23076=CARTESIAN_POINT('Ctrl Pts',(-18.9405917318877,34.0701812775203,124.531785628182)) ;
#23077=CARTESIAN_POINT('Ctrl Pts',(-18.823429392135,33.8901921971574,124.811777112252)) ;
#23078=CARTESIAN_POINT('Ctrl Pts',(-18.6953484784507,34.0834130269018,124.393891815293)) ;
#23079=CARTESIAN_POINT('Ctrl Pts',(-18.5168908225473,33.903423946539,124.639429121269)) ;
#23080=CARTESIAN_POINT('Ctrl Pts',(-18.4950002821873,34.0967362917189,124.198208396693)) ;
#23081=CARTESIAN_POINT('Ctrl Pts',(-18.266416953034,33.916747211356,124.394788919274)) ;
#23082=CARTESIAN_POINT('Ctrl Pts',(-18.3736497757206,34.1066119979366,124.029725845387)) ;
#23083=CARTESIAN_POINT('Ctrl Pts',(-18.1147393757088,33.9266229175737,124.184190734435)) ;
#23084=CARTESIAN_POINT('Ctrl Pts',(-18.2821299159748,34.1166015890366,123.840730802708)) ;
#23085=CARTESIAN_POINT('Ctrl Pts',(-18.0003398463956,33.9366125086737,123.947943873737)) ;
#23086=CARTESIAN_POINT('Ctrl Pts',(-18.2250270269363,34.126528685492,123.639969576889)) ;
#23087=CARTESIAN_POINT('Ctrl Pts',(-17.9289645288639,33.9465396051291,123.69699206503)) ;
#23088=CARTESIAN_POINT('Ctrl Pts',(-18.2034190105843,34.1365538339966,123.430338906527)) ;
#23089=CARTESIAN_POINT('Ctrl Pts',(-17.9019571311773,33.9565647536337,123.434953214904)) ;
#23090=CARTESIAN_POINT('Ctrl Pts',(-18.2182165399645,34.1464494881433,123.22280972338)) ;
#23091=CARTESIAN_POINT('Ctrl Pts',(-17.920456867938,33.9664604077804,123.175542057052)) ;
#23092=CARTESIAN_POINT('Ctrl Pts',(-18.2690763393294,34.1564530225215,123.018767205604)) ;
#23093=CARTESIAN_POINT('Ctrl Pts',(-17.9840343132116,33.9764639421586,122.920489516577)) ;
#23094=CARTESIAN_POINT('Ctrl Pts',(-18.3544753384947,34.1664381609615,122.826969229147)) ;
#23095=CARTESIAN_POINT('Ctrl Pts',(-18.0907856147797,33.9864490805987,122.680743142477)) ;
#23096=CARTESIAN_POINT('Ctrl Pts',(-18.472628068217,34.1764740855569,122.652181840679)) ;
#23097=CARTESIAN_POINT('Ctrl Pts',(-18.2384789185145,33.996485005194,122.462260358717)) ;
#23098=CARTESIAN_POINT('Ctrl Pts',(-18.6164655673293,34.1863253609846,122.503176356432)) ;
#23099=CARTESIAN_POINT('Ctrl Pts',(-18.4182776203018,34.0063362806217,122.276005602402)) ;
#23100=CARTESIAN_POINT('Ctrl Pts',(-18.7860413391488,34.1963176221459,122.379176678945)) ;
#23101=CARTESIAN_POINT('Ctrl Pts',(-18.6302489538193,34.0163285417831,122.121008187001)) ;
#23102=CARTESIAN_POINT('Ctrl Pts',(-18.9756890039157,34.2063575061635,122.28655058311)) ;
#23103=CARTESIAN_POINT('Ctrl Pts',(-18.8673098715377,34.0263684258007,122.00522798075)) ;
#23104=CARTESIAN_POINT('Ctrl Pts',(-19.1742841833314,34.216192280666,122.228937175601)) ;
#23105=CARTESIAN_POINT('Ctrl Pts',(-19.1155543481873,34.0362032003031,121.933213929773)) ;
#23106=CARTESIAN_POINT('Ctrl Pts',(-19.3848491923498,34.2262686616863,122.206064095347)) ;
#23107=CARTESIAN_POINT('Ctrl Pts',(-19.3787606441446,34.0462795813234,121.904625237353)) ;
#23108=CARTESIAN_POINT('Ctrl Pts',(-19.5914235484233,34.2361149348369,122.219725589952)) ;
#23109=CARTESIAN_POINT('Ctrl Pts',(-19.636979964933,34.056125854474,121.921704730838)) ;
#23110=CARTESIAN_POINT('Ctrl Pts',(-19.8644290889112,34.2494794561221,122.286150104752)) ;
#23111=CARTESIAN_POINT('Ctrl Pts',(-19.9782262367002,34.0694903757593,122.004738916925)) ;
#23112=CARTESIAN_POINT('Ctrl Pts',(-20.1107333011822,34.2626857005566,122.421054667692)) ;
#23113=CARTESIAN_POINT('Ctrl Pts',(-20.2860725515586,34.0826966201937,122.173341752895)) ;
#23114=CARTESIAN_POINT('Ctrl Pts',(-20.3128900283233,34.2759506552338,122.613069418679)) ;
#23115=CARTESIAN_POINT('Ctrl Pts',(-20.5388137926812,34.0959615748709,122.413398914322)) ;
#23116=CARTESIAN_POINT('Ctrl Pts',(-20.438205183774,34.2859829357855,122.782731790521)) ;
#23117=CARTESIAN_POINT('Ctrl Pts',(-20.6954462284396,34.1059938554226,122.625471146507)) ;
#23118=CARTESIAN_POINT('Ctrl Pts',(-20.5310032145783,34.2958916693034,122.96922602419)) ;
#23119=CARTESIAN_POINT('Ctrl Pts',(-20.8114438350329,34.1159025889405,122.858591933872)) ;
#23120=CARTESIAN_POINT('Ctrl Pts',(-20.5907085275571,34.3058292201709,123.169440553708)) ;
#23121=CARTESIAN_POINT('Ctrl Pts',(-20.8860726329882,34.125840139808,123.108858926557)) ;
#23122=CARTESIAN_POINT('Ctrl Pts',(-20.6147885837747,34.3158590677648,123.378897155107)) ;
#23123=CARTESIAN_POINT('Ctrl Pts',(-20.9161696354576,34.1358699874019,123.370684085346)) ;
#23124=CARTESIAN_POINT('Ctrl Pts',(-20.5984660377212,34.3290942076852,123.656745178139)) ;
#23125=CARTESIAN_POINT('Ctrl Pts',(-20.8957675550664,34.1491051273224,123.717974610671)) ;
#23126=CARTESIAN_POINT('Ctrl Pts',(-20.4868736795983,34.3457626720564,123.993002939098)) ;
#23127=CARTESIAN_POINT('Ctrl Pts',(-20.7562726268257,34.1657735916935,124.138314956001)) ;
#23128=CARTESIAN_POINT('Ctrl Pts',(-20.2251415994005,34.3656336839303,124.324854114814)) ;
#23129=CARTESIAN_POINT('Ctrl Pts',(-20.4290861791078,34.1856446035674,124.553127465598)) ;
#23130=CARTESIAN_POINT('Ctrl Pts',(-19.9231542481283,34.3823407683133,124.511841033235)) ;
#23131=CARTESIAN_POINT('Ctrl Pts',(-20.0516612997823,34.2023516879504,124.786832185012)) ;
#23132=CARTESIAN_POINT('Ctrl Pts',(-19.657904162901,34.3955180496239,124.591763757733)) ;
#23133=CARTESIAN_POINT('Ctrl Pts',(-19.7200431655426,34.215528969261,124.88675620924)) ;
#23134=CARTESIAN_POINT('Ctrl Pts',(-19.3810401547888,34.408785510138,124.625633782009)) ;
#23135=CARTESIAN_POINT('Ctrl Pts',(-19.3739840223207,34.2287964297751,124.92908813568)) ;
#23136=CARTESIAN_POINT('Ctrl Pts',(-19.0312401721135,34.4253994008252,124.576410369976)) ;
#23137=CARTESIAN_POINT('Ctrl Pts',(-18.936720024018,34.2454103204623,124.86755517988)) ;
#23138=CARTESIAN_POINT('Ctrl Pts',(-18.6565409852236,34.4453482002526,124.377526322459)) ;
#23139=CARTESIAN_POINT('Ctrl Pts',(-18.4683529488932,34.2653591198897,124.618947214226)) ;
#23140=CARTESIAN_POINT('Ctrl Pts',(-18.372722975046,34.4652693117834,124.063178650212)) ;
#23141=CARTESIAN_POINT('Ctrl Pts',(-18.1135823385577,34.2852802314206,124.226010700003)) ;
#23142=CARTESIAN_POINT('Ctrl Pts',(-18.2127872385282,34.4851357599563,123.672140863886)) ;
#23143=CARTESIAN_POINT('Ctrl Pts',(-17.9136663305497,34.3051466795934,123.737213595555)) ;
#23144=CARTESIAN_POINT('Ctrl Pts',(-18.1960174572984,34.5051621065734,123.246703868946)) ;
#23145=CARTESIAN_POINT('Ctrl Pts',(-17.8927069831386,34.3251730262106,123.205416904764)) ;
#23146=CARTESIAN_POINT('Ctrl Pts',(-18.3244861075331,34.525024150963,122.844320049915)) ;
#23147=CARTESIAN_POINT('Ctrl Pts',(-18.0532950837359,34.3450350706001,122.702439446676)) ;
#23148=CARTESIAN_POINT('Ctrl Pts',(-18.5830265246617,34.5449694536441,122.508225439242)) ;
#23149=CARTESIAN_POINT('Ctrl Pts',(-18.3764719974847,34.3649803732812,122.282323158732)) ;
#23150=CARTESIAN_POINT('Ctrl Pts',(-18.9399371008137,34.564864760703,122.281121704416)) ;
#23151=CARTESIAN_POINT('Ctrl Pts',(-18.8226102498659,34.3848756803401,121.998446004947)) ;
#23152=CARTESIAN_POINT('Ctrl Pts',(-19.3527127164133,34.5847580308706,122.188711680669)) ;
#23153=CARTESIAN_POINT('Ctrl Pts',(-19.3385786404572,34.4047689505077,121.882935209767)) ;
#23154=CARTESIAN_POINT('Ctrl Pts',(-19.7737254388914,34.604723623551,122.242987808738)) ;
#23155=CARTESIAN_POINT('Ctrl Pts',(-19.864843872694,34.4247345431882,121.950781567567)) ;
#23156=CARTESIAN_POINT('Ctrl Pts',(-20.1494199931143,34.6245989472359,122.436554500858)) ;
#23157=CARTESIAN_POINT('Ctrl Pts',(-20.3344600160615,34.444609866873,122.192739799094)) ;
#23158=CARTESIAN_POINT('Ctrl Pts',(-20.4382613496929,34.6445740098108,122.747966146561)) ;
#23159=CARTESIAN_POINT('Ctrl Pts',(-20.6955112754201,34.464584929448,122.582004291072)) ;
#23160=CARTESIAN_POINT('Ctrl Pts',(-20.6027074825129,34.6645264194419,123.139039458747)) ;
#23161=CARTESIAN_POINT('Ctrl Pts',(-20.9010681970121,34.4845373390791,123.070845431308)) ;
#23162=CARTESIAN_POINT('Ctrl Pts',(-20.6245230947549,34.684362473678,123.560242571632)) ;
#23163=CARTESIAN_POINT('Ctrl Pts',(-20.9283379623324,34.5043733933152,123.597346656962)) ;
#23164=CARTESIAN_POINT('Ctrl Pts',(-20.5008638045205,34.7043403850956,123.9666287374)) ;
#23165=CARTESIAN_POINT('Ctrl Pts',(-20.7737648833637,34.5243513047327,124.105329355223)) ;
#23166=CARTESIAN_POINT('Ctrl Pts',(-20.2463289326715,34.7242584345991,124.305081206645)) ;
#23167=CARTESIAN_POINT('Ctrl Pts',(-20.4555977349369,34.5442693542362,124.528394482397)) ;
#23168=CARTESIAN_POINT('Ctrl Pts',(-19.8929765679083,34.7441265783672,124.53677216459)) ;
#23169=CARTESIAN_POINT('Ctrl Pts',(-20.0139097341758,34.5641374980043,124.818008765311)) ;
#23170=CARTESIAN_POINT('Ctrl Pts',(-19.4780285765812,34.7641774349545,124.634188159113)) ;
#23171=CARTESIAN_POINT('Ctrl Pts',(-19.4952245290992,34.5841883545916,124.939780508264)) ;
#23172=CARTESIAN_POINT('Ctrl Pts',(-19.060179710771,34.7839578714104,124.585251419341)) ;
#23173=CARTESIAN_POINT('Ctrl Pts',(-18.9729159061863,34.6039687910475,124.878612004196)) ;
#23174=CARTESIAN_POINT('Ctrl Pts',(-18.6792558296266,34.8039879270882,124.394988896057)) ;
#23175=CARTESIAN_POINT('Ctrl Pts',(-18.496759486199,34.6239988467253,124.640786108479)) ;
#23176=CARTESIAN_POINT('Ctrl Pts',(-18.3887123278353,34.823869032263,124.087835513571)) ;
#23177=CARTESIAN_POINT('Ctrl Pts',(-18.1335792137849,34.6438799519001,124.256847057463)) ;
#23178=CARTESIAN_POINT('Ctrl Pts',(-18.2193821090019,34.8437494946307,123.70056629443)) ;
#23179=CARTESIAN_POINT('Ctrl Pts',(-17.9219139096296,34.6637604142679,123.772762991353)) ;
#23180=CARTESIAN_POINT('Ctrl Pts',(-18.1923412672095,34.8637346417751,123.276475566402)) ;
#23181=CARTESIAN_POINT('Ctrl Pts',(-17.8881094855176,34.6837455614122,123.242649910961)) ;
#23182=CARTESIAN_POINT('Ctrl Pts',(-18.3111763931638,34.8836252203115,122.870576698358)) ;
#23183=CARTESIAN_POINT('Ctrl Pts',(-18.0366497415648,34.7036361399486,122.735276316463)) ;
#23184=CARTESIAN_POINT('Ctrl Pts',(-18.5608208396316,34.9035192401859,122.529106310762)) ;
#23185=CARTESIAN_POINT('Ctrl Pts',(-18.3487015779653,34.723530159823,122.308436690887)) ;
#23186=CARTESIAN_POINT('Ctrl Pts',(-18.9123762892436,34.9234406849123,122.292940920012)) ;
#23187=CARTESIAN_POINT('Ctrl Pts',(-18.7881430602527,34.7434516045494,122.013226846896)) ;
#23188=CARTESIAN_POINT('Ctrl Pts',(-19.322937407292,34.9433388229677,122.190263489512)) ;
#23189=CARTESIAN_POINT('Ctrl Pts',(-19.3013427498124,34.7633497426048,121.884875817397)) ;
#23190=CARTESIAN_POINT('Ctrl Pts',(-19.7472655180878,34.9634095781838,122.235024621243)) ;
#23191=CARTESIAN_POINT('Ctrl Pts',(-19.8317538659919,34.7834204978209,121.940822959894)) ;
#23192=CARTESIAN_POINT('Ctrl Pts',(-20.1256368241744,34.983195128235,122.419137958029)) ;
#23193=CARTESIAN_POINT('Ctrl Pts',(-20.3047188071783,34.8032060478722,122.170959918835)) ;
#23194=CARTESIAN_POINT('Ctrl Pts',(-20.4220114238497,35.0031782031124,122.723491321835)) ;
#23195=CARTESIAN_POINT('Ctrl Pts',(-20.6751904640124,34.8231891227495,122.55139832022)) ;
#23196=CARTESIAN_POINT('Ctrl Pts',(-20.5955208583163,35.0230872857583,123.109625284551)) ;
#23197=CARTESIAN_POINT('Ctrl Pts',(-20.8920819873269,34.8430982053954,123.034062768714)) ;
#23198=CARTESIAN_POINT('Ctrl Pts',(-20.6279870536071,35.0429458448811,123.530675885179)) ;
#23199=CARTESIAN_POINT('Ctrl Pts',(-20.9326680570592,34.8629567645182,123.560377307948)) ;
#23200=CARTESIAN_POINT('Ctrl Pts',(-20.5133192729208,35.0629892887198,123.941055703616)) ;
#23201=CARTESIAN_POINT('Ctrl Pts',(-20.7893451366516,34.8830002083569,124.073345382285)) ;
#23202=CARTESIAN_POINT('Ctrl Pts',(-20.3093835063598,35.079489353449,124.226623757706)) ;
#23203=CARTESIAN_POINT('Ctrl Pts',(-20.5344079580577,34.8995002730861,124.43033347796)) ;
#23204=CARTESIAN_POINT('Ctrl Pts',(-20.092268777163,35.0928790932979,124.405758678577)) ;
#23205=CARTESIAN_POINT('Ctrl Pts',(-20.2630356079764,34.912890012935,124.654232063007)) ;
#23206=CARTESIAN_POINT('Ctrl Pts',(-19.9119702886458,35.1027359945063,124.507953316112)) ;
#23207=CARTESIAN_POINT('Ctrl Pts',(-20.0376601532639,34.9227469141434,124.781982024209)) ;
#23208=CARTESIAN_POINT('Ctrl Pts',(-19.7141970013292,35.1127275203528,124.578624517524)) ;
#23209=CARTESIAN_POINT('Ctrl Pts',(-19.7904462531825,34.9327384399899,124.870322609915)) ;
#23210=CARTESIAN_POINT('Ctrl Pts',(-19.5084940721676,35.1226522008037,124.613732527868)) ;
#23211=CARTESIAN_POINT('Ctrl Pts',(-19.5333148830126,34.9426631204409,124.914209741491)) ;
#23212=CARTESIAN_POINT('Ctrl Pts',(-19.2980655867416,35.1326627908481,124.612658643822)) ;
#23213=CARTESIAN_POINT('Ctrl Pts',(-19.2702905171994,34.9526737104853,124.912873328828)) ;
#23214=CARTESIAN_POINT('Ctrl Pts',(-19.0237133873326,35.1459220515518,124.563175266845)) ;
#23215=CARTESIAN_POINT('Ctrl Pts',(-18.9272936377873,34.9659329711889,124.851006430555)) ;
#23216=CARTESIAN_POINT('Ctrl Pts',(-18.7669990026085,35.1592731267021,124.442141475141)) ;
#23217=CARTESIAN_POINT('Ctrl Pts',(-18.606436005865,34.9792840463392,124.69972105366)) ;
#23218=CARTESIAN_POINT('Ctrl Pts',(-18.5548922307535,35.1724794359369,124.262885149978)) ;
#23219=CARTESIAN_POINT('Ctrl Pts',(-18.3413122765646,34.992490355574,124.475665673841)) ;
#23220=CARTESIAN_POINT('Ctrl Pts',(-18.4202016194479,35.1824662695272,124.101878407724)) ;
#23221=CARTESIAN_POINT('Ctrl Pts',(-18.1729444100433,35.0024771891643,124.274406568228)) ;
#23222=CARTESIAN_POINT('Ctrl Pts',(-18.3157421931826,35.1924189970233,123.920538588917)) ;
#23223=CARTESIAN_POINT('Ctrl Pts',(-18.0423683362087,35.0124299166604,124.047733829672)) ;
#23224=CARTESIAN_POINT('Ctrl Pts',(-18.243859696856,35.2024670938648,123.721927113406)) ;
#23225=CARTESIAN_POINT('Ctrl Pts',(-17.9525123755645,35.022478013502,123.799470169266)) ;
#23226=CARTESIAN_POINT('Ctrl Pts',(-18.2080532676477,35.2123085507367,123.518130094329)) ;
#23227=CARTESIAN_POINT('Ctrl Pts',(-17.9077516294115,35.0323194703738,123.544724476242)) ;
#23228=CARTESIAN_POINT('Ctrl Pts',(-18.2077298878391,35.2222948176502,123.308221872427)) ;
#23229=CARTESIAN_POINT('Ctrl Pts',(-17.9073445683786,35.0423057372873,123.282339109367)) ;
#23230=CARTESIAN_POINT('Ctrl Pts',(-18.2435874649064,35.2322314185506,123.102388357164)) ;
#23231=CARTESIAN_POINT('Ctrl Pts',(-17.9521637827218,35.0522423381877,123.025046666914)) ;
#23232=CARTESIAN_POINT('Ctrl Pts',(-18.3155310783834,35.2422813613376,122.903755486322)) ;
#23233=CARTESIAN_POINT('Ctrl Pts',(-18.0420906679866,35.0622922809748,122.776754559742)) ;
#23234=CARTESIAN_POINT('Ctrl Pts',(-18.4186601658913,35.2521315610234,122.724163217864)) ;
#23235=CARTESIAN_POINT('Ctrl Pts',(-18.1709996406622,35.0721424806605,122.552262724124)) ;
#23236=CARTESIAN_POINT('Ctrl Pts',(-18.5526102972871,35.2621044659555,122.562900255392)) ;
#23237=CARTESIAN_POINT('Ctrl Pts',(-18.3384352196694,35.0821153855926,122.350682137594)) ;
#23238=CARTESIAN_POINT('Ctrl Pts',(-18.7130161190752,35.2721028404351,122.427018538122)) ;
#23239=CARTESIAN_POINT('Ctrl Pts',(-18.5389407429953,35.0921137600722,122.180827804113)) ;
#23240=CARTESIAN_POINT('Ctrl Pts',(-18.8950233937213,35.2821230143051,122.320968913956)) ;
#23241=CARTESIAN_POINT('Ctrl Pts',(-18.7664484679922,35.1021339339422,122.048263316574)) ;
#23242=CARTESIAN_POINT('Ctrl Pts',(-19.0902785173193,35.2920240582471,122.248825467389)) ;
#23243=CARTESIAN_POINT('Ctrl Pts',(-19.0105165623716,35.1120349778842,121.958081319082)) ;
#23244=CARTESIAN_POINT('Ctrl Pts',(-19.2968437850745,35.3020128619714,122.211027115049)) ;
#23245=CARTESIAN_POINT('Ctrl Pts',(-19.2687227454526,35.1220237816085,121.910830619248)) ;
#23246=CARTESIAN_POINT('Ctrl Pts',(-19.5063361205008,35.3119783288032,122.209821899411)) ;
#23247=CARTESIAN_POINT('Ctrl Pts',(-19.5305882706686,35.1319892484403,121.909321300949)) ;
#23248=CARTESIAN_POINT('Ctrl Pts',(-19.7116863669934,35.3218818910762,122.244299443621)) ;
#23249=CARTESIAN_POINT('Ctrl Pts',(-19.7872767838356,35.1418928107133,121.952415553993)) ;
#23250=CARTESIAN_POINT('Ctrl Pts',(-19.9109411377999,35.3319425689542,122.31516138068)) ;
#23251=CARTESIAN_POINT('Ctrl Pts',(-20.0363461469721,35.1519534885913,122.040990349835)) ;
#23252=CARTESIAN_POINT('Ctrl Pts',(-20.0910169677187,35.3417828669036,122.417053554877)) ;
#23253=CARTESIAN_POINT('Ctrl Pts',(-20.2614426416287,35.1617937865408,122.168353377903)) ;
#23254=CARTESIAN_POINT('Ctrl Pts',(-20.2543967354931,35.3518458618131,122.551408724914)) ;
#23255=CARTESIAN_POINT('Ctrl Pts',(-20.4656690482286,35.1718567814502,122.33629520841)) ;
#23256=CARTESIAN_POINT('Ctrl Pts',(-20.389561216917,35.3617401559602,122.709546984576)) ;
#23257=CARTESIAN_POINT('Ctrl Pts',(-20.6346269466373,35.1817510755973,122.533966500745)) ;
#23258=CARTESIAN_POINT('Ctrl Pts',(-20.4961856714635,35.3716819536571,122.889282267769)) ;
#23259=CARTESIAN_POINT('Ctrl Pts',(-20.7679099510609,35.1916928732942,122.758634465352)) ;
#23260=CARTESIAN_POINT('Ctrl Pts',(-20.5705249428159,35.3816845311862,123.08601924968)) ;
#23261=CARTESIAN_POINT('Ctrl Pts',(-20.8608365588192,35.2016954508233,123.004554830575)) ;
#23262=CARTESIAN_POINT('Ctrl Pts',(-20.6093729379891,35.3917189951073,123.293356771096)) ;
#23263=CARTESIAN_POINT('Ctrl Pts',(-20.9093992123313,35.2117299147444,123.263726218813)) ;
#23264=CARTESIAN_POINT('Ctrl Pts',(-20.6119121965854,35.4015651336283,123.500344351237)) ;
#23265=CARTESIAN_POINT('Ctrl Pts',(-20.912575954229,35.2215760532655,123.522461220006)) ;
#23266=CARTESIAN_POINT('Ctrl Pts',(-20.5784797869807,35.4115463068653,123.707482594867)) ;
#23267=CARTESIAN_POINT('Ctrl Pts',(-20.8707879748683,35.2315572265025,123.781384610257)) ;
#23268=CARTESIAN_POINT('Ctrl Pts',(-20.5097340551168,35.4214986008226,123.905101498051)) ;
#23269=CARTESIAN_POINT('Ctrl Pts',(-20.7848581741263,35.2415095204597,124.028409346698)) ;
#23270=CARTESIAN_POINT('Ctrl Pts',(-20.4074763823881,35.4314973959572,124.088777449656)) ;
#23271=CARTESIAN_POINT('Ctrl Pts',(-20.6570382603351,35.2515083155943,124.258005618651)) ;
#23272=CARTESIAN_POINT('Ctrl Pts',(-20.2740486464451,35.441536504218,124.252287560575)) ;
#23273=CARTESIAN_POINT('Ctrl Pts',(-20.4902556612724,35.2615474238551,124.462394870675)) ;
#23274=CARTESIAN_POINT('Ctrl Pts',(-20.1179375824698,35.4513614456571,124.387557243279)) ;
#23275=CARTESIAN_POINT('Ctrl Pts',(-20.2951179160963,35.2713723652943,124.631484396849)) ;
#23276=CARTESIAN_POINT('Ctrl Pts',(-19.9367669407761,35.4614161327315,124.496432561187)) ;
#23277=CARTESIAN_POINT('Ctrl Pts',(-20.0686559821828,35.2814270523687,124.767580615175)) ;
#23278=CARTESIAN_POINT('Ctrl Pts',(-19.7414940311369,35.4713589376717,124.571026731004)) ;
#23279=CARTESIAN_POINT('Ctrl Pts',(-19.8245654449264,35.2913698573088,124.860825828368)) ;
#23280=CARTESIAN_POINT('Ctrl Pts',(-19.5371642498936,35.4812627236682,124.611053711609)) ;
#23281=CARTESIAN_POINT('Ctrl Pts',(-19.5691531625667,35.3012736433053,124.910862029586)) ;
#23282=CARTESIAN_POINT('Ctrl Pts',(-19.3260021505189,35.491309540233,124.614922626693)) ;
#23283=CARTESIAN_POINT('Ctrl Pts',(-19.3052006854437,35.3113204598701,124.915700617854)) ;
#23284=CARTESIAN_POINT('Ctrl Pts',(-19.1204374563193,35.5012050597117,124.582740242867)) ;
#23285=CARTESIAN_POINT('Ctrl Pts',(-19.0482438728121,35.3212159793488,124.875474923149)) ;
#23286=CARTESIAN_POINT('Ctrl Pts',(-18.9203301984494,35.5112671450361,124.514241085289)) ;
#23287=CARTESIAN_POINT('Ctrl Pts',(-18.7981091918514,35.3312780646732,124.789853312718)) ;
#23288=CARTESIAN_POINT('Ctrl Pts',(-18.7390904234207,35.521109855994,124.414343573593)) ;
#23289=CARTESIAN_POINT('Ctrl Pts',(-18.571557569673,35.3411207756312,124.664983089902)) ;
#23290=CARTESIAN_POINT('Ctrl Pts',(-18.575252732091,35.5311005733001,124.282960921875)) ;
#23291=CARTESIAN_POINT('Ctrl Pts',(-18.3667589020139,35.3511114929372,124.500756432804)) ;
#23292=CARTESIAN_POINT('Ctrl Pts',(-18.4375879398549,35.5410286563966,124.126065100434)) ;
#23293=CARTESIAN_POINT('Ctrl Pts',(-18.1946758847601,35.3610395760338,124.304637787655)) ;
#23294=CARTESIAN_POINT('Ctrl Pts',(-18.3282912493656,35.5510165865084,123.94676509158)) ;
#23295=CARTESIAN_POINT('Ctrl Pts',(-18.0580530664321,35.3710275061455,124.080513754998)) ;
#23296=CARTESIAN_POINT('Ctrl Pts',(-18.2517565825726,35.5610524126357,123.750158377981)) ;
#23297=CARTESIAN_POINT('Ctrl Pts',(-17.9623826480587,35.3810633322728,123.83475626619)) ;
#23298=CARTESIAN_POINT('Ctrl Pts',(-18.2109351619,35.5709077497493,123.547017923555)) ;
#23299=CARTESIAN_POINT('Ctrl Pts',(-17.9113535514333,35.3909186693864,123.580830234499)) ;
#23300=CARTESIAN_POINT('Ctrl Pts',(-18.2056029932862,35.5809054845995,123.336924382834)) ;
#23301=CARTESIAN_POINT('Ctrl Pts',(-17.9046862415223,35.4009164042366,123.318213209581)) ;
#23302=CARTESIAN_POINT('Ctrl Pts',(-18.2364854342571,35.5908133885839,123.130921758617)) ;
#23303=CARTESIAN_POINT('Ctrl Pts',(-17.9432873405184,35.4108243082211,123.060708970242)) ;
#23304=CARTESIAN_POINT('Ctrl Pts',(-18.3030212952615,35.6008244631324,122.931244855466)) ;
#23305=CARTESIAN_POINT('Ctrl Pts',(-18.0264553068263,35.4208353827695,122.811112169827)) ;
#23306=CARTESIAN_POINT('Ctrl Pts',(-18.4037616999809,35.610852318668,122.746053058714)) ;
#23307=CARTESIAN_POINT('Ctrl Pts',(-18.1523789389796,35.4308632383051,122.579621476818)) ;
#23308=CARTESIAN_POINT('Ctrl Pts',(-18.532602474964,35.6207099125732,122.583737923954)) ;
#23309=CARTESIAN_POINT('Ctrl Pts',(-18.3134289650525,35.4407208322104,122.376725539727)) ;
#23310=CARTESIAN_POINT('Ctrl Pts',(-18.6900489868914,35.6307365994113,122.443575063873)) ;
#23311=CARTESIAN_POINT('Ctrl Pts',(-18.5102358433116,35.4507475190485,122.201520587918)) ;
#23312=CARTESIAN_POINT('Ctrl Pts',(-18.8697550672844,35.6407652685651,122.333303125857)) ;
#23313=CARTESIAN_POINT('Ctrl Pts',(-18.7348673255698,35.4607761882022,122.063678979707)) ;
#23314=CARTESIAN_POINT('Ctrl Pts',(-19.0621320904684,35.6506104768465,122.256973154102)) ;
#23315=CARTESIAN_POINT('Ctrl Pts',(-18.9753389392073,35.4706213964836,121.968264330612)) ;
#23316=CARTESIAN_POINT('Ctrl Pts',(-19.2677365853568,35.6606011658096,122.214031607131)) ;
#23317=CARTESIAN_POINT('Ctrl Pts',(-19.232344395239,35.4806120854467,121.914585662056)) ;
#23318=CARTESIAN_POINT('Ctrl Pts',(-19.4786728867515,35.6706390420919,122.207881553144)) ;
#23319=CARTESIAN_POINT('Ctrl Pts',(-19.4960145845419,35.490649961729,121.906896220203)) ;
#23320=CARTESIAN_POINT('Ctrl Pts',(-19.6835091491884,35.6804834197341,122.237505000338)) ;
#23321=CARTESIAN_POINT('Ctrl Pts',(-19.7520613231325,35.5004943393712,121.943923950967)) ;
#23322=CARTESIAN_POINT('Ctrl Pts',(-19.8829904576665,35.6904682241255,122.302762495252)) ;
#23323=CARTESIAN_POINT('Ctrl Pts',(-20.0014137029836,35.5104791437627,122.025494346825)) ;
#23324=CARTESIAN_POINT('Ctrl Pts',(-20.0673637367163,35.7004077543441,122.401163727744)) ;
#23325=CARTESIAN_POINT('Ctrl Pts',(-20.2318815338735,35.5204186739812,122.148494733348)) ;
#23326=CARTESIAN_POINT('Ctrl Pts',(-20.2334425789832,35.710447442381,122.531393346306)) ;
#23327=CARTESIAN_POINT('Ctrl Pts',(-20.4394809697131,35.5304583620181,122.311280393352)) ;
#23328=CARTESIAN_POINT('Ctrl Pts',(-20.3723559056366,35.7203357317493,122.686064760268)) ;
#23329=CARTESIAN_POINT('Ctrl Pts',(-20.6131244207075,35.5403466513864,122.504619288811)) ;
#23330=CARTESIAN_POINT('Ctrl Pts',(-20.4837508188583,35.7303248554341,122.864079606437)) ;
#23331=CARTESIAN_POINT('Ctrl Pts',(-20.7523694041922,35.5503357750712,122.72713725888)) ;
#23332=CARTESIAN_POINT('Ctrl Pts',(-20.5621646542934,35.7402848651087,123.058229679049)) ;
#23333=CARTESIAN_POINT('Ctrl Pts',(-20.8503882560538,35.5602957847458,122.969824688647)) ;
#23334=CARTESIAN_POINT('Ctrl Pts',(-20.6059033424676,35.7501852948129,123.261726613465)) ;
#23335=CARTESIAN_POINT('Ctrl Pts',(-20.9050630989688,35.57019621445,123.224196430447)) ;
#23336=CARTESIAN_POINT('Ctrl Pts',(-20.6137449772283,35.7602283762197,123.472709317713)) ;
#23337=CARTESIAN_POINT('Ctrl Pts',(-20.9148664709882,35.5802392958568,123.487924566708)) ;
#23338=CARTESIAN_POINT('Ctrl Pts',(-20.5852260061574,35.7701357701273,123.67904320518)) ;
#23339=CARTESIAN_POINT('Ctrl Pts',(-20.8792189654738,35.5901466897644,123.74584291802)) ;
#23340=CARTESIAN_POINT('Ctrl Pts',(-20.5210141564566,35.7801475011165,123.879489186249)) ;
#23341=CARTESIAN_POINT('Ctrl Pts',(-20.7989552795368,35.6001584207536,123.996400804876)) ;
#23342=CARTESIAN_POINT('Ctrl Pts',(-20.4224008662751,35.7901797188313,124.06593183367)) ;
#23343=CARTESIAN_POINT('Ctrl Pts',(-20.6756899073301,35.6101906384684,124.229454654533)) ;
#23344=CARTESIAN_POINT('Ctrl Pts',(-20.2954649937383,35.8000322280774,124.229594024067)) ;
#23345=CARTESIAN_POINT('Ctrl Pts',(-20.5170202759795,35.6200431477146,124.434034154075)) ;
#23346=CARTESIAN_POINT('Ctrl Pts',(-20.1408226833668,35.8099901646204,124.370712894289)) ;
#23347=CARTESIAN_POINT('Ctrl Pts',(-20.3237177193579,35.6300010842576,124.610433802406)) ;
#23348=CARTESIAN_POINT('Ctrl Pts',(-19.9624034194556,35.8200290346287,124.483417161163)) ;
#23349=CARTESIAN_POINT('Ctrl Pts',(-20.1006943914862,35.6400399542659,124.751315017522)) ;
#23350=CARTESIAN_POINT('Ctrl Pts',(-19.7704532057316,35.829902189787,124.56248627394)) ;
#23351=CARTESIAN_POINT('Ctrl Pts',(-19.8607559657353,35.6499131094241,124.850152762012)) ;
#23352=CARTESIAN_POINT('Ctrl Pts',(-19.5636408193586,35.8399754646367,124.607848543225)) ;
#23353=CARTESIAN_POINT('Ctrl Pts',(-19.6022411196816,35.6599863842738,124.906856510779)) ;
#23354=CARTESIAN_POINT('Ctrl Pts',(-19.3573296065172,35.8497957818141,124.616666849155)) ;
#23355=CARTESIAN_POINT('Ctrl Pts',(-19.3443505908473,35.6698067014512,124.917880380727)) ;
#23356=CARTESIAN_POINT('Ctrl Pts',(-19.1473070231254,35.8598744676076,124.58902082137)) ;
#23357=CARTESIAN_POINT('Ctrl Pts',(-19.0818227174019,35.6798853872447,124.883323751729)) ;
#23358=CARTESIAN_POINT('Ctrl Pts',(-18.9497113689918,35.8697259789907,124.526804413324)) ;
#23359=CARTESIAN_POINT('Ctrl Pts',(-18.8348266453424,35.6897368986278,124.805553629414)) ;
#23360=CARTESIAN_POINT('Ctrl Pts',(-18.7617765756378,35.8797994252973,124.429271647714)) ;
#23361=CARTESIAN_POINT('Ctrl Pts',(-18.5999081950905,35.6998103449344,124.683638544709)) ;
#23362=CARTESIAN_POINT('Ctrl Pts',(-18.597467101793,35.889640700422,124.303505365942)) ;
#23363=CARTESIAN_POINT('Ctrl Pts',(-18.3945197612094,35.7096516200591,124.526430434708)) ;
#23364=CARTESIAN_POINT('Ctrl Pts',(-18.4549920931084,35.8996258000788,124.149368497595)) ;
#23365=CARTESIAN_POINT('Ctrl Pts',(-18.2164254320828,35.7196367197159,124.333759479541)) ;
#23366=CARTESIAN_POINT('Ctrl Pts',(-18.3414173666157,35.9096332762131,123.972250384681)) ;
#23367=CARTESIAN_POINT('Ctrl Pts',(-18.0744564633631,35.7296441958502,124.112362113073)) ;
#23368=CARTESIAN_POINT('Ctrl Pts',(-18.2608430560108,35.919555863922,123.779847146659)) ;
#23369=CARTESIAN_POINT('Ctrl Pts',(-17.9737377684653,35.7395667835592,123.871857563518)) ;
#23370=CARTESIAN_POINT('Ctrl Pts',(-18.2142645919712,35.9295424681954,123.575109420464)) ;
#23371=CARTESIAN_POINT('Ctrl Pts',(-17.915514233427,35.7495533878325,123.61593526692)) ;
#23372=CARTESIAN_POINT('Ctrl Pts',(-18.2042845382939,35.9395825965295,123.364287204911)) ;
#23373=CARTESIAN_POINT('Ctrl Pts',(-17.9030386020177,35.7595935161666,123.352407710946)) ;
#23374=CARTESIAN_POINT('Ctrl Pts',(-18.2300836682839,35.9494220310629,123.159025741679)) ;
#23375=CARTESIAN_POINT('Ctrl Pts',(-17.9352873093838,35.7694329507,123.095829361004)) ;
#23376=CARTESIAN_POINT('Ctrl Pts',(-18.2923429640459,35.9594860855539,122.956842133847)) ;
#23377=CARTESIAN_POINT('Ctrl Pts',(-18.0131110083021,35.779497005191,122.843100123072)) ;
#23378=CARTESIAN_POINT('Ctrl Pts',(-18.3872080620054,35.969377004791,122.771780131143)) ;
#23379=CARTESIAN_POINT('Ctrl Pts',(-18.1316925352344,35.7893879244282,122.611771524711)) ;
#23380=CARTESIAN_POINT('Ctrl Pts',(-18.5136711614344,35.9793689980971,122.604062443733)) ;
#23381=CARTESIAN_POINT('Ctrl Pts',(-18.2897713917017,35.7993799177342,122.402124132987)) ;
#23382=CARTESIAN_POINT('Ctrl Pts',(-18.6670229740416,35.9893318620564,122.461407293779)) ;
#23383=CARTESIAN_POINT('Ctrl Pts',(-18.4814613118421,35.8093427816935,122.223804692162)) ;
#23384=CARTESIAN_POINT('Ctrl Pts',(-18.8415130358515,35.9992361218741,122.347760866079)) ;
#23385=CARTESIAN_POINT('Ctrl Pts',(-18.6995746479886,35.8192470415113,122.081746101379)) ;
#23386=CARTESIAN_POINT('Ctrl Pts',(-19.0361390397703,36.0092966124456,122.26503638611)) ;
#23387=CARTESIAN_POINT('Ctrl Pts',(-18.9428567780933,35.8293075320827,121.978340523878)) ;
#23388=CARTESIAN_POINT('Ctrl Pts',(-19.2376557259542,36.0191369620766,122.218129994328)) ;
#23389=CARTESIAN_POINT('Ctrl Pts',(-19.1947540652062,35.8391478817137,121.919707183759)) ;
#23390=CARTESIAN_POINT('Ctrl Pts',(-19.4488594057997,36.0291999375666,122.206420949229)) ;
#23391=CARTESIAN_POINT('Ctrl Pts',(-19.4587582959314,35.8492108572037,121.905070980687)) ;
#23392=CARTESIAN_POINT('Ctrl Pts',(-19.6553963029658,36.03909425771,122.231316246705)) ;
#23393=CARTESIAN_POINT('Ctrl Pts',(-19.716930430725,35.8591051773471,121.936190237955)) ;
#23394=CARTESIAN_POINT('Ctrl Pts',(-19.8555419191766,36.0490359708416,122.291429452583)) ;
#23395=CARTESIAN_POINT('Ctrl Pts',(-19.9671129941824,35.8690468904787,122.011332156098)) ;
#23396=CARTESIAN_POINT('Ctrl Pts',(-20.0434534803591,36.0590388606357,122.385905221195)) ;
#23397=CARTESIAN_POINT('Ctrl Pts',(-20.2020024297301,35.8790497802728,122.129427167199)) ;
#23398=CARTESIAN_POINT('Ctrl Pts',(-20.2124564475029,36.0690787177962,122.512316557016)) ;
#23399=CARTESIAN_POINT('Ctrl Pts',(-20.4132559197395,35.8890896374333,122.28744132461)) ;
#23400=CARTESIAN_POINT('Ctrl Pts',(-20.3542066989014,36.0789028986338,122.662550738687)) ;
#23401=CARTESIAN_POINT('Ctrl Pts',(-20.5904446049363,35.8989138182709,122.475235422024)) ;
#23402=CARTESIAN_POINT('Ctrl Pts',(-20.4706332696789,36.088959872137,122.839015977808)) ;
#23403=CARTESIAN_POINT('Ctrl Pts',(-20.7359772784035,35.9089707917741,122.695816923843)) ;
#23404=CARTESIAN_POINT('Ctrl Pts',(-20.5533425088199,36.0988879963241,123.030662056921)) ;
#23405=CARTESIAN_POINT('Ctrl Pts',(-20.8393638309279,35.9188989159612,122.935375322683)) ;
#23406=CARTESIAN_POINT('Ctrl Pts',(-20.6021853906492,36.1088416913975,123.234141443748)) ;
#23407=CARTESIAN_POINT('Ctrl Pts',(-20.9004170383969,35.9288526110346,123.189725205683)) ;
#23408=CARTESIAN_POINT('Ctrl Pts',(-20.6147732903502,36.1188878849728,123.444966785403)) ;
#23409=CARTESIAN_POINT('Ctrl Pts',(-20.9161514803797,35.9388988046099,123.453256665995)) ;
#23410=CARTESIAN_POINT('Ctrl Pts',(-20.5912389874168,36.1287359873327,123.65066140107)) ;
#23411=CARTESIAN_POINT('Ctrl Pts',(-20.8867329496708,35.9487469069698,123.710376268567)) ;
#23412=CARTESIAN_POINT('Ctrl Pts',(-20.5322920817203,36.1386975755603,123.851608665551)) ;
#23413=CARTESIAN_POINT('Ctrl Pts',(-20.813048468652,35.9587084951974,123.961560575043)) ;
#23414=CARTESIAN_POINT('Ctrl Pts',(-20.4384766708263,36.1487262457165,124.040434185181)) ;
#23415=CARTESIAN_POINT('Ctrl Pts',(-20.6957786698797,35.9687371653537,124.19759210035)) ;
#23416=CARTESIAN_POINT('Ctrl Pts',(-20.3148448154568,36.1586365485983,124.208121309133)) ;
#23417=CARTESIAN_POINT('Ctrl Pts',(-20.5412377893036,35.9786474682354,124.407201312219)) ;
#23418=CARTESIAN_POINT('Ctrl Pts',(-20.1639673049378,36.1685714324062,124.352558297041)) ;
#23419=CARTESIAN_POINT('Ctrl Pts',(-20.3526398125085,35.9885823520433,124.587747365873)) ;
#23420=CARTESIAN_POINT('Ctrl Pts',(-19.9883464931502,36.1786125740968,124.4696744726)) ;
#23421=CARTESIAN_POINT('Ctrl Pts',(-20.1331135059456,35.9986234937339,124.734141809642)) ;
#23422=CARTESIAN_POINT('Ctrl Pts',(-19.7980654386768,36.1884996952608,124.553357993941)) ;
#23423=CARTESIAN_POINT('Ctrl Pts',(-19.8952608881985,36.0085106148979,124.838745840386)) ;
#23424=CARTESIAN_POINT('Ctrl Pts',(-19.5941039539844,36.1984920381093,124.603590833534)) ;
#23425=CARTESIAN_POINT('Ctrl Pts',(-19.6403085962477,36.0185029577464,124.901535971408)) ;
#23426=CARTESIAN_POINT('Ctrl Pts',(-19.3854139464057,36.2084403393333,124.617526696654)) ;
#23427=CARTESIAN_POINT('Ctrl Pts',(-19.3794454821469,36.0284512589704,124.918954868183)) ;
#23428=CARTESIAN_POINT('Ctrl Pts',(-19.1776885830865,36.2183779170154,124.595344537768)) ;
#23429=CARTESIAN_POINT('Ctrl Pts',(-19.1197882532334,36.0383888366525,124.8912260194)) ;
#23430=CARTESIAN_POINT('Ctrl Pts',(-18.9758949839322,36.228364491466,124.537343966283)) ;
#23431=CARTESIAN_POINT('Ctrl Pts',(-18.8675463523897,36.0483754111031,124.818724120264)) ;
#23432=CARTESIAN_POINT('Ctrl Pts',(-18.7865605948736,36.2383933013744,124.444585421192)) ;
#23433=CARTESIAN_POINT('Ctrl Pts',(-18.6308789216368,36.0584042210115,124.702775017872)) ;
#23434=CARTESIAN_POINT('Ctrl Pts',(-18.6186460163788,36.2482716226812,124.322389246568)) ;
#23435=CARTESIAN_POINT('Ctrl Pts',(-18.4209855121877,36.0682825423183,124.550028242115)) ;
#23436=CARTESIAN_POINT('Ctrl Pts',(-18.4724839475725,36.2582632700286,124.171514768616)) ;
#23437=CARTESIAN_POINT('Ctrl Pts',(-18.2382837456184,36.0782741896657,124.361434085726)) ;
#23438=CARTESIAN_POINT('Ctrl Pts',(-18.3546005152364,36.2682977934664,123.996579143374)) ;
#23439=CARTESIAN_POINT('Ctrl Pts',(-18.0909304837619,36.0883087131035,124.142763989122)) ;
#23440=CARTESIAN_POINT('Ctrl Pts',(-18.2699376189153,36.278161150345,123.80726784102)) ;
#23441=CARTESIAN_POINT('Ctrl Pts',(-17.9851026047473,36.0981720699821,123.906123266323)) ;
#23442=CARTESIAN_POINT('Ctrl Pts',(-18.2183426275422,36.2882313770253,123.601966412164)) ;
#23443=CARTESIAN_POINT('Ctrl Pts',(-17.9206102595099,36.1082422966624,123.649496524002)) ;
#23444=CARTESIAN_POINT('Ctrl Pts',(-18.2035300755518,36.2980736851599,123.395572554759)) ;
#23445=CARTESIAN_POINT('Ctrl Pts',(-17.9020958099089,36.1180846047971,123.391502808904)) ;
#23446=CARTESIAN_POINT('Ctrl Pts',(-18.2242647172834,36.3080344171834,123.187200743274)) ;
#23447=CARTESIAN_POINT('Ctrl Pts',(-17.9280157514707,36.1280453368205,123.131037798645)) ;
#23448=CARTESIAN_POINT('Ctrl Pts',(-18.2817044009816,36.3180723063815,122.984147670972)) ;
#23449=CARTESIAN_POINT('Ctrl Pts',(-17.999816726095,36.1380832260186,122.877221984986)) ;
#23450=CARTESIAN_POINT('Ctrl Pts',(-18.3716994134048,36.3279465893003,122.797053220826)) ;
#23451=CARTESIAN_POINT('Ctrl Pts',(-18.1123123668843,36.1479575089374,122.643353698666)) ;
#23452=CARTESIAN_POINT('Ctrl Pts',(-18.4951890966193,36.3380163339178,122.625139380423)) ;
#23453=CARTESIAN_POINT('Ctrl Pts',(-18.2666755578384,36.1580272535549,122.428462610188)) ;
#23454=CARTESIAN_POINT('Ctrl Pts',(-18.6430502592492,36.3478496442634,122.480641003559)) ;
#23455=CARTESIAN_POINT('Ctrl Pts',(-18.4515040641022,36.1678605639005,122.247839904849)) ;
#23456=CARTESIAN_POINT('Ctrl Pts',(-18.8168167962975,36.3578798876161,122.361190643597)) ;
#23457=CARTESIAN_POINT('Ctrl Pts',(-18.6687131962433,36.1778908072532,122.098528505516)) ;
#23458=CARTESIAN_POINT('Ctrl Pts',(-19.0089931407264,36.3679121755945,122.274279269825)) ;
#23459=CARTESIAN_POINT('Ctrl Pts',(-18.9089342117129,36.1879230952316,121.98989079608)) ;
#23460=CARTESIAN_POINT('Ctrl Pts',(-19.2090377913951,36.3777393520626,122.222649776035)) ;
#23461=CARTESIAN_POINT('Ctrl Pts',(-19.1589917224903,36.1977502716997,121.925355327248)) ;
#23462=CARTESIAN_POINT('Ctrl Pts',(-19.4186819898018,36.3877447349294,122.205814654101)) ;
#23463=CARTESIAN_POINT('Ctrl Pts',(-19.4210472098018,36.2077556545666,121.904313326992)) ;
#23464=CARTESIAN_POINT('Ctrl Pts',(-19.6276479448215,36.3977273739222,122.225666562334)) ;
#23465=CARTESIAN_POINT('Ctrl Pts',(-19.6822546897857,36.2177382935593,121.929130110005)) ;
#23466=CARTESIAN_POINT('Ctrl Pts',(-19.831109521622,36.4077714410588,122.282077039624)) ;
#23467=CARTESIAN_POINT('Ctrl Pts',(-19.9365810271852,36.2277823606959,121.999644910744)) ;
#23468=CARTESIAN_POINT('Ctrl Pts',(-20.0176363662993,36.4175926598628,122.370629532132)) ;
#23469=CARTESIAN_POINT('Ctrl Pts',(-20.1697398906336,36.2376035794999,122.110337795579)) ;
#23470=CARTESIAN_POINT('Ctrl Pts',(-20.1899535608722,36.4276294988008,122.49240362926)) ;
#23471=CARTESIAN_POINT('Ctrl Pts',(-20.3851350977547,36.247640418438,122.262557053081)) ;
#23472=CARTESIAN_POINT('Ctrl Pts',(-20.3379053809418,36.4376539108986,122.642492380833)) ;
#23473=CARTESIAN_POINT('Ctrl Pts',(-20.5700735002195,36.2576648305357,122.450169309994)) ;
#23474=CARTESIAN_POINT('Ctrl Pts',(-20.4558677797191,36.4475059953039,122.812743968213)) ;
#23475=CARTESIAN_POINT('Ctrl Pts',(-20.7175254012894,36.267516914941,122.662985785925)) ;
#23476=CARTESIAN_POINT('Ctrl Pts',(-20.5439760773838,36.457496892047,123.003382833653)) ;
#23477=CARTESIAN_POINT('Ctrl Pts',(-20.827658912847,36.2775078116842,122.901285416374)) ;
#23478=CARTESIAN_POINT('Ctrl Pts',(-20.5973974591388,36.467414883948,123.20495630849)) ;
#23479=CARTESIAN_POINT('Ctrl Pts',(-20.894433698142,36.2874258035851,123.153253367672)) ;
#23480=CARTESIAN_POINT('Ctrl Pts',(-20.6152498950623,36.477442999405,123.415005149614)) ;
#23481=CARTESIAN_POINT('Ctrl Pts',(-20.9167470714456,36.2974539190421,123.415814568147)) ;
#23482=CARTESIAN_POINT('Ctrl Pts',(-20.5967150299844,36.4873281753471,123.621999291059)) ;
#23483=CARTESIAN_POINT('Ctrl Pts',(-20.8935762347595,36.3073390949842,123.674557784478)) ;
#23484=CARTESIAN_POINT('Ctrl Pts',(-20.5424427129043,36.497317533754,123.824877571005)) ;
#23485=CARTESIAN_POINT('Ctrl Pts',(-20.8257335492576,36.3173284533911,123.928155184694)) ;
#23486=CARTESIAN_POINT('Ctrl Pts',(-20.4529063543909,36.5073586813343,124.016044649924)) ;
#23487=CARTESIAN_POINT('Ctrl Pts',(-20.7138111338408,36.3273696009714,124.167113009814)) ;
#23488=CARTESIAN_POINT('Ctrl Pts',(-20.3343398025796,36.5171913043407,124.185369576253)) ;
#23489=CARTESIAN_POINT('Ctrl Pts',(-20.5656005075822,36.3372022239778,124.378768633685)) ;
#23490=CARTESIAN_POINT('Ctrl Pts',(-20.1861956020173,36.5271853754515,124.334353336419)) ;
#23491=CARTESIAN_POINT('Ctrl Pts',(-20.3804184420739,36.3471962950886,124.564996698335)) ;
#23492=CARTESIAN_POINT('Ctrl Pts',(-20.013585956424,36.5372140330923,124.455438892729)) ;
#23493=CARTESIAN_POINT('Ctrl Pts',(-20.1646550508293,36.3572249527295,124.716351716207)) ;
#23494=CARTESIAN_POINT('Ctrl Pts',(-19.8254390215131,36.5470983592851,124.543627316343)) ;
#23495=CARTESIAN_POINT('Ctrl Pts',(-19.9294697798766,36.3671092789223,124.82658534845)) ;
#23496=CARTESIAN_POINT('Ctrl Pts',(-19.6233034874049,36.5570641027758,124.598757212987)) ;
#23497=CARTESIAN_POINT('Ctrl Pts',(-19.6767994745705,36.3770750224129,124.895495364823)) ;
#23498=CARTESIAN_POINT('Ctrl Pts',(-19.4133432163963,36.567092481907,124.617767958151)) ;
#23499=CARTESIAN_POINT('Ctrl Pts',(-19.4143489319624,36.3871034015441,124.91925636217)) ;
#23500=CARTESIAN_POINT('Ctrl Pts',(-19.2058808015427,36.5769933281139,124.600571301318)) ;
#23501=CARTESIAN_POINT('Ctrl Pts',(-19.1550206095445,36.397004247751,124.897758003346)) ;
#23502=CARTESIAN_POINT('Ctrl Pts',(-19.0014191299385,36.587051985531,124.546729537717)) ;
#23503=CARTESIAN_POINT('Ctrl Pts',(-18.8994442732755,36.4070629051681,124.830453416065)) ;
#23504=CARTESIAN_POINT('Ctrl Pts',(-18.813096638073,36.5969095483129,124.460143866391)) ;
#23505=CARTESIAN_POINT('Ctrl Pts',(-18.6640416210879,36.41692046795,124.722218749263)) ;
#23506=CARTESIAN_POINT('Ctrl Pts',(-18.6390013358373,36.6069779508661,124.339804591474)) ;
#23507=CARTESIAN_POINT('Ctrl Pts',(-18.4464240794683,36.4269888705032,124.571792635111)) ;
#23508=CARTESIAN_POINT('Ctrl Pts',(-18.4916105941839,36.6168333496057,124.194162637956)) ;
#23509=CARTESIAN_POINT('Ctrl Pts',(-18.2621870024575,36.4368442692428,124.389737932051)) ;
#23510=CARTESIAN_POINT('Ctrl Pts',(-18.3695504756262,36.6268282166796,124.023135375574)) ;
#23511=CARTESIAN_POINT('Ctrl Pts',(-18.1096139658518,36.4468391363167,124.175952224907)) ;
#23512=CARTESIAN_POINT('Ctrl Pts',(-18.2791165716848,36.636859511663,123.832615497264)) ;
#23513=CARTESIAN_POINT('Ctrl Pts',(-17.9965739248701,36.4568704313002,123.937801266144)) ;
#23514=CARTESIAN_POINT('Ctrl Pts',(-18.2237360833858,36.6467260363896,123.632712396887)) ;
#23515=CARTESIAN_POINT('Ctrl Pts',(-17.9273507223424,36.4667369560267,123.68792118455)) ;
#23516=CARTESIAN_POINT('Ctrl Pts',(-18.2033310226805,36.6567135070853,123.423763661605)) ;
#23517=CARTESIAN_POINT('Ctrl Pts',(-17.9018470654154,36.4767244267224,123.426734881173)) ;
#23518=CARTESIAN_POINT('Ctrl Pts',(-18.2193352845113,36.6666582666492,123.215274762374)) ;
#23519=CARTESIAN_POINT('Ctrl Pts',(-17.9218551058738,36.4866691862863,123.166123729046)) ;
#23520=CARTESIAN_POINT('Ctrl Pts',(-18.2719370323567,36.676703822598,123.010765439361)) ;
#23521=CARTESIAN_POINT('Ctrl Pts',(-17.9876098911621,36.4967147422351,122.910487765929)) ;
#23522=CARTESIAN_POINT('Ctrl Pts',(-18.3574522060071,36.6865634109731,122.82192143973)) ;
#23523=CARTESIAN_POINT('Ctrl Pts',(-18.0945065089563,36.5065743306102,122.674433491217)) ;
#23524=CARTESIAN_POINT('Ctrl Pts',(-18.4758403465642,36.6965643661092,122.648211025078)) ;
#23525=CARTESIAN_POINT('Ctrl Pts',(-18.2424940102238,36.5165752857463,122.457296954355)) ;
#23526=CARTESIAN_POINT('Ctrl Pts',(-18.6211027599908,36.7064685933867,122.49899007134)) ;
#23527=CARTESIAN_POINT('Ctrl Pts',(-18.4240741922966,36.5264795130239,122.270772500049)) ;
#23528=CARTESIAN_POINT('Ctrl Pts',(-18.7923364863628,36.7165106702819,122.37555164078)) ;
#23529=CARTESIAN_POINT('Ctrl Pts',(-18.6381179777294,36.536521589919,122.116476705951)) ;
#23530=CARTESIAN_POINT('Ctrl Pts',(-18.9798717838469,36.726418282968,122.28482859885)) ;
#23531=CARTESIAN_POINT('Ctrl Pts',(-18.8725385168482,36.5464292026052,122.003075302597)) ;
#23532=CARTESIAN_POINT('Ctrl Pts',(-19.1832128493394,36.7364728135838,122.227207958605)) ;
#23533=CARTESIAN_POINT('Ctrl Pts',(-19.1267156102874,36.5564837332209,121.931052177972)) ;
#23534=CARTESIAN_POINT('Ctrl Pts',(-19.3894625931079,36.7463336001326,122.206055828831)) ;
#23535=CARTESIAN_POINT('Ctrl Pts',(-19.3845283469667,36.5663445197698,121.904614760594)) ;
#23536=CARTESIAN_POINT('Ctrl Pts',(-19.5990077419193,36.7563273552037,122.220846428092)) ;
#23537=CARTESIAN_POINT('Ctrl Pts',(-19.646459660601,36.5763382748409,121.923105823683)) ;
#23538=CARTESIAN_POINT('Ctrl Pts',(-19.8014959540694,36.7662527154437,122.271364787942)) ;
#23539=CARTESIAN_POINT('Ctrl Pts',(-19.8995693751158,36.5862636350808,121.986256533974)) ;
#23540=CARTESIAN_POINT('Ctrl Pts',(-19.9940544316431,36.776280644839,122.357120402506)) ;
#23541=CARTESIAN_POINT('Ctrl Pts',(-20.1402663825485,36.5962915644761,122.093453651258)) ;
#23542=CARTESIAN_POINT('Ctrl Pts',(-20.1664982335649,36.7861669116383,122.473197134529)) ;
#23543=CARTESIAN_POINT('Ctrl Pts',(-20.3558196617263,36.6061778312754,122.23855197328)) ;
#23544=CARTESIAN_POINT('Ctrl Pts',(-20.3183982755101,36.7961986805365,122.619450743956)) ;
#23545=CARTESIAN_POINT('Ctrl Pts',(-20.5456928031172,36.6162096001737,122.421371062193)) ;
#23546=CARTESIAN_POINT('Ctrl Pts',(-20.4409436536401,36.8060802763801,122.787245264454)) ;
#23547=CARTESIAN_POINT('Ctrl Pts',(-20.6988722845905,36.6260911960173,122.631115950227)) ;
#23548=CARTESIAN_POINT('Ctrl Pts',(-20.5341804059787,36.8161421618481,122.977086052336)) ;
#23549=CARTESIAN_POINT('Ctrl Pts',(-20.815415738362,36.6361530814852,122.868418182703)) ;
#23550=CARTESIAN_POINT('Ctrl Pts',(-20.5919244424178,36.825999595867,123.176140531021)) ;
#23551=CARTESIAN_POINT('Ctrl Pts',(-20.8875930298801,36.6460105155041,123.11723735423)) ;
#23552=CARTESIAN_POINT('Ctrl Pts',(-20.6149712049277,36.8359928389089,123.384935530242)) ;
#23553=CARTESIAN_POINT('Ctrl Pts',(-20.9163988743177,36.6560037585461,123.37823043788)) ;
#23554=CARTESIAN_POINT('Ctrl Pts',(-20.6015124206239,36.8459235997953,123.593287168939)) ;
#23555=CARTESIAN_POINT('Ctrl Pts',(-20.8995719078508,36.6659345194324,123.638673612031)) ;
#23556=CARTESIAN_POINT('Ctrl Pts',(-20.5353308402502,36.8592725919925,123.866051377186)) ;
#23557=CARTESIAN_POINT('Ctrl Pts',(-20.8168446966216,36.6792835116296,123.979609103864)) ;
#23558=CARTESIAN_POINT('Ctrl Pts',(-20.3999609319661,36.8725409648089,124.11357862058)) ;
#23559=CARTESIAN_POINT('Ctrl Pts',(-20.6476556408436,36.692551884446,124.288994177467)) ;
#23560=CARTESIAN_POINT('Ctrl Pts',(-20.2075188150344,36.8858239061933,124.315902403528)) ;
#23561=CARTESIAN_POINT('Ctrl Pts',(-20.4070652076398,36.7058348258304,124.541941671544)) ;
#23562=CARTESIAN_POINT('Ctrl Pts',(-20.0375727801162,36.8958666920355,124.441171046121)) ;
#23563=CARTESIAN_POINT('Ctrl Pts',(-20.1946380684897,36.7158776116726,124.698516250031)) ;
#23564=CARTESIAN_POINT('Ctrl Pts',(-19.8521787979742,36.9057166345876,124.533432305183)) ;
#23565=CARTESIAN_POINT('Ctrl Pts',(-19.9628921814832,36.7257275542247,124.813842499232)) ;
#23566=CARTESIAN_POINT('Ctrl Pts',(-19.6507731123258,36.9157138675065,124.593480412264)) ;
#23567=CARTESIAN_POINT('Ctrl Pts',(-19.7111366687982,36.7357247871437,124.888900023742)) ;
#23568=CARTESIAN_POINT('Ctrl Pts',(-19.4415809415258,36.9257287628411,124.617367629168)) ;
#23569=CARTESIAN_POINT('Ctrl Pts',(-19.4496388355441,36.7457396824782,124.918754107173)) ;
#23570=CARTESIAN_POINT('Ctrl Pts',(-19.1637149095619,36.9389684394793,124.600711262707)) ;
#23571=CARTESIAN_POINT('Ctrl Pts',(-19.1023419164485,36.7589793591164,124.897941856105)) ;
#23572=CARTESIAN_POINT('Ctrl Pts',(-18.8297170296114,36.9555156638846,124.490312279794)) ;
#23573=CARTESIAN_POINT('Ctrl Pts',(-18.6847931249913,36.7755265835217,124.759912521952)) ;
#23574=CARTESIAN_POINT('Ctrl Pts',(-18.5515569849989,36.9721631010157,124.271299498721)) ;
#23575=CARTESIAN_POINT('Ctrl Pts',(-18.3371603330514,36.7921740206528,124.486198909286)) ;
#23576=CARTESIAN_POINT('Ctrl Pts',(-18.3844875359923,36.9854525984939,124.047410122767)) ;
#23577=CARTESIAN_POINT('Ctrl Pts',(-18.1282776888068,36.805463518131,124.206288377136)) ;
#23578=CARTESIAN_POINT('Ctrl Pts',(-18.2905524045651,36.9953260063163,123.862298699992)) ;
#23579=CARTESIAN_POINT('Ctrl Pts',(-18.0108710102114,36.8153369259534,123.974907927257)) ;
#23580=CARTESIAN_POINT('Ctrl Pts',(-18.2290667315247,37.005378383909,123.660120832007)) ;
#23581=CARTESIAN_POINT('Ctrl Pts',(-17.9340138084422,36.8253893035461,123.722181735766)) ;
#23582=CARTESIAN_POINT('Ctrl Pts',(-18.2040801154488,37.0152820374499,123.45340205248)) ;
#23583=CARTESIAN_POINT('Ctrl Pts',(-17.9027830695279,36.835292957087,123.463785283055)) ;
#23584=CARTESIAN_POINT('Ctrl Pts',(-18.214904553946,37.0252263064452,123.244652571559)) ;
#23585=CARTESIAN_POINT('Ctrl Pts',(-17.9163185741068,36.8452372260823,123.20284412538)) ;
#23586=CARTESIAN_POINT('Ctrl Pts',(-18.2776834319682,37.0385573147779,122.97143393021)) ;
#23587=CARTESIAN_POINT('Ctrl Pts',(-17.9947816309639,36.858568234415,122.86134409118)) ;
#23588=CARTESIAN_POINT('Ctrl Pts',(-18.4435275534842,37.0551788953021,122.659444683358)) ;
#23589=CARTESIAN_POINT('Ctrl Pts',(-18.2021201495934,36.8751898149393,122.471324046481)) ;
#23590=CARTESIAN_POINT('Ctrl Pts',(-18.704290384894,37.0717215660005,122.423272162924)) ;
#23591=CARTESIAN_POINT('Ctrl Pts',(-18.5280140338344,36.8917324856377,122.176159129624)) ;
#23592=CARTESIAN_POINT('Ctrl Pts',(-18.9539020590981,37.0850707255635,122.295120923871)) ;
#23593=CARTESIAN_POINT('Ctrl Pts',(-18.8400831149496,36.9050816452006,122.015936356967)) ;
#23594=CARTESIAN_POINT('Ctrl Pts',(-19.2195445907984,37.098298875723,122.212649877143)) ;
#23595=CARTESIAN_POINT('Ctrl Pts',(-19.1721122727388,36.9183097953601,121.912858361427)) ;
#23596=CARTESIAN_POINT('Ctrl Pts',(-19.5728022237674,37.1149295528605,122.198387297674)) ;
#23597=CARTESIAN_POINT('Ctrl Pts',(-19.6137036972869,36.9349404724976,121.895030598863)) ;
#23598=CARTESIAN_POINT('Ctrl Pts',(-19.9761409789066,37.1348324921486,122.326670598827)) ;
#23599=CARTESIAN_POINT('Ctrl Pts',(-20.1178689307979,36.9548434117857,122.055389405996)) ;
#23600=CARTESIAN_POINT('Ctrl Pts',(-20.3116476022959,37.1547353587518,122.584460179412)) ;
#23601=CARTESIAN_POINT('Ctrl Pts',(-20.5372508618261,36.974746278389,122.377628584719)) ;
#23602=CARTESIAN_POINT('Ctrl Pts',(-20.539804233534,37.1746485238567,122.941249904607)) ;
#23603=CARTESIAN_POINT('Ctrl Pts',(-20.8224429652518,36.9946594434938,122.823616943194)) ;
#23604=CARTESIAN_POINT('Ctrl Pts',(-20.6323994014347,37.194684352998,123.35701958835)) ;
#23605=CARTESIAN_POINT('Ctrl Pts',(-20.9381837029395,37.0146952726351,123.343330198138)) ;
#23606=CARTESIAN_POINT('Ctrl Pts',(-20.5783831690263,37.2145029278761,123.775043446031)) ;
#23607=CARTESIAN_POINT('Ctrl Pts',(-20.870660430698,37.0345138475132,123.865857791706)) ;
#23608=CARTESIAN_POINT('Ctrl Pts',(-20.3841900567002,37.2344732289181,124.152499639715)) ;
#23609=CARTESIAN_POINT('Ctrl Pts',(-20.6279168053025,37.0544841485552,124.337676429547)) ;
#23610=CARTESIAN_POINT('Ctrl Pts',(-20.0739514395831,37.2543647612826,124.440192864302)) ;
#23611=CARTESIAN_POINT('Ctrl Pts',(-20.2401177850533,37.0743756809197,124.697290350133)) ;
#23612=CARTESIAN_POINT('Ctrl Pts',(-19.6816910451499,37.2743878590991,124.605446609559)) ;
#23613=CARTESIAN_POINT('Ctrl Pts',(-19.7497910668488,37.0943987787363,124.90385539926)) ;
#23614=CARTESIAN_POINT('Ctrl Pts',(-19.2612575086077,37.2941846120191,124.626987367423)) ;
#23615=CARTESIAN_POINT('Ctrl Pts',(-19.2242516782472,37.1141955316562,124.930779156354)) ;
#23616=CARTESIAN_POINT('Ctrl Pts',(-18.8551235164096,37.3141457005079,124.503854762639)) ;
#23617=CARTESIAN_POINT('Ctrl Pts',(-18.7165851062784,37.134156620145,124.77686253658)) ;
#23618=CARTESIAN_POINT('Ctrl Pts',(-18.5155691321444,37.33412396944,124.248549659237)) ;
#23619=CARTESIAN_POINT('Ctrl Pts',(-18.2921431805836,37.1541348890772,124.457730120068)) ;
#23620=CARTESIAN_POINT('Ctrl Pts',(-18.2848840893229,37.353943984231,123.895912818502)) ;
#23621=CARTESIAN_POINT('Ctrl Pts',(-18.0037890981737,37.1739549038682,124.016935959716)) ;
#23622=CARTESIAN_POINT('Ctrl Pts',(-18.1867266757181,37.3738823934829,123.483465881593)) ;
#23623=CARTESIAN_POINT('Ctrl Pts',(-17.8810922820256,37.19389331312,123.50137832524)) ;
#23624=CARTESIAN_POINT('Ctrl Pts',(-18.2364290835758,37.3939295108753,123.060063699983)) ;
#23625=CARTESIAN_POINT('Ctrl Pts',(-17.9432206011059,37.2139404305124,122.97212475137)) ;
#23626=CARTESIAN_POINT('Ctrl Pts',(-18.425848548575,37.4137757567091,122.683031202947)) ;
#23627=CARTESIAN_POINT('Ctrl Pts',(-18.1799938362226,37.2337866763463,122.500836491877)) ;
#23628=CARTESIAN_POINT('Ctrl Pts',(-18.7315064002048,37.4336247252212,122.391977885503)) ;
#23629=CARTESIAN_POINT('Ctrl Pts',(-18.5620635941251,37.2536356448583,122.137020325925)) ;
#23630=CARTESIAN_POINT('Ctrl Pts',(-19.1222176535589,37.4536750275325,122.221508253603)) ;
#23631=CARTESIAN_POINT('Ctrl Pts',(-19.0504528465872,37.2736859471696,121.923931865139)) ;
#23632=CARTESIAN_POINT('Ctrl Pts',(-19.5432296563708,37.4735099499637,122.194969642124)) ;
#23633=CARTESIAN_POINT('Ctrl Pts',(-19.5767155011093,37.2935208696008,121.890757346003)) ;
#23634=CARTESIAN_POINT('Ctrl Pts',(-19.9499494548822,37.4934403511896,122.313396694246)) ;
#23635=CARTESIAN_POINT('Ctrl Pts',(-20.08511494409,37.3134512708267,122.038788804448)) ;
#23636=CARTESIAN_POINT('Ctrl Pts',(-20.2916433860762,37.5133252965484,122.562694249305)) ;
#23637=CARTESIAN_POINT('Ctrl Pts',(-20.5122328950149,37.3333362161856,122.35040788788)) ;
#23638=CARTESIAN_POINT('Ctrl Pts',(-20.5292680047328,37.5333979046998,122.917125700607)) ;
#23639=CARTESIAN_POINT('Ctrl Pts',(-20.8092661802658,37.353408824337,122.793446550335)) ;
#23640=CARTESIAN_POINT('Ctrl Pts',(-20.6303478789093,37.5531892210279,123.325688691572)) ;
#23641=CARTESIAN_POINT('Ctrl Pts',(-20.9356180404718,37.3732001406651,123.304147384377)) ;
#23642=CARTESIAN_POINT('Ctrl Pts',(-20.5868633210281,37.5731540107952,123.747925395275)) ;
#23643=CARTESIAN_POINT('Ctrl Pts',(-20.8812658706226,37.3931649304323,123.8319433124)) ;
#23644=CARTESIAN_POINT('Ctrl Pts',(-20.400758322157,37.5931369665455,124.129898349839)) ;
#23645=CARTESIAN_POINT('Ctrl Pts',(-20.6486375255731,37.4131478861826,124.309410738548)) ;
#23646=CARTESIAN_POINT('Ctrl Pts',(-20.0987238949301,37.6129454885216,124.423499457933)) ;
#23647=CARTESIAN_POINT('Ctrl Pts',(-20.2710983170399,37.4329564081588,124.676413569009)) ;
#23648=CARTESIAN_POINT('Ctrl Pts',(-19.7115115108839,37.6329310632575,124.598340112043)) ;
#23649=CARTESIAN_POINT('Ctrl Pts',(-19.7870846025984,37.4529419828946,124.894968051368)) ;
#23650=CARTESIAN_POINT('Ctrl Pts',(-19.2898630183284,37.6528137033259,124.630311193854)) ;
#23651=CARTESIAN_POINT('Ctrl Pts',(-19.2600251516879,37.472824622963,124.934935958172)) ;
#23652=CARTESIAN_POINT('Ctrl Pts',(-18.8812143689227,37.6727690154578,124.516434264361)) ;
#23653=CARTESIAN_POINT('Ctrl Pts',(-18.7492134555832,37.4927799350949,124.792594096249)) ;
#23654=CARTESIAN_POINT('Ctrl Pts',(-18.5370718720123,37.6926433720656,124.271071448135)) ;
#23655=CARTESIAN_POINT('Ctrl Pts',(-18.319033254551,37.5126542917027,124.485894779788)) ;
#23656=CARTESIAN_POINT('Ctrl Pts',(-18.295856749821,37.7126255789266,123.921365626854)) ;
#23657=CARTESIAN_POINT('Ctrl Pts',(-18.0175106060064,37.5326364985638,124.048765115388)) ;
#23658=CARTESIAN_POINT('Ctrl Pts',(-18.1889170459794,37.7325566568766,123.511199159604)) ;
#23659=CARTESIAN_POINT('Ctrl Pts',(-17.8838308617942,37.5525675765137,123.536059048149)) ;
#23660=CARTESIAN_POINT('Ctrl Pts',(-18.2282802535352,37.7524836317316,123.089417927906)) ;
#23661=CARTESIAN_POINT('Ctrl Pts',(-17.9330320754365,37.5724945513687,123.008830582015)) ;
#23662=CARTESIAN_POINT('Ctrl Pts',(-18.4076686429173,37.7723160906805,122.707716966432)) ;
#23663=CARTESIAN_POINT('Ctrl Pts',(-18.157254622848,37.5923270103176,122.531709623646)) ;
#23664=CARTESIAN_POINT('Ctrl Pts',(-18.6583803627313,37.7889737748557,122.457695839393)) ;
#23665=CARTESIAN_POINT('Ctrl Pts',(-18.4706659458096,37.6089846944928,122.219158784054)) ;
#23666=CARTESIAN_POINT('Ctrl Pts',(-18.8998510224225,37.8022229987628,122.318670298478)) ;
#23667=CARTESIAN_POINT('Ctrl Pts',(-18.7724796762074,37.6222339183999,122.045392670349)) ;
#23668=CARTESIAN_POINT('Ctrl Pts',(-19.0983967328829,37.812272020214,122.246576703272)) ;
#23669=CARTESIAN_POINT('Ctrl Pts',(-19.0206690089167,37.6322829398511,121.955269929733)) ;
#23670=CARTESIAN_POINT('Ctrl Pts',(-19.3025665370279,37.8221320284445,122.210682156202)) ;
#23671=CARTESIAN_POINT('Ctrl Pts',(-19.2758657649021,37.6421429480816,121.910397904174)) ;
#23672=CARTESIAN_POINT('Ctrl Pts',(-19.5818034711638,37.8354155416691,122.209888694931)) ;
#23673=CARTESIAN_POINT('Ctrl Pts',(-19.6249794284296,37.6554264613062,121.909413584284)) ;
#23674=CARTESIAN_POINT('Ctrl Pts',(-19.9238580353541,37.8520614606699,122.300927522182)) ;
#23675=CARTESIAN_POINT('Ctrl Pts',(-20.0524638778648,37.672072380307,122.023188295616)) ;
#23676=CARTESIAN_POINT('Ctrl Pts',(-20.2129442647701,37.868615438486,122.501691868279)) ;
#23677=CARTESIAN_POINT('Ctrl Pts',(-20.413880776944,37.6886263581231,122.274169668414)) ;
#23678=CARTESIAN_POINT('Ctrl Pts',(-20.3943636779236,37.8819751674576,122.716138212852)) ;
#23679=CARTESIAN_POINT('Ctrl Pts',(-20.6406243713132,37.7019860870947,122.542201540504)) ;
#23680=CARTESIAN_POINT('Ctrl Pts',(-20.4992200878676,37.8918682192543,122.895764414402)) ;
#23681=CARTESIAN_POINT('Ctrl Pts',(-20.771703979078,37.7118791388914,122.766737576687)) ;
#23682=CARTESIAN_POINT('Ctrl Pts',(-20.5722587350757,37.9018581845353,123.092651468805)) ;
#23683=CARTESIAN_POINT('Ctrl Pts',(-20.8630031282262,37.7218691041725,123.012844193469)) ;
#23684=CARTESIAN_POINT('Ctrl Pts',(-20.6099889776979,37.9118100653962,123.298474001835)) ;
#23685=CARTESIAN_POINT('Ctrl Pts',(-20.9101691765086,37.7318209850333,123.270122215449)) ;
#23686=CARTESIAN_POINT('Ctrl Pts',(-20.6112435236213,37.921858417088,123.509695858603)) ;
#23687=CARTESIAN_POINT('Ctrl Pts',(-20.9117400295103,37.7418693367251,123.534149528085)) ;
#23688=CARTESIAN_POINT('Ctrl Pts',(-20.5767689441837,37.9316997011942,123.713719442)) ;
#23689=CARTESIAN_POINT('Ctrl Pts',(-20.8686496157947,37.7517106208313,123.789179451331)) ;
#23690=CARTESIAN_POINT('Ctrl Pts',(-20.5068028273446,37.9416864043198,123.911631328625)) ;
#23691=CARTESIAN_POINT('Ctrl Pts',(-20.7811945958756,37.761697323957,124.0365703206)) ;
#23692=CARTESIAN_POINT('Ctrl Pts',(-20.4041443174755,37.9516214331373,124.093573751061)) ;
#23693=CARTESIAN_POINT('Ctrl Pts',(-20.6528738763807,37.7716323527744,124.263999794878)) ;
#23694=CARTESIAN_POINT('Ctrl Pts',(-20.2697516088806,37.9616772280442,124.256720400925)) ;
#23695=CARTESIAN_POINT('Ctrl Pts',(-20.4848851322175,37.7816881476813,124.467934944113)) ;
#23696=CARTESIAN_POINT('Ctrl Pts',(-20.112868940614,37.9715055913335,124.391230410189)) ;
#23697=CARTESIAN_POINT('Ctrl Pts',(-20.2887835292672,37.7915165109706,124.636074676787)) ;
#23698=CARTESIAN_POINT('Ctrl Pts',(-19.9310077930652,37.9815665612314,124.499176168369)) ;
#23699=CARTESIAN_POINT('Ctrl Pts',(-20.0614584855971,37.8015774808685,124.771009318032)) ;
#23700=CARTESIAN_POINT('Ctrl Pts',(-19.7359423603849,37.9914808401212,124.572672275179)) ;
#23701=CARTESIAN_POINT('Ctrl Pts',(-19.8176275658583,37.8114917597583,124.862882128275)) ;
#23702=CARTESIAN_POINT('Ctrl Pts',(-19.5292180654532,38.0014898345894,124.611953243679)) ;
#23703=CARTESIAN_POINT('Ctrl Pts',(-19.5592226441299,37.8215007542265,124.911986102219)) ;
#23704=CARTESIAN_POINT('Ctrl Pts',(-19.3183758075429,38.0115196691532,124.614317888065)) ;
#23705=CARTESIAN_POINT('Ctrl Pts',(-19.2956698137528,37.8315305887903,124.914944725245)) ;
#23706=CARTESIAN_POINT('Ctrl Pts',(-19.1138048120896,38.0213778992254,124.581009867866)) ;
#23707=CARTESIAN_POINT('Ctrl Pts',(-19.0399553923332,37.8413888188625,124.873312424771)) ;
#23708=CARTESIAN_POINT('Ctrl Pts',(-18.9152985830758,38.0313766049678,124.51196923972)) ;
#23709=CARTESIAN_POINT('Ctrl Pts',(-18.7918216048471,37.8513875246049,124.787014243601)) ;
#23710=CARTESIAN_POINT('Ctrl Pts',(-18.7335213440721,38.0412712608866,124.410757402581)) ;
#23711=CARTESIAN_POINT('Ctrl Pts',(-18.5645984860679,37.8612821805237,124.660501733372)) ;
#23712=CARTESIAN_POINT('Ctrl Pts',(-18.5694307222782,38.0513343252705,124.27728255479)) ;
#23713=CARTESIAN_POINT('Ctrl Pts',(-18.3594834848053,37.8713452449077,124.493660346681)) ;
#23714=CARTESIAN_POINT('Ctrl Pts',(-18.4338627813113,38.0611739835504,124.120992090027)) ;
#23715=CARTESIAN_POINT('Ctrl Pts',(-18.1900212161876,37.8811849031876,124.298298757576)) ;
#23716=CARTESIAN_POINT('Ctrl Pts',(-18.3248772146404,38.0712371506323,123.939698712811)) ;
#23717=CARTESIAN_POINT('Ctrl Pts',(-18.0537869453756,37.8912480702694,124.071683477115)) ;
#23718=CARTESIAN_POINT('Ctrl Pts',(-18.2504447417178,38.0811313957594,123.745439174698)) ;
#23719=CARTESIAN_POINT('Ctrl Pts',(-17.9607436771395,37.9011423153965,123.828859729569)) ;
#23720=CARTESIAN_POINT('Ctrl Pts',(-18.2101341066762,38.091073217364,123.54038139259)) ;
#23721=CARTESIAN_POINT('Ctrl Pts',(-17.9103527062584,37.9110841370011,123.572537760102)) ;
#23722=CARTESIAN_POINT('Ctrl Pts',(-18.2059368471232,38.1010757482821,123.330110491768)) ;
#23723=CARTESIAN_POINT('Ctrl Pts',(-17.9051034699468,37.9210866679192,123.309699103469)) ;
#23724=CARTESIAN_POINT('Ctrl Pts',(-18.238734440385,38.1111103747396,123.12172723179)) ;
#23725=CARTESIAN_POINT('Ctrl Pts',(-17.946097783474,37.9311212943767,123.049219622139)) ;
#23726=CARTESIAN_POINT('Ctrl Pts',(-18.305619068495,38.120955909726,122.925840042337)) ;
#23727=CARTESIAN_POINT('Ctrl Pts',(-18.0297012300919,37.9409668293631,122.804359246479)) ;
#23728=CARTESIAN_POINT('Ctrl Pts',(-18.4064882596098,38.130939334565,122.74180463094)) ;
#23729=CARTESIAN_POINT('Ctrl Pts',(-18.1557855280744,37.9509502542022,122.574313582137)) ;
#23730=CARTESIAN_POINT('Ctrl Pts',(-18.537392601509,38.1408897249301,122.578629160492)) ;
#23731=CARTESIAN_POINT('Ctrl Pts',(-18.3194140988036,37.9609006445672,122.370342409505)) ;
#23732=CARTESIAN_POINT('Ctrl Pts',(-18.6952097088462,38.1508873652272,122.439785210272)) ;
#23733=CARTESIAN_POINT('Ctrl Pts',(-18.5166838775539,37.9708982848643,122.196785487703)) ;
#23734=CARTESIAN_POINT('Ctrl Pts',(-18.8756765943063,38.1609264457904,122.330377777602)) ;
#23735=CARTESIAN_POINT('Ctrl Pts',(-18.7422660732146,37.9809373654275,122.060023983283)) ;
#23736=CARTESIAN_POINT('Ctrl Pts',(-19.0680799590173,38.1707525965595,122.255148656096)) ;
#23737=CARTESIAN_POINT('Ctrl Pts',(-18.9827700674646,37.9907635161966,121.965984935098)) ;
#23738=CARTESIAN_POINT('Ctrl Pts',(-19.2752831931946,38.1808091714886,122.213190167837)) ;
#23739=CARTESIAN_POINT('Ctrl Pts',(-19.2417735141306,38.0008200911257,121.913534414804)) ;
#23740=CARTESIAN_POINT('Ctrl Pts',(-19.4842136350837,38.1907497108689,122.208272468333)) ;
#23741=CARTESIAN_POINT('Ctrl Pts',(-19.5029368385389,38.010760630506,121.907384733562)) ;
#23742=CARTESIAN_POINT('Ctrl Pts',(-19.6901672000189,38.2006541038453,122.238947693484)) ;
#23743=CARTESIAN_POINT('Ctrl Pts',(-19.7603796758828,38.0206650234824,121.94572645087)) ;
#23744=CARTESIAN_POINT('Ctrl Pts',(-19.8904397603091,38.2107007580502,122.305985318567)) ;
#23745=CARTESIAN_POINT('Ctrl Pts',(-20.0107210558662,38.0307116776873,122.029521129623)) ;
#23746=CARTESIAN_POINT('Ctrl Pts',(-20.073374575685,38.2205963199886,122.405120062079)) ;
#23747=CARTESIAN_POINT('Ctrl Pts',(-20.2393912303446,38.0406072396257,122.153437722029)) ;
#23748=CARTESIAN_POINT('Ctrl Pts',(-20.239009195266,38.2306583978341,122.536650134801)) ;
#23749=CARTESIAN_POINT('Ctrl Pts',(-20.4464358604614,38.0506693174713,122.317848314889)) ;
#23750=CARTESIAN_POINT('Ctrl Pts',(-20.3763552173519,38.2405010962479,122.691451330782)) ;
#23751=CARTESIAN_POINT('Ctrl Pts',(-20.6181207395519,38.060512015885,122.511348876402)) ;
#23752=CARTESIAN_POINT('Ctrl Pts',(-20.4867630860936,38.2504918712094,122.870097720652)) ;
#23753=CARTESIAN_POINT('Ctrl Pts',(-20.7561325943481,38.0705027908465,122.734655821582)) ;
#23754=CARTESIAN_POINT('Ctrl Pts',(-20.5639707241842,38.2604197362285,123.064019607399)) ;
#23755=CARTESIAN_POINT('Ctrl Pts',(-20.8526444302202,38.0804306558656,122.977057792993)) ;
#23756=CARTESIAN_POINT('Ctrl Pts',(-20.606936524891,38.2704084809947,123.269576207478)) ;
#23757=CARTESIAN_POINT('Ctrl Pts',(-20.9063538531691,38.0904194006318,123.234003272381)) ;
#23758=CARTESIAN_POINT('Ctrl Pts',(-20.6132774081827,38.2804412665816,123.480405040988)) ;
#23759=CARTESIAN_POINT('Ctrl Pts',(-20.9142822162603,38.1004521862187,123.497539173054)) ;
#23760=CARTESIAN_POINT('Ctrl Pts',(-20.5836278378137,38.2903079512023,123.685696146507)) ;
#23761=CARTESIAN_POINT('Ctrl Pts',(-20.8772223147212,38.1103188708394,123.754154223928)) ;
#23762=CARTESIAN_POINT('Ctrl Pts',(-20.5187275010846,38.3002698433654,123.884820325634)) ;
#23763=CARTESIAN_POINT('Ctrl Pts',(-20.7960987290107,38.1202807630025,124.00306041153)) ;
#23764=CARTESIAN_POINT('Ctrl Pts',(-20.4192419119231,38.310303320278,124.070811287122)) ;
#23765=CARTESIAN_POINT('Ctrl Pts',(-20.6717436692743,38.1303142399151,124.235550043403)) ;
#23766=CARTESIAN_POINT('Ctrl Pts',(-20.2911476331738,38.3201876615263,124.234467456338)) ;
#23767=CARTESIAN_POINT('Ctrl Pts',(-20.5116269403932,38.1401985811634,124.440122137364)) ;
#23768=CARTESIAN_POINT('Ctrl Pts',(-20.1338310125617,38.3302506036474,124.375873737008)) ;
#23769=CARTESIAN_POINT('Ctrl Pts',(-20.3149827227567,38.1502615232845,124.616881340023)) ;
#23770=CARTESIAN_POINT('Ctrl Pts',(-19.9581597878484,38.340101005267,124.485559805927)) ;
#23771=CARTESIAN_POINT('Ctrl Pts',(-20.0953938752767,38.1601119249041,124.75399118927)) ;
#23772=CARTESIAN_POINT('Ctrl Pts',(-19.7628910644464,38.3501278940566,124.564952690496)) ;
#23773=CARTESIAN_POINT('Ctrl Pts',(-19.8513087068426,38.1701388136938,124.853234002042)) ;
#23774=CARTESIAN_POINT('Ctrl Pts',(-19.5566368100917,38.3601565090128,124.608705273283)) ;
#23775=CARTESIAN_POINT('Ctrl Pts',(-19.593491376287,38.18016742865,124.907926696643)) ;
#23776=CARTESIAN_POINT('Ctrl Pts',(-19.3498081641325,38.3700017321329,124.616238591243)) ;
#23777=CARTESIAN_POINT('Ctrl Pts',(-19.3349545228551,38.19001265177,124.917345289566)) ;
#23778=CARTESIAN_POINT('Ctrl Pts',(-19.1416901454092,38.3799924159389,124.587880295423)) ;
#23779=CARTESIAN_POINT('Ctrl Pts',(-19.0748065717966,38.200003335576,124.88189910921)) ;
#23780=CARTESIAN_POINT('Ctrl Pts',(-18.9408634995236,38.3900302980113,124.52306847004)) ;
#23781=CARTESIAN_POINT('Ctrl Pts',(-18.8237728136893,38.2100412176484,124.80088615643)) ;
#23782=CARTESIAN_POINT('Ctrl Pts',(-18.7577593662331,38.3998746576501,124.426589014127)) ;
#23783=CARTESIAN_POINT('Ctrl Pts',(-18.5948907896328,38.2198855772873,124.680287851483)) ;
#23784=CARTESIAN_POINT('Ctrl Pts',(-18.5916294729954,38.4098595282649,124.298321906934)) ;
#23785=CARTESIAN_POINT('Ctrl Pts',(-18.3872272286847,38.229870447902,124.519955106578)) ;
#23786=CARTESIAN_POINT('Ctrl Pts',(-18.4508291327248,38.4197988115935,124.14388654102)) ;
#23787=CARTESIAN_POINT('Ctrl Pts',(-18.2112252563883,38.2398097312307,124.326911572828)) ;
#23788=CARTESIAN_POINT('Ctrl Pts',(-18.3379263587694,38.4298394209667,123.965558708293)) ;
#23789=CARTESIAN_POINT('Ctrl Pts',(-18.0700954992362,38.2498503406038,124.104002776353)) ;
#23790=CARTESIAN_POINT('Ctrl Pts',(-18.2587866795904,38.4397242718799,123.77338134412)) ;
#23791=CARTESIAN_POINT('Ctrl Pts',(-17.9711690914586,38.259735191517,123.863780801288)) ;
#23792=CARTESIAN_POINT('Ctrl Pts',(-18.2134543934735,38.4497262280487,123.568085773831)) ;
#23793=CARTESIAN_POINT('Ctrl Pts',(-17.9145022539865,38.2697371476858,123.607161518794)) ;
#23794=CARTESIAN_POINT('Ctrl Pts',(-18.2043619080485,38.4596448247692,123.359731016795)) ;
#23795=CARTESIAN_POINT('Ctrl Pts',(-17.9031351939843,38.2796557444063,123.34671741945)) ;
#23796=CARTESIAN_POINT('Ctrl Pts',(-18.2319694185159,38.469691646845,123.150356999405)) ;
#23797=CARTESIAN_POINT('Ctrl Pts',(-17.9376431227796,38.2897025664821,123.084999919376)) ;
#23798=CARTESIAN_POINT('Ctrl Pts',(-18.2942537247054,38.4795659279577,122.952295745254)) ;
#23799=CARTESIAN_POINT('Ctrl Pts',(-18.0154975116536,38.2995768475948,122.837421943665)) ;
#23800=CARTESIAN_POINT('Ctrl Pts',(-18.3915795652772,38.4896201280023,122.764705800279)) ;
#23801=CARTESIAN_POINT('Ctrl Pts',(-18.1371535108144,38.3096310476394,122.602934129142)) ;
#23802=CARTESIAN_POINT('Ctrl Pts',(-18.517948341089,38.4995155576375,122.599403244728)) ;
#23803=CARTESIAN_POINT('Ctrl Pts',(-18.2951140075871,38.3195264772746,122.396304412918)) ;
#23804=CARTESIAN_POINT('Ctrl Pts',(-18.6735897291934,38.5095771859549,122.456195028724)) ;
#23805=CARTESIAN_POINT('Ctrl Pts',(-18.489664634007,38.329588105592,122.217293421697)) ;
#23806=CARTESIAN_POINT('Ctrl Pts',(-18.8479034008404,38.5194218147848,122.344605396143)) ;
#23807=CARTESIAN_POINT('Ctrl Pts',(-18.7075571482892,38.3394327344219,122.077804596519)) ;
#23808=CARTESIAN_POINT('Ctrl Pts',(-19.0408840506454,38.5293818623904,122.263352848004)) ;
#23809=CARTESIAN_POINT('Ctrl Pts',(-18.9487829946581,38.3493927820275,121.976237815657)) ;
#23810=CARTESIAN_POINT('Ctrl Pts',(-19.2467307026046,38.5394201685644,122.216882947286)) ;
#23811=CARTESIAN_POINT('Ctrl Pts',(-19.2060908983608,38.3594310882016,121.918149353435)) ;
#23812=CARTESIAN_POINT('Ctrl Pts',(-19.4540764654965,38.5492934679971,122.206624033393)) ;
#23813=CARTESIAN_POINT('Ctrl Pts',(-19.4652741750424,38.3693043876342,121.905324657195)) ;
#23814=CARTESIAN_POINT('Ctrl Pts',(-19.6641424754752,38.5593667295834,122.233106532609)) ;
#23815=CARTESIAN_POINT('Ctrl Pts',(-19.7278563927704,38.3793776492205,121.938426707961)) ;
#23816=CARTESIAN_POINT('Ctrl Pts',(-19.8615036156616,38.5691869555401,122.293853612687)) ;
#23817=CARTESIAN_POINT('Ctrl Pts',(-19.9745595742938,38.3891978751772,122.014360134831)) ;
#23818=CARTESIAN_POINT('Ctrl Pts',(-20.0501587943975,38.5792660194796,122.390213788691)) ;
#23819=CARTESIAN_POINT('Ctrl Pts',(-20.2103785146625,38.3992769391167,122.134809378916)) ;
#23820=CARTESIAN_POINT('Ctrl Pts',(-20.2155221291384,38.5891161094994,122.514954133078)) ;
#23821=CARTESIAN_POINT('Ctrl Pts',(-20.4170842341087,38.4091270291365,122.29073495999)) ;
#23822=CARTESIAN_POINT('Ctrl Pts',(-20.3599977542973,38.5991948631132,122.669874910187)) ;
#23823=CARTESIAN_POINT('Ctrl Pts',(-20.5976790049717,38.4192057827503,122.484385049267)) ;
#23824=CARTESIAN_POINT('Ctrl Pts',(-20.4726208048676,38.6090163303726,122.842988026387)) ;
#23825=CARTESIAN_POINT('Ctrl Pts',(-20.7384592821363,38.4290272500098,122.700777392782)) ;
#23826=CARTESIAN_POINT('Ctrl Pts',(-20.5557471903728,38.6190819287303,123.037535696826)) ;
#23827=CARTESIAN_POINT('Ctrl Pts',(-20.8423676549778,38.4390928483674,122.943961403778)) ;
#23828=CARTESIAN_POINT('Ctrl Pts',(-20.6030203243983,38.628984584505,123.240335099083)) ;
#23829=CARTESIAN_POINT('Ctrl Pts',(-20.9014598751906,38.4489955041421,123.197461404665)) ;
#23830=CARTESIAN_POINT('Ctrl Pts',(-20.6145926696744,38.6390354103346,123.451275235179)) ;
#23831=CARTESIAN_POINT('Ctrl Pts',(-20.9159258761711,38.4590463299717,123.461136272486)) ;
#23832=CARTESIAN_POINT('Ctrl Pts',(-20.5899961792857,38.6489096146735,123.657445196275)) ;
#23833=CARTESIAN_POINT('Ctrl Pts',(-20.8851806308957,38.4689205343106,123.718849938155)) ;
#23834=CARTESIAN_POINT('Ctrl Pts',(-20.5288093864204,38.6589820647126,123.860120703039)) ;
#23835=CARTESIAN_POINT('Ctrl Pts',(-20.808697747039,38.4789929843497,123.972194060034)) ;
#23836=CARTESIAN_POINT('Ctrl Pts',(-20.4358076287803,38.6688110814861,124.044689523101)) ;
#23837=CARTESIAN_POINT('Ctrl Pts',(-20.6924452330028,38.4888220011232,124.202906653744)) ;
#23838=CARTESIAN_POINT('Ctrl Pts',(-20.3094581014981,38.6788779274009,124.214427563999)) ;
#23839=CARTESIAN_POINT('Ctrl Pts',(-20.5345088117265,38.498888847038,124.415079071641)) ;
#23840=CARTESIAN_POINT('Ctrl Pts',(-20.1581204946843,38.6887680987027,124.357044093307)) ;
#23841=CARTESIAN_POINT('Ctrl Pts',(-20.3453362910282,38.5087790183398,124.593350718177)) ;
#23842=CARTESIAN_POINT('Ctrl Pts',(-19.9828118483022,38.6987602923265,124.472759650499)) ;
#23843=CARTESIAN_POINT('Ctrl Pts',(-20.1262004053155,38.5187712119636,124.737995435515)) ;
#23844=CARTESIAN_POINT('Ctrl Pts',(-19.7905552310231,38.7087231029499,124.555852659848)) ;
#23845=CARTESIAN_POINT('Ctrl Pts',(-19.8858793197356,38.5287340225871,124.841862120209)) ;
#23846=CARTESIAN_POINT('Ctrl Pts',(-19.5880898351678,38.7186273757934,124.604536143381)) ;
#23847=CARTESIAN_POINT('Ctrl Pts',(-19.6327966736522,38.5386382954305,124.9027167446)) ;
#23848=CARTESIAN_POINT('Ctrl Pts',(-19.3770005006573,38.728687867598,124.617340881454)) ;
#23849=CARTESIAN_POINT('Ctrl Pts',(-19.3689353661875,38.5486987872351,124.918722771456)) ;
#23850=CARTESIAN_POINT('Ctrl Pts',(-19.1714080286777,38.7385281992703,124.594087546926)) ;
#23851=CARTESIAN_POINT('Ctrl Pts',(-19.1119433120646,38.5585391189074,124.8896559552)) ;
#23852=CARTESIAN_POINT('Ctrl Pts',(-18.9684668170041,38.7485912453621,124.53442387862)) ;
#23853=CARTESIAN_POINT('Ctrl Pts',(-18.858267179598,38.5686021649992,124.815076395297)) ;
#23854=CARTESIAN_POINT('Ctrl Pts',(-18.7821841412429,38.7584853010572,124.441832669131)) ;
#23855=CARTESIAN_POINT('Ctrl Pts',(-18.6254129262552,38.5784962206943,124.699336919331)) ;
#23856=CARTESIAN_POINT('Ctrl Pts',(-18.613681541493,38.7684280013801,124.318182967995)) ;
#23857=CARTESIAN_POINT('Ctrl Pts',(-18.4147842988255,38.5884389210173,124.544774213898)) ;
#23858=CARTESIAN_POINT('Ctrl Pts',(-18.4682304496749,38.7784337423077,124.166191909922)) ;
#23859=CARTESIAN_POINT('Ctrl Pts',(-18.2329705623296,38.5984446619449,124.354785151136)) ;
#23860=CARTESIAN_POINT('Ctrl Pts',(-18.3514150571057,38.7884546528233,123.990879578772)) ;
#23861=CARTESIAN_POINT('Ctrl Pts',(-18.086951476104,38.6084655724604,124.135644682199)) ;
#23862=CARTESIAN_POINT('Ctrl Pts',(-18.2676887679517,38.7983453882732,123.800540045983)) ;
#23863=CARTESIAN_POINT('Ctrl Pts',(-17.9822934308915,38.6183563079104,123.897719206915)) ;
#23864=CARTESIAN_POINT('Ctrl Pts',(-18.2174815072807,38.8083369290021,123.596583556656)) ;
#23865=CARTESIAN_POINT('Ctrl Pts',(-17.9195346698227,38.6283478486392,123.642773296593)) ;
#23866=CARTESIAN_POINT('Ctrl Pts',(-18.2035708832846,38.8182847894237,123.387913191954)) ;
#23867=CARTESIAN_POINT('Ctrl Pts',(-17.9021467020347,38.6382957090609,123.381934725884)) ;
#23868=CARTESIAN_POINT('Ctrl Pts',(-18.2256918881132,38.8282314586101,123.17996466364)) ;
#23869=CARTESIAN_POINT('Ctrl Pts',(-17.9297985346469,38.6482423782472,123.121998548221)) ;
#23870=CARTESIAN_POINT('Ctrl Pts',(-18.2843906460259,38.8382795347457,122.977049468211)) ;
#23871=CARTESIAN_POINT('Ctrl Pts',(-18.0031723206151,38.6582904543828,122.868354913034)) ;
#23872=CARTESIAN_POINT('Ctrl Pts',(-18.3754224094433,38.8481271327513,122.79110855479)) ;
#23873=CARTESIAN_POINT('Ctrl Pts',(-18.1169630845849,38.6681380523884,122.635927730738)) ;
#23874=CARTESIAN_POINT('Ctrl Pts',(-18.4982316363328,38.8580888558358,122.621481919964)) ;
#23875=CARTESIAN_POINT('Ctrl Pts',(-18.2704754939803,38.6780997754729,122.423894509235)) ;
#23876=CARTESIAN_POINT('Ctrl Pts',(-18.6498412742199,38.8681174909188,122.474952850286)) ;
#23877=CARTESIAN_POINT('Ctrl Pts',(-18.459987920288,38.6881284105559,122.240733703719)) ;
#23878=CARTESIAN_POINT('Ctrl Pts',(-18.822471332867,38.8780277992368,122.358322296909)) ;
#23879=CARTESIAN_POINT('Ctrl Pts',(-18.6757765964958,38.6980387188739,122.094945578105)) ;
#23880=CARTESIAN_POINT('Ctrl Pts',(-19.0129931752722,38.8879626963727,122.272721130062)) ;
#23881=CARTESIAN_POINT('Ctrl Pts',(-18.9139298646634,38.7079736160098,121.987944654687)) ;
#23882=CARTESIAN_POINT('Ctrl Pts',(-19.2176845439249,38.8980037793153,122.221146163374)) ;
#23883=CARTESIAN_POINT('Ctrl Pts',(-19.1697940908906,38.7180146989524,121.92347677505)) ;
#23884=CARTESIAN_POINT('Ctrl Pts',(-19.4250041735291,38.9078911221435,122.205985759555)) ;
#23885=CARTESIAN_POINT('Ctrl Pts',(-19.4289447281885,38.7279020417806,121.904527054462)) ;
#23886=CARTESIAN_POINT('Ctrl Pts',(-19.6340005528841,38.9178826370828,122.22691350164)) ;
#23887=CARTESIAN_POINT('Ctrl Pts',(-19.6901903067169,38.73789355672,121.930687744959)) ;
#23888=CARTESIAN_POINT('Ctrl Pts',(-19.8353682152375,38.9278340282793,122.283672510292)) ;
#23889=CARTESIAN_POINT('Ctrl Pts',(-19.9419001392369,38.7478449479164,122.001637581168)) ;
#23890=CARTESIAN_POINT('Ctrl Pts',(-20.0236163341247,38.9377665616119,122.374032890848)) ;
#23891=CARTESIAN_POINT('Ctrl Pts',(-20.1772104092053,38.7577774812491,122.114589337141)) ;
#23892=CARTESIAN_POINT('Ctrl Pts',(-20.1944626039504,38.9477637195114,122.496427038679)) ;
#23893=CARTESIAN_POINT('Ctrl Pts',(-20.3907677132585,38.7677746391485,122.267583026891)) ;
#23894=CARTESIAN_POINT('Ctrl Pts',(-20.3413685794426,38.9577487296749,122.646417878081)) ;
#23895=CARTESIAN_POINT('Ctrl Pts',(-20.5743995160923,38.777759649312,122.455072551218)) ;
#23896=CARTESIAN_POINT('Ctrl Pts',(-20.46039600103,38.9677915562447,122.820765432393)) ;
#23897=CARTESIAN_POINT('Ctrl Pts',(-20.7231828307075,38.7878024758818,122.673007430821)) ;
#23898=CARTESIAN_POINT('Ctrl Pts',(-20.5459597437265,38.9776217905496,123.00891851305)) ;
#23899=CARTESIAN_POINT('Ctrl Pts',(-20.8301369986688,38.7976327101868,122.908200598567)) ;
#23900=CARTESIAN_POINT('Ctrl Pts',(-20.5989170245634,38.9876978157843,123.213977187539)) ;
#23901=CARTESIAN_POINT('Ctrl Pts',(-20.8963322764258,38.8077087354214,123.164523836751)) ;
#23902=CARTESIAN_POINT('Ctrl Pts',(-20.6152120888322,38.9975500522752,123.42050479598)) ;
#23903=CARTESIAN_POINT('Ctrl Pts',(-20.9166999184839,38.8175609719123,123.422684680524)) ;
#23904=CARTESIAN_POINT('Ctrl Pts',(-20.5951407332866,39.0076232587093,123.631287792169)) ;
#23905=CARTESIAN_POINT('Ctrl Pts',(-20.8916094132905,38.8276341783464,123.686162896882)) ;
#23906=CARTESIAN_POINT('Ctrl Pts',(-20.5400039210857,39.0174647682165,123.830719200316)) ;
#23907=CARTESIAN_POINT('Ctrl Pts',(-20.8226867659829,38.8374756878536,123.935453060471)) ;
#23908=CARTESIAN_POINT('Ctrl Pts',(-20.4507189099979,39.0274257149963,124.020134101284)) ;
#23909=CARTESIAN_POINT('Ctrl Pts',(-20.711078874135,38.8474366346334,124.172221368131)) ;
#23910=CARTESIAN_POINT('Ctrl Pts',(-20.3286238637453,39.0374635437963,124.192245807622)) ;
#23911=CARTESIAN_POINT('Ctrl Pts',(-20.558458951886,38.8574744634334,124.387360046542)) ;
#23912=CARTESIAN_POINT('Ctrl Pts',(-20.1811938017144,39.0473378535508,124.338423480837)) ;
#23913=CARTESIAN_POINT('Ctrl Pts',(-20.3741695323438,38.8673487731879,124.570081720976)) ;
#23914=CARTESIAN_POINT('Ctrl Pts',(-20.0072836350948,39.0574075512239,124.45908427213)) ;
#23915=CARTESIAN_POINT('Ctrl Pts',(-20.1567812055592,38.8774184708611,124.72090620419)) ;
#23916=CARTESIAN_POINT('Ctrl Pts',(-19.8195805182457,39.0672410225113,124.545752922959)) ;
#23917=CARTESIAN_POINT('Ctrl Pts',(-19.9221504638818,38.8872519421485,124.82924108008)) ;
#23918=CARTESIAN_POINT('Ctrl Pts',(-19.6158666766055,39.0772706690413,124.600148476529)) ;
#23919=CARTESIAN_POINT('Ctrl Pts',(-19.6675077755331,38.8972815886784,124.897233739368)) ;
#23920=CARTESIAN_POINT('Ctrl Pts',(-19.4056375158977,39.0873051833686,124.617714671404)) ;
#23921=CARTESIAN_POINT('Ctrl Pts',(-19.4047212779265,38.9073161030058,124.919189865937)) ;
#23922=CARTESIAN_POINT('Ctrl Pts',(-19.1998910206002,39.0971304688395,124.599407552797)) ;
#23923=CARTESIAN_POINT('Ctrl Pts',(-19.1475370275011,38.9171413884767,124.896304082123)) ;
#23924=CARTESIAN_POINT('Ctrl Pts',(-18.9967244321837,39.1071347103881,124.545112550832)) ;
#23925=CARTESIAN_POINT('Ctrl Pts',(-18.8935792031542,38.9271456300252,124.828433457309)) ;
#23926=CARTESIAN_POINT('Ctrl Pts',(-18.8064617759764,39.1171173554672,124.456450033526)) ;
#23927=CARTESIAN_POINT('Ctrl Pts',(-18.6557514840931,38.9371282751043,124.717603510386)) ;
#23928=CARTESIAN_POINT('Ctrl Pts',(-18.6335954547731,39.1271625525587,124.335184104469)) ;
#23929=CARTESIAN_POINT('Ctrl Pts',(-18.439669749991,38.9471734721958,124.566019704998)) ;
#23930=CARTESIAN_POINT('Ctrl Pts',(-18.4874417294713,39.1369856683188,124.189274410091)) ;
#23931=CARTESIAN_POINT('Ctrl Pts',(-18.2569780632649,38.9569965879559,124.383630345431)) ;
#23932=CARTESIAN_POINT('Ctrl Pts',(-18.3658597551784,39.1470202801191,124.016878296206)) ;
#23933=CARTESIAN_POINT('Ctrl Pts',(-18.1050023548241,38.9670311997562,124.168134092341)) ;
#23934=CARTESIAN_POINT('Ctrl Pts',(-18.2766733676231,39.1570452888922,123.825914539901)) ;
#23935=CARTESIAN_POINT('Ctrl Pts',(-17.9935211048472,38.9770562085294,123.929428614842)) ;
#23936=CARTESIAN_POINT('Ctrl Pts',(-18.2225068331294,39.1668972137338,123.626000802301)) ;
#23937=CARTESIAN_POINT('Ctrl Pts',(-17.9258146375031,38.9869081333709,123.679534933401)) ;
#23938=CARTESIAN_POINT('Ctrl Pts',(-18.2032934378515,39.1768881520565,123.416865948046)) ;
#23939=CARTESIAN_POINT('Ctrl Pts',(-17.9017999976252,38.9968990716936,123.418116000194)) ;
#23940=CARTESIAN_POINT('Ctrl Pts',(-18.2204270850265,39.186806137203,123.209038883101)) ;
#23941=CARTESIAN_POINT('Ctrl Pts',(-17.9232192572526,39.0068170568401,123.158331775182)) ;
#23942=CARTESIAN_POINT('Ctrl Pts',(-18.2739141189626,39.1968342380985,123.005131243804)) ;
#23943=CARTESIAN_POINT('Ctrl Pts',(-17.9900801459671,39.0168451577356,122.903447812489)) ;
#23944=CARTESIAN_POINT('Ctrl Pts',(-18.3606686893931,39.2067194790411,122.816282003128)) ;
#23945=CARTESIAN_POINT('Ctrl Pts',(-18.0985256645866,39.0267303986782,122.66738650819)) ;
#23946=CARTESIAN_POINT('Ctrl Pts',(-18.4797149154803,39.2167085920077,122.643274137874)) ;
#23947=CARTESIAN_POINT('Ctrl Pts',(-18.2473354546933,39.0367195116448,122.451127866607)) ;
#23948=CARTESIAN_POINT('Ctrl Pts',(-18.6280950699641,39.2267506563485,122.493104045599)) ;
#23949=CARTESIAN_POINT('Ctrl Pts',(-18.4328121554963,39.0467615759856,122.263416874408)) ;
#23950=CARTESIAN_POINT('Ctrl Pts',(-18.7964289728388,39.236579857753,122.37324034441)) ;
#23951=CARTESIAN_POINT('Ctrl Pts',(-18.6432316642718,39.0565907773901,122.113588566168)) ;
#23952=CARTESIAN_POINT('Ctrl Pts',(-18.9861633069281,39.2465866985112,122.282419196658)) ;
#23953=CARTESIAN_POINT('Ctrl Pts',(-18.8804006960058,39.0665976181483,122.000064282247)) ;
#23954=CARTESIAN_POINT('Ctrl Pts',(-19.1884846108807,39.2565742227031,122.226135721448)) ;
#23955=CARTESIAN_POINT('Ctrl Pts',(-19.1333031196278,39.0765851423402,121.929712194851)) ;
#23956=CARTESIAN_POINT('Ctrl Pts',(-19.3983474426324,39.2666038685117,122.205902107928)) ;
#23957=CARTESIAN_POINT('Ctrl Pts',(-19.3956318554856,39.0866147881488,121.90442252384)) ;
#23958=CARTESIAN_POINT('Ctrl Pts',(-19.6053336272935,39.2764778992504,122.221912828081)) ;
#23959=CARTESIAN_POINT('Ctrl Pts',(-19.6543650766534,39.0964888188876,121.924438378725)) ;
#23960=CARTESIAN_POINT('Ctrl Pts',(-19.8089581741731,39.2864772221145,122.274010548513)) ;
#23961=CARTESIAN_POINT('Ctrl Pts',(-19.9088952559089,39.1064881417517,121.989562946881)) ;
#23962=CARTESIAN_POINT('Ctrl Pts',(-19.9988971817539,39.2963880576901,122.359747483072)) ;
#23963=CARTESIAN_POINT('Ctrl Pts',(-20.1463184204116,39.1163989773273,122.096736593804)) ;
#23964=CARTESIAN_POINT('Ctrl Pts',(-20.173454632489,39.3064423056642,122.478884560245)) ;
#23965=CARTESIAN_POINT('Ctrl Pts',(-20.3645137350782,39.1264532253013,122.245659936878)) ;
#23966=CARTESIAN_POINT('Ctrl Pts',(-20.321953767156,39.3163010499269,122.623523272663)) ;
#23967=CARTESIAN_POINT('Ctrl Pts',(-20.5501363523251,39.136311969564,122.426460600573)) ;
#23968=CARTESIAN_POINT('Ctrl Pts',(-20.4457184725392,39.3263691359999,122.79519306141)) ;
#23969=CARTESIAN_POINT('Ctrl Pts',(-20.7048400636721,39.146380055637,122.641049209758)) ;
#23970=CARTESIAN_POINT('Ctrl Pts',(-20.5358574260446,39.3362246191794,122.981770543194)) ;
#23971=CARTESIAN_POINT('Ctrl Pts',(-20.8175117263284,39.1562355388165,122.87427274074)) ;
#23972=CARTESIAN_POINT('Ctrl Pts',(-20.593627567202,39.3462194649736,123.183789054105)) ;
#23973=CARTESIAN_POINT('Ctrl Pts',(-20.889721867706,39.1662303846107,123.126796707764)) ;
#23974=CARTESIAN_POINT('Ctrl Pts',(-20.6150717947813,39.3562507606361,123.393589597854)) ;
#23975=CARTESIAN_POINT('Ctrl Pts',(-20.9165245762999,39.1762616802733,123.389047651322)) ;
#23976=CARTESIAN_POINT('Ctrl Pts',(-20.6003432400617,39.366117303926,123.600498782211)) ;
#23977=CARTESIAN_POINT('Ctrl Pts',(-20.8981112102425,39.1861282235631,123.647684462324)) ;
#23978=CARTESIAN_POINT('Ctrl Pts',(-20.5496307755805,39.3761046996894,123.804223422372)) ;
#23979=CARTESIAN_POINT('Ctrl Pts',(-20.8347179859735,39.1961156193265,123.902339731277)) ;
#23980=CARTESIAN_POINT('Ctrl Pts',(-20.4647567854182,39.3860497404194,123.995331104397)) ;
#23981=CARTESIAN_POINT('Ctrl Pts',(-20.728622932385,39.2060606600565,124.14122345198)) ;
#23982=CARTESIAN_POINT('Ctrl Pts',(-20.3467526330684,39.3960942466361,124.170424565575)) ;
#23983=CARTESIAN_POINT('Ctrl Pts',(-20.5811155220166,39.2161051662732,124.360088757602)) ;
#23984=CARTESIAN_POINT('Ctrl Pts',(-20.2028876578197,39.4059577527734,124.31979097255)) ;
#23985=CARTESIAN_POINT('Ctrl Pts',(-20.4012820501656,39.2259686724105,124.546795194446)) ;
#23986=CARTESIAN_POINT('Ctrl Pts',(-20.0333359133557,39.4159506136095,124.443780975724)) ;
#23987=CARTESIAN_POINT('Ctrl Pts',(-20.1893406639608,39.2359615332466,124.701780528445)) ;
#23988=CARTESIAN_POINT('Ctrl Pts',(-19.8460776642137,39.4258768073284,124.535944097192)) ;
#23989=CARTESIAN_POINT('Ctrl Pts',(-19.9552664329016,39.2458877269655,124.816982053056)) ;
#23990=CARTESIAN_POINT('Ctrl Pts',(-19.6438526109254,39.435895733361,124.594760442334)) ;
#23991=CARTESIAN_POINT('Ctrl Pts',(-19.7024842949339,39.2559066529981,124.890499840195)) ;
#23992=CARTESIAN_POINT('Ctrl Pts',(-19.4366243471817,39.4458107327286,124.617535468965)) ;
#23993=CARTESIAN_POINT('Ctrl Pts',(-19.4434484431289,39.2658216523657,124.918965884066)) ;
#23994=CARTESIAN_POINT('Ctrl Pts',(-19.2257177733582,39.4558655042859,124.603751642872)) ;
#23995=CARTESIAN_POINT('Ctrl Pts',(-19.1798154010535,39.275876423923,124.901733325748)) ;
#23996=CARTESIAN_POINT('Ctrl Pts',(-19.024324659477,39.4657244665834,124.554651862093)) ;
#23997=CARTESIAN_POINT('Ctrl Pts',(-18.9280744033614,39.2857353862206,124.840355827184)) ;
#23998=CARTESIAN_POINT('Ctrl Pts',(-18.8318078658274,39.4757187104213,124.47057126686)) ;
#23999=CARTESIAN_POINT('Ctrl Pts',(-18.6874294683808,39.2957296300584,124.735252472311)) ;
#24000=CARTESIAN_POINT('Ctrl Pts',(-18.6579134178425,39.4856439398455,124.355188357993)) ;
#24001=CARTESIAN_POINT('Ctrl Pts',(-18.4700628513266,39.3056548594826,124.591021419432)) ;
#24002=CARTESIAN_POINT('Ctrl Pts',(-18.505167355136,39.495671903737,124.209924117878)) ;
#24003=CARTESIAN_POINT('Ctrl Pts',(-18.2791321697973,39.3156828233741,124.409439034504)) ;
#24004=CARTESIAN_POINT('Ctrl Pts',(-18.3815260589152,39.5055581633674,124.042821017598)) ;
#24005=CARTESIAN_POINT('Ctrl Pts',(-18.1245827427517,39.3255690830045,124.200558385393)) ;
#24006=CARTESIAN_POINT('Ctrl Pts',(-18.2873441788241,39.5155899264452,123.854158630485)) ;
#24007=CARTESIAN_POINT('Ctrl Pts',(-18.0068578913663,39.3356008460823,123.964729079241)) ;
#24008=CARTESIAN_POINT('Ctrl Pts',(-18.2280346546859,39.5254715527393,123.655023225739)) ;
#24009=CARTESIAN_POINT('Ctrl Pts',(-17.9327236697777,39.3454824723765,123.715808953631)) ;
#24010=CARTESIAN_POINT('Ctrl Pts',(-18.2037205041182,39.5355333222255,123.444926394971)) ;
#24011=CARTESIAN_POINT('Ctrl Pts',(-17.9023337792867,39.3555442418626,123.453187507275)) ;
#24012=CARTESIAN_POINT('Ctrl Pts',(-18.2159436021786,39.545391189721,123.238018443075)) ;
#24013=CARTESIAN_POINT('Ctrl Pts',(-17.9176154685571,39.3654021093581,123.194552719115)) ;
#24014=CARTESIAN_POINT('Ctrl Pts',(-18.2640935145991,39.5553828148383,123.033581530344)) ;
#24015=CARTESIAN_POINT('Ctrl Pts',(-17.9778056084377,39.3753937344755,122.939007178567)) ;
#24016=CARTESIAN_POINT('Ctrl Pts',(-18.346604236998,39.5653196139466,122.841649932194)) ;
#24017=CARTESIAN_POINT('Ctrl Pts',(-18.0809465923163,39.3853305335837,122.699093789421)) ;
#24018=CARTESIAN_POINT('Ctrl Pts',(-18.4615503978526,39.5753104435039,122.665852839243)) ;
#24019=CARTESIAN_POINT('Ctrl Pts',(-18.2246316582653,39.3953213631411,122.479348914402)) ;
#24020=CARTESIAN_POINT('Ctrl Pts',(-18.6059214023956,39.5853336792171,122.512353088395)) ;
#24021=CARTESIAN_POINT('Ctrl Pts',(-18.4050975254076,39.4053445988542,122.287476075996)) ;
#24022=CARTESIAN_POINT('Ctrl Pts',(-18.7725024087154,39.5952300272463,122.38771377753)) ;
#24023=CARTESIAN_POINT('Ctrl Pts',(-18.6133254066964,39.4152409468834,122.131679228761)) ;
#24024=CARTESIAN_POINT('Ctrl Pts',(-18.9597546314449,39.6052195897488,122.292601295741)) ;
#24025=CARTESIAN_POINT('Ctrl Pts',(-18.8473919143103,39.4252305093859,122.012791074316)) ;
#24026=CARTESIAN_POINT('Ctrl Pts',(-19.1618012116734,39.6152598974333,122.231549580434)) ;
#24027=CARTESIAN_POINT('Ctrl Pts',(-19.0999512728563,39.4352708170704,121.936479082214)) ;
#24028=CARTESIAN_POINT('Ctrl Pts',(-19.367227076232,39.6251022007805,122.206604242828)) ;
#24029=CARTESIAN_POINT('Ctrl Pts',(-19.3567329848095,39.4451131204176,121.905300141157)) ;
#24030=CARTESIAN_POINT('Ctrl Pts',(-19.5776342598679,39.6351259090596,122.217627035733)) ;
#24031=CARTESIAN_POINT('Ctrl Pts',(-19.6197445019835,39.4551368286967,121.919081532484)) ;
#24032=CARTESIAN_POINT('Ctrl Pts',(-19.8485635991152,39.6483480865273,122.280050363964)) ;
#24033=CARTESIAN_POINT('Ctrl Pts',(-19.9583923044283,39.4683590061644,121.997113385212)) ;
#24034=CARTESIAN_POINT('Ctrl Pts',(-20.0983757230061,39.6616406715866,122.4121455033)) ;
#24035=CARTESIAN_POINT('Ctrl Pts',(-20.2706261181306,39.4816515912237,122.162206025503)) ;
#24036=CARTESIAN_POINT('Ctrl Pts',(-20.3030677190675,39.6749255275082,122.602175666116)) ;
#24037=CARTESIAN_POINT('Ctrl Pts',(-20.5265366200315,39.4949364471453,122.399782063078)) ;
#24038=CARTESIAN_POINT('Ctrl Pts',(-20.4297258307919,39.684897754681,122.76921101663)) ;
#24039=CARTESIAN_POINT('Ctrl Pts',(-20.6848475062148,39.5049086743181,122.608570519109)) ;
#24040=CARTESIAN_POINT('Ctrl Pts',(-20.5251856164806,39.69480637112,122.95438797765)) ;
#24041=CARTESIAN_POINT('Ctrl Pts',(-20.8041722375231,39.5148172907571,122.840044926829)) ;
#24042=CARTESIAN_POINT('Ctrl Pts',(-20.587851626912,39.7048595765037,123.156213626947)) ;
#24043=CARTESIAN_POINT('Ctrl Pts',(-20.8825021974907,39.5248704961408,123.09232602936)) ;
#24044=CARTESIAN_POINT('Ctrl Pts',(-20.6141617899061,39.714724710264,123.361949025928)) ;
#24045=CARTESIAN_POINT('Ctrl Pts',(-20.9153854640603,39.5347356299011,123.349500706136)) ;
#24046=CARTESIAN_POINT('Ctrl Pts',(-20.6014061829563,39.7280637678903,123.642094545317)) ;
#24047=CARTESIAN_POINT('Ctrl Pts',(-20.8994475638338,39.5480746875274,123.699654940672)) ;
#24048=CARTESIAN_POINT('Ctrl Pts',(-20.4948803150655,39.7446329552234,123.977922234663)) ;
#24049=CARTESIAN_POINT('Ctrl Pts',(-20.7662626209752,39.5646438748606,124.119481950554)) ;
#24050=CARTESIAN_POINT('Ctrl Pts',(-20.279368944222,39.7612780950745,124.258669320355)) ;
#24051=CARTESIAN_POINT('Ctrl Pts',(-20.4969232972869,39.5812890147116,124.470352991445)) ;
#24052=CARTESIAN_POINT('Ctrl Pts',(-20.057952056873,39.7745503975479,124.428460036515)) ;
#24053=CARTESIAN_POINT('Ctrl Pts',(-20.2201055636797,39.594561317185,124.682635504472)) ;
#24054=CARTESIAN_POINT('Ctrl Pts',(-19.8719346516173,39.7845313609955,124.525525802343)) ;
#24055=CARTESIAN_POINT('Ctrl Pts',(-19.9875926506158,39.6045422806326,124.803956293346)) ;
#24056=CARTESIAN_POINT('Ctrl Pts',(-19.6726840160093,39.7944731930648,124.588696431075)) ;
#24057=CARTESIAN_POINT('Ctrl Pts',(-19.7385233068285,39.6144841127019,124.882919421765)) ;
#24058=CARTESIAN_POINT('Ctrl Pts',(-19.3951538397195,39.8077927622802,124.625793701431)) ;
#24059=CARTESIAN_POINT('Ctrl Pts',(-19.3916274184842,39.6278036819174,124.929289096296)) ;
#24060=CARTESIAN_POINT('Ctrl Pts',(-19.0464383279096,39.824322917213,124.581253491284)) ;
#24061=CARTESIAN_POINT('Ctrl Pts',(-18.9557155359981,39.6443338368501,124.873608604834)) ;
#24062=CARTESIAN_POINT('Ctrl Pts',(-18.668086969949,39.8443446427051,124.386327800272)) ;
#24063=CARTESIAN_POINT('Ctrl Pts',(-18.4827841914937,39.6643555623422,124.629948165702)) ;
#24064=CARTESIAN_POINT('Ctrl Pts',(-18.3816863058028,39.8641560393119,124.077284990008)) ;
#24065=CARTESIAN_POINT('Ctrl Pts',(-18.1247857375982,39.684166958949,124.243642886315)) ;
#24066=CARTESIAN_POINT('Ctrl Pts',(-18.2159257669221,39.8841412880207,123.686114821925)) ;
#24067=CARTESIAN_POINT('Ctrl Pts',(-17.9175888921553,39.7041522076579,123.754678947954)) ;
#24068=CARTESIAN_POINT('Ctrl Pts',(-18.1939835367103,39.9040353506567,123.263614550275)) ;
#24069=CARTESIAN_POINT('Ctrl Pts',(-17.8901646194333,39.7240462702938,123.226554358752)) ;
#24070=CARTESIAN_POINT('Ctrl Pts',(-18.317143757237,39.9239670298303,122.858111488064)) ;
#24071=CARTESIAN_POINT('Ctrl Pts',(-18.0441177194512,39.7439779494674,122.719677099901)) ;
#24072=CARTESIAN_POINT('Ctrl Pts',(-18.5719284249735,39.9439310843023,122.518586193573)) ;
#24073=CARTESIAN_POINT('Ctrl Pts',(-18.3626008286604,39.7639420039394,122.295272619757)) ;
#24074=CARTESIAN_POINT('Ctrl Pts',(-18.9256419898356,39.9638119860652,122.287076377155)) ;
#24075=CARTESIAN_POINT('Ctrl Pts',(-18.8047431638309,39.7838229057023,122.005888410444)) ;
#24076=CARTESIAN_POINT('Ctrl Pts',(-19.3381892305123,39.9837506476736,122.189510079094)) ;
#24077=CARTESIAN_POINT('Ctrl Pts',(-19.3204270314315,39.8037615673107,121.883932996576)) ;
#24078=CARTESIAN_POINT('Ctrl Pts',(-19.7583997067115,40.0036471729289,122.23841409713)) ;
#24079=CARTESIAN_POINT('Ctrl Pts',(-19.8456885699466,39.823658092566,121.945064977875)) ;
#24080=CARTESIAN_POINT('Ctrl Pts',(-20.1370001314726,40.0235422113832,122.427152769696)) ;
#24081=CARTESIAN_POINT('Ctrl Pts',(-20.3189371293568,39.8435531310203,122.180988955681)) ;
#24082=CARTESIAN_POINT('Ctrl Pts',(-20.4293996902846,40.0435060346893,122.734826780891)) ;
#24083=CARTESIAN_POINT('Ctrl Pts',(-20.684435302286,39.8635169543264,122.565581974928)) ;
#24084=CARTESIAN_POINT('Ctrl Pts',(-20.598804014177,40.0633801588183,123.121996946429)) ;
#24085=CARTESIAN_POINT('Ctrl Pts',(-20.8961892011034,39.8833910784555,123.049543285432)) ;
#24086=CARTESIAN_POINT('Ctrl Pts',(-20.6264486511241,40.0833552345456,123.545839265876)) ;
#24087=CARTESIAN_POINT('Ctrl Pts',(-20.9307446999035,39.9033661541827,123.579345858903)) ;
#24088=CARTESIAN_POINT('Ctrl Pts',(-20.5073509704462,40.1033088039022,123.953040176851)) ;
#24089=CARTESIAN_POINT('Ctrl Pts',(-20.7818723368726,39.9233197235393,124.088346140046)) ;
#24090=CARTESIAN_POINT('Ctrl Pts',(-20.2585393963816,40.12314671409,124.293652583633)) ;
#24091=CARTESIAN_POINT('Ctrl Pts',(-20.4708597448831,39.9431576337272,124.514109737929)) ;
#24092=CARTESIAN_POINT('Ctrl Pts',(-19.9062499760645,40.143122542661,124.530920991778)) ;
#24093=CARTESIAN_POINT('Ctrl Pts',(-20.0304987770853,39.9631334622981,124.810695893572)) ;
#24094=CARTESIAN_POINT('Ctrl Pts',(-19.4952472081866,40.1630405873712,124.63297354376)) ;
#24095=CARTESIAN_POINT('Ctrl Pts',(-19.5167467254977,39.9830515070084,124.938262136295)) ;
#24096=CARTESIAN_POINT('Ctrl Pts',(-19.0748749833404,40.1829108331589,124.58981024594)) ;
#24097=CARTESIAN_POINT('Ctrl Pts',(-18.9912829799873,40.002921752796,124.884310017349)) ;
#24098=CARTESIAN_POINT('Ctrl Pts',(-18.6914968706604,40.2029598362585,124.403647517381)) ;
#24099=CARTESIAN_POINT('Ctrl Pts',(-18.512059067701,40.0229707558956,124.651607827821)) ;
#24100=CARTESIAN_POINT('Ctrl Pts',(-18.3981552231749,40.2227390774993,124.10210693945)) ;
#24101=CARTESIAN_POINT('Ctrl Pts',(-18.1453823899898,40.0427499971364,124.274685535331)) ;
#24102=CARTESIAN_POINT('Ctrl Pts',(-18.2226350296879,40.2427691412082,123.714169214818)) ;
#24103=CARTESIAN_POINT('Ctrl Pts',(-17.9259795061986,40.0627800608453,123.789764142162)) ;
#24104=CARTESIAN_POINT('Ctrl Pts',(-18.1909445920671,40.2626514261102,123.292541082987)) ;
#24105=CARTESIAN_POINT('Ctrl Pts',(-17.8863640755832,40.0826623457473,123.26273048994)) ;
#24106=CARTESIAN_POINT('Ctrl Pts',(-18.3038777435817,40.2825337270031,122.885191709277)) ;
#24107=CARTESIAN_POINT('Ctrl Pts',(-18.0275270007879,40.1025446466403,122.753544083108)) ;
#24108=CARTESIAN_POINT('Ctrl Pts',(-18.5504210038991,40.3025168366215,122.539129314307)) ;
#24109=CARTESIAN_POINT('Ctrl Pts',(-18.3357032518353,40.1225277562586,122.320964219485)) ;
#24110=CARTESIAN_POINT('Ctrl Pts',(-18.8986806428871,40.3224072319994,122.29912255241)) ;
#24111=CARTESIAN_POINT('Ctrl Pts',(-18.7710249752049,40.1424181516365,122.020953450762)) ;
#24112=CARTESIAN_POINT('Ctrl Pts',(-19.3078266805979,40.3423040220336,122.191737778741)) ;
#24113=CARTESIAN_POINT('Ctrl Pts',(-19.2824556627369,40.1623149416708,121.886718883341)) ;
#24114=CARTESIAN_POINT('Ctrl Pts',(-19.7296085524883,40.3622210759752,122.230003374302)) ;
#24115=CARTESIAN_POINT('Ctrl Pts',(-19.809682792952,40.1822319956124,121.93454660401)) ;
#24116=CARTESIAN_POINT('Ctrl Pts',(-20.1146489811739,40.3822246241788,122.410827144587)) ;
#24117=CARTESIAN_POINT('Ctrl Pts',(-20.290985297749,40.2022355438159,122.160572440253)) ;
#24118=CARTESIAN_POINT('Ctrl Pts',(-20.4133927271247,40.4021629178314,122.711596083807)) ;
#24119=CARTESIAN_POINT('Ctrl Pts',(-20.6644175476188,40.2221738374685,122.536530476513)) ;
#24120=CARTESIAN_POINT('Ctrl Pts',(-20.5914685302538,40.4219844052643,123.093592798811)) ;
#24121=CARTESIAN_POINT('Ctrl Pts',(-20.8870164933769,40.2419953249014,123.014022848812)) ;
#24122=CARTESIAN_POINT('Ctrl Pts',(-20.6292190379642,40.4419627982552,123.516656820411)) ;
#24123=CARTESIAN_POINT('Ctrl Pts',(-20.9342078753314,40.2619737178923,123.54285440319)) ;
#24124=CARTESIAN_POINT('Ctrl Pts',(-20.5204888317716,40.4618611798689,123.925614309865)) ;
#24125=CARTESIAN_POINT('Ctrl Pts',(-20.798306014332,40.281872099506,124.054044528013)) ;
#24126=CARTESIAN_POINT('Ctrl Pts',(-20.3195216622248,40.4784441105988,124.215207938259)) ;
#24127=CARTESIAN_POINT('Ctrl Pts',(-20.5470819880528,40.2984550302359,124.416062159147)) ;
#24128=CARTESIAN_POINT('Ctrl Pts',(-20.1066630617855,40.4917183461876,124.395787910796)) ;
#24129=CARTESIAN_POINT('Ctrl Pts',(-20.281028441282,40.3117292658247,124.641768863592)) ;
#24130=CARTESIAN_POINT('Ctrl Pts',(-19.9242973164539,40.5017647636438,124.502269830301)) ;
#24131=CARTESIAN_POINT('Ctrl Pts',(-20.0530654837522,40.3217756832809,124.774877815114)) ;
#24132=CARTESIAN_POINT('Ctrl Pts',(-19.7302037187856,40.5116099888631,124.57423387795)) ;
#24133=CARTESIAN_POINT('Ctrl Pts',(-19.810464403995,40.3316209085002,124.864833820521)) ;
#24134=CARTESIAN_POINT('Ctrl Pts',(-19.4546005991835,40.5249449599025,124.625166757655)) ;
#24135=CARTESIAN_POINT('Ctrl Pts',(-19.4658929191224,40.3449558795396,124.928504806225)) ;
#24136=CARTESIAN_POINT('Ctrl Pts',(-19.102968767351,40.5415278166951,124.597279021719)) ;
#24137=CARTESIAN_POINT('Ctrl Pts',(-19.0264390688312,40.3615387363322,124.893652813554)) ;
#24138=CARTESIAN_POINT('Ctrl Pts',(-18.7810021390429,40.5581708190445,124.450732297002)) ;
#24139=CARTESIAN_POINT('Ctrl Pts',(-18.6239205040509,40.3781817386816,124.71045606654)) ;
#24140=CARTESIAN_POINT('Ctrl Pts',(-18.5658420171576,40.5714145500762,124.273876479058)) ;
#24141=CARTESIAN_POINT('Ctrl Pts',(-18.3550031410799,40.3914254697133,124.489405088402)) ;
#24142=CARTESIAN_POINT('Ctrl Pts',(-18.428371398618,40.5814689447508,124.113372164029)) ;
#24143=CARTESIAN_POINT('Ctrl Pts',(-18.1831556506858,40.4014798643879,124.288773158582)) ;
#24144=CARTESIAN_POINT('Ctrl Pts',(-18.322862621758,40.5913100061393,123.935361777761)) ;
#24145=CARTESIAN_POINT('Ctrl Pts',(-18.0512693189918,40.4113209257765,124.066262657595)) ;
#24146=CARTESIAN_POINT('Ctrl Pts',(-18.2480294467794,40.6013762304958,123.737449279801)) ;
#24147=CARTESIAN_POINT('Ctrl Pts',(-17.9577246777451,40.421387150133,123.818872622899)) ;
#24148=CARTESIAN_POINT('Ctrl Pts',(-18.2094701938353,40.6112568434155,123.533303511753)) ;
#24149=CARTESIAN_POINT('Ctrl Pts',(-17.9095230457467,40.4312677630526,123.563691114021)) ;
#24150=CARTESIAN_POINT('Ctrl Pts',(-18.206516541867,40.6212501365751,123.323267667439)) ;
#24151=CARTESIAN_POINT('Ctrl Pts',(-17.9058281378729,40.4412610562122,123.30114626875)) ;
#24152=CARTESIAN_POINT('Ctrl Pts',(-18.2398673386455,40.6312011447987,123.11670429861)) ;
#24153=CARTESIAN_POINT('Ctrl Pts',(-17.9475138799179,40.4512120644359,123.042941598617)) ;
#24154=CARTESIAN_POINT('Ctrl Pts',(-18.3093839574438,40.6412496591607,122.917243416711)) ;
#24155=CARTESIAN_POINT('Ctrl Pts',(-18.0344070397604,40.4612605787978,122.793614478542)) ;
#24156=CARTESIAN_POINT('Ctrl Pts',(-18.4101694123091,40.6510911652234,122.736528533016)) ;
#24157=CARTESIAN_POINT('Ctrl Pts',(-18.1603863836437,40.4711020848605,122.567719550063)) ;
#24158=CARTESIAN_POINT('Ctrl Pts',(-18.542325109746,40.6610768178531,122.573458997662)) ;
#24159=CARTESIAN_POINT('Ctrl Pts',(-18.3255788630243,40.4810877374902,122.36388078949)) ;
#24160=CARTESIAN_POINT('Ctrl Pts',(-18.7000440263116,40.671015826698,122.436353330348)) ;
#24161=CARTESIAN_POINT('Ctrl Pts',(-18.5227257140879,40.4910267463351,122.192496536557)) ;
#24162=CARTESIAN_POINT('Ctrl Pts',(-18.8809941836839,40.681056751991,122.327685783444)) ;
#24163=CARTESIAN_POINT('Ctrl Pts',(-18.7489120153398,40.5010676716281,122.056659651422)) ;
#24164=CARTESIAN_POINT('Ctrl Pts',(-19.0750989997885,40.6909470737459,122.253093211541)) ;
#24165=CARTESIAN_POINT('Ctrl Pts',(-18.9915421154482,40.510957993383,121.963416273453)) ;
#24166=CARTESIAN_POINT('Ctrl Pts',(-19.2812929576741,40.7009430470793,122.212614380291)) ;
#24167=CARTESIAN_POINT('Ctrl Pts',(-19.249284101431,40.5209539667164,121.912814957505)) ;
#24168=CARTESIAN_POINT('Ctrl Pts',(-19.4900519469436,40.7108744466613,122.208562124172)) ;
#24169=CARTESIAN_POINT('Ctrl Pts',(-19.5102329048635,40.5308853662985,121.907746825893)) ;
#24170=CARTESIAN_POINT('Ctrl Pts',(-19.6979309739298,40.7208799871384,122.240764687343)) ;
#24171=CARTESIAN_POINT('Ctrl Pts',(-19.7700821945994,40.5408909067755,121.947997275359)) ;
#24172=CARTESIAN_POINT('Ctrl Pts',(-19.8974653853249,40.7309129710697,122.30911862514)) ;
#24173=CARTESIAN_POINT('Ctrl Pts',(-20.0195011590798,40.5509238907068,122.033437044935)) ;
#24174=CARTESIAN_POINT('Ctrl Pts',(-20.0790342263548,40.7407686018965,122.40896792997)) ;
#24175=CARTESIAN_POINT('Ctrl Pts',(-20.2464637604241,40.5607795215337,122.158246335581)) ;
#24176=CARTESIAN_POINT('Ctrl Pts',(-20.2429931194927,40.7507680040897,122.540475873946)) ;
#24177=CARTESIAN_POINT('Ctrl Pts',(-20.4514141919689,40.5707789237268,122.322629146748)) ;
#24178=CARTESIAN_POINT('Ctrl Pts',(-20.3804016988981,40.7606624734508,122.696694794566)) ;
#24179=CARTESIAN_POINT('Ctrl Pts',(-20.623177160939,40.5806733930879,122.517901168788)) ;
#24180=CARTESIAN_POINT('Ctrl Pts',(-20.4903492131892,40.770725587615,122.877396553859)) ;
#24181=CARTESIAN_POINT('Ctrl Pts',(-20.7606139057598,40.5907365072521,122.743776897285)) ;
#24182=CARTESIAN_POINT('Ctrl Pts',(-20.565781026169,40.7805652333314,123.070050005765)) ;
#24183=CARTESIAN_POINT('Ctrl Pts',(-20.8549063786372,40.6005761529685,122.984593090461)) ;
#24184=CARTESIAN_POINT('Ctrl Pts',(-20.6077950411033,40.7906284008871,123.277366104284)) ;
#24185=CARTESIAN_POINT('Ctrl Pts',(-20.9074265587478,40.6106393205242,123.243737629738)) ;
#24186=CARTESIAN_POINT('Ctrl Pts',(-20.6129087024178,40.800522656682,123.485334552873)) ;
#24187=CARTESIAN_POINT('Ctrl Pts',(-20.9138213840196,40.6205335763191,123.50369845043)) ;
#24188=CARTESIAN_POINT('Ctrl Pts',(-20.5822552704826,40.8104644351417,123.692055896881)) ;
#24189=CARTESIAN_POINT('Ctrl Pts',(-20.8755072031584,40.6304753547788,123.762100783259)) ;
#24190=CARTESIAN_POINT('Ctrl Pts',(-20.5158234904619,40.8204671279719,123.891604227127)) ;
#24191=CARTESIAN_POINT('Ctrl Pts',(-20.7924699762297,40.640478047609,124.011537115954)) ;
#24192=CARTESIAN_POINT('Ctrl Pts',(-20.4151748597048,40.8305011499257,124.076979654914)) ;
#24193=CARTESIAN_POINT('Ctrl Pts',(-20.6666615752292,40.6505120695628,124.243257679907)) ;
#24194=CARTESIAN_POINT('Ctrl Pts',(-20.2865434555371,40.8403489410147,124.239210149898)) ;
#24195=CARTESIAN_POINT('Ctrl Pts',(-20.5058740591058,40.6603598606518,124.446047890609)) ;
#24196=CARTESIAN_POINT('Ctrl Pts',(-20.1299205089068,40.8503304655638,124.378837643327)) ;
#24197=CARTESIAN_POINT('Ctrl Pts',(-20.3100969713907,40.6703413852009,124.620584309683)) ;
#24198=CARTESIAN_POINT('Ctrl Pts',(-19.951972487446,40.8602796890547,124.488778577698)) ;
#24199=CARTESIAN_POINT('Ctrl Pts',(-20.0876630799493,40.6802906086918,124.75801282759)) ;
#24200=CARTESIAN_POINT('Ctrl Pts',(-19.7567802099133,40.8702773452713,124.566778486158)) ;
#24201=CARTESIAN_POINT('Ctrl Pts',(-19.8436735816779,40.6902882649084,124.85551512015)) ;
#24202=CARTESIAN_POINT('Ctrl Pts',(-19.5500818247868,40.8803175583263,124.609481079621)) ;
#24203=CARTESIAN_POINT('Ctrl Pts',(-19.5853011891557,40.7003284779634,124.908895920478)) ;
#24204=CARTESIAN_POINT('Ctrl Pts',(-19.3435554371878,40.8901456056026,124.615967681651)) ;
#24205=CARTESIAN_POINT('Ctrl Pts',(-19.3271425182227,40.7101565252397,124.917006738006)) ;
#24206=CARTESIAN_POINT('Ctrl Pts',(-19.1343072045349,40.9001999526349,124.586146876164)) ;
#24207=CARTESIAN_POINT('Ctrl Pts',(-19.0655819825205,40.7202108722721,124.87973320103)) ;
#24208=CARTESIAN_POINT('Ctrl Pts',(-18.9357705406544,40.9101410889635,124.520845573056)) ;
#24209=CARTESIAN_POINT('Ctrl Pts',(-18.8174100404169,40.7301520086006,124.798108890604)) ;
#24210=CARTESIAN_POINT('Ctrl Pts',(-18.7519690818306,40.9200453220432,124.423000581694)) ;
#24211=CARTESIAN_POINT('Ctrl Pts',(-18.5876566119404,40.7400562416803,124.675804537039)) ;
#24212=CARTESIAN_POINT('Ctrl Pts',(-18.585688282195,40.9300920188868,124.292792552293)) ;
#24213=CARTESIAN_POINT('Ctrl Pts',(-18.3798041844874,40.7501029385239,124.513046489696)) ;
#24214=CARTESIAN_POINT('Ctrl Pts',(-18.4464901568893,40.9399875701671,124.138142420818)) ;
#24215=CARTESIAN_POINT('Ctrl Pts',(-18.2058043531865,40.7599984898042,124.319735002295)) ;
#24216=CARTESIAN_POINT('Ctrl Pts',(-18.3344376414912,40.9500496480066,123.958756744201)) ;
#24217=CARTESIAN_POINT('Ctrl Pts',(-18.0657367626924,40.7700605676437,124.095504335531)) ;
#24218=CARTESIAN_POINT('Ctrl Pts',(-18.2568316622771,40.9598923571026,123.766911195192)) ;
#24219=CARTESIAN_POINT('Ctrl Pts',(-17.9687267603788,40.7799032767398,123.855697491767)) ;
#24220=CARTESIAN_POINT('Ctrl Pts',(-18.2125910584586,40.9698830893411,123.561614077019)) ;
#24221=CARTESIAN_POINT('Ctrl Pts',(-17.9134237543617,40.7898940089782,123.599076400319)) ;
#24222=CARTESIAN_POINT('Ctrl Pts',(-18.204750664211,40.9798111145698,123.353032026553)) ;
#24223=CARTESIAN_POINT('Ctrl Pts',(-17.9036209757213,40.799822034207,123.33834843595)) ;
#24224=CARTESIAN_POINT('Ctrl Pts',(-18.2330639112473,40.9897992612204,123.14496244916)) ;
#24225=CARTESIAN_POINT('Ctrl Pts',(-17.9390103972283,40.8098101808575,123.07826099235)) ;
#24226=CARTESIAN_POINT('Ctrl Pts',(-18.297681746232,40.9998342790604,122.944131359391)) ;
#24227=CARTESIAN_POINT('Ctrl Pts',(-18.0197805146774,40.8198451986975,122.827221506658)) ;
#24228=CARTESIAN_POINT('Ctrl Pts',(-18.3943201381265,41.0096990761655,122.760643431724)) ;
#24229=CARTESIAN_POINT('Ctrl Pts',(-18.1405769536225,40.8297099958027,122.597859805826)) ;
#24230=CARTESIAN_POINT('Ctrl Pts',(-18.5221077214792,41.0196598085217,122.594742227815)) ;
#24231=CARTESIAN_POINT('Ctrl Pts',(-18.3003100262152,40.8396707281588,122.390481778754)) ;
#24232=CARTESIAN_POINT('Ctrl Pts',(-18.6781171729852,41.0296932709187,122.452788170327)) ;
#24233=CARTESIAN_POINT('Ctrl Pts',(-18.4953203364736,40.8497041905558,122.213037685501)) ;
#24234=CARTESIAN_POINT('Ctrl Pts',(-18.8536177054508,41.0395788051301,122.341428905828)) ;
#24235=CARTESIAN_POINT('Ctrl Pts',(-18.7146955767961,40.8595897247672,122.073836456238)) ;
#24236=CARTESIAN_POINT('Ctrl Pts',(-19.0492301850846,41.0496436458101,122.260823818413)) ;
#24237=CARTESIAN_POINT('Ctrl Pts',(-18.9592101605245,40.8696545654472,121.973078301155)) ;
#24238=CARTESIAN_POINT('Ctrl Pts',(-19.2514386207072,41.0594917775389,122.216286024392)) ;
#24239=CARTESIAN_POINT('Ctrl Pts',(-19.2119712899475,40.8795026971761,121.917403865115)) ;
#24240=CARTESIAN_POINT('Ctrl Pts',(-19.4620301676676,41.0695192745291,122.206830853245)) ;
#24241=CARTESIAN_POINT('Ctrl Pts',(-19.4752106016322,40.8895301941662,121.905583046178)) ;
#24242=CARTESIAN_POINT('Ctrl Pts',(-19.6710285196364,41.0795477265741,122.234643377154)) ;
#24243=CARTESIAN_POINT('Ctrl Pts',(-19.7364587404572,40.8995586462113,121.940346685251)) ;
#24244=CARTESIAN_POINT('Ctrl Pts',(-19.8684484239612,41.0893929931382,122.29677641338)) ;
#24245=CARTESIAN_POINT('Ctrl Pts',(-19.9832352577145,40.9094039127754,122.018011497405)) ;
#24246=CARTESIAN_POINT('Ctrl Pts',(-20.05506817094,41.0993836660792,122.39316265703)) ;
#24247=CARTESIAN_POINT('Ctrl Pts',(-20.2165109099258,40.9193945857163,122.138492853158)) ;
#24248=CARTESIAN_POINT('Ctrl Pts',(-20.2226153017789,41.1094215481676,122.521458694971)) ;
#24249=CARTESIAN_POINT('Ctrl Pts',(-20.4259458604295,40.9294324678048,122.29886132802)) ;
#24250=CARTESIAN_POINT('Ctrl Pts',(-20.3628619913098,41.1192659186073,122.673663617627)) ;
#24251=CARTESIAN_POINT('Ctrl Pts',(-20.6012563123727,40.9392768382444,122.489117146691)) ;
#24252=CARTESIAN_POINT('Ctrl Pts',(-20.4764734479912,41.1292507460027,122.850139489613)) ;
#24253=CARTESIAN_POINT('Ctrl Pts',(-20.7432721400069,40.9492616656398,122.709711313099)) ;
#24254=CARTESIAN_POINT('Ctrl Pts',(-20.5574566491448,41.139190191408,123.042799763275)) ;
#24255=CARTESIAN_POINT('Ctrl Pts',(-20.844502824681,40.9592011110451,122.950536538216)) ;
#24256=CARTESIAN_POINT('Ctrl Pts',(-20.6041559807991,41.1492301956939,123.248619953668)) ;
#24257=CARTESIAN_POINT('Ctrl Pts',(-20.9028785373405,40.969241115331,123.20781127082)) ;
#24258=CARTESIAN_POINT('Ctrl Pts',(-20.6143967382331,41.1591173048795,123.456249137288)) ;
#24259=CARTESIAN_POINT('Ctrl Pts',(-20.9156810985871,40.9791282245166,123.46734861019)) ;
#24260=CARTESIAN_POINT('Ctrl Pts',(-20.5883994319064,41.169117364782,123.664835776685)) ;
#24261=CARTESIAN_POINT('Ctrl Pts',(-20.8831859202662,40.9891282844191,123.728082234662)) ;
#24262=CARTESIAN_POINT('Ctrl Pts',(-20.5272409128475,41.1790347806967,123.864195390867)) ;
#24263=CARTESIAN_POINT('Ctrl Pts',(-20.8067389220528,40.9990457003338,123.977282854265)) ;
#24264=CARTESIAN_POINT('Ctrl Pts',(-20.4311340846493,41.1890815954375,124.052246102088)) ;
#24265=CARTESIAN_POINT('Ctrl Pts',(-20.6866067690655,41.0090925150746,124.212346711425)) ;
#24266=CARTESIAN_POINT('Ctrl Pts',(-20.3061390393343,41.1989570726341,124.218058301868)) ;
#24267=CARTESIAN_POINT('Ctrl Pts',(-20.5303634279957,41.0189679922713,124.419613620439)) ;
#24268=CARTESIAN_POINT('Ctrl Pts',(-20.1516052416653,41.2090131683554,124.362275980325)) ;
#24269=CARTESIAN_POINT('Ctrl Pts',(-20.3371972791705,41.0290240879925,124.599886515678)) ;
#24270=CARTESIAN_POINT('Ctrl Pts',(-19.977229302393,41.2189063303704,124.475710615594)) ;
#24271=CARTESIAN_POINT('Ctrl Pts',(-20.1192272911797,41.0389172500076,124.741681401867)) ;
#24272=CARTESIAN_POINT('Ctrl Pts',(-19.782620580465,41.228968566393,124.558568223159)) ;
#24273=CARTESIAN_POINT('Ctrl Pts',(-19.8759671921668,41.0489794860302,124.845254462117)) ;
#24274=CARTESIAN_POINT('Ctrl Pts',(-19.5810123835409,41.238813032022,124.605369966311)) ;
#24275=CARTESIAN_POINT('Ctrl Pts',(-19.6239559484601,41.0588239516591,124.903758180381)) ;
#24276=CARTESIAN_POINT('Ctrl Pts',(-19.3719656317782,41.2487731247261,124.617339157751)) ;
#24277=CARTESIAN_POINT('Ctrl Pts',(-19.3626471098562,41.0687840443633,124.918720690763)) ;
#24278=CARTESIAN_POINT('Ctrl Pts',(-19.1624388090685,41.2588114137072,124.592224884282)) ;
#24279=CARTESIAN_POINT('Ctrl Pts',(-19.1007386053563,41.0788223333443,124.887329010187)) ;
#24280=CARTESIAN_POINT('Ctrl Pts',(-18.9636200217074,41.2686847368134,124.532486383853)) ;
#24281=CARTESIAN_POINT('Ctrl Pts',(-18.8522137572535,41.0886956564505,124.812656518733)) ;
#24282=CARTESIAN_POINT('Ctrl Pts',(-18.7745367667636,41.2787579208985,124.437217363327)) ;
#24283=CARTESIAN_POINT('Ctrl Pts',(-18.6158596069558,41.0987688405356,124.693571352366)) ;
#24284=CARTESIAN_POINT('Ctrl Pts',(-18.6088938849064,41.2885784331864,124.313905580801)) ;
#24285=CARTESIAN_POINT('Ctrl Pts',(-18.4088042083935,41.1085893528235,124.539431437794)) ;
#24286=CARTESIAN_POINT('Ctrl Pts',(-18.4633794200554,41.2986564293022,124.159977351109)) ;
#24287=CARTESIAN_POINT('Ctrl Pts',(-18.2269108302998,41.1186673489393,124.347022071441)) ;
#24288=CARTESIAN_POINT('Ctrl Pts',(-18.34929862132,41.3085105042855,123.986997787861)) ;
#24289=CARTESIAN_POINT('Ctrl Pts',(-18.0843084263497,41.1285214239226,124.130796993338)) ;
#24290=CARTESIAN_POINT('Ctrl Pts',(-18.2650562986397,41.3185743858692,123.79296185912)) ;
#24291=CARTESIAN_POINT('Ctrl Pts',(-17.9790049811939,41.1385853055063,123.888252695276)) ;
#24292=CARTESIAN_POINT('Ctrl Pts',(-18.2166879254847,41.3284578118429,123.590852828316)) ;
#24293=CARTESIAN_POINT('Ctrl Pts',(-17.9185435301409,41.14846873148,123.63561553845)) ;
#24294=CARTESIAN_POINT('Ctrl Pts',(-18.2036681221716,41.338458415764,123.381049020955)) ;
#24295=CARTESIAN_POINT('Ctrl Pts',(-17.9022681371798,41.1584693354011,123.37336067713)) ;
#24296=CARTESIAN_POINT('Ctrl Pts',(-18.2269611110855,41.3483782001018,123.173770725139)) ;
#24297=CARTESIAN_POINT('Ctrl Pts',(-17.931383888056,41.168389119739,123.114261971927)) ;
#24298=CARTESIAN_POINT('Ctrl Pts',(-18.2866756180986,41.3584255504587,122.971196494413)) ;
#24299=CARTESIAN_POINT('Ctrl Pts',(-18.0060263785442,41.1784364700958,122.861044240447)) ;
#24300=CARTESIAN_POINT('Ctrl Pts',(-18.3788795710986,41.368302892693,122.785091205517)) ;
#24301=CARTESIAN_POINT('Ctrl Pts',(-18.1212813811983,41.1883138123301,122.62841137183)) ;
#24302=CARTESIAN_POINT('Ctrl Pts',(-18.5043585823623,41.3783727737676,122.614637642039)) ;
#24303=CARTESIAN_POINT('Ctrl Pts',(-18.2781294851284,41.1983836934047,122.415344458296)) ;
#24304=CARTESIAN_POINT('Ctrl Pts',(-18.6537818292948,41.3882024789693,122.471833456278)) ;
#24305=CARTESIAN_POINT('Ctrl Pts',(-18.4649093676713,41.2082133986064,122.236837854703)) ;
#24306=CARTESIAN_POINT('Ctrl Pts',(-18.8296579695578,41.3982691401357,122.35418375427)) ;
#24307=CARTESIAN_POINT('Ctrl Pts',(-18.684754038693,41.2182800597728,122.089775689271)) ;
#24308=CARTESIAN_POINT('Ctrl Pts',(-19.0200041203782,41.408159362003,122.270450878119)) ;
#24309=CARTESIAN_POINT('Ctrl Pts',(-18.922687539533,41.2281702816401,121.985108837478)) ;
#24310=CARTESIAN_POINT('Ctrl Pts',(-19.2239333482095,41.4181515381132,122.220092117685)) ;
#24311=CARTESIAN_POINT('Ctrl Pts',(-19.1775992382533,41.2381624577503,121.922160157756)) ;
#24312=CARTESIAN_POINT('Ctrl Pts',(-19.432913401362,41.4281143682258,122.206147099919)) ;
#24313=CARTESIAN_POINT('Ctrl Pts',(-19.4388247420797,41.2481252878629,121.904728591906)) ;
#24314=CARTESIAN_POINT('Ctrl Pts',(-19.6399945794,41.4380185806261,122.228042536446)) ;
#24315=CARTESIAN_POINT('Ctrl Pts',(-19.6976771545585,41.2580295002633,121.932097935364)) ;
#24316=CARTESIAN_POINT('Ctrl Pts',(-19.84319524037,41.448079294714,122.286638879611)) ;
#24317=CARTESIAN_POINT('Ctrl Pts',(-19.9516776747255,41.2680902143511,122.005343143406)) ;
#24318=CARTESIAN_POINT('Ctrl Pts',(-20.0291359735094,41.4579187976968,122.377353855789)) ;
#24319=CARTESIAN_POINT('Ctrl Pts',(-20.1841049252899,41.2779297173339,122.118737500505)) ;
#24320=CARTESIAN_POINT('Ctrl Pts',(-20.2004294013988,41.4679849362632,122.501563731977)) ;
#24321=CARTESIAN_POINT('Ctrl Pts',(-20.3982213435744,41.2879958559003,122.273999666852)) ;
#24322=CARTESIAN_POINT('Ctrl Pts',(-20.3448588998162,41.4778674507492,122.650955267273)) ;
#24323=CARTESIAN_POINT('Ctrl Pts',(-20.5787589735412,41.2978783703863,122.460739928102)) ;
#24324=CARTESIAN_POINT('Ctrl Pts',(-20.4627539040108,41.4878597501047,122.824784252551)) ;
#24325=CARTESIAN_POINT('Ctrl Pts',(-20.7261276816334,41.3078706697419,122.678026456324)) ;
#24326=CARTESIAN_POINT('Ctrl Pts',(-20.5484123348916,41.4978128170581,123.01572690911)) ;
#24327=CARTESIAN_POINT('Ctrl Pts',(-20.8332007283246,41.3178237366953,122.916705335846)) ;
#24328=CARTESIAN_POINT('Ctrl Pts',(-20.5999387117747,41.5078475252634,123.220282510794)) ;
#24329=CARTESIAN_POINT('Ctrl Pts',(-20.8976084793145,41.3278584449005,123.172399737523)) ;
#24330=CARTESIAN_POINT('Ctrl Pts',(-20.6150963668154,41.5177357461675,123.42762288197)) ;
#24331=CARTESIAN_POINT('Ctrl Pts',(-20.9165553817096,41.3377466658047,123.431576287923)) ;
#24332=CARTESIAN_POINT('Ctrl Pts',(-20.5941420991674,41.527730169198,123.636678083396)) ;
#24333=CARTESIAN_POINT('Ctrl Pts',(-20.8903621464779,41.3477410888351,123.692895458737)) ;
#24334=CARTESIAN_POINT('Ctrl Pts',(-20.5374038460003,41.5376755086441,123.837915099807)) ;
#24335=CARTESIAN_POINT('Ctrl Pts',(-20.8194388311831,41.3576864282813,123.944442205965)) ;
#24336=CARTESIAN_POINT('Ctrl Pts',(-20.4469513423603,41.5476228532555,124.026477171833)) ;
#24337=CARTESIAN_POINT('Ctrl Pts',(-20.7063724848582,41.3676337728926,124.180145089931)) ;
#24338=CARTESIAN_POINT('Ctrl Pts',(-20.3237166893896,41.5576707486665,124.198034788354)) ;
#24339=CARTESIAN_POINT('Ctrl Pts',(-20.5523289698857,41.3776816683036,124.394591659)) ;
#24340=CARTESIAN_POINT('Ctrl Pts',(-20.1756958626887,41.5675183941458,124.342779195868)) ;
#24341=CARTESIAN_POINT('Ctrl Pts',(-20.3673015896202,41.387529313783,124.575522794134)) ;
#24342=CARTESIAN_POINT('Ctrl Pts',(-20.0031915988338,41.5774801080598,124.461512163313)) ;
#24343=CARTESIAN_POINT('Ctrl Pts',(-20.1516704586702,41.397491027697,124.723938642442)) ;
#24344=CARTESIAN_POINT('Ctrl Pts',(-19.8112800553437,41.5875087323508,124.548840187101)) ;
#24345=CARTESIAN_POINT('Ctrl Pts',(-19.911780850099,41.4075196519879,124.833098044345)) ;
#24346=CARTESIAN_POINT('Ctrl Pts',(-19.6095677146579,41.5974190930075,124.600957112613)) ;
#24347=CARTESIAN_POINT('Ctrl Pts',(-19.6596394073023,41.4174300126446,124.898243770015)) ;
#24348=CARTESIAN_POINT('Ctrl Pts',(-19.4013858198479,41.6073537915808,124.617849546448)) ;
#24349=CARTESIAN_POINT('Ctrl Pts',(-19.3994113076568,41.4273647112179,124.91935848404)) ;
#24350=CARTESIAN_POINT('Ctrl Pts',(-19.1912280423145,41.617395616435,124.597921301321)) ;
#24351=CARTESIAN_POINT('Ctrl Pts',(-19.1367143515178,41.4374065360721,124.894447395017)) ;
#24352=CARTESIAN_POINT('Ctrl Pts',(-18.990832747362,41.6272801901794,124.542852864692)) ;
#24353=CARTESIAN_POINT('Ctrl Pts',(-18.8862194476765,41.4472911098165,124.825610729058)) ;
#24354=CARTESIAN_POINT('Ctrl Pts',(-18.8007506253046,41.6372820395426,124.453017154148)) ;
#24355=CARTESIAN_POINT('Ctrl Pts',(-18.6486170762246,41.4572929591797,124.713315149718)) ;
#24356=CARTESIAN_POINT('Ctrl Pts',(-18.6304363747329,41.6472013411166,124.332637276004)) ;
#24357=CARTESIAN_POINT('Ctrl Pts',(-18.4357242323319,41.4672122607537,124.562839022651)) ;
#24358=CARTESIAN_POINT('Ctrl Pts',(-18.4817919543754,41.6572454494619,124.182685192246)) ;
#24359=CARTESIAN_POINT('Ctrl Pts',(-18.2499195837942,41.477256369099,124.375398346987)) ;
#24360=CARTESIAN_POINT('Ctrl Pts',(-18.3632889695078,41.6671298729041,124.011973794938)) ;
#24361=CARTESIAN_POINT('Ctrl Pts',(-18.1017911287502,41.4871407925413,124.162007655832)) ;
#24362=CARTESIAN_POINT('Ctrl Pts',(-18.2746407632442,41.6771462348136,123.820958583722)) ;
#24363=CARTESIAN_POINT('Ctrl Pts',(-17.9909819762134,41.4971571544507,123.923238127084)) ;
#24364=CARTESIAN_POINT('Ctrl Pts',(-18.2209377342613,41.687182890319,123.616916772057)) ;
#24365=CARTESIAN_POINT('Ctrl Pts',(-17.9238542028585,41.5071938099561,123.66818572458)) ;
#24366=CARTESIAN_POINT('Ctrl Pts',(-18.2032737429254,41.6970130205083,123.410988166114)) ;
#24367=CARTESIAN_POINT('Ctrl Pts',(-17.9017753134138,41.5170239401454,123.410773438911)) ;
#24368=CARTESIAN_POINT('Ctrl Pts',(-18.2220155993058,41.7070890735982,123.200029060193)) ;
#24369=CARTESIAN_POINT('Ctrl Pts',(-17.9252038428856,41.5270999932353,123.147075094843)) ;
#24370=CARTESIAN_POINT('Ctrl Pts',(-18.2757906963554,41.716941302784,122.999961670963)) ;
#24371=CARTESIAN_POINT('Ctrl Pts',(-17.9924242809587,41.5369522224211,122.896990000681)) ;
#24372=CARTESIAN_POINT('Ctrl Pts',(-18.3652603008448,41.7270145105833,122.808056320445)) ;
#24373=CARTESIAN_POINT('Ctrl Pts',(-18.1042623444851,41.5470254302204,122.657109249406)) ;
#24374=CARTESIAN_POINT('Ctrl Pts',(-18.4839724624689,41.7368560219347,122.638585553312)) ;
#24375=CARTESIAN_POINT('Ctrl Pts',(-18.2526543868681,41.5568669415718,122.445270485562)) ;
#24376=CARTESIAN_POINT('Ctrl Pts',(-18.6315099791709,41.7468169599722,122.489983799293)) ;
#24377=CARTESIAN_POINT('Ctrl Pts',(-18.4370777102109,41.5668278796093,122.259519138152)) ;
#24378=CARTESIAN_POINT('Ctrl Pts',(-18.8041736856207,41.7568548218972,122.368670001095)) ;
#24379=CARTESIAN_POINT('Ctrl Pts',(-18.6529080737898,41.5768657415343,122.107878162832)) ;
#24380=CARTESIAN_POINT('Ctrl Pts',(-18.9920269431984,41.7667290078943,122.280273355514)) ;
#24381=CARTESIAN_POINT('Ctrl Pts',(-18.8877262423687,41.5867399275314,121.997383365689)) ;
#24382=CARTESIAN_POINT('Ctrl Pts',(-19.1963027713809,41.7767991674721,122.224790072043)) ;
#24383=CARTESIAN_POINT('Ctrl Pts',(-19.1430711045837,41.5968100871093,121.928030886543)) ;
#24384=CARTESIAN_POINT('Ctrl Pts',(-19.4021553537775,41.786630914898,122.205937341071)) ;
#24385=CARTESIAN_POINT('Ctrl Pts',(-19.4003882644743,41.6066418345351,121.904466477439)) ;
#24386=CARTESIAN_POINT('Ctrl Pts',(-19.6124500007053,41.7966669949693,122.222921105174)) ;
#24387=CARTESIAN_POINT('Ctrl Pts',(-19.6632563157754,41.6166779146064,121.925697979521)) ;
#24388=CARTESIAN_POINT('Ctrl Pts',(-19.8161003455475,41.8066840418218,122.27657994795)) ;
#24389=CARTESIAN_POINT('Ctrl Pts',(-19.9178188413347,41.6266949614589,121.992773118902)) ;
#24390=CARTESIAN_POINT('Ctrl Pts',(-20.004923629097,41.8165662999884,122.363238250864)) ;
#24391=CARTESIAN_POINT('Ctrl Pts',(-20.1538480381938,41.6365772196255,122.10109797781)) ;
#24392=CARTESIAN_POINT('Ctrl Pts',(-20.1777719329602,41.8265539827847,122.482413681147)) ;
#24393=CARTESIAN_POINT('Ctrl Pts',(-20.3699075386073,41.6465649024218,122.250068895617)) ;
#24394=CARTESIAN_POINT('Ctrl Pts',(-20.326844928488,41.8365006395015,122.629102840794)) ;
#24395=CARTESIAN_POINT('Ctrl Pts',(-20.556247785553,41.6565115591386,122.433432011487)) ;
#24396=CARTESIAN_POINT('Ctrl Pts',(-20.4493206526294,41.8465576975816,122.801419365625)) ;
#24397=CARTESIAN_POINT('Ctrl Pts',(-20.7093408277522,41.6665686172188,122.648828544842)) ;
#24398=CARTESIAN_POINT('Ctrl Pts',(-20.5381348768749,41.8563758771311,122.98775540366)) ;
#24399=CARTESIAN_POINT('Ctrl Pts',(-20.8203574276063,41.6763867967682,122.881750559428)) ;
#24400=CARTESIAN_POINT('Ctrl Pts',(-20.5950148919747,41.86641181157,123.190925085264)) ;
#24401=CARTESIAN_POINT('Ctrl Pts',(-20.8914554133569,41.6864227312072,123.135713115928)) ;
#24402=CARTESIAN_POINT('Ctrl Pts',(-20.615129903165,41.876436465999,123.400720653862)) ;
#24403=CARTESIAN_POINT('Ctrl Pts',(-20.9165972820437,41.6964473856362,123.397957733958)) ;
#24404=CARTESIAN_POINT('Ctrl Pts',(-20.5992555683587,41.8862884855786,123.607234834638)) ;
#24405=CARTESIAN_POINT('Ctrl Pts',(-20.8967522553727,41.7062994052157,123.656101312759)) ;
#24406=CARTESIAN_POINT('Ctrl Pts',(-20.5473561444667,41.8962793992935,123.810736345392)) ;
#24407=CARTESIAN_POINT('Ctrl Pts',(-20.8318758704315,41.7162903189306,123.910477841226)) ;
#24408=CARTESIAN_POINT('Ctrl Pts',(-20.4616446993946,41.9061973881331,124.000839502752)) ;
#24409=CARTESIAN_POINT('Ctrl Pts',(-20.7247343585358,41.7262083077702,124.148106422392)) ;
#24410=CARTESIAN_POINT('Ctrl Pts',(-20.3429884977472,41.9162254988639,124.175080591613)) ;
#24411=CARTESIAN_POINT('Ctrl Pts',(-20.5764123274112,41.736236418501,124.365906529172)) ;
#24412=CARTESIAN_POINT('Ctrl Pts',(-20.1980255650348,41.9261106967723,124.323996156688)) ;
#24413=CARTESIAN_POINT('Ctrl Pts',(-20.395206571467,41.7461216164094,124.552049981452)) ;
#24414=CARTESIAN_POINT('Ctrl Pts',(-20.0279320557978,41.9360999720403,124.447175593972)) ;
#24415=CARTESIAN_POINT('Ctrl Pts',(-20.1825881915492,41.7561108916774,124.706022484706)) ;
#24416=CARTESIAN_POINT('Ctrl Pts',(-19.837857448319,41.9461414302098,124.539013945011)) ;
#24417=CARTESIAN_POINT('Ctrl Pts',(-19.944994054816,41.7661523498469,124.820818389465)) ;
#24418=CARTESIAN_POINT('Ctrl Pts',(-19.6390644945786,41.9559728939981,124.595621547206)) ;
#24419=CARTESIAN_POINT('Ctrl Pts',(-19.6965012965203,41.7759838136352,124.891575936423)) ;
#24420=CARTESIAN_POINT('Ctrl Pts',(-19.4299150619604,41.965977826302,124.617688613248)) ;
#24421=CARTESIAN_POINT('Ctrl Pts',(-19.4350641759092,41.7859887459391,124.919157369809)) ;
#24422=CARTESIAN_POINT('Ctrl Pts',(-19.2204473086949,41.9759641901967,124.603013545437)) ;
#24423=CARTESIAN_POINT('Ctrl Pts',(-19.1732294916453,41.7959751098338,124.900811143185)) ;
#24424=CARTESIAN_POINT('Ctrl Pts',(-19.0159203877433,41.9859938190826,124.551823701844)) ;
#24425=CARTESIAN_POINT('Ctrl Pts',(-18.9175714408772,41.8060047387197,124.836821562451)) ;
#24426=CARTESIAN_POINT('Ctrl Pts',(-18.8262081647961,41.995869041191,124.467451255716)) ;
#24427=CARTESIAN_POINT('Ctrl Pts',(-18.6804315219461,41.8158799608281,124.731353527358)) ;
#24428=CARTESIAN_POINT('Ctrl Pts',(-18.6517356024177,42.0058702535881,124.350176231649)) ;
#24429=CARTESIAN_POINT('Ctrl Pts',(-18.4623421036418,41.8258811732252,124.584757637499)) ;
#24430=CARTESIAN_POINT('Ctrl Pts',(-18.5014918306554,42.0157788328236,124.205833220851)) ;
#24431=CARTESIAN_POINT('Ctrl Pts',(-18.2745387790295,41.8357897524607,124.404326737909)) ;
#24432=CARTESIAN_POINT('Ctrl Pts',(-18.376872413352,42.0258336853796,124.035131663706)) ;
#24433=CARTESIAN_POINT('Ctrl Pts',(-18.1187665880947,41.8458446050167,124.190948411598)) ;
#24434=CARTESIAN_POINT('Ctrl Pts',(-18.285357700117,42.0356922676544,123.849131188738)) ;
#24435=CARTESIAN_POINT('Ctrl Pts',(-18.0043751834666,41.8557031872915,123.958446111396)) ;
#24436=CARTESIAN_POINT('Ctrl Pts',(-18.2261951447151,42.0457603970971,123.645935941914)) ;
#24437=CARTESIAN_POINT('Ctrl Pts',(-17.93042449407,41.8657713167342,123.70445148532)) ;
#24438=CARTESIAN_POINT('Ctrl Pts',(-18.2037096295155,42.0556158687862,123.439949227679)) ;
#24439=CARTESIAN_POINT('Ctrl Pts',(-17.9023200741687,41.8756267884233,123.446967189866)) ;
#24440=CARTESIAN_POINT('Ctrl Pts',(-18.2168940215252,42.0656107171724,123.230246957662)) ;
#24441=CARTESIAN_POINT('Ctrl Pts',(-17.9188032302922,41.8856216368096,123.184839420313)) ;
#24442=CARTESIAN_POINT('Ctrl Pts',(-18.2669137943528,42.0756420139569,123.025370929616)) ;
#24443=CARTESIAN_POINT('Ctrl Pts',(-17.9813304619599,41.895652933594,122.928744998837)) ;
#24444=CARTESIAN_POINT('Ctrl Pts',(-18.3500517364716,42.085508550167,122.835328127626)) ;
#24445=CARTESIAN_POINT('Ctrl Pts',(-18.0852555186611,41.9055194698041,122.691192079478)) ;
#24446=CARTESIAN_POINT('Ctrl Pts',(-18.4660321364788,42.0954959731278,122.660329302149)) ;
#24447=CARTESIAN_POINT('Ctrl Pts',(-18.2302333322929,41.9155068927649,122.472444933182)) ;
#24448=CARTESIAN_POINT('Ctrl Pts',(-18.6099789814412,42.1054409121476,122.508661371675)) ;
#24449=CARTESIAN_POINT('Ctrl Pts',(-18.4101690101242,41.9254518317847,122.282861709824)) ;
#24450=CARTESIAN_POINT('Ctrl Pts',(-18.7797885338698,42.1154857980076,122.383148139199)) ;
#24451=CARTESIAN_POINT('Ctrl Pts',(-18.6224325374237,41.9354967176447,122.125972345834)) ;
#24452=CARTESIAN_POINT('Ctrl Pts',(-18.9654610961427,42.1253543330938,122.290568762634)) ;
#24453=CARTESIAN_POINT('Ctrl Pts',(-18.8545248231622,41.9453652527309,122.010250360349)) ;
#24454=CARTESIAN_POINT('Ctrl Pts',(-19.1661696006187,42.1353202011005,122.230497998175)) ;
#24455=CARTESIAN_POINT('Ctrl Pts',(-19.1054113849967,41.9553311207376,121.935164518734)) ;
#24456=CARTESIAN_POINT('Ctrl Pts',(-19.3754959713858,42.145342848553,122.206283829226)) ;
#24457=CARTESIAN_POINT('Ctrl Pts',(-19.3670697024523,41.9653537681901,121.904899528248)) ;
#24458=CARTESIAN_POINT('Ctrl Pts',(-19.5837472933625,42.1552664875606,122.218600651272)) ;
#24459=CARTESIAN_POINT('Ctrl Pts',(-19.6273839317657,41.9752774071977,121.920298317369)) ;
#24460=CARTESIAN_POINT('Ctrl Pts',(-19.7872248880091,42.1652092125663,122.266499710306)) ;
#24461=CARTESIAN_POINT('Ctrl Pts',(-19.8817304496807,41.9852201322034,121.980174899417)) ;
#24462=CARTESIAN_POINT('Ctrl Pts',(-19.98116015884,42.1752548186182,122.350078644094)) ;
#24463=CARTESIAN_POINT('Ctrl Pts',(-20.1241484576752,41.9952657382553,122.084651122132)) ;
#24464=CARTESIAN_POINT('Ctrl Pts',(-20.1545514692075,42.1851162411393,122.463760650406)) ;
#24465=CARTESIAN_POINT('Ctrl Pts',(-20.3408862916986,42.0051271607764,122.22675611249)) ;
#24466=CARTESIAN_POINT('Ctrl Pts',(-20.3078045675298,42.1951098095885,122.607431591005)) ;
#24467=CARTESIAN_POINT('Ctrl Pts',(-20.5324507967766,42.0151207292256,122.406346888385)) ;
#24468=CARTESIAN_POINT('Ctrl Pts',(-20.4330485966864,42.2050352803438,122.774367875557)) ;
#24469=CARTESIAN_POINT('Ctrl Pts',(-20.6890036597013,42.0250461999809,122.615019061482)) ;
#24470=CARTESIAN_POINT('Ctrl Pts',(-20.528359134433,42.2150629542996,122.96237648736)) ;
#24471=CARTESIAN_POINT('Ctrl Pts',(-20.808139363818,42.0350738739368,122.850031069966)) ;
#24472=CARTESIAN_POINT('Ctrl Pts',(-20.5889282022475,42.2249501323413,123.161244468246)) ;
#24473=CARTESIAN_POINT('Ctrl Pts',(-20.8838479741626,42.0449610519785,123.098617303755)) ;
#24474=CARTESIAN_POINT('Ctrl Pts',(-20.6145455202288,42.2349785117095,123.370482821943)) ;
#24475=CARTESIAN_POINT('Ctrl Pts',(-20.9158670631571,42.0549894313466,123.360164459768)) ;
#24476=CARTESIAN_POINT('Ctrl Pts',(-20.6037026584376,42.244872754431,123.57823145244)) ;
#24477=CARTESIAN_POINT('Ctrl Pts',(-20.9023097751863,42.0648836740681,123.619854631483)) ;
#24478=CARTESIAN_POINT('Ctrl Pts',(-20.5408518696117,42.2582256710819,123.851819040007)) ;
#24479=CARTESIAN_POINT('Ctrl Pts',(-20.8237470249053,42.078236590719,123.961816174747)) ;
#24480=CARTESIAN_POINT('Ctrl Pts',(-20.4095172303577,42.2714281888286,124.099989933585)) ;
#24481=CARTESIAN_POINT('Ctrl Pts',(-20.6595997814835,42.0914391084657,124.272009590654)) ;
#24482=CARTESIAN_POINT('Ctrl Pts',(-20.2186534632653,42.2847840941096,124.305832996325)) ;
#24483=CARTESIAN_POINT('Ctrl Pts',(-20.4209837962718,42.1047950137467,124.529355053645)) ;
#24484=CARTESIAN_POINT('Ctrl Pts',(-20.0529351292621,42.2946807427474,124.431692913237)) ;
#24485=CARTESIAN_POINT('Ctrl Pts',(-20.2138409514704,42.1146916623845,124.686668820964)) ;
#24486=CARTESIAN_POINT('Ctrl Pts',(-19.8651277354385,42.3047288807999,124.528356903845)) ;
#24487=CARTESIAN_POINT('Ctrl Pts',(-19.9790784982733,42.124739800437,124.807498749042)) ;
#24488=CARTESIAN_POINT('Ctrl Pts',(-19.6665158493402,42.3146198409776,124.58996703809)) ;
#24489=CARTESIAN_POINT('Ctrl Pts',(-19.7308134332186,42.1346307606148,124.884508092935)) ;
#24490=CARTESIAN_POINT('Ctrl Pts',(-19.4581683197363,42.3246126768544,124.616948547445)) ;
#24491=CARTESIAN_POINT('Ctrl Pts',(-19.4703782998092,42.1446235964915,124.918232356421)) ;
#24492=CARTESIAN_POINT('Ctrl Pts',(-19.2473681600248,42.334651771856,124.606814985885)) ;
#24493=CARTESIAN_POINT('Ctrl Pts',(-19.2068788945409,42.1546626914931,124.905562765929)) ;
#24494=CARTESIAN_POINT('Ctrl Pts',(-19.0455307327722,42.3444891277071,124.561634051858)) ;
#24495=CARTESIAN_POINT('Ctrl Pts',(-18.9545800921988,42.1645000473443,124.849083179674)) ;
#24496=CARTESIAN_POINT('Ctrl Pts',(-18.7855849758638,42.3578820756379,124.453519111834)) ;
#24497=CARTESIAN_POINT('Ctrl Pts',(-18.629663451881,42.177892995275,124.713940021359)) ;
#24498=CARTESIAN_POINT('Ctrl Pts',(-18.5635083695273,42.3710487520648,124.282885771656)) ;
#24499=CARTESIAN_POINT('Ctrl Pts',(-18.3520925365356,42.1910596717019,124.500678451702)) ;
#24500=CARTESIAN_POINT('Ctrl Pts',(-18.392149943478,42.3844335334716,124.059804324477)) ;
#24501=CARTESIAN_POINT('Ctrl Pts',(-18.1378563760038,42.2044444531087,124.221781306289)) ;
#24502=CARTESIAN_POINT('Ctrl Pts',(-18.2962255678194,42.3942953161154,123.875955923581)) ;
#24503=CARTESIAN_POINT('Ctrl Pts',(-18.0179616237773,42.2143062357526,123.991978653527)) ;
#24504=CARTESIAN_POINT('Ctrl Pts',(-18.2325120769393,42.4042944640685,123.675676595792)) ;
#24505=CARTESIAN_POINT('Ctrl Pts',(-17.9383202716689,42.2243053837056,123.741625973935)) ;
#24506=CARTESIAN_POINT('Ctrl Pts',(-18.2046075101168,42.4141972566856,123.469320833634)) ;
#24507=CARTESIAN_POINT('Ctrl Pts',(-17.9034419632737,42.2342081763227,123.483683307464)) ;
#24508=CARTESIAN_POINT('Ctrl Pts',(-18.2131324921205,42.4242468365765,123.258275057059)) ;
#24509=CARTESIAN_POINT('Ctrl Pts',(-17.9141036164672,42.2442577562136,123.21987047093)) ;
#24510=CARTESIAN_POINT('Ctrl Pts',(-18.271742279274,42.437433910386,122.987181315059)) ;
#24511=CARTESIAN_POINT('Ctrl Pts',(-17.9873542558445,42.2574448300231,122.881031053165)) ;
#24512=CARTESIAN_POINT('Ctrl Pts',(-18.4346521343874,42.4541867003572,122.670610361465)) ;
#24513=CARTESIAN_POINT('Ctrl Pts',(-18.1910268972478,42.2741976199943,122.48527825742)) ;
#24514=CARTESIAN_POINT('Ctrl Pts',(-18.6920409930995,42.4706753524519,122.432258546102)) ;
#24515=CARTESIAN_POINT('Ctrl Pts',(-18.5127023287359,42.290686272089,122.187393477367)) ;
#24516=CARTESIAN_POINT('Ctrl Pts',(-18.9400618332129,42.4840321786353,122.300845882537)) ;
#24517=CARTESIAN_POINT('Ctrl Pts',(-18.8227825349679,42.3040430982724,122.023091316242)) ;
#24518=CARTESIAN_POINT('Ctrl Pts',(-19.1380453310715,42.4939285635132,122.236723926044)) ;
#24519=CARTESIAN_POINT('Ctrl Pts',(-19.0702507619016,42.3139394831503,121.942948929694)) ;
#24520=CARTESIAN_POINT('Ctrl Pts',(-19.346318954824,42.5039350780337,122.2075435774)) ;
#24521=CARTESIAN_POINT('Ctrl Pts',(-19.3305991665012,42.3239459976708,121.906474651851)) ;
#24522=CARTESIAN_POINT('Ctrl Pts',(-19.623580125889,42.5171252015501,122.216652416966)) ;
#24523=CARTESIAN_POINT('Ctrl Pts',(-19.6771578660426,42.3371361211872,121.917859655171)) ;
#24524=CARTESIAN_POINT('Ctrl Pts',(-19.9644761073968,42.5338917626996,122.32049383106)) ;
#24525=CARTESIAN_POINT('Ctrl Pts',(-20.1032957575407,42.3539026823368,122.047670197675)) ;
#24526=CARTESIAN_POINT('Ctrl Pts',(-20.3009572251947,42.5536762514077,122.573177848514)) ;
#24527=CARTESIAN_POINT('Ctrl Pts',(-20.5238873611168,42.3736871710448,122.363526341007)) ;
#24528=CARTESIAN_POINT('Ctrl Pts',(-20.5338536920251,42.5736216990041,122.927472083475)) ;
#24529=CARTESIAN_POINT('Ctrl Pts',(-20.8150059840566,42.3936326186413,122.806396279347)) ;
#24530=CARTESIAN_POINT('Ctrl Pts',(-20.6313376491033,42.5935333611601,123.339481760479)) ;
#24531=CARTESIAN_POINT('Ctrl Pts',(-20.9368565339894,42.4135442807972,123.32140844695)) ;
#24532=CARTESIAN_POINT('Ctrl Pts',(-20.5833429972544,42.6134255531789,123.75977761235)) ;
#24533=CARTESIAN_POINT('Ctrl Pts',(-20.8768601174002,42.4334364728161,123.846776921239)) ;
#24534=CARTESIAN_POINT('Ctrl Pts',(-20.3928775516324,42.6334666837336,124.140904242147)) ;
#24535=CARTESIAN_POINT('Ctrl Pts',(-20.6387749464663,42.4534776033707,124.323184054214)) ;
#24536=CARTESIAN_POINT('Ctrl Pts',(-20.0872595412336,42.6532850183492,124.431171962633)) ;
#24537=CARTESIAN_POINT('Ctrl Pts',(-20.2567515623942,42.4732959379863,124.686015098705)) ;
#24538=CARTESIAN_POINT('Ctrl Pts',(-19.6984277741902,42.6732575835688,124.601563615224)) ;
#24539=CARTESIAN_POINT('Ctrl Pts',(-19.7707111217134,42.4932685032059,124.899002007876)) ;
#24540=CARTESIAN_POINT('Ctrl Pts',(-19.2762631710593,42.6931467997404,124.629052850656)) ;
#24541=CARTESIAN_POINT('Ctrl Pts',(-19.2430064355605,42.5131577193775,124.933361056965)) ;
#24542=CARTESIAN_POINT('Ctrl Pts',(-18.8676531896362,42.7131703740631,124.5098269493)) ;
#24543=CARTESIAN_POINT('Ctrl Pts',(-18.7322443545962,42.5331812937002,124.784326245752)) ;
#24544=CARTESIAN_POINT('Ctrl Pts',(-18.5278123839697,42.7329675371513,124.26130431907)) ;
#24545=CARTESIAN_POINT('Ctrl Pts',(-18.3074466869106,42.5529784567885,124.473672881631)) ;
#24546=CARTESIAN_POINT('Ctrl Pts',(-18.2904261749242,42.7529330309751,123.909466884417)) ;
#24547=CARTESIAN_POINT('Ctrl Pts',(-18.0107152101051,42.5729439506122,124.03387590139)) ;
#24548=CARTESIAN_POINT('Ctrl Pts',(-18.187872486649,42.7728867387165,123.49766130319)) ;
#24549=CARTESIAN_POINT('Ctrl Pts',(-17.8825244705871,42.5928976583536,123.51911914368)) ;
#24550=CARTESIAN_POINT('Ctrl Pts',(-18.2318581554824,42.7927941154431,123.076763552661)) ;
#24551=CARTESIAN_POINT('Ctrl Pts',(-17.9375074674537,42.6128050350802,122.992998485349)) ;
#24552=CARTESIAN_POINT('Ctrl Pts',(-18.4153780545509,42.8126463269917,122.696553693905)) ;
#24553=CARTESIAN_POINT('Ctrl Pts',(-18.1669062692067,42.6326572466288,122.517738273591)) ;
#24554=CARTESIAN_POINT('Ctrl Pts',(-18.7212077898556,42.8327187139374,122.398884993394)) ;
#24555=CARTESIAN_POINT('Ctrl Pts',(-18.5491943143349,42.6527296335745,122.145651577482)) ;
#24556=CARTESIAN_POINT('Ctrl Pts',(-19.1059608983857,42.8525565835777,122.225998547386)) ;
#24557=CARTESIAN_POINT('Ctrl Pts',(-19.0301333322148,42.6725675032148,121.929544757103)) ;
#24558=CARTESIAN_POINT('Ctrl Pts',(-19.526741490911,42.8724072381308,122.192939772244)) ;
#24559=CARTESIAN_POINT('Ctrl Pts',(-19.5561067931665,42.6924181577679,121.88822002276)) ;
#24560=CARTESIAN_POINT('Ctrl Pts',(-19.9374721598721,42.8924591724712,122.307188454904)) ;
#24561=CARTESIAN_POINT('Ctrl Pts',(-20.0695211678143,42.7124700921084,122.031029897398)) ;
#24562=CARTESIAN_POINT('Ctrl Pts',(-20.2808472333612,42.9122923600373,122.552162407161)) ;
#24563=CARTESIAN_POINT('Ctrl Pts',(-20.4987389792293,42.7323032796744,122.33724488066)) ;
#24564=CARTESIAN_POINT('Ctrl Pts',(-20.5217209474624,42.932221572268,122.90060218186)) ;
#24565=CARTESIAN_POINT('Ctrl Pts',(-20.7998323714999,42.7522324919051,122.772792578482)) ;
#24566=CARTESIAN_POINT('Ctrl Pts',(-20.6295592118292,42.9521065374824,123.309594803802)) ;
#24567=CARTESIAN_POINT('Ctrl Pts',(-20.9346324231233,42.7721174571195,123.284031475315)) ;
#24568=CARTESIAN_POINT('Ctrl Pts',(-20.5903609500711,42.972180278627,123.734525663825)) ;
#24569=CARTESIAN_POINT('Ctrl Pts',(-20.8856369561692,42.7921911982641,123.815196128951)) ;
#24570=CARTESIAN_POINT('Ctrl Pts',(-20.4110322867297,42.9919734604074,124.115338189697)) ;
#24571=CARTESIAN_POINT('Ctrl Pts',(-20.6614795251124,42.8119843800445,124.291210805294)) ;
#24572=CARTESIAN_POINT('Ctrl Pts',(-20.1109437575518,43.0119361684101,124.415478901693)) ;
#24573=CARTESIAN_POINT('Ctrl Pts',(-20.2863715695943,42.8319470880472,124.666388958395)) ;
#24574=CARTESIAN_POINT('Ctrl Pts',(-19.7255846738428,43.0319191201525,124.594466908089)) ;
#24575=CARTESIAN_POINT('Ctrl Pts',(-19.8046741907438,42.8519300397896,124.890126754003)) ;
#24576=CARTESIAN_POINT('Ctrl Pts',(-19.3059710828873,43.0517297399247,124.631722413805)) ;
#24577=CARTESIAN_POINT('Ctrl Pts',(-19.2801592562473,42.8717406595618,124.936699673532)) ;
#24578=CARTESIAN_POINT('Ctrl Pts',(-18.8952733972345,43.0717134559576,124.523123476909)) ;
#24579=CARTESIAN_POINT('Ctrl Pts',(-18.7667862152892,42.8917243755947,124.800954951219)) ;
#24580=CARTESIAN_POINT('Ctrl Pts',(-18.547948160276,43.0915949198549,124.281962291053)) ;
#24581=CARTESIAN_POINT('Ctrl Pts',(-18.3326279856665,42.911605839492,124.499507379797)) ;
#24582=CARTESIAN_POINT('Ctrl Pts',(-18.3027271825646,43.1115502496993,123.935800002761)) ;
#24583=CARTESIAN_POINT('Ctrl Pts',(-18.0260984755986,42.9315611693364,124.066807185146)) ;
#24584=CARTESIAN_POINT('Ctrl Pts',(-18.1904651269619,43.1314257105047,123.528307608364)) ;
#24585=CARTESIAN_POINT('Ctrl Pts',(-17.8857662260403,42.9514366301419,123.557444062347)) ;
#24586=CARTESIAN_POINT('Ctrl Pts',(-18.2239197601607,43.1514100305563,123.104753802092)) ;
#24587=CARTESIAN_POINT('Ctrl Pts',(-17.9275815086194,42.9714209501934,123.027999899649)) ;
#24588=CARTESIAN_POINT('Ctrl Pts',(-18.3996847638181,43.1713380633459,122.719094804955)) ;
#24589=CARTESIAN_POINT('Ctrl Pts',(-18.1472767537667,42.991348982983,122.545930346273)) ;
#24590=CARTESIAN_POINT('Ctrl Pts',(-18.646890943322,43.1879468252857,122.467036487721)) ;
#24591=CARTESIAN_POINT('Ctrl Pts',(-18.4563016259536,43.0079577449228,122.230836526374)) ;
#24592=CARTESIAN_POINT('Ctrl Pts',(-18.8854093868125,43.2011344639758,122.325626761766)) ;
#24593=CARTESIAN_POINT('Ctrl Pts',(-18.7544287787532,43.0211453836129,122.054087877132)) ;
#24594=CARTESIAN_POINT('Ctrl Pts',(-19.0816631258239,43.2111208983359,122.25109404408)) ;
#24595=CARTESIAN_POINT('Ctrl Pts',(-18.9997521034799,43.031131817973,121.960916807132)) ;
#24596=CARTESIAN_POINT('Ctrl Pts',(-19.2884287473412,43.2211302722953,122.211885729769)) ;
#24597=CARTESIAN_POINT('Ctrl Pts',(-19.2581944108813,43.0411411919324,121.911902702877)) ;
#24598=CARTESIAN_POINT('Ctrl Pts',(-19.5677559979308,43.2344203058605,122.208091123803)) ;
#24599=CARTESIAN_POINT('Ctrl Pts',(-19.6074202778413,43.0544312254977,121.907165841963)) ;
#24600=CARTESIAN_POINT('Ctrl Pts',(-19.9099408495608,43.251014293523,122.294450351363)) ;
#24601=CARTESIAN_POINT('Ctrl Pts',(-20.0350687767284,43.0710252131601,122.015093622791)) ;
#24602=CARTESIAN_POINT('Ctrl Pts',(-20.2026638187543,43.2676465487985,122.492780810066)) ;
#24603=CARTESIAN_POINT('Ctrl Pts',(-20.4010277793674,43.0876574684357,122.26302842487)) ;
#24604=CARTESIAN_POINT('Ctrl Pts',(-20.3849853860425,43.2808889324664,122.703218028358)) ;
#24605=CARTESIAN_POINT('Ctrl Pts',(-20.6289019817072,43.1008998521035,122.526052209373)) ;
#24606=CARTESIAN_POINT('Ctrl Pts',(-20.4925880976511,43.2908031406938,122.881725152075)) ;
#24607=CARTESIAN_POINT('Ctrl Pts',(-20.7634137015571,43.1108140603309,122.749188831555)) ;
#24608=CARTESIAN_POINT('Ctrl Pts',(-20.5684111030146,43.3008597799655,123.079068387712)) ;
#24609=CARTESIAN_POINT('Ctrl Pts',(-20.8581936477321,43.1208706996026,122.995865179697)) ;
#24610=CARTESIAN_POINT('Ctrl Pts',(-20.6082199665284,43.3107055863856,123.282209920598)) ;
#24611=CARTESIAN_POINT('Ctrl Pts',(-20.9079570487934,43.1307165060227,123.249794573028)) ;
#24612=CARTESIAN_POINT('Ctrl Pts',(-20.6125910585015,43.3207505860188,123.493341268355)) ;
#24613=CARTESIAN_POINT('Ctrl Pts',(-20.9134264774939,43.1407615056559,123.513697714177)) ;
#24614=CARTESIAN_POINT('Ctrl Pts',(-20.569416287465,43.3340316083915,123.769136883137)) ;
#24615=CARTESIAN_POINT('Ctrl Pts',(-20.8594473356749,43.1540425280286,123.858497845333)) ;
#24616=CARTESIAN_POINT('Ctrl Pts',(-20.4566616002104,43.3472290549162,124.026134355986)) ;
#24617=CARTESIAN_POINT('Ctrl Pts',(-20.718508196259,43.1672399745533,124.17971260659)) ;
#24618=CARTESIAN_POINT('Ctrl Pts',(-20.2801208783856,43.3606433527231,124.246084172849)) ;
#24619=CARTESIAN_POINT('Ctrl Pts',(-20.4978485962577,43.1806542723603,124.454637161235)) ;
#24620=CARTESIAN_POINT('Ctrl Pts',(-20.1246767207839,43.3704824181259,124.382563644853)) ;
#24621=CARTESIAN_POINT('Ctrl Pts',(-20.3035425807458,43.190493337763,124.625241624044)) ;
#24622=CARTESIAN_POINT('Ctrl Pts',(-19.9456198245211,43.3804656244036,124.492010358693)) ;
#24623=CARTESIAN_POINT('Ctrl Pts',(-20.0797235876443,43.2004765440407,124.762051652017)) ;
#24624=CARTESIAN_POINT('Ctrl Pts',(-19.7508481450483,43.3904168593164,124.568404517536)) ;
#24625=CARTESIAN_POINT('Ctrl Pts',(-19.8362597616934,43.2104277789535,124.8575472145)) ;
#24626=CARTESIAN_POINT('Ctrl Pts',(-19.5447971219931,43.400417859018,124.610275376094)) ;
#24627=CARTESIAN_POINT('Ctrl Pts',(-19.5786965198764,43.2204287786551,124.909888505183)) ;
#24628=CARTESIAN_POINT('Ctrl Pts',(-19.3339717832248,43.4104492048053,124.615418235309)) ;
#24629=CARTESIAN_POINT('Ctrl Pts',(-19.3151648430061,43.2304601244425,124.916319914135)) ;
#24630=CARTESIAN_POINT('Ctrl Pts',(-19.1290970717957,43.4203029695104,124.584716305653)) ;
#24631=CARTESIAN_POINT('Ctrl Pts',(-19.0590709276985,43.2403138891475,124.877945266862)) ;
#24632=CARTESIAN_POINT('Ctrl Pts',(-18.9302029392523,43.4302736231787,124.518609768227)) ;
#24633=CARTESIAN_POINT('Ctrl Pts',(-18.8104522663154,43.2502845428158,124.79531472401)) ;
#24634=CARTESIAN_POINT('Ctrl Pts',(-18.7452726680142,43.4402708668359,124.418674434814)) ;
#24635=CARTESIAN_POINT('Ctrl Pts',(-18.5792880259183,43.260281786473,124.670397983482)) ;
#24636=CARTESIAN_POINT('Ctrl Pts',(-18.5801137359114,43.4503043227801,124.28749236113)) ;
#24637=CARTESIAN_POINT('Ctrl Pts',(-18.3728375783555,43.2703152424172,124.506422572522)) ;
#24638=CARTESIAN_POINT('Ctrl Pts',(-18.4424457993828,43.4601598270805,124.132620980022)) ;
#24639=CARTESIAN_POINT('Ctrl Pts',(-18.2007504134058,43.2801707467176,124.31283503278)) ;
#24640=CARTESIAN_POINT('Ctrl Pts',(-18.3319639426538,43.4701592633666,123.953818397867)) ;
#24641=CARTESIAN_POINT('Ctrl Pts',(-18.0626456729148,43.2901701830037,124.089333194053)) ;
#24642=CARTESIAN_POINT('Ctrl Pts',(-18.2547737206712,43.4800537228825,123.760615819088)) ;
#24643=CARTESIAN_POINT('Ctrl Pts',(-17.9661552350075,43.3000646425196,123.847830753989)) ;
#24644=CARTESIAN_POINT('Ctrl Pts',(-18.2116553133487,43.4901168423341,123.553535266331)) ;
#24645=CARTESIAN_POINT('Ctrl Pts',(-17.9122545173091,43.3101277619712,123.588980661551)) ;
#24646=CARTESIAN_POINT('Ctrl Pts',(-18.2050619663453,43.4999564767461,123.346745963906)) ;
#24647=CARTESIAN_POINT('Ctrl Pts',(-17.9040100749574,43.3199673963832,123.330493713353)) ;
#24648=CARTESIAN_POINT('Ctrl Pts',(-18.23486765756,43.5100196842319,123.137325469672)) ;
#24649=CARTESIAN_POINT('Ctrl Pts',(-17.9412644855324,43.330030603869,123.068717754911)) ;
#24650=CARTESIAN_POINT('Ctrl Pts',(-18.2996597954055,43.5199137916111,122.939643533093)) ;
#24651=CARTESIAN_POINT('Ctrl Pts',(-18.0222521551209,43.3399247112482,122.821614169064)) ;
#24652=CARTESIAN_POINT('Ctrl Pts',(-18.3977518129424,43.5298561238035,122.755103321263)) ;
#24653=CARTESIAN_POINT('Ctrl Pts',(-18.1448649357578,43.3498670434406,122.590937416187)) ;
#24654=CARTESIAN_POINT('Ctrl Pts',(-18.5271067731501,43.5398567501185,122.589320233305)) ;
#24655=CARTESIAN_POINT('Ctrl Pts',(-18.3065565946206,43.3598676697556,122.383706851709)) ;
#24656=CARTESIAN_POINT('Ctrl Pts',(-18.6841488510847,43.5498984844004,122.448264779539)) ;
#24657=CARTESIAN_POINT('Ctrl Pts',(-18.5028573530525,43.3699094040375,122.207385535582)) ;
#24658=CARTESIAN_POINT('Ctrl Pts',(-18.8592239504986,43.5597239103495,122.33861707734)) ;
#24659=CARTESIAN_POINT('Ctrl Pts',(-18.7217003533941,43.3797348299866,122.070323331608)) ;
#24660=CARTESIAN_POINT('Ctrl Pts',(-19.0550398152044,43.5697807368771,122.258927424476)) ;
#24661=CARTESIAN_POINT('Ctrl Pts',(-18.9664691272905,43.3897916565143,121.970708884775)) ;
#24662=CARTESIAN_POINT('Ctrl Pts',(-19.2591461901148,43.5797081699987,122.215302018421)) ;
#24663=CARTESIAN_POINT('Ctrl Pts',(-19.2216018609428,43.3997190896358,121.916174470016)) ;
#24664=CARTESIAN_POINT('Ctrl Pts',(-19.4681756382475,43.5896581624049,122.207163663793)) ;
#24665=CARTESIAN_POINT('Ctrl Pts',(-19.4828888562582,43.4096690820421,121.905998966867)) ;
#24666=CARTESIAN_POINT('Ctrl Pts',(-19.6775616742312,43.5997133634789,122.236109466576)) ;
#24667=CARTESIAN_POINT('Ctrl Pts',(-19.7446216548047,43.4197242831161,121.942178613796)) ;
#24668=CARTESIAN_POINT('Ctrl Pts',(-19.874223881596,43.6095356375312,122.299123887037)) ;
#24669=CARTESIAN_POINT('Ctrl Pts',(-19.9904509322207,43.4295465571684,122.02094445218)) ;
#24670=CARTESIAN_POINT('Ctrl Pts',(-20.0614519230175,43.6195915314905,122.397267586826)) ;
#24671=CARTESIAN_POINT('Ctrl Pts',(-20.2244870380784,43.4396024511276,122.143621831466)) ;
#24672=CARTESIAN_POINT('Ctrl Pts',(-20.2266685259505,43.6295322533356,122.525258130833)) ;
#24673=CARTESIAN_POINT('Ctrl Pts',(-20.4310096168158,43.4495431729727,122.303608199071)) ;
#24674=CARTESIAN_POINT('Ctrl Pts',(-20.3671176125788,43.6394365974222,122.678983059671)) ;
#24675=CARTESIAN_POINT('Ctrl Pts',(-20.6065731184016,43.4594475170593,122.495763120482)) ;
#24676=CARTESIAN_POINT('Ctrl Pts',(-20.4802208408433,43.6494832647217,122.857339300403)) ;
#24677=CARTESIAN_POINT('Ctrl Pts',(-20.7479541652507,43.4694941843588,122.718707024721)) ;
#24678=CARTESIAN_POINT('Ctrl Pts',(-20.5596229425746,43.6593788231716,123.049662217343)) ;
#24679=CARTESIAN_POINT('Ctrl Pts',(-20.8472092355886,43.4793897428087,122.95911028977)) ;
#24680=CARTESIAN_POINT('Ctrl Pts',(-20.6051653987093,43.6694409018763,123.256207404328)) ;
#24681=CARTESIAN_POINT('Ctrl Pts',(-20.904139618028,43.4894518215134,123.217291078424)) ;
#24682=CARTESIAN_POINT('Ctrl Pts',(-20.614077706757,43.6792836003421,123.462962817774)) ;
#24683=CARTESIAN_POINT('Ctrl Pts',(-20.9152824166523,43.4992945199792,123.475736104278)) ;
#24684=CARTESIAN_POINT('Ctrl Pts',(-20.587046897207,43.6892743742365,123.671227339976)) ;
#24685=CARTESIAN_POINT('Ctrl Pts',(-20.8814961280243,43.5092852938737,123.736067222342)) ;
#24686=CARTESIAN_POINT('Ctrl Pts',(-20.5246153399661,43.6992022434715,123.870395640026)) ;
#24687=CARTESIAN_POINT('Ctrl Pts',(-20.8034587033046,43.5192131631086,123.985028739388)) ;
#24688=CARTESIAN_POINT('Ctrl Pts',(-20.4282901507528,43.7091909724413,124.0570066794)) ;
#24689=CARTESIAN_POINT('Ctrl Pts',(-20.6830540646815,43.5292018920784,124.218293703487)) ;
#24690=CARTESIAN_POINT('Ctrl Pts',(-20.300083088921,43.7192303744251,124.224651641945)) ;
#24691=CARTESIAN_POINT('Ctrl Pts',(-20.5227971110946,43.5392412940622,124.427851205494)) ;
#24692=CARTESIAN_POINT('Ctrl Pts',(-20.1480587442798,43.7290705421618,124.364969335422)) ;
#24693=CARTESIAN_POINT('Ctrl Pts',(-20.3327674227349,43.549081461799,124.603250592089)) ;
#24694=CARTESIAN_POINT('Ctrl Pts',(-19.9704841404498,43.7391187525363,124.479372090359)) ;
#24695=CARTESIAN_POINT('Ctrl Pts',(-20.1108004287422,43.5591296721735,124.746255706704)) ;
#24696=CARTESIAN_POINT('Ctrl Pts',(-19.7775615457972,43.7490659228241,124.560080673461)) ;
#24697=CARTESIAN_POINT('Ctrl Pts',(-19.8696476488821,43.5690768424612,124.84714360705)) ;
#24698=CARTESIAN_POINT('Ctrl Pts',(-19.5744358323149,43.7589767710792,124.606507407475)) ;
#24699=CARTESIAN_POINT('Ctrl Pts',(-19.6157403076391,43.5789876907163,124.905179129313)) ;
#24700=CARTESIAN_POINT('Ctrl Pts',(-19.3632888752703,43.7690330987569,124.616913341482)) ;
#24701=CARTESIAN_POINT('Ctrl Pts',(-19.3518069355752,43.5890440183941,124.91818859538)) ;
#24702=CARTESIAN_POINT('Ctrl Pts',(-19.1577934192907,43.7788835115255,124.591215482131)) ;
#24703=CARTESIAN_POINT('Ctrl Pts',(-19.0949363387433,43.5988944311626,124.886068138014)) ;
#24704=CARTESIAN_POINT('Ctrl Pts',(-18.9561968908211,43.7889103973592,124.529628376844)) ;
#24705=CARTESIAN_POINT('Ctrl Pts',(-18.8429401699179,43.6089213169963,124.809086046414)) ;
#24706=CARTESIAN_POINT('Ctrl Pts',(-18.7685615510423,43.79893901299,124.433463237905)) ;
#24707=CARTESIAN_POINT('Ctrl Pts',(-18.608395133658,43.6189499326271,124.688881455388)) ;
#24708=CARTESIAN_POINT('Ctrl Pts',(-18.6033288718835,43.8087842363675,124.30883132978)) ;
#24709=CARTESIAN_POINT('Ctrl Pts',(-18.4018522456686,43.6287951560046,124.53309241998)) ;
#24710=CARTESIAN_POINT('Ctrl Pts',(-18.4597378892454,43.8187749184691,124.155537858628)) ;
#24711=CARTESIAN_POINT('Ctrl Pts',(-18.2223621198309,43.6387858381062,124.34147662207)) ;
#24712=CARTESIAN_POINT('Ctrl Pts',(-18.3448008532577,43.8288128071015,123.978559187435)) ;
#24713=CARTESIAN_POINT('Ctrl Pts',(-18.0786893213183,43.6488237267386,124.120254417819)) ;
#24714=CARTESIAN_POINT('Ctrl Pts',(-18.2635921715876,43.8386571422047,123.78819018194)) ;
#24715=CARTESIAN_POINT('Ctrl Pts',(-17.977176387725,43.6586680618418,123.882292776737)) ;
#24716=CARTESIAN_POINT('Ctrl Pts',(-18.2156072803135,43.8486421044022,123.583862375105)) ;
#24717=CARTESIAN_POINT('Ctrl Pts',(-17.917193628408,43.6686530240393,123.626883148383)) ;
#24718=CARTESIAN_POINT('Ctrl Pts',(-18.2037829776996,43.8585810459356,123.375218987753)) ;
#24719=CARTESIAN_POINT('Ctrl Pts',(-17.9024116244684,43.6785919655727,123.366078461576)) ;
#24720=CARTESIAN_POINT('Ctrl Pts',(-18.2286806326614,43.868622930907,123.165600430253)) ;
#24721=CARTESIAN_POINT('Ctrl Pts',(-17.9335320666697,43.6886338505441,123.104055220491)) ;
#24722=CARTESIAN_POINT('Ctrl Pts',(-18.2885381500914,43.8785094788153,122.96653880576)) ;
#24723=CARTESIAN_POINT('Ctrl Pts',(-18.008352723709,43.6985203984524,122.855226846736)) ;
#24724=CARTESIAN_POINT('Ctrl Pts',(-18.3827677761836,43.8885034043153,122.778780845212)) ;
#24725=CARTESIAN_POINT('Ctrl Pts',(-18.1261385188554,43.7085143239524,122.620528575572)) ;
#24726=CARTESIAN_POINT('Ctrl Pts',(-18.507397260208,43.8984394954417,122.611106118602)) ;
#24727=CARTESIAN_POINT('Ctrl Pts',(-18.2819245676956,43.7184504150789,122.410933846051)) ;
#24728=CARTESIAN_POINT('Ctrl Pts',(-18.6606561201383,43.9084687644217,122.466343302757)) ;
#24729=CARTESIAN_POINT('Ctrl Pts',(-18.4734970875813,43.7284796840588,122.229979319978)) ;
#24730=CARTESIAN_POINT('Ctrl Pts',(-18.8340470507955,43.918351146981,122.351835718989)) ;
#24731=CARTESIAN_POINT('Ctrl Pts',(-18.6902358432055,43.7383620666181,122.086843147979)) ;
#24732=CARTESIAN_POINT('Ctrl Pts',(-19.0278824329128,43.9284036640689,122.267711760247)) ;
#24733=CARTESIAN_POINT('Ctrl Pts',(-18.9325293093004,43.748414583706,121.981687073779)) ;
#24734=CARTESIAN_POINT('Ctrl Pts',(-19.2301849856646,43.9382977848928,122.219177390576)) ;
#24735=CARTESIAN_POINT('Ctrl Pts',(-19.1854080916355,43.7583087045299,121.921017634688)) ;
#24736=CARTESIAN_POINT('Ctrl Pts',(-19.441298301709,43.9483597643132,122.206244667768)) ;
#24737=CARTESIAN_POINT('Ctrl Pts',(-19.4492993318414,43.7683706839503,121.904850471576)) ;
#24738=CARTESIAN_POINT('Ctrl Pts',(-19.6469435683342,43.9582042975421,122.229626514128)) ;
#24739=CARTESIAN_POINT('Ctrl Pts',(-19.7063573702631,43.7782152171792,121.934076663056)) ;
#24740=CARTESIAN_POINT('Ctrl Pts',(-19.8479372841435,43.9681643764484,122.288322728641)) ;
#24741=CARTESIAN_POINT('Ctrl Pts',(-19.9576002327423,43.7881752960855,122.007446102476)) ;
#24742=CARTESIAN_POINT('Ctrl Pts',(-20.0369708079469,43.978202653021,122.38212312448)) ;
#24743=CARTESIAN_POINT('Ctrl Pts',(-20.1938925036668,43.7982135726581,122.124695495129)) ;
#24744=CARTESIAN_POINT('Ctrl Pts',(-20.2043238205213,43.9880760395588,122.504967849574)) ;
#24745=CARTESIAN_POINT('Ctrl Pts',(-20.403085266942,43.8080869591959,122.278251260109)) ;
#24746=CARTESIAN_POINT('Ctrl Pts',(-20.3506106823668,43.9981489823259,122.658028324524)) ;
#24747=CARTESIAN_POINT('Ctrl Pts',(-20.5859442921562,43.818159901963,122.469575837394)) ;
#24748=CARTESIAN_POINT('Ctrl Pts',(-20.465419038605,44.0079703964542,122.82969122843)) ;
#24749=CARTESIAN_POINT('Ctrl Pts',(-20.7294563688574,43.8279813160913,122.684155238316)) ;
#24750=CARTESIAN_POINT('Ctrl Pts',(-20.5510249351871,44.0180450265265,123.023378752783)) ;
#24751=CARTESIAN_POINT('Ctrl Pts',(-20.8364643232835,43.8380559461636,122.926263897482)) ;
#24752=CARTESIAN_POINT('Ctrl Pts',(-20.6005844279953,44.0279116638434,123.224825343159)) ;
#24753=CARTESIAN_POINT('Ctrl Pts',(-20.8984148212984,43.8479225834805,123.178073112069)) ;
#24754=CARTESIAN_POINT('Ctrl Pts',(-20.6151706977744,44.0379352092152,123.435036739168)) ;
#24755=CARTESIAN_POINT('Ctrl Pts',(-20.9166483132866,43.8579461288523,123.440837266538)) ;
#24756=CARTESIAN_POINT('Ctrl Pts',(-20.5925229977775,44.0479609607324,123.644602262895)) ;
#24757=CARTESIAN_POINT('Ctrl Pts',(-20.8883395523817,43.8679718803695,123.702794177763)) ;
#24758=CARTESIAN_POINT('Ctrl Pts',(-20.5351790535078,44.0578145477417,123.843648615532)) ;
#24759=CARTESIAN_POINT('Ctrl Pts',(-20.8166599479504,43.8778254673789,123.951603594725)) ;
#24760=CARTESIAN_POINT('Ctrl Pts',(-20.4434995838773,44.0677915079697,124.032303037785)) ;
#24761=CARTESIAN_POINT('Ctrl Pts',(-20.702060923653,43.8878024276068,124.187422142841)) ;
#24762=CARTESIAN_POINT('Ctrl Pts',(-20.3196315257472,44.0778126509981,124.202704231129)) ;
#24763=CARTESIAN_POINT('Ctrl Pts',(-20.5472263847729,43.8978235706353,124.400424003541)) ;
#24764=CARTESIAN_POINT('Ctrl Pts',(-20.1704166426939,44.0876952570181,124.347313905858)) ;
#24765=CARTESIAN_POINT('Ctrl Pts',(-20.3607073265626,43.9077061766552,124.581187205771)) ;
#24766=CARTESIAN_POINT('Ctrl Pts',(-19.9951290913081,44.0977637276508,124.465904961827)) ;
#24767=CARTESIAN_POINT('Ctrl Pts',(-20.141598516524,43.9177746472879,124.729426223139)) ;
#24768=CARTESIAN_POINT('Ctrl Pts',(-19.8065219734023,44.1075938108345,124.550461991308)) ;
#24769=CARTESIAN_POINT('Ctrl Pts',(-19.9058383854937,43.9276047304716,124.835123522503)) ;
#24770=CARTESIAN_POINT('Ctrl Pts',(-19.6014110884651,44.1176603705148,124.602451546472)) ;
#24771=CARTESIAN_POINT('Ctrl Pts',(-19.6494502413749,43.937671290152,124.900110672069)) ;
#24772=CARTESIAN_POINT('Ctrl Pts',(-19.3940171097119,44.1275506203441,124.617639758843)) ;
#24773=CARTESIAN_POINT('Ctrl Pts',(-19.3902067493444,43.9475615399812,124.919096378298)) ;
#24774=CARTESIAN_POINT('Ctrl Pts',(-19.1849952546928,44.1375427860929,124.596831802444)) ;
#24775=CARTESIAN_POINT('Ctrl Pts',(-19.1289291993489,43.95755370573,124.893086593962)) ;
#24776=CARTESIAN_POINT('Ctrl Pts',(-18.9834025895948,44.147505629689,124.540019916616)) ;
#24777=CARTESIAN_POINT('Ctrl Pts',(-18.8769378575391,43.9675165493261,124.822071866951)) ;
#24778=CARTESIAN_POINT('Ctrl Pts',(-18.7955966982782,44.1574097985167,124.450071701931)) ;
#24779=CARTESIAN_POINT('Ctrl Pts',(-18.6421796236828,43.9774207181539,124.709636238937)) ;
#24780=CARTESIAN_POINT('Ctrl Pts',(-18.6237306354897,44.1674706734111,124.326834768521)) ;
#24781=CARTESIAN_POINT('Ctrl Pts',(-18.4273472596352,43.9874815930482,124.555590382771)) ;
#24782=CARTESIAN_POINT('Ctrl Pts',(-18.4788866563946,44.1773095767404,124.179124043168)) ;
#24783=CARTESIAN_POINT('Ctrl Pts',(-18.2462912417937,43.9973204963776,124.370950929424)) ;
#24784=CARTESIAN_POINT('Ctrl Pts',(-18.3590318669185,44.1873779531143,124.004699120229)) ;
#24785=CARTESIAN_POINT('Ctrl Pts',(-18.096473040413,44.0073888727515,124.152920066805)) ;
#24786=CARTESIAN_POINT('Ctrl Pts',(-18.2729573990922,44.197258569747,123.815617005926)) ;
#24787=CARTESIAN_POINT('Ctrl Pts',(-17.9888795242822,44.0172694893841,123.916566377132)) ;
#24788=CARTESIAN_POINT('Ctrl Pts',(-18.2200454094595,44.207249729976,123.612376766819)) ;
#24789=CARTESIAN_POINT('Ctrl Pts',(-17.9227396809683,44.0272606496131,123.662515814642)) ;
#24790=CARTESIAN_POINT('Ctrl Pts',(-18.2032518304312,44.2172028034081,123.403775478978)) ;
#24791=CARTESIAN_POINT('Ctrl Pts',(-17.9017478866056,44.0372137230452,123.40176367561)) ;
#24792=CARTESIAN_POINT('Ctrl Pts',(-18.2231612060629,44.2272386390207,123.19374932302)) ;
#24793=CARTESIAN_POINT('Ctrl Pts',(-17.9266347799871,44.0472495586578,123.139231148737)) ;
#24794=CARTESIAN_POINT('Ctrl Pts',(-18.2782926365655,44.2371287657509,122.993256824972)) ;
#24795=CARTESIAN_POINT('Ctrl Pts',(-17.9955495886584,44.057139685388,122.888614558069)) ;
#24796=CARTESIAN_POINT('Ctrl Pts',(-18.368002893643,44.2471209475202,122.803320931818)) ;
#24797=CARTESIAN_POINT('Ctrl Pts',(-18.1076878440328,44.0671318671573,122.651194666647)) ;
#24798=CARTESIAN_POINT('Ctrl Pts',(-18.4888319440295,44.2570668874946,122.632672480447)) ;
#24799=CARTESIAN_POINT('Ctrl Pts',(-18.2587247866769,44.0770778071318,122.437883820146)) ;
#24800=CARTESIAN_POINT('Ctrl Pts',(-18.6371833756394,44.2670140712541,122.485268515715)) ;
#24801=CARTESIAN_POINT('Ctrl Pts',(-18.4441648499972,44.0870249908912,122.253628827194)) ;
#24802=CARTESIAN_POINT('Ctrl Pts',(-18.810735082372,44.2770620095444,122.364857154366)) ;
#24803=CARTESIAN_POINT('Ctrl Pts',(-18.6611045195494,44.0970729291816,122.103115117568)) ;
#24804=CARTESIAN_POINT('Ctrl Pts',(-18.9986676053786,44.286909644358,122.278010090229)) ;
#24805=CARTESIAN_POINT('Ctrl Pts',(-18.8960216519544,44.1069205639951,121.9945561486)) ;
#24806=CARTESIAN_POINT('Ctrl Pts',(-19.2009643648431,44.296871358056,122.223868979964)) ;
#24807=CARTESIAN_POINT('Ctrl Pts',(-19.1488932353645,44.1168822776931,121.926880369107)) ;
#24808=CARTESIAN_POINT('Ctrl Pts',(-19.4110368321455,44.3068999938771,122.205817721847)) ;
#24809=CARTESIAN_POINT('Ctrl Pts',(-19.4114837782062,44.1269109135143,121.904316948058)) ;
#24810=CARTESIAN_POINT('Ctrl Pts',(-19.6185576126464,44.3168103086289,122.224226084689)) ;
#24811=CARTESIAN_POINT('Ctrl Pts',(-19.6708855677709,44.136821228266,121.927328148373)) ;
#24812=CARTESIAN_POINT('Ctrl Pts',(-19.8203871123028,44.3267451792916,122.277995841482)) ;
#24813=CARTESIAN_POINT('Ctrl Pts',(-19.923172854028,44.1467560989287,121.994541369525)) ;
#24814=CARTESIAN_POINT('Ctrl Pts',(-20.0117417687553,44.3367863616933,122.367111250582)) ;
#24815=CARTESIAN_POINT('Ctrl Pts',(-20.1623656622643,44.1567972813305,122.105936279633)) ;
#24816=CARTESIAN_POINT('Ctrl Pts',(-20.182178194294,44.3466733331581,122.48611803753)) ;
#24817=CARTESIAN_POINT('Ctrl Pts',(-20.3754115587803,44.1666842527952,122.254696080828)) ;
#24818=CARTESIAN_POINT('Ctrl Pts',(-20.3311931711049,44.3566727654207,122.634359060664)) ;
#24819=CARTESIAN_POINT('Ctrl Pts',(-20.5616797006254,44.1766836850578,122.439998156239)) ;
#24820=CARTESIAN_POINT('Ctrl Pts',(-20.4513895888392,44.3665928306773,122.804819406772)) ;
#24821=CARTESIAN_POINT('Ctrl Pts',(-20.7119248209942,44.1866037503144,122.653074790023)) ;
#24822=CARTESIAN_POINT('Ctrl Pts',(-20.5412304164301,44.3766296832615,122.995731464311)) ;
#24823=CARTESIAN_POINT('Ctrl Pts',(-20.8242248480084,44.1966406028986,122.89171516179)) ;
#24824=CARTESIAN_POINT('Ctrl Pts',(-20.5958716500195,44.3865423426014,123.196839523156)) ;
#24825=CARTESIAN_POINT('Ctrl Pts',(-20.8925256088344,44.2065532622386,123.143101297578)) ;
#24826=CARTESIAN_POINT('Ctrl Pts',(-20.6153694128764,44.3965335545164,123.405991946571)) ;
#24827=CARTESIAN_POINT('Ctrl Pts',(-20.9168966357386,44.2165444741535,123.404542148438)) ;
#24828=CARTESIAN_POINT('Ctrl Pts',(-20.5976979683511,44.4065751959195,123.616341273831)) ;
#24829=CARTESIAN_POINT('Ctrl Pts',(-20.8948063197256,44.2265861155566,123.667478543077)) ;
#24830=CARTESIAN_POINT('Ctrl Pts',(-20.54540602134,44.4164039901265,123.816275966712)) ;
#24831=CARTESIAN_POINT('Ctrl Pts',(-20.8294398407361,44.2364149097636,123.917397995982)) ;
#24832=CARTESIAN_POINT('Ctrl Pts',(-20.4571322193429,44.4264804012478,124.008799381337)) ;
#24833=CARTESIAN_POINT('Ctrl Pts',(-20.7190966284838,44.2464913208849,124.158051348321)) ;
#24834=CARTESIAN_POINT('Ctrl Pts',(-20.3394898621036,44.4363325342902,124.179323371872)) ;
#24835=CARTESIAN_POINT('Ctrl Pts',(-20.5720419186679,44.2563434539274,124.371206621261)) ;
#24836=CARTESIAN_POINT('Ctrl Pts',(-20.1909447204641,44.4464057686315,124.330210550994)) ;
#24837=CARTESIAN_POINT('Ctrl Pts',(-20.3863598082827,44.2664166882687,124.559814357932)) ;
#24838=CARTESIAN_POINT('Ctrl Pts',(-20.0223534222565,44.4562472699582,124.450168274092)) ;
#24839=CARTESIAN_POINT('Ctrl Pts',(-20.1756188492781,44.2762581895953,124.709761183194)) ;
#24840=CARTESIAN_POINT('Ctrl Pts',(-19.8335848822427,44.466208221553,124.540812132209)) ;
#24841=CARTESIAN_POINT('Ctrl Pts',(-19.9396571120249,44.2862191411901,124.823064731638)) ;
#24842=CARTESIAN_POINT('Ctrl Pts',(-19.6302748014164,44.4762460392736,124.597332076024)) ;
#24843=CARTESIAN_POINT('Ctrl Pts',(-19.6855192485354,44.2962569589108,124.893713217866)) ;
#24844=CARTESIAN_POINT('Ctrl Pts',(-19.4236658402343,44.4861203885307,124.617747552604)) ;
#24845=CARTESIAN_POINT('Ctrl Pts',(-19.4272568805915,44.3061313081678,124.919231077549)) ;
#24846=CARTESIAN_POINT('Ctrl Pts',(-19.2126136916866,44.4961899392729,124.601657803566)) ;
#24847=CARTESIAN_POINT('Ctrl Pts',(-19.1634421663118,44.31620085891,124.899117334135)) ;
#24848=CARTESIAN_POINT('Ctrl Pts',(-19.0122816584332,44.5060239587815,124.550498030164)) ;
#24849=CARTESIAN_POINT('Ctrl Pts',(-18.9130262792897,44.3260348784186,124.835165719918)) ;
#24850=CARTESIAN_POINT('Ctrl Pts',(-18.8198408604291,44.516058113361,124.464118183293)) ;
#24851=CARTESIAN_POINT('Ctrl Pts',(-18.6724761256092,44.3360690329981,124.727189304434)) ;
#24852=CARTESIAN_POINT('Ctrl Pts',(-18.6459125382961,44.5260740391835,124.345407050209)) ;
#24853=CARTESIAN_POINT('Ctrl Pts',(-18.4550666358706,44.3460849588206,124.578799029693)) ;
#24854=CARTESIAN_POINT('Ctrl Pts',(-18.4969953236926,44.5359562943777,124.200536328678)) ;
#24855=CARTESIAN_POINT('Ctrl Pts',(-18.2689206934433,44.3559672140149,124.397708730824)) ;
#24856=CARTESIAN_POINT('Ctrl Pts',(-18.3739888329453,44.5459451008887,124.030365635577)) ;
#24857=CARTESIAN_POINT('Ctrl Pts',(-18.1151639542311,44.3659560205258,124.184994122571)) ;
#24858=CARTESIAN_POINT('Ctrl Pts',(-18.2825994603111,44.5558936681514,123.842202089097)) ;
#24859=CARTESIAN_POINT('Ctrl Pts',(-18.0009287364672,44.3759045877885,123.949788452977)) ;
#24860=CARTESIAN_POINT('Ctrl Pts',(-18.2248894304791,44.5659484734534,123.638872201841)) ;
#24861=CARTESIAN_POINT('Ctrl Pts',(-17.9287930124207,44.3859593930905,123.695625807384)) ;
#24862=CARTESIAN_POINT('Ctrl Pts',(-18.2035656681982,44.575767256717,123.433544830677)) ;
#24863=CARTESIAN_POINT('Ctrl Pts',(-17.9021400804517,44.3957781763541,123.438965134921)) ;
#24864=CARTESIAN_POINT('Ctrl Pts',(-18.2179757066852,44.5858030290775,123.223058832807)) ;
#24865=CARTESIAN_POINT('Ctrl Pts',(-17.9201546965115,44.4058139487147,123.175857889878)) ;
#24866=CARTESIAN_POINT('Ctrl Pts',(-18.2692459499617,44.5958277281062,123.018631696878)) ;
#24867=CARTESIAN_POINT('Ctrl Pts',(-17.9842443392215,44.4158386477433,122.920324456169)) ;
#24868=CARTESIAN_POINT('Ctrl Pts',(-18.3533314311282,44.6056797313652,122.829344467355)) ;
#24869=CARTESIAN_POINT('Ctrl Pts',(-18.0893534627256,44.4256906510024,122.683715321304)) ;
#24870=CARTESIAN_POINT('Ctrl Pts',(-18.4703557315628,44.6156706657625,122.65495463514)) ;
#24871=CARTESIAN_POINT('Ctrl Pts',(-18.2356357013134,44.4356815853996,122.46572907487)) ;
#24872=CARTESIAN_POINT('Ctrl Pts',(-18.6147549951052,44.6255885881936,122.504508089155)) ;
#24873=CARTESIAN_POINT('Ctrl Pts',(-18.41613673709,44.4455995078307,122.277671975149)) ;
#24874=CARTESIAN_POINT('Ctrl Pts',(-18.7848954850902,44.6356169438759,122.380036959605)) ;
#24875=CARTESIAN_POINT('Ctrl Pts',(-18.6288136047377,44.455627863513,122.122084840499)) ;
#24876=CARTESIAN_POINT('Ctrl Pts',(-18.9713236852492,44.6455012283865,122.288233366533)) ;
#24877=CARTESIAN_POINT('Ctrl Pts',(-18.8618504936233,44.4655121480236,122.007331995514)) ;
#24878=CARTESIAN_POINT('Ctrl Pts',(-19.1729084480282,44.6554939122944,122.229103541019)) ;
#24879=CARTESIAN_POINT('Ctrl Pts',(-19.1138322342733,44.4755048319315,121.933421901147)) ;
#24880=CARTESIAN_POINT('Ctrl Pts',(-19.382493485015,44.6655226493021,122.206156839358)) ;
#24881=CARTESIAN_POINT('Ctrl Pts',(-19.3758137501504,44.4855335689392,121.904740742867)) ;
#24882=CARTESIAN_POINT('Ctrl Pts',(-19.5898954585969,44.675408045931,122.219478540037)) ;
#24883=CARTESIAN_POINT('Ctrl Pts',(-19.6350667634332,44.4954189655681,121.921395206069)) ;
#24884=CARTESIAN_POINT('Ctrl Pts',(-19.793970597842,44.6853959313449,122.268821405339)) ;
#24885=CARTESIAN_POINT('Ctrl Pts',(-19.8901602887943,44.505406850982,121.983076127047)) ;
#24886=CARTESIAN_POINT('Ctrl Pts',(-19.9857471745296,44.6953466340055,122.352468749605)) ;
#24887=CARTESIAN_POINT('Ctrl Pts',(-20.1298803582596,44.5153575536426,122.087637628189)) ;
#24888=CARTESIAN_POINT('Ctrl Pts',(-20.1615504334524,44.7053869521029,122.469253001426)) ;
#24889=CARTESIAN_POINT('Ctrl Pts',(-20.3496330623717,44.52539787174,122.233619868658)) ;
#24890=CARTESIAN_POINT('Ctrl Pts',(-20.3120561281735,44.7152615174361,122.612267502799)) ;
#24891=CARTESIAN_POINT('Ctrl Pts',(-20.5377640234238,44.5352724370732,122.412390214829)) ;
#24892=CARTESIAN_POINT('Ctrl Pts',(-20.4371874370457,44.7252611774972,122.78115208881)) ;
#24893=CARTESIAN_POINT('Ctrl Pts',(-20.6941762400211,44.5452720971343,122.62349750357)) ;
#24894=CARTESIAN_POINT('Ctrl Pts',(-20.5304535414409,44.7351701726649,122.967466993672)) ;
#24895=CARTESIAN_POINT('Ctrl Pts',(-20.8107568463258,44.555181092302,122.856392682696)) ;
#24896=CARTESIAN_POINT('Ctrl Pts',(-20.5907433449701,44.7452249138281,123.170033529265)) ;
#24897=CARTESIAN_POINT('Ctrl Pts',(-20.8861166779856,44.5652358334653,123.109601455861)) ;
#24898=CARTESIAN_POINT('Ctrl Pts',(-20.6147190095158,44.7550835257419,123.375937676543)) ;
#24899=CARTESIAN_POINT('Ctrl Pts',(-20.9160838152059,44.5750944453791,123.36698258296)) ;
#24900=CARTESIAN_POINT('Ctrl Pts',(-20.60245263379,44.7651516480213,123.587214744072)) ;
#24901=CARTESIAN_POINT('Ctrl Pts',(-20.9007482951995,44.5851625676584,123.631078613714)) ;
#24902=CARTESIAN_POINT('Ctrl Pts',(-20.5546908139825,44.7750071187245,123.788845425538)) ;
#24903=CARTESIAN_POINT('Ctrl Pts',(-20.8410433869187,44.5950180383616,123.883116987979)) ;
#24904=CARTESIAN_POINT('Ctrl Pts',(-20.4720727117349,44.7850019782178,123.9820375159)) ;
#24905=CARTESIAN_POINT('Ctrl Pts',(-20.737768269546,44.605012897855,124.124606144448)) ;
#24906=CARTESIAN_POINT('Ctrl Pts',(-20.3563607572283,44.7950332315598,124.158351468293)) ;
#24907=CARTESIAN_POINT('Ctrl Pts',(-20.5931261612872,44.6150441511969,124.344997164701)) ;
#24908=CARTESIAN_POINT('Ctrl Pts',(-20.2144020973158,44.8048999304329,124.309603441992)) ;
#24909=CARTESIAN_POINT('Ctrl Pts',(-20.4156755541826,44.62491085007,124.534060702266)) ;
#24910=CARTESIAN_POINT('Ctrl Pts',(-20.0465467747764,44.8148867461841,124.435681086058)) ;
#24911=CARTESIAN_POINT('Ctrl Pts',(-20.2058546846897,44.6348976658212,124.691655677439)) ;
#24912=CARTESIAN_POINT('Ctrl Pts',(-19.8600899400834,44.8248339513795,124.530430266587)) ;
#24913=CARTESIAN_POINT('Ctrl Pts',(-19.9727822075021,44.6448448710167,124.810089850081)) ;
#24914=CARTESIAN_POINT('Ctrl Pts',(-19.6581014765466,44.8348769395058,124.591850093754)) ;
#24915=CARTESIAN_POINT('Ctrl Pts',(-19.7202958616412,44.6548878591429,124.886862052342)) ;
#24916=CARTESIAN_POINT('Ctrl Pts',(-19.4521749099809,44.8447442941273,124.616945312236)) ;
#24917=CARTESIAN_POINT('Ctrl Pts',(-19.4628869098935,44.6647552137644,124.91822843966)) ;
#24918=CARTESIAN_POINT('Ctrl Pts',(-19.242936933169,44.8547101874254,124.606358445387)) ;
#24919=CARTESIAN_POINT('Ctrl Pts',(-19.201339436511,44.6747211070625,124.904992081208)) ;
#24920=CARTESIAN_POINT('Ctrl Pts',(-19.0375566117157,44.8647339648015,124.559112347747)) ;
#24921=CARTESIAN_POINT('Ctrl Pts',(-18.9446146117008,44.6847448844386,124.845931776589)) ;
#24922=CARTESIAN_POINT('Ctrl Pts',(-18.8454040569223,44.8746595127332,124.477781348015)) ;
#24923=CARTESIAN_POINT('Ctrl Pts',(-18.7044247703961,44.6946704323703,124.744265398415)) ;
#24924=CARTESIAN_POINT('Ctrl Pts',(-18.6697413624025,44.8845999891542,124.364553604711)) ;
#24925=CARTESIAN_POINT('Ctrl Pts',(-18.4848477732278,44.7046109087913,124.602728279973)) ;
#24926=CARTESIAN_POINT('Ctrl Pts',(-18.5149584063942,44.8946461988171,124.220874734381)) ;
#24927=CARTESIAN_POINT('Ctrl Pts',(-18.2913709521149,44.7146571184542,124.423127645142)) ;
#24928=CARTESIAN_POINT('Ctrl Pts',(-18.3896255165691,44.9045074554789,124.055712470621)) ;
#24929=CARTESIAN_POINT('Ctrl Pts',(-18.1347068986328,44.724518375116,124.216672914137)) ;
#24930=CARTESIAN_POINT('Ctrl Pts',(-18.2933036607311,44.9145010837542,123.869030082729)) ;
#24931=CARTESIAN_POINT('Ctrl Pts',(-18.0143070451238,44.7345120033913,123.983318570089)) ;
#24932=CARTESIAN_POINT('Ctrl Pts',(-18.2311629194592,44.9244264810644,123.669801758037)) ;
#24933=CARTESIAN_POINT('Ctrl Pts',(-17.936633762989,44.7444374007015,123.734282199344)) ;
#24934=CARTESIAN_POINT('Ctrl Pts',(-18.2042856489682,44.9344543889746,123.46073131352)) ;
#24935=CARTESIAN_POINT('Ctrl Pts',(-17.9030399617659,44.7544653086117,123.472943722699)) ;
#24936=CARTESIAN_POINT('Ctrl Pts',(-18.2137679240456,44.9443407046438,123.253075539075)) ;
#24937=CARTESIAN_POINT('Ctrl Pts',(-17.9148956263581,44.7643516242809,123.213374011942)) ;
#24938=CARTESIAN_POINT('Ctrl Pts',(-18.2597049737886,44.9543722995476,123.047278072271)) ;
#24939=CARTESIAN_POINT('Ctrl Pts',(-17.9723197114155,44.7743832191847,122.95612772885)) ;
#24940=CARTESIAN_POINT('Ctrl Pts',(-18.339321156955,44.9642545424993,122.855346311805)) ;
#24941=CARTESIAN_POINT('Ctrl Pts',(-18.0718425713874,44.7842654621364,122.716214046185)) ;
#24942=CARTESIAN_POINT('Ctrl Pts',(-18.4529511231331,44.9743140135291,122.677012970206)) ;
#24943=CARTESIAN_POINT('Ctrl Pts',(-18.2138824565932,44.7943249331663,122.493298818431)) ;
#24944=CARTESIAN_POINT('Ctrl Pts',(-18.5931221037197,44.9841804581923,122.524103073492)) ;
#24945=CARTESIAN_POINT('Ctrl Pts',(-18.3890982744024,44.8041913778294,122.302163339125)) ;
#24946=CARTESIAN_POINT('Ctrl Pts',(-18.7589604520614,44.994146582641,122.3960648915)) ;
#24947=CARTESIAN_POINT('Ctrl Pts',(-18.5963979569655,44.8141575022781,122.142117824611)) ;
#24948=CARTESIAN_POINT('Ctrl Pts',(-18.9458650964473,45.0041768260321,122.298439068355)) ;
#24949=CARTESIAN_POINT('Ctrl Pts',(-18.8300300927451,44.8241877456692,122.020087986119)) ;
#24950=CARTESIAN_POINT('Ctrl Pts',(-19.1440629077566,45.0140698609852,122.235330723378)) ;
#24951=CARTESIAN_POINT('Ctrl Pts',(-19.0777784031114,44.8340807806223,121.941205272921)) ;
#24952=CARTESIAN_POINT('Ctrl Pts',(-19.3534531145185,45.024120775222,122.207100463021)) ;
#24953=CARTESIAN_POINT('Ctrl Pts',(-19.3395157430304,44.8441316948591,121.905920090679)) ;
#24954=CARTESIAN_POINT('Ctrl Pts',(-19.5612049836232,45.0340106014466,122.215495999718)) ;
#24955=CARTESIAN_POINT('Ctrl Pts',(-19.5992088007417,44.8540215210837,121.916417743617)) ;
#24956=CARTESIAN_POINT('Ctrl Pts',(-19.8352568409963,45.0473454164935,122.274745540189)) ;
#24957=CARTESIAN_POINT('Ctrl Pts',(-19.9417558495349,44.8673563361306,121.990481112151)) ;
#24958=CARTESIAN_POINT('Ctrl Pts',(-20.0861970248156,45.060622507665,122.404050574181)) ;
#24959=CARTESIAN_POINT('Ctrl Pts',(-20.2554040575952,44.8806334273021,122.152088557895)) ;
#24960=CARTESIAN_POINT('Ctrl Pts',(-20.2927670242742,45.0738707962633,122.590851363296)) ;
#24961=CARTESIAN_POINT('Ctrl Pts',(-20.5136611155883,44.8938817159004,122.385626670228)) ;
#24962=CARTESIAN_POINT('Ctrl Pts',(-20.4224319151714,45.0839256377574,122.757766119149)) ;
#24963=CARTESIAN_POINT('Ctrl Pts',(-20.6757307463464,44.9039365573945,122.59426491759)) ;
#24964=CARTESIAN_POINT('Ctrl Pts',(-20.5192820589709,45.0937566270649,122.940386196395)) ;
#24965=CARTESIAN_POINT('Ctrl Pts',(-20.7967932245961,44.913767546702,122.822543238522)) ;
#24966=CARTESIAN_POINT('Ctrl Pts',(-20.584670046844,45.1038331913881,123.141847213542)) ;
#24967=CARTESIAN_POINT('Ctrl Pts',(-20.8785256178797,44.9238441110252,123.074368365477)) ;
#24968=CARTESIAN_POINT('Ctrl Pts',(-20.6134250008506,45.1136825165221,123.34692196347)) ;
#24969=CARTESIAN_POINT('Ctrl Pts',(-20.9144646604309,44.9336934361592,123.330718388823)) ;
#24970=CARTESIAN_POINT('Ctrl Pts',(-20.6042179421268,45.1270305161593,123.627426871071)) ;
#24971=CARTESIAN_POINT('Ctrl Pts',(-20.9029627808752,44.9470414357965,123.681317025944)) ;
#24972=CARTESIAN_POINT('Ctrl Pts',(-20.501477245052,45.1436152756959,123.964696954444)) ;
#24973=CARTESIAN_POINT('Ctrl Pts',(-20.7745082951822,44.963626195333,124.10295325502)) ;
#24974=CARTESIAN_POINT('Ctrl Pts',(-20.2906509977138,45.160183827044,124.247002494003)) ;
#24975=CARTESIAN_POINT('Ctrl Pts',(-20.5110259009966,44.9801947466811,124.455768261803)) ;
#24976=CARTESIAN_POINT('Ctrl Pts',(-20.0699761701848,45.173543651863,124.420705346495)) ;
#24977=CARTESIAN_POINT('Ctrl Pts',(-20.2351348038895,44.9935545715001,124.672943272086)) ;
#24978=CARTESIAN_POINT('Ctrl Pts',(-19.8865323634229,45.1834490606937,124.519294728282)) ;
#24979=CARTESIAN_POINT('Ctrl Pts',(-20.0058393288218,45.0034599803308,124.796167835363)) ;
#24980=CARTESIAN_POINT('Ctrl Pts',(-19.6878012033677,45.1934090872777,124.585169308581)) ;
#24981=CARTESIAN_POINT('Ctrl Pts',(-19.757418400852,45.0134200069148,124.878510971796)) ;
#24982=CARTESIAN_POINT('Ctrl Pts',(-19.4120405401479,45.206666671463,124.625957687893)) ;
#24983=CARTESIAN_POINT('Ctrl Pts',(-19.4127381950797,45.0266775911001,124.929494089017)) ;
#24984=CARTESIAN_POINT('Ctrl Pts',(-19.0603261711488,45.2233178829577,124.585513512105)) ;
#24985=CARTESIAN_POINT('Ctrl Pts',(-18.9730728854828,45.0433288025948,124.878933487773)) ;
#24986=CARTESIAN_POINT('Ctrl Pts',(-18.6814904591991,45.243236097068,124.396215063051)) ;
#24987=CARTESIAN_POINT('Ctrl Pts',(-18.4995381186548,45.0632470167051,124.642306903848)) ;
#24988=CARTESIAN_POINT('Ctrl Pts',(-18.3898754544286,45.2631138602888,124.090194523484)) ;
#24989=CARTESIAN_POINT('Ctrl Pts',(-18.1350210819867,45.0831247799259,124.259778759138)) ;
#24990=CARTESIAN_POINT('Ctrl Pts',(-18.2194472690857,45.283126528076,123.70037612657)) ;
#24991=CARTESIAN_POINT('Ctrl Pts',(-17.9219902774577,45.1031374477131,123.772503946077)) ;
#24992=CARTESIAN_POINT('Ctrl Pts',(-18.1921410054773,45.3029390507426,123.279913832054)) ;
#24993=CARTESIAN_POINT('Ctrl Pts',(-17.8878614143457,45.1229499703797,123.246927329174)) ;
#24994=CARTESIAN_POINT('Ctrl Pts',(-18.3102817888919,45.3229223507425,122.871855648759)) ;
#24995=CARTESIAN_POINT('Ctrl Pts',(-18.0355408684965,45.1429332703796,122.736855760796)) ;
#24996=CARTESIAN_POINT('Ctrl Pts',(-18.5597996288413,45.3428166278438,122.530199318799)) ;
#24997=CARTESIAN_POINT('Ctrl Pts',(-18.3474404946756,45.1628275474809,122.309788228837)) ;
#24998=CARTESIAN_POINT('Ctrl Pts',(-18.9111760068349,45.3627493896015,122.293234594438)) ;
#24999=CARTESIAN_POINT('Ctrl Pts',(-18.786662149823,45.1827603092387,122.0135853007)) ;
#25000=CARTESIAN_POINT('Ctrl Pts',(-19.3230940340298,45.3827153953663,122.190513539357)) ;
#25001=CARTESIAN_POINT('Ctrl Pts',(-19.3015601046736,45.2027263150034,121.885187082688)) ;
#25002=CARTESIAN_POINT('Ctrl Pts',(-19.7435470242779,45.4025939275311,122.234031106994)) ;
#25003=CARTESIAN_POINT('Ctrl Pts',(-19.8271247057948,45.2226048471683,121.939586650986)) ;
#25004=CARTESIAN_POINT('Ctrl Pts',(-20.1251936183417,45.4225335941915,122.418585683632)) ;
#25005=CARTESIAN_POINT('Ctrl Pts',(-20.3041812489775,45.2425445138286,122.170281678288)) ;
#25006=CARTESIAN_POINT('Ctrl Pts',(-20.4204383603451,45.4424284688368,122.721592637798)) ;
#25007=CARTESIAN_POINT('Ctrl Pts',(-20.673234757221,45.262439388474,122.549040856896)) ;
#25008=CARTESIAN_POINT('Ctrl Pts',(-20.5949902534563,45.4623356081302,123.107099332329)) ;
#25009=CARTESIAN_POINT('Ctrl Pts',(-20.8914226002841,45.2823465277673,123.03092366853)) ;
#25010=CARTESIAN_POINT('Ctrl Pts',(-20.6282585414511,45.4822461562087,123.529280154733)) ;
#25011=CARTESIAN_POINT('Ctrl Pts',(-20.933006994823,45.3022570758458,123.558648564266)) ;
#25012=CARTESIAN_POINT('Ctrl Pts',(-20.5136884964889,45.5023147415659,123.940226483196)) ;
#25013=CARTESIAN_POINT('Ctrl Pts',(-20.7897928711044,45.322325661203,124.072332126759)) ;
#25014=CARTESIAN_POINT('Ctrl Pts',(-20.2695153225536,45.5220965388806,124.282881980283)) ;
#25015=CARTESIAN_POINT('Ctrl Pts',(-20.4845776581537,45.3421074585177,124.500648372566)) ;
#25016=CARTESIAN_POINT('Ctrl Pts',(-19.9197219519249,45.5421040858251,124.52470903084)) ;
#25017=CARTESIAN_POINT('Ctrl Pts',(-20.0473359397164,45.3621150054623,124.802932073758)) ;
#25018=CARTESIAN_POINT('Ctrl Pts',(-19.5119563590964,45.561925824128,124.631740685911)) ;
#25019=CARTESIAN_POINT('Ctrl Pts',(-19.5376317009415,45.3819367437651,124.936721152217)) ;
#25020=CARTESIAN_POINT('Ctrl Pts',(-19.0888978513631,45.5819058440321,124.593677351388)) ;
#25021=CARTESIAN_POINT('Ctrl Pts',(-19.0088087615849,45.4019167636693,124.889143040385)) ;
#25022=CARTESIAN_POINT('Ctrl Pts',(-18.7055922778892,45.6018232952944,124.413561871822)) ;
#25023=CARTESIAN_POINT('Ctrl Pts',(-18.5296775435496,45.4218342149315,124.664000015216)) ;
#25024=CARTESIAN_POINT('Ctrl Pts',(-18.4066895135121,45.6216982164671,124.114786478611)) ;
#25025=CARTESIAN_POINT('Ctrl Pts',(-18.1560490205525,45.4417091361042,124.2905332235)) ;
#25026=CARTESIAN_POINT('Ctrl Pts',(-18.2266120856884,45.6417225850179,123.729001322783)) ;
#25027=CARTESIAN_POINT('Ctrl Pts',(-17.9309504550834,45.461733504655,123.80830220994)) ;
#25028=CARTESIAN_POINT('Ctrl Pts',(-18.1894029579917,45.6615892693914,123.308154855926)) ;
#25029=CARTESIAN_POINT('Ctrl Pts',(-17.8844372685422,45.4816001890285,123.282245957211)) ;
#25030=CARTESIAN_POINT('Ctrl Pts',(-18.2977756961196,45.6815330912376,122.898226280014)) ;
#25031=CARTESIAN_POINT('Ctrl Pts',(-18.0199005695342,45.5015440108747,122.769835234287)) ;
#25032=CARTESIAN_POINT('Ctrl Pts',(-18.5392315029753,45.7014404604891,122.55056181091)) ;
#25033=CARTESIAN_POINT('Ctrl Pts',(-18.3217175474885,45.5214513801262,122.335254029468)) ;
#25034=CARTESIAN_POINT('Ctrl Pts',(-18.8838051537408,45.7213151582358,122.30592410139)) ;
#25035=CARTESIAN_POINT('Ctrl Pts',(-18.7524316861596,45.5413260778729,122.029454998175)) ;
#25036=CARTESIAN_POINT('Ctrl Pts',(-19.2933757524993,45.7412971007575,122.192842071119)) ;
#25037=CARTESIAN_POINT('Ctrl Pts',(-19.2643939100382,45.5613080203947,121.888099189238)) ;
#25038=CARTESIAN_POINT('Ctrl Pts',(-19.7151717006801,45.7611997676684,122.226529361424)) ;
#25039=CARTESIAN_POINT('Ctrl Pts',(-19.7916381676523,45.5812106873055,121.930204794695)) ;
#25040=CARTESIAN_POINT('Ctrl Pts',(-20.0998523433655,45.7810551252071,122.400620470514)) ;
#25041=CARTESIAN_POINT('Ctrl Pts',(-20.2724895989063,45.6010660448442,122.147814462636)) ;
#25042=CARTESIAN_POINT('Ctrl Pts',(-20.4047844549801,45.8011191639231,122.698883119931)) ;
#25043=CARTESIAN_POINT('Ctrl Pts',(-20.6536580199716,45.6211300835602,122.520640262332)) ;
#25044=CARTESIAN_POINT('Ctrl Pts',(-20.5876495556406,45.8209743436481,123.079572690105)) ;
#25045=CARTESIAN_POINT('Ctrl Pts',(-20.8822424651067,45.6409852632853,122.996499598304)) ;
#25046=CARTESIAN_POINT('Ctrl Pts',(-20.6301960454336,45.8409544483126,123.502103273831)) ;
#25047=CARTESIAN_POINT('Ctrl Pts',(-20.9354305273725,45.6609653679497,123.524661889087)) ;
#25048=CARTESIAN_POINT('Ctrl Pts',(-20.5273174567824,45.8607635534824,123.910665052776)) ;
#25049=CARTESIAN_POINT('Ctrl Pts',(-20.8068347567717,45.6807744731195,124.035365380666)) ;
#25050=CARTESIAN_POINT('Ctrl Pts',(-20.2894986913643,45.8807561738231,124.262859185796)) ;
#25051=CARTESIAN_POINT('Ctrl Pts',(-20.5095739145416,45.7007670934602,124.475605981024)) ;
#25052=CARTESIAN_POINT('Ctrl Pts',(-20.0050296007185,45.8972956563272,124.469758288625)) ;
#25053=CARTESIAN_POINT('Ctrl Pts',(-20.1539637829234,45.7173065759643,124.734247767366)) ;
#25054=CARTESIAN_POINT('Ctrl Pts',(-19.7428533033287,45.9106599743914,124.570733072106)) ;
#25055=CARTESIAN_POINT('Ctrl Pts',(-19.826276696828,45.7306708940285,124.860455779892)) ;
#25056=CARTESIAN_POINT('Ctrl Pts',(-19.4702042971827,45.9238775768929,124.624395490945)) ;
#25057=CARTESIAN_POINT('Ctrl Pts',(-19.4853999049105,45.74388849653,124.927543476285)) ;
#25058=CARTESIAN_POINT('Ctrl Pts',(-19.1168393550171,45.9405351711707,124.600762737389)) ;
#25059=CARTESIAN_POINT('Ctrl Pts',(-19.0437646821752,45.7605460908078,124.897999792884)) ;
#25060=CARTESIAN_POINT('Ctrl Pts',(-18.7301975068277,45.9604008732124,124.430507653493)) ;
#25061=CARTESIAN_POINT('Ctrl Pts',(-18.5604443553513,45.7804117928495,124.685196121248)) ;
#25062=CARTESIAN_POINT('Ctrl Pts',(-18.4743625889817,45.9770305999024,124.186562575314)) ;
#25063=CARTESIAN_POINT('Ctrl Pts',(-18.240630590451,45.7970415195396,124.380241225691)) ;
#25064=CARTESIAN_POINT('Ctrl Pts',(-18.3289929824002,45.9903197150403,123.947896155844)) ;
#25065=CARTESIAN_POINT('Ctrl Pts',(-18.0589348454478,45.8103306346774,124.081934291346)) ;
#25066=CARTESIAN_POINT('Ctrl Pts',(-18.2525232753599,46.0002840620174,123.752891385966)) ;
#25067=CARTESIAN_POINT('Ctrl Pts',(-17.9633418369383,45.8202949816545,123.838171148512)) ;
#25068=CARTESIAN_POINT('Ctrl Pts',(-18.2110838319254,46.0102124300189,123.548318215047)) ;
#25069=CARTESIAN_POINT('Ctrl Pts',(-17.9115389081574,45.830223349656,123.582470100099)) ;
#25070=CARTESIAN_POINT('Ctrl Pts',(-18.2034517091304,46.0234958631076,123.269181346863)) ;
#25071=CARTESIAN_POINT('Ctrl Pts',(-17.9020047414413,45.8435067827447,123.233481404821)) ;
#25072=CARTESIAN_POINT('Ctrl Pts',(-18.2859373810871,46.0401479408479,122.924806830037)) ;
#25073=CARTESIAN_POINT('Ctrl Pts',(-18.0050894429486,45.8601588604851,122.80309786385)) ;
#25074=CARTESIAN_POINT('Ctrl Pts',(-18.479608382182,46.0566993101488,122.631034753051)) ;
#25075=CARTESIAN_POINT('Ctrl Pts',(-18.2472042450846,45.8767102297859,122.435821289861)) ;
#25076=CARTESIAN_POINT('Ctrl Pts',(-18.6881326465127,46.0699867382977,122.445080340454)) ;
#25077=CARTESIAN_POINT('Ctrl Pts',(-18.5078328375495,45.8899976579349,122.203411111269)) ;
#25078=CARTESIAN_POINT('Ctrl Pts',(-18.8678435030827,46.0800312779978,122.334231053414)) ;
#25079=CARTESIAN_POINT('Ctrl Pts',(-18.7324749007102,45.900042197635,122.064839904029)) ;
#25080=CARTESIAN_POINT('Ctrl Pts',(-19.060066473483,46.0898741198217,122.257583029304)) ;
#25081=CARTESIAN_POINT('Ctrl Pts',(-18.9727512214166,45.9098850394588,121.969029204104)) ;
#25082=CARTESIAN_POINT('Ctrl Pts',(-19.2654570004802,46.0998584040686,122.214404145467)) ;
#25083=CARTESIAN_POINT('Ctrl Pts',(-19.2294892302823,45.9198693237057,121.91505230479)) ;
#25084=CARTESIAN_POINT('Ctrl Pts',(-19.474529222648,46.1098080494678,122.207609739844)) ;
#25085=CARTESIAN_POINT('Ctrl Pts',(-19.4908293876516,45.9298189691049,121.906556619496)) ;
#25086=CARTESIAN_POINT('Ctrl Pts',(-19.6826867659275,46.1198078111562,122.237114286998)) ;
#25087=CARTESIAN_POINT('Ctrl Pts',(-19.7510268140243,45.9398187307933,121.943434488528)) ;
#25088=CARTESIAN_POINT('Ctrl Pts',(-19.8830689863678,46.1298391571151,122.30284594859)) ;
#25089=CARTESIAN_POINT('Ctrl Pts',(-20.0015055166855,45.9498500767522,122.02559641534)) ;
#25090=CARTESIAN_POINT('Ctrl Pts',(-20.0658738233849,46.1396941115922,122.400357303943)) ;
#25091=CARTESIAN_POINT('Ctrl Pts',(-20.230012990869,45.9597050312293,122.147483174595)) ;
#25092=CARTESIAN_POINT('Ctrl Pts',(-20.2311978485199,46.1496666495927,122.529251790254)) ;
#25093=CARTESIAN_POINT('Ctrl Pts',(-20.4366698390954,45.9696775692299,122.308599139529)) ;
#25094=CARTESIAN_POINT('Ctrl Pts',(-20.371971249445,46.1596616433277,122.68529494029)) ;
#25095=CARTESIAN_POINT('Ctrl Pts',(-20.6126387229705,45.9796725629648,122.503651259972)) ;
#25096=CARTESIAN_POINT('Ctrl Pts',(-20.4837019140822,46.1696957021218,122.864201377535)) ;
#25097=CARTESIAN_POINT('Ctrl Pts',(-20.7523044634586,45.9897066217589,122.727282847818)) ;
#25098=CARTESIAN_POINT('Ctrl Pts',(-20.5615851923955,46.1795510449448,123.056218498459)) ;
#25099=CARTESIAN_POINT('Ctrl Pts',(-20.8496612407523,45.9995619645819,122.967303410869)) ;
#25100=CARTESIAN_POINT('Ctrl Pts',(-20.6058435319962,46.1895505242904,123.261688930267)) ;
#25101=CARTESIAN_POINT('Ctrl Pts',(-20.9049869101856,46.0095614439275,123.224140951696)) ;
#25102=CARTESIAN_POINT('Ctrl Pts',(-20.613909648338,46.1994449730457,123.469584195291)) ;
#25103=CARTESIAN_POINT('Ctrl Pts',(-20.9150723248034,46.0194558926828,123.484010185289)) ;
#25104=CARTESIAN_POINT('Ctrl Pts',(-20.5852243576683,46.2095080924802,123.679152099285)) ;
#25105=CARTESIAN_POINT('Ctrl Pts',(-20.8792184641045,46.0295190121173,123.745970407933)) ;
#25106=CARTESIAN_POINT('Ctrl Pts',(-20.5222181496825,46.2193477377214,123.87621952154)) ;
#25107=CARTESIAN_POINT('Ctrl Pts',(-20.8004631964166,46.0393586573585,123.992305910844)) ;
#25108=CARTESIAN_POINT('Ctrl Pts',(-20.4240329883721,46.2294109019075,124.06358200029)) ;
#25109=CARTESIAN_POINT('Ctrl Pts',(-20.6777341782391,46.0494218215446,124.226510235197)) ;
#25110=CARTESIAN_POINT('Ctrl Pts',(-20.2968048807207,46.2393051716563,124.228173665467)) ;
#25111=CARTESIAN_POINT('Ctrl Pts',(-20.5187010120317,46.0593160912934,124.432251752361)) ;
#25112=CARTESIAN_POINT('Ctrl Pts',(-20.1426117795388,46.2492468976701,124.369228950053)) ;
#25113=CARTESIAN_POINT('Ctrl Pts',(-20.3259612493778,46.0692578173072,124.608573010416)) ;
#25114=CARTESIAN_POINT('Ctrl Pts',(-19.9651819070724,46.2592497863295,124.482167683482)) ;
#25115=CARTESIAN_POINT('Ctrl Pts',(-20.1041752620859,46.0792607059666,124.749748717296)) ;
#25116=CARTESIAN_POINT('Ctrl Pts',(-19.7700203195679,46.2692896351235,124.562503209581)) ;
#25117=CARTESIAN_POINT('Ctrl Pts',(-19.8602243413917,46.0893005547606,124.850170623594)) ;
#25118=CARTESIAN_POINT('Ctrl Pts',(-19.5683677612482,46.2791138505843,124.607227073809)) ;
#25119=CARTESIAN_POINT('Ctrl Pts',(-19.6081586045614,46.0991247702215,124.906078173757)) ;
#25120=CARTESIAN_POINT('Ctrl Pts',(-19.3571724462641,46.2891706940779,124.61676513193)) ;
#25121=CARTESIAN_POINT('Ctrl Pts',(-19.3441646598656,46.109181613715,124.918003343611)) ;
#25122=CARTESIAN_POINT('Ctrl Pts',(-19.1502130268079,46.2990993034739,124.589560068272)) ;
#25123=CARTESIAN_POINT('Ctrl Pts',(-19.0854647176779,46.119110223111,124.883999596897)) ;
#25124=CARTESIAN_POINT('Ctrl Pts',(-18.9504791865377,46.3090511875118,124.527247497498)) ;
#25125=CARTESIAN_POINT('Ctrl Pts',(-18.8357963857665,46.1290621071489,124.806111234111)) ;
#25126=CARTESIAN_POINT('Ctrl Pts',(-18.7629062407361,46.3191041403194,124.429897592764)) ;
#25127=CARTESIAN_POINT('Ctrl Pts',(-18.6013290923237,46.1391150599565,124.684426223968)) ;
#25128=CARTESIAN_POINT('Ctrl Pts',(-18.5986696134654,46.3289270167856,124.304685324782)) ;
#25129=CARTESIAN_POINT('Ctrl Pts',(-18.3960311454174,46.1489379364227,124.527912441961)) ;
#25130=CARTESIAN_POINT('Ctrl Pts',(-18.4550971880899,46.3389827493557,124.149533035185)) ;
#25131=CARTESIAN_POINT('Ctrl Pts',(-18.2165638688177,46.1589936689928,124.333973843009)) ;
#25132=CARTESIAN_POINT('Ctrl Pts',(-18.34225300586,46.3489235143433,123.973622295558)) ;
#25133=CARTESIAN_POINT('Ctrl Pts',(-18.0755063145666,46.1689344339805,124.114086515428)) ;
#25134=CARTESIAN_POINT('Ctrl Pts',(-18.2613628141207,46.358827847249,123.78175251306)) ;
#25135=CARTESIAN_POINT('Ctrl Pts',(-17.9743911402895,46.1788387668861,123.874249737998)) ;
#25136=CARTESIAN_POINT('Ctrl Pts',(-18.2144855602519,46.3688745161297,123.575825795225)) ;
#25137=CARTESIAN_POINT('Ctrl Pts',(-17.9157922099519,46.1888854357668,123.616841983496)) ;
#25138=CARTESIAN_POINT('Ctrl Pts',(-18.2040405773316,46.3787700794355,123.368018792122)) ;
#25139=CARTESIAN_POINT('Ctrl Pts',(-17.9027335515217,46.1987809990726,123.357082770937)) ;
#25140=CARTESIAN_POINT('Ctrl Pts',(-18.2302623333417,46.3888321371358,123.158144461646)) ;
#25141=CARTESIAN_POINT('Ctrl Pts',(-17.9355083348723,46.2088430567729,123.094739738878)) ;
#25142=CARTESIAN_POINT('Ctrl Pts',(-18.2910726090505,46.3986749147633,122.960331021879)) ;
#25143=CARTESIAN_POINT('Ctrl Pts',(-18.0115191596736,46.2186858344004,122.847471415839)) ;
#25144=CARTESIAN_POINT('Ctrl Pts',(-18.3862537401612,46.4086653930151,122.773135377991)) ;
#25145=CARTESIAN_POINT('Ctrl Pts',(-18.1304936326855,46.2286763126523,122.613475678947)) ;
#25146=CARTESIAN_POINT('Ctrl Pts',(-18.5117634998611,46.4185943656587,122.606329099744)) ;
#25147=CARTESIAN_POINT('Ctrl Pts',(-18.2873793152529,46.2386052852958,122.404966075839)) ;
#25148=CARTESIAN_POINT('Ctrl Pts',(-18.6650531697513,46.4285855025382,122.462726172881)) ;
#25149=CARTESIAN_POINT('Ctrl Pts',(-18.4789900283898,46.2485964221754,122.225460708948)) ;
#25150=CARTESIAN_POINT('Ctrl Pts',(-18.8416348523983,46.4386076200272,122.347776529069)) ;
#25151=CARTESIAN_POINT('Ctrl Pts',(-18.6997158872876,46.2586185396643,122.081771774985)) ;
#25152=CARTESIAN_POINT('Ctrl Pts',(-19.033062714252,46.4485081304294,122.266054468037)) ;
#25153=CARTESIAN_POINT('Ctrl Pts',(-18.9390004515799,46.2685190500665,121.97961691748)) ;
#25154=CARTESIAN_POINT('Ctrl Pts',(-19.2375063165582,46.4584971231755,122.218070769825)) ;
#25155=CARTESIAN_POINT('Ctrl Pts',(-19.1945546489749,46.2785080428126,121.919635191703)) ;
#25156=CARTESIAN_POINT('Ctrl Pts',(-19.4466780664343,46.4684623672261,122.206487877889)) ;
#25157=CARTESIAN_POINT('Ctrl Pts',(-19.4560195398829,46.2884732868632,121.905154403475)) ;
#25158=CARTESIAN_POINT('Ctrl Pts',(-19.6534929917255,46.4783666317393,122.230762789135)) ;
#25159=CARTESIAN_POINT('Ctrl Pts',(-19.7145391120576,46.2983775513764,121.93549611882)) ;
#25160=CARTESIAN_POINT('Ctrl Pts',(-19.8559786184111,46.4884247234375,122.291626495888)) ;
#25161=CARTESIAN_POINT('Ctrl Pts',(-19.9676465193919,46.3084356430746,122.011573715253)) ;
#25162=CARTESIAN_POINT('Ctrl Pts',(-20.0410082512781,46.4982746638659,122.384630025382)) ;
#25163=CARTESIAN_POINT('Ctrl Pts',(-20.1989353902242,46.318285583503,122.127826794879)) ;
#25164=CARTESIAN_POINT('Ctrl Pts',(-20.2103627890321,46.5083016750394,122.510144547104)) ;
#25165=CARTESIAN_POINT('Ctrl Pts',(-20.4106296400589,46.3283125946766,122.284718430549)) ;
#25166=CARTESIAN_POINT('Ctrl Pts',(-20.354983799268,46.5183302616515,122.66357001132)) ;
#25167=CARTESIAN_POINT('Ctrl Pts',(-20.5914073282754,46.3383411812886,122.476498822217)) ;
#25168=CARTESIAN_POINT('Ctrl Pts',(-20.4689669278839,46.5281754757642,122.836320633626)) ;
#25169=CARTESIAN_POINT('Ctrl Pts',(-20.7338884447941,46.3481863954013,122.692436981991)) ;
#25170=CARTESIAN_POINT('Ctrl Pts',(-20.5529614777016,46.5381662239437,123.028836720587)) ;
#25171=CARTESIAN_POINT('Ctrl Pts',(-20.838883297733,46.3581771435809,122.933081577216)) ;
#25172=CARTESIAN_POINT('Ctrl Pts',(-20.6020311758152,46.5482038575292,123.234075060244)) ;
#25173=CARTESIAN_POINT('Ctrl Pts',(-20.9002222159883,46.3682147771664,123.1896289369)) ;
#25174=CARTESIAN_POINT('Ctrl Pts',(-20.6148200501619,46.5580491467421,123.440660845129)) ;
#25175=CARTESIAN_POINT('Ctrl Pts',(-20.9162101455242,46.3780600663792,123.447862222641)) ;
#25176=CARTESIAN_POINT('Ctrl Pts',(-20.5916887931145,46.568030547548,123.649206343481)) ;
#25177=CARTESIAN_POINT('Ctrl Pts',(-20.8872976540046,46.3880414671851,123.708544539136)) ;
#25178=CARTESIAN_POINT('Ctrl Pts',(-20.5328161463453,46.5779827805379,123.849986028359)) ;
#25179=CARTESIAN_POINT('Ctrl Pts',(-20.8137082785738,46.397993700175,123.959520057968)) ;
#25180=CARTESIAN_POINT('Ctrl Pts',(-20.4397820483577,46.5879815919945,124.038501912924)) ;
#25181=CARTESIAN_POINT('Ctrl Pts',(-20.6974169783614,46.4079925116317,124.195165716517)) ;
#25182=CARTESIAN_POINT('Ctrl Pts',(-20.3146171869605,46.5980206959252,124.208420179491)) ;
#25183=CARTESIAN_POINT('Ctrl Pts',(-20.5409623495954,46.4180316155623,124.407564420263)) ;
#25184=CARTESIAN_POINT('Ctrl Pts',(-20.1653985323656,46.6078456383445,124.351256112857)) ;
#25185=CARTESIAN_POINT('Ctrl Pts',(-20.3544390959673,46.4278565579816,124.586111387913)) ;
#25186=CARTESIAN_POINT('Ctrl Pts',(-19.989843192052,46.6179003258204,124.468971674532)) ;
#25187=CARTESIAN_POINT('Ctrl Pts',(-20.134995919871,46.4379112454576,124.733256870576)) ;
#25188=CARTESIAN_POINT('Ctrl Pts',(-19.7985051156906,46.6278431281773,124.553146705472)) ;
#25189=CARTESIAN_POINT('Ctrl Pts',(-19.8958234362632,46.4478540478144,124.838477290274)) ;
#25190=CARTESIAN_POINT('Ctrl Pts',(-19.5964092228832,46.637746924117,124.603245253759)) ;
#25191=CARTESIAN_POINT('Ctrl Pts',(-19.6432030628621,46.4577578437542,124.901101950844)) ;
#25192=CARTESIAN_POINT('Ctrl Pts',(-19.3856978448509,46.6477937034921,124.617570281629)) ;
#25193=CARTESIAN_POINT('Ctrl Pts',(-19.3798141419767,46.4678046231292,124.919009575157)) ;
#25194=CARTESIAN_POINT('Ctrl Pts',(-19.1787922985653,46.6576893617867,124.595604702868)) ;
#25195=CARTESIAN_POINT('Ctrl Pts',(-19.1211811679258,46.4777002814238,124.891553789188)) ;
#25196=CARTESIAN_POINT('Ctrl Pts',(-18.9755356634845,46.6677509290373,124.537120494577)) ;
#25197=CARTESIAN_POINT('Ctrl Pts',(-18.8671103311317,46.4877618486744,124.818449852984)) ;
#25198=CARTESIAN_POINT('Ctrl Pts',(-18.7895780705822,46.6775955734746,124.446252644844)) ;
#25199=CARTESIAN_POINT('Ctrl Pts',(-18.6346615958398,46.4976064931117,124.704865605345)) ;
#25200=CARTESIAN_POINT('Ctrl Pts',(-18.6198270026623,46.6875556197173,124.323663154049)) ;
#25201=CARTESIAN_POINT('Ctrl Pts',(-18.4224718070244,46.5075665393544,124.551629282646)) ;
#25202=CARTESIAN_POINT('Ctrl Pts',(-18.4730960397559,46.6975939157357,124.171998085648)) ;
#25203=CARTESIAN_POINT('Ctrl Pts',(-18.2390573894743,46.5176048353728,124.362048863107)) ;
#25204=CARTESIAN_POINT('Ctrl Pts',(-18.3565170418454,46.707467257154,124.0002223481)) ;
#25205=CARTESIAN_POINT('Ctrl Pts',(-18.0933321835797,46.5274781767911,124.147328823137)) ;
#25206=CARTESIAN_POINT('Ctrl Pts',(-18.2699035021467,46.7175403609533,123.807021171241)) ;
#25207=CARTESIAN_POINT('Ctrl Pts',(-17.9850644966569,46.5375512805904,123.905828159884)) ;
#25208=CARTESIAN_POINT('Ctrl Pts',(-18.2191778694931,46.7273611760722,123.606843477145)) ;
#25209=CARTESIAN_POINT('Ctrl Pts',(-17.9216561766812,46.5473720957093,123.655604769692)) ;
#25210=CARTESIAN_POINT('Ctrl Pts',(-18.2033482281936,46.7374380411502,123.395627154277)) ;
#25211=CARTESIAN_POINT('Ctrl Pts',(-17.9018683250634,46.5574489607873,123.391584873684)) ;
#25212=CARTESIAN_POINT('Ctrl Pts',(-18.2240747598041,46.7473027808054,123.189252605334)) ;
#25213=CARTESIAN_POINT('Ctrl Pts',(-17.9277757499098,46.5673137004426,123.133615388447)) ;
#25214=CARTESIAN_POINT('Ctrl Pts',(-18.2806784571676,46.7573251840468,122.986304105928)) ;
#25215=CARTESIAN_POINT('Ctrl Pts',(-17.9985297244048,46.5773361036839,122.879929630516)) ;
#25216=CARTESIAN_POINT('Ctrl Pts',(-18.3721757227985,46.7673509083353,122.796412957651)) ;
#25217=CARTESIAN_POINT('Ctrl Pts',(-18.1129004945136,46.5873618279724,122.642565399525)) ;
#25218=CARTESIAN_POINT('Ctrl Pts',(-18.4928445279093,46.7772056913566,122.628018609058)) ;
#25219=CARTESIAN_POINT('Ctrl Pts',(-18.2637366876288,46.5972166109937,122.432070963929)) ;
#25220=CARTESIAN_POINT('Ctrl Pts',(-18.6424131075352,46.7871845350798,122.480907272402)) ;
#25221=CARTESIAN_POINT('Ctrl Pts',(-18.4506972916997,46.607195454717,122.248181197861)) ;
#25222=CARTESIAN_POINT('Ctrl Pts',(-18.8161403685394,46.7972034273165,122.361831711629)) ;
#25223=CARTESIAN_POINT('Ctrl Pts',(-18.6678559884878,46.6172143469536,122.099336220667)) ;
#25224=CARTESIAN_POINT('Ctrl Pts',(-19.0051621248725,46.8070866363575,122.275502154482)) ;
#25225=CARTESIAN_POINT('Ctrl Pts',(-18.9041339832422,46.6270975559946,121.991423381431)) ;
#25226=CARTESIAN_POINT('Ctrl Pts',(-19.210031702073,46.8171549456977,122.222428926557)) ;
#25227=CARTESIAN_POINT('Ctrl Pts',(-19.1602204279234,46.6371658653348,121.925081449906)) ;
#25228=CARTESIAN_POINT('Ctrl Pts',(-19.4160633040709,46.8269850710304,122.205881850251)) ;
#25229=CARTESIAN_POINT('Ctrl Pts',(-19.4177614318243,46.6469959906675,121.904397063364)) ;
#25230=CARTESIAN_POINT('Ctrl Pts',(-19.6267444353502,46.8370516234074,122.22554880192)) ;
#25231=CARTESIAN_POINT('Ctrl Pts',(-19.6811124793488,46.6570625430445,121.928980404509)) ;
#25232=CARTESIAN_POINT('Ctrl Pts',(-19.8272585672866,46.8469418603011,122.280657735595)) ;
#25233=CARTESIAN_POINT('Ctrl Pts',(-19.93175625164,46.6669527799382,121.997866497326)) ;
#25234=CARTESIAN_POINT('Ctrl Pts',(-20.0172576560397,46.8569340850951,122.370232887069)) ;
#25235=CARTESIAN_POINT('Ctrl Pts',(-20.1692553844016,46.6769450047322,122.109835361796)) ;
#25236=CARTESIAN_POINT('Ctrl Pts',(-20.1882040593248,46.866896705446,122.491242308474)) ;
#25237=CARTESIAN_POINT('Ctrl Pts',(-20.3829389131417,46.6869076250832,122.261097188161)) ;
#25238=CARTESIAN_POINT('Ctrl Pts',(-20.3350687567512,46.8768017082092,122.638883740388)) ;
#25239=CARTESIAN_POINT('Ctrl Pts',(-20.5665204839457,46.6968126278463,122.445649602459)) ;
#25240=CARTESIAN_POINT('Ctrl Pts',(-20.4557645798383,46.8868594706073,122.812475638472)) ;
#25241=CARTESIAN_POINT('Ctrl Pts',(-20.7173901651887,46.7068703902444,122.662639131591)) ;
#25242=CARTESIAN_POINT('Ctrl Pts',(-20.5428264939987,46.8967099899861,123.000391779581)) ;
#25243=CARTESIAN_POINT('Ctrl Pts',(-20.8262181894773,46.7167209096232,122.89753556539)) ;
#25244=CARTESIAN_POINT('Ctrl Pts',(-20.5973539637941,46.9067415669843,123.204102169364)) ;
#25245=CARTESIAN_POINT('Ctrl Pts',(-20.8943773618054,46.7267524866214,123.15217347503)) ;
#25246=CARTESIAN_POINT('Ctrl Pts',(-20.6152416325616,46.9167513020892,123.413800001265)) ;
#25247=CARTESIAN_POINT('Ctrl Pts',(-20.9167369790523,46.7367622217263,123.414295804395)) ;
#25248=CARTESIAN_POINT('Ctrl Pts',(-20.5968220041765,46.9266608787155,123.621296181329)) ;
#25249=CARTESIAN_POINT('Ctrl Pts',(-20.8937123153054,46.7466717983526,123.673666920638)) ;
#25250=CARTESIAN_POINT('Ctrl Pts',(-20.5430662397492,46.9365882645721,123.822968750851)) ;
#25251=CARTESIAN_POINT('Ctrl Pts',(-20.8265171674148,46.7565991842093,123.925758286608)) ;
#25252=CARTESIAN_POINT('Ctrl Pts',(-20.4539206450829,46.9466331990624,124.014396648142)) ;
#25253=CARTESIAN_POINT('Ctrl Pts',(-20.7150850922258,46.7666441186995,124.165042883978)) ;
#25254=CARTESIAN_POINT('Ctrl Pts',(-20.3348959674513,46.9565191312504,124.184787009017)) ;
#25255=CARTESIAN_POINT('Ctrl Pts',(-20.566303423748,46.7765300508875,124.378031588581)) ;
#25256=CARTESIAN_POINT('Ctrl Pts',(-20.1867731077761,46.9665124372034,124.333759281434)) ;
#25257=CARTESIAN_POINT('Ctrl Pts',(-20.3811494336437,46.7865233568405,124.56424680321)) ;
#25258=CARTESIAN_POINT('Ctrl Pts',(-20.0157955120954,46.9764580749853,124.454112395529)) ;
#25259=CARTESIAN_POINT('Ctrl Pts',(-20.167426750717,46.7964689946224,124.714688252167)) ;
#25260=CARTESIAN_POINT('Ctrl Pts',(-19.8266604007549,46.9864053433312,124.543356690271)) ;
#25261=CARTESIAN_POINT('Ctrl Pts',(-19.9310071201226,46.8064162629683,124.826243396208)) ;
#25262=CARTESIAN_POINT('Ctrl Pts',(-19.6228151224958,46.9964532454683,124.598728489148)) ;
#25263=CARTESIAN_POINT('Ctrl Pts',(-19.6762006528589,46.8164641651054,124.895457669008)) ;
#25264=CARTESIAN_POINT('Ctrl Pts',(-19.4166526981356,47.0063009403085,124.617657767281)) ;
#25265=CARTESIAN_POINT('Ctrl Pts',(-19.4184961828357,46.8263118599456,124.91911890289)) ;
#25266=CARTESIAN_POINT('Ctrl Pts',(-19.2079050762096,47.0162624500529,124.600964149911)) ;
#25267=CARTESIAN_POINT('Ctrl Pts',(-19.1575612607115,46.83627336969,124.898251094209)) ;
#25268=CARTESIAN_POINT('Ctrl Pts',(-19.0039009099091,47.0262918416617,124.54764239375)) ;
#25269=CARTESIAN_POINT('Ctrl Pts',(-18.902556312997,46.8463027612989,124.831598304346)) ;
#25270=CARTESIAN_POINT('Ctrl Pts',(-18.8145419924307,47.0361993372165,124.460883485285)) ;
#25271=CARTESIAN_POINT('Ctrl Pts',(-18.6658571373904,46.8562102568536,124.723148671996)) ;
#25272=CARTESIAN_POINT('Ctrl Pts',(-18.642246189298,47.0461447288795,124.342465094977)) ;
#25273=CARTESIAN_POINT('Ctrl Pts',(-18.4504873824993,46.8661556485166,124.575124657286)) ;
#25274=CARTESIAN_POINT('Ctrl Pts',(-18.4921614871914,47.0561466464769,124.1951532533)) ;
#25275=CARTESIAN_POINT('Ctrl Pts',(-18.262882041295,46.876157566114,124.390984128)) ;
#25276=CARTESIAN_POINT('Ctrl Pts',(-18.3698136381604,47.0661867140291,124.023179183361)) ;
#25277=CARTESIAN_POINT('Ctrl Pts',(-18.1099479381027,46.8861976336662,124.176016249327)) ;
#25278=CARTESIAN_POINT('Ctrl Pts',(-18.2806928887342,47.0760110254689,123.836839708192)) ;
#25279=CARTESIAN_POINT('Ctrl Pts',(-17.998547175216,46.896021945106,123.943090129844)) ;
#25280=CARTESIAN_POINT('Ctrl Pts',(-18.2237020979738,47.086067266625,123.633273731581)) ;
#25281=CARTESIAN_POINT('Ctrl Pts',(-17.9273097685191,46.9060781862621,123.688632681324)) ;
#25282=CARTESIAN_POINT('Ctrl Pts',(-18.203421628533,47.0959981883606,123.425458332389)) ;
#25283=CARTESIAN_POINT('Ctrl Pts',(-17.9019600484687,46.9160091079977,123.4288626675)) ;
#25284=CARTESIAN_POINT('Ctrl Pts',(-18.2191232760878,47.1059414244368,123.217037662918)) ;
#25285=CARTESIAN_POINT('Ctrl Pts',(-17.9215882488076,46.925952344074,123.168336310537)) ;
#25286=CARTESIAN_POINT('Ctrl Pts',(-18.2707913644975,47.1159227084493,123.013627488194)) ;
#25287=CARTESIAN_POINT('Ctrl Pts',(-17.9861745623724,46.9359336280864,122.914073624315)) ;
#25288=CARTESIAN_POINT('Ctrl Pts',(-18.3578456878256,47.125967010075,122.821273166394)) ;
#25289=CARTESIAN_POINT('Ctrl Pts',(-18.0949933336756,46.9459779297121,122.673631325158)) ;
#25290=CARTESIAN_POINT('Ctrl Pts',(-18.4740478321358,47.1357950912944,122.650390408871)) ;
#25291=CARTESIAN_POINT('Ctrl Pts',(-18.2402478329783,46.9558060109315,122.460027367171)) ;
#25292=CARTESIAN_POINT('Ctrl Pts',(-18.6216725538285,47.1458716941436,122.498517159224)) ;
#25293=CARTESIAN_POINT('Ctrl Pts',(-18.4247793331419,46.9658826137807,122.270186990604)) ;
#25294=CARTESIAN_POINT('Ctrl Pts',(-18.789608451275,47.1557237732621,122.377209771896)) ;
#25295=CARTESIAN_POINT('Ctrl Pts',(-18.6347009617729,46.9757346928992,122.118553078034)) ;
#25296=CARTESIAN_POINT('Ctrl Pts',(-18.980091407923,47.165797031571,122.284749398737)) ;
#25297=CARTESIAN_POINT('Ctrl Pts',(-18.8728048873028,46.9858079512082,122.002979006205)) ;
#25298=CARTESIAN_POINT('Ctrl Pts',(-19.1791102852178,47.1756384909513,122.228144087822)) ;
#25299=CARTESIAN_POINT('Ctrl Pts',(-19.1215801045156,46.9956494105884,121.93222329205)) ;
#25300=CARTESIAN_POINT('Ctrl Pts',(-19.3873332175923,47.1855995863637,122.205917819797)) ;
#25301=CARTESIAN_POINT('Ctrl Pts',(-19.381859343394,47.0056105060008,121.904442012515)) ;
#25302=CARTESIAN_POINT('Ctrl Pts',(-19.5978250311267,47.1956368707604,122.220705841968)) ;
#25303=CARTESIAN_POINT('Ctrl Pts',(-19.6449738782894,47.0156477903975,121.922928491226)) ;
#25304=CARTESIAN_POINT('Ctrl Pts',(-19.7993828425593,47.2055132094957,122.270652196407)) ;
#25305=CARTESIAN_POINT('Ctrl Pts',(-19.8969217299239,47.0255241291328,121.985363214302)) ;
#25306=CARTESIAN_POINT('Ctrl Pts',(-19.9927485786675,47.2155753356489,122.356364369119)) ;
#25307=CARTESIAN_POINT('Ctrl Pts',(-20.1386279884017,47.0355862552861,122.092504779786)) ;
#25308=CARTESIAN_POINT('Ctrl Pts',(-20.1649812697198,47.2254435096255,122.472061623222)) ;
#25309=CARTESIAN_POINT('Ctrl Pts',(-20.3539188130597,47.0454544292626,122.237128270037)) ;
#25310=CARTESIAN_POINT('Ctrl Pts',(-20.3168466409141,47.2354490581293,122.61756598711)) ;
#25311=CARTESIAN_POINT('Ctrl Pts',(-20.5437493740665,47.0554599777664,122.419010050859)) ;
#25312=CARTESIAN_POINT('Ctrl Pts',(-20.4408371920724,47.2454316900249,122.7869363998)) ;
#25313=CARTESIAN_POINT('Ctrl Pts',(-20.6987362985448,47.065442609662,122.630724270001)) ;
#25314=CARTESIAN_POINT('Ctrl Pts',(-20.5338834735868,47.2554756324466,122.976466219455)) ;
#25315=CARTESIAN_POINT('Ctrl Pts',(-20.8150425909332,47.0754865520838,122.867637130232)) ;
#25316=CARTESIAN_POINT('Ctrl Pts',(-20.5916167588128,47.2653037804738,123.17485450326)) ;
#25317=CARTESIAN_POINT('Ctrl Pts',(-20.8872078791894,47.0853147001109,123.115624213289)) ;
#25318=CARTESIAN_POINT('Ctrl Pts',(-20.6150653225155,47.2752936478482,123.383560571913)) ;
#25319=CARTESIAN_POINT('Ctrl Pts',(-20.9165166534759,47.0953045674853,123.37650718992)) ;
#25320=CARTESIAN_POINT('Ctrl Pts',(-20.601300740418,47.2853373868037,123.594262445601)) ;
#25321=CARTESIAN_POINT('Ctrl Pts',(-20.8993091493922,47.1053483064408,123.639884268201)) ;
#25322=CARTESIAN_POINT('Ctrl Pts',(-20.552687444503,47.2951591353416,123.794940800993)) ;
#25323=CARTESIAN_POINT('Ctrl Pts',(-20.8385403650369,47.1151700549788,123.890732974447)) ;
#25324=CARTESIAN_POINT('Ctrl Pts',(-20.4686462395042,47.3051941129514,123.988445576631)) ;
#25325=CARTESIAN_POINT('Ctrl Pts',(-20.7334869965978,47.1252050325885,124.132613019297)) ;
#25326=CARTESIAN_POINT('Ctrl Pts',(-20.3519069360569,47.3152190257091,124.163922378538)) ;
#25327=CARTESIAN_POINT('Ctrl Pts',(-20.5875612969449,47.1352299453462,124.351957946675)) ;
#25328=CARTESIAN_POINT('Ctrl Pts',(-20.2093112218679,47.3250709688029,124.314143088258)) ;
#25329=CARTESIAN_POINT('Ctrl Pts',(-20.4093144805832,47.14508188844,124.539733165987)) ;
#25330=CARTESIAN_POINT('Ctrl Pts',(-20.0406636984681,47.335061930132,124.439301449808)) ;
#25331=CARTESIAN_POINT('Ctrl Pts',(-20.1985036701278,47.1550728497691,124.69617951058)) ;
#25332=CARTESIAN_POINT('Ctrl Pts',(-19.8542359453285,47.3449798050004,124.532734343896)) ;
#25333=CARTESIAN_POINT('Ctrl Pts',(-19.9654674976531,47.1649907246376,124.812968953075)) ;
#25334=CARTESIAN_POINT('Ctrl Pts',(-19.6522424998238,47.3550083240017,124.593072966075)) ;
#25335=CARTESIAN_POINT('Ctrl Pts',(-19.71297510293,47.1750192436388,124.88839013585)) ;
#25336=CARTESIAN_POINT('Ctrl Pts',(-19.4458515602898,47.3648920027995,124.617180149755)) ;
#25337=CARTESIAN_POINT('Ctrl Pts',(-19.4549854354218,47.1849029224366,124.918522015687)) ;
#25338=CARTESIAN_POINT('Ctrl Pts',(-19.2360564520279,47.3748869462393,124.605411359256)) ;
#25339=CARTESIAN_POINT('Ctrl Pts',(-19.1927415406444,47.1948978658764,124.903808702217)) ;
#25340=CARTESIAN_POINT('Ctrl Pts',(-19.0309200127824,47.3849138000617,124.556888090555)) ;
#25341=CARTESIAN_POINT('Ctrl Pts',(-18.9363215273581,47.2049247196988,124.843152452533)) ;
#25342=CARTESIAN_POINT('Ctrl Pts',(-18.8399600132762,47.3947979644006,124.474930121574)) ;
#25343=CARTESIAN_POINT('Ctrl Pts',(-18.6976217950589,47.2148088840377,124.740702605869)) ;
#25344=CARTESIAN_POINT('Ctrl Pts',(-18.6641751096275,47.404786062443,124.360112233341)) ;
#25345=CARTESIAN_POINT('Ctrl Pts',(-18.4778918251213,47.2247969820801,124.597178175501)) ;
#25346=CARTESIAN_POINT('Ctrl Pts',(-18.5114500487226,47.4147371689001,124.217101265402)) ;
#25347=CARTESIAN_POINT('Ctrl Pts',(-18.2869868870465,47.2347480885372,124.418412493407)) ;
#25348=CARTESIAN_POINT('Ctrl Pts',(-18.3848081572941,47.4247822200682,124.048124629567)) ;
#25349=CARTESIAN_POINT('Ctrl Pts',(-18.1286864683151,47.2447931397053,124.207190353518)) ;
#25350=CARTESIAN_POINT('Ctrl Pts',(-18.2910618402465,47.4346439804265,123.86320370385)) ;
#25351=CARTESIAN_POINT('Ctrl Pts',(-18.0115053675036,47.2546549000636,123.976037450219)) ;
#25352=CARTESIAN_POINT('Ctrl Pts',(-18.2296126467464,47.4446067972569,123.662969790822)) ;
#25353=CARTESIAN_POINT('Ctrl Pts',(-17.9346962187188,47.264617716894,123.725744078448)) ;
#25354=CARTESIAN_POINT('Ctrl Pts',(-18.2040389740413,47.4546414785377,123.45357433271)) ;
#25355=CARTESIAN_POINT('Ctrl Pts',(-17.9027315659369,47.2746523981748,123.463999492697)) ;
#25356=CARTESIAN_POINT('Ctrl Pts',(-18.2146920724958,47.4645265083184,123.246004580245)) ;
#25357=CARTESIAN_POINT('Ctrl Pts',(-17.9160504867167,47.2845374279556,123.204536864795)) ;
#25358=CARTESIAN_POINT('Ctrl Pts',(-18.2621069746344,47.4745921017164,123.039809498366)) ;
#25359=CARTESIAN_POINT('Ctrl Pts',(-17.9753215326006,47.2946030213536,122.946793722897)) ;
#25360=CARTESIAN_POINT('Ctrl Pts',(-18.3425816794122,47.4844312700779,122.849220328905)) ;
#25361=CARTESIAN_POINT('Ctrl Pts',(-18.0759175402315,47.3044421897151,122.708557598471)) ;
#25362=CARTESIAN_POINT('Ctrl Pts',(-18.457201944164,47.4944938678194,122.671444955583)) ;
#25363=CARTESIAN_POINT('Ctrl Pts',(-18.2191949884316,47.3145047874566,122.486339905974)) ;
#25364=CARTESIAN_POINT('Ctrl Pts',(-18.5987718864396,47.5043908802264,122.518950167232)) ;
#25365=CARTESIAN_POINT('Ctrl Pts',(-18.396159615514,47.3244017998635,122.295722821703)) ;
#25366=CARTESIAN_POINT('Ctrl Pts',(-18.7648105631557,47.514322202052,122.392374159236)) ;
#25367=CARTESIAN_POINT('Ctrl Pts',(-18.6037098264549,47.3343331216891,122.137504758704)) ;
#25368=CARTESIAN_POINT('Ctrl Pts',(-18.9524743880465,47.5243639648065,122.295687498941)) ;
#25369=CARTESIAN_POINT('Ctrl Pts',(-18.8382907890392,47.3443748844436,122.016648795488)) ;
#25370=CARTESIAN_POINT('Ctrl Pts',(-19.1509626646768,47.5342521636972,122.233865751707)) ;
#25371=CARTESIAN_POINT('Ctrl Pts',(-19.0864023365642,47.3542630833343,121.939374027969)) ;
#25372=CARTESIAN_POINT('Ctrl Pts',(-19.3593042021687,47.544246102297,122.206837954189)) ;
#25373=CARTESIAN_POINT('Ctrl Pts',(-19.3468297085847,47.3642570219342,121.905591956175)) ;
#25374=CARTESIAN_POINT('Ctrl Pts',(-19.5680879347369,47.5541869233339,122.216359937286)) ;
#25375=CARTESIAN_POINT('Ctrl Pts',(-19.6078094898697,47.374197842971,121.917497147633)) ;
#25376=CARTESIAN_POINT('Ctrl Pts',(-19.7724614957895,47.5641463056221,122.26180879175)) ;
#25377=CARTESIAN_POINT('Ctrl Pts',(-19.8632760200849,47.3841572252593,121.974310927408)) ;
#25378=CARTESIAN_POINT('Ctrl Pts',(-19.966662779158,47.5741440652745,122.342257817906)) ;
#25379=CARTESIAN_POINT('Ctrl Pts',(-20.1060266518377,47.3941549849116,122.074874782439)) ;
#25380=CARTESIAN_POINT('Ctrl Pts',(-20.1444477349424,47.5841802014768,122.455869269298)) ;
#25381=CARTESIAN_POINT('Ctrl Pts',(-20.3282563986287,47.4041911211139,122.216891398893)) ;
#25382=CARTESIAN_POINT('Ctrl Pts',(-20.2971040279646,47.5940309989677,122.595810595244)) ;
#25383=CARTESIAN_POINT('Ctrl Pts',(-20.5190751999569,47.4140419186048,122.391820347718)) ;
#25384=CARTESIAN_POINT('Ctrl Pts',(-20.425042108738,47.603991864044,122.761583938118)) ;
#25385=CARTESIAN_POINT('Ctrl Pts',(-20.6789956607079,47.4240027836811,122.599038839022)) ;
#25386=CARTESIAN_POINT('Ctrl Pts',(-20.5226996631887,47.6140207316744,122.948455189612)) ;
#25387=CARTESIAN_POINT('Ctrl Pts',(-20.8010651623618,47.4340316513115,122.832629226849)) ;
#25388=CARTESIAN_POINT('Ctrl Pts',(-20.5857281504088,47.6239309678108,123.147028040722)) ;
#25389=CARTESIAN_POINT('Ctrl Pts',(-20.8798481803655,47.4439418874479,123.080846336945)) ;
#25390=CARTESIAN_POINT('Ctrl Pts',(-20.6139336283943,47.6338659211253,123.353984814139)) ;
#25391=CARTESIAN_POINT('Ctrl Pts',(-20.9151022554273,47.4538768407624,123.339542816455)) ;
#25392=CARTESIAN_POINT('Ctrl Pts',(-20.605496943485,47.6439068515349,123.564903134672)) ;
#25393=CARTESIAN_POINT('Ctrl Pts',(-20.9045535939109,47.463917771172,123.603190649991)) ;
#25394=CARTESIAN_POINT('Ctrl Pts',(-20.5613779871071,47.6537947483165,123.768050424334)) ;
#25395=CARTESIAN_POINT('Ctrl Pts',(-20.849402115707,47.4738056679536,123.857124325427)) ;
#25396=CARTESIAN_POINT('Ctrl Pts',(-20.4822143423052,47.6637841999752,123.962563095657)) ;
#25397=CARTESIAN_POINT('Ctrl Pts',(-20.750444918412,47.4837951196123,124.1002641636)) ;
#25398=CARTESIAN_POINT('Ctrl Pts',(-20.370678012507,47.6737432903405,124.139744915088)) ;
#25399=CARTESIAN_POINT('Ctrl Pts',(-20.6110220669267,47.4937542099777,124.321740017003)) ;
#25400=CARTESIAN_POINT('Ctrl Pts',(-20.2313246232406,47.6836406026468,124.294278132182)) ;
#25401=CARTESIAN_POINT('Ctrl Pts',(-20.4368281965108,47.503651522284,124.514904688104)) ;
#25402=CARTESIAN_POINT('Ctrl Pts',(-20.0645809253998,47.6936970285471,124.424226886793)) ;
#25403=CARTESIAN_POINT('Ctrl Pts',(-20.2283967744204,47.5137079481842,124.677338457595)) ;
#25404=CARTESIAN_POINT('Ctrl Pts',(-19.8812864921283,47.7035670311368,124.521524514142)) ;
#25405=CARTESIAN_POINT('Ctrl Pts',(-19.9992773799533,47.523577950774,124.798958001509)) ;
#25406=CARTESIAN_POINT('Ctrl Pts',(-19.6813729094116,47.7135709643141,124.586772503536)) ;
#25407=CARTESIAN_POINT('Ctrl Pts',(-19.7493845402161,47.5335818839512,124.880515352736)) ;
#25408=CARTESIAN_POINT('Ctrl Pts',(-19.4734437265146,47.723558224778,124.616166289177)) ;
#25409=CARTESIAN_POINT('Ctrl Pts',(-19.4894723640348,47.5435691444151,124.917254732859)) ;
#25410=CARTESIAN_POINT('Ctrl Pts',(-19.2627853496724,47.7335852763637,124.608859964159)) ;
#25411=CARTESIAN_POINT('Ctrl Pts',(-19.2261503135035,47.5535961960008,124.908119289949)) ;
#25412=CARTESIAN_POINT('Ctrl Pts',(-19.0593193011781,47.7434763661898,124.565875611357)) ;
#25413=CARTESIAN_POINT('Ctrl Pts',(-18.9718149570964,47.5634872858269,124.854385043497)) ;
#25414=CARTESIAN_POINT('Ctrl Pts',(-18.7998791514015,47.7567741209708,124.46180634869)) ;
#25415=CARTESIAN_POINT('Ctrl Pts',(-18.6475331408761,47.576785040608,124.724300286802)) ;
#25416=CARTESIAN_POINT('Ctrl Pts',(-18.5749055156603,47.769972180579,124.293953042302)) ;
#25417=CARTESIAN_POINT('Ctrl Pts',(-18.3663382799237,47.5899831002161,124.51451143139)) ;
#25418=CARTESIAN_POINT('Ctrl Pts',(-18.4005844763,47.7833689211482,124.072822952987)) ;
#25419=CARTESIAN_POINT('Ctrl Pts',(-18.1483991888473,47.6033798407853,124.238054641967)) ;
#25420=CARTESIAN_POINT('Ctrl Pts',(-18.3021342969201,47.7932398332216,123.890089252221)) ;
#25421=CARTESIAN_POINT('Ctrl Pts',(-18.025347143704,47.6132507528587,124.009644853001)) ;
#25422=CARTESIAN_POINT('Ctrl Pts',(-18.2356106700847,47.8033133949897,123.689082460906)) ;
#25423=CARTESIAN_POINT('Ctrl Pts',(-17.9421929511721,47.6233243146269,123.758382877817)) ;
#25424=CARTESIAN_POINT('Ctrl Pts',(-18.2055029737511,47.8131348075781,123.484761908509)) ;
#25425=CARTESIAN_POINT('Ctrl Pts',(-17.9045616883877,47.6331457272152,123.502983370987)) ;
#25426=CARTESIAN_POINT('Ctrl Pts',(-18.2112771538204,47.8232088248091,123.273106955294)) ;
#25427=CARTESIAN_POINT('Ctrl Pts',(-17.911781843042,47.6432197444462,123.238412336144)) ;
#25428=CARTESIAN_POINT('Ctrl Pts',(-18.2665340735366,47.8363676117737,123.001975829454)) ;
#25429=CARTESIAN_POINT('Ctrl Pts',(-17.9808569614933,47.6563785314108,122.899509564629)) ;
#25430=CARTESIAN_POINT('Ctrl Pts',(-18.3927847313785,47.8497337148678,122.747421002799)) ;
#25431=CARTESIAN_POINT('Ctrl Pts',(-18.1386436633673,47.669744634505,122.581350825213)) ;
#25432=CARTESIAN_POINT('Ctrl Pts',(-18.5783616406369,47.8630476497569,122.537834672679)) ;
#25433=CARTESIAN_POINT('Ctrl Pts',(-18.370652315842,47.683058569394,122.319320691079)) ;
#25434=CARTESIAN_POINT('Ctrl Pts',(-18.7409869953793,47.8729476892044,122.407978701696)) ;
#25435=CARTESIAN_POINT('Ctrl Pts',(-18.5739282398627,47.6929586088415,122.157012936139)) ;
#25436=CARTESIAN_POINT('Ctrl Pts',(-18.924736336014,47.8829120923389,122.307361857159)) ;
#25437=CARTESIAN_POINT('Ctrl Pts',(-18.8036181717246,47.702923011976,122.031241515346)) ;
#25438=CARTESIAN_POINT('Ctrl Pts',(-19.124525129965,47.89294205946,122.239917422604)) ;
#25439=CARTESIAN_POINT('Ctrl Pts',(-19.0533535758895,47.7129529790972,121.946938831321)) ;
#25440=CARTESIAN_POINT('Ctrl Pts',(-19.3303060797298,47.9028443360691,122.20850438304)) ;
#25441=CARTESIAN_POINT('Ctrl Pts',(-19.3105838879911,47.7228552557062,121.907675661922)) ;
#25442=CARTESIAN_POINT('Ctrl Pts',(-19.6091875472562,47.9161102652382,122.214220010693)) ;
#25443=CARTESIAN_POINT('Ctrl Pts',(-19.6591650885652,47.7361211848754,121.914819682812)) ;
#25444=CARTESIAN_POINT('Ctrl Pts',(-19.9485239198388,47.9327317963447,122.312705470027)) ;
#25445=CARTESIAN_POINT('Ctrl Pts',(-20.0833550247634,47.7527427159818,122.037930509702)) ;
#25446=CARTESIAN_POINT('Ctrl Pts',(-20.2902037781463,47.9526066249893,122.561462918073)) ;
#25447=CARTESIAN_POINT('Ctrl Pts',(-20.510453729545,47.7726175446265,122.348898697034)) ;
#25448=CARTESIAN_POINT('Ctrl Pts',(-20.4884640691053,47.9692798330912,122.855376240776)) ;
#25449=CARTESIAN_POINT('Ctrl Pts',(-20.7582479358267,47.7892907527283,122.71623189636)) ;
#25450=CARTESIAN_POINT('Ctrl Pts',(-20.5789910924744,47.9825309580725,123.118806998675)) ;
#25451=CARTESIAN_POINT('Ctrl Pts',(-20.8714295868913,47.8025418777096,123.04557591284)) ;
#25452=CARTESIAN_POINT('Ctrl Pts',(-20.6233964771784,47.9957732768933,123.393706926206)) ;
#25453=CARTESIAN_POINT('Ctrl Pts',(-20.9269298434521,47.8157841965304,123.389178316211)) ;
#25454=CARTESIAN_POINT('Ctrl Pts',(-20.5867718231029,48.0125065172328,123.747531507057)) ;
#25455=CARTESIAN_POINT('Ctrl Pts',(-20.881145520325,47.8325174368699,123.831476120658)) ;
#25456=CARTESIAN_POINT('Ctrl Pts',(-20.4028036698389,48.0323356654207,124.126994342041)) ;
#25457=CARTESIAN_POINT('Ctrl Pts',(-20.6511822086368,47.8523465850579,124.305796219641)) ;
#25458=CARTESIAN_POINT('Ctrl Pts',(-20.0997742547527,48.0522603605214,124.422927439283)) ;
#25459=CARTESIAN_POINT('Ctrl Pts',(-20.2723934902227,47.8722712801585,124.675711001554)) ;
#25460=CARTESIAN_POINT('Ctrl Pts',(-19.7138146747958,48.0721835891048,124.597703149849)) ;
#25461=CARTESIAN_POINT('Ctrl Pts',(-19.7899432576281,47.8921945087419,124.89417687357)) ;
#25462=CARTESIAN_POINT('Ctrl Pts',(-19.2914240334227,48.0921107282309,124.630406193651)) ;
#25463=CARTESIAN_POINT('Ctrl Pts',(-19.2619554888101,47.912121647868,124.935052545408)) ;
#25464=CARTESIAN_POINT('Ctrl Pts',(-18.8840463674362,48.1119871908466,124.517801066557)) ;
#25465=CARTESIAN_POINT('Ctrl Pts',(-18.7527354696576,47.9319981104837,124.794293876189)) ;
#25466=CARTESIAN_POINT('Ctrl Pts',(-18.5376979877752,48.1319644194519,124.271899046843)) ;
#25467=CARTESIAN_POINT('Ctrl Pts',(-18.3198015893089,47.951975339089,124.486914551041)) ;
#25468=CARTESIAN_POINT('Ctrl Pts',(-18.2968188645784,48.1518992774256,123.923081812922)) ;
#25469=CARTESIAN_POINT('Ctrl Pts',(-18.0187050938315,47.9719101970627,124.050892286809)) ;
#25470=CARTESIAN_POINT('Ctrl Pts',(-18.1892385120565,48.1717957263564,123.513969714441)) ;
#25471=CARTESIAN_POINT('Ctrl Pts',(-17.8842318765923,47.9918066459935,123.539502996666)) ;
#25472=CARTESIAN_POINT('Ctrl Pts',(-18.2273051805781,48.191717010423,123.092084857011)) ;
#25473=CARTESIAN_POINT('Ctrl Pts',(-17.9318165298211,48.0117279300601,123.012148120241)) ;
#25474=CARTESIAN_POINT('Ctrl Pts',(-18.4074959386059,48.2116736600939,122.707887148316)) ;
#25475=CARTESIAN_POINT('Ctrl Pts',(-18.1570558911766,48.0316845797311,122.53190203543)) ;
#25476=CARTESIAN_POINT('Ctrl Pts',(-18.7066336703321,48.2315509532055,122.409391624937)) ;
#25477=CARTESIAN_POINT('Ctrl Pts',(-18.5309774065162,48.0515618728427,122.158784664484)) ;
#25478=CARTESIAN_POINT('Ctrl Pts',(-19.0894690754,48.251437425434,122.229752123671)) ;
#25479=CARTESIAN_POINT('Ctrl Pts',(-19.0095199143223,48.0714483450711,121.934235959805)) ;
#25480=CARTESIAN_POINT('Ctrl Pts',(-19.5143590700572,48.271498991358,122.191844649005)) ;
#25481=CARTESIAN_POINT('Ctrl Pts',(-19.540633493891,48.0915099109951,121.886851609452)) ;
#25482=CARTESIAN_POINT('Ctrl Pts',(-19.9220000869853,48.2913393988987,122.300380775824)) ;
#25483=CARTESIAN_POINT('Ctrl Pts',(-20.0501821768271,48.1113503185359,122.022521216227)) ;
#25484=CARTESIAN_POINT('Ctrl Pts',(-20.2693591113835,48.3111907228717,122.540208509566)) ;
#25485=CARTESIAN_POINT('Ctrl Pts',(-20.4843799802069,48.1312016425088,122.322303458234)) ;
#25486=CARTESIAN_POINT('Ctrl Pts',(-20.515946924029,48.3312439928231,122.887990451022)) ;
#25487=CARTESIAN_POINT('Ctrl Pts',(-20.7926161664346,48.1512549124602,122.757030819445)) ;
#25488=CARTESIAN_POINT('Ctrl Pts',(-20.6278740447954,48.3510646502064,123.29441743572)) ;
#25489=CARTESIAN_POINT('Ctrl Pts',(-20.93252583496,48.1710755698436,123.265061844735)) ;
#25490=CARTESIAN_POINT('Ctrl Pts',(-20.594840913384,48.3710360715369,123.717637162342)) ;
#25491=CARTESIAN_POINT('Ctrl Pts',(-20.8912365983079,48.1910469911741,123.794086280571)) ;
#25492=CARTESIAN_POINT('Ctrl Pts',(-20.4200275936189,48.3909295639006,124.102979449163)) ;
#25493=CARTESIAN_POINT('Ctrl Pts',(-20.6727225902505,48.2109404835378,124.275764014104)) ;
#25494=CARTESIAN_POINT('Ctrl Pts',(-20.1222338289871,48.4109536501417,124.407148329069)) ;
#25495=CARTESIAN_POINT('Ctrl Pts',(-20.3004819424767,48.2309645697788,124.655976968053)) ;
#25496=CARTESIAN_POINT('Ctrl Pts',(-19.7426972067717,48.4307585292546,124.589684508702)) ;
#25497=CARTESIAN_POINT('Ctrl Pts',(-19.8260643109497,48.2507694488917,124.884148701362)) ;
#25498=CARTESIAN_POINT('Ctrl Pts',(-19.3205665484207,48.4507175449524,124.633213336041)) ;
#25499=CARTESIAN_POINT('Ctrl Pts',(-19.298401689414,48.2707284645896,124.938563164576)) ;
#25500=CARTESIAN_POINT('Ctrl Pts',(-18.9085978348677,48.4707035685815,124.528976750497)) ;
#25501=CARTESIAN_POINT('Ctrl Pts',(-18.7834401752579,48.2907144882186,124.808270536172)) ;
#25502=CARTESIAN_POINT('Ctrl Pts',(-18.5595521592662,48.490512064342,124.293192736646)) ;
#25503=CARTESIAN_POINT('Ctrl Pts',(-18.3471324483424,48.3105229839791,124.513544556307)) ;
#25504=CARTESIAN_POINT('Ctrl Pts',(-18.3093912570992,48.5104947034476,123.949871011709)) ;
#25505=CARTESIAN_POINT('Ctrl Pts',(-18.0344280932835,48.3305056230847,124.084394876722)) ;
#25506=CARTESIAN_POINT('Ctrl Pts',(-18.1920511017376,48.5303761512416,123.543638375906)) ;
#25507=CARTESIAN_POINT('Ctrl Pts',(-17.8877491679608,48.3503870708787,123.576606049549)) ;
#25508=CARTESIAN_POINT('Ctrl Pts',(-18.2201380169056,48.5503326179791,123.120331661826)) ;
#25509=CARTESIAN_POINT('Ctrl Pts',(-17.9228534217252,48.3703435376163,123.047472668677)) ;
#25510=CARTESIAN_POINT('Ctrl Pts',(-18.3901149333137,48.5702100149347,122.733295429989)) ;
#25511=CARTESIAN_POINT('Ctrl Pts',(-18.1353200268485,48.3902209345718,122.563676201082)) ;
#25512=CARTESIAN_POINT('Ctrl Pts',(-18.6832494392057,48.59019196111,122.425805232135)) ;
#25513=CARTESIAN_POINT('Ctrl Pts',(-18.5017348375152,48.4102028807471,122.179310317759)) ;
#25514=CARTESIAN_POINT('Ctrl Pts',(-19.0629244099466,48.6101210601467,122.237437305555)) ;
#25515=CARTESIAN_POINT('Ctrl Pts',(-18.9763255338847,48.4301319797839,121.943845821942)) ;
#25516=CARTESIAN_POINT('Ctrl Pts',(-19.483901793505,48.6300496833594,122.189890024133)) ;
#25517=CARTESIAN_POINT('Ctrl Pts',(-19.5025485758174,48.4500606029965,121.8844085627)) ;
#25518=CARTESIAN_POINT('Ctrl Pts',(-19.8941924839498,48.6498840074658,122.2876543526)) ;
#25519=CARTESIAN_POINT('Ctrl Pts',(-20.0154041734413,48.4698949271029,122.006602474331)) ;
#25520=CARTESIAN_POINT('Ctrl Pts',(-20.1900657132766,48.6665362948492,122.481970833508)) ;
#25521=CARTESIAN_POINT('Ctrl Pts',(-20.3852740340378,48.4865472144863,122.249514009236)) ;
#25522=CARTESIAN_POINT('Ctrl Pts',(-20.375507427574,48.6797967958714,122.690222552236)) ;
#25523=CARTESIAN_POINT('Ctrl Pts',(-20.6170557319961,48.4998077155085,122.509808729621)) ;
#25524=CARTESIAN_POINT('Ctrl Pts',(-20.4862754015006,48.6897982730727,122.868932780703)) ;
#25525=CARTESIAN_POINT('Ctrl Pts',(-20.7555225669231,48.5098091927098,122.73319887295)) ;
#25526=CARTESIAN_POINT('Ctrl Pts',(-20.5642475378503,48.6998302939322,123.064902655755)) ;
#25527=CARTESIAN_POINT('Ctrl Pts',(-20.8529891978789,48.5198412135693,122.978158629166)) ;
#25528=CARTESIAN_POINT('Ctrl Pts',(-20.6065360548538,48.7096938376577,123.267899186555)) ;
#25529=CARTESIAN_POINT('Ctrl Pts',(-20.9058519382839,48.5297047572949,123.231906669117)) ;
#25530=CARTESIAN_POINT('Ctrl Pts',(-20.6135560240591,48.7196625513279,123.477368148513)) ;
#25531=CARTESIAN_POINT('Ctrl Pts',(-20.9146324101858,48.539673470965,123.493731289981)) ;
#25532=CARTESIAN_POINT('Ctrl Pts',(-20.5737423786962,48.7330082987316,123.755033330118)) ;
#25533=CARTESIAN_POINT('Ctrl Pts',(-20.8648547231583,48.5530192183687,123.840870176946)) ;
#25534=CARTESIAN_POINT('Ctrl Pts',(-20.4644055794944,48.7461588538042,124.012444095883)) ;
#25535=CARTESIAN_POINT('Ctrl Pts',(-20.7281894338226,48.5661697734414,124.16259745941)) ;
#25536=CARTESIAN_POINT('Ctrl Pts',(-20.2913023971137,48.7595442343541,124.234297005858)) ;
#25537=CARTESIAN_POINT('Ctrl Pts',(-20.5118249048892,48.5795551539912,124.439903596676)) ;
#25538=CARTESIAN_POINT('Ctrl Pts',(-20.1368920609285,48.7694321703469,124.373504586034)) ;
#25539=CARTESIAN_POINT('Ctrl Pts',(-20.3188115906214,48.5894430899841,124.613917552832)) ;
#25540=CARTESIAN_POINT('Ctrl Pts',(-19.9590459239484,48.7794233601596,124.485212508452)) ;
#25541=CARTESIAN_POINT('Ctrl Pts',(-20.0965059871697,48.5994342797967,124.753554193822)) ;
#25542=CARTESIAN_POINT('Ctrl Pts',(-19.7652457599506,48.7893754586979,124.564139501548)) ;
#25543=CARTESIAN_POINT('Ctrl Pts',(-19.8542566549361,48.609386378335,124.852215716831)) ;
#25544=CARTESIAN_POINT('Ctrl Pts',(-19.5587662011907,48.7994217151483,124.608490141116)) ;
#25545=CARTESIAN_POINT('Ctrl Pts',(-19.5961577410576,48.6194326347855,124.907656726796)) ;
#25546=CARTESIAN_POINT('Ctrl Pts',(-19.3518437628438,48.8092711625425,124.616313912249)) ;
#25547=CARTESIAN_POINT('Ctrl Pts',(-19.337504837007,48.6292820821796,124.917439257159)) ;
#25548=CARTESIAN_POINT('Ctrl Pts',(-19.1442698754285,48.8192338150376,124.588420325865)) ;
#25549=CARTESIAN_POINT('Ctrl Pts',(-19.078037022272,48.6392447346748,124.882575057759)) ;
#25550=CARTESIAN_POINT('Ctrl Pts',(-18.9435612342431,48.8292569006798,124.52425240661)) ;
#25551=CARTESIAN_POINT('Ctrl Pts',(-18.8271502999389,48.6492678203169,124.802367820736)) ;
#25552=CARTESIAN_POINT('Ctrl Pts',(-18.7587343657275,48.8391820164367,124.427368142674)) ;
#25553=CARTESIAN_POINT('Ctrl Pts',(-18.5961153422512,48.6591929360738,124.681264951306)) ;
#25554=CARTESIAN_POINT('Ctrl Pts',(-18.5915035853904,48.8492344948365,124.298186724899)) ;
#25555=CARTESIAN_POINT('Ctrl Pts',(-18.3870750955819,48.6692454144736,124.519790373217)) ;
#25556=CARTESIAN_POINT('Ctrl Pts',(-18.4519608110317,48.8590859935392,124.14512278795)) ;
#25557=CARTESIAN_POINT('Ctrl Pts',(-18.2126444694148,48.6790969131764,124.328462267053)) ;
#25558=CARTESIAN_POINT('Ctrl Pts',(-18.3393227852187,48.8690577327418,123.968347894014)) ;
#25559=CARTESIAN_POINT('Ctrl Pts',(-18.0718445075732,48.6890686523789,124.107495060904)) ;
#25560=CARTESIAN_POINT('Ctrl Pts',(-18.2589016789919,48.8790529405074,123.774178747308)) ;
#25561=CARTESIAN_POINT('Ctrl Pts',(-17.9713155069276,48.6990638601446,123.86478462589)) ;
#25562=CARTESIAN_POINT('Ctrl Pts',(-18.2135023400313,48.8890869419765,123.568194672117)) ;
#25563=CARTESIAN_POINT('Ctrl Pts',(-17.9145635742469,48.7090978616136,123.607305099869)) ;
#25564=CARTESIAN_POINT('Ctrl Pts',(-18.2043860504649,48.8989423000689,123.361183900461)) ;
#25565=CARTESIAN_POINT('Ctrl Pts',(-17.9031654069168,48.718953219706,123.348541528174)) ;
#25566=CARTESIAN_POINT('Ctrl Pts',(-18.2314583491406,48.9089417756622,123.152751792762)) ;
#25567=CARTESIAN_POINT('Ctrl Pts',(-17.937003026666,48.7289526952993,123.088000944887)) ;
#25568=CARTESIAN_POINT('Ctrl Pts',(-18.2934466731116,48.9188362241573,122.954149298326)) ;
#25569=CARTESIAN_POINT('Ctrl Pts',(-18.0144858731634,48.7388471437944,122.839746756377)) ;
#25570=CARTESIAN_POINT('Ctrl Pts',(-18.3906263668652,48.928899348385,122.766272454152)) ;
#25571=CARTESIAN_POINT('Ctrl Pts',(-18.1359580112243,48.7489102680221,122.604899456879)) ;
#25572=CARTESIAN_POINT('Ctrl Pts',(-18.5159623132325,48.9387389747136,122.601663674346)) ;
#25573=CARTESIAN_POINT('Ctrl Pts',(-18.2926260056632,48.7587498943507,122.399136493447)) ;
#25574=CARTESIAN_POINT('Ctrl Pts',(-18.6712011618515,48.9488022097566,122.457974021879)) ;
#25575=CARTESIAN_POINT('Ctrl Pts',(-18.4866726839865,48.7688131293937,122.219522458127)) ;
#25576=CARTESIAN_POINT('Ctrl Pts',(-18.8461785268419,48.9586962149906,122.345468773217)) ;
#25577=CARTESIAN_POINT('Ctrl Pts',(-18.7053931823134,48.7787071346277,122.078888414331)) ;
#25578=CARTESIAN_POINT('Ctrl Pts',(-19.038712835581,48.9686389282064,122.264147456417)) ;
#25579=CARTESIAN_POINT('Ctrl Pts',(-18.9460602718396,48.7886498478435,121.977234200229)) ;
#25580=CARTESIAN_POINT('Ctrl Pts',(-19.2437694434536,48.9786446680046,122.217145600225)) ;
#25581=CARTESIAN_POINT('Ctrl Pts',(-19.2023805082056,48.7986555876417,121.918479266341)) ;
#25582=CARTESIAN_POINT('Ctrl Pts',(-19.4541758562915,48.988665570151,122.206684633886)) ;
#25583=CARTESIAN_POINT('Ctrl Pts',(-19.4653884139487,48.8086764897881,121.905400360003)) ;
#25584=CARTESIAN_POINT('Ctrl Pts',(-19.6605286713295,48.9985563401998,122.232339508242)) ;
#25585=CARTESIAN_POINT('Ctrl Pts',(-19.7233301714243,48.818567259837,121.937466358609)) ;
#25586=CARTESIAN_POINT('Ctrl Pts',(-19.8613941607014,49.0085477509796,122.29375208743)) ;
#25587=CARTESIAN_POINT('Ctrl Pts',(-19.9744129235702,48.8285586706167,122.014229612701)) ;
#25588=CARTESIAN_POINT('Ctrl Pts',(-20.0477097453618,49.0184960966441,122.388760410401)) ;
#25589=CARTESIAN_POINT('Ctrl Pts',(-20.2073088426993,48.8385070162812,122.13298779378)) ;
#25590=CARTESIAN_POINT('Ctrl Pts',(-20.2149235430791,49.0284409547052,122.514293134598)) ;
#25591=CARTESIAN_POINT('Ctrl Pts',(-20.4163278633967,48.8484518743424,122.289901832939)) ;
#25592=CARTESIAN_POINT('Ctrl Pts',(-20.3591274679965,49.0384957900982,122.668825290875)) ;
#25593=CARTESIAN_POINT('Ctrl Pts',(-20.5965846062851,48.8585067097353,122.483065165235)) ;
#25594=CARTESIAN_POINT('Ctrl Pts',(-20.4719672533018,49.0483181621996,122.841786669687)) ;
#25595=CARTESIAN_POINT('Ctrl Pts',(-20.7376368968491,48.8683290818368,122.699266149593)) ;
#25596=CARTESIAN_POINT('Ctrl Pts',(-20.5553257636715,49.0583740296434,123.036047834246)) ;
#25597=CARTESIAN_POINT('Ctrl Pts',(-20.8418372689003,48.8783849492805,122.942091527948)) ;
#25598=CARTESIAN_POINT('Ctrl Pts',(-20.6027766814193,49.0683147595013,123.239583217983)) ;
#25599=CARTESIAN_POINT('Ctrl Pts',(-20.9011534756052,48.8883256791384,123.196510502706)) ;
#25600=CARTESIAN_POINT('Ctrl Pts',(-20.6147759350692,49.0782190980524,123.447461236143)) ;
#25601=CARTESIAN_POINT('Ctrl Pts',(-20.9161549876618,48.8982300176895,123.456358415646)) ;
#25602=CARTESIAN_POINT('Ctrl Pts',(-20.5900184388483,49.0882657794809,123.657200174385)) ;
#25603=CARTESIAN_POINT('Ctrl Pts',(-20.8852105592629,48.908276699118,123.718532273713)) ;
#25604=CARTESIAN_POINT('Ctrl Pts',(-20.5303023151086,49.0981612869501,123.856515276786)) ;
#25605=CARTESIAN_POINT('Ctrl Pts',(-20.810567540589,48.9181722065873,123.967677397249)) ;
#25606=CARTESIAN_POINT('Ctrl Pts',(-20.4353377015861,49.1082235554488,124.045507278438)) ;
#25607=CARTESIAN_POINT('Ctrl Pts',(-20.6918640066937,48.9282344750859,124.203918318717)) ;
#25608=CARTESIAN_POINT('Ctrl Pts',(-20.3118353609742,49.1180655457194,124.211547456422)) ;
#25609=CARTESIAN_POINT('Ctrl Pts',(-20.5374874732684,48.9380764653565,124.4114706526)) ;
#25610=CARTESIAN_POINT('Ctrl Pts',(-20.1594306056428,49.1280589626003,124.356110189049)) ;
#25611=CARTESIAN_POINT('Ctrl Pts',(-20.346982966348,48.9480698822375,124.59217583248)) ;
#25612=CARTESIAN_POINT('Ctrl Pts',(-19.9854133922224,49.1379834504525,124.471260343078)) ;
#25613=CARTESIAN_POINT('Ctrl Pts',(-20.1294622771985,48.9579943700896,124.736115686117)) ;
#25614=CARTESIAN_POINT('Ctrl Pts',(-19.7927208813877,49.147983084361,124.555263507083)) ;
#25615=CARTESIAN_POINT('Ctrl Pts',(-19.8885974147487,48.9679940039981,124.841121711921)) ;
#25616=CARTESIAN_POINT('Ctrl Pts',(-19.5886002486788,49.1579691946177,124.604484612063)) ;
#25617=CARTESIAN_POINT('Ctrl Pts',(-19.6334469697658,48.9779801142549,124.9026502756)) ;
#25618=CARTESIAN_POINT('Ctrl Pts',(-19.3780258214189,49.1680051458049,124.617357030462)) ;
#25619=CARTESIAN_POINT('Ctrl Pts',(-19.3702291570135,48.988016065442,124.918743054803)) ;
#25620=CARTESIAN_POINT('Ctrl Pts',(-19.1720854488287,49.1778617841397,124.594203709604)) ;
#25621=CARTESIAN_POINT('Ctrl Pts',(-19.1128025382839,48.9978727037768,124.889803469788)) ;
#25622=CARTESIAN_POINT('Ctrl Pts',(-18.9703969120688,49.1878607442177,124.535088681931)) ;
#25623=CARTESIAN_POINT('Ctrl Pts',(-18.8606911455665,49.0078716638548,124.815911669425)) ;
#25624=CARTESIAN_POINT('Ctrl Pts',(-18.7838271969103,49.1977559745315,124.442990126703)) ;
#25625=CARTESIAN_POINT('Ctrl Pts',(-18.6274774420179,49.0177668941686,124.700789980476)) ;
#25626=CARTESIAN_POINT('Ctrl Pts',(-18.6133446048038,49.2078164870001,124.317858094273)) ;
#25627=CARTESIAN_POINT('Ctrl Pts',(-18.4143731818113,49.0278274066372,124.544376734575)) ;
#25628=CARTESIAN_POINT('Ctrl Pts',(-18.470133520923,49.2176657785463,124.168284568055)) ;
#25629=CARTESIAN_POINT('Ctrl Pts',(-18.2353571530203,49.0376766981834,124.357410469631)) ;
#25630=CARTESIAN_POINT('Ctrl Pts',(-18.3525585485733,49.2276929644785,123.993322107595)) ;
#25631=CARTESIAN_POINT('Ctrl Pts',(-18.0883869155088,49.0477038841156,124.13870846236)) ;
#25632=CARTESIAN_POINT('Ctrl Pts',(-18.2676375468135,49.2377215009378,123.800338049473)) ;
#25633=CARTESIAN_POINT('Ctrl Pts',(-17.9822338382996,49.0577324205749,123.89747926818)) ;
#25634=CARTESIAN_POINT('Ctrl Pts',(-18.2180547672955,49.2475667409028,123.599398819481)) ;
#25635=CARTESIAN_POINT('Ctrl Pts',(-17.9202532459207,49.0675776605399,123.646304603655)) ;
#25636=CARTESIAN_POINT('Ctrl Pts',(-18.2033462478986,49.257557435826,123.389873464327)) ;
#25637=CARTESIAN_POINT('Ctrl Pts',(-17.9018658552473,49.0775683554631,123.384397836007)) ;
#25638=CARTESIAN_POINT('Ctrl Pts',(-18.2258094823577,49.2675952565846,123.180046491113)) ;
#25639=CARTESIAN_POINT('Ctrl Pts',(-17.9299430170255,49.0876061762217,123.122114050778)) ;
#25640=CARTESIAN_POINT('Ctrl Pts',(-18.282899951332,49.2774398503615,122.981108060184)) ;
#25641=CARTESIAN_POINT('Ctrl Pts',(-18.0013047262961,49.0974507699987,122.873439403411)) ;
#25642=CARTESIAN_POINT('Ctrl Pts',(-18.3745381888825,49.2874238457376,122.792294663389)) ;
#25643=CARTESIAN_POINT('Ctrl Pts',(-18.1158511804771,49.1074347653747,122.637421711162)) ;
#25644=CARTESIAN_POINT('Ctrl Pts',(-18.4971732872616,49.297372894299,122.622845943854)) ;
#25645=CARTESIAN_POINT('Ctrl Pts',(-18.2691440175312,49.1173838139361,122.425609469171)) ;
#25646=CARTESIAN_POINT('Ctrl Pts',(-18.6480139790816,49.3073753332735,122.476322024514)) ;
#25647=CARTESIAN_POINT('Ctrl Pts',(-18.4576938725769,49.1273862529106,122.242453382412)) ;
#25648=CARTESIAN_POINT('Ctrl Pts',(-18.8224872342568,49.3173965745699,122.358233047741)) ;
#25649=CARTESIAN_POINT('Ctrl Pts',(-18.6757844901155,49.137407494207,122.094840814009)) ;
#25650=CARTESIAN_POINT('Ctrl Pts',(-19.0122435632454,49.3272892530094,122.273107300004)) ;
#25651=CARTESIAN_POINT('Ctrl Pts',(-18.912980073684,49.1473001726465,121.988431832938)) ;
#25652=CARTESIAN_POINT('Ctrl Pts',(-19.2157981994734,49.337279306957,122.221395750134)) ;
#25653=CARTESIAN_POINT('Ctrl Pts',(-19.1674232251513,49.1572902265941,121.923790931797)) ;
#25654=CARTESIAN_POINT('Ctrl Pts',(-19.4245809336143,49.3472376681055,122.206012139912)) ;
#25655=CARTESIAN_POINT('Ctrl Pts',(-19.4284019621495,49.1672485877426,121.904559887262)) ;
#25656=CARTESIAN_POINT('Ctrl Pts',(-19.6317061321161,49.3571372949903,122.226481358477)) ;
#25657=CARTESIAN_POINT('Ctrl Pts',(-19.6873094646854,49.1771482146274,121.930145178779)) ;
#25658=CARTESIAN_POINT('Ctrl Pts',(-19.8350793181158,49.3671851917937,122.283506518214)) ;
#25659=CARTESIAN_POINT('Ctrl Pts',(-19.941526102593,49.1871961114308,122.001425268329)) ;
#25660=CARTESIAN_POINT('Ctrl Pts',(-20.0226907344885,49.3770805494297,122.373464971147)) ;
#25661=CARTESIAN_POINT('Ctrl Pts',(-20.1760417540059,49.1970914690668,122.113872563223)) ;
#25662=CARTESIAN_POINT('Ctrl Pts',(-20.1946471925884,49.3871422018863,122.496611414451)) ;
#25663=CARTESIAN_POINT('Ctrl Pts',(-20.3909878097268,49.2071531215235,122.267804384145)) ;
#25664=CARTESIAN_POINT('Ctrl Pts',(-20.3394609229976,49.3969868061583,122.644483147191)) ;
#25665=CARTESIAN_POINT('Ctrl Pts',(-20.5720068053571,49.2169977257954,122.452644101985)) ;
#25666=CARTESIAN_POINT('Ctrl Pts',(-20.4583844624104,49.4069469278563,122.816823206098)) ;
#25667=CARTESIAN_POINT('Ctrl Pts',(-20.7206623097227,49.2269578474934,122.668068984939)) ;
#25668=CARTESIAN_POINT('Ctrl Pts',(-20.5458863827844,49.4169849622188,123.008849967238)) ;
#25669=CARTESIAN_POINT('Ctrl Pts',(-20.8300406886576,49.2369958818559,122.90810181371)) ;
#25670=CARTESIAN_POINT('Ctrl Pts',(-20.5982321140661,49.4268592748053,123.209757190274)) ;
#25671=CARTESIAN_POINT('Ctrl Pts',(-20.895474107219,49.2468701944424,123.15923667191)) ;
#25672=CARTESIAN_POINT('Ctrl Pts',(-20.6152137828225,49.436928755588,123.420738615319)) ;
#25673=CARTESIAN_POINT('Ctrl Pts',(-20.9167021696326,49.2569396752251,123.422962968094)) ;
#25674=CARTESIAN_POINT('Ctrl Pts',(-20.5958761668654,49.4467630916051,123.62659808383)) ;
#25675=CARTESIAN_POINT('Ctrl Pts',(-20.8925309748415,49.2667740112422,123.680288852952)) ;
#25676=CARTESIAN_POINT('Ctrl Pts',(-20.540545363407,49.4567960493333,123.83012921168)) ;
#25677=CARTESIAN_POINT('Ctrl Pts',(-20.8233682239885,49.2768069689704,123.934702843844)) ;
#25678=CARTESIAN_POINT('Ctrl Pts',(-20.4502978778667,49.4668164479085,124.020482337261)) ;
#25679=CARTESIAN_POINT('Ctrl Pts',(-20.7105597644519,49.2868273675456,124.172644633411)) ;
#25680=CARTESIAN_POINT('Ctrl Pts',(-20.3306741561224,49.4766820216797,124.189933002317)) ;
#25681=CARTESIAN_POINT('Ctrl Pts',(-20.5610300420917,49.2966929413168,124.38445939655)) ;
#25682=CARTESIAN_POINT('Ctrl Pts',(-20.1804401966572,49.4867508963358,124.339026315722)) ;
#25683=CARTESIAN_POINT('Ctrl Pts',(-20.3732384290242,49.3067618159729,124.570826297004)) ;
#25684=CARTESIAN_POINT('Ctrl Pts',(-20.0104505357021,49.4965963272413,124.45713399561)) ;
#25685=CARTESIAN_POINT('Ctrl Pts',(-20.1607506292362,49.3166072468784,124.718462326025)) ;
#25686=CARTESIAN_POINT('Ctrl Pts',(-19.8202741615974,49.506575952112,124.545721379773)) ;
#25687=CARTESIAN_POINT('Ctrl Pts',(-19.9230300882037,49.3265868717491,124.829197136237)) ;
#25688=CARTESIAN_POINT('Ctrl Pts',(-19.6167083846425,49.5165946350261,124.599768391812)) ;
#25689=CARTESIAN_POINT('Ctrl Pts',(-19.6685730451368,49.3366055546632,124.896756529863)) ;
#25690=CARTESIAN_POINT('Ctrl Pts',(-19.4096938931667,49.5264779002099,124.617848281754)) ;
#25691=CARTESIAN_POINT('Ctrl Pts',(-19.4098038796016,49.346488819847,124.919356964503)) ;
#25692=CARTESIAN_POINT('Ctrl Pts',(-19.198877107358,49.5365461943013,124.599282994167)) ;
#25693=CARTESIAN_POINT('Ctrl Pts',(-19.1462832607712,49.3565571139384,124.89615090551)) ;
#25694=CARTESIAN_POINT('Ctrl Pts',(-18.9991919639653,49.5463763244866,124.54591031217)) ;
#25695=CARTESIAN_POINT('Ctrl Pts',(-18.8966752356581,49.3663872441237,124.829435060277)) ;
#25696=CARTESIAN_POINT('Ctrl Pts',(-18.8072474578189,49.5564428727018,124.456856220617)) ;
#25697=CARTESIAN_POINT('Ctrl Pts',(-18.656744831752,49.3764537923389,124.718117896912)) ;
#25698=CARTESIAN_POINT('Ctrl Pts',(-18.6367469946914,49.5663331213904,124.337807634366)) ;
#25699=CARTESIAN_POINT('Ctrl Pts',(-18.4436181844938,49.3863440410275,124.569306863408)) ;
#25700=CARTESIAN_POINT('Ctrl Pts',(-18.4876920453678,49.5763253031664,124.189801919102)) ;
#25701=CARTESIAN_POINT('Ctrl Pts',(-18.2572992166369,49.3963362228035,124.384299698902)) ;
#25702=CARTESIAN_POINT('Ctrl Pts',(-18.3671123398386,49.5862880837942,124.018548544852)) ;
#25703=CARTESIAN_POINT('Ctrl Pts',(-18.1065741069592,49.4062990034313,124.170232758712)) ;
#25704=CARTESIAN_POINT('Ctrl Pts',(-18.2781412601889,49.5961924884679,123.830276313694)) ;
#25705=CARTESIAN_POINT('Ctrl Pts',(-17.9953598077173,49.4162034081051,123.934891647468)) ;
#25706=CARTESIAN_POINT('Ctrl Pts',(-18.222510202651,49.606252482947,123.626250710745)) ;
#25707=CARTESIAN_POINT('Ctrl Pts',(-17.9258209627765,49.4262634025841,123.679859999836)) ;
#25708=CARTESIAN_POINT('Ctrl Pts',(-18.203376410996,49.6161011049168,123.420072742586)) ;
#25709=CARTESIAN_POINT('Ctrl Pts',(-17.9019035489539,49.4361120245539,123.422136143483)) ;
#25710=CARTESIAN_POINT('Ctrl Pts',(-18.2201708403545,49.6261315443286,123.209883238116)) ;
#25711=CARTESIAN_POINT('Ctrl Pts',(-17.9228967151139,49.4461424639657,123.159399391363)) ;
#25712=CARTESIAN_POINT('Ctrl Pts',(-18.2735161472999,49.6361412599634,123.00629722832)) ;
#25713=CARTESIAN_POINT('Ctrl Pts',(-17.9895783325629,49.4561521796005,122.90491683128)) ;
#25714=CARTESIAN_POINT('Ctrl Pts',(-18.3603293584098,49.646052012656,122.816911028997)) ;
#25715=CARTESIAN_POINT('Ctrl Pts',(-18.0980952655541,49.4660629322931,122.668183285469)) ;
#25716=CARTESIAN_POINT('Ctrl Pts',(-18.4785136980993,49.6559812856024,122.644833121426)) ;
#25717=CARTESIAN_POINT('Ctrl Pts',(-18.245826326081,49.4759922052395,122.453085432562)) ;
#25718=CARTESIAN_POINT('Ctrl Pts',(-18.6265668723548,49.666023976995,122.494326841967)) ;
#25719=CARTESIAN_POINT('Ctrl Pts',(-18.4308927790873,49.4860348966322,122.264952869192)) ;
#25720=CARTESIAN_POINT('Ctrl Pts',(-18.7957677209067,49.6759105102126,122.373596637961)) ;
#25721=CARTESIAN_POINT('Ctrl Pts',(-18.6423948660931,49.4959214298497,122.114039679069)) ;
#25722=CARTESIAN_POINT('Ctrl Pts',(-18.985209711551,49.6859036551446,122.282802300609)) ;
#25723=CARTESIAN_POINT('Ctrl Pts',(-18.8791977037883,49.5059145747817,122.000547015104)) ;
#25724=CARTESIAN_POINT('Ctrl Pts',(-19.1866107318813,49.6958493359811,122.226622842635)) ;
#25725=CARTESIAN_POINT('Ctrl Pts',(-19.1309496466814,49.5158602556182,121.930322869947)) ;
#25726=CARTESIAN_POINT('Ctrl Pts',(-19.3947080629283,49.7057965931296,122.205836498686)) ;
#25727=CARTESIAN_POINT('Ctrl Pts',(-19.3910719340289,49.5258075127667,121.904340399635)) ;
#25728=CARTESIAN_POINT('Ctrl Pts',(-19.6053289184389,49.7158444970016,122.221892340969)) ;
#25729=CARTESIAN_POINT('Ctrl Pts',(-19.6543477211243,49.5358554166387,121.924410607122)) ;
#25730=CARTESIAN_POINT('Ctrl Pts',(-19.8059348665026,49.7256921960996,122.273064256038)) ;
#25731=CARTESIAN_POINT('Ctrl Pts',(-19.9051063909627,49.5457031157367,121.988376325681)) ;
#25732=CARTESIAN_POINT('Ctrl Pts',(-19.9970522744167,49.7356536870782,122.358669039494)) ;
#25733=CARTESIAN_POINT('Ctrl Pts',(-20.1440032593785,49.5556646067154,122.095383178499)) ;
#25734=CARTESIAN_POINT('Ctrl Pts',(-20.1714411232963,49.7456831494922,122.477202699067)) ;
#25735=CARTESIAN_POINT('Ctrl Pts',(-20.3619888762732,49.5656940691293,122.243550726972)) ;
#25736=CARTESIAN_POINT('Ctrl Pts',(-20.3208300958534,49.7555903805921,122.622336917083)) ;
#25737=CARTESIAN_POINT('Ctrl Pts',(-20.5487252565727,49.5756013002292,122.424969613015)) ;
#25738=CARTESIAN_POINT('Ctrl Pts',(-20.4435688894129,49.7655367592695,122.791613197818)) ;
#25739=CARTESIAN_POINT('Ctrl Pts',(-20.7021484057419,49.5855476789066,122.636565942067)) ;
#25740=CARTESIAN_POINT('Ctrl Pts',(-20.5356692060204,49.7755415280784,122.980728511161)) ;
#25741=CARTESIAN_POINT('Ctrl Pts',(-20.817273052069,49.5955524477155,122.872960551607)) ;
#25742=CARTESIAN_POINT('Ctrl Pts',(-20.5933907296624,49.7855626490986,123.183338291841)) ;
#25743=CARTESIAN_POINT('Ctrl Pts',(-20.8894241945035,49.6055735687357,123.126222955828)) ;
#25744=CARTESIAN_POINT('Ctrl Pts',(-20.615012812427,49.7954535149512,123.390155066676)) ;
#25745=CARTESIAN_POINT('Ctrl Pts',(-20.9164510303163,49.6154644345883,123.384745011977)) ;
#25746=CARTESIAN_POINT('Ctrl Pts',(-20.6005593145487,49.8054443237105,123.599683369761)) ;
#25747=CARTESIAN_POINT('Ctrl Pts',(-20.8983831554368,49.6254552433476,123.64665553533)) ;
#25748=CARTESIAN_POINT('Ctrl Pts',(-20.5501038609146,49.8153949818908,123.802712023402)) ;
#25749=CARTESIAN_POINT('Ctrl Pts',(-20.8353127628865,49.6354059015279,123.900441641724)) ;
#25750=CARTESIAN_POINT('Ctrl Pts',(-20.4655527395291,49.8253311915329,123.993707680392)) ;
#25751=CARTESIAN_POINT('Ctrl Pts',(-20.7296226128942,49.64534211117,124.139186358957)) ;
#25752=CARTESIAN_POINT('Ctrl Pts',(-20.3487747189752,49.8353143582578,124.168128009877)) ;
#25753=CARTESIAN_POINT('Ctrl Pts',(-20.5836489640743,49.6553252778949,124.357211327668)) ;
#25754=CARTESIAN_POINT('Ctrl Pts',(-20.2023558449378,49.8453581554681,124.320235724213)) ;
#25755=CARTESIAN_POINT('Ctrl Pts',(-20.4006247563479,49.6653690751052,124.547345114736)) ;
#25756=CARTESIAN_POINT('Ctrl Pts',(-20.0356569177011,49.8551863716364,124.442367095108)) ;
#25757=CARTESIAN_POINT('Ctrl Pts',(-20.1922492122206,49.6751972912734,124.70000920038)) ;
#25758=CARTESIAN_POINT('Ctrl Pts',(-19.8457113842319,49.8652629391056,124.536063834955)) ;
#25759=CARTESIAN_POINT('Ctrl Pts',(-19.9548171286621,49.6852738587427,124.817128808093)) ;
#25760=CARTESIAN_POINT('Ctrl Pts',(-19.6468577220022,49.875115024795,124.594160167334)) ;
#25761=CARTESIAN_POINT('Ctrl Pts',(-19.706248503042,49.6951259444321,124.889748332412)) ;
#25762=CARTESIAN_POINT('Ctrl Pts',(-19.4364134670954,49.8851882922004,124.617525881756)) ;
#25763=CARTESIAN_POINT('Ctrl Pts',(-19.4431934347657,49.7051992118375,124.918954084388)) ;
#25764=CARTESIAN_POINT('Ctrl Pts',(-19.2299283765432,49.895029708624,124.604248514442)) ;
#25765=CARTESIAN_POINT('Ctrl Pts',(-19.1850858539182,49.7150406282611,124.902355961624)) ;
#25766=CARTESIAN_POINT('Ctrl Pts',(-19.0262747705676,49.9049909667667,124.55549141664)) ;
#25767=CARTESIAN_POINT('Ctrl Pts',(-18.93051882681,49.7250018864038,124.841407931651)) ;
#25768=CARTESIAN_POINT('Ctrl Pts',(-18.8328848698317,49.9150276431986,124.471106946337)) ;
#25769=CARTESIAN_POINT('Ctrl Pts',(-18.6887821551517,49.7350385628358,124.735926054212)) ;
#25770=CARTESIAN_POINT('Ctrl Pts',(-18.6596380225063,49.9249062510625,124.35654118208)) ;
#25771=CARTESIAN_POINT('Ctrl Pts',(-18.472223638631,49.7449171706996,124.592716974689)) ;
#25772=CARTESIAN_POINT('Ctrl Pts',(-18.5061473019625,49.9349664797013,124.211075267504)) ;
#25773=CARTESIAN_POINT('Ctrl Pts',(-18.2803615486336,49.7549773993384,124.410883615209)) ;
#25774=CARTESIAN_POINT('Ctrl Pts',(-18.3825837811286,49.9448334638621,124.044425289918)) ;
#25775=CARTESIAN_POINT('Ctrl Pts',(-18.1259078276829,49.7648443834992,124.2025693445)) ;
#25776=CARTESIAN_POINT('Ctrl Pts',(-18.2881916231086,49.9548390301148,123.856476139896)) ;
#25777=CARTESIAN_POINT('Ctrl Pts',(-18.007919160607,49.7748499497519,123.967632043592)) ;
#25778=CARTESIAN_POINT('Ctrl Pts',(-18.2280312076151,49.9648228185294,123.655353475487)) ;
#25779=CARTESIAN_POINT('Ctrl Pts',(-17.9327202356782,49.7848337381665,123.716228002346)) ;
#25780=CARTESIAN_POINT('Ctrl Pts',(-18.2037899064989,49.974868675332,123.445570734123)) ;
#25781=CARTESIAN_POINT('Ctrl Pts',(-17.9024202751919,49.7948795949691,123.453999545748)) ;
#25782=CARTESIAN_POINT('Ctrl Pts',(-18.2157993043397,49.984694552548,123.239349234005)) ;
#25783=CARTESIAN_POINT('Ctrl Pts',(-17.9174338428605,49.8047054721851,123.196221483282)) ;
#25784=CARTESIAN_POINT('Ctrl Pts',(-18.2635625382729,49.9946850283893,123.034820965476)) ;
#25785=CARTESIAN_POINT('Ctrl Pts',(-17.9771398351836,49.8146959480264,122.940561425494)) ;
#25786=CARTESIAN_POINT('Ctrl Pts',(-18.3470621028792,50.0047286042881,122.840884623417)) ;
#25787=CARTESIAN_POINT('Ctrl Pts',(-18.0815158765867,49.8247395239252,122.698141841169)) ;
#25788=CARTESIAN_POINT('Ctrl Pts',(-18.4600443984035,50.0145503965861,122.668054220945)) ;
#25789=CARTESIAN_POINT('Ctrl Pts',(-18.2227460406671,49.8345613162232,122.482103844544)) ;
#25790=CARTESIAN_POINT('Ctrl Pts',(-18.604009794299,50.024585362212,122.513843576675)) ;
#25791=CARTESIAN_POINT('Ctrl Pts',(-18.4027042307795,49.8445962818491,122.289342033901)) ;
#25792=CARTESIAN_POINT('Ctrl Pts',(-18.7727524722638,50.034610279145,122.387565767662)) ;
#25793=CARTESIAN_POINT('Ctrl Pts',(-18.6136336981396,49.8546211987822,122.131496311253)) ;
#25794=CARTESIAN_POINT('Ctrl Pts',(-18.957405994649,50.0444622175212,122.293741975346)) ;
#25795=CARTESIAN_POINT('Ctrl Pts',(-18.844452425863,49.8644731371583,122.014217927815)) ;
#25796=CARTESIAN_POINT('Ctrl Pts',(-19.1582192780616,50.0544531935459,122.23225581094)) ;
#25797=CARTESIAN_POINT('Ctrl Pts',(-19.0954698169911,49.8744641131831,121.937362207403)) ;
#25798=CARTESIAN_POINT('Ctrl Pts',(-19.3651677350279,50.0643710143496,122.206614010036)) ;
#25799=CARTESIAN_POINT('Ctrl Pts',(-19.3541562238253,49.8843819339867,121.905312031361)) ;
#25800=CARTESIAN_POINT('Ctrl Pts',(-19.5757056924692,50.0743997349142,122.217377366657)) ;
#25801=CARTESIAN_POINT('Ctrl Pts',(-19.6173285205986,49.8944106545513,121.918768394832)) ;
#25802=CARTESIAN_POINT('Ctrl Pts',(-19.7782617157918,50.0842826615234,122.263718063625)) ;
#25803=CARTESIAN_POINT('Ctrl Pts',(-19.8705237928236,49.9042935811605,121.976696588945)) ;
#25804=CARTESIAN_POINT('Ctrl Pts',(-19.9721356284537,50.0942869466428,122.345192272109)) ;
#25805=CARTESIAN_POINT('Ctrl Pts',(-20.1128653758692,49.91429786628,122.078541501099)) ;
#25806=CARTESIAN_POINT('Ctrl Pts',(-20.1485909447356,50.1042706278507,122.458909425641)) ;
#25807=CARTESIAN_POINT('Ctrl Pts',(-20.3334334359267,49.9242815474878,122.22068996082)) ;
#25808=CARTESIAN_POINT('Ctrl Pts',(-20.3033028222086,50.1143116265806,122.602499485329)) ;
#25809=CARTESIAN_POINT('Ctrl Pts',(-20.5268216963565,49.9343225462177,122.400179102875)) ;
#25810=CARTESIAN_POINT('Ctrl Pts',(-20.4283285557546,50.1241440714477,122.767114268604)) ;
#25811=CARTESIAN_POINT('Ctrl Pts',(-20.683102613612,49.9441549910849,122.605949735523)) ;
#25812=CARTESIAN_POINT('Ctrl Pts',(-20.5249823851883,50.1341390698781,122.95368511086)) ;
#25813=CARTESIAN_POINT('Ctrl Pts',(-20.8039177883312,49.9541499895152,122.839164524174)) ;
#25814=CARTESIAN_POINT('Ctrl Pts',(-20.5875768112403,50.1441706186277,123.155088324659)) ;
#25815=CARTESIAN_POINT('Ctrl Pts',(-20.8821585762413,49.9641815382648,123.090919199762)) ;
#25816=CARTESIAN_POINT('Ctrl Pts',(-20.6140645488152,50.1540359969332,123.360779768465)) ;
#25817=CARTESIAN_POINT('Ctrl Pts',(-20.9152659613685,49.9740469165703,123.348034537658)) ;
#25818=CARTESIAN_POINT('Ctrl Pts',(-20.6049313505838,50.1639978443934,123.570016308224)) ;
#25819=CARTESIAN_POINT('Ctrl Pts',(-20.9038469302478,49.9840087640306,123.609580354995)) ;
#25820=CARTESIAN_POINT('Ctrl Pts',(-20.5589419047173,50.1740327852077,123.775896953256)) ;
#25821=CARTESIAN_POINT('Ctrl Pts',(-20.8463577366402,49.9940437048448,123.8669305923)) ;
#25822=CARTESIAN_POINT('Ctrl Pts',(-20.4794221936391,50.1839177462248,123.967925666986)) ;
#25823=CARTESIAN_POINT('Ctrl Pts',(-20.7469555508652,50.003928665862,124.106966043971)) ;
#25824=CARTESIAN_POINT('Ctrl Pts',(-20.3657227466916,50.1939833551437,124.146355086132)) ;
#25825=CARTESIAN_POINT('Ctrl Pts',(-20.6048292012254,50.0139942747808,124.330001338928)) ;
#25826=CARTESIAN_POINT('Ctrl Pts',(-20.2260937776423,50.2038225301854,124.299012275186)) ;
#25827=CARTESIAN_POINT('Ctrl Pts',(-20.4302906277304,50.0238334498225,124.520821628096)) ;
#25828=CARTESIAN_POINT('Ctrl Pts',(-20.0585794048684,50.2138850856853,124.428165424389)) ;
#25829=CARTESIAN_POINT('Ctrl Pts',(-20.2208961768224,50.0338960053224,124.682260919657)) ;
#25830=CARTESIAN_POINT('Ctrl Pts',(-19.8741279084005,50.2237822603782,124.524475108692)) ;
#25831=CARTESIAN_POINT('Ctrl Pts',(-19.990330202873,50.0437931800154,124.802645968509)) ;
#25832=CARTESIAN_POINT('Ctrl Pts',(-19.675310997847,50.2337129753016,124.588171794171)) ;
#25833=CARTESIAN_POINT('Ctrl Pts',(-19.7418079589796,50.0537238949387,124.882264366511)) ;
#25834=CARTESIAN_POINT('Ctrl Pts',(-19.4660617887297,50.2437570033792,124.616460712568)) ;
#25835=CARTESIAN_POINT('Ctrl Pts',(-19.4802461248259,50.0637679230163,124.91762289268)) ;
#25836=CARTESIAN_POINT('Ctrl Pts',(-19.2583695225843,50.2536432052325,124.608282274617)) ;
#25837=CARTESIAN_POINT('Ctrl Pts',(-19.2206304688887,50.0736541248696,124.907397165842)) ;
#25838=CARTESIAN_POINT('Ctrl Pts',(-19.0530229072309,50.2636363716993,124.564006896081)) ;
#25839=CARTESIAN_POINT('Ctrl Pts',(-18.9639476699514,50.0836472913365,124.852050273482)) ;
#25840=CARTESIAN_POINT('Ctrl Pts',(-18.8594602487142,50.2735758426865,124.485214042851)) ;
#25841=CARTESIAN_POINT('Ctrl Pts',(-18.7219951492464,50.0935867623236,124.753556604735)) ;
#25842=CARTESIAN_POINT('Ctrl Pts',(-18.6811659538875,50.2835923570407,124.373207861046)) ;
#25843=CARTESIAN_POINT('Ctrl Pts',(-18.4991286839628,50.1036032766778,124.613546547454)) ;
#25844=CARTESIAN_POINT('Ctrl Pts',(-18.5262199735624,50.2935223835175,124.233262173088)) ;
#25845=CARTESIAN_POINT('Ctrl Pts',(-18.305447857855,50.1135333031546,124.438612238836)) ;
#25846=CARTESIAN_POINT('Ctrl Pts',(-18.3964464306137,50.303574919027,124.066486390739)) ;
#25847=CARTESIAN_POINT('Ctrl Pts',(-18.1432330982203,50.1235858386641,124.23014085339)) ;
#25848=CARTESIAN_POINT('Ctrl Pts',(-18.2995125290276,50.3134213222466,123.883574583666)) ;
#25849=CARTESIAN_POINT('Ctrl Pts',(-18.0220679537995,50.1334322418838,124.001499451881)) ;
#25850=CARTESIAN_POINT('Ctrl Pts',(-18.2344247285052,50.3233833651007,123.684524259499)) ;
#25851=CARTESIAN_POINT('Ctrl Pts',(-17.9407108291128,50.1433942847378,123.752685556883)) ;
#25852=CARTESIAN_POINT('Ctrl Pts',(-18.204957703029,50.3334119158914,123.475747879046)) ;
#25853=CARTESIAN_POINT('Ctrl Pts',(-17.903879790198,50.1534228355285,123.491714650898)) ;
#25854=CARTESIAN_POINT('Ctrl Pts',(-18.2120324651509,50.343322241609,123.267531291762)) ;
#25855=CARTESIAN_POINT('Ctrl Pts',(-17.9127260347505,50.1633331612461,123.23144379837)) ;
#25856=CARTESIAN_POINT('Ctrl Pts',(-18.2547290771079,50.3532571534386,123.063072199955)) ;
#25857=CARTESIAN_POINT('Ctrl Pts',(-17.9660995838745,50.1732680730757,122.975870378448)) ;
#25858=CARTESIAN_POINT('Ctrl Pts',(-18.3332815125372,50.3632981602067,122.867144842082)) ;
#25859=CARTESIAN_POINT('Ctrl Pts',(-18.0642927488552,50.1833090798438,122.730962183356)) ;
#25860=CARTESIAN_POINT('Ctrl Pts',(-18.4428498626735,50.3731857930389,122.69048500063)) ;
#25861=CARTESIAN_POINT('Ctrl Pts',(-18.201255664043,50.193196712676,122.510138724716)) ;
#25862=CARTESIAN_POINT('Ctrl Pts',(-18.5825766741435,50.3831762241369,122.533689688026)) ;
#25863=CARTESIAN_POINT('Ctrl Pts',(-18.3759163267486,50.203187143774,122.314146410369)) ;
#25864=CARTESIAN_POINT('Ctrl Pts',(-18.7469116188207,50.3931316606941,122.404071107336)) ;
#25865=CARTESIAN_POINT('Ctrl Pts',(-18.5813368510253,50.2131425803313,122.152125343484)) ;
#25866=CARTESIAN_POINT('Ctrl Pts',(-18.930235657484,50.4030426087935,122.305070551018)) ;
#25867=CARTESIAN_POINT('Ctrl Pts',(-18.8104932141694,50.2230535284306,122.028377092564)) ;
#25868=CARTESIAN_POINT('Ctrl Pts',(-19.1299354241263,50.4130546848912,122.238492971298)) ;
#25869=CARTESIAN_POINT('Ctrl Pts',(-19.0601191774314,50.2330656045283,121.945157820195)) ;
#25870=CARTESIAN_POINT('Ctrl Pts',(-19.3385035067007,50.4230820069661,122.207980233689)) ;
#25871=CARTESIAN_POINT('Ctrl Pts',(-19.3208286510922,50.2430929266033,121.907019503274)) ;
#25872=CARTESIAN_POINT('Ctrl Pts',(-19.5457289876827,50.4329407819203,122.213520699819)) ;
#25873=CARTESIAN_POINT('Ctrl Pts',(-19.5798646279409,50.2529517015574,121.913948569486)) ;
#25874=CARTESIAN_POINT('Ctrl Pts',(-19.822185156653,50.4463669747327,122.270169175991)) ;
#25875=CARTESIAN_POINT('Ctrl Pts',(-19.9254133373517,50.2663778943698,121.984759551957)) ;
#25876=CARTESIAN_POINT('Ctrl Pts',(-20.0713938613618,50.4594509905141,122.394125106127)) ;
#25877=CARTESIAN_POINT('Ctrl Pts',(-20.2369013110527,50.2794619101513,122.13968280904)) ;
#25878=CARTESIAN_POINT('Ctrl Pts',(-20.2838339244026,50.4729244392694,122.581328585295)) ;
#25879=CARTESIAN_POINT('Ctrl Pts',(-20.5024950621529,50.2929353589065,122.373723117195)) ;
#25880=CARTESIAN_POINT('Ctrl Pts',(-20.4126445774875,50.4827573970752,122.743055891855)) ;
#25881=CARTESIAN_POINT('Ctrl Pts',(-20.6634968410946,50.3027683167123,122.575877232274)) ;
#25882=CARTESIAN_POINT('Ctrl Pts',(-20.5134783735398,50.4927206705259,122.926629074294)) ;
#25883=CARTESIAN_POINT('Ctrl Pts',(-20.7895391335986,50.312731590163,122.805346777483)) ;
#25884=CARTESIAN_POINT('Ctrl Pts',(-20.5809791036652,50.5027577443438,123.126549900042)) ;
#25885=CARTESIAN_POINT('Ctrl Pts',(-20.8739118055342,50.322768663981,123.05524832364)) ;
#25886=CARTESIAN_POINT('Ctrl Pts',(-20.6126206713393,50.5126327473555,123.331753130747)) ;
#25887=CARTESIAN_POINT('Ctrl Pts',(-20.9134611751376,50.3326436669926,123.311752830501)) ;
#25888=CARTESIAN_POINT('Ctrl Pts',(-20.608057270493,50.5227004269817,123.543329168377)) ;
#25889=CARTESIAN_POINT('Ctrl Pts',(-20.9077542261225,50.3427113466188,123.576222416539)) ;
#25890=CARTESIAN_POINT('Ctrl Pts',(-20.5678626540345,50.5325412771994,123.746296518726)) ;
#25891=CARTESIAN_POINT('Ctrl Pts',(-20.857508009601,50.3525521968365,123.829932935511)) ;
#25892=CARTESIAN_POINT('Ctrl Pts',(-20.4670213376231,50.5458774756753,124.007888589382)) ;
#25893=CARTESIAN_POINT('Ctrl Pts',(-20.7314548291478,50.3658883953125,124.156910684336)) ;
#25894=CARTESIAN_POINT('Ctrl Pts',(-20.3015547858526,50.5590949994898,124.235123685654)) ;
#25895=CARTESIAN_POINT('Ctrl Pts',(-20.524653068368,50.3791059191269,124.440925618285)) ;
#25896=CARTESIAN_POINT('Ctrl Pts',(-20.0837840031638,50.572429925981,124.411566237074)) ;
#25897=CARTESIAN_POINT('Ctrl Pts',(-20.252395006723,50.3924408456182,124.66151880778)) ;
#25898=CARTESIAN_POINT('Ctrl Pts',(-19.9002502528585,50.5824130265756,124.513455062962)) ;
#25899=CARTESIAN_POINT('Ctrl Pts',(-20.0229851842833,50.4024239462128,124.788869046757)) ;
#25900=CARTESIAN_POINT('Ctrl Pts',(-19.7005468923068,50.5924578024753,124.582032085012)) ;
#25901=CARTESIAN_POINT('Ctrl Pts',(-19.7733522297728,50.4124687221124,124.874590001612)) ;
#25902=CARTESIAN_POINT('Ctrl Pts',(-19.4967087425705,50.6022757256612,124.614562625887)) ;
#25903=CARTESIAN_POINT('Ctrl Pts',(-19.5185568926512,50.4222866452983,124.915250650633)) ;
#25904=CARTESIAN_POINT('Ctrl Pts',(-19.2854718592234,50.6123250396165,124.611560869832)) ;
#25905=CARTESIAN_POINT('Ctrl Pts',(-19.2545052235582,50.4323359592536,124.911493375565)) ;
#25906=CARTESIAN_POINT('Ctrl Pts',(-19.0108573397302,50.6256287802391,124.558525690301)) ;
#25907=CARTESIAN_POINT('Ctrl Pts',(-18.9112636456039,50.4456396998762,124.845209773811)) ;
#25908=CARTESIAN_POINT('Ctrl Pts',(-18.6949673472923,50.6421189757157,124.406294928456)) ;
#25909=CARTESIAN_POINT('Ctrl Pts',(-18.5163636183236,50.4621298953529,124.654888417403)) ;
#25910=CARTESIAN_POINT('Ctrl Pts',(-18.4467378433555,50.6588381406404,124.151872297138)) ;
#25911=CARTESIAN_POINT('Ctrl Pts',(-18.2061311342259,50.4788490602775,124.336917792434)) ;
#25912=CARTESIAN_POINT('Ctrl Pts',(-18.311368251597,50.6719991343105,123.910554451692)) ;
#25913=CARTESIAN_POINT('Ctrl Pts',(-18.0368827272804,50.4920100539476,124.035219084609)) ;
#25914=CARTESIAN_POINT('Ctrl Pts',(-18.2412163964924,50.6819953564158,123.7124638999)) ;
#25915=CARTESIAN_POINT('Ctrl Pts',(-17.9492027072533,50.5020062760529,123.787616040863)) ;
#25916=CARTESIAN_POINT('Ctrl Pts',(-18.2069016120642,50.6920191959495,123.504545752087)) ;
#25917=CARTESIAN_POINT('Ctrl Pts',(-17.9063100733637,50.5120301155866,123.527712476807)) ;
#25918=CARTESIAN_POINT('Ctrl Pts',(-18.209328291179,50.7052125179428,123.227157565911)) ;
#25919=CARTESIAN_POINT('Ctrl Pts',(-17.9093431973629,50.5252234375799,123.180991999699)) ;
#25920=CARTESIAN_POINT('Ctrl Pts',(-18.3035425854847,50.7218716897201,122.88574552881)) ;
#25921=CARTESIAN_POINT('Ctrl Pts',(-18.027118283777,50.5418826093572,122.754212984447)) ;
#25922=CARTESIAN_POINT('Ctrl Pts',(-18.5489966287471,50.7417818652058,122.540800163354)) ;
#25923=CARTESIAN_POINT('Ctrl Pts',(-18.333937561739,50.5617927848429,122.323039035125)) ;
#25924=CARTESIAN_POINT('Ctrl Pts',(-18.8965967981805,50.7616718530502,122.299823800529)) ;
#25925=CARTESIAN_POINT('Ctrl Pts',(-18.7684393921744,50.5816827726873,122.021820822919)) ;
#25926=CARTESIAN_POINT('Ctrl Pts',(-19.3079195621711,50.781677301065,122.191706071761)) ;
#25927=CARTESIAN_POINT('Ctrl Pts',(-19.2825937715403,50.6016882207021,121.886677539595)) ;
#25928=CARTESIAN_POINT('Ctrl Pts',(-19.728095167199,50.8015136950923,122.229696970735)) ;
#25929=CARTESIAN_POINT('Ctrl Pts',(-19.8078113963263,50.6215246147294,121.934169205366)) ;
#25930=CARTESIAN_POINT('Ctrl Pts',(-20.1132481010553,50.821521488989,122.410089592141)) ;
#25931=CARTESIAN_POINT('Ctrl Pts',(-20.2892513212485,50.6415324086261,122.159662815759)) ;
#25932=CARTESIAN_POINT('Ctrl Pts',(-20.4112416238867,50.8413481252829,122.708392112376)) ;
#25933=CARTESIAN_POINT('Ctrl Pts',(-20.6617398847741,50.66135904492,122.532541564671)) ;
#25934=CARTESIAN_POINT('Ctrl Pts',(-20.5915810372585,50.8613270682368,123.093001610394)) ;
#25935=CARTESIAN_POINT('Ctrl Pts',(-20.8871620269531,50.6813379878739,123.013304098428)) ;
#25936=CARTESIAN_POINT('Ctrl Pts',(-20.6290028587678,50.8812588701058,123.51509334654)) ;
#25937=CARTESIAN_POINT('Ctrl Pts',(-20.9339369378857,50.701269789743,123.540918150504)) ;
#25938=CARTESIAN_POINT('Ctrl Pts',(-20.5220534572003,50.9010831706034,123.922954659986)) ;
#25939=CARTESIAN_POINT('Ctrl Pts',(-20.8002489892957,50.7210940902405,124.050742162796)) ;
#25940=CARTESIAN_POINT('Ctrl Pts',(-20.2786120446289,50.9211791719433,124.273908281155)) ;
#25941=CARTESIAN_POINT('Ctrl Pts',(-20.4959470937685,50.7411900915803,124.489434446394)) ;
#25942=CARTESIAN_POINT('Ctrl Pts',(-19.9357982920383,50.9409375880472,124.517186763173)) ;
#25943=CARTESIAN_POINT('Ctrl Pts',(-20.0674250455001,50.7609485076843,124.793529199864)) ;
#25944=CARTESIAN_POINT('Ctrl Pts',(-19.5241716085477,50.9610312809313,124.630773509642)) ;
#25945=CARTESIAN_POINT('Ctrl Pts',(-19.5529196248031,50.7810422005684,124.935512899744)) ;
#25946=CARTESIAN_POINT('Ctrl Pts',(-19.2461442415946,50.9741422468379,124.608669218602)) ;
#25947=CARTESIAN_POINT('Ctrl Pts',(-19.2053312341041,50.7941531664751,124.907880339345)) ;
#25948=CARTESIAN_POINT('Ctrl Pts',(-19.1099467513572,50.9808556216258,124.573813086965)) ;
#25949=CARTESIAN_POINT('Ctrl Pts',(-19.035117438896,50.8008665412629,124.864312062334)) ;
#25950=CARTESIAN_POINT('',(-18.3453504609641,12.1170521379794,124.06799281052)) ;
#25951=CARTESIAN_POINT('',(-18.1677493295881,12.0000000003486,124.153922006539)) ;
#25952=CARTESIAN_POINT('Ctrl Pts',(-18.3453506846598,12.1170517297128,124.067992703577)) ;
#25953=CARTESIAN_POINT('Ctrl Pts',(-18.3273547545627,12.1040527313448,124.079975178566)) ;
#25954=CARTESIAN_POINT('Ctrl Pts',(-18.3083333684475,12.0907998558922,124.09127094444)) ;
#25955=CARTESIAN_POINT('Ctrl Pts',(-18.2886731982766,12.0775160379758,124.101757360079)) ;
#25956=CARTESIAN_POINT('Ctrl Pts',(-18.2692156830702,12.0643691482562,124.112135682849)) ;
#25957=CARTESIAN_POINT('Ctrl Pts',(-18.2491324210418,12.0511919516622,124.121719977723)) ;
#25958=CARTESIAN_POINT('Ctrl Pts',(-18.2288350990488,12.0382005709879,124.130431431038)) ;
#25959=CARTESIAN_POINT('Ctrl Pts',(-18.2099998134723,12.0261449724652,124.138515389653)) ;
#25960=CARTESIAN_POINT('Ctrl Pts',(-18.1909807008646,12.0142493854672,124.145847642283)) ;
#25961=CARTESIAN_POINT('Ctrl Pts',(-18.1721346154261,12.0026865128952,124.152408160415)) ;
#25962=CARTESIAN_POINT('Ctrl Pts',(-18.1706717407006,12.0017889772188,124.152917402304)) ;
#25963=CARTESIAN_POINT('Ctrl Pts',(-18.1692099210947,12.0008934462135,124.153422017229)) ;
#25964=CARTESIAN_POINT('Ctrl Pts',(-18.1677493297433,12.0000000006492,124.15392200753)) ;
#25965=CARTESIAN_POINT('',(-20.4774766531755,11.9999999945496,124.060997935139)) ;
#25966=CARTESIAN_POINT('Ctrl Pts',(-18.1677493286892,12.0000000000044,124.153922007891)) ;
#25967=CARTESIAN_POINT('Ctrl Pts',(-18.1945949699472,12.0000000000052,124.192762375168)) ;
#25968=CARTESIAN_POINT('Ctrl Pts',(-18.2231913450481,12.,124.230077351763)) ;
#25969=CARTESIAN_POINT('Ctrl Pts',(-18.2533557201733,12.,124.265730705607)) ;
#25970=CARTESIAN_POINT('Ctrl Pts',(-18.3070716273031,12.,124.329221238262)) ;
#25971=CARTESIAN_POINT('Ctrl Pts',(-18.3658179607988,12.,124.387509039275)) ;
#25972=CARTESIAN_POINT('Ctrl Pts',(-18.4293591975901,12.,124.440302750152)) ;
#25973=CARTESIAN_POINT('Ctrl Pts',(-18.4721278246092,12.,124.475837383148)) ;
#25974=CARTESIAN_POINT('Ctrl Pts',(-18.5170404532172,11.9999999780286,124.508860536102)) ;
#25975=CARTESIAN_POINT('Ctrl Pts',(-18.5633173760341,11.9999999870879,124.538960478783)) ;
#25976=CARTESIAN_POINT('Ctrl Pts',(-18.5859252873497,11.9999999915136,124.553665363925)) ;
#25977=CARTESIAN_POINT('Ctrl Pts',(-18.6088594509681,12.,124.5676730489)) ;
#25978=CARTESIAN_POINT('Ctrl Pts',(-18.6320326861663,12.,124.580938074486)) ;
#25979=CARTESIAN_POINT('Ctrl Pts',(-18.6893271138161,12.,124.613735050922)) ;
#25980=CARTESIAN_POINT('Ctrl Pts',(-18.7481011236149,12.0000000184731,124.642002547875)) ;
#25981=CARTESIAN_POINT('Ctrl Pts',(-18.808591238206,12.0000000058446,124.665966773295)) ;
#25982=CARTESIAN_POINT('Ctrl Pts',(-18.8228268816011,12.0000000028726,124.67160647442)) ;
#25983=CARTESIAN_POINT('Ctrl Pts',(-18.8371573708013,12.,124.677007733495)) ;
#25984=CARTESIAN_POINT('Ctrl Pts',(-18.8515854105586,12.,124.682173315896)) ;
#25985=CARTESIAN_POINT('Ctrl Pts',(-18.9030665387764,12.,124.700604787836)) ;
#25986=CARTESIAN_POINT('Ctrl Pts',(-18.9557905285045,11.9999999840944,124.716036106706)) ;
#25987=CARTESIAN_POINT('Ctrl Pts',(-19.008882066701,11.9999999908829,124.72827599868)) ;
#25988=CARTESIAN_POINT('Ctrl Pts',(-19.0340552814171,11.9999999941016,124.734079511617)) ;
#25989=CARTESIAN_POINT('Ctrl Pts',(-19.0593118422177,12.,124.739165805691)) ;
#25990=CARTESIAN_POINT('Ctrl Pts',(-19.0845623342861,12.,124.74351576159)) ;
#25991=CARTESIAN_POINT('Ctrl Pts',(-19.1577583409821,12.,124.756125393127)) ;
#25992=CARTESIAN_POINT('Ctrl Pts',(-19.230888238426,12.0000000080437,124.762545609574)) ;
#25993=CARTESIAN_POINT('Ctrl Pts',(-19.3039949949029,12.000000000871,124.763034471808)) ;
#25994=CARTESIAN_POINT('Ctrl Pts',(-19.3094679922311,12.0000000003341,124.763071069543)) ;
#25995=CARTESIAN_POINT('Ctrl Pts',(-19.3149408364502,12.,124.763074419256)) ;
#25996=CARTESIAN_POINT('Ctrl Pts',(-19.3204135341477,12.,124.763044626916)) ;
#25997=CARTESIAN_POINT('Ctrl Pts',(-19.3794328487692,12.,124.762723336828)) ;
#25998=CARTESIAN_POINT('Ctrl Pts',(-19.4384497074752,11.9999999923458,124.758547342743)) ;
#25999=CARTESIAN_POINT('Ctrl Pts',(-19.4965921528861,11.9999999967179,124.750604967653)) ;
#26000=CARTESIAN_POINT('Ctrl Pts',(-19.5160203292204,11.9999999981788,124.747951039654)) ;
#26001=CARTESIAN_POINT('Ctrl Pts',(-19.5353513049696,12.,124.744876594293)) ;
#26002=CARTESIAN_POINT('Ctrl Pts',(-19.5545538432223,12.,124.741384949252)) ;
#26003=CARTESIAN_POINT('Ctrl Pts',(-19.6197198756548,12.,124.729535648341)) ;
#26004=CARTESIAN_POINT('Ctrl Pts',(-19.6833426730566,11.9999999984792,124.712894770648)) ;
#26005=CARTESIAN_POINT('Ctrl Pts',(-19.7447602360297,11.9999999996238,124.691979808156)) ;
#26006=CARTESIAN_POINT('Ctrl Pts',(-19.7558013132351,11.9999999998296,124.688219911077)) ;
#26007=CARTESIAN_POINT('Ctrl Pts',(-19.7667712412664,12.,124.684321819739)) ;
#26008=CARTESIAN_POINT('Ctrl Pts',(-19.7776663287723,12.,124.680288453161)) ;
#26009=CARTESIAN_POINT('Ctrl Pts',(-19.8493651138227,12.,124.653745528828)) ;
#26010=CARTESIAN_POINT('Ctrl Pts',(-19.9179051001858,12.,124.621313026741)) ;
#26011=CARTESIAN_POINT('Ctrl Pts',(-19.9832030943918,12.,124.583131212673)) ;
#26012=CARTESIAN_POINT('Ctrl Pts',(-20.0330168871335,12.,124.554003503689)) ;
#26013=CARTESIAN_POINT('Ctrl Pts',(-20.0809465543055,11.9999999945779,124.521528166539)) ;
#26014=CARTESIAN_POINT('Ctrl Pts',(-20.1262764357416,11.9999999978038,124.486203412323)) ;
#26015=CARTESIAN_POINT('Ctrl Pts',(-20.14045609981,11.9999999988129,124.475153457366)) ;
#26016=CARTESIAN_POINT('Ctrl Pts',(-20.1543817184891,12.,124.463824515856)) ;
#26017=CARTESIAN_POINT('Ctrl Pts',(-20.168032314776,12.,124.452231354919)) ;
#26018=CARTESIAN_POINT('Ctrl Pts',(-20.2125408174554,12.,124.414431230746)) ;
#26019=CARTESIAN_POINT('Ctrl Pts',(-20.2540726431959,11.9999999905181,124.373868567748)) ;
#26020=CARTESIAN_POINT('Ctrl Pts',(-20.2922988408341,11.9999999963922,124.331241807081)) ;
#26021=CARTESIAN_POINT('Ctrl Pts',(-20.3034097999745,11.9999999980996,124.318851765033)) ;
#26022=CARTESIAN_POINT('Ctrl Pts',(-20.3142416754177,12.,124.306287061013)) ;
#26023=CARTESIAN_POINT('Ctrl Pts',(-20.3247868528159,12.,124.293564166379)) ;
#26024=CARTESIAN_POINT('Ctrl Pts',(-20.3674983751124,12.,124.242032155362)) ;
#26025=CARTESIAN_POINT('Ctrl Pts',(-20.4055506162159,12.0000000087182,124.187851504183)) ;
#26026=CARTESIAN_POINT('Ctrl Pts',(-20.43911209806,12.0000000012434,124.130991328396)) ;
#26027=CARTESIAN_POINT('Ctrl Pts',(-20.4424600811825,12.0000000004977,124.125319144142)) ;
#26028=CARTESIAN_POINT('Ctrl Pts',(-20.4457633499417,12.,124.119620329616)) ;
#26029=CARTESIAN_POINT('Ctrl Pts',(-20.449022055999,12.,124.113894878083)) ;
#26030=CARTESIAN_POINT('Ctrl Pts',(-20.4589227820742,12.,124.09649959103)) ;
#26031=CARTESIAN_POINT('Ctrl Pts',(-20.4684137702848,11.999999998883,124.078855580405)) ;
#26032=CARTESIAN_POINT('Ctrl Pts',(-20.4774766407636,11.9999999981016,124.06099792884)) ;
#26033=CARTESIAN_POINT('Ctrl Pts',(-20.4774766589072,11.9999999855698,124.060997939105)) ;
#26034=CARTESIAN_POINT('Ctrl Pts',(-20.4738210693409,12.0003235019738,124.067013058878)) ;
#26035=CARTESIAN_POINT('Ctrl Pts',(-20.4701147454655,12.0006473274418,124.072997181455)) ;
#26036=CARTESIAN_POINT('Ctrl Pts',(-20.4599245187432,12.0015264826127,124.089143747839)) ;
#26037=CARTESIAN_POINT('Ctrl Pts',(-20.4533438467063,12.0020823228166,124.099244203208)) ;
#26038=CARTESIAN_POINT('Ctrl Pts',(-20.4376630195742,12.0033791105184,124.122567490034)) ;
#26039=CARTESIAN_POINT('Ctrl Pts',(-20.428452184928,12.00412012563,124.13571341996)) ;
#26040=CARTESIAN_POINT('Ctrl Pts',(-20.4137874661628,12.0052668735873,124.155808361001)) ;
#26041=CARTESIAN_POINT('Ctrl Pts',(-20.4085087918783,12.0056733952083,124.162883083463)) ;
#26042=CARTESIAN_POINT('Ctrl Pts',(-20.3995692854148,12.0063514271215,124.174603146536)) ;
#26043=CARTESIAN_POINT('Ctrl Pts',(-20.3959496291952,12.0066232068953,124.179279473883)) ;
#26044=CARTESIAN_POINT('Ctrl Pts',(-20.389035901371,12.0071371506433,124.188081737764)) ;
#26045=CARTESIAN_POINT('Ctrl Pts',(-20.3857486085966,12.0073793602748,124.192212832432)) ;
#26046=CARTESIAN_POINT('Ctrl Pts',(-20.3788189177888,12.0078854994504,124.200808937747)) ;
#26047=CARTESIAN_POINT('Ctrl Pts',(-20.3751716169832,12.0081493836918,124.205269839539)) ;
#26048=CARTESIAN_POINT('Ctrl Pts',(-20.3655403449871,12.0088397827434,124.216884728752)) ;
#26049=CARTESIAN_POINT('Ctrl Pts',(-20.3595069177169,12.0092658930284,124.223997249251)) ;
#26050=CARTESIAN_POINT('Ctrl Pts',(-20.3387248785043,12.0107130376805,124.247947606164)) ;
#26051=CARTESIAN_POINT('Ctrl Pts',(-20.3236038917401,12.0117313025691,124.2644565148)) ;
#26052=CARTESIAN_POINT('Ctrl Pts',(-20.2970853611994,12.0134701087367,124.291892010138)) ;
#26053=CARTESIAN_POINT('Ctrl Pts',(-20.285909288432,12.0141897642512,124.303024936002)) ;
#26054=CARTESIAN_POINT('Ctrl Pts',(-20.2687677941853,12.0152756144541,124.319465750278)) ;
#26055=CARTESIAN_POINT('Ctrl Pts',(-20.2629573020348,12.0156406853718,124.324932900176)) ;
#26056=CARTESIAN_POINT('Ctrl Pts',(-20.251036665777,12.0163837308229,124.335935903857)) ;
#26057=CARTESIAN_POINT('Ctrl Pts',(-20.2449232877602,12.0167617110627,124.341467683723)) ;
#26058=CARTESIAN_POINT('Ctrl Pts',(-20.2220121681254,12.0181669907764,124.361790538748)) ;
#26059=CARTESIAN_POINT('Ctrl Pts',(-20.2048728639287,12.0191962596192,124.376190102632)) ;
#26060=CARTESIAN_POINT('Ctrl Pts',(-20.1805077183176,12.020627613373,124.395568605511)) ;
#26061=CARTESIAN_POINT('Ctrl Pts',(-20.1736021343383,12.0210298357192,124.40094346769)) ;
#26062=CARTESIAN_POINT('Ctrl Pts',(-20.1618123540089,12.0217104198955,124.409922680335)) ;
#26063=CARTESIAN_POINT('Ctrl Pts',(-20.1569573042242,12.0219889590695,124.413564771728)) ;
#26064=CARTESIAN_POINT('Ctrl Pts',(-20.1481685120957,12.0224899453031,124.42005833285)) ;
#26065=CARTESIAN_POINT('Ctrl Pts',(-20.144244314968,12.0227124739396,124.422922494172)) ;
#26066=CARTESIAN_POINT('Ctrl Pts',(-20.1318578952527,12.0234112809899,124.431852782512)) ;
#26067=CARTESIAN_POINT('Ctrl Pts',(-20.12333651938,12.0238869104373,124.437836103776)) ;
#26068=CARTESIAN_POINT('Ctrl Pts',(-20.0999049834915,12.0251830662214,124.453855348649)) ;
#26069=CARTESIAN_POINT('Ctrl Pts',(-20.0848515943592,12.0260031798493,124.463677252077)) ;
#26070=CARTESIAN_POINT('Ctrl Pts',(-20.0624930779402,12.0272072193321,124.477587525388)) ;
#26071=CARTESIAN_POINT('Ctrl Pts',(-20.0553503676959,12.0275897944985,124.481932557054)) ;
#26072=CARTESIAN_POINT('Ctrl Pts',(-20.0425338660351,12.0282728948922,124.489553957019)) ;
#26073=CARTESIAN_POINT('Ctrl Pts',(-20.0368768872401,12.0285732479674,124.492857991191)) ;
#26074=CARTESIAN_POINT('Ctrl Pts',(-20.0234686598769,12.029282547681,124.500548526906)) ;
#26075=CARTESIAN_POINT('Ctrl Pts',(-20.0156959971541,12.0296917004838,124.504896952722)) ;
#26076=CARTESIAN_POINT('Ctrl Pts',(-19.9832852508231,12.0313896109435,124.522577080194)) ;
#26077=CARTESIAN_POINT('Ctrl Pts',(-19.9582490050827,12.0326821394932,124.535161706767)) ;
#26078=CARTESIAN_POINT('Ctrl Pts',(-19.9230189690532,12.0344692748047,124.551411041485)) ;
#26079=CARTESIAN_POINT('Ctrl Pts',(-19.9131686659644,12.0349656308202,124.55580067594)) ;
#26080=CARTESIAN_POINT('Ctrl Pts',(-19.8963223391377,12.0358088084923,124.563048175201)) ;
#26081=CARTESIAN_POINT('Ctrl Pts',(-19.8893549590441,12.0361558985472,124.565971056342)) ;
#26082=CARTESIAN_POINT('Ctrl Pts',(-19.8789376232523,12.0366724659772,124.570230572808)) ;
#26083=CARTESIAN_POINT('Ctrl Pts',(-19.8755075506304,12.0368421718385,124.57161534704)) ;
#26084=CARTESIAN_POINT('Ctrl Pts',(-19.8648462191222,12.0373684864209,124.575864555093)) ;
#26085=CARTESIAN_POINT('Ctrl Pts',(-19.8575943272026,12.0377248296873,124.578676739984)) ;
#26086=CARTESIAN_POINT('Ctrl Pts',(-19.8378010135038,12.0386931774225,124.586140557026)) ;
#26087=CARTESIAN_POINT('Ctrl Pts',(-19.8252104081584,12.0393045167842,124.590658865802)) ;
#26088=CARTESIAN_POINT('Ctrl Pts',(-19.7956964157781,12.0407285350002,124.600718645363)) ;
#26089=CARTESIAN_POINT('Ctrl Pts',(-19.7787223471021,12.0415406448223,124.606102290676)) ;
#26090=CARTESIAN_POINT('Ctrl Pts',(-19.7516131399652,12.0428310586428,124.614067211164)) ;
#26091=CARTESIAN_POINT('Ctrl Pts',(-19.7415506724082,12.0433086936194,124.616887076666)) ;
#26092=CARTESIAN_POINT('Ctrl Pts',(-19.7206893896845,12.0442965319979,124.62245200034)) ;
#26093=CARTESIAN_POINT('Ctrl Pts',(-19.7098868378585,12.0448067489102,124.625179515279)) ;
#26094=CARTESIAN_POINT('Ctrl Pts',(-19.6757140325349,12.0464169892136,124.633323363431)) ;
#26095=CARTESIAN_POINT('Ctrl Pts',(-19.6522235742641,12.0475184551027,124.638211570731)) ;
#26096=CARTESIAN_POINT('Ctrl Pts',(-19.6171103822421,12.04915641197,124.64446990586)) ;
#26097=CARTESIAN_POINT('Ctrl Pts',(-19.6055854942518,12.0496926476333,124.646357795818)) ;
#26098=CARTESIAN_POINT('Ctrl Pts',(-19.5857186916462,12.0506143194798,124.649326939591)) ;
#26099=CARTESIAN_POINT('Ctrl Pts',(-19.5773891963475,12.0509999315481,124.650485997081)) ;
#26100=CARTESIAN_POINT('Ctrl Pts',(-19.5624628516343,12.0516892997172,124.652409678574)) ;
#26101=CARTESIAN_POINT('Ctrl Pts',(-19.5558704031638,12.0519931973621,124.653205952913)) ;
#26102=CARTESIAN_POINT('Ctrl Pts',(-19.5293790930094,12.0532118418825,124.656191758732)) ;
#26103=CARTESIAN_POINT('Ctrl Pts',(-19.5094352662898,12.0541231886579,124.657955659061)) ;
#26104=CARTESIAN_POINT('Ctrl Pts',(-19.4793903244375,12.0554955416909,124.659886970216)) ;
#26105=CARTESIAN_POINT('Ctrl Pts',(-19.4693155323012,12.0559555993903,124.660412209013)) ;
#26106=CARTESIAN_POINT('Ctrl Pts',(-19.4532847238482,12.056688238072,124.661053482769)) ;
#26107=CARTESIAN_POINT('Ctrl Pts',(-19.4473323281987,12.0569604032001,124.661248997778)) ;
#26108=CARTESIAN_POINT('Ctrl Pts',(-19.4411847351566,12.0572417066106,124.661406952228)) ;
#26109=CARTESIAN_POINT('Ctrl Pts',(-19.4409906964236,12.0572505857107,124.661411892577)) ;
#26110=CARTESIAN_POINT('Ctrl Pts',(-19.4406116208727,12.057267932418,124.661421455728)) ;
#26111=CARTESIAN_POINT('Ctrl Pts',(-19.4404265840258,12.0572764000064,124.661426082631)) ;
#26112=CARTESIAN_POINT('Ctrl Pts',(-19.4400644514001,12.0572929721822,124.661435057384)) ;
#26113=CARTESIAN_POINT('Ctrl Pts',(-19.439887355894,12.05730107674,124.661439408682)) ;
#26114=CARTESIAN_POINT('Ctrl Pts',(-19.4395401349731,12.0573169672439,124.661447866165)) ;
#26115=CARTESIAN_POINT('Ctrl Pts',(-19.439370009467,12.0573247531797,124.661451975259)) ;
#26116=CARTESIAN_POINT('Ctrl Pts',(-19.4390358319261,12.0573400474351,124.661459978471)) ;
#26117=CARTESIAN_POINT('Ctrl Pts',(-19.438871779903,12.057347555742,124.661463875027)) ;
#26118=CARTESIAN_POINT('Ctrl Pts',(-19.4385489143416,12.0573623329221,124.661471480101)) ;
#26119=CARTESIAN_POINT('Ctrl Pts',(-19.4383901011446,12.0573696017696,124.661475190643)) ;
#26120=CARTESIAN_POINT('Ctrl Pts',(-19.438076929371,12.0573839358809,124.661482447917)) ;
#26121=CARTESIAN_POINT('Ctrl Pts',(-19.4379225708226,12.0573910011349,124.661485996324)) ;
#26122=CARTESIAN_POINT('Ctrl Pts',(-19.437617563227,12.057404962142,124.661492951323)) ;
#26123=CARTESIAN_POINT('Ctrl Pts',(-19.4374669140344,12.0574118578949,124.661496359277)) ;
#26124=CARTESIAN_POINT('Ctrl Pts',(-19.4371686066429,12.0574255127705,124.661503053555)) ;
#26125=CARTESIAN_POINT('Ctrl Pts',(-19.4370209486558,12.0574322718779,124.661506340945)) ;
#26126=CARTESIAN_POINT('Ctrl Pts',(-19.436727922283,12.0574456855551,124.661512812793)) ;
#26127=CARTESIAN_POINT('Ctrl Pts',(-19.4365825538598,12.0574523401223,124.661515998056)) ;
#26128=CARTESIAN_POINT('Ctrl Pts',(-19.4362934092924,12.0574655766305,124.661522283219)) ;
#26129=CARTESIAN_POINT('Ctrl Pts',(-19.4361496331152,12.0574721585701,124.661525383671)) ;
#26130=CARTESIAN_POINT('Ctrl Pts',(-19.4358629669209,12.0574852821421,124.661531515974)) ;
#26131=CARTESIAN_POINT('Ctrl Pts',(-19.4357200770283,12.0574918237673,124.661534548127)) ;
#26132=CARTESIAN_POINT('Ctrl Pts',(-19.4354344547226,12.0575049000676,124.661540560083)) ;
#26133=CARTESIAN_POINT('Ctrl Pts',(-19.4352917223177,12.0575114347421,124.66154353994)) ;
#26134=CARTESIAN_POINT('Ctrl Pts',(-19.4350056466662,12.0575245323185,124.661549463377)) ;
#26135=CARTESIAN_POINT('Ctrl Pts',(-19.434862303283,12.0575310952277,124.661552406749)) ;
#26136=CARTESIAN_POINT('Ctrl Pts',(-19.4345741763691,12.0575442872488,124.661558273474)) ;
#26137=CARTESIAN_POINT('Ctrl Pts',(-19.4344293929624,12.0575509163576,124.661561196325)) ;
#26138=CARTESIAN_POINT('Ctrl Pts',(-19.4341374718464,12.0575642826441,124.661567038807)) ;
#26139=CARTESIAN_POINT('Ctrl Pts',(-19.4339903339254,12.057571019836,124.661569957617)) ;
#26140=CARTESIAN_POINT('Ctrl Pts',(-19.4336926702877,12.0575846496269,124.661575809852)) ;
#26141=CARTESIAN_POINT('Ctrl Pts',(-19.4335421444777,12.0575915422368,124.66157874207)) ;
#26142=CARTESIAN_POINT('Ctrl Pts',(-19.4332365079462,12.0576055377026,124.661584640579)) ;
#26143=CARTESIAN_POINT('Ctrl Pts',(-19.4330813976021,12.0576126405504,124.661587605182)) ;
#26144=CARTESIAN_POINT('Ctrl Pts',(-19.4327651732268,12.0576271214925,124.661593590244)) ;
#26145=CARTESIAN_POINT('Ctrl Pts',(-19.4326040590737,12.0576344996049,124.661596608426)) ;
#26146=CARTESIAN_POINT('Ctrl Pts',(-19.4322740989793,12.0576496102551,124.661602725804)) ;
#26147=CARTESIAN_POINT('Ctrl Pts',(-19.4321052529801,12.0576573428126,124.661605821939)) ;
#26148=CARTESIAN_POINT('Ctrl Pts',(-19.4317576680302,12.0576732613833,124.661612125155)) ;
#26149=CARTESIAN_POINT('Ctrl Pts',(-19.4315789289088,12.0576814474273,124.661615328111)) ;
#26150=CARTESIAN_POINT('Ctrl Pts',(-19.4312087741874,12.0576984005296,124.661621881751)) ;
#26151=CARTESIAN_POINT('Ctrl Pts',(-19.4310173582948,12.0577071676329,124.661625226807)) ;
#26152=CARTESIAN_POINT('Ctrl Pts',(-19.4306181438283,12.0577254527075,124.661632111472)) ;
#26153=CARTESIAN_POINT('Ctrl Pts',(-19.430410345223,12.0577349707246,124.661635643229)) ;
#26154=CARTESIAN_POINT('Ctrl Pts',(-19.4299732384347,12.0577549926066,124.66164296328)) ;
#26155=CARTESIAN_POINT('Ctrl Pts',(-19.4297439301276,12.0577654965416,124.661646740289)) ;
#26156=CARTESIAN_POINT('Ctrl Pts',(-19.4293241206059,12.0577847274385,124.661653539537)) ;
#26157=CARTESIAN_POINT('Ctrl Pts',(-19.4291336196373,12.0577934542766,124.661656581331)) ;
#26158=CARTESIAN_POINT('Ctrl Pts',(-19.4284938709738,12.0578227619729,124.661666650114)) ;
#26159=CARTESIAN_POINT('Ctrl Pts',(-19.4280446201722,12.0578433441248,124.66167347844)) ;
#26160=CARTESIAN_POINT('Ctrl Pts',(-19.4228496320521,12.0580813658386,124.661749637377)) ;
#26161=CARTESIAN_POINT('Ctrl Pts',(-19.4181035494019,12.0582989796514,124.661792180226)) ;
#26162=CARTESIAN_POINT('Ctrl Pts',(-19.4085663181077,12.0587366393522,124.661823348918)) ;
#26163=CARTESIAN_POINT('Ctrl Pts',(-19.4037752472262,12.0589566851438,124.661811461456)) ;
#26164=CARTESIAN_POINT('Ctrl Pts',(-19.3928182714876,12.0594603775997,124.661721279295)) ;
#26165=CARTESIAN_POINT('Ctrl Pts',(-19.386652646881,12.059744143375,124.661624903119)) ;
#26166=CARTESIAN_POINT('Ctrl Pts',(-19.3702485254162,12.0605000334054,124.661247058863)) ;
#26167=CARTESIAN_POINT('Ctrl Pts',(-19.3600123721226,12.0609726605192,124.660885368162)) ;
#26168=CARTESIAN_POINT('Ctrl Pts',(-19.3194505221568,12.0628488770994,124.658952746186)) ;
#26169=CARTESIAN_POINT('Ctrl Pts',(-19.2891818541446,12.0642565609159,124.656402808202)) ;
#26170=CARTESIAN_POINT('Ctrl Pts',(-19.2499488244313,12.0660792864179,124.651653000755)) ;
#26171=CARTESIAN_POINT('Ctrl Pts',(-19.2408739165736,12.0665008166201,124.650453053011)) ;
#26172=CARTESIAN_POINT('Ctrl Pts',(-19.2271113608395,12.0671398600002,124.648479226377)) ;
#26173=CARTESIAN_POINT('Ctrl Pts',(-19.2224136208351,12.0673579534745,124.647778127388)) ;
#26174=CARTESIAN_POINT('Ctrl Pts',(-19.2141602182459,12.0677410520105,124.646498244024)) ;
#26175=CARTESIAN_POINT('Ctrl Pts',(-19.2106028531344,12.067906152505,124.645930833164)) ;
#26176=CARTESIAN_POINT('Ctrl Pts',(-19.2033761632301,12.0682415114393,124.644746097007)) ;
#26177=CARTESIAN_POINT('Ctrl Pts',(-19.199707041974,12.0684117591614,124.644127749704)) ;
#26178=CARTESIAN_POINT('Ctrl Pts',(-19.1958534322709,12.0685905524619,124.643460602479)) ;
#26179=CARTESIAN_POINT('Ctrl Pts',(-19.1956661421711,12.0685992419969,124.643428134312)) ;
#26180=CARTESIAN_POINT('Ctrl Pts',(-19.195275631099,12.0686173601248,124.643360344485)) ;
#26181=CARTESIAN_POINT('Ctrl Pts',(-19.1950724114504,12.0686267886501,124.643325015241)) ;
#26182=CARTESIAN_POINT('Ctrl Pts',(-19.194648853637,12.0686464398438,124.643251272729)) ;
#26183=CARTESIAN_POINT('Ctrl Pts',(-19.1944285169969,12.0686566624344,124.643212850616)) ;
#26184=CARTESIAN_POINT('Ctrl Pts',(-19.1941166032895,12.0686711337091,124.643158373109)) ;
#26185=CARTESIAN_POINT('Ctrl Pts',(-19.1940250176593,12.0686753828279,124.643142366626)) ;
#26186=CARTESIAN_POINT('Ctrl Pts',(-19.1938174574849,12.0686850125726,124.643106067329)) ;
#26187=CARTESIAN_POINT('Ctrl Pts',(-19.1937014843561,12.0686903931282,124.643085768406)) ;
#26188=CARTESIAN_POINT('Ctrl Pts',(-19.1888127984142,12.0689172024584,124.642229383663)) ;
#26189=CARTESIAN_POINT('Ctrl Pts',(-19.1840449741949,12.0691383833535,124.641365568702)) ;
#26190=CARTESIAN_POINT('Ctrl Pts',(-19.1717441788884,12.0697090229041,124.639063011384)) ;
#26191=CARTESIAN_POINT('Ctrl Pts',(-19.1642191986178,12.0700581093992,124.637582625163)) ;
#26192=CARTESIAN_POINT('Ctrl Pts',(-19.1410204071488,12.0711346979073,124.632796570008)) ;
#26193=CARTESIAN_POINT('Ctrl Pts',(-19.125396130456,12.0718602549915,124.629258799168)) ;
#26194=CARTESIAN_POINT('Ctrl Pts',(-19.0835714685436,12.0738088310328,124.618939578824)) ;
#26195=CARTESIAN_POINT('Ctrl Pts',(-19.0575162399829,12.0750312482448,124.611606008327)) ;
#26196=CARTESIAN_POINT('Ctrl Pts',(-19.0268513532554,12.0764976026809,124.601890140989)) ;
#26197=CARTESIAN_POINT('Ctrl Pts',(-19.0219924989272,12.0767307445927,124.600317831159)) ;
#26198=CARTESIAN_POINT('Ctrl Pts',(-19.0145022832069,12.0770914495912,124.597843211721)) ;
#26199=CARTESIAN_POINT('Ctrl Pts',(-19.0118640612916,12.0772187483851,124.596961817217)) ;
#26200=CARTESIAN_POINT('Ctrl Pts',(-19.0066141860477,12.0774725732244,124.595188403482)) ;
#26201=CARTESIAN_POINT('Ctrl Pts',(-19.0040025015199,12.0775990967851,124.594296526557)) ;
#26202=CARTESIAN_POINT('Ctrl Pts',(-18.9988368058538,12.0778498558955,124.592513343906)) ;
#26203=CARTESIAN_POINT('Ctrl Pts',(-18.9962826919722,12.0779740863863,124.591622382254)) ;
#26204=CARTESIAN_POINT('Ctrl Pts',(-18.9917075901926,12.0781970608444,124.590009754347)) ;
#26205=CARTESIAN_POINT('Ctrl Pts',(-18.9896855291606,12.0782957651326,124.589291160662)) ;
#26206=CARTESIAN_POINT('Ctrl Pts',(-18.983382918585,12.0786039071758,124.587033062199)) ;
#26207=CARTESIAN_POINT('Ctrl Pts',(-18.9791089268567,12.0788135723052,124.585475399608)) ;
#26208=CARTESIAN_POINT('Ctrl Pts',(-18.9670217508405,12.0794085061267,124.580995316588)) ;
#26209=CARTESIAN_POINT('Ctrl Pts',(-18.9592292173005,12.0797944240482,124.578017978943)) ;
#26210=CARTESIAN_POINT('Ctrl Pts',(-18.9292645887745,12.0812870577032,124.566224161847)) ;
#26211=CARTESIAN_POINT('Ctrl Pts',(-18.9073169515415,12.0823991197782,124.556851570734)) ;
#26212=CARTESIAN_POINT('Ctrl Pts',(-18.8845552145466,12.083564050551,124.54635105798)) ;
#26213=CARTESIAN_POINT('Ctrl Pts',(-18.8834600262495,12.0836201305224,124.545843897419)) ;
#26214=CARTESIAN_POINT('Ctrl Pts',(-18.8657605416334,12.0845269026316,124.537616455553)) ;
#26215=CARTESIAN_POINT('Ctrl Pts',(-18.8493269893566,12.0853751245775,124.529533758679)) ;
#26216=CARTESIAN_POINT('Ctrl Pts',(-18.8286249753884,12.0864499439215,124.518780456604)) ;
#26217=CARTESIAN_POINT('Ctrl Pts',(-18.8241871357782,12.0866807379356,124.516441268088)) ;
#26218=CARTESIAN_POINT('Ctrl Pts',(-18.8172357565421,12.0870428640428,124.512723547234)) ;
#26219=CARTESIAN_POINT('Ctrl Pts',(-18.8147126834728,12.0871744294068,124.511362981065)) ;
#26220=CARTESIAN_POINT('Ctrl Pts',(-18.8096721717043,12.0874375275458,124.508622464916)) ;
#26221=CARTESIAN_POINT('Ctrl Pts',(-18.8071547625425,12.0875690591694,124.507242497448)) ;
#26222=CARTESIAN_POINT('Ctrl Pts',(-18.801501631591,12.0878647324247,124.504118247187)) ;
#26223=CARTESIAN_POINT('Ctrl Pts',(-18.798368619582,12.0880288083069,124.502369109239)) ;
#26224=CARTESIAN_POINT('Ctrl Pts',(-18.7888867428192,12.0885260484879,124.49702176359)) ;
#26225=CARTESIAN_POINT('Ctrl Pts',(-18.782561801549,12.0888586530077,124.493381418098)) ;
#26226=CARTESIAN_POINT('Ctrl Pts',(-18.7674488831082,12.0896559170703,124.484506032573)) ;
#26227=CARTESIAN_POINT('Ctrl Pts',(-18.7586925736956,12.0901199194689,124.479218100648)) ;
#26228=CARTESIAN_POINT('Ctrl Pts',(-18.7341723556921,12.0914267461618,124.463996526492)) ;
#26229=CARTESIAN_POINT('Ctrl Pts',(-18.7185642720902,12.0922673334528,124.453817080138)) ;
#26230=CARTESIAN_POINT('Ctrl Pts',(-18.686447694152,12.0940265539756,124.431832167163)) ;
#26231=CARTESIAN_POINT('Ctrl Pts',(-18.6699874579514,12.0949456966258,124.419965960952)) ;
#26232=CARTESIAN_POINT('Ctrl Pts',(-18.6498073608539,12.0961005888327,124.404658016493)) ;
#26233=CARTESIAN_POINT('Ctrl Pts',(-18.6458097753173,12.0963307583701,124.401587310526)) ;
#26234=CARTESIAN_POINT('Ctrl Pts',(-18.6395464583661,12.0966936287847,124.396715683008)) ;
#26235=CARTESIAN_POINT('Ctrl Pts',(-18.6372682144919,12.0968260930661,124.394930924558)) ;
#26236=CARTESIAN_POINT('Ctrl Pts',(-18.6327133843536,12.0970918813463,124.391337110293)) ;
#26237=CARTESIAN_POINT('Ctrl Pts',(-18.6304368717348,12.0972252056011,124.389527990721)) ;
#26238=CARTESIAN_POINT('Ctrl Pts',(-18.6258596232342,12.097494251951,124.385864370794)) ;
#26239=CARTESIAN_POINT('Ctrl Pts',(-18.6235591099065,12.0976299769295,124.384009622674)) ;
#26240=CARTESIAN_POINT('Ctrl Pts',(-18.6205214380454,12.0978098601505,124.381542728985)) ;
#26241=CARTESIAN_POINT('Ctrl Pts',(-18.6197783720828,12.0978539157672,124.380937865914)) ;
#26242=CARTESIAN_POINT('Ctrl Pts',(-18.6171912011342,12.0980074916404,124.378826932835)) ;
#26243=CARTESIAN_POINT('Ctrl Pts',(-18.6153507066691,12.0981170728674,124.377316450639)) ;
#26244=CARTESIAN_POINT('Ctrl Pts',(-18.6089361744421,12.0985001331964,124.372021341065)) ;
#26245=CARTESIAN_POINT('Ctrl Pts',(-18.6043848064618,12.0987739753247,124.368209405571)) ;
#26246=CARTESIAN_POINT('Ctrl Pts',(-18.5901353086799,12.0996376696245,124.356101173324)) ;
#26247=CARTESIAN_POINT('Ctrl Pts',(-18.5805370220431,12.1002288535301,124.347688728406)) ;
#26248=CARTESIAN_POINT('Ctrl Pts',(-18.5500842274618,12.1021322209924,124.320162394536)) ;
#26249=CARTESIAN_POINT('Ctrl Pts',(-18.5297487021016,12.1034434568904,124.30048673222)) ;
#26250=CARTESIAN_POINT('Ctrl Pts',(-18.5049979413526,12.1050847841069,124.274856604347)) ;
#26251=CARTESIAN_POINT('Ctrl Pts',(-18.4999444178514,12.1054225466107,124.269530417417)) ;
#26252=CARTESIAN_POINT('Ctrl Pts',(-18.4913785673575,12.105999728123,124.260341598713)) ;
#26253=CARTESIAN_POINT('Ctrl Pts',(-18.4878429846463,12.1062393536411,124.256500927122)) ;
#26254=CARTESIAN_POINT('Ctrl Pts',(-18.4807312329972,12.1067242527057,124.248677708956)) ;
#26255=CARTESIAN_POINT('Ctrl Pts',(-18.4771563770096,12.1069695105611,124.24469411402)) ;
#26256=CARTESIAN_POINT('Ctrl Pts',(-18.4698242084639,12.1074757731801,124.236417271705)) ;
#26257=CARTESIAN_POINT('Ctrl Pts',(-18.4660704798358,12.1077367446997,124.232121013496)) ;
#26258=CARTESIAN_POINT('Ctrl Pts',(-18.4441523147958,12.1092714977858,124.206685639786)) ;
#26259=CARTESIAN_POINT('Ctrl Pts',(-18.4266695721527,12.1105399709451,124.184969470474)) ;
#26260=CARTESIAN_POINT('Ctrl Pts',(-18.3980911222504,12.1127080177427,124.146934089148)) ;
#26261=CARTESIAN_POINT('Ctrl Pts',(-18.3866290928262,12.1136070143731,124.130903545692)) ;
#26262=CARTESIAN_POINT('Ctrl Pts',(-18.3701432296329,12.1149475624964,124.106654934539)) ;
#26263=CARTESIAN_POINT('Ctrl Pts',(-18.3648276190754,12.115387648517,124.098638906238)) ;
#26264=CARTESIAN_POINT('Ctrl Pts',(-18.3547732830454,12.1162356186954,124.083090121085)) ;
#26265=CARTESIAN_POINT('Ctrl Pts',(-18.3500214397369,12.1166434238422,124.075566527033)) ;
#26266=CARTESIAN_POINT('Ctrl Pts',(-18.3453503415257,12.1170515107657,124.067992850388)) ;
#26267=CARTESIAN_POINT('Ctrl Pts',(-20.8283303706881,10.,122.926041870813)) ;
#26268=CARTESIAN_POINT('Ctrl Pts',(-20.5445170967909,9.82001091963712,123.023196933748)) ;
#26269=CARTESIAN_POINT('Ctrl Pts',(-20.8845408159969,10.0066268508181,123.090165629856)) ;
#26270=CARTESIAN_POINT('Ctrl Pts',(-20.5894888524673,9.82663777045524,123.154521539138)) ;
#26271=CARTESIAN_POINT('Ctrl Pts',(-20.9394617690737,10.0198574772991,123.437507823531)) ;
#26272=CARTESIAN_POINT('Ctrl Pts',(-20.633420846741,9.83986839693625,123.432353293108)) ;
#26273=CARTESIAN_POINT('Ctrl Pts',(-20.8387858493119,10.0398330985578,123.958797508285)) ;
#26274=CARTESIAN_POINT('Ctrl Pts',(-20.5528814274113,9.85984401819488,123.849407562291)) ;
#26275=CARTESIAN_POINT('Ctrl Pts',(-20.5666727975867,10.0597504334597,124.412849839357)) ;
#26276=CARTESIAN_POINT('Ctrl Pts',(-20.3351890331055,9.87976135309682,124.212644574099)) ;
#26277=CARTESIAN_POINT('Ctrl Pts',(-20.157556275784,10.0796237101757,124.747029739186)) ;
#26278=CARTESIAN_POINT('Ctrl Pts',(-20.007894029438,9.89963462981282,124.479989709356)) ;
#26279=CARTESIAN_POINT('Ctrl Pts',(-19.6551315118144,10.0996482003397,124.922482691163)) ;
#26280=CARTESIAN_POINT('Ctrl Pts',(-19.6059539581694,9.91965911997678,124.6203502007)) ;
#26281=CARTESIAN_POINT('Ctrl Pts',(-19.1270395366036,10.1195160414904,124.915890798164)) ;
#26282=CARTESIAN_POINT('Ctrl Pts',(-19.183479078867,9.9395269611275,124.615075206311)) ;
#26283=CARTESIAN_POINT('Ctrl Pts',(-18.6307952228403,10.1394616923699,124.72957580943)) ;
#26284=CARTESIAN_POINT('Ctrl Pts',(-18.7864838467008,9.95947261200706,124.466021078065)) ;
#26285=CARTESIAN_POINT('Ctrl Pts',(-18.2288224078826,10.1593670929869,124.385607616877)) ;
#26286=CARTESIAN_POINT('Ctrl Pts',(-18.4649063275282,9.97937801262402,124.19084435197)) ;
#26287=CARTESIAN_POINT('Ctrl Pts',(-17.9678535157127,10.1792413208033,123.926349000794)) ;
#26288=CARTESIAN_POINT('Ctrl Pts',(-18.2561329793354,9.99925224044038,123.823435269459)) ;
#26289=CARTESIAN_POINT('Ctrl Pts',(-17.878734209588,10.1992271116809,123.402675114316)) ;
#26290=CARTESIAN_POINT('Ctrl Pts',(-18.1848402358937,10.019238031318,123.404495614569)) ;
#26291=CARTESIAN_POINT('Ctrl Pts',(-17.973517700436,10.2191213543406,122.882519965019)) ;
#26292=CARTESIAN_POINT('Ctrl Pts',(-18.2606699231879,10.0391322739778,122.988371207676)) ;
#26293=CARTESIAN_POINT('Ctrl Pts',(-18.2387528910803,10.2390000704127,122.425502981447)) ;
#26294=CARTESIAN_POINT('Ctrl Pts',(-18.4728612986517,10.0590109900498,122.62275860733)) ;
#26295=CARTESIAN_POINT('Ctrl Pts',(-18.647614090005,10.2590395202573,122.084258749108)) ;
#26296=CARTESIAN_POINT('Ctrl Pts',(-18.7999520972875,10.0790504398944,122.349765888777)) ;
#26297=CARTESIAN_POINT('Ctrl Pts',(-19.1441721121047,10.2789026817952,121.90452088182)) ;
#26298=CARTESIAN_POINT('Ctrl Pts',(-19.1972003931787,10.0989136014323,122.205978444044)) ;
#26299=CARTESIAN_POINT('Ctrl Pts',(-19.6750232066901,10.2988820498094,121.904721686728)) ;
#26300=CARTESIAN_POINT('Ctrl Pts',(-19.6218814079036,10.1188929694465,122.206142590273)) ;
#26301=CARTESIAN_POINT('Ctrl Pts',(-20.1701799765179,10.3186926303322,122.084083785786)) ;
#26302=CARTESIAN_POINT('Ctrl Pts',(-20.0180064135448,10.1387035499693,122.349636107043)) ;
#26303=CARTESIAN_POINT('Ctrl Pts',(-20.578226084171,10.3386735586178,122.423812224567)) ;
#26304=CARTESIAN_POINT('Ctrl Pts',(-20.3444408940403,10.1586844782549,122.621421767106)) ;
#26305=CARTESIAN_POINT('Ctrl Pts',(-20.8444469588477,10.3585662304872,122.880680954098)) ;
#26306=CARTESIAN_POINT('Ctrl Pts',(-20.5574140513056,10.1785771501243,122.986919611144)) ;
#26307=CARTESIAN_POINT('Ctrl Pts',(-20.9398341757817,10.3784925607743,123.40162915944)) ;
#26308=CARTESIAN_POINT('Ctrl Pts',(-20.6337210673662,10.1985034804115,123.403677177554)) ;
#26309=CARTESIAN_POINT('Ctrl Pts',(-20.8510572230715,10.3984631148666,123.924927290891)) ;
#26310=CARTESIAN_POINT('Ctrl Pts',(-20.5626906127405,10.2184740345037,123.822322291595)) ;
#26311=CARTESIAN_POINT('Ctrl Pts',(-20.6345446351863,10.4149949539542,124.307272603886)) ;
#26312=CARTESIAN_POINT('Ctrl Pts',(-20.3894922234183,10.2350058735914,124.128174543065)) ;
#26313=CARTESIAN_POINT('Ctrl Pts',(-20.3891097552813,10.4283346927818,124.557601822174)) ;
#26314=CARTESIAN_POINT('Ctrl Pts',(-20.1931290434829,10.2483456124189,124.328455837242)) ;
#26315=CARTESIAN_POINT('Ctrl Pts',(-20.1744300570267,10.4383669350004,124.710615084593)) ;
#26316=CARTESIAN_POINT('Ctrl Pts',(-20.0213869924123,10.2583778546375,124.450860682641)) ;
#26317=CARTESIAN_POINT('Ctrl Pts',(-19.9407404802418,10.4482246356439,124.822421617883)) ;
#26318=CARTESIAN_POINT('Ctrl Pts',(-19.8344327400403,10.268235555281,124.540305070127)) ;
#26319=CARTESIAN_POINT('Ctrl Pts',(-19.6879423525307,10.4582165002831,124.893352629427)) ;
#26320=CARTESIAN_POINT('Ctrl Pts',(-19.6321963403517,10.2782274199202,124.597047919264)) ;
#26321=CARTESIAN_POINT('Ctrl Pts',(-19.4284710425139,10.4681390500432,124.919080315321)) ;
#26322=CARTESIAN_POINT('Ctrl Pts',(-19.4246096943487,10.2881499696804,124.61762631767)) ;
#26323=CARTESIAN_POINT('Ctrl Pts',(-19.0804105140851,10.4814168235367,124.893583985624)) ;
#26324=CARTESIAN_POINT('Ctrl Pts',(-19.14620736525,10.3014277431738,124.597234554234)) ;
#26325=CARTESIAN_POINT('Ctrl Pts',(-18.7455859092888,10.4947641624773,124.776616835755)) ;
#26326=CARTESIAN_POINT('Ctrl Pts',(-18.8783191462352,10.3147750821144,124.503658407746)) ;
#26327=CARTESIAN_POINT('Ctrl Pts',(-18.4584522382473,10.5079713942705,124.581549246914)) ;
#26328=CARTESIAN_POINT('Ctrl Pts',(-18.648603078249,10.3279823139076,124.347593121025)) ;
#26329=CARTESIAN_POINT('Ctrl Pts',(-18.269958838059,10.5179585103602,124.398989341533)) ;
#26330=CARTESIAN_POINT('Ctrl Pts',(-18.497812104421,10.3379694299973,124.201545371492)) ;
#26331=CARTESIAN_POINT('Ctrl Pts',(-18.1163933969716,10.52790941594,124.187269395838)) ;
#26332=CARTESIAN_POINT('Ctrl Pts',(-18.3749610183035,10.3479203355771,124.032167599002)) ;
#26333=CARTESIAN_POINT('Ctrl Pts',(-18.0010345813923,10.5379645179474,123.949583784548)) ;
#26334=CARTESIAN_POINT('Ctrl Pts',(-18.2826761214566,10.3579754375845,123.842018479487)) ;
#26335=CARTESIAN_POINT('Ctrl Pts',(-17.9299233421522,10.5477861912685,123.701439503961)) ;
#26336=CARTESIAN_POINT('Ctrl Pts',(-18.2257894437957,10.3677971109056,123.643501792389)) ;
#26337=CARTESIAN_POINT('Ctrl Pts',(-17.9019040586336,10.5578446623434,123.43862866708)) ;
#26338=CARTESIAN_POINT('Ctrl Pts',(-18.2033755364028,10.3778555819805,123.43325511011)) ;
#26339=CARTESIAN_POINT('Ctrl Pts',(-17.9200547531203,10.5677692735199,123.178437417212)) ;
#26340=CARTESIAN_POINT('Ctrl Pts',(-18.2179011304931,10.387780193157,123.22509433493)) ;
#26341=CARTESIAN_POINT('Ctrl Pts',(-18.0035329037317,10.5810466124203,122.839624585047)) ;
#26342=CARTESIAN_POINT('Ctrl Pts',(-18.2846726619434,10.4010575320574,122.954084471608)) ;
#26343=CARTESIAN_POINT('Ctrl Pts',(-18.174078890485,10.5943454916579,122.53009645584)) ;
#26344=CARTESIAN_POINT('Ctrl Pts',(-18.4211116702471,10.414356411295,122.706442742821)) ;
#26345=CARTESIAN_POINT('Ctrl Pts',(-18.4148290889509,10.6075843638286,122.278909287836)) ;
#26346=CARTESIAN_POINT('Ctrl Pts',(-18.61372828438,10.4275952834657,122.505480269817)) ;
#26347=CARTESIAN_POINT('Ctrl Pts',(-18.6267237904145,10.6175909819652,122.123170592624)) ;
#26348=CARTESIAN_POINT('Ctrl Pts',(-18.7832424340302,10.4376019016023,122.380894154854)) ;
#26349=CARTESIAN_POINT('Ctrl Pts',(-18.8632279358434,10.6276219270267,122.006771081612)) ;
#26350=CARTESIAN_POINT('Ctrl Pts',(-18.9724474943499,10.4476328466638,122.287775782223)) ;
#26351=CARTESIAN_POINT('Ctrl Pts',(-19.1118308518252,10.6374781003785,121.93402103227)) ;
#26352=CARTESIAN_POINT('Ctrl Pts',(-19.1713300681509,10.4574890200157,122.229578162461)) ;
#26353=CARTESIAN_POINT('Ctrl Pts',(-19.3729271808616,10.6474773713414,121.904805274484)) ;
#26354=CARTESIAN_POINT('Ctrl Pts',(-19.3802073636504,10.4674882909785,122.206207726809)) ;
#26355=CARTESIAN_POINT('Ctrl Pts',(-19.63249343999,10.6573718230987,121.920897070182)) ;
#26356=CARTESIAN_POINT('Ctrl Pts',(-19.5878600087485,10.4773827427359,122.219083373213)) ;
#26357=CARTESIAN_POINT('Ctrl Pts',(-19.8895240952696,10.6674351389081,121.982913347126)) ;
#26358=CARTESIAN_POINT('Ctrl Pts',(-19.7934840442871,10.4874460585452,122.268698557826)) ;
#26359=CARTESIAN_POINT('Ctrl Pts',(-20.1266813029374,10.6772739956477,122.086019825898)) ;
#26360=CARTESIAN_POINT('Ctrl Pts',(-19.9832086272329,10.4972849152848,122.351185625972)) ;
#26361=CARTESIAN_POINT('Ctrl Pts',(-20.3474018172676,10.6873401174653,122.231740902041)) ;
#26362=CARTESIAN_POINT('Ctrl Pts',(-20.1597838722231,10.5073510371024,122.46776433411)) ;
#26363=CARTESIAN_POINT('Ctrl Pts',(-20.5359503275351,10.6972233451896,122.410409425907)) ;
#26364=CARTESIAN_POINT('Ctrl Pts',(-20.3106209609387,10.5172342648267,122.6107005406)) ;
#26365=CARTESIAN_POINT('Ctrl Pts',(-20.6926994160287,10.7072128064683,122.620953380555)) ;
#26366=CARTESIAN_POINT('Ctrl Pts',(-20.4360184466383,10.5272237261055,122.779136903454)) ;
#26367=CARTESIAN_POINT('Ctrl Pts',(-20.8101391925705,10.7171765168948,122.854988704109)) ;
#26368=CARTESIAN_POINT('Ctrl Pts',(-20.5299682760089,10.5371874365319,122.966365995585)) ;
#26369=CARTESIAN_POINT('Ctrl Pts',(-20.8856615342042,10.7271715196257,123.106575647569)) ;
#26370=CARTESIAN_POINT('Ctrl Pts',(-20.5903840854433,10.5471824392628,123.167636082224)) ;
#26371=CARTESIAN_POINT('Ctrl Pts',(-20.9160649147156,10.737207850636,123.368548316933)) ;
#26372=CARTESIAN_POINT('Ctrl Pts',(-20.6147046374483,10.5572187702731,123.377214485628)) ;
#26373=CARTESIAN_POINT('Ctrl Pts',(-20.901237668564,10.7470540799783,123.626888226543)) ;
#26374=CARTESIAN_POINT('Ctrl Pts',(-20.6028407406531,10.5670649996154,123.583885836904)) ;
#26375=CARTESIAN_POINT('Ctrl Pts',(-20.8414280631531,10.7570395782535,123.88234711985)) ;
#26376=CARTESIAN_POINT('Ctrl Pts',(-20.5549910573095,10.5770504978907,123.788252351213)) ;
#26377=CARTESIAN_POINT('Ctrl Pts',(-20.7388329136923,10.7669744812365,124.122475498249)) ;
#26378=CARTESIAN_POINT('Ctrl Pts',(-20.4729131488679,10.5869854008736,123.98035400456)) ;
#26379=CARTESIAN_POINT('Ctrl Pts',(-20.5941893977946,10.7770319843317,124.343638489499)) ;
#26380=CARTESIAN_POINT('Ctrl Pts',(-20.3571965368945,10.5970429039689,124.157283333151)) ;
#26381=CARTESIAN_POINT('Ctrl Pts',(-20.4178270374552,10.7868536407023,124.532127444505)) ;
#26382=CARTESIAN_POINT('Ctrl Pts',(-20.216105589301,10.6068645603394,124.308072644051)) ;
#26383=CARTESIAN_POINT('Ctrl Pts',(-20.2068264505713,10.7969097033674,124.691194003415)) ;
#26384=CARTESIAN_POINT('Ctrl Pts',(-20.0473038554878,10.6169206230045,124.435324362058)) ;
#26385=CARTESIAN_POINT('Ctrl Pts',(-19.9738709151238,10.8068503680706,124.809425923824)) ;
#26386=CARTESIAN_POINT('Ctrl Pts',(-19.8609387422743,10.6268612877077,124.529907956941)) ;
#26387=CARTESIAN_POINT('Ctrl Pts',(-19.7250819168071,10.8167547720191,124.885913848072)) ;
#26388=CARTESIAN_POINT('Ctrl Pts',(-19.6619073830525,10.6367656916563,124.591096321636)) ;
#26389=CARTESIAN_POINT('Ctrl Pts',(-19.4630900672441,10.8268012570127,124.918337587752)) ;
#26390=CARTESIAN_POINT('Ctrl Pts',(-19.4523135810077,10.6468121766498,124.617033381453)) ;
#26391=CARTESIAN_POINT('Ctrl Pts',(-19.2033217042056,10.8366974848244,124.905200421478)) ;
#26392=CARTESIAN_POINT('Ctrl Pts',(-19.2444994521855,10.6567084044615,124.606521750019)) ;
#26393=CARTESIAN_POINT('Ctrl Pts',(-18.9456501548748,10.8467570683879,124.846258925075)) ;
#26394=CARTESIAN_POINT('Ctrl Pts',(-19.0383625055845,10.666767988025,124.559366649145)) ;
#26395=CARTESIAN_POINT('Ctrl Pts',(-18.7071032762899,10.8566090780567,124.745604613553)) ;
#26396=CARTESIAN_POINT('Ctrl Pts',(-18.8475263594419,10.6766199976938,124.478841692918)) ;
#26397=CARTESIAN_POINT('Ctrl Pts',(-18.4867618466311,10.8665716094963,124.604236201826)) ;
#26398=CARTESIAN_POINT('Ctrl Pts',(-18.6712543942556,10.6865825291334,124.36574560245)) ;
#26399=CARTESIAN_POINT('Ctrl Pts',(-18.2932415519936,10.8766031577357,124.425213596724)) ;
#26400=CARTESIAN_POINT('Ctrl Pts',(-18.5164393722649,10.6966140773728,124.222526126703)) ;
#26401=CARTESIAN_POINT('Ctrl Pts',(-18.1357799386366,10.8864945689487,124.218398117847)) ;
#26402=CARTESIAN_POINT('Ctrl Pts',(-18.3904718496513,10.7065054885858,124.057073085295)) ;
#26403=CARTESIAN_POINT('Ctrl Pts',(-18.0146891209222,10.8965108226567,123.984678099418)) ;
#26404=CARTESIAN_POINT('Ctrl Pts',(-18.2936007418435,10.7165217422938,123.870096295635)) ;
#26405=CARTESIAN_POINT('Ctrl Pts',(-17.9364599064937,10.9065409255014,123.732978598351)) ;
#26406=CARTESIAN_POINT('Ctrl Pts',(-18.2310191023128,10.7265518451385,123.66873611636)) ;
#26407=CARTESIAN_POINT('Ctrl Pts',(-17.9032046926023,10.9163973744551,123.476088297528)) ;
#26408=CARTESIAN_POINT('Ctrl Pts',(-18.2044167490604,10.7364082940922,123.463224374815)) ;
#26409=CARTESIAN_POINT('Ctrl Pts',(-17.9148974747618,10.9263963852274,123.213627004979)) ;
#26410=CARTESIAN_POINT('Ctrl Pts',(-18.2137726540653,10.7464073048645,123.253255524932)) ;
#26411=CARTESIAN_POINT('Ctrl Pts',(-17.9711291549323,10.9362916021454,122.959700121601)) ;
#26412=CARTESIAN_POINT('Ctrl Pts',(-18.2587594621295,10.7563025217825,123.050114944414)) ;
#26413=CARTESIAN_POINT('Ctrl Pts',(-18.0722565351528,10.9463521175027,122.715462501341)) ;
#26414=CARTESIAN_POINT('Ctrl Pts',(-18.3396629540108,10.7663630371399,122.854725296797)) ;
#26415=CARTESIAN_POINT('Ctrl Pts',(-18.2111793287984,10.9562014108898,122.497051143162)) ;
#26416=CARTESIAN_POINT('Ctrl Pts',(-18.4508020993981,10.7762123305269,122.679997778405)) ;
#26417=CARTESIAN_POINT('Ctrl Pts',(-18.388559678523,10.9662285865698,122.302199917963)) ;
#26418=CARTESIAN_POINT('Ctrl Pts',(-18.5927074978848,10.7862395062069,122.524117774987)) ;
#26419=CARTESIAN_POINT('Ctrl Pts',(-18.5975457775489,10.976257162197,122.141622604304)) ;
#26420=CARTESIAN_POINT('Ctrl Pts',(-18.7598974069773,10.7962680818341,122.395657172665)) ;
#26421=CARTESIAN_POINT('Ctrl Pts',(-18.8267122580128,10.9861022557429,122.021573575598)) ;
#26422=CARTESIAN_POINT('Ctrl Pts',(-18.9432305035226,10.80611317538,122.299619713947)) ;
#26423=CARTESIAN_POINT('Ctrl Pts',(-19.0767061726053,10.9960934971746,121.941311591283)) ;
#26424=CARTESIAN_POINT('Ctrl Pts',(-19.1432259108285,10.8161044168118,122.235411491827)) ;
#26425=CARTESIAN_POINT('Ctrl Pts',(-19.3380760888337,11.0061292783179,121.906059986019)) ;
#26426=CARTESIAN_POINT('Ctrl Pts',(-19.3523221423469,10.826140197955,122.20721167611)) ;
#26427=CARTESIAN_POINT('Ctrl Pts',(-19.5967752495355,11.0159814840476,121.916185579079)) ;
#26428=CARTESIAN_POINT('Ctrl Pts',(-19.5592805072898,10.8359924036847,122.215313538143)) ;
#26429=CARTESIAN_POINT('Ctrl Pts',(-19.8527735772293,11.0259435781646,121.970943280899)) ;
#26430=CARTESIAN_POINT('Ctrl Pts',(-19.7640785909624,10.8459544978017,122.259120868789)) ;
#26431=CARTESIAN_POINT('Ctrl Pts',(-20.0967309229679,11.0359661389917,122.070215768955)) ;
#26432=CARTESIAN_POINT('Ctrl Pts',(-19.9592439949302,10.8559770586288,122.338540107306)) ;
#26433=CARTESIAN_POINT('Ctrl Pts',(-20.3177943873502,11.0458939106433,122.208809071659)) ;
#26434=CARTESIAN_POINT('Ctrl Pts',(-20.1360936655196,10.8659048302804,122.449415566975)) ;
#26435=CARTESIAN_POINT('Ctrl Pts',(-20.513619210783,11.0559362947681,122.385690857822)) ;
#26436=CARTESIAN_POINT('Ctrl Pts',(-20.2927527608326,10.8759472144052,122.590922041084)) ;
#26437=CARTESIAN_POINT('Ctrl Pts',(-20.6733901753496,11.0658255188387,122.590674219405)) ;
#26438=CARTESIAN_POINT('Ctrl Pts',(-20.4205680784334,10.8858364384758,122.754908921902)) ;
#26439=CARTESIAN_POINT('Ctrl Pts',(-20.7967974985103,11.075814767006,122.822355021181)) ;
#26440=CARTESIAN_POINT('Ctrl Pts',(-20.5192928376293,10.8958256866432,122.940253955908)) ;
#26441=CARTESIAN_POINT('Ctrl Pts',(-20.8776639039544,11.085773344048,123.07124139589)) ;
#26442=CARTESIAN_POINT('Ctrl Pts',(-20.5839847120867,10.9057842636851,123.139363096927)) ;
#26443=CARTESIAN_POINT('Ctrl Pts',(-20.9145104547189,11.0956729131393,123.328785419539)) ;
#26444=CARTESIAN_POINT('Ctrl Pts',(-20.6134608083522,10.9156838327764,123.34539776855)) ;
#26445=CARTESIAN_POINT('Ctrl Pts',(-20.9058609614056,11.1057208252233,123.592665004876)) ;
#26446=CARTESIAN_POINT('Ctrl Pts',(-20.6065401309608,10.9257317448604,123.556501576119)) ;
#26447=CARTESIAN_POINT('Ctrl Pts',(-20.8525354819136,11.1156161795305,123.847220118537)) ;
#26448=CARTESIAN_POINT('Ctrl Pts',(-20.5638788889721,10.9356270991676,123.760144740549)) ;
#26449=CARTESIAN_POINT('Ctrl Pts',(-20.7542573598821,11.1256778300217,124.092654877015)) ;
#26450=CARTESIAN_POINT('Ctrl Pts',(-20.485255344439,10.9456887496588,123.95649240933)) ;
#26451=CARTESIAN_POINT('Ctrl Pts',(-20.6178768119318,11.1355224454842,124.31250491989)) ;
#26452=CARTESIAN_POINT('Ctrl Pts',(-20.3761506014328,10.9555333651213,124.132371010177)) ;
#26453=CARTESIAN_POINT('Ctrl Pts',(-20.4440816600714,11.1454825243856,124.508211665868)) ;
#26454=CARTESIAN_POINT('Ctrl Pts',(-20.2371141294296,10.9654934440227,124.288935606726)) ;
#26455=CARTESIAN_POINT('Ctrl Pts',(-20.2370227832588,11.1555207187439,124.671637321506)) ;
#26456=CARTESIAN_POINT('Ctrl Pts',(-20.0714663599296,10.9755316383811,124.419675493237)) ;
#26457=CARTESIAN_POINT('Ctrl Pts',(-20.0087297938616,11.1653944341435,124.795026404838)) ;
#26458=CARTESIAN_POINT('Ctrl Pts',(-19.8888323768802,10.9854053537807,124.518385630322)) ;
#26459=CARTESIAN_POINT('Ctrl Pts',(-19.7576006730884,11.1754661436778,124.87849507525)) ;
#26460=CARTESIAN_POINT('Ctrl Pts',(-19.6879285180809,10.9954770633149,124.585159904661)) ;
#26461=CARTESIAN_POINT('Ctrl Pts',(-19.5019775459593,11.1852985841303,124.916330182897)) ;
#26462=CARTESIAN_POINT('Ctrl Pts',(-19.4834310649531,11.0053095037674,124.61542705853)) ;
#26463=CARTESIAN_POINT('Ctrl Pts',(-19.2384391664689,11.1953304050557,124.909797495667)) ;
#26464=CARTESIAN_POINT('Ctrl Pts',(-19.2726002800821,11.0153413246928,124.610200312681)) ;
#26465=CARTESIAN_POINT('Ctrl Pts',(-18.9804733109709,11.2053507749413,124.856926970494)) ;
#26466=CARTESIAN_POINT('Ctrl Pts',(-19.0662277209886,11.0253616945784,124.567903126728)) ;
#26467=CARTESIAN_POINT('Ctrl Pts',(-18.7390964607104,11.215217546075,124.762178595596)) ;
#26468=CARTESIAN_POINT('Ctrl Pts',(-18.8731273657641,11.0352284657122,124.492104212861)) ;
#26469=CARTESIAN_POINT('Ctrl Pts',(-18.5133063352698,11.2252883172644,124.624178813688)) ;
#26470=CARTESIAN_POINT('Ctrl Pts',(-18.6924953042277,11.0452992369015,124.381703691916)) ;
#26471=CARTESIAN_POINT('Ctrl Pts',(-18.3193404016488,11.235131477786,124.453023478491)) ;
#26472=CARTESIAN_POINT('Ctrl Pts',(-18.5373238034759,11.0551423974231,124.24477971788)) ;
#26473=CARTESIAN_POINT('Ctrl Pts',(-18.1551353492722,11.2451117109724,124.248529269541)) ;
#26474=CARTESIAN_POINT('Ctrl Pts',(-18.4059602224555,11.0651226306096,124.081184300254)) ;
#26475=CARTESIAN_POINT('Ctrl Pts',(-18.028891195577,11.2551302310076,124.017503067163)) ;
#26476=CARTESIAN_POINT('Ctrl Pts',(-18.3049653496854,11.0751411506447,123.896363082341)) ;
#26477=CARTESIAN_POINT('Ctrl Pts',(-17.94527872475,11.2650135393913,123.771572840937)) ;
#26478=CARTESIAN_POINT('Ctrl Pts',(-18.2380760136292,11.0850244590284,123.699619611155)) ;
#26479=CARTESIAN_POINT('Ctrl Pts',(-17.9050223248742,11.2750818235621,123.510113552435)) ;
#26480=CARTESIAN_POINT('Ctrl Pts',(-18.2058712472604,11.0950927431992,123.490451793453)) ;
#26481=CARTESIAN_POINT('Ctrl Pts',(-17.9103370638304,11.2849119502298,123.251798025967)) ;
#26482=CARTESIAN_POINT('Ctrl Pts',(-18.2101233434264,11.1049228698669,123.283800611474)) ;
#26483=CARTESIAN_POINT('Ctrl Pts',(-17.9612752714376,11.2949785224363,122.992253063296)) ;
#26484=CARTESIAN_POINT('Ctrl Pts',(-18.2508742115829,11.1149894420734,123.07616437634)) ;
#26485=CARTESIAN_POINT('Ctrl Pts',(-18.0550114914209,11.304868678677,122.749806436418)) ;
#26486=CARTESIAN_POINT('Ctrl Pts',(-18.3258631525923,11.1248795983141,122.882207960884)) ;
#26487=CARTESIAN_POINT('Ctrl Pts',(-18.1902998279982,11.3148612062534,122.524765958901)) ;
#26488=CARTESIAN_POINT('Ctrl Pts',(-18.4340938564837,11.1348721258905,122.702175798357)) ;
#26489=CARTESIAN_POINT('Ctrl Pts',(-18.362252777776,11.3248226961277,122.327384835979)) ;
#26490=CARTESIAN_POINT('Ctrl Pts',(-18.57165612635,11.1448336157648,122.544271311536)) ;
#26491=CARTESIAN_POINT('Ctrl Pts',(-18.5644303505552,11.3347319180149,122.163249256382)) ;
#26492=CARTESIAN_POINT('Ctrl Pts',(-18.7333976447445,11.154742837652,122.412963346025)) ;
#26493=CARTESIAN_POINT('Ctrl Pts',(-18.7952595963488,11.3447804978252,122.035028175252)) ;
#26494=CARTESIAN_POINT('Ctrl Pts',(-18.9180612583401,11.1647914174624,122.310386442191)) ;
#26495=CARTESIAN_POINT('Ctrl Pts',(-19.0407305551564,11.3546634722953,121.950157334317)) ;
#26496=CARTESIAN_POINT('Ctrl Pts',(-19.1144372025468,11.1746743919324,122.242490108327)) ;
#26497=CARTESIAN_POINT('Ctrl Pts',(-19.3000011957523,11.364658383438,121.908176471057)) ;
#26498=CARTESIAN_POINT('Ctrl Pts',(-19.3218535588989,11.1846693030751,122.208905345717)) ;
#26499=CARTESIAN_POINT('Ctrl Pts',(-19.5633130308643,11.3746787700116,121.912223489131)) ;
#26500=CARTESIAN_POINT('Ctrl Pts',(-19.532503054688,11.1946896896487,122.212142961274)) ;
#26501=CARTESIAN_POINT('Ctrl Pts',(-19.8190707586081,11.3845888738687,121.961229817149)) ;
#26502=CARTESIAN_POINT('Ctrl Pts',(-19.7371085224044,11.2045997935058,122.251347849191)) ;
#26503=CARTESIAN_POINT('Ctrl Pts',(-20.0631345837218,11.3945165860786,122.053434027889)) ;
#26504=CARTESIAN_POINT('Ctrl Pts',(-19.9323591038037,11.2145275057157,122.325110807346)) ;
#26505=CARTESIAN_POINT('Ctrl Pts',(-20.2899581915959,11.4045596958458,122.18834359306)) ;
#26506=CARTESIAN_POINT('Ctrl Pts',(-20.1138182163407,11.2245706154829,122.433038412383)) ;
#26507=CARTESIAN_POINT('Ctrl Pts',(-20.4869200798739,11.4144461163014,122.357790944953)) ;
#26508=CARTESIAN_POINT('Ctrl Pts',(-20.2713871970456,11.2344570359385,122.568595575828)) ;
#26509=CARTESIAN_POINT('Ctrl Pts',(-20.653571934063,11.424439293907,122.560728657171)) ;
#26510=CARTESIAN_POINT('Ctrl Pts',(-20.4047088177741,11.2444502135441,122.730945421941)) ;
#26511=CARTESIAN_POINT('Ctrl Pts',(-20.7817631202176,11.4343849568109,122.788494689918)) ;
#26512=CARTESIAN_POINT('Ctrl Pts',(-20.5072617816881,11.254395876448,122.913157693448)) ;
#26513=CARTESIAN_POINT('Ctrl Pts',(-20.8689810112581,11.4443322530161,123.034933251578)) ;
#26514=CARTESIAN_POINT('Ctrl Pts',(-20.5770363372179,11.2643431726532,123.11030796952)) ;
#26515=CARTESIAN_POINT('Ctrl Pts',(-20.9122274632139,11.454380018594,123.295405142899)) ;
#26516=CARTESIAN_POINT('Ctrl Pts',(-20.611633872492,11.2743909382311,123.318685623006)) ;
#26517=CARTESIAN_POINT('Ctrl Pts',(-20.909847955661,11.4642282318116,123.554192250672)) ;
#26518=CARTESIAN_POINT('Ctrl Pts',(-20.6097306740805,11.2842391514487,123.525714196094)) ;
#26519=CARTESIAN_POINT('Ctrl Pts',(-20.8628861917845,11.4741878046057,123.811671085768)) ;
#26520=CARTESIAN_POINT('Ctrl Pts',(-20.5721619350103,11.2941987242428,123.731697005072)) ;
#26521=CARTESIAN_POINT('Ctrl Pts',(-20.7707963194684,11.4842244256382,124.058815012756)) ;
#26522=CARTESIAN_POINT('Ctrl Pts',(-20.4984904591295,11.3042353452753,123.929412437981)) ;
#26523=CARTESIAN_POINT('Ctrl Pts',(-20.6396015638057,11.4941049404486,124.282914554949)) ;
#26524=CARTESIAN_POINT('Ctrl Pts',(-20.3935356247347,11.3141158600857,124.108691603462)) ;
#26525=CARTESIAN_POINT('Ctrl Pts',(-20.4686789714687,11.5041575917556,124.484292270277)) ;
#26526=CARTESIAN_POINT('Ctrl Pts',(-20.2567978844015,11.3241685113927,124.26979434849)) ;
#26527=CARTESIAN_POINT('Ctrl Pts',(-20.2685707709031,11.5140529900356,124.650429772369)) ;
#26528=CARTESIAN_POINT('Ctrl Pts',(-20.0967123281824,11.3340639096727,124.402704356806)) ;
#26529=CARTESIAN_POINT('Ctrl Pts',(-20.0392516106828,11.5241031117417,124.781376915193)) ;
#26530=CARTESIAN_POINT('Ctrl Pts',(-19.9132571537407,11.3441140313788,124.50746276443)) ;
#26531=CARTESIAN_POINT('Ctrl Pts',(-19.794737934636,11.5339873912836,124.869107009898)) ;
#26532=CARTESIAN_POINT('Ctrl Pts',(-19.7176472402292,11.3539983109207,124.577647198776)) ;
#26533=CARTESIAN_POINT('Ctrl Pts',(-19.5359779545354,11.5439821725755,124.914016452958)) ;
#26534=CARTESIAN_POINT('Ctrl Pts',(-19.5106395508264,11.3639930922127,124.613575518455)) ;
#26535=CARTESIAN_POINT('Ctrl Pts',(-19.2745423776044,11.5539300177623,124.913217278818)) ;
#26536=CARTESIAN_POINT('Ctrl Pts',(-19.3014915210338,11.3739409373994,124.612936961295)) ;
#26537=CARTESIAN_POINT('Ctrl Pts',(-19.0174715357979,11.5638669811497,124.867467500935)) ;
#26538=CARTESIAN_POINT('Ctrl Pts',(-19.0958351968564,11.3838779007868,124.576338085747)) ;
#26539=CARTESIAN_POINT('Ctrl Pts',(-18.7709478903475,11.5738499458869,124.77765044511)) ;
#26540=CARTESIAN_POINT('Ctrl Pts',(-18.8986161489032,11.3938608655241,124.504485401762)) ;
#26541=CARTESIAN_POINT('Ctrl Pts',(-18.5426769439724,11.5838937973026,124.645205762056)) ;
#26542=CARTESIAN_POINT('Ctrl Pts',(-18.7159988423959,11.4039047169397,124.398530300539)) ;
#26543=CARTESIAN_POINT('Ctrl Pts',(-18.3447570490132,11.5937219986373,124.479210868658)) ;
#26544=CARTESIAN_POINT('Ctrl Pts',(-18.5576631821431,11.4137329182744,124.265735876442)) ;
#26545=CARTESIAN_POINT('Ctrl Pts',(-18.1744334770806,11.6037985712354,124.27652667465)) ;
#26546=CARTESIAN_POINT('Ctrl Pts',(-18.4214033306732,11.4238094908725,124.103588905207)) ;
#26547=CARTESIAN_POINT('Ctrl Pts',(-18.0446742700679,11.6136506512429,124.052422800966)) ;
#26548=CARTESIAN_POINT('Ctrl Pts',(-18.3175955633479,11.43366157088,123.924307178956)) ;
#26549=CARTESIAN_POINT('Ctrl Pts',(-17.9536271837052,11.623723936247,123.80390465869)) ;
#26550=CARTESIAN_POINT('Ctrl Pts',(-18.2447567627859,11.4437348558841,123.725492737883)) ;
#26551=CARTESIAN_POINT('Ctrl Pts',(-17.9082400349615,11.6335652879575,123.549277141686)) ;
#26552=CARTESIAN_POINT('Ctrl Pts',(-18.2084461725825,11.4535762075946,123.521791939049)) ;
#26553=CARTESIAN_POINT('Ctrl Pts',(-17.9067818389188,11.643526787354,123.287519099378)) ;
#26554=CARTESIAN_POINT('Ctrl Pts',(-18.2072783316507,11.4635377069911,123.312385832505)) ;
#26555=CARTESIAN_POINT('Ctrl Pts',(-17.951583816689,11.653562563484,123.027613430416)) ;
#26556=CARTESIAN_POINT('Ctrl Pts',(-18.2431187615393,11.4735734831211,123.104461008452)) ;
#26557=CARTESIAN_POINT('Ctrl Pts',(-18.0392630064654,11.6634509901216,122.782997517006)) ;
#26558=CARTESIAN_POINT('Ctrl Pts',(-18.3132606925425,11.4834619097587,122.908768552732)) ;
#26559=CARTESIAN_POINT('Ctrl Pts',(-18.169309686562,11.6734663121965,122.55416670281)) ;
#26560=CARTESIAN_POINT('Ctrl Pts',(-18.4172968626864,11.4934772318336,122.72570323888)) ;
#26561=CARTESIAN_POINT('Ctrl Pts',(-18.337832034103,11.6834966610967,122.351486710983)) ;
#26562=CARTESIAN_POINT('Ctrl Pts',(-18.5521138475697,11.5035075807338,122.563558413002)) ;
#26563=CARTESIAN_POINT('Ctrl Pts',(-18.5348954406339,11.6933400367034,122.18392868398)) ;
#26564=CARTESIAN_POINT('Ctrl Pts',(-18.7097629733351,11.5133509563405,122.429511607795)) ;
#26565=CARTESIAN_POINT('Ctrl Pts',(-18.7619871989816,11.7033694736005,122.05014873987)) ;
#26566=CARTESIAN_POINT('Ctrl Pts',(-18.8914356924309,11.5233803932376,122.322486374189)) ;
#26567=CARTESIAN_POINT('Ctrl Pts',(-19.0091747229,11.7134013515334,121.958483598159)) ;
#26568=CARTESIAN_POINT('Ctrl Pts',(-19.0891853235092,11.5334122711706,122.24915301597)) ;
#26569=CARTESIAN_POINT('Ctrl Pts',(-19.2631763810942,11.7232309746389,121.91157223852)) ;
#26570=CARTESIAN_POINT('Ctrl Pts',(-19.2923853954677,11.543241894276,122.211622724481)) ;
#26571=CARTESIAN_POINT('Ctrl Pts',(-19.5256800788775,11.733220445792,121.908654949481)) ;
#26572=CARTESIAN_POINT('Ctrl Pts',(-19.5023881948005,11.5532313654291,122.209287326421)) ;
#26573=CARTESIAN_POINT('Ctrl Pts',(-19.7859934259949,11.7432642945544,121.95225353693)) ;
#26574=CARTESIAN_POINT('Ctrl Pts',(-19.7106392257516,11.5632752141915,122.244164799925)) ;
#26575=CARTESIAN_POINT('Ctrl Pts',(-20.0294606191008,11.7530860000861,122.037936667196)) ;
#26576=CARTESIAN_POINT('Ctrl Pts',(-19.9054125518466,11.5730969197232,122.312709519324)) ;
#26577=CARTESIAN_POINT('Ctrl Pts',(-20.2595522204667,11.7631210399139,122.166778899388)) ;
#26578=CARTESIAN_POINT('Ctrl Pts',(-20.0894867189853,11.583131959551,122.415781895507)) ;
#26579=CARTESIAN_POINT('Ctrl Pts',(-20.4631137171743,11.7731457468054,122.334014058184)) ;
#26580=CARTESIAN_POINT('Ctrl Pts',(-20.2523368993887,11.5931566664425,122.549568855976)) ;
#26581=CARTESIAN_POINT('Ctrl Pts',(-20.6320140503155,11.7829984511461,122.530257519376)) ;
#26582=CARTESIAN_POINT('Ctrl Pts',(-20.3874578756258,11.6030093707832,122.706561953202)) ;
#26583=CARTESIAN_POINT('Ctrl Pts',(-20.7664764699797,11.7929865733538,122.755655719711)) ;
#26584=CARTESIAN_POINT('Ctrl Pts',(-20.4950292060904,11.6129974929909,122.886879510142)) ;
#26585=CARTESIAN_POINT('Ctrl Pts',(-20.8592244692304,11.8029150434611,122.999531121806)) ;
#26586=CARTESIAN_POINT('Ctrl Pts',(-20.5692290568483,11.6229259630982,123.081978836487)) ;
#26587=CARTESIAN_POINT('Ctrl Pts',(-20.9089464870837,11.8129040206283,123.257291767332)) ;
#26588=CARTESIAN_POINT('Ctrl Pts',(-20.609008398413,11.6329149402654,123.288186875209)) ;
#26589=CARTESIAN_POINT('Ctrl Pts',(-20.912726728438,11.822941827908,123.521040547069)) ;
#26590=CARTESIAN_POINT('Ctrl Pts',(-20.6120343028068,11.6429527475451,123.499185942152)) ;
#26591=CARTESIAN_POINT('Ctrl Pts',(-20.8718727620384,11.8327881287713,123.776548267499)) ;
#26592=CARTESIAN_POINT('Ctrl Pts',(-20.5793530040237,11.6527990484084,123.703591663681)) ;
#26593=CARTESIAN_POINT('Ctrl Pts',(-20.7862889531826,11.8428138721506,124.025729898005)) ;
#26594=CARTESIAN_POINT('Ctrl Pts',(-20.5108877193562,11.6628247917877,123.902937607542)) ;
#26595=CARTESIAN_POINT('Ctrl Pts',(-20.6580711492051,11.8528447385896,124.256054351195)) ;
#26596=CARTESIAN_POINT('Ctrl Pts',(-20.4083150016841,11.6728556582267,124.087198055119)) ;
#26597=CARTESIAN_POINT('Ctrl Pts',(-20.4954300469777,11.8626820973884,124.456984258248)) ;
#26598=CARTESIAN_POINT('Ctrl Pts',(-20.2782040287213,11.6826930170255,124.24794255801)) ;
#26599=CARTESIAN_POINT('Ctrl Pts',(-20.2977609080492,11.8726740583222,124.62982526479)) ;
#26600=CARTESIAN_POINT('Ctrl Pts',(-20.1200700801293,11.6926849779593,124.386216765177)) ;
#26601=CARTESIAN_POINT('Ctrl Pts',(-20.0718918884167,11.8827064208787,124.765820716401)) ;
#26602=CARTESIAN_POINT('Ctrl Pts',(-19.9393758049619,11.7027173405158,124.495014745963)) ;
#26603=CARTESIAN_POINT('Ctrl Pts',(-19.830074922632,11.8925715814531,124.859237594725)) ;
#26604=CARTESIAN_POINT('Ctrl Pts',(-19.7459234677896,11.7125825010902,124.569749829709)) ;
#26605=CARTESIAN_POINT('Ctrl Pts',(-19.5733413955139,11.9025334860308,124.910472534242)) ;
#26606=CARTESIAN_POINT('Ctrl Pts',(-19.5405372387899,11.7225444056679,124.610739722214)) ;
#26607=CARTESIAN_POINT('Ctrl Pts',(-19.3097054567228,11.9125684161065,124.915962853087)) ;
#26608=CARTESIAN_POINT('Ctrl Pts',(-19.3296285015763,11.7325793357437,124.615133939698)) ;
#26609=CARTESIAN_POINT('Ctrl Pts',(-19.0528979312036,11.9224533629601,124.876622619197)) ;
#26610=CARTESIAN_POINT('Ctrl Pts',(-19.1241826214947,11.7424642825973,124.583663814499)) ;
#26611=CARTESIAN_POINT('Ctrl Pts',(-18.8024198540435,11.9325190392716,124.791735612442)) ;
#26612=CARTESIAN_POINT('Ctrl Pts',(-18.9237994015907,11.7525299589087,124.515756076817)) ;
#26613=CARTESIAN_POINT('Ctrl Pts',(-18.5755065294971,11.9423579589065,124.667701912514)) ;
#26614=CARTESIAN_POINT('Ctrl Pts',(-18.7422682586687,11.7623688785436,124.416531178168)) ;
#26615=CARTESIAN_POINT('Ctrl Pts',(-18.3688173844643,11.9524214686409,124.502784044984)) ;
#26616=CARTESIAN_POINT('Ctrl Pts',(-18.576915561043,11.7724323882781,124.284598445225)) ;
#26617=CARTESIAN_POINT('Ctrl Pts',(-18.1969723593472,11.9623150818027,124.307637940785)) ;
#26618=CARTESIAN_POINT('Ctrl Pts',(-18.4394382482953,11.7823260014398,124.128483203739)) ;
#26619=CARTESIAN_POINT('Ctrl Pts',(-18.0603757685369,11.9722590886161,124.08490476088)) ;
#26620=CARTESIAN_POINT('Ctrl Pts',(-18.3301592733883,11.7922700082532,123.950297959954)) ;
#26621=CARTESIAN_POINT('Ctrl Pts',(-17.9638367967476,11.9822600429704,123.840420099808)) ;
#26622=CARTESIAN_POINT('Ctrl Pts',(-18.2529261323973,11.8022709626075,123.754711076634)) ;
#26623=CARTESIAN_POINT('Ctrl Pts',(-17.9114896578375,11.9922988006627,123.58188181945)) ;
#26624=CARTESIAN_POINT('Ctrl Pts',(-18.2110463657214,11.8123097202998,123.547880858099)) ;
#26625=CARTESIAN_POINT('Ctrl Pts',(-17.9044041219212,12.0021229848327,123.323787975382)) ;
#26626=CARTESIAN_POINT('Ctrl Pts',(-18.2053758050296,11.8221339044698,123.341406308645)) ;
#26627=CARTESIAN_POINT('Ctrl Pts',(-17.9427499485555,12.0121810504321,123.062292370625)) ;
#26628=CARTESIAN_POINT('Ctrl Pts',(-18.2360503193674,11.8321919700692,123.132209452442)) ;
#26629=CARTESIAN_POINT('Ctrl Pts',(-18.0251977237691,12.0221110972068,122.814691316201)) ;
#26630=CARTESIAN_POINT('Ctrl Pts',(-18.3020064298566,11.8421220168439,122.934128140568)) ;
#26631=CARTESIAN_POINT('Ctrl Pts',(-18.1490393731302,12.0320625395439,122.584356522223)) ;
#26632=CARTESIAN_POINT('Ctrl Pts',(-18.4010777391838,11.8520734591811,122.749859395245)) ;
#26633=CARTESIAN_POINT('Ctrl Pts',(-18.3128249788135,12.0421093367232,122.377284739554)) ;
#26634=CARTESIAN_POINT('Ctrl Pts',(-18.5321045207289,11.8621202563603,122.584200615192)) ;
#26635=CARTESIAN_POINT('Ctrl Pts',(-18.5060148098008,12.0519572774033,122.205087588693)) ;
#26636=CARTESIAN_POINT('Ctrl Pts',(-18.6866546893362,11.8719681970404,122.446441468451)) ;
#26637=CARTESIAN_POINT('Ctrl Pts',(-18.7282729224672,12.0619189087459,122.066794754727)) ;
#26638=CARTESIAN_POINT('Ctrl Pts',(-18.8644599124411,11.881929828383,122.335805352937)) ;
#26639=CARTESIAN_POINT('Ctrl Pts',(-18.9729503385559,12.0719475681218,121.968835081685)) ;
#26640=CARTESIAN_POINT('Ctrl Pts',(-19.0602009883113,11.8919584877589,122.257435568384)) ;
#26641=CARTESIAN_POINT('Ctrl Pts',(-19.227831787757,12.08185787101,121.915407496624)) ;
#26642=CARTESIAN_POINT('Ctrl Pts',(-19.2641055266912,11.9018687906471,122.214691356274)) ;
#26643=CARTESIAN_POINT('Ctrl Pts',(-19.4887612039821,12.0917927655722,121.906342273827)) ;
#26644=CARTESIAN_POINT('Ctrl Pts',(-19.472848876618,11.9118036852093,122.207436933983)) ;
#26645=CARTESIAN_POINT('Ctrl Pts',(-19.7500144690061,12.1018338642391,121.943349818059)) ;
#26646=CARTESIAN_POINT('Ctrl Pts',(-19.6818517658866,11.9218447838762,122.23704074526)) ;
#26647=CARTESIAN_POINT('Ctrl Pts',(-19.9971083719985,12.1117211467435,122.023739879768)) ;
#26648=CARTESIAN_POINT('Ctrl Pts',(-19.8795274617952,11.9317320663806,122.301350619632)) ;
#26649=CARTESIAN_POINT('Ctrl Pts',(-20.2290950029525,12.121712887254,122.146694306298)) ;
#26650=CARTESIAN_POINT('Ctrl Pts',(-20.0651177734983,11.9417238068911,122.399712142644)) ;
#26651=CARTESIAN_POINT('Ctrl Pts',(-20.4353231818005,12.1316634364894,122.307485013012)) ;
#26652=CARTESIAN_POINT('Ctrl Pts',(-20.230101643679,11.9516743561265,122.528342886444)) ;
#26653=CARTESIAN_POINT('Ctrl Pts',(-20.6105080303125,12.1415991141242,122.501068844292)) ;
#26654=CARTESIAN_POINT('Ctrl Pts',(-20.3702511605467,11.9616100337613,122.683208400421)) ;
#26655=CARTESIAN_POINT('Ctrl Pts',(-20.750371753253,12.151584531917,122.723117938316)) ;
#26656=CARTESIAN_POINT('Ctrl Pts',(-20.4821440178031,11.9715954515541,122.860846434547)) ;
#26657=CARTESIAN_POINT('Ctrl Pts',(-20.8496752814087,12.1616133247875,122.967237619846)) ;
#26658=CARTESIAN_POINT('Ctrl Pts',(-20.5615889029913,11.9816242444246,123.056141266303)) ;
#26659=CARTESIAN_POINT('Ctrl Pts',(-20.9045281450594,12.1714928360155,123.220996340645)) ;
#26660=CARTESIAN_POINT('Ctrl Pts',(-20.6054733938422,11.9915037556526,123.259147756982)) ;
#26661=CARTESIAN_POINT('Ctrl Pts',(-20.9152054113298,12.1814863726884,123.483408955597)) ;
#26662=CARTESIAN_POINT('Ctrl Pts',(-20.6140174445098,12.0014972923255,123.469077721808)) ;
#26663=CARTESIAN_POINT('Ctrl Pts',(-20.8794802827671,12.1915186409522,123.744603500789)) ;
#26664=CARTESIAN_POINT('Ctrl Pts',(-20.5854395864625,12.0115295605894,123.678033578765)) ;
#26665=CARTESIAN_POINT('Ctrl Pts',(-20.8008139737887,12.2013826029581,123.991621606298)) ;
#26666=CARTESIAN_POINT('Ctrl Pts',(-20.522508650298,12.0213935225952,123.875648805063)) ;
#26667=CARTESIAN_POINT('Ctrl Pts',(-20.678002189668,12.211452664303,124.225997440401)) ;
#26668=CARTESIAN_POINT('Ctrl Pts',(-20.4242612619508,12.0314635839401,124.063150402527)) ;
#26669=CARTESIAN_POINT('Ctrl Pts',(-20.5199833626838,12.2212950286517,124.430776031763)) ;
#26670=CARTESIAN_POINT('Ctrl Pts',(-20.2978478905724,12.0413059482889,124.22697474946)) ;
#26671=CARTESIAN_POINT('Ctrl Pts',(-20.327174746647,12.2312557011542,124.607803018266)) ;
#26672=CARTESIAN_POINT('Ctrl Pts',(-20.1436024451247,12.0512666207913,124.368597976752)) ;
#26673=CARTESIAN_POINT('Ctrl Pts',(-20.1045650508631,12.241293772222,124.749310160051)) ;
#26674=CARTESIAN_POINT('Ctrl Pts',(-19.9655159909283,12.0613046918591,124.48180549562)) ;
#26675=CARTESIAN_POINT('Ctrl Pts',(-19.8649051459857,12.2511673871824,124.84884392232)) ;
#26676=CARTESIAN_POINT('Ctrl Pts',(-19.7737886892284,12.0711783068196,124.561434593888)) ;
#26677=CARTESIAN_POINT('Ctrl Pts',(-19.6065797304044,12.2612396217637,124.906300997495)) ;
#26678=CARTESIAN_POINT('Ctrl Pts',(-19.5671291439869,12.0812505414008,124.607402358508)) ;
#26679=CARTESIAN_POINT('Ctrl Pts',(-19.3486297183306,12.2710636402125,124.918040759663)) ;
#26680=CARTESIAN_POINT('Ctrl Pts',(-19.3607684323741,12.0910745598496,124.616796316392)) ;
#26681=CARTESIAN_POINT('Ctrl Pts',(-19.0863456687476,12.2811285611885,124.884353810211)) ;
#26682=CARTESIAN_POINT('Ctrl Pts',(-19.1509427633031,12.1011394808256,124.589849001883)) ;
#26683=CARTESIAN_POINT('Ctrl Pts',(-18.7548496615759,12.2943388594833,124.781008020348)) ;
#26684=CARTESIAN_POINT('Ctrl Pts',(-18.8857366261165,12.1143497791204,124.507174493907)) ;
#26685=CARTESIAN_POINT('Ctrl Pts',(-18.4555083325038,12.3076543062152,124.592460114452)) ;
#26686=CARTESIAN_POINT('Ctrl Pts',(-18.646238230641,12.1276652258523,124.356312323164)) ;
#26687=CARTESIAN_POINT('Ctrl Pts',(-18.2182158984291,12.3209445514825,124.336043204847)) ;
#26688=CARTESIAN_POINT('Ctrl Pts',(-18.4564387255934,12.1409554711196,124.15121228678)) ;
#26689=CARTESIAN_POINT('Ctrl Pts',(-18.0753697674858,12.3309953010896,124.113946532571)) ;
#26690=CARTESIAN_POINT('Ctrl Pts',(-18.3421528585355,12.1510062207267,123.973529844557)) ;
#26691=CARTESIAN_POINT('Ctrl Pts',(-17.9751686262583,12.3408079080718,123.876303265546)) ;
#26692=CARTESIAN_POINT('Ctrl Pts',(-18.261991656828,12.160818827709,123.783417405138)) ;
#26693=CARTESIAN_POINT('Ctrl Pts',(-17.9159132713503,12.3508790060661,123.61839959421)) ;
#26694=CARTESIAN_POINT('Ctrl Pts',(-18.2145854546591,12.1708899257032,123.577093729689)) ;
#26695=CARTESIAN_POINT('Ctrl Pts',(-17.9028470180164,12.360768578841,123.358821518713)) ;
#26696=CARTESIAN_POINT('Ctrl Pts',(-18.2041287543014,12.1807794984781,123.369434895776)) ;
#26697=CARTESIAN_POINT('Ctrl Pts',(-17.9449900324593,12.3740386856443,123.012644489447)) ;
#26698=CARTESIAN_POINT('Ctrl Pts',(-18.2378495546872,12.1940496052814,123.092473752692)) ;
#26699=CARTESIAN_POINT('Ctrl Pts',(-18.1100382420715,12.3906553725668,122.603018959482)) ;
#26700=CARTESIAN_POINT('Ctrl Pts',(-18.3698647094851,12.2106662922039,122.764802568865)) ;
#26701=CARTESIAN_POINT('Ctrl Pts',(-18.403953809166,12.407229415883,122.274921978595)) ;
#26702=CARTESIAN_POINT('Ctrl Pts',(-18.6050396625321,12.2272403355201,122.502279805884)) ;
#26703=CARTESIAN_POINT('Ctrl Pts',(-18.6963080999561,12.4205259833148,122.083501484983)) ;
#26704=CARTESIAN_POINT('Ctrl Pts',(-18.838884457567,12.2405369029519,122.349174750329)) ;
#26705=CARTESIAN_POINT('Ctrl Pts',(-18.9385791929077,12.4305560468922,121.979673523522)) ;
#26706=CARTESIAN_POINT('Ctrl Pts',(-19.0327084258361,12.2505669665293,122.266104229579)) ;
#26707=CARTESIAN_POINT('Ctrl Pts',(-19.1916818709481,12.4404499387414,121.920281628208)) ;
#26708=CARTESIAN_POINT('Ctrl Pts',(-19.2351869221464,12.2604608583786,122.218590195066)) ;
#26709=CARTESIAN_POINT('Ctrl Pts',(-19.5394009792638,12.453702694527,121.899549493621)) ;
#26710=CARTESIAN_POINT('Ctrl Pts',(-19.5133723354866,12.2737136141641,122.202003998467)) ;
#26711=CARTESIAN_POINT('Ctrl Pts',(-19.9747293753154,12.4704307995194,121.989564308867)) ;
#26712=CARTESIAN_POINT('Ctrl Pts',(-19.8616245760486,12.2904417191566,122.274010791926)) ;
#26713=CARTESIAN_POINT('Ctrl Pts',(-20.423556659189,12.4902616359979,122.266069036656)) ;
#26714=CARTESIAN_POINT('Ctrl Pts',(-20.2206924545975,12.3102725556351,122.495213082915)) ;
#26715=CARTESIAN_POINT('Ctrl Pts',(-20.7535327226879,12.5101870278881,122.680135635484)) ;
#26716=CARTESIAN_POINT('Ctrl Pts',(-20.4846749563749,12.3301979475252,122.826464874533)) ;
#26717=CARTESIAN_POINT('Ctrl Pts',(-20.9224041261077,12.5301122412401,123.18215712058)) ;
#26718=CARTESIAN_POINT('Ctrl Pts',(-20.6197750512931,12.3501231608772,123.228081791924)) ;
#26719=CARTESIAN_POINT('Ctrl Pts',(-20.9099617273115,12.5500372547252,123.711523704258)) ;
#26720=CARTESIAN_POINT('Ctrl Pts',(-20.6098235773023,12.3700481743623,123.651575730201)) ;
#26721=CARTESIAN_POINT('Ctrl Pts',(-20.7187360422604,12.5699137264252,124.204018044716)) ;
#26722=CARTESIAN_POINT('Ctrl Pts',(-20.4568446351546,12.3899246460623,124.045573021246)) ;
#26723=CARTESIAN_POINT('Ctrl Pts',(-20.3693300643289,12.5898930443341,124.603877601687)) ;
#26724=CARTESIAN_POINT('Ctrl Pts',(-20.1773211406971,12.4099039639712,124.365462064758)) ;
#26725=CARTESIAN_POINT('Ctrl Pts',(-19.9052905888142,12.6098260479101,124.859582769263)) ;
#26726=CARTESIAN_POINT('Ctrl Pts',(-19.8060899284359,12.4298369675472,124.570028153243)) ;
#26727=CARTESIAN_POINT('Ctrl Pts',(-19.3829989743676,12.6297213179378,124.941977004567)) ;
#26728=CARTESIAN_POINT('Ctrl Pts',(-19.388255790433,12.4497322375749,124.635945220169)) ;
#26729=CARTESIAN_POINT('Ctrl Pts',(-18.8631060156455,12.6496426558436,124.841587523865)) ;
#26730=CARTESIAN_POINT('Ctrl Pts',(-18.9723403696999,12.4696535754807,124.555634564112)) ;
#26731=CARTESIAN_POINT('Ctrl Pts',(-18.4079042835162,12.6696002791098,124.569214868981)) ;
#26732=CARTESIAN_POINT('Ctrl Pts',(-18.6081780879779,12.4896111987469,124.337737060207)) ;
#26733=CARTESIAN_POINT('Ctrl Pts',(-18.0742532724176,12.689480111067,124.15962015315)) ;
#26734=CARTESIAN_POINT('Ctrl Pts',(-18.3412557256098,12.5094910307041,124.010060596195)) ;
#26735=CARTESIAN_POINT('Ctrl Pts',(-17.8989480657597,12.7093619623639,123.661012507451)) ;
#26736=CARTESIAN_POINT('Ctrl Pts',(-18.2010112129469,12.529372882001,123.611173006021)) ;
#26737=CARTESIAN_POINT('Ctrl Pts',(-17.9053743363839,12.7294329794677,123.127663535506)) ;
#26738=CARTESIAN_POINT('Ctrl Pts',(-18.206152086956,12.5494438991048,123.184494766924)) ;
#26739=CARTESIAN_POINT('Ctrl Pts',(-18.0909224032866,12.7492402032208,122.634900991628)) ;
#26740=CARTESIAN_POINT('Ctrl Pts',(-18.3545915317239,12.5692511228579,122.79028245245)) ;
#26741=CARTESIAN_POINT('Ctrl Pts',(-18.4354537167374,12.7692213387896,122.230824135122)) ;
#26742=CARTESIAN_POINT('Ctrl Pts',(-18.630217413786,12.5892322584267,122.467021418923)) ;
#26743=CARTESIAN_POINT('Ctrl Pts',(-18.8964641846084,12.7891488321288,121.970176160961)) ;
#26744=CARTESIAN_POINT('Ctrl Pts',(-18.9990268654917,12.6091597517659,122.258503153768)) ;
#26745=CARTESIAN_POINT('Ctrl Pts',(-19.415834432645,12.8089694934866,121.881151656097)) ;
#26746=CARTESIAN_POINT('Ctrl Pts',(-19.4145251819836,12.6289804131237,122.187284802725)) ;
#26747=CARTESIAN_POINT('Ctrl Pts',(-19.9411566590933,12.8290666827084,121.976780870031)) ;
#26748=CARTESIAN_POINT('Ctrl Pts',(-19.8347817388246,12.6490776023455,122.26378939332)) ;
#26749=CARTESIAN_POINT('Ctrl Pts',(-20.3952240684518,12.8488303617167,122.241384544964)) ;
#26750=CARTESIAN_POINT('Ctrl Pts',(-20.1980368260556,12.6688412813539,122.475474968688)) ;
#26751=CARTESIAN_POINT('Ctrl Pts',(-20.7368987004041,12.8688876403898,122.650278783027)) ;
#26752=CARTESIAN_POINT('Ctrl Pts',(-20.471374567732,12.6888985600269,122.802591330888)) ;
#26753=CARTESIAN_POINT('Ctrl Pts',(-20.915999998585,12.8886830641372,123.145136393717)) ;
#26754=CARTESIAN_POINT('Ctrl Pts',(-20.6146542216816,12.7086939837743,123.198479843696)) ;
#26755=CARTESIAN_POINT('Ctrl Pts',(-20.9171224626081,12.9086467088648,123.675675466344)) ;
#26756=CARTESIAN_POINT('Ctrl Pts',(-20.6155493596477,12.7286576285019,123.62291137376)) ;
#26757=CARTESIAN_POINT('Ctrl Pts',(-20.7357148689362,12.9286302001389,124.174870580485)) ;
#26758=CARTESIAN_POINT('Ctrl Pts',(-20.4704208498852,12.748641119776,124.022266714748)) ;
#26759=CARTESIAN_POINT('Ctrl Pts',(-20.3986521463145,12.9484376952882,124.579332558867)) ;
#26760=CARTESIAN_POINT('Ctrl Pts',(-20.2007674929157,12.7684486149253,124.345835452123)) ;
#26761=CARTESIAN_POINT('Ctrl Pts',(-19.9402235763069,12.9684202860083,124.847283742868)) ;
#26762=CARTESIAN_POINT('Ctrl Pts',(-19.8340229155712,12.7884312056454,124.560193612836)) ;
#26763=CARTESIAN_POINT('Ctrl Pts',(-19.4202416053834,12.9883029399995,124.942191223807)) ;
#26764=CARTESIAN_POINT('Ctrl Pts',(-19.4180360713643,12.8083138596367,124.636116448561)) ;
#26765=CARTESIAN_POINT('Ctrl Pts',(-18.8972653738817,13.0082611848626,124.854056149815)) ;
#26766=CARTESIAN_POINT('Ctrl Pts',(-18.9996554343786,12.8282721044997,124.565604873839)) ;
#26767=CARTESIAN_POINT('Ctrl Pts',(-18.4373467193133,13.0281367719042,124.594021898923)) ;
#26768=CARTESIAN_POINT('Ctrl Pts',(-18.6317218256589,12.8481476915413,124.357573939608)) ;
#26769=CARTESIAN_POINT('Ctrl Pts',(-18.0917408140289,13.0481176600395,124.190855292359)) ;
#26770=CARTESIAN_POINT('Ctrl Pts',(-18.355239878661,12.8681285796766,124.035038248343)) ;
#26771=CARTESIAN_POINT('Ctrl Pts',(-17.9052414355018,13.0680528011505,123.694844185524)) ;
#26772=CARTESIAN_POINT('Ctrl Pts',(-18.2060442903282,12.8880637207876,123.63822733448)) ;
#26773=CARTESIAN_POINT('Ctrl Pts',(-17.8988271166947,13.0879648191615,123.165702838927)) ;
#26774=CARTESIAN_POINT('Ctrl Pts',(-18.200915253109,12.9079757387987,123.21491552465)) ;
#26775=CARTESIAN_POINT('Ctrl Pts',(-18.072637630343,13.1078530374051,122.666485551976)) ;
#26776=CARTESIAN_POINT('Ctrl Pts',(-18.3399734826579,12.9278639570422,122.815536572551)) ;
#26777=CARTESIAN_POINT('Ctrl Pts',(-18.3508356377982,13.124451341252,122.324166060085)) ;
#26778=CARTESIAN_POINT('Ctrl Pts',(-18.562516670019,12.9444622608891,122.54170220006)) ;
#26779=CARTESIAN_POINT('Ctrl Pts',(-18.6332461345771,13.1377239311548,122.119417599801)) ;
#26780=CARTESIAN_POINT('Ctrl Pts',(-18.7884633789187,12.957734850792,122.37788874013)) ;
#26781=CARTESIAN_POINT('Ctrl Pts',(-18.8696106143661,13.1477313461057,122.004127651261)) ;
#26782=CARTESIAN_POINT('Ctrl Pts',(-18.9775498041114,12.9677422657428,122.285661949653)) ;
#26783=CARTESIAN_POINT('Ctrl Pts',(-19.1224757065835,13.1577386928383,121.931849416177)) ;
#26784=CARTESIAN_POINT('Ctrl Pts',(-19.1798541601348,12.9777496124754,122.22784121804)) ;
#26785=CARTESIAN_POINT('Ctrl Pts',(-19.4692111889447,13.1710050526399,121.895476582139)) ;
#26786=CARTESIAN_POINT('Ctrl Pts',(-19.4571883101494,12.991015972277,122.198742524881)) ;
#26787=CARTESIAN_POINT('Ctrl Pts',(-19.9027886653172,13.1875197102629,121.963391453896)) ;
#26788=CARTESIAN_POINT('Ctrl Pts',(-19.8041192330616,13.0075306299,122.253086454829)) ;
#26789=CARTESIAN_POINT('Ctrl Pts',(-20.2896179416635,13.2041171435055,122.175375538865)) ;
#26790=CARTESIAN_POINT('Ctrl Pts',(-20.1135332169725,13.0241280631426,122.422657930658)) ;
#26791=CARTESIAN_POINT('Ctrl Pts',(-20.5428541366256,13.2174651406505,122.418153018463)) ;
#26792=CARTESIAN_POINT('Ctrl Pts',(-20.3161488901095,13.0374760602876,122.61689817093)) ;
#26793=CARTESIAN_POINT('Ctrl Pts',(-20.6967627804406,13.2273608950021,122.62776755716)) ;
#26794=CARTESIAN_POINT('Ctrl Pts',(-20.4392682594011,13.0473718146392,122.784587934019)) ;
#26795=CARTESIAN_POINT('Ctrl Pts',(-20.8132896637095,13.2373488489335,122.862934128972)) ;
#26796=CARTESIAN_POINT('Ctrl Pts',(-20.5324892841562,13.0573597685706,122.972723020215)) ;
#26797=CARTESIAN_POINT('Ctrl Pts',(-20.887111769064,13.2473060726382,123.114002366625)) ;
#26798=CARTESIAN_POINT('Ctrl Pts',(-20.591544390908,13.0673169922753,123.17357799442)) ;
#26799=CARTESIAN_POINT('Ctrl Pts',(-20.9163194697392,13.2573416191949,123.376085199788)) ;
#26800=CARTESIAN_POINT('Ctrl Pts',(-20.6149084219131,13.077352538832,123.383244498507)) ;
#26801=CARTESIAN_POINT('Ctrl Pts',(-20.9000197111728,13.267228730471,123.635413520908)) ;
#26802=CARTESIAN_POINT('Ctrl Pts',(-20.6018663387177,13.0872396501081,123.590707013406)) ;
#26803=CARTESIAN_POINT('Ctrl Pts',(-20.8387093067046,13.2772201355718,123.890705618829)) ;
#26804=CARTESIAN_POINT('Ctrl Pts',(-20.5528158398965,13.0972310552089,123.794940111806)) ;
#26805=CARTESIAN_POINT('Ctrl Pts',(-20.7344045824693,13.2871657567866,124.130350209159)) ;
#26806=CARTESIAN_POINT('Ctrl Pts',(-20.4693700045889,13.1071766764237,123.986654845543)) ;
#26807=CARTESIAN_POINT('Ctrl Pts',(-20.5904556480587,13.2971150050549,124.348628887742)) ;
#26808=CARTESIAN_POINT('Ctrl Pts',(-20.3542090074305,13.117125924692,124.161276491165)) ;
#26809=CARTESIAN_POINT('Ctrl Pts',(-20.4088310489179,13.3071615002235,124.540222615066)) ;
#26810=CARTESIAN_POINT('Ctrl Pts',(-20.208907719291,13.1271724198607,124.314549885357)) ;
#26811=CARTESIAN_POINT('Ctrl Pts',(-20.2009526790891,13.3170128430151,124.69453910851)) ;
#26812=CARTESIAN_POINT('Ctrl Pts',(-20.0426037537448,13.1370237626522,124.438001210113)) ;
#26813=CARTESIAN_POINT('Ctrl Pts',(-19.9669434550335,13.3269846231424,124.812406349802)) ;
#26814=CARTESIAN_POINT('Ctrl Pts',(-19.85539544562,13.1469955427795,124.532292952135)) ;
#26815=CARTESIAN_POINT('Ctrl Pts',(-19.7153564891379,13.3369798231201,124.888022808457)) ;
#26816=CARTESIAN_POINT('Ctrl Pts',(-19.6541252878157,13.1569907427572,124.592783951486)) ;
#26817=CARTESIAN_POINT('Ctrl Pts',(-19.4534753611638,13.3470138148161,124.918598821052)) ;
#26818=CARTESIAN_POINT('Ctrl Pts',(-19.4446201537456,13.1670247344533,124.617242515926)) ;
#26819=CARTESIAN_POINT('Ctrl Pts',(-19.1948766730221,13.3568692197886,124.903920505576)) ;
#26820=CARTESIAN_POINT('Ctrl Pts',(-19.2377415186523,13.1768801394258,124.605497635822)) ;
#26821=CARTESIAN_POINT('Ctrl Pts',(-18.9390603846793,13.3668685176344,124.844062381727)) ;
#26822=CARTESIAN_POINT('Ctrl Pts',(-19.0330890674642,13.1868794372715,124.557608978315)) ;
#26823=CARTESIAN_POINT('Ctrl Pts',(-18.6998481883594,13.3767636302396,124.741995186928)) ;
#26824=CARTESIAN_POINT('Ctrl Pts',(-18.8417203716604,13.1967745498767,124.475953269536)) ;
#26825=CARTESIAN_POINT('Ctrl Pts',(-18.4784292945889,13.3868242757746,124.597585675323)) ;
#26826=CARTESIAN_POINT('Ctrl Pts',(-18.6645864484423,13.2068351954117,124.360423788125)) ;
#26827=CARTESIAN_POINT('Ctrl Pts',(-18.2893688821215,13.3966731527638,124.420799145494)) ;
#26828=CARTESIAN_POINT('Ctrl Pts',(-18.5133398551408,13.2166840724009,124.218993165454)) ;
#26829=CARTESIAN_POINT('Ctrl Pts',(-18.1305208053495,13.4067018638574,124.210511784196)) ;
#26830=CARTESIAN_POINT('Ctrl Pts',(-18.3862631410708,13.2267127834945,124.050761997541)) ;
#26831=CARTESIAN_POINT('Ctrl Pts',(-18.0112247910287,13.4167312651135,123.975488167396)) ;
#26832=CARTESIAN_POINT('Ctrl Pts',(-18.2908283055355,13.2367421847506,123.862742104803)) ;
#26833=CARTESIAN_POINT('Ctrl Pts',(-17.9354445009214,13.4265714569095,123.72824647118)) ;
#26834=CARTESIAN_POINT('Ctrl Pts',(-18.2302062650651,13.2465823765466,123.664948483144)) ;
#26835=CARTESIAN_POINT('Ctrl Pts',(-17.9027395319079,13.4365748861025,123.467435684465)) ;
#26836=CARTESIAN_POINT('Ctrl Pts',(-18.2040444166883,13.2565858057396,123.456299663574)) ;
#26837=CARTESIAN_POINT('Ctrl Pts',(-17.9158814573718,13.4465603985687,123.205311390375)) ;
#26838=CARTESIAN_POINT('Ctrl Pts',(-18.2145600879431,13.2665713182058,123.24660043712)) ;
#26839=CARTESIAN_POINT('Ctrl Pts',(-17.9749065837832,13.4566014949527,122.948155155583)) ;
#26840=CARTESIAN_POINT('Ctrl Pts',(-18.2617823053095,13.2766124145898,123.040875912254)) ;
#26841=CARTESIAN_POINT('Ctrl Pts',(-18.0753470360815,13.4664446909037,122.709757985454)) ;
#26842=CARTESIAN_POINT('Ctrl Pts',(-18.3421364530239,13.2864556105408,122.850159423479)) ;
#26843=CARTESIAN_POINT('Ctrl Pts',(-18.217218281521,13.4764310019581,122.489035231126)) ;
#26844=CARTESIAN_POINT('Ctrl Pts',(-18.455635132101,13.2964419215952,122.673582454515)) ;
#26845=CARTESIAN_POINT('Ctrl Pts',(-18.3942732512551,13.4863656872158,122.297106419642)) ;
#26846=CARTESIAN_POINT('Ctrl Pts',(-18.5972804423146,13.3063766068529,122.520040993049)) ;
#26847=CARTESIAN_POINT('Ctrl Pts',(-18.6046031877743,13.4964232484328,122.137116873894)) ;
#26848=CARTESIAN_POINT('Ctrl Pts',(-18.7655457306992,13.31643416807,122.392050961701)) ;
#26849=CARTESIAN_POINT('Ctrl Pts',(-18.8338850495127,13.5062448900414,122.018535713195)) ;
#26850=CARTESIAN_POINT('Ctrl Pts',(-18.9489715980104,13.3262558096786,122.297188133943)) ;
#26851=CARTESIAN_POINT('Ctrl Pts',(-19.0859583258846,13.5163009536324,121.939273611562)) ;
#26852=CARTESIAN_POINT('Ctrl Pts',(-19.1506308986353,13.3363118732695,122.233780316748)) ;
#26853=CARTESIAN_POINT('Ctrl Pts',(-19.3450516698222,13.5262416293942,121.905839973782)) ;
#26854=CARTESIAN_POINT('Ctrl Pts',(-19.3579055692691,13.3462525490313,122.207035465221)) ;
#26855=CARTESIAN_POINT('Ctrl Pts',(-19.6050909750196,13.5361459881825,121.917041144644)) ;
#26856=CARTESIAN_POINT('Ctrl Pts',(-19.565936503742,13.3561569078197,122.215998316432)) ;
#26857=CARTESIAN_POINT('Ctrl Pts',(-19.862825851585,13.5461926427583,121.97418792217)) ;
#26858=CARTESIAN_POINT('Ctrl Pts',(-19.7721240620941,13.3662035623955,122.261717666906)) ;
#26859=CARTESIAN_POINT('Ctrl Pts',(-20.1031997643857,13.5560882374012,122.073508487898)) ;
#26860=CARTESIAN_POINT('Ctrl Pts',(-19.9644220277355,13.3760991570383,122.341175720192)) ;
#26861=CARTESIAN_POINT('Ctrl Pts',(-20.3263218440362,13.5661501840581,122.215343672236)) ;
#26862=CARTESIAN_POINT('Ctrl Pts',(-20.1429187779707,13.3861611036952,122.454645564345)) ;
#26863=CARTESIAN_POINT('Ctrl Pts',(-20.5173749645332,13.5759998079902,122.38999462014)) ;
#26864=CARTESIAN_POINT('Ctrl Pts',(-20.295759491306,13.3960107276274,122.594367286313)) ;
#26865=CARTESIAN_POINT('Ctrl Pts',(-20.6776884554839,13.5859630470201,122.596980439567)) ;
#26866=CARTESIAN_POINT('Ctrl Pts',(-20.4240087199095,13.4059739666572,122.759956837706)) ;
#26867=CARTESIAN_POINT('Ctrl Pts',(-20.8000704181908,13.5959876217959,122.830280403309)) ;
#26868=CARTESIAN_POINT('Ctrl Pts',(-20.5219126738478,13.415998541433,122.946597684399)) ;
#26869=CARTESIAN_POINT('Ctrl Pts',(-20.8793920083737,13.6059061844836,123.07855998187)) ;
#26870=CARTESIAN_POINT('Ctrl Pts',(-20.5853680842003,13.4259171041207,123.145221485307)) ;
#26871=CARTESIAN_POINT('Ctrl Pts',(-20.9151199375489,13.6158983712076,123.338717822216)) ;
#26872=CARTESIAN_POINT('Ctrl Pts',(-20.6139486858676,13.4359092908447,123.353347860863)) ;
#26873=CARTESIAN_POINT('Ctrl Pts',(-20.9046168525977,13.6259331697918,123.6022019633)) ;
#26874=CARTESIAN_POINT('Ctrl Pts',(-20.605544399225,13.4459440894289,123.564135168279)) ;
#26875=CARTESIAN_POINT('Ctrl Pts',(-20.8499556627768,13.6357883604655,123.855372966742)) ;
#26876=CARTESIAN_POINT('Ctrl Pts',(-20.5618138995585,13.4557992801026,123.766670884377)) ;
#26877=CARTESIAN_POINT('Ctrl Pts',(-20.7510855573927,13.6457877086185,124.098788324435)) ;
#26878=CARTESIAN_POINT('Ctrl Pts',(-20.4827162949927,13.4657986282556,123.961402436991)) ;
#26879=CARTESIAN_POINT('Ctrl Pts',(-20.6130996723433,13.6556828342936,124.319242233489)) ;
#26880=CARTESIAN_POINT('Ctrl Pts',(-20.3723265173656,13.4756937539307,124.137764200893)) ;
#26881=CARTESIAN_POINT('Ctrl Pts',(-20.4360519660016,13.6657433772417,124.515540628893)) ;
#26882=CARTESIAN_POINT('Ctrl Pts',(-20.2306870063593,13.4857542968788,124.294801963191)) ;
#26883=CARTESIAN_POINT('Ctrl Pts',(-20.2320341456861,13.6755926515086,124.674850714962)) ;
#26884=CARTESIAN_POINT('Ctrl Pts',(-20.0674724171004,13.4956035711457,124.422248249584)) ;
#26885=CARTESIAN_POINT('Ctrl Pts',(-19.9996623311131,13.6856198760785,124.799086161189)) ;
#26886=CARTESIAN_POINT('Ctrl Pts',(-19.8815742380617,13.5056307957156,124.521635311594)) ;
#26887=CARTESIAN_POINT('Ctrl Pts',(-19.7489854254844,13.6956482752663,124.880448501815)) ;
#26888=CARTESIAN_POINT('Ctrl Pts',(-19.6810321616281,13.5156591949034,124.586723663228)) ;
#26889=CARTESIAN_POINT('Ctrl Pts',(-19.4928401900497,13.7054940256798,124.916853671087)) ;
#26890=CARTESIAN_POINT('Ctrl Pts',(-19.4761166444092,13.5255049453169,124.615846163914)) ;
#26891=CARTESIAN_POINT('Ctrl Pts',(-19.230454887784,13.7154828160805,124.908839488335)) ;
#26892=CARTESIAN_POINT('Ctrl Pts',(-19.2662086080236,13.5354937357177,124.609433445062)) ;
#26893=CARTESIAN_POINT('Ctrl Pts',(-18.9721627761797,13.7255277444802,124.854438840815)) ;
#26894=CARTESIAN_POINT('Ctrl Pts',(-19.0595750986044,13.5455386641174,124.565911420256)) ;
#26895=CARTESIAN_POINT('Ctrl Pts',(-18.7323658376547,13.7353522292692,124.758724681303)) ;
#26896=CARTESIAN_POINT('Ctrl Pts',(-18.8677390346098,13.5553631489063,124.489339193207)) ;
#26897=CARTESIAN_POINT('Ctrl Pts',(-18.507457139982,13.7454096268104,124.619951807237)) ;
#26898=CARTESIAN_POINT('Ctrl Pts',(-18.6878125850875,13.5654205464475,124.378319667226)) ;
#26899=CARTESIAN_POINT('Ctrl Pts',(-18.3128349524813,13.7553357183966,124.44624656969)) ;
#26900=CARTESIAN_POINT('Ctrl Pts',(-18.5321161260099,13.5753466380337,124.239354778128)) ;
#26901=CARTESIAN_POINT('Ctrl Pts',(-18.1503452309715,13.7652905035412,124.241231958245)) ;
#26902=CARTESIAN_POINT('Ctrl Pts',(-18.4021255453027,13.5853014231783,124.075342601526)) ;
#26903=CARTESIAN_POINT('Ctrl Pts',(-18.0251465109341,13.7753278731988,124.009068223143)) ;
#26904=CARTESIAN_POINT('Ctrl Pts',(-18.3019676694534,13.5953387928359,123.889610906895)) ;
#26905=CARTESIAN_POINT('Ctrl Pts',(-17.9431959784106,13.7852166833204,123.762452941019)) ;
#26906=CARTESIAN_POINT('Ctrl Pts',(-18.2364086692508,13.6052276029575,123.692318981433)) ;
#26907=CARTESIAN_POINT('Ctrl Pts',(-17.9044614031139,13.7952060423715,123.502822293364)) ;
#26908=CARTESIAN_POINT('Ctrl Pts',(-18.2054221786113,13.6152169620086,123.484614462953)) ;
#26909=CARTESIAN_POINT('Ctrl Pts',(-17.9115693386521,13.8051645898276,123.241226463732)) ;
#26910=CARTESIAN_POINT('Ctrl Pts',(-18.2111097180374,13.6251755094647,123.275338178328)) ;
#26911=CARTESIAN_POINT('Ctrl Pts',(-17.9630567197968,13.8150641663786,122.986205100608)) ;
#26912=CARTESIAN_POINT('Ctrl Pts',(-18.2523005182494,13.6350750860157,123.071321986717)) ;
#26913=CARTESIAN_POINT('Ctrl Pts',(-18.0595361492998,13.8251120782093,122.740443216478)) ;
#26914=CARTESIAN_POINT('Ctrl Pts',(-18.329485128724,13.6451229978464,122.874712710548)) ;
#26915=CARTESIAN_POINT('Ctrl Pts',(-18.1949930036132,13.8350074260699,122.518422190268)) ;
#26916=CARTESIAN_POINT('Ctrl Pts',(-18.4378511109109,13.655018345707,122.697097049966)) ;
#26917=CARTESIAN_POINT('Ctrl Pts',(-18.3697572977927,13.845069102601,122.320042659935)) ;
#26918=CARTESIAN_POINT('Ctrl Pts',(-18.5776634866624,13.6650800222382,122.538393906198)) ;
#26919=CARTESIAN_POINT('Ctrl Pts',(-18.5718588198519,13.8549136203502,122.158525512922)) ;
#26920=CARTESIAN_POINT('Ctrl Pts',(-18.7393445112275,13.6749245399873,122.409181641225)) ;
#26921=CARTESIAN_POINT('Ctrl Pts',(-18.8011469810602,13.864874064065,122.032284729829)) ;
#26922=CARTESIAN_POINT('Ctrl Pts',(-18.9227751038679,13.6848849837021,122.308189886519)) ;
#26923=CARTESIAN_POINT('Ctrl Pts',(-19.0509301231226,13.8749108968832,121.947590007007)) ;
#26924=CARTESIAN_POINT('Ctrl Pts',(-19.1226020288338,13.6949218165203,122.240434931693)) ;
#26925=CARTESIAN_POINT('Ctrl Pts',(-19.3074865101994,13.88478969363,121.907757156992)) ;
#26926=CARTESIAN_POINT('Ctrl Pts',(-19.3278463927919,13.7048006132671,122.208569584531)) ;
#26927=CARTESIAN_POINT('Ctrl Pts',(-19.5717537455678,13.8948490097584,121.91308802529)) ;
#26928=CARTESIAN_POINT('Ctrl Pts',(-19.5392604248098,13.7148599293955,122.212835072421)) ;
#26929=CARTESIAN_POINT('Ctrl Pts',(-19.8262549511952,13.9047194565116,121.963266910915)) ;
#26930=CARTESIAN_POINT('Ctrl Pts',(-19.7428603300386,13.7247303761487,122.252978777756)) ;
#26931=CARTESIAN_POINT('Ctrl Pts',(-20.0714142577279,13.9147120947696,122.057363864517)) ;
#26932=CARTESIAN_POINT('Ctrl Pts',(-19.9389874113429,13.7347230144067,122.328256860103)) ;
#26933=CARTESIAN_POINT('Ctrl Pts',(-20.2970965036502,13.9247441103175,122.193613633218)) ;
#26934=CARTESIAN_POINT('Ctrl Pts',(-20.1195328981886,13.7447550299547,122.437257373362)) ;
#26935=CARTESIAN_POINT('Ctrl Pts',(-20.4928009018349,13.9346099666241,122.363706237578)) ;
#26936=CARTESIAN_POINT('Ctrl Pts',(-20.2760952675698,13.7546208862612,122.573331276944)) ;
#26937=CARTESIAN_POINT('Ctrl Pts',(-20.6593476164435,13.9446792560932,122.569291069351)) ;
#26938=CARTESIAN_POINT('Ctrl Pts',(-20.4093323747788,13.7646901757304,122.737799786026)) ;
#26939=CARTESIAN_POINT('Ctrl Pts',(-20.7848399902421,13.9545228136445,122.795508554596)) ;
#26940=CARTESIAN_POINT('Ctrl Pts',(-20.509725196703,13.7745337332817,122.91877307958)) ;
#26941=CARTESIAN_POINT('Ctrl Pts',(-20.871120064522,13.9645029404324,123.043168459414)) ;
#26942=CARTESIAN_POINT('Ctrl Pts',(-20.578748805291,13.7845138600695,123.116900896814)) ;
#26943=CARTESIAN_POINT('Ctrl Pts',(-20.9127502836893,13.9745214890323,123.303126129535)) ;
#26944=CARTESIAN_POINT('Ctrl Pts',(-20.6120524706176,13.7945324086694,123.324867123436)) ;
#26945=CARTESIAN_POINT('Ctrl Pts',(-20.9092186327094,13.9844047895555,123.562857078074)) ;
#26946=CARTESIAN_POINT('Ctrl Pts',(-20.609226783806,13.8044157091926,123.532650998994)) ;
#26947=CARTESIAN_POINT('Ctrl Pts',(-20.8596340362664,13.9944730766036,123.822708783211)) ;
#26948=CARTESIAN_POINT('Ctrl Pts',(-20.5695586439728,13.8144839962408,123.740532609343)) ;
#26949=CARTESIAN_POINT('Ctrl Pts',(-20.7681595371697,14.0043031996223,124.064344085627)) ;
#26950=CARTESIAN_POINT('Ctrl Pts',(-20.4963791721871,13.8243141192594,123.933839581481)) ;
#26951=CARTESIAN_POINT('Ctrl Pts',(-20.6332814623007,14.0143697835476,124.291865630646)) ;
#26952=CARTESIAN_POINT('Ctrl Pts',(-20.3884763385761,13.8343807031847,124.11585696606)) ;
#26953=CARTESIAN_POINT('Ctrl Pts',(-20.4637992773007,14.0242598965621,124.488951781943)) ;
#26954=CARTESIAN_POINT('Ctrl Pts',(-20.2528909214938,13.8442708161992,124.273525063999)) ;
#26955=CARTESIAN_POINT('Ctrl Pts',(-20.2609821100153,14.0342525853247,124.655717889191)) ;
#26956=CARTESIAN_POINT('Ctrl Pts',(-20.090637223389,13.8542635049618,124.406937730911)) ;
#26957=CARTESIAN_POINT('Ctrl Pts',(-20.0328972096088,14.0442134736805,124.784181661414)) ;
#26958=CARTESIAN_POINT('Ctrl Pts',(-19.9081695446619,13.8642243933176,124.509708392774)) ;
#26959=CARTESIAN_POINT('Ctrl Pts',(-19.7872119388903,14.0541314185605,124.87112949854)) ;
#26960=CARTESIAN_POINT('Ctrl Pts',(-19.7116219327022,13.8741423381976,124.579266367016)) ;
#26961=CARTESIAN_POINT('Ctrl Pts',(-19.527842932523,14.0641391716567,124.914794637581)) ;
#26962=CARTESIAN_POINT('Ctrl Pts',(-19.5041267743093,13.8841500912938,124.614198467582)) ;
#26963=CARTESIAN_POINT('Ctrl Pts',(-19.2642632651857,14.0741702656157,124.912222739613)) ;
#26964=CARTESIAN_POINT('Ctrl Pts',(-19.2932629428853,13.8941811852529,124.612140811124)) ;
#26965=CARTESIAN_POINT('Ctrl Pts',(-19.0097259981526,14.0840182336437,124.865371406458)) ;
#26966=CARTESIAN_POINT('Ctrl Pts',(-19.0896342385044,13.9040291532808,124.57465995883)) ;
#26967=CARTESIAN_POINT('Ctrl Pts',(-18.7618772164016,14.0940801897696,124.773301901415)) ;
#26968=CARTESIAN_POINT('Ctrl Pts',(-18.89135492329,13.9140911094067,124.501004319296)) ;
#26969=CARTESIAN_POINT('Ctrl Pts',(-18.5376101429091,14.1039774013707,124.641559789166)) ;
#26970=CARTESIAN_POINT('Ctrl Pts',(-18.7119419501136,13.9239883210078,124.395611039838)) ;
#26971=CARTESIAN_POINT('Ctrl Pts',(-18.3384000135968,14.1139085680353,124.472965869001)) ;
#26972=CARTESIAN_POINT('Ctrl Pts',(-18.5525741413936,13.9339194876725,124.26073644889)) ;
#26973=CARTESIAN_POINT('Ctrl Pts',(-18.169843513441,14.1239507522395,124.269917095288)) ;
#26974=CARTESIAN_POINT('Ctrl Pts',(-18.4177287173971,13.9439616718766,124.098297399059)) ;
#26975=CARTESIAN_POINT('Ctrl Pts',(-18.0409566998773,14.1338374204927,124.044314253981)) ;
#26976=CARTESIAN_POINT('Ctrl Pts',(-18.3146195241724,13.9538483401298,123.91781597991)) ;
#26977=CARTESIAN_POINT('Ctrl Pts',(-17.9518498698231,14.1438305324709,123.797299870393)) ;
#26978=CARTESIAN_POINT('Ctrl Pts',(-18.2433338227016,13.963841452108,123.720204732081)) ;
#26979=CARTESIAN_POINT('Ctrl Pts',(-17.9072936184703,14.1537762100867,123.539763194409)) ;
#26980=CARTESIAN_POINT('Ctrl Pts',(-18.2076886217236,13.9737871297239,123.514175908959)) ;
#26981=CARTESIAN_POINT('Ctrl Pts',(-17.9075982211722,14.1637235130717,123.278346044345)) ;
#26982=CARTESIAN_POINT('Ctrl Pts',(-18.2079318833263,13.9837344327088,123.305042647858)) ;
#26983=CARTESIAN_POINT('Ctrl Pts',(-17.9540338467725,14.1737712368185,123.018424649771)) ;
#26984=CARTESIAN_POINT('Ctrl Pts',(-18.245080078658,13.9937821564556,123.097105274778)) ;
#26985=CARTESIAN_POINT('Ctrl Pts',(-18.0429036250617,14.183619610581,122.775359841272)) ;
#26986=CARTESIAN_POINT('Ctrl Pts',(-18.3161751445601,14.0036305302181,122.90265434045)) ;
#26987=CARTESIAN_POINT('Ctrl Pts',(-18.1733306008267,14.1935785830267,122.54846390798)) ;
#26988=CARTESIAN_POINT('Ctrl Pts',(-18.4205160052355,14.0135895026638,122.721137613016)) ;
#26989=CARTESIAN_POINT('Ctrl Pts',(-18.3428801887918,14.2036174449079,122.346364098552)) ;
#26990=CARTESIAN_POINT('Ctrl Pts',(-18.5561553752817,14.023628364545,122.559457349719)) ;
#26991=CARTESIAN_POINT('Ctrl Pts',(-18.5414813532127,14.2134960490797,122.179140432255)) ;
#26992=CARTESIAN_POINT('Ctrl Pts',(-18.7150352359828,14.0335069687168,122.425678533261)) ;
#26993=CARTESIAN_POINT('Ctrl Pts',(-18.7699215575239,14.223547590283,122.046595739492)) ;
#26994=CARTESIAN_POINT('Ctrl Pts',(-18.8977872771299,14.0435585099201,122.319642127634)) ;
#26995=CARTESIAN_POINT('Ctrl Pts',(-19.0141015690712,14.2334429882633,121.957035255779)) ;
#26996=CARTESIAN_POINT('Ctrl Pts',(-19.0931303423171,14.0534539079004,122.247993398259)) ;
#26997=CARTESIAN_POINT('Ctrl Pts',(-19.2740491001981,14.2434942208086,121.910385335695)) ;
#26998=CARTESIAN_POINT('Ctrl Pts',(-19.3010884541272,14.0635051404457,122.210672757379)) ;
#26999=CARTESIAN_POINT('Ctrl Pts',(-19.5338747027506,14.2533804114329,121.909562985904)) ;
#27000=CARTESIAN_POINT('Ctrl Pts',(-19.5089480881137,14.07339133107,122.210014195614)) ;
#27001=CARTESIAN_POINT('Ctrl Pts',(-19.7926811889532,14.2633729507487,121.953859464746)) ;
#27002=CARTESIAN_POINT('Ctrl Pts',(-19.7159932556982,14.0833838703858,122.245450559124)) ;
#27003=CARTESIAN_POINT('Ctrl Pts',(-20.0387837794866,14.2733213966434,122.042123340413)) ;
#27004=CARTESIAN_POINT('Ctrl Pts',(-19.9128751830492,14.0933323162805,122.316060778059)) ;
#27005=CARTESIAN_POINT('Ctrl Pts',(-20.2657069288235,14.2832581991753,122.171283774759)) ;
#27006=CARTESIAN_POINT('Ctrl Pts',(-20.0944136903199,14.1032691188124,122.419388116494)) ;
#27007=CARTESIAN_POINT('Ctrl Pts',(-20.4679459835233,14.2932412066266,122.338438899069)) ;
#27008=CARTESIAN_POINT('Ctrl Pts',(-20.2562053796479,14.1132521262637,122.55311135473)) ;
#27009=CARTESIAN_POINT('Ctrl Pts',(-20.6387149774407,14.3032850480414,122.539652891498)) ;
#27010=CARTESIAN_POINT('Ctrl Pts',(-20.3928213084693,14.1232959676785,122.714082124582)) ;
#27011=CARTESIAN_POINT('Ctrl Pts',(-20.7696539436816,14.3131132466653,122.762322078436)) ;
#27012=CARTESIAN_POINT('Ctrl Pts',(-20.4975727394675,14.1331241663024,122.892215983891)) ;
#27013=CARTESIAN_POINT('Ctrl Pts',(-20.8623069213888,14.3231898401075,123.010327296333)) ;
#27014=CARTESIAN_POINT('Ctrl Pts',(-20.5716961867102,14.1432007597447,123.090620129128)) ;
#27015=CARTESIAN_POINT('Ctrl Pts',(-20.909567306365,14.3330418394491,123.264936220785)) ;
#27016=CARTESIAN_POINT('Ctrl Pts',(-20.6095053328595,14.1530527590862,123.294306109493)) ;
#27017=CARTESIAN_POINT('Ctrl Pts',(-20.9121706248892,14.343115426273,123.529600919858)) ;
#27018=CARTESIAN_POINT('Ctrl Pts',(-20.6115890777029,14.1631263459101,123.506038179509)) ;
#27019=CARTESIAN_POINT('Ctrl Pts',(-20.8697248958235,14.3529556513705,123.784708643342)) ;
#27020=CARTESIAN_POINT('Ctrl Pts',(-20.5776337239948,14.1729665710076,123.710123503099)) ;
#27021=CARTESIAN_POINT('Ctrl Pts',(-20.7834156858806,14.3629213553991,124.031943418832)) ;
#27022=CARTESIAN_POINT('Ctrl Pts',(-20.5085876682656,14.1829322750362,123.907911452828)) ;
#27023=CARTESIAN_POINT('Ctrl Pts',(-20.6543560175008,14.3729479887057,124.26167893838)) ;
#27024=CARTESIAN_POINT('Ctrl Pts',(-20.405340950833,14.1929589083428,124.091700497226)) ;
#27025=CARTESIAN_POINT('Ctrl Pts',(-20.4893881315526,14.3828622844175,124.463327357308)) ;
#27026=CARTESIAN_POINT('Ctrl Pts',(-20.273367967042,14.2028732040546,124.253019557366)) ;
#27027=CARTESIAN_POINT('Ctrl Pts',(-20.29073289972,14.39285057311,124.634911409917)) ;
#27028=CARTESIAN_POINT('Ctrl Pts',(-20.1144447718736,14.2128614927471,124.390287707971)) ;
#27029=CARTESIAN_POINT('Ctrl Pts',(-20.0639385669575,14.4028893062683,124.769650931547)) ;
#27030=CARTESIAN_POINT('Ctrl Pts',(-19.933009840498,14.2229002259054,124.498080437852)) ;
#27031=CARTESIAN_POINT('Ctrl Pts',(-19.8221438934761,14.4127326380959,124.861560677325)) ;
#27032=CARTESIAN_POINT('Ctrl Pts',(-19.7395754882741,14.232743557733,124.571609123733)) ;
#27033=CARTESIAN_POINT('Ctrl Pts',(-19.5634174500474,14.4227603639755,124.911597480083)) ;
#27034=CARTESIAN_POINT('Ctrl Pts',(-19.532594551231,14.2427712836126,124.611640002553)) ;
#27035=CARTESIAN_POINT('Ctrl Pts',(-19.2997938732283,14.432792700364,124.915236180486)) ;
#27036=CARTESIAN_POINT('Ctrl Pts',(-19.3216956393782,14.2528036200011,124.614552265305)) ;
#27037=CARTESIAN_POINT('Ctrl Pts',(-19.0447452472327,14.4426222006646,124.874418148553)) ;
#27038=CARTESIAN_POINT('Ctrl Pts',(-19.1176575176957,14.2626331203018,124.581899394182)) ;
#27039=CARTESIAN_POINT('Ctrl Pts',(-18.796407103076,14.4526117045814,124.789299015739)) ;
#27040=CARTESIAN_POINT('Ctrl Pts',(-18.9189866276755,14.2726226242185,124.513805617526)) ;
#27041=CARTESIAN_POINT('Ctrl Pts',(-18.5657044122553,14.4626555450938,124.661080239922)) ;
#27042=CARTESIAN_POINT('Ctrl Pts',(-18.734423674689,14.2826664647309,124.411231794536)) ;
#27043=CARTESIAN_POINT('Ctrl Pts',(-18.3649628204512,14.4724772508619,124.498843726449)) ;
#27044=CARTESIAN_POINT('Ctrl Pts',(-18.5738302074953,14.292488170499,124.281444409)) ;
#27045=CARTESIAN_POINT('Ctrl Pts',(-18.1912720235427,14.4825122979942,124.300414746533)) ;
#27046=CARTESIAN_POINT('Ctrl Pts',(-18.4348762631959,14.3025232176314,124.122702256751)) ;
#27047=CARTESIAN_POINT('Ctrl Pts',(-18.055432254409,14.4925369754311,124.074689127998)) ;
#27048=CARTESIAN_POINT('Ctrl Pts',(-18.3262031311123,14.3125478950683,123.942122532093)) ;
#27049=CARTESIAN_POINT('Ctrl Pts',(-17.9619640242889,14.5023897902856,123.833226852752)) ;
#27050=CARTESIAN_POINT('Ctrl Pts',(-18.2514273185047,14.3224007099227,123.748954049798)) ;
#27051=CARTESIAN_POINT('Ctrl Pts',(-17.9107066774369,14.5123774998931,123.575833839664)) ;
#27052=CARTESIAN_POINT('Ctrl Pts',(-18.210419791455,14.3323884195303,123.543040117254)) ;
#27053=CARTESIAN_POINT('Ctrl Pts',(-17.9049402191342,14.5223075098872,123.314937805648)) ;
#27054=CARTESIAN_POINT('Ctrl Pts',(-18.2058049219443,14.3423184295243,123.33432374461)) ;
#27055=CARTESIAN_POINT('Ctrl Pts',(-17.9443990827381,14.5322972651064,123.055394867544)) ;
#27056=CARTESIAN_POINT('Ctrl Pts',(-18.237370231834,14.3523081847435,123.126689256779)) ;
#27057=CARTESIAN_POINT('Ctrl Pts',(-18.0289554645481,14.5423238737893,122.80583753216)) ;
#27058=CARTESIAN_POINT('Ctrl Pts',(-18.3050137161035,14.3623347934264,122.927042810016)) ;
#27059=CARTESIAN_POINT('Ctrl Pts',(-18.1535342537274,14.5522078138111,122.577928818094)) ;
#27060=CARTESIAN_POINT('Ctrl Pts',(-18.4046749159261,14.3722187334482,122.744715509039)) ;
#27061=CARTESIAN_POINT('Ctrl Pts',(-18.3170525414426,14.5621970413496,122.372560685954)) ;
#27062=CARTESIAN_POINT('Ctrl Pts',(-18.5354880122314,14.3822079609867,122.580419941737)) ;
#27063=CARTESIAN_POINT('Ctrl Pts',(-18.5151557257719,14.5722399118733,122.198188061704)) ;
#27064=CARTESIAN_POINT('Ctrl Pts',(-18.6939694414926,14.3922508315104,122.440920462388)) ;
#27065=CARTESIAN_POINT('Ctrl Pts',(-18.7355880780577,14.5820722986287,122.063388638443)) ;
#27066=CARTESIAN_POINT('Ctrl Pts',(-18.8703137118598,14.4020832182658,122.333079750593)) ;
#27067=CARTESIAN_POINT('Ctrl Pts',(-18.9797323076057,14.5920655918003,121.966658037112)) ;
#27068=CARTESIAN_POINT('Ctrl Pts',(-19.0656282824221,14.4120765114374,122.255693489777)) ;
#27069=CARTESIAN_POINT('Ctrl Pts',(-19.2380876823601,14.6020975974487,121.914120317295)) ;
#27070=CARTESIAN_POINT('Ctrl Pts',(-19.2723122376113,14.4221085170859,122.213661473719)) ;
#27071=CARTESIAN_POINT('Ctrl Pts',(-19.4972262784199,14.6119628534177,121.907034280981)) ;
#27072=CARTESIAN_POINT('Ctrl Pts',(-19.479622479628,14.4319737730548,122.207990741055)) ;
#27073=CARTESIAN_POINT('Ctrl Pts',(-19.7562992627137,14.6219247333252,121.944692330567)) ;
#27074=CARTESIAN_POINT('Ctrl Pts',(-19.6868809582063,14.4419356529623,122.238115153452)) ;
#27075=CARTESIAN_POINT('Ctrl Pts',(-20.0065648350329,14.6319596666871,122.027765848265)) ;
#27076=CARTESIAN_POINT('Ctrl Pts',(-19.8870940599284,14.4519705863242,122.304572113767)) ;
#27077=CARTESIAN_POINT('Ctrl Pts',(-20.2353895991265,14.6418446250664,122.150798715635)) ;
#27078=CARTESIAN_POINT('Ctrl Pts',(-20.0701544291512,14.4618555447035,122.402996417728)) ;
#27079=CARTESIAN_POINT('Ctrl Pts',(-20.4430039039663,14.6519102519891,122.314630587451)) ;
#27080=CARTESIAN_POINT('Ctrl Pts',(-20.2362472126455,14.4719211716262,122.534060408975)) ;
#27081=CARTESIAN_POINT('Ctrl Pts',(-20.6153099874822,14.6617493576534,122.507469086936)) ;
#27082=CARTESIAN_POINT('Ctrl Pts',(-20.3740932248574,14.4817602772905,122.688329427988)) ;
#27083=CARTESIAN_POINT('Ctrl Pts',(-20.7548702754188,14.6718121726588,122.732041086105)) ;
#27084=CARTESIAN_POINT('Ctrl Pts',(-20.4857432796024,14.4918230922959,122.867986018619)) ;
#27085=CARTESIAN_POINT('Ctrl Pts',(-20.8514895076296,14.6817083787074,122.973518167656)) ;
#27086=CARTESIAN_POINT('Ctrl Pts',(-20.5630404332213,14.5017192983446,123.061166569921)) ;
#27087=CARTESIAN_POINT('Ctrl Pts',(-20.905652298732,14.6916492017327,123.229045388477)) ;
#27088=CARTESIAN_POINT('Ctrl Pts',(-20.6063727060311,14.5116601213698,123.265587688841)) ;
#27089=CARTESIAN_POINT('Ctrl Pts',(-20.9147482972179,14.7016537847114,123.49182757385)) ;
#27090=CARTESIAN_POINT('Ctrl Pts',(-20.6136516339194,14.5216647043485,123.475813306976)) ;
#27091=CARTESIAN_POINT('Ctrl Pts',(-20.8777060565819,14.7116746791561,123.752541737872)) ;
#27092=CARTESIAN_POINT('Ctrl Pts',(-20.584019929086,14.5316855987932,123.684384908824)) ;
#27093=CARTESIAN_POINT('Ctrl Pts',(-20.7973137583484,14.7215665997455,123.999754867603)) ;
#27094=CARTESIAN_POINT('Ctrl Pts',(-20.5197082201853,14.5415775193826,123.882155761826)) ;
#27095=CARTESIAN_POINT('Ctrl Pts',(-20.6743041569518,14.7315600320909,124.231770792966)) ;
#27096=CARTESIAN_POINT('Ctrl Pts',(-20.4213024934147,14.551570951728,124.067769440875)) ;
#27097=CARTESIAN_POINT('Ctrl Pts',(-20.5135786631871,14.7415056369908,124.437867633095)) ;
#27098=CARTESIAN_POINT('Ctrl Pts',(-20.2927239143119,14.5615165566279,124.232648095339)) ;
#27099=CARTESIAN_POINT('Ctrl Pts',(-20.3198218573511,14.7514529104723,124.613360457444)) ;
#27100=CARTESIAN_POINT('Ctrl Pts',(-20.137720063294,14.5714638301094,124.373043875978)) ;
#27101=CARTESIAN_POINT('Ctrl Pts',(-20.0961599099383,14.7615008249487,124.753689774848)) ;
#27102=CARTESIAN_POINT('Ctrl Pts',(-19.9587916558263,14.5815117445858,124.485309178269)) ;
#27103=CARTESIAN_POINT('Ctrl Pts',(-19.8564776376663,14.771348465296,124.851279444888)) ;
#27104=CARTESIAN_POINT('Ctrl Pts',(-19.7670469592938,14.5913593849331,124.563382825184)) ;
#27105=CARTESIAN_POINT('Ctrl Pts',(-19.6007489896213,14.7813101806726,124.907199618394)) ;
#27106=CARTESIAN_POINT('Ctrl Pts',(-19.5624646160184,14.6013211003097,124.608121129999)) ;
#27107=CARTESIAN_POINT('Ctrl Pts',(-19.3373962978428,14.7913388042454,124.917606836282)) ;
#27108=CARTESIAN_POINT('Ctrl Pts',(-19.3517825852773,14.6113497238825,124.616449119218)) ;
#27109=CARTESIAN_POINT('Ctrl Pts',(-19.0793336231031,14.8012491663118,124.882634265756)) ;
#27110=CARTESIAN_POINT('Ctrl Pts',(-19.1453323129572,14.6212600859489,124.58847329103)) ;
#27111=CARTESIAN_POINT('Ctrl Pts',(-18.8304237660988,14.8111838599642,124.803839977348)) ;
#27112=CARTESIAN_POINT('Ctrl Pts',(-18.9462038486766,14.6311947796013,124.52544003625)) ;
#27113=CARTESIAN_POINT('Ctrl Pts',(-18.5966220485025,14.8212257030921,124.681499373881)) ;
#27114=CARTESIAN_POINT('Ctrl Pts',(-18.7591614689245,14.6412366227292,124.427569556202)) ;
#27115=CARTESIAN_POINT('Ctrl Pts',(-18.390716860511,14.8311102086625,124.523104155642)) ;
#27116=CARTESIAN_POINT('Ctrl Pts',(-18.5944360498318,14.6511211282996,124.300855240205)) ;
#27117=CARTESIAN_POINT('Ctrl Pts',(-18.2131739736385,14.8411123124477,124.329336878928)) ;
#27118=CARTESIAN_POINT('Ctrl Pts',(-18.4524001167752,14.6611232320848,124.145842979682)) ;
#27119=CARTESIAN_POINT('Ctrl Pts',(-18.0729290956816,14.8510306638627,124.109588770675)) ;
#27120=CARTESIAN_POINT('Ctrl Pts',(-18.3402023497202,14.6710415834998,123.970045780687)) ;
#27121=CARTESIAN_POINT('Ctrl Pts',(-17.9717628132547,14.8610783198836,123.865741080711)) ;
#27122=CARTESIAN_POINT('Ctrl Pts',(-18.2592672790845,14.6810892395207,123.774968483768)) ;
#27123=CARTESIAN_POINT('Ctrl Pts',(-17.9151745106479,14.8709495129118,123.612528140335)) ;
#27124=CARTESIAN_POINT('Ctrl Pts',(-18.2139943885735,14.6909604325489,123.572398901037)) ;
#27125=CARTESIAN_POINT('Ctrl Pts',(-17.9031429831484,14.8810152260553,123.34834743098)) ;
#27126=CARTESIAN_POINT('Ctrl Pts',(-18.204367144922,14.7010261456924,123.361053634231)) ;
#27127=CARTESIAN_POINT('Ctrl Pts',(-17.9361624249687,14.890867686628,123.091474379834)) ;
#27128=CARTESIAN_POINT('Ctrl Pts',(-18.2307796125064,14.7108786062651,123.155558165158)) ;
#27129=CARTESIAN_POINT('Ctrl Pts',(-18.0413449335706,14.9042961493505,122.754742299802)) ;
#27130=CARTESIAN_POINT('Ctrl Pts',(-18.3149269800469,14.7243070689876,122.88615548597)) ;
#27131=CARTESIAN_POINT('Ctrl Pts',(-18.2267874470069,14.9173770968676,122.460483907588)) ;
#27132=CARTESIAN_POINT('Ctrl Pts',(-18.4633001749267,14.7373880165047,122.65073212564)) ;
#27133=CARTESIAN_POINT('Ctrl Pts',(-18.4863543902938,14.9308515951022,122.219747666857)) ;
#27134=CARTESIAN_POINT('Ctrl Pts',(-18.6709215324032,14.7508625147393,122.458175060593)) ;
#27135=CARTESIAN_POINT('Ctrl Pts',(-18.7036544341988,14.9406836987116,122.079886991967)) ;
#27136=CARTESIAN_POINT('Ctrl Pts',(-18.8447666073225,14.7606946183488,122.346277773026)) ;
#27137=CARTESIAN_POINT('Ctrl Pts',(-18.9446987351203,14.9506496018383,121.977572951031)) ;
#27138=CARTESIAN_POINT('Ctrl Pts',(-19.0375992137508,14.7706605214754,122.264426179784)) ;
#27139=CARTESIAN_POINT('Ctrl Pts',(-19.2015765911018,14.9606770111485,121.918685704724)) ;
#27140=CARTESIAN_POINT('Ctrl Pts',(-19.2431028113862,14.7806879307857,122.217314368209)) ;
#27141=CARTESIAN_POINT('Ctrl Pts',(-19.4616556588049,14.9705880425151,121.905384721623)) ;
#27142=CARTESIAN_POINT('Ctrl Pts',(-19.4511604538144,14.7905989621522,122.206669246989)) ;
#27143=CARTESIAN_POINT('Ctrl Pts',(-19.8072618039374,14.9838323501362,121.947128778354)) ;
#27144=CARTESIAN_POINT('Ctrl Pts',(-19.7276732696558,14.8038432697733,122.24007284524)) ;
#27145=CARTESIAN_POINT('Ctrl Pts',(-20.2188550941679,15.0005328328073,122.113045312188)) ;
#27146=CARTESIAN_POINT('Ctrl Pts',(-20.0569081396409,14.8205437524445,122.372778876184)) ;
#27147=CARTESIAN_POINT('Ctrl Pts',(-20.5455679441702,15.0170396619631,122.405960959497)) ;
#27148=CARTESIAN_POINT('Ctrl Pts',(-20.3183298372832,14.8370505816002,122.607156832751)) ;
#27149=CARTESIAN_POINT('Ctrl Pts',(-20.7373262391937,15.0303502902007,122.698457845509)) ;
#27150=CARTESIAN_POINT('Ctrl Pts',(-20.4717022185341,14.8503612098378,122.841112812095)) ;
#27151=CARTESIAN_POINT('Ctrl Pts',(-20.8410482037776,15.0403428537408,122.939743261889)) ;
#27152=CARTESIAN_POINT('Ctrl Pts',(-20.5546889224827,14.8603537733779,123.034149304461)) ;
#27153=CARTESIAN_POINT('Ctrl Pts',(-20.9012011780977,15.0503729367423,123.196334518998)) ;
#27154=CARTESIAN_POINT('Ctrl Pts',(-20.6028117682902,14.8703838563795,123.239415751326)) ;
#27155=CARTESIAN_POINT('Ctrl Pts',(-20.9212136813736,15.0635465407401,123.542009444152)) ;
#27156=CARTESIAN_POINT('Ctrl Pts',(-20.6188231356047,14.8835574603772,123.515975765134)) ;
#27157=CARTESIAN_POINT('Ctrl Pts',(-20.8322977307926,15.0801842459715,123.97501211203)) ;
#27158=CARTESIAN_POINT('Ctrl Pts',(-20.5476923868234,14.9001951656086,123.862358789437)) ;
#27159=CARTESIAN_POINT('Ctrl Pts',(-20.5559470864143,15.1000660085389,124.425649304088)) ;
#27160=CARTESIAN_POINT('Ctrl Pts',(-20.3266297541307,14.9200769281761,124.222868808078)) ;
#27161=CARTESIAN_POINT('Ctrl Pts',(-20.2087222530336,15.1167623607554,124.70175262575)) ;
#27162=CARTESIAN_POINT('Ctrl Pts',(-20.0488038623269,14.9367732803926,124.443780904704)) ;
#27163=CARTESIAN_POINT('Ctrl Pts',(-19.8917080630513,15.1299193885445,124.839949683673)) ;
#27164=CARTESIAN_POINT('Ctrl Pts',(-19.7952369425697,14.9499303081817,124.554316138444)) ;
#27165=CARTESIAN_POINT('Ctrl Pts',(-19.5501536847632,15.1432967431881,124.92300774244)) ;
#27166=CARTESIAN_POINT('Ctrl Pts',(-19.5219730467639,14.9633076628252,124.620769728734)) ;
#27167=CARTESIAN_POINT('Ctrl Pts',(-19.1108554066313,15.1598275774469,124.912748434119)) ;
#27168=CARTESIAN_POINT('Ctrl Pts',(-19.170551068665,14.979838497084,124.612563667479)) ;
#27169=CARTESIAN_POINT('Ctrl Pts',(-18.616168502824,15.17979226719,124.720920100906)) ;
#27170=CARTESIAN_POINT('Ctrl Pts',(-18.7747945577077,14.9998031868271,124.45910447757)) ;
#27171=CARTESIAN_POINT('Ctrl Pts',(-18.2178819295255,15.1997087606136,124.372224270615)) ;
#27172=CARTESIAN_POINT('Ctrl Pts',(-18.4561642627655,15.0197196802507,124.180149816018)) ;
#27173=CARTESIAN_POINT('Ctrl Pts',(-17.9618943674429,15.2195984799632,123.909642300137)) ;
#27174=CARTESIAN_POINT('Ctrl Pts',(-18.2513709039393,15.0396093996003,123.810084995758)) ;
#27175=CARTESIAN_POINT('Ctrl Pts',(-17.8790867340295,15.239605209611,123.384461553137)) ;
#27176=CARTESIAN_POINT('Ctrl Pts',(-18.1851220450662,15.0596161292481,123.389940905044)) ;
#27177=CARTESIAN_POINT('Ctrl Pts',(-17.9792551414852,15.2594432632579,122.866690154571)) ;
#27178=CARTESIAN_POINT('Ctrl Pts',(-18.2652543890131,15.079454182895,122.975722039237)) ;
#27179=CARTESIAN_POINT('Ctrl Pts',(-18.2516493430185,15.2794366014715,122.410539526417)) ;
#27180=CARTESIAN_POINT('Ctrl Pts',(-18.4831677681727,15.0994475211086,122.610800270065)) ;
#27181=CARTESIAN_POINT('Ctrl Pts',(-18.661435692982,15.2993194008781,122.076711965965)) ;
#27182=CARTESIAN_POINT('Ctrl Pts',(-18.8109961779416,15.1193303205152,122.34373578517)) ;
#27183=CARTESIAN_POINT('Ctrl Pts',(-19.1602442446391,15.3192115817968,121.901912195536)) ;
#27184=CARTESIAN_POINT('Ctrl Pts',(-19.2100434562284,15.1392225014339,122.203893842988)) ;
#27185=CARTESIAN_POINT('Ctrl Pts',(-19.6893450348153,15.3391137602919,121.906937811211)) ;
#27186=CARTESIAN_POINT('Ctrl Pts',(-19.6333250670439,15.159124679929,122.207913017499)) ;
#27187=CARTESIAN_POINT('Ctrl Pts',(-20.1877316480936,15.3591510714956,122.094234259217)) ;
#27188=CARTESIAN_POINT('Ctrl Pts',(-20.0320345164081,15.1791619911328,122.357748581197)) ;
#27189=CARTESIAN_POINT('Ctrl Pts',(-20.5885091138174,15.3789635130365,122.4361550605)) ;
#27190=CARTESIAN_POINT('Ctrl Pts',(-20.352658713179,15.1989744326736,122.631285748145)) ;
#27191=CARTESIAN_POINT('Ctrl Pts',(-20.8514802727897,15.3990287537714,122.899819819407)) ;
#27192=CARTESIAN_POINT('Ctrl Pts',(-20.5630361534512,15.2190396734085,123.002216473756)) ;
#27193=CARTESIAN_POINT('Ctrl Pts',(-20.939569466923,15.4187859586272,123.417748054594)) ;
#27194=CARTESIAN_POINT('Ctrl Pts',(-20.6335085384984,15.2387968782644,123.416561832562)) ;
#27195=CARTESIAN_POINT('Ctrl Pts',(-20.8451846342489,15.4388192312729,123.941494843128)) ;
#27196=CARTESIAN_POINT('Ctrl Pts',(-20.5580007277665,15.2588301509101,123.835558979513)) ;
#27197=CARTESIAN_POINT('Ctrl Pts',(-20.5803681949361,15.4586321397268,124.396932991369)) ;
#27198=CARTESIAN_POINT('Ctrl Pts',(-20.3461462373689,15.2786430593639,124.199911406604)) ;
#27199=CARTESIAN_POINT('Ctrl Pts',(-20.1731096405733,15.4786282858542,124.738024765008)) ;
#27200=CARTESIAN_POINT('Ctrl Pts',(-20.0203388220478,15.2986392054913,124.472784322776)) ;
#27201=CARTESIAN_POINT('Ctrl Pts',(-19.6769061894164,15.4984900390767,124.918856330261)) ;
#27202=CARTESIAN_POINT('Ctrl Pts',(-19.6233743087396,15.3185009587138,124.617449135294)) ;
#27203=CARTESIAN_POINT('Ctrl Pts',(-19.1436360482035,15.5185585562048,124.919177517765)) ;
#27204=CARTESIAN_POINT('Ctrl Pts',(-19.1967589767419,15.3385694758419,124.617705010039)) ;
#27205=CARTESIAN_POINT('Ctrl Pts',(-18.6481039856445,15.5383894292016,124.739248841471)) ;
#27206=CARTESIAN_POINT('Ctrl Pts',(-18.8003319653689,15.3584003488387,124.473760421146)) ;
#27207=CARTESIAN_POINT('Ctrl Pts',(-18.2411262734598,15.5583113400183,124.400722475563)) ;
#27208=CARTESIAN_POINT('Ctrl Pts',(-18.4747503480826,15.3783222596554,124.202937369334)) ;
#27209=CARTESIAN_POINT('Ctrl Pts',(-17.9740267390617,15.5782407834536,123.943204335233)) ;
#27210=CARTESIAN_POINT('Ctrl Pts',(-18.2610720716113,15.3982517030907,123.836921334488)) ;
#27211=CARTESIAN_POINT('Ctrl Pts',(-17.8790194223619,15.59815045357,123.422718308582)) ;
#27212=CARTESIAN_POINT('Ctrl Pts',(-18.1850681984714,15.4181613732071,123.42053129134)) ;
#27213=CARTESIAN_POINT('Ctrl Pts',(-17.9662605748662,15.6180238108329,122.901708304058)) ;
#27214=CARTESIAN_POINT('Ctrl Pts',(-18.254863873094,15.43803473047,123.00372270003)) ;
#27215=CARTESIAN_POINT('Ctrl Pts',(-18.2276238439571,15.6380153454508,122.439173769157)) ;
#27216=CARTESIAN_POINT('Ctrl Pts',(-18.4639568825122,15.4580262650879,122.633696362136)) ;
#27217=CARTESIAN_POINT('Ctrl Pts',(-18.6285678009232,15.6578809628615,122.095505124988)) ;
#27218=CARTESIAN_POINT('Ctrl Pts',(-18.7847146580216,15.4778918824987,122.358763014861)) ;
#27219=CARTESIAN_POINT('Ctrl Pts',(-19.1253095706751,15.6778618926898,121.907746174012)) ;
#27220=CARTESIAN_POINT('Ctrl Pts',(-19.1821092675839,15.4978728123269,122.208558782164)) ;
#27221=CARTESIAN_POINT('Ctrl Pts',(-19.6552143908038,15.6978003547729,121.901373660419)) ;
#27222=CARTESIAN_POINT('Ctrl Pts',(-19.6060335509028,15.51781127441,122.203463873449)) ;
#27223=CARTESIAN_POINT('Ctrl Pts',(-20.1546433032014,15.7176925479946,122.075043824401)) ;
#27224=CARTESIAN_POINT('Ctrl Pts',(-20.0055761682767,15.5377034676318,122.342403428384)) ;
#27225=CARTESIAN_POINT('Ctrl Pts',(-20.5661496331982,15.73766326303,122.410119645807)) ;
#27226=CARTESIAN_POINT('Ctrl Pts',(-20.3347791384015,15.5576741826671,122.610466906619)) ;
#27227=CARTESIAN_POINT('Ctrl Pts',(-20.8373123753955,15.7574729346961,122.861577302707)) ;
#27228=CARTESIAN_POINT('Ctrl Pts',(-20.5517067350592,15.5774838543332,122.97163565789)) ;
#27229=CARTESIAN_POINT('Ctrl Pts',(-20.9393997364478,15.7774661513873,123.382866096592)) ;
#27230=CARTESIAN_POINT('Ctrl Pts',(-20.6333723462591,15.5974770710244,123.388667788783)) ;
#27231=CARTESIAN_POINT('Ctrl Pts',(-20.8584216081124,15.7973170635836,123.904440437728)) ;
#27232=CARTESIAN_POINT('Ctrl Pts',(-20.5685874513888,15.6173279832208,123.805925914107)) ;
#27233=CARTESIAN_POINT('Ctrl Pts',(-20.6013666268889,15.8173916699027,124.371819409561)) ;
#27234=CARTESIAN_POINT('Ctrl Pts',(-20.3629338879566,15.6374025895398,124.17983155202)) ;
#27235=CARTESIAN_POINT('Ctrl Pts',(-20.2709357008999,15.833908301786,124.661071335312)) ;
#27236=CARTESIAN_POINT('Ctrl Pts',(-20.098605819619,15.6539192214231,124.411216220692)) ;
#27237=CARTESIAN_POINT('Ctrl Pts',(-19.9567400193657,15.8472470094801,124.816295036982)) ;
#27238=CARTESIAN_POINT('Ctrl Pts',(-19.8472304865429,15.6672579291172,124.535405548964)) ;
#27239=CARTESIAN_POINT('Ctrl Pts',(-19.7085577801769,15.8570893837884,124.889269258747)) ;
#27240=CARTESIAN_POINT('Ctrl Pts',(-19.6486898643955,15.6771003034255,124.593781066732)) ;
#27241=CARTESIAN_POINT('Ctrl Pts',(-19.4460289923727,15.8671444037711,124.918903925048)) ;
#27242=CARTESIAN_POINT('Ctrl Pts',(-19.438655254333,15.6871553234083,124.617484843905)) ;
#27243=CARTESIAN_POINT('Ctrl Pts',(-19.0989283678214,15.8803765604287,124.897309206157)) ;
#27244=CARTESIAN_POINT('Ctrl Pts',(-19.1610280086618,15.7003874800658,124.600218444694)) ;
#27245=CARTESIAN_POINT('Ctrl Pts',(-18.680086550223,15.8969915277738,124.757481852894)) ;
#27246=CARTESIAN_POINT('Ctrl Pts',(-18.8258890338263,15.717002447411,124.488333567479)) ;
#27247=CARTESIAN_POINT('Ctrl Pts',(-18.3346327392559,15.913586114785,124.48329340641)) ;
#27248=CARTESIAN_POINT('Ctrl Pts',(-18.549571248321,15.7335970344222,124.26900587412)) ;
#27249=CARTESIAN_POINT('Ctrl Pts',(-18.1268897362054,15.9268196831404,124.204366870051)) ;
#27250=CARTESIAN_POINT('Ctrl Pts',(-18.3833541247988,15.7468306027775,124.045842691326)) ;
#27251=CARTESIAN_POINT('Ctrl Pts',(-18.0083439444997,15.9368633009491,123.968576154149)) ;
#27252=CARTESIAN_POINT('Ctrl Pts',(-18.288524508184,15.7568742205862,123.857213407479)) ;
#27253=CARTESIAN_POINT('Ctrl Pts',(-17.9336253681816,15.9467502251839,123.719711066793)) ;
#27254=CARTESIAN_POINT('Ctrl Pts',(-18.228750615402,15.766761144821,123.658118921018)) ;
#27255=CARTESIAN_POINT('Ctrl Pts',(-17.9024744065932,15.9567408796307,123.459039355824)) ;
#27256=CARTESIAN_POINT('Ctrl Pts',(-18.2038316647778,15.7767517992678,123.44958390152)) ;
#27257=CARTESIAN_POINT('Ctrl Pts',(-17.9170694041595,15.9667026380847,123.197660756749)) ;
#27258=CARTESIAN_POINT('Ctrl Pts',(-18.2155127307376,15.7867135577218,123.240472575159)) ;
#27259=CARTESIAN_POINT('Ctrl Pts',(-17.9967391763496,15.9800425031519,122.856207482281)) ;
#27260=CARTESIAN_POINT('Ctrl Pts',(-18.2792369334935,15.800053422789,122.967353118238)) ;
#27261=CARTESIAN_POINT('Ctrl Pts',(-18.1639736695918,15.9933512860652,122.544568270991)) ;
#27262=CARTESIAN_POINT('Ctrl Pts',(-18.4130291807897,15.8133622057023,122.718017643817)) ;
#27263=CARTESIAN_POINT('Ctrl Pts',(-18.4009205226991,16.0065470435093,122.291373958012)) ;
#27264=CARTESIAN_POINT('Ctrl Pts',(-18.6026009981143,15.8265579631464,122.515452269556)) ;
#27265=CARTESIAN_POINT('Ctrl Pts',(-18.6098352782094,16.0165089271858,122.133609050801)) ;
#27266=CARTESIAN_POINT('Ctrl Pts',(-18.7697316665217,15.8365198468229,122.389244599765)) ;
#27267=CARTESIAN_POINT('Ctrl Pts',(-18.8450601920169,16.0265520367004,122.013933523829)) ;
#27268=CARTESIAN_POINT('Ctrl Pts',(-18.9579132372001,15.8465629563375,122.293505565848)) ;
#27269=CARTESIAN_POINT('Ctrl Pts',(-19.0926161288735,16.0364042866996,121.938083702946)) ;
#27270=CARTESIAN_POINT('Ctrl Pts',(-19.1559583816547,15.8564152063368,122.232828069619)) ;
#27271=CARTESIAN_POINT('Ctrl Pts',(-19.3525761374353,16.0463758236501,121.90535120371)) ;
#27272=CARTESIAN_POINT('Ctrl Pts',(-19.3639266242928,15.8663867432872,122.206644267402)) ;
#27273=CARTESIAN_POINT('Ctrl Pts',(-19.6149622143192,16.0563710891276,121.918309627861)) ;
#27274=CARTESIAN_POINT('Ctrl Pts',(-19.5738352989783,15.8763820087648,122.217013257549)) ;
#27275=CARTESIAN_POINT('Ctrl Pts',(-19.8719707676213,16.0664050620013,121.977157725234)) ;
#27276=CARTESIAN_POINT('Ctrl Pts',(-19.7794416116365,15.8864159816384,122.264093925763)) ;
#27277=CARTESIAN_POINT('Ctrl Pts',(-20.1107386746183,16.0762604767636,122.077550542983)) ;
#27278=CARTESIAN_POINT('Ctrl Pts',(-19.9704548934143,15.8962713964007,122.344410174474)) ;
#27279=CARTESIAN_POINT('Ctrl Pts',(-20.3317609231274,16.0862597542724,122.219585083318)) ;
#27280=CARTESIAN_POINT('Ctrl Pts',(-20.1472714239141,15.9062706739096,122.458039646496)) ;
#27281=CARTESIAN_POINT('Ctrl Pts',(-20.5230102658078,16.0961549384354,122.395838020282)) ;
#27282=CARTESIAN_POINT('Ctrl Pts',(-20.3002692442417,15.9161658580725,122.599043480994)) ;
#27283=CARTESIAN_POINT('Ctrl Pts',(-20.6833117694189,16.1062153180762,122.606026601043)) ;
#27284=CARTESIAN_POINT('Ctrl Pts',(-20.4285086974711,15.9262262377133,122.76719571147)) ;
#27285=CARTESIAN_POINT('Ctrl Pts',(-20.8023123453152,16.1160651870843,122.835923343469)) ;
#27286=CARTESIAN_POINT('Ctrl Pts',(-20.5237070533521,15.9360761067214,122.951113839647)) ;
#27287=CARTESIAN_POINT('Ctrl Pts',(-20.8815749658397,16.1260967482922,123.087326542233)) ;
#27288=CARTESIAN_POINT('Ctrl Pts',(-20.5871150742216,15.9461076679293,123.152237028848)) ;
#27289=CARTESIAN_POINT('Ctrl Pts',(-20.9153886455586,16.1361071971745,123.3482327168)) ;
#27290=CARTESIAN_POINT('Ctrl Pts',(-20.6141638267646,15.9561181168116,123.360962211071)) ;
#27291=CARTESIAN_POINT('Ctrl Pts',(-20.9038000062041,16.1460139365915,123.608304860459)) ;
#27292=CARTESIAN_POINT('Ctrl Pts',(-20.604890742972,15.9660248562286,123.569019582891)) ;
#27293=CARTESIAN_POINT('Ctrl Pts',(-20.8475493442764,16.1559519526599,123.863320444448)) ;
#27294=CARTESIAN_POINT('Ctrl Pts',(-20.5598881638927,15.9759628722971,123.773031376224)) ;
#27295=CARTESIAN_POINT('Ctrl Pts',(-20.7473434745622,16.1659571991111,124.106434248665)) ;
#27296=CARTESIAN_POINT('Ctrl Pts',(-20.4797215247247,15.9859681187482,123.967521547182)) ;
#27297=CARTESIAN_POINT('Ctrl Pts',(-20.6056840713685,16.1759912601674,124.328819428175)) ;
#27298=CARTESIAN_POINT('Ctrl Pts',(-20.3663921647497,15.9960021798045,124.145428536233)) ;
#27299=CARTESIAN_POINT('Ctrl Pts',(-20.4312280688443,16.1858363412255,124.519891626386)) ;
#27300=CARTESIAN_POINT('Ctrl Pts',(-20.2268260969221,16.0058472608626,124.298284524298)) ;
#27301=CARTESIAN_POINT('Ctrl Pts',(-20.2236607634961,16.195822147179,124.680379963816)) ;
#27302=CARTESIAN_POINT('Ctrl Pts',(-20.0607710803416,16.0158330668161,124.426673466983)) ;
#27303=CARTESIAN_POINT('Ctrl Pts',(-19.9925740517516,16.2057569677332,124.801974564811)) ;
#27304=CARTESIAN_POINT('Ctrl Pts',(-19.8759009849248,16.0257678873703,124.523947205164)) ;
#27305=CARTESIAN_POINT('Ctrl Pts',(-19.7408239243177,16.2158144928654,124.88232980859)) ;
#27306=CARTESIAN_POINT('Ctrl Pts',(-19.674500158399,16.0358254125025,124.588229439226)) ;
#27307=CARTESIAN_POINT('Ctrl Pts',(-19.4850756391553,16.2256361435168,124.917322735119)) ;
#27308=CARTESIAN_POINT('Ctrl Pts',(-19.4699018773493,16.0456470631539,124.616221674339)) ;
#27309=CARTESIAN_POINT('Ctrl Pts',(-19.2210119356238,16.2356922070215,124.90763544783)) ;
#27310=CARTESIAN_POINT('Ctrl Pts',(-19.258650898185,16.0557031266586,124.608469860502)) ;
#27311=CARTESIAN_POINT('Ctrl Pts',(-18.965674000184,16.2456328740854,124.852413667813)) ;
#27312=CARTESIAN_POINT('Ctrl Pts',(-19.0543812431617,16.0656437937226,124.564290497931)) ;
#27313=CARTESIAN_POINT('Ctrl Pts',(-18.7243829673979,16.2555372677514,124.754815092852)) ;
#27314=CARTESIAN_POINT('Ctrl Pts',(-18.8613495382106,16.0755481873885,124.486210004982)) ;
#27315=CARTESIAN_POINT('Ctrl Pts',(-18.5006518515227,16.2655837915144,124.614693286642)) ;
#27316=CARTESIAN_POINT('Ctrl Pts',(-18.6823656136091,16.0855947111516,124.374110855756)) ;
#27317=CARTESIAN_POINT('Ctrl Pts',(-18.3073636533246,16.2754798745308,124.440639733717)) ;
#27318=CARTESIAN_POINT('Ctrl Pts',(-18.5277366902723,16.0954907941679,124.234866901715)) ;
#27319=CARTESIAN_POINT('Ctrl Pts',(-18.1445816442607,16.2855465737608,124.232170442766)) ;
#27320=CARTESIAN_POINT('Ctrl Pts',(-18.3975125052179,16.105557493398,124.068090149545)) ;
#27321=CARTESIAN_POINT('Ctrl Pts',(-18.0231616074987,16.2953701841619,124.004307681981)) ;
#27322=CARTESIAN_POINT('Ctrl Pts',(-18.3003785015697,16.115381103799,123.885799728941)) ;
#27323=CARTESIAN_POINT('Ctrl Pts',(-17.9408403240638,16.3054260443394,123.753235338654)) ;
#27324=CARTESIAN_POINT('Ctrl Pts',(-18.2345231623342,16.1254369639765,123.684941163944)) ;
#27325=CARTESIAN_POINT('Ctrl Pts',(-17.904145201317,16.3153591906443,123.494762458891)) ;
#27326=CARTESIAN_POINT('Ctrl Pts',(-18.2051689666766,16.1353701102815,123.478162945526)) ;
#27327=CARTESIAN_POINT('Ctrl Pts',(-17.9123613233359,16.3253044464149,123.233570994404)) ;
#27328=CARTESIAN_POINT('Ctrl Pts',(-18.2117436421572,16.1453153660521,123.269210168122)) ;
#27329=CARTESIAN_POINT('Ctrl Pts',(-17.9658149650056,16.3352877448534,122.976690048544)) ;
#27330=CARTESIAN_POINT('Ctrl Pts',(-18.2545082370437,16.1552986644905,123.063705923525)) ;
#27331=CARTESIAN_POINT('Ctrl Pts',(-18.0638986666255,16.345324925,122.731859880856)) ;
#27332=CARTESIAN_POINT('Ctrl Pts',(-18.3329769087346,16.1653358446372,122.867842396204)) ;
#27333=CARTESIAN_POINT('Ctrl Pts',(-18.2001537297579,16.3551794777095,122.511606700127)) ;
#27334=CARTESIAN_POINT('Ctrl Pts',(-18.4419820544397,16.1751903973466,122.691641395589)) ;
#27335=CARTESIAN_POINT('Ctrl Pts',(-18.3747984971053,16.3651789961568,122.315323705892)) ;
#27336=CARTESIAN_POINT('Ctrl Pts',(-18.5816990552253,16.185189915794,122.534616199794)) ;
#27337=CARTESIAN_POINT('Ctrl Pts',(-18.5786176379803,16.3750740786189,122.153776522294)) ;
#27338=CARTESIAN_POINT('Ctrl Pts',(-18.7447549194951,16.195084998256,122.405380095778)) ;
#27339=CARTESIAN_POINT('Ctrl Pts',(-18.8111591522696,16.385134624125,122.028064933009)) ;
#27340=CARTESIAN_POINT('Ctrl Pts',(-18.9307890798417,16.2051455437621,122.304812173805)) ;
#27341=CARTESIAN_POINT('Ctrl Pts',(-19.0567347651697,16.394983931373,121.946236873333)) ;
#27342=CARTESIAN_POINT('Ctrl Pts',(-19.1272492874052,16.2149948510101,122.239351517279)) ;
#27343=CARTESIAN_POINT('Ctrl Pts',(-19.3172847594668,16.4050110214604,121.906948036796)) ;
#27344=CARTESIAN_POINT('Ctrl Pts',(-19.3356895344519,16.2250219410975,122.207921911425)) ;
#27345=CARTESIAN_POINT('Ctrl Pts',(-19.5807454043777,16.4150399255973,121.91419747043)) ;
#27346=CARTESIAN_POINT('Ctrl Pts',(-19.5464580626688,16.2350508452344,122.213723077586)) ;
#27347=CARTESIAN_POINT('Ctrl Pts',(-19.8342636546748,16.4248837906966,121.965599859095)) ;
#27348=CARTESIAN_POINT('Ctrl Pts',(-19.7492714785227,16.2448947103337,122.254846299181)) ;
#27349=CARTESIAN_POINT('Ctrl Pts',(-20.0789676317228,16.434879617405,122.0611017389)) ;
#27350=CARTESIAN_POINT('Ctrl Pts',(-19.9450340249279,16.2548905370421,122.331249046834)) ;
#27351=CARTESIAN_POINT('Ctrl Pts',(-20.3037842341569,16.444904834054,122.198459857618)) ;
#27352=CARTESIAN_POINT('Ctrl Pts',(-20.1248865660534,16.2649157536911,122.441136831011)) ;
#27353=CARTESIAN_POINT('Ctrl Pts',(-20.4988993121104,16.4547946662116,122.370150559373)) ;
#27354=CARTESIAN_POINT('Ctrl Pts',(-20.2809771772072,16.2748055858487,122.578490004565)) ;
#27355=CARTESIAN_POINT('Ctrl Pts',(-20.6631697043296,16.4647855222963,122.574949866266)) ;
#27356=CARTESIAN_POINT('Ctrl Pts',(-20.4123923501296,16.2847964419335,122.742330173249)) ;
#27357=CARTESIAN_POINT('Ctrl Pts',(-20.7887677400445,16.4747306168892,122.804137700936)) ;
#27358=CARTESIAN_POINT('Ctrl Pts',(-20.512869395449,16.2947415365263,122.925680738138)) ;
#27359=CARTESIAN_POINT('Ctrl Pts',(-20.8731883104183,16.4846825206573,123.051673973059)) ;
#27360=CARTESIAN_POINT('Ctrl Pts',(-20.5804045428109,16.3046934402944,123.123709795798)) ;
#27361=CARTESIAN_POINT('Ctrl Pts',(-20.9134563188917,16.4947189201267,123.312320962728)) ;
#27362=CARTESIAN_POINT('Ctrl Pts',(-20.612617681498,16.3147298397639,123.332227690102)) ;
#27363=CARTESIAN_POINT('Ctrl Pts',(-20.9081282976239,16.5046079902154,123.572149884728)) ;
#27364=CARTESIAN_POINT('Ctrl Pts',(-20.6083540200427,16.3246189098525,123.540090066167)) ;
#27365=CARTESIAN_POINT('Ctrl Pts',(-20.8577220598271,16.5145972795863,123.829766727629)) ;
#27366=CARTESIAN_POINT('Ctrl Pts',(-20.5680279279272,16.3346081992234,123.746183149683)) ;
#27367=CARTESIAN_POINT('Ctrl Pts',(-20.76345961891,16.524555845796,124.073893348995)) ;
#27368=CARTESIAN_POINT('Ctrl Pts',(-20.4926169796923,16.3445667654331,123.941483690802)) ;
#27369=CARTESIAN_POINT('Ctrl Pts',(-20.6295786198911,16.5344554170128,124.296968784774)) ;
#27370=CARTESIAN_POINT('Ctrl Pts',(-20.3855116377468,16.3544663366499,124.119942892736)) ;
#27371=CARTESIAN_POINT('Ctrl Pts',(-20.4564004098396,16.5445033314271,124.49625876178)) ;
#27372=CARTESIAN_POINT('Ctrl Pts',(-20.246968141716,16.3645142510642,124.279374299401)) ;
#27373=CARTESIAN_POINT('Ctrl Pts',(-20.254440134761,16.5543986742876,124.660130610446)) ;
#27374=CARTESIAN_POINT('Ctrl Pts',(-20.0853998401919,16.3744095939248,124.410470518004)) ;
#27375=CARTESIAN_POINT('Ctrl Pts',(-20.0233532789183,16.5644603682351,124.788566418278)) ;
#27376=CARTESIAN_POINT('Ctrl Pts',(-19.9005296298809,16.3844712878722,124.513218396484)) ;
#27377=CARTESIAN_POINT('Ctrl Pts',(-19.7788459931032,16.5743048213192,124.873119039239)) ;
#27378=CARTESIAN_POINT('Ctrl Pts',(-19.7049244705946,16.3943157409564,124.580859189868)) ;
#27379=CARTESIAN_POINT('Ctrl Pts',(-19.5205255375102,16.5842655062777,124.915317433973)) ;
#27380=CARTESIAN_POINT('Ctrl Pts',(-19.4982683335334,16.4042764259148,124.614617059786)) ;
#27381=CARTESIAN_POINT('Ctrl Pts',(-19.2568102129339,16.5943014387862,124.911553126493)) ;
#27382=CARTESIAN_POINT('Ctrl Pts',(-19.2872959783146,16.4143123584233,124.611604711671)) ;
#27383=CARTESIAN_POINT('Ctrl Pts',(-19.0015211293968,16.6041900544743,124.863040443295)) ;
#27384=CARTESIAN_POINT('Ctrl Pts',(-19.0830656658347,16.4242009741114,124.572793892405)) ;
#27385=CARTESIAN_POINT('Ctrl Pts',(-18.7552356821971,16.6142044636167,124.770248444018)) ;
#27386=CARTESIAN_POINT('Ctrl Pts',(-18.8860375696502,16.4342153832538,124.498559626099)) ;
#27387=CARTESIAN_POINT('Ctrl Pts',(-18.5287435554736,16.6242382725745,124.635270964711)) ;
#27388=CARTESIAN_POINT('Ctrl Pts',(-18.7048442231239,16.4442491922116,124.390576829673)) ;
#27389=CARTESIAN_POINT('Ctrl Pts',(-18.3326680459431,16.6340687268307,124.467023867572)) ;
#27390=CARTESIAN_POINT('Ctrl Pts',(-18.5479851753716,16.4540796464678,124.255979389229)) ;
#27391=CARTESIAN_POINT('Ctrl Pts',(-18.164649593129,16.6441463944089,124.262383242805)) ;
#27392=CARTESIAN_POINT('Ctrl Pts',(-18.4135707132439,16.464157314046,124.092266173035)) ;
#27393=CARTESIAN_POINT('Ctrl Pts',(-18.037457177748,16.6539982625311,124.03681949593)) ;
#27394=CARTESIAN_POINT('Ctrl Pts',(-18.3118178639604,16.4740091821683,123.911815773256)) ;
#27395=CARTESIAN_POINT('Ctrl Pts',(-17.949256848314,16.6640713000965,123.787285292001)) ;
#27396=CARTESIAN_POINT('Ctrl Pts',(-18.241258048914,16.4840822197336,123.712187880445)) ;
#27397=CARTESIAN_POINT('Ctrl Pts',(-17.9067465102641,16.6739138534474,123.53212739955)) ;
#27398=CARTESIAN_POINT('Ctrl Pts',(-18.2072505652693,16.4939247730845,123.508062584724)) ;
#27399=CARTESIAN_POINT('Ctrl Pts',(-17.908337764321,16.6838942489408,123.269869124294)) ;
#27400=CARTESIAN_POINT('Ctrl Pts',(-18.208523956492,16.5039051685779,123.29825621506)) ;
#27401=CARTESIAN_POINT('Ctrl Pts',(-17.9561266808866,16.6939127269186,123.010973721011)) ;
#27402=CARTESIAN_POINT('Ctrl Pts',(-18.2467556009483,16.5139236465557,123.091139978071)) ;
#27403=CARTESIAN_POINT('Ctrl Pts',(-18.046394284067,16.7037960412247,122.767407615452)) ;
#27404=CARTESIAN_POINT('Ctrl Pts',(-18.3189697326464,16.5238069608618,122.896288048403)) ;
#27405=CARTESIAN_POINT('Ctrl Pts',(-18.1800998015951,16.7138643437634,122.539143460683)) ;
#27406=CARTESIAN_POINT('Ctrl Pts',(-18.4259346651635,16.5338752634005,122.713676647449)) ;
#27407=CARTESIAN_POINT('Ctrl Pts',(-18.3471784469217,16.7236943910368,122.342066798614)) ;
#27408=CARTESIAN_POINT('Ctrl Pts',(-18.5595970360175,16.543705310674,122.556016471638)) ;
#27409=CARTESIAN_POINT('Ctrl Pts',(-18.5504420735912,16.7337612624523,122.172817736648)) ;
#27410=CARTESIAN_POINT('Ctrl Pts',(-18.7222083400755,16.5537721820895,122.420617207245)) ;
#27411=CARTESIAN_POINT('Ctrl Pts',(-18.7760904676618,16.7436503012514,122.043833574538)) ;
#27412=CARTESIAN_POINT('Ctrl Pts',(-18.9027264648716,16.5636612208885,122.317430542113)) ;
#27413=CARTESIAN_POINT('Ctrl Pts',(-19.0231340623094,16.7536469993855,121.95457073187)) ;
#27414=CARTESIAN_POINT('Ctrl Pts',(-19.1003612452814,16.5736579190226,122.246020463371)) ;
#27415=CARTESIAN_POINT('Ctrl Pts',(-19.2808414151497,16.7635994250975,121.909859064209)) ;
#27416=CARTESIAN_POINT('Ctrl Pts',(-19.306526737126,16.5836103447346,122.210251379847)) ;
#27417=CARTESIAN_POINT('Ctrl Pts',(-19.5420687997964,16.7735407273304,121.910209653822)) ;
#27418=CARTESIAN_POINT('Ctrl Pts',(-19.515508139504,16.5935516469676,122.210531942016)) ;
#27419=CARTESIAN_POINT('Ctrl Pts',(-19.8004505578449,16.7835239664143,121.955836958364)) ;
#27420=CARTESIAN_POINT('Ctrl Pts',(-19.7222133350524,16.6035348860515,122.247033765642)) ;
#27421=CARTESIAN_POINT('Ctrl Pts',(-20.0481664431086,16.7935627679829,122.04650185724)) ;
#27422=CARTESIAN_POINT('Ctrl Pts',(-19.9203861326362,16.6135736876201,122.319565851317)) ;
#27423=CARTESIAN_POINT('Ctrl Pts',(-20.27233537467,16.8034108741046,122.175874106053)) ;
#27424=CARTESIAN_POINT('Ctrl Pts',(-20.0997202925184,16.6234217937417,122.423063076114)) ;
#27425=CARTESIAN_POINT('Ctrl Pts',(-20.4750293998556,16.8134710696799,122.345566817946)) ;
#27426=CARTESIAN_POINT('Ctrl Pts',(-20.2618757772164,16.633481989317,122.55881737648)) ;
#27427=CARTESIAN_POINT('Ctrl Pts',(-20.6422713390571,16.8233687529913,122.544786148084)) ;
#27428=CARTESIAN_POINT('Ctrl Pts',(-20.3956688189713,16.6433796726285,122.718192224318)) ;
#27429=CARTESIAN_POINT('Ctrl Pts',(-20.7735531876702,16.8332997933653,122.770334392659)) ;
#27430=CARTESIAN_POINT('Ctrl Pts',(-20.5006942028639,16.6533107130024,122.898630207615)) ;
#27431=CARTESIAN_POINT('Ctrl Pts',(-20.864420100794,16.8433420110219,123.018091751125)) ;
#27432=CARTESIAN_POINT('Ctrl Pts',(-20.5733879339271,16.6633529306591,123.096836198398)) ;
#27433=CARTESIAN_POINT('Ctrl Pts',(-20.9103551819919,16.8532286717559,123.273822728003)) ;
#27434=CARTESIAN_POINT('Ctrl Pts',(-20.61013604196,16.673239591393,123.30142008903)) ;
#27435=CARTESIAN_POINT('Ctrl Pts',(-20.9116383536201,16.8632217803584,123.536414570098)) ;
#27436=CARTESIAN_POINT('Ctrl Pts',(-20.6111628897148,16.6832326999955,123.511493398078)) ;
#27437=CARTESIAN_POINT('Ctrl Pts',(-20.8674180471858,16.8731674789966,123.794009449891)) ;
#27438=CARTESIAN_POINT('Ctrl Pts',(-20.5757870061501,16.6931783986337,123.717568881039)) ;
#27439=CARTESIAN_POINT('Ctrl Pts',(-20.7796283027966,16.8831147012677,124.04024353424)) ;
#27440=CARTESIAN_POINT('Ctrl Pts',(-20.5055557607933,16.7031256209048,123.91455585675)) ;
#27441=CARTESIAN_POINT('Ctrl Pts',(-20.6488602156385,16.8931627268478,124.269630633099)) ;
#27442=CARTESIAN_POINT('Ctrl Pts',(-20.4009414915831,16.7131736464849,124.0980658808)) ;
#27443=CARTESIAN_POINT('Ctrl Pts',(-20.4837823786232,16.9030099739907,124.468914512535)) ;
#27444=CARTESIAN_POINT('Ctrl Pts',(-20.2688802436977,16.7230208936278,124.257492376889)) ;
#27445=CARTESIAN_POINT('Ctrl Pts',(-20.2848296697992,16.9129731510814,124.639107596571)) ;
#27446=CARTESIAN_POINT('Ctrl Pts',(-20.1097187494631,16.7329840707186,124.393647070472)) ;
#27447=CARTESIAN_POINT('Ctrl Pts',(-20.0576375877666,16.9230028721148,124.772718133945)) ;
#27448=CARTESIAN_POINT('Ctrl Pts',(-19.9279652726105,16.743013791752,124.500535980068)) ;
#27449=CARTESIAN_POINT('Ctrl Pts',(-19.8138676646833,16.9329073396477,124.864008421836)) ;
#27450=CARTESIAN_POINT('Ctrl Pts',(-19.7329502140236,16.7529182592849,124.573568505699)) ;
#27451=CARTESIAN_POINT('Ctrl Pts',(-19.5549188176407,16.9429318254775,124.912240141092)) ;
#27452=CARTESIAN_POINT('Ctrl Pts',(-19.5257912019944,16.7629427451146,124.612154489046)) ;
#27453=CARTESIAN_POINT('Ctrl Pts',(-19.2946338276999,16.9528356606014,124.914963066489)) ;
#27454=CARTESIAN_POINT('Ctrl Pts',(-19.3175639397184,16.7728465802385,124.614333480641)) ;
#27455=CARTESIAN_POINT('Ctrl Pts',(-19.0340655773043,16.9628868513114,124.871886584455)) ;
#27456=CARTESIAN_POINT('Ctrl Pts',(-19.1091090337395,16.7828977709485,124.579872926838)) ;
#27457=CARTESIAN_POINT('Ctrl Pts',(-18.7889990253017,16.9727712939697,124.785703184415)) ;
#27458=CARTESIAN_POINT('Ctrl Pts',(-18.9130563598052,16.7927822136068,124.510927134029)) ;
#27459=CARTESIAN_POINT('Ctrl Pts',(-18.5599373549121,16.9827643018216,124.657327597577)) ;
#27460=CARTESIAN_POINT('Ctrl Pts',(-18.7298067701624,16.8027752214587,124.408227443796)) ;
#27461=CARTESIAN_POINT('Ctrl Pts',(-18.3575795915092,16.9927126215379,124.491777975001)) ;
#27462=CARTESIAN_POINT('Ctrl Pts',(-18.5679204008152,16.812723541175,124.275788625095)) ;
#27463=CARTESIAN_POINT('Ctrl Pts',(-18.186980138861,17.0026494602473,124.294109650112)) ;
#27464=CARTESIAN_POINT('Ctrl Pts',(-18.4314405125063,16.8226603798844,124.117654920075)) ;
#27465=CARTESIAN_POINT('Ctrl Pts',(-18.0523597654586,17.0126324491669,124.06890152174)) ;
#27466=CARTESIAN_POINT('Ctrl Pts',(-18.3237435055854,16.832643368804,123.93748907981)) ;
#27467=CARTESIAN_POINT('Ctrl Pts',(-17.9587951854769,17.022676328531,123.82213239202)) ;
#27468=CARTESIAN_POINT('Ctrl Pts',(-18.2488910084418,16.8426872481681,123.740073929916)) ;
#27469=CARTESIAN_POINT('Ctrl Pts',(-17.9099416408422,17.0325043938894,123.568481191394)) ;
#27470=CARTESIAN_POINT('Ctrl Pts',(-18.2098074301906,16.8525153135265,123.537154287906)) ;
#27471=CARTESIAN_POINT('Ctrl Pts',(-17.9056580144789,17.0425814824443,123.303759681484)) ;
#27472=CARTESIAN_POINT('Ctrl Pts',(-18.2063795179285,16.8625924020815,123.325376748704)) ;
#27473=CARTESIAN_POINT('Ctrl Pts',(-17.9463150166963,17.0524316346006,123.048052157451)) ;
#27474=CARTESIAN_POINT('Ctrl Pts',(-18.2389039336585,16.8724425542378,123.120811549314)) ;
#27475=CARTESIAN_POINT('Ctrl Pts',(-18.032582786432,17.062512115053,122.797658849589)) ;
#27476=CARTESIAN_POINT('Ctrl Pts',(-18.3079172569512,16.8825230346901,122.920496215202)) ;
#27477=CARTESIAN_POINT('Ctrl Pts',(-18.1574904407852,17.0723266128218,122.571941098829)) ;
#27478=CARTESIAN_POINT('Ctrl Pts',(-18.4078418212507,16.8923375324589,122.739922521317)) ;
#27479=CARTESIAN_POINT('Ctrl Pts',(-18.3234861663821,17.0823949088419,122.36598619016)) ;
#27480=CARTESIAN_POINT('Ctrl Pts',(-18.5406376345855,16.9024058284791,122.575157613041)) ;
#27481=CARTESIAN_POINT('Ctrl Pts',(-18.5195111943069,17.0922937413247,122.194881832912)) ;
#27482=CARTESIAN_POINT('Ctrl Pts',(-18.697456370269,16.9123046609618,122.438273670192)) ;
#27483=CARTESIAN_POINT('Ctrl Pts',(-18.7455842875903,17.1023466213392,122.058305557914)) ;
#27484=CARTESIAN_POINT('Ctrl Pts',(-18.878314382243,16.9223575409764,122.329011510998)) ;
#27485=CARTESIAN_POINT('Ctrl Pts',(-18.9874629412991,17.1122164368354,121.964526142813)) ;
#27486=CARTESIAN_POINT('Ctrl Pts',(-19.0718160746585,16.9322273564725,122.253987102022)) ;
#27487=CARTESIAN_POINT('Ctrl Pts',(-19.2470688770235,17.1222891179182,121.913081725806)) ;
#27488=CARTESIAN_POINT('Ctrl Pts',(-19.2795008526622,16.9423000375553,122.212830257528)) ;
#27489=CARTESIAN_POINT('Ctrl Pts',(-19.505422587486,17.1321215964892,121.907524515032)) ;
#27490=CARTESIAN_POINT('Ctrl Pts',(-19.4861827690057,16.9521325161263,122.208383209402)) ;
#27491=CARTESIAN_POINT('Ctrl Pts',(-19.7660419704814,17.1421522304753,121.946947546496)) ;
#27492=CARTESIAN_POINT('Ctrl Pts',(-19.6946785626933,16.9621631501124,122.239920201912)) ;
#27493=CARTESIAN_POINT('Ctrl Pts',(-20.0156574864725,17.1521837876944,122.031770159067)) ;
#27494=CARTESIAN_POINT('Ctrl Pts',(-19.8943714558458,16.9721947073315,122.307777083162)) ;
#27495=CARTESIAN_POINT('Ctrl Pts',(-20.2423350956265,17.1620134965661,122.155604235088)) ;
#27496=CARTESIAN_POINT('Ctrl Pts',(-20.075713330144,16.9820244162032,122.406842617996)) ;
#27497=CARTESIAN_POINT('Ctrl Pts',(-20.4478540416198,17.1720029453682,122.318940433098)) ;
#27498=CARTESIAN_POINT('Ctrl Pts',(-20.2401293518006,16.9920138650053,122.537510260585)) ;
#27499=CARTESIAN_POINT('Ctrl Pts',(-20.6223297569369,17.1820467977682,122.516986010216)) ;
#27500=CARTESIAN_POINT('Ctrl Pts',(-20.379711079171,17.0020577174053,122.69594586157)) ;
#27501=CARTESIAN_POINT('Ctrl Pts',(-20.7571853342976,17.1918685111003,122.737058592109)) ;
#27502=CARTESIAN_POINT('Ctrl Pts',(-20.4875963345862,17.0118794307374,122.872002271996)) ;
#27503=CARTESIAN_POINT('Ctrl Pts',(-20.8544363834582,17.201903516089,122.982179630652)) ;
#27504=CARTESIAN_POINT('Ctrl Pts',(-20.5653987506376,17.0219144357261,123.068098568077)) ;
#27505=CARTESIAN_POINT('Ctrl Pts',(-20.9068811373926,17.2119283545366,123.240357855693)) ;
#27506=CARTESIAN_POINT('Ctrl Pts',(-20.6073560524299,17.0319392741737,123.274640863138)) ;
#27507=CARTESIAN_POINT('Ctrl Pts',(-20.9141373279082,17.2217805674918,123.499162698651)) ;
#27508=CARTESIAN_POINT('Ctrl Pts',(-20.6131626102164,17.0417914871289,123.481683887994)) ;
#27509=CARTESIAN_POINT('Ctrl Pts',(-20.8762617532287,17.2317705236856,123.758921385039)) ;
#27510=CARTESIAN_POINT('Ctrl Pts',(-20.5828638652605,17.0517814433227,123.689490938947)) ;
#27511=CARTESIAN_POINT('Ctrl Pts',(-20.7943806135892,17.2416986339689,124.006649024893)) ;
#27512=CARTESIAN_POINT('Ctrl Pts',(-20.5173607099962,17.061709553606,123.887673192447)) ;
#27513=CARTESIAN_POINT('Ctrl Pts',(-20.670345385213,17.2516872340484,124.237992487124)) ;
#27514=CARTESIAN_POINT('Ctrl Pts',(-20.4181341594561,17.0716981536855,124.07274868766)) ;
#27515=CARTESIAN_POINT('Ctrl Pts',(-20.5071235397933,17.2617138259759,124.444842800166)) ;
#27516=CARTESIAN_POINT('Ctrl Pts',(-20.2875580171586,17.081724745613,124.23823002585)) ;
#27517=CARTESIAN_POINT('Ctrl Pts',(-20.3134293623449,17.2715989540401,124.617932746978)) ;
#27518=CARTESIAN_POINT('Ctrl Pts',(-20.1326042907807,17.0916098736772,124.376702907249)) ;
#27519=CARTESIAN_POINT('Ctrl Pts',(-20.0905573668405,17.2815900715136,124.756745161351)) ;
#27520=CARTESIAN_POINT('Ctrl Pts',(-19.9543077846783,17.1016009911507,124.487754352768)) ;
#27521=CARTESIAN_POINT('Ctrl Pts',(-19.8455645964301,17.2916306873654,124.854716110604)) ;
#27522=CARTESIAN_POINT('Ctrl Pts',(-19.7583141598722,17.1116416070025,124.566132786485)) ;
#27523=CARTESIAN_POINT('Ctrl Pts',(-19.5927130154484,17.3014636782191,124.907962066392)) ;
#27524=CARTESIAN_POINT('Ctrl Pts',(-19.5560340209557,17.1214745978562,124.60873119612)) ;
#27525=CARTESIAN_POINT('Ctrl Pts',(-19.330277450202,17.3114568096694,124.917387511024)) ;
#27526=CARTESIAN_POINT('Ctrl Pts',(-19.3460857391731,17.1314677293065,124.616273501047)) ;
#27527=CARTESIAN_POINT('Ctrl Pts',(-19.0692386893252,17.3214888581048,124.88041535309)) ;
#27528=CARTESIAN_POINT('Ctrl Pts',(-19.1372544392363,17.1414997777419,124.58669762411)) ;
#27529=CARTESIAN_POINT('Ctrl Pts',(-18.822677257513,17.3313541046472,124.800350459875)) ;
#27530=CARTESIAN_POINT('Ctrl Pts',(-18.9400052547958,17.1513650242843,124.522647715831)) ;
#27531=CARTESIAN_POINT('Ctrl Pts',(-18.5911545600622,17.341315979474,124.678145049276)) ;
#27532=CARTESIAN_POINT('Ctrl Pts',(-18.7547863323555,17.1613268991111,124.424885267182)) ;
#27533=CARTESIAN_POINT('Ctrl Pts',(-18.38313341919,17.3513509425853,124.516091097511)) ;
#27534=CARTESIAN_POINT('Ctrl Pts',(-18.5883681924007,17.1713618622224,124.295243637103)) ;
#27535=CARTESIAN_POINT('Ctrl Pts',(-18.2086914290502,17.3612357870477,124.323563591818)) ;
#27536=CARTESIAN_POINT('Ctrl Pts',(-18.4488134084025,17.1812467066848,124.1412233211)) ;
#27537=CARTESIAN_POINT('Ctrl Pts',(-18.0678947666769,17.3713018398884,124.099676485538)) ;
#27538=CARTESIAN_POINT('Ctrl Pts',(-18.3361743120959,17.1913127595256,123.962114606341)) ;
#27539=CARTESIAN_POINT('Ctrl Pts',(-17.9700726313909,17.3811393557974,123.860326944384)) ;
#27540=CARTESIAN_POINT('Ctrl Pts',(-18.2579149281125,17.2011502754345,123.770636270255)) ;
#27541=CARTESIAN_POINT('Ctrl Pts',(-17.9137531151006,17.3912081039063,123.601841075206)) ;
#27542=CARTESIAN_POINT('Ctrl Pts',(-18.2128572598282,17.2112190235434,123.563847905866)) ;
#27543=CARTESIAN_POINT('Ctrl Pts',(-17.9034613928053,17.4010886209373,123.342355402501)) ;
#27544=CARTESIAN_POINT('Ctrl Pts',(-18.2046218361467,17.2210995405744,123.356259859083)) ;
#27545=CARTESIAN_POINT('Ctrl Pts',(-17.9382344928248,17.4110798078718,123.082149155382)) ;
#27546=CARTESIAN_POINT('Ctrl Pts',(-18.2324382019981,17.2310907275089,123.148094673223)) ;
#27547=CARTESIAN_POINT('Ctrl Pts',(-18.0173408799565,17.4210328741467,122.832800782693)) ;
#27548=CARTESIAN_POINT('Ctrl Pts',(-18.2957212338474,17.2410437937838,122.948615510215)) ;
#27549=CARTESIAN_POINT('Ctrl Pts',(-18.1395964065383,17.4310687116793,122.599142062341)) ;
#27550=CARTESIAN_POINT('Ctrl Pts',(-18.3935237856952,17.2510796313164,122.761687546562)) ;
#27551=CARTESIAN_POINT('Ctrl Pts',(-18.2981116221672,17.4409588378907,122.393154239559)) ;
#27552=CARTESIAN_POINT('Ctrl Pts',(-18.5203340659042,17.2609697575279,122.596896255148)) ;
#27553=CARTESIAN_POINT('Ctrl Pts',(-18.4916578231572,17.4509510197987,122.215719190812)) ;
#27554=CARTESIAN_POINT('Ctrl Pts',(-18.6751695002837,17.2709619394358,122.454946675199)) ;
#27555=CARTESIAN_POINT('Ctrl Pts',(-18.7121069676179,17.4608969597373,122.075305569039)) ;
#27556=CARTESIAN_POINT('Ctrl Pts',(-18.8515275002128,17.2809078793744,122.342614056364)) ;
#27557=CARTESIAN_POINT('Ctrl Pts',(-18.9534274542707,17.4708441435014,121.974794440461)) ;
#27558=CARTESIAN_POINT('Ctrl Pts',(-19.0445828970662,17.2908550631385,122.262203186491)) ;
#27559=CARTESIAN_POINT('Ctrl Pts',(-19.211160386698,17.4808920818088,121.917426601221)) ;
#27560=CARTESIAN_POINT('Ctrl Pts',(-19.2507687776007,17.300903001446,122.216306788302)) ;
#27561=CARTESIAN_POINT('Ctrl Pts',(-19.4696824314095,17.4907397165491,121.905695967141)) ;
#27562=CARTESIAN_POINT('Ctrl Pts',(-19.4575859964064,17.3107506361862,122.206920105047)) ;
#27563=CARTESIAN_POINT('Ctrl Pts',(-19.7293772423961,17.5007014305229,121.938602055784)) ;
#27564=CARTESIAN_POINT('Ctrl Pts',(-19.6653420282454,17.3207123501601,122.233242742379)) ;
#27565=CARTESIAN_POINT('Ctrl Pts',(-19.9810217545707,17.5107300653138,122.016948020053)) ;
#27566=CARTESIAN_POINT('Ctrl Pts',(-19.8666582637803,17.3307409849509,122.295917385593)) ;
#27567=CARTESIAN_POINT('Ctrl Pts',(-20.2124907996332,17.5206403839109,122.136283881726)) ;
#27568=CARTESIAN_POINT('Ctrl Pts',(-20.0518343705786,17.340651303548,122.391384019584)) ;
#27569=CARTESIAN_POINT('Ctrl Pts',(-20.4206686080383,17.5305752402224,122.293854796919)) ;
#27570=CARTESIAN_POINT('Ctrl Pts',(-20.2183778909395,17.3505861598595,122.517438895075)) ;
#27571=CARTESIAN_POINT('Ctrl Pts',(-20.6000255828736,17.5406164761831,122.487384162176)) ;
#27572=CARTESIAN_POINT('Ctrl Pts',(-20.3618650889074,17.3606273958202,122.672260836499)) ;
#27573=CARTESIAN_POINT('Ctrl Pts',(-20.7410561133952,17.5505032477631,122.70562002418)) ;
#27574=CARTESIAN_POINT('Ctrl Pts',(-20.4746913307344,17.3705141674002,122.846848200213)) ;
#27575=CARTESIAN_POINT('Ctrl Pts',(-20.8434772707178,17.5605034264693,122.947591960567)) ;
#27576=CARTESIAN_POINT('Ctrl Pts',(-20.5566303111727,17.3805143461064,123.040424818321)) ;
#27577=CARTESIAN_POINT('Ctrl Pts',(-20.9020786278622,17.5704207046789,123.201578349681)) ;
#27578=CARTESIAN_POINT('Ctrl Pts',(-20.6035135750036,17.390431624316,123.24361335474)) ;
#27579=CARTESIAN_POINT('Ctrl Pts',(-20.91578288945,17.5804679510926,123.465216930615)) ;
#27580=CARTESIAN_POINT('Ctrl Pts',(-20.6144792336198,17.4004788707297,123.454524044763)) ;
#27581=CARTESIAN_POINT('Ctrl Pts',(-20.8843256015444,17.5903418400739,123.722819361991)) ;
#27582=CARTESIAN_POINT('Ctrl Pts',(-20.5893156441907,17.410352759711,123.660606216813)) ;
#27583=CARTESIAN_POINT('Ctrl Pts',(-20.8073356878369,17.6004038576544,123.975747950634)) ;
#27584=CARTESIAN_POINT('Ctrl Pts',(-20.527725890698,17.4204147772915,123.862949679042)) ;
#27585=CARTESIAN_POINT('Ctrl Pts',(-20.6898154915697,17.6102749193887,124.207021563565)) ;
#27586=CARTESIAN_POINT('Ctrl Pts',(-20.4337117468578,17.4302858390258,124.047969580495)) ;
#27587=CARTESIAN_POINT('Ctrl Pts',(-20.5325789116341,17.620268982749,124.417385133982)) ;
#27588=CARTESIAN_POINT('Ctrl Pts',(-20.307924299848,17.4402799023861,124.216261749645)) ;
#27589=CARTESIAN_POINT('Ctrl Pts',(-20.3400800616733,17.6303011407824,124.597505830153)) ;
#27590=CARTESIAN_POINT('Ctrl Pts',(-20.1539268192864,17.4503120604195,124.360359893607)) ;
#27591=CARTESIAN_POINT('Ctrl Pts',(-20.1232165512678,17.6401650170226,124.739545873156)) ;
#27592=CARTESIAN_POINT('Ctrl Pts',(-19.9804371926355,17.4601759366597,124.473993837202)) ;
#27593=CARTESIAN_POINT('Ctrl Pts',(-19.8800594521067,17.6502355316608,124.843920027478)) ;
#27594=CARTESIAN_POINT('Ctrl Pts',(-19.7859124646786,17.470246451298,124.557495161762)) ;
#27595=CARTESIAN_POINT('Ctrl Pts',(-19.6283095577294,17.6600761686018,124.90314183829)) ;
#27596=CARTESIAN_POINT('Ctrl Pts',(-19.5845130945949,17.4800870882389,124.60487484599)) ;
#27597=CARTESIAN_POINT('Ctrl Pts',(-19.366875274711,17.670043297442,124.918801259543)) ;
#27598=CARTESIAN_POINT('Ctrl Pts',(-19.375365146763,17.4900542170791,124.61740447096)) ;
#27599=CARTESIAN_POINT('Ctrl Pts',(-19.1054626465016,17.6800572705665,124.888408905222)) ;
#27600=CARTESIAN_POINT('Ctrl Pts',(-19.1662371963715,17.5000681902037,124.593093168698)) ;
#27601=CARTESIAN_POINT('Ctrl Pts',(-18.7709105569482,17.6933420044298,124.788587304081)) ;
#27602=CARTESIAN_POINT('Ctrl Pts',(-18.8985830635496,17.5133529240669,124.513236786793)) ;
#27603=CARTESIAN_POINT('Ctrl Pts',(-18.4713115759659,17.7065672691446,124.604860086354)) ;
#27604=CARTESIAN_POINT('Ctrl Pts',(-18.6588815387832,17.5265781887817,124.36623312436)) ;
#27605=CARTESIAN_POINT('Ctrl Pts',(-18.23024753484,17.7198777916994,124.351352544017)) ;
#27606=CARTESIAN_POINT('Ctrl Pts',(-18.4660643742217,17.5398887113366,124.163459835131)) ;
#27607=CARTESIAN_POINT('Ctrl Pts',(-18.0847456433107,17.7299064366016,124.131627885447)) ;
#27608=CARTESIAN_POINT('Ctrl Pts',(-18.3496538990184,17.5499173562387,123.987675132136)) ;
#27609=CARTESIAN_POINT('Ctrl Pts',(-17.9809344252587,17.7397874689555,123.893612632043)) ;
#27610=CARTESIAN_POINT('Ctrl Pts',(-18.2666046634578,17.5597983885926,123.797265517451)) ;
#27611=CARTESIAN_POINT('Ctrl Pts',(-17.9188829813947,17.7497684416356,123.638771587196)) ;
#27612=CARTESIAN_POINT('Ctrl Pts',(-18.2169614863476,17.5697793612727,123.593391459913)) ;
#27613=CARTESIAN_POINT('Ctrl Pts',(-17.9022490540845,17.7597495692216,123.377020959202)) ;
#27614=CARTESIAN_POINT('Ctrl Pts',(-18.2036504220169,17.5797604888587,123.383995815664)) ;
#27615=CARTESIAN_POINT('Ctrl Pts',(-17.940086062115,17.772992759483,123.030998917188)) ;
#27616=CARTESIAN_POINT('Ctrl Pts',(-18.233927074126,17.5930036791201,123.10715455913)) ;
#27617=CARTESIAN_POINT('Ctrl Pts',(-18.1006895820262,17.7896607548438,122.618237447441)) ;
#27618=CARTESIAN_POINT('Ctrl Pts',(-18.3623849444853,17.6096716744809,122.776980015619)) ;
#27619=CARTESIAN_POINT('Ctrl Pts',(-18.3897812209932,17.8061812548558,122.28765824502)) ;
#27620=CARTESIAN_POINT('Ctrl Pts',(-18.5937018866241,17.626192174493,122.512467686169)) ;
#27621=CARTESIAN_POINT('Ctrl Pts',(-18.6800705190158,17.8194942711718,122.092466331838)) ;
#27622=CARTESIAN_POINT('Ctrl Pts',(-18.8258934626634,17.639505190809,122.356347530936)) ;
#27623=CARTESIAN_POINT('Ctrl Pts',(-18.9181973224567,17.8294108294048,121.986503440751)) ;
#27624=CARTESIAN_POINT('Ctrl Pts',(-19.016402860702,17.649421749042,122.271568344734)) ;
#27625=CARTESIAN_POINT('Ctrl Pts',(-19.1738622433935,17.8394384977077,121.92290647105)) ;
#27626=CARTESIAN_POINT('Ctrl Pts',(-19.2209295533305,17.6594494173448,122.220690413991)) ;
#27627=CARTESIAN_POINT('Ctrl Pts',(-19.5194723945054,17.8526190874524,121.898080551952)) ;
#27628=CARTESIAN_POINT('Ctrl Pts',(-19.4974317792493,17.6726300070895,122.200829004453)) ;
#27629=CARTESIAN_POINT('Ctrl Pts',(-19.9563231936178,17.8693672265717,121.982455382444)) ;
#27630=CARTESIAN_POINT('Ctrl Pts',(-19.8468977311799,17.6893781462089,122.268323444308)) ;
#27631=CARTESIAN_POINT('Ctrl Pts',(-20.4081951552472,17.8891619690823,122.252387033747)) ;
#27632=CARTESIAN_POINT('Ctrl Pts',(-20.2084028189433,17.7091728887194,122.484267129473)) ;
#27633=CARTESIAN_POINT('Ctrl Pts',(-20.7451718132866,17.9092063618911,122.66478304066)) ;
#27634=CARTESIAN_POINT('Ctrl Pts',(-20.4779852136411,17.7292172815282,122.814181443718)) ;
#27635=CARTESIAN_POINT('Ctrl Pts',(-20.9190608630453,17.9290455441898,123.162728597956)) ;
#27636=CARTESIAN_POINT('Ctrl Pts',(-20.6171002151294,17.7490564638269,123.212537829593)) ;
#27637=CARTESIAN_POINT('Ctrl Pts',(-20.9138698455996,17.9489708678827,123.692157121899)) ;
#27638=CARTESIAN_POINT('Ctrl Pts',(-20.6129501230136,17.7689817875198,123.636081264938)) ;
#27639=CARTESIAN_POINT('Ctrl Pts',(-20.7282004987486,17.9688945059342,124.188169695646)) ;
#27640=CARTESIAN_POINT('Ctrl Pts',(-20.4644169876035,17.7889054255713,124.032892793635)) ;
#27641=CARTESIAN_POINT('Ctrl Pts',(-20.3846133570625,17.9888193793997,124.591069561661)) ;
#27642=CARTESIAN_POINT('Ctrl Pts',(-20.1895487840061,17.8088302990368,124.355214802049)) ;
#27643=CARTESIAN_POINT('Ctrl Pts',(-19.9254924402877,18.0086979864787,124.852574068712)) ;
#27644=CARTESIAN_POINT('Ctrl Pts',(-19.8222521396401,17.8287089061158,124.564420818094)) ;
#27645=CARTESIAN_POINT('Ctrl Pts',(-19.4021887856867,18.0286754293106,124.94239921452)) ;
#27646=CARTESIAN_POINT('Ctrl Pts',(-19.403609335955,17.8486863489478,124.636282835405)) ;
#27647=CARTESIAN_POINT('Ctrl Pts',(-18.8808448567372,18.0486072773953,124.848094480769)) ;
#27648=CARTESIAN_POINT('Ctrl Pts',(-18.9865332449473,17.8686181970324,124.560840796153)) ;
#27649=CARTESIAN_POINT('Ctrl Pts',(-18.4236271458194,18.0685025457379,124.582520931676)) ;
#27650=CARTESIAN_POINT('Ctrl Pts',(-18.620757360624,17.888513465375,124.348382725567)) ;
#27651=CARTESIAN_POINT('Ctrl Pts',(-18.083533966346,18.08842504415,124.176653707817)) ;
#27652=CARTESIAN_POINT('Ctrl Pts',(-18.3486814135184,17.9084359637871,124.023689002201)) ;
#27653=CARTESIAN_POINT('Ctrl Pts',(-17.9021445000866,18.108384526026,123.678105539859)) ;
#27654=CARTESIAN_POINT('Ctrl Pts',(-18.2035687540983,17.9283954456631,123.624850383669)) ;
#27655=CARTESIAN_POINT('Ctrl Pts',(-17.901677043034,18.1282622784854,123.149870596743)) ;
#27656=CARTESIAN_POINT('Ctrl Pts',(-18.2031940192158,17.9482731981225,123.202260912629)) ;
#27657=CARTESIAN_POINT('Ctrl Pts',(-18.0801792550787,18.1481440692199,122.65239779122)) ;
#27658=CARTESIAN_POINT('Ctrl Pts',(-18.3459964494123,17.9681549888571,122.804281306169)) ;
#27659=CARTESIAN_POINT('Ctrl Pts',(-18.4216843162061,18.1682174080709,122.242598944837)) ;
#27660=CARTESIAN_POINT('Ctrl Pts',(-18.6191997939776,17.988228327708,122.476442865587)) ;
#27661=CARTESIAN_POINT('Ctrl Pts',(-18.8764446818162,18.1880218753067,121.977323375824)) ;
#27662=CARTESIAN_POINT('Ctrl Pts',(-18.983010300815,18.0080327949438,122.26422127326)) ;
#27663=CARTESIAN_POINT('Ctrl Pts',(-19.3987200282656,18.2080052157145,121.881178045719)) ;
#27664=CARTESIAN_POINT('Ctrl Pts',(-19.4008309101687,18.0280161353516,122.187305861256)) ;
#27665=CARTESIAN_POINT('Ctrl Pts',(-19.9205934708167,18.2279201803125,121.969578565073)) ;
#27666=CARTESIAN_POINT('Ctrl Pts',(-19.8183305317221,18.0479310999496,122.258027130134)) ;
#27667=CARTESIAN_POINT('Ctrl Pts',(-20.3807158505364,18.2477887150289,122.228912632756)) ;
#27668=CARTESIAN_POINT('Ctrl Pts',(-20.1864289023512,18.067799634666,122.465496375139)) ;
#27669=CARTESIAN_POINT('Ctrl Pts',(-20.7270809482803,18.2678410992406,122.6337729235)) ;
#27670=CARTESIAN_POINT('Ctrl Pts',(-20.4635196475679,18.0878520188777,122.789385098956)) ;
#27671=CARTESIAN_POINT('Ctrl Pts',(-20.9126860426018,18.2876150630298,123.125692137824)) ;
#27672=CARTESIAN_POINT('Ctrl Pts',(-20.6120028561782,18.1076259826669,123.182923161825)) ;
#27673=CARTESIAN_POINT('Ctrl Pts',(-20.919787056096,18.3076694420512,123.658444810698)) ;
#27674=CARTESIAN_POINT('Ctrl Pts',(-20.6176815610967,18.1276803616883,123.609124837985)) ;
#27675=CARTESIAN_POINT('Ctrl Pts',(-20.7465962162573,18.3274661796244,124.155452562203)) ;
#27676=CARTESIAN_POINT('Ctrl Pts',(-20.4791262659657,18.1474770992615,124.006732040671)) ;
#27677=CARTESIAN_POINT('Ctrl Pts',(-20.4126446942546,18.3474339919759,124.567768827108)) ;
#27678=CARTESIAN_POINT('Ctrl Pts',(-20.2119627251939,18.167444911613,124.336583477204)) ;
#27679=CARTESIAN_POINT('Ctrl Pts',(-19.9576212451287,18.3673929680409,124.840656736435)) ;
#27680=CARTESIAN_POINT('Ctrl Pts',(-19.8479423832508,18.187403887678,124.554891689415)) ;
#27681=CARTESIAN_POINT('Ctrl Pts',(-19.4386451944303,18.3872878863183,124.941871042673)) ;
#27682=CARTESIAN_POINT('Ctrl Pts',(-19.4327602304496,18.2072988059554,124.635860461353)) ;
#27683=CARTESIAN_POINT('Ctrl Pts',(-18.9161726453232,18.4071841987686,124.860555263088)) ;
#27684=CARTESIAN_POINT('Ctrl Pts',(-19.0147819951874,18.2271951184057,124.570804600373)) ;
#27685=CARTESIAN_POINT('Ctrl Pts',(-18.4521815633956,18.4270921321427,124.606153931591)) ;
#27686=CARTESIAN_POINT('Ctrl Pts',(-18.6435902854391,18.2471030517799,124.367280294003)) ;
#27687=CARTESIAN_POINT('Ctrl Pts',(-18.1022181077,18.4470420224312,124.207874213592)) ;
#27688=CARTESIAN_POINT('Ctrl Pts',(-18.3636220163142,18.2670529420683,124.048653992795)) ;
#27689=CARTESIAN_POINT('Ctrl Pts',(-17.9093397630461,18.4669192529325,123.715982843254)) ;
#27690=CARTESIAN_POINT('Ctrl Pts',(-18.2093224069639,18.2869301725696,123.655139058645)) ;
#27691=CARTESIAN_POINT('Ctrl Pts',(-17.8955552161801,18.4869019218035,123.185081472576)) ;
#27692=CARTESIAN_POINT('Ctrl Pts',(-18.1982991666636,18.3069128414406,123.230417568849)) ;
#27693=CARTESIAN_POINT('Ctrl Pts',(-18.0637189576036,18.5068348083839,122.682625101242)) ;
#27694=CARTESIAN_POINT('Ctrl Pts',(-18.3328317622398,18.326845728021,122.82845440733)) ;
#27695=CARTESIAN_POINT('Ctrl Pts',(-18.3925705510188,18.5267475544018,122.267998602716)) ;
#27696=CARTESIAN_POINT('Ctrl Pts',(-18.5959242479568,18.3467584740389,122.496751834392)) ;
#27697=CARTESIAN_POINT('Ctrl Pts',(-18.767281881698,18.5433172757436,122.036622749478)) ;
#27698=CARTESIAN_POINT('Ctrl Pts',(-18.8956708387233,18.3633281953808,122.311665074245)) ;
#27699=CARTESIAN_POINT('Ctrl Pts',(-19.1020056145289,18.5566172870486,121.936011376313)) ;
#27700=CARTESIAN_POINT('Ctrl Pts',(-19.1634797346767,18.3766282066857,122.231169157369)) ;
#27701=CARTESIAN_POINT('Ctrl Pts',(-19.4482877506077,18.5698874747985,121.89465138511)) ;
#27702=CARTESIAN_POINT('Ctrl Pts',(-19.4404490281102,18.3898983944356,122.198083477283)) ;
#27703=CARTESIAN_POINT('Ctrl Pts',(-19.8857560482088,18.5865148571639,121.957313792384)) ;
#27704=CARTESIAN_POINT('Ctrl Pts',(-19.7904920476466,18.406525776801,122.248222840253)) ;
#27705=CARTESIAN_POINT('Ctrl Pts',(-20.2753787251303,18.6031371469091,122.165595250357)) ;
#27706=CARTESIAN_POINT('Ctrl Pts',(-20.1021439506729,18.4231480665462,122.414835475618)) ;
#27707=CARTESIAN_POINT('Ctrl Pts',(-20.5295847929134,18.6163823613036,122.403352527217)) ;
#27708=CARTESIAN_POINT('Ctrl Pts',(-20.3055329796882,18.4363932809408,122.60505706455)) ;
#27709=CARTESIAN_POINT('Ctrl Pts',(-20.6866624263127,18.6262943262643,122.611158628173)) ;
#27710=CARTESIAN_POINT('Ctrl Pts',(-20.4311881581819,18.4463052459014,122.771300643665)) ;
#27711=CARTESIAN_POINT('Ctrl Pts',(-20.8067318368115,18.6363529494288,122.846612050245)) ;
#27712=CARTESIAN_POINT('Ctrl Pts',(-20.5272430699789,18.4563638690659,122.959664983458)) ;
#27713=CARTESIAN_POINT('Ctrl Pts',(-20.882799746978,18.6461930635446,123.093798587262)) ;
#27714=CARTESIAN_POINT('Ctrl Pts',(-20.5880949652043,18.4662039831817,123.157414861851)) ;
#27715=CARTESIAN_POINT('Ctrl Pts',(-20.9157793856879,18.6562588485022,123.356213554678)) ;
#27716=CARTESIAN_POINT('Ctrl Pts',(-20.6144765429298,18.4762697681393,123.367347025587)) ;
#27717=CARTESIAN_POINT('Ctrl Pts',(-20.9028157443252,18.6661421662901,123.615646798569)) ;
#27718=CARTESIAN_POINT('Ctrl Pts',(-20.6041033763825,18.4861530859272,123.574893593804)) ;
#27719=CARTESIAN_POINT('Ctrl Pts',(-20.8449533316139,18.6761316041487,123.871675964814)) ;
#27720=CARTESIAN_POINT('Ctrl Pts',(-20.5578112681338,18.4961425237858,123.779716386074)) ;
#27721=CARTESIAN_POINT('Ctrl Pts',(-20.7436744284095,18.6860953182014,124.113145006398)) ;
#27722=CARTESIAN_POINT('Ctrl Pts',(-20.4767860825283,18.5061062378385,123.972890731368)) ;
#27723=CARTESIAN_POINT('Ctrl Pts',(-20.6017905558508,18.6960903298606,124.334207674781)) ;
#27724=CARTESIAN_POINT('Ctrl Pts',(-20.3632771185327,18.5161012494978,124.149739604004)) ;
#27725=CARTESIAN_POINT('Ctrl Pts',(-20.4226612590053,18.7061266215549,124.527770408748)) ;
#27726=CARTESIAN_POINT('Ctrl Pts',(-20.2199720814813,18.526137541192,124.304588217699)) ;
#27727=CARTESIAN_POINT('Ctrl Pts',(-20.2168518529892,18.7159729992483,124.684624557531)) ;
#27728=CARTESIAN_POINT('Ctrl Pts',(-20.0553231661172,18.5359839188854,124.430069764472)) ;
#27729=CARTESIAN_POINT('Ctrl Pts',(-19.9839760536042,18.725957943399,124.805452933041)) ;
#27730=CARTESIAN_POINT('Ctrl Pts',(-19.8690215418316,18.5459688630361,124.526730426201)) ;
#27731=CARTESIAN_POINT('Ctrl Pts',(-19.7348307743134,18.735894914529,124.883803103654)) ;
#27732=CARTESIAN_POINT('Ctrl Pts',(-19.6697046968684,18.5559058341661,124.589408393291)) ;
#27733=CARTESIAN_POINT('Ctrl Pts',(-19.4729748038764,18.7459446991607,124.917940423187)) ;
#27734=CARTESIAN_POINT('Ctrl Pts',(-19.4602196750584,18.5659556187978,124.616716001048)) ;
#27735=CARTESIAN_POINT('Ctrl Pts',(-19.21434799551,18.7557951612382,124.906522324717)) ;
#27736=CARTESIAN_POINT('Ctrl Pts',(-19.2533184225446,18.5758060808753,124.607579270633)) ;
#27737=CARTESIAN_POINT('Ctrl Pts',(-18.9584174462669,18.7657671747586,124.850357148989)) ;
#27738=CARTESIAN_POINT('Ctrl Pts',(-19.0485745563845,18.5857780943957,124.562644952603)) ;
#27739=CARTESIAN_POINT('Ctrl Pts',(-18.7155078312172,18.775762321878,124.750315034863)) ;
#27740=CARTESIAN_POINT('Ctrl Pts',(-18.8542477777451,18.5957732415151,124.48260921036)) ;
#27741=CARTESIAN_POINT('Ctrl Pts',(-18.493022848757,18.7857962916141,124.608834245128)) ;
#27742=CARTESIAN_POINT('Ctrl Pts',(-18.6762610286674,18.6058072112512,124.369422690082)) ;
#27743=CARTESIAN_POINT('Ctrl Pts',(-18.3016334315015,18.7956518372847,124.434305714712)) ;
#27744=CARTESIAN_POINT('Ctrl Pts',(-18.5231511449158,18.6156627569218,124.229798335907)) ;
#27745=CARTESIAN_POINT('Ctrl Pts',(-18.140904940295,18.8056505942979,124.226495189743)) ;
#27746=CARTESIAN_POINT('Ctrl Pts',(-18.394570163324,18.6256615139351,124.063548607924)) ;
#27747=CARTESIAN_POINT('Ctrl Pts',(-18.019684455447,18.8155477295351,123.99634137885)) ;
#27748=CARTESIAN_POINT('Ctrl Pts',(-18.2975958304662,18.6355586491722,123.87942470902)) ;
#27749=CARTESIAN_POINT('Ctrl Pts',(-17.93899129175,18.8256008253747,123.744810345997)) ;
#27750=CARTESIAN_POINT('Ctrl Pts',(-18.2330434068114,18.6456117450119,123.678199198287)) ;
#27751=CARTESIAN_POINT('Ctrl Pts',(-17.9037702162779,18.8354843341053,123.487463211661)) ;
#27752=CARTESIAN_POINT('Ctrl Pts',(-18.2048687720169,18.6554952537425,123.472321440138)) ;
#27753=CARTESIAN_POINT('Ctrl Pts',(-17.9132654845491,18.8454792067514,123.224988077224)) ;
#27754=CARTESIAN_POINT('Ctrl Pts',(-18.2124671563329,18.6654901263886,123.262341496769)) ;
#27755=CARTESIAN_POINT('Ctrl Pts',(-17.9687343278623,18.8554991683871,122.967567757792)) ;
#27756=CARTESIAN_POINT('Ctrl Pts',(-18.2568443761274,18.6755100880243,123.056405729243)) ;
#27757=CARTESIAN_POINT('Ctrl Pts',(-18.0667115840973,18.865404532187,122.726412358638)) ;
#27758=CARTESIAN_POINT('Ctrl Pts',(-18.3352281137652,18.6854154518241,122.863482464888)) ;
#27759=CARTESIAN_POINT('Ctrl Pts',(-18.2051056278125,18.8753451197945,122.504876382137)) ;
#27760=CARTESIAN_POINT('Ctrl Pts',(-18.4459450547457,18.6953560394316,122.68625500378)) ;
#27761=CARTESIAN_POINT('Ctrl Pts',(-18.3808775940096,18.8853479378952,122.309383985207)) ;
#27762=CARTESIAN_POINT('Ctrl Pts',(-18.5865641665979,18.7053588575323,122.529862558861)) ;
#27763=CARTESIAN_POINT('Ctrl Pts',(-18.5888129419843,18.8953826496193,122.147230647452)) ;
#27764=CARTESIAN_POINT('Ctrl Pts',(-18.7529137900349,18.7153935692564,122.40014159165)) ;
#27765=CARTESIAN_POINT('Ctrl Pts',(-18.8171608789422,18.9052275563566,122.025580674038)) ;
#27766=CARTESIAN_POINT('Ctrl Pts',(-18.9355927397188,18.7252384759937,122.302823704996)) ;
#27767=CARTESIAN_POINT('Ctrl Pts',(-19.066475495053,18.9152134089256,121.943828689904)) ;
#27768=CARTESIAN_POINT('Ctrl Pts',(-19.1350449591221,18.7352243285627,122.237424137714)) ;
#27769=CARTESIAN_POINT('Ctrl Pts',(-19.3249330398174,18.9251482173387,121.906600838846)) ;
#27770=CARTESIAN_POINT('Ctrl Pts',(-19.3418110288155,18.7451591369758,122.207643930442)) ;
#27771=CARTESIAN_POINT('Ctrl Pts',(-19.5890580305708,18.9352057444197,121.915149697282)) ;
#27772=CARTESIAN_POINT('Ctrl Pts',(-19.5531110478041,18.7552166640568,122.214485107576)) ;
#27773=CARTESIAN_POINT('Ctrl Pts',(-19.8417664438443,18.9450273994168,121.967782613312)) ;
#27774=CARTESIAN_POINT('Ctrl Pts',(-19.7552767463782,18.7650383190539,122.256593308813)) ;
#27775=CARTESIAN_POINT('Ctrl Pts',(-20.0873540689241,18.9550834435898,122.065301218056)) ;
#27776=CARTESIAN_POINT('Ctrl Pts',(-19.9517461977428,18.775094363227,122.334610067724)) ;
#27777=CARTESIAN_POINT('Ctrl Pts',(-20.3094798342934,18.965024183635,122.20280861514)) ;
#27778=CARTESIAN_POINT('Ctrl Pts',(-20.1294455077566,18.7850351032721,122.444617579698)) ;
#27779=CARTESIAN_POINT('Ctrl Pts',(-20.5041752042223,18.9749283047079,122.375539516404)) ;
#27780=CARTESIAN_POINT('Ctrl Pts',(-20.2852002006892,18.794939224345,122.582803465436)) ;
#27781=CARTESIAN_POINT('Ctrl Pts',(-20.6681231446912,18.9849758458621,122.58248803559)) ;
#27782=CARTESIAN_POINT('Ctrl Pts',(-20.416357069613,18.8049867654992,122.748363557921)) ;
#27783=CARTESIAN_POINT('Ctrl Pts',(-20.7919825435621,18.9948745974625,122.811275811282)) ;
#27784=CARTESIAN_POINT('Ctrl Pts',(-20.5154426771701,18.8148855170996,122.931394296776)) ;
#27785=CARTESIAN_POINT('Ctrl Pts',(-20.8755683816824,19.0049230764283,123.061730492506)) ;
#27786=CARTESIAN_POINT('Ctrl Pts',(-20.5823095619046,18.8249339960654,123.131758740942)) ;
#27787=CARTESIAN_POINT('Ctrl Pts',(-20.9138033739238,19.014810573512,123.318762800787)) ;
#27788=CARTESIAN_POINT('Ctrl Pts',(-20.612895591588,18.8348214931492,123.33738436397)) ;
#27789=CARTESIAN_POINT('Ctrl Pts',(-20.9072423074913,19.0248036638101,123.581265757207)) ;
#27790=CARTESIAN_POINT('Ctrl Pts',(-20.6076449012029,18.8448145834472,123.547386559869)) ;
#27791=CARTESIAN_POINT('Ctrl Pts',(-20.8553184944048,19.0347558338704,123.837608299615)) ;
#27792=CARTESIAN_POINT('Ctrl Pts',(-20.5661040904152,18.8547667535075,123.752459944652)) ;
#27793=CARTESIAN_POINT('Ctrl Pts',(-20.7601517684657,19.0446942537849,124.080804362951)) ;
#27794=CARTESIAN_POINT('Ctrl Pts',(-20.4899691655713,18.864705173422,123.947015810628)) ;
#27795=CARTESIAN_POINT('Ctrl Pts',(-20.6237942335491,19.0546793838705,124.305021774752)) ;
#27796=CARTESIAN_POINT('Ctrl Pts',(-20.3808817246997,18.8746903035076,124.126388699509)) ;
#27797=CARTESIAN_POINT('Ctrl Pts',(-20.4494165139908,19.0647160732846,124.502884010772)) ;
#27798=CARTESIAN_POINT('Ctrl Pts',(-20.2413781403973,18.8847269929217,124.284677342677)) ;
#27799=CARTESIAN_POINT('Ctrl Pts',(-20.2472957009717,19.0745707572771,124.664826057112)) ;
#27800=CARTESIAN_POINT('Ctrl Pts',(-20.0796809747905,18.8945816769142,124.414229158598)) ;
#27801=CARTESIAN_POINT('Ctrl Pts',(-20.0170234288064,19.0845702413249,124.791326058903)) ;
#27802=CARTESIAN_POINT('Ctrl Pts',(-19.8954624401579,18.9045811609621,124.515427632247)) ;
#27803=CARTESIAN_POINT('Ctrl Pts',(-19.7708869846679,19.0944653301018,124.875329679388)) ;
#27804=CARTESIAN_POINT('Ctrl Pts',(-19.6985533150144,18.914476249739,124.582628795942)) ;
#27805=CARTESIAN_POINT('Ctrl Pts',(-19.5096800897201,19.104525884748,124.915950078661)) ;
#27806=CARTESIAN_POINT('Ctrl Pts',(-19.4895873565871,18.9245368043851,124.61512352611)) ;
#27807=CARTESIAN_POINT('Ctrl Pts',(-19.2508813050788,19.1143751491209,124.910856545189)) ;
#27808=CARTESIAN_POINT('Ctrl Pts',(-19.2825491948916,18.934386068758,124.611047106101)) ;
#27809=CARTESIAN_POINT('Ctrl Pts',(-18.99220707569,19.1244024015687,124.86066175785)) ;
#27810=CARTESIAN_POINT('Ctrl Pts',(-19.0756100641405,18.9444133212059,124.570889813033)) ;
#27811=CARTESIAN_POINT('Ctrl Pts',(-18.7463833099064,19.1344306991389,124.765652294078)) ;
#27812=CARTESIAN_POINT('Ctrl Pts',(-18.8789515818906,18.954441618776,124.49488071212)) ;
#27813=CARTESIAN_POINT('Ctrl Pts',(-18.5246504442198,19.1442768281449,124.632315524006)) ;
#27814=CARTESIAN_POINT('Ctrl Pts',(-18.7015668443456,18.964287747782,124.388210457223)) ;
#27815=CARTESIAN_POINT('Ctrl Pts',(-18.3260692253604,19.154270733507,124.460445802928)) ;
#27816=CARTESIAN_POINT('Ctrl Pts',(-18.54270288402,18.9742816531441,124.250713721188)) ;
#27817=CARTESIAN_POINT('Ctrl Pts',(-18.1602075359614,19.16429483119,124.255787351941)) ;
#27818=CARTESIAN_POINT('Ctrl Pts',(-18.4100146618778,18.9843057508271,124.0869859934)) ;
#27819=CARTESIAN_POINT('Ctrl Pts',(-18.0338280399953,19.174184659044,124.028684394348)) ;
#27820=CARTESIAN_POINT('Ctrl Pts',(-18.3089126375273,18.9941955786812,123.905303536338)) ;
#27821=CARTESIAN_POINT('Ctrl Pts',(-17.947565914458,19.1841766404745,123.780690475578)) ;
#27822=CARTESIAN_POINT('Ctrl Pts',(-18.2399042544237,19.0041875601116,123.706908101772)) ;
#27823=CARTESIAN_POINT('Ctrl Pts',(-17.9059220811503,19.1941236452403,123.522631607328)) ;
#27824=CARTESIAN_POINT('Ctrl Pts',(-18.2065905909474,19.0141345648774,123.500461190172)) ;
#27825=CARTESIAN_POINT('Ctrl Pts',(-17.9092390395663,19.2040732966301,123.261175270493)) ;
#27826=CARTESIAN_POINT('Ctrl Pts',(-18.2092454041741,19.0240842162672,123.291296521161)) ;
#27827=CARTESIAN_POINT('Ctrl Pts',(-17.958538306793,19.2141102996075,123.002069408009)) ;
#27828=CARTESIAN_POINT('Ctrl Pts',(-18.2486861142578,19.0341212192446,123.084011970538)) ;
#27829=CARTESIAN_POINT('Ctrl Pts',(-18.0505326598567,19.2239992080425,122.759016798404)) ;
#27830=CARTESIAN_POINT('Ctrl Pts',(-18.3222825144302,19.0440101276797,122.88957101701)) ;
#27831=CARTESIAN_POINT('Ctrl Pts',(-18.1842635126106,19.23398854052,122.533132432072)) ;
#27832=CARTESIAN_POINT('Ctrl Pts',(-18.429268104139,19.0539994601571,122.708864261039)) ;
#27833=CARTESIAN_POINT('Ctrl Pts',(-18.3548053010277,19.2439470959571,122.334641591459)) ;
#27834=CARTESIAN_POINT('Ctrl Pts',(-18.5657022198966,19.0639580155942,122.550072634139)) ;
#27835=CARTESIAN_POINT('Ctrl Pts',(-18.5556335270977,19.2538466671576,122.169248739393)) ;
#27836=CARTESIAN_POINT('Ctrl Pts',(-18.7263649283418,19.0738575867947,122.417759614696)) ;
#27837=CARTESIAN_POINT('Ctrl Pts',(-18.7855306745994,19.2638945924096,122.039423510114)) ;
#27838=CARTESIAN_POINT('Ctrl Pts',(-18.910283328349,19.0839055120467,122.313900283675)) ;
#27839=CARTESIAN_POINT('Ctrl Pts',(-19.0306926009335,19.2737898919356,121.952607002251)) ;
#27840=CARTESIAN_POINT('Ctrl Pts',(-19.1064125243075,19.0938008115727,122.244448292274)) ;
#27841=CARTESIAN_POINT('Ctrl Pts',(-19.2914444276105,19.2838517483836,121.908933829335)) ;
#27842=CARTESIAN_POINT('Ctrl Pts',(-19.3150144124183,19.1038626680207,122.209510720343)) ;
#27843=CARTESIAN_POINT('Ctrl Pts',(-19.5501343610573,19.2936955948002,121.911097613413)) ;
#27844=CARTESIAN_POINT('Ctrl Pts',(-19.5219652921603,19.1137065144373,122.211242751695)) ;
#27845=CARTESIAN_POINT('Ctrl Pts',(-19.8077343935755,19.3036585439283,121.957822195286)) ;
#27846=CARTESIAN_POINT('Ctrl Pts',(-19.7280448206616,19.1236694635654,122.248623138328)) ;
#27847=CARTESIAN_POINT('Ctrl Pts',(-20.0549291177178,19.3136925803563,122.049626315006)) ;
#27848=CARTESIAN_POINT('Ctrl Pts',(-19.9258003882064,19.1337034999934,122.322067316074)) ;
#27849=CARTESIAN_POINT('Ctrl Pts',(-20.2792335465816,19.3235800073143,122.18076820435)) ;
#27850=CARTESIAN_POINT('Ctrl Pts',(-20.1052428067102,19.1435909269514,122.426981141854)) ;
#27851=CARTESIAN_POINT('Ctrl Pts',(-20.4802444747173,19.3335944416507,122.350655841088)) ;
#27852=CARTESIAN_POINT('Ctrl Pts',(-20.2660510795986,19.1536053612878,122.562891792175)) ;
#27853=CARTESIAN_POINT('Ctrl Pts',(-20.6485175407954,19.3436293862856,122.553674509814)) ;
#27854=CARTESIAN_POINT('Ctrl Pts',(-20.4006689258585,19.1636403059227,122.725307374417)) ;
#27855=CARTESIAN_POINT('Ctrl Pts',(-20.7769890298325,19.3534617363166,122.777893029322)) ;
#27856=CARTESIAN_POINT('Ctrl Pts',(-20.5034449148929,19.1734726559537,122.904681511226)) ;
#27857=CARTESIAN_POINT('Ctrl Pts',(-20.8667862746344,19.3635371754338,123.026918659849)) ;
#27858=CARTESIAN_POINT('Ctrl Pts',(-20.5752821883899,19.183548095071,123.103902590368)) ;
#27859=CARTESIAN_POINT('Ctrl Pts',(-20.9111458115105,19.3733896406684,123.282059452494)) ;
#27860=CARTESIAN_POINT('Ctrl Pts',(-20.6107689973514,19.1934005603056,123.308014298688)) ;
#27861=CARTESIAN_POINT('Ctrl Pts',(-20.9107290324318,19.3834625182453,123.546718673386)) ;
#27862=CARTESIAN_POINT('Ctrl Pts',(-20.6104349741825,19.2034734378824,123.519742024396)) ;
#27863=CARTESIAN_POINT('Ctrl Pts',(-20.8653781808651,19.3933051144378,123.801387925564)) ;
#27864=CARTESIAN_POINT('Ctrl Pts',(-20.5741538923526,19.2133160340749,123.723476203268)) ;
#27865=CARTESIAN_POINT('Ctrl Pts',(-20.7760923678515,19.4032854985531,124.047984519831)) ;
#27866=CARTESIAN_POINT('Ctrl Pts',(-20.5027249602154,19.2232964181902,123.920753112728)) ;
#27867=CARTESIAN_POINT('Ctrl Pts',(-20.6443997501556,19.4133039792019,124.275948701137)) ;
#27868=CARTESIAN_POINT('Ctrl Pts',(-20.3973704129932,19.233314898839,124.103124205952)) ;
#27869=CARTESIAN_POINT('Ctrl Pts',(-20.4778099653252,19.4231872942023,124.475248963833)) ;
#27870=CARTESIAN_POINT('Ctrl Pts',(-20.2640988584677,19.2431982138394,124.262563499982)) ;
#27871=CARTESIAN_POINT('Ctrl Pts',(-20.2754104277972,19.4332555912927,124.645589428262)) ;
#27872=CARTESIAN_POINT('Ctrl Pts',(-20.1021787138093,19.2532665109298,124.398835770553)) ;
#27873=CARTESIAN_POINT('Ctrl Pts',(-20.0520012191522,19.443085659665,124.775372441285)) ;
#27874=CARTESIAN_POINT('Ctrl Pts',(-19.9234522479264,19.2630965793021,124.502661276645)) ;
#27875=CARTESIAN_POINT('Ctrl Pts',(-19.8038135625138,19.4531524521334,124.86681341649)) ;
#27876=CARTESIAN_POINT('Ctrl Pts',(-19.7249017349538,19.2731633717705,124.575813934512)) ;
#27877=CARTESIAN_POINT('Ctrl Pts',(-19.5479941097252,19.4630417856219,124.912847154411)) ;
#27878=CARTESIAN_POINT('Ctrl Pts',(-19.5202469635521,19.2830527052591,124.612640501714)) ;
#27879=CARTESIAN_POINT('Ctrl Pts',(-19.2851987471319,19.473043917038,124.914186378401)) ;
#27880=CARTESIAN_POINT('Ctrl Pts',(-19.3100107840446,19.2930548366751,124.613711708274)) ;
#27881=CARTESIAN_POINT('Ctrl Pts',(-19.0280693627692,19.482967786659,124.870372052193)) ;
#27882=CARTESIAN_POINT('Ctrl Pts',(-19.1043078948215,19.3029787062961,124.578660218181)) ;
#27883=CARTESIAN_POINT('Ctrl Pts',(-18.7796000674895,19.4930113021762,124.781474531052)) ;
#27884=CARTESIAN_POINT('Ctrl Pts',(-18.9055323440351,19.3130222218133,124.507542000366)) ;
#27885=CARTESIAN_POINT('Ctrl Pts',(-18.5537969176444,19.5028935150645,124.653102676941)) ;
#27886=CARTESIAN_POINT('Ctrl Pts',(-18.7248906370469,19.3229044347016,124.404844891224)) ;
#27887=CARTESIAN_POINT('Ctrl Pts',(-18.3500292628219,19.5129615922839,124.484417808806)) ;
#27888=CARTESIAN_POINT('Ctrl Pts',(-18.5618763184921,19.332972511921,124.269896733581)) ;
#27889=CARTESIAN_POINT('Ctrl Pts',(-18.1823173295114,19.5228000970181,124.287590469283)) ;
#27890=CARTESIAN_POINT('Ctrl Pts',(-18.4277075526952,19.3428110166552,124.112435753387)) ;
#27891=CARTESIAN_POINT('Ctrl Pts',(-18.04805852035,19.5328628654475,124.059806889975)) ;
#27892=CARTESIAN_POINT('Ctrl Pts',(-18.3203002879426,19.3528737850846,123.930208672601)) ;
#27893=CARTESIAN_POINT('Ctrl Pts',(-17.9571650618813,19.5427598587302,123.816107138229)) ;
#27894=CARTESIAN_POINT('Ctrl Pts',(-18.247585798284,19.3627707783674,123.735249623978)) ;
#27895=CARTESIAN_POINT('Ctrl Pts',(-17.9089504191746,19.552691086365,123.559623490826)) ;
#27896=CARTESIAN_POINT('Ctrl Pts',(-18.2090139678198,19.3727020060021,123.530063314493)) ;
#27897=CARTESIAN_POINT('Ctrl Pts',(-17.9062584823097,19.5627332450072,123.295743025407)) ;
#27898=CARTESIAN_POINT('Ctrl Pts',(-18.2068602643135,19.3827441646443,123.318958777135)) ;
#27899=CARTESIAN_POINT('Ctrl Pts',(-17.9485751372052,19.5726199545382,123.039387974114)) ;
#27900=CARTESIAN_POINT('Ctrl Pts',(-18.240713249619,19.3926308741753,123.113875561071)) ;
#27901=CARTESIAN_POINT('Ctrl Pts',(-18.035260566707,19.5826129269668,122.791515506251)) ;
#27902=CARTESIAN_POINT('Ctrl Pts',(-18.3100612446795,19.4026238466039,122.915577638234)) ;
#27903=CARTESIAN_POINT('Ctrl Pts',(-18.1631676695922,19.5925591215034,122.563579250553)) ;
#27904=CARTESIAN_POINT('Ctrl Pts',(-18.4123864487675,19.4125700411405,122.733228908367)) ;
#27905=CARTESIAN_POINT('Ctrl Pts',(-18.3282687771438,19.6025044963549,122.360947075224)) ;
#27906=CARTESIAN_POINT('Ctrl Pts',(-18.5444667060827,19.422515415992,122.571123262125)) ;
#27907=CARTESIAN_POINT('Ctrl Pts',(-18.5284509193618,19.6125594157148,122.188521930226)) ;
#27908=CARTESIAN_POINT('Ctrl Pts',(-18.7046123935706,19.4325703353519,122.433182741857)) ;
#27909=CARTESIAN_POINT('Ctrl Pts',(-18.750061582201,19.6223809351583,122.056150769602)) ;
#27910=CARTESIAN_POINT('Ctrl Pts',(-18.8818995815922,19.4423918547954,122.327286088883)) ;
#27911=CARTESIAN_POINT('Ctrl Pts',(-18.9970975872,19.6324467039252,121.961712899097)) ;
#27912=CARTESIAN_POINT('Ctrl Pts',(-19.0795284847268,19.4524576235623,122.251735185212)) ;
#27913=CARTESIAN_POINT('Ctrl Pts',(-19.2526602063055,19.6423486255803,121.912488218236)) ;
#27914=CARTESIAN_POINT('Ctrl Pts',(-19.2839777620693,19.4623595452174,122.212355084193)) ;
#27915=CARTESIAN_POINT('Ctrl Pts',(-19.5165208729935,19.6523916844013,121.908094752818)) ;
#27916=CARTESIAN_POINT('Ctrl Pts',(-19.4950664570593,19.4724026040384,122.208839744185)) ;
#27917=CARTESIAN_POINT('Ctrl Pts',(-19.7735886685139,19.662297678444,121.949158051718)) ;
#27918=CARTESIAN_POINT('Ctrl Pts',(-19.7007200621191,19.4823085980811,122.241689749395)) ;
#27919=CARTESIAN_POINT('Ctrl Pts',(-20.0206528799151,19.6722354515258,122.033777229908)) ;
#27920=CARTESIAN_POINT('Ctrl Pts',(-19.8983711686072,19.4922463711629,122.30938424429)) ;
#27921=CARTESIAN_POINT('Ctrl Pts',(-20.2514911587077,19.6822758152581,122.161558568198)) ;
#27922=CARTESIAN_POINT('Ctrl Pts',(-20.0830422357934,19.5022867348952,122.411608819251)) ;
#27923=CARTESIAN_POINT('Ctrl Pts',(-20.4536472526372,19.6921631589816,122.324810150255)) ;
#27924=CARTESIAN_POINT('Ctrl Pts',(-20.2447669012231,19.5121740786187,122.542209021845)) ;
#27925=CARTESIAN_POINT('Ctrl Pts',(-20.6265036649569,19.7021553895503,122.522452222942)) ;
#27926=CARTESIAN_POINT('Ctrl Pts',(-20.3830525266567,19.5221663091874,122.700322030319)) ;
#27927=CARTESIAN_POINT('Ctrl Pts',(-20.7617787531808,19.7121039173339,122.746188030278)) ;
#27928=CARTESIAN_POINT('Ctrl Pts',(-20.4912730421252,19.532114836971,122.879309900702)) ;
#27929=CARTESIAN_POINT('Ctrl Pts',(-20.856369565108,19.7220407010572,122.989558473137)) ;
#27930=CARTESIAN_POINT('Ctrl Pts',(-20.5669463183877,19.5420516206943,123.074005464355)) ;
#27931=CARTESIAN_POINT('Ctrl Pts',(-20.9078402627332,19.7320237018542,123.246836830907)) ;
#27932=CARTESIAN_POINT('Ctrl Pts',(-20.6081237656465,19.5520346214913,123.279827763413)) ;
#27933=CARTESIAN_POINT('Ctrl Pts',(-20.9134056044351,19.7420675886949,123.510689929292)) ;
#27934=CARTESIAN_POINT('Ctrl Pts',(-20.6125768755946,19.562078508332,123.490910375999)) ;
#27935=CARTESIAN_POINT('Ctrl Pts',(-20.8745366916682,19.7518956122695,123.766060949729)) ;
#27936=CARTESIAN_POINT('Ctrl Pts',(-20.5814828864297,19.5719065319066,123.69520619847)) ;
#27937=CARTESIAN_POINT('Ctrl Pts',(-20.7899593277774,19.7619728604831,124.016948250578)) ;
#27938=CARTESIAN_POINT('Ctrl Pts',(-20.513821837292,19.5819837801202,123.895916689788)) ;
#27939=CARTESIAN_POINT('Ctrl Pts',(-20.6660660069028,19.7718224157884,124.244285226899)) ;
#27940=CARTESIAN_POINT('Ctrl Pts',(-20.4147085725534,19.5918333354255,124.077785895298)) ;
#27941=CARTESIAN_POINT('Ctrl Pts',(-20.5009161893016,19.7819051239861,124.451396677659)) ;
#27942=CARTESIAN_POINT('Ctrl Pts',(-20.2825893295826,19.6019160436232,124.243476002834)) ;
#27943=CARTESIAN_POINT('Ctrl Pts',(-20.307696830118,19.7917177169126,124.622248846254)) ;
#27944=CARTESIAN_POINT('Ctrl Pts',(-20.1280154809097,19.6117286365497,124.380157782015)) ;
#27945=CARTESIAN_POINT('Ctrl Pts',(-20.0823669714035,19.8017849091705,124.760755273323)) ;
#27946=CARTESIAN_POINT('Ctrl Pts',(-19.9477519880674,19.6217958288076,124.490964105197)) ;
#27947=CARTESIAN_POINT('Ctrl Pts',(-19.8403718039497,19.8116837386331,124.856362880226)) ;
#27948=CARTESIAN_POINT('Ctrl Pts',(-19.7541569135087,19.6316946582702,124.567451052078)) ;
#27949=CARTESIAN_POINT('Ctrl Pts',(-19.581599257843,19.8217377298233,124.90940442077)) ;
#27950=CARTESIAN_POINT('Ctrl Pts',(-19.5471389315843,19.6417486494604,124.609885512907)) ;
#27951=CARTESIAN_POINT('Ctrl Pts',(-19.3222318233483,19.8316094546065,124.916810422138)) ;
#27952=CARTESIAN_POINT('Ctrl Pts',(-19.339645850064,19.6516203742436,124.615811552476)) ;
#27953=CARTESIAN_POINT('Ctrl Pts',(-19.0604406240858,19.8416798967367,124.878387276188)) ;
#27954=CARTESIAN_POINT('Ctrl Pts',(-19.1302124239704,19.6616908163738,124.585074260848)) ;
#27955=CARTESIAN_POINT('Ctrl Pts',(-18.8151144576531,19.851512975167,124.797145106877)) ;
#27956=CARTESIAN_POINT('Ctrl Pts',(-18.9339520539141,19.6715238948041,124.52008208332)) ;
#27957=CARTESIAN_POINT('Ctrl Pts',(-18.5827297027157,19.8615434486684,124.672758530689)) ;
#27958=CARTESIAN_POINT('Ctrl Pts',(-18.7480434996773,19.6815543683055,124.420574076199)) ;
#27959=CARTESIAN_POINT('Ctrl Pts',(-18.3759053294246,19.8715750479671,124.509274829673)) ;
#27960=CARTESIAN_POINT('Ctrl Pts',(-18.5825831437698,19.6915859676042,124.289788093677)) ;
#27961=CARTESIAN_POINT('Ctrl Pts',(-18.2037555511074,19.8814047490052,124.31670801897)) ;
#27962=CARTESIAN_POINT('Ctrl Pts',(-18.4448629441187,19.7014156686424,124.135736342827)) ;
#27963=CARTESIAN_POINT('Ctrl Pts',(-18.0647658072952,19.8913941870617,124.094000670336)) ;
#27964=CARTESIAN_POINT('Ctrl Pts',(-18.3336698936195,19.7114051066988,123.957571414372)) ;
#27965=CARTESIAN_POINT('Ctrl Pts',(-17.9666480383149,19.9014380902778,123.848976044792)) ;
#27966=CARTESIAN_POINT('Ctrl Pts',(-18.2551743019667,19.7214490099149,123.761552138209)) ;
#27967=CARTESIAN_POINT('Ctrl Pts',(-17.9132339251412,19.9112596110913,123.596462120658)) ;
#27968=CARTESIAN_POINT('Ctrl Pts',(-18.212441709217,19.7312705307284,123.559542293389)) ;
#27969=CARTESIAN_POINT('Ctrl Pts',(-17.9036546813369,19.9212953353384,123.332913768264)) ;
#27970=CARTESIAN_POINT('Ctrl Pts',(-18.2047766510836,19.7413062549755,123.348703585753)) ;
#27971=CARTESIAN_POINT('Ctrl Pts',(-17.9406113337571,19.9313174892709,123.072128085455)) ;
#27972=CARTESIAN_POINT('Ctrl Pts',(-18.2343404591825,19.751328408908,123.140074813286)) ;
#27973=CARTESIAN_POINT('Ctrl Pts',(-18.0205697573143,19.9411797210282,122.825622198603)) ;
#27974=CARTESIAN_POINT('Ctrl Pts',(-18.2983054242486,19.7611906406653,122.942870341222)) ;
#27975=CARTESIAN_POINT('Ctrl Pts',(-18.1426708877126,19.9511387914861,122.594127929803)) ;
#27976=CARTESIAN_POINT('Ctrl Pts',(-18.3959846585781,19.7711497111232,122.757674351822)) ;
#27977=CARTESIAN_POINT('Ctrl Pts',(-18.3046496822276,19.9611739638623,122.386036391047)) ;
#27978=CARTESIAN_POINT('Ctrl Pts',(-18.525566417151,19.7811848834994,122.591200043048)) ;
#27979=CARTESIAN_POINT('Ctrl Pts',(-18.4970491714254,19.9710543490205,122.211642765681)) ;
#27980=CARTESIAN_POINT('Ctrl Pts',(-18.6794843828221,19.7910652686577,122.451684269361)) ;
#27981=CARTESIAN_POINT('Ctrl Pts',(-18.720627652709,19.9811110636145,122.070778322321)) ;
#27982=CARTESIAN_POINT('Ctrl Pts',(-18.8583463631659,19.8011219832516,122.338991147531)) ;
#27983=CARTESIAN_POINT('Ctrl Pts',(-18.960996130641,19.9909903321865,121.972639347132)) ;
#27984=CARTESIAN_POINT('Ctrl Pts',(-19.0506399085198,19.8110012518237,122.260478581221)) ;
#27985=CARTESIAN_POINT('Ctrl Pts',(-19.2174586026876,20.0009812896722,121.916419162101)) ;
#27986=CARTESIAN_POINT('Ctrl Pts',(-19.2558093721547,19.8209922093093,122.21550063503)) ;
#27987=CARTESIAN_POINT('Ctrl Pts',(-19.4811173295918,20.0110219483074,121.906111456795)) ;
#27988=CARTESIAN_POINT('Ctrl Pts',(-19.4667363549532,19.8310328679445,122.207252696804)) ;
#27989=CARTESIAN_POINT('Ctrl Pts',(-19.7372046092749,20.0208549280154,121.940573290861)) ;
#27990=CARTESIAN_POINT('Ctrl Pts',(-19.6716056688886,19.8408658476525,122.234820236614)) ;
#27991=CARTESIAN_POINT('Ctrl Pts',(-19.9876565139675,20.0308480612651,122.019537420732)) ;
#27992=CARTESIAN_POINT('Ctrl Pts',(-19.871967684399,19.8508589809022,122.297989646812)) ;
#27993=CARTESIAN_POINT('Ctrl Pts',(-20.2212609501245,20.0408801136485,122.141754795336)) ;
#27994=CARTESIAN_POINT('Ctrl Pts',(-20.0588521268464,19.8608910332856,122.395761901234)) ;
#27995=CARTESIAN_POINT('Ctrl Pts',(-20.4267990069944,20.0507453425998,122.29973257063)) ;
#27996=CARTESIAN_POINT('Ctrl Pts',(-20.2232832806594,19.8707562622369,122.522142243935)) ;
#27997=CARTESIAN_POINT('Ctrl Pts',(-20.6040593213488,20.060707283843,122.492388017739)) ;
#27998=CARTESIAN_POINT('Ctrl Pts',(-20.3650928817087,19.8807182034801,122.676265086268)) ;
#27999=CARTESIAN_POINT('Ctrl Pts',(-20.7458379853386,20.0707419988798,122.71471883926)) ;
#28000=CARTESIAN_POINT('Ctrl Pts',(-20.4785174821517,19.8907529185169,122.854128710767)) ;
#28001=CARTESIAN_POINT('Ctrl Pts',(-20.8457638320152,20.0806277692238,122.954554133205)) ;
#28002=CARTESIAN_POINT('Ctrl Pts',(-20.5584598470704,19.9006386888609,123.045995755698)) ;
#28003=CARTESIAN_POINT('Ctrl Pts',(-20.9035264743855,20.0906903666126,123.212570178599)) ;
#28004=CARTESIAN_POINT('Ctrl Pts',(-20.6046719531102,19.9107012862497,123.252408261689)) ;
#28005=CARTESIAN_POINT('Ctrl Pts',(-20.9154749497781,20.1005407784478,123.471173528851)) ;
#28006=CARTESIAN_POINT('Ctrl Pts',(-20.6142327359483,19.9205516980849,123.459290308044)) ;
#28007=CARTESIAN_POINT('Ctrl Pts',(-20.8824212203225,20.1105679477337,123.732588303383)) ;
#28008=CARTESIAN_POINT('Ctrl Pts',(-20.5877918409855,19.9305788673709,123.668422402238)) ;
#28009=CARTESIAN_POINT('Ctrl Pts',(-20.8038130480593,20.1205954284479,123.984115444725)) ;
#28010=CARTESIAN_POINT('Ctrl Pts',(-20.5249072402036,19.940606348085,123.86964471591)) ;
#28011=CARTESIAN_POINT('Ctrl Pts',(-20.6854052876472,20.1304384810272,124.214077225316)) ;
#28012=CARTESIAN_POINT('Ctrl Pts',(-20.4301831161523,19.9504494006643,124.053614646428)) ;
#28013=CARTESIAN_POINT('Ctrl Pts',(-20.5269966913248,20.1404323844658,124.423553915828)) ;
#28014=CARTESIAN_POINT('Ctrl Pts',(-20.3034580001774,19.9604433041029,124.221197233981)) ;
#28015=CARTESIAN_POINT('Ctrl Pts',(-20.3336481312429,20.1504595072422,124.602587618317)) ;
#28016=CARTESIAN_POINT('Ctrl Pts',(-20.1487805945953,19.9704704268793,124.364425725248)) ;
#28017=CARTESIAN_POINT('Ctrl Pts',(-20.1153421998912,20.1603502121343,124.743661057522)) ;
#28018=CARTESIAN_POINT('Ctrl Pts',(-19.9741372834993,19.9803611317714,124.477286090543)) ;
#28019=CARTESIAN_POINT('Ctrl Pts',(-19.873563628878,20.1703422389846,124.846066786522)) ;
#28020=CARTESIAN_POINT('Ctrl Pts',(-19.7807153501285,19.9903531586217,124.559212634884)) ;
#28021=CARTESIAN_POINT('Ctrl Pts',(-19.618831660715,20.1802882204731,124.904591118333)) ;
#28022=CARTESIAN_POINT('Ctrl Pts',(-19.5769304388928,20.0002991401102,124.60603416333)) ;
#28023=CARTESIAN_POINT('Ctrl Pts',(-19.3577875500338,20.190235393095,124.918525903528)) ;
#28024=CARTESIAN_POINT('Ctrl Pts',(-19.3680954272052,20.0102463127322,124.61718417711)) ;
#28025=CARTESIAN_POINT('Ctrl Pts',(-19.0957195762214,20.2002833344212,124.886313111744)) ;
#28026=CARTESIAN_POINT('Ctrl Pts',(-19.1584407747982,20.0202942540583,124.591416103589)) ;
#28027=CARTESIAN_POINT('Ctrl Pts',(-18.8481841830687,20.210130968229,124.810831448379)) ;
#28028=CARTESIAN_POINT('Ctrl Pts',(-18.9604121247911,20.0301418878661,124.531032963021)) ;
#28029=CARTESIAN_POINT('Ctrl Pts',(-18.6144848557031,20.220092682914,124.692895466025)) ;
#28030=CARTESIAN_POINT('Ctrl Pts',(-18.7734517428529,20.0401036025511,124.436686220242)) ;
#28031=CARTESIAN_POINT('Ctrl Pts',(-18.4035822760522,20.2301213157925,124.534835645106)) ;
#28032=CARTESIAN_POINT('Ctrl Pts',(-18.6047283766993,20.0501322354297,124.310240160807)) ;
#28033=CARTESIAN_POINT('Ctrl Pts',(-18.2254094105789,20.2400316413277,124.34490354003)) ;
#28034=CARTESIAN_POINT('Ctrl Pts',(-18.4621885771613,20.0600425609648,124.158296117052)) ;
#28035=CARTESIAN_POINT('Ctrl Pts',(-18.0819921054121,20.2499664717994,124.126739575367)) ;
#28036=CARTESIAN_POINT('Ctrl Pts',(-18.347452906344,20.0699773914365,123.983766287248)) ;
#28037=CARTESIAN_POINT('Ctrl Pts',(-17.9777343205273,20.2600078041814,123.884334153632)) ;
#28038=CARTESIAN_POINT('Ctrl Pts',(-18.2640446533727,20.0800187238185,123.789842799783)) ;
#28039=CARTESIAN_POINT('Ctrl Pts',(-17.9179543452334,20.2699006776202,123.631328380915)) ;
#28040=CARTESIAN_POINT('Ctrl Pts',(-18.2162184451713,20.0899115972573,123.587439083643)) ;
#28041=CARTESIAN_POINT('Ctrl Pts',(-17.9022315156781,20.2798698434381,123.369810686241)) ;
#28042=CARTESIAN_POINT('Ctrl Pts',(-18.2036382029103,20.0998807630752,123.37822414266)) ;
#28043=CARTESIAN_POINT('Ctrl Pts',(-17.9327660607719,20.2898985771546,123.108061591331)) ;
#28044=CARTESIAN_POINT('Ctrl Pts',(-18.2280625915591,20.1099094967917,123.168828314924)) ;
#28045=CARTESIAN_POINT('Ctrl Pts',(-18.0314212956118,20.3030910959258,122.775637805959)) ;
#28046=CARTESIAN_POINT('Ctrl Pts',(-18.3069888734284,20.1231020155629,122.902870362102)) ;
#28047=CARTESIAN_POINT('Ctrl Pts',(-18.2167817772954,20.3164509639684,122.472918789065)) ;
#28048=CARTESIAN_POINT('Ctrl Pts',(-18.455294322149,20.1364618836056,122.660681237817)) ;
#28049=CARTESIAN_POINT('Ctrl Pts',(-18.4689719567282,20.3296763011173,122.233665328807)) ;
#28050=CARTESIAN_POINT('Ctrl Pts',(-18.657015967816,20.1496872207544,122.469309185131)) ;
#28051=CARTESIAN_POINT('Ctrl Pts',(-18.6872891439649,20.3396575269579,122.0882957323)) ;
#28052=CARTESIAN_POINT('Ctrl Pts',(-18.8316741569079,20.1596684465951,122.353005054526)) ;
#28053=CARTESIAN_POINT('Ctrl Pts',(-18.9290457583576,20.3496930939408,121.982939786469)) ;
#28054=CARTESIAN_POINT('Ctrl Pts',(-19.0250769393784,20.1697040135779,122.268720036234)) ;
#28055=CARTESIAN_POINT('Ctrl Pts',(-19.1809279027677,20.3595561719029,121.921703115503)) ;
#28056=CARTESIAN_POINT('Ctrl Pts',(-19.2265826009953,20.17956709154,122.219728036107)) ;
#28057=CARTESIAN_POINT('Ctrl Pts',(-19.4449915418395,20.369626470704,121.904729894139)) ;
#28058=CARTESIAN_POINT('Ctrl Pts',(-19.4378331366122,20.1896373903411,122.206147360686)) ;
#28059=CARTESIAN_POINT('Ctrl Pts',(-19.7020745055463,20.3794687692718,121.933224576347)) ;
#28060=CARTESIAN_POINT('Ctrl Pts',(-19.6434999173445,20.1994796889089,122.228940862857)) ;
#28061=CARTESIAN_POINT('Ctrl Pts',(-19.9535442296739,20.3894294674416,122.005865433082)) ;
#28062=CARTESIAN_POINT('Ctrl Pts',(-19.844676334268,20.2094403870787,122.287051467107)) ;
#28063=CARTESIAN_POINT('Ctrl Pts',(-20.1901714045228,20.3994675016211,122.122429978516)) ;
#28064=CARTESIAN_POINT('Ctrl Pts',(-20.0339789452335,20.2194784212582,122.380301057783)) ;
#28065=CARTESIAN_POINT('Ctrl Pts',(-20.3998046709007,20.4093412384676,122.275390622965)) ;
#28066=CARTESIAN_POINT('Ctrl Pts',(-20.2016870029984,20.2293521581047,122.502667926402)) ;
#28067=CARTESIAN_POINT('Ctrl Pts',(-20.5832300951106,20.4194130223928,122.466148916955)) ;
#28068=CARTESIAN_POINT('Ctrl Pts',(-20.3484287872655,20.2394239420299,122.655272907251)) ;
#28069=CARTESIAN_POINT('Ctrl Pts',(-20.7274022481108,20.429245143594,122.680593266604)) ;
#28070=CARTESIAN_POINT('Ctrl Pts',(-20.4637684999712,20.2492560632311,122.826827448914)) ;
#28071=CARTESIAN_POINT('Ctrl Pts',(-20.83492227229,20.4392781676194,122.921317142792)) ;
#28072=CARTESIAN_POINT('Ctrl Pts',(-20.549786401994,20.2592890872566,123.019405611083)) ;
#28073=CARTESIAN_POINT('Ctrl Pts',(-20.8982551027824,20.4492940478161,123.176808341218)) ;
#28074=CARTESIAN_POINT('Ctrl Pts',(-20.6004547451558,20.2693049674532,123.223797857408)) ;
#28075=CARTESIAN_POINT('Ctrl Pts',(-20.9165069215087,20.4591775669103,123.435894221683)) ;
#28076=CARTESIAN_POINT('Ctrl Pts',(-20.615058364723,20.2791884865474,123.43106704069)) ;
#28077=CARTESIAN_POINT('Ctrl Pts',(-20.8895420040221,20.469167979274,123.697025786576)) ;
#28078=CARTESIAN_POINT('Ctrl Pts',(-20.5934884233315,20.2891788989111,123.639971206989)) ;
#28079=CARTESIAN_POINT('Ctrl Pts',(-20.7941934591565,20.4824311424774,124.032297261989)) ;
#28080=CARTESIAN_POINT('Ctrl Pts',(-20.5172126368922,20.3024420621145,123.908195802062)) ;
#28081=CARTESIAN_POINT('Ctrl Pts',(-20.61364497499,20.4957087127286,124.335469275498)) ;
#28082=CARTESIAN_POINT('Ctrl Pts',(-20.3727498733357,20.3157196323657,124.15076100523)) ;
#28083=CARTESIAN_POINT('Ctrl Pts',(-20.3624251620307,20.5090390152352,124.579659196355)) ;
#28084=CARTESIAN_POINT('Ctrl Pts',(-20.1718067039307,20.3290499348723,124.346077405116)) ;
#28085=CARTESIAN_POINT('Ctrl Pts',(-20.1474678125217,20.5189376970516,124.726143222167)) ;
#28086=CARTESIAN_POINT('Ctrl Pts',(-19.9998354017675,20.3389486166887,124.463273991554)) ;
#28087=CARTESIAN_POINT('Ctrl Pts',(-19.9082988338251,20.5289272120991,124.834343756603)) ;
#28088=CARTESIAN_POINT('Ctrl Pts',(-19.8085028501753,20.3489381317363,124.549834241605)) ;
#28089=CARTESIAN_POINT('Ctrl Pts',(-19.6550087594271,20.5388752638742,124.899096739163)) ;
#28090=CARTESIAN_POINT('Ctrl Pts',(-19.6058699022926,20.3588861835113,124.601638844772)) ;
#28091=CARTESIAN_POINT('Ctrl Pts',(-19.3945515389815,20.5488166671527,124.919199688652)) ;
#28092=CARTESIAN_POINT('Ctrl Pts',(-19.3975068666403,20.3688275867898,124.617723886778)) ;
#28093=CARTESIAN_POINT('Ctrl Pts',(-19.0469745337114,20.5621033319336,124.885630332357)) ;
#28094=CARTESIAN_POINT('Ctrl Pts',(-19.1194311731786,20.3821142515707,124.590866211464)) ;
#28095=CARTESIAN_POINT('Ctrl Pts',(-18.6334863377988,20.5787137535884,124.731039345078)) ;
#28096=CARTESIAN_POINT('Ctrl Pts',(-18.788654663985,20.3987246732255,124.467201404259)) ;
#28097=CARTESIAN_POINT('Ctrl Pts',(-18.2305106418667,20.5986250158392,124.387975748647)) ;
#28098=CARTESIAN_POINT('Ctrl Pts',(-18.4662665446094,20.4186359354763,124.192751186382)) ;
#28099=CARTESIAN_POINT('Ctrl Pts',(-17.9681790722083,20.6185691450041,123.927324296484)) ;
#28100=CARTESIAN_POINT('Ctrl Pts',(-18.2563995729899,20.4385800646412,123.824231859657)) ;
#28101=CARTESIAN_POINT('Ctrl Pts',(-17.8789643904274,20.6384923076093,123.405418987404)) ;
#28102=CARTESIAN_POINT('Ctrl Pts',(-18.1850241788991,20.4585032272464,123.406707562409)) ;
#28103=CARTESIAN_POINT('Ctrl Pts',(-17.9722011638597,20.6583824300158,122.884976490813)) ;
#28104=CARTESIAN_POINT('Ctrl Pts',(-18.2596109762183,20.4783933496529,122.990352318436)) ;
#28105=CARTESIAN_POINT('Ctrl Pts',(-18.2392413285999,20.6783873836159,122.425297035635)) ;
#28106=CARTESIAN_POINT('Ctrl Pts',(-18.4732405399828,20.498398303253,122.622607344408)) ;
#28107=CARTESIAN_POINT('Ctrl Pts',(-18.6435876221089,20.6982256406315,122.086739272797)) ;
#28108=CARTESIAN_POINT('Ctrl Pts',(-18.7967168578306,20.5182365602686,122.35175829032)) ;
#28109=CARTESIAN_POINT('Ctrl Pts',(-19.1427514572152,20.718219941418,121.904613931299)) ;
#28110=CARTESIAN_POINT('Ctrl Pts',(-19.1960471830647,20.5382308610552,122.206055793577)) ;
#28111=CARTESIAN_POINT('Ctrl Pts',(-19.6712810445263,20.7381051834625,121.904239572849)) ;
#28112=CARTESIAN_POINT('Ctrl Pts',(-19.6188718571092,20.5581161030996,122.205753939832)) ;
#28113=CARTESIAN_POINT('Ctrl Pts',(-20.168447470455,20.7579801299384,122.082748587511)) ;
#28114=CARTESIAN_POINT('Ctrl Pts',(-20.0166067329943,20.5779910495756,122.348559983418)) ;
#28115=CARTESIAN_POINT('Ctrl Pts',(-20.5778609764888,20.7780131998795,122.423240113376)) ;
#28116=CARTESIAN_POINT('Ctrl Pts',(-20.3441382911306,20.5980241195166,122.620951670167)) ;
#28117=CARTESIAN_POINT('Ctrl Pts',(-20.8439482662448,20.7979017067799,122.879935963145)) ;
#28118=CARTESIAN_POINT('Ctrl Pts',(-20.5570102575303,20.617912626417,122.986308438082)) ;
#28119=CARTESIAN_POINT('Ctrl Pts',(-20.9398845189848,20.8177565665612,123.398932664504)) ;
#28120=CARTESIAN_POINT('Ctrl Pts',(-20.6337603893495,20.6377674861983,123.401507281384)) ;
#28121=CARTESIAN_POINT('Ctrl Pts',(-20.8512719992327,20.8378074003489,123.924305207163)) ;
#28122=CARTESIAN_POINT('Ctrl Pts',(-20.5628715067338,20.657818319986,123.821804891128)) ;
#28123=CARTESIAN_POINT('Ctrl Pts',(-20.5928049104702,20.8575733422382,124.381835472892)) ;
#28124=CARTESIAN_POINT('Ctrl Pts',(-20.3560969395519,20.6775842618753,124.187831867116)) ;
#28125=CARTESIAN_POINT('Ctrl Pts',(-20.1896580437569,20.8775860736975,124.728578782344)) ;
#28126=CARTESIAN_POINT('Ctrl Pts',(-20.0335794046623,20.6975969933346,124.465226382195)) ;
#28127=CARTESIAN_POINT('Ctrl Pts',(-19.6948360554275,20.8974789086411,124.915243821142)) ;
#28128=CARTESIAN_POINT('Ctrl Pts',(-19.6377205723978,20.7174898282782,124.61455887421)) ;
#28129=CARTESIAN_POINT('Ctrl Pts',(-19.1659236264529,20.9173859319806,124.922728039924)) ;
#28130=CARTESIAN_POINT('Ctrl Pts',(-19.2145894369091,20.7373968516177,124.620545637084)) ;
#28131=CARTESIAN_POINT('Ctrl Pts',(-18.6655619227043,20.9373011968813,124.749682544139)) ;
#28132=CARTESIAN_POINT('Ctrl Pts',(-18.8142995780805,20.7573121165184,124.482107923995)) ;
#28133=CARTESIAN_POINT('Ctrl Pts',(-18.2524397020174,20.957332889041,124.413908184194)) ;
#28134=CARTESIAN_POINT('Ctrl Pts',(-18.4838026915331,20.7773438086781,124.21348792732)) ;
#28135=CARTESIAN_POINT('Ctrl Pts',(-17.9811972981208,20.977175935614,123.961546540794)) ;
#28136=CARTESIAN_POINT('Ctrl Pts',(-18.2668088563855,20.7971868552511,123.8515965203)) ;
#28137=CARTESIAN_POINT('Ctrl Pts',(-17.8790621516814,20.9970924835138,123.442223784006)) ;
#28138=CARTESIAN_POINT('Ctrl Pts',(-18.1851023793624,20.8171034031509,123.436137129649)) ;
#28139=CARTESIAN_POINT('Ctrl Pts',(-17.9604499278885,21.0170247265051,122.918699625149)) ;
#28140=CARTESIAN_POINT('Ctrl Pts',(-18.2502146020831,20.8370356461422,123.017317483767)) ;
#28141=CARTESIAN_POINT('Ctrl Pts',(-18.2149540834011,21.0369285613144,122.454965536719)) ;
#28142=CARTESIAN_POINT('Ctrl Pts',(-18.4538202863488,20.8569394809515,122.646330486718)) ;
#28143=CARTESIAN_POINT('Ctrl Pts',(-18.6119399166127,21.0568289615019,122.105461255144)) ;
#28144=CARTESIAN_POINT('Ctrl Pts',(-18.7714112568372,20.876839881139,122.366728442058)) ;
#28145=CARTESIAN_POINT('Ctrl Pts',(-19.1055245267092,21.0767786378812,121.91171422936)) ;
#28146=CARTESIAN_POINT('Ctrl Pts',(-19.1662802778635,20.8967895575183,122.211733244875)) ;
#28147=CARTESIAN_POINT('Ctrl Pts',(-19.6351319246211,21.0967111621016,121.898157078062)) ;
#28148=CARTESIAN_POINT('Ctrl Pts',(-19.5899667460685,20.9167220817387,122.200890351572)) ;
#28149=CARTESIAN_POINT('Ctrl Pts',(-20.1374331359232,21.1166311710878,122.065615887878)) ;
#28150=CARTESIAN_POINT('Ctrl Pts',(-19.9918072525265,20.9366420907249,122.334860475937)) ;
#28151=CARTESIAN_POINT('Ctrl Pts',(-20.5530840765956,21.136588077264,122.395047352195)) ;
#28152=CARTESIAN_POINT('Ctrl Pts',(-20.3243262285862,20.9565989969011,122.598408332127)) ;
#28153=CARTESIAN_POINT('Ctrl Pts',(-20.8308668599276,21.1564739167655,122.844813593085)) ;
#28154=CARTESIAN_POINT('Ctrl Pts',(-20.5465500430235,20.9764848364026,122.958223574526)) ;
#28155=CARTESIAN_POINT('Ctrl Pts',(-20.9388483133597,21.1764450889013,123.364394953387)) ;
#28156=CARTESIAN_POINT('Ctrl Pts',(-20.6329313716892,20.9964560085384,123.373889855656)) ;
#28157=CARTESIAN_POINT('Ctrl Pts',(-20.8643333248033,21.1962592858857,123.885809151916)) ;
#28158=CARTESIAN_POINT('Ctrl Pts',(-20.5733172829464,21.0162702055228,123.791020397466)) ;
#28159=CARTESIAN_POINT('Ctrl Pts',(-20.6149914724651,21.2162404718539,124.35458992427)) ;
#28160=CARTESIAN_POINT('Ctrl Pts',(-20.3738339226301,21.0362513914911,124.166047707023)) ;
#28161=CARTESIAN_POINT('Ctrl Pts',(-20.2875771231592,21.2328159772432,124.649450004713)) ;
#28162=CARTESIAN_POINT('Ctrl Pts',(-20.1119198605758,21.0528268968803,124.401919518092)) ;
#28163=CARTESIAN_POINT('Ctrl Pts',(-19.976190695121,21.2461254251068,124.808734121278)) ;
#28164=CARTESIAN_POINT('Ctrl Pts',(-19.8627850672793,21.0661363447439,124.529357922434)) ;
#28165=CARTESIAN_POINT('Ctrl Pts',(-19.6403422561752,21.2594931228834,124.911767929916)) ;
#28166=CARTESIAN_POINT('Ctrl Pts',(-19.5941577979202,21.0795040425205,124.611771756262)) ;
#28167=CARTESIAN_POINT('Ctrl Pts',(-19.2023540010426,21.2759836945493,124.927912591737)) ;
#28168=CARTESIAN_POINT('Ctrl Pts',(-19.2437108124987,21.0959946141864,124.62469560568)) ;
#28169=CARTESIAN_POINT('Ctrl Pts',(-18.6980130161789,21.2959039668821,124.76705541604)) ;
#28170=CARTESIAN_POINT('Ctrl Pts',(-18.8402511097492,21.1159148865192,124.495996295646)) ;
#28171=CARTESIAN_POINT('Ctrl Pts',(-18.3484015779916,21.3125210026031,124.497134075246)) ;
#28172=CARTESIAN_POINT('Ctrl Pts',(-18.5605800541927,21.1325319222402,124.280076149471)) ;
#28173=CARTESIAN_POINT('Ctrl Pts',(-18.1364098503999,21.3258118528842,124.219524949621)) ;
#28174=CARTESIAN_POINT('Ctrl Pts',(-18.3909714359101,21.1458227725213,124.057970053224)) ;
#28175=CARTESIAN_POINT('Ctrl Pts',(-18.0158871388316,21.3357808980387,123.986950081581)) ;
#28176=CARTESIAN_POINT('Ctrl Pts',(-18.2945586408566,21.1557918176758,123.871912706625)) ;
#28177=CARTESIAN_POINT('Ctrl Pts',(-17.9375848219816,21.3456842886722,123.7387264045)) ;
#28178=CARTESIAN_POINT('Ctrl Pts',(-18.2319181148261,21.1656952083094,123.673331434388)) ;
#28179=CARTESIAN_POINT('Ctrl Pts',(-17.9031917373362,21.355742074785,123.476694986446)) ;
#28180=CARTESIAN_POINT('Ctrl Pts',(-18.2044053250832,21.1757529944221,123.463708741263)) ;
#28181=CARTESIAN_POINT('Ctrl Pts',(-17.9143537185253,21.3655941114347,123.218009520766)) ;
#28182=CARTESIAN_POINT('Ctrl Pts',(-18.2133399425486,21.1856050310718,123.256751469431)) ;
#28183=CARTESIAN_POINT('Ctrl Pts',(-17.9896212280947,21.3789592355779,122.874956968011)) ;
#28184=CARTESIAN_POINT('Ctrl Pts',(-18.2735425071571,21.198970155215,122.982353715324)) ;
#28185=CARTESIAN_POINT('Ctrl Pts',(-18.1513956643206,21.3921852985409,122.562838107837)) ;
#28186=CARTESIAN_POINT('Ctrl Pts',(-18.4029674268594,21.2121962181781,122.732632497982)) ;
#28187=CARTESIAN_POINT('Ctrl Pts',(-18.3866109363659,21.4054889468232,122.304222180962)) ;
#28188=CARTESIAN_POINT('Ctrl Pts',(-18.5911529954546,21.2254998664603,122.525730915353)) ;
#28189=CARTESIAN_POINT('Ctrl Pts',(-18.5942688365872,21.4154804779862,122.143483381919)) ;
#28190=CARTESIAN_POINT('Ctrl Pts',(-18.7572784100833,21.2354913976233,122.397143875669)) ;
#28191=CARTESIAN_POINT('Ctrl Pts',(-18.8279161165822,21.4255199257855,122.020995347853)) ;
#28192=CARTESIAN_POINT('Ctrl Pts',(-18.9441978151252,21.2455308454226,122.299154881713)) ;
#28193=CARTESIAN_POINT('Ctrl Pts',(-19.0743002770801,21.4353637012994,121.942115783865)) ;
#28194=CARTESIAN_POINT('Ctrl Pts',(-19.1413056995706,21.2553746209365,122.236053522357)) ;
#28195=CARTESIAN_POINT('Ctrl Pts',(-19.3342026170286,21.445349342687,121.90619908811)) ;
#28196=CARTESIAN_POINT('Ctrl Pts',(-19.3492278602432,21.2653602623241,122.207322374569)) ;
#28197=CARTESIAN_POINT('Ctrl Pts',(-19.5951977714836,21.4552861270488,121.915768063468)) ;
#28198=CARTESIAN_POINT('Ctrl Pts',(-19.5580238317526,21.2752970466859,122.214979818382)) ;
#28199=CARTESIAN_POINT('Ctrl Pts',(-19.8533761099886,21.4653359615162,121.971250859302)) ;
#28200=CARTESIAN_POINT('Ctrl Pts',(-19.7645659845222,21.2853468811533,122.259368252402)) ;
#28201=CARTESIAN_POINT('Ctrl Pts',(-20.0932613278945,21.4751864110193,122.068581121297)) ;
#28202=CARTESIAN_POINT('Ctrl Pts',(-19.9564732213435,21.2951973306564,122.337234519556)) ;
#28203=CARTESIAN_POINT('Ctrl Pts',(-20.3156279272745,21.4851584250014,122.207174295959)) ;
#28204=CARTESIAN_POINT('Ctrl Pts',(-20.1343652320431,21.3051693446385,122.448110919028)) ;
#28205=CARTESIAN_POINT('Ctrl Pts',(-20.5110376061981,21.4951535828485,122.382755229701)) ;
#28206=CARTESIAN_POINT('Ctrl Pts',(-20.290691427895,21.3151645024856,122.588577292965)) ;
#28207=CARTESIAN_POINT('Ctrl Pts',(-20.6733301023097,21.5051875092122,122.590546133602)) ;
#28208=CARTESIAN_POINT('Ctrl Pts',(-20.4205236271332,21.3251984288494,122.754811381595)) ;
#28209=CARTESIAN_POINT('Ctrl Pts',(-20.7952585397872,21.5150432176446,122.819075138393)) ;
#28210=CARTESIAN_POINT('Ctrl Pts',(-20.5180643101211,21.3350541372817,122.937635474695)) ;
#28211=CARTESIAN_POINT('Ctrl Pts',(-20.8771547988309,21.5250413669833,123.068682710145)) ;
#28212=CARTESIAN_POINT('Ctrl Pts',(-20.5835791727783,21.3450522866204,123.13732215833)) ;
#28213=CARTESIAN_POINT('Ctrl Pts',(-20.9143410126104,21.5349407701568,123.326195883179)) ;
#28214=CARTESIAN_POINT('Ctrl Pts',(-20.6133259222408,21.354951689794,123.343332810001)) ;
#28215=CARTESIAN_POINT('Ctrl Pts',(-20.9061846999684,21.5449919670453,123.590176807784)) ;
#28216=CARTESIAN_POINT('Ctrl Pts',(-20.6067986577069,21.3650028866824,123.554517489311)) ;
#28217=CARTESIAN_POINT('Ctrl Pts',(-20.853249823519,21.5548742908582,123.844441837906)) ;
#28218=CARTESIAN_POINT('Ctrl Pts',(-20.5644486425954,21.3748852104953,123.7579288163)) ;
#28219=CARTESIAN_POINT('Ctrl Pts',(-20.7564330306425,21.5648691865148,124.088593766656)) ;
#28220=CARTESIAN_POINT('Ctrl Pts',(-20.4869932187418,21.3848801061519,123.953249478274)) ;
#28221=CARTESIAN_POINT('Ctrl Pts',(-20.6179931768872,21.5748902858973,124.312627761359)) ;
#28222=CARTESIAN_POINT('Ctrl Pts',(-20.3762394774589,21.3949012055344,124.132475496053)) ;
#28223=CARTESIAN_POINT('Ctrl Pts',(-20.4449112034606,21.5847975537594,124.507113190861)) ;
#28224=CARTESIAN_POINT('Ctrl Pts',(-20.2377724303908,21.4048084733965,124.288062198318)) ;
#28225=CARTESIAN_POINT('Ctrl Pts',(-20.2403849662515,21.5947358975846,124.669500522451)) ;
#28226=CARTESIAN_POINT('Ctrl Pts',(-20.0741502752422,21.4147468172218,124.417970248963)) ;
#28227=CARTESIAN_POINT('Ctrl Pts',(-20.0093045735368,21.6047393168851,124.79489097273)) ;
#28228=CARTESIAN_POINT('Ctrl Pts',(-19.8892850037941,21.4247502365222,124.518280706296)) ;
#28229=CARTESIAN_POINT('Ctrl Pts',(-19.7590892507398,21.6147738675922,124.878084487071)) ;
#28230=CARTESIAN_POINT('Ctrl Pts',(-19.6891120481609,21.4347847872293,124.584833462809)) ;
#28231=CARTESIAN_POINT('Ctrl Pts',(-19.5031930456652,21.6246188171978,124.916282417656)) ;
#28232=CARTESIAN_POINT('Ctrl Pts',(-19.4843952188806,21.4446297368349,124.615389634999)) ;
#28233=CARTESIAN_POINT('Ctrl Pts',(-19.2408957415365,21.6346046593107,124.909864611199)) ;
#28234=CARTESIAN_POINT('Ctrl Pts',(-19.274557555605,21.4546155789478,124.610253310096)) ;
#28235=CARTESIAN_POINT('Ctrl Pts',(-18.9848863453834,21.6445394666798,124.858431106566)) ;
#28236=CARTESIAN_POINT('Ctrl Pts',(-19.0697507008442,21.4645503863169,124.569104541095)) ;
#28237=CARTESIAN_POINT('Ctrl Pts',(-18.738859338082,21.6545970083931,124.761963952245)) ;
#28238=CARTESIAN_POINT('Ctrl Pts',(-18.8729297698642,21.4746079280302,124.491928838993)) ;
#28239=CARTESIAN_POINT('Ctrl Pts',(-18.5183469904694,21.6644186059052,124.627779140097)) ;
#28240=CARTESIAN_POINT('Ctrl Pts',(-18.696521489678,21.4844295255424,124.384579574157)) ;
#28241=CARTESIAN_POINT('Ctrl Pts',(-18.3195680415686,21.6744748653857,124.453674665829)) ;
#28242=CARTESIAN_POINT('Ctrl Pts',(-18.5374995695825,21.4944857850228,124.245294444731)) ;
#28243=CARTESIAN_POINT('Ctrl Pts',(-18.1562878546674,21.6844148016861,124.249767117428)) ;
#28244=CARTESIAN_POINT('Ctrl Pts',(-18.4068771805631,21.5044257213232,124.082167340354)) ;
#28245=CARTESIAN_POINT('Ctrl Pts',(-18.0306281552504,21.6943219224305,124.021754765608)) ;
#28246=CARTESIAN_POINT('Ctrl Pts',(-18.3063513226383,21.5143328420676,123.899756895081)) ;
#28247=CARTESIAN_POINT('Ctrl Pts',(-17.9454073048491,21.7043648283558,123.771982422679)) ;
#28248=CARTESIAN_POINT('Ctrl Pts',(-18.2381764644056,21.5243757479929,123.699938324042)) ;
#28249=CARTESIAN_POINT('Ctrl Pts',(-17.9053416812303,21.714272609455,123.51470692144)) ;
#28250=CARTESIAN_POINT('Ctrl Pts',(-18.2061259509787,21.5342835290921,123.494118036696)) ;
#28251=CARTESIAN_POINT('Ctrl Pts',(-17.9101476585179,21.7242829784574,123.251680239082)) ;
#28252=CARTESIAN_POINT('Ctrl Pts',(-18.2099726089032,21.5442938980945,123.283696771005)) ;
#28253=CARTESIAN_POINT('Ctrl Pts',(-17.9611784249865,21.7343138170262,122.993069233019)) ;
#28254=CARTESIAN_POINT('Ctrl Pts',(-18.25079914997,21.5543247366633,123.076808307396)) ;
#28255=CARTESIAN_POINT('Ctrl Pts',(-18.0542181019441,21.7441666566659,122.751434398998)) ;
#28256=CARTESIAN_POINT('Ctrl Pts',(-18.3252324147839,21.564177576303,122.883501741555)) ;
#28257=CARTESIAN_POINT('Ctrl Pts',(-18.1892070598107,21.7541546578309,122.526357242308)) ;
#28258=CARTESIAN_POINT('Ctrl Pts',(-18.433225062823,21.574165577468,122.703441075812)) ;
#28259=CARTESIAN_POINT('Ctrl Pts',(-18.3602212353183,21.76408347681,122.32928753721)) ;
#28260=CARTESIAN_POINT('Ctrl Pts',(-18.5700375178516,21.5840943964472,122.545786794347)) ;
#28261=CARTESIAN_POINT('Ctrl Pts',(-18.5637837492857,21.7740711795323,122.163582862095)) ;
#28262=CARTESIAN_POINT('Ctrl Pts',(-18.7328885150387,21.5940820991695,122.413224497597)) ;
#28263=CARTESIAN_POINT('Ctrl Pts',(-18.7943281092038,21.784107179335,122.035521757821)) ;
#28264=CARTESIAN_POINT('Ctrl Pts',(-18.9173249461088,21.6041180989721,122.310777167978)) ;
#28265=CARTESIAN_POINT('Ctrl Pts',(-19.038997751584,21.7939620491364,121.950573239043)) ;
#28266=CARTESIAN_POINT('Ctrl Pts',(-19.1130605360951,21.6139729687736,122.242820240775)) ;
#28267=CARTESIAN_POINT('Ctrl Pts',(-19.2983295791008,21.80396147956,121.908451210414)) ;
#28268=CARTESIAN_POINT('Ctrl Pts',(-19.3205261622003,21.6239723991971,122.209124297681)) ;
#28269=CARTESIAN_POINT('Ctrl Pts',(-19.5583862373949,21.8138565970253,121.911683181411)) ;
#28270=CARTESIAN_POINT('Ctrl Pts',(-19.5285708804354,21.6338675166624,122.21171149709)) ;
#28271=CARTESIAN_POINT('Ctrl Pts',(-19.8181211650492,21.8239170905422,121.96083913654)) ;
#28272=CARTESIAN_POINT('Ctrl Pts',(-19.7363587075279,21.6439280101794,122.251037906807)) ;
#28273=CARTESIAN_POINT('Ctrl Pts',(-20.0602885784198,21.8337665707434,122.052271697296)) ;
#28274=CARTESIAN_POINT('Ctrl Pts',(-19.930091288856,21.6537774903805,122.324185167146)) ;
#28275=CARTESIAN_POINT('Ctrl Pts',(-20.2872285089844,21.8437930210072,122.186139952124)) ;
#28276=CARTESIAN_POINT('Ctrl Pts',(-20.1116425053652,21.6638039406443,122.431281064082)) ;
#28277=CARTESIAN_POINT('Ctrl Pts',(-20.4871079315352,21.8538243114853,122.35801891506)) ;
#28278=CARTESIAN_POINT('Ctrl Pts',(-20.2715450314613,21.6738352311224,122.568785502684)) ;
#28279=CARTESIAN_POINT('Ctrl Pts',(-20.6513791646752,21.8636656991371,122.557772038563)) ;
#28280=CARTESIAN_POINT('Ctrl Pts',(-20.4029602709634,21.6836766187742,122.728588256116)) ;
#28281=CARTESIAN_POINT('Ctrl Pts',(-20.7809938111829,21.8736691000283,122.786445434062)) ;
#28282=CARTESIAN_POINT('Ctrl Pts',(-20.5066507156167,21.6936800196655,122.91152759353)) ;
#28283=CARTESIAN_POINT('Ctrl Pts',(-20.8686887483206,21.8836534828195,123.033784325657)) ;
#28284=CARTESIAN_POINT('Ctrl Pts',(-20.5768052604981,21.7036644024566,123.109399027828)) ;
#28285=CARTESIAN_POINT('Ctrl Pts',(-20.9120839655183,21.8936925728329,123.293981074003)) ;
#28286=CARTESIAN_POINT('Ctrl Pts',(-20.6115199849103,21.71370349247,123.317556776986)) ;
#28287=CARTESIAN_POINT('Ctrl Pts',(-20.9100499298834,21.9035383817421,123.552730180815)) ;
#28288=CARTESIAN_POINT('Ctrl Pts',(-20.609891351577,21.7235493013792,123.524555112863)) ;
#28289=CARTESIAN_POINT('Ctrl Pts',(-20.8629939222876,21.9135228045611,123.810817924676)) ;
#28290=CARTESIAN_POINT('Ctrl Pts',(-20.5722453017055,21.7335337241982,123.73102487777)) ;
#28291=CARTESIAN_POINT('Ctrl Pts',(-20.7723283116897,21.9234624298023,124.05581995963)) ;
#28292=CARTESIAN_POINT('Ctrl Pts',(-20.4997117680828,21.7434733494394,123.927025654345)) ;
#28293=CARTESIAN_POINT('Ctrl Pts',(-20.6391479210158,21.9335021193209,124.283546922036)) ;
#28294=CARTESIAN_POINT('Ctrl Pts',(-20.3931662819036,21.7535130389581,124.109206674248)) ;
#28295=CARTESIAN_POINT('Ctrl Pts',(-20.4711013650952,21.9433903077395,124.481766445994)) ;
#28296=CARTESIAN_POINT('Ctrl Pts',(-20.2587285516933,21.7634012273766,124.267780913417)) ;
#28297=CARTESIAN_POINT('Ctrl Pts',(-20.2694747065142,21.9533798337416,124.649861363959)) ;
#28298=CARTESIAN_POINT('Ctrl Pts',(-20.097426616492,21.7733907533787,124.402255850537)) ;
#28299=CARTESIAN_POINT('Ctrl Pts',(-20.0423296292845,21.9633383350968,124.779814856002)) ;
#28300=CARTESIAN_POINT('Ctrl Pts',(-19.915710259167,21.7833492547339,124.506217429302)) ;
#28301=CARTESIAN_POINT('Ctrl Pts',(-19.7977240449736,21.9732379291004,124.868443422786)) ;
#28302=CARTESIAN_POINT('Ctrl Pts',(-19.7200260940079,21.7932488487375,124.577119050715)) ;
#28303=CARTESIAN_POINT('Ctrl Pts',(-19.5376330731142,21.9832858172217,124.913825837491)) ;
#28304=CARTESIAN_POINT('Ctrl Pts',(-19.5119529591425,21.8032967368588,124.61342395089)) ;
#28305=CARTESIAN_POINT('Ctrl Pts',(-19.2775503015537,21.9931812424672,124.913569399124)) ;
#28306=CARTESIAN_POINT('Ctrl Pts',(-19.3038874739033,21.8131921621044,124.613217771097)) ;
#28307=CARTESIAN_POINT('Ctrl Pts',(-19.017233305932,22.0032426331678,124.86744619023)) ;
#28308=CARTESIAN_POINT('Ctrl Pts',(-19.0956337981961,21.8232535528049,124.576318149791)) ;
#28309=CARTESIAN_POINT('Ctrl Pts',(-18.7741467328486,22.0130882168545,124.778797095436)) ;
#28310=CARTESIAN_POINT('Ctrl Pts',(-18.9011658833268,21.8330991364916,124.505398287498)) ;
#28311=CARTESIAN_POINT('Ctrl Pts',(-18.5470623486079,22.0230511901637,124.648524437436)) ;
#28312=CARTESIAN_POINT('Ctrl Pts',(-18.7194990790042,21.8430621098008,124.401179638259)) ;
#28313=CARTESIAN_POINT('Ctrl Pts',(-18.3449798305692,22.0330768569895,124.479454619294)) ;
#28314=CARTESIAN_POINT('Ctrl Pts',(-18.5578335854537,21.8530877766266,124.265923060778)) ;
#28315=CARTESIAN_POINT('Ctrl Pts',(-18.1771126653133,22.0429913348558,124.28020996493)) ;
#28316=CARTESIAN_POINT('Ctrl Pts',(-18.4235409199083,21.8630022544929,124.106527278134)) ;
#28317=CARTESIAN_POINT('Ctrl Pts',(-18.0449474119808,22.0529798495308,124.053398711337)) ;
#28318=CARTESIAN_POINT('Ctrl Pts',(-18.317809439298,21.8729907691679,123.925078062203)) ;
#28319=CARTESIAN_POINT('Ctrl Pts',(-17.954211848732,22.0630239604462,123.805561752125)) ;
#28320=CARTESIAN_POINT('Ctrl Pts',(-18.2452217507632,21.8830348800833,123.726808050528)) ;
#28321=CARTESIAN_POINT('Ctrl Pts',(-17.9082542485454,22.0728520980408,123.551371969022)) ;
#28322=CARTESIAN_POINT('Ctrl Pts',(-18.2084565831269,21.8928630176779,123.523457276199)) ;
#28323=CARTESIAN_POINT('Ctrl Pts',(-17.9069805912369,22.0829286660997,123.286627562761)) ;
#28324=CARTESIAN_POINT('Ctrl Pts',(-18.2074383400266,21.9029395857368,123.311661381763)) ;
#28325=CARTESIAN_POINT('Ctrl Pts',(-17.9505873022016,22.0927808280039,123.031363437666)) ;
#28326=CARTESIAN_POINT('Ctrl Pts',(-18.2423241725982,21.912791747641,123.107451229462)) ;
#28327=CARTESIAN_POINT('Ctrl Pts',(-18.0395690380517,22.1028537899607,122.782109150564)) ;
#28328=CARTESIAN_POINT('Ctrl Pts',(-18.3135102432881,21.9228647095978,122.908047671536)) ;
#28329=CARTESIAN_POINT('Ctrl Pts',(-18.1675496052933,22.1126963519636,122.557311692099)) ;
#28330=CARTESIAN_POINT('Ctrl Pts',(-18.4158946651662,21.9327072716007,122.728210991207)) ;
#28331=CARTESIAN_POINT('Ctrl Pts',(-18.3342296705409,22.1226767884574,122.354827390352)) ;
#28332=CARTESIAN_POINT('Ctrl Pts',(-18.5492388606532,21.9426877080945,122.566223989023)) ;
#28333=CARTESIAN_POINT('Ctrl Pts',(-18.5346278830778,22.1326950937818,122.184094281001)) ;
#28334=CARTESIAN_POINT('Ctrl Pts',(-18.7095577721264,21.9527060134189,122.429637890191)) ;
#28335=CARTESIAN_POINT('Ctrl Pts',(-18.7583362356547,22.1425790577013,122.052058163512)) ;
#28336=CARTESIAN_POINT('Ctrl Pts',(-18.8885238944235,21.9625899773384,122.32400976912)) ;
#28337=CARTESIAN_POINT('Ctrl Pts',(-19.0060171333251,22.1526449344398,121.959277593487)) ;
#28338=CARTESIAN_POINT('Ctrl Pts',(-19.0866690470502,21.9726558540769,122.249785576266)) ;
#28339=CARTESIAN_POINT('Ctrl Pts',(-19.2602098520566,22.1624840353007,121.911823353389)) ;
#28340=CARTESIAN_POINT('Ctrl Pts',(-19.2900221324471,21.9824949549378,122.211822750592)) ;
#28341=CARTESIAN_POINT('Ctrl Pts',(-19.5238350449174,22.1725171181664,121.908510218283)) ;
#28342=CARTESIAN_POINT('Ctrl Pts',(-19.5009223790608,21.9925280378036,122.209172428358)) ;
#28343=CARTESIAN_POINT('Ctrl Pts',(-19.7836614016497,22.1825388034419,121.951624796669)) ;
#28344=CARTESIAN_POINT('Ctrl Pts',(-19.7087834435619,22.002549723079,122.243664446075)) ;
#28345=CARTESIAN_POINT('Ctrl Pts',(-20.0283161574298,22.1924054985404,122.037437936202)) ;
#28346=CARTESIAN_POINT('Ctrl Pts',(-19.9045062201637,22.0124164181775,122.312314862293)) ;
#28347=CARTESIAN_POINT('Ctrl Pts',(-20.2568547840646,22.2023653882749,122.165037255751)) ;
#28348=CARTESIAN_POINT('Ctrl Pts',(-20.0873367614171,22.0223763079121,122.414394197747)) ;
#28349=CARTESIAN_POINT('Ctrl Pts',(-20.4610185638516,22.2124003761004,122.331922477437)) ;
#28350=CARTESIAN_POINT('Ctrl Pts',(-20.2506677635409,22.0324112957375,122.547902586744)) ;
#28351=CARTESIAN_POINT('Ctrl Pts',(-20.6309241388541,22.2222870801747,122.528528183517)) ;
#28352=CARTESIAN_POINT('Ctrl Pts',(-20.3865915994159,22.0422979998118,122.705186531169)) ;
#28353=CARTESIAN_POINT('Ctrl Pts',(-20.766416856272,22.2323522244076,122.755640405164)) ;
#28354=CARTESIAN_POINT('Ctrl Pts',(-20.4949858643928,22.0523631440447,122.88687662059)) ;
#28355=CARTESIAN_POINT('Ctrl Pts',(-20.8585847061565,22.2421915151362,122.997265190441)) ;
#28356=CARTESIAN_POINT('Ctrl Pts',(-20.5687197080449,22.0622024347733,123.080175347708)) ;
#28357=CARTESIAN_POINT('Ctrl Pts',(-20.9088481489483,22.2522540725746,123.256845872699)) ;
#28358=CARTESIAN_POINT('Ctrl Pts',(-20.6089305940997,22.0722649922117,123.287840171023)) ;
#28359=CARTESIAN_POINT('Ctrl Pts',(-20.9129252441028,22.2621511238267,123.516913308371)) ;
#28360=CARTESIAN_POINT('Ctrl Pts',(-20.6121922611426,22.0821620434638,123.495893317472)) ;
#28361=CARTESIAN_POINT('Ctrl Pts',(-20.8725051637196,22.272082330575,123.774739999813)) ;
#28362=CARTESIAN_POINT('Ctrl Pts',(-20.5798565101102,22.0920932502121,123.702154136205)) ;
#28363=CARTESIAN_POINT('Ctrl Pts',(-20.786712131682,22.2821245147938,124.024299304319)) ;
#28364=CARTESIAN_POINT('Ctrl Pts',(-20.5112221742166,22.1021354344309,123.901801786887)) ;
#28365=CARTESIAN_POINT('Ctrl Pts',(-20.6610284500015,22.2920111429047,124.25170115506)) ;
#28366=CARTESIAN_POINT('Ctrl Pts',(-20.4106758246915,22.1120220625418,124.083722603376)) ;
#28367=CARTESIAN_POINT('Ctrl Pts',(-20.4963649928319,22.3020044154371,124.45625910245)) ;
#28368=CARTESIAN_POINT('Ctrl Pts',(-20.2789454023778,22.1220153350742,124.247369029717)) ;
#28369=CARTESIAN_POINT('Ctrl Pts',(-20.2995680280399,22.3119494909786,124.628229064092)) ;
#28370=CARTESIAN_POINT('Ctrl Pts',(-20.1215083814713,22.1319604106157,124.384944899341)) ;
#28371=CARTESIAN_POINT('Ctrl Pts',(-20.0760548364874,22.3218990417068,124.763918115327)) ;
#28372=CARTESIAN_POINT('Ctrl Pts',(-19.9426984210111,22.141909961344,124.493496265617)) ;
#28373=CARTESIAN_POINT('Ctrl Pts',(-19.8301102215282,22.3319383765548,124.859349625922)) ;
#28374=CARTESIAN_POINT('Ctrl Pts',(-19.7459427347351,22.1519492961919,124.569841851037)) ;
#28375=CARTESIAN_POINT('Ctrl Pts',(-19.5752934234394,22.3418245154987,124.910085821145)) ;
#28376=CARTESIAN_POINT('Ctrl Pts',(-19.5420902200881,22.1618354351359,124.610431044817)) ;
#28377=CARTESIAN_POINT('Ctrl Pts',(-19.3126560173104,22.3518226284724,124.916205138615)) ;
#28378=CARTESIAN_POINT('Ctrl Pts',(-19.3319804315117,22.1718335481096,124.615326989773)) ;
#28379=CARTESIAN_POINT('Ctrl Pts',(-19.0548963059002,22.3617423908249,124.877085616116)) ;
#28380=CARTESIAN_POINT('Ctrl Pts',(-19.1257731976824,22.181753310462,124.584031994196)) ;
#28381=CARTESIAN_POINT('Ctrl Pts',(-18.8048804750818,22.3717817864375,124.792892259255)) ;
#28382=CARTESIAN_POINT('Ctrl Pts',(-18.9257602220697,22.1917927060747,124.51667778619)) ;
#28383=CARTESIAN_POINT('Ctrl Pts',(-18.5763093840162,22.3816909722258,124.668127742339)) ;
#28384=CARTESIAN_POINT('Ctrl Pts',(-18.7429037235827,22.2017018918629,124.41686698238)) ;
#28385=CARTESIAN_POINT('Ctrl Pts',(-18.3718830460784,22.3916261563833,124.505717216813)) ;
#28386=CARTESIAN_POINT('Ctrl Pts',(-18.5793626191556,22.2116370760204,124.286939448208)) ;
#28387=CARTESIAN_POINT('Ctrl Pts',(-18.1971172156532,22.4016672137692,124.308030847448)) ;
#28388=CARTESIAN_POINT('Ctrl Pts',(-18.4395493697844,22.2216781334063,124.128790671233)) ;
#28389=CARTESIAN_POINT('Ctrl Pts',(-18.0612726927552,22.4115543718025,124.086530580778)) ;
#28390=CARTESIAN_POINT('Ctrl Pts',(-18.330873593402,22.2315652914396,123.951591529793)) ;
#28391=CARTESIAN_POINT('Ctrl Pts',(-17.9645436848904,22.4215466514784,123.842428732897)) ;
#28392=CARTESIAN_POINT('Ctrl Pts',(-18.2534897026088,22.2415575711155,123.756310497809)) ;
#28393=CARTESIAN_POINT('Ctrl Pts',(-17.9119640315032,22.4314951685235,123.586318714181)) ;
#28394=CARTESIAN_POINT('Ctrl Pts',(-18.211425301115,22.2515060881606,123.551423064664)) ;
#28395=CARTESIAN_POINT('Ctrl Pts',(-17.9042933598069,22.4414319460939,123.325324977717)) ;
#28396=CARTESIAN_POINT('Ctrl Pts',(-18.2052879085007,22.261442865731,123.342628610746)) ;
#28397=CARTESIAN_POINT('Ctrl Pts',(-17.9419119920911,22.4514149822408,123.065658904093)) ;
#28398=CARTESIAN_POINT('Ctrl Pts',(-18.235381847005,22.2714259018779,123.134895818999)) ;
#28399=CARTESIAN_POINT('Ctrl Pts',(-18.0249844510094,22.4614587338345,122.815165001349)) ;
#28400=CARTESIAN_POINT('Ctrl Pts',(-18.3018390701171,22.2814696534717,122.934500290776)) ;
#28401=CARTESIAN_POINT('Ctrl Pts',(-18.1471041894676,22.4712872630471,122.587531223368)) ;
#28402=CARTESIAN_POINT('Ctrl Pts',(-18.3995334548748,22.2912981826842,122.752393822393)) ;
#28403=CARTESIAN_POINT('Ctrl Pts',(-18.310736925562,22.4813626239558,122.379445782567)) ;
#28404=CARTESIAN_POINT('Ctrl Pts',(-18.5304390610458,22.3013735435929,122.585924577045)) ;
#28405=CARTESIAN_POINT('Ctrl Pts',(-18.5037504475988,22.491219222843,122.2066258693)) ;
#28406=CARTESIAN_POINT('Ctrl Pts',(-18.684848467763,22.3112301424801,122.447668526044)) ;
#28407=CARTESIAN_POINT('Ctrl Pts',(-18.7282113464719,22.5012822168609,122.066906399844)) ;
#28408=CARTESIAN_POINT('Ctrl Pts',(-18.8644168289928,22.321293136498,122.335891884029)) ;
#28409=CARTESIAN_POINT('Ctrl Pts',(-18.9691081441337,22.5111601511503,121.970077874885)) ;
#28410=CARTESIAN_POINT('Ctrl Pts',(-19.0571331080001,22.3311710707875,122.258428360996)) ;
#28411=CARTESIAN_POINT('Ctrl Pts',(-19.2261379991879,22.5211607987084,121.915505689096)) ;
#28412=CARTESIAN_POINT('Ctrl Pts',(-19.2627566457403,22.3411717183456,122.214769480072)) ;
#28413=CARTESIAN_POINT('Ctrl Pts',(-19.4866516087189,22.5310786451465,121.906267040837)) ;
#28414=CARTESIAN_POINT('Ctrl Pts',(-19.4711669227681,22.3510895647836,122.207377364757)) ;
#28415=CARTESIAN_POINT('Ctrl Pts',(-19.7481817747748,22.5411297621521,121.942948938101)) ;
#28416=CARTESIAN_POINT('Ctrl Pts',(-19.6803913883822,22.3611406817893,122.236721714525)) ;
#28417=CARTESIAN_POINT('Ctrl Pts',(-19.9950390178656,22.5510004974627,122.022770439589)) ;
#28418=CARTESIAN_POINT('Ctrl Pts',(-19.8778767883679,22.3710114170999,122.300577456873)) ;
#28419=CARTESIAN_POINT('Ctrl Pts',(-20.2288742155722,22.5610712047057,122.146611832965)) ;
#28420=CARTESIAN_POINT('Ctrl Pts',(-20.0649457944915,22.3810821243429,122.399649573841)) ;
#28421=CARTESIAN_POINT('Ctrl Pts',(-20.432852059648,22.5709042121576,122.305284591667)) ;
#28422=CARTESIAN_POINT('Ctrl Pts',(-20.2281280611383,22.3909151317947,122.526586124132)) ;
#28423=CARTESIAN_POINT('Ctrl Pts',(-20.6101957114275,22.5809347044599,122.50028265826)) ;
#28424=CARTESIAN_POINT('Ctrl Pts',(-20.3700041091279,22.400945624097,122.682583647088)) ;
#28425=CARTESIAN_POINT('Ctrl Pts',(-20.7503657377508,22.5909662995333,122.723566173364)) ;
#28426=CARTESIAN_POINT('Ctrl Pts',(-20.4821412655094,22.4109772191704,122.861209824262)) ;
#28427=CARTESIAN_POINT('Ctrl Pts',(-20.848126630718,22.6007959986715,122.962648437251)) ;
#28428=CARTESIAN_POINT('Ctrl Pts',(-20.5603509034017,22.4208069183087,123.052474161789)) ;
#28429=CARTESIAN_POINT('Ctrl Pts',(-20.904551077241,22.6107854485531,123.219033095629)) ;
#28430=CARTESIAN_POINT('Ctrl Pts',(-20.6054919617955,22.4307963681902,123.257581413107)) ;
#28431=CARTESIAN_POINT('Ctrl Pts',(-20.9149919746047,22.6208293063688,123.482765312887)) ;
#28432=CARTESIAN_POINT('Ctrl Pts',(-20.6138461187708,22.4408402260059,123.46856724786)) ;
#28433=CARTESIAN_POINT('Ctrl Pts',(-20.8807975538298,22.630650996959,123.738595413769)) ;
#28434=CARTESIAN_POINT('Ctrl Pts',(-20.5864922425363,22.4506619165961,123.673230544663)) ;
#28435=CARTESIAN_POINT('Ctrl Pts',(-20.8016166335874,22.6406860874994,123.990134218036)) ;
#28436=CARTESIAN_POINT('Ctrl Pts',(-20.5231490649285,22.4606970071365,123.874462168931)) ;
#28437=CARTESIAN_POINT('Ctrl Pts',(-20.6794595798729,22.6507106064821,124.223553358068)) ;
#28438=CARTESIAN_POINT('Ctrl Pts',(-20.4254247725794,22.4707215261192,124.061198201126)) ;
#28439=CARTESIAN_POINT('Ctrl Pts',(-20.5216428899484,22.6605704518923,124.429030130044)) ;
#28440=CARTESIAN_POINT('Ctrl Pts',(-20.2991731733227,22.4805813715294,124.22557998796)) ;
#28441=CARTESIAN_POINT('Ctrl Pts',(-20.3290800370369,22.670530228208,124.606303874563)) ;
#28442=CARTESIAN_POINT('Ctrl Pts',(-20.1451242645067,22.4905411478451,124.367400086112)) ;
#28443=CARTESIAN_POINT('Ctrl Pts',(-20.1069583810948,22.6805584255226,124.748107125882)) ;
#28444=CARTESIAN_POINT('Ctrl Pts',(-19.9674278116215,22.5005693451597,124.480844120942)) ;
#28445=CARTESIAN_POINT('Ctrl Pts',(-19.8666123895492,22.6904659678129,124.848267265594)) ;
#28446=CARTESIAN_POINT('Ctrl Pts',(-19.7751521487821,22.51047688745,124.5609736348)) ;
#28447=CARTESIAN_POINT('Ctrl Pts',(-19.6093776535577,22.7004986183768,124.905971284957)) ;
#28448=CARTESIAN_POINT('Ctrl Pts',(-19.569364702959,22.5205095380139,124.607138561972)) ;
#28449=CARTESIAN_POINT('Ctrl Pts',(-19.349909838197,22.7103825748034,124.918032249207)) ;
#28450=CARTESIAN_POINT('Ctrl Pts',(-19.3617911229907,22.5303934944406,124.616789062543)) ;
#28451=CARTESIAN_POINT('Ctrl Pts',(-19.0894539708058,22.7203722761653,124.88515179817)) ;
#28452=CARTESIAN_POINT('Ctrl Pts',(-19.1534263193822,22.5403831958024,124.590486565815)) ;
#28453=CARTESIAN_POINT('Ctrl Pts',(-18.8375462307077,22.7304132714413,124.806612946757)) ;
#28454=CARTESIAN_POINT('Ctrl Pts',(-18.9518995301889,22.5504241910784,124.527657156544)) ;
#28455=CARTESIAN_POINT('Ctrl Pts',(-18.6077694357356,22.7402461607097,124.68841772116)) ;
#28456=CARTESIAN_POINT('Ctrl Pts',(-18.7680779300007,22.5602570803468,124.4331029628)) ;
#28457=CARTESIAN_POINT('Ctrl Pts',(-18.3981964690907,22.7502393190771,124.530174726569)) ;
#28458=CARTESIAN_POINT('Ctrl Pts',(-18.6004184592641,22.5702502387142,124.306510187023)) ;
#28459=CARTESIAN_POINT('Ctrl Pts',(-18.2189780474116,22.7602713614292,124.336812835409)) ;
#28460=CARTESIAN_POINT('Ctrl Pts',(-18.457042329262,22.5802822810663,124.151821925346)) ;
#28461=CARTESIAN_POINT('Ctrl Pts',(-18.078177052041,22.7701366053876,124.11914781899)) ;
#28462=CARTESIAN_POINT('Ctrl Pts',(-18.3444002370286,22.5901475250248,123.97769144434)) ;
#28463=CARTESIAN_POINT('Ctrl Pts',(-17.9756297430813,22.7800984966336,123.878272519234)) ;
#28464=CARTESIAN_POINT('Ctrl Pts',(-18.262360610908,22.6001094162708,123.784992180742)) ;
#28465=CARTESIAN_POINT('Ctrl Pts',(-17.9164527324428,22.7901333966521,123.621304920688)) ;
#28466=CARTESIAN_POINT('Ctrl Pts',(-18.2150170837711,22.6101443162892,123.579418516256)) ;
#28467=CARTESIAN_POINT('Ctrl Pts',(-17.9025653496462,22.8000184770667,123.361873137659)) ;
#28468=CARTESIAN_POINT('Ctrl Pts',(-18.2039051888414,22.6200293967038,123.371873646667)) ;
#28469=CARTESIAN_POINT('Ctrl Pts',(-17.9345250196897,22.8100836491915,123.099344214703)) ;
#28470=CARTESIAN_POINT('Ctrl Pts',(-18.229470937305,22.6300945688287,123.161850152158)) ;
#28471=CARTESIAN_POINT('Ctrl Pts',(-18.0097882001565,22.819930883915,122.851728714304)) ;
#28472=CARTESIAN_POINT('Ctrl Pts',(-18.2896793803027,22.6399418035521,122.963757680924)) ;
#28473=CARTESIAN_POINT('Ctrl Pts',(-18.1285132437623,22.8299616952328,122.616400101498)) ;
#28474=CARTESIAN_POINT('Ctrl Pts',(-18.3846575488646,22.6499726148699,122.775493825297)) ;
#28475=CARTESIAN_POINT('Ctrl Pts',(-18.2864226563192,22.8399713111463,122.40599165732)) ;
#28476=CARTESIAN_POINT('Ctrl Pts',(-18.5109834183892,22.6599822307834,122.607165884196)) ;
#28477=CARTESIAN_POINT('Ctrl Pts',(-18.4763564295643,22.84988209055,122.227822802769)) ;
#28478=CARTESIAN_POINT('Ctrl Pts',(-18.6629287774965,22.6698930101871,122.464629519222)) ;
#28479=CARTESIAN_POINT('Ctrl Pts',(-18.6944202111758,22.859811356339,122.084505529354)) ;
#28480=CARTESIAN_POINT('Ctrl Pts',(-18.8373784211579,22.6798222759761,122.349974053439)) ;
#28481=CARTESIAN_POINT('Ctrl Pts',(-18.9368601501301,22.8698540496516,121.980263237278)) ;
#28482=CARTESIAN_POINT('Ctrl Pts',(-19.0313295614933,22.6898649692887,122.266578267691)) ;
#28483=CARTESIAN_POINT('Ctrl Pts',(-19.1897096706424,22.8797405823464,121.920470478153)) ;
#28484=CARTESIAN_POINT('Ctrl Pts',(-19.2336083570812,22.6997515019835,122.218742067114)) ;
#28485=CARTESIAN_POINT('Ctrl Pts',(-19.4518420605083,22.8897337274496,121.904884777647)) ;
#28486=CARTESIAN_POINT('Ctrl Pts',(-19.4433140578841,22.7097446470868,122.206271347572)) ;
#28487=CARTESIAN_POINT('Ctrl Pts',(-19.7114632832621,22.8996794081237,121.935008316747)) ;
#28488=CARTESIAN_POINT('Ctrl Pts',(-19.6510111009045,22.7196903277608,122.230368013377)) ;
#28489=CARTESIAN_POINT('Ctrl Pts',(-19.9621146837926,22.9096266657504,122.009255961602)) ;
#28490=CARTESIAN_POINT('Ctrl Pts',(-19.8515326922247,22.7296375853876,122.289763976907)) ;
#28491=CARTESIAN_POINT('Ctrl Pts',(-20.1982818352397,22.9196745678719,122.127332902665)) ;
#28492=CARTESIAN_POINT('Ctrl Pts',(-20.0404673939253,22.739685487509,122.38422358596)) ;
#28493=CARTESIAN_POINT('Ctrl Pts',(-20.4062715090379,22.9295222734936,122.281319880695)) ;
#28494=CARTESIAN_POINT('Ctrl Pts',(-20.2068601821527,22.7495331931307,122.507411217)) ;
#28495=CARTESIAN_POINT('Ctrl Pts',(-20.5870134936696,22.9394837401277,122.470672801482)) ;
#28496=CARTESIAN_POINT('Ctrl Pts',(-20.3514553209462,22.7594946597648,122.658891935936)) ;
#28497=CARTESIAN_POINT('Ctrl Pts',(-20.7328386955894,22.9495132933959,122.690234279952)) ;
#28498=CARTESIAN_POINT('Ctrl Pts',(-20.4681173105457,22.769524213033,122.834539862625)) ;
#28499=CARTESIAN_POINT('Ctrl Pts',(-20.8371700436695,22.9594201854233,122.928761227148)) ;
#28500=CARTESIAN_POINT('Ctrl Pts',(-20.5515843614637,22.7794311050604,123.025360373342)) ;
#28501=CARTESIAN_POINT('Ctrl Pts',(-20.8992391770811,22.9693678295363,123.182677656175)) ;
#28502=CARTESIAN_POINT('Ctrl Pts',(-20.6012418268376,22.7893787491735,123.228492885336)) ;
#28503=CARTESIAN_POINT('Ctrl Pts',(-20.9165341377211,22.9793678725652,123.444932969306)) ;
#28504=CARTESIAN_POINT('Ctrl Pts',(-20.6150800337761,22.7993787922023,123.438296931167)) ;
#28505=CARTESIAN_POINT('Ctrl Pts',(-20.8874593437994,22.9894066385592,123.707113721901)) ;
#28506=CARTESIAN_POINT('Ctrl Pts',(-20.5918224275554,22.8094175581963,123.648041733911)) ;
#28507=CARTESIAN_POINT('Ctrl Pts',(-20.8153966815368,22.9992317005814,123.955064177239)) ;
#28508=CARTESIAN_POINT('Ctrl Pts',(-20.5341744977842,22.8192426202186,123.846402585896)) ;
#28509=CARTESIAN_POINT('Ctrl Pts',(-20.6991206973961,23.0092862479078,124.192308936938)) ;
#28510=CARTESIAN_POINT('Ctrl Pts',(-20.4411557498176,22.8292971675449,124.036199358367)) ;
#28511=CARTESIAN_POINT('Ctrl Pts',(-20.5447615013441,23.019229491357,124.403151003466)) ;
#28512=CARTESIAN_POINT('Ctrl Pts',(-20.3176702602204,22.8392404109942,124.204874274932)) ;
#28513=CARTESIAN_POINT('Ctrl Pts',(-20.357481348229,23.0291316629649,124.583821375332)) ;
#28514=CARTESIAN_POINT('Ctrl Pts',(-20.1678477266094,22.849142582602,124.349412166951)) ;
#28515=CARTESIAN_POINT('Ctrl Pts',(-20.1383129462667,23.0391844985751,124.731298547748)) ;
#28516=CARTESIAN_POINT('Ctrl Pts',(-19.9925143364415,22.8591954182122,124.4673957384)) ;
#28517=CARTESIAN_POINT('Ctrl Pts',(-19.9012076725115,23.0490575562606,124.836667408501)) ;
#28518=CARTESIAN_POINT('Ctrl Pts',(-19.8028309876301,22.8690684758978,124.551692871464)) ;
#28519=CARTESIAN_POINT('Ctrl Pts',(-19.6464624451115,23.0590528177863,124.90066823185)) ;
#28520=CARTESIAN_POINT('Ctrl Pts',(-19.5990355883761,22.8790637374234,124.602895734181)) ;
#28521=CARTESIAN_POINT('Ctrl Pts',(-19.3836439744441,23.0690781872068,124.919051527796)) ;
#28522=CARTESIAN_POINT('Ctrl Pts',(-19.3887803013881,22.8890891068439,124.617604464544)) ;
#28523=CARTESIAN_POINT('Ctrl Pts',(-19.1251242692714,23.0789680197334,124.892233416081)) ;
#28524=CARTESIAN_POINT('Ctrl Pts',(-19.1819670497776,22.8989789393705,124.59615274981)) ;
#28525=CARTESIAN_POINT('Ctrl Pts',(-18.7890035337137,23.0922659905428,124.796782825436)) ;
#28526=CARTESIAN_POINT('Ctrl Pts',(-18.9130558291102,22.9122769101799,124.519792421691)) ;
#28527=CARTESIAN_POINT('Ctrl Pts',(-18.4874072190834,23.105464385652,124.617549791502)) ;
#28528=CARTESIAN_POINT('Ctrl Pts',(-18.6717586476981,22.9254753052891,124.376385659626)) ;
#28529=CARTESIAN_POINT('Ctrl Pts',(-18.2417519026231,23.1188598279314,124.365440342986)) ;
#28530=CARTESIAN_POINT('Ctrl Pts',(-18.4752682092803,22.9388707475686,124.1747301264)) ;
#28531=CARTESIAN_POINT('Ctrl Pts',(-18.0954516814504,23.1287356661704,124.151032241541)) ;
#28532=CARTESIAN_POINT('Ctrl Pts',(-18.3582189589316,22.9487465858075,124.003198627306)) ;
#28533=CARTESIAN_POINT('Ctrl Pts',(-17.9865146772214,23.1387970687681,123.910158781384)) ;
#28534=CARTESIAN_POINT('Ctrl Pts',(-18.2710692167074,22.9588079884053,123.810502898505)) ;
#28535=CARTESIAN_POINT('Ctrl Pts',(-17.922240462111,23.1486621257033,123.658970587668)) ;
#28536=CARTESIAN_POINT('Ctrl Pts',(-18.2196477108387,22.9686730453404,123.60955078964)) ;
#28537=CARTESIAN_POINT('Ctrl Pts',(-17.9018022904604,23.1586742216521,123.396691351192)) ;
#28538=CARTESIAN_POINT('Ctrl Pts',(-18.2032931318325,22.9786851412892,123.399733036954)) ;
#28539=CARTESIAN_POINT('Ctrl Pts',(-17.9355630207714,23.1719515307975,123.049376976604)) ;
#28540=CARTESIAN_POINT('Ctrl Pts',(-18.230309065925,22.9919624504346,123.121854826151)) ;
#28541=CARTESIAN_POINT('Ctrl Pts',(-18.0899419028751,23.1885505563048,122.636110521846)) ;
#28542=CARTESIAN_POINT('Ctrl Pts',(-18.3537865821073,23.0085614759419,122.791280237995)) ;
#28543=CARTESIAN_POINT('Ctrl Pts',(-18.3760258329839,23.2051496043378,122.300311520429)) ;
#28544=CARTESIAN_POINT('Ctrl Pts',(-18.5826974346445,23.025160523975,122.522589580736)) ;
#28545=CARTESIAN_POINT('Ctrl Pts',(-18.6623130734036,23.2183930163688,122.102367993719)) ;
#28546=CARTESIAN_POINT('Ctrl Pts',(-18.8116871062911,23.0384039360059,122.364269513183)) ;
#28547=CARTESIAN_POINT('Ctrl Pts',(-18.9019676656497,23.2284304440572,121.992209381467)) ;
#28548=CARTESIAN_POINT('Ctrl Pts',(-19.0034183798067,23.0484413636943,122.27613348672)) ;
#28549=CARTESIAN_POINT('Ctrl Pts',(-19.1537511180854,23.2383347460128,121.926257438649)) ;
#28550=CARTESIAN_POINT('Ctrl Pts',(-19.2048396762017,23.0583456656499,122.223371601155)) ;
#28551=CARTESIAN_POINT('Ctrl Pts',(-19.5011668383559,23.251601585988,121.896906683047)) ;
#28552=CARTESIAN_POINT('Ctrl Pts',(-19.4827890606653,23.0716125056251,122.199889201105)) ;
#28553=CARTESIAN_POINT('Ctrl Pts',(-19.9361152832958,23.2682277840779,121.974875772965)) ;
#28554=CARTESIAN_POINT('Ctrl Pts',(-19.8307319806188,23.088238703715,122.262263124349)) ;
#28555=CARTESIAN_POINT('Ctrl Pts',(-20.394142712814,23.2881468994613,122.240416456631)) ;
#28556=CARTESIAN_POINT('Ctrl Pts',(-20.1971528580598,23.1081578190985,122.474678337376)) ;
#28557=CARTESIAN_POINT('Ctrl Pts',(-20.6777956763041,23.3047533225956,122.578559316856)) ;
#28558=CARTESIAN_POINT('Ctrl Pts',(-20.4241051196912,23.1247642422327,122.745236815236)) ;
#28559=CARTESIAN_POINT('Ctrl Pts',(-20.8254141685684,23.3180495430913,122.895260367424)) ;
#28560=CARTESIAN_POINT('Ctrl Pts',(-20.5421769247472,23.1380604627284,122.998554989249)) ;
#28561=CARTESIAN_POINT('Ctrl Pts',(-20.9163840285696,23.3313183754327,123.231954203337)) ;
#28562=CARTESIAN_POINT('Ctrl Pts',(-20.614959974584,23.1513292950698,123.26792816828)) ;
#28563=CARTESIAN_POINT('Ctrl Pts',(-20.9167633041339,23.3480096234658,123.675476169135)) ;
#28564=CARTESIAN_POINT('Ctrl Pts',(-20.6152647077734,23.1680205431029,123.622731052057)) ;
#28565=CARTESIAN_POINT('Ctrl Pts',(-20.7380527826187,23.3678193551386,124.170798980292)) ;
#28566=CARTESIAN_POINT('Ctrl Pts',(-20.4722993945024,23.1878302747757,124.018996228655)) ;
#28567=CARTESIAN_POINT('Ctrl Pts',(-20.3990487800684,23.3877969624672,124.579436972735)) ;
#28568=CARTESIAN_POINT('Ctrl Pts',(-20.2010981192601,23.2078078821043,124.345907297091)) ;
#28569=CARTESIAN_POINT('Ctrl Pts',(-19.9416700356385,23.407723271525,124.846309372867)) ;
#28570=CARTESIAN_POINT('Ctrl Pts',(-19.8351962131263,23.2277341911621,124.559408404364)) ;
#28571=CARTESIAN_POINT('Ctrl Pts',(-19.423672280542,23.4275401316897,124.942420637845)) ;
#28572=CARTESIAN_POINT('Ctrl Pts',(-19.4207968852883,23.2475510513268,124.636299832249)) ;
#28573=CARTESIAN_POINT('Ctrl Pts',(-18.897005210854,23.4476399472837,124.853997620555)) ;
#28574=CARTESIAN_POINT('Ctrl Pts',(-18.9994637104009,23.2676508669208,124.565563970077)) ;
#28575=CARTESIAN_POINT('Ctrl Pts',(-18.4395858732156,23.4673969111663,124.595670036021)) ;
#28576=CARTESIAN_POINT('Ctrl Pts',(-18.6335252687433,23.2874078308034,124.358902707329)) ;
#28577=CARTESIAN_POINT('Ctrl Pts',(-18.0924014778527,23.4874338372357,124.192088863914)) ;
#28578=CARTESIAN_POINT('Ctrl Pts',(-18.3557767077419,23.3074447568728,124.036039090244)) ;
#28579=CARTESIAN_POINT('Ctrl Pts',(-17.9060208621862,23.5073034196172,123.697826439083)) ;
#28580=CARTESIAN_POINT('Ctrl Pts',(-18.206670079505,23.3273143392544,123.64062860021)) ;
#28581=CARTESIAN_POINT('Ctrl Pts',(-17.8981510516399,23.5272079913704,123.168957382108)) ;
#28582=CARTESIAN_POINT('Ctrl Pts',(-18.2003731028714,23.3472189110075,123.217532238313)) ;
#28583=CARTESIAN_POINT('Ctrl Pts',(-18.0717585757874,23.5471605935689,122.667777463739)) ;
#28584=CARTESIAN_POINT('Ctrl Pts',(-18.3392584148753,23.367171513206,122.816587536918)) ;
#28585=CARTESIAN_POINT('Ctrl Pts',(-18.4052588840874,23.5670700845392,122.257079257931)) ;
#28586=CARTESIAN_POINT('Ctrl Pts',(-18.6060587086755,23.3870810041763,122.488027567399)) ;
#28587=CARTESIAN_POINT('Ctrl Pts',(-18.8570010753677,23.5869214532386,121.984239388305)) ;
#28588=CARTESIAN_POINT('Ctrl Pts',(-18.9674541463767,23.4069323728757,122.269754763327)) ;
#28589=CARTESIAN_POINT('Ctrl Pts',(-19.3806182677798,23.6070016493746,121.881570519937)) ;
#28590=CARTESIAN_POINT('Ctrl Pts',(-19.3863468682687,23.4270125690117,122.187619790065)) ;
#28591=CARTESIAN_POINT('Ctrl Pts',(-19.9007519851589,23.62680259295,121.962636023239)) ;
#28592=CARTESIAN_POINT('Ctrl Pts',(-19.8024563004733,23.4468135125871,122.252472687978)) ;
#28593=CARTESIAN_POINT('Ctrl Pts',(-20.366645013507,23.6467865694595,122.217519363045)) ;
#28594=CARTESIAN_POINT('Ctrl Pts',(-20.1751704371761,23.4667974890966,122.456380235725)) ;
#28595=CARTESIAN_POINT('Ctrl Pts',(-20.7158350928187,23.6667025324351,122.615335633075)) ;
#28596=CARTESIAN_POINT('Ctrl Pts',(-20.4545226369622,23.4867134520722,122.774634459819)) ;
#28597=CARTESIAN_POINT('Ctrl Pts',(-20.909269753505,23.686572967257,123.106869748193)) ;
#28598=CARTESIAN_POINT('Ctrl Pts',(-20.6092694713509,23.5065838868942,123.167863591692)) ;
#28599=CARTESIAN_POINT('Ctrl Pts',(-20.922587690353,23.7066232524901,123.639453176953)) ;
#28600=CARTESIAN_POINT('Ctrl Pts',(-20.6199224768603,23.5266341721272,123.593929874628)) ;
#28601=CARTESIAN_POINT('Ctrl Pts',(-20.7562955195823,23.7263972212494,124.138232320058)) ;
#28602=CARTESIAN_POINT('Ctrl Pts',(-20.4868863698106,23.5464081408865,123.992954730668)) ;
#28603=CARTESIAN_POINT('Ctrl Pts',(-20.4256681461167,23.746453679369,124.556107455173)) ;
#28604=CARTESIAN_POINT('Ctrl Pts',(-20.2223831283312,23.5664645990061,124.327253151564)) ;
#28605=CARTESIAN_POINT('Ctrl Pts',(-19.9777988611578,23.76624856236,124.832456311627)) ;
#28606=CARTESIAN_POINT('Ctrl Pts',(-19.8640850333811,23.5862594819971,124.548331359068)) ;
#28607=CARTESIAN_POINT('Ctrl Pts',(-19.4586032621524,23.7862152176623,124.941723989977)) ;
#28608=CARTESIAN_POINT('Ctrl Pts',(-19.4487277454471,23.6062261372994,124.635742813942)) ;
#28609=CARTESIAN_POINT('Ctrl Pts',(-18.9333997951415,23.8061741877388,124.86638911577)) ;
#28610=CARTESIAN_POINT('Ctrl Pts',(-19.0285650781102,23.6261851073759,124.575472274884)) ;
#28611=CARTESIAN_POINT('Ctrl Pts',(-18.466838553606,23.8260702753289,124.617539311619)) ;
#28612=CARTESIAN_POINT('Ctrl Pts',(-18.6553167537536,23.6460811949661,124.376389529742)) ;
#28613=CARTESIAN_POINT('Ctrl Pts',(-18.1127087822637,23.8459684452405,124.224807490326)) ;
#28614=CARTESIAN_POINT('Ctrl Pts',(-18.3720148240515,23.6659793648776,124.062201436306)) ;
#28615=CARTESIAN_POINT('Ctrl Pts',(-17.9132245363324,23.8658742806076,123.734750368409)) ;
#28616=CARTESIAN_POINT('Ctrl Pts',(-18.2124303796564,23.6858852002447,123.670153955737)) ;
#28617=CARTESIAN_POINT('Ctrl Pts',(-17.8929172316979,23.8858242055455,123.204950398228)) ;
#28618=CARTESIAN_POINT('Ctrl Pts',(-18.1961880248625,23.7058351251827,123.246313584245)) ;
#28619=CARTESIAN_POINT('Ctrl Pts',(-18.0536055022471,23.9057033954559,122.701563671004)) ;
#28620=CARTESIAN_POINT('Ctrl Pts',(-18.3247423344152,23.725714315093,122.843604744158)) ;
#28621=CARTESIAN_POINT('Ctrl Pts',(-18.3778029519875,23.9256847197365,122.280987362701)) ;
#28622=CARTESIAN_POINT('Ctrl Pts',(-18.584103378577,23.7456956393736,122.507146042841)) ;
#28623=CARTESIAN_POINT('Ctrl Pts',(-18.8251843464588,23.9456145039448,121.997171158723)) ;
#28624=CARTESIAN_POINT('Ctrl Pts',(-18.9420106639801,23.765625423582,122.280096052287)) ;
#28625=CARTESIAN_POINT('Ctrl Pts',(-19.3420527237489,23.9655344933356,121.8830575886)) ;
#28626=CARTESIAN_POINT('Ctrl Pts',(-19.3555069146509,23.7855454129728,122.188809484294)) ;
#28627=CARTESIAN_POINT('Ctrl Pts',(-19.8655341729859,23.9853896886896,121.950798016933)) ;
#28628=CARTESIAN_POINT('Ctrl Pts',(-19.7742905208817,23.8054006083268,122.243004187493)) ;
#28629=CARTESIAN_POINT('Ctrl Pts',(-20.3385180584329,24.005435690349,122.195770834828)) ;
#28630=CARTESIAN_POINT('Ctrl Pts',(-20.1526809568724,23.8254466099861,122.438992919313)) ;
#28631=CARTESIAN_POINT('Ctrl Pts',(-20.6359495242104,24.0219354375588,122.518207743344)) ;
#28632=CARTESIAN_POINT('Ctrl Pts',(-20.3906069626951,23.8419463571959,122.696923825608)) ;
#28633=CARTESIAN_POINT('Ctrl Pts',(-20.7997715920691,24.0353240420069,122.829526935845)) ;
#28634=CARTESIAN_POINT('Ctrl Pts',(-20.5216768386143,23.855334961644,122.945999782161)) ;
#28635=CARTESIAN_POINT('Ctrl Pts',(-20.8788004514205,24.0451858703418,123.076353832387)) ;
#28636=CARTESIAN_POINT('Ctrl Pts',(-20.5848955788943,23.8651967899789,123.143455681254)) ;
#28637=CARTESIAN_POINT('Ctrl Pts',(-20.9149604443776,24.0551520130994,123.335751428972)) ;
#28638=CARTESIAN_POINT('Ctrl Pts',(-20.6138199293417,23.8751629327365,123.350985772304)) ;
#28639=CARTESIAN_POINT('Ctrl Pts',(-20.9016757192965,24.0685137592243,123.68657640661)) ;
#28640=CARTESIAN_POINT('Ctrl Pts',(-20.6032002770534,23.8885246788614,123.631591920217)) ;
#28641=CARTESIAN_POINT('Ctrl Pts',(-20.7738010339285,24.0849680881794,124.104947280262)) ;
#28642=CARTESIAN_POINT('Ctrl Pts',(-20.5008787101127,23.9049790078165,123.966355119094)) ;
#28643=CARTESIAN_POINT('Ctrl Pts',(-20.506074005893,24.1017353332277,124.460989068715)) ;
#28644=CARTESIAN_POINT('Ctrl Pts',(-20.2867199296873,23.9217462528648,124.251141688073)) ;
#28645=CARTESIAN_POINT('Ctrl Pts',(-20.2328267963323,24.1149218985017,124.674311881725)) ;
#28646=CARTESIAN_POINT('Ctrl Pts',(-20.0681001136612,23.9349328181389,124.421823903416)) ;
#28647=CARTESIAN_POINT('Ctrl Pts',(-20.0014355866622,24.1249113572463,124.798149275947)) ;
#28648=CARTESIAN_POINT('Ctrl Pts',(-19.8829901714832,23.9449222768835,124.520886542304)) ;
#28649=CARTESIAN_POINT('Ctrl Pts',(-19.7528479925732,24.1348651297274,124.879719694348)) ;
#28650=CARTESIAN_POINT('Ctrl Pts',(-19.6841183272593,23.9548760493646,124.586142147501)) ;
#28651=CARTESIAN_POINT('Ctrl Pts',(-19.4914820582763,24.1449129462601,124.917021763208)) ;
#28652=CARTESIAN_POINT('Ctrl Pts',(-19.4750256307248,23.9649238658972,124.615981190194)) ;
#28653=CARTESIAN_POINT('Ctrl Pts',(-19.2329600579686,24.1547544793826,124.90885452434)) ;
#28654=CARTESIAN_POINT('Ctrl Pts',(-19.268207989371,23.9747653990197,124.609445249634)) ;
#28655=CARTESIAN_POINT('Ctrl Pts',(-18.9760140363379,24.1647407216023,124.855708116863)) ;
#28656=CARTESIAN_POINT('Ctrl Pts',(-19.0626517155432,23.9847516412394,124.566925893019)) ;
#28657=CARTESIAN_POINT('Ctrl Pts',(-18.7332816198796,24.1746773450272,124.759326036302)) ;
#28658=CARTESIAN_POINT('Ctrl Pts',(-18.8684666629235,23.9946882646643,124.489818160608)) ;
#28659=CARTESIAN_POINT('Ctrl Pts',(-18.5085675410313,24.1847272224102,124.620623799681)) ;
#28660=CARTESIAN_POINT('Ctrl Pts',(-18.6886966289881,24.0047381420473,124.378854470344)) ;
#28661=CARTESIAN_POINT('Ctrl Pts',(-18.3151003354371,24.1945776611878,124.448610838)) ;
#28662=CARTESIAN_POINT('Ctrl Pts',(-18.5339244352023,24.0145885808249,124.241242476954)) ;
#28663=CARTESIAN_POINT('Ctrl Pts',(-18.1519526133633,24.2045496751565,124.243579488805)) ;
#28664=CARTESIAN_POINT('Ctrl Pts',(-18.4034080760509,24.0245605947936,124.077216069596)) ;
#28665=CARTESIAN_POINT('Ctrl Pts',(-18.0265886284109,24.2145448437826,124.012717326557)) ;
#28666=CARTESIAN_POINT('Ctrl Pts',(-18.303118890646,24.0345557634197,123.892525324631)) ;
#28667=CARTESIAN_POINT('Ctrl Pts',(-17.9432101173695,24.2245787270438,123.762588848226)) ;
#28668=CARTESIAN_POINT('Ctrl Pts',(-18.2364182327103,24.0445896466809,123.692421857217)) ;
#28669=CARTESIAN_POINT('Ctrl Pts',(-17.9048199953682,24.2344345971071,123.506429025599)) ;
#28670=CARTESIAN_POINT('Ctrl Pts',(-18.2057083811246,24.0544455167443,123.487493852008)) ;
#28671=CARTESIAN_POINT('Ctrl Pts',(-17.9111670277577,24.2444321430243,123.243809194865)) ;
#28672=CARTESIAN_POINT('Ctrl Pts',(-18.2107882352827,24.0644430626614,123.277398119021)) ;
#28673=CARTESIAN_POINT('Ctrl Pts',(-17.9624791058961,24.2543402699236,122.988529382377)) ;
#28674=CARTESIAN_POINT('Ctrl Pts',(-18.2518400388648,24.0743511895607,123.073174891986)) ;
#28675=CARTESIAN_POINT('Ctrl Pts',(-18.0578908532251,24.2643506414457,122.743365948088)) ;
#28676=CARTESIAN_POINT('Ctrl Pts',(-18.3281714650137,24.0843615610829,122.877044994232)) ;
#28677=CARTESIAN_POINT('Ctrl Pts',(-18.1951870356825,24.2743810841931,122.518367543358)) ;
#28678=CARTESIAN_POINT('Ctrl Pts',(-18.4380103114372,24.0943920038303,122.697047441839)) ;
#28679=CARTESIAN_POINT('Ctrl Pts',(-18.3658593160879,24.2842290367464,122.323803295538)) ;
#28680=CARTESIAN_POINT('Ctrl Pts',(-18.574549574067,24.1042399563836,122.541397733003)) ;
#28681=CARTESIAN_POINT('Ctrl Pts',(-18.5719589574334,24.2942917057674,122.158164871478)) ;
#28682=CARTESIAN_POINT('Ctrl Pts',(-18.7394306821448,24.1143026254045,122.408888674427)) ;
#28683=CARTESIAN_POINT('Ctrl Pts',(-18.7999455381362,24.3041860812313,122.033096218261)) ;
#28684=CARTESIAN_POINT('Ctrl Pts',(-18.9218207704429,24.1241970008685,122.308835803467)) ;
#28685=CARTESIAN_POINT('Ctrl Pts',(-19.0470862012802,24.3141278795495,121.948467825779)) ;
#28686=CARTESIAN_POINT('Ctrl Pts',(-19.1195337945076,24.1341387991866,122.24113518591)) ;
#28687=CARTESIAN_POINT('Ctrl Pts',(-19.306793360523,24.3241303732768,121.9076794678)) ;
#28688=CARTESIAN_POINT('Ctrl Pts',(-19.3272997862454,24.1441412929139,122.208506614045)) ;
#28689=CARTESIAN_POINT('Ctrl Pts',(-19.5704262020177,24.3341651717837,121.913035104117)) ;
#28690=CARTESIAN_POINT('Ctrl Pts',(-19.5382060289476,24.1541760914208,122.212793292696)) ;
#28691=CARTESIAN_POINT('Ctrl Pts',(-19.8243456090835,24.3440100557631,121.962698662003)) ;
#28692=CARTESIAN_POINT('Ctrl Pts',(-19.7413407004111,24.1640209754002,122.252526140925)) ;
#28693=CARTESIAN_POINT('Ctrl Pts',(-20.069363913774,24.3539959125811,122.056545067836)) ;
#28694=CARTESIAN_POINT('Ctrl Pts',(-19.937354478382,24.1740068322182,122.327605165077)) ;
#28695=CARTESIAN_POINT('Ctrl Pts',(-20.2933885436929,24.3639307267559,122.190706447143)) ;
#28696=CARTESIAN_POINT('Ctrl Pts',(-20.1165729005004,24.183941646393,122.434935898804)) ;
#28697=CARTESIAN_POINT('Ctrl Pts',(-20.4929322997301,24.3739882265412,122.363960667453)) ;
#28698=CARTESIAN_POINT('Ctrl Pts',(-20.2762066070936,24.1939991461783,122.573540913657)) ;
#28699=CARTESIAN_POINT('Ctrl Pts',(-20.6558088061112,24.3838099849595,122.564221525997)) ;
#28700=CARTESIAN_POINT('Ctrl Pts',(-20.4065058327547,24.2038209045966,122.733750399107)) ;
#28701=CARTESIAN_POINT('Ctrl Pts',(-20.7848399620391,24.3938656427435,122.794804496023)) ;
#28702=CARTESIAN_POINT('Ctrl Pts',(-20.5097290712294,24.2138765623806,122.918217820985)) ;
#28703=CARTESIAN_POINT('Ctrl Pts',(-20.8704564403244,24.4038078249235,123.041662828752)) ;
#28704=CARTESIAN_POINT('Ctrl Pts',(-20.5782202377542,24.2238187445607,123.11570490205)) ;
#28705=CARTESIAN_POINT('Ctrl Pts',(-20.9125354801232,24.4137130336182,123.298533938)) ;
#28706=CARTESIAN_POINT('Ctrl Pts',(-20.6118814893409,24.2337239532553,123.321201684156)) ;
#28707=CARTESIAN_POINT('Ctrl Pts',(-20.909246248355,24.4237548245807,123.562396507273)) ;
#28708=CARTESIAN_POINT('Ctrl Pts',(-20.6092481539301,24.2437657442178,123.532291786414)) ;
#28709=CARTESIAN_POINT('Ctrl Pts',(-20.8608714359243,24.4336625990529,123.818239689833)) ;
#28710=CARTESIAN_POINT('Ctrl Pts',(-20.5705464711203,24.25367351869,123.736965560673)) ;
#28711=CARTESIAN_POINT('Ctrl Pts',(-20.7683009426795,24.4436740992805,124.064515066611)) ;
#28712=CARTESIAN_POINT('Ctrl Pts',(-20.496488335269,24.2636850189176,123.933985158452)) ;
#28713=CARTESIAN_POINT('Ctrl Pts',(-20.6336219825576,24.4537068596732,124.291169915681)) ;
#28714=CARTESIAN_POINT('Ctrl Pts',(-20.388743464398,24.2737177793103,124.115308070656)) ;
#28715=CARTESIAN_POINT('Ctrl Pts',(-20.4650972755638,24.4635574288081,124.487670909562)) ;
#28716=CARTESIAN_POINT('Ctrl Pts',(-20.2539226994214,24.2835683484452,124.272507129792)) ;
#28717=CARTESIAN_POINT('Ctrl Pts',(-20.262546647733,24.473546038338,124.654592807145)) ;
#28718=CARTESIAN_POINT('Ctrl Pts',(-20.0918811554699,24.2935569579751,124.40604315333)) ;
#28719=CARTESIAN_POINT('Ctrl Pts',(-20.035434390892,24.4834746943621,124.783046651201)) ;
#28720=CARTESIAN_POINT('Ctrl Pts',(-19.910190795979,24.3034856139992,124.508804458404)) ;
#28721=CARTESIAN_POINT('Ctrl Pts',(-19.788147480938,24.4934624405399,124.871054527459)) ;
#28722=CARTESIAN_POINT('Ctrl Pts',(-19.7123608220074,24.313473360177,124.579209069275)) ;
#28723=CARTESIAN_POINT('Ctrl Pts',(-19.5280364525962,24.5034984294756,124.914557400059)) ;
#28724=CARTESIAN_POINT('Ctrl Pts',(-19.5042716307132,24.3235093491128,124.614009587492)) ;
#28725=CARTESIAN_POINT('Ctrl Pts',(-19.2690459880752,24.5133532992892,124.912706949231)) ;
#28726=CARTESIAN_POINT('Ctrl Pts',(-19.2970800077781,24.3333642189264,124.612527489391)) ;
#28727=CARTESIAN_POINT('Ctrl Pts',(-19.0105743992336,24.523352740531,124.865592193593)) ;
#28728=CARTESIAN_POINT('Ctrl Pts',(-19.0903031443664,24.3433636601681,124.574834047047)) ;
#28729=CARTESIAN_POINT('Ctrl Pts',(-18.7666019329129,24.5332478147111,124.775498416424)) ;
#28730=CARTESIAN_POINT('Ctrl Pts',(-18.8951262877469,24.3532587343482,124.502757699957)) ;
#28731=CARTESIAN_POINT('Ctrl Pts',(-18.5383021509909,24.5433084705508,124.642232833805)) ;
#28732=CARTESIAN_POINT('Ctrl Pts',(-18.7124871214675,24.3633193901879,124.39614372167)) ;
#28733=CARTESIAN_POINT('Ctrl Pts',(-18.3407179161461,24.5531573447464,124.475027408876)) ;
#28734=CARTESIAN_POINT('Ctrl Pts',(-18.5544214106381,24.3731682643835,124.262378691614)) ;
#28735=CARTESIAN_POINT('Ctrl Pts',(-18.1716495641239,24.5631860567097,124.272865839476)) ;
#28736=CARTESIAN_POINT('Ctrl Pts',(-18.4191678481287,24.3831969763468,124.100648461118)) ;
#28737=CARTESIAN_POINT('Ctrl Pts',(-18.0408595712216,24.5732154572928,124.044039432676)) ;
#28738=CARTESIAN_POINT('Ctrl Pts',(-18.3145372315862,24.3932263769299,123.917586479356)) ;
#28739=CARTESIAN_POINT('Ctrl Pts',(-17.9529267054046,24.5830556509096,123.80085466428)) ;
#28740=CARTESIAN_POINT('Ctrl Pts',(-18.2441926703123,24.4030665705467,123.723039009644)) ;
#28741=CARTESIAN_POINT('Ctrl Pts',(-17.9073440510645,24.5930590734848,123.541984051105)) ;
#28742=CARTESIAN_POINT('Ctrl Pts',(-18.2077279538104,24.4130699931219,123.515942359835)) ;
#28743=CARTESIAN_POINT('Ctrl Pts',(-17.9074876720707,24.6030446105779,123.279530447817)) ;
#28744=CARTESIAN_POINT('Ctrl Pts',(-18.2078442820345,24.423055530215,123.305979644887)) ;
#28745=CARTESIAN_POINT('Ctrl Pts',(-17.953701474388,24.6130856150647,123.019767558698)) ;
#28746=CARTESIAN_POINT('Ctrl Pts',(-18.2448168072216,24.4330965347018,123.098169488521)) ;
#28747=CARTESIAN_POINT('Ctrl Pts',(-18.0422190940517,24.6229291540059,122.776684574555)) ;
#28748=CARTESIAN_POINT('Ctrl Pts',(-18.3156319085525,24.442940073643,122.903704466201)) ;
#28749=CARTESIAN_POINT('Ctrl Pts',(-18.1729536422505,24.6329141849967,122.549220386111)) ;
#28750=CARTESIAN_POINT('Ctrl Pts',(-18.42022057525,24.4529251046338,122.72173393716)) ;
#28751=CARTESIAN_POINT('Ctrl Pts',(-18.3403982888488,24.6428536475187,122.348704583029)) ;
#28752=CARTESIAN_POINT('Ctrl Pts',(-18.5541769923721,24.4628645671558,122.56132244681)) ;
#28753=CARTESIAN_POINT('Ctrl Pts',(-18.5421236161833,24.6528933797425,122.178692975382)) ;
#28754=CARTESIAN_POINT('Ctrl Pts',(-18.7155581760706,24.4729042993796,122.425314071837)) ;
#28755=CARTESIAN_POINT('Ctrl Pts',(-18.766826532383,24.6627815600597,122.048158969798)) ;
#28756=CARTESIAN_POINT('Ctrl Pts',(-18.8953205045771,24.4827924796968,122.320888330278)) ;
#28757=CARTESIAN_POINT('Ctrl Pts',(-19.0130885634454,24.6727710757622,121.957251380598)) ;
#28758=CARTESIAN_POINT('Ctrl Pts',(-19.0923303688238,24.4927819953993,122.248163402219)) ;
#28759=CARTESIAN_POINT('Ctrl Pts',(-19.2706307855915,24.6827296264169,121.910828202634)) ;
#28760=CARTESIAN_POINT('Ctrl Pts',(-19.2983640185096,24.502740546054,122.211026103761)) ;
#28761=CARTESIAN_POINT('Ctrl Pts',(-19.5307897392351,24.6926290335219,121.909185754216)) ;
#28762=CARTESIAN_POINT('Ctrl Pts',(-19.5064904836855,24.5126399531591,122.209713204043)) ;
#28763=CARTESIAN_POINT('Ctrl Pts',(-19.7910790035536,24.7026776199382,121.953496342207)) ;
#28764=CARTESIAN_POINT('Ctrl Pts',(-19.7147218884372,24.5226885395753,122.245162768907)) ;
#28765=CARTESIAN_POINT('Ctrl Pts',(-20.0360311856884,24.7125704389027,122.040742561825)) ;
#28766=CARTESIAN_POINT('Ctrl Pts',(-19.9106825930213,24.5325813585398,122.31496045899)) ;
#28767=CARTESIAN_POINT('Ctrl Pts',(-20.2660472328048,24.7226415564325,122.171540812148)) ;
#28768=CARTESIAN_POINT('Ctrl Pts',(-20.0946951781208,24.5426524760696,122.419600117649)) ;
#28769=CARTESIAN_POINT('Ctrl Pts',(-20.4649896868534,24.7324572503985,122.33580820644)) ;
#28770=CARTESIAN_POINT('Ctrl Pts',(-20.2538475822672,24.5524681700357,122.55101399222)) ;
#28771=CARTESIAN_POINT('Ctrl Pts',(-20.6368834830163,24.7425236278958,122.536807653796)) ;
#28772=CARTESIAN_POINT('Ctrl Pts',(-20.3913621437234,24.562534547533,122.711814344018)) ;
#28773=CARTESIAN_POINT('Ctrl Pts',(-20.7690258159267,24.7524226139777,122.760956322212)) ;
#28774=CARTESIAN_POINT('Ctrl Pts',(-20.4970748780025,24.5724335336148,122.891133115402)) ;
#28775=CARTESIAN_POINT('Ctrl Pts',(-20.8617232642626,24.7624767939712,123.008312860307)) ;
#28776=CARTESIAN_POINT('Ctrl Pts',(-20.5712320948138,24.5824877136083,123.089018856006)) ;
#28777=CARTESIAN_POINT('Ctrl Pts',(-20.9094544648808,24.7723476069039,123.263341038962)) ;
#28778=CARTESIAN_POINT('Ctrl Pts',(-20.6094160886339,24.592358526541,123.293040642391)) ;
#28779=CARTESIAN_POINT('Ctrl Pts',(-20.9122265609454,24.7824215077577,123.527995577717)) ;
#28780=CARTESIAN_POINT('Ctrl Pts',(-20.6116329563875,24.6024324273948,123.504764628738)) ;
#28781=CARTESIAN_POINT('Ctrl Pts',(-20.8703860648763,24.7922416631444,123.782706579754)) ;
#28782=CARTESIAN_POINT('Ctrl Pts',(-20.5781600363798,24.6122525827815,123.708532082081)) ;
#28783=CARTESIAN_POINT('Ctrl Pts',(-20.7829843523247,24.8023203700966,124.032658419494)) ;
#28784=CARTESIAN_POINT('Ctrl Pts',(-20.5082379034631,24.6223312897337,123.90849368722)) ;
#28785=CARTESIAN_POINT('Ctrl Pts',(-20.6564437174401,24.8121719586354,124.258586397133)) ;
#28786=CARTESIAN_POINT('Ctrl Pts',(-20.4070053415969,24.6321828782725,124.08923482883)) ;
#28787=CARTESIAN_POINT('Ctrl Pts',(-20.4891628443996,24.8222450751604,124.463680852311)) ;
#28788=CARTESIAN_POINT('Ctrl Pts',(-20.2731799578671,24.6422559947975,124.253310286516)) ;
#28789=CARTESIAN_POINT('Ctrl Pts',(-20.2933179390205,24.8320875922562,124.632670356776)) ;
#28790=CARTESIAN_POINT('Ctrl Pts',(-20.116504494174,24.6520985118933,124.388500688278)) ;
#28791=CARTESIAN_POINT('Ctrl Pts',(-20.0684748873038,24.8420680538102,124.767681031673)) ;
#28792=CARTESIAN_POINT('Ctrl Pts',(-19.9366300648084,24.6620789734473,124.496508766413)) ;
#28793=CARTESIAN_POINT('Ctrl Pts',(-19.8224883546883,24.8520863038009,124.861485946865)) ;
#28794=CARTESIAN_POINT('Ctrl Pts',(-19.7398406470911,24.6720972234381,124.571552218075)) ;
#28795=CARTESIAN_POINT('Ctrl Pts',(-19.5674837085229,24.8619704639947,124.911020996683)) ;
#28796=CARTESIAN_POINT('Ctrl Pts',(-19.535837716226,24.6819813836318,124.611179716792)) ;
#28797=CARTESIAN_POINT('Ctrl Pts',(-19.3030511330044,24.8720356109697,124.915550386411)) ;
#28798=CARTESIAN_POINT('Ctrl Pts',(-19.3242913349557,24.6920465306068,124.614802835819)) ;
#28799=CARTESIAN_POINT('Ctrl Pts',(-19.0475737608601,24.8818774346105,124.875152002711)) ;
#28800=CARTESIAN_POINT('Ctrl Pts',(-19.1199106517723,24.7018883542476,124.582483957355)) ;
#28801=CARTESIAN_POINT('Ctrl Pts',(-18.7981220481967,24.8919069070713,124.790082006543)) ;
#28802=CARTESIAN_POINT('Ctrl Pts',(-18.9203492635413,24.7119178267085,124.514427763563)) ;
#28803=CARTESIAN_POINT('Ctrl Pts',(-18.5676370265376,24.9019337623334,124.662373648599)) ;
#28804=CARTESIAN_POINT('Ctrl Pts',(-18.7359613597194,24.7219446819705,124.41226071562)) ;
#28805=CARTESIAN_POINT('Ctrl Pts',(-18.3661893963596,24.9117770124439,124.500103756191)) ;
#28806=CARTESIAN_POINT('Ctrl Pts',(-18.5748042848117,24.731787932081,124.282445362066)) ;
#28807=CARTESIAN_POINT('Ctrl Pts',(-18.1921666070184,24.9218254520271,124.30150622892)) ;
#28808=CARTESIAN_POINT('Ctrl Pts',(-18.4355860078039,24.7418363716642,124.123567103051)) ;
#28809=CARTESIAN_POINT('Ctrl Pts',(-18.056967678217,24.931774946275,124.077710500125)) ;
#28810=CARTESIAN_POINT('Ctrl Pts',(-18.3274273007974,24.7517858659121,123.944530798796)) ;
#28811=CARTESIAN_POINT('Ctrl Pts',(-17.9623422828139,24.941682802001,123.835129981)) ;
#28812=CARTESIAN_POINT('Ctrl Pts',(-18.25172727253,24.7616937216381,123.750467050901)) ;
#28813=CARTESIAN_POINT('Ctrl Pts',(-17.9107761380726,24.9517422786509,123.575884197323)) ;
#28814=CARTESIAN_POINT('Ctrl Pts',(-18.2104744001724,24.771753198288,123.543070133189)) ;
#28815=CARTESIAN_POINT('Ctrl Pts',(-17.9047808645182,24.9615830880596,123.317314560702)) ;
#28816=CARTESIAN_POINT('Ctrl Pts',(-18.2056782172109,24.7815940076967,123.336215598447)) ;
#28817=CARTESIAN_POINT('Ctrl Pts',(-17.9443132377084,24.9716452383604,123.055891956674)) ;
#28818=CARTESIAN_POINT('Ctrl Pts',(-18.237304086214,24.7916561579975,123.127077212028)) ;
#28819=CARTESIAN_POINT('Ctrl Pts',(-18.027522505227,24.981542399483,122.809459900675)) ;
#28820=CARTESIAN_POINT('Ctrl Pts',(-18.3038712398251,24.8015533191201,122.929932325436)) ;
#28821=CARTESIAN_POINT('Ctrl Pts',(-18.15191407074,24.991473573887,122.580036852208)) ;
#28822=CARTESIAN_POINT('Ctrl Pts',(-18.4033840182732,24.8114844935241,122.746394285566)) ;
#28823=CARTESIAN_POINT('Ctrl Pts',(-18.3162936300384,25.001515777612,122.373591256392)) ;
#28824=CARTESIAN_POINT('Ctrl Pts',(-18.5348876504328,24.8215266972492,122.581237583697)) ;
#28825=CARTESIAN_POINT('Ctrl Pts',(-18.5108445770742,25.0114023600425,122.201377852405)) ;
#28826=CARTESIAN_POINT('Ctrl Pts',(-18.6905276243258,24.8314132796796,122.443467286876)) ;
#28827=CARTESIAN_POINT('Ctrl Pts',(-18.7344855027603,25.0213957957908,122.063738108185)) ;
#28828=CARTESIAN_POINT('Ctrl Pts',(-18.8694400641659,24.8414067154279,122.333355312054)) ;
#28829=CARTESIAN_POINT('Ctrl Pts',(-18.9774777481212,25.031340264149,121.967563232072)) ;
#28830=CARTESIAN_POINT('Ctrl Pts',(-19.0638333079419,24.8513511837861,122.256415320713)) ;
#28831=CARTESIAN_POINT('Ctrl Pts',(-19.2335763972328,25.0412920803945,121.914516693683)) ;
#28832=CARTESIAN_POINT('Ctrl Pts',(-19.2687117105756,24.8613030000317,122.213977773435)) ;
#28833=CARTESIAN_POINT('Ctrl Pts',(-19.4972265998584,25.051329516509,121.906917954592)) ;
#28834=CARTESIAN_POINT('Ctrl Pts',(-19.4796319935927,24.8713404361461,122.207898425137)) ;
#28835=CARTESIAN_POINT('Ctrl Pts',(-19.7542997604475,25.0612144756854,121.944387345544)) ;
#28836=CARTESIAN_POINT('Ctrl Pts',(-19.6852897308738,24.8812253953225,122.237873404825)) ;
#28837=CARTESIAN_POINT('Ctrl Pts',(-20.0038315528282,25.0712125938973,122.026544562977)) ;
#28838=CARTESIAN_POINT('Ctrl Pts',(-19.8849152007323,24.8912235135344,122.303598670447)) ;
#28839=CARTESIAN_POINT('Ctrl Pts',(-20.2336588620757,25.0811335264093,122.149690526495)) ;
#28840=CARTESIAN_POINT('Ctrl Pts',(-20.0687767521282,24.9011444460464,122.402114675573)) ;
#28841=CARTESIAN_POINT('Ctrl Pts',(-20.4411095234431,25.0911748266313,122.31274727971)) ;
#28842=CARTESIAN_POINT('Ctrl Pts',(-20.2347377340864,24.9111857462685,122.532559732178)) ;
#28843=CARTESIAN_POINT('Ctrl Pts',(-20.6146855652456,25.1010817450213,122.506787487702)) ;
#28844=CARTESIAN_POINT('Ctrl Pts',(-20.3735984857151,24.9210926646584,122.687791010339)) ;
#28845=CARTESIAN_POINT('Ctrl Pts',(-20.7529678400047,25.1110175367304,122.728267052382)) ;
#28846=CARTESIAN_POINT('Ctrl Pts',(-20.4842246343113,24.9310284563675,122.86497383834)) ;
#28847=CARTESIAN_POINT('Ctrl Pts',(-20.8514767358832,25.1210584313083,122.973046599286)) ;
#28848=CARTESIAN_POINT('Ctrl Pts',(-20.5630324089093,24.9410693509454,123.060797371555)) ;
#28849=CARTESIAN_POINT('Ctrl Pts',(-20.9053425589782,25.1309456330221,123.227241473632)) ;
#28850=CARTESIAN_POINT('Ctrl Pts',(-20.6061255751286,24.9509565526592,123.264152313877)) ;
#28851=CARTESIAN_POINT('Ctrl Pts',(-20.9147827032288,25.1409379007837,123.489640019812)) ;
#28852=CARTESIAN_POINT('Ctrl Pts',(-20.6136784849478,24.9609488204208,123.474070959372)) ;
#28853=CARTESIAN_POINT('Ctrl Pts',(-20.8786010725189,25.1508864218055,123.748576028363)) ;
#28854=CARTESIAN_POINT('Ctrl Pts',(-20.5847340147397,24.9708973414426,123.681219445159)) ;
#28855=CARTESIAN_POINT('Ctrl Pts',(-20.7984664179347,25.1608231953832,123.997081667606)) ;
#28856=CARTESIAN_POINT('Ctrl Pts',(-20.5206272762469,24.9808341150203,123.880023738464)) ;
#28857=CARTESIAN_POINT('Ctrl Pts',(-20.6760989906385,25.1708062435242,124.229175844446)) ;
#28858=CARTESIAN_POINT('Ctrl Pts',(-20.4227342680816,24.9908171631614,124.065699340434)) ;
#28859=CARTESIAN_POINT('Ctrl Pts',(-20.5139718407011,25.1808499511343,124.437414474404)) ;
#28860=CARTESIAN_POINT('Ctrl Pts',(-20.2930331145472,25.0008608707714,124.232290876119)) ;
#28861=CARTESIAN_POINT('Ctrl Pts',(-20.3226951495202,25.1906786442876,124.611032523133)) ;
#28862=CARTESIAN_POINT('Ctrl Pts',(-20.1400132673799,25.0106895639247,124.371185263449)) ;
#28863=CARTESIAN_POINT('Ctrl Pts',(-20.098868954127,25.200753393417,124.752367074633)) ;
#28864=CARTESIAN_POINT('Ctrl Pts',(-19.9609525783771,25.0207643130542,124.484253941825)) ;
#28865=CARTESIAN_POINT('Ctrl Pts',(-19.858910190644,25.2106187192126,124.850577176108)) ;
#28866=CARTESIAN_POINT('Ctrl Pts',(-19.7689867940253,25.0306296388497,124.562822605687)) ;
#28867=CARTESIAN_POINT('Ctrl Pts',(-19.6016970937392,25.2206408935695,124.907156637884)) ;
#28868=CARTESIAN_POINT('Ctrl Pts',(-19.5632165305531,25.0406518132067,124.608087310509)) ;
#28869=CARTESIAN_POINT('Ctrl Pts',(-19.33841109203,25.2306669467765,124.91757426496)) ;
#28870=CARTESIAN_POINT('Ctrl Pts',(-19.3525877130776,25.0506778664136,124.616422422536)) ;
#28871=CARTESIAN_POINT('Ctrl Pts',(-19.0817846505437,25.2405206436227,124.883149004069)) ;
#28872=CARTESIAN_POINT('Ctrl Pts',(-19.1472873801373,25.0605315632599,124.588883436946)) ;
#28873=CARTESIAN_POINT('Ctrl Pts',(-18.8321213569949,25.2504800483757,124.804588928289)) ;
#28874=CARTESIAN_POINT('Ctrl Pts',(-18.9475566863649,25.0704909680128,124.526036697892)) ;
#28875=CARTESIAN_POINT('Ctrl Pts',(-18.5982908950502,25.2605182940806,124.68251138002)) ;
#28876=CARTESIAN_POINT('Ctrl Pts',(-18.7604916748522,25.0805292137177,124.428375651128)) ;
#28877=CARTESIAN_POINT('Ctrl Pts',(-18.3923032184799,25.2703924782426,124.52465527997)) ;
#28878=CARTESIAN_POINT('Ctrl Pts',(-18.5957014002325,25.0904033978798,124.302092277131)) ;
#28879=CARTESIAN_POINT('Ctrl Pts',(-18.2134348354326,25.2804622613806,124.32968799242)) ;
#28880=CARTESIAN_POINT('Ctrl Pts',(-18.4526055652732,25.1004731810177,124.146119103615)) ;
#28881=CARTESIAN_POINT('Ctrl Pts',(-18.0743301698985,25.2902955164013,124.111890050986)) ;
#28882=CARTESIAN_POINT('Ctrl Pts',(-18.341321285219,25.1103064360384,123.971882314404)) ;
#28883=CARTESIAN_POINT('Ctrl Pts',(-17.9724906536207,25.300325942533,123.868778335182)) ;
#28884=CARTESIAN_POINT('Ctrl Pts',(-18.2598482995309,25.1203368621701,123.777393441329)) ;
#28885=CARTESIAN_POINT('Ctrl Pts',(-17.9151462002579,25.31035755472,123.611455902983)) ;
#28886=CARTESIAN_POINT('Ctrl Pts',(-18.213971454411,25.1303684743571,123.571535713818)) ;
#28887=CARTESIAN_POINT('Ctrl Pts',(-17.9030533678709,25.3201872515746,123.353441667699)) ;
#28888=CARTESIAN_POINT('Ctrl Pts',(-18.2042958249843,25.1401981712117,123.365125405049)) ;
#28889=CARTESIAN_POINT('Ctrl Pts',(-17.935703946638,25.3301766934771,123.092960405583)) ;
#28890=CARTESIAN_POINT('Ctrl Pts',(-18.2304147144429,25.1501876131142,123.156740340782)) ;
#28891=CARTESIAN_POINT('Ctrl Pts',(-18.01414488107,25.3402205854928,122.840945210804)) ;
#28892=CARTESIAN_POINT('Ctrl Pts',(-18.293166125743,25.1602315051299,122.955127645986)) ;
#28893=CARTESIAN_POINT('Ctrl Pts',(-18.1320014123289,25.350042147262,122.611326074322)) ;
#28894=CARTESIAN_POINT('Ctrl Pts',(-18.3874495259112,25.1700530668991,122.771432519081)) ;
#28895=CARTESIAN_POINT('Ctrl Pts',(-18.290812004256,25.3600777188862,122.400775785575)) ;
#28896=CARTESIAN_POINT('Ctrl Pts',(-18.5144967171378,25.1800886385233,122.602991221329)) ;
#28897=CARTESIAN_POINT('Ctrl Pts',(-18.4841839838092,25.370106993168,122.221692735608)) ;
#28898=CARTESIAN_POINT('Ctrl Pts',(-18.6691932985931,25.1901179128051,122.459723641306)) ;
#28899=CARTESIAN_POINT('Ctrl Pts',(-18.7010269361118,25.3799408302867,122.081101987193)) ;
#28900=CARTESIAN_POINT('Ctrl Pts',(-18.8426660234848,25.1999517499238,122.347250143643)) ;
#28901=CARTESIAN_POINT('Ctrl Pts',(-18.9441309444256,25.3899932263748,121.977771975232)) ;
#28902=CARTESIAN_POINT('Ctrl Pts',(-19.037148711284,25.2100041460119,122.264584503233)) ;
#28903=CARTESIAN_POINT('Ctrl Pts',(-19.1986250893084,25.3999299933253,121.919230643914)) ;
#28904=CARTESIAN_POINT('Ctrl Pts',(-19.2407432792532,25.2199409129625,122.21774992714)) ;
#28905=CARTESIAN_POINT('Ctrl Pts',(-19.459301128586,25.4098642283046,121.905097168243)) ;
#28906=CARTESIAN_POINT('Ctrl Pts',(-19.4492836234959,25.2298751479417,122.206441411335)) ;
#28907=CARTESIAN_POINT('Ctrl Pts',(-19.72078773703,25.4198879916314,121.936883279556)) ;
#28908=CARTESIAN_POINT('Ctrl Pts',(-19.6584731310004,25.2398989112685,122.231868582496)) ;
#28909=CARTESIAN_POINT('Ctrl Pts',(-19.9693851432808,25.429774333016,122.012355109386)) ;
#28910=CARTESIAN_POINT('Ctrl Pts',(-19.8573510090563,25.2497852526532,122.292244189265)) ;
#28911=CARTESIAN_POINT('Ctrl Pts',(-20.2037937296493,25.439763381783,122.130525368287)) ;
#28912=CARTESIAN_POINT('Ctrl Pts',(-20.0448786033805,25.2597743014202,122.38677867719)) ;
#28913=CARTESIAN_POINT('Ctrl Pts',(-20.4148854638875,25.4498046024804,122.288855457116)) ;
#28914=CARTESIAN_POINT('Ctrl Pts',(-20.213753113731,25.2698155221175,122.513441372726)) ;
#28915=CARTESIAN_POINT('Ctrl Pts',(-20.5918392755866,25.4596372426583,122.477141002139)) ;
#28916=CARTESIAN_POINT('Ctrl Pts',(-20.3553169822991,25.2796481622954,122.664067990868)) ;
#28917=CARTESIAN_POINT('Ctrl Pts',(-20.7363655379612,25.4696311719663,122.696425976588)) ;
#28918=CARTESIAN_POINT('Ctrl Pts',(-20.4709395700862,25.2896420916034,122.839494814172)) ;
#28919=CARTESIAN_POINT('Ctrl Pts',(-20.8404780632738,25.4796603796468,122.93854969465)) ;
#28920=CARTESIAN_POINT('Ctrl Pts',(-20.5542313158732,25.2996712992839,123.033193065027)) ;
#28921=CARTESIAN_POINT('Ctrl Pts',(-20.9004575630717,25.4895361913509,123.191064817286)) ;
#28922=CARTESIAN_POINT('Ctrl Pts',(-20.6022166706708,25.309547110988,123.235204193094)) ;
#28923=CARTESIAN_POINT('Ctrl Pts',(-20.9161564441938,25.4995354183223,123.453329386861)) ;
#28924=CARTESIAN_POINT('Ctrl Pts',(-20.6147777399727,25.3195463379594,123.445015642034)) ;
#28925=CARTESIAN_POINT('Ctrl Pts',(-20.8865881009697,25.509444899478,123.712094698215)) ;
#28926=CARTESIAN_POINT('Ctrl Pts',(-20.5911250962336,25.3294558191151,123.65202774278)) ;
#28927=CARTESIAN_POINT('Ctrl Pts',(-20.81145089258,25.5194981297789,123.965343699702)) ;
#28928=CARTESIAN_POINT('Ctrl Pts',(-20.5310172244404,25.339509049416,123.854627590473)) ;
#28929=CARTESIAN_POINT('Ctrl Pts',(-20.6957175422055,25.52936874633,124.197502953534)) ;
#28930=CARTESIAN_POINT('Ctrl Pts',(-20.438432564313,25.3493796659671,124.040355455078)) ;
#28931=CARTESIAN_POINT('Ctrl Pts',(-20.5395534186836,25.539390408062,124.409561109384)) ;
#28932=CARTESIAN_POINT('Ctrl Pts',(-20.3135029430388,25.3594013276991,124.210003211742)) ;
#28933=CARTESIAN_POINT('Ctrl Pts',(-20.3484908449209,25.5494132212431,124.590878299816)) ;
#28934=CARTESIAN_POINT('Ctrl Pts',(-20.1606542784881,25.3694241408802,124.355058414572)) ;
#28935=CARTESIAN_POINT('Ctrl Pts',(-20.1325195803171,25.5592803857031,124.734357216796)) ;
#28936=CARTESIAN_POINT('Ctrl Pts',(-19.987878794653,25.3792913053402,124.469843008238)) ;
#28937=CARTESIAN_POINT('Ctrl Pts',(-19.8920996177146,25.569273827923,124.840044812153)) ;
#28938=CARTESIAN_POINT('Ctrl Pts',(-19.7955437603287,25.3892847475601,124.554394994497)) ;
#28939=CARTESIAN_POINT('Ctrl Pts',(-19.6358915111173,25.5793055015233,124.902119378316)) ;
#28940=CARTESIAN_POINT('Ctrl Pts',(-19.5905777624909,25.3993164211604,124.604056661626)) ;
#28941=CARTESIAN_POINT('Ctrl Pts',(-19.377143513442,25.5891719366363,124.918889100785)) ;
#28942=CARTESIAN_POINT('Ctrl Pts',(-19.3835799123551,25.4091828562734,124.617474520486)) ;
#28943=CARTESIAN_POINT('Ctrl Pts',(-19.1162493958071,25.5991593871694,124.890557819024)) ;
#28944=CARTESIAN_POINT('Ctrl Pts',(-19.1748644832375,25.4191703068065,124.594811646345)) ;
#28945=CARTESIAN_POINT('Ctrl Pts',(-18.8652039002789,25.6091043169973,124.817783333034)) ;
#28946=CARTESIAN_POINT('Ctrl Pts',(-18.9740276649419,25.4291152366345,124.536594184406)) ;
#28947=CARTESIAN_POINT('Ctrl Pts',(-18.6283721225821,25.6191492120525,124.701260743701)) ;
#28948=CARTESIAN_POINT('Ctrl Pts',(-18.784561279619,25.4391601316896,124.443378036371)) ;
#28949=CARTESIAN_POINT('Ctrl Pts',(-18.419077049514,25.6290112737383,124.548382059341)) ;
#28950=CARTESIAN_POINT('Ctrl Pts',(-18.6171242178969,25.4490221933754,124.321077040016)) ;
#28951=CARTESIAN_POINT('Ctrl Pts',(-18.2367942709095,25.6390029965252,124.359421375143)) ;
#28952=CARTESIAN_POINT('Ctrl Pts',(-18.4712964601253,25.4590139161623,124.169910079133)) ;
#28953=CARTESIAN_POINT('Ctrl Pts',(-18.091029495205,25.6489352107651,124.142904444548)) ;
#28954=CARTESIAN_POINT('Ctrl Pts',(-18.3546829152542,25.4689461304023,123.996697908865)) ;
#28955=CARTESIAN_POINT('Ctrl Pts',(-17.9844458363519,25.6588745293309,123.904437503963)) ;
#28956=CARTESIAN_POINT('Ctrl Pts',(-18.2694140074215,25.478885448968,123.805925391818)) ;
#28957=CARTESIAN_POINT('Ctrl Pts',(-17.9204539831751,25.6689187041067,123.648365609469)) ;
#28958=CARTESIAN_POINT('Ctrl Pts',(-18.2182183772246,25.4889296237439,123.60106842999)) ;
#28959=CARTESIAN_POINT('Ctrl Pts',(-17.9020768058315,25.6787892581717,123.389630116784)) ;
#28960=CARTESIAN_POINT('Ctrl Pts',(-18.2035144291742,25.4988001778088,123.394080402049)) ;
#28961=CARTESIAN_POINT('Ctrl Pts',(-17.9284060681277,25.6887542405259,123.1290873224)) ;
#28962=CARTESIAN_POINT('Ctrl Pts',(-18.2245755901221,25.508765160163,123.185646014976)) ;
#28963=CARTESIAN_POINT('Ctrl Pts',(-18.000430199717,25.6987849434157,122.875529417126)) ;
#28964=CARTESIAN_POINT('Ctrl Pts',(-18.2821927290592,25.5187958630528,122.98279912396)) ;
#28965=CARTESIAN_POINT('Ctrl Pts',(-18.1134771988756,25.7086772834409,122.641401239108)) ;
#28966=CARTESIAN_POINT('Ctrl Pts',(-18.3726282522614,25.528688203078,122.795495711768)) ;
#28967=CARTESIAN_POINT('Ctrl Pts',(-18.2678679863379,25.7187305166009,122.427066576845)) ;
#28968=CARTESIAN_POINT('Ctrl Pts',(-18.4961390336313,25.538741436238,122.624026697012)) ;
#28969=CARTESIAN_POINT('Ctrl Pts',(-18.4538393268546,25.7286117610776,122.245777047898)) ;
#28970=CARTESIAN_POINT('Ctrl Pts',(-18.6449144658524,25.5486226807147,122.478993530744)) ;
#28971=CARTESIAN_POINT('Ctrl Pts',(-18.6715752593228,25.7386448819486,122.097176077592)) ;
#28972=CARTESIAN_POINT('Ctrl Pts',(-18.8191018953641,25.5586558015858,122.360110920692)) ;
#28973=CARTESIAN_POINT('Ctrl Pts',(-18.9081608033064,25.7485260922237,121.990030737852)) ;
#28974=CARTESIAN_POINT('Ctrl Pts',(-19.0083693555972,25.5685370118608,122.274392619025)) ;
#28975=CARTESIAN_POINT('Ctrl Pts',(-19.1642552672847,25.758588167993,121.924365385186)) ;
#28976=CARTESIAN_POINT('Ctrl Pts',(-19.2132442996693,25.5785990876302,122.2218581685)) ;
#28977=CARTESIAN_POINT('Ctrl Pts',(-19.4225607860531,25.7684452263748,121.904478285387)) ;
#28978=CARTESIAN_POINT('Ctrl Pts',(-19.4198885350739,25.5884561460119,122.205946244612)) ;
#28979=CARTESIAN_POINT('Ctrl Pts',(-19.6839642883553,25.7784397816638,121.929561151871)) ;
#28980=CARTESIAN_POINT('Ctrl Pts',(-19.6290115124918,25.5984507013009,122.226010297302)) ;
#28981=CARTESIAN_POINT('Ctrl Pts',(-19.9354025958823,25.7883656691993,121.999101330404)) ;
#28982=CARTESIAN_POINT('Ctrl Pts',(-19.8301627662093,25.6083765888364,122.281640286907)) ;
#28983=CARTESIAN_POINT('Ctrl Pts',(-20.1732821454297,25.7983906891946,122.112270545144)) ;
#28984=CARTESIAN_POINT('Ctrl Pts',(-20.020467298116,25.6184016088317,122.372173604384)) ;
#28985=CARTESIAN_POINT('Ctrl Pts',(-20.3852412939983,25.8082880662982,122.26301982624)) ;
#28986=CARTESIAN_POINT('Ctrl Pts',(-20.1900359672413,25.6282989859354,122.49277124775)) ;
#28987=CARTESIAN_POINT('Ctrl Pts',(-20.5699265939808,25.8182783033791,122.449617357553)) ;
#28988=CARTESIAN_POINT('Ctrl Pts',(-20.3377857573925,25.6382892230162,122.64204770688)) ;
#28989=CARTESIAN_POINT('Ctrl Pts',(-20.7196773404664,25.8283149161879,122.666729559919)) ;
#28990=CARTESIAN_POINT('Ctrl Pts',(-20.4575881296598,25.648325835825,122.815736096847)) ;
#28991=CARTESIAN_POINT('Ctrl Pts',(-20.8278012350198,25.8381647996059,122.901920140004)) ;
#28992=CARTESIAN_POINT('Ctrl Pts',(-20.5440893331541,25.658175719243,123.003887861845)) ;
#28993=CARTESIAN_POINT('Ctrl Pts',(-20.8949727103039,25.8481684165084,123.156051177432)) ;
#28994=CARTESIAN_POINT('Ctrl Pts',(-20.5978286197024,25.6681793361455,123.207191954639)) ;
#28995=CARTESIAN_POINT('Ctrl Pts',(-20.9168297433397,25.8581578282735,123.417692998704)) ;
#28996=CARTESIAN_POINT('Ctrl Pts',(-20.6153163642316,25.6781687479106,123.416505743654)) ;
#28997=CARTESIAN_POINT('Ctrl Pts',(-20.8926982525151,25.8681765896183,123.67984195633)) ;
#28998=CARTESIAN_POINT('Ctrl Pts',(-20.5960135622755,25.6881875092555,123.626222991465)) ;
#28999=CARTESIAN_POINT('Ctrl Pts',(-20.8017581311539,25.8813952649994,124.015153473732)) ;
#29000=CARTESIAN_POINT('Ctrl Pts',(-20.5232632286193,25.7014061846365,123.894483244612)) ;
#29001=CARTESIAN_POINT('Ctrl Pts',(-20.6243920028856,25.8947055722441,124.321133430442)) ;
#29002=CARTESIAN_POINT('Ctrl Pts',(-20.3813483028792,25.7147164918812,124.139291566757)) ;
#29003=CARTESIAN_POINT('Ctrl Pts',(-20.3779377392562,25.9079432384701,124.566705392269)) ;
#29004=CARTESIAN_POINT('Ctrl Pts',(-20.1842168620273,25.7279541581072,124.335714004042)) ;
#29005=CARTESIAN_POINT('Ctrl Pts',(-20.1646098417396,25.9178629338808,124.716521317829)) ;
#29006=CARTESIAN_POINT('Ctrl Pts',(-20.0135493900519,25.7378738535179,124.455576016923)) ;
#29007=CARTESIAN_POINT('Ctrl Pts',(-19.9252257840937,25.9279158008794,124.828226044214)) ;
#29008=CARTESIAN_POINT('Ctrl Pts',(-19.8220451597961,25.7479267205165,124.544939701704)) ;
#29009=CARTESIAN_POINT('Ctrl Pts',(-19.6751350635831,25.9377712092086,124.895616007158)) ;
#29010=CARTESIAN_POINT('Ctrl Pts',(-19.6219710432747,25.7577821288458,124.598853833472)) ;
#29011=CARTESIAN_POINT('Ctrl Pts',(-19.4124225556355,25.9478098408852,124.919414322609)) ;
#29012=CARTESIAN_POINT('Ctrl Pts',(-19.4118058300607,25.7678207605223,124.617896055851)) ;
#29013=CARTESIAN_POINT('Ctrl Pts',(-19.0641152659986,25.9611120231522,124.889602889987)) ;
#29014=CARTESIAN_POINT('Ctrl Pts',(-19.1331381422336,25.7811229427894,124.594040874612)) ;
#29015=CARTESIAN_POINT('Ctrl Pts',(-18.6502847526992,25.9776570362351,124.740819809691)) ;
#29016=CARTESIAN_POINT('Ctrl Pts',(-18.8021063710032,25.7976679558722,124.475037523198)) ;
#29017=CARTESIAN_POINT('Ctrl Pts',(-18.3098802866931,25.9943090523113,124.458074394266)) ;
#29018=CARTESIAN_POINT('Ctrl Pts',(-18.5297345562069,25.8143199719484,124.248799717003)) ;
#29019=CARTESIAN_POINT('Ctrl Pts',(-18.1090436808664,26.0075321432166,124.174455573223)) ;
#29020=CARTESIAN_POINT('Ctrl Pts',(-18.369098690815,25.8275430628537,124.021942719457)) ;
#29021=CARTESIAN_POINT('Ctrl Pts',(-17.9965176539852,26.0174931027759,123.938117510176)) ;
#29022=CARTESIAN_POINT('Ctrl Pts',(-18.2790691278245,25.837504022413,123.832864843426)) ;
#29023=CARTESIAN_POINT('Ctrl Pts',(-17.9266031351628,26.027517899527,123.684128674994)) ;
#29024=CARTESIAN_POINT('Ctrl Pts',(-18.223137350365,25.8475288191641,123.629678646653)) ;
#29025=CARTESIAN_POINT('Ctrl Pts',(-17.8934600554389,26.0407423469228,123.338151922398)) ;
#29026=CARTESIAN_POINT('Ctrl Pts',(-18.1966218500974,25.8607532665599,123.352885080339)) ;
#29027=CARTESIAN_POINT('Ctrl Pts',(-17.9661098980233,26.0573761316219,122.902122581917)) ;
#29028=CARTESIAN_POINT('Ctrl Pts',(-18.2547370849816,25.877387051259,123.004073841914)) ;
#29029=CARTESIAN_POINT('Ctrl Pts',(-18.2260016702492,26.0772787983468,122.441338078492)) ;
#29030=CARTESIAN_POINT('Ctrl Pts',(-18.4626485568475,25.897289717984,122.6354399701)) ;
#29031=CARTESIAN_POINT('Ctrl Pts',(-18.6269689740633,26.0971790261287,122.096464789941)) ;
#29032=CARTESIAN_POINT('Ctrl Pts',(-18.7834208261286,25.9171899457658,122.359539719814)) ;
#29033=CARTESIAN_POINT('Ctrl Pts',(-19.1218834344603,26.1170965136602,121.908606135804)) ;
#29034=CARTESIAN_POINT('Ctrl Pts',(-19.1793520415274,25.9371074332973,122.209249695182)) ;
#29035=CARTESIAN_POINT('Ctrl Pts',(-19.6515421009118,26.1370260394771,121.900579250022)) ;
#29036=CARTESIAN_POINT('Ctrl Pts',(-19.6030795010678,25.9570369591142,122.202825735213)) ;
#29037=CARTESIAN_POINT('Ctrl Pts',(-20.1529386123422,26.1569883073634,122.074158377623)) ;
#29038=CARTESIAN_POINT('Ctrl Pts',(-20.0041977734396,25.9769992270005,122.341686821222)) ;
#29039=CARTESIAN_POINT('Ctrl Pts',(-20.5634651727886,26.1768785023156,122.407118082729)) ;
#29040=CARTESIAN_POINT('Ctrl Pts',(-20.3326212396169,25.9968894219527,122.608053440236)) ;
#29041=CARTESIAN_POINT('Ctrl Pts',(-20.8369695350651,26.1967687470618,122.859653772299)) ;
#29042=CARTESIAN_POINT('Ctrl Pts',(-20.5514266616668,26.016779666699,122.970082039285)) ;
#29043=CARTESIAN_POINT('Ctrl Pts',(-20.9394612388346,26.2168431196243,123.383189522101)) ;
#29044=CARTESIAN_POINT('Ctrl Pts',(-20.6334217424483,26.0368540392614,123.388909499368)) ;
#29045=CARTESIAN_POINT('Ctrl Pts',(-20.858478621002,26.2366284969846,123.902848054689)) ;
#29046=CARTESIAN_POINT('Ctrl Pts',(-20.5686369629156,26.0566394166217,123.80463880822)) ;
#29047=CARTESIAN_POINT('Ctrl Pts',(-20.604272042101,26.2565903710517,124.368482650199)) ;
#29048=CARTESIAN_POINT('Ctrl Pts',(-20.3652721856668,26.0766012906889,124.177147290224)) ;
#29049=CARTESIAN_POINT('Ctrl Pts',(-20.2051802401964,26.2765703465422,124.718824795122)) ;
#29050=CARTESIAN_POINT('Ctrl Pts',(-20.0459994054117,26.0965812661794,124.457422009913)) ;
#29051=CARTESIAN_POINT('Ctrl Pts',(-19.7149987089246,26.2963827764202,124.911292999828)) ;
#29052=CARTESIAN_POINT('Ctrl Pts',(-19.6538521960381,26.1163936960573,124.611397916623)) ;
#29053=CARTESIAN_POINT('Ctrl Pts',(-19.1842547999823,26.3163628845105,124.925735636618)) ;
#29054=CARTESIAN_POINT('Ctrl Pts',(-19.2292567523326,26.1363738041476,124.622952026166)) ;
#29055=CARTESIAN_POINT('Ctrl Pts',(-18.6824717518944,26.3362572681077,124.758627144309)) ;
#29056=CARTESIAN_POINT('Ctrl Pts',(-18.8278291137582,26.1562681877448,124.489264722442)) ;
#29057=CARTESIAN_POINT('Ctrl Pts',(-18.2670439988586,26.3561841960849,124.430303289928)) ;
#29058=CARTESIAN_POINT('Ctrl Pts',(-18.4954865238769,26.1761951157221,124.226604620263)) ;
#29059=CARTESIAN_POINT('Ctrl Pts',(-17.9883141683562,26.3760790533862,123.980817223551)) ;
#29060=CARTESIAN_POINT('Ctrl Pts',(-18.2725029335029,26.1960899730233,123.867014230406)) ;
#29061=CARTESIAN_POINT('Ctrl Pts',(-17.8794749235701,26.3961182469898,123.459500138785)) ;
#29062=CARTESIAN_POINT('Ctrl Pts',(-18.1854325963948,26.2161291666269,123.449960783738)) ;
#29063=CARTESIAN_POINT('Ctrl Pts',(-17.9544430376458,26.4159582149006,122.937489228161)) ;
#29064=CARTESIAN_POINT('Ctrl Pts',(-18.2454084587968,26.2359691345377,123.032350471907)) ;
#29065=CARTESIAN_POINT('Ctrl Pts',(-18.2027276437108,26.4358730318646,122.470081707864)) ;
#29066=CARTESIAN_POINT('Ctrl Pts',(-18.4440381844851,26.2558839515018,122.658424577818)) ;
#29067=CARTESIAN_POINT('Ctrl Pts',(-18.596400995126,26.4558152772609,122.115240379138)) ;
#29068=CARTESIAN_POINT('Ctrl Pts',(-18.7589785547177,26.275826196898,122.374552517246)) ;
#29069=CARTESIAN_POINT('Ctrl Pts',(-19.0856111707764,26.4756873253754,121.915849802114)) ;
#29070=CARTESIAN_POINT('Ctrl Pts',(-19.1503485944393,26.2956982450125,122.215041802279)) ;
#29071=CARTESIAN_POINT('Ctrl Pts',(-19.6169161682822,26.4956983903295,121.895626311636)) ;
#29072=CARTESIAN_POINT('Ctrl Pts',(-19.57539261041,26.3157093099666,122.198865364486)) ;
#29073=CARTESIAN_POINT('Ctrl Pts',(-20.118823655691,26.5155099146331,122.055636433992)) ;
#29074=CARTESIAN_POINT('Ctrl Pts',(-19.9769191395575,26.3355208342703,122.326876501952)) ;
#29075=CARTESIAN_POINT('Ctrl Pts',(-20.5414187886625,26.5356051265965,122.381904092641)) ;
#29076=CARTESIAN_POINT('Ctrl Pts',(-20.3149929725486,26.3556160462336,122.587892382152)) ;
#29077=CARTESIAN_POINT('Ctrl Pts',(-20.8229786362358,26.5553858505163,122.826139617815)) ;
#29078=CARTESIAN_POINT('Ctrl Pts',(-20.5402392941985,26.3753967701534,122.943283661868)) ;
#29079=CARTESIAN_POINT('Ctrl Pts',(-20.9383530388371,26.5753769261591,123.344589665565)) ;
#29080=CARTESIAN_POINT('Ctrl Pts',(-20.6325355740105,26.3953878457962,123.358044462546)) ;
#29081=CARTESIAN_POINT('Ctrl Pts',(-20.86985320622,26.5952588652021,123.868710610695)) ;
#29082=CARTESIAN_POINT('Ctrl Pts',(-20.577732355409,26.4152697848392,123.777341477282)) ;
#29083=CARTESIAN_POINT('Ctrl Pts',(-20.6263804833536,26.6152114697054,124.339726432393)) ;
#29084=CARTESIAN_POINT('Ctrl Pts',(-20.3829508664611,26.4352223893425,124.154152702177)) ;
#29085=CARTESIAN_POINT('Ctrl Pts',(-20.2377323609478,26.635110338436,124.698507478413)) ;
#29086=CARTESIAN_POINT('Ctrl Pts',(-20.0720296498314,26.4551212580731,124.441175303376)) ;
#29087=CARTESIAN_POINT('Ctrl Pts',(-19.750506384729,26.6550037382456,124.903616092832)) ;
#29088=CARTESIAN_POINT('Ctrl Pts',(-19.6822465171285,26.4750146578827,124.605258460819)) ;
#29089=CARTESIAN_POINT('Ctrl Pts',(-19.2219548120851,26.6749128690856,124.930993209538)) ;
#29090=CARTESIAN_POINT('Ctrl Pts',(-19.2594063325904,26.4949237887228,124.627157492375)) ;
#29091=CARTESIAN_POINT('Ctrl Pts',(-18.7130356342311,26.6949449688492,124.774763267432)) ;
#29092=CARTESIAN_POINT('Ctrl Pts',(-18.8522664567341,26.5149558884863,124.502164665301)) ;
#29093=CARTESIAN_POINT('Ctrl Pts',(-18.3620528555376,26.7114770420187,124.510268121194)) ;
#29094=CARTESIAN_POINT('Ctrl Pts',(-18.5715001976287,26.5314879616558,124.290581423656)) ;
#29095=CARTESIAN_POINT('Ctrl Pts',(-18.1460617747501,26.7248123826246,124.234367496516)) ;
#29096=CARTESIAN_POINT('Ctrl Pts',(-18.3986933386626,26.5448233022617,124.069844646193)) ;
#29097=CARTESIAN_POINT('Ctrl Pts',(-18.0239800547126,26.7346549411643,124.006303612785)) ;
#29098=CARTESIAN_POINT('Ctrl Pts',(-18.3010327997462,26.5546658608015,123.887397815469)) ;
#29099=CARTESIAN_POINT('Ctrl Pts',(-17.9413973813911,26.7447068480142,123.755428033597)) ;
#29100=CARTESIAN_POINT('Ctrl Pts',(-18.2349681691499,26.5647177676514,123.686685201408)) ;
#29101=CARTESIAN_POINT('Ctrl Pts',(-17.891686149238,26.7579553624051,123.410787353362)) ;
#29102=CARTESIAN_POINT('Ctrl Pts',(-18.1952008751101,26.5779662820423,123.411026738166)) ;
#29103=CARTESIAN_POINT('Ctrl Pts',(-17.9431815127596,26.7745545373529,122.972680824458)) ;
#29104=CARTESIAN_POINT('Ctrl Pts',(-18.2364062949001,26.59456545699,123.060472645166)) ;
#29105=CARTESIAN_POINT('Ctrl Pts',(-18.1408483242503,26.7911433231479,122.578566000262)) ;
#29106=CARTESIAN_POINT('Ctrl Pts',(-18.3945264353871,26.6111542427851,122.745229800877)) ;
#29107=CARTESIAN_POINT('Ctrl Pts',(-18.3723926843041,26.8044191394899,122.317598644227)) ;
#29108=CARTESIAN_POINT('Ctrl Pts',(-18.5797786876683,26.624430059127,122.536429224287)) ;
#29109=CARTESIAN_POINT('Ctrl Pts',(-18.5775216542846,26.8143929902837,122.15442033865)) ;
#29110=CARTESIAN_POINT('Ctrl Pts',(-18.7438803146688,26.6344039099208,122.405894095803)) ;
#29111=CARTESIAN_POINT('Ctrl Pts',(-18.8092589677791,26.8244220223761,122.028905565457)) ;
#29112=CARTESIAN_POINT('Ctrl Pts',(-18.9292719326846,26.6444329420132,122.305482723991)) ;
#29113=CARTESIAN_POINT('Ctrl Pts',(-19.0557421895212,26.834312147878,121.946421302957)) ;
#29114=CARTESIAN_POINT('Ctrl Pts',(-19.1264590870646,26.6543230675151,122.239497816618)) ;
#29115=CARTESIAN_POINT('Ctrl Pts',(-19.3153650354541,26.8443046261495,121.907247691411)) ;
#29116=CARTESIAN_POINT('Ctrl Pts',(-19.3341577092669,26.6643155457866,122.208161046948)) ;
#29117=CARTESIAN_POINT('Ctrl Pts',(-19.5768371046668,26.8542558412469,121.913582155201)) ;
#29118=CARTESIAN_POINT('Ctrl Pts',(-19.5433352791444,26.674266760884,122.213230894477)) ;
#29119=CARTESIAN_POINT('Ctrl Pts',(-19.8356332457282,26.8643043430019,121.965922317603)) ;
#29120=CARTESIAN_POINT('Ctrl Pts',(-19.7503716736977,26.6843152626391,122.255105201927)) ;
#29121=CARTESIAN_POINT('Ctrl Pts',(-20.0765024472187,26.8741456926187,122.060153190044)) ;
#29122=CARTESIAN_POINT('Ctrl Pts',(-19.9430662458474,26.6941566122558,122.330492010687)) ;
#29123=CARTESIAN_POINT('Ctrl Pts',(-20.3008378724975,26.8841319836389,122.196241980051)) ;
#29124=CARTESIAN_POINT('Ctrl Pts',(-20.1225333562957,26.7041429032761,122.439364943551)) ;
#29125=CARTESIAN_POINT('Ctrl Pts',(-20.4973053062689,26.8940685953675,122.368314358404)) ;
#29126=CARTESIAN_POINT('Ctrl Pts',(-20.2797057735737,26.7140795150047,122.577024505294)) ;
#29127=CARTESIAN_POINT('Ctrl Pts',(-20.662628518743,26.9041184707351,122.574234184223)) ;
#29128=CARTESIAN_POINT('Ctrl Pts',(-20.4119625510863,26.7241293903722,122.741761744443)) ;
#29129=CARTESIAN_POINT('Ctrl Pts',(-20.7873567686691,26.9139689292705,122.801084418396)) ;
#29130=CARTESIAN_POINT('Ctrl Pts',(-20.5117431267573,26.7339798489077,122.92324293676)) ;
#29131=CARTESIAN_POINT('Ctrl Pts',(-20.8724634669083,26.9239408662233,123.048897162386)) ;
#29132=CARTESIAN_POINT('Ctrl Pts',(-20.5798263274072,26.7439517858604,123.121493774499)) ;
#29133=CARTESIAN_POINT('Ctrl Pts',(-20.9133152577875,26.9339363231554,123.308411671272)) ;
#29134=CARTESIAN_POINT('Ctrl Pts',(-20.6125055330845,26.7539472427925,123.329105668054)) ;
#29135=CARTESIAN_POINT('Ctrl Pts',(-20.9081708679061,26.9439691302085,123.571995622508)) ;
#29136=CARTESIAN_POINT('Ctrl Pts',(-20.6083877656907,26.7639800498456,123.539972753807)) ;
#29137=CARTESIAN_POINT('Ctrl Pts',(-20.8585534427238,26.9538290167985,123.826321841959)) ;
#29138=CARTESIAN_POINT('Ctrl Pts',(-20.5686916578816,26.7738399364356,123.743433118056)) ;
#29139=CARTESIAN_POINT('Ctrl Pts',(-20.7647835915375,26.9638180973637,124.071480590036)) ;
#29140=CARTESIAN_POINT('Ctrl Pts',(-20.4936737272855,26.7838290170008,123.939559239062)) ;
#29141=CARTESIAN_POINT('Ctrl Pts',(-20.6306305349959,26.9737495765729,124.29536007837)) ;
#29142=CARTESIAN_POINT('Ctrl Pts',(-20.3863494522034,26.79376049621,124.118661555198)) ;
#29143=CARTESIAN_POINT('Ctrl Pts',(-20.4590264458182,26.9837354360188,124.493916247248)) ;
#29144=CARTESIAN_POINT('Ctrl Pts',(-20.2490645750113,26.8037463556559,124.277504981672)) ;
#29145=CARTESIAN_POINT('Ctrl Pts',(-20.254221659418,26.993773586666,124.66014484481)) ;
#29146=CARTESIAN_POINT('Ctrl Pts',(-20.0852193413478,26.8137845063031,124.410486127387)) ;
#29147=CARTESIAN_POINT('Ctrl Pts',(-20.0282504284219,27.0036216771704,124.786342691733)) ;
#29148=CARTESIAN_POINT('Ctrl Pts',(-19.9044415680484,26.8236325968075,124.511442329042)) ;
#29149=CARTESIAN_POINT('Ctrl Pts',(-19.7786397745395,27.0136825856884,124.873419336829)) ;
#29150=CARTESIAN_POINT('Ctrl Pts',(-19.7047522927702,26.8336935053255,124.581101595474)) ;
#29151=CARTESIAN_POINT('Ctrl Pts',(-19.5219286374244,27.0235774328464,124.914963808306)) ;
#29152=CARTESIAN_POINT('Ctrl Pts',(-19.4993832936596,26.8435883524835,124.614334963387)) ;
#29153=CARTESIAN_POINT('Ctrl Pts',(-19.2607200330095,27.0335191048914,124.911983091372)) ;
#29154=CARTESIAN_POINT('Ctrl Pts',(-19.2904166467755,26.8535300245285,124.611948249213)) ;
#29155=CARTESIAN_POINT('Ctrl Pts',(-19.002340474553,27.0435216320169,124.863486618766)) ;
#29156=CARTESIAN_POINT('Ctrl Pts',(-19.0837134587159,26.863532551654,124.573148990088)) ;
#29157=CARTESIAN_POINT('Ctrl Pts',(-18.755708647713,27.0535564232043,124.770193481186)) ;
#29158=CARTESIAN_POINT('Ctrl Pts',(-18.8864087522121,26.8735673428414,124.498512445791)) ;
#29159=CARTESIAN_POINT('Ctrl Pts',(-18.53306086531,27.0634013030634,124.63840012197)) ;
#29160=CARTESIAN_POINT('Ctrl Pts',(-18.7082920013057,26.8834122227005,124.393076157916)) ;
#29161=CARTESIAN_POINT('Ctrl Pts',(-18.3335903392706,27.0733871836819,124.467951336687)) ;
#29162=CARTESIAN_POINT('Ctrl Pts',(-18.5487170321478,26.893398103319,124.256715629541)) ;
#29163=CARTESIAN_POINT('Ctrl Pts',(-18.1673965821684,27.0833219067751,124.266543402248)) ;
#29164=CARTESIAN_POINT('Ctrl Pts',(-18.4157637799795,26.9033328264122,124.095588174979)) ;
#29165=CARTESIAN_POINT('Ctrl Pts',(-18.0373591121067,27.0933797470863,124.03648134582)) ;
#29166=CARTESIAN_POINT('Ctrl Pts',(-18.3117355760186,26.9133906667234,123.911537419721)) ;
#29167=CARTESIAN_POINT('Ctrl Pts',(-17.9509061764655,27.1032002344828,123.793285094069)) ;
#29168=CARTESIAN_POINT('Ctrl Pts',(-18.242575359153,26.9232111541199,123.716980330585)) ;
#29169=CARTESIAN_POINT('Ctrl Pts',(-17.9065238901742,27.1132606358279,123.532692664086)) ;
#29170=CARTESIAN_POINT('Ctrl Pts',(-18.2070714726686,26.9332715554651,123.508505957209)) ;
#29171=CARTESIAN_POINT('Ctrl Pts',(-17.9083966530251,27.1231916013808,123.271694164607)) ;
#29172=CARTESIAN_POINT('Ctrl Pts',(-18.2085717099821,26.943202521018,123.299707472759)) ;
#29173=CARTESIAN_POINT('Ctrl Pts',(-17.9550143490479,27.1331304637173,123.014732779571)) ;
#29174=CARTESIAN_POINT('Ctrl Pts',(-18.2458677394245,26.9531413833544,123.094139009809)) ;
#29175=CARTESIAN_POINT('Ctrl Pts',(-18.0458227293772,27.1431161946435,122.768499870868)) ;
#29176=CARTESIAN_POINT('Ctrl Pts',(-18.3185162096812,26.9631271142806,122.897153472277)) ;
#29177=CARTESIAN_POINT('Ctrl Pts',(-18.1787338062467,27.1531405800709,122.54108010085)) ;
#29178=CARTESIAN_POINT('Ctrl Pts',(-18.4248467768607,26.9731514997081,122.715218646662)) ;
#29179=CARTESIAN_POINT('Ctrl Pts',(-18.3467863406668,27.1630438644242,122.342321573022)) ;
#29180=CARTESIAN_POINT('Ctrl Pts',(-18.5592899783311,26.9830547840613,122.556213402555)) ;
#29181=CARTESIAN_POINT('Ctrl Pts',(-18.5499675318017,27.1731038690022,122.173235543931)) ;
#29182=CARTESIAN_POINT('Ctrl Pts',(-18.7218362738242,26.9931147886393,122.420945971278)) ;
#29183=CARTESIAN_POINT('Ctrl Pts',(-18.7744378365037,27.1829471380713,122.044638016558)) ;
#29184=CARTESIAN_POINT('Ctrl Pts',(-18.9014128616889,27.0029580577084,122.318069943643)) ;
#29185=CARTESIAN_POINT('Ctrl Pts',(-19.0212070083882,27.192937703679,121.955103241881)) ;
#29186=CARTESIAN_POINT('Ctrl Pts',(-19.0988286849585,27.0129486233161,122.246443874494)) ;
#29187=CARTESIAN_POINT('Ctrl Pts',(-19.2782077784814,27.2028658354578,121.910092465526)) ;
#29188=CARTESIAN_POINT('Ctrl Pts',(-19.3044292293712,27.022876755095,122.210437108631)) ;
#29189=CARTESIAN_POINT('Ctrl Pts',(-19.5406906769413,27.2128537225387,121.909933250644)) ;
#29190=CARTESIAN_POINT('Ctrl Pts',(-19.5144154029953,27.0328646421759,122.210311478194)) ;
#29191=CARTESIAN_POINT('Ctrl Pts',(-19.8003580009036,27.2228896721074,121.956008127035)) ;
#29192=CARTESIAN_POINT('Ctrl Pts',(-19.7221490136593,27.0429005917445,122.247173180015)) ;
#29193=CARTESIAN_POINT('Ctrl Pts',(-20.0437890490973,27.2327445584862,122.044444124203)) ;
#29194=CARTESIAN_POINT('Ctrl Pts',(-19.9168925651677,27.0527554781234,122.317923364294)) ;
#29195=CARTESIAN_POINT('Ctrl Pts',(-20.2715790260407,27.2427439728341,122.175359156114)) ;
#29196=CARTESIAN_POINT('Ctrl Pts',(-20.0991236143385,27.0627548924712,122.422656796826)) ;
#29197=CARTESIAN_POINT('Ctrl Pts',(-20.47132188163,27.2526391380246,122.341923187153)) ;
#29198=CARTESIAN_POINT('Ctrl Pts',(-20.2589164031302,27.0726500576617,122.555908896478)) ;
#29199=CARTESIAN_POINT('Ctrl Pts',(-20.6418377253297,27.2626994567166,122.543912452748)) ;
#29200=CARTESIAN_POINT('Ctrl Pts',(-20.3953279507184,27.0827103763537,122.717501514616)) ;
#29201=CARTESIAN_POINT('Ctrl Pts',(-20.7720769168341,27.2725495884926,122.767639569015)) ;
#29202=CARTESIAN_POINT('Ctrl Pts',(-20.4995174924838,27.0925605081298,122.89648329143)) ;
#29203=CARTESIAN_POINT('Ctrl Pts',(-20.8637005068752,27.2825801589429,123.014783157539)) ;
#29204=CARTESIAN_POINT('Ctrl Pts',(-20.5728149832003,27.10259107858,123.094198725936)) ;
#29205=CARTESIAN_POINT('Ctrl Pts',(-20.9103706252309,27.2925943096157,123.273787983254)) ;
#29206=CARTESIAN_POINT('Ctrl Pts',(-20.6101494956889,27.1126052292528,123.301402858841)) ;
#29207=CARTESIAN_POINT('Ctrl Pts',(-20.911768495837,27.3024872431611,123.533764947733)) ;
#29208=CARTESIAN_POINT('Ctrl Pts',(-20.6112662665047,27.1224981627982,123.509383800559)) ;
#29209=CARTESIAN_POINT('Ctrl Pts',(-20.8678776029836,27.3124767571514,123.792558185261)) ;
#29210=CARTESIAN_POINT('Ctrl Pts',(-20.5761521325388,27.1324876767885,123.716417986733)) ;
#29211=CARTESIAN_POINT('Ctrl Pts',(-20.7801754400193,27.3224305278038,124.03903194835)) ;
#29212=CARTESIAN_POINT('Ctrl Pts',(-20.505989170069,27.1424414474409,123.913596190151)) ;
#29213=CARTESIAN_POINT('Ctrl Pts',(-20.6496157399914,27.3324782964644,124.26850963764)) ;
#29214=CARTESIAN_POINT('Ctrl Pts',(-20.4015400481253,27.1524892161015,124.097177744708)) ;
#29215=CARTESIAN_POINT('Ctrl Pts',(-20.4848531000536,27.3423200229042,124.467895083723)) ;
#29216=CARTESIAN_POINT('Ctrl Pts',(-20.2697294497831,27.1623309425413,124.256684466489)) ;
#29217=CARTESIAN_POINT('Ctrl Pts',(-20.2855162962699,27.3523055397269,124.638488743857)) ;
#29218=CARTESIAN_POINT('Ctrl Pts',(-20.1102593118314,27.172316459364,124.393158279408)) ;
#29219=CARTESIAN_POINT('Ctrl Pts',(-20.0606131128351,27.3622448714225,124.771385186807)) ;
#29220=CARTESIAN_POINT('Ctrl Pts',(-19.9303364915707,27.1822557910596,124.499474112979)) ;
#29221=CARTESIAN_POINT('Ctrl Pts',(-19.8136159800649,27.37228464112,124.864066326302)) ;
#29222=CARTESIAN_POINT('Ctrl Pts',(-19.7327382216027,27.1922955607571,124.57361785765)) ;
#29223=CARTESIAN_POINT('Ctrl Pts',(-19.5581817302825,27.3821728023688,124.911855032732)) ;
#29224=CARTESIAN_POINT('Ctrl Pts',(-19.5283913156951,27.2021837220059,124.61184744574)) ;
#29225=CARTESIAN_POINT('Ctrl Pts',(-19.2956955404914,27.3921623568712,124.915085978907)) ;
#29226=CARTESIAN_POINT('Ctrl Pts',(-19.318402520903,27.2121732765083,124.614431045079)) ;
#29227=CARTESIAN_POINT('Ctrl Pts',(-19.0374725439821,27.4021207713948,124.872626590807)) ;
#29228=CARTESIAN_POINT('Ctrl Pts',(-19.1118246609645,27.222131691032,124.580462405806)) ;
#29229=CARTESIAN_POINT('Ctrl Pts',(-18.7917647458714,27.4120206842242,124.787079499337)) ;
#29230=CARTESIAN_POINT('Ctrl Pts',(-18.9152594335383,27.2320316038613,124.51202396635)) ;
#29231=CARTESIAN_POINT('Ctrl Pts',(-18.5613480077617,27.4220673838741,124.658240132733)) ;
#29232=CARTESIAN_POINT('Ctrl Pts',(-18.7309264191264,27.2420783035112,124.40895145111)) ;
#29233=CARTESIAN_POINT('Ctrl Pts',(-18.3596364546277,27.4319672441797,124.493876043428)) ;
#29234=CARTESIAN_POINT('Ctrl Pts',(-18.5695583841052,27.2519781638168,124.277459828361)) ;
#29235=CARTESIAN_POINT('Ctrl Pts',(-18.186909253097,27.4420186483852,124.294086730336)) ;
#29236=CARTESIAN_POINT('Ctrl Pts',(-18.4313772630263,27.2620295680223,124.117627563925)) ;
#29237=CARTESIAN_POINT('Ctrl Pts',(-18.0536713291326,27.4518996853063,124.071168267617)) ;
#29238=CARTESIAN_POINT('Ctrl Pts',(-18.3247881999234,27.2719106049434,123.939292985394)) ;
#29239=CARTESIAN_POINT('Ctrl Pts',(-17.9597465513536,27.4618995174838,123.825788262627)) ;
#29240=CARTESIAN_POINT('Ctrl Pts',(-18.24964927092,27.2819104371209,123.742988761484)) ;
#29241=CARTESIAN_POINT('Ctrl Pts',(-17.9100347106082,27.4718175204687,123.56989145949)) ;
#29242=CARTESIAN_POINT('Ctrl Pts',(-18.2098807623671,27.2918284401058,123.538271752722)) ;
#29243=CARTESIAN_POINT('Ctrl Pts',(-17.9055372820663,27.4818688263432,123.305836914717)) ;
#29244=CARTESIAN_POINT('Ctrl Pts',(-18.2062837024167,27.3018797459804,123.327027911082)) ;
#29245=CARTESIAN_POINT('Ctrl Pts',(-17.9459117765369,27.4917386497348,123.049572996332)) ;
#29246=CARTESIAN_POINT('Ctrl Pts',(-18.2385839520129,27.3117495693719,123.122017805772)) ;
#29247=CARTESIAN_POINT('Ctrl Pts',(-18.0318915985893,27.5018128157851,122.799249602971)) ;
#29248=CARTESIAN_POINT('Ctrl Pts',(-18.3073686920026,27.3218237354222,122.921759028966)) ;
#29249=CARTESIAN_POINT('Ctrl Pts',(-18.1565773494833,27.5116328999267,122.573239483822)) ;
#29250=CARTESIAN_POINT('Ctrl Pts',(-18.4071173341134,27.3316438195639,122.740952378761)) ;
#29251=CARTESIAN_POINT('Ctrl Pts',(-18.3226042808018,27.5217116266626,122.366962086733)) ;
#29252=CARTESIAN_POINT('Ctrl Pts',(-18.5399396427468,27.3417225462997,122.575930590935)) ;
#29253=CARTESIAN_POINT('Ctrl Pts',(-18.5174703780383,27.5315632073121,122.196424414338)) ;
#29254=CARTESIAN_POINT('Ctrl Pts',(-18.6958321561076,27.3515741269492,122.439501639971)) ;
#29255=CARTESIAN_POINT('Ctrl Pts',(-18.7437532834736,27.5416363356105,122.05915550415)) ;
#29256=CARTESIAN_POINT('Ctrl Pts',(-18.8768590906674,27.3616472552476,122.329686841586)) ;
#29257=CARTESIAN_POINT('Ctrl Pts',(-18.9848658829686,27.5514788135019,121.965469396346)) ;
#29258=CARTESIAN_POINT('Ctrl Pts',(-19.0697483336544,27.3714897331391,122.25473893346)) ;
#29259=CARTESIAN_POINT('Ctrl Pts',(-19.2419340497948,27.5614594201,121.913511275121)) ;
#29260=CARTESIAN_POINT('Ctrl Pts',(-19.2754027022882,27.3814703397371,122.213172868281)) ;
#29261=CARTESIAN_POINT('Ctrl Pts',(-19.505118136635,27.5714771291188,121.907449255122)) ;
#29262=CARTESIAN_POINT('Ctrl Pts',(-19.4859499875362,27.3914880487559,122.208323766678)) ;
#29263=CARTESIAN_POINT('Ctrl Pts',(-19.7620374996728,27.5813633081562,121.946159440311)) ;
#29264=CARTESIAN_POINT('Ctrl Pts',(-19.6914845708838,27.4013742277934,122.239292171034)) ;
#29265=CARTESIAN_POINT('Ctrl Pts',(-20.0125674013974,27.5914209207286,122.030295059284)) ;
#29266=CARTESIAN_POINT('Ctrl Pts',(-19.8919086080025,27.4114318403657,122.306601108605)) ;
#29267=CARTESIAN_POINT('Ctrl Pts',(-20.2405477178494,27.6012973141007,122.154372035112)) ;
#29268=CARTESIAN_POINT('Ctrl Pts',(-20.0742918644194,27.4213082337378,122.405862575282)) ;
#29269=CARTESIAN_POINT('Ctrl Pts',(-20.4463485472987,27.6112923422511,122.317564461287)) ;
#29270=CARTESIAN_POINT('Ctrl Pts',(-20.2389322836839,27.4313032618883,122.53641659574)) ;
#29271=CARTESIAN_POINT('Ctrl Pts',(-20.6208115759906,27.6213130890971,122.51483046535)) ;
#29272=CARTESIAN_POINT('Ctrl Pts',(-20.3785024861279,27.4413240087343,122.694229642115)) ;
#29273=CARTESIAN_POINT('Ctrl Pts',(-20.7569960330264,27.6312151577635,122.736562250952)) ;
#29274=CARTESIAN_POINT('Ctrl Pts',(-20.4874494348297,27.4512260774006,122.871614548114)) ;
#29275=CARTESIAN_POINT('Ctrl Pts',(-20.8538296011518,27.6412058975832,122.980600241119)) ;
#29276=CARTESIAN_POINT('Ctrl Pts',(-20.5649160765477,27.4612168172203,123.066844821881)) ;
#29277=CARTESIAN_POINT('Ctrl Pts',(-20.9064812123952,27.6511690937935,123.237061229662)) ;
#29278=CARTESIAN_POINT('Ctrl Pts',(-20.6070370952218,27.4711800134306,123.272013299712)) ;
#29279=CARTESIAN_POINT('Ctrl Pts',(-20.9144047817725,27.6610732780936,123.497236530681)) ;
#29280=CARTESIAN_POINT('Ctrl Pts',(-20.6133758900281,27.4810841977308,123.480152789572)) ;
#29281=CARTESIAN_POINT('Ctrl Pts',(-20.8762301626549,27.6711337384845,123.758811110914)) ;
#29282=CARTESIAN_POINT('Ctrl Pts',(-20.5828360598664,27.4911446581216,123.689412720083)) ;
#29283=CARTESIAN_POINT('Ctrl Pts',(-20.7953249519176,27.6809742843553,124.004465402187)) ;
#29284=CARTESIAN_POINT('Ctrl Pts',(-20.5181122497151,27.5009852039924,123.88593503245)) ;
#29285=CARTESIAN_POINT('Ctrl Pts',(-20.6705674371017,27.6910365050671,124.237576347375)) ;
#29286=CARTESIAN_POINT('Ctrl Pts',(-20.4183061644665,27.5110474247042,124.072424084696)) ;
#29287=CARTESIAN_POINT('Ctrl Pts',(-20.5096693378974,27.7009336480836,124.441939302609)) ;
#29288=CARTESIAN_POINT('Ctrl Pts',(-20.2895881841943,27.5209445677207,124.235913821433)) ;
#29289=CARTESIAN_POINT('Ctrl Pts',(-20.315658373556,27.7108648245008,124.61649018712)) ;
#29290=CARTESIAN_POINT('Ctrl Pts',(-20.1343799929666,27.5308757441379,124.375554311888)) ;
#29291=CARTESIAN_POINT('Ctrl Pts',(-20.091657303987,27.7209070382794,124.756002912722)) ;
#29292=CARTESIAN_POINT('Ctrl Pts',(-19.9551790760134,27.5409179579165,124.487164709501)) ;
#29293=CARTESIAN_POINT('Ctrl Pts',(-19.8506842942627,27.7307935784821,124.85316185408)) ;
#29294=CARTESIAN_POINT('Ctrl Pts',(-19.7624015506141,27.5508044981193,124.564891723896)) ;
#29295=CARTESIAN_POINT('Ctrl Pts',(-19.5938710456304,27.7407871730876,124.907993194414)) ;
#29296=CARTESIAN_POINT('Ctrl Pts',(-19.5569511707671,27.5607980927247,124.608757063164)) ;
#29297=CARTESIAN_POINT('Ctrl Pts',(-19.3327071093546,27.7507310482451,124.917315275339)) ;
#29298=CARTESIAN_POINT('Ctrl Pts',(-19.3480205279212,27.5707419678822,124.616215008341)) ;
#29299=CARTESIAN_POINT('Ctrl Pts',(-19.0734423500519,27.7606915843599,124.881432829596)) ;
#29300=CARTESIAN_POINT('Ctrl Pts',(-19.1406090425669,27.5807025039971,124.587509484983)) ;
#29301=CARTESIAN_POINT('Ctrl Pts',(-18.823353749831,27.7706881876827,124.800925220385)) ;
#29302=CARTESIAN_POINT('Ctrl Pts',(-18.9405381483672,27.5906991073198,124.523103835156)) ;
#29303=CARTESIAN_POINT('Ctrl Pts',(-18.5903995182117,27.7807212706372,124.677453935382)) ;
#29304=CARTESIAN_POINT('Ctrl Pts',(-18.7541745110723,27.6007321902743,124.424327045669)) ;
#29305=CARTESIAN_POINT('Ctrl Pts',(-18.3859904696139,27.7905724393387,124.518604840361)) ;
#29306=CARTESIAN_POINT('Ctrl Pts',(-18.5906478871506,27.6105833589758,124.297248765221)) ;
#29307=CARTESIAN_POINT('Ctrl Pts',(-18.2097360022858,27.8005349300376,124.325031213336)) ;
#29308=CARTESIAN_POINT('Ctrl Pts',(-18.4496441165959,27.6205458496747,124.142390542805)) ;
#29309=CARTESIAN_POINT('Ctrl Pts',(-18.0691061956658,27.8105633584554,124.102135115778)) ;
#29310=CARTESIAN_POINT('Ctrl Pts',(-18.3371397875157,27.6305742780925,123.964073876923)) ;
#29311=CARTESIAN_POINT('Ctrl Pts',(-17.9704213296521,27.8204737258199,123.861134793012)) ;
#29312=CARTESIAN_POINT('Ctrl Pts',(-18.2581916587335,27.640484645457,123.771274472976)) ;
#29313=CARTESIAN_POINT('Ctrl Pts',(-17.9142719852206,27.830408593435,123.606158130962)) ;
#29314=CARTESIAN_POINT('Ctrl Pts',(-18.2132716018524,27.6504195130721,123.567293812213)) ;
#29315=CARTESIAN_POINT('Ctrl Pts',(-17.9033759753097,27.840449735414,123.342521266579)) ;
#29316=CARTESIAN_POINT('Ctrl Pts',(-18.2045541379343,27.6604606550512,123.356384198053)) ;
#29317=CARTESIAN_POINT('Ctrl Pts',(-17.9377060396121,27.8503368716172,123.084960416994)) ;
#29318=CARTESIAN_POINT('Ctrl Pts',(-18.2320173908359,27.6703477912543,123.150336250561)) ;
#29319=CARTESIAN_POINT('Ctrl Pts',(-18.0166431581778,27.8603291540206,122.834538577221)) ;
#29320=CARTESIAN_POINT('Ctrl Pts',(-18.2951662729315,27.6803400736577,122.94999869318)) ;
#29321=CARTESIAN_POINT('Ctrl Pts',(-18.137412126526,27.8702776819858,122.602650848213)) ;
#29322=CARTESIAN_POINT('Ctrl Pts',(-18.3917805539364,27.6902886016229,122.764488533233)) ;
#29323=CARTESIAN_POINT('Ctrl Pts',(-18.2961056898845,27.8802144131479,122.395304507949)) ;
#29324=CARTESIAN_POINT('Ctrl Pts',(-18.5187344032728,27.7002253327851,122.598611336762)) ;
#29325=CARTESIAN_POINT('Ctrl Pts',(-18.4891076721817,27.8901976240079,122.217558370946)) ;
#29326=CARTESIAN_POINT('Ctrl Pts',(-18.6731351964962,27.710208543645,122.456413869143)) ;
#29327=CARTESIAN_POINT('Ctrl Pts',(-18.7115707177152,27.9002407231578,122.075605016214)) ;
#29328=CARTESIAN_POINT('Ctrl Pts',(-18.8511053106445,27.7202516427949,122.342850400546)) ;
#29329=CARTESIAN_POINT('Ctrl Pts',(-18.9499871891245,27.9100716874327,121.976015433695)) ;
#29330=CARTESIAN_POINT('Ctrl Pts',(-19.041837051544,27.7300826070698,122.263178278936)) ;
#29331=CARTESIAN_POINT('Ctrl Pts',(-19.2081615249894,27.9201445398186,121.917767583989)) ;
#29332=CARTESIAN_POINT('Ctrl Pts',(-19.2483766156714,27.7401554594558,122.216578932533)) ;
#29333=CARTESIAN_POINT('Ctrl Pts',(-19.4671216625185,27.9300086675304,121.905533740892)) ;
#29334=CARTESIAN_POINT('Ctrl Pts',(-19.4555437647533,27.7500195871675,122.206790898622)) ;
#29335=CARTESIAN_POINT('Ctrl Pts',(-19.7284352632182,27.9400308696653,121.938326646805)) ;
#29336=CARTESIAN_POINT('Ctrl Pts',(-19.6645948238701,27.7600417893024,122.233024081806)) ;
#29337=CARTESIAN_POINT('Ctrl Pts',(-19.980050984628,27.9500580626337,122.016636385366)) ;
#29338=CARTESIAN_POINT('Ctrl Pts',(-19.8658877542819,27.7700689822708,122.295670925777)) ;
#29339=CARTESIAN_POINT('Ctrl Pts',(-20.2103950643466,27.9599136566007,122.135000592785)) ;
#29340=CARTESIAN_POINT('Ctrl Pts',(-20.0501626545512,27.7799245762378,122.39036086436)) ;
#29341=CARTESIAN_POINT('Ctrl Pts',(-20.4193072748828,27.969870828466,122.29257198083)) ;
#29342=CARTESIAN_POINT('Ctrl Pts',(-20.2172929209471,27.7898817481031,122.5164167495)) ;
#29343=CARTESIAN_POINT('Ctrl Pts',(-20.5987996284151,27.9799096724644,122.485885053549)) ;
#29344=CARTESIAN_POINT('Ctrl Pts',(-20.3608877406853,27.7999205921015,122.67106648784)) ;
#29345=CARTESIAN_POINT('Ctrl Pts',(-20.7400613604965,27.98978369634,122.703583668428)) ;
#29346=CARTESIAN_POINT('Ctrl Pts',(-20.4738977561458,27.8097946159771,122.845224005242)) ;
#29347=CARTESIAN_POINT('Ctrl Pts',(-20.8433506853364,27.9998535223304,122.947177423952)) ;
#29348=CARTESIAN_POINT('Ctrl Pts',(-20.5565304991962,27.8198644419675,123.040098768756)) ;
#29349=CARTESIAN_POINT('Ctrl Pts',(-20.9015266940339,28.0096867662276,123.198973980949)) ;
#29350=CARTESIAN_POINT('Ctrl Pts',(-20.6030723456922,27.8296976858648,123.241534723945)) ;
#29351=CARTESIAN_POINT('Ctrl Pts',(-20.9161142994382,28.0197171940007,123.462150342134)) ;
#29352=CARTESIAN_POINT('Ctrl Pts',(-20.6147438907103,27.8397281136378,123.452075801618)) ;
#29353=CARTESIAN_POINT('Ctrl Pts',(-20.8840166201033,28.0297488107458,123.72382387547)) ;
#29354=CARTESIAN_POINT('Ctrl Pts',(-20.5890670287782,27.8497597303829,123.661414851897)) ;
#29355=CARTESIAN_POINT('Ctrl Pts',(-20.80904662986,28.0395784877265,123.971001465148)) ;
#29356=CARTESIAN_POINT('Ctrl Pts',(-20.5290926826595,27.8595894073637,123.859156362875)) ;
#29357=CARTESIAN_POINT('Ctrl Pts',(-20.6910868706554,28.0495680045665,124.205529304447)) ;
#29358=CARTESIAN_POINT('Ctrl Pts',(-20.4347263402333,27.8695789242036,124.046779212421)) ;
#29359=CARTESIAN_POINT('Ctrl Pts',(-20.5328182779669,28.0596116167062,124.416742316167)) ;
#29360=CARTESIAN_POINT('Ctrl Pts',(-20.308112543254,27.8796225363434,124.215750577102)) ;
#29361=CARTESIAN_POINT('Ctrl Pts',(-20.3448814894554,28.0694342230415,124.593693576125)) ;
#29362=CARTESIAN_POINT('Ctrl Pts',(-20.1577648989237,27.8894451426787,124.357312023611)) ;
#29363=CARTESIAN_POINT('Ctrl Pts',(-20.124678185504,28.0794724529408,124.73892784558)) ;
#29364=CARTESIAN_POINT('Ctrl Pts',(-19.9816030855766,27.8994833725779,124.473500876513)) ;
#29365=CARTESIAN_POINT('Ctrl Pts',(-19.8829899980489,28.0894834877327,124.842887131756)) ;
#29366=CARTESIAN_POINT('Ctrl Pts',(-19.7882531778609,27.9094944073698,124.556669703237)) ;
#29367=CARTESIAN_POINT('Ctrl Pts',(-19.6299384968335,28.0993812186998,124.903017471924)) ;
#29368=CARTESIAN_POINT('Ctrl Pts',(-19.5858129211223,27.919392138337,124.60477541441)) ;
#29369=CARTESIAN_POINT('Ctrl Pts',(-19.3678981582499,28.1093708465503,124.918781274721)) ;
#29370=CARTESIAN_POINT('Ctrl Pts',(-19.3761808908369,27.9293817661874,124.617388123224)) ;
#29371=CARTESIAN_POINT('Ctrl Pts',(-19.1079954571358,28.1193266369963,124.888817431813)) ;
#29372=CARTESIAN_POINT('Ctrl Pts',(-19.1682588492881,27.9393375566334,124.593418735249)) ;
#29373=CARTESIAN_POINT('Ctrl Pts',(-18.8578037171305,28.1292540355584,124.814868421456)) ;
#29374=CARTESIAN_POINT('Ctrl Pts',(-18.968105356819,27.9492649551955,124.534261321663)) ;
#29375=CARTESIAN_POINT('Ctrl Pts',(-18.6219935808609,28.1392796306682,124.697390886151)) ;
#29376=CARTESIAN_POINT('Ctrl Pts',(-18.7794564590463,27.9592905503054,124.440280839266)) ;
#29377=CARTESIAN_POINT('Ctrl Pts',(-18.413012495007,28.1491654813378,124.543058534145)) ;
#29378=CARTESIAN_POINT('Ctrl Pts',(-18.612271014501,27.9691764009749,124.316816723086)) ;
#29379=CARTESIAN_POINT('Ctrl Pts',(-18.2316780606301,28.159154661182,124.353241304876)) ;
#29380=CARTESIAN_POINT('Ctrl Pts',(-18.4672022077259,27.9791655808191,124.164964317004)) ;
#29381=CARTESIAN_POINT('Ctrl Pts',(-18.085762555499,28.1691958482856,124.133385523761)) ;
#29382=CARTESIAN_POINT('Ctrl Pts',(-18.3504682851199,27.9892067679227,123.989080612378)) ;
#29383=CARTESIAN_POINT('Ctrl Pts',(-17.9820414176768,28.1790284917615,123.896729581303)) ;
#29384=CARTESIAN_POINT('Ctrl Pts',(-18.2674899943736,27.9990394113987,123.799757297218)) ;
#29385=CARTESIAN_POINT('Ctrl Pts',(-17.9192545217861,28.189022441471,123.641716424028)) ;
#29386=CARTESIAN_POINT('Ctrl Pts',(-18.2172586037933,28.0090333611081,123.595747332759)) ;
#29387=CARTESIAN_POINT('Ctrl Pts',(-17.9021928664862,28.1990515642475,123.378711840277)) ;
#29388=CARTESIAN_POINT('Ctrl Pts',(-18.2036074112526,28.0190624838847,123.385343770105)) ;
#29389=CARTESIAN_POINT('Ctrl Pts',(-17.9302039422221,28.2089276951662,123.120680343544)) ;
#29390=CARTESIAN_POINT('Ctrl Pts',(-18.2260142937599,28.0289386148033,123.178918899042)) ;
#29391=CARTESIAN_POINT('Ctrl Pts',(-18.0031776926144,28.2189257301832,122.86831261201)) ;
#29392=CARTESIAN_POINT('Ctrl Pts',(-18.2843913725109,28.0389366498204,122.977024252251)) ;
#29393=CARTESIAN_POINT('Ctrl Pts',(-18.117736776842,28.2288396599419,122.634287677194)) ;
#29394=CARTESIAN_POINT('Ctrl Pts',(-18.376036681339,28.0488505795791,122.789803759949)) ;
#29395=CARTESIAN_POINT('Ctrl Pts',(-18.2731150794606,28.2388828476797,122.420974122389)) ;
#29396=CARTESIAN_POINT('Ctrl Pts',(-18.5003377353294,28.0588937673169,122.619151688384)) ;
#29397=CARTESIAN_POINT('Ctrl Pts',(-18.4604722427515,28.2487826898201,122.24045743561)) ;
#29398=CARTESIAN_POINT('Ctrl Pts',(-18.6502217887544,28.0687936094572,122.474737169911)) ;
#29399=CARTESIAN_POINT('Ctrl Pts',(-18.6779981948743,28.2587739566281,122.093415286291)) ;
#29400=CARTESIAN_POINT('Ctrl Pts',(-18.8242413102653,28.0787848762652,122.357101786154)) ;
#29401=CARTESIAN_POINT('Ctrl Pts',(-18.918918044841,28.2688060587601,121.986355077235)) ;
#29402=CARTESIAN_POINT('Ctrl Pts',(-19.0169763807828,28.0888169783972,122.271451769572)) ;
#29403=CARTESIAN_POINT('Ctrl Pts',(-19.1704626082505,28.2786729397148,121.923469734543)) ;
#29404=CARTESIAN_POINT('Ctrl Pts',(-19.2182110752363,28.098683859352,122.221141611949)) ;
#29405=CARTESIAN_POINT('Ctrl Pts',(-19.432345213223,28.288664731003,121.904359612356)) ;
#29406=CARTESIAN_POINT('Ctrl Pts',(-19.4277169183523,28.1086756506401,122.20585140049)) ;
#29407=CARTESIAN_POINT('Ctrl Pts',(-19.694564039776,28.2986968469145,121.93162572317)) ;
#29408=CARTESIAN_POINT('Ctrl Pts',(-19.6374921940647,28.1187077665516,122.227662228157)) ;
#29409=CARTESIAN_POINT('Ctrl Pts',(-19.943995852301,28.3085631637145,122.002434913296)) ;
#29410=CARTESIAN_POINT('Ctrl Pts',(-19.8370378243453,28.1285740833517,122.284307435928)) ;
#29411=CARTESIAN_POINT('Ctrl Pts',(-20.1803573809643,28.3185506451881,122.116461326157)) ;
#29412=CARTESIAN_POINT('Ctrl Pts',(-20.0261278945652,28.1385615648253,122.375526584252)) ;
#29413=CARTESIAN_POINT('Ctrl Pts',(-20.3925607131235,28.328495569567,122.269070719418)) ;
#29414=CARTESIAN_POINT('Ctrl Pts',(-20.1958916697619,28.1485064892042,122.497612235911)) ;
#29415=CARTESIAN_POINT('Ctrl Pts',(-20.5767268496923,28.3385404554777,122.458146387094)) ;
#29416=CARTESIAN_POINT('Ctrl Pts',(-20.343226130455,28.1585513751149,122.648871279974)) ;
#29417=CARTESIAN_POINT('Ctrl Pts',(-20.7227745276264,28.3484025591903,122.672264744843)) ;
#29418=CARTESIAN_POINT('Ctrl Pts',(-20.4600658712918,28.1684134788274,122.820164463442)) ;
#29419=CARTESIAN_POINT('Ctrl Pts',(-20.8312927348308,28.3583941230148,122.911337082898)) ;
#29420=CARTESIAN_POINT('Ctrl Pts',(-20.5468824144814,28.1784050426519,123.011421352625)) ;
#29421=CARTESIAN_POINT('Ctrl Pts',(-20.8961668071842,28.3683269310777,123.164169825498)) ;
#29422=CARTESIAN_POINT('Ctrl Pts',(-20.5987837570556,28.1883378507148,123.213686829248)) ;
#29423=CARTESIAN_POINT('Ctrl Pts',(-20.9168053566465,28.378264033314,123.424505796562)) ;
#29424=CARTESIAN_POINT('Ctrl Pts',(-20.615296810215,28.1982749529511,123.421955292323)) ;
#29425=CARTESIAN_POINT('Ctrl Pts',(-20.8912939664117,28.3883164795844,123.687418366482)) ;
#29426=CARTESIAN_POINT('Ctrl Pts',(-20.5948899052389,28.2083273992215,123.632285549448)) ;
#29427=CARTESIAN_POINT('Ctrl Pts',(-20.8223185569164,28.398162595166,123.936824298385)) ;
#29428=CARTESIAN_POINT('Ctrl Pts',(-20.5397117877283,28.2181735148031,123.831810673226)) ;
#29429=CARTESIAN_POINT('Ctrl Pts',(-20.709193147176,28.4082106148809,124.175395051952)) ;
#29430=CARTESIAN_POINT('Ctrl Pts',(-20.4492134944853,28.228221534518,124.022668227718)) ;
#29431=CARTESIAN_POINT('Ctrl Pts',(-20.5576594223878,28.4181525665098,124.388243230741)) ;
#29432=CARTESIAN_POINT('Ctrl Pts',(-20.3279884025434,28.238163486147,124.192947972631)) ;
#29433=CARTESIAN_POINT('Ctrl Pts',(-20.3719920554206,28.4280913475089,124.571940487482)) ;
#29434=CARTESIAN_POINT('Ctrl Pts',(-20.1794561524199,28.248102267146,124.339907313728)) ;
#29435=CARTESIAN_POINT('Ctrl Pts',(-20.155266255181,28.438117396235,124.721739105602)) ;
#29436=CARTESIAN_POINT('Ctrl Pts',(-20.0060768524774,28.2581283158721,124.45974803094)) ;
#29437=CARTESIAN_POINT('Ctrl Pts',(-19.9192398618305,28.4480042566432,124.830426395165)) ;
#29438=CARTESIAN_POINT('Ctrl Pts',(-19.8172566995611,28.2680151762803,124.546699853667)) ;
#29439=CARTESIAN_POINT('Ctrl Pts',(-19.6643603212813,28.458035531775,124.897541005947)) ;
#29440=CARTESIAN_POINT('Ctrl Pts',(-19.6133539336829,28.2780464514121,124.600393764835)) ;
#29441=CARTESIAN_POINT('Ctrl Pts',(-19.405507635062,28.4679185090754,124.919330220156)) ;
#29442=CARTESIAN_POINT('Ctrl Pts',(-19.4062711317406,28.2879294287125,124.617827171934)) ;
#29443=CARTESIAN_POINT('Ctrl Pts',(-19.14236864725,28.4779753624826,124.895445755536)) ;
#29444=CARTESIAN_POINT('Ctrl Pts',(-19.1957631355811,28.2979862821197,124.598722613177)) ;
#29445=CARTESIAN_POINT('Ctrl Pts',(-18.8081529113529,28.4911436035585,124.80533200887)) ;
#29446=CARTESIAN_POINT('Ctrl Pts',(-18.9283732060215,28.3111545231956,124.526630734819)) ;
#29447=CARTESIAN_POINT('Ctrl Pts',(-18.4999549682012,28.504544632785,124.627092881207)) ;
#29448=CARTESIAN_POINT('Ctrl Pts',(-18.681798248427,28.3245555524222,124.384021484789)) ;
#29449=CARTESIAN_POINT('Ctrl Pts',(-18.2548346129752,28.5177575495159,124.381018273064)) ;
#29450=CARTESIAN_POINT('Ctrl Pts',(-18.4857344323844,28.337768469153,124.187192189279)) ;
#29451=CARTESIAN_POINT('Ctrl Pts',(-18.1049098192041,28.5276859439691,124.167554176501)) ;
#29452=CARTESIAN_POINT('Ctrl Pts',(-18.3657857952432,28.3476968636062,124.016416466804)) ;
#29453=CARTESIAN_POINT('Ctrl Pts',(-17.9935167509591,28.5376674440972,123.930036177092)) ;
#29454=CARTESIAN_POINT('Ctrl Pts',(-18.2766712098695,28.3576783637344,123.826404555807)) ;
#29455=CARTESIAN_POINT('Ctrl Pts',(-17.9250194853092,28.5477079873673,123.675241990111)) ;
#29456=CARTESIAN_POINT('Ctrl Pts',(-18.2218707823498,28.3677189070045,123.622569449493)) ;
#29457=CARTESIAN_POINT('Ctrl Pts',(-17.9019033242933,28.5575573191504,123.417442838969)) ;
#29458=CARTESIAN_POINT('Ctrl Pts',(-18.2033757289784,28.3775682387876,123.416330378134)) ;
#29459=CARTESIAN_POINT('Ctrl Pts',(-17.9235537436292,28.5675527236221,123.155670875178)) ;
#29460=CARTESIAN_POINT('Ctrl Pts',(-18.2206940100474,28.3875636432592,123.206912092977)) ;
#29461=CARTESIAN_POINT('Ctrl Pts',(-17.990923682755,28.5775690510707,122.901217359065)) ;
#29462=CARTESIAN_POINT('Ctrl Pts',(-18.2745872927144,28.3975799707078,123.003350782383)) ;
#29463=CARTESIAN_POINT('Ctrl Pts',(-18.1363563321866,28.5907927082372,122.585573838039)) ;
#29464=CARTESIAN_POINT('Ctrl Pts',(-18.3909334946143,28.4108036278744,122.750824793006)) ;
#29465=CARTESIAN_POINT('Ctrl Pts',(-18.361738888197,28.6040869996266,122.313564150216)) ;
#29466=CARTESIAN_POINT('Ctrl Pts',(-18.5712653371683,28.4240979192637,122.533196651324)) ;
#29467=CARTESIAN_POINT('Ctrl Pts',(-18.6465253994931,28.6173713505581,122.111531614028)) ;
#29468=CARTESIAN_POINT('Ctrl Pts',(-18.7990570818657,28.4373822701952,122.371600047551)) ;
#29469=CARTESIAN_POINT('Ctrl Pts',(-18.8832307222806,28.6273437316199,121.999158080089)) ;
#29470=CARTESIAN_POINT('Ctrl Pts',(-18.9884277554392,28.447354651257,122.281692950129)) ;
#29471=CARTESIAN_POINT('Ctrl Pts',(-19.1341788049863,28.6372521112455,121.929579826141)) ;
#29472=CARTESIAN_POINT('Ctrl Pts',(-19.1891837168037,28.4572630308826,122.22602983351)) ;
#29473=CARTESIAN_POINT('Ctrl Pts',(-19.3971551455222,28.6473061099936,121.904389073441)) ;
#29474=CARTESIAN_POINT('Ctrl Pts',(-19.3995659464143,28.4673170296307,122.205875390456)) ;
#29475=CARTESIAN_POINT('Ctrl Pts',(-19.6555567772795,28.6571683071099,121.924649710965)) ;
#29476=CARTESIAN_POINT('Ctrl Pts',(-19.6062837665613,28.477179226747,122.222079569028)) ;
#29477=CARTESIAN_POINT('Ctrl Pts',(-19.9952798306344,28.670515433484,122.011813758423)) ;
#29478=CARTESIAN_POINT('Ctrl Pts',(-19.8780825920856,28.4905263531211,122.291820399844)) ;
#29479=CARTESIAN_POINT('Ctrl Pts',(-20.3783371558031,28.6870523991254,122.227433848027)) ;
#29480=CARTESIAN_POINT('Ctrl Pts',(-20.1845001448543,28.5070633187626,122.464288220489)) ;
#29481=CARTESIAN_POINT('Ctrl Pts',(-20.6669572705968,28.7036870032994,122.562229846375)) ;
#29482=CARTESIAN_POINT('Ctrl Pts',(-20.4154369512327,28.5236979229365,122.73217404382)) ;
#29483=CARTESIAN_POINT('Ctrl Pts',(-20.818619503667,28.716976796542,122.876897221786)) ;
#29484=CARTESIAN_POINT('Ctrl Pts',(-20.536739963039,28.5369877161791,122.983864515057)) ;
#29485=CARTESIAN_POINT('Ctrl Pts',(-20.8898646071741,28.7269294278014,123.12852052043)) ;
#29486=CARTESIAN_POINT('Ctrl Pts',(-20.5937435077852,28.5469403474385,123.185172022197)) ;
#29487=CARTESIAN_POINT('Ctrl Pts',(-20.916646989976,28.7368813951061,123.388702342932)) ;
#29488=CARTESIAN_POINT('Ctrl Pts',(-20.6151704550531,28.5568923147432,123.393312774312)) ;
#29489=CARTESIAN_POINT('Ctrl Pts',(-20.891192739327,28.7502486535699,123.739016958567)) ;
#29490=CARTESIAN_POINT('Ctrl Pts',(-20.5948058393565,28.570259573207,123.673577519016)) ;
#29491=CARTESIAN_POINT('Ctrl Pts',(-20.7477418810432,28.7667654655191,124.154036877155)) ;
#29492=CARTESIAN_POINT('Ctrl Pts',(-20.4800520421779,28.5867763851562,124.005580886931)) ;
#29493=CARTESIAN_POINT('Ctrl Pts',(-20.4126932064644,28.7867913605254,124.567418944492)) ;
#29494=CARTESIAN_POINT('Ctrl Pts',(-20.2120144196254,28.6068022801626,124.336293127083)) ;
#29495=CARTESIAN_POINT('Ctrl Pts',(-19.9614615275447,28.8066020906556,124.838970603354)) ;
#29496=CARTESIAN_POINT('Ctrl Pts',(-19.8510300684342,28.6266130102927,124.553536623259)) ;
#29497=CARTESIAN_POINT('Ctrl Pts',(-19.4406750274565,28.8265793067854,124.942183198345)) ;
#29498=CARTESIAN_POINT('Ctrl Pts',(-19.4344011473137,28.6465902264226,124.636109825958)) ;
#29499=CARTESIAN_POINT('Ctrl Pts',(-18.9173848458449,28.8465061821807,124.860730356123)) ;
#29500=CARTESIAN_POINT('Ctrl Pts',(-19.015768045154,28.6665171018178,124.570950325204)) ;
#29501=CARTESIAN_POINT('Ctrl Pts',(-18.4548495376105,28.866327643657,124.608386572972)) ;
#29502=CARTESIAN_POINT('Ctrl Pts',(-18.6457373585372,28.6863385632941,124.36907662557)) ;
#29503=CARTESIAN_POINT('Ctrl Pts',(-18.1021082199431,28.8864019614663,124.20819190284)) ;
#29504=CARTESIAN_POINT('Ctrl Pts',(-18.3635430360855,28.7064128811034,124.048922914079)) ;
#29505=CARTESIAN_POINT('Ctrl Pts',(-17.9097030414757,28.9062499304742,123.716849978485)) ;
#29506=CARTESIAN_POINT('Ctrl Pts',(-18.2096162521416,28.7262608501113,123.655848998423)) ;
#29507=CARTESIAN_POINT('Ctrl Pts',(-17.8953659112392,28.9261969645374,123.187000088179)) ;
#29508=CARTESIAN_POINT('Ctrl Pts',(-18.1981447291151,28.7462078841745,123.231968583052)) ;
#29509=CARTESIAN_POINT('Ctrl Pts',(-18.0624463345147,28.9460929155096,122.685244684184)) ;
#29510=CARTESIAN_POINT('Ctrl Pts',(-18.3318078029622,28.7661038351467,122.830562717796)) ;
#29511=CARTESIAN_POINT('Ctrl Pts',(-18.3899816868081,28.9659883951278,122.270147568337)) ;
#29512=CARTESIAN_POINT('Ctrl Pts',(-18.5938359071739,28.7859993147649,122.498483387)) ;
#29513=CARTESIAN_POINT('Ctrl Pts',(-18.8408757372252,28.9859445060926,121.990748528834)) ;
#29514=CARTESIAN_POINT('Ctrl Pts',(-18.9545510633946,28.8059554257297,122.274963123727)) ;
#29515=CARTESIAN_POINT('Ctrl Pts',(-19.3586261760562,29.0058490541326,121.882442313881)) ;
#29516=CARTESIAN_POINT('Ctrl Pts',(-19.3687524196573,28.8258599737697,122.188317114002)) ;
#29517=CARTESIAN_POINT('Ctrl Pts',(-19.8818129365437,29.0257231784517,121.95590917428)) ;
#29518=CARTESIAN_POINT('Ctrl Pts',(-19.7873033983275,28.8457340980888,122.24709086078)) ;
#29519=CARTESIAN_POINT('Ctrl Pts',(-20.3522418344828,29.0457777084507,122.206339109689)) ;
#29520=CARTESIAN_POINT('Ctrl Pts',(-20.1636459491141,28.8657886280878,122.447434352417)) ;
#29521=CARTESIAN_POINT('Ctrl Pts',(-20.7048254925126,29.0655852222107,122.597429836113)) ;
#29522=CARTESIAN_POINT('Ctrl Pts',(-20.4457143874069,28.8855961418478,122.760308841788)) ;
#29523=CARTESIAN_POINT('Ctrl Pts',(-20.9055115949536,29.0855685779784,123.089100356984)) ;
#29524=CARTESIAN_POINT('Ctrl Pts',(-20.6062625174432,28.9055794976156,123.153645765125)) ;
#29525=CARTESIAN_POINT('Ctrl Pts',(-20.9255057422183,29.1054868805624,123.618111697477)) ;
#29526=CARTESIAN_POINT('Ctrl Pts',(-20.622257172822,28.9254978001995,123.576855858986)) ;
#29527=CARTESIAN_POINT('Ctrl Pts',(-20.7655021762044,29.1253550960081,124.121463964361)) ;
#29528=CARTESIAN_POINT('Ctrl Pts',(-20.4942524673024,28.9453660156452,123.979538536319)) ;
#29529=CARTESIAN_POINT('Ctrl Pts',(-20.4398756731327,29.1454054128044,124.543114839599)) ;
#29530=CARTESIAN_POINT('Ctrl Pts',(-20.2337505118372,28.9654163324415,124.316858031653)) ;
#29531=CARTESIAN_POINT('Ctrl Pts',(-19.9961359923068,29.1651814746869,124.82522657557)) ;
#29532=CARTESIAN_POINT('Ctrl Pts',(-19.878755955537,28.985192394324,124.542547120948)) ;
#29533=CARTESIAN_POINT('Ctrl Pts',(-19.4760372478541,29.1852360803793,124.9408742549)) ;
#29534=CARTESIAN_POINT('Ctrl Pts',(-19.4626769826316,29.0052470000165,124.63506310846)) ;
#29535=CARTESIAN_POINT('Ctrl Pts',(-18.9542188864203,29.2050297695352,124.872787108227)) ;
#29536=CARTESIAN_POINT('Ctrl Pts',(-19.0452207775086,29.0250406891723,124.580591027841)) ;
#29537=CARTESIAN_POINT('Ctrl Pts',(-18.4824497195716,29.2249964611296,124.630017164074)) ;
#29538=CARTESIAN_POINT('Ctrl Pts',(-18.667806512202,29.0450073807667,124.386372476876)) ;
#29539=CARTESIAN_POINT('Ctrl Pts',(-18.1224282621344,29.2449565068806,124.240242601981)) ;
#29540=CARTESIAN_POINT('Ctrl Pts',(-18.3797910944419,29.0649674265177,124.074550845858)) ;
#29541=CARTESIAN_POINT('Ctrl Pts',(-17.9173907834527,29.2648547670308,123.752777846934)) ;
#29542=CARTESIAN_POINT('Ctrl Pts',(-18.2157634593431,29.084865686668,123.68457721216)) ;
#29543=CARTESIAN_POINT('Ctrl Pts',(-17.8903701259974,29.28474968258,123.224718223152)) ;
#29544=CARTESIAN_POINT('Ctrl Pts',(-18.1941500680826,29.1047606022171,123.262128658022)) ;
#29545=CARTESIAN_POINT('Ctrl Pts',(-18.0448227791641,29.3046598629936,122.718584462674)) ;
#29546=CARTESIAN_POINT('Ctrl Pts',(-18.3177155786987,29.1246707826307,122.857222129875)) ;
#29547=CARTESIAN_POINT('Ctrl Pts',(-18.3629508949474,29.3245956621079,122.294833096222)) ;
#29548=CARTESIAN_POINT('Ctrl Pts',(-18.5722211306576,29.144606581745,122.518222926126)) ;
#29549=CARTESIAN_POINT('Ctrl Pts',(-18.8065966645385,29.344533523762,122.005031573975)) ;
#29550=CARTESIAN_POINT('Ctrl Pts',(-18.9271398869184,29.1645444433991,122.28638447727)) ;
#29551=CARTESIAN_POINT('Ctrl Pts',(-19.3219781329333,29.3644525703997,121.88380547982)) ;
#29552=CARTESIAN_POINT('Ctrl Pts',(-19.339446619592,29.1844634900368,122.189407632627)) ;
#29553=CARTESIAN_POINT('Ctrl Pts',(-19.8485530096058,29.3844014684538,121.945745518254)) ;
#29554=CARTESIAN_POINT('Ctrl Pts',(-19.7607049211448,29.2044123880909,122.238961921839)) ;
#29555=CARTESIAN_POINT('Ctrl Pts',(-20.3214474198052,29.4043072958969,122.18303123303)) ;
#29556=CARTESIAN_POINT('Ctrl Pts',(-20.1390239324075,29.224318215534,122.428800199034)) ;
#29557=CARTESIAN_POINT('Ctrl Pts',(-20.6245684184595,29.4208899912622,122.502888255951)) ;
#29558=CARTESIAN_POINT('Ctrl Pts',(-20.381503037069,29.2409009108993,122.684669703668)) ;
#29559=CARTESIAN_POINT('Ctrl Pts',(-20.791234180934,29.4341642049858,122.809390920718)) ;
#29560=CARTESIAN_POINT('Ctrl Pts',(-20.5148468140483,29.2541751246229,122.929890379545)) ;
#29561=CARTESIAN_POINT('Ctrl Pts',(-20.8750220852076,29.4442109241851,123.05973121324)) ;
#29562=CARTESIAN_POINT('Ctrl Pts',(-20.5818729237177,29.2642218438223,123.13015699649)) ;
#29563=CARTESIAN_POINT('Ctrl Pts',(-20.9135737768039,29.4540549588308,123.315549607641)) ;
#29564=CARTESIAN_POINT('Ctrl Pts',(-20.6127109316255,29.2740658784679,123.334824035889)) ;
#29565=CARTESIAN_POINT('Ctrl Pts',(-20.9056110532671,29.4673893437353,123.665862635849)) ;
#29566=CARTESIAN_POINT('Ctrl Pts',(-20.6063479581414,29.2874002633725,123.615020710436)) ;
#29567=CARTESIAN_POINT('Ctrl Pts',(-20.7817183691016,29.4839765610351,124.089008121444)) ;
#29568=CARTESIAN_POINT('Ctrl Pts',(-20.5072137252115,29.3039874806722,123.953603177572)) ;
#29569=CARTESIAN_POINT('Ctrl Pts',(-20.5204871039959,29.500609773073,124.445591168462)) ;
#29570=CARTESIAN_POINT('Ctrl Pts',(-20.2982490932776,29.3206206927101,124.238824480431)) ;
#29571=CARTESIAN_POINT('Ctrl Pts',(-20.2482786094575,29.5138922153452,124.664142759317)) ;
#29572=CARTESIAN_POINT('Ctrl Pts',(-20.0804621387608,29.3339031349823,124.413688421931)) ;
#29573=CARTESIAN_POINT('Ctrl Pts',(-20.0203496111071,29.5237981032594,124.789853895898)) ;
#29574=CARTESIAN_POINT('Ctrl Pts',(-19.8981216151747,29.3438090228965,124.514250475789)) ;
#29575=CARTESIAN_POINT('Ctrl Pts',(-19.7720804977814,29.5337865213645,124.875101645455)) ;
#29576=CARTESIAN_POINT('Ctrl Pts',(-19.699504035617,29.3537974410017,124.582447706781)) ;
#29577=CARTESIAN_POINT('Ctrl Pts',(-19.5118312861888,29.5438099486033,124.9158105401)) ;
#29578=CARTESIAN_POINT('Ctrl Pts',(-19.4913069695219,29.3638208682404,124.615012953148)) ;
#29579=CARTESIAN_POINT('Ctrl Pts',(-19.2516162816116,29.5537143797203,124.910922144998)) ;
#29580=CARTESIAN_POINT('Ctrl Pts',(-19.2831262502567,29.3737252993574,124.611097513249)) ;
#29581=CARTESIAN_POINT('Ctrl Pts',(-18.9093488133413,29.5669775323307,124.844857601197)) ;
#29582=CARTESIAN_POINT('Ctrl Pts',(-19.0093557497466,29.3869884519678,124.558255787372)) ;
#29583=CARTESIAN_POINT('Ctrl Pts',(-18.5909285364746,29.5803024302346,124.689972489664)) ;
#29584=CARTESIAN_POINT('Ctrl Pts',(-18.7545953313426,29.4003133498717,124.434343999134)) ;
#29585=CARTESIAN_POINT('Ctrl Pts',(-18.3276416499704,29.5935581738502,124.461801734779)) ;
#29586=CARTESIAN_POINT('Ctrl Pts',(-18.5439553434392,29.4135690934873,124.251793461498)) ;
#29587=CARTESIAN_POINT('Ctrl Pts',(-18.1623453454126,29.6035175472975,124.258928464813)) ;
#29588=CARTESIAN_POINT('Ctrl Pts',(-18.4117225892705,29.4235284669346,124.089495803923)) ;
#29589=CARTESIAN_POINT('Ctrl Pts',(-18.0346636089127,29.6134613712245,124.030895956569)) ;
#29590=CARTESIAN_POINT('Ctrl Pts',(-18.3095785285436,29.4334722908616,123.907068119568)) ;
#29591=CARTESIAN_POINT('Ctrl Pts',(-17.9478442966657,29.6235093153718,123.781548712612)) ;
#29592=CARTESIAN_POINT('Ctrl Pts',(-18.2401254083158,29.4435202350089,123.707589793291)) ;
#29593=CARTESIAN_POINT('Ctrl Pts',(-17.906234953778,29.6333602865899,123.526025793516)) ;
#29594=CARTESIAN_POINT('Ctrl Pts',(-18.2068401299479,29.4533712062271,123.503171143586)) ;
#29595=CARTESIAN_POINT('Ctrl Pts',(-17.9089904954044,29.643332104032,123.264021399714)) ;
#29596=CARTESIAN_POINT('Ctrl Pts',(-18.2090468245195,29.4633430236691,123.293567757575)) ;
#29597=CARTESIAN_POINT('Ctrl Pts',(-17.9573656877064,29.6533275263241,123.005808163303)) ;
#29598=CARTESIAN_POINT('Ctrl Pts',(-18.2477491698236,29.4733384459612,123.086997640274)) ;
#29599=CARTESIAN_POINT('Ctrl Pts',(-18.0504309097234,29.6633605914478,122.75912999775)) ;
#29600=CARTESIAN_POINT('Ctrl Pts',(-18.3222034468051,29.4833715110849,122.88965593636)) ;
#29601=CARTESIAN_POINT('Ctrl Pts',(-18.1824501820335,29.673225924113,122.536018472183)) ;
#29602=CARTESIAN_POINT('Ctrl Pts',(-18.4278207101303,29.4932368437501,122.711168011498)) ;
#29603=CARTESIAN_POINT('Ctrl Pts',(-18.352254460823,29.6831864667106,122.336809734032)) ;
#29604=CARTESIAN_POINT('Ctrl Pts',(-18.5636657405991,29.5031973863477,122.551802554504)) ;
#29605=CARTESIAN_POINT('Ctrl Pts',(-18.5558196647205,29.6932201522123,122.169242143868)) ;
#29606=CARTESIAN_POINT('Ctrl Pts',(-18.7265193140521,29.5132310718494,122.417750218351)) ;
#29607=CARTESIAN_POINT('Ctrl Pts',(-18.7818025397086,29.7031049842026,122.041072921772)) ;
#29608=CARTESIAN_POINT('Ctrl Pts',(-18.9073065097523,29.5231159038397,122.315216877536)) ;
#29609=CARTESIAN_POINT('Ctrl Pts',(-19.0310733364163,29.7131724109624,121.952565569517)) ;
#29610=CARTESIAN_POINT('Ctrl Pts',(-19.1067239210886,29.5331833305995,122.24441307792)) ;
#29611=CARTESIAN_POINT('Ctrl Pts',(-19.286036901977,29.7230109001213,121.909416064618)) ;
#29612=CARTESIAN_POINT('Ctrl Pts',(-19.3106948134357,29.5430218197584,122.209895699158)) ;
#29613=CARTESIAN_POINT('Ctrl Pts',(-19.550453199473,29.7330743813114,121.910880737687)) ;
#29614=CARTESIAN_POINT('Ctrl Pts',(-19.5222278763447,29.5530853009485,122.211069619433)) ;
#29615=CARTESIAN_POINT('Ctrl Pts',(-19.8062464008285,29.7429685391265,121.957671456219)) ;
#29616=CARTESIAN_POINT('Ctrl Pts',(-19.7268617815842,29.5629794587636,122.248504306379)) ;
#29617=CARTESIAN_POINT('Ctrl Pts',(-20.0513931602021,29.7529103958708,122.047912589705)) ;
#29618=CARTESIAN_POINT('Ctrl Pts',(-19.9229782497092,29.5729213155079,122.320699150998)) ;
#29619=CARTESIAN_POINT('Ctrl Pts',(-20.27863327422,29.7629128735422,122.180100002924)) ;
#29620=CARTESIAN_POINT('Ctrl Pts',(-20.1047692120472,29.5829237931793,122.426450889047)) ;
#29621=CARTESIAN_POINT('Ctrl Pts',(-20.4798098359431,29.7729476778465,122.350566712122)) ;
#29622=CARTESIAN_POINT('Ctrl Pts',(-20.265709069093,29.5929585974836,122.562825920578)) ;
#29623=CARTESIAN_POINT('Ctrl Pts',(-20.64549843004,29.7827925546922,122.549284780308)) ;
#29624=CARTESIAN_POINT('Ctrl Pts',(-20.3982580187208,29.6028034743293,122.721801389537)) ;
#29625=CARTESIAN_POINT('Ctrl Pts',(-20.7764071388104,29.7927784342477,122.776669844146)) ;
#29626=CARTESIAN_POINT('Ctrl Pts',(-20.5029831155846,29.6127893538848,122.903710368416)) ;
#29627=CARTESIAN_POINT('Ctrl Pts',(-20.8655976909384,29.8027131646062,123.022090489185)) ;
#29628=CARTESIAN_POINT('Ctrl Pts',(-20.5743335346531,29.6227240842433,123.100047340193)) ;
#29629=CARTESIAN_POINT('Ctrl Pts',(-20.911118673284,29.8127709769191,123.2824053866)) ;
#29630=CARTESIAN_POINT('Ctrl Pts',(-20.6107482780399,29.6327818965562,123.308299712704)) ;
#29631=CARTESIAN_POINT('Ctrl Pts',(-20.9112011989042,29.8225915690435,123.540523528446)) ;
#29632=CARTESIAN_POINT('Ctrl Pts',(-20.610812264355,29.6426024886806,123.514793589066)) ;
#29633=CARTESIAN_POINT('Ctrl Pts',(-20.8656816934186,29.8326581546532,123.801062971402)) ;
#29634=CARTESIAN_POINT('Ctrl Pts',(-20.5743946700159,29.6526690742904,123.723224921033)) ;
#29635=CARTESIAN_POINT('Ctrl Pts',(-20.7770260888292,29.8425577352351,124.045706385067)) ;
#29636=CARTESIAN_POINT('Ctrl Pts',(-20.503468442044,29.6625686548722,123.918938590259)) ;
#29637=CARTESIAN_POINT('Ctrl Pts',(-20.6453879764234,29.8526093349133,124.274656477308)) ;
#29638=CARTESIAN_POINT('Ctrl Pts',(-20.398156179075,29.6726202545505,124.102097751505)) ;
#29639=CARTESIAN_POINT('Ctrl Pts',(-20.4790736605817,29.8624835213303,124.473897491922)) ;
#29640=CARTESIAN_POINT('Ctrl Pts',(-20.2651035506588,29.6824944409674,124.261488905988)) ;
#29641=CARTESIAN_POINT('Ctrl Pts',(-20.2772141277769,29.8725399972112,124.644389380226)) ;
#29642=CARTESIAN_POINT('Ctrl Pts',(-20.1036145883348,29.6925509168483,124.39788099837)) ;
#29643=CARTESIAN_POINT('Ctrl Pts',(-20.0524919644059,29.8824329285138,124.775217544899)) ;
#29644=CARTESIAN_POINT('Ctrl Pts',(-19.9238362960661,29.7024438481509,124.502541627271)) ;
#29645=CARTESIAN_POINT('Ctrl Pts',(-19.8043884253136,29.8924957072264,124.866595201475)) ;
#29646=CARTESIAN_POINT('Ctrl Pts',(-19.7253526612113,29.7125066268636,124.57564199753)) ;
#29647=CARTESIAN_POINT('Ctrl Pts',(-19.5498333322758,29.9023382328076,124.91262179111)) ;
#29648=CARTESIAN_POINT('Ctrl Pts',(-19.5217089312482,29.7223491524447,124.612461273201)) ;
#29649=CARTESIAN_POINT('Ctrl Pts',(-19.2873260771025,29.9123289982325,124.914394172825)) ;
#29650=CARTESIAN_POINT('Ctrl Pts',(-19.3117032550328,29.7323399178696,124.613877366799)) ;
#29651=CARTESIAN_POINT('Ctrl Pts',(-19.0300851291776,29.9222570742305,124.870781057726)) ;
#29652=CARTESIAN_POINT('Ctrl Pts',(-19.1059111853094,29.7422679938676,124.578985150407)) ;
#29653=CARTESIAN_POINT('Ctrl Pts',(-18.7826904157509,29.9322449846175,124.783069756764)) ;
#29654=CARTESIAN_POINT('Ctrl Pts',(-18.9079961342318,29.7522559042547,124.508814517184)) ;
#29655=CARTESIAN_POINT('Ctrl Pts',(-18.5534253143983,29.9422808967425,124.652734665094)) ;
#29656=CARTESIAN_POINT('Ctrl Pts',(-18.7245848901154,29.7622918163796,124.404544830416)) ;
#29657=CARTESIAN_POINT('Ctrl Pts',(-18.3536388771245,29.9521359095901,124.487912827377)) ;
#29658=CARTESIAN_POINT('Ctrl Pts',(-18.5647574170873,29.7721468292273,124.272686483657)) ;
#29659=CARTESIAN_POINT('Ctrl Pts',(-18.1828123336801,29.9621348555064,124.288313606199)) ;
#29660=CARTESIAN_POINT('Ctrl Pts',(-18.4280975323811,29.7821457751435,124.113006096126)) ;
#29661=CARTESIAN_POINT('Ctrl Pts',(-18.0503403718914,29.9720317679544,124.064451745925)) ;
#29662=CARTESIAN_POINT('Ctrl Pts',(-18.3221216633801,29.7920426875915,123.933916272445)) ;
#29663=CARTESIAN_POINT('Ctrl Pts',(-17.9572951648542,29.9820855660479,123.817209301492)) ;
#29664=CARTESIAN_POINT('Ctrl Pts',(-18.2476869703767,29.802096485685,123.736121602035)) ;
#29665=CARTESIAN_POINT('Ctrl Pts',(-17.9093444927588,29.9919664868746,123.56198502385)) ;
#29666=CARTESIAN_POINT('Ctrl Pts',(-18.2093281437484,29.8119774065117,123.53194254377)) ;
#29667=CARTESIAN_POINT('Ctrl Pts',(-17.9059278138796,30.0019710128723,123.299129283876)) ;
#29668=CARTESIAN_POINT('Ctrl Pts',(-18.2065963307077,29.8219819325095,123.321658010208)) ;
#29669=CARTESIAN_POINT('Ctrl Pts',(-17.9482064112771,30.0119549764898,123.040145215749)) ;
#29670=CARTESIAN_POINT('Ctrl Pts',(-18.2404207028938,29.8319658961269,123.114471165854)) ;
#29671=CARTESIAN_POINT('Ctrl Pts',(-18.035508186737,30.0219946170411,122.791197498885)) ;
#29672=CARTESIAN_POINT('Ctrl Pts',(-18.3102636613557,29.8420055366782,122.915313421293)) ;
#29673=CARTESIAN_POINT('Ctrl Pts',(-18.161925212928,30.0318386426558,122.565497657734)) ;
#29674=CARTESIAN_POINT('Ctrl Pts',(-18.411398175043,29.8518495622929,122.734755088774)) ;
#29675=CARTESIAN_POINT('Ctrl Pts',(-18.3274685805744,30.0418296484732,122.361708399386)) ;
#29676=CARTESIAN_POINT('Ctrl Pts',(-18.5438338428557,29.8618405681103,122.571724671418)) ;
#29677=CARTESIAN_POINT('Ctrl Pts',(-18.5272036340267,30.0518674400053,122.189409573137)) ;
#29678=CARTESIAN_POINT('Ctrl Pts',(-18.7036229469901,29.8718783596425,122.433886677935)) ;
#29679=CARTESIAN_POINT('Ctrl Pts',(-18.749230903998,30.0617118397937,122.056613364073)) ;
#29680=CARTESIAN_POINT('Ctrl Pts',(-18.8812446799317,29.8817227594309,122.327651401076)) ;
#29681=CARTESIAN_POINT('Ctrl Pts',(-18.994164126273,30.0716966403505,121.962602178295)) ;
#29682=CARTESIAN_POINT('Ctrl Pts',(-19.0771915377067,29.8917075599876,122.252443739457)) ;
#29683=CARTESIAN_POINT('Ctrl Pts',(-19.2505801464928,30.0816361637616,121.912649736868)) ;
#29684=CARTESIAN_POINT('Ctrl Pts',(-19.2823241699332,29.9016470833988,122.212483121513)) ;
#29685=CARTESIAN_POINT('Ctrl Pts',(-19.5143516088782,30.0916758828626,121.907994125418)) ;
#29686=CARTESIAN_POINT('Ctrl Pts',(-19.4933414803542,29.9116868024998,122.208759920945)) ;
#29687=CARTESIAN_POINT('Ctrl Pts',(-19.7710473972636,30.1015640547819,121.948463714533)) ;
#29688=CARTESIAN_POINT('Ctrl Pts',(-19.6986971847122,29.921574974419,122.241136724367)) ;
#29689=CARTESIAN_POINT('Ctrl Pts',(-20.0194726827981,30.1115536171989,122.033282181041)) ;
#29690=CARTESIAN_POINT('Ctrl Pts',(-19.897436877706,29.931564536836,122.30899253618)) ;
#29691=CARTESIAN_POINT('Ctrl Pts',(-20.2485888048623,30.1215119893936,122.159725978258)) ;
#29692=CARTESIAN_POINT('Ctrl Pts',(-20.0807288910839,29.9415229090307,122.410148456545)) ;
#29693=CARTESIAN_POINT('Ctrl Pts',(-20.451481155513,30.1314120636243,122.322590700227)) ;
#29694=CARTESIAN_POINT('Ctrl Pts',(-20.2430415629541,29.9514229832614,122.540440622386)) ;
#29695=CARTESIAN_POINT('Ctrl Pts',(-20.6255019413428,30.1414581599979,122.521102011054)) ;
#29696=CARTESIAN_POINT('Ctrl Pts',(-20.3822574929672,29.961469079635,122.699250490915)) ;
#29697=CARTESIAN_POINT('Ctrl Pts',(-20.7605632740528,30.151366743995,122.743737177707)) ;
#29698=CARTESIAN_POINT('Ctrl Pts',(-20.4903053110624,29.9713776636321,122.877358615472)) ;
#29699=CARTESIAN_POINT('Ctrl Pts',(-20.8563375787038,30.1613773225859,122.988755129718)) ;
#29700=CARTESIAN_POINT('Ctrl Pts',(-20.5669238525766,29.981388242223,123.073373289288)) ;
#29701=CARTESIAN_POINT('Ctrl Pts',(-20.9076881587369,30.1714064806987,123.247269528944)) ;
#29702=CARTESIAN_POINT('Ctrl Pts',(-20.6080032779403,29.9914174003359,123.28018509895)) ;
#29703=CARTESIAN_POINT('Ctrl Pts',(-20.913643859901,30.1812593625368,123.506108579083)) ;
#29704=CARTESIAN_POINT('Ctrl Pts',(-20.6127668237937,30.0012702821739,123.4872553494)) ;
#29705=CARTESIAN_POINT('Ctrl Pts',(-20.8749374874299,30.1912189236878,123.764965708006)) ;
#29706=CARTESIAN_POINT('Ctrl Pts',(-20.5818009891085,30.0112298433249,123.694340561445)) ;
#29707=CARTESIAN_POINT('Ctrl Pts',(-20.7907663164554,30.2012573582769,124.014958246547)) ;
#29708=CARTESIAN_POINT('Ctrl Pts',(-20.5144631445051,30.021268277914,123.89433442643)) ;
#29709=CARTESIAN_POINT('Ctrl Pts',(-20.6669470046296,30.211130630504,124.243014320118)) ;
#29710=CARTESIAN_POINT('Ctrl Pts',(-20.4154074251945,30.0311415501411,124.07677811357)) ;
#29711=CARTESIAN_POINT('Ctrl Pts',(-20.5021342923516,30.2212038724976,124.450093173102)) ;
#29712=CARTESIAN_POINT('Ctrl Pts',(-20.2835564026306,30.0412147921347,124.242440954527)) ;
#29713=CARTESIAN_POINT('Ctrl Pts',(-20.3089888716899,30.2310242040306,124.621335698669)) ;
#29714=CARTESIAN_POINT('Ctrl Pts',(-20.1290405109537,30.0510351236678,124.379433600609)) ;
#29715=CARTESIAN_POINT('Ctrl Pts',(-20.0834917211719,30.2411028652574,124.760137415769)) ;
#29716=CARTESIAN_POINT('Ctrl Pts',(-19.9486421144359,30.0611137848945,124.49047459601)) ;
#29717=CARTESIAN_POINT('Ctrl Pts',(-19.8427824861803,30.2509544605516,124.855609977345)) ;
#29718=CARTESIAN_POINT('Ctrl Pts',(-19.7560754671688,30.0709653801888,124.566851648864)) ;
#29719=CARTESIAN_POINT('Ctrl Pts',(-19.5836045391597,30.2610275957804,124.909215904106)) ;
#29720=CARTESIAN_POINT('Ctrl Pts',(-19.5487326449223,30.0810385154176,124.609735875249)) ;
#29721=CARTESIAN_POINT('Ctrl Pts',(-19.3250420856673,30.2708700313055,124.916790254833)) ;
#29722=CARTESIAN_POINT('Ctrl Pts',(-19.3418837978834,30.0908809509426,124.615794714185)) ;
#29723=CARTESIAN_POINT('Ctrl Pts',(-19.0654078751379,30.2808508004389,124.879699535808)) ;
#29724=CARTESIAN_POINT('Ctrl Pts',(-19.1341767293187,30.100861720076,124.58612178724)) ;
#29725=CARTESIAN_POINT('Ctrl Pts',(-18.8153894691253,30.2908679016827,124.797325621791)) ;
#29726=CARTESIAN_POINT('Ctrl Pts',(-18.9341621618172,30.1108788213199,124.520222166044)) ;
#29727=CARTESIAN_POINT('Ctrl Pts',(-18.5862012535222,30.3007563492846,124.674812609811)) ;
#29728=CARTESIAN_POINT('Ctrl Pts',(-18.75081252989,30.1207672689217,124.422211818588)) ;
#29729=CARTESIAN_POINT('Ctrl Pts',(-18.378326748722,30.3108120634654,124.511700910524)) ;
#29730=CARTESIAN_POINT('Ctrl Pts',(-18.5845129649496,30.1308229831026,124.29172200353)) ;
#29731=CARTESIAN_POINT('Ctrl Pts',(-18.2050407985295,30.3206872698793,124.31849941652)) ;
#29732=CARTESIAN_POINT('Ctrl Pts',(-18.4458851060229,30.1406981895164,124.137161249517)) ;
#29733=CARTESIAN_POINT('Ctrl Pts',(-18.065746667546,30.330682322352,124.095826539079)) ;
#29734=CARTESIAN_POINT('Ctrl Pts',(-18.3344500579577,30.1506932419891,123.959022954298)) ;
#29735=CARTESIAN_POINT('Ctrl Pts',(-17.9673568014916,30.3407042063141,123.851520456621)) ;
#29736=CARTESIAN_POINT('Ctrl Pts',(-18.2557384543419,30.1607151259512,123.763577933142)) ;
#29737=CARTESIAN_POINT('Ctrl Pts',(-17.9132391133063,30.3506081788434,123.596944459868)) ;
#29738=CARTESIAN_POINT('Ctrl Pts',(-18.2124447103049,30.1706190984805,123.559917834642)) ;
#29739=CARTESIAN_POINT('Ctrl Pts',(-17.9036909635563,30.3605966755043,123.334628818861)) ;
#29740=CARTESIAN_POINT('Ctrl Pts',(-18.2048063513031,30.1806075951414,123.350065504462)) ;
#29741=CARTESIAN_POINT('Ctrl Pts',(-17.9399190541115,30.3705604727523,123.075322497842)) ;
#29742=CARTESIAN_POINT('Ctrl Pts',(-18.2337889737254,30.1905713923894,123.142620833117)) ;
#29743=CARTESIAN_POINT('Ctrl Pts',(-18.019542401481,30.3804644960603,122.827507706759)) ;
#29744=CARTESIAN_POINT('Ctrl Pts',(-18.2974874574404,30.2004754156974,122.944369728192)) ;
#29745=CARTESIAN_POINT('Ctrl Pts',(-18.1430719623568,30.3905249993819,122.593799613876)) ;
#29746=CARTESIAN_POINT('Ctrl Pts',(-18.3963113223776,30.2105359190191,122.757403048071)) ;
#29747=CARTESIAN_POINT('Ctrl Pts',(-18.3015384279696,30.4003655345218,122.38939813401)) ;
#29748=CARTESIAN_POINT('Ctrl Pts',(-18.5230837819883,30.2203764541589,122.593882800201)) ;
#29749=CARTESIAN_POINT('Ctrl Pts',(-18.4971286724099,30.4104277552264,122.211494771059)) ;
#29750=CARTESIAN_POINT('Ctrl Pts',(-18.6795561458151,30.2304386748635,122.451559855394)) ;
#29751=CARTESIAN_POINT('Ctrl Pts',(-18.7171521979687,30.4203249090026,122.072778646605)) ;
#29752=CARTESIAN_POINT('Ctrl Pts',(-18.8555742859337,30.2403358286398,122.340587380024)) ;
#29753=CARTESIAN_POINT('Ctrl Pts',(-18.9583979844501,30.4302560423881,121.973238309069)) ;
#29754=CARTESIAN_POINT('Ctrl Pts',(-19.0485702956595,30.2502669620252,122.260955120397)) ;
#29755=CARTESIAN_POINT('Ctrl Pts',(-19.216180617271,30.4402984175338,121.916755158295)) ;
#29756=CARTESIAN_POINT('Ctrl Pts',(-19.2547965323524,30.260309337171,122.215768415683)) ;
#29757=CARTESIAN_POINT('Ctrl Pts',(-19.4757597411927,30.4501843553,121.905857590778)) ;
#29758=CARTESIAN_POINT('Ctrl Pts',(-19.4624589536106,30.2701952749371,122.207050197027)) ;
#29759=CARTESIAN_POINT('Ctrl Pts',(-19.7361687240311,30.4601801982848,121.940170527014)) ;
#29760=CARTESIAN_POINT('Ctrl Pts',(-19.6707860227431,30.2801911179219,122.234500220989)) ;
#29761=CARTESIAN_POINT('Ctrl Pts',(-19.9853388632678,30.4701221761634,122.018791502423)) ;
#29762=CARTESIAN_POINT('Ctrl Pts',(-19.8701217511132,30.2901330958005,122.297396567724)) ;
#29763=CARTESIAN_POINT('Ctrl Pts',(-20.2176167858868,30.4800815506444,122.139363771227)) ;
#29764=CARTESIAN_POINT('Ctrl Pts',(-20.0559439306465,30.3000924702815,122.393853866718)) ;
#29765=CARTESIAN_POINT('Ctrl Pts',(-20.4263236161457,30.4900781664782,122.298948878856)) ;
#29766=CARTESIAN_POINT('Ctrl Pts',(-20.2229095545966,30.3100890861153,122.521521545282)) ;
#29767=CARTESIAN_POINT('Ctrl Pts',(-20.6045380695498,30.5001123850517,122.493286837832)) ;
#29768=CARTESIAN_POINT('Ctrl Pts',(-20.3654814345688,30.3201233046888,122.676991771903)) ;
#29769=CARTESIAN_POINT('Ctrl Pts',(-20.7440103711108,30.5099654522623,122.711437778196)) ;
#29770=CARTESIAN_POINT('Ctrl Pts',(-20.477059029593,30.3299763718994,122.851511380086)) ;
#29771=CARTESIAN_POINT('Ctrl Pts',(-20.8452704862501,30.5199257101399,122.952793072304)) ;
#29772=CARTESIAN_POINT('Ctrl Pts',(-20.5580675344423,30.339936629777,123.044595041422)) ;
#29773=CARTESIAN_POINT('Ctrl Pts',(-20.9031858777252,30.5299547368455,123.209917654151)) ;
#29774=CARTESIAN_POINT('Ctrl Pts',(-20.604400374506,30.3499656564826,123.250294668849)) ;
#29775=CARTESIAN_POINT('Ctrl Pts',(-20.9155052003231,30.5398649438799,123.470044892547)) ;
#29776=CARTESIAN_POINT('Ctrl Pts',(-20.6142563408965,30.3598758635171,123.458395733584)) ;
#29777=CARTESIAN_POINT('Ctrl Pts',(-20.8830672767706,30.5497998545275,123.729108750999)) ;
#29778=CARTESIAN_POINT('Ctrl Pts',(-20.5883067737471,30.3698107741647,123.665646384641)) ;
#29779=CARTESIAN_POINT('Ctrl Pts',(-20.8050869196827,30.5598409847068,123.981184304442)) ;
#29780=CARTESIAN_POINT('Ctrl Pts',(-20.5259230651749,30.3798519043439,123.867307162557)) ;
#29781=CARTESIAN_POINT('Ctrl Pts',(-20.6865234424483,30.5697281250767,124.212396007676)) ;
#29782=CARTESIAN_POINT('Ctrl Pts',(-20.4310732809217,30.3897390447139,124.052276102492)) ;
#29783=CARTESIAN_POINT('Ctrl Pts',(-20.5283158328247,30.5797204026127,124.421949250781)) ;
#29784=CARTESIAN_POINT('Ctrl Pts',(-20.3045079305415,30.3997313222498,124.219919049695)) ;
#29785=CARTESIAN_POINT('Ctrl Pts',(-20.336893127493,30.589668945881,124.600034325977)) ;
#29786=CARTESIAN_POINT('Ctrl Pts',(-20.1513706158548,30.4096798655181,124.362387386942)) ;
#29787=CARTESIAN_POINT('Ctrl Pts',(-20.117949669728,30.5996056206982,124.742302120517)) ;
#29788=CARTESIAN_POINT('Ctrl Pts',(-19.9762167528585,30.4196165403353,124.476202075347)) ;
#29789=CARTESIAN_POINT('Ctrl Pts',(-19.8765801266705,30.6095890416346,124.845182022236)) ;
#29790=CARTESIAN_POINT('Ctrl Pts',(-19.7831216739518,30.4295999612717,124.558506786004)) ;
#29791=CARTESIAN_POINT('Ctrl Pts',(-19.619448424608,30.6196313568238,124.904513792509)) ;
#29792=CARTESIAN_POINT('Ctrl Pts',(-19.577416370328,30.4396422764609,124.605973056573)) ;
#29793=CARTESIAN_POINT('Ctrl Pts',(-19.3612267210301,30.629471674263,124.918439915204)) ;
#29794=CARTESIAN_POINT('Ctrl Pts',(-19.3708401454886,30.4494825939001,124.617114839488)) ;
#29795=CARTESIAN_POINT('Ctrl Pts',(-19.0994956244019,30.6395013783205,124.887333257162)) ;
#29796=CARTESIAN_POINT('Ctrl Pts',(-19.1614550554373,30.4595122979576,124.592230579924)) ;
#29797=CARTESIAN_POINT('Ctrl Pts',(-18.84757050077,30.649522335043,124.810642476183)) ;
#29798=CARTESIAN_POINT('Ctrl Pts',(-18.9599146662731,30.4695332546801,124.530878830767)) ;
#29799=CARTESIAN_POINT('Ctrl Pts',(-18.6160882477537,30.6593888773466,124.69379526334)) ;
#29800=CARTESIAN_POINT('Ctrl Pts',(-18.7747291880007,30.4793997969837,124.437402426566)) ;
#29801=CARTESIAN_POINT('Ctrl Pts',(-18.4041389450964,30.6694599772918,124.535339469786)) ;
#29802=CARTESIAN_POINT('Ctrl Pts',(-18.6051688617141,30.4894708969289,124.310638472156)) ;
#29803=CARTESIAN_POINT('Ctrl Pts',(-18.2270241518516,30.6793020514693,124.346845255088)) ;
#29804=CARTESIAN_POINT('Ctrl Pts',(-18.4634769547701,30.4993129711065,124.159844592022)) ;
#29805=CARTESIAN_POINT('Ctrl Pts',(-18.0828214570917,30.6892628460564,124.128395071014)) ;
#29806=CARTESIAN_POINT('Ctrl Pts',(-18.3481139027231,30.5092737656935,123.98508542601)) ;
#29807=CARTESIAN_POINT('Ctrl Pts',(-17.9784145006715,30.6993007189572,123.886162207482)) ;
#29808=CARTESIAN_POINT('Ctrl Pts',(-18.2645872182837,30.5193116385943,123.791299501671)) ;
#29809=CARTESIAN_POINT('Ctrl Pts',(-17.9181661940265,30.7091750045013,123.63373426702)) ;
#29810=CARTESIAN_POINT('Ctrl Pts',(-18.216387518212,30.5291859241384,123.589358233217)) ;
#29811=CARTESIAN_POINT('Ctrl Pts',(-17.9023753757216,30.7192447549152,123.369619175597)) ;
#29812=CARTESIAN_POINT('Ctrl Pts',(-18.203753574066,30.5392556745523,123.378065957705)) ;
#29813=CARTESIAN_POINT('Ctrl Pts',(-17.9318397718058,30.7290780394499,123.112874144442)) ;
#29814=CARTESIAN_POINT('Ctrl Pts',(-18.2273236794525,30.549088959087,123.172670800708)) ;
#29815=CARTESIAN_POINT('Ctrl Pts',(-18.0061852690051,30.7391083802499,122.859997359419)) ;
#29816=CARTESIAN_POINT('Ctrl Pts',(-18.2867986965905,30.559119299887,122.970368894539)) ;
#29817=CARTESIAN_POINT('Ctrl Pts',(-18.1240293775023,30.7491403042495,122.624160309324)) ;
#29818=CARTESIAN_POINT('Ctrl Pts',(-18.381072852259,30.5691512238866,122.781698614195)) ;
#29819=CARTESIAN_POINT('Ctrl Pts',(-18.2773844645063,30.7589688391854,122.416346355351)) ;
#29820=CARTESIAN_POINT('Ctrl Pts',(-18.5037551769327,30.5789797588226,122.615447430621)) ;
#29821=CARTESIAN_POINT('Ctrl Pts',(-18.4671493140597,30.7689626169501,122.234795344671)) ;
#29822=CARTESIAN_POINT('Ctrl Pts',(-18.6555658924433,30.5889735365872,122.470205578814)) ;
#29823=CARTESIAN_POINT('Ctrl Pts',(-18.6865926220814,30.7789903274356,122.088882738916)) ;
#29824=CARTESIAN_POINT('Ctrl Pts',(-18.8311197585545,30.5990012470728,122.353474263841)) ;
#29825=CARTESIAN_POINT('Ctrl Pts',(-18.924548918543,30.7888787382696,121.984461740876)) ;
#29826=CARTESIAN_POINT('Ctrl Pts',(-19.0214835756871,30.6088896579067,122.269936340011)) ;
#29827=CARTESIAN_POINT('Ctrl Pts',(-19.1791493957345,30.7988555888051,121.921954029357)) ;
#29828=CARTESIAN_POINT('Ctrl Pts',(-19.2251633755617,30.6188665084423,122.219928660186)) ;
#29829=CARTESIAN_POINT('Ctrl Pts',(-19.4411836962534,30.8088473853556,121.904551040875)) ;
#29830=CARTESIAN_POINT('Ctrl Pts',(-19.4347905867356,30.6288583049927,122.206004671625)) ;
#29831=CARTESIAN_POINT('Ctrl Pts',(-19.7033209422536,30.8188833914493,121.933349289194)) ;
#29832=CARTESIAN_POINT('Ctrl Pts',(-19.6445006241245,30.6388943110864,122.229041739031)) ;
#29833=CARTESIAN_POINT('Ctrl Pts',(-19.9519531581678,30.8287341257121,122.005489324719)) ;
#29834=CARTESIAN_POINT('Ctrl Pts',(-19.84340606214,30.6487450453492,122.286751981054)) ;
#29835=CARTESIAN_POINT('Ctrl Pts',(-20.1877451626918,30.8387253842403,122.12090221111)) ;
#29836=CARTESIAN_POINT('Ctrl Pts',(-20.0320402961377,30.6587363038774,122.379080697725)) ;
#29837=CARTESIAN_POINT('Ctrl Pts',(-20.3985067246429,30.8486432791435,122.274284311981)) ;
#29838=CARTESIAN_POINT('Ctrl Pts',(-20.2006501933195,30.6686541987806,122.50178471108)) ;
#29839=CARTESIAN_POINT('Ctrl Pts',(-20.5814557895788,30.8586714208065,122.463931047394)) ;
#29840=CARTESIAN_POINT('Ctrl Pts',(-20.3470107187746,30.6786823404437,122.653500909386)) ;
#29841=CARTESIAN_POINT('Ctrl Pts',(-20.726703975958,30.8685565889224,122.679309656422)) ;
#29842=CARTESIAN_POINT('Ctrl Pts',(-20.4632103980333,30.6885675085595,122.82580232508)) ;
#29843=CARTESIAN_POINT('Ctrl Pts',(-20.8340446604117,30.8785459524284,122.918876333056)) ;
#29844=CARTESIAN_POINT('Ctrl Pts',(-20.5490845941834,30.6985568720655,123.017454790216)) ;
#29845=CARTESIAN_POINT('Ctrl Pts',(-20.8979488651774,30.8885870874385,123.174891648262)) ;
#29846=CARTESIAN_POINT('Ctrl Pts',(-20.6002096966955,30.7085980070756,123.222266683441)) ;
#29847=CARTESIAN_POINT('Ctrl Pts',(-20.916470523059,30.8984197556265,123.432614768819)) ;
#29848=CARTESIAN_POINT('Ctrl Pts',(-20.6150288055355,30.7184306752636,123.42844428619)) ;
#29849=CARTESIAN_POINT('Ctrl Pts',(-20.8902751541959,30.908413658581,123.693933046635)) ;
#29850=CARTESIAN_POINT('Ctrl Pts',(-20.5940744640968,30.7284245782181,123.637499006698)) ;
#29851=CARTESIAN_POINT('Ctrl Pts',(-20.8183135578191,30.9184429436655,123.947479863912)) ;
#29852=CARTESIAN_POINT('Ctrl Pts',(-20.5365069824791,30.7384538633026,123.840336987593)) ;
#29853=CARTESIAN_POINT('Ctrl Pts',(-20.705558307434,30.9283184721074,124.181239071671)) ;
#29854=CARTESIAN_POINT('Ctrl Pts',(-20.4463047552757,30.7483293917445,124.027344708354)) ;
#29855=CARTESIAN_POINT('Ctrl Pts',(-20.55227636311,30.9383187547235,124.394663488926)) ;
#29856=CARTESIAN_POINT('Ctrl Pts',(-20.3236808563954,30.7583296743606,124.198085320578)) ;
#29857=CARTESIAN_POINT('Ctrl Pts',(-20.3660263502005,30.9482307707805,124.576805636963)) ;
#29858=CARTESIAN_POINT('Ctrl Pts',(-20.1746825091219,30.7682416904176,124.343800207381)) ;
#29859=CARTESIAN_POINT('Ctrl Pts',(-20.148238159027,30.9582728461195,124.725798531691)) ;
#29860=CARTESIAN_POINT('Ctrl Pts',(-20.0004530415488,30.7782837657566,124.462996211481)) ;
#29861=CARTESIAN_POINT('Ctrl Pts',(-19.9112599341149,30.9681726787756,124.833177229003)) ;
#29862=CARTESIAN_POINT('Ctrl Pts',(-19.8108716507074,30.7881835984127,124.548900832387)) ;
#29863=CARTESIAN_POINT('Ctrl Pts',(-19.6570385216495,30.9781650793536,124.898943043692)) ;
#29864=CARTESIAN_POINT('Ctrl Pts',(-19.6074951324964,30.7981759989908,124.601515467701)) ;
#29865=CARTESIAN_POINT('Ctrl Pts',(-19.3941289164041,30.988199101113,124.91918719167)) ;
#29866=CARTESIAN_POINT('Ctrl Pts',(-19.3971675920454,30.8082100207501,124.617712800097)) ;
#29867=CARTESIAN_POINT('Ctrl Pts',(-19.1361050769742,30.9980637119542,124.894240456014)) ;
#29868=CARTESIAN_POINT('Ctrl Pts',(-19.1907487911247,30.8180746315913,124.597757506025)) ;
#29869=CARTESIAN_POINT('Ctrl Pts',(-18.8829168166101,31.0080561114154,124.824588928341)) ;
#29870=CARTESIAN_POINT('Ctrl Pts',(-18.9881977022827,30.8280670310525,124.542038356411)) ;
#29871=CARTESIAN_POINT('Ctrl Pts',(-18.6449556256928,31.0180880647483,124.711122383822)) ;
#29872=CARTESIAN_POINT('Ctrl Pts',(-18.7978278575721,30.8380989843854,124.451266991065)) ;
#29873=CARTESIAN_POINT('Ctrl Pts',(-18.433613598993,31.0279544236899,124.56090527812)) ;
#29874=CARTESIAN_POINT('Ctrl Pts',(-18.6287533485745,30.8479653433271,124.331095266806)) ;
#29875=CARTESIAN_POINT('Ctrl Pts',(-18.2490556295149,31.0379418991757,124.374338785496)) ;
#29876=CARTESIAN_POINT('Ctrl Pts',(-18.4811055111565,30.8579528188129,124.181843656717)) ;
#29877=CARTESIAN_POINT('Ctrl Pts',(-18.1001763827017,31.0478868053642,124.159502137119)) ;
#29878=CARTESIAN_POINT('Ctrl Pts',(-18.3620004446378,30.8678977250013,124.009975722139)) ;
#29879=CARTESIAN_POINT('Ctrl Pts',(-17.9899251037199,31.0579317700244,123.919685682728)) ;
#29880=CARTESIAN_POINT('Ctrl Pts',(-18.2737974607781,30.8779426896616,123.818123443375)) ;
#29881=CARTESIAN_POINT('Ctrl Pts',(-17.9239698947395,31.0677935769293,123.669038395262)) ;
#29882=CARTESIAN_POINT('Ctrl Pts',(-18.221031284142,30.8878044965664,123.617606494588)) ;
#29883=CARTESIAN_POINT('Ctrl Pts',(-17.9017545884407,31.0777862492351,123.407409964502)) ;
#29884=CARTESIAN_POINT('Ctrl Pts',(-18.2032568478911,30.8977971688722,123.408304011957)) ;
#29885=CARTESIAN_POINT('Ctrl Pts',(-17.9251878868137,31.0877149201804,123.147532162219)) ;
#29886=CARTESIAN_POINT('Ctrl Pts',(-18.2220012797528,30.9077258398175,123.200401751263)) ;
#29887=CARTESIAN_POINT('Ctrl Pts',(-17.9931295756622,31.0976674624057,122.894987346514)) ;
#29888=CARTESIAN_POINT('Ctrl Pts',(-18.2763524482962,30.9176783820428,122.998365442682)) ;
#29889=CARTESIAN_POINT('Ctrl Pts',(-18.1043255909368,31.1076688184016,122.656813330348)) ;
#29890=CARTESIAN_POINT('Ctrl Pts',(-18.3653072153254,30.9276797380387,122.807825340817)) ;
#29891=CARTESIAN_POINT('Ctrl Pts',(-18.2558710625769,31.1176974306763,122.441217023634)) ;
#29892=CARTESIAN_POINT('Ctrl Pts',(-18.486541760213,30.9377083503134,122.63534705266)) ;
#29893=CARTESIAN_POINT('Ctrl Pts',(-18.4392436560099,31.1275617652258,122.257966085798)) ;
#29894=CARTESIAN_POINT('Ctrl Pts',(-18.6332381127442,30.9475726848629,122.488744871235)) ;
#29895=CARTESIAN_POINT('Ctrl Pts',(-18.6541277020736,31.1375540893024,122.107106052772)) ;
#29896=CARTESIAN_POINT('Ctrl Pts',(-18.805144006808,30.9575650089395,122.368055041523)) ;
#29897=CARTESIAN_POINT('Ctrl Pts',(-18.8903979931826,31.1474815816683,121.99639777191)) ;
#29898=CARTESIAN_POINT('Ctrl Pts',(-18.9941591920697,30.9674925013054,122.279486427225)) ;
#29899=CARTESIAN_POINT('Ctrl Pts',(-19.1447705223875,31.1575089402191,121.927739862365)) ;
#29900=CARTESIAN_POINT('Ctrl Pts',(-19.1976565800842,30.9775198598562,122.224557940461)) ;
#29901=CARTESIAN_POINT('Ctrl Pts',(-19.403557785468,31.1673953582702,121.904339822956)) ;
#29902=CARTESIAN_POINT('Ctrl Pts',(-19.40468609459,30.9874062779074,122.205835676203)) ;
#29903=CARTESIAN_POINT('Ctrl Pts',(-19.6662117593913,31.1774270930056,121.926411212978)) ;
#29904=CARTESIAN_POINT('Ctrl Pts',(-19.6148094082564,30.9974380126427,122.223490535075)) ;
#29905=CARTESIAN_POINT('Ctrl Pts',(-19.9173816828502,31.1873086742489,121.992520931665)) ;
#29906=CARTESIAN_POINT('Ctrl Pts',(-19.815745871323,31.007319593886,122.276376119868)) ;
#29907=CARTESIAN_POINT('Ctrl Pts',(-20.1575099536661,31.1973706522812,122.103127502672)) ;
#29908=CARTESIAN_POINT('Ctrl Pts',(-20.0078493692217,31.0173815719183,122.364859298836)) ;
#29909=CARTESIAN_POINT('Ctrl Pts',(-20.3704779128565,31.2072277306429,122.250647114545)) ;
#29910=CARTESIAN_POINT('Ctrl Pts',(-20.1782250129861,31.02723865028,122.482873132973)) ;
#29911=CARTESIAN_POINT('Ctrl Pts',(-20.557479635411,31.2172223037489,122.435014859895)) ;
#29912=CARTESIAN_POINT('Ctrl Pts',(-20.3278279402508,31.037233223386,122.630365704853)) ;
#29913=CARTESIAN_POINT('Ctrl Pts',(-20.7087042530508,31.2271481000365,122.647587798087)) ;
#29914=CARTESIAN_POINT('Ctrl Pts',(-20.4488094657624,31.0471590196736,122.8004227559)) ;
#29915=CARTESIAN_POINT('Ctrl Pts',(-20.8218837391766,31.2371734672062,122.885470873075)) ;
#29916=CARTESIAN_POINT('Ctrl Pts',(-20.539355037212,31.0571843868434,122.99072823021)) ;
#29917=CARTESIAN_POINT('Ctrl Pts',(-20.8912500206041,31.2470695468601,123.136118325641)) ;
#29918=CARTESIAN_POINT('Ctrl Pts',(-20.594850255258,31.0670804664972,123.191245492355)) ;
#29919=CARTESIAN_POINT('Ctrl Pts',(-20.916817797818,31.2570646265657,123.397534145115)) ;
#29920=CARTESIAN_POINT('Ctrl Pts',(-20.6153065879517,31.0770755462028,123.400378543151)) ;
#29921=CARTESIAN_POINT('Ctrl Pts',(-20.8960973227342,31.2670897143815,123.660166672547)) ;
#29922=CARTESIAN_POINT('Ctrl Pts',(-20.5987327498281,31.0871006340186,123.610482259063)) ;
#29923=CARTESIAN_POINT('Ctrl Pts',(-20.809893476644,31.2802735367488,123.995726533553)) ;
#29924=CARTESIAN_POINT('Ctrl Pts',(-20.5297709305419,31.1002844563859,123.87894293253)) ;
#29925=CARTESIAN_POINT('Ctrl Pts',(-20.6369390480152,31.2935956548947,124.30466223955)) ;
#29926=CARTESIAN_POINT('Ctrl Pts',(-20.3913865526123,31.1136065745318,124.126114241275)) ;
#29927=CARTESIAN_POINT('Ctrl Pts',(-20.3908148582284,31.3069748645223,124.555818133117)) ;
#29928=CARTESIAN_POINT('Ctrl Pts',(-20.1945187656795,31.1269857841594,124.327003669048)) ;
#29929=CARTESIAN_POINT('Ctrl Pts',(-20.1809438414753,31.3168131017665,124.706820601801)) ;
#29930=CARTESIAN_POINT('Ctrl Pts',(-20.0266169655379,31.1368240214036,124.447815030813)) ;
#29931=CARTESIAN_POINT('Ctrl Pts',(-19.9425721439745,31.3268860250252,124.821852782534)) ;
#29932=CARTESIAN_POINT('Ctrl Pts',(-19.8359226633174,31.1468969446624,124.539840740485)) ;
#29933=CARTESIAN_POINT('Ctrl Pts',(-19.6932575438715,31.3367426664803,124.89218888602)) ;
#29934=CARTESIAN_POINT('Ctrl Pts',(-19.6364695236485,31.1567535861175,124.596111832383)) ;
#29935=CARTESIAN_POINT('Ctrl Pts',(-19.4322556852193,31.3467280419864,124.919201640466)) ;
#29936=CARTESIAN_POINT('Ctrl Pts',(-19.4276731793723,31.1667389616235,124.617725775355)) ;
#29937=CARTESIAN_POINT('Ctrl Pts',(-19.0841345592013,31.3600120734468,124.893999424143)) ;
#29938=CARTESIAN_POINT('Ctrl Pts',(-19.1491518620383,31.180022993084,124.597557799836)) ;
#29939=CARTESIAN_POINT('Ctrl Pts',(-18.6686831095259,31.3765308653172,124.751522351196)) ;
#29940=CARTESIAN_POINT('Ctrl Pts',(-18.8168267270378,31.1965417849543,124.483599784169)) ;
#29941=CARTESIAN_POINT('Ctrl Pts',(-18.3221176258635,31.3933165823238,124.470780414967)) ;
#29942=CARTESIAN_POINT('Ctrl Pts',(-18.5395236640967,31.2133275019609,124.258964588696)) ;
#29943=CARTESIAN_POINT('Ctrl Pts',(-18.1195171640873,31.4064297308328,124.19192546978)) ;
#29944=CARTESIAN_POINT('Ctrl Pts',(-18.3774781924197,31.2264406504699,124.035919165873)) ;
#29945=CARTESIAN_POINT('Ctrl Pts',(-18.0029767278721,31.416465279913,123.955390640417)) ;
#29946=CARTESIAN_POINT('Ctrl Pts',(-18.2842367998029,31.2364761995501,123.846683979849)) ;
#29947=CARTESIAN_POINT('Ctrl Pts',(-17.930131161295,31.4264813360924,123.702427282653)) ;
#29948=CARTESIAN_POINT('Ctrl Pts',(-18.2259601153952,31.2464922557295,123.644318871564)) ;
#29949=CARTESIAN_POINT('Ctrl Pts',(-17.8927981854828,31.4396593719584,123.358188928687)) ;
#29950=CARTESIAN_POINT('Ctrl Pts',(-18.1960923899022,31.2596702915955,123.368912638922)) ;
#29951=CARTESIAN_POINT('Ctrl Pts',(-17.9589427761027,31.4562612491455,122.921846253614)) ;
#29952=CARTESIAN_POINT('Ctrl Pts',(-18.2490034305915,31.2762721687826,123.019854359994)) ;
#29953=CARTESIAN_POINT('Ctrl Pts',(-18.2153452936868,31.4763243937614,122.454312103361)) ;
#29954=CARTESIAN_POINT('Ctrl Pts',(-18.4541225899952,31.2963353133985,122.645820297505)) ;
#29955=CARTESIAN_POINT('Ctrl Pts',(-18.6105119795525,31.4961252838451,122.106643007625)) ;
#29956=CARTESIAN_POINT('Ctrl Pts',(-18.7702543020853,31.3161362034822,122.36768303858)) ;
#29957=CARTESIAN_POINT('Ctrl Pts',(-19.1034924936999,31.5160684091238,121.912133008607)) ;
#29958=CARTESIAN_POINT('Ctrl Pts',(-19.164637971874,31.3360793287609,122.212071605184)) ;
#29959=CARTESIAN_POINT('Ctrl Pts',(-19.6321465341764,31.5359664542434,121.89791137193)) ;
#29960=CARTESIAN_POINT('Ctrl Pts',(-19.5875618065476,31.3559773738805,122.200691277358)) ;
#29961=CARTESIAN_POINT('Ctrl Pts',(-20.1341066883384,31.5558522138702,122.063616102464)) ;
#29962=CARTESIAN_POINT('Ctrl Pts',(-19.9891315918773,31.3758631335073,122.333252851735)) ;
#29963=CARTESIAN_POINT('Ctrl Pts',(-20.5525283110554,31.57591738905,122.394200252169)) ;
#29964=CARTESIAN_POINT('Ctrl Pts',(-20.3238701259959,31.3959283086872,122.597717694145)) ;
#29965=CARTESIAN_POINT('Ctrl Pts',(-20.8296000415882,31.5957440321528,122.84254361497)) ;
#29966=CARTESIAN_POINT('Ctrl Pts',(-20.5455305086285,31.41575495179,122.95639217086)) ;
#29967=CARTESIAN_POINT('Ctrl Pts',(-20.9388687495492,31.6156527416012,123.360136077141)) ;
#29968=CARTESIAN_POINT('Ctrl Pts',(-20.6329476561718,31.4356636612383,123.370466593898)) ;
#29969=CARTESIAN_POINT('Ctrl Pts',(-20.8648791195812,31.635604578633,123.885385533411)) ;
#29970=CARTESIAN_POINT('Ctrl Pts',(-20.573757693884,31.4556154982701,123.790666808917)) ;
#29971=CARTESIAN_POINT('Ctrl Pts',(-20.6147262487971,31.6556130533361,124.354604940983)) ;
#29972=CARTESIAN_POINT('Ctrl Pts',(-20.3736372170781,31.4756239729733,124.166043186308)) ;
#29973=CARTESIAN_POINT('Ctrl Pts',(-20.2239265792252,31.6754145120976,124.70712499995)) ;
#29974=CARTESIAN_POINT('Ctrl Pts',(-20.0609969972757,31.4954254317348,124.448061814946)) ;
#29975=CARTESIAN_POINT('Ctrl Pts',(-19.7329944592127,31.6953714003336,124.907950846951)) ;
#29976=CARTESIAN_POINT('Ctrl Pts',(-19.6682511534378,31.5153823199707,124.608723469387)) ;
#29977=CARTESIAN_POINT('Ctrl Pts',(-19.2022559885623,31.7153552377477,124.928017723692)) ;
#29978=CARTESIAN_POINT('Ctrl Pts',(-19.2436602612597,31.5353661573848,124.624778160052)) ;
#29979=CARTESIAN_POINT('Ctrl Pts',(-18.7005580952729,31.7351636769686,124.768181953029)) ;
#29980=CARTESIAN_POINT('Ctrl Pts',(-18.8422995577168,31.5551745966057,124.496909315192)) ;
#29981=CARTESIAN_POINT('Ctrl Pts',(-18.2796327533169,31.7551493863488,124.444432947283)) ;
#29982=CARTESIAN_POINT('Ctrl Pts',(-18.505559042595,31.5751603059859,124.237909991823)) ;
#29983=CARTESIAN_POINT('Ctrl Pts',(-17.9957625956122,31.7750189093641,123.998861683797)) ;
#29984=CARTESIAN_POINT('Ctrl Pts',(-18.2784622930544,31.5950298290012,123.881451524151)) ;
#29985=CARTESIAN_POINT('Ctrl Pts',(-17.8804111930879,31.7950396484813,123.479601508631)) ;
#29986=CARTESIAN_POINT('Ctrl Pts',(-18.1861815644187,31.6150505681184,123.466043484708)) ;
#29987=CARTESIAN_POINT('Ctrl Pts',(-17.947813732566,31.8148437134583,122.957375358431)) ;
#29988=CARTESIAN_POINT('Ctrl Pts',(-18.240104726759,31.6348546330954,123.048260409413)) ;
#29989=CARTESIAN_POINT('Ctrl Pts',(-18.1922019497661,31.834905677189,122.483631625261)) ;
#29990=CARTESIAN_POINT('Ctrl Pts',(-18.4356159960294,31.6549165968261,122.669266566499)) ;
#29991=CARTESIAN_POINT('Ctrl Pts',(-18.579670503548,31.8547388574775,122.126047237428)) ;
#29992=CARTESIAN_POINT('Ctrl Pts',(-18.7455928985157,31.6747497771146,122.383198612062)) ;
#29993=CARTESIAN_POINT('Ctrl Pts',(-19.0672415407129,31.8746580548036,121.919977102834)) ;
#29994=CARTESIAN_POINT('Ctrl Pts',(-19.1356512341748,31.6946689744407,122.218343904972)) ;
#29995=CARTESIAN_POINT('Ctrl Pts',(-19.596473798273,31.8945960799169,121.892968380712)) ;
#29996=CARTESIAN_POINT('Ctrl Pts',(-19.559037724007,31.714606999554,122.196738778409)) ;
#29997=CARTESIAN_POINT('Ctrl Pts',(-20.1018977424829,31.914474125973,122.047010861552)) ;
#29998=CARTESIAN_POINT('Ctrl Pts',(-19.9633772292207,31.7344850456101,122.319975266152)) ;
#29999=CARTESIAN_POINT('Ctrl Pts',(-20.5266155989396,31.934458860261,122.365876034326)) ;
#30000=CARTESIAN_POINT('Ctrl Pts',(-20.3031501256687,31.7544697798982,122.575069435507)) ;
#30001=CARTESIAN_POINT('Ctrl Pts',(-20.8161540516341,31.9543696769395,122.809022005469)) ;
#30002=CARTESIAN_POINT('Ctrl Pts',(-20.5347790794781,31.7743805965766,122.92958819007)) ;
#30003=CARTESIAN_POINT('Ctrl Pts',(-20.9372264313366,31.9743686524582,123.326459903439)) ;
#30004=CARTESIAN_POINT('Ctrl Pts',(-20.6316344224308,31.7943795720954,123.343539156427)) ;
#30005=CARTESIAN_POINT('Ctrl Pts',(-20.8757007542274,31.9941735731034,123.849340834267)) ;
#30006=CARTESIAN_POINT('Ctrl Pts',(-20.5824107852335,31.8141844927406,123.761844941543)) ;
#30007=CARTESIAN_POINT('Ctrl Pts',(-20.6381061492539,32.0141575333947,124.324236585198)) ;
#30008=CARTESIAN_POINT('Ctrl Pts',(-20.3923321320177,31.8341684530318,124.141760152678)) ;
#30009=CARTESIAN_POINT('Ctrl Pts',(-20.254277484515,32.0340437371186,124.687750970673)) ;
#30010=CARTESIAN_POINT('Ctrl Pts',(-20.085266409861,31.8540546567557,124.432569686706)) ;
#30011=CARTESIAN_POINT('Ctrl Pts',(-19.7682819396191,32.0539929154418,124.89962239012)) ;
#30012=CARTESIAN_POINT('Ctrl Pts',(-19.696468384716,31.8740038350789,124.60206379762)) ;
#30013=CARTESIAN_POINT('Ctrl Pts',(-19.2403770539516,32.0738947146813,124.932732853793)) ;
#30014=CARTESIAN_POINT('Ctrl Pts',(-19.2741434998259,31.8939056343185,124.628548078608)) ;
#30015=CARTESIAN_POINT('Ctrl Pts',(-18.7330993587673,32.0937733197337,124.784941725984)) ;
#30016=CARTESIAN_POINT('Ctrl Pts',(-18.868322906955,31.9137842393708,124.510313181707)) ;
#30017=CARTESIAN_POINT('Ctrl Pts',(-18.3035498467669,32.1138056794594,124.470304693559)) ;
#30018=CARTESIAN_POINT('Ctrl Pts',(-18.5246822315973,31.9338165990965,124.258593399843)) ;
#30019=CARTESIAN_POINT('Ctrl Pts',(-18.0587930611329,32.1303874054155,124.103782576889)) ;
#30020=CARTESIAN_POINT('Ctrl Pts',(-18.3288903810443,31.9503983250526,123.965395758089)) ;
#30021=CARTESIAN_POINT('Ctrl Pts',(-17.9464384610694,32.1435815757134,123.775785395635)) ;
#30022=CARTESIAN_POINT('Ctrl Pts',(-18.2389994529127,31.9635924953505,123.702969740174)) ;
#30023=CARTESIAN_POINT('Ctrl Pts',(-17.8916962164165,32.1568937538066,123.430264324837)) ;
#30024=CARTESIAN_POINT('Ctrl Pts',(-18.1952099799321,31.9769046734437,123.426608864667)) ;
#30025=CARTESIAN_POINT('Ctrl Pts',(-17.9374894753685,32.1734599333999,122.99232521224)) ;
#30026=CARTESIAN_POINT('Ctrl Pts',(-18.2318514252023,31.9934708530371,123.076188915836)) ;
#30027=CARTESIAN_POINT('Ctrl Pts',(-18.1302718088824,32.1900881282601,122.594703559392)) ;
#30028=CARTESIAN_POINT('Ctrl Pts',(-18.3860665483606,32.0100990478972,122.758138239794)) ;
#30029=CARTESIAN_POINT('Ctrl Pts',(-18.3588141057148,32.2033767099699,122.330591540781)) ;
#30030=CARTESIAN_POINT('Ctrl Pts',(-18.5689151874287,32.023387629607,122.546823962737)) ;
#30031=CARTESIAN_POINT('Ctrl Pts',(-18.5618539277949,32.2133449580735,122.165112713871)) ;
#30032=CARTESIAN_POINT('Ctrl Pts',(-18.7313457221629,32.0333558777106,122.414447852175)) ;
#30033=CARTESIAN_POINT('Ctrl Pts',(-18.7891790717996,32.2232597143296,122.037790376024)) ;
#30034=CARTESIAN_POINT('Ctrl Pts',(-18.9132084602232,32.0432706339667,122.312590559703)) ;
#30035=CARTESIAN_POINT('Ctrl Pts',(-19.037513591275,32.2332728649808,121.95074327932)) ;
#30036=CARTESIAN_POINT('Ctrl Pts',(-19.1118736703297,32.0532837846179,122.242954838167)) ;
#30037=CARTESIAN_POINT('Ctrl Pts',(-19.2972230251791,32.2432855721828,121.908553873528)) ;
#30038=CARTESIAN_POINT('Ctrl Pts',(-19.3196523089538,32.0632964918199,122.209207408094)) ;
#30039=CARTESIAN_POINT('Ctrl Pts',(-19.6446403660395,32.2565048608741,121.9125795524)) ;
#30040=CARTESIAN_POINT('Ctrl Pts',(-19.5975327596128,32.0765157805112,122.212420869537)) ;
#30041=CARTESIAN_POINT('Ctrl Pts',(-20.0699198327109,32.2731235418722,122.031411460383)) ;
#30042=CARTESIAN_POINT('Ctrl Pts',(-19.937823277613,32.0931344615093,122.307507212326)) ;
#30043=CARTESIAN_POINT('Ctrl Pts',(-20.4284615240151,32.2896884496456,122.28707638829)) ;
#30044=CARTESIAN_POINT('Ctrl Pts',(-20.224607600475,32.1096993692827,122.512015776509)) ;
#30045=CARTESIAN_POINT('Ctrl Pts',(-20.6522321703216,32.3030869212564,122.55890721292)) ;
#30046=CARTESIAN_POINT('Ctrl Pts',(-20.4036500863331,32.1230978408936,122.729503326657)) ;
#30047=CARTESIAN_POINT('Ctrl Pts',(-20.7796679108865,32.3129281767434,122.783972393412)) ;
#30048=CARTESIAN_POINT('Ctrl Pts',(-20.5055910403937,32.1329390963805,122.909552376083)) ;
#30049=CARTESIAN_POINT('Ctrl Pts',(-20.8678841148157,32.3229144923316,123.031085830974)) ;
#30050=CARTESIAN_POINT('Ctrl Pts',(-20.576163376053,32.1429254119687,123.107244959995)) ;
#30051=CARTESIAN_POINT('Ctrl Pts',(-20.9117732133019,32.332851099918,123.288538866815)) ;
#30052=CARTESIAN_POINT('Ctrl Pts',(-20.6112720124456,32.1528620195551,123.313207406856)) ;
#30053=CARTESIAN_POINT('Ctrl Pts',(-20.910145815352,32.3429009672863,123.552606824038)) ;
#30054=CARTESIAN_POINT('Ctrl Pts',(-20.6099679432151,32.1629118869234,123.524461792942)) ;
#30055=CARTESIAN_POINT('Ctrl Pts',(-20.8638163142715,32.3527514619611,123.807307622436)) ;
#30056=CARTESIAN_POINT('Ctrl Pts',(-20.5729021084178,32.1727623815982,123.72822191254)) ;
#30057=CARTESIAN_POINT('Ctrl Pts',(-20.773519983493,32.3627232623556,124.053271401024)) ;
#30058=CARTESIAN_POINT('Ctrl Pts',(-20.5006629717372,32.1827341819927,123.924992078725)) ;
#30059=CARTESIAN_POINT('Ctrl Pts',(-20.6415042015941,32.3727192293814,124.280422776241)) ;
#30060=CARTESIAN_POINT('Ctrl Pts',(-20.3950484362192,32.1927301490186,124.106711993813)) ;
#30061=CARTESIAN_POINT('Ctrl Pts',(-20.4711197706811,32.3827566887626,124.481749462152)) ;
#30062=CARTESIAN_POINT('Ctrl Pts',(-20.2587391854302,32.2027676083997,124.267771863989)) ;
#30063=CARTESIAN_POINT('Ctrl Pts',(-20.2726207381904,32.3925973896634,124.6475312724)) ;
#30064=CARTESIAN_POINT('Ctrl Pts',(-20.0999386785007,32.2126083093005,124.400395461972)) ;
#30065=CARTESIAN_POINT('Ctrl Pts',(-20.0438481628859,32.4026454109307,124.779365277945)) ;
#30066=CARTESIAN_POINT('Ctrl Pts',(-19.9169195251314,32.2226563305678,124.50586072606)) ;
#30067=CARTESIAN_POINT('Ctrl Pts',(-19.7979892008617,32.4125928040134,124.868183348147)) ;
#30068=CARTESIAN_POINT('Ctrl Pts',(-19.7202316993048,32.2326037236505,124.576913031386)) ;
#30069=CARTESIAN_POINT('Ctrl Pts',(-19.5415342218403,32.4225029500598,124.913581797367)) ;
#30070=CARTESIAN_POINT('Ctrl Pts',(-19.515067529213,32.2425138696969,124.613229582587)) ;
#30071=CARTESIAN_POINT('Ctrl Pts',(-19.277223918375,32.4325618639094,124.913465271175)) ;
#30072=CARTESIAN_POINT('Ctrl Pts',(-19.3036192607228,32.2525727835465,124.613134137926)) ;
#30073=CARTESIAN_POINT('Ctrl Pts',(-19.022469311543,32.4424026341987,124.868802452506)) ;
#30074=CARTESIAN_POINT('Ctrl Pts',(-19.099816280715,32.2624135538358,124.577401773527)) ;
#30075=CARTESIAN_POINT('Ctrl Pts',(-18.7738114256327,32.4524655037773,124.778908029314)) ;
#30076=CARTESIAN_POINT('Ctrl Pts',(-18.9008906793119,32.2724764234145,124.505484170492)) ;
#30077=CARTESIAN_POINT('Ctrl Pts',(-18.5484324346786,32.4623598269078,124.649195864268)) ;
#30078=CARTESIAN_POINT('Ctrl Pts',(-18.7205888114285,32.2823707465449,124.401712667753)) ;
#30079=CARTESIAN_POINT('Ctrl Pts',(-18.3476349380033,32.4723016340023,124.482101731582)) ;
#30080=CARTESIAN_POINT('Ctrl Pts',(-18.5599523479521,32.2923125536394,124.268035850005)) ;
#30081=CARTESIAN_POINT('Ctrl Pts',(-18.1777508202333,32.4823041449576,124.281474853431)) ;
#30082=CARTESIAN_POINT('Ctrl Pts',(-18.4240467225334,32.3023150645948,124.10753302208)) ;
#30083=CARTESIAN_POINT('Ctrl Pts',(-18.0452392633268,32.492338865776,124.053503454134)) ;
#30084=CARTESIAN_POINT('Ctrl Pts',(-18.3180393459561,32.3123497854131,123.925154800795)) ;
#30085=CARTESIAN_POINT('Ctrl Pts',(-17.9556292696089,32.5021840432817,123.810780412352)) ;
#30086=CARTESIAN_POINT('Ctrl Pts',(-18.24635350555,32.3221949629189,123.73097605505)) ;
#30087=CARTESIAN_POINT('Ctrl Pts',(-17.9083727783839,32.5121688036828,123.552719582534)) ;
#30088=CARTESIAN_POINT('Ctrl Pts',(-18.2085503837353,32.3321797233199,123.524527146658)) ;
#30089=CARTESIAN_POINT('Ctrl Pts',(-17.9065240318847,32.5221077099992,123.291502653985)) ;
#30090=CARTESIAN_POINT('Ctrl Pts',(-18.2070734512826,32.3421186296363,123.315553837412)) ;
#30091=CARTESIAN_POINT('Ctrl Pts',(-17.9505907657664,32.5321499376349,123.031335993592)) ;
#30092=CARTESIAN_POINT('Ctrl Pts',(-18.242328891931,32.3521608572721,123.107420816645)) ;
#30093=CARTESIAN_POINT('Ctrl Pts',(-18.0376192936705,32.5420351492193,122.786543593569)) ;
#30094=CARTESIAN_POINT('Ctrl Pts',(-18.3119535058972,32.3620460688564,122.911587983726)) ;
#30095=CARTESIAN_POINT('Ctrl Pts',(-18.1669767556182,32.5520340794212,122.557873550048)) ;
#30096=CARTESIAN_POINT('Ctrl Pts',(-18.4154411876375,32.3720449990584,122.728653018332)) ;
#30097=CARTESIAN_POINT('Ctrl Pts',(-18.3326104946629,32.5619515023317,122.356600741746)) ;
#30098=CARTESIAN_POINT('Ctrl Pts',(-18.5479494908398,32.3819624219688,122.567636304059)) ;
#30099=CARTESIAN_POINT('Ctrl Pts',(-18.5332526173871,32.5719994344104,122.185007966984)) ;
#30100=CARTESIAN_POINT('Ctrl Pts',(-18.7084645480787,32.3920103540475,122.430363551794)) ;
#30101=CARTESIAN_POINT('Ctrl Pts',(-18.7567232187338,32.5818768102198,122.052875232647)) ;
#30102=CARTESIAN_POINT('Ctrl Pts',(-18.8872415842206,32.4018877298569,122.324659316094)) ;
#30103=CARTESIAN_POINT('Ctrl Pts',(-19.0039525695959,32.5919307033877,121.95982536141)) ;
#30104=CARTESIAN_POINT('Ctrl Pts',(-19.0850258485824,32.4119416230248,122.250221203348)) ;
#30105=CARTESIAN_POINT('Ctrl Pts',(-19.2595182815849,32.601824326641,121.911755678648)) ;
#30106=CARTESIAN_POINT('Ctrl Pts',(-19.2894783105699,32.4218352462781,122.211767438031)) ;
#30107=CARTESIAN_POINT('Ctrl Pts',(-19.5238926627054,32.611886920264,121.908700188409)) ;
#30108=CARTESIAN_POINT('Ctrl Pts',(-19.5009779851935,32.4318978399011,122.209324968628)) ;
#30109=CARTESIAN_POINT('Ctrl Pts',(-19.7791709674073,32.6217294942531,121.950535647314)) ;
#30110=CARTESIAN_POINT('Ctrl Pts',(-19.7051996362344,32.4417404138902,122.242795101324)) ;
#30111=CARTESIAN_POINT('Ctrl Pts',(-20.0271280441419,32.631720251136,122.036735366636)) ;
#30112=CARTESIAN_POINT('Ctrl Pts',(-19.9035645706121,32.4517311707731,122.311756541242)) ;
#30113=CARTESIAN_POINT('Ctrl Pts',(-20.2549311093635,32.6416483128939,122.163938821337)) ;
#30114=CARTESIAN_POINT('Ctrl Pts',(-20.0858057967329,32.4616592325311,122.413520699274)) ;
#30115=CARTESIAN_POINT('Ctrl Pts',(-20.4586943445291,32.6516362887831,122.329402962598)) ;
#30116=CARTESIAN_POINT('Ctrl Pts',(-20.2488151736051,32.4716472084202,122.545893272239)) ;
#30117=CARTESIAN_POINT('Ctrl Pts',(-20.6311078851739,32.6616719531395,122.528955452347)) ;
#30118=CARTESIAN_POINT('Ctrl Pts',(-20.3867446776176,32.4816828727767,122.705536503265)) ;
#30119=CARTESIAN_POINT('Ctrl Pts',(-20.76419350534,32.6715278915592,122.751167847475)) ;
#30120=CARTESIAN_POINT('Ctrl Pts',(-20.4932112993434,32.4915388111963,122.88330668774)) ;
#30121=CARTESIAN_POINT('Ctrl Pts',(-20.8583709770248,32.6815233829561,122.99634558384)) ;
#30122=CARTESIAN_POINT('Ctrl Pts',(-20.5685516696912,32.5015343025932,123.079449363677)) ;
#30123=CARTESIAN_POINT('Ctrl Pts',(-20.9082019158921,32.6914331879096,123.251966021349)) ;
#30124=CARTESIAN_POINT('Ctrl Pts',(-20.6084146932958,32.5114441075467,123.283945511149)) ;
#30125=CARTESIAN_POINT('Ctrl Pts',(-20.913367466307,32.7014454101763,123.515032024856)) ;
#30126=CARTESIAN_POINT('Ctrl Pts',(-20.6125455536325,32.5214563298134,123.494398306009)) ;
#30127=CARTESIAN_POINT('Ctrl Pts',(-20.8722060909322,32.7114732908691,123.775321815842)) ;
#30128=CARTESIAN_POINT('Ctrl Pts',(-20.5796147887184,32.5314842105063,123.702629927723)) ;
#30129=CARTESIAN_POINT('Ctrl Pts',(-20.7883600167789,32.7213296868517,124.02038977865)) ;
#30130=CARTESIAN_POINT('Ctrl Pts',(-20.5125366813953,32.5413406064889,123.898683026209)) ;
#30131=CARTESIAN_POINT('Ctrl Pts',(-20.6615779007813,32.7313544840317,124.25132140461)) ;
#30132=CARTESIAN_POINT('Ctrl Pts',(-20.4111096709629,32.5513654036688,124.083427628986)) ;
#30133=CARTESIAN_POINT('Ctrl Pts',(-20.4960157375153,32.7413854140155,124.456454889738)) ;
#30134=CARTESIAN_POINT('Ctrl Pts',(-20.2786586468199,32.5613963336526,124.247533447329)) ;
#30135=CARTESIAN_POINT('Ctrl Pts',(-20.3013621684409,32.7512300165242,124.626844922445)) ;
#30136=CARTESIAN_POINT('Ctrl Pts',(-20.1229354628895,32.5712409361613,124.38384373688)) ;
#30137=CARTESIAN_POINT('Ctrl Pts',(-20.0771483650704,32.7612208677483,124.763458712167)) ;
#30138=CARTESIAN_POINT('Ctrl Pts',(-19.9435638346434,32.5812317873854,124.493133506793)) ;
#30139=CARTESIAN_POINT('Ctrl Pts',(-19.8312628601083,32.7712587007595,124.858962378708)) ;
#30140=CARTESIAN_POINT('Ctrl Pts',(-19.7468547876405,32.5912696203966,124.569535079804)) ;
#30141=CARTESIAN_POINT('Ctrl Pts',(-19.5775920832475,32.7811030892249,124.909777937782)) ;
#30142=CARTESIAN_POINT('Ctrl Pts',(-19.5439188102841,32.6011140088621,124.610185961714)) ;
#30143=CARTESIAN_POINT('Ctrl Pts',(-19.3153197757331,32.7910878935945,124.916379101424)) ;
#30144=CARTESIAN_POINT('Ctrl Pts',(-19.3341011312526,32.6110988132316,124.615465586228)) ;
#30145=CARTESIAN_POINT('Ctrl Pts',(-19.0569748481772,32.8010274130773,124.877619388893)) ;
#30146=CARTESIAN_POINT('Ctrl Pts',(-19.1274258094831,32.6210383327145,124.584456619583)) ;
#30147=CARTESIAN_POINT('Ctrl Pts',(-18.8068609697535,32.8110671440787,124.793713447214)) ;
#30148=CARTESIAN_POINT('Ctrl Pts',(-18.9273350056697,32.6310780637158,124.517330604952)) ;
#30149=CARTESIAN_POINT('Ctrl Pts',(-18.5785199696836,32.820955272325,124.669655218426)) ;
#30150=CARTESIAN_POINT('Ctrl Pts',(-18.7446634574821,32.6409661919621,124.418083265181)) ;
#30151=CARTESIAN_POINT('Ctrl Pts',(-18.3728153330768,32.8309449975335,124.506569798915)) ;
#30152=CARTESIAN_POINT('Ctrl Pts',(-18.5801006004135,32.6509559171706,124.287614130099)) ;
#30153=CARTESIAN_POINT('Ctrl Pts',(-18.1992468678326,32.840902762235,124.310742518053)) ;
#30154=CARTESIAN_POINT('Ctrl Pts',(-18.4412469568537,32.6609136818721,124.130951769751)) ;
#30155=CARTESIAN_POINT('Ctrl Pts',(-18.0625524288157,32.850805103647,124.089302873787)) ;
#30156=CARTESIAN_POINT('Ctrl Pts',(-18.3318926747522,32.6708160232841,123.95380009295)) ;
#30157=CARTESIAN_POINT('Ctrl Pts',(-17.9650377613778,32.8608492993534,123.844039624706)) ;
#30158=CARTESIAN_POINT('Ctrl Pts',(-18.2538818733743,32.6808602189905,123.757588954974)) ;
#30159=CARTESIAN_POINT('Ctrl Pts',(-17.9122844842802,32.8707567001127,123.58906943826)) ;
#30160=CARTESIAN_POINT('Ctrl Pts',(-18.2116804247751,32.6907676197498,123.553613231978)) ;
#30161=CARTESIAN_POINT('Ctrl Pts',(-17.9040614841339,32.880767299987,123.326126151249)) ;
#30162=CARTESIAN_POINT('Ctrl Pts',(-18.2051029793148,32.7007782196241,123.34325861009)) ;
#30163=CARTESIAN_POINT('Ctrl Pts',(-17.9421976273555,32.8907975958992,123.065306227518)) ;
#30164=CARTESIAN_POINT('Ctrl Pts',(-18.2356129698765,32.7108085155363,123.134602745316)) ;
#30165=CARTESIAN_POINT('Ctrl Pts',(-18.0232436735507,32.9006523755489,122.819357208247)) ;
#30166=CARTESIAN_POINT('Ctrl Pts',(-18.3004504322419,32.720663295186,122.937844802407)) ;
#30167=CARTESIAN_POINT('Ctrl Pts',(-18.1463463293519,32.9106097037664,122.588444800357)) ;
#30168=CARTESIAN_POINT('Ctrl Pts',(-18.3989330865564,32.7306206234035,122.753115585193)) ;
#30169=CARTESIAN_POINT('Ctrl Pts',(-18.3093474042476,32.9206487366733,122.381033273986)) ;
#30170=CARTESIAN_POINT('Ctrl Pts',(-18.5293347464535,32.7406596563104,122.587186824327)) ;
#30171=CARTESIAN_POINT('Ctrl Pts',(-18.5023603004912,32.9305218485626,122.207583253798)) ;
#30172=CARTESIAN_POINT('Ctrl Pts',(-18.6837449255098,32.7505327681997,122.448428002608)) ;
#30173=CARTESIAN_POINT('Ctrl Pts',(-18.7269817759468,32.9405951335897,122.067617063673)) ;
#30174=CARTESIAN_POINT('Ctrl Pts',(-18.8634428286131,32.7606060532268,122.336455563458)) ;
#30175=CARTESIAN_POINT('Ctrl Pts',(-18.9663055363985,32.9504154533265,121.970905134139)) ;
#30176=CARTESIAN_POINT('Ctrl Pts',(-19.0549009577353,32.7704263729636,122.259087166004)) ;
#30177=CARTESIAN_POINT('Ctrl Pts',(-19.2252558871534,32.9604941187049,121.915591458617)) ;
#30178=CARTESIAN_POINT('Ctrl Pts',(-19.262061748827,32.780505038342,122.214836808385)) ;
#30179=CARTESIAN_POINT('Ctrl Pts',(-19.4840372151867,32.9703457091887,121.906199287805)) ;
#30180=CARTESIAN_POINT('Ctrl Pts',(-19.4690857796967,32.7903566288258,122.207323762619)) ;
#30181=CARTESIAN_POINT('Ctrl Pts',(-19.7462073716882,32.9804188595076,121.942441422299)) ;
#30182=CARTESIAN_POINT('Ctrl Pts',(-19.6788221704482,32.8004297791447,122.236318111422)) ;
#30183=CARTESIAN_POINT('Ctrl Pts',(-19.9923907933803,32.9902612394826,122.021850824201)) ;
#30184=CARTESIAN_POINT('Ctrl Pts',(-19.8757676411912,32.8102721591198,122.299845862724)) ;
#30185=CARTESIAN_POINT('Ctrl Pts',(-20.2246277641436,33.0002422157257,122.143718242006)) ;
#30186=CARTESIAN_POINT('Ctrl Pts',(-20.0615568191512,32.8202531353628,122.397340033153)) ;
#30187=CARTESIAN_POINT('Ctrl Pts',(-20.4326666594073,33.010258544081,122.304997705767)) ;
#30188=CARTESIAN_POINT('Ctrl Pts',(-20.2279876169795,32.8302694637181,122.52636399411)) ;
#30189=CARTESIAN_POINT('Ctrl Pts',(-20.6076780088902,33.0201563410721,122.497403957948)) ;
#30190=CARTESIAN_POINT('Ctrl Pts',(-20.3679958534134,32.8401672607093,122.680288693608)) ;
#30191=CARTESIAN_POINT('Ctrl Pts',(-20.7486295700232,33.0301688978042,122.719608055138)) ;
#30192=CARTESIAN_POINT('Ctrl Pts',(-20.4807568301996,32.8501798174413,122.858052122149)) ;
#30193=CARTESIAN_POINT('Ctrl Pts',(-20.8484637130917,33.0402009326507,122.96359161389)) ;
#30194=CARTESIAN_POINT('Ctrl Pts',(-20.5606237531606,32.8602118522878,123.053239243088)) ;
#30195=CARTESIAN_POINT('Ctrl Pts',(-20.9039796443904,33.0500403334661,123.216152649294)) ;
#30196=CARTESIAN_POINT('Ctrl Pts',(-20.6050359484339,32.8700512531033,123.255286987946)) ;
#30197=CARTESIAN_POINT('Ctrl Pts',(-20.9152463774755,33.0601061191177,123.480399984258)) ;
#30198=CARTESIAN_POINT('Ctrl Pts',(-20.6140490933859,32.8801170387548,123.466685170754)) ;
#30199=CARTESIAN_POINT('Ctrl Pts',(-20.8809372575507,33.0699965742323,123.738064421165)) ;
#30200=CARTESIAN_POINT('Ctrl Pts',(-20.5866016261539,32.8900074938694,123.672815854496)) ;
#30201=CARTESIAN_POINT('Ctrl Pts',(-20.8021533889854,33.0799886928681,123.98853537261)) ;
#30202=CARTESIAN_POINT('Ctrl Pts',(-20.523574446852,32.8999996125052,123.873192408795)) ;
#30203=CARTESIAN_POINT('Ctrl Pts',(-20.6812106073249,33.0899515196311,124.220732031348)) ;
#30204=CARTESIAN_POINT('Ctrl Pts',(-20.4268202076342,32.9099624392683,124.058949317243)) ;
#30205=CARTESIAN_POINT('Ctrl Pts',(-20.5232306933288,33.099855802904,124.427605321835)) ;
#30206=CARTESIAN_POINT('Ctrl Pts',(-20.3004367035077,32.9198667225411,124.22444733005)) ;
#30207=CARTESIAN_POINT('Ctrl Pts',(-20.3285971107455,33.1099162368511,124.606480559927)) ;
#30208=CARTESIAN_POINT('Ctrl Pts',(-20.1447295646736,32.9299271564882,124.36754764172)) ;
#30209=CARTESIAN_POINT('Ctrl Pts',(-20.1108525131507,33.1197567895243,124.746047511506)) ;
#30210=CARTESIAN_POINT('Ctrl Pts',(-19.970534871693,32.9397677091614,124.479200559667)) ;
#30211=CARTESIAN_POINT('Ctrl Pts',(-19.8669950901314,33.12981900947,124.84821784105)) ;
#30212=CARTESIAN_POINT('Ctrl Pts',(-19.7754486895611,32.9498299291071,124.560937006756)) ;
#30213=CARTESIAN_POINT('Ctrl Pts',(-19.6132318493154,33.1397161487486,124.905283007203)) ;
#30214=CARTESIAN_POINT('Ctrl Pts',(-19.5724388798712,32.9597270683857,124.606588967545)) ;
#30215=CARTESIAN_POINT('Ctrl Pts',(-19.3525812289575,33.1496473408836,124.918328736674)) ;
#30216=CARTESIAN_POINT('Ctrl Pts',(-19.3639189712111,32.9696582605208,124.617025749215)) ;
#30217=CARTESIAN_POINT('Ctrl Pts',(-19.090770522027,33.1596894955287,124.885264797401)) ;
#30218=CARTESIAN_POINT('Ctrl Pts',(-19.1544702195643,32.9797004151658,124.590574725584)) ;
#30219=CARTESIAN_POINT('Ctrl Pts',(-18.842487870914,33.169576256548,124.808646986439)) ;
#30220=CARTESIAN_POINT('Ctrl Pts',(-18.9558448766533,32.9895871761851,124.529280933374)) ;
#30221=CARTESIAN_POINT('Ctrl Pts',(-18.6085457635101,33.1795755582652,124.689058201042)) ;
#30222=CARTESIAN_POINT('Ctrl Pts',(-18.7686911704573,32.9995864779024,124.433610222531)) ;
#30223=CARTESIAN_POINT('Ctrl Pts',(-18.4004044124469,33.189496356432,124.532007686267)) ;
#30224=CARTESIAN_POINT('Ctrl Pts',(-18.6021783869313,33.0095072760691,124.307970451747)) ;
#30225=CARTESIAN_POINT('Ctrl Pts',(-18.2206897370185,33.1995304100287,124.339091714962)) ;
#30226=CARTESIAN_POINT('Ctrl Pts',(-18.4584063193687,33.0195413296658,124.153637825087)) ;
#30227=CARTESIAN_POINT('Ctrl Pts',(-18.0786177880743,33.2094535275951,124.120374761366)) ;
#30228=CARTESIAN_POINT('Ctrl Pts',(-18.344748777028,33.0294644472322,123.978664981646)) ;
#30229=CARTESIAN_POINT('Ctrl Pts',(-17.9753934550452,33.2195096510942,123.87713368977)) ;
#30230=CARTESIAN_POINT('Ctrl Pts',(-18.2621688831962,33.0395205707314,123.784072046529)) ;
#30231=CARTESIAN_POINT('Ctrl Pts',(-17.9170984303965,33.2293550927491,123.625046988953)) ;
#30232=CARTESIAN_POINT('Ctrl Pts',(-18.2155327344032,33.0493660123862,123.582403874291)) ;
#30233=CARTESIAN_POINT('Ctrl Pts',(-17.9024396209619,33.2393173938732,123.363675275733)) ;
#30234=CARTESIAN_POINT('Ctrl Pts',(-18.2038050999464,33.0593283135103,123.373306898927)) ;
#30235=CARTESIAN_POINT('Ctrl Pts',(-17.9339408232565,33.2493458731483,123.102009100134)) ;
#30236=CARTESIAN_POINT('Ctrl Pts',(-18.2290055541262,33.0693567927855,123.163973819942)) ;
#30237=CARTESIAN_POINT('Ctrl Pts',(-18.009402919707,33.259256226658,122.852760854094)) ;
#30238=CARTESIAN_POINT('Ctrl Pts',(-18.2893745088673,33.0792671462951,122.964575736527)) ;
#30239=CARTESIAN_POINT('Ctrl Pts',(-18.1266871223674,33.2691910988352,122.61950036567)) ;
#30240=CARTESIAN_POINT('Ctrl Pts',(-18.3832009980876,33.0892020184723,122.777967498192)) ;
#30241=CARTESIAN_POINT('Ctrl Pts',(-18.2845465433898,33.2792322364209,122.40806845954)) ;
#30242=CARTESIAN_POINT('Ctrl Pts',(-18.5094881032574,33.099243156058,122.608821464249)) ;
#30243=CARTESIAN_POINT('Ctrl Pts',(-18.4736647676083,33.2891193856355,122.229881635933)) ;
#30244=CARTESIAN_POINT('Ctrl Pts',(-18.6607816011752,33.1091303052726,122.466272069737)) ;
#30245=CARTESIAN_POINT('Ctrl Pts',(-18.6928889148738,33.2991116203865,122.085373784708)) ;
#30246=CARTESIAN_POINT('Ctrl Pts',(-18.8361603422665,33.1191225400237,122.350665209582)) ;
#30247=CARTESIAN_POINT('Ctrl Pts',(-18.9328841091275,33.3090603259495,121.981637584403)) ;
#30248=CARTESIAN_POINT('Ctrl Pts',(-19.0281557898517,33.1290712455866,122.267675703838)) ;
#30249=CARTESIAN_POINT('Ctrl Pts',(-19.1868031331839,33.3189963943732,121.920862306553)) ;
#30250=CARTESIAN_POINT('Ctrl Pts',(-19.2312903095408,33.1390073140103,122.219054752622)) ;
#30251=CARTESIAN_POINT('Ctrl Pts',(-19.4487454010854,33.328982078589,121.90471788781)) ;
#30252=CARTESIAN_POINT('Ctrl Pts',(-19.4408438645719,33.1489929982261,122.20613828772)) ;
#30253=CARTESIAN_POINT('Ctrl Pts',(-19.7108540776556,33.3390225051576,121.934873930191)) ;
#30254=CARTESIAN_POINT('Ctrl Pts',(-19.6505310372627,33.1590334247948,122.230262297346)) ;
#30255=CARTESIAN_POINT('Ctrl Pts',(-19.9588162424853,33.3488616186214,122.008165761205)) ;
#30256=CARTESIAN_POINT('Ctrl Pts',(-19.8488999925423,33.1688725382585,122.288894547529)) ;
#30257=CARTESIAN_POINT('Ctrl Pts',(-20.1950323307625,33.3588913527972,122.125097981869)) ;
#30258=CARTESIAN_POINT('Ctrl Pts',(-20.0378734209598,33.1789022724343,122.38243939003)) ;
#30259=CARTESIAN_POINT('Ctrl Pts',(-20.406784218548,33.3689134523031,122.281698617158)) ;
#30260=CARTESIAN_POINT('Ctrl Pts',(-20.2072754977896,33.1889243719402,122.507719170111)) ;
#30261=CARTESIAN_POINT('Ctrl Pts',(-20.5858350552601,33.3787818921965,122.469326974363)) ;
#30262=CARTESIAN_POINT('Ctrl Pts',(-20.350516319059,33.1987928118337,122.657820459907)) ;
#30263=CARTESIAN_POINT('Ctrl Pts',(-20.732476955186,33.3888507568821,122.68954538537)) ;
#30264=CARTESIAN_POINT('Ctrl Pts',(-20.4678308998726,33.2088616765193,122.833994843785)) ;
#30265=CARTESIAN_POINT('Ctrl Pts',(-20.8362904559934,33.3986934299808,122.926463443138)) ;
#30266=CARTESIAN_POINT('Ctrl Pts',(-20.5508822680002,33.2187043496179,123.023527908559)) ;
#30267=CARTESIAN_POINT('Ctrl Pts',(-20.8990494415645,33.4086540641432,123.180578146984)) ;
#30268=CARTESIAN_POINT('Ctrl Pts',(-20.6010906294462,33.2286649837803,123.226819047015)) ;
#30269=CARTESIAN_POINT('Ctrl Pts',(-20.916351249052,33.4186919798213,123.443786581483)) ;
#30270=CARTESIAN_POINT('Ctrl Pts',(-20.6149332528463,33.2387028994585,123.43738582393)) ;
#30271=CARTESIAN_POINT('Ctrl Pts',(-20.8886281343362,33.4285662546808,123.701819630219)) ;
#30272=CARTESIAN_POINT('Ctrl Pts',(-20.592756117805,33.2485771743179,123.643811594593)) ;
#30273=CARTESIAN_POINT('Ctrl Pts',(-20.8151004364326,33.4386360050559,123.95598455471)) ;
#30274=CARTESIAN_POINT('Ctrl Pts',(-20.5339351068565,33.258646924693,123.84714415652)) ;
#30275=CARTESIAN_POINT('Ctrl Pts',(-20.7013946872375,33.4484693004304,124.188056231771)) ;
#30276=CARTESIAN_POINT('Ctrl Pts',(-20.442972128081,33.2684802200675,124.03280115278)) ;
#30277=CARTESIAN_POINT('Ctrl Pts',(-20.5466931297227,33.45849959791,124.401459336272)) ;
#30278=CARTESIAN_POINT('Ctrl Pts',(-20.3192120229929,33.2785105175472,124.20352454908)) ;
#30279=CARTESIAN_POINT('Ctrl Pts',(-20.3567007162318,33.4685316843515,124.58424663072)) ;
#30280=CARTESIAN_POINT('Ctrl Pts',(-20.1672189437675,33.2885426039886,124.34975536662)) ;
#30281=CARTESIAN_POINT('Ctrl Pts',(-20.1426457143214,33.4783596128404,124.728735741513)) ;
#30282=CARTESIAN_POINT('Ctrl Pts',(-19.9959765796565,33.2983705324775,124.465347258471)) ;
#30283=CARTESIAN_POINT('Ctrl Pts',(-19.9029989792466,33.4883556539512,124.836308043002)) ;
#30284=CARTESIAN_POINT('Ctrl Pts',(-19.8042599394586,33.3083665735883,124.551406472735)) ;
#30285=CARTESIAN_POINT('Ctrl Pts',(-19.6474220237301,33.4983814660524,124.900335793291)) ;
#30286=CARTESIAN_POINT('Ctrl Pts',(-19.5997986983396,33.3183923856895,124.602630093288)) ;
#30287=CARTESIAN_POINT('Ctrl Pts',(-19.3882695560054,33.5082687009472,124.919091810044)) ;
#30288=CARTESIAN_POINT('Ctrl Pts',(-19.3924774972755,33.3282796205843,124.617636375343)) ;
#30289=CARTESIAN_POINT('Ctrl Pts',(-19.1274334857693,33.5182455671582,124.892759807624)) ;
#30290=CARTESIAN_POINT('Ctrl Pts',(-19.1838086836,33.3382564867954,124.596572391666)) ;
#30291=CARTESIAN_POINT('Ctrl Pts',(-18.8746590268341,33.52823851103,124.821451907867)) ;
#30292=CARTESIAN_POINT('Ctrl Pts',(-18.9815887977188,33.3482494306672,124.539527654376)) ;
#30293=CARTESIAN_POINT('Ctrl Pts',(-18.6372374521722,33.5382764337014,124.706546424498)) ;
#30294=CARTESIAN_POINT('Ctrl Pts',(-18.7916507985739,33.3582873533385,124.447604630339)) ;
#30295=CARTESIAN_POINT('Ctrl Pts',(-18.4271493677989,33.5481248979631,124.555368999614)) ;
#30296=CARTESIAN_POINT('Ctrl Pts',(-18.6235800486874,33.3681358176002,124.326664485506)) ;
#30297=CARTESIAN_POINT('Ctrl Pts',(-18.2435773439465,33.5581167647071,124.367679767415)) ;
#30298=CARTESIAN_POINT('Ctrl Pts',(-18.4767213025052,33.3781276843442,124.176514389402)) ;
#30299=CARTESIAN_POINT('Ctrl Pts',(-18.096319636919,33.5680344967483,124.152599028164)) ;
#30300=CARTESIAN_POINT('Ctrl Pts',(-18.3589139685211,33.3880454163854,124.004451152358)) ;
#30301=CARTESIAN_POINT('Ctrl Pts',(-17.9874040348388,33.5780626816436,123.912652984584)) ;
#30302=CARTESIAN_POINT('Ctrl Pts',(-18.271779888472,33.3980736012807,123.812495012593)) ;
#30303=CARTESIAN_POINT('Ctrl Pts',(-17.9226291155959,33.5879478396924,123.661079753393)) ;
#30304=CARTESIAN_POINT('Ctrl Pts',(-18.2199583955529,33.4079587593295,123.611237435979)) ;
#30305=CARTESIAN_POINT('Ctrl Pts',(-17.9016709287819,33.5979372002341,123.399402541443)) ;
#30306=CARTESIAN_POINT('Ctrl Pts',(-18.2031899993243,33.4179481198712,123.401895940217)) ;
#30307=CARTESIAN_POINT('Ctrl Pts',(-17.9271501704679,33.6079783571685,123.1367648659)) ;
#30308=CARTESIAN_POINT('Ctrl Pts',(-18.2235716341578,33.4279892768056,123.191785556007)) ;
#30309=CARTESIAN_POINT('Ctrl Pts',(-17.9959631146861,33.6178109406236,122.887710030823)) ;
#30310=CARTESIAN_POINT('Ctrl Pts',(-18.2786200105537,33.4378218602607,122.992541933455)) ;
#30311=CARTESIAN_POINT('Ctrl Pts',(-18.1081263093149,33.6278051605856,122.650231330554)) ;
#30312=CARTESIAN_POINT('Ctrl Pts',(-18.3683487586546,33.4478160802227,122.802558226559)) ;
#30313=CARTESIAN_POINT('Ctrl Pts',(-18.2607792875272,33.6378332623729,122.435411305488)) ;
#30314=CARTESIAN_POINT('Ctrl Pts',(-18.4904696240239,33.45784418201,122.630701109372)) ;
#30315=CARTESIAN_POINT('Ctrl Pts',(-18.4453797141511,33.647713206996,122.252832221367)) ;
#30316=CARTESIAN_POINT('Ctrl Pts',(-18.6381482311407,33.4677241266331,122.484636845497)) ;
#30317=CARTESIAN_POINT('Ctrl Pts',(-18.6610157891126,33.657703533553,122.10310705135)) ;
#30318=CARTESIAN_POINT('Ctrl Pts',(-18.8106558663145,33.4777144531901,122.364855145268)) ;
#30319=CARTESIAN_POINT('Ctrl Pts',(-18.8982140305105,33.6676444652073,121.993631136502)) ;
#30320=CARTESIAN_POINT('Ctrl Pts',(-19.0004133768427,33.4876553848444,122.277272732784)) ;
#30321=CARTESIAN_POINT('Ctrl Pts',(-19.1519080089799,33.6776315837102,121.92632833614)) ;
#30322=CARTESIAN_POINT('Ctrl Pts',(-19.2033679299254,33.4976425033473,122.223428561246)) ;
#30323=CARTESIAN_POINT('Ctrl Pts',(-19.4146423301779,33.6876649166074,121.904411969349)) ;
#30324=CARTESIAN_POINT('Ctrl Pts',(-19.4135552411739,33.5076758362445,122.20589349727)) ;
#30325=CARTESIAN_POINT('Ctrl Pts',(-19.6729091690056,33.6975310210521,121.927545767156)) ;
#30326=CARTESIAN_POINT('Ctrl Pts',(-19.6201683942856,33.5175419406893,122.224398461816)) ;
#30327=CARTESIAN_POINT('Ctrl Pts',(-19.9282681240009,33.7075971349325,121.996466980296)) ;
#30328=CARTESIAN_POINT('Ctrl Pts',(-19.8244562056054,33.5276080545696,122.279533486686)) ;
#30329=CARTESIAN_POINT('Ctrl Pts',(-20.1628320829574,33.7174531467009,122.10634520991)) ;
#30330=CARTESIAN_POINT('Ctrl Pts',(-20.0121077897334,33.537464066338,122.367434006079)) ;
#30331=CARTESIAN_POINT('Ctrl Pts',(-20.3781604555604,33.7274478503322,122.256728476995)) ;
#30332=CARTESIAN_POINT('Ctrl Pts',(-20.184371642184,33.5474587699693,122.487738827655)) ;
#30333=CARTESIAN_POINT('Ctrl Pts',(-20.5643974693118,33.7374791860571,122.443302838799)) ;
#30334=CARTESIAN_POINT('Ctrl Pts',(-20.3333627176559,33.5574901056942,122.636996853287)) ;
#30335=CARTESIAN_POINT('Ctrl Pts',(-20.713269761922,33.7473457112607,122.655597325724)) ;
#30336=CARTESIAN_POINT('Ctrl Pts',(-20.4524620449125,33.5673566308979,122.806830892729)) ;
#30337=CARTESIAN_POINT('Ctrl Pts',(-20.8247303532555,33.7573331393065,122.893178808627)) ;
#30338=CARTESIAN_POINT('Ctrl Pts',(-20.5416324255552,33.5773440589437,122.99689507574)) ;
#30339=CARTESIAN_POINT('Ctrl Pts',(-20.8931087336896,33.767278068993,123.145457142139)) ;
#30340=CARTESIAN_POINT('Ctrl Pts',(-20.5963371660383,33.5872889886301,123.198716996963)) ;
#30341=CARTESIAN_POINT('Ctrl Pts',(-20.9167263518425,33.7773229871015,123.408343079754)) ;
#30342=CARTESIAN_POINT('Ctrl Pts',(-20.6152334042726,33.5973339067386,123.409025569641)) ;
#30343=CARTESIAN_POINT('Ctrl Pts',(-20.8949748056446,33.7871849567154,123.666612207482)) ;
#30344=CARTESIAN_POINT('Ctrl Pts',(-20.5978343558141,33.6071958763525,123.61564071411)) ;
#30345=CARTESIAN_POINT('Ctrl Pts',(-20.8283422293108,33.7971770247366,123.920571241178)) ;
#30346=CARTESIAN_POINT('Ctrl Pts',(-20.5445304472365,33.6171879443737,123.818808427627)) ;
#30347=CARTESIAN_POINT('Ctrl Pts',(-20.7192376865205,33.8071079501112,124.157662672187)) ;
#30348=CARTESIAN_POINT('Ctrl Pts',(-20.4572488862588,33.6271188697483,124.008482329076)) ;
#30349=CARTESIAN_POINT('Ctrl Pts',(-20.5707091129721,33.8170585783346,124.372854625881)) ;
#30350=CARTESIAN_POINT('Ctrl Pts',(-20.3384279325118,33.6370694979717,124.180637052448)) ;
#30351=CARTESIAN_POINT('Ctrl Pts',(-20.3862313186414,33.8270588173937,124.560056609312)) ;
#30352=CARTESIAN_POINT('Ctrl Pts',(-20.1908473210986,33.6470697370308,124.330400159823)) ;
#30353=CARTESIAN_POINT('Ctrl Pts',(-20.1712584195521,33.8370872727629,124.71248063517)) ;
#30354=CARTESIAN_POINT('Ctrl Pts',(-20.0188703330059,33.6570981924,124.45234117015)) ;
#30355=CARTESIAN_POINT('Ctrl Pts',(-19.9370901885251,33.8469533073462,124.823799494521)) ;
#30356=CARTESIAN_POINT('Ctrl Pts',(-19.8315368156364,33.6669642269833,124.541398163761)) ;
#30357=CARTESIAN_POINT('Ctrl Pts',(-19.6841021964421,33.8569456290936,124.894057284954)) ;
#30358=CARTESIAN_POINT('Ctrl Pts',(-19.6291473694453,33.6769565487307,124.597606616661)) ;
#30359=CARTESIAN_POINT('Ctrl Pts',(-19.424287490384,33.8668779187706,124.9192160717)) ;
#30360=CARTESIAN_POINT('Ctrl Pts',(-19.4212948596349,33.6868888384077,124.617735604572)) ;
#30361=CARTESIAN_POINT('Ctrl Pts',(-19.1622401128872,33.8768795637414,124.898995670993)) ;
#30362=CARTESIAN_POINT('Ctrl Pts',(-19.2116608120875,33.6968904833785,124.60156252601)) ;
#30363=CARTESIAN_POINT('Ctrl Pts',(-18.823429392135,33.8901921971574,124.811777112252)) ;
#30364=CARTESIAN_POINT('Ctrl Pts',(-18.9405918138416,33.7102031167945,124.531785666973)) ;
#30365=CARTESIAN_POINT('Ctrl Pts',(-18.5168908225473,33.903423946539,124.639429121269)) ;
#30366=CARTESIAN_POINT('Ctrl Pts',(-18.6953483850143,33.7234348661761,124.393891756695)) ;
#30367=CARTESIAN_POINT('Ctrl Pts',(-18.266416953034,33.916747211356,124.394788919274)) ;
#30368=CARTESIAN_POINT('Ctrl Pts',(-18.4950002778242,33.7367581309931,124.198208384198)) ;
#30369=CARTESIAN_POINT('Ctrl Pts',(-18.1147393757088,33.9266229175737,124.184190734435)) ;
#30370=CARTESIAN_POINT('Ctrl Pts',(-18.3736497561591,33.7466338372108,124.029725816734)) ;
#30371=CARTESIAN_POINT('Ctrl Pts',(-18.0003398463956,33.9366125086737,123.947943873737)) ;
#30372=CARTESIAN_POINT('Ctrl Pts',(-18.2821299057794,33.7566234283109,123.840730774139)) ;
#30373=CARTESIAN_POINT('Ctrl Pts',(-17.9289645288639,33.9465396051291,123.69699206503)) ;
#30374=CARTESIAN_POINT('Ctrl Pts',(-18.2250270203462,33.7665505247663,123.639969543988)) ;
#30375=CARTESIAN_POINT('Ctrl Pts',(-17.9019571311773,33.9565647536337,123.434953214904)) ;
#30376=CARTESIAN_POINT('Ctrl Pts',(-18.2034190100901,33.7765756732709,123.430338874046)) ;
#30377=CARTESIAN_POINT('Ctrl Pts',(-17.920456867938,33.9664604077804,123.175542057052)) ;
#30378=CARTESIAN_POINT('Ctrl Pts',(-18.2182165454262,33.7864713274175,123.222809688118)) ;
#30379=CARTESIAN_POINT('Ctrl Pts',(-17.9840343132116,33.9764639421586,122.920489516577)) ;
#30380=CARTESIAN_POINT('Ctrl Pts',(-18.2690763509193,33.7964748617957,123.018767172028)) ;
#30381=CARTESIAN_POINT('Ctrl Pts',(-18.0907856147797,33.9864490805987,122.680743142477)) ;
#30382=CARTESIAN_POINT('Ctrl Pts',(-18.3544753559251,33.8064600002358,122.826969197833)) ;
#30383=CARTESIAN_POINT('Ctrl Pts',(-18.2384789185145,33.996485005194,122.462260358717)) ;
#30384=CARTESIAN_POINT('Ctrl Pts',(-18.4726280899805,33.8164959248312,122.652181813698)) ;
#30385=CARTESIAN_POINT('Ctrl Pts',(-18.4182776203018,34.0063362806217,122.276005602402)) ;
#30386=CARTESIAN_POINT('Ctrl Pts',(-18.6164655966101,33.8263472002588,122.503176330571)) ;
#30387=CARTESIAN_POINT('Ctrl Pts',(-18.6302489538193,34.0163285417831,122.121008187001)) ;
#30388=CARTESIAN_POINT('Ctrl Pts',(-18.7860413729788,33.8363394614202,122.379176658812)) ;
#30389=CARTESIAN_POINT('Ctrl Pts',(-18.8673098715377,34.0263684258007,122.00522798075)) ;
#30390=CARTESIAN_POINT('Ctrl Pts',(-18.9756890388998,33.8463793454378,122.2865505691)) ;
#30391=CARTESIAN_POINT('Ctrl Pts',(-19.1155543481873,34.0362032003031,121.933213929773)) ;
#30392=CARTESIAN_POINT('Ctrl Pts',(-19.1742842270233,33.8562141199402,122.228937167852)) ;
#30393=CARTESIAN_POINT('Ctrl Pts',(-19.3787606441446,34.0462795813234,121.904625237353)) ;
#30394=CARTESIAN_POINT('Ctrl Pts',(-19.3848492266586,33.8662905009605,122.20606409206)) ;
#30395=CARTESIAN_POINT('Ctrl Pts',(-19.636979964933,34.056125854474,121.921704730838)) ;
#30396=CARTESIAN_POINT('Ctrl Pts',(-19.591423616235,33.8761367741112,122.219725605663)) ;
#30397=CARTESIAN_POINT('Ctrl Pts',(-19.9782262367002,34.0694903757593,122.004738916925)) ;
#30398=CARTESIAN_POINT('Ctrl Pts',(-19.8644290060011,33.8895012953964,122.286150073343)) ;
#30399=CARTESIAN_POINT('Ctrl Pts',(-20.2860725515586,34.0826966201937,122.173341752895)) ;
#30400=CARTESIAN_POINT('Ctrl Pts',(-20.1107333615667,33.9027075398308,122.421054696917)) ;
#30401=CARTESIAN_POINT('Ctrl Pts',(-20.5388137926812,34.0959615748709,122.413398914322)) ;
#30402=CARTESIAN_POINT('Ctrl Pts',(-20.3128900569695,33.9159724945081,122.613069455434)) ;
#30403=CARTESIAN_POINT('Ctrl Pts',(-20.6954462284396,34.1059938554226,122.625471146507)) ;
#30404=CARTESIAN_POINT('Ctrl Pts',(-20.4382052101993,33.9260047750597,122.782731831385)) ;
#30405=CARTESIAN_POINT('Ctrl Pts',(-20.8114438350329,34.1159025889405,122.858591933872)) ;
#30406=CARTESIAN_POINT('Ctrl Pts',(-20.5310032327312,33.9359135085776,122.969226073235)) ;
#30407=CARTESIAN_POINT('Ctrl Pts',(-20.8860726329882,34.125840139808,123.108858926557)) ;
#30408=CARTESIAN_POINT('Ctrl Pts',(-20.5907085395253,33.9458510594451,123.169440598116)) ;
#30409=CARTESIAN_POINT('Ctrl Pts',(-20.9161696354576,34.1358699874019,123.370684085346)) ;
#30410=CARTESIAN_POINT('Ctrl Pts',(-20.6147885800743,33.9558809070391,123.37889723275)) ;
#30411=CARTESIAN_POINT('Ctrl Pts',(-20.8957675550664,34.1491051273224,123.717974610671)) ;
#30412=CARTESIAN_POINT('Ctrl Pts',(-20.5984660541345,33.9691160469595,123.656745092967)) ;
#30413=CARTESIAN_POINT('Ctrl Pts',(-20.7562726268257,34.1657735916935,124.138314956001)) ;
#30414=CARTESIAN_POINT('Ctrl Pts',(-20.4868736501461,33.9857845113307,123.993003032338)) ;
#30415=CARTESIAN_POINT('Ctrl Pts',(-20.4290861791078,34.1856446035674,124.553127465598)) ;
#30416=CARTESIAN_POINT('Ctrl Pts',(-20.2251415375173,34.0056555232046,124.32485414861)) ;
#30417=CARTESIAN_POINT('Ctrl Pts',(-20.0516612997823,34.2023516879504,124.786832185012)) ;
#30418=CARTESIAN_POINT('Ctrl Pts',(-19.9231542599151,34.0223626075875,124.511841034845)) ;
#30419=CARTESIAN_POINT('Ctrl Pts',(-19.7200431655426,34.215528969261,124.88675620924)) ;
#30420=CARTESIAN_POINT('Ctrl Pts',(-19.6579040689418,34.0355398888981,124.591763773494)) ;
#30421=CARTESIAN_POINT('Ctrl Pts',(-19.3739840223207,34.2287964297751,124.92908813568)) ;
#30422=CARTESIAN_POINT('Ctrl Pts',(-19.3810402452549,34.0488073494122,124.625633782971)) ;
#30423=CARTESIAN_POINT('Ctrl Pts',(-18.936720024018,34.2454103204623,124.86755517988)) ;
#30424=CARTESIAN_POINT('Ctrl Pts',(-19.0312400607427,34.0654212400994,124.576410349906)) ;
#30425=CARTESIAN_POINT('Ctrl Pts',(-18.4683529488932,34.2653591198897,124.618947214226)) ;
#30426=CARTESIAN_POINT('Ctrl Pts',(-18.6565409486287,34.0853700395268,124.377526283527)) ;
#30427=CARTESIAN_POINT('Ctrl Pts',(-18.1135823385577,34.2852802314206,124.226010700003)) ;
#30428=CARTESIAN_POINT('Ctrl Pts',(-18.3727229363681,34.1052911510577,124.063178594994)) ;
#30429=CARTESIAN_POINT('Ctrl Pts',(-17.9136663305497,34.3051466795934,123.737213595555)) ;
#30430=CARTESIAN_POINT('Ctrl Pts',(-18.2127872251194,34.1251575992306,123.672140797996)) ;
#30431=CARTESIAN_POINT('Ctrl Pts',(-17.8927069831386,34.3251730262106,123.205416904764)) ;
#30432=CARTESIAN_POINT('Ctrl Pts',(-18.1960174659992,34.1451839458477,123.246703802556)) ;
#30433=CARTESIAN_POINT('Ctrl Pts',(-18.0532950837359,34.3450350706001,122.702439446676)) ;
#30434=CARTESIAN_POINT('Ctrl Pts',(-18.3244861394055,34.1650459902372,122.844319988715)) ;
#30435=CARTESIAN_POINT('Ctrl Pts',(-18.3764719974847,34.3649803732812,122.282323158732)) ;
#30436=CARTESIAN_POINT('Ctrl Pts',(-18.5830265759983,34.1849912929184,122.50822539218)) ;
#30437=CARTESIAN_POINT('Ctrl Pts',(-18.8226102498659,34.3848756803401,121.998446004947)) ;
#30438=CARTESIAN_POINT('Ctrl Pts',(-18.9399371661432,34.2048865999772,122.281121677154)) ;
#30439=CARTESIAN_POINT('Ctrl Pts',(-19.3385786404572,34.4047689505077,121.882935209767)) ;
#30440=CARTESIAN_POINT('Ctrl Pts',(-19.3527127879478,34.2247798701449,122.188711677315)) ;
#30441=CARTESIAN_POINT('Ctrl Pts',(-19.864843872694,34.4247345431882,121.950781567567)) ;
#30442=CARTESIAN_POINT('Ctrl Pts',(-19.773725507496,34.2447454628253,122.242987830082)) ;
#30443=CARTESIAN_POINT('Ctrl Pts',(-20.3344600160615,34.444609866873,122.192739799094)) ;
#30444=CARTESIAN_POINT('Ctrl Pts',(-20.149420050782,34.2646207865101,122.436554544585)) ;
#30445=CARTESIAN_POINT('Ctrl Pts',(-20.6955112754201,34.464584929448,122.582004291072)) ;
#30446=CARTESIAN_POINT('Ctrl Pts',(-20.4382613889304,34.2845958490851,122.74796620737)) ;
#30447=CARTESIAN_POINT('Ctrl Pts',(-20.9010681970121,34.4845373390791,123.070845431308)) ;
#30448=CARTESIAN_POINT('Ctrl Pts',(-20.6027074986626,34.3045482587162,123.139039529433)) ;
#30449=CARTESIAN_POINT('Ctrl Pts',(-20.9283379623324,34.5043733933152,123.597346656962)) ;
#30450=CARTESIAN_POINT('Ctrl Pts',(-20.6245230859658,34.3243843129523,123.560242643287)) ;
#30451=CARTESIAN_POINT('Ctrl Pts',(-20.7737648833637,34.5243513047327,124.105329355223)) ;
#30452=CARTESIAN_POINT('Ctrl Pts',(-20.5008637718727,34.3443622243698,123.966628801619)) ;
#30453=CARTESIAN_POINT('Ctrl Pts',(-20.4555977349369,34.5442693542362,124.528394482397)) ;
#30454=CARTESIAN_POINT('Ctrl Pts',(-20.2463288803223,34.3642802738733,124.305081255519)) ;
#30455=CARTESIAN_POINT('Ctrl Pts',(-20.0139097341758,34.5641374980043,124.818008765311)) ;
#30456=CARTESIAN_POINT('Ctrl Pts',(-19.8929765031619,34.3841484176414,124.536772192443)) ;
#30457=CARTESIAN_POINT('Ctrl Pts',(-19.4952245290992,34.5841883545916,124.939780508264)) ;
#30458=CARTESIAN_POINT('Ctrl Pts',(-19.4780285056584,34.4041992742287,124.634188162972)) ;
#30459=CARTESIAN_POINT('Ctrl Pts',(-18.9729159061863,34.6039687910475,124.878612004196)) ;
#30460=CARTESIAN_POINT('Ctrl Pts',(-19.0601796451305,34.4239797106846,124.585251399659)) ;
#30461=CARTESIAN_POINT('Ctrl Pts',(-18.496759486199,34.6239988467253,124.640786108479)) ;
#30462=CARTESIAN_POINT('Ctrl Pts',(-18.6792557743103,34.4440097663624,124.394988854983)) ;
#30463=CARTESIAN_POINT('Ctrl Pts',(-18.1335792137849,34.6438799519001,124.256847057463)) ;
#30464=CARTESIAN_POINT('Ctrl Pts',(-18.3887122909116,34.4638908715372,124.087835457315)) ;
#30465=CARTESIAN_POINT('Ctrl Pts',(-17.9219139096296,34.6637604142679,123.772762991353)) ;
#30466=CARTESIAN_POINT('Ctrl Pts',(-18.2193820937176,34.483771333905,123.700566231009)) ;
#30467=CARTESIAN_POINT('Ctrl Pts',(-17.8881094855176,34.6837455614122,123.242649910961)) ;
#30468=CARTESIAN_POINT('Ctrl Pts',(-18.1923412744921,34.5037564810494,123.276475501805)) ;
#30469=CARTESIAN_POINT('Ctrl Pts',(-18.0366497415648,34.7036361399486,122.735276316463)) ;
#30470=CARTESIAN_POINT('Ctrl Pts',(-18.3111764212583,34.5236470595857,122.87057664201)) ;
#30471=CARTESIAN_POINT('Ctrl Pts',(-18.3487015779653,34.723530159823,122.308436690887)) ;
#30472=CARTESIAN_POINT('Ctrl Pts',(-18.5608208835814,34.5435410794601,122.529106268789)) ;
#30473=CARTESIAN_POINT('Ctrl Pts',(-18.7881430602527,34.7434516045494,122.013226846896)) ;
#30474=CARTESIAN_POINT('Ctrl Pts',(-18.9123763432651,34.5634625241865,122.292940896369)) ;
#30475=CARTESIAN_POINT('Ctrl Pts',(-19.3013427498124,34.7633497426048,121.884875817397)) ;
#30476=CARTESIAN_POINT('Ctrl Pts',(-19.3229374638322,34.583360662242,122.190263485441)) ;
#30477=CARTESIAN_POINT('Ctrl Pts',(-19.8317538659919,34.7834204978209,121.940822959894)) ;
#30478=CARTESIAN_POINT('Ctrl Pts',(-19.7472655742941,34.603431417458,122.235024637541)) ;
#30479=CARTESIAN_POINT('Ctrl Pts',(-20.3047188071783,34.8032060478722,122.170959918835)) ;
#30480=CARTESIAN_POINT('Ctrl Pts',(-20.1256368670043,34.6232169675093,122.419137989732)) ;
#30481=CARTESIAN_POINT('Ctrl Pts',(-20.6751904640124,34.8231891227495,122.55139832022)) ;
#30482=CARTESIAN_POINT('Ctrl Pts',(-20.4220114541107,34.6432000423866,122.72349136495)) ;
#30483=CARTESIAN_POINT('Ctrl Pts',(-20.8920819873269,34.8430982053954,123.034062768714)) ;
#30484=CARTESIAN_POINT('Ctrl Pts',(-20.5955208682009,34.6631091250326,123.109625335908)) ;
#30485=CARTESIAN_POINT('Ctrl Pts',(-20.9326680570592,34.8629567645182,123.560377307948)) ;
#30486=CARTESIAN_POINT('Ctrl Pts',(-20.6279870568241,34.6829676841553,123.53067592304)) ;
#30487=CARTESIAN_POINT('Ctrl Pts',(-20.7893451366516,34.8830002083569,124.073345382285)) ;
#30488=CARTESIAN_POINT('Ctrl Pts',(-20.5133192229244,34.703011127994,123.941055778839)) ;
#30489=CARTESIAN_POINT('Ctrl Pts',(-20.5344079580577,34.8995002730861,124.43033347796)) ;
#30490=CARTESIAN_POINT('Ctrl Pts',(-20.309383562949,34.7195111927232,124.226623694968)) ;
#30491=CARTESIAN_POINT('Ctrl Pts',(-20.2630356079764,34.912890012935,124.654232063007)) ;
#30492=CARTESIAN_POINT('Ctrl Pts',(-20.0922687245513,34.7329009325721,124.405758721467)) ;
#30493=CARTESIAN_POINT('Ctrl Pts',(-20.0376601532639,34.9227469141434,124.781982024209)) ;
#30494=CARTESIAN_POINT('Ctrl Pts',(-19.911970256192,34.7427578337805,124.507953327853)) ;
#30495=CARTESIAN_POINT('Ctrl Pts',(-19.7904462531825,34.9327384399899,124.870322609915)) ;
#30496=CARTESIAN_POINT('Ctrl Pts',(-19.7141969621559,34.752749359627,124.578624529211)) ;
#30497=CARTESIAN_POINT('Ctrl Pts',(-19.5333148830126,34.9426631204409,124.914209741491)) ;
#30498=CARTESIAN_POINT('Ctrl Pts',(-19.5084940323309,34.762674040078,124.613732529277)) ;
#30499=CARTESIAN_POINT('Ctrl Pts',(-19.2702905171994,34.9526737104853,124.912873328828)) ;
#30500=CARTESIAN_POINT('Ctrl Pts',(-19.2980655576572,34.7726846301224,124.61265864524)) ;
#30501=CARTESIAN_POINT('Ctrl Pts',(-18.9272936377873,34.9659329711889,124.851006430555)) ;
#30502=CARTESIAN_POINT('Ctrl Pts',(-19.0237133047444,34.7859438908261,124.563175229187)) ;
#30503=CARTESIAN_POINT('Ctrl Pts',(-18.606436005865,34.9792840463392,124.69972105366)) ;
#30504=CARTESIAN_POINT('Ctrl Pts',(-18.7669990812473,34.7992949659763,124.442141522519)) ;
#30505=CARTESIAN_POINT('Ctrl Pts',(-18.3413122765646,34.992490355574,124.475665673841)) ;
#30506=CARTESIAN_POINT('Ctrl Pts',(-18.5548921869106,34.8125012752111,124.262885113938)) ;
#30507=CARTESIAN_POINT('Ctrl Pts',(-18.1729444100433,35.0024771891643,124.274406568228)) ;
#30508=CARTESIAN_POINT('Ctrl Pts',(-18.4202016064083,34.8224881088014,124.101878384377)) ;
#30509=CARTESIAN_POINT('Ctrl Pts',(-18.0423683362087,35.0124299166604,124.047733829672)) ;
#30510=CARTESIAN_POINT('Ctrl Pts',(-18.3157421784876,34.8324408362975,123.920538559733)) ;
#30511=CARTESIAN_POINT('Ctrl Pts',(-17.9525123755645,35.022478013502,123.799470169266)) ;
#30512=CARTESIAN_POINT('Ctrl Pts',(-18.2438596889398,34.8424889331391,123.721927081998)) ;
#30513=CARTESIAN_POINT('Ctrl Pts',(-17.9077516294115,35.0323194703738,123.544724476242)) ;
#30514=CARTESIAN_POINT('Ctrl Pts',(-18.208053265257,34.8523303900109,123.518130066413)) ;
#30515=CARTESIAN_POINT('Ctrl Pts',(-17.9073445683786,35.0423057372873,123.282339109367)) ;
#30516=CARTESIAN_POINT('Ctrl Pts',(-18.2077298902901,34.8623166569244,123.308221845002)) ;
#30517=CARTESIAN_POINT('Ctrl Pts',(-17.9521637827218,35.0522423381877,123.025046666914)) ;
#30518=CARTESIAN_POINT('Ctrl Pts',(-18.2435874714704,34.8722532578248,123.10238833231)) ;
#30519=CARTESIAN_POINT('Ctrl Pts',(-18.0420906679866,35.0622922809748,122.776754559742)) ;
#30520=CARTESIAN_POINT('Ctrl Pts',(-18.3155310899466,34.8823032006119,122.903755461618)) ;
#30521=CARTESIAN_POINT('Ctrl Pts',(-18.1709996406622,35.0721424806605,122.552262724124)) ;
#30522=CARTESIAN_POINT('Ctrl Pts',(-18.4186601790438,34.8921534002976,122.724163199285)) ;
#30523=CARTESIAN_POINT('Ctrl Pts',(-18.3384352196694,35.0821153855926,122.350682137594)) ;
#30524=CARTESIAN_POINT('Ctrl Pts',(-18.5526103127129,34.9021263052297,122.562900239816)) ;
#30525=CARTESIAN_POINT('Ctrl Pts',(-18.5389407429953,35.0921137600722,122.180827804113)) ;
#30526=CARTESIAN_POINT('Ctrl Pts',(-18.7130161369838,34.9121246797094,122.427018525397)) ;
#30527=CARTESIAN_POINT('Ctrl Pts',(-18.7664484679922,35.1021339339422,122.048263316574)) ;
#30528=CARTESIAN_POINT('Ctrl Pts',(-18.8950234142683,34.9221448535794,122.320968904354)) ;
#30529=CARTESIAN_POINT('Ctrl Pts',(-19.0105165623716,35.1120349778842,121.958081319082)) ;
#30530=CARTESIAN_POINT('Ctrl Pts',(-19.0902785364057,34.9320458975213,122.24882546228)) ;
#30531=CARTESIAN_POINT('Ctrl Pts',(-19.2687227454526,35.1220237816085,121.910830619248)) ;
#30532=CARTESIAN_POINT('Ctrl Pts',(-19.2968438044793,34.9420347012456,122.211027113215)) ;
#30533=CARTESIAN_POINT('Ctrl Pts',(-19.5305882706686,35.1319892484403,121.909321300949)) ;
#30534=CARTESIAN_POINT('Ctrl Pts',(-19.5063361388599,34.9520001680775,122.209821901071)) ;
#30535=CARTESIAN_POINT('Ctrl Pts',(-19.7872767838356,35.1418928107133,121.952415553993)) ;
#30536=CARTESIAN_POINT('Ctrl Pts',(-19.7116863821234,34.9619037303504,122.244299447509)) ;
#30537=CARTESIAN_POINT('Ctrl Pts',(-20.0363461469721,35.1519534885913,122.040990349835)) ;
#30538=CARTESIAN_POINT('Ctrl Pts',(-19.9109411536517,34.9719644082284,122.315161388044)) ;
#30539=CARTESIAN_POINT('Ctrl Pts',(-20.2614426416287,35.1617937865408,122.168353377903)) ;
#30540=CARTESIAN_POINT('Ctrl Pts',(-20.0910169782063,34.9818047061779,122.417053562184)) ;
#30541=CARTESIAN_POINT('Ctrl Pts',(-20.4656690482286,35.1718567814502,122.33629520841)) ;
#30542=CARTESIAN_POINT('Ctrl Pts',(-20.2543967460004,34.9918677010873,122.551408735198)) ;
#30543=CARTESIAN_POINT('Ctrl Pts',(-20.6346269466373,35.1817510755973,122.533966500745)) ;
#30544=CARTESIAN_POINT('Ctrl Pts',(-20.389561223534,35.0017619952345,122.709546994155)) ;
#30545=CARTESIAN_POINT('Ctrl Pts',(-20.7679099510609,35.1916928732942,122.758634465352)) ;
#30546=CARTESIAN_POINT('Ctrl Pts',(-20.4961856757514,35.0117037929313,122.889282276775)) ;
#30547=CARTESIAN_POINT('Ctrl Pts',(-20.8608365588192,35.2016954508233,123.004554830575)) ;
#30548=CARTESIAN_POINT('Ctrl Pts',(-20.5705249456458,35.0217063704604,123.086019259422)) ;
#30549=CARTESIAN_POINT('Ctrl Pts',(-20.9093992123313,35.2117299147444,123.263726218813)) ;
#30550=CARTESIAN_POINT('Ctrl Pts',(-20.6093729389667,35.0317408343815,123.293356782246)) ;
#30551=CARTESIAN_POINT('Ctrl Pts',(-20.912575954229,35.2215760532655,123.522461220006)) ;
#30552=CARTESIAN_POINT('Ctrl Pts',(-20.6119121959131,35.0415869729026,123.500344358)) ;
#30553=CARTESIAN_POINT('Ctrl Pts',(-20.8707879748683,35.2315572265025,123.781384610257)) ;
#30554=CARTESIAN_POINT('Ctrl Pts',(-20.5784797854132,35.0515681461396,123.707482601004)) ;
#30555=CARTESIAN_POINT('Ctrl Pts',(-20.7848581741263,35.2415095204597,124.028409346698)) ;
#30556=CARTESIAN_POINT('Ctrl Pts',(-20.5097340530019,35.0615204400968,123.905101502577)) ;
#30557=CARTESIAN_POINT('Ctrl Pts',(-20.6570382603351,35.2515083155943,124.258005618651)) ;
#30558=CARTESIAN_POINT('Ctrl Pts',(-20.4074763796465,35.0715192352314,124.088777453895)) ;
#30559=CARTESIAN_POINT('Ctrl Pts',(-20.4902556612724,35.2615474238551,124.462394870675)) ;
#30560=CARTESIAN_POINT('Ctrl Pts',(-20.2740486420064,35.0815583434922,124.252287564926)) ;
#30561=CARTESIAN_POINT('Ctrl Pts',(-20.2951179160963,35.2713723652943,124.631484396849)) ;
#30562=CARTESIAN_POINT('Ctrl Pts',(-20.117937581225,35.0913832849314,124.387557244038)) ;
#30563=CARTESIAN_POINT('Ctrl Pts',(-20.0686559821828,35.2814270523687,124.767580615175)) ;
#30564=CARTESIAN_POINT('Ctrl Pts',(-19.9367669380912,35.1014379720058,124.496432562579)) ;
#30565=CARTESIAN_POINT('Ctrl Pts',(-19.8245654449264,35.2913698573088,124.860825828368)) ;
#30566=CARTESIAN_POINT('Ctrl Pts',(-19.74149402968,35.1113807769459,124.571026731217)) ;
#30567=CARTESIAN_POINT('Ctrl Pts',(-19.5691531625667,35.3012736433053,124.910862029586)) ;
#30568=CARTESIAN_POINT('Ctrl Pts',(-19.5371642509211,35.1212845629424,124.61105371151)) ;
#30569=CARTESIAN_POINT('Ctrl Pts',(-19.3052006854437,35.3113204598701,124.915700617854)) ;
#30570=CARTESIAN_POINT('Ctrl Pts',(-19.3260021502799,35.1313313795072,124.614922626619)) ;
#30571=CARTESIAN_POINT('Ctrl Pts',(-19.0482438728121,35.3212159793488,124.875474923149)) ;
#30572=CARTESIAN_POINT('Ctrl Pts',(-19.1204374586696,35.1412268989859,124.582740243431)) ;
#30573=CARTESIAN_POINT('Ctrl Pts',(-18.7981091918514,35.3312780646732,124.789853312718)) ;
#30574=CARTESIAN_POINT('Ctrl Pts',(-18.9203301991824,35.1512889843104,124.514241085553)) ;
#30575=CARTESIAN_POINT('Ctrl Pts',(-18.571557569673,35.3411207756312,124.664983089902)) ;
#30576=CARTESIAN_POINT('Ctrl Pts',(-18.7390904274587,35.1611316952683,124.4143435761)) ;
#30577=CARTESIAN_POINT('Ctrl Pts',(-18.3667589020139,35.3511114929372,124.500756432804)) ;
#30578=CARTESIAN_POINT('Ctrl Pts',(-18.5752527356648,35.1711224125743,124.282960925271)) ;
#30579=CARTESIAN_POINT('Ctrl Pts',(-18.1946758847601,35.3610395760338,124.304637787655)) ;
#30580=CARTESIAN_POINT('Ctrl Pts',(-18.4375879438694,35.1810504956709,124.126065105729)) ;
#30581=CARTESIAN_POINT('Ctrl Pts',(-18.0580530664321,35.3710275061455,124.080513754998)) ;
#30582=CARTESIAN_POINT('Ctrl Pts',(-18.3282912523427,35.1910384257827,123.946765097769)) ;
#30583=CARTESIAN_POINT('Ctrl Pts',(-17.9623826480587,35.3810633322728,123.83475626619)) ;
#30584=CARTESIAN_POINT('Ctrl Pts',(-18.2517565843422,35.20107425191,123.750158383688)) ;
#30585=CARTESIAN_POINT('Ctrl Pts',(-17.9113535514333,35.3909186693864,123.580830234499)) ;
#30586=CARTESIAN_POINT('Ctrl Pts',(-18.2109351630595,35.2109295890236,123.547017932825)) ;
#30587=CARTESIAN_POINT('Ctrl Pts',(-17.9046862415223,35.4009164042366,123.318213209581)) ;
#30588=CARTESIAN_POINT('Ctrl Pts',(-18.205602992744,35.2209273238737,123.336924392206)) ;
#30589=CARTESIAN_POINT('Ctrl Pts',(-17.9432873405184,35.4108243082211,123.060708970242)) ;
#30590=CARTESIAN_POINT('Ctrl Pts',(-18.2364854316828,35.2308352278582,123.130921769729)) ;
#30591=CARTESIAN_POINT('Ctrl Pts',(-18.0264553068263,35.4208353827695,122.811112169827)) ;
#30592=CARTESIAN_POINT('Ctrl Pts',(-18.3030212907696,35.2408463024066,122.931244865584)) ;
#30593=CARTESIAN_POINT('Ctrl Pts',(-18.1523789389796,35.4308632383051,122.579621476818)) ;
#30594=CARTESIAN_POINT('Ctrl Pts',(-18.403761694324,35.2508741579423,122.746053067434)) ;
#30595=CARTESIAN_POINT('Ctrl Pts',(-18.3134289650525,35.4407208322104,122.376725539727)) ;
#30596=CARTESIAN_POINT('Ctrl Pts',(-18.5326024658146,35.2607317518475,122.583737933796)) ;
#30597=CARTESIAN_POINT('Ctrl Pts',(-18.5102358433116,35.4507475190485,122.201520587918)) ;
#30598=CARTESIAN_POINT('Ctrl Pts',(-18.6900489765213,35.2707584386856,122.443575071446)) ;
#30599=CARTESIAN_POINT('Ctrl Pts',(-18.7348673255698,35.4607761882022,122.063678979707)) ;
#30600=CARTESIAN_POINT('Ctrl Pts',(-18.8697550564223,35.2807871078393,122.333303131403)) ;
#30601=CARTESIAN_POINT('Ctrl Pts',(-18.9753389392073,35.4706213964836,121.968264330612)) ;
#30602=CARTESIAN_POINT('Ctrl Pts',(-19.0621320757983,35.2906323161207,122.256973158654)) ;
#30603=CARTESIAN_POINT('Ctrl Pts',(-19.232344395239,35.4806120854467,121.914585662056)) ;
#30604=CARTESIAN_POINT('Ctrl Pts',(-19.2677365699942,35.3006230050839,122.214031608862)) ;
#30605=CARTESIAN_POINT('Ctrl Pts',(-19.4960145845419,35.490649961729,121.906896220203)) ;
#30606=CARTESIAN_POINT('Ctrl Pts',(-19.4786728720695,35.3106608813661,122.207881552385)) ;
#30607=CARTESIAN_POINT('Ctrl Pts',(-19.7520613231325,35.5004943393712,121.943923950967)) ;
#30608=CARTESIAN_POINT('Ctrl Pts',(-19.6835091319941,35.3205052590084,122.237504996433)) ;
#30609=CARTESIAN_POINT('Ctrl Pts',(-20.0014137029836,35.5104791437627,122.025494346825)) ;
#30610=CARTESIAN_POINT('Ctrl Pts',(-19.8829904412346,35.3304900633998,122.302762488264)) ;
#30611=CARTESIAN_POINT('Ctrl Pts',(-20.2318815338735,35.5204186739812,122.148494733348)) ;
#30612=CARTESIAN_POINT('Ctrl Pts',(-20.0673637209045,35.3404295936183,122.401163717447)) ;
#30613=CARTESIAN_POINT('Ctrl Pts',(-20.4394809697131,35.5304583620181,122.311280393352)) ;
#30614=CARTESIAN_POINT('Ctrl Pts',(-20.2334425657068,35.3504692816552,122.53139333392)) ;
#30615=CARTESIAN_POINT('Ctrl Pts',(-20.6131244207075,35.5403466513864,122.504619288811)) ;
#30616=CARTESIAN_POINT('Ctrl Pts',(-20.3723558935254,35.3603575710235,122.686064744329)) ;
#30617=CARTESIAN_POINT('Ctrl Pts',(-20.7523694041922,35.5503357750712,122.72713725888)) ;
#30618=CARTESIAN_POINT('Ctrl Pts',(-20.4837508097204,35.3703466947083,122.864079588493)) ;
#30619=CARTESIAN_POINT('Ctrl Pts',(-20.8503882560538,35.5602957847458,122.969824688647)) ;
#30620=CARTESIAN_POINT('Ctrl Pts',(-20.5621646481119,35.3803067043829,123.058229659203)) ;
#30621=CARTESIAN_POINT('Ctrl Pts',(-20.9050630989688,35.57019621445,123.224196430447)) ;
#30622=CARTESIAN_POINT('Ctrl Pts',(-20.6059033396929,35.3902071340872,123.261726591413)) ;
#30623=CARTESIAN_POINT('Ctrl Pts',(-20.9148664709882,35.5802392958568,123.487924566708)) ;
#30624=CARTESIAN_POINT('Ctrl Pts',(-20.6137449783066,35.4002502154939,123.472709296187)) ;
#30625=CARTESIAN_POINT('Ctrl Pts',(-20.8792189654738,35.5901466897644,123.74584291802)) ;
#30626=CARTESIAN_POINT('Ctrl Pts',(-20.5852260111583,35.4101576094016,123.679043182914)) ;
#30627=CARTESIAN_POINT('Ctrl Pts',(-20.7989552795368,35.6001584207536,123.996400804876)) ;
#30628=CARTESIAN_POINT('Ctrl Pts',(-20.5210141652758,35.4201693403907,123.879489165425)) ;
#30629=CARTESIAN_POINT('Ctrl Pts',(-20.6756899073301,35.6101906384684,124.229454654533)) ;
#30630=CARTESIAN_POINT('Ctrl Pts',(-20.4224008782605,35.4302015581055,124.065931815006)) ;
#30631=CARTESIAN_POINT('Ctrl Pts',(-20.5170202759795,35.6200431477146,124.434034154075)) ;
#30632=CARTESIAN_POINT('Ctrl Pts',(-20.2954650100176,35.4400540673517,124.229594006282)) ;
#30633=CARTESIAN_POINT('Ctrl Pts',(-20.3237177193579,35.6300010842576,124.610433802406)) ;
#30634=CARTESIAN_POINT('Ctrl Pts',(-20.1408227029007,35.4500120038947,124.370712879431)) ;
#30635=CARTESIAN_POINT('Ctrl Pts',(-20.1006943914862,35.6400399542659,124.751315017522)) ;
#30636=CARTESIAN_POINT('Ctrl Pts',(-19.9624034408403,35.460050873903,124.483417150071)) ;
#30637=CARTESIAN_POINT('Ctrl Pts',(-19.8607559657353,35.6499131094241,124.850152762012)) ;
#30638=CARTESIAN_POINT('Ctrl Pts',(-19.7704532300316,35.4699240290612,124.562486266306)) ;
#30639=CARTESIAN_POINT('Ctrl Pts',(-19.6022411196816,35.6599863842738,124.906856510779)) ;
#30640=CARTESIAN_POINT('Ctrl Pts',(-19.5636408438425,35.4799973039109,124.607848540031)) ;
#30641=CARTESIAN_POINT('Ctrl Pts',(-19.3443505908473,35.6698067014512,124.917880380727)) ;
#30642=CARTESIAN_POINT('Ctrl Pts',(-19.3573296329594,35.4898176210883,124.616666850261)) ;
#30643=CARTESIAN_POINT('Ctrl Pts',(-19.0818227174019,35.6798853872447,124.883323751729)) ;
#30644=CARTESIAN_POINT('Ctrl Pts',(-19.147307048226,35.4998963068818,124.589020826947)) ;
#30645=CARTESIAN_POINT('Ctrl Pts',(-18.8348266453424,35.6897368986278,124.805553629414)) ;
#30646=CARTESIAN_POINT('Ctrl Pts',(-18.9497113939592,35.5097478182649,124.526804423587)) ;
#30647=CARTESIAN_POINT('Ctrl Pts',(-18.5999081950905,35.6998103449344,124.683638544709)) ;
#30648=CARTESIAN_POINT('Ctrl Pts',(-18.7617765978972,35.5198212645716,124.429271661873)) ;
#30649=CARTESIAN_POINT('Ctrl Pts',(-18.3945197612094,35.7096516200591,124.526430434708)) ;
#30650=CARTESIAN_POINT('Ctrl Pts',(-18.5974671222276,35.5296625396963,124.303505384468)) ;
#30651=CARTESIAN_POINT('Ctrl Pts',(-18.2164254320828,35.7196367197159,124.333759479541)) ;
#30652=CARTESIAN_POINT('Ctrl Pts',(-18.4549921099954,35.539647639353,124.149368519473)) ;
#30653=CARTESIAN_POINT('Ctrl Pts',(-18.0744564633631,35.7296441958502,124.112362113073)) ;
#30654=CARTESIAN_POINT('Ctrl Pts',(-18.3414173794509,35.5496551154873,123.972250409102)) ;
#30655=CARTESIAN_POINT('Ctrl Pts',(-17.9737377684653,35.7395667835592,123.871857563518)) ;
#30656=CARTESIAN_POINT('Ctrl Pts',(-18.2608430645821,35.5595777031963,123.779847173338)) ;
#30657=CARTESIAN_POINT('Ctrl Pts',(-17.915514233427,35.7495533878325,123.61593526692)) ;
#30658=CARTESIAN_POINT('Ctrl Pts',(-18.2142645957526,35.5695643074696,123.575109448264)) ;
#30659=CARTESIAN_POINT('Ctrl Pts',(-17.9030386020177,35.7595935161666,123.352407710946)) ;
#30660=CARTESIAN_POINT('Ctrl Pts',(-18.2042845372192,35.5796044358037,123.364287232758)) ;
#30661=CARTESIAN_POINT('Ctrl Pts',(-17.9352873093838,35.7694329507,123.095829361004)) ;
#30662=CARTESIAN_POINT('Ctrl Pts',(-18.2300836623065,35.5894438703371,123.159025769629)) ;
#30663=CARTESIAN_POINT('Ctrl Pts',(-18.0131110083021,35.779497005191,122.843100123072)) ;
#30664=CARTESIAN_POINT('Ctrl Pts',(-18.2923429533616,35.5995079248281,122.956842160068)) ;
#30665=CARTESIAN_POINT('Ctrl Pts',(-18.1316925352344,35.7893879244282,122.611771524711)) ;
#30666=CARTESIAN_POINT('Ctrl Pts',(-18.3872080467958,35.6093988440653,122.771780155463)) ;
#30667=CARTESIAN_POINT('Ctrl Pts',(-18.2897713917017,35.7993799177342,122.402124132987)) ;
#30668=CARTESIAN_POINT('Ctrl Pts',(-18.5136711422251,35.6193908373713,122.604062465028)) ;
#30669=CARTESIAN_POINT('Ctrl Pts',(-18.4814613118421,35.8093427816935,122.223804692162)) ;
#30670=CARTESIAN_POINT('Ctrl Pts',(-18.6670229513666,35.6293537013306,122.461407311499)) ;
#30671=CARTESIAN_POINT('Ctrl Pts',(-18.6995746479886,35.8192470415113,122.081746101379)) ;
#30672=CARTESIAN_POINT('Ctrl Pts',(-18.8415130103748,35.6392579611484,122.347760879673)) ;
#30673=CARTESIAN_POINT('Ctrl Pts',(-18.9428567780933,35.8293075320827,121.978340523878)) ;
#30674=CARTESIAN_POINT('Ctrl Pts',(-19.0361390123414,35.6493184517198,122.265036395034)) ;
#30675=CARTESIAN_POINT('Ctrl Pts',(-19.1947540652062,35.8391478817137,121.919707183759)) ;
#30676=CARTESIAN_POINT('Ctrl Pts',(-19.2376556973774,35.6591588013508,122.218129998438)) ;
#30677=CARTESIAN_POINT('Ctrl Pts',(-19.4587582959314,35.8492108572037,121.905070980687)) ;
#30678=CARTESIAN_POINT('Ctrl Pts',(-19.448859376931,35.6692217768408,122.206420948279)) ;
#30679=CARTESIAN_POINT('Ctrl Pts',(-19.716930430725,35.8591051773471,121.936190237955)) ;
#30680=CARTESIAN_POINT('Ctrl Pts',(-19.6553962747645,35.6791160969842,122.231316240817)) ;
#30681=CARTESIAN_POINT('Ctrl Pts',(-19.9671129941824,35.8690468904787,122.011332156098)) ;
#30682=CARTESIAN_POINT('Ctrl Pts',(-19.8555418925478,35.6890578101158,122.291429441969)) ;
#30683=CARTESIAN_POINT('Ctrl Pts',(-20.2020024297301,35.8790497802728,122.129427167199)) ;
#30684=CARTESIAN_POINT('Ctrl Pts',(-20.0434534559638,35.69906069991,122.385905206129)) ;
#30685=CARTESIAN_POINT('Ctrl Pts',(-20.4132559197395,35.8890896374333,122.28744132461)) ;
#30686=CARTESIAN_POINT('Ctrl Pts',(-20.2124564260292,35.7091005570704,122.512316537818)) ;
#30687=CARTESIAN_POINT('Ctrl Pts',(-20.5904446049363,35.8989138182709,122.475235422024)) ;
#30688=CARTESIAN_POINT('Ctrl Pts',(-20.3542066813593,35.7189247379081,122.662550716544)) ;
#30689=CARTESIAN_POINT('Ctrl Pts',(-20.7359772784035,35.9089707917741,122.695816923843)) ;
#30690=CARTESIAN_POINT('Ctrl Pts',(-20.4706332561571,35.7289817114113,122.839015952767)) ;
#30691=CARTESIAN_POINT('Ctrl Pts',(-20.8393638309279,35.9188989159612,122.935375322683)) ;
#30692=CARTESIAN_POINT('Ctrl Pts',(-20.5533424999389,35.7389098355983,123.030662030176)) ;
#30693=CARTESIAN_POINT('Ctrl Pts',(-20.9004170383969,35.9288526110346,123.189725205683)) ;
#30694=CARTESIAN_POINT('Ctrl Pts',(-20.602185386523,35.7488635306717,123.234141416124)) ;
#30695=CARTESIAN_POINT('Ctrl Pts',(-20.9161514803797,35.9388988046099,123.453256665995)) ;
#30696=CARTESIAN_POINT('Ctrl Pts',(-20.6147732911417,35.758909724247,123.444966757205)) ;
#30697=CARTESIAN_POINT('Ctrl Pts',(-20.8867329496708,35.9487469069698,123.710376268567)) ;
#30698=CARTESIAN_POINT('Ctrl Pts',(-20.5912389928801,35.7687578266069,123.650661374287)) ;
#30699=CARTESIAN_POINT('Ctrl Pts',(-20.813048468652,35.9587084951974,123.961560575043)) ;
#30700=CARTESIAN_POINT('Ctrl Pts',(-20.5322920915651,35.7787194148345,123.851608640381)) ;
#30701=CARTESIAN_POINT('Ctrl Pts',(-20.6957786698797,35.9687371653537,124.19759210035)) ;
#30702=CARTESIAN_POINT('Ctrl Pts',(-20.4384766850489,35.7887480849908,124.04043416191)) ;
#30703=CARTESIAN_POINT('Ctrl Pts',(-20.5412377893036,35.9786474682354,124.407201312219)) ;
#30704=CARTESIAN_POINT('Ctrl Pts',(-20.3148448330596,35.7986583878725,124.208121289199)) ;
#30705=CARTESIAN_POINT('Ctrl Pts',(-20.3526398125085,35.9885823520433,124.587747365873)) ;
#30706=CARTESIAN_POINT('Ctrl Pts',(-20.1639673252218,35.8085932716804,124.352558280755)) ;
#30707=CARTESIAN_POINT('Ctrl Pts',(-20.1331135059456,35.9986234937339,124.734141809642)) ;
#30708=CARTESIAN_POINT('Ctrl Pts',(-19.9883465163358,35.8186344133711,124.469674459931)) ;
#30709=CARTESIAN_POINT('Ctrl Pts',(-19.8952608881985,36.0085106148979,124.838745840386)) ;
#30710=CARTESIAN_POINT('Ctrl Pts',(-19.7980654626942,35.828521534535,124.553357985807)) ;
#30711=CARTESIAN_POINT('Ctrl Pts',(-19.6403085962477,36.0185029577464,124.901535971408)) ;
#30712=CARTESIAN_POINT('Ctrl Pts',(-19.5941039789621,35.8385138773836,124.603590829665)) ;
#30713=CARTESIAN_POINT('Ctrl Pts',(-19.3794454821469,36.0284512589704,124.918954868183)) ;
#30714=CARTESIAN_POINT('Ctrl Pts',(-19.3854139711554,35.8484621786075,124.617526697189)) ;
#30715=CARTESIAN_POINT('Ctrl Pts',(-19.1197882532334,36.0383888366525,124.8912260194)) ;
#30716=CARTESIAN_POINT('Ctrl Pts',(-19.1776886066464,35.8583997562896,124.595344542413)) ;
#30717=CARTESIAN_POINT('Ctrl Pts',(-18.8675463523897,36.0483754111031,124.818724120264)) ;
#30718=CARTESIAN_POINT('Ctrl Pts',(-18.9758950062236,35.8683863307402,124.537343974835)) ;
#30719=CARTESIAN_POINT('Ctrl Pts',(-18.6308789216368,36.0584042210115,124.702775017872)) ;
#30720=CARTESIAN_POINT('Ctrl Pts',(-18.7865606156517,35.8784151406487,124.444585433762)) ;
#30721=CARTESIAN_POINT('Ctrl Pts',(-18.4209855121877,36.0682825423183,124.550028242115)) ;
#30722=CARTESIAN_POINT('Ctrl Pts',(-18.6186460335251,35.8882934619554,124.322389261554)) ;
#30723=CARTESIAN_POINT('Ctrl Pts',(-18.2382837456184,36.0782741896657,124.361434085726)) ;
#30724=CARTESIAN_POINT('Ctrl Pts',(-18.4724839618908,35.8982851093029,124.17151478619)) ;
#30725=CARTESIAN_POINT('Ctrl Pts',(-18.0909304837619,36.0883087131035,124.142763989122)) ;
#30726=CARTESIAN_POINT('Ctrl Pts',(-18.3546005264068,35.9083196327406,123.996579163665)) ;
#30727=CARTESIAN_POINT('Ctrl Pts',(-17.9851026047473,36.0981720699821,123.906123266323)) ;
#30728=CARTESIAN_POINT('Ctrl Pts',(-18.2699376258738,35.9181829896192,123.807267861114)) ;
#30729=CARTESIAN_POINT('Ctrl Pts',(-17.9206102595099,36.1082422966624,123.649496524002)) ;
#30730=CARTESIAN_POINT('Ctrl Pts',(-18.2183426310434,35.9282532162995,123.601966434206)) ;
#30731=CARTESIAN_POINT('Ctrl Pts',(-17.9020958099089,36.1180846047971,123.391502808904)) ;
#30732=CARTESIAN_POINT('Ctrl Pts',(-18.2035300751442,35.9380955244342,123.39557257472)) ;
#30733=CARTESIAN_POINT('Ctrl Pts',(-17.9280157514707,36.1280453368205,123.131037798645)) ;
#30734=CARTESIAN_POINT('Ctrl Pts',(-18.2242647137395,35.9480562564576,123.187200762251)) ;
#30735=CARTESIAN_POINT('Ctrl Pts',(-17.999816726095,36.1380832260186,122.877221984986)) ;
#30736=CARTESIAN_POINT('Ctrl Pts',(-18.2817043938246,35.9580941456557,122.984147689638)) ;
#30737=CARTESIAN_POINT('Ctrl Pts',(-18.1123123668843,36.1479575089374,122.643353698666)) ;
#30738=CARTESIAN_POINT('Ctrl Pts',(-18.3716994042814,35.9679684285746,122.797053236207)) ;
#30739=CARTESIAN_POINT('Ctrl Pts',(-18.2666755578384,36.1580272535549,122.428462610188)) ;
#30740=CARTESIAN_POINT('Ctrl Pts',(-18.4951890841048,35.978038173192,122.625139394901)) ;
#30741=CARTESIAN_POINT('Ctrl Pts',(-18.4515040641022,36.1678605639005,122.247839904849)) ;
#30742=CARTESIAN_POINT('Ctrl Pts',(-18.6430502466827,35.9878714835377,122.480641013743)) ;
#30743=CARTESIAN_POINT('Ctrl Pts',(-18.6687131962433,36.1778908072532,122.098528505516)) ;
#30744=CARTESIAN_POINT('Ctrl Pts',(-18.8168167817684,35.9979017268903,122.361190651918)) ;
#30745=CARTESIAN_POINT('Ctrl Pts',(-18.9089342117129,36.1879230952316,121.98989079608)) ;
#30746=CARTESIAN_POINT('Ctrl Pts',(-19.0089931242432,36.0079340148687,122.274279275505)) ;
#30747=CARTESIAN_POINT('Ctrl Pts',(-19.1589917224903,36.1977502716997,121.925355327248)) ;
#30748=CARTESIAN_POINT('Ctrl Pts',(-19.2090377774814,36.0177611913368,122.222649778263)) ;
#30749=CARTESIAN_POINT('Ctrl Pts',(-19.4210472098018,36.2077556545666,121.904313326992)) ;
#30750=CARTESIAN_POINT('Ctrl Pts',(-19.4186819756106,36.0277665742037,122.205814653997)) ;
#30751=CARTESIAN_POINT('Ctrl Pts',(-19.6822546897857,36.2177382935593,121.929130110005)) ;
#30752=CARTESIAN_POINT('Ctrl Pts',(-19.6276479311042,36.0377492131964,122.225666559862)) ;
#30753=CARTESIAN_POINT('Ctrl Pts',(-19.9365810271852,36.2277823606959,121.999644910744)) ;
#30754=CARTESIAN_POINT('Ctrl Pts',(-19.8311095076827,36.047793280333,122.282077034315)) ;
#30755=CARTESIAN_POINT('Ctrl Pts',(-20.1697398906336,36.2376035794999,122.110337795579)) ;
#30756=CARTESIAN_POINT('Ctrl Pts',(-20.0176363566891,36.057614499137,122.370629526365)) ;
#30757=CARTESIAN_POINT('Ctrl Pts',(-20.3851350977547,36.247640418438,122.262557053081)) ;
#30758=CARTESIAN_POINT('Ctrl Pts',(-20.1899535516625,36.0676513380751,122.492403621598)) ;
#30759=CARTESIAN_POINT('Ctrl Pts',(-20.5700735002195,36.2576648305357,122.450169309994)) ;
#30760=CARTESIAN_POINT('Ctrl Pts',(-20.3379053729967,36.0776757501728,122.64249237106)) ;
#30761=CARTESIAN_POINT('Ctrl Pts',(-20.7175254012894,36.267516914941,122.662985785925)) ;
#30762=CARTESIAN_POINT('Ctrl Pts',(-20.4558677751605,36.0875278345781,122.812743960038)) ;
#30763=CARTESIAN_POINT('Ctrl Pts',(-20.827658912847,36.2775078116842,122.901285416374)) ;
#30764=CARTESIAN_POINT('Ctrl Pts',(-20.5439760743343,36.0975187313213,123.003382825012)) ;
#30765=CARTESIAN_POINT('Ctrl Pts',(-20.894433698142,36.2874258035851,123.153253367672)) ;
#30766=CARTESIAN_POINT('Ctrl Pts',(-20.597397457909,36.1074367232222,123.204956301286)) ;
#30767=CARTESIAN_POINT('Ctrl Pts',(-20.9167470714456,36.2974539190421,123.415814568147)) ;
#30768=CARTESIAN_POINT('Ctrl Pts',(-20.6152498951296,36.1174648386792,123.415005141595)) ;
#30769=CARTESIAN_POINT('Ctrl Pts',(-20.8935762347595,36.3073390949842,123.674557784478)) ;
#30770=CARTESIAN_POINT('Ctrl Pts',(-20.5967150310461,36.1273500146213,123.621999285867)) ;
#30771=CARTESIAN_POINT('Ctrl Pts',(-20.8257335492576,36.3173284533911,123.928155184694)) ;
#30772=CARTESIAN_POINT('Ctrl Pts',(-20.5424427145472,36.1373393730282,123.824877566207)) ;
#30773=CARTESIAN_POINT('Ctrl Pts',(-20.7138111338408,36.3273696009714,124.167113009814)) ;
#30774=CARTESIAN_POINT('Ctrl Pts',(-20.4529063575782,36.1473805206085,124.016044644643)) ;
#30775=CARTESIAN_POINT('Ctrl Pts',(-20.5656005075822,36.3372022239778,124.378768633685)) ;
#30776=CARTESIAN_POINT('Ctrl Pts',(-20.334339803994,36.157213143615,124.185369574841)) ;
#30777=CARTESIAN_POINT('Ctrl Pts',(-20.3804184420739,36.3471962950886,124.564996698335)) ;
#30778=CARTESIAN_POINT('Ctrl Pts',(-20.1861956033881,36.1672072147257,124.334353335145)) ;
#30779=CARTESIAN_POINT('Ctrl Pts',(-20.1646550508293,36.3572249527295,124.716351716207)) ;
#30780=CARTESIAN_POINT('Ctrl Pts',(-20.013585958757,36.1772358723666,124.455438891468)) ;
#30781=CARTESIAN_POINT('Ctrl Pts',(-19.9294697798766,36.3671092789223,124.82658534845)) ;
#30782=CARTESIAN_POINT('Ctrl Pts',(-19.8254390212486,36.1871201985594,124.543627316612)) ;
#30783=CARTESIAN_POINT('Ctrl Pts',(-19.6767994745705,36.3770750224129,124.895495364823)) ;
#30784=CARTESIAN_POINT('Ctrl Pts',(-19.6233034862338,36.19708594205,124.598757213134)) ;
#30785=CARTESIAN_POINT('Ctrl Pts',(-19.4143489319624,36.3871034015441,124.91925636217)) ;
#30786=CARTESIAN_POINT('Ctrl Pts',(-19.4133432160735,36.2071143211812,124.617767958243)) ;
#30787=CARTESIAN_POINT('Ctrl Pts',(-19.1550206095445,36.397004247751,124.897758003346)) ;
#30788=CARTESIAN_POINT('Ctrl Pts',(-19.2058807986506,36.2170151673881,124.600571300824)) ;
#30789=CARTESIAN_POINT('Ctrl Pts',(-18.8994442732755,36.4070629051681,124.830453416065)) ;
#30790=CARTESIAN_POINT('Ctrl Pts',(-19.0014191286445,36.2270738248052,124.546729537339)) ;
#30791=CARTESIAN_POINT('Ctrl Pts',(-18.6640416210879,36.41692046795,124.722218749263)) ;
#30792=CARTESIAN_POINT('Ctrl Pts',(-18.8130966335472,36.2369313875871,124.460143863879)) ;
#30793=CARTESIAN_POINT('Ctrl Pts',(-18.4464240794683,36.4269888705032,124.571792635111)) ;
#30794=CARTESIAN_POINT('Ctrl Pts',(-18.6390013333269,36.2469997901403,124.339804589422)) ;
#30795=CARTESIAN_POINT('Ctrl Pts',(-18.2621870024575,36.4368442692428,124.389737932051)) ;
#30796=CARTESIAN_POINT('Ctrl Pts',(-18.4916105893428,36.2568551888799,124.194162632583)) ;
#30797=CARTESIAN_POINT('Ctrl Pts',(-18.1096139658518,36.4468391363167,124.175952224907)) ;
#30798=CARTESIAN_POINT('Ctrl Pts',(-18.3695504720034,36.2668500559538,124.023135369185)) ;
#30799=CARTESIAN_POINT('Ctrl Pts',(-17.9965739248701,36.4568704313002,123.937801266144)) ;
#30800=CARTESIAN_POINT('Ctrl Pts',(-18.2791165693549,36.2768813509373,123.832615491336)) ;
#30801=CARTESIAN_POINT('Ctrl Pts',(-17.9273507223424,36.4667369560267,123.68792118455)) ;
#30802=CARTESIAN_POINT('Ctrl Pts',(-18.2237360813941,36.2867478756638,123.632712386933)) ;
#30803=CARTESIAN_POINT('Ctrl Pts',(-17.9018470654154,36.4767244267224,123.426734881173)) ;
#30804=CARTESIAN_POINT('Ctrl Pts',(-18.2033310225224,36.2967353463596,123.423763651116)) ;
#30805=CARTESIAN_POINT('Ctrl Pts',(-17.9218551058738,36.4866691862863,123.166123729046)) ;
#30806=CARTESIAN_POINT('Ctrl Pts',(-18.2193352864995,36.3066801059234,123.215274750521)) ;
#30807=CARTESIAN_POINT('Ctrl Pts',(-17.9876098911621,36.4967147422351,122.910487765929)) ;
#30808=CARTESIAN_POINT('Ctrl Pts',(-18.2719370358106,36.3167256618723,123.010765429301)) ;
#30809=CARTESIAN_POINT('Ctrl Pts',(-18.0945065089563,36.5065743306102,122.674433491217)) ;
#30810=CARTESIAN_POINT('Ctrl Pts',(-18.3574522130804,36.3265852502474,122.821921426848)) ;
#30811=CARTESIAN_POINT('Ctrl Pts',(-18.2424940102238,36.5165752857463,122.457296954355)) ;
#30812=CARTESIAN_POINT('Ctrl Pts',(-18.4758403558108,36.3365862053834,122.648211013651)) ;
#30813=CARTESIAN_POINT('Ctrl Pts',(-18.4240741922966,36.5264795130239,122.270772500049)) ;
#30814=CARTESIAN_POINT('Ctrl Pts',(-18.6211027732019,36.346490432661,122.498990059894)) ;
#30815=CARTESIAN_POINT('Ctrl Pts',(-18.6381179777294,36.536521589919,122.116476705951)) ;
#30816=CARTESIAN_POINT('Ctrl Pts',(-18.7923365002083,36.3565325095561,122.375551632485)) ;
#30817=CARTESIAN_POINT('Ctrl Pts',(-18.8725385168482,36.5464292026052,122.003075302597)) ;
#30818=CARTESIAN_POINT('Ctrl Pts',(-18.979871801407,36.3664401222423,122.284828592145)) ;
#30819=CARTESIAN_POINT('Ctrl Pts',(-19.1267156102874,36.5564837332209,121.931052177972)) ;
#30820=CARTESIAN_POINT('Ctrl Pts',(-19.1832128661274,36.376494652858,122.227207955336)) ;
#30821=CARTESIAN_POINT('Ctrl Pts',(-19.3845283469667,36.5663445197698,121.904614760594)) ;
#30822=CARTESIAN_POINT('Ctrl Pts',(-19.3894626144026,36.3863554394069,122.206055828326)) ;
#30823=CARTESIAN_POINT('Ctrl Pts',(-19.646459660601,36.5763382748409,121.923105823683)) ;
#30824=CARTESIAN_POINT('Ctrl Pts',(-19.5990077631151,36.396349194478,122.220846431411)) ;
#30825=CARTESIAN_POINT('Ctrl Pts',(-19.8995693751158,36.5862636350808,121.986256533974)) ;
#30826=CARTESIAN_POINT('Ctrl Pts',(-19.8014959764349,36.406274554718,122.271364795615)) ;
#30827=CARTESIAN_POINT('Ctrl Pts',(-20.1402663825485,36.5962915644761,122.093453651258)) ;
#30828=CARTESIAN_POINT('Ctrl Pts',(-19.9940544515842,36.4163024841132,122.357120413461)) ;
#30829=CARTESIAN_POINT('Ctrl Pts',(-20.3558196617263,36.6061778312754,122.23855197328)) ;
#30830=CARTESIAN_POINT('Ctrl Pts',(-20.1664982539507,36.4261887509125,122.473197150911)) ;
#30831=CARTESIAN_POINT('Ctrl Pts',(-20.5456928031172,36.6162096001737,122.421371062193)) ;
#30832=CARTESIAN_POINT('Ctrl Pts',(-20.3183982921077,36.4362205198108,122.619450762827)) ;
#30833=CARTESIAN_POINT('Ctrl Pts',(-20.6988722845905,36.6260911960173,122.631115950227)) ;
#30834=CARTESIAN_POINT('Ctrl Pts',(-20.4409436684768,36.4461021156544,122.787245289088)) ;
#30835=CARTESIAN_POINT('Ctrl Pts',(-20.815415738362,36.6361530814852,122.868418182703)) ;
#30836=CARTESIAN_POINT('Ctrl Pts',(-20.5341804158425,36.4561640011224,122.97708607685)) ;
#30837=CARTESIAN_POINT('Ctrl Pts',(-20.8875930298801,36.6460105155041,123.11723735423)) ;
#30838=CARTESIAN_POINT('Ctrl Pts',(-20.5919244479909,36.4660214351412,123.176140562993)) ;
#30839=CARTESIAN_POINT('Ctrl Pts',(-20.9163988743177,36.6560037585461,123.37823043788)) ;
#30840=CARTESIAN_POINT('Ctrl Pts',(-20.6149712081136,36.4760146781832,123.384935555596)) ;
#30841=CARTESIAN_POINT('Ctrl Pts',(-20.8995719078508,36.6659345194324,123.638673612031)) ;
#30842=CARTESIAN_POINT('Ctrl Pts',(-20.6015124065235,36.4859454390695,123.593287223642)) ;
#30843=CARTESIAN_POINT('Ctrl Pts',(-20.8168446966216,36.6792835116296,123.979609103864)) ;
#30844=CARTESIAN_POINT('Ctrl Pts',(-20.535330876497,36.4992944312667,123.866051291918)) ;
#30845=CARTESIAN_POINT('Ctrl Pts',(-20.6476556408436,36.692551884446,124.288994177467)) ;
#30846=CARTESIAN_POINT('Ctrl Pts',(-20.3999608846557,36.5125628040832,124.113578703363)) ;
#30847=CARTESIAN_POINT('Ctrl Pts',(-20.4070652076398,36.7058348258304,124.541941671544)) ;
#30848=CARTESIAN_POINT('Ctrl Pts',(-20.2075187930554,36.5258457454675,124.31590241707)) ;
#30849=CARTESIAN_POINT('Ctrl Pts',(-20.1946380684897,36.7158776116726,124.698516250031)) ;
#30850=CARTESIAN_POINT('Ctrl Pts',(-20.0375727496872,36.5358885313097,124.441171067068)) ;
#30851=CARTESIAN_POINT('Ctrl Pts',(-19.9628921814832,36.7257275542247,124.813842499232)) ;
#30852=CARTESIAN_POINT('Ctrl Pts',(-19.8521787603597,36.5457384738618,124.53343231864)) ;
#30853=CARTESIAN_POINT('Ctrl Pts',(-19.7111366687982,36.7357247871437,124.888900023742)) ;
#30854=CARTESIAN_POINT('Ctrl Pts',(-19.6507730800588,36.5557357067808,124.593480421543)) ;
#30855=CARTESIAN_POINT('Ctrl Pts',(-19.4496388355441,36.7457396824782,124.918754107173)) ;
#30856=CARTESIAN_POINT('Ctrl Pts',(-19.4415808798337,36.5657506021153,124.617367625246)) ;
#30857=CARTESIAN_POINT('Ctrl Pts',(-19.1023419164485,36.7589793591164,124.897941856105)) ;
#30858=CARTESIAN_POINT('Ctrl Pts',(-19.163714991499,36.5789902787535,124.600711280948)) ;
#30859=CARTESIAN_POINT('Ctrl Pts',(-18.6847931249913,36.7755265835217,124.759912521952)) ;
#30860=CARTESIAN_POINT('Ctrl Pts',(-18.8297169408902,36.5955375031589,124.490312244877)) ;
#30861=CARTESIAN_POINT('Ctrl Pts',(-18.3371603330514,36.7921740206528,124.486198909286)) ;
#30862=CARTESIAN_POINT('Ctrl Pts',(-18.5515569759396,36.6121849402899,124.27129948126)) ;
#30863=CARTESIAN_POINT('Ctrl Pts',(-18.1282776888068,36.805463518131,124.206288377136)) ;
#30864=CARTESIAN_POINT('Ctrl Pts',(-18.3844875071243,36.6254744377682,124.047410080626)) ;
#30865=CARTESIAN_POINT('Ctrl Pts',(-18.0108710102114,36.8153369259534,123.974907927257)) ;
#30866=CARTESIAN_POINT('Ctrl Pts',(-18.2905523869042,36.6353478455905,123.86229865506)) ;
#30867=CARTESIAN_POINT('Ctrl Pts',(-17.9340138084422,36.8253893035461,123.722181735766)) ;
#30868=CARTESIAN_POINT('Ctrl Pts',(-18.2290667220401,36.6454002231832,123.660120782758)) ;
#30869=CARTESIAN_POINT('Ctrl Pts',(-17.9027830695279,36.835292957087,123.463785283055)) ;
#30870=CARTESIAN_POINT('Ctrl Pts',(-18.2040801107792,36.6553038767241,123.453402008484)) ;
#30871=CARTESIAN_POINT('Ctrl Pts',(-17.9163185741068,36.8452372260823,123.20284412538)) ;
#30872=CARTESIAN_POINT('Ctrl Pts',(-18.2149045717325,36.6652481457194,123.244652494399)) ;
#30873=CARTESIAN_POINT('Ctrl Pts',(-17.9947816309639,36.858568234415,122.86134409118)) ;
#30874=CARTESIAN_POINT('Ctrl Pts',(-18.2776833949051,36.6785791540521,122.971434015951)) ;
#30875=CARTESIAN_POINT('Ctrl Pts',(-18.2021201495934,36.8751898149393,122.471324046481)) ;
#30876=CARTESIAN_POINT('Ctrl Pts',(-18.4435276248863,36.6952007345764,122.65944458022)) ;
#30877=CARTESIAN_POINT('Ctrl Pts',(-18.5280140338344,36.8917324856377,122.176159129624)) ;
#30878=CARTESIAN_POINT('Ctrl Pts',(-18.7042903718315,36.7117434052748,122.423272175924)) ;
#30879=CARTESIAN_POINT('Ctrl Pts',(-18.8400831149496,36.9050816452006,122.015936356967)) ;
#30880=CARTESIAN_POINT('Ctrl Pts',(-18.9539021452591,36.7250925648377,122.295120890868)) ;
#30881=CARTESIAN_POINT('Ctrl Pts',(-19.1721122727388,36.9183097953601,121.912858361427)) ;
#30882=CARTESIAN_POINT('Ctrl Pts',(-19.2195445013812,36.7383207149972,122.212649893044)) ;
#30883=CARTESIAN_POINT('Ctrl Pts',(-19.6137036972869,36.9349404724976,121.895030598863)) ;
#30884=CARTESIAN_POINT('Ctrl Pts',(-19.5728023332913,36.7549513921347,122.198387296976)) ;
#30885=CARTESIAN_POINT('Ctrl Pts',(-20.1178689307979,36.9548434117857,122.055389405996)) ;
#30886=CARTESIAN_POINT('Ctrl Pts',(-19.9761410205625,36.7748543314228,122.326670629609)) ;
#30887=CARTESIAN_POINT('Ctrl Pts',(-20.5372508618261,36.974746278389,122.377628584719)) ;
#30888=CARTESIAN_POINT('Ctrl Pts',(-20.3116476493232,36.7947571980261,122.584460225814)) ;
#30889=CARTESIAN_POINT('Ctrl Pts',(-20.8224429652518,36.9946594434938,122.823616943194)) ;
#30890=CARTESIAN_POINT('Ctrl Pts',(-20.5398042577158,36.8146703631309,122.941249965246)) ;
#30891=CARTESIAN_POINT('Ctrl Pts',(-20.9381837029395,37.0146952726351,123.343330198138)) ;
#30892=CARTESIAN_POINT('Ctrl Pts',(-20.6323994047383,36.8347061922723,123.357019653058)) ;
#30893=CARTESIAN_POINT('Ctrl Pts',(-20.870660430698,37.0345138475132,123.865857791706)) ;
#30894=CARTESIAN_POINT('Ctrl Pts',(-20.5783831490658,36.8545247671503,123.775043510851)) ;
#30895=CARTESIAN_POINT('Ctrl Pts',(-20.6279168053025,37.0544841485552,124.337676429547)) ;
#30896=CARTESIAN_POINT('Ctrl Pts',(-20.3841900155139,36.8744950681923,124.152499694084)) ;
#30897=CARTESIAN_POINT('Ctrl Pts',(-20.2401177850533,37.0743756809197,124.697290350133)) ;
#30898=CARTESIAN_POINT('Ctrl Pts',(-20.0739513811675,36.8943866005569,124.440192902116)) ;
#30899=CARTESIAN_POINT('Ctrl Pts',(-19.7497910668488,37.0943987787363,124.90385539926)) ;
#30900=CARTESIAN_POINT('Ctrl Pts',(-19.6816909775682,36.9144096983734,124.60544662509)) ;
#30901=CARTESIAN_POINT('Ctrl Pts',(-19.2242516782472,37.1141955316562,124.930779156354)) ;
#30902=CARTESIAN_POINT('Ctrl Pts',(-19.2612574376801,36.9342064512933,124.626987358956)) ;
#30903=CARTESIAN_POINT('Ctrl Pts',(-18.7165851062784,37.134156620145,124.77686253658)) ;
#30904=CARTESIAN_POINT('Ctrl Pts',(-18.8551234525687,36.9541675397821,124.503854730213)) ;
#30905=CARTESIAN_POINT('Ctrl Pts',(-18.2921431805836,37.1541348890772,124.457730120068)) ;
#30906=CARTESIAN_POINT('Ctrl Pts',(-18.5155690830116,36.9741458087143,124.24854960687)) ;
#30907=CARTESIAN_POINT('Ctrl Pts',(-18.0037890981737,37.1739549038682,124.016935959716)) ;
#30908=CARTESIAN_POINT('Ctrl Pts',(-18.2848840606162,36.9939658235053,123.89591275192)) ;
#30909=CARTESIAN_POINT('Ctrl Pts',(-17.8810922820256,37.19389331312,123.50137832524)) ;
#30910=CARTESIAN_POINT('Ctrl Pts',(-18.1867266714987,37.0139042327571,123.483465809288)) ;
#30911=CARTESIAN_POINT('Ctrl Pts',(-17.9432206011059,37.2139404305124,122.97212475137)) ;
#30912=CARTESIAN_POINT('Ctrl Pts',(-18.2364291043745,37.0339513501496,123.06006363056)) ;
#30913=CARTESIAN_POINT('Ctrl Pts',(-18.1799938362226,37.2337866763463,122.500836491877)) ;
#30914=CARTESIAN_POINT('Ctrl Pts',(-18.4258485917207,37.0537975959834,122.683031144881)) ;
#30915=CARTESIAN_POINT('Ctrl Pts',(-18.5620635941251,37.2536356448583,122.137020325925)) ;
#30916=CARTESIAN_POINT('Ctrl Pts',(-18.7315064596815,37.0736465644954,122.391977845995)) ;
#30917=CARTESIAN_POINT('Ctrl Pts',(-19.0504528465872,37.2736859471696,121.923931865139)) ;
#30918=CARTESIAN_POINT('Ctrl Pts',(-19.1222177233639,37.0936968668067,122.221508236812)) ;
#30919=CARTESIAN_POINT('Ctrl Pts',(-19.5767155011093,37.2935208696008,121.890757346003)) ;
#30920=CARTESIAN_POINT('Ctrl Pts',(-19.5432297263916,37.113531789238,122.194969649968)) ;
#30921=CARTESIAN_POINT('Ctrl Pts',(-20.08511494409,37.3134512708267,122.038788804448)) ;
#30922=CARTESIAN_POINT('Ctrl Pts',(-19.9499495172448,37.1334621904638,122.313396725135)) ;
#30923=CARTESIAN_POINT('Ctrl Pts',(-20.5122328950149,37.3333362161856,122.35040788788)) ;
#30924=CARTESIAN_POINT('Ctrl Pts',(-20.2916434333738,37.1533471358227,122.562694298399)) ;
#30925=CARTESIAN_POINT('Ctrl Pts',(-20.8092661802658,37.353408824337,122.793446550335)) ;
#30926=CARTESIAN_POINT('Ctrl Pts',(-20.5292680326244,37.1734197439741,122.917125764005)) ;
#30927=CARTESIAN_POINT('Ctrl Pts',(-20.9356180404718,37.3732001406651,123.304147384377)) ;
#30928=CARTESIAN_POINT('Ctrl Pts',(-20.6303478832511,37.1932110603022,123.325688757585)) ;
#30929=CARTESIAN_POINT('Ctrl Pts',(-20.8812658706226,37.3931649304323,123.8319433124)) ;
#30930=CARTESIAN_POINT('Ctrl Pts',(-20.5868633031295,37.2131758500695,123.747925458238)) ;
#30931=CARTESIAN_POINT('Ctrl Pts',(-20.6486375255731,37.4131478861826,124.309410738548)) ;
#30932=CARTESIAN_POINT('Ctrl Pts',(-20.4007582836289,37.2331588058198,124.129898402551)) ;
#30933=CARTESIAN_POINT('Ctrl Pts',(-20.2710983170399,37.4329564081588,124.676413569009)) ;
#30934=CARTESIAN_POINT('Ctrl Pts',(-20.0987238439308,37.2529673277959,124.423499492388)) ;
#30935=CARTESIAN_POINT('Ctrl Pts',(-19.7870846025984,37.4529419828946,124.894968051368)) ;
#30936=CARTESIAN_POINT('Ctrl Pts',(-19.7115114515686,37.2729529025317,124.598340127017)) ;
#30937=CARTESIAN_POINT('Ctrl Pts',(-19.2600251516879,37.472824622963,124.934935958172)) ;
#30938=CARTESIAN_POINT('Ctrl Pts',(-19.2898629599609,37.2928355426001,124.630311187914)) ;
#30939=CARTESIAN_POINT('Ctrl Pts',(-18.7492134555832,37.4927799350949,124.792594096249)) ;
#30940=CARTESIAN_POINT('Ctrl Pts',(-18.8812143169606,37.312790854732,124.516434239319)) ;
#30941=CARTESIAN_POINT('Ctrl Pts',(-18.319033254551,37.5126542917027,124.485894779788)) ;
#30942=CARTESIAN_POINT('Ctrl Pts',(-18.5370718339478,37.3326652113398,124.27107140888)) ;
#30943=CARTESIAN_POINT('Ctrl Pts',(-18.0175106060064,37.5326364985638,124.048765115388)) ;
#30944=CARTESIAN_POINT('Ctrl Pts',(-18.2958567266438,37.3526474182009,123.921365577981)) ;
#30945=CARTESIAN_POINT('Ctrl Pts',(-17.8838308617942,37.5525675765137,123.536059048149)) ;
#30946=CARTESIAN_POINT('Ctrl Pts',(-18.1889170443655,37.3725784961509,123.5111991052)) ;
#30947=CARTESIAN_POINT('Ctrl Pts',(-17.9330320754365,37.5724945513687,123.008830582015)) ;
#30948=CARTESIAN_POINT('Ctrl Pts',(-18.2282802580598,37.3925054710058,123.089417886411)) ;
#30949=CARTESIAN_POINT('Ctrl Pts',(-18.157254622848,37.5923270103176,122.531709623646)) ;
#30950=CARTESIAN_POINT('Ctrl Pts',(-18.4076687041876,37.4123379299547,122.707716901662)) ;
#30951=CARTESIAN_POINT('Ctrl Pts',(-18.4706659458096,37.6089846944928,122.219158784054)) ;
#30952=CARTESIAN_POINT('Ctrl Pts',(-18.658380296989,37.4289956141299,122.457695891381)) ;
#30953=CARTESIAN_POINT('Ctrl Pts',(-18.7724796762074,37.6222339183999,122.045392670349)) ;
#30954=CARTESIAN_POINT('Ctrl Pts',(-18.8998510804845,37.442244838037,122.318670265349)) ;
#30955=CARTESIAN_POINT('Ctrl Pts',(-19.0206690089167,37.6322829398511,121.955269929733)) ;
#30956=CARTESIAN_POINT('Ctrl Pts',(-19.0983967704762,37.4522938594882,122.246576695617)) ;
#30957=CARTESIAN_POINT('Ctrl Pts',(-19.2758657649021,37.6421429480816,121.910397904174)) ;
#30958=CARTESIAN_POINT('Ctrl Pts',(-19.3025665790804,37.4621538677187,122.210682152963)) ;
#30959=CARTESIAN_POINT('Ctrl Pts',(-19.6249794284296,37.6554264613062,121.909413584284)) ;
#30960=CARTESIAN_POINT('Ctrl Pts',(-19.5818035064809,37.4754373809433,122.20988869481)) ;
#30961=CARTESIAN_POINT('Ctrl Pts',(-20.0524638778648,37.672072380307,122.023188295616)) ;
#30962=CARTESIAN_POINT('Ctrl Pts',(-19.9238581002366,37.4920832999442,122.300927565958)) ;
#30963=CARTESIAN_POINT('Ctrl Pts',(-20.413880776944,37.6886263581231,122.274169668414)) ;
#30964=CARTESIAN_POINT('Ctrl Pts',(-20.2129442060005,37.5086372777602,122.501691816295)) ;
#30965=CARTESIAN_POINT('Ctrl Pts',(-20.6406243713132,37.7019860870947,122.542201540504)) ;
#30966=CARTESIAN_POINT('Ctrl Pts',(-20.3943637147157,37.5219970067318,122.716138256514)) ;
#30967=CARTESIAN_POINT('Ctrl Pts',(-20.771703979078,37.7118791388914,122.766737576687)) ;
#30968=CARTESIAN_POINT('Ctrl Pts',(-20.4992200975137,37.5318900585285,122.895764440336)) ;
#30969=CARTESIAN_POINT('Ctrl Pts',(-20.8630031282262,37.7218691041725,123.012844193469)) ;
#30970=CARTESIAN_POINT('Ctrl Pts',(-20.5722587448008,37.5418800238096,123.092651501254)) ;
#30971=CARTESIAN_POINT('Ctrl Pts',(-20.9101691765086,37.7318209850333,123.270122215449)) ;
#30972=CARTESIAN_POINT('Ctrl Pts',(-20.609988980369,37.5518319046704,123.298474032624)) ;
#30973=CARTESIAN_POINT('Ctrl Pts',(-20.9117400295103,37.7418693367251,123.534149528085)) ;
#30974=CARTESIAN_POINT('Ctrl Pts',(-20.6112435209441,37.5618802563622,123.509695891286)) ;
#30975=CARTESIAN_POINT('Ctrl Pts',(-20.8686496157947,37.7517106208313,123.789179451331)) ;
#30976=CARTESIAN_POINT('Ctrl Pts',(-20.576768936994,37.5717215404684,123.713719468987)) ;
#30977=CARTESIAN_POINT('Ctrl Pts',(-20.7811945958756,37.761697323957,124.0365703206)) ;
#30978=CARTESIAN_POINT('Ctrl Pts',(-20.5068028158722,37.5817082435941,123.911631353683)) ;
#30979=CARTESIAN_POINT('Ctrl Pts',(-20.6528738763807,37.7716323527744,124.263999794878)) ;
#30980=CARTESIAN_POINT('Ctrl Pts',(-20.4041443030014,37.5916432724115,124.093573772257)) ;
#30981=CARTESIAN_POINT('Ctrl Pts',(-20.4848851322175,37.7816881476813,124.467934944113)) ;
#30982=CARTESIAN_POINT('Ctrl Pts',(-20.2697515895762,37.6016990673184,124.256720420404)) ;
#30983=CARTESIAN_POINT('Ctrl Pts',(-20.2887835292672,37.7915165109706,124.636074676787)) ;
#30984=CARTESIAN_POINT('Ctrl Pts',(-20.1128689225267,37.6115274306077,124.391230423038)) ;
#30985=CARTESIAN_POINT('Ctrl Pts',(-20.0614584855971,37.8015774808685,124.771009318032)) ;
#30986=CARTESIAN_POINT('Ctrl Pts',(-19.931007771351,37.6215884005056,124.49917617883)) ;
#30987=CARTESIAN_POINT('Ctrl Pts',(-19.8176275658583,37.8114917597583,124.862882128275)) ;
#30988=CARTESIAN_POINT('Ctrl Pts',(-19.735942339562,37.6315026793954,124.572672280903)) ;
#30989=CARTESIAN_POINT('Ctrl Pts',(-19.5592226441299,37.8215007542265,124.911986102219)) ;
#30990=CARTESIAN_POINT('Ctrl Pts',(-19.5292180435957,37.6415116738637,124.611953245993)) ;
#30991=CARTESIAN_POINT('Ctrl Pts',(-19.2956698137528,37.8315305887903,124.914944725245)) ;
#30992=CARTESIAN_POINT('Ctrl Pts',(-19.3183757846655,37.6515415084274,124.614317886194)) ;
#30993=CARTESIAN_POINT('Ctrl Pts',(-19.0399553923332,37.8413888188625,124.873312424771)) ;
#30994=CARTESIAN_POINT('Ctrl Pts',(-19.113804794043,37.6613997384997,124.581009863178)) ;
#30995=CARTESIAN_POINT('Ctrl Pts',(-18.7918216048471,37.8513875246049,124.787014243601)) ;
#30996=CARTESIAN_POINT('Ctrl Pts',(-18.915298566103,37.6713984442421,124.511969231989)) ;
#30997=CARTESIAN_POINT('Ctrl Pts',(-18.5645984860679,37.8612821805237,124.660501733372)) ;
#30998=CARTESIAN_POINT('Ctrl Pts',(-18.7335213311777,37.6812931001609,124.410757393858)) ;
#30999=CARTESIAN_POINT('Ctrl Pts',(-18.3594834848053,37.8713452449077,124.493660346681)) ;
#31000=CARTESIAN_POINT('Ctrl Pts',(-18.5694307097895,37.6913561645448,124.277282542542)) ;
#31001=CARTESIAN_POINT('Ctrl Pts',(-18.1900212161876,37.8811849031876,124.298298757576)) ;
#31002=CARTESIAN_POINT('Ctrl Pts',(-18.4338627738789,37.7011958228247,124.120992079632)) ;
#31003=CARTESIAN_POINT('Ctrl Pts',(-18.0537869453756,37.8912480702694,124.071683477115)) ;
#31004=CARTESIAN_POINT('Ctrl Pts',(-18.3248772081804,37.7112589899066,123.939698699603)) ;
#31005=CARTESIAN_POINT('Ctrl Pts',(-17.9607436771395,37.9011423153965,123.828859729569)) ;
#31006=CARTESIAN_POINT('Ctrl Pts',(-18.2504447386895,37.7211532350337,123.745439163456)) ;
#31007=CARTESIAN_POINT('Ctrl Pts',(-17.9103527062584,37.9110841370011,123.572537760102)) ;
#31008=CARTESIAN_POINT('Ctrl Pts',(-18.2101341056503,37.7310950566383,123.540381382668)) ;
#31009=CARTESIAN_POINT('Ctrl Pts',(-17.9051034699468,37.9210866679192,123.309699103469)) ;
#31010=CARTESIAN_POINT('Ctrl Pts',(-18.2059368477175,37.7410975875563,123.330110481641)) ;
#31011=CARTESIAN_POINT('Ctrl Pts',(-17.946097783474,37.9311212943767,123.049219622139)) ;
#31012=CARTESIAN_POINT('Ctrl Pts',(-18.238734443196,37.7511322140138,123.121727220956)) ;
#31013=CARTESIAN_POINT('Ctrl Pts',(-18.0297012300919,37.9409668293631,122.804359246479)) ;
#31014=CARTESIAN_POINT('Ctrl Pts',(-18.3056190713924,37.7609777490003,122.925840036189)) ;
#31015=CARTESIAN_POINT('Ctrl Pts',(-18.1557855280744,37.9509502542022,122.574313582137)) ;
#31016=CARTESIAN_POINT('Ctrl Pts',(-18.4064882631411,37.7709611738393,122.741804625682)) ;
#31017=CARTESIAN_POINT('Ctrl Pts',(-18.3194140988036,37.9609006445672,122.370342409505)) ;
#31018=CARTESIAN_POINT('Ctrl Pts',(-18.5373926050169,37.7809115642044,122.578629156935)) ;
#31019=CARTESIAN_POINT('Ctrl Pts',(-18.5166838775539,37.9708982848643,122.196785487703)) ;
#31020=CARTESIAN_POINT('Ctrl Pts',(-18.6952097128482,37.7909092045014,122.439785207195)) ;
#31021=CARTESIAN_POINT('Ctrl Pts',(-18.7422660732146,37.9809373654275,122.060023983283)) ;
#31022=CARTESIAN_POINT('Ctrl Pts',(-18.8756765999443,37.8009482850646,122.330377774988)) ;
#31023=CARTESIAN_POINT('Ctrl Pts',(-18.9827700674646,37.9907635161966,121.965984935098)) ;
#31024=CARTESIAN_POINT('Ctrl Pts',(-19.068079960445,37.8107744358337,122.255148655797)) ;
#31025=CARTESIAN_POINT('Ctrl Pts',(-19.2417735141306,38.0008200911257,121.913534414804)) ;
#31026=CARTESIAN_POINT('Ctrl Pts',(-19.2752831961908,37.8208310107629,122.213190167423)) ;
#31027=CARTESIAN_POINT('Ctrl Pts',(-19.5029368385389,38.010760630506,121.907384733562)) ;
#31028=CARTESIAN_POINT('Ctrl Pts',(-19.4842136365279,37.8307715501431,122.20827246862)) ;
#31029=CARTESIAN_POINT('Ctrl Pts',(-19.7603796758828,38.0206650234824,121.94572645087)) ;
#31030=CARTESIAN_POINT('Ctrl Pts',(-19.6901671990176,37.8406759431195,122.238947693233)) ;
#31031=CARTESIAN_POINT('Ctrl Pts',(-20.0107210558662,38.0307116776873,122.029521129623)) ;
#31032=CARTESIAN_POINT('Ctrl Pts',(-19.8904397605092,37.8507225973244,122.305985318718)) ;
#31033=CARTESIAN_POINT('Ctrl Pts',(-20.2393912303446,38.0406072396257,122.153437722029)) ;
#31034=CARTESIAN_POINT('Ctrl Pts',(-20.0733745736591,37.8606181592628,122.405120060761)) ;
#31035=CARTESIAN_POINT('Ctrl Pts',(-20.4464358604614,38.0506693174713,122.317848314889)) ;
#31036=CARTESIAN_POINT('Ctrl Pts',(-20.2390091946635,37.8706802371084,122.536650134307)) ;
#31037=CARTESIAN_POINT('Ctrl Pts',(-20.6181207395519,38.060512015885,122.511348876402)) ;
#31038=CARTESIAN_POINT('Ctrl Pts',(-20.3763552143861,37.8805229355222,122.691451327068)) ;
#31039=CARTESIAN_POINT('Ctrl Pts',(-20.7561325943481,38.0705027908465,122.734655821582)) ;
#31040=CARTESIAN_POINT('Ctrl Pts',(-20.4867630838622,37.8905137104836,122.870097716257)) ;
#31041=CARTESIAN_POINT('Ctrl Pts',(-20.8526444302202,38.0804306558656,122.977057792993)) ;
#31042=CARTESIAN_POINT('Ctrl Pts',(-20.5639707221755,37.9004415755027,123.064019601063)) ;
#31043=CARTESIAN_POINT('Ctrl Pts',(-20.9063538531691,38.0904194006318,123.234003272381)) ;
#31044=CARTESIAN_POINT('Ctrl Pts',(-20.6069365241512,37.9104303202689,123.269576200659)) ;
#31045=CARTESIAN_POINT('Ctrl Pts',(-20.9142822162603,38.1004521862187,123.497539173054)) ;
#31046=CARTESIAN_POINT('Ctrl Pts',(-20.6132774084487,37.9204631058559,123.480405034982)) ;
#31047=CARTESIAN_POINT('Ctrl Pts',(-20.8772223147212,38.1103188708394,123.754154223928)) ;
#31048=CARTESIAN_POINT('Ctrl Pts',(-20.5836278397377,37.9303297904765,123.685696137519)) ;
#31049=CARTESIAN_POINT('Ctrl Pts',(-20.7960987290107,38.1202807630025,124.00306041153)) ;
#31050=CARTESIAN_POINT('Ctrl Pts',(-20.5187275050565,37.9402916826396,123.884820316478)) ;
#31051=CARTESIAN_POINT('Ctrl Pts',(-20.6717436692743,38.1303142399151,124.235550043403)) ;
#31052=CARTESIAN_POINT('Ctrl Pts',(-20.4192419168591,37.9503251595522,124.070811279402)) ;
#31053=CARTESIAN_POINT('Ctrl Pts',(-20.5116269403932,38.1401985811634,124.440122137364)) ;
#31054=CARTESIAN_POINT('Ctrl Pts',(-20.291147641117,37.9602095008005,124.2344674478)) ;
#31055=CARTESIAN_POINT('Ctrl Pts',(-20.3149827227567,38.1502615232845,124.616881340023)) ;
#31056=CARTESIAN_POINT('Ctrl Pts',(-20.1338310207247,37.9702724429217,124.37587373082)) ;
#31057=CARTESIAN_POINT('Ctrl Pts',(-20.0953938752767,38.1601119249041,124.75399118927)) ;
#31058=CARTESIAN_POINT('Ctrl Pts',(-19.9581597997883,37.9801228445412,124.48555979968)) ;
#31059=CARTESIAN_POINT('Ctrl Pts',(-19.8513087068426,38.1701388136938,124.853234002042)) ;
#31060=CARTESIAN_POINT('Ctrl Pts',(-19.7628910767466,37.9901497333309,124.564952686841)) ;
#31061=CARTESIAN_POINT('Ctrl Pts',(-19.593491376287,38.18016742865,124.907926696643)) ;
#31062=CARTESIAN_POINT('Ctrl Pts',(-19.5566368221853,38.0001783482871,124.60870527169)) ;
#31063=CARTESIAN_POINT('Ctrl Pts',(-19.3349545228551,38.19001265177,124.917345289566)) ;
#31064=CARTESIAN_POINT('Ctrl Pts',(-19.3498081794795,38.0100235714072,124.616238591865)) ;
#31065=CARTESIAN_POINT('Ctrl Pts',(-19.0748065717966,38.200003335576,124.88189910921)) ;
#31066=CARTESIAN_POINT('Ctrl Pts',(-19.1416901604654,38.0200142552131,124.587880298934)) ;
#31067=CARTESIAN_POINT('Ctrl Pts',(-18.8237728136893,38.2100412176484,124.80088615643)) ;
#31068=CARTESIAN_POINT('Ctrl Pts',(-18.9408635131046,38.0300521372856,124.52306847567)) ;
#31069=CARTESIAN_POINT('Ctrl Pts',(-18.5948907896328,38.2198855772873,124.680287851483)) ;
#31070=CARTESIAN_POINT('Ctrl Pts',(-18.7577593811284,38.0398964969244,124.426589023562)) ;
#31071=CARTESIAN_POINT('Ctrl Pts',(-18.3872272286847,38.229870447902,124.519955106578)) ;
#31072=CARTESIAN_POINT('Ctrl Pts',(-18.5916294861403,38.0498813675391,124.298321919019)) ;
#31073=CARTESIAN_POINT('Ctrl Pts',(-18.2112252563883,38.2398097312307,124.326911572828)) ;
#31074=CARTESIAN_POINT('Ctrl Pts',(-18.4508291441772,38.0598206508678,124.143886556018)) ;
#31075=CARTESIAN_POINT('Ctrl Pts',(-18.0700954992362,38.2498503406038,124.104002776353)) ;
#31076=CARTESIAN_POINT('Ctrl Pts',(-18.3379263671355,38.0698612602409,123.9655587244)) ;
#31077=CARTESIAN_POINT('Ctrl Pts',(-17.9711690914586,38.259735191517,123.863780801288)) ;
#31078=CARTESIAN_POINT('Ctrl Pts',(-18.2587866856612,38.0797461111542,123.773381363225)) ;
#31079=CARTESIAN_POINT('Ctrl Pts',(-17.9145022539865,38.2697371476858,123.607161518794)) ;
#31080=CARTESIAN_POINT('Ctrl Pts',(-18.2134543961033,38.089748067323,123.568085793676)) ;
#31081=CARTESIAN_POINT('Ctrl Pts',(-17.9031351939843,38.2796557444063,123.34671741945)) ;
#31082=CARTESIAN_POINT('Ctrl Pts',(-18.2043619071338,38.0996666640434,123.359731038019)) ;
#31083=CARTESIAN_POINT('Ctrl Pts',(-17.9376431227796,38.2897025664821,123.084999919376)) ;
#31084=CARTESIAN_POINT('Ctrl Pts',(-18.2319694141101,38.1097134861192,123.150357019419)) ;
#31085=CARTESIAN_POINT('Ctrl Pts',(-18.0154975116536,38.2995768475948,122.837421943665)) ;
#31086=CARTESIAN_POINT('Ctrl Pts',(-18.2942537162335,38.1195877672319,122.95229576589)) ;
#31087=CARTESIAN_POINT('Ctrl Pts',(-18.1371535108144,38.3096310476394,122.602934129142)) ;
#31088=CARTESIAN_POINT('Ctrl Pts',(-18.391579553754,38.1296419672765,122.764705818433)) ;
#31089=CARTESIAN_POINT('Ctrl Pts',(-18.2951140075871,38.3195264772746,122.396304412918)) ;
#31090=CARTESIAN_POINT('Ctrl Pts',(-18.5179483256354,38.1395373969118,122.599403261707)) ;
#31091=CARTESIAN_POINT('Ctrl Pts',(-18.489664634007,38.329588105592,122.217293421697)) ;
#31092=CARTESIAN_POINT('Ctrl Pts',(-18.6735897116982,38.1495990252291,122.456195042217)) ;
#31093=CARTESIAN_POINT('Ctrl Pts',(-18.7075571482892,38.3394327344219,122.077804596519)) ;
#31094=CARTESIAN_POINT('Ctrl Pts',(-18.8479033795345,38.159443654059,122.344605407475)) ;
#31095=CARTESIAN_POINT('Ctrl Pts',(-18.9487829946581,38.3493927820275,121.976237815657)) ;
#31096=CARTESIAN_POINT('Ctrl Pts',(-19.0408840272685,38.1694037016646,122.26335285546)) ;
#31097=CARTESIAN_POINT('Ctrl Pts',(-19.2060908983608,38.3594310882016,121.918149353435)) ;
#31098=CARTESIAN_POINT('Ctrl Pts',(-19.2467306787397,38.1794420078387,122.216882950581)) ;
#31099=CARTESIAN_POINT('Ctrl Pts',(-19.4652741750424,38.3693043876342,121.905324657195)) ;
#31100=CARTESIAN_POINT('Ctrl Pts',(-19.4540764400432,38.1893153072714,122.206624032452)) ;
#31101=CARTESIAN_POINT('Ctrl Pts',(-19.7278563927704,38.3793776492205,121.938426707961)) ;
#31102=CARTESIAN_POINT('Ctrl Pts',(-19.6641424513348,38.1993885688576,122.233106527423)) ;
#31103=CARTESIAN_POINT('Ctrl Pts',(-19.9745595742938,38.3891978751772,122.014360134831)) ;
#31104=CARTESIAN_POINT('Ctrl Pts',(-19.8615035911148,38.2092087948143,122.293853602793)) ;
#31105=CARTESIAN_POINT('Ctrl Pts',(-20.2103785146625,38.3992769391167,122.134809378916)) ;
#31106=CARTESIAN_POINT('Ctrl Pts',(-20.0501587726125,38.2192878587538,122.390213775036)) ;
#31107=CARTESIAN_POINT('Ctrl Pts',(-20.4170842341087,38.4091270291365,122.29073495999)) ;
#31108=CARTESIAN_POINT('Ctrl Pts',(-20.2155221090438,38.2291379487737,122.514954115043)) ;
#31109=CARTESIAN_POINT('Ctrl Pts',(-20.5976790049717,38.4192057827503,122.484385049267)) ;
#31110=CARTESIAN_POINT('Ctrl Pts',(-20.359997738072,38.2392167023874,122.669874889421)) ;
#31111=CARTESIAN_POINT('Ctrl Pts',(-20.7384592821363,38.4290272500098,122.700777392782)) ;
#31112=CARTESIAN_POINT('Ctrl Pts',(-20.4726207917741,38.2490381696469,122.842988001983)) ;
#31113=CARTESIAN_POINT('Ctrl Pts',(-20.8423676549778,38.4390928483674,122.943961403778)) ;
#31114=CARTESIAN_POINT('Ctrl Pts',(-20.5557471819317,38.2591037680045,123.037535670951)) ;
#31115=CARTESIAN_POINT('Ctrl Pts',(-20.9014598751906,38.4489955041421,123.197461404665)) ;
#31116=CARTESIAN_POINT('Ctrl Pts',(-20.6030203204311,38.2690064237792,123.240335071546)) ;
#31117=CARTESIAN_POINT('Ctrl Pts',(-20.9159258761711,38.4590463299717,123.461136272486)) ;
#31118=CARTESIAN_POINT('Ctrl Pts',(-20.6145926705631,38.2790572496089,123.451275207691)) ;
#31119=CARTESIAN_POINT('Ctrl Pts',(-20.8851806308957,38.4689205343106,123.718849938155)) ;
#31120=CARTESIAN_POINT('Ctrl Pts',(-20.5899961850183,38.2889314539477,123.657445168674)) ;
#31121=CARTESIAN_POINT('Ctrl Pts',(-20.808697747039,38.4789929843497,123.972194060034)) ;
#31122=CARTESIAN_POINT('Ctrl Pts',(-20.5288093967578,38.2990039039868,123.860120677196)) ;
#31123=CARTESIAN_POINT('Ctrl Pts',(-20.6924452330028,38.4888220011232,124.202906653744)) ;
#31124=CARTESIAN_POINT('Ctrl Pts',(-20.4358076437675,38.3088329207603,124.044689498754)) ;
#31125=CARTESIAN_POINT('Ctrl Pts',(-20.5345088117265,38.498888847038,124.415079071641)) ;
#31126=CARTESIAN_POINT('Ctrl Pts',(-20.3094581203434,38.3188997666751,124.214427542869)) ;
#31127=CARTESIAN_POINT('Ctrl Pts',(-20.3453362910282,38.5087790183398,124.593350718177)) ;
#31128=CARTESIAN_POINT('Ctrl Pts',(-20.1581205171573,38.3287899379769,124.35704407548)) ;
#31129=CARTESIAN_POINT('Ctrl Pts',(-20.1262004053155,38.5187712119636,124.737995435515)) ;
#31130=CARTESIAN_POINT('Ctrl Pts',(-19.9828118735316,38.3387821316008,124.472759636862)) ;
#31131=CARTESIAN_POINT('Ctrl Pts',(-19.8858793197356,38.5287340225871,124.841862120209)) ;
#31132=CARTESIAN_POINT('Ctrl Pts',(-19.7905552583215,38.3487449422242,124.55585265074)) ;
#31133=CARTESIAN_POINT('Ctrl Pts',(-19.6327966736522,38.5386382954305,124.9027167446)) ;
#31134=CARTESIAN_POINT('Ctrl Pts',(-19.5880898637253,38.3586492150676,124.604536139099)) ;
#31135=CARTESIAN_POINT('Ctrl Pts',(-19.3689353661875,38.5486987872351,124.918722771456)) ;
#31136=CARTESIAN_POINT('Ctrl Pts',(-19.3770005294909,38.3687097068723,124.617340882227)) ;
#31137=CARTESIAN_POINT('Ctrl Pts',(-19.1119433120646,38.5585391189074,124.8896559552)) ;
#31138=CARTESIAN_POINT('Ctrl Pts',(-19.1714080569819,38.3785500385446,124.594087552618)) ;
#31139=CARTESIAN_POINT('Ctrl Pts',(-18.858267179598,38.5686021649992,124.815076395297)) ;
#31140=CARTESIAN_POINT('Ctrl Pts',(-18.9684668438895,38.3886130846363,124.534423889178)) ;
#31141=CARTESIAN_POINT('Ctrl Pts',(-18.6254129262552,38.5784962206943,124.699336919331)) ;
#31142=CARTESIAN_POINT('Ctrl Pts',(-18.782184165847,38.3985071403314,124.441832684119)) ;
#31143=CARTESIAN_POINT('Ctrl Pts',(-18.4147842988255,38.5884389210173,124.544774213898)) ;
#31144=CARTESIAN_POINT('Ctrl Pts',(-18.6136815630311,38.4084498406544,124.318182986908)) ;
#31145=CARTESIAN_POINT('Ctrl Pts',(-18.2329705623296,38.5984446619449,124.354785151136)) ;
#31146=CARTESIAN_POINT('Ctrl Pts',(-18.4682304676226,38.418455581582,124.166191932299)) ;
#31147=CARTESIAN_POINT('Ctrl Pts',(-18.086951476104,38.6084655724604,124.135644682199)) ;
#31148=CARTESIAN_POINT('Ctrl Pts',(-18.3514150709044,38.4284764920975,123.990879603999)) ;
#31149=CARTESIAN_POINT('Ctrl Pts',(-17.9822934308915,38.6183563079104,123.897719206915)) ;
#31150=CARTESIAN_POINT('Ctrl Pts',(-18.2676887771091,38.4383672275475,123.800540072914)) ;
#31151=CARTESIAN_POINT('Ctrl Pts',(-17.9195346698227,38.6283478486392,123.642773296593)) ;
#31152=CARTESIAN_POINT('Ctrl Pts',(-18.2174815116301,38.4483587682763,123.596583584727)) ;
#31153=CARTESIAN_POINT('Ctrl Pts',(-17.9021467020347,38.6382957090609,123.381934725884)) ;
#31154=CARTESIAN_POINT('Ctrl Pts',(-18.2035708827029,38.458306628698,123.387913220143)) ;
#31155=CARTESIAN_POINT('Ctrl Pts',(-17.9297985346469,38.6482423782472,123.121998548221)) ;
#31156=CARTESIAN_POINT('Ctrl Pts',(-18.225691882754,38.4682532978843,123.179964691049)) ;
#31157=CARTESIAN_POINT('Ctrl Pts',(-18.0031723206151,38.6582904543828,122.868354913034)) ;
#31158=CARTESIAN_POINT('Ctrl Pts',(-18.2843906358415,38.4783013740199,122.977049494518)) ;
#31159=CARTESIAN_POINT('Ctrl Pts',(-18.1169630845849,38.6681380523884,122.635927730738)) ;
#31160=CARTESIAN_POINT('Ctrl Pts',(-18.3754223953298,38.4881489720256,122.791108578199)) ;
#31161=CARTESIAN_POINT('Ctrl Pts',(-18.2704754939803,38.6780997754729,122.423894509235)) ;
#31162=CARTESIAN_POINT('Ctrl Pts',(-18.498231618631,38.49811069511,122.621481940386)) ;
#31163=CARTESIAN_POINT('Ctrl Pts',(-18.459987920288,38.6881284105559,122.240733703719)) ;
#31164=CARTESIAN_POINT('Ctrl Pts',(-18.6498412530283,38.508139330193,122.474952867454)) ;
#31165=CARTESIAN_POINT('Ctrl Pts',(-18.6757765964958,38.6980387188739,122.094945578105)) ;
#31166=CARTESIAN_POINT('Ctrl Pts',(-18.822471309607,38.5180496385111,122.358322309801)) ;
#31167=CARTESIAN_POINT('Ctrl Pts',(-18.9139298646634,38.7079736160098,121.987944654687)) ;
#31168=CARTESIAN_POINT('Ctrl Pts',(-19.0129931507068,38.5279845356469,122.272721138619)) ;
#31169=CARTESIAN_POINT('Ctrl Pts',(-19.1697940908906,38.7180146989524,121.92347677505)) ;
#31170=CARTESIAN_POINT('Ctrl Pts',(-19.2176845178362,38.5380256185895,122.221146167551)) ;
#31171=CARTESIAN_POINT('Ctrl Pts',(-19.4289447281885,38.7279020417806,121.904527054462)) ;
#31172=CARTESIAN_POINT('Ctrl Pts',(-19.4250041481742,38.5479129614178,122.20598575918)) ;
#31173=CARTESIAN_POINT('Ctrl Pts',(-19.6901903067169,38.73789355672,121.930687744959)) ;
#31174=CARTESIAN_POINT('Ctrl Pts',(-19.634000528053,38.5579044763571,122.226913496927)) ;
#31175=CARTESIAN_POINT('Ctrl Pts',(-19.9419001392369,38.7478449479164,122.001637581168)) ;
#31176=CARTESIAN_POINT('Ctrl Pts',(-19.8353681920912,38.5678558675536,122.283672501495)) ;
#31177=CARTESIAN_POINT('Ctrl Pts',(-20.1772104092053,38.7577774812491,122.114589337141)) ;
#31178=CARTESIAN_POINT('Ctrl Pts',(-20.0236163134936,38.5777884008862,122.374032878613)) ;
#31179=CARTESIAN_POINT('Ctrl Pts',(-20.3907677132585,38.7677746391485,122.267583026891)) ;
#31180=CARTESIAN_POINT('Ctrl Pts',(-20.1944625857522,38.5877855587856,122.496427023054)) ;
#31181=CARTESIAN_POINT('Ctrl Pts',(-20.5743995160923,38.777759649312,122.455072551218)) ;
#31182=CARTESIAN_POINT('Ctrl Pts',(-20.3413685642757,38.5977705689491,122.646417859673)) ;
#31183=CARTESIAN_POINT('Ctrl Pts',(-20.7231828307075,38.7878024758818,122.673007430821)) ;
#31184=CARTESIAN_POINT('Ctrl Pts',(-20.4603959891244,38.6078133955189,122.82076541107)) ;
#31185=CARTESIAN_POINT('Ctrl Pts',(-20.8301369986688,38.7976327101868,122.908200598567)) ;
#31186=CARTESIAN_POINT('Ctrl Pts',(-20.5459597363222,38.6176436298239,123.008918492089)) ;
#31187=CARTESIAN_POINT('Ctrl Pts',(-20.8963322764258,38.8077087354214,123.164523836751)) ;
#31188=CARTESIAN_POINT('Ctrl Pts',(-20.5989170207742,38.6277196550586,123.213977164575)) ;
#31189=CARTESIAN_POINT('Ctrl Pts',(-20.9166999184839,38.8175609719123,123.422684680524)) ;
#31190=CARTESIAN_POINT('Ctrl Pts',(-20.6152120890159,38.6375718915494,123.420504774744)) ;
#31191=CARTESIAN_POINT('Ctrl Pts',(-20.8916094132905,38.8276341783464,123.686162896882)) ;
#31192=CARTESIAN_POINT('Ctrl Pts',(-20.5951407373615,38.6476450979836,123.631287770219)) ;
#31193=CARTESIAN_POINT('Ctrl Pts',(-20.8226867659829,38.8374756878536,123.935453060471)) ;
#31194=CARTESIAN_POINT('Ctrl Pts',(-20.5400039281525,38.6574866074907,123.830719181644)) ;
#31195=CARTESIAN_POINT('Ctrl Pts',(-20.711078874135,38.8474366346334,124.172221368131)) ;
#31196=CARTESIAN_POINT('Ctrl Pts',(-20.4507189196892,38.6674475542705,124.020134084588)) ;
#31197=CARTESIAN_POINT('Ctrl Pts',(-20.558458951886,38.8574744634334,124.387360046542)) ;
#31198=CARTESIAN_POINT('Ctrl Pts',(-20.3286238767375,38.6774853830706,124.192245792429)) ;
#31199=CARTESIAN_POINT('Ctrl Pts',(-20.3741695323438,38.8673487731879,124.570081720976)) ;
#31200=CARTESIAN_POINT('Ctrl Pts',(-20.1811938154597,38.687359692825,124.338423469398)) ;
#31201=CARTESIAN_POINT('Ctrl Pts',(-20.1567812055592,38.8774184708611,124.72090620419)) ;
#31202=CARTESIAN_POINT('Ctrl Pts',(-20.0072836517336,38.6974293904982,124.459084262676)) ;
#31203=CARTESIAN_POINT('Ctrl Pts',(-19.9221504638818,38.8872519421485,124.82924108008)) ;
#31204=CARTESIAN_POINT('Ctrl Pts',(-19.8195805334962,38.7072628617856,124.545752917569)) ;
#31205=CARTESIAN_POINT('Ctrl Pts',(-19.6675077755331,38.8972815886784,124.897233739368)) ;
#31206=CARTESIAN_POINT('Ctrl Pts',(-19.615866693082,38.7172925083155,124.600148473551)) ;
#31207=CARTESIAN_POINT('Ctrl Pts',(-19.4047212779265,38.9073161030058,124.919189865937)) ;
#31208=CARTESIAN_POINT('Ctrl Pts',(-19.4056375333307,38.7273270226429,124.61771467157)) ;
#31209=CARTESIAN_POINT('Ctrl Pts',(-19.1475370275011,38.9171413884767,124.896304082123)) ;
#31210=CARTESIAN_POINT('Ctrl Pts',(-19.1998910344568,38.7371523081138,124.599407555355)) ;
#31211=CARTESIAN_POINT('Ctrl Pts',(-18.8935792031542,38.9271456300252,124.828433457309)) ;
#31212=CARTESIAN_POINT('Ctrl Pts',(-18.9967244455218,38.7471565496623,124.545112555679)) ;
#31213=CARTESIAN_POINT('Ctrl Pts',(-18.6557514840931,38.9371282751043,124.717603510386)) ;
#31214=CARTESIAN_POINT('Ctrl Pts',(-18.8064617880754,38.7571391947414,124.456450040447)) ;
#31215=CARTESIAN_POINT('Ctrl Pts',(-18.439669749991,38.9471734721958,124.566019704998)) ;
#31216=CARTESIAN_POINT('Ctrl Pts',(-18.633595466131,38.7671843918329,124.335184114137)) ;
#31217=CARTESIAN_POINT('Ctrl Pts',(-18.2569780632649,38.9569965879559,124.383630345431)) ;
#31218=CARTESIAN_POINT('Ctrl Pts',(-18.4874417365958,38.7770075075931,124.189274418743)) ;
#31219=CARTESIAN_POINT('Ctrl Pts',(-18.1050023548241,38.9670311997562,124.168134092341)) ;
#31220=CARTESIAN_POINT('Ctrl Pts',(-18.3658597612924,38.7870421193933,124.016878306509)) ;
#31221=CARTESIAN_POINT('Ctrl Pts',(-17.9935211048472,38.9770562085294,123.929428614842)) ;
#31222=CARTESIAN_POINT('Ctrl Pts',(-18.2766733718385,38.7970671281665,123.825914551769)) ;
#31223=CARTESIAN_POINT('Ctrl Pts',(-17.9258146375031,38.9869081333709,123.679534933401)) ;
#31224=CARTESIAN_POINT('Ctrl Pts',(-18.2225068346885,38.8069190530081,123.62600081153)) ;
#31225=CARTESIAN_POINT('Ctrl Pts',(-17.9017999976252,38.9968990716936,123.418116000194)) ;
#31226=CARTESIAN_POINT('Ctrl Pts',(-18.2032934378327,38.8169099913308,123.416865957209)) ;
#31227=CARTESIAN_POINT('Ctrl Pts',(-17.9232192572526,39.0068170568401,123.158331775182)) ;
#31228=CARTESIAN_POINT('Ctrl Pts',(-18.2204270837738,38.8268279764772,123.209038890302)) ;
#31229=CARTESIAN_POINT('Ctrl Pts',(-17.9900801459671,39.0168451577356,122.903447812489)) ;
#31230=CARTESIAN_POINT('Ctrl Pts',(-18.2739141162152,38.8368560773727,123.005131251338)) ;
#31231=CARTESIAN_POINT('Ctrl Pts',(-18.0985256645866,39.0267303986782,122.66738650819)) ;
#31232=CARTESIAN_POINT('Ctrl Pts',(-18.3606686866534,38.8467413183153,122.816282007666)) ;
#31233=CARTESIAN_POINT('Ctrl Pts',(-18.2473354546933,39.0367195116448,122.451127866607)) ;
#31234=CARTESIAN_POINT('Ctrl Pts',(-18.4797149123304,38.8567304312819,122.643274141846)) ;
#31235=CARTESIAN_POINT('Ctrl Pts',(-18.4328121554963,39.0467615759856,122.263416874408)) ;
#31236=CARTESIAN_POINT('Ctrl Pts',(-18.628095065177,38.8667724956227,122.49310404951)) ;
#31237=CARTESIAN_POINT('Ctrl Pts',(-18.6432316642718,39.0565907773901,122.113588566168)) ;
#31238=CARTESIAN_POINT('Ctrl Pts',(-18.7964289710917,38.8766016970272,122.373240345266)) ;
#31239=CARTESIAN_POINT('Ctrl Pts',(-18.8804006960058,39.0665976181483,122.000064282247)) ;
#31240=CARTESIAN_POINT('Ctrl Pts',(-18.986163304992,38.8866085377854,122.282419197407)) ;
#31241=CARTESIAN_POINT('Ctrl Pts',(-19.1333031196278,39.0765851423402,121.929712194851)) ;
#31242=CARTESIAN_POINT('Ctrl Pts',(-19.1884846090727,38.8965960619773,122.226135721828)) ;
#31243=CARTESIAN_POINT('Ctrl Pts',(-19.3956318554856,39.0866147881488,121.90442252384)) ;
#31244=CARTESIAN_POINT('Ctrl Pts',(-19.3983474399373,38.9066257077859,122.205902107864)) ;
#31245=CARTESIAN_POINT('Ctrl Pts',(-19.6543650766534,39.0964888188876,121.924438378725)) ;
#31246=CARTESIAN_POINT('Ctrl Pts',(-19.6053336278132,38.9164997385247,122.221912828069)) ;
#31247=CARTESIAN_POINT('Ctrl Pts',(-19.9088952559089,39.1064881417517,121.989562946881)) ;
#31248=CARTESIAN_POINT('Ctrl Pts',(-19.8089581746776,38.9264990613888,122.274010548606)) ;
#31249=CARTESIAN_POINT('Ctrl Pts',(-20.1463184204116,39.1163989773273,122.096736593804)) ;
#31250=CARTESIAN_POINT('Ctrl Pts',(-19.9988971842688,38.9364098969644,122.359747484487)) ;
#31251=CARTESIAN_POINT('Ctrl Pts',(-20.3645137350782,39.1264532253013,122.245659936878)) ;
#31252=CARTESIAN_POINT('Ctrl Pts',(-20.1734546335938,38.9464641449384,122.47888456104)) ;
#31253=CARTESIAN_POINT('Ctrl Pts',(-20.5501363523251,39.136311969564,122.426460600573)) ;
#31254=CARTESIAN_POINT('Ctrl Pts',(-20.3219537705766,38.9563228892011,122.623523276543)) ;
#31255=CARTESIAN_POINT('Ctrl Pts',(-20.7048400636721,39.146380055637,122.641049209758)) ;
#31256=CARTESIAN_POINT('Ctrl Pts',(-20.445718474219,38.9663909752741,122.795193064183)) ;
#31257=CARTESIAN_POINT('Ctrl Pts',(-20.8175117263284,39.1562355388165,122.87427274074)) ;
#31258=CARTESIAN_POINT('Ctrl Pts',(-20.5358574288074,38.9762464584537,122.981770549878)) ;
#31259=CARTESIAN_POINT('Ctrl Pts',(-20.889721867706,39.1662303846107,123.126796707764)) ;
#31260=CARTESIAN_POINT('Ctrl Pts',(-20.5936275684775,38.9862413042478,123.183789061337)) ;
#31261=CARTESIAN_POINT('Ctrl Pts',(-20.9165245762999,39.1762616802733,123.389047651322)) ;
#31262=CARTESIAN_POINT('Ctrl Pts',(-20.6150717949923,38.9962725999104,123.393589604221)) ;
#31263=CARTESIAN_POINT('Ctrl Pts',(-20.8981112102425,39.1861282235631,123.647684462324)) ;
#31264=CARTESIAN_POINT('Ctrl Pts',(-20.6003432386068,39.0061391432003,123.600498792257)) ;
#31265=CARTESIAN_POINT('Ctrl Pts',(-20.8347179859735,39.1961156193265,123.902339731277)) ;
#31266=CARTESIAN_POINT('Ctrl Pts',(-20.5496307722175,39.0161265389636,123.804223432309)) ;
#31267=CARTESIAN_POINT('Ctrl Pts',(-20.728622932385,39.2060606600565,124.14122345198)) ;
#31268=CARTESIAN_POINT('Ctrl Pts',(-20.4647567795798,39.0260715796936,123.9953311149)) ;
#31269=CARTESIAN_POINT('Ctrl Pts',(-20.5811155220166,39.2161051662732,124.360088757602)) ;
#31270=CARTESIAN_POINT('Ctrl Pts',(-20.3467526264366,39.0361160859103,124.170424573902)) ;
#31271=CARTESIAN_POINT('Ctrl Pts',(-20.4012820501656,39.2259686724105,124.546795194446)) ;
#31272=CARTESIAN_POINT('Ctrl Pts',(-20.2028876468785,39.0459795920477,124.319790982306)) ;
#31273=CARTESIAN_POINT('Ctrl Pts',(-20.1893406639608,39.2359615332466,124.701780528445)) ;
#31274=CARTESIAN_POINT('Ctrl Pts',(-20.033335900681,39.0559724528837,124.443780983451)) ;
#31275=CARTESIAN_POINT('Ctrl Pts',(-19.9552664329016,39.2458877269655,124.816982053056)) ;
#31276=CARTESIAN_POINT('Ctrl Pts',(-19.8460776484438,39.0658986466027,124.535944103352)) ;
#31277=CARTESIAN_POINT('Ctrl Pts',(-19.7024842949339,39.2559066529981,124.890499840195)) ;
#31278=CARTESIAN_POINT('Ctrl Pts',(-19.643852594965,39.0759175726352,124.594760445571)) ;
#31279=CARTESIAN_POINT('Ctrl Pts',(-19.4434484431289,39.2658216523657,124.918965884066)) ;
#31280=CARTESIAN_POINT('Ctrl Pts',(-19.4366243284276,39.0858325720028,124.61753546939)) ;
#31281=CARTESIAN_POINT('Ctrl Pts',(-19.1798154010535,39.275876423923,124.901733325748)) ;
#31282=CARTESIAN_POINT('Ctrl Pts',(-19.2257177564351,39.0958873435601,124.603751640336)) ;
#31283=CARTESIAN_POINT('Ctrl Pts',(-18.9280744033614,39.2857353862206,124.840355827184)) ;
#31284=CARTESIAN_POINT('Ctrl Pts',(-19.0243246392442,39.1057463058577,124.55465185544)) ;
#31285=CARTESIAN_POINT('Ctrl Pts',(-18.6874294683808,39.2957296300584,124.735252472311)) ;
#31286=CARTESIAN_POINT('Ctrl Pts',(-18.8318078469648,39.1157405496955,124.470571256637)) ;
#31287=CARTESIAN_POINT('Ctrl Pts',(-18.4700628513266,39.3056548594826,124.591021419432)) ;
#31288=CARTESIAN_POINT('Ctrl Pts',(-18.6579133993353,39.1256657791198,124.355188343277)) ;
#31289=CARTESIAN_POINT('Ctrl Pts',(-18.2791321697973,39.3156828233741,124.409439034504)) ;
#31290=CARTESIAN_POINT('Ctrl Pts',(-18.5051673400138,39.1356937430112,124.209924100878)) ;
#31291=CARTESIAN_POINT('Ctrl Pts',(-18.1245827427517,39.3255690830045,124.200558385393)) ;
#31292=CARTESIAN_POINT('Ctrl Pts',(-18.381526045183,39.1455800026416,124.042820995344)) ;
#31293=CARTESIAN_POINT('Ctrl Pts',(-18.0068578913663,39.3356008460823,123.964729079241)) ;
#31294=CARTESIAN_POINT('Ctrl Pts',(-18.2873441695228,39.1556117657195,123.854158607123)) ;
#31295=CARTESIAN_POINT('Ctrl Pts',(-17.9327236697777,39.3454824723765,123.715808953631)) ;
#31296=CARTESIAN_POINT('Ctrl Pts',(-18.2280346488682,39.1654933920136,123.65502319765)) ;
#31297=CARTESIAN_POINT('Ctrl Pts',(-17.9023337792867,39.3555442418626,123.453187507275)) ;
#31298=CARTESIAN_POINT('Ctrl Pts',(-18.2037205033373,39.1755551614998,123.444926368231)) ;
#31299=CARTESIAN_POINT('Ctrl Pts',(-17.9176154685571,39.3654021093581,123.194552719115)) ;
#31300=CARTESIAN_POINT('Ctrl Pts',(-18.2159436064791,39.1854130289952,123.238018412343)) ;
#31301=CARTESIAN_POINT('Ctrl Pts',(-17.9778056084377,39.3753937344755,122.939007178567)) ;
#31302=CARTESIAN_POINT('Ctrl Pts',(-18.2640935243759,39.1954046541126,123.033581500678)) ;
#31303=CARTESIAN_POINT('Ctrl Pts',(-18.0809465923163,39.3853305335837,122.699093789421)) ;
#31304=CARTESIAN_POINT('Ctrl Pts',(-18.3466042525769,39.2053414532208,122.841649902938)) ;
#31305=CARTESIAN_POINT('Ctrl Pts',(-18.2246316582653,39.3953213631411,122.479348914402)) ;
#31306=CARTESIAN_POINT('Ctrl Pts',(-18.4615504185501,39.2153322827782,122.66585281308)) ;
#31307=CARTESIAN_POINT('Ctrl Pts',(-18.4050975254076,39.4053445988542,122.287476075996)) ;
#31308=CARTESIAN_POINT('Ctrl Pts',(-18.6059214265816,39.2253555184914,122.512353066652)) ;
#31309=CARTESIAN_POINT('Ctrl Pts',(-18.6133254066964,39.4152409468834,122.131679228761)) ;
#31310=CARTESIAN_POINT('Ctrl Pts',(-18.7725024389883,39.2352518665205,122.387713758651)) ;
#31311=CARTESIAN_POINT('Ctrl Pts',(-18.8473919143103,39.4252305093859,122.012791074316)) ;
#31312=CARTESIAN_POINT('Ctrl Pts',(-18.9597546642961,39.245241429023,122.292601282324)) ;
#31313=CARTESIAN_POINT('Ctrl Pts',(-19.0999512728563,39.4352708170704,121.936479082214)) ;
#31314=CARTESIAN_POINT('Ctrl Pts',(-19.1618012471887,39.2552817367076,122.231549573829)) ;
#31315=CARTESIAN_POINT('Ctrl Pts',(-19.3567329848095,39.4451131204176,121.905300141157)) ;
#31316=CARTESIAN_POINT('Ctrl Pts',(-19.3672271092616,39.2651240400548,122.206604238954)) ;
#31317=CARTESIAN_POINT('Ctrl Pts',(-19.6197445019835,39.4551368286967,121.919081532484)) ;
#31318=CARTESIAN_POINT('Ctrl Pts',(-19.5776343212279,39.2751477483338,122.217627049978)) ;
#31319=CARTESIAN_POINT('Ctrl Pts',(-19.9583923044283,39.4683590061644,121.997113385212)) ;
#31320=CARTESIAN_POINT('Ctrl Pts',(-19.8485635151233,39.2883699258015,122.280050331721)) ;
#31321=CARTESIAN_POINT('Ctrl Pts',(-20.2706261181306,39.4816515912237,122.162206025503)) ;
#31322=CARTESIAN_POINT('Ctrl Pts',(-20.0983757918957,39.3016625108608,122.412145538287)) ;
#31323=CARTESIAN_POINT('Ctrl Pts',(-20.5265366200315,39.4949364471453,122.399782063078)) ;
#31324=CARTESIAN_POINT('Ctrl Pts',(-20.3030677424335,39.3149473667824,122.602175696939)) ;
#31325=CARTESIAN_POINT('Ctrl Pts',(-20.6848475062148,39.5049086743181,122.608570519109)) ;
#31326=CARTESIAN_POINT('Ctrl Pts',(-20.4297258566199,39.3249195939552,122.769211054602)) ;
#31327=CARTESIAN_POINT('Ctrl Pts',(-20.8041722375231,39.5148172907571,122.840044926829)) ;
#31328=CARTESIAN_POINT('Ctrl Pts',(-20.5251856336139,39.3348282103942,122.954388023249)) ;
#31329=CARTESIAN_POINT('Ctrl Pts',(-20.8825021974907,39.5248704961408,123.09232602936)) ;
#31330=CARTESIAN_POINT('Ctrl Pts',(-20.5878516382789,39.3448814157779,123.156213664846)) ;
#31331=CARTESIAN_POINT('Ctrl Pts',(-20.9153854640603,39.5347356299011,123.349500706136)) ;
#31332=CARTESIAN_POINT('Ctrl Pts',(-20.6141617865867,39.3547465495382,123.361949101435)) ;
#31333=CARTESIAN_POINT('Ctrl Pts',(-20.8994475638338,39.5480746875274,123.699654940672)) ;
#31334=CARTESIAN_POINT('Ctrl Pts',(-20.6014062025632,39.3680856071645,123.642094456117)) ;
#31335=CARTESIAN_POINT('Ctrl Pts',(-20.7662626209752,39.5646438748606,124.119481950554)) ;
#31336=CARTESIAN_POINT('Ctrl Pts',(-20.4948802699597,39.3846547944977,123.977922342078)) ;
#31337=CARTESIAN_POINT('Ctrl Pts',(-20.4969232972869,39.5812890147116,124.470352991445)) ;
#31338=CARTESIAN_POINT('Ctrl Pts',(-20.2793689415074,39.4012999343487,124.258669314264)) ;
#31339=CARTESIAN_POINT('Ctrl Pts',(-20.2201055636797,39.594561317185,124.682635504472)) ;
#31340=CARTESIAN_POINT('Ctrl Pts',(-20.0579520034563,39.4145722368221,124.428460073727)) ;
#31341=CARTESIAN_POINT('Ctrl Pts',(-19.9875926506158,39.6045422806326,124.803956293346)) ;
#31342=CARTESIAN_POINT('Ctrl Pts',(-19.8719346104858,39.4245532002698,124.525525821103)) ;
#31343=CARTESIAN_POINT('Ctrl Pts',(-19.7385233068285,39.6144841127019,124.882919421765)) ;
#31344=CARTESIAN_POINT('Ctrl Pts',(-19.6726839339702,39.4344950323391,124.588696443466)) ;
#31345=CARTESIAN_POINT('Ctrl Pts',(-19.3916274184842,39.6278036819174,124.929289096296)) ;
#31346=CARTESIAN_POINT('Ctrl Pts',(-19.3951539287029,39.4478146015545,124.625793702536)) ;
#31347=CARTESIAN_POINT('Ctrl Pts',(-18.9557155359981,39.6443338368501,124.873608604834)) ;
#31348=CARTESIAN_POINT('Ctrl Pts',(-19.0464382212822,39.4643447564872,124.581253473117)) ;
#31349=CARTESIAN_POINT('Ctrl Pts',(-18.4827841914937,39.6643555623422,124.629948165702)) ;
#31350=CARTESIAN_POINT('Ctrl Pts',(-18.6680869357579,39.4843664819793,124.386327764593)) ;
#31351=CARTESIAN_POINT('Ctrl Pts',(-18.1247857375982,39.684166958949,124.243642886315)) ;
#31352=CARTESIAN_POINT('Ctrl Pts',(-18.3816862675463,39.5041778785861,124.077284936914)) ;
#31353=CARTESIAN_POINT('Ctrl Pts',(-17.9175888921553,39.7041522076579,123.754678947954)) ;
#31354=CARTESIAN_POINT('Ctrl Pts',(-18.2159257535573,39.524163127295,123.686114759911)) ;
#31355=CARTESIAN_POINT('Ctrl Pts',(-17.8901646194333,39.7240462702938,123.226554358752)) ;
#31356=CARTESIAN_POINT('Ctrl Pts',(-18.1939835441653,39.5440571899309,123.263614485181)) ;
#31357=CARTESIAN_POINT('Ctrl Pts',(-18.0441177194512,39.7439779494674,122.719677099901)) ;
#31358=CARTESIAN_POINT('Ctrl Pts',(-18.3171437873971,39.5639888691045,122.858111428602)) ;
#31359=CARTESIAN_POINT('Ctrl Pts',(-18.3626008286604,39.7639420039394,122.295272619757)) ;
#31360=CARTESIAN_POINT('Ctrl Pts',(-18.5719284738746,39.5839529235765,122.518586147516)) ;
#31361=CARTESIAN_POINT('Ctrl Pts',(-18.8047431638309,39.7838229057023,122.005888410444)) ;
#31362=CARTESIAN_POINT('Ctrl Pts',(-18.9256420531025,39.6038338253394,122.287076349787)) ;
#31363=CARTESIAN_POINT('Ctrl Pts',(-19.3204270314315,39.8037615673107,121.883932996576)) ;
#31364=CARTESIAN_POINT('Ctrl Pts',(-19.3381893000524,39.6237724869478,122.189510074961)) ;
#31365=CARTESIAN_POINT('Ctrl Pts',(-19.8456885699466,39.823658092566,121.945064977875)) ;
#31366=CARTESIAN_POINT('Ctrl Pts',(-19.7583997745947,39.6436690122031,122.238414117191)) ;
#31367=CARTESIAN_POINT('Ctrl Pts',(-20.3189371293568,39.8435531310203,122.180988955681)) ;
#31368=CARTESIAN_POINT('Ctrl Pts',(-20.1370001890922,39.6635640506575,122.427152812222)) ;
#31369=CARTESIAN_POINT('Ctrl Pts',(-20.684435302286,39.8635169543264,122.565581974928)) ;
#31370=CARTESIAN_POINT('Ctrl Pts',(-20.4293997300506,39.6835278739635,122.734826840731)) ;
#31371=CARTESIAN_POINT('Ctrl Pts',(-20.8961892011034,39.8833910784555,123.049543285432)) ;
#31372=CARTESIAN_POINT('Ctrl Pts',(-20.5988040313383,39.7034019980926,123.121997016737)) ;
#31373=CARTESIAN_POINT('Ctrl Pts',(-20.9307446999035,39.9033661541827,123.579345858903)) ;
#31374=CARTESIAN_POINT('Ctrl Pts',(-20.6264486432097,39.7233770738199,123.54583933781)) ;
#31375=CARTESIAN_POINT('Ctrl Pts',(-20.7818723368726,39.9233197235393,124.088346140046)) ;
#31376=CARTESIAN_POINT('Ctrl Pts',(-20.5073509383854,39.7433306431764,123.953040241885)) ;
#31377=CARTESIAN_POINT('Ctrl Pts',(-20.4708597448831,39.9431576337272,124.514109737929)) ;
#31378=CARTESIAN_POINT('Ctrl Pts',(-20.2585393443571,39.7631685533643,124.293652633685)) ;
#31379=CARTESIAN_POINT('Ctrl Pts',(-20.0304987770853,39.9631334622981,124.810695893572)) ;
#31380=CARTESIAN_POINT('Ctrl Pts',(-19.9062499102217,39.7831443819352,124.53092102101)) ;
#31381=CARTESIAN_POINT('Ctrl Pts',(-19.5167467254977,39.9830515070084,124.938262136295)) ;
#31382=CARTESIAN_POINT('Ctrl Pts',(-19.4952471367361,39.8030624266455,124.632973548658)) ;
#31383=CARTESIAN_POINT('Ctrl Pts',(-18.9912829799873,40.002921752796,124.884310017349)) ;
#31384=CARTESIAN_POINT('Ctrl Pts',(-19.0748749155325,39.8229326724332,124.589810226705)) ;
#31385=CARTESIAN_POINT('Ctrl Pts',(-18.512059067701,40.0229707558956,124.651607827821)) ;
#31386=CARTESIAN_POINT('Ctrl Pts',(-18.691496813196,39.8429816755327,124.403647475634)) ;
#31387=CARTESIAN_POINT('Ctrl Pts',(-18.1453823899898,40.0427499971364,124.274685535331)) ;
#31388=CARTESIAN_POINT('Ctrl Pts',(-18.3981551846587,39.8627609167736,124.10210688277)) ;
#31389=CARTESIAN_POINT('Ctrl Pts',(-17.9259795061986,40.0627800608453,123.789764142162)) ;
#31390=CARTESIAN_POINT('Ctrl Pts',(-18.2226350126772,39.8827909804824,123.714169148054)) ;
#31391=CARTESIAN_POINT('Ctrl Pts',(-17.8863640755832,40.0826623457473,123.26273048994)) ;
#31392=CARTESIAN_POINT('Ctrl Pts',(-18.1909445989057,39.9026732653844,123.292541016045)) ;
#31393=CARTESIAN_POINT('Ctrl Pts',(-18.0275270007879,40.1025446466403,122.753544083108)) ;
#31394=CARTESIAN_POINT('Ctrl Pts',(-18.3038777717334,39.9225555662774,122.885191650426)) ;
#31395=CARTESIAN_POINT('Ctrl Pts',(-18.3357032518353,40.1225277562586,122.320964219485)) ;
#31396=CARTESIAN_POINT('Ctrl Pts',(-18.5504210502982,39.9425386758957,122.539129268786)) ;
#31397=CARTESIAN_POINT('Ctrl Pts',(-18.7710249752049,40.1424181516365,122.020953450762)) ;
#31398=CARTESIAN_POINT('Ctrl Pts',(-18.8986807002394,39.9624290712736,122.299122526392)) ;
#31399=CARTESIAN_POINT('Ctrl Pts',(-19.2824556627369,40.1623149416708,121.886718883341)) ;
#31400=CARTESIAN_POINT('Ctrl Pts',(-19.3078267411535,39.9823258613079,122.191737773976)) ;
#31401=CARTESIAN_POINT('Ctrl Pts',(-19.809682792952,40.1822319956124,121.93454660401)) ;
#31402=CARTESIAN_POINT('Ctrl Pts',(-19.7296086094093,40.0022429152495,122.230003389753)) ;
#31403=CARTESIAN_POINT('Ctrl Pts',(-20.290985297749,40.2022355438159,122.160572440253)) ;
#31404=CARTESIAN_POINT('Ctrl Pts',(-20.1146490294153,40.022246463453,122.410827178833)) ;
#31405=CARTESIAN_POINT('Ctrl Pts',(-20.6644175476188,40.2221738374685,122.536530476513)) ;
#31406=CARTESIAN_POINT('Ctrl Pts',(-20.4133927604481,40.0421847571056,122.711596130847)) ;
#31407=CARTESIAN_POINT('Ctrl Pts',(-20.8870164933769,40.2419953249014,123.014022848812)) ;
#31408=CARTESIAN_POINT('Ctrl Pts',(-20.591468541711,40.0620062445386,123.093592852938)) ;
#31409=CARTESIAN_POINT('Ctrl Pts',(-20.9342078753314,40.2619737178923,123.54285440319)) ;
#31410=CARTESIAN_POINT('Ctrl Pts',(-20.629219041352,40.0819846375294,123.51665686398)) ;
#31411=CARTESIAN_POINT('Ctrl Pts',(-20.798306014332,40.281872099506,124.054044528013)) ;
#31412=CARTESIAN_POINT('Ctrl Pts',(-20.5204887803847,40.1018830191431,123.925614389338)) ;
#31413=CARTESIAN_POINT('Ctrl Pts',(-20.5470819880528,40.2984550302359,124.416062159147)) ;
#31414=CARTESIAN_POINT('Ctrl Pts',(-20.319521718774,40.118465949873,124.215207873857)) ;
#31415=CARTESIAN_POINT('Ctrl Pts',(-20.281028441282,40.3117292658247,124.641768863592)) ;
#31416=CARTESIAN_POINT('Ctrl Pts',(-20.1066630077281,40.1317401854619,124.39578795603)) ;
#31417=CARTESIAN_POINT('Ctrl Pts',(-20.0530654837522,40.3217756832809,124.774877815114)) ;
#31418=CARTESIAN_POINT('Ctrl Pts',(-19.9242972790721,40.1417866029181,124.50226984556)) ;
#31419=CARTESIAN_POINT('Ctrl Pts',(-19.810464403995,40.3316209085002,124.864833820521)) ;
#31420=CARTESIAN_POINT('Ctrl Pts',(-19.7302036734289,40.1516318281373,124.574233889448)) ;
#31421=CARTESIAN_POINT('Ctrl Pts',(-19.4658929191224,40.3449558795396,124.928504806225)) ;
#31422=CARTESIAN_POINT('Ctrl Pts',(-19.4546005727731,40.1649667991767,124.625166764035)) ;
#31423=CARTESIAN_POINT('Ctrl Pts',(-19.0264390688312,40.3615387363322,124.893652813554)) ;
#31424=CARTESIAN_POINT('Ctrl Pts',(-19.1029686872478,40.1815496559694,124.597278988789)) ;
#31425=CARTESIAN_POINT('Ctrl Pts',(-18.6239205040509,40.3781817386816,124.71045606654)) ;
#31426=CARTESIAN_POINT('Ctrl Pts',(-18.7810022090588,40.1981926583188,124.450732338554)) ;
#31427=CARTESIAN_POINT('Ctrl Pts',(-18.3550031410799,40.3914254697133,124.489405088402)) ;
#31428=CARTESIAN_POINT('Ctrl Pts',(-18.5658419708258,40.2114363893504,124.273876441203)) ;
#31429=CARTESIAN_POINT('Ctrl Pts',(-18.1831556506858,40.4014798643879,124.288773158582)) ;
#31430=CARTESIAN_POINT('Ctrl Pts',(-18.4283713813035,40.221490784025,124.113372135424)) ;
#31431=CARTESIAN_POINT('Ctrl Pts',(-18.0512693189918,40.4113209257765,124.066262657595)) ;
#31432=CARTESIAN_POINT('Ctrl Pts',(-18.3228626055422,40.2313318454136,123.935361746005)) ;
#31433=CARTESIAN_POINT('Ctrl Pts',(-17.9577246777451,40.421387150133,123.818872622899)) ;
#31434=CARTESIAN_POINT('Ctrl Pts',(-18.2480294373586,40.2413980697701,123.737449245068)) ;
#31435=CARTESIAN_POINT('Ctrl Pts',(-17.9095230457467,40.4312677630526,123.563691114021)) ;
#31436=CARTESIAN_POINT('Ctrl Pts',(-18.2094701905773,40.2512786826897,123.533303479069)) ;
#31437=CARTESIAN_POINT('Ctrl Pts',(-17.9058281378729,40.4412610562122,123.30114626875)) ;
#31438=CARTESIAN_POINT('Ctrl Pts',(-18.2065165443278,40.2612719758493,123.323267634952)) ;
#31439=CARTESIAN_POINT('Ctrl Pts',(-17.9475138799179,40.4512120644359,123.042941598617)) ;
#31440=CARTESIAN_POINT('Ctrl Pts',(-18.2398673462306,40.271222984073,123.116704268342)) ;
#31441=CARTESIAN_POINT('Ctrl Pts',(-18.0344070397604,40.4612605787978,122.793614478542)) ;
#31442=CARTESIAN_POINT('Ctrl Pts',(-18.3093839709595,40.281271498435,122.917243386907)) ;
#31443=CARTESIAN_POINT('Ctrl Pts',(-18.1603863836437,40.4711020848605,122.567719550063)) ;
#31444=CARTESIAN_POINT('Ctrl Pts',(-18.4101694281105,40.2911130044976,122.736528509964)) ;
#31445=CARTESIAN_POINT('Ctrl Pts',(-18.3255788630243,40.4810877374902,122.36388078949)) ;
#31446=CARTESIAN_POINT('Ctrl Pts',(-18.5423251289196,40.3010986571273,122.573458977904)) ;
#31447=CARTESIAN_POINT('Ctrl Pts',(-18.5227257140879,40.4910267463351,122.192496536557)) ;
#31448=CARTESIAN_POINT('Ctrl Pts',(-18.7000440471516,40.3110376659722,122.436353315188)) ;
#31449=CARTESIAN_POINT('Ctrl Pts',(-18.7489120153398,40.5010676716281,122.056659651422)) ;
#31450=CARTESIAN_POINT('Ctrl Pts',(-18.8809942079959,40.3210785912652,122.327685771661)) ;
#31451=CARTESIAN_POINT('Ctrl Pts',(-18.9915421154482,40.510957993383,121.963416273453)) ;
#31452=CARTESIAN_POINT('Ctrl Pts',(-19.0750990226228,40.3309689130201,122.253093205079)) ;
#31453=CARTESIAN_POINT('Ctrl Pts',(-19.249284101431,40.5209539667164,121.912814957505)) ;
#31454=CARTESIAN_POINT('Ctrl Pts',(-19.2812929812387,40.3409648863536,122.212614377811)) ;
#31455=CARTESIAN_POINT('Ctrl Pts',(-19.5102329048635,40.5308853662985,121.907746825893)) ;
#31456=CARTESIAN_POINT('Ctrl Pts',(-19.4900519685887,40.3508962859356,122.208562125718)) ;
#31457=CARTESIAN_POINT('Ctrl Pts',(-19.7700821945994,40.5408909067755,121.947997275359)) ;
#31458=CARTESIAN_POINT('Ctrl Pts',(-19.697930995272,40.3609018264127,122.240764692487)) ;
#31459=CARTESIAN_POINT('Ctrl Pts',(-20.0195011590798,40.5509238907068,122.033437044935)) ;
#31460=CARTESIAN_POINT('Ctrl Pts',(-19.8974654062638,40.370934810344,122.30911863456)) ;
#31461=CARTESIAN_POINT('Ctrl Pts',(-20.2464637604241,40.5607795215337,122.158246335581)) ;
#31462=CARTESIAN_POINT('Ctrl Pts',(-20.0790342417892,40.3807904411708,122.408967940428)) ;
#31463=CARTESIAN_POINT('Ctrl Pts',(-20.4514141919689,40.5707789237268,122.322629146748)) ;
#31464=CARTESIAN_POINT('Ctrl Pts',(-20.2429931328991,40.390789843364,122.540475886912)) ;
#31465=CARTESIAN_POINT('Ctrl Pts',(-20.623177160939,40.5806733930879,122.517901168788)) ;
#31466=CARTESIAN_POINT('Ctrl Pts',(-20.3804017081287,40.400684312725,122.696694807102)) ;
#31467=CARTESIAN_POINT('Ctrl Pts',(-20.7606139057598,40.5907365072521,122.743776897285)) ;
#31468=CARTESIAN_POINT('Ctrl Pts',(-20.4903492208581,40.4107474268893,122.87739656958)) ;
#31469=CARTESIAN_POINT('Ctrl Pts',(-20.8549063786372,40.6005761529685,122.984593090461)) ;
#31470=CARTESIAN_POINT('Ctrl Pts',(-20.5657810296931,40.4205870726056,123.070050018048)) ;
#31471=CARTESIAN_POINT('Ctrl Pts',(-20.9074265587478,40.6106393205242,123.243737629738)) ;
#31472=CARTESIAN_POINT('Ctrl Pts',(-20.6077950427695,40.4306502401614,123.277366118892)) ;
#31473=CARTESIAN_POINT('Ctrl Pts',(-20.9138213840196,40.6205335763191,123.50369845043)) ;
#31474=CARTESIAN_POINT('Ctrl Pts',(-20.6129087015084,40.4405444959563,123.48533456448)) ;
#31475=CARTESIAN_POINT('Ctrl Pts',(-20.8755072031584,40.6304753547788,123.762100783259)) ;
#31476=CARTESIAN_POINT('Ctrl Pts',(-20.5822552681282,40.4504862744159,123.692055906574)) ;
#31477=CARTESIAN_POINT('Ctrl Pts',(-20.7924699762297,40.640478047609,124.011537115954)) ;
#31478=CARTESIAN_POINT('Ctrl Pts',(-20.5158234865121,40.4604889672461,123.891604236471)) ;
#31479=CARTESIAN_POINT('Ctrl Pts',(-20.6666615752292,40.6505120695628,124.243257679907)) ;
#31480=CARTESIAN_POINT('Ctrl Pts',(-20.4151748534295,40.4705229891999,124.076979664182)) ;
#31481=CARTESIAN_POINT('Ctrl Pts',(-20.5058740591058,40.6603598606518,124.446047890609)) ;
#31482=CARTESIAN_POINT('Ctrl Pts',(-20.2865434507489,40.480370780289,124.239210154722)) ;
#31483=CARTESIAN_POINT('Ctrl Pts',(-20.3100969713907,40.6703413852009,124.620584309683)) ;
#31484=CARTESIAN_POINT('Ctrl Pts',(-20.1299205038193,40.490352304838,124.378837647099)) ;
#31485=CARTESIAN_POINT('Ctrl Pts',(-20.0876630799493,40.6802906086918,124.75801282759)) ;
#31486=CARTESIAN_POINT('Ctrl Pts',(-19.9519724829499,40.5003015283289,124.488778579875)) ;
#31487=CARTESIAN_POINT('Ctrl Pts',(-19.8436735816779,40.6902882649084,124.85551512015)) ;
#31488=CARTESIAN_POINT('Ctrl Pts',(-19.7567802051122,40.5102991845455,124.566778487717)) ;
#31489=CARTESIAN_POINT('Ctrl Pts',(-19.5853011891557,40.7003284779634,124.908895920478)) ;
#31490=CARTESIAN_POINT('Ctrl Pts',(-19.5500818185997,40.5203393976006,124.609481080196)) ;
#31491=CARTESIAN_POINT('Ctrl Pts',(-19.3271425182227,40.7101565252397,124.917006738006)) ;
#31492=CARTESIAN_POINT('Ctrl Pts',(-19.3435554357432,40.5301674448768,124.615967681454)) ;
#31493=CARTESIAN_POINT('Ctrl Pts',(-19.0655819825205,40.7202108722721,124.87973320103)) ;
#31494=CARTESIAN_POINT('Ctrl Pts',(-19.1343072015728,40.5402217919092,124.58614687555)) ;
#31495=CARTESIAN_POINT('Ctrl Pts',(-18.8174100404169,40.7301520086006,124.798108890604)) ;
#31496=CARTESIAN_POINT('Ctrl Pts',(-18.9357705393896,40.5501629282377,124.520845572302)) ;
#31497=CARTESIAN_POINT('Ctrl Pts',(-18.5876566119404,40.7400562416803,124.675804537039)) ;
#31498=CARTESIAN_POINT('Ctrl Pts',(-18.7519690826901,40.5600671613174,124.423000582265)) ;
#31499=CARTESIAN_POINT('Ctrl Pts',(-18.3798041844874,40.7501029385239,124.513046489696)) ;
#31500=CARTESIAN_POINT('Ctrl Pts',(-18.5856882820567,40.5701138581611,124.292792552084)) ;
#31501=CARTESIAN_POINT('Ctrl Pts',(-18.2058043531865,40.7599984898042,124.319735002295)) ;
#31502=CARTESIAN_POINT('Ctrl Pts',(-18.4464901583571,40.5800094094413,124.138142422738)) ;
#31503=CARTESIAN_POINT('Ctrl Pts',(-18.0657367626924,40.7700605676437,124.095504335531)) ;
#31504=CARTESIAN_POINT('Ctrl Pts',(-18.3344376418936,40.5900714872808,123.958756744868)) ;
#31505=CARTESIAN_POINT('Ctrl Pts',(-17.9687267603788,40.7799032767398,123.855697491767)) ;
#31506=CARTESIAN_POINT('Ctrl Pts',(-18.2568316638286,40.5999141963769,123.766911199684)) ;
#31507=CARTESIAN_POINT('Ctrl Pts',(-17.9134237543617,40.7898940089782,123.599076400319)) ;
#31508=CARTESIAN_POINT('Ctrl Pts',(-18.2125910590899,40.6099049286153,123.561614081908)) ;
#31509=CARTESIAN_POINT('Ctrl Pts',(-17.9036209757213,40.799822034207,123.33834843595)) ;
#31510=CARTESIAN_POINT('Ctrl Pts',(-18.2047506639829,40.6198329538441,123.353032033196)) ;
#31511=CARTESIAN_POINT('Ctrl Pts',(-17.9390103972283,40.8098101808575,123.07826099235)) ;
#31512=CARTESIAN_POINT('Ctrl Pts',(-18.2330639096619,40.6298211004947,123.144962455833)) ;
#31513=CARTESIAN_POINT('Ctrl Pts',(-18.0197805146774,40.8198451986975,122.827221506658)) ;
#31514=CARTESIAN_POINT('Ctrl Pts',(-18.2976817439703,40.6398561183346,122.944131364963)) ;
#31515=CARTESIAN_POINT('Ctrl Pts',(-18.1405769536225,40.8297099958027,122.597859805826)) ;
#31516=CARTESIAN_POINT('Ctrl Pts',(-18.394320133305,40.6497209154398,122.76064343955)) ;
#31517=CARTESIAN_POINT('Ctrl Pts',(-18.3003100262152,40.8396707281588,122.390481778754)) ;
#31518=CARTESIAN_POINT('Ctrl Pts',(-18.5221077146717,40.6596816477959,122.594742235113)) ;
#31519=CARTESIAN_POINT('Ctrl Pts',(-18.4953203364736,40.8497041905558,122.213037685501)) ;
#31520=CARTESIAN_POINT('Ctrl Pts',(-18.6781171657498,40.6697151101929,122.452788175949)) ;
#31521=CARTESIAN_POINT('Ctrl Pts',(-18.7146955767961,40.8595897247672,122.073836456238)) ;
#31522=CARTESIAN_POINT('Ctrl Pts',(-18.8536176951084,40.6796006444043,122.341428911214)) ;
#31523=CARTESIAN_POINT('Ctrl Pts',(-18.9592101605245,40.8696545654472,121.973078301155)) ;
#31524=CARTESIAN_POINT('Ctrl Pts',(-19.0492301753213,40.6896654850843,122.260823821511)) ;
#31525=CARTESIAN_POINT('Ctrl Pts',(-19.2119712899475,40.8795026971761,121.917403865115)) ;
#31526=CARTESIAN_POINT('Ctrl Pts',(-19.2514386073647,40.6995136168132,122.216286026283)) ;
#31527=CARTESIAN_POINT('Ctrl Pts',(-19.4752106016322,40.8895301941662,121.905583046178)) ;
#31528=CARTESIAN_POINT('Ctrl Pts',(-19.4620301548535,40.7095411138033,122.206830852572)) ;
#31529=CARTESIAN_POINT('Ctrl Pts',(-19.7364587404572,40.8995586462113,121.940346685251)) ;
#31530=CARTESIAN_POINT('Ctrl Pts',(-19.6710285077072,40.7195695658484,122.234643374607)) ;
#31531=CARTESIAN_POINT('Ctrl Pts',(-19.9832352577145,40.9094039127754,122.018011497405)) ;
#31532=CARTESIAN_POINT('Ctrl Pts',(-19.8684484097077,40.7294148324125,122.296776407657)) ;
#31533=CARTESIAN_POINT('Ctrl Pts',(-20.2165109099258,40.9193945857163,122.138492853158)) ;
#31534=CARTESIAN_POINT('Ctrl Pts',(-20.0550681579274,40.7394055053534,122.393162648683)) ;
#31535=CARTESIAN_POINT('Ctrl Pts',(-20.4259458604295,40.9294324678048,122.29886132802)) ;
#31536=CARTESIAN_POINT('Ctrl Pts',(-20.2226152908657,40.7494433874419,122.521458685121)) ;
#31537=CARTESIAN_POINT('Ctrl Pts',(-20.6012563123727,40.9392768382444,122.489117146691)) ;
#31538=CARTESIAN_POINT('Ctrl Pts',(-20.3628619804321,40.7592877578816,122.67366360375)) ;
#31539=CARTESIAN_POINT('Ctrl Pts',(-20.7432721400069,40.9492616656398,122.709711313099)) ;
#31540=CARTESIAN_POINT('Ctrl Pts',(-20.4764734396498,40.7692725852769,122.850139473825)) ;
#31541=CARTESIAN_POINT('Ctrl Pts',(-20.844502824681,40.9592011110451,122.950536538216)) ;
#31542=CARTESIAN_POINT('Ctrl Pts',(-20.5574566433733,40.7792120306822,123.042799745308)) ;
#31543=CARTESIAN_POINT('Ctrl Pts',(-20.9028785373405,40.969241115331,123.20781127082)) ;
#31544=CARTESIAN_POINT('Ctrl Pts',(-20.6041559783071,40.7892520349681,123.24861993569)) ;
#31545=CARTESIAN_POINT('Ctrl Pts',(-20.9156810985871,40.9791282245166,123.46734861019)) ;
#31546=CARTESIAN_POINT('Ctrl Pts',(-20.6143967389084,40.7991391441538,123.456249117252)) ;
#31547=CARTESIAN_POINT('Ctrl Pts',(-20.8831859202662,40.9891282844191,123.728082234662)) ;
#31548=CARTESIAN_POINT('Ctrl Pts',(-20.5883994360712,40.8091392040562,123.664835757104)) ;
#31549=CARTESIAN_POINT('Ctrl Pts',(-20.8067389220528,40.9990457003338,123.977282854265)) ;
#31550=CARTESIAN_POINT('Ctrl Pts',(-20.5272409208135,40.8190566199709,123.864195371173)) ;
#31551=CARTESIAN_POINT('Ctrl Pts',(-20.6866067690655,41.0090925150746,124.212346711425)) ;
#31552=CARTESIAN_POINT('Ctrl Pts',(-20.4311340955001,40.8291034347117,124.052246084703)) ;
#31553=CARTESIAN_POINT('Ctrl Pts',(-20.5303634279957,41.0189679922713,124.419613620439)) ;
#31554=CARTESIAN_POINT('Ctrl Pts',(-20.3061390542249,40.8389789119084,124.218058285258)) ;
#31555=CARTESIAN_POINT('Ctrl Pts',(-20.3371972791705,41.0290240879925,124.599886515678)) ;
#31556=CARTESIAN_POINT('Ctrl Pts',(-20.1516052586008,40.8490350076296,124.362275967077)) ;
#31557=CARTESIAN_POINT('Ctrl Pts',(-20.1192272911797,41.0389172500076,124.741681401867)) ;
#31558=CARTESIAN_POINT('Ctrl Pts',(-19.9772293226388,40.8589281696447,124.475710604766)) ;
#31559=CARTESIAN_POINT('Ctrl Pts',(-19.8759671921668,41.0489794860302,124.845254462117)) ;
#31560=CARTESIAN_POINT('Ctrl Pts',(-19.7826206014674,40.8689904056673,124.558568216301)) ;
#31561=CARTESIAN_POINT('Ctrl Pts',(-19.6239559484601,41.0588239516591,124.903758180381)) ;
#31562=CARTESIAN_POINT('Ctrl Pts',(-19.5810124074109,40.8788348712962,124.605369962764)) ;
#31563=CARTESIAN_POINT('Ctrl Pts',(-19.3626471098562,41.0687840443633,124.918720690763)) ;
#31564=CARTESIAN_POINT('Ctrl Pts',(-19.3719656563023,40.8887949640004,124.61733915855)) ;
#31565=CARTESIAN_POINT('Ctrl Pts',(-19.1007386053563,41.0788223333443,124.887329010187)) ;
#31566=CARTESIAN_POINT('Ctrl Pts',(-19.16243883266,40.8988332529814,124.592224889164)) ;
#31567=CARTESIAN_POINT('Ctrl Pts',(-18.8522137572535,41.0886956564505,124.812656518733)) ;
#31568=CARTESIAN_POINT('Ctrl Pts',(-18.9636200453775,40.9087065760876,124.532486393259)) ;
#31569=CARTESIAN_POINT('Ctrl Pts',(-18.6158596069558,41.0987688405356,124.693571352366)) ;
#31570=CARTESIAN_POINT('Ctrl Pts',(-18.7745367877756,40.9187797601727,124.437217376295)) ;
#31571=CARTESIAN_POINT('Ctrl Pts',(-18.4088042083935,41.1085893528235,124.539431437794)) ;
#31572=CARTESIAN_POINT('Ctrl Pts',(-18.6088939047249,40.9286002724607,124.313905598339)) ;
#31573=CARTESIAN_POINT('Ctrl Pts',(-18.2269108302998,41.1186673489393,124.347022071441)) ;
#31574=CARTESIAN_POINT('Ctrl Pts',(-18.4633794360143,40.9386782685765,124.159977371275)) ;
#31575=CARTESIAN_POINT('Ctrl Pts',(-18.0843084263497,41.1285214239226,124.130796993338)) ;
#31576=CARTESIAN_POINT('Ctrl Pts',(-18.349298634213,40.9485323435597,123.986997811558)) ;
#31577=CARTESIAN_POINT('Ctrl Pts',(-17.9790049811939,41.1385853055063,123.888252695276)) ;
#31578=CARTESIAN_POINT('Ctrl Pts',(-18.2650563069979,40.9585962251434,123.792961884212)) ;
#31579=CARTESIAN_POINT('Ctrl Pts',(-17.9185435301409,41.14846873148,123.63561553845)) ;
#31580=CARTESIAN_POINT('Ctrl Pts',(-18.2166879295781,40.9684796511172,123.590852855347)) ;
#31581=CARTESIAN_POINT('Ctrl Pts',(-17.9022681371798,41.1584693354011,123.37336067713)) ;
#31582=CARTESIAN_POINT('Ctrl Pts',(-18.2036681214858,40.9784802550382,123.381049048255)) ;
#31583=CARTESIAN_POINT('Ctrl Pts',(-17.931383888056,41.168389119739,123.114261971927)) ;
#31584=CARTESIAN_POINT('Ctrl Pts',(-18.2269611056014,40.9884000393761,123.17377075239)) ;
#31585=CARTESIAN_POINT('Ctrl Pts',(-18.0060263785442,41.1784364700958,122.861044240447)) ;
#31586=CARTESIAN_POINT('Ctrl Pts',(-18.2866756080612,40.998447389733,122.971196520026)) ;
#31587=CARTESIAN_POINT('Ctrl Pts',(-18.1212813811983,41.1883138123301,122.62841137183)) ;
#31588=CARTESIAN_POINT('Ctrl Pts',(-18.3788795564563,41.0083247319672,122.785091229606)) ;
#31589=CARTESIAN_POINT('Ctrl Pts',(-18.2781294851284,41.1983836934047,122.415344458296)) ;
#31590=CARTESIAN_POINT('Ctrl Pts',(-18.504358563971,41.0183946130419,122.614637662932)) ;
#31591=CARTESIAN_POINT('Ctrl Pts',(-18.4649093676713,41.2082133986064,122.236837854703)) ;
#31592=CARTESIAN_POINT('Ctrl Pts',(-18.6537818070225,41.0282243182436,122.471833474203)) ;
#31593=CARTESIAN_POINT('Ctrl Pts',(-18.684754038693,41.2182800597728,122.089775689271)) ;
#31594=CARTESIAN_POINT('Ctrl Pts',(-18.829657944727,41.03829097941,122.354183767872)) ;
#31595=CARTESIAN_POINT('Ctrl Pts',(-18.922687539533,41.2281702816401,121.985108837478)) ;
#31596=CARTESIAN_POINT('Ctrl Pts',(-19.0200040932344,41.0481812012773,122.270450887395)) ;
#31597=CARTESIAN_POINT('Ctrl Pts',(-19.1775992382533,41.2381624577503,121.922160157756)) ;
#31598=CARTESIAN_POINT('Ctrl Pts',(-19.223933319871,41.0581733773874,122.22009212209)) ;
#31599=CARTESIAN_POINT('Ctrl Pts',(-19.4388247420797,41.2481252878629,121.904728591906)) ;
#31600=CARTESIAN_POINT('Ctrl Pts',(-19.4329133725897,41.0681362075001,122.206147099364)) ;
#31601=CARTESIAN_POINT('Ctrl Pts',(-19.6976771545585,41.2580295002633,121.932097935364)) ;
#31602=CARTESIAN_POINT('Ctrl Pts',(-19.6399945510564,41.0780404199004,122.228042530922)) ;
#31603=CARTESIAN_POINT('Ctrl Pts',(-19.9516776747255,41.2680902143511,122.005343143406)) ;
#31604=CARTESIAN_POINT('Ctrl Pts',(-19.8431952134582,41.0881011339882,122.286638869231)) ;
#31605=CARTESIAN_POINT('Ctrl Pts',(-20.1841049252899,41.2779297173339,122.118737500505)) ;
#31606=CARTESIAN_POINT('Ctrl Pts',(-20.0291359487438,41.097940636971,122.377353840953)) ;
#31607=CARTESIAN_POINT('Ctrl Pts',(-20.3982213435744,41.2879958559003,122.273999666852)) ;
#31608=CARTESIAN_POINT('Ctrl Pts',(-20.2004293795964,41.1080067755374,122.501563713022)) ;
#31609=CARTESIAN_POINT('Ctrl Pts',(-20.5787589735412,41.2978783703863,122.460739928102)) ;
#31610=CARTESIAN_POINT('Ctrl Pts',(-20.3448588816564,41.1178892900235,122.650955244937)) ;
#31611=CARTESIAN_POINT('Ctrl Pts',(-20.7261276816334,41.3078706697419,122.678026456324)) ;
#31612=CARTESIAN_POINT('Ctrl Pts',(-20.4627538900193,41.127881589379,122.82478422743)) ;
#31613=CARTESIAN_POINT('Ctrl Pts',(-20.8332007283246,41.3178237366953,122.916705335846)) ;
#31614=CARTESIAN_POINT('Ctrl Pts',(-20.5484123254759,41.1378346563324,123.01572688204)) ;
#31615=CARTESIAN_POINT('Ctrl Pts',(-20.8976084793145,41.3278584449005,123.172399737523)) ;
#31616=CARTESIAN_POINT('Ctrl Pts',(-20.5999387072137,41.1478693645376,123.220282482398)) ;
#31617=CARTESIAN_POINT('Ctrl Pts',(-20.9165553817096,41.3377466658047,123.431576287923)) ;
#31618=CARTESIAN_POINT('Ctrl Pts',(-20.6150963672015,41.1577575854418,123.427622853528)) ;
#31619=CARTESIAN_POINT('Ctrl Pts',(-20.8903621464779,41.3477410888351,123.692895458737)) ;
#31620=CARTESIAN_POINT('Ctrl Pts',(-20.5941421044658,41.1677520084722,123.636678055488)) ;
#31621=CARTESIAN_POINT('Ctrl Pts',(-20.8194388311831,41.3576864282813,123.944442205965)) ;
#31622=CARTESIAN_POINT('Ctrl Pts',(-20.5374038559839,41.1776973479184,123.837915073439)) ;
#31623=CARTESIAN_POINT('Ctrl Pts',(-20.7063724848582,41.3676337728926,124.180145089931)) ;
#31624=CARTESIAN_POINT('Ctrl Pts',(-20.446951356585,41.1876446925297,124.026477147799)) ;
#31625=CARTESIAN_POINT('Ctrl Pts',(-20.5523289698857,41.3776816683036,124.394591659)) ;
#31626=CARTESIAN_POINT('Ctrl Pts',(-20.3237167077923,41.1976925879407,124.198034766973)) ;
#31627=CARTESIAN_POINT('Ctrl Pts',(-20.3673015896202,41.387529313783,124.575522794134)) ;
#31628=CARTESIAN_POINT('Ctrl Pts',(-20.1756958838239,41.2075402334201,124.342779178533)) ;
#31629=CARTESIAN_POINT('Ctrl Pts',(-20.1516704586702,41.397491027697,124.723938642442)) ;
#31630=CARTESIAN_POINT('Ctrl Pts',(-20.0031916223503,41.2175019473341,124.461512149995)) ;
#31631=CARTESIAN_POINT('Ctrl Pts',(-19.911780850099,41.4075196519879,124.833098044345)) ;
#31632=CARTESIAN_POINT('Ctrl Pts',(-19.8112800810594,41.227530571625,124.548840178017)) ;
#31633=CARTESIAN_POINT('Ctrl Pts',(-19.6596394073023,41.4174300126446,124.898243770015)) ;
#31634=CARTESIAN_POINT('Ctrl Pts',(-19.6095677408918,41.2374409322817,124.600957108251)) ;
#31635=CARTESIAN_POINT('Ctrl Pts',(-19.3994113076568,41.4273647112179,124.91935848404)) ;
#31636=CARTESIAN_POINT('Ctrl Pts',(-19.4013858458597,41.247375630855,124.617849546606)) ;
#31637=CARTESIAN_POINT('Ctrl Pts',(-19.1367143515178,41.4374065360721,124.894447395017)) ;
#31638=CARTESIAN_POINT('Ctrl Pts',(-19.1912280682996,41.2574174557092,124.597921306122)) ;
#31639=CARTESIAN_POINT('Ctrl Pts',(-18.8862194476765,41.4472911098165,124.825610729058)) ;
#31640=CARTESIAN_POINT('Ctrl Pts',(-18.9908327711166,41.2673020294536,124.542852873517)) ;
#31641=CARTESIAN_POINT('Ctrl Pts',(-18.6486170762246,41.4572929591797,124.713315149718)) ;
#31642=CARTESIAN_POINT('Ctrl Pts',(-18.8007506471708,41.2773038788168,124.45301716696)) ;
#31643=CARTESIAN_POINT('Ctrl Pts',(-18.4357242323319,41.4672122607537,124.562839022651)) ;
#31644=CARTESIAN_POINT('Ctrl Pts',(-18.6304363934291,41.2872231803909,124.332637291821)) ;
#31645=CARTESIAN_POINT('Ctrl Pts',(-18.2499195837942,41.477256369099,124.375398346987)) ;
#31646=CARTESIAN_POINT('Ctrl Pts',(-18.4817919703577,41.2972672887361,124.182685211504)) ;
#31647=CARTESIAN_POINT('Ctrl Pts',(-18.1017911287502,41.4871407925413,124.162007655832)) ;
#31648=CARTESIAN_POINT('Ctrl Pts',(-18.3632889812558,41.3071517121784,124.011973815533)) ;
#31649=CARTESIAN_POINT('Ctrl Pts',(-17.9909819762134,41.4971571544507,123.923238127084)) ;
#31650=CARTESIAN_POINT('Ctrl Pts',(-18.27464077142,41.3171680740879,123.820958606205)) ;
#31651=CARTESIAN_POINT('Ctrl Pts',(-17.9238542028585,41.5071938099561,123.66818572458)) ;
#31652=CARTESIAN_POINT('Ctrl Pts',(-18.2209377383296,41.3272047295932,123.616916796119)) ;
#31653=CARTESIAN_POINT('Ctrl Pts',(-17.9017753134138,41.5170239401454,123.410773438911)) ;
#31654=CARTESIAN_POINT('Ctrl Pts',(-18.2032737428897,41.3370348597826,123.410988188349)) ;
#31655=CARTESIAN_POINT('Ctrl Pts',(-17.9252038428856,41.5270999932353,123.147075094843)) ;
#31656=CARTESIAN_POINT('Ctrl Pts',(-18.2220155951886,41.3471109128724,123.2000290831)) ;
#31657=CARTESIAN_POINT('Ctrl Pts',(-17.9924242809587,41.5369522224211,122.896990000681)) ;
#31658=CARTESIAN_POINT('Ctrl Pts',(-18.2757906890744,41.3569631420582,122.999961690913)) ;
#31659=CARTESIAN_POINT('Ctrl Pts',(-18.1042623444851,41.5470254302204,122.657109249406)) ;
#31660=CARTESIAN_POINT('Ctrl Pts',(-18.3652602896576,41.3670363498575,122.808056339764)) ;
#31661=CARTESIAN_POINT('Ctrl Pts',(-18.2526543868681,41.5568669415718,122.445270485562)) ;
#31662=CARTESIAN_POINT('Ctrl Pts',(-18.4839724495599,41.3768778612089,122.638585568541)) ;
#31663=CARTESIAN_POINT('Ctrl Pts',(-18.4370777102109,41.5668278796093,122.259519138152)) ;
#31664=CARTESIAN_POINT('Ctrl Pts',(-18.6315099644499,41.3868387992465,122.489983811783)) ;
#31665=CARTESIAN_POINT('Ctrl Pts',(-18.6529080737898,41.5768657415343,122.107878162832)) ;
#31666=CARTESIAN_POINT('Ctrl Pts',(-18.804173668292,41.3968766611714,122.368670011063)) ;
#31667=CARTESIAN_POINT('Ctrl Pts',(-18.8877262423687,41.5867399275314,121.997383365689)) ;
#31668=CARTESIAN_POINT('Ctrl Pts',(-18.9920269264179,41.4067508471685,122.280273361693)) ;
#31669=CARTESIAN_POINT('Ctrl Pts',(-19.1430711045837,41.5968100871093,121.928030886543)) ;
#31670=CARTESIAN_POINT('Ctrl Pts',(-19.1963027525332,41.4168210067464,122.22479007538)) ;
#31671=CARTESIAN_POINT('Ctrl Pts',(-19.4003882644743,41.6066418345351,121.904466477439)) ;
#31672=CARTESIAN_POINT('Ctrl Pts',(-19.4021553376179,41.4266527541722,122.205937341054)) ;
#31673=CARTESIAN_POINT('Ctrl Pts',(-19.6632563157754,41.6166779146064,121.925697979521)) ;
#31674=CARTESIAN_POINT('Ctrl Pts',(-19.6124499841248,41.4366888342435,122.222921102434)) ;
#31675=CARTESIAN_POINT('Ctrl Pts',(-19.9178188413347,41.6266949614589,121.992773118902)) ;
#31676=CARTESIAN_POINT('Ctrl Pts',(-19.8161003293912,41.446705881096,122.276579942071)) ;
#31677=CARTESIAN_POINT('Ctrl Pts',(-20.1538480381938,41.6365772196255,122.10109797781)) ;
#31678=CARTESIAN_POINT('Ctrl Pts',(-20.0049236160898,41.4565881392626,122.363238243392)) ;
#31679=CARTESIAN_POINT('Ctrl Pts',(-20.3699075386073,41.6465649024218,122.250068895617)) ;
#31680=CARTESIAN_POINT('Ctrl Pts',(-20.1777719215884,41.466575822059,122.482413671685)) ;
#31681=CARTESIAN_POINT('Ctrl Pts',(-20.556247785553,41.6565115591386,122.433432011487)) ;
#31682=CARTESIAN_POINT('Ctrl Pts',(-20.3268449195173,41.4765224787757,122.629102830338)) ;
#31683=CARTESIAN_POINT('Ctrl Pts',(-20.7093408277522,41.6665686172188,122.648828544842)) ;
#31684=CARTESIAN_POINT('Ctrl Pts',(-20.4493206451329,41.4865795368559,122.801419352681)) ;
#31685=CARTESIAN_POINT('Ctrl Pts',(-20.8203574276063,41.6763867967682,122.881750559428)) ;
#31686=CARTESIAN_POINT('Ctrl Pts',(-20.5381348730655,41.4963977164053,122.987755393131)) ;
#31687=CARTESIAN_POINT('Ctrl Pts',(-20.8914554133569,41.6864227312072,123.135713115928)) ;
#31688=CARTESIAN_POINT('Ctrl Pts',(-20.5950148896598,41.5064336508443,123.190925073507)) ;
#31689=CARTESIAN_POINT('Ctrl Pts',(-20.9165972820437,41.6964473856362,123.397957733958)) ;
#31690=CARTESIAN_POINT('Ctrl Pts',(-20.6151299031663,41.5164583052733,123.400720641268)) ;
#31691=CARTESIAN_POINT('Ctrl Pts',(-20.8967522553727,41.7062994052157,123.656101312759)) ;
#31692=CARTESIAN_POINT('Ctrl Pts',(-20.5992555699789,41.5263103248528,123.607234825418)) ;
#31693=CARTESIAN_POINT('Ctrl Pts',(-20.8318758704315,41.7162903189306,123.910477841226)) ;
#31694=CARTESIAN_POINT('Ctrl Pts',(-20.5473561475517,41.5363012385678,123.810736336764)) ;
#31695=CARTESIAN_POINT('Ctrl Pts',(-20.7247343585358,41.7262083077702,124.148106422392)) ;
#31696=CARTESIAN_POINT('Ctrl Pts',(-20.4616447029852,41.5462192274073,124.000839496386)) ;
#31697=CARTESIAN_POINT('Ctrl Pts',(-20.5764123274112,41.736236418501,124.365906529172)) ;
#31698=CARTESIAN_POINT('Ctrl Pts',(-20.3429885028579,41.5562473381381,124.175080585433)) ;
#31699=CARTESIAN_POINT('Ctrl Pts',(-20.395206571467,41.7461216164094,124.552049981452)) ;
#31700=CARTESIAN_POINT('Ctrl Pts',(-20.1980255691353,41.5661325360465,124.323996153329)) ;
#31701=CARTESIAN_POINT('Ctrl Pts',(-20.1825881915492,41.7561108916774,124.706022484706)) ;
#31702=CARTESIAN_POINT('Ctrl Pts',(-20.0279320600952,41.5761218113145,124.447175591284)) ;
#31703=CARTESIAN_POINT('Ctrl Pts',(-19.944994054816,41.7661523498469,124.820818389465)) ;
#31704=CARTESIAN_POINT('Ctrl Pts',(-19.837857454139,41.586163269484,124.539013942928)) ;
#31705=CARTESIAN_POINT('Ctrl Pts',(-19.6965012965203,41.7759838136352,124.891575936423)) ;
#31706=CARTESIAN_POINT('Ctrl Pts',(-19.6390644965111,41.5959947332723,124.595621546985)) ;
#31707=CARTESIAN_POINT('Ctrl Pts',(-19.4350641759092,41.7859887459391,124.919157369809)) ;
#31708=CARTESIAN_POINT('Ctrl Pts',(-19.4299150640357,41.6059996655762,124.61768861319)) ;
#31709=CARTESIAN_POINT('Ctrl Pts',(-19.1732294916453,41.7959751098338,124.900811143185)) ;
#31710=CARTESIAN_POINT('Ctrl Pts',(-19.2204473105258,41.615986029471,124.603013545684)) ;
#31711=CARTESIAN_POINT('Ctrl Pts',(-18.9175714408772,41.8060047387197,124.836821562451)) ;
#31712=CARTESIAN_POINT('Ctrl Pts',(-19.0159203902611,41.6260156583568,124.551823702806)) ;
#31713=CARTESIAN_POINT('Ctrl Pts',(-18.6804315219461,41.8158799608281,124.731353527358)) ;
#31714=CARTESIAN_POINT('Ctrl Pts',(-18.8262081643028,41.6358908804652,124.467451255553)) ;
#31715=CARTESIAN_POINT('Ctrl Pts',(-18.4623421036418,41.8258811732252,124.584757637499)) ;
#31716=CARTESIAN_POINT('Ctrl Pts',(-18.6517356019732,41.6458920928623,124.350176231393)) ;
#31717=CARTESIAN_POINT('Ctrl Pts',(-18.2745387790295,41.8357897524607,124.404326737909)) ;
#31718=CARTESIAN_POINT('Ctrl Pts',(-18.5014918287593,41.6558006720979,124.205833218676)) ;
#31719=CARTESIAN_POINT('Ctrl Pts',(-18.1187665880947,41.8458446050167,124.190948411598)) ;
#31720=CARTESIAN_POINT('Ctrl Pts',(-18.3768724125768,41.6658555246539,124.035131662587)) ;
#31721=CARTESIAN_POINT('Ctrl Pts',(-18.0043751834666,41.8557031872915,123.958446111396)) ;
#31722=CARTESIAN_POINT('Ctrl Pts',(-18.2853576981926,41.6757141069286,123.849131183936)) ;
#31723=CARTESIAN_POINT('Ctrl Pts',(-17.93042449407,41.8657713167342,123.70445148532)) ;
#31724=CARTESIAN_POINT('Ctrl Pts',(-18.2261951440607,41.6857822363713,123.645935938738)) ;
#31725=CARTESIAN_POINT('Ctrl Pts',(-17.9023200741687,41.8756267884233,123.446967189866)) ;
#31726=CARTESIAN_POINT('Ctrl Pts',(-18.2037096291495,41.6956377080604,123.439949220456)) ;
#31727=CARTESIAN_POINT('Ctrl Pts',(-17.9188032302922,41.8856216368096,123.184839420313)) ;
#31728=CARTESIAN_POINT('Ctrl Pts',(-18.2168940227441,41.7056325564467,123.23024695042)) ;
#31729=CARTESIAN_POINT('Ctrl Pts',(-17.9813304619599,41.895652933594,122.928744998837)) ;
#31730=CARTESIAN_POINT('Ctrl Pts',(-18.2669137962854,41.7156638532311,123.025370923546)) ;
#31731=CARTESIAN_POINT('Ctrl Pts',(-18.0852555186611,41.9055194698041,122.691192079478)) ;
#31732=CARTESIAN_POINT('Ctrl Pts',(-18.3500517412046,41.7255303894412,122.835328118647)) ;
#31733=CARTESIAN_POINT('Ctrl Pts',(-18.2302333322929,41.9155068927649,122.472444933182)) ;
#31734=CARTESIAN_POINT('Ctrl Pts',(-18.4660321429773,41.7355178124021,122.66032929391)) ;
#31735=CARTESIAN_POINT('Ctrl Pts',(-18.4101690101242,41.9254518317847,122.282861709824)) ;
#31736=CARTESIAN_POINT('Ctrl Pts',(-18.6099789904463,41.7454627514218,122.508661363733)) ;
#31737=CARTESIAN_POINT('Ctrl Pts',(-18.6224325374237,41.9354967176447,122.125972345834)) ;
#31738=CARTESIAN_POINT('Ctrl Pts',(-18.7797885429512,41.7555076372818,122.38314813357)) ;
#31739=CARTESIAN_POINT('Ctrl Pts',(-18.8545248231622,41.9453652527309,122.010250360349)) ;
#31740=CARTESIAN_POINT('Ctrl Pts',(-18.9654611095548,41.7653761723681,122.290568757108)) ;
#31741=CARTESIAN_POINT('Ctrl Pts',(-19.1054113849967,41.9553311207376,121.935164518734)) ;
#31742=CARTESIAN_POINT('Ctrl Pts',(-19.1661696157605,41.7753420403747,122.230497995113)) ;
#31743=CARTESIAN_POINT('Ctrl Pts',(-19.3670697024523,41.9653537681901,121.904899528248)) ;
#31744=CARTESIAN_POINT('Ctrl Pts',(-19.3754959860251,41.7853646878272,122.206283828786)) ;
#31745=CARTESIAN_POINT('Ctrl Pts',(-19.6273839317657,41.9752774071977,121.920298317369)) ;
#31746=CARTESIAN_POINT('Ctrl Pts',(-19.583747310097,41.7952883268348,122.218600653541)) ;
#31747=CARTESIAN_POINT('Ctrl Pts',(-19.8817304496807,41.9852201322034,121.980174899417)) ;
#31748=CARTESIAN_POINT('Ctrl Pts',(-19.7872249056599,41.8052310518406,122.266499716191)) ;
#31749=CARTESIAN_POINT('Ctrl Pts',(-20.1241484576752,41.9952657382553,122.084651122132)) ;
#31750=CARTESIAN_POINT('Ctrl Pts',(-19.9811601739826,41.8152766578924,122.350078652144)) ;
#31751=CARTESIAN_POINT('Ctrl Pts',(-20.3408862916986,42.0051271607764,122.22675611249)) ;
#31752=CARTESIAN_POINT('Ctrl Pts',(-20.1545514860313,41.8251380804135,122.463760663456)) ;
#31753=CARTESIAN_POINT('Ctrl Pts',(-20.5324507967766,42.0151207292256,122.406346888385)) ;
#31754=CARTESIAN_POINT('Ctrl Pts',(-20.3078045818973,41.8351316488627,122.607431606924)) ;
#31755=CARTESIAN_POINT('Ctrl Pts',(-20.6890036597013,42.0250461999809,122.615019061482)) ;
#31756=CARTESIAN_POINT('Ctrl Pts',(-20.4330486091548,41.845057119618,122.774367895725)) ;
#31757=CARTESIAN_POINT('Ctrl Pts',(-20.808139363818,42.0350738739368,122.850031069966)) ;
#31758=CARTESIAN_POINT('Ctrl Pts',(-20.528359143158,41.8550847935739,122.962376508046)) ;
#31759=CARTESIAN_POINT('Ctrl Pts',(-20.8838479741626,42.0449610519785,123.098617303755)) ;
#31760=CARTESIAN_POINT('Ctrl Pts',(-20.5889282071218,41.8649719716156,123.161244495286)) ;
#31761=CARTESIAN_POINT('Ctrl Pts',(-20.9158670631571,42.0549894313466,123.360164459768)) ;
#31762=CARTESIAN_POINT('Ctrl Pts',(-20.6145455234739,41.8750003509838,123.370482841574)) ;
#31763=CARTESIAN_POINT('Ctrl Pts',(-20.9023097751863,42.0648836740681,123.619854631483)) ;
#31764=CARTESIAN_POINT('Ctrl Pts',(-20.6037026459315,41.8848945937052,123.578231501373)) ;
#31765=CARTESIAN_POINT('Ctrl Pts',(-20.8237470249053,42.078236590719,123.961816174747)) ;
#31766=CARTESIAN_POINT('Ctrl Pts',(-20.540851905552,41.8982475103561,123.851818955548)) ;
#31767=CARTESIAN_POINT('Ctrl Pts',(-20.6595997814835,42.0914391084657,124.272009590654)) ;
#31768=CARTESIAN_POINT('Ctrl Pts',(-20.4095171791971,41.9114500281029,124.099990022592)) ;
#31769=CARTESIAN_POINT('Ctrl Pts',(-20.4209837962718,42.1047950137467,124.529355053645)) ;
#31770=CARTESIAN_POINT('Ctrl Pts',(-20.2186534466242,41.9248059333838,124.305833005313)) ;
#31771=CARTESIAN_POINT('Ctrl Pts',(-20.2138409514704,42.1146916623845,124.686668820964)) ;
#31772=CARTESIAN_POINT('Ctrl Pts',(-20.0529350989336,41.9347025820217,124.431692934571)) ;
#31773=CARTESIAN_POINT('Ctrl Pts',(-19.9790784982733,42.124739800437,124.807498749042)) ;
#31774=CARTESIAN_POINT('Ctrl Pts',(-19.8651277057987,41.9447507200741,124.528356915192)) ;
#31775=CARTESIAN_POINT('Ctrl Pts',(-19.7308134332186,42.1346307606148,124.884508092935)) ;
#31776=CARTESIAN_POINT('Ctrl Pts',(-19.6665158148451,41.9546416802519,124.589967046328)) ;
#31777=CARTESIAN_POINT('Ctrl Pts',(-19.4703782998092,42.1446235964915,124.918232356421)) ;
#31778=CARTESIAN_POINT('Ctrl Pts',(-19.4581682824578,41.9646345161287,124.616948547809)) ;
#31779=CARTESIAN_POINT('Ctrl Pts',(-19.2068788945409,42.1546626914931,124.905562765929)) ;
#31780=CARTESIAN_POINT('Ctrl Pts',(-19.2473681313206,41.9746736111302,124.606814984764)) ;
#31781=CARTESIAN_POINT('Ctrl Pts',(-18.9545800921988,42.1645000473443,124.849083179674)) ;
#31782=CARTESIAN_POINT('Ctrl Pts',(-19.0455306742898,41.9845109669814,124.56163402756)) ;
#31783=CARTESIAN_POINT('Ctrl Pts',(-18.629663451881,42.177892995275,124.713940021359)) ;
#31784=CARTESIAN_POINT('Ctrl Pts',(-18.7855850543186,41.9979039149121,124.453519158685)) ;
#31785=CARTESIAN_POINT('Ctrl Pts',(-18.3520925365356,42.1910596717019,124.500678451702)) ;
#31786=CARTESIAN_POINT('Ctrl Pts',(-18.5635083043611,42.0110705913391,124.282885722299)) ;
#31787=CARTESIAN_POINT('Ctrl Pts',(-18.1378563760038,42.2044444531087,124.221781306289)) ;
#31788=CARTESIAN_POINT('Ctrl Pts',(-18.3921499280378,42.0244553727458,124.059804293663)) ;
#31789=CARTESIAN_POINT('Ctrl Pts',(-18.0179616237773,42.2143062357526,123.991978653527)) ;
#31790=CARTESIAN_POINT('Ctrl Pts',(-18.2962255485433,42.0343171553897,123.875955881791)) ;
#31791=CARTESIAN_POINT('Ctrl Pts',(-17.9383202716689,42.2243053837056,123.741625973935)) ;
#31792=CARTESIAN_POINT('Ctrl Pts',(-18.2325120682241,42.0443163033428,123.675676550641)) ;
#31793=CARTESIAN_POINT('Ctrl Pts',(-17.9034419632737,42.2342081763227,123.483683307464)) ;
#31794=CARTESIAN_POINT('Ctrl Pts',(-18.2046075051605,42.0542190959598,123.469320792753)) ;
#31795=CARTESIAN_POINT('Ctrl Pts',(-17.9141036164672,42.2442577562136,123.21987047093)) ;
#31796=CARTESIAN_POINT('Ctrl Pts',(-18.2131325074826,42.0642686758508,123.258274986974)) ;
#31797=CARTESIAN_POINT('Ctrl Pts',(-17.9873542558445,42.2574448300231,122.881031053165)) ;
#31798=CARTESIAN_POINT('Ctrl Pts',(-18.2717422460334,42.0774557496602,122.987181397706)) ;
#31799=CARTESIAN_POINT('Ctrl Pts',(-18.1910268972478,42.2741976199943,122.48527825742)) ;
#31800=CARTESIAN_POINT('Ctrl Pts',(-18.4346521928802,42.0942085396314,122.670610268033)) ;
#31801=CARTESIAN_POINT('Ctrl Pts',(-18.5127023287359,42.290686272089,122.187393477367)) ;
#31802=CARTESIAN_POINT('Ctrl Pts',(-18.6920409981402,42.1106971917261,122.432258549758)) ;
#31803=CARTESIAN_POINT('Ctrl Pts',(-18.8227825349679,42.3040430982724,122.023091316242)) ;
#31804=CARTESIAN_POINT('Ctrl Pts',(-18.9400618893494,42.1240540179095,122.300845856215)) ;
#31805=CARTESIAN_POINT('Ctrl Pts',(-19.0702507619016,42.3139394831503,121.942948929694)) ;
#31806=CARTESIAN_POINT('Ctrl Pts',(-19.1380453748036,42.1339504027875,122.236723914257)) ;
#31807=CARTESIAN_POINT('Ctrl Pts',(-19.3305991665012,42.3239459976708,121.906474651851)) ;
#31808=CARTESIAN_POINT('Ctrl Pts',(-19.3463190360728,42.1439569173079,122.2075435789)) ;
#31809=CARTESIAN_POINT('Ctrl Pts',(-19.6771578660426,42.3371361211872,121.917859655171)) ;
#31810=CARTESIAN_POINT('Ctrl Pts',(-19.623580039702,42.1571470408243,122.216652401464)) ;
#31811=CARTESIAN_POINT('Ctrl Pts',(-20.1032957575407,42.3539026823368,122.047670197675)) ;
#31812=CARTESIAN_POINT('Ctrl Pts',(-19.9644762057803,42.1739136019739,122.320493865006)) ;
#31813=CARTESIAN_POINT('Ctrl Pts',(-20.5238873611168,42.3736871710448,122.363526341007)) ;
#31814=CARTESIAN_POINT('Ctrl Pts',(-20.3009572541404,42.1936980906819,122.573177890101)) ;
#31815=CARTESIAN_POINT('Ctrl Pts',(-20.8150059840566,42.3936326186413,122.806396279347)) ;
#31816=CARTESIAN_POINT('Ctrl Pts',(-20.5338537200683,42.2136435382784,122.927472140951)) ;
#31817=CARTESIAN_POINT('Ctrl Pts',(-20.9368565339894,42.4135442807972,123.32140844695)) ;
#31818=CARTESIAN_POINT('Ctrl Pts',(-20.6313376522247,42.2335552004343,123.33948182386)) ;
#31819=CARTESIAN_POINT('Ctrl Pts',(-20.8768601174002,42.4334364728161,123.846776921239)) ;
#31820=CARTESIAN_POINT('Ctrl Pts',(-20.583342978862,42.2534473924532,123.759777675271)) ;
#31821=CARTESIAN_POINT('Ctrl Pts',(-20.6387749464663,42.4534776033707,124.323184054214)) ;
#31822=CARTESIAN_POINT('Ctrl Pts',(-20.3928775130821,42.2734885230078,124.140904294275)) ;
#31823=CARTESIAN_POINT('Ctrl Pts',(-20.2567515623942,42.4732959379863,124.686015098705)) ;
#31824=CARTESIAN_POINT('Ctrl Pts',(-20.087259484934,42.2933068576234,124.431172000379)) ;
#31825=CARTESIAN_POINT('Ctrl Pts',(-19.7707111217134,42.4932685032059,124.899002007876)) ;
#31826=CARTESIAN_POINT('Ctrl Pts',(-19.6984277079127,42.313279422843,124.601563631414)) ;
#31827=CARTESIAN_POINT('Ctrl Pts',(-19.2430064355605,42.5131577193775,124.933361056965)) ;
#31828=CARTESIAN_POINT('Ctrl Pts',(-19.2762631018856,42.3331686390146,124.629052843148)) ;
#31829=CARTESIAN_POINT('Ctrl Pts',(-18.7322443545962,42.5331812937002,124.784326245752)) ;
#31830=CARTESIAN_POINT('Ctrl Pts',(-18.8676531273989,42.3531922133373,124.509826918718)) ;
#31831=CARTESIAN_POINT('Ctrl Pts',(-18.3074466869106,42.5529784567885,124.473672881631)) ;
#31832=CARTESIAN_POINT('Ctrl Pts',(-18.5278123342791,42.3729893764256,124.261304267751)) ;
#31833=CARTESIAN_POINT('Ctrl Pts',(-18.0107152101051,42.5729439506122,124.03387590139)) ;
#31834=CARTESIAN_POINT('Ctrl Pts',(-18.2904261458476,42.3929548702494,123.909466818997)) ;
#31835=CARTESIAN_POINT('Ctrl Pts',(-17.8825244705871,42.5928976583536,123.51911914368)) ;
#31836=CARTESIAN_POINT('Ctrl Pts',(-18.1878724815504,42.4129085779908,123.497661231514)) ;
#31837=CARTESIAN_POINT('Ctrl Pts',(-17.9375074674537,42.6128050350802,122.992998485349)) ;
#31838=CARTESIAN_POINT('Ctrl Pts',(-18.2318581752466,42.4328159547174,123.076763483073)) ;
#31839=CARTESIAN_POINT('Ctrl Pts',(-18.1669062692067,42.6326572466288,122.517738273591)) ;
#31840=CARTESIAN_POINT('Ctrl Pts',(-18.4153780968803,42.4526681662659,122.696553635092)) ;
#31841=CARTESIAN_POINT('Ctrl Pts',(-18.5491943143349,42.6527296335745,122.145651577482)) ;
#31842=CARTESIAN_POINT('Ctrl Pts',(-18.721207849793,42.4727405532116,122.398884952664)) ;
#31843=CARTESIAN_POINT('Ctrl Pts',(-19.0301333322148,42.6725675032148,121.929544757103)) ;
#31844=CARTESIAN_POINT('Ctrl Pts',(-19.1059609684924,42.4925784228519,122.225998529547)) ;
#31845=CARTESIAN_POINT('Ctrl Pts',(-19.5561067931665,42.6924181577679,121.88822002276)) ;
#31846=CARTESIAN_POINT('Ctrl Pts',(-19.5267415619836,42.5124290774051,122.19293977911)) ;
#31847=CARTESIAN_POINT('Ctrl Pts',(-20.0695211678143,42.7124700921084,122.031029897398)) ;
#31848=CARTESIAN_POINT('Ctrl Pts',(-19.9374722246251,42.5324810117455,122.307188485913)) ;
#31849=CARTESIAN_POINT('Ctrl Pts',(-20.4987389792293,42.7323032796744,122.33724488066)) ;
#31850=CARTESIAN_POINT('Ctrl Pts',(-20.2808472827428,42.5523141993116,122.552162457419)) ;
#31851=CARTESIAN_POINT('Ctrl Pts',(-20.7998323714999,42.7522324919051,122.772792578482)) ;
#31852=CARTESIAN_POINT('Ctrl Pts',(-20.5217209763658,42.5722434115422,122.900602245168)) ;
#31853=CARTESIAN_POINT('Ctrl Pts',(-20.9346324231233,42.7721174571195,123.284031475315)) ;
#31854=CARTESIAN_POINT('Ctrl Pts',(-20.6295592175581,42.5921283767566,123.309594871732)) ;
#31855=CARTESIAN_POINT('Ctrl Pts',(-20.8856369561692,42.7921911982641,123.815196128951)) ;
#31856=CARTESIAN_POINT('Ctrl Pts',(-20.5903609317186,42.6122021179012,123.734525730611)) ;
#31857=CARTESIAN_POINT('Ctrl Pts',(-20.6614795251124,42.8119843800445,124.291210805294)) ;
#31858=CARTESIAN_POINT('Ctrl Pts',(-20.4110322484531,42.6319952996816,124.115338243655)) ;
#31859=CARTESIAN_POINT('Ctrl Pts',(-20.2863715695943,42.8319470880472,124.666388958395)) ;
#31860=CARTESIAN_POINT('Ctrl Pts',(-20.1109437039454,42.6519580076843,124.415478939255)) ;
#31861=CARTESIAN_POINT('Ctrl Pts',(-19.8046741907438,42.8519300397896,124.890126754003)) ;
#31862=CARTESIAN_POINT('Ctrl Pts',(-19.7255846106919,42.6719409594268,124.594466924686)) ;
#31863=CARTESIAN_POINT('Ctrl Pts',(-19.2801592562473,42.8717406595618,124.936699673532)) ;
#31864=CARTESIAN_POINT('Ctrl Pts',(-19.3059710215937,42.6917515791989,124.631722408354)) ;
#31865=CARTESIAN_POINT('Ctrl Pts',(-18.7667862152892,42.8917243755947,124.800954951219)) ;
#31866=CARTESIAN_POINT('Ctrl Pts',(-18.8952733417193,42.7117352952318,124.523123451149)) ;
#31867=CARTESIAN_POINT('Ctrl Pts',(-18.3326279856665,42.911605839492,124.499507379797)) ;
#31868=CARTESIAN_POINT('Ctrl Pts',(-18.5479481189047,42.7316167591292,124.281962249473)) ;
#31869=CARTESIAN_POINT('Ctrl Pts',(-18.0260984755986,42.9315611693364,124.066807185146)) ;
#31870=CARTESIAN_POINT('Ctrl Pts',(-18.3027271574083,42.7515720889735,123.935799951114)) ;
#31871=CARTESIAN_POINT('Ctrl Pts',(-17.8857662260403,42.9514366301419,123.557444062347)) ;
#31872=CARTESIAN_POINT('Ctrl Pts',(-18.1904651245614,42.771447549779,123.528307551792)) ;
#31873=CARTESIAN_POINT('Ctrl Pts',(-17.9275815086194,42.9714209501934,123.027999899649)) ;
#31874=CARTESIAN_POINT('Ctrl Pts',(-18.2239197641623,42.7914318698305,123.104753757388)) ;
#31875=CARTESIAN_POINT('Ctrl Pts',(-18.1472767537667,42.991348982983,122.545930346273)) ;
#31876=CARTESIAN_POINT('Ctrl Pts',(-18.3996848299053,42.8113599026202,122.719094732473)) ;
#31877=CARTESIAN_POINT('Ctrl Pts',(-18.4563016259536,43.0079577449228,122.230836526374)) ;
#31878=CARTESIAN_POINT('Ctrl Pts',(-18.6468908763838,42.82796866456,122.467036542162)) ;
#31879=CARTESIAN_POINT('Ctrl Pts',(-18.7544287787532,43.0211453836129,122.054087877132)) ;
#31880=CARTESIAN_POINT('Ctrl Pts',(-18.8854094489693,42.84115630325,122.325626725663)) ;
#31881=CARTESIAN_POINT('Ctrl Pts',(-18.9997521034799,43.031131817973,121.960916807132)) ;
#31882=CARTESIAN_POINT('Ctrl Pts',(-19.0816631635093,42.8511427376102,122.251094035391)) ;
#31883=CARTESIAN_POINT('Ctrl Pts',(-19.2581944108813,43.0411411919324,121.911902702877)) ;
#31884=CARTESIAN_POINT('Ctrl Pts',(-19.2884287994832,42.8611521115695,122.211885725831)) ;
#31885=CARTESIAN_POINT('Ctrl Pts',(-19.6074202778413,43.0544312254977,121.907165841963)) ;
#31886=CARTESIAN_POINT('Ctrl Pts',(-19.5677560175321,42.8744421451348,122.208091120847)) ;
#31887=CARTESIAN_POINT('Ctrl Pts',(-20.0350687767284,43.0710252131601,122.015093622791)) ;
#31888=CARTESIAN_POINT('Ctrl Pts',(-19.9099409302065,42.8910361327973,122.294450399826)) ;
#31889=CARTESIAN_POINT('Ctrl Pts',(-20.4010277793674,43.0876574684357,122.26302842487)) ;
#31890=CARTESIAN_POINT('Ctrl Pts',(-20.2026637544341,42.9076683880728,122.492780756029)) ;
#31891=CARTESIAN_POINT('Ctrl Pts',(-20.6289019817072,43.1008998521035,122.526052209373)) ;
#31892=CARTESIAN_POINT('Ctrl Pts',(-20.3849854274242,42.9209107717406,122.70321807601)) ;
#31893=CARTESIAN_POINT('Ctrl Pts',(-20.7634137015571,43.1108140603309,122.749188831555)) ;
#31894=CARTESIAN_POINT('Ctrl Pts',(-20.49258810908,42.9308249799681,122.881725181544)) ;
#31895=CARTESIAN_POINT('Ctrl Pts',(-20.8581936477321,43.1208706996026,122.995865179697)) ;
#31896=CARTESIAN_POINT('Ctrl Pts',(-20.5684111153363,42.9408816192397,123.079068425544)) ;
#31897=CARTESIAN_POINT('Ctrl Pts',(-20.9079570487934,43.1307165060227,123.249794573028)) ;
#31898=CARTESIAN_POINT('Ctrl Pts',(-20.6082199684139,42.9507274256599,123.282209957339)) ;
#31899=CARTESIAN_POINT('Ctrl Pts',(-20.9134264774939,43.1407615056559,123.513697714177)) ;
#31900=CARTESIAN_POINT('Ctrl Pts',(-20.6125910612325,42.960772425293,123.493341293603)) ;
#31901=CARTESIAN_POINT('Ctrl Pts',(-20.8594473356749,43.1540425280286,123.858497845333)) ;
#31902=CARTESIAN_POINT('Ctrl Pts',(-20.569416250521,42.9740534476658,123.769136972112)) ;
#31903=CARTESIAN_POINT('Ctrl Pts',(-20.718508196259,43.1672399745533,124.17971260659)) ;
#31904=CARTESIAN_POINT('Ctrl Pts',(-20.4566616453272,42.9872508941904,124.026134275498)) ;
#31905=CARTESIAN_POINT('Ctrl Pts',(-20.4978485962577,43.1806542723603,124.454637161235)) ;
#31906=CARTESIAN_POINT('Ctrl Pts',(-20.2801208442663,43.0006651919974,124.246084216616)) ;
#31907=CARTESIAN_POINT('Ctrl Pts',(-20.3035425807458,43.190493337763,124.625241624044)) ;
#31908=CARTESIAN_POINT('Ctrl Pts',(-20.124676701218,43.0105042574002,124.382563655871)) ;
#31909=CARTESIAN_POINT('Ctrl Pts',(-20.0797235876443,43.2004765440407,124.762051652017)) ;
#31910=CARTESIAN_POINT('Ctrl Pts',(-19.9456197990869,43.0204874636778,124.492010372349)) ;
#31911=CARTESIAN_POINT('Ctrl Pts',(-19.8362597616934,43.2104277789535,124.8575472145)) ;
#31912=CARTESIAN_POINT('Ctrl Pts',(-19.7508481203091,43.0304386985906,124.568404524437)) ;
#31913=CARTESIAN_POINT('Ctrl Pts',(-19.5786965198764,43.2204287786551,124.909888505183)) ;
#31914=CARTESIAN_POINT('Ctrl Pts',(-19.544797096,43.0404396982923,124.610275379233)) ;
#31915=CARTESIAN_POINT('Ctrl Pts',(-19.3151648430061,43.2304601244425,124.916319914135)) ;
#31916=CARTESIAN_POINT('Ctrl Pts',(-19.3339717561267,43.0504710440796,124.615418233467)) ;
#31917=CARTESIAN_POINT('Ctrl Pts',(-19.0590709276985,43.2403138891475,124.877945266862)) ;
#31918=CARTESIAN_POINT('Ctrl Pts',(-19.1290970496758,43.0603248087846,124.584716300181)) ;
#31919=CARTESIAN_POINT('Ctrl Pts',(-18.8104522663154,43.2502845428158,124.79531472401)) ;
#31920=CARTESIAN_POINT('Ctrl Pts',(-18.9302029191281,43.0702954624529,124.518609759504)) ;
#31921=CARTESIAN_POINT('Ctrl Pts',(-18.5792880259183,43.260281786473,124.670397983482)) ;
#31922=CARTESIAN_POINT('Ctrl Pts',(-18.7452726496911,43.0802927061101,124.418674422827)) ;
#31923=CARTESIAN_POINT('Ctrl Pts',(-18.3728375783555,43.2703152424172,124.506422572522)) ;
#31924=CARTESIAN_POINT('Ctrl Pts',(-18.5801137193159,43.0903261620543,124.287492345244)) ;
#31925=CARTESIAN_POINT('Ctrl Pts',(-18.2007504134058,43.2801707467176,124.31283503278)) ;
#31926=CARTESIAN_POINT('Ctrl Pts',(-18.4424457883443,43.1001816663547,124.132620965001)) ;
#31927=CARTESIAN_POINT('Ctrl Pts',(-18.0626456729148,43.2901701830037,124.089333194053)) ;
#31928=CARTESIAN_POINT('Ctrl Pts',(-18.3319639343597,43.1101811026408,123.953818381161)) ;
#31929=CARTESIAN_POINT('Ctrl Pts',(-17.9661552350075,43.3000646425196,123.847830753989)) ;
#31930=CARTESIAN_POINT('Ctrl Pts',(-18.2547737161696,43.1200755621567,123.760615804186)) ;
#31931=CARTESIAN_POINT('Ctrl Pts',(-17.9122545173091,43.3101277619712,123.588980661551)) ;
#31932=CARTESIAN_POINT('Ctrl Pts',(-18.2116553113845,43.1301386816084,123.55353524895)) ;
#31933=CARTESIAN_POINT('Ctrl Pts',(-17.9040100749574,43.3199673963832,123.330493713353)) ;
#31934=CARTESIAN_POINT('Ctrl Pts',(-18.2050619671359,43.1399783160204,123.346745951152)) ;
#31935=CARTESIAN_POINT('Ctrl Pts',(-17.9412644855324,43.330030603869,123.068717754911)) ;
#31936=CARTESIAN_POINT('Ctrl Pts',(-18.2348676608804,43.1500415235061,123.137325455349)) ;
#31937=CARTESIAN_POINT('Ctrl Pts',(-18.0222521551209,43.3399247112482,122.821614169064)) ;
#31938=CARTESIAN_POINT('Ctrl Pts',(-18.2996598001454,43.1599356308853,122.939643522461)) ;
#31939=CARTESIAN_POINT('Ctrl Pts',(-18.1448649357578,43.3498670434406,122.590937416187)) ;
#31940=CARTESIAN_POINT('Ctrl Pts',(-18.3977518184139,43.1698779630777,122.755103312914)) ;
#31941=CARTESIAN_POINT('Ctrl Pts',(-18.3065565946206,43.3598676697556,122.383706851709)) ;
#31942=CARTESIAN_POINT('Ctrl Pts',(-18.5271067799686,43.1798785893927,122.589320225833)) ;
#31943=CARTESIAN_POINT('Ctrl Pts',(-18.5028573530525,43.3699094040375,122.207385535582)) ;
#31944=CARTESIAN_POINT('Ctrl Pts',(-18.6841488602168,43.1899203236746,122.448264772866)) ;
#31945=CARTESIAN_POINT('Ctrl Pts',(-18.7217003533941,43.3797348299866,122.070323331608)) ;
#31946=CARTESIAN_POINT('Ctrl Pts',(-18.8592239561885,43.1997457496237,122.338617074552)) ;
#31947=CARTESIAN_POINT('Ctrl Pts',(-18.9664691272905,43.3897916565143,121.970708884775)) ;
#31948=CARTESIAN_POINT('Ctrl Pts',(-19.0550398228914,43.2098025761514,122.258927422049)) ;
#31949=CARTESIAN_POINT('Ctrl Pts',(-19.2216018609428,43.3997190896358,121.916174470016)) ;
#31950=CARTESIAN_POINT('Ctrl Pts',(-19.2591461961739,43.219730009273,122.215302017841)) ;
#31951=CARTESIAN_POINT('Ctrl Pts',(-19.4828888562582,43.4096690820421,121.905998966867)) ;
#31952=CARTESIAN_POINT('Ctrl Pts',(-19.4681756430009,43.2296800016792,122.207163663939)) ;
#31953=CARTESIAN_POINT('Ctrl Pts',(-19.7446216548047,43.4197242831161,121.942178613796)) ;
#31954=CARTESIAN_POINT('Ctrl Pts',(-19.6775616803327,43.2397352027532,122.236109468103)) ;
#31955=CARTESIAN_POINT('Ctrl Pts',(-19.9904509322207,43.4295465571684,122.02094445218)) ;
#31956=CARTESIAN_POINT('Ctrl Pts',(-19.8742238828704,43.2495574768055,122.299123887706)) ;
#31957=CARTESIAN_POINT('Ctrl Pts',(-20.2244870380784,43.4396024511276,122.143621831466)) ;
#31958=CARTESIAN_POINT('Ctrl Pts',(-20.0614519256092,43.2596133707647,122.397267588395)) ;
#31959=CARTESIAN_POINT('Ctrl Pts',(-20.4310096168158,43.4495431729727,122.303608199071)) ;
#31960=CARTESIAN_POINT('Ctrl Pts',(-20.2266685268885,43.2695540926099,122.525258131967)) ;
#31961=CARTESIAN_POINT('Ctrl Pts',(-20.6065731184016,43.4594475170593,122.495763120482)) ;
#31962=CARTESIAN_POINT('Ctrl Pts',(-20.3671176119606,43.2794584366965,122.678983058845)) ;
#31963=CARTESIAN_POINT('Ctrl Pts',(-20.7479541652507,43.4694941843588,122.718707024721)) ;
#31964=CARTESIAN_POINT('Ctrl Pts',(-20.4802208409037,43.2895051039959,122.857339300646)) ;
#31965=CARTESIAN_POINT('Ctrl Pts',(-20.8472092355886,43.4793897428087,122.95911028977)) ;
#31966=CARTESIAN_POINT('Ctrl Pts',(-20.5596229418343,43.2994006624459,123.049662215042)) ;
#31967=CARTESIAN_POINT('Ctrl Pts',(-20.904139618028,43.4894518215134,123.217291078424)) ;
#31968=CARTESIAN_POINT('Ctrl Pts',(-20.6051653985535,43.3094627411505,123.256207403565)) ;
#31969=CARTESIAN_POINT('Ctrl Pts',(-20.9152824166523,43.4992945199792,123.475736104278)) ;
#31970=CARTESIAN_POINT('Ctrl Pts',(-20.6140777067984,43.3193054396163,123.462962813021)) ;
#31971=CARTESIAN_POINT('Ctrl Pts',(-20.8814961280243,43.5092852938737,123.736067222342)) ;
#31972=CARTESIAN_POINT('Ctrl Pts',(-20.5870468982505,43.3292962135108,123.671227335157)) ;
#31973=CARTESIAN_POINT('Ctrl Pts',(-20.8034587033046,43.5192131631086,123.985028739388)) ;
#31974=CARTESIAN_POINT('Ctrl Pts',(-20.5246153423973,43.3392240827457,123.870395633847)) ;
#31975=CARTESIAN_POINT('Ctrl Pts',(-20.6830540646815,43.5292018920784,124.218293703487)) ;
#31976=CARTESIAN_POINT('Ctrl Pts',(-20.4282901545074,43.3492128117156,124.057006673629)) ;
#31977=CARTESIAN_POINT('Ctrl Pts',(-20.5227971110946,43.5392412940622,124.427851205494)) ;
#31978=CARTESIAN_POINT('Ctrl Pts',(-20.3000830928166,43.3592522136993,124.224651637506)) ;
#31979=CARTESIAN_POINT('Ctrl Pts',(-20.3327674227349,43.549081461799,124.603250592089)) ;
#31980=CARTESIAN_POINT('Ctrl Pts',(-20.1480587518174,43.3690923814361,124.36496932946)) ;
#31981=CARTESIAN_POINT('Ctrl Pts',(-20.1108004287422,43.5591296721735,124.746255706704)) ;
#31982=CARTESIAN_POINT('Ctrl Pts',(-19.9704841479097,43.3791405918106,124.479372086508)) ;
#31983=CARTESIAN_POINT('Ctrl Pts',(-19.8696476488821,43.5690768424612,124.84714360705)) ;
#31984=CARTESIAN_POINT('Ctrl Pts',(-19.7775615548716,43.3890877620984,124.560080670385)) ;
#31985=CARTESIAN_POINT('Ctrl Pts',(-19.6157403076391,43.5789876907163,124.905179129313)) ;
#31986=CARTESIAN_POINT('Ctrl Pts',(-19.5744358437637,43.3989986103534,124.606507405916)) ;
#31987=CARTESIAN_POINT('Ctrl Pts',(-19.3518069355752,43.5890440183941,124.91818859538)) ;
#31988=CARTESIAN_POINT('Ctrl Pts',(-19.3632888855343,43.4090549380312,124.616913341816)) ;
#31989=CARTESIAN_POINT('Ctrl Pts',(-19.0949363387433,43.5988944311626,124.886068138014)) ;
#31990=CARTESIAN_POINT('Ctrl Pts',(-19.1577934324893,43.4189053507997,124.591215484819)) ;
#31991=CARTESIAN_POINT('Ctrl Pts',(-18.8429401699179,43.6089213169963,124.809086046414)) ;
#31992=CARTESIAN_POINT('Ctrl Pts',(-18.9561969026727,43.4289322366334,124.529628381766)) ;
#31993=CARTESIAN_POINT('Ctrl Pts',(-18.608395133658,43.6189499326271,124.688881455388)) ;
#31994=CARTESIAN_POINT('Ctrl Pts',(-18.7685615614303,43.4389608522643,124.433463244299)) ;
#31995=CARTESIAN_POINT('Ctrl Pts',(-18.4018522456686,43.6287951560046,124.53309241998)) ;
#31996=CARTESIAN_POINT('Ctrl Pts',(-18.6033288833992,43.4488060756417,124.308831339944)) ;
#31997=CARTESIAN_POINT('Ctrl Pts',(-18.2223621198309,43.6387858381062,124.34147662207)) ;
#31998=CARTESIAN_POINT('Ctrl Pts',(-18.4597378987131,43.4587967577433,124.15553787085)) ;
#31999=CARTESIAN_POINT('Ctrl Pts',(-18.0786893213183,43.6488237267386,124.120254417819)) ;
#32000=CARTESIAN_POINT('Ctrl Pts',(-18.344800860244,43.4688346463758,123.97855920037)) ;
#32001=CARTESIAN_POINT('Ctrl Pts',(-17.977176387725,43.6586680618418,123.882292776737)) ;
#32002=CARTESIAN_POINT('Ctrl Pts',(-18.2635921771929,43.4786789814789,123.788190198657)) ;
#32003=CARTESIAN_POINT('Ctrl Pts',(-17.917193628408,43.6686530240393,123.626883148383)) ;
#32004=CARTESIAN_POINT('Ctrl Pts',(-18.2156072828888,43.4886639436764,123.583862392775)) ;
#32005=CARTESIAN_POINT('Ctrl Pts',(-17.9024116244684,43.6785919655727,123.366078461576)) ;
#32006=CARTESIAN_POINT('Ctrl Pts',(-18.2037829771252,43.4986028852098,123.375219006614)) ;
#32007=CARTESIAN_POINT('Ctrl Pts',(-17.9335320666697,43.6886338505441,123.104055220491)) ;
#32008=CARTESIAN_POINT('Ctrl Pts',(-18.2286806289882,43.5086447701812,123.165600448032)) ;
#32009=CARTESIAN_POINT('Ctrl Pts',(-18.008352723709,43.6985203984524,122.855226846736)) ;
#32010=CARTESIAN_POINT('Ctrl Pts',(-18.2885381427592,43.5185313180895,122.966538824401)) ;
#32011=CARTESIAN_POINT('Ctrl Pts',(-18.1261385188554,43.7085143239524,122.620528575572)) ;
#32012=CARTESIAN_POINT('Ctrl Pts',(-18.3827677656657,43.5285252435895,122.778780862316)) ;
#32013=CARTESIAN_POINT('Ctrl Pts',(-18.2819245676956,43.7184504150789,122.410933846051)) ;
#32014=CARTESIAN_POINT('Ctrl Pts',(-18.5073972462572,43.538461334716,122.61110613432)) ;
#32015=CARTESIAN_POINT('Ctrl Pts',(-18.4734970875813,43.7284796840588,122.229979319978)) ;
#32016=CARTESIAN_POINT('Ctrl Pts',(-18.6606561040544,43.5484906036959,122.466343315554)) ;
#32017=CARTESIAN_POINT('Ctrl Pts',(-18.6902358432055,43.7383620666181,122.086843147979)) ;
#32018=CARTESIAN_POINT('Ctrl Pts',(-18.8340470312142,43.5583729862552,122.351835729643)) ;
#32019=CARTESIAN_POINT('Ctrl Pts',(-18.9325293093004,43.748414583706,121.981687073779)) ;
#32020=CARTESIAN_POINT('Ctrl Pts',(-19.0278824125168,43.5684255033431,122.267711767066)) ;
#32021=CARTESIAN_POINT('Ctrl Pts',(-19.1854080916355,43.7583087045299,121.921017634688)) ;
#32022=CARTESIAN_POINT('Ctrl Pts',(-19.2301849629632,43.578319624167,122.219177394001)) ;
#32023=CARTESIAN_POINT('Ctrl Pts',(-19.4492993318414,43.7683706839503,121.904850471576)) ;
#32024=CARTESIAN_POINT('Ctrl Pts',(-19.4412982796223,43.5883816035874,122.2062446672)) ;
#32025=CARTESIAN_POINT('Ctrl Pts',(-19.7063573702631,43.7782152171792,121.934076663056)) ;
#32026=CARTESIAN_POINT('Ctrl Pts',(-19.6469435446541,43.5982261368164,122.22962650948)) ;
#32027=CARTESIAN_POINT('Ctrl Pts',(-19.9576002327423,43.7881752960855,122.007446102476)) ;
#32028=CARTESIAN_POINT('Ctrl Pts',(-19.8479372613017,43.6081862157226,122.288322719679)) ;
#32029=CARTESIAN_POINT('Ctrl Pts',(-20.1938925036668,43.7982135726581,122.124695495129)) ;
#32030=CARTESIAN_POINT('Ctrl Pts',(-20.0369707873508,43.6182244922952,122.382123111982)) ;
#32031=CARTESIAN_POINT('Ctrl Pts',(-20.403085266942,43.8080869591959,122.278251260109)) ;
#32032=CARTESIAN_POINT('Ctrl Pts',(-20.2043238013652,43.6280978788331,122.504967832787)) ;
#32033=CARTESIAN_POINT('Ctrl Pts',(-20.5859442921562,43.818159901963,122.469575837394)) ;
#32034=CARTESIAN_POINT('Ctrl Pts',(-20.3506106669078,43.6381708216001,122.65802830527)) ;
#32035=CARTESIAN_POINT('Ctrl Pts',(-20.7294563688574,43.8279813160913,122.684155238316)) ;
#32036=CARTESIAN_POINT('Ctrl Pts',(-20.4654190257997,43.6479922357285,122.829691205274)) ;
#32037=CARTESIAN_POINT('Ctrl Pts',(-20.8364643232835,43.8380559461636,122.926263897482)) ;
#32038=CARTESIAN_POINT('Ctrl Pts',(-20.5510249269012,43.6580668658008,123.023378728422)) ;
#32039=CARTESIAN_POINT('Ctrl Pts',(-20.8984148212984,43.8479225834805,123.178073112069)) ;
#32040=CARTESIAN_POINT('Ctrl Pts',(-20.6005844237704,43.6679335031176,123.224825316576)) ;
#32041=CARTESIAN_POINT('Ctrl Pts',(-20.9166483132866,43.8579461288523,123.440837266538)) ;
#32042=CARTESIAN_POINT('Ctrl Pts',(-20.6151706983292,43.6779570484894,123.435036712492)) ;
#32043=CARTESIAN_POINT('Ctrl Pts',(-20.8883395523817,43.8679718803695,123.702794177763)) ;
#32044=CARTESIAN_POINT('Ctrl Pts',(-20.5925230028488,43.6879828000066,123.644602236926)) ;
#32045=CARTESIAN_POINT('Ctrl Pts',(-20.8166599479504,43.8778254673789,123.951603594725)) ;
#32046=CARTESIAN_POINT('Ctrl Pts',(-20.5351790633335,43.697836387016,123.843648589782)) ;
#32047=CARTESIAN_POINT('Ctrl Pts',(-20.702060923653,43.8878024276068,124.187422142841)) ;
#32048=CARTESIAN_POINT('Ctrl Pts',(-20.4434995981191,43.7078133472439,124.032303014082)) ;
#32049=CARTESIAN_POINT('Ctrl Pts',(-20.5472263847729,43.8978235706353,124.400424003541)) ;
#32050=CARTESIAN_POINT('Ctrl Pts',(-20.3196315437923,43.7178344902724,124.202704210316)) ;
#32051=CARTESIAN_POINT('Ctrl Pts',(-20.3607073265626,43.9077061766552,124.581187205771)) ;
#32052=CARTESIAN_POINT('Ctrl Pts',(-20.1704166645511,43.7277170962923,124.34731388807)) ;
#32053=CARTESIAN_POINT('Ctrl Pts',(-20.141598516524,43.9177746472879,124.729426223139)) ;
#32054=CARTESIAN_POINT('Ctrl Pts',(-19.9951291156329,43.737785566925,124.465904948293)) ;
#32055=CARTESIAN_POINT('Ctrl Pts',(-19.9058383854937,43.9276047304716,124.835123522503)) ;
#32056=CARTESIAN_POINT('Ctrl Pts',(-19.8065220003896,43.7476156501087,124.550461981873)) ;
#32057=CARTESIAN_POINT('Ctrl Pts',(-19.6494502413749,43.937671290152,124.900110672069)) ;
#32058=CARTESIAN_POINT('Ctrl Pts',(-19.6014111164167,43.7576822097891,124.602451541965)) ;
#32059=CARTESIAN_POINT('Ctrl Pts',(-19.3902067493444,43.9475615399812,124.919096378298)) ;
#32060=CARTESIAN_POINT('Ctrl Pts',(-19.3940171383949,43.7675724596183,124.617639759188)) ;
#32061=CARTESIAN_POINT('Ctrl Pts',(-19.1289291993489,43.95755370573,124.893086593962)) ;
#32062=CARTESIAN_POINT('Ctrl Pts',(-19.1849952828708,43.7775646253671,124.59683180778)) ;
#32063=CARTESIAN_POINT('Ctrl Pts',(-18.8769378575391,43.9675165493261,124.822071866951)) ;
#32064=CARTESIAN_POINT('Ctrl Pts',(-18.9834026165215,43.7875274689632,124.54001992677)) ;
#32065=CARTESIAN_POINT('Ctrl Pts',(-18.6421796236828,43.9774207181539,124.709636238937)) ;
#32066=CARTESIAN_POINT('Ctrl Pts',(-18.7955967231379,43.797431637791,124.450071716623)) ;
#32067=CARTESIAN_POINT('Ctrl Pts',(-18.4273472596352,43.9874815930482,124.555590382771)) ;
#32068=CARTESIAN_POINT('Ctrl Pts',(-18.6237306573745,43.8074925126853,124.32683478731)) ;
#32069=CARTESIAN_POINT('Ctrl Pts',(-18.2462912417937,43.9973204963776,124.370950929424)) ;
#32070=CARTESIAN_POINT('Ctrl Pts',(-18.4788866747654,43.8173314160147,124.179124065439)) ;
#32071=CARTESIAN_POINT('Ctrl Pts',(-18.096473040413,44.0073888727515,124.152920066805)) ;
#32072=CARTESIAN_POINT('Ctrl Pts',(-18.3590318811178,43.8273997923886,124.004699145389)) ;
#32073=CARTESIAN_POINT('Ctrl Pts',(-17.9888795242822,44.0172694893841,123.916566377132)) ;
#32074=CARTESIAN_POINT('Ctrl Pts',(-18.2729574087279,43.8372804090212,123.815617033052)) ;
#32075=CARTESIAN_POINT('Ctrl Pts',(-17.9227396809683,44.0272606496131,123.662515814642)) ;
#32076=CARTESIAN_POINT('Ctrl Pts',(-18.2200454142358,43.8472715692502,123.612376795175)) ;
#32077=CARTESIAN_POINT('Ctrl Pts',(-17.9017478866056,44.0372137230452,123.40176367561)) ;
#32078=CARTESIAN_POINT('Ctrl Pts',(-18.2032518302433,43.8572246426823,123.403775507638)) ;
#32079=CARTESIAN_POINT('Ctrl Pts',(-17.9266347799871,44.0472495586578,123.139231148737)) ;
#32080=CARTESIAN_POINT('Ctrl Pts',(-18.2231612008556,43.867260478295,123.193749351306)) ;
#32081=CARTESIAN_POINT('Ctrl Pts',(-17.9955495886584,44.057139685388,122.888614558069)) ;
#32082=CARTESIAN_POINT('Ctrl Pts',(-18.2782926266805,43.8771506050251,122.993256851643)) ;
#32083=CARTESIAN_POINT('Ctrl Pts',(-18.1076878440328,44.0671318671573,122.651194666647)) ;
#32084=CARTESIAN_POINT('Ctrl Pts',(-18.3680028793089,43.8871427867944,122.803320956342)) ;
#32085=CARTESIAN_POINT('Ctrl Pts',(-18.2587247866769,44.0770778071318,122.437883820146)) ;
#32086=CARTESIAN_POINT('Ctrl Pts',(-18.4888319257956,43.8970887267689,122.632672501952)) ;
#32087=CARTESIAN_POINT('Ctrl Pts',(-18.4441648499972,44.0870249908912,122.253628827194)) ;
#32088=CARTESIAN_POINT('Ctrl Pts',(-18.6371833541905,43.9070359105284,122.485268533601)) ;
#32089=CARTESIAN_POINT('Ctrl Pts',(-18.6611045195494,44.0970729291816,122.103115117568)) ;
#32090=CARTESIAN_POINT('Ctrl Pts',(-18.8107350578741,43.9170838488187,122.364857168353)) ;
#32091=CARTESIAN_POINT('Ctrl Pts',(-18.8960216519544,44.1069205639951,121.9945561486)) ;
#32092=CARTESIAN_POINT('Ctrl Pts',(-18.9986675796601,43.9269314836323,122.278010099489)) ;
#32093=CARTESIAN_POINT('Ctrl Pts',(-19.1488932353645,44.1168822776931,121.926880369107)) ;
#32094=CARTESIAN_POINT('Ctrl Pts',(-19.200964338225,43.9368931973302,122.223868984643)) ;
#32095=CARTESIAN_POINT('Ctrl Pts',(-19.4114837782062,44.1269109135143,121.904316948058)) ;
#32096=CARTESIAN_POINT('Ctrl Pts',(-19.4110368048726,43.9469218331514,122.205817721799)) ;
#32097=CARTESIAN_POINT('Ctrl Pts',(-19.6708855677709,44.136821228266,121.927328148373)) ;
#32098=CARTESIAN_POINT('Ctrl Pts',(-19.6185575864657,43.9568321479032,122.224226080018)) ;
#32099=CARTESIAN_POINT('Ctrl Pts',(-19.923172854028,44.1467560989287,121.994541369525)) ;
#32100=CARTESIAN_POINT('Ctrl Pts',(-19.8203870878445,43.9667670185658,122.277995832626)) ;
#32101=CARTESIAN_POINT('Ctrl Pts',(-20.1623656622643,44.1567972813305,122.105936279633)) ;
#32102=CARTESIAN_POINT('Ctrl Pts',(-20.011741745876,43.9768082009676,122.367111237361)) ;
#32103=CARTESIAN_POINT('Ctrl Pts',(-20.3754115587803,44.1666842527952,122.254696080828)) ;
#32104=CARTESIAN_POINT('Ctrl Pts',(-20.1821781748641,43.9866951724323,122.486118021261)) ;
#32105=CARTESIAN_POINT('Ctrl Pts',(-20.5616797006254,44.1766836850578,122.439998156239)) ;
#32106=CARTESIAN_POINT('Ctrl Pts',(-20.3311931547893,43.9966946046949,122.634359041277)) ;
#32107=CARTESIAN_POINT('Ctrl Pts',(-20.7119248209942,44.1866037503144,122.653074790023)) ;
#32108=CARTESIAN_POINT('Ctrl Pts',(-20.4513895765128,44.0066146699516,122.804819385592)) ;
#32109=CARTESIAN_POINT('Ctrl Pts',(-20.8242248480084,44.1966406028986,122.89171516179)) ;
#32110=CARTESIAN_POINT('Ctrl Pts',(-20.5412304078257,44.0166515225357,122.995731440884)) ;
#32111=CARTESIAN_POINT('Ctrl Pts',(-20.8925256088344,44.2065532622386,123.143101297578)) ;
#32112=CARTESIAN_POINT('Ctrl Pts',(-20.5958716458054,44.0265641818757,123.19683949956)) ;
#32113=CARTESIAN_POINT('Ctrl Pts',(-20.9168966357386,44.2165444741535,123.404542148438)) ;
#32114=CARTESIAN_POINT('Ctrl Pts',(-20.6153694127085,44.0365553937906,123.405991922717)) ;
#32115=CARTESIAN_POINT('Ctrl Pts',(-20.8948063197256,44.2265861155566,123.667478543077)) ;
#32116=CARTESIAN_POINT('Ctrl Pts',(-20.597697972569,44.0465970351937,123.616341249776)) ;
#32117=CARTESIAN_POINT('Ctrl Pts',(-20.8294398407361,44.2364149097636,123.917397995982)) ;
#32118=CARTESIAN_POINT('Ctrl Pts',(-20.5454060288172,44.0564258294008,123.816275945776)) ;
#32119=CARTESIAN_POINT('Ctrl Pts',(-20.7190966284838,44.2464913208849,124.158051348321)) ;
#32120=CARTESIAN_POINT('Ctrl Pts',(-20.45713223089,44.066502240522,124.008799361129)) ;
#32121=CARTESIAN_POINT('Ctrl Pts',(-20.5720419186679,44.2563434539274,124.371206621261)) ;
#32122=CARTESIAN_POINT('Ctrl Pts',(-20.3394898756421,44.0763543735645,124.179323355511)) ;
#32123=CARTESIAN_POINT('Ctrl Pts',(-20.3863598082827,44.2664166882687,124.559814357932)) ;
#32124=CARTESIAN_POINT('Ctrl Pts',(-20.1909447374728,44.0864276079058,124.330210536534)) ;
#32125=CARTESIAN_POINT('Ctrl Pts',(-20.1756188492781,44.2762581895953,124.709761183194)) ;
#32126=CARTESIAN_POINT('Ctrl Pts',(-20.0223534395185,44.0962691092324,124.450168264063)) ;
#32127=CARTESIAN_POINT('Ctrl Pts',(-19.9396571120249,44.2862191411901,124.823064731638)) ;
#32128=CARTESIAN_POINT('Ctrl Pts',(-19.833584900295,44.1062300608272,124.540812125368)) ;
#32129=CARTESIAN_POINT('Ctrl Pts',(-19.6855192485354,44.2962569589108,124.893713217866)) ;
#32130=CARTESIAN_POINT('Ctrl Pts',(-19.630274821082,44.1162678785479,124.597332072431)) ;
#32131=CARTESIAN_POINT('Ctrl Pts',(-19.4272568805915,44.3061313081678,124.919231077549)) ;
#32132=CARTESIAN_POINT('Ctrl Pts',(-19.4236658581151,44.1261422278049,124.617747552398)) ;
#32133=CARTESIAN_POINT('Ctrl Pts',(-19.1634421663118,44.31620085891,124.899117334135)) ;
#32134=CARTESIAN_POINT('Ctrl Pts',(-19.2126137105638,44.1362117785471,124.601657806731)) ;
#32135=CARTESIAN_POINT('Ctrl Pts',(-18.9130262792897,44.3260348784186,124.835165719918)) ;
#32136=CARTESIAN_POINT('Ctrl Pts',(-19.0122816736547,44.1460457980557,124.55049803559)) ;
#32137=CARTESIAN_POINT('Ctrl Pts',(-18.6724761256092,44.3360690329981,124.727189304434)) ;
#32138=CARTESIAN_POINT('Ctrl Pts',(-18.8198408751358,44.1560799526353,124.464118191425)) ;
#32139=CARTESIAN_POINT('Ctrl Pts',(-18.4550666358706,44.3460849588206,124.578799029693)) ;
#32140=CARTESIAN_POINT('Ctrl Pts',(-18.6459125515534,44.1660958784577,124.345407061156)) ;
#32141=CARTESIAN_POINT('Ctrl Pts',(-18.2689206934433,44.3559672140149,124.397708730824)) ;
#32142=CARTESIAN_POINT('Ctrl Pts',(-18.4969953334488,44.175978133652,124.200536340073)) ;
#32143=CARTESIAN_POINT('Ctrl Pts',(-18.1151639542311,44.3659560205258,124.184994122571)) ;
#32144=CARTESIAN_POINT('Ctrl Pts',(-18.3739888404937,44.1859669401629,124.030365648299)) ;
#32145=CARTESIAN_POINT('Ctrl Pts',(-18.0009287364672,44.3759045877885,123.949788452977)) ;
#32146=CARTESIAN_POINT('Ctrl Pts',(-18.2825994652639,44.1959155074256,123.842202101952)) ;
#32147=CARTESIAN_POINT('Ctrl Pts',(-17.9287930124207,44.3859593930905,123.695625807384)) ;
#32148=CARTESIAN_POINT('Ctrl Pts',(-18.2248894332105,44.2059703127276,123.638872216548)) ;
#32149=CARTESIAN_POINT('Ctrl Pts',(-17.9021400804517,44.3957781763541,123.438965134921)) ;
#32150=CARTESIAN_POINT('Ctrl Pts',(-18.2035656682634,44.2157890959912,123.433544841874)) ;
#32151=CARTESIAN_POINT('Ctrl Pts',(-17.9201546965115,44.4058139487147,123.175857889878)) ;
#32152=CARTESIAN_POINT('Ctrl Pts',(-18.2179757049312,44.2258248683518,123.223058844661)) ;
#32153=CARTESIAN_POINT('Ctrl Pts',(-17.9842443392215,44.4158386477433,122.920324456169)) ;
#32154=CARTESIAN_POINT('Ctrl Pts',(-18.2692459457446,44.2358495673804,123.018631708746)) ;
#32155=CARTESIAN_POINT('Ctrl Pts',(-18.0893534627256,44.4256906510024,122.683715321304)) ;
#32156=CARTESIAN_POINT('Ctrl Pts',(-18.3533314265156,44.2457015706395,122.8293444755)) ;
#32157=CARTESIAN_POINT('Ctrl Pts',(-18.2356357013134,44.4356815853996,122.46572907487)) ;
#32158=CARTESIAN_POINT('Ctrl Pts',(-18.4703557257671,44.2556925050367,122.654954642238)) ;
#32159=CARTESIAN_POINT('Ctrl Pts',(-18.41613673709,44.4455995078307,122.277671975149)) ;
#32160=CARTESIAN_POINT('Ctrl Pts',(-18.6147549895924,44.2656104274678,122.504508093951)) ;
#32161=CARTESIAN_POINT('Ctrl Pts',(-18.6288136047377,44.455627863513,122.122084840499)) ;
#32162=CARTESIAN_POINT('Ctrl Pts',(-18.7848954782,44.2756387831502,122.380036963716)) ;
#32163=CARTESIAN_POINT('Ctrl Pts',(-18.8618504936233,44.4655121480236,122.007331995514)) ;
#32164=CARTESIAN_POINT('Ctrl Pts',(-18.9713236802826,44.2855230676607,122.288233368328)) ;
#32165=CARTESIAN_POINT('Ctrl Pts',(-19.1138322342733,44.4755048319315,121.933421901147)) ;
#32166=CARTESIAN_POINT('Ctrl Pts',(-19.1729084429983,44.2955157515686,122.229103542104)) ;
#32167=CARTESIAN_POINT('Ctrl Pts',(-19.3758137501504,44.4855335689392,121.904740742867)) ;
#32168=CARTESIAN_POINT('Ctrl Pts',(-19.3824934791347,44.3055444885763,122.206156839405)) ;
#32169=CARTESIAN_POINT('Ctrl Pts',(-19.6350667634332,44.4954189655681,121.921395206069)) ;
#32170=CARTESIAN_POINT('Ctrl Pts',(-19.5898954555801,44.3154298852052,122.219478539478)) ;
#32171=CARTESIAN_POINT('Ctrl Pts',(-19.8901602887943,44.505406850982,121.983076127047)) ;
#32172=CARTESIAN_POINT('Ctrl Pts',(-19.7939705951904,44.3254177706191,122.268821404401)) ;
#32173=CARTESIAN_POINT('Ctrl Pts',(-20.1298803582596,44.5153575536426,122.087637628189)) ;
#32174=CARTESIAN_POINT('Ctrl Pts',(-19.9857471730679,44.3353684732797,122.35246874884)) ;
#32175=CARTESIAN_POINT('Ctrl Pts',(-20.3496330623717,44.52539787174,122.233619868658)) ;
#32176=CARTESIAN_POINT('Ctrl Pts',(-20.1615504313535,44.3454087913771,122.469252999656)) ;
#32177=CARTESIAN_POINT('Ctrl Pts',(-20.5377640234238,44.5352724370732,122.412390214829)) ;
#32178=CARTESIAN_POINT('Ctrl Pts',(-20.3120561285973,44.3552833567104,122.612267503124)) ;
#32179=CARTESIAN_POINT('Ctrl Pts',(-20.6941762400211,44.5452720971343,122.62349750357)) ;
#32180=CARTESIAN_POINT('Ctrl Pts',(-20.4371874373751,44.3652830167714,122.781152089198)) ;
#32181=CARTESIAN_POINT('Ctrl Pts',(-20.8107568463258,44.555181092302,122.856392682696)) ;
#32182=CARTESIAN_POINT('Ctrl Pts',(-20.5304535425006,44.3751920119392,122.967466996356)) ;
#32183=CARTESIAN_POINT('Ctrl Pts',(-20.8861166779856,44.5652358334653,123.109601455861)) ;
#32184=CARTESIAN_POINT('Ctrl Pts',(-20.5907433453259,44.3852467531024,123.170033530578)) ;
#32185=CARTESIAN_POINT('Ctrl Pts',(-20.9160838152059,44.5750944453791,123.36698258296)) ;
#32186=CARTESIAN_POINT('Ctrl Pts',(-20.6147190097219,44.3951053650162,123.375937681712)) ;
#32187=CARTESIAN_POINT('Ctrl Pts',(-20.9007482951995,44.5851625676584,123.631078613714)) ;
#32188=CARTESIAN_POINT('Ctrl Pts',(-20.6024526333435,44.4051734872955,123.587214747284)) ;
#32189=CARTESIAN_POINT('Ctrl Pts',(-20.8410433869187,44.5950180383616,123.883116987979)) ;
#32190=CARTESIAN_POINT('Ctrl Pts',(-20.5546908119095,44.4150289579987,123.788845432467)) ;
#32191=CARTESIAN_POINT('Ctrl Pts',(-20.737768269546,44.605012897855,124.124606144448)) ;
#32192=CARTESIAN_POINT('Ctrl Pts',(-20.4720727081621,44.4250238174921,123.982037522316)) ;
#32193=CARTESIAN_POINT('Ctrl Pts',(-20.5931261612872,44.6150441511969,124.344997164701)) ;
#32194=CARTESIAN_POINT('Ctrl Pts',(-20.3563607533755,44.435055070834,124.158351473366)) ;
#32195=CARTESIAN_POINT('Ctrl Pts',(-20.4156755541826,44.62491085007,124.534060702266)) ;
#32196=CARTESIAN_POINT('Ctrl Pts',(-20.2144020898501,44.4449217697071,124.309603448869)) ;
#32197=CARTESIAN_POINT('Ctrl Pts',(-20.2058546846897,44.6348976658212,124.691655677439)) ;
#32198=CARTESIAN_POINT('Ctrl Pts',(-20.0465467658949,44.4549085854583,124.435681091647)) ;
#32199=CARTESIAN_POINT('Ctrl Pts',(-19.9727822075021,44.6448448710167,124.810089850081)) ;
#32200=CARTESIAN_POINT('Ctrl Pts',(-19.8600899289393,44.4648557906538,124.530430271056)) ;
#32201=CARTESIAN_POINT('Ctrl Pts',(-19.7202958616412,44.6548878591429,124.886862052342)) ;
#32202=CARTESIAN_POINT('Ctrl Pts',(-19.6581014661053,44.4748987787801,124.591850096019)) ;
#32203=CARTESIAN_POINT('Ctrl Pts',(-19.4628869098935,44.6647552137644,124.91822843966)) ;
#32204=CARTESIAN_POINT('Ctrl Pts',(-19.4521748954927,44.4847661334015,124.616945312954)) ;
#32205=CARTESIAN_POINT('Ctrl Pts',(-19.201339436511,44.6747211070625,124.904992081208)) ;
#32206=CARTESIAN_POINT('Ctrl Pts',(-19.242936917876,44.4947320266996,124.606358443205)) ;
#32207=CARTESIAN_POINT('Ctrl Pts',(-18.9446146117008,44.6847448844386,124.845931776589)) ;
#32208=CARTESIAN_POINT('Ctrl Pts',(-19.0375565977731,44.5047558040757,124.559112343262)) ;
#32209=CARTESIAN_POINT('Ctrl Pts',(-18.7044247703961,44.6946704323703,124.744265398415)) ;
#32210=CARTESIAN_POINT('Ctrl Pts',(-18.8454040419128,44.5146813520074,124.477781340274)) ;
#32211=CARTESIAN_POINT('Ctrl Pts',(-18.4848477732278,44.7046109087913,124.602728279973)) ;
#32212=CARTESIAN_POINT('Ctrl Pts',(-18.6697413477393,44.5246218284284,124.364553593259)) ;
#32213=CARTESIAN_POINT('Ctrl Pts',(-18.2913709521149,44.7146571184542,124.423127645142)) ;
#32214=CARTESIAN_POINT('Ctrl Pts',(-18.5149583948213,44.5346680380913,124.220874721725)) ;
#32215=CARTESIAN_POINT('Ctrl Pts',(-18.1347068986328,44.724518375116,124.216672914137)) ;
#32216=CARTESIAN_POINT('Ctrl Pts',(-18.3896255050784,44.5445292947531,124.055712452699)) ;
#32217=CARTESIAN_POINT('Ctrl Pts',(-18.0143070451238,44.7345120033913,123.983318570089)) ;
#32218=CARTESIAN_POINT('Ctrl Pts',(-18.2933036525415,44.5545229230284,123.869030062897)) ;
#32219=CARTESIAN_POINT('Ctrl Pts',(-17.936633762989,44.7444374007015,123.734282199344)) ;
#32220=CARTESIAN_POINT('Ctrl Pts',(-18.2311629143838,44.5644483203386,123.669801734943)) ;
#32221=CARTESIAN_POINT('Ctrl Pts',(-17.9030399617659,44.7544653086117,123.472943722699)) ;
#32222=CARTESIAN_POINT('Ctrl Pts',(-18.2042856479589,44.5744762282489,123.46073129079)) ;
#32223=CARTESIAN_POINT('Ctrl Pts',(-17.9148956263581,44.7643516242809,123.213374011942)) ;
#32224=CARTESIAN_POINT('Ctrl Pts',(-18.2137679274287,44.584362543918,123.253075513145)) ;
#32225=CARTESIAN_POINT('Ctrl Pts',(-17.9723197114155,44.7743832191847,122.95612772885)) ;
#32226=CARTESIAN_POINT('Ctrl Pts',(-18.2597049813133,44.5943941388218,123.047278048275)) ;
#32227=CARTESIAN_POINT('Ctrl Pts',(-18.0718425713874,44.7842654621364,122.716214046185)) ;
#32228=CARTESIAN_POINT('Ctrl Pts',(-18.3393211701474,44.6042763817735,122.855346286345)) ;
#32229=CARTESIAN_POINT('Ctrl Pts',(-18.2138824565932,44.7943249331663,122.493298818431)) ;
#32230=CARTESIAN_POINT('Ctrl Pts',(-18.452951139445,44.6143358528034,122.677012948951)) ;
#32231=CARTESIAN_POINT('Ctrl Pts',(-18.3890982744024,44.8041913778294,122.302163339125)) ;
#32232=CARTESIAN_POINT('Ctrl Pts',(-18.5931221262605,44.6242022974665,122.524103052415)) ;
#32233=CARTESIAN_POINT('Ctrl Pts',(-18.5963979569655,44.8141575022781,122.142117824611)) ;
#32234=CARTESIAN_POINT('Ctrl Pts',(-18.7589604790486,44.6341684219152,122.396064874445)) ;
#32235=CARTESIAN_POINT('Ctrl Pts',(-18.8300300927451,44.8241877456692,122.020087986119)) ;
#32236=CARTESIAN_POINT('Ctrl Pts',(-18.9458651244295,44.6441986653064,122.298439056251)) ;
#32237=CARTESIAN_POINT('Ctrl Pts',(-19.0777784031114,44.8340807806223,121.941205272921)) ;
#32238=CARTESIAN_POINT('Ctrl Pts',(-19.1440629425059,44.6540917002594,122.235330716498)) ;
#32239=CARTESIAN_POINT('Ctrl Pts',(-19.3395157430304,44.8441316948591,121.905920090679)) ;
#32240=CARTESIAN_POINT('Ctrl Pts',(-19.3534531408236,44.6641426144963,122.207100459181)) ;
#32241=CARTESIAN_POINT('Ctrl Pts',(-19.5992088007417,44.8540215210837,121.916417743617)) ;
#32242=CARTESIAN_POINT('Ctrl Pts',(-19.561205041554,44.6740324407208,122.215496012711)) ;
#32243=CARTESIAN_POINT('Ctrl Pts',(-19.9417558495349,44.8673563361306,121.990481112151)) ;
#32244=CARTESIAN_POINT('Ctrl Pts',(-19.8352567550235,44.6873672557678,122.274745507017)) ;
#32245=CARTESIAN_POINT('Ctrl Pts',(-20.2554040575952,44.8806334273021,122.152088557895)) ;
#32246=CARTESIAN_POINT('Ctrl Pts',(-20.0861971038527,44.7006443469392,122.404050615546)) ;
#32247=CARTESIAN_POINT('Ctrl Pts',(-20.5136611155883,44.8938817159004,122.385626670228)) ;
#32248=CARTESIAN_POINT('Ctrl Pts',(-20.2927670421858,44.7138926355375,122.590851388565)) ;
#32249=CARTESIAN_POINT('Ctrl Pts',(-20.6757307463464,44.9039365573945,122.59426491759)) ;
#32250=CARTESIAN_POINT('Ctrl Pts',(-20.4224319383683,44.7239474770316,122.757766151545)) ;
#32251=CARTESIAN_POINT('Ctrl Pts',(-20.7967932245961,44.913767546702,122.822543238522)) ;
#32252=CARTESIAN_POINT('Ctrl Pts',(-20.5192820748052,44.7337784663392,122.940386237297)) ;
#32253=CARTESIAN_POINT('Ctrl Pts',(-20.8785256178797,44.9238441110252,123.074368365477)) ;
#32254=CARTESIAN_POINT('Ctrl Pts',(-20.5846700573935,44.7438550306624,123.141847246608)) ;
#32255=CARTESIAN_POINT('Ctrl Pts',(-20.9144646604309,44.9336934361592,123.330718388823)) ;
#32256=CARTESIAN_POINT('Ctrl Pts',(-20.6134249986564,44.7537043557963,123.346922032747)) ;
#32257=CARTESIAN_POINT('Ctrl Pts',(-20.9029627808752,44.9470414357965,123.681317025944)) ;
#32258=CARTESIAN_POINT('Ctrl Pts',(-20.60421795921,44.7670523554336,123.627426785072)) ;
#32259=CARTESIAN_POINT('Ctrl Pts',(-20.7745082951822,44.963626195333,124.10295325502)) ;
#32260=CARTESIAN_POINT('Ctrl Pts',(-20.5014772079403,44.7836371149701,123.964697051323)) ;
#32261=CARTESIAN_POINT('Ctrl Pts',(-20.5110259009966,44.9801947466811,124.455768261803)) ;
#32262=CARTESIAN_POINT('Ctrl Pts',(-20.2906509869384,44.8002056663183,124.247002496847)) ;
#32263=CARTESIAN_POINT('Ctrl Pts',(-20.2351348038895,44.9935545715001,124.672943272086)) ;
#32264=CARTESIAN_POINT('Ctrl Pts',(-20.0699761236227,44.8135654911373,124.420705379304)) ;
#32265=CARTESIAN_POINT('Ctrl Pts',(-20.0058393288218,45.0034599803308,124.796167835363)) ;
#32266=CARTESIAN_POINT('Ctrl Pts',(-19.8865323249825,44.8234708999679,124.519294746871)) ;
#32267=CARTESIAN_POINT('Ctrl Pts',(-19.757418400852,45.0134200069148,124.878510971796)) ;
#32268=CARTESIAN_POINT('Ctrl Pts',(-19.6878011258136,44.833430926552,124.585169321105)) ;
#32269=CARTESIAN_POINT('Ctrl Pts',(-19.4127381950797,45.0266775911001,124.929494089017)) ;
#32270=CARTESIAN_POINT('Ctrl Pts',(-19.4120406279165,44.8466885107373,124.62595768779)) ;
#32271=CARTESIAN_POINT('Ctrl Pts',(-18.9730728854828,45.0433288025948,124.878933487773)) ;
#32272=CARTESIAN_POINT('Ctrl Pts',(-19.0603260702002,44.8633397222319,124.585513496632)) ;
#32273=CARTESIAN_POINT('Ctrl Pts',(-18.4995381186548,45.0632470167051,124.642306903848)) ;
#32274=CARTESIAN_POINT('Ctrl Pts',(-18.6814904260909,44.8832579363422,124.396215029442)) ;
#32275=CARTESIAN_POINT('Ctrl Pts',(-18.1350210819867,45.0831247799259,124.259778759138)) ;
#32276=CARTESIAN_POINT('Ctrl Pts',(-18.3898754178223,44.9031356995631,124.090194473814)) ;
#32277=CARTESIAN_POINT('Ctrl Pts',(-17.9219902774577,45.1031374477131,123.772503946077)) ;
#32278=CARTESIAN_POINT('Ctrl Pts',(-18.219447255777,44.9231483673502,123.700376068826)) ;
#32279=CARTESIAN_POINT('Ctrl Pts',(-17.8878614143457,45.1229499703797,123.246927329174)) ;
#32280=CARTESIAN_POINT('Ctrl Pts',(-18.1921410117766,44.9429608900168,123.279913768998)) ;
#32281=CARTESIAN_POINT('Ctrl Pts',(-18.0355408684965,45.1429332703796,122.736855760796)) ;
#32282=CARTESIAN_POINT('Ctrl Pts',(-18.3102818169754,44.9629441900167,122.8718555916)) ;
#32283=CARTESIAN_POINT('Ctrl Pts',(-18.3474404946756,45.1628275474809,122.309788228837)) ;
#32284=CARTESIAN_POINT('Ctrl Pts',(-18.5597996758674,44.982838467118,122.530199273158)) ;
#32285=CARTESIAN_POINT('Ctrl Pts',(-18.786662149823,45.1827603092387,122.0135853007)) ;
#32286=CARTESIAN_POINT('Ctrl Pts',(-18.9111760676998,45.0027712288758,122.293234567284)) ;
#32287=CARTESIAN_POINT('Ctrl Pts',(-19.3015601046736,45.2027263150034,121.885187082688)) ;
#32288=CARTESIAN_POINT('Ctrl Pts',(-19.3230941010408,45.0227372346405,122.190513534484)) ;
#32289=CARTESIAN_POINT('Ctrl Pts',(-19.8271247057948,45.2226048471683,121.939586650986)) ;
#32290=CARTESIAN_POINT('Ctrl Pts',(-19.7435470906285,45.0426157668054,122.234031125667)) ;
#32291=CARTESIAN_POINT('Ctrl Pts',(-20.3041812489775,45.2425445138286,122.170281678288)) ;
#32292=CARTESIAN_POINT('Ctrl Pts',(-20.125193674908,45.0625554334657,122.418585724291)) ;
#32293=CARTESIAN_POINT('Ctrl Pts',(-20.673234757221,45.262439388474,122.549040856896)) ;
#32294=CARTESIAN_POINT('Ctrl Pts',(-20.4204384003569,45.0824503081111,122.721592696201)) ;
#32295=CARTESIAN_POINT('Ctrl Pts',(-20.8914226002841,45.2823465277673,123.03092366853)) ;
#32296=CARTESIAN_POINT('Ctrl Pts',(-20.5949902713448,45.1023574474044,123.107099401626)) ;
#32297=CARTESIAN_POINT('Ctrl Pts',(-20.933006994823,45.3022570758458,123.558648564266)) ;
#32298=CARTESIAN_POINT('Ctrl Pts',(-20.6282585345272,45.1222679954829,123.529280226432)) ;
#32299=CARTESIAN_POINT('Ctrl Pts',(-20.7897928711044,45.322325661203,124.072332126759)) ;
#32300=CARTESIAN_POINT('Ctrl Pts',(-20.513688465567,45.1423365808401,123.940226547894)) ;
#32301=CARTESIAN_POINT('Ctrl Pts',(-20.4845776581537,45.3421074585177,124.500648372566)) ;
#32302=CARTESIAN_POINT('Ctrl Pts',(-20.269515271003,45.1621183781549,124.282882031287)) ;
#32303=CARTESIAN_POINT('Ctrl Pts',(-20.0473359397164,45.3621150054623,124.802932073758)) ;
#32304=CARTESIAN_POINT('Ctrl Pts',(-19.9197218860292,45.1821259250994,124.524709061024)) ;
#32305=CARTESIAN_POINT('Ctrl Pts',(-19.5376317009415,45.3819367437651,124.936721152217)) ;
#32306=CARTESIAN_POINT('Ctrl Pts',(-19.5119562871531,45.2019476634022,124.631740691942)) ;
#32307=CARTESIAN_POINT('Ctrl Pts',(-19.0088087615849,45.4019167636693,124.889143040385)) ;
#32308=CARTESIAN_POINT('Ctrl Pts',(-19.0888977818351,45.2219276833064,124.593677332525)) ;
#32309=CARTESIAN_POINT('Ctrl Pts',(-18.5296775435496,45.4218342149315,124.664000015216)) ;
#32310=CARTESIAN_POINT('Ctrl Pts',(-18.7055922193586,45.2418451345686,124.413561830565)) ;
#32311=CARTESIAN_POINT('Ctrl Pts',(-18.1560490205525,45.4417091361042,124.2905332235)) ;
#32312=CARTESIAN_POINT('Ctrl Pts',(-18.4066894730446,45.2617200557413,124.114786420847)) ;
#32313=CARTESIAN_POINT('Ctrl Pts',(-17.9309504550834,45.461733504655,123.80830220994)) ;
#32314=CARTESIAN_POINT('Ctrl Pts',(-18.2266120673935,45.2817444242922,123.729001254374)) ;
#32315=CARTESIAN_POINT('Ctrl Pts',(-17.8844372685422,45.4816001890285,123.282245957211)) ;
#32316=CARTESIAN_POINT('Ctrl Pts',(-18.1894029640175,45.3016111086656,123.308154786778)) ;
#32317=CARTESIAN_POINT('Ctrl Pts',(-18.0199005695342,45.5015440108747,122.769835234287)) ;
#32318=CARTESIAN_POINT('Ctrl Pts',(-18.2977757249971,45.3215549305118,122.898226217715)) ;
#32319=CARTESIAN_POINT('Ctrl Pts',(-18.3217175474885,45.5214513801262,122.335254029468)) ;
#32320=CARTESIAN_POINT('Ctrl Pts',(-18.5392315505227,45.3414622997634,122.550561763219)) ;
#32321=CARTESIAN_POINT('Ctrl Pts',(-18.7524316861596,45.5413260778729,122.029454998175)) ;
#32322=CARTESIAN_POINT('Ctrl Pts',(-18.8838052127124,45.3613369975101,122.305924073514)) ;
#32323=CARTESIAN_POINT('Ctrl Pts',(-19.2643939100382,45.5613080203947,121.888099189238)) ;
#32324=CARTESIAN_POINT('Ctrl Pts',(-19.2933758171969,45.3813189400318,122.192842065019)) ;
#32325=CARTESIAN_POINT('Ctrl Pts',(-19.7916381676523,45.5812106873055,121.930204794695)) ;
#32326=CARTESIAN_POINT('Ctrl Pts',(-19.7151717616758,45.4012216069426,122.226529377587)) ;
#32327=CARTESIAN_POINT('Ctrl Pts',(-20.2724895989063,45.6010660448442,122.147814462636)) ;
#32328=CARTESIAN_POINT('Ctrl Pts',(-20.0998523930469,45.4210769644813,122.400620504394)) ;
#32329=CARTESIAN_POINT('Ctrl Pts',(-20.6536580199716,45.6211300835602,122.520640262332)) ;
#32330=CARTESIAN_POINT('Ctrl Pts',(-20.4047844905581,45.4411410031973,122.698883170157)) ;
#32331=CARTESIAN_POINT('Ctrl Pts',(-20.8822424651067,45.6409852632853,122.996499598304)) ;
#32332=CARTESIAN_POINT('Ctrl Pts',(-20.5876495721056,45.4609961829224,123.07957274604)) ;
#32333=CARTESIAN_POINT('Ctrl Pts',(-20.9354305273725,45.6609653679497,123.524661889087)) ;
#32334=CARTESIAN_POINT('Ctrl Pts',(-20.6301960379111,45.4809762875868,123.502103333297)) ;
#32335=CARTESIAN_POINT('Ctrl Pts',(-20.8068347567717,45.6807744731195,124.035365380666)) ;
#32336=CARTESIAN_POINT('Ctrl Pts',(-20.5273174457036,45.5007853927566,123.910665095287)) ;
#32337=CARTESIAN_POINT('Ctrl Pts',(-20.5095739145416,45.7007670934602,124.475605981024)) ;
#32338=CARTESIAN_POINT('Ctrl Pts',(-20.2894986134957,45.5207780130973,124.262859246648)) ;
#32339=CARTESIAN_POINT('Ctrl Pts',(-20.1539637829234,45.7173065759643,124.734247767366)) ;
#32340=CARTESIAN_POINT('Ctrl Pts',(-20.005029677627,45.5373174956014,124.469758245705)) ;
#32341=CARTESIAN_POINT('Ctrl Pts',(-19.826276696828,45.7306708940285,124.860455779892)) ;
#32342=CARTESIAN_POINT('Ctrl Pts',(-19.7428532302614,45.5506818136656,124.570733098296)) ;
#32343=CARTESIAN_POINT('Ctrl Pts',(-19.4853999049105,45.74388849653,124.927543476285)) ;
#32344=CARTESIAN_POINT('Ctrl Pts',(-19.4702042800056,45.5638994161671,124.624395485871)) ;
#32345=CARTESIAN_POINT('Ctrl Pts',(-19.0437646821752,45.7605460908078,124.897999792884)) ;
#32346=CARTESIAN_POINT('Ctrl Pts',(-19.1168393059101,45.5805570104449,124.60076273691)) ;
#32347=CARTESIAN_POINT('Ctrl Pts',(-18.5604443553513,45.7804117928495,124.685196121248)) ;
#32348=CARTESIAN_POINT('Ctrl Pts',(-18.7301974465919,45.6004227124867,124.430507595726)) ;
#32349=CARTESIAN_POINT('Ctrl Pts',(-18.240630590451,45.7970415195396,124.380241225691)) ;
#32350=CARTESIAN_POINT('Ctrl Pts',(-18.4743626408579,45.6170524391767,124.186562638723)) ;
#32351=CARTESIAN_POINT('Ctrl Pts',(-18.0589348454478,45.8103306346774,124.081934291346)) ;
#32352=CARTESIAN_POINT('Ctrl Pts',(-18.3289929495072,45.6303415543145,123.947896101221)) ;
#32353=CARTESIAN_POINT('Ctrl Pts',(-17.9633418369383,45.8202949816545,123.838171148512)) ;
#32354=CARTESIAN_POINT('Ctrl Pts',(-18.2525232679131,45.6403059012916,123.752891352259)) ;
#32355=CARTESIAN_POINT('Ctrl Pts',(-17.9115389081574,45.830223349656,123.582470100099)) ;
#32356=CARTESIAN_POINT('Ctrl Pts',(-18.2110838276306,45.6502342692931,123.548318177483)) ;
#32357=CARTESIAN_POINT('Ctrl Pts',(-17.9020047414413,45.8435067827447,123.233481404821)) ;
#32358=CARTESIAN_POINT('Ctrl Pts',(-18.2034517092472,45.6635177023819,123.269181304791)) ;
#32359=CARTESIAN_POINT('Ctrl Pts',(-18.0050894429486,45.8601588604851,122.80309786385)) ;
#32360=CARTESIAN_POINT('Ctrl Pts',(-18.2859374204291,45.6801697801222,122.924806771228)) ;
#32361=CARTESIAN_POINT('Ctrl Pts',(-18.2472042450846,45.8767102297859,122.435821289861)) ;
#32362=CARTESIAN_POINT('Ctrl Pts',(-18.4796083339964,45.696721149423,122.631034810004)) ;
#32363=CARTESIAN_POINT('Ctrl Pts',(-18.5078328375495,45.8899976579349,122.203411111269)) ;
#32364=CARTESIAN_POINT('Ctrl Pts',(-18.6881326846269,45.710008577572,122.445080306261)) ;
#32365=CARTESIAN_POINT('Ctrl Pts',(-18.7324749007102,45.900042197635,122.064839904029)) ;
#32366=CARTESIAN_POINT('Ctrl Pts',(-18.8678435288482,45.7200531172721,122.334231042964)) ;
#32367=CARTESIAN_POINT('Ctrl Pts',(-18.9727512214166,45.9098850394588,121.969029204104)) ;
#32368=CARTESIAN_POINT('Ctrl Pts',(-19.0600665012445,45.7298959590959,122.257583020281)) ;
#32369=CARTESIAN_POINT('Ctrl Pts',(-19.2294892302823,45.9198693237057,121.91505230479)) ;
#32370=CARTESIAN_POINT('Ctrl Pts',(-19.2654570275077,45.7398802433429,122.214404142504)) ;
#32371=CARTESIAN_POINT('Ctrl Pts',(-19.4908293876516,45.9298189691049,121.906556619496)) ;
#32372=CARTESIAN_POINT('Ctrl Pts',(-19.4745292486748,45.749829888742,122.207609741249)) ;
#32373=CARTESIAN_POINT('Ctrl Pts',(-19.7510268140243,45.9398187307933,121.943434488528)) ;
#32374=CARTESIAN_POINT('Ctrl Pts',(-19.6826867913636,45.7598296504304,122.23711429284)) ;
#32375=CARTESIAN_POINT('Ctrl Pts',(-20.0015055166855,45.9498500767522,122.02559641534)) ;
#32376=CARTESIAN_POINT('Ctrl Pts',(-19.8830690113146,45.7698609963893,122.302845959369)) ;
#32377=CARTESIAN_POINT('Ctrl Pts',(-20.230012990869,45.9597050312293,122.147483174595)) ;
#32378=CARTESIAN_POINT('Ctrl Pts',(-20.0658738423898,45.7797159508665,122.400357316511)) ;
#32379=CARTESIAN_POINT('Ctrl Pts',(-20.4366698390954,45.9696775692299,122.308599139529)) ;
#32380=CARTESIAN_POINT('Ctrl Pts',(-20.2311978645646,45.789688488867,122.529251805209)) ;
#32381=CARTESIAN_POINT('Ctrl Pts',(-20.6126387229705,45.9796725629648,122.503651259972)) ;
#32382=CARTESIAN_POINT('Ctrl Pts',(-20.3719712626983,45.7996834826019,122.685294957718)) ;
#32383=CARTESIAN_POINT('Ctrl Pts',(-20.7523044634586,45.9897066217589,122.727282847818)) ;
#32384=CARTESIAN_POINT('Ctrl Pts',(-20.4837019244027,45.809717541396,122.86420139806)) ;
#32385=CARTESIAN_POINT('Ctrl Pts',(-20.8496612407523,45.9995619645819,122.967303410869)) ;
#32386=CARTESIAN_POINT('Ctrl Pts',(-20.5615851977692,45.819572884219,123.056218516308)) ;
#32387=CARTESIAN_POINT('Ctrl Pts',(-20.9049869101856,46.0095614439275,123.224140951696)) ;
#32388=CARTESIAN_POINT('Ctrl Pts',(-20.6058435342198,45.8295723635646,123.261688948786)) ;
#32389=CARTESIAN_POINT('Ctrl Pts',(-20.9150723248034,46.0194558926828,123.484010185289)) ;
#32390=CARTESIAN_POINT('Ctrl Pts',(-20.6139096475916,45.8394668123199,123.469584210841)) ;
#32391=CARTESIAN_POINT('Ctrl Pts',(-20.8792184641045,46.0295190121173,123.745970407933)) ;
#32392=CARTESIAN_POINT('Ctrl Pts',(-20.5852243537012,45.8495299317544,123.67915211632)) ;
#32393=CARTESIAN_POINT('Ctrl Pts',(-20.8004631964166,46.0393586573585,123.992305910844)) ;
#32394=CARTESIAN_POINT('Ctrl Pts',(-20.5222181446683,45.8593695769957,123.876219533294)) ;
#32395=CARTESIAN_POINT('Ctrl Pts',(-20.6777341782391,46.0494218215446,124.226510235197)) ;
#32396=CARTESIAN_POINT('Ctrl Pts',(-20.4240329804487,45.8694327411817,124.063582012675)) ;
#32397=CARTESIAN_POINT('Ctrl Pts',(-20.5187010120317,46.0593160912934,124.432251752361)) ;
#32398=CARTESIAN_POINT('Ctrl Pts',(-20.2968048726953,45.8793270109305,124.228173673899)) ;
#32399=CARTESIAN_POINT('Ctrl Pts',(-20.3259612493778,46.0692578173072,124.608573010416)) ;
#32400=CARTESIAN_POINT('Ctrl Pts',(-20.1426117715884,45.8892687369444,124.369228956089)) ;
#32401=CARTESIAN_POINT('Ctrl Pts',(-20.1041752620859,46.0792607059666,124.749748717296)) ;
#32402=CARTESIAN_POINT('Ctrl Pts',(-19.965181898146,45.8992716256037,124.48216768824)) ;
#32403=CARTESIAN_POINT('Ctrl Pts',(-19.8602243413917,46.0893005547606,124.850170623594)) ;
#32404=CARTESIAN_POINT('Ctrl Pts',(-19.770020308728,45.9093114743977,124.562503212813)) ;
#32405=CARTESIAN_POINT('Ctrl Pts',(-19.6081586045614,46.0991247702215,124.906078173757)) ;
#32406=CARTESIAN_POINT('Ctrl Pts',(-19.5683677549541,45.9191356898586,124.607227074532)) ;
#32407=CARTESIAN_POINT('Ctrl Pts',(-19.3441646598656,46.109181613715,124.918003343611)) ;
#32408=CARTESIAN_POINT('Ctrl Pts',(-19.3571724382085,45.9291925333521,124.616765131644)) ;
#32409=CARTESIAN_POINT('Ctrl Pts',(-19.0854647176779,46.119110223111,124.883999596897)) ;
#32410=CARTESIAN_POINT('Ctrl Pts',(-19.150213020904,45.9391211427481,124.589560066791)) ;
#32411=CARTESIAN_POINT('Ctrl Pts',(-18.8357963857665,46.1290621071489,124.806111234111)) ;
#32412=CARTESIAN_POINT('Ctrl Pts',(-18.9504791821078,45.949073026786,124.527247495769)) ;
#32413=CARTESIAN_POINT('Ctrl Pts',(-18.6013290923237,46.1391150599565,124.684426223968)) ;
#32414=CARTESIAN_POINT('Ctrl Pts',(-18.7629062354974,45.9591259795936,124.429897589284)) ;
#32415=CARTESIAN_POINT('Ctrl Pts',(-18.3960311454174,46.1489379364227,124.527912441961)) ;
#32416=CARTESIAN_POINT('Ctrl Pts',(-18.5986696124886,45.9689488560598,124.304685323724)) ;
#32417=CARTESIAN_POINT('Ctrl Pts',(-18.2165638688177,46.1589936689928,124.333973843009)) ;
#32418=CARTESIAN_POINT('Ctrl Pts',(-18.455097186173,45.9790045886299,124.149533032839)) ;
#32419=CARTESIAN_POINT('Ctrl Pts',(-18.0755063145666,46.1689344339805,124.114086515428)) ;
#32420=CARTESIAN_POINT('Ctrl Pts',(-18.3422530053555,45.9889453536176,123.973622294175)) ;
#32421=CARTESIAN_POINT('Ctrl Pts',(-17.9743911402895,46.1788387668861,123.874249737998)) ;
#32422=CARTESIAN_POINT('Ctrl Pts',(-18.2613628144267,45.9988496865232,123.781752514046)) ;
#32423=CARTESIAN_POINT('Ctrl Pts',(-17.9157922099519,46.1888854357668,123.616841983496)) ;
#32424=CARTESIAN_POINT('Ctrl Pts',(-18.2144855602764,46.0088963554039,123.575825794976)) ;
#32425=CARTESIAN_POINT('Ctrl Pts',(-17.9027335515217,46.1987809990726,123.357082770937)) ;
#32426=CARTESIAN_POINT('Ctrl Pts',(-18.2040405772589,46.0187919187097,123.368018794538)) ;
#32427=CARTESIAN_POINT('Ctrl Pts',(-17.9355083348723,46.2088430567729,123.094739738878)) ;
#32428=CARTESIAN_POINT('Ctrl Pts',(-18.2302623332334,46.02885397641,123.158144462417)) ;
#32429=CARTESIAN_POINT('Ctrl Pts',(-18.0115191596736,46.2186858344004,122.847471415839)) ;
#32430=CARTESIAN_POINT('Ctrl Pts',(-18.2910726074192,46.0386967540375,122.960331026345)) ;
#32431=CARTESIAN_POINT('Ctrl Pts',(-18.1304936326855,46.2286763126523,122.613475678947)) ;
#32432=CARTESIAN_POINT('Ctrl Pts',(-18.3862537375702,46.0486872322894,122.773135382181)) ;
#32433=CARTESIAN_POINT('Ctrl Pts',(-18.2873793152529,46.2386052852958,122.404966075839)) ;
#32434=CARTESIAN_POINT('Ctrl Pts',(-18.5117634954812,46.0586162049329,122.60632910476)) ;
#32435=CARTESIAN_POINT('Ctrl Pts',(-18.4789900283898,46.2485964221754,122.225460708948)) ;
#32436=CARTESIAN_POINT('Ctrl Pts',(-18.6650531643566,46.0686073418125,122.462726177038)) ;
#32437=CARTESIAN_POINT('Ctrl Pts',(-18.6997158872876,46.2586185396643,122.081771774985)) ;
#32438=CARTESIAN_POINT('Ctrl Pts',(-18.8416348469598,46.0786294593014,122.347776532043)) ;
#32439=CARTESIAN_POINT('Ctrl Pts',(-18.9390004515799,46.2685190500665,121.97961691748)) ;
#32440=CARTESIAN_POINT('Ctrl Pts',(-19.0330627062083,46.0885299697036,122.266054470778)) ;
#32441=CARTESIAN_POINT('Ctrl Pts',(-19.1945546489749,46.2785080428126,121.919635191703)) ;
#32442=CARTESIAN_POINT('Ctrl Pts',(-19.2375063079573,46.0985189624497,122.218070771051)) ;
#32443=CARTESIAN_POINT('Ctrl Pts',(-19.4560195398829,46.2884732868632,121.905154403475)) ;
#32444=CARTESIAN_POINT('Ctrl Pts',(-19.4466780569291,46.1084842065003,122.206487877725)) ;
#32445=CARTESIAN_POINT('Ctrl Pts',(-19.7145391120576,46.2983775513764,121.93549611882)) ;
#32446=CARTESIAN_POINT('Ctrl Pts',(-19.653492980395,46.1183884710135,122.230762786779)) ;
#32447=CARTESIAN_POINT('Ctrl Pts',(-19.9676465193919,46.3084356430746,122.011573715253)) ;
#32448=CARTESIAN_POINT('Ctrl Pts',(-19.8559786088564,46.1284465627118,122.291626492136)) ;
#32449=CARTESIAN_POINT('Ctrl Pts',(-20.1989353902242,46.318285583503,122.127826794879)) ;
#32450=CARTESIAN_POINT('Ctrl Pts',(-20.0410082397393,46.1382965031402,122.384630018431)) ;
#32451=CARTESIAN_POINT('Ctrl Pts',(-20.4106296400589,46.3283125946766,122.284718430549)) ;
#32452=CARTESIAN_POINT('Ctrl Pts',(-20.2103627795123,46.1483235143137,122.510144538498)) ;
#32453=CARTESIAN_POINT('Ctrl Pts',(-20.5914073282754,46.3383411812886,122.476498822217)) ;
#32454=CARTESIAN_POINT('Ctrl Pts',(-20.3549837916193,46.1583521009257,122.663570001819)) ;
#32455=CARTESIAN_POINT('Ctrl Pts',(-20.7338884447941,46.3481863954013,122.692436981991)) ;
#32456=CARTESIAN_POINT('Ctrl Pts',(-20.4689669204349,46.1681973150384,122.836320620193)) ;
#32457=CARTESIAN_POINT('Ctrl Pts',(-20.838883297733,46.3581771435809,122.933081577216)) ;
#32458=CARTESIAN_POINT('Ctrl Pts',(-20.5529614728706,46.178188063218,123.028836705902)) ;
#32459=CARTESIAN_POINT('Ctrl Pts',(-20.9002222159883,46.3682147771664,123.1896289369)) ;
#32460=CARTESIAN_POINT('Ctrl Pts',(-20.6020311735636,46.1882256968035,123.234075045714)) ;
#32461=CARTESIAN_POINT('Ctrl Pts',(-20.9162101455242,46.3780600663792,123.447862222641)) ;
#32462=CARTESIAN_POINT('Ctrl Pts',(-20.614820050469,46.1980709860163,123.440660827507)) ;
#32463=CARTESIAN_POINT('Ctrl Pts',(-20.8872976540046,46.3880414671851,123.708544539136)) ;
#32464=CARTESIAN_POINT('Ctrl Pts',(-20.5916887966278,46.2080523868222,123.649206325939)) ;
#32465=CARTESIAN_POINT('Ctrl Pts',(-20.8137082785738,46.397993700175,123.959520057968)) ;
#32466=CARTESIAN_POINT('Ctrl Pts',(-20.5328161531047,46.2180046198121,123.849986010889)) ;
#32467=CARTESIAN_POINT('Ctrl Pts',(-20.6974169783614,46.4079925116317,124.195165716517)) ;
#32468=CARTESIAN_POINT('Ctrl Pts',(-20.4397820581274,46.2280034312688,124.038501896986)) ;
#32469=CARTESIAN_POINT('Ctrl Pts',(-20.5409623495954,46.4180316155623,124.407564420263)) ;
#32470=CARTESIAN_POINT('Ctrl Pts',(-20.3146171987756,46.2380425351995,124.208420165923)) ;
#32471=CARTESIAN_POINT('Ctrl Pts',(-20.3544390959673,46.4278565579816,124.586111387913)) ;
#32472=CARTESIAN_POINT('Ctrl Pts',(-20.1653985485672,46.2478674776188,124.351256099726)) ;
#32473=CARTESIAN_POINT('Ctrl Pts',(-20.134995919871,46.4379112454576,124.733256870576)) ;
#32474=CARTESIAN_POINT('Ctrl Pts',(-19.9898432095306,46.2579221650947,124.468971664984)) ;
#32475=CARTESIAN_POINT('Ctrl Pts',(-19.8958234362632,46.4478540478144,124.838477290274)) ;
#32476=CARTESIAN_POINT('Ctrl Pts',(-19.7985051353793,46.2678649674515,124.553146698639)) ;
#32477=CARTESIAN_POINT('Ctrl Pts',(-19.6432030628621,46.4577578437542,124.901101950844)) ;
#32478=CARTESIAN_POINT('Ctrl Pts',(-19.5964092448346,46.2777687633913,124.603245250316)) ;
#32479=CARTESIAN_POINT('Ctrl Pts',(-19.3798141419767,46.4678046231292,124.919009575157)) ;
#32480=CARTESIAN_POINT('Ctrl Pts',(-19.3856978663707,46.2878155427663,124.61757028202)) ;
#32481=CARTESIAN_POINT('Ctrl Pts',(-19.1211811679258,46.4777002814238,124.891553789188)) ;
#32482=CARTESIAN_POINT('Ctrl Pts',(-19.1787923210989,46.2977112010609,124.595604707242)) ;
#32483=CARTESIAN_POINT('Ctrl Pts',(-18.8671103311317,46.4877618486744,124.818449852984)) ;
#32484=CARTESIAN_POINT('Ctrl Pts',(-18.9755356841084,46.3077727683115,124.537120502504)) ;
#32485=CARTESIAN_POINT('Ctrl Pts',(-18.6346615958398,46.4976064931117,124.704865605345)) ;
#32486=CARTESIAN_POINT('Ctrl Pts',(-18.7895780913401,46.3176174127489,124.446252657151)) ;
#32487=CARTESIAN_POINT('Ctrl Pts',(-18.4224718070244,46.5075665393544,124.551629282646)) ;
#32488=CARTESIAN_POINT('Ctrl Pts',(-18.6198270211866,46.3275774589915,124.32366317014)) ;
#32489=CARTESIAN_POINT('Ctrl Pts',(-18.2390573894743,46.5176048353728,124.362048863107)) ;
#32490=CARTESIAN_POINT('Ctrl Pts',(-18.4730960549805,46.3376157550099,124.171998104319)) ;
#32491=CARTESIAN_POINT('Ctrl Pts',(-18.0933321835797,46.5274781767911,124.147328823137)) ;
#32492=CARTESIAN_POINT('Ctrl Pts',(-18.3565170542774,46.3474890964282,124.00022237033)) ;
#32493=CARTESIAN_POINT('Ctrl Pts',(-17.9850644966569,46.5375512805904,123.905828159884)) ;
#32494=CARTESIAN_POINT('Ctrl Pts',(-18.2699035102688,46.3575622002275,123.80702119456)) ;
#32495=CARTESIAN_POINT('Ctrl Pts',(-17.9216561766812,46.5473720957093,123.655604769692)) ;
#32496=CARTESIAN_POINT('Ctrl Pts',(-18.219177873809,46.3673830153464,123.606843503252)) ;
#32497=CARTESIAN_POINT('Ctrl Pts',(-17.9018683250634,46.5574489607873,123.391584873684)) ;
#32498=CARTESIAN_POINT('Ctrl Pts',(-18.2033482278461,46.3774598804244,123.395627180007)) ;
#32499=CARTESIAN_POINT('Ctrl Pts',(-17.9277757499098,46.5673137004426,123.133615388447)) ;
#32500=CARTESIAN_POINT('Ctrl Pts',(-18.2240747548872,46.3873246200797,123.189252631798)) ;
#32501=CARTESIAN_POINT('Ctrl Pts',(-17.9985297244048,46.5773361036839,122.879929630516)) ;
#32502=CARTESIAN_POINT('Ctrl Pts',(-18.2806784477161,46.397347023321,122.98630413088)) ;
#32503=CARTESIAN_POINT('Ctrl Pts',(-18.1129004945136,46.5873618279724,122.642565399525)) ;
#32504=CARTESIAN_POINT('Ctrl Pts',(-18.3721757093272,46.4073727476095,122.796412980426)) ;
#32505=CARTESIAN_POINT('Ctrl Pts',(-18.2637366876288,46.5972166109937,122.432070963929)) ;
#32506=CARTESIAN_POINT('Ctrl Pts',(-18.4928445100312,46.4172275306308,122.628018630033)) ;
#32507=CARTESIAN_POINT('Ctrl Pts',(-18.4506972916997,46.607195454717,122.248181197861)) ;
#32508=CARTESIAN_POINT('Ctrl Pts',(-18.6424130861803,46.4272063743541,122.48090728997)) ;
#32509=CARTESIAN_POINT('Ctrl Pts',(-18.6678559884878,46.6172143469536,122.099336220667)) ;
#32510=CARTESIAN_POINT('Ctrl Pts',(-18.8161403445689,46.4372252665907,122.361831725201)) ;
#32511=CARTESIAN_POINT('Ctrl Pts',(-18.9041339832422,46.6270975559946,121.991423381431)) ;
#32512=CARTESIAN_POINT('Ctrl Pts',(-19.0051620983221,46.4471084756317,122.275502163927)) ;
#32513=CARTESIAN_POINT('Ctrl Pts',(-19.1602204279234,46.6371658653348,121.925081449906)) ;
#32514=CARTESIAN_POINT('Ctrl Pts',(-19.2100316746212,46.4571767849719,122.222428931168)) ;
#32515=CARTESIAN_POINT('Ctrl Pts',(-19.4177614318243,46.6469959906675,121.904397063364)) ;
#32516=CARTESIAN_POINT('Ctrl Pts',(-19.4160632754822,46.4670069103046,122.205881850108)) ;
#32517=CARTESIAN_POINT('Ctrl Pts',(-19.6811124793488,46.6570625430445,121.928980404509)) ;
#32518=CARTESIAN_POINT('Ctrl Pts',(-19.6267444075026,46.4770734626816,122.22554879681)) ;
#32519=CARTESIAN_POINT('Ctrl Pts',(-19.93175625164,46.6669527799382,121.997866497326)) ;
#32520=CARTESIAN_POINT('Ctrl Pts',(-19.8272585403738,46.4869636995753,122.280657725669)) ;
#32521=CARTESIAN_POINT('Ctrl Pts',(-20.1692553844016,46.6769450047322,122.109835361796)) ;
#32522=CARTESIAN_POINT('Ctrl Pts',(-20.0172576312731,46.4969559243693,122.370232872609)) ;
#32523=CARTESIAN_POINT('Ctrl Pts',(-20.3829389131417,46.6869076250832,122.261097188161)) ;
#32524=CARTESIAN_POINT('Ctrl Pts',(-20.1882040373504,46.5069185447203,122.491242289893)) ;
#32525=CARTESIAN_POINT('Ctrl Pts',(-20.5665204839457,46.6968126278463,122.445649602459)) ;
#32526=CARTESIAN_POINT('Ctrl Pts',(-20.3350687382439,46.5168235474834,122.638883718221)) ;
#32527=CARTESIAN_POINT('Ctrl Pts',(-20.7173901651887,46.7068703902444,122.662639131591)) ;
#32528=CARTESIAN_POINT('Ctrl Pts',(-20.4557645655042,46.5268813098816,122.812475613443)) ;
#32529=CARTESIAN_POINT('Ctrl Pts',(-20.8262181894773,46.7167209096232,122.89753556539)) ;
#32530=CARTESIAN_POINT('Ctrl Pts',(-20.5428264841465,46.5367318292604,123.000391752439)) ;
#32531=CARTESIAN_POINT('Ctrl Pts',(-20.8943773618054,46.7267524866214,123.15217347503)) ;
#32532=CARTESIAN_POINT('Ctrl Pts',(-20.5973539588229,46.5467634062585,123.204102140928)) ;
#32533=CARTESIAN_POINT('Ctrl Pts',(-20.9167369790523,46.7367622217263,123.414295804395)) ;
#32534=CARTESIAN_POINT('Ctrl Pts',(-20.6152416326084,46.5567731413635,123.413799972381)) ;
#32535=CARTESIAN_POINT('Ctrl Pts',(-20.8937123153054,46.7466717983526,123.673666920638)) ;
#32536=CARTESIAN_POINT('Ctrl Pts',(-20.596822009193,46.5666827179897,123.621296152954)) ;
#32537=CARTESIAN_POINT('Ctrl Pts',(-20.8265171674148,46.7565991842093,123.925758286608)) ;
#32538=CARTESIAN_POINT('Ctrl Pts',(-20.5430662495124,46.5766101038464,123.822968723922)) ;
#32539=CARTESIAN_POINT('Ctrl Pts',(-20.7150850922258,46.7666441186995,124.165042883978)) ;
#32540=CARTESIAN_POINT('Ctrl Pts',(-20.4539206594605,46.5866550383367,124.014396623228)) ;
#32541=CARTESIAN_POINT('Ctrl Pts',(-20.566303423748,46.7765300508875,124.378031588581)) ;
#32542=CARTESIAN_POINT('Ctrl Pts',(-20.3348959856929,46.5965409705246,124.184786987194)) ;
#32543=CARTESIAN_POINT('Ctrl Pts',(-20.3811494336437,46.7865233568405,124.56424680321)) ;
#32544=CARTESIAN_POINT('Ctrl Pts',(-20.1867731294926,46.6065342764777,124.333759263123)) ;
#32545=CARTESIAN_POINT('Ctrl Pts',(-20.167426750717,46.7964689946224,124.714688252167)) ;
#32546=CARTESIAN_POINT('Ctrl Pts',(-20.0157955364757,46.6164799142595,124.454112381368)) ;
#32547=CARTESIAN_POINT('Ctrl Pts',(-19.9310071201226,46.8064162629683,124.826243396208)) ;
#32548=CARTESIAN_POINT('Ctrl Pts',(-19.8266604269535,46.6264271826054,124.543356680596)) ;
#32549=CARTESIAN_POINT('Ctrl Pts',(-19.6762006528589,46.8164641651054,124.895457669008)) ;
#32550=CARTESIAN_POINT('Ctrl Pts',(-19.6228151502625,46.6364750847425,124.598728484168)) ;
#32551=CARTESIAN_POINT('Ctrl Pts',(-19.4184961828357,46.8263118599456,124.91911890289)) ;
#32552=CARTESIAN_POINT('Ctrl Pts',(-19.4166527254704,46.6463227795827,124.617657767164)) ;
#32553=CARTESIAN_POINT('Ctrl Pts',(-19.1575612607115,46.83627336969,124.898251094209)) ;
#32554=CARTESIAN_POINT('Ctrl Pts',(-19.2079051028574,46.6562842893271,124.600964154411)) ;
#32555=CARTESIAN_POINT('Ctrl Pts',(-18.902556312997,46.8463027612989,124.831598304346)) ;
#32556=CARTESIAN_POINT('Ctrl Pts',(-19.0039009355955,46.666313680936,124.54764240293)) ;
#32557=CARTESIAN_POINT('Ctrl Pts',(-18.6658571373904,46.8562102568536,124.723148671996)) ;
#32558=CARTESIAN_POINT('Ctrl Pts',(-18.8145420155273,46.6762211764908,124.460883498429)) ;
#32559=CARTESIAN_POINT('Ctrl Pts',(-18.4504873824993,46.8661556485166,124.575124657286)) ;
#32560=CARTESIAN_POINT('Ctrl Pts',(-18.6422462094197,46.6861665681538,124.342465111585)) ;
#32561=CARTESIAN_POINT('Ctrl Pts',(-18.262882041295,46.876157566114,124.390984128)) ;
#32562=CARTESIAN_POINT('Ctrl Pts',(-18.4921615041804,46.6961684857511,124.195153273134)) ;
#32563=CARTESIAN_POINT('Ctrl Pts',(-18.1099479381027,46.8861976336662,124.176016249327)) ;
#32564=CARTESIAN_POINT('Ctrl Pts',(-18.3698136515618,46.7062085533033,124.023179206255)) ;
#32565=CARTESIAN_POINT('Ctrl Pts',(-17.998547175216,46.896021945106,123.943090129844)) ;
#32566=CARTESIAN_POINT('Ctrl Pts',(-18.280692897445,46.7160328647431,123.836839731432)) ;
#32567=CARTESIAN_POINT('Ctrl Pts',(-17.9273097685191,46.9060781862621,123.688632681324)) ;
#32568=CARTESIAN_POINT('Ctrl Pts',(-18.2237021026595,46.7260891058992,123.633273756565)) ;
#32569=CARTESIAN_POINT('Ctrl Pts',(-17.9019600484687,46.9160091079977,123.4288626675)) ;
#32570=CARTESIAN_POINT('Ctrl Pts',(-18.2034216287563,46.7360200276349,123.425458357104)) ;
#32571=CARTESIAN_POINT('Ctrl Pts',(-17.9215882488076,46.925952344074,123.168336310537)) ;
#32572=CARTESIAN_POINT('Ctrl Pts',(-18.2191232721713,46.7459632637111,123.217037686628)) ;
#32573=CARTESIAN_POINT('Ctrl Pts',(-17.9861745623724,46.9359336280864,122.914073624315)) ;
#32574=CARTESIAN_POINT('Ctrl Pts',(-18.2707913566683,46.7559445477236,123.01362751071)) ;
#32575=CARTESIAN_POINT('Ctrl Pts',(-18.0949933336756,46.9459779297121,122.673631325158)) ;
#32576=CARTESIAN_POINT('Ctrl Pts',(-18.3578456757999,46.7659888493492,122.821273187654)) ;
#32577=CARTESIAN_POINT('Ctrl Pts',(-18.2402478329783,46.9558060109315,122.460027367171)) ;
#32578=CARTESIAN_POINT('Ctrl Pts',(-18.474047818082,46.7758169305687,122.650390426094)) ;
#32579=CARTESIAN_POINT('Ctrl Pts',(-18.4247793331419,46.9658826137807,122.270186990604)) ;
#32580=CARTESIAN_POINT('Ctrl Pts',(-18.6216725361831,46.7858935334178,122.498517174402)) ;
#32581=CARTESIAN_POINT('Ctrl Pts',(-18.6347009617729,46.9757346928992,122.118553078034)) ;
#32582=CARTESIAN_POINT('Ctrl Pts',(-18.789608433041,46.7957456125364,122.377209782781)) ;
#32583=CARTESIAN_POINT('Ctrl Pts',(-18.8728048873028,46.9858079512082,122.002979006205)) ;
#32584=CARTESIAN_POINT('Ctrl Pts',(-18.9800913870549,46.8058188708453,122.28474940667)) ;
#32585=CARTESIAN_POINT('Ctrl Pts',(-19.1215801045156,46.9956494105884,121.93222329205)) ;
#32586=CARTESIAN_POINT('Ctrl Pts',(-19.1791102655951,46.8156603302256,122.228144091495)) ;
#32587=CARTESIAN_POINT('Ctrl Pts',(-19.381859343394,47.0056105060008,121.904442012515)) ;
#32588=CARTESIAN_POINT('Ctrl Pts',(-19.3873331982892,46.8256214256379,122.205917820199)) ;
#32589=CARTESIAN_POINT('Ctrl Pts',(-19.6449738782894,47.0156477903975,121.922928491226)) ;
#32590=CARTESIAN_POINT('Ctrl Pts',(-19.5978250114014,46.8356587100347,122.220705838776)) ;
#32591=CARTESIAN_POINT('Ctrl Pts',(-19.8969217299239,47.0255241291328,121.985363214302)) ;
#32592=CARTESIAN_POINT('Ctrl Pts',(-19.7993828256105,46.8455350487699,122.270652190592)) ;
#32593=CARTESIAN_POINT('Ctrl Pts',(-20.1386279884017,47.0355862552861,122.092504779786)) ;
#32594=CARTESIAN_POINT('Ctrl Pts',(-19.9927485620531,46.8555971749232,122.356364359904)) ;
#32595=CARTESIAN_POINT('Ctrl Pts',(-20.3539188130597,47.0454544292626,122.237128270037)) ;
#32596=CARTESIAN_POINT('Ctrl Pts',(-20.1649812567676,46.8654653488997,122.472061612692)) ;
#32597=CARTESIAN_POINT('Ctrl Pts',(-20.5437493740665,47.0554599777664,122.419010050859)) ;
#32598=CARTESIAN_POINT('Ctrl Pts',(-20.3168466298338,46.8754708974035,122.617565974457)) ;
#32599=CARTESIAN_POINT('Ctrl Pts',(-20.6987362985448,47.065442609662,122.630724270001)) ;
#32600=CARTESIAN_POINT('Ctrl Pts',(-20.440837183443,46.8854535292991,122.786936385641)) ;
#32601=CARTESIAN_POINT('Ctrl Pts',(-20.8150425909332,47.0754865520838,122.867637130232)) ;
#32602=CARTESIAN_POINT('Ctrl Pts',(-20.5338834673555,46.8954974717209,122.976466203145)) ;
#32603=CARTESIAN_POINT('Ctrl Pts',(-20.8872078791894,47.0853147001109,123.115624213289)) ;
#32604=CARTESIAN_POINT('Ctrl Pts',(-20.5916167561873,46.9053256197481,123.174854489363)) ;
#32605=CARTESIAN_POINT('Ctrl Pts',(-20.9165166534759,47.0953045674853,123.37650718992)) ;
#32606=CARTESIAN_POINT('Ctrl Pts',(-20.6150653220902,46.9153154871225,123.383560557976)) ;
#32607=CARTESIAN_POINT('Ctrl Pts',(-20.8993091493922,47.1053483064408,123.639884268201)) ;
#32608=CARTESIAN_POINT('Ctrl Pts',(-20.6013007427833,46.925359226078,123.594262430873)) ;
#32609=CARTESIAN_POINT('Ctrl Pts',(-20.8385403650369,47.1151700549788,123.890732974447)) ;
#32610=CARTESIAN_POINT('Ctrl Pts',(-20.5526874481851,46.9351809746159,123.794940790409)) ;
#32611=CARTESIAN_POINT('Ctrl Pts',(-20.7334869965978,47.1252050325885,124.132613019297)) ;
#32612=CARTESIAN_POINT('Ctrl Pts',(-20.4686462451259,46.9452159522256,123.988445566052)) ;
#32613=CARTESIAN_POINT('Ctrl Pts',(-20.5875612969449,47.1352299453462,124.351957946675)) ;
#32614=CARTESIAN_POINT('Ctrl Pts',(-20.3519069440029,46.9552408649833,124.163922368766)) ;
#32615=CARTESIAN_POINT('Ctrl Pts',(-20.4093144805832,47.14508188844,124.539733165987)) ;
#32616=CARTESIAN_POINT('Ctrl Pts',(-20.209311228941,46.9650928080772,124.314143082127)) ;
#32617=CARTESIAN_POINT('Ctrl Pts',(-20.1985036701278,47.1550728497691,124.69617951058)) ;
#32618=CARTESIAN_POINT('Ctrl Pts',(-20.0406637063053,46.9750837694063,124.439301445059)) ;
#32619=CARTESIAN_POINT('Ctrl Pts',(-19.9654674976531,47.1649907246376,124.812968953075)) ;
#32620=CARTESIAN_POINT('Ctrl Pts',(-19.8542359521288,46.9850016442747,124.532734341221)) ;
#32621=CARTESIAN_POINT('Ctrl Pts',(-19.71297510293,47.1750192436388,124.88839013585)) ;
#32622=CARTESIAN_POINT('Ctrl Pts',(-19.652242507693,46.9950301632759,124.593072964507)) ;
#32623=CARTESIAN_POINT('Ctrl Pts',(-19.4549854354218,47.1849029224366,124.918522015687)) ;
#32624=CARTESIAN_POINT('Ctrl Pts',(-19.4458515655707,47.0049138420738,124.617180149726)) ;
#32625=CARTESIAN_POINT('Ctrl Pts',(-19.1927415406444,47.1948978658764,124.903808702217)) ;
#32626=CARTESIAN_POINT('Ctrl Pts',(-19.2360564571309,47.0149087855135,124.605411359916)) ;
#32627=CARTESIAN_POINT('Ctrl Pts',(-18.9363215273581,47.2049247196988,124.843152452533)) ;
#32628=CARTESIAN_POINT('Ctrl Pts',(-19.0309200183396,47.0249356393359,124.55688809248)) ;
#32629=CARTESIAN_POINT('Ctrl Pts',(-18.6976217950589,47.2148088840377,124.740702605869)) ;
#32630=CARTESIAN_POINT('Ctrl Pts',(-18.8399600159307,47.0348198036749,124.47493012311)) ;
#32631=CARTESIAN_POINT('Ctrl Pts',(-18.4778918251213,47.2247969820801,124.597178175501)) ;
#32632=CARTESIAN_POINT('Ctrl Pts',(-18.6641751118157,47.0448079017172,124.360112235116)) ;
#32633=CARTESIAN_POINT('Ctrl Pts',(-18.2869868870465,47.2347480885372,124.418412493407)) ;
#32634=CARTESIAN_POINT('Ctrl Pts',(-18.511450049831,47.0547590081743,124.2171012666)) ;
#32635=CARTESIAN_POINT('Ctrl Pts',(-18.1286864683151,47.2447931397053,124.207190353518)) ;
#32636=CARTESIAN_POINT('Ctrl Pts',(-18.3848081587268,47.0648040593424,124.048124631986)) ;
#32637=CARTESIAN_POINT('Ctrl Pts',(-18.0115053675036,47.2546549000636,123.976037450219)) ;
#32638=CARTESIAN_POINT('Ctrl Pts',(-18.2910618397786,47.0746658197007,123.863203703224)) ;
#32639=CARTESIAN_POINT('Ctrl Pts',(-17.9346962187188,47.264617716894,123.725744078448)) ;
#32640=CARTESIAN_POINT('Ctrl Pts',(-18.2296126464617,47.0846286365312,123.662969789116)) ;
#32641=CARTESIAN_POINT('Ctrl Pts',(-17.9027315659369,47.2746523981748,123.463999492697)) ;
#32642=CARTESIAN_POINT('Ctrl Pts',(-18.2040389739103,47.0946633178119,123.453574331988)) ;
#32643=CARTESIAN_POINT('Ctrl Pts',(-17.9160504867167,47.2845374279556,123.204536864795)) ;
#32644=CARTESIAN_POINT('Ctrl Pts',(-18.214692073012,47.1045483475927,123.246004576489)) ;
#32645=CARTESIAN_POINT('Ctrl Pts',(-17.9753215326006,47.2946030213536,122.946793722897)) ;
#32646=CARTESIAN_POINT('Ctrl Pts',(-18.2621069751575,47.1146139409907,123.039809496486)) ;
#32647=CARTESIAN_POINT('Ctrl Pts',(-18.0759175402315,47.3044421897151,122.708557598471)) ;
#32648=CARTESIAN_POINT('Ctrl Pts',(-18.3425816822834,47.1244531093522,122.84922032325)) ;
#32649=CARTESIAN_POINT('Ctrl Pts',(-18.2191949884316,47.3145047874566,122.486339905974)) ;
#32650=CARTESIAN_POINT('Ctrl Pts',(-18.4572019469866,47.1345157070937,122.671444952012)) ;
#32651=CARTESIAN_POINT('Ctrl Pts',(-18.396159615514,47.3244017998635,122.295722821703)) ;
#32652=CARTESIAN_POINT('Ctrl Pts',(-18.5987718917569,47.1444127195006,122.518950162102)) ;
#32653=CARTESIAN_POINT('Ctrl Pts',(-18.6037098264549,47.3343331216891,122.137504758704)) ;
#32654=CARTESIAN_POINT('Ctrl Pts',(-18.7648105710639,47.1543440413262,122.392374154288)) ;
#32655=CARTESIAN_POINT('Ctrl Pts',(-18.8382907890392,47.3443748844436,122.016648795488)) ;
#32656=CARTESIAN_POINT('Ctrl Pts',(-18.9524743954627,47.1643858040807,122.295687495838)) ;
#32657=CARTESIAN_POINT('Ctrl Pts',(-19.0864023365642,47.3542630833343,121.939374027969)) ;
#32658=CARTESIAN_POINT('Ctrl Pts',(-19.1509626756622,47.1742740029714,122.233865749171)) ;
#32659=CARTESIAN_POINT('Ctrl Pts',(-19.3468297085847,47.3642570219342,121.905591956175)) ;
#32660=CARTESIAN_POINT('Ctrl Pts',(-19.3593042135663,47.1842679415713,122.206837953697)) ;
#32661=CARTESIAN_POINT('Ctrl Pts',(-19.6078094898697,47.374197842971,121.917497147633)) ;
#32662=CARTESIAN_POINT('Ctrl Pts',(-19.568087947677,47.1942087626082,122.216359938901)) ;
#32663=CARTESIAN_POINT('Ctrl Pts',(-19.8632760200849,47.3841572252593,121.974310927408)) ;
#32664=CARTESIAN_POINT('Ctrl Pts',(-19.772461509312,47.2041681448964,122.261808795976)) ;
#32665=CARTESIAN_POINT('Ctrl Pts',(-20.1060266518377,47.3941549849116,122.074874782439)) ;
#32666=CARTESIAN_POINT('Ctrl Pts',(-19.966662791665,47.2141659045487,122.342257824521)) ;
#32667=CARTESIAN_POINT('Ctrl Pts',(-20.3282563986287,47.4041911211139,122.216891398893)) ;
#32668=CARTESIAN_POINT('Ctrl Pts',(-20.1444477453573,47.224202040751,122.455869277174)) ;
#32669=CARTESIAN_POINT('Ctrl Pts',(-20.5190751999569,47.4140419186048,122.391820347718)) ;
#32670=CARTESIAN_POINT('Ctrl Pts',(-20.2971040399441,47.2340528382419,122.595810607946)) ;
#32671=CARTESIAN_POINT('Ctrl Pts',(-20.6789956607079,47.4240027836811,122.599038839022)) ;
#32672=CARTESIAN_POINT('Ctrl Pts',(-20.4250421187195,47.2440137033182,122.76158395382)) ;
#32673=CARTESIAN_POINT('Ctrl Pts',(-20.8010651623618,47.4340316513115,122.832629226849)) ;
#32674=CARTESIAN_POINT('Ctrl Pts',(-20.5226996700031,47.2540425709486,122.948455205887)) ;
#32675=CARTESIAN_POINT('Ctrl Pts',(-20.8798481803655,47.4439418874479,123.080846336945)) ;
#32676=CARTESIAN_POINT('Ctrl Pts',(-20.5857281550626,47.263952807085,123.147028060503)) ;
#32677=CARTESIAN_POINT('Ctrl Pts',(-20.9151022554273,47.4538768407624,123.339542816455)) ;
#32678=CARTESIAN_POINT('Ctrl Pts',(-20.6139336294218,47.2738877603996,123.353984836361)) ;
#32679=CARTESIAN_POINT('Ctrl Pts',(-20.9045535939109,47.463917771172,123.603190649991)) ;
#32680=CARTESIAN_POINT('Ctrl Pts',(-20.605496940888,47.2839286908091,123.564903155438)) ;
#32681=CARTESIAN_POINT('Ctrl Pts',(-20.849402115707,47.4738056679536,123.857124325427)) ;
#32682=CARTESIAN_POINT('Ctrl Pts',(-20.5613779800688,47.2938165875907,123.768050447587)) ;
#32683=CARTESIAN_POINT('Ctrl Pts',(-20.750444918412,47.4837951196123,124.1002641636)) ;
#32684=CARTESIAN_POINT('Ctrl Pts',(-20.4822143310711,47.3038060392494,123.962563117497)) ;
#32685=CARTESIAN_POINT('Ctrl Pts',(-20.6110220669267,47.4937542099777,124.321740017003)) ;
#32686=CARTESIAN_POINT('Ctrl Pts',(-20.3706779971095,47.3137651296148,124.13974493574)) ;
#32687=CARTESIAN_POINT('Ctrl Pts',(-20.4368281965108,47.503651522284,124.514904688104)) ;
#32688=CARTESIAN_POINT('Ctrl Pts',(-20.2313246021344,47.3236624419211,124.294278151825)) ;
#32689=CARTESIAN_POINT('Ctrl Pts',(-20.2283967744204,47.5137079481842,124.677338457595)) ;
#32690=CARTESIAN_POINT('Ctrl Pts',(-20.064580902708,47.3337188678213,124.424226901582)) ;
#32691=CARTESIAN_POINT('Ctrl Pts',(-19.9992773799533,47.523577950774,124.798958001509)) ;
#32692=CARTESIAN_POINT('Ctrl Pts',(-19.8812864635495,47.3435888704111,124.521524526354)) ;
#32693=CARTESIAN_POINT('Ctrl Pts',(-19.7493845402161,47.5335818839512,124.880515352736)) ;
#32694=CARTESIAN_POINT('Ctrl Pts',(-19.6813728797849,47.3535928035883,124.586772510695)) ;
#32695=CARTESIAN_POINT('Ctrl Pts',(-19.4894723640348,47.5435691444151,124.917254732859)) ;
#32696=CARTESIAN_POINT('Ctrl Pts',(-19.4734436940258,47.3635800640522,124.616166289918)) ;
#32697=CARTESIAN_POINT('Ctrl Pts',(-19.2261503135035,47.5535961960008,124.908119289949)) ;
#32698=CARTESIAN_POINT('Ctrl Pts',(-19.2627853251842,47.3736071156379,124.608859963816)) ;
#32699=CARTESIAN_POINT('Ctrl Pts',(-18.9718149570964,47.5634872858269,124.854385043497)) ;
#32700=CARTESIAN_POINT('Ctrl Pts',(-19.0593192486441,47.383498205464,124.565875589659)) ;
#32701=CARTESIAN_POINT('Ctrl Pts',(-18.6475331408761,47.576785040608,124.724300286802)) ;
#32702=CARTESIAN_POINT('Ctrl Pts',(-18.7998792298712,47.3967959602451,124.461806395647)) ;
#32703=CARTESIAN_POINT('Ctrl Pts',(-18.3663382799237,47.5899831002161,124.51451143139)) ;
#32704=CARTESIAN_POINT('Ctrl Pts',(-18.5749054443382,47.4099940198532,124.29395298759)) ;
#32705=CARTESIAN_POINT('Ctrl Pts',(-18.1483991888473,47.6033798407853,124.238054641967)) ;
#32706=CARTESIAN_POINT('Ctrl Pts',(-18.4005844644017,47.4233907604224,124.072822927662)) ;
#32707=CARTESIAN_POINT('Ctrl Pts',(-18.025347143704,47.6132507528587,124.009644853001)) ;
#32708=CARTESIAN_POINT('Ctrl Pts',(-18.3021342785884,47.4332616724959,123.890089214301)) ;
#32709=CARTESIAN_POINT('Ctrl Pts',(-17.9421929511721,47.6233243146269,123.758382877817)) ;
#32710=CARTESIAN_POINT('Ctrl Pts',(-18.2356106624253,47.443335234264,123.689082422527)) ;
#32711=CARTESIAN_POINT('Ctrl Pts',(-17.9045616883877,47.6331457272152,123.502983370987)) ;
#32712=CARTESIAN_POINT('Ctrl Pts',(-18.2055029686415,47.4531566468523,123.484761871704)) ;
#32713=CARTESIAN_POINT('Ctrl Pts',(-17.911781843042,47.6432197444462,123.238412336144)) ;
#32714=CARTESIAN_POINT('Ctrl Pts',(-18.2112771669349,47.4632306640834,123.273106890456)) ;
#32715=CARTESIAN_POINT('Ctrl Pts',(-17.9808569614933,47.6563785314108,122.899509564629)) ;
#32716=CARTESIAN_POINT('Ctrl Pts',(-18.2665340443339,47.4763894510479,123.001975913631)) ;
#32717=CARTESIAN_POINT('Ctrl Pts',(-18.1386436633673,47.669744634505,122.581350825213)) ;
#32718=CARTESIAN_POINT('Ctrl Pts',(-18.3927847615618,47.4897555541421,122.74742093734)) ;
#32719=CARTESIAN_POINT('Ctrl Pts',(-18.370652315842,47.683058569394,122.319320691079)) ;
#32720=CARTESIAN_POINT('Ctrl Pts',(-18.5783616726508,47.5030694890312,122.537834646464)) ;
#32721=CARTESIAN_POINT('Ctrl Pts',(-18.5739282398627,47.6929586088415,122.157012936139)) ;
#32722=CARTESIAN_POINT('Ctrl Pts',(-18.7409870352096,47.5129695284786,122.407978673393)) ;
#32723=CARTESIAN_POINT('Ctrl Pts',(-18.8036181717246,47.702923011976,122.031241515346)) ;
#32724=CARTESIAN_POINT('Ctrl Pts',(-18.9247363827808,47.5229339316132,122.307361838149)) ;
#32725=CARTESIAN_POINT('Ctrl Pts',(-19.0533535758895,47.7129529790972,121.946938831321)) ;
#32726=CARTESIAN_POINT('Ctrl Pts',(-19.1245251698578,47.5329638987343,122.239917409977)) ;
#32727=CARTESIAN_POINT('Ctrl Pts',(-19.3105838879911,47.7228552557062,121.907675661922)) ;
#32728=CARTESIAN_POINT('Ctrl Pts',(-19.3303061564412,47.5428661753434,122.208504383687)) ;
#32729=CARTESIAN_POINT('Ctrl Pts',(-19.6591650885652,47.7361211848754,121.914819682812)) ;
#32730=CARTESIAN_POINT('Ctrl Pts',(-19.609187461542,47.5561321045125,122.214219997551)) ;
#32731=CARTESIAN_POINT('Ctrl Pts',(-20.0833550247634,47.7527427159818,122.037930509702)) ;
#32732=CARTESIAN_POINT('Ctrl Pts',(-19.9485240134624,47.5727536356189,122.312705495618)) ;
#32733=CARTESIAN_POINT('Ctrl Pts',(-20.510453729545,47.7726175446265,122.348898697034)) ;
#32734=CARTESIAN_POINT('Ctrl Pts',(-20.2902038142842,47.5926284642636,122.561462978366)) ;
#32735=CARTESIAN_POINT('Ctrl Pts',(-20.7582479358267,47.7892907527283,122.71623189636)) ;
#32736=CARTESIAN_POINT('Ctrl Pts',(-20.4884640703777,47.6093016723655,122.855376229388)) ;
#32737=CARTESIAN_POINT('Ctrl Pts',(-20.8714295868913,47.8025418777096,123.04557591284)) ;
#32738=CARTESIAN_POINT('Ctrl Pts',(-20.5789911114765,47.6225527973467,123.118807090608)) ;
#32739=CARTESIAN_POINT('Ctrl Pts',(-20.9269298434521,47.8157841965304,123.389178316211)) ;
#32740=CARTESIAN_POINT('Ctrl Pts',(-20.6233964746189,47.6357951161676,123.393706836067)) ;
#32741=CARTESIAN_POINT('Ctrl Pts',(-20.881145520325,47.8325174368699,123.831476120658)) ;
#32742=CARTESIAN_POINT('Ctrl Pts',(-20.5867718080052,47.652528356507,123.747531615695)) ;
#32743=CARTESIAN_POINT('Ctrl Pts',(-20.6511822086368,47.8523465850579,124.305796219641)) ;
#32744=CARTESIAN_POINT('Ctrl Pts',(-20.4028036328943,47.672357504695,124.126994379831)) ;
#32745=CARTESIAN_POINT('Ctrl Pts',(-20.2723934902227,47.8722712801585,124.675711001554)) ;
#32746=CARTESIAN_POINT('Ctrl Pts',(-20.0997742015209,47.6922821997956,124.422927479501)) ;
#32747=CARTESIAN_POINT('Ctrl Pts',(-19.7899432576281,47.8921945087419,124.89417687357)) ;
#32748=CARTESIAN_POINT('Ctrl Pts',(-19.7138146109579,47.7122054283791,124.597703165401)) ;
#32749=CARTESIAN_POINT('Ctrl Pts',(-19.2619554888101,47.912121647868,124.935052545408)) ;
#32750=CARTESIAN_POINT('Ctrl Pts',(-19.2914239665457,47.7321325675052,124.630406187641)) ;
#32751=CARTESIAN_POINT('Ctrl Pts',(-18.7527354696576,47.9319981104837,124.794293876189)) ;
#32752=CARTESIAN_POINT('Ctrl Pts',(-18.8840463051201,47.7520090301208,124.51780103702)) ;
#32753=CARTESIAN_POINT('Ctrl Pts',(-18.3198015893089,47.951975339089,124.486914551041)) ;
#32754=CARTESIAN_POINT('Ctrl Pts',(-18.5376979391742,47.7719862587261,124.271898997653)) ;
#32755=CARTESIAN_POINT('Ctrl Pts',(-18.0187050938315,47.9719101970627,124.050892286809)) ;
#32756=CARTESIAN_POINT('Ctrl Pts',(-18.2968188352507,47.7919211166998,123.923081749406)) ;
#32757=CARTESIAN_POINT('Ctrl Pts',(-17.8842318765923,47.9918066459935,123.539502996666)) ;
#32758=CARTESIAN_POINT('Ctrl Pts',(-18.1892385060343,47.8118175656306,123.51396964369)) ;
#32759=CARTESIAN_POINT('Ctrl Pts',(-17.9318165298211,48.0117279300601,123.012148120241)) ;
#32760=CARTESIAN_POINT('Ctrl Pts',(-18.227305199235,47.8317388496972,123.092084787911)) ;
#32761=CARTESIAN_POINT('Ctrl Pts',(-18.1570558911766,48.0316845797311,122.53190203543)) ;
#32762=CARTESIAN_POINT('Ctrl Pts',(-18.4074959798686,47.8516954993682,122.7078870895)) ;
#32763=CARTESIAN_POINT('Ctrl Pts',(-18.5309774065162,48.0515618728427,122.158784664484)) ;
#32764=CARTESIAN_POINT('Ctrl Pts',(-18.7066337296029,47.8715727924798,122.409391583344)) ;
#32765=CARTESIAN_POINT('Ctrl Pts',(-19.0095199143223,48.0714483450711,121.934235959805)) ;
#32766=CARTESIAN_POINT('Ctrl Pts',(-19.0894691453368,47.8914592647082,122.229752104761)) ;
#32767=CARTESIAN_POINT('Ctrl Pts',(-19.540633493891,48.0915099109951,121.886851609452)) ;
#32768=CARTESIAN_POINT('Ctrl Pts',(-19.5143591422602,47.9115208306322,122.191844655207)) ;
#32769=CARTESIAN_POINT('Ctrl Pts',(-20.0501821768271,48.1113503185359,122.022521216227)) ;
#32770=CARTESIAN_POINT('Ctrl Pts',(-19.9220001526352,47.931361238173,122.300380806211)) ;
#32771=CARTESIAN_POINT('Ctrl Pts',(-20.4843799802069,48.1312016425088,122.322303458234)) ;
#32772=CARTESIAN_POINT('Ctrl Pts',(-20.2693591621974,47.9512125621459,122.540208559723)) ;
#32773=CARTESIAN_POINT('Ctrl Pts',(-20.7926161664346,48.1512549124602,122.757030819445)) ;
#32774=CARTESIAN_POINT('Ctrl Pts',(-20.5159469547042,47.9712658320974,122.887990515959)) ;
#32775=CARTESIAN_POINT('Ctrl Pts',(-20.93252583496,48.1710755698436,123.265061844735)) ;
#32776=CARTESIAN_POINT('Ctrl Pts',(-20.627874051427,47.9910864894807,123.294417505765)) ;
#32777=CARTESIAN_POINT('Ctrl Pts',(-20.8912365983079,48.1910469911741,123.794086280571)) ;
#32778=CARTESIAN_POINT('Ctrl Pts',(-20.5948408958009,48.0110579108112,123.717637230084)) ;
#32779=CARTESIAN_POINT('Ctrl Pts',(-20.6727225902505,48.2109404835378,124.275764014104)) ;
#32780=CARTESIAN_POINT('Ctrl Pts',(-20.4200275548019,48.0309514031749,124.102979505904)) ;
#32781=CARTESIAN_POINT('Ctrl Pts',(-20.3004819424767,48.2309645697788,124.655976968053)) ;
#32782=CARTESIAN_POINT('Ctrl Pts',(-20.1222337727236,48.050975489416,124.407148369197)) ;
#32783=CARTESIAN_POINT('Ctrl Pts',(-19.8260643109497,48.2507694488917,124.884148701362)) ;
#32784=CARTESIAN_POINT('Ctrl Pts',(-19.7426971430051,48.0707803685288,124.589684526452)) ;
#32785=CARTESIAN_POINT('Ctrl Pts',(-19.298401689414,48.2707284645896,124.938563164576)) ;
#32786=CARTESIAN_POINT('Ctrl Pts',(-19.3205664831375,48.0907393842267,124.633213331361)) ;
#32787=CARTESIAN_POINT('Ctrl Pts',(-18.7834401752579,48.2907144882186,124.808270536172)) ;
#32788=CARTESIAN_POINT('Ctrl Pts',(-18.9085977754014,48.1107254078558,124.528976723537)) ;
#32789=CARTESIAN_POINT('Ctrl Pts',(-18.3471324483424,48.3105229839791,124.513544556307)) ;
#32790=CARTESIAN_POINT('Ctrl Pts',(-18.5595521151312,48.1305339036163,124.29319269375)) ;
#32791=CARTESIAN_POINT('Ctrl Pts',(-18.0344280932835,48.3305056230847,124.084394876722)) ;
#32792=CARTESIAN_POINT('Ctrl Pts',(-18.3093912303342,48.1505165427219,123.949870956698)) ;
#32793=CARTESIAN_POINT('Ctrl Pts',(-17.8877491679608,48.3503870708787,123.576606049549)) ;
#32794=CARTESIAN_POINT('Ctrl Pts',(-18.1920510956395,48.1703979905159,123.543638317555)) ;
#32795=CARTESIAN_POINT('Ctrl Pts',(-17.9228534217252,48.3703435376163,123.047472668677)) ;
#32796=CARTESIAN_POINT('Ctrl Pts',(-18.2201380308155,48.1903544572534,123.120331605847)) ;
#32797=CARTESIAN_POINT('Ctrl Pts',(-18.1353200268485,48.3902209345718,122.563676201082)) ;
#32798=CARTESIAN_POINT('Ctrl Pts',(-18.3901149639764,48.210231854209,122.733295384716)) ;
#32799=CARTESIAN_POINT('Ctrl Pts',(-18.5017348375152,48.4102028807471,122.179310317759)) ;
#32800=CARTESIAN_POINT('Ctrl Pts',(-18.6832494823206,48.2302138003843,122.425805199473)) ;
#32801=CARTESIAN_POINT('Ctrl Pts',(-18.9763255338847,48.4301319797839,121.943845821942)) ;
#32802=CARTESIAN_POINT('Ctrl Pts',(-19.0629244628759,48.250142899421,122.237437292873)) ;
#32803=CARTESIAN_POINT('Ctrl Pts',(-19.5025485758174,48.4500606029965,121.8844085627)) ;
#32804=CARTESIAN_POINT('Ctrl Pts',(-19.4839018350502,48.2700715226336,122.189890020095)) ;
#32805=CARTESIAN_POINT('Ctrl Pts',(-20.0154041734413,48.4698949271029,122.006602474331)) ;
#32806=CARTESIAN_POINT('Ctrl Pts',(-19.8941925598735,48.28990584674,122.287654399379)) ;
#32807=CARTESIAN_POINT('Ctrl Pts',(-20.3852740340378,48.4865472144863,122.249514009236)) ;
#32808=CARTESIAN_POINT('Ctrl Pts',(-20.1900656488884,48.3065581341234,122.481970779686)) ;
#32809=CARTESIAN_POINT('Ctrl Pts',(-20.6170557319961,48.4998077155085,122.509808729621)) ;
#32810=CARTESIAN_POINT('Ctrl Pts',(-20.3755074720273,48.3198186351457,122.690222602484)) ;
#32811=CARTESIAN_POINT('Ctrl Pts',(-20.7555225669231,48.5098091927098,122.73319887295)) ;
#32812=CARTESIAN_POINT('Ctrl Pts',(-20.4862754159992,48.3298201123469,122.868932815288)) ;
#32813=CARTESIAN_POINT('Ctrl Pts',(-20.8529891978789,48.5198412135693,122.978158629166)) ;
#32814=CARTESIAN_POINT('Ctrl Pts',(-20.5642475521182,48.3398521332064,123.064902698722)) ;
#32815=CARTESIAN_POINT('Ctrl Pts',(-20.9058519382839,48.5297047572949,123.231906669117)) ;
#32816=CARTESIAN_POINT('Ctrl Pts',(-20.6065360580068,48.349715676932,123.267899228391)) ;
#32817=CARTESIAN_POINT('Ctrl Pts',(-20.9146324101858,48.539673470965,123.493731289981)) ;
#32818=CARTESIAN_POINT('Ctrl Pts',(-20.613556026208,48.3596843906021,123.477368180223)) ;
#32819=CARTESIAN_POINT('Ctrl Pts',(-20.8648547231583,48.5530192183687,123.840870176946)) ;
#32820=CARTESIAN_POINT('Ctrl Pts',(-20.5737423451447,48.3730301380058,123.755033409764)) ;
#32821=CARTESIAN_POINT('Ctrl Pts',(-20.7281894338226,48.5661697734414,124.16259745941)) ;
#32822=CARTESIAN_POINT('Ctrl Pts',(-20.4644056241511,48.3861806930785,124.012444016206)) ;
#32823=CARTESIAN_POINT('Ctrl Pts',(-20.5118249048892,48.5795551539912,124.439903596676)) ;
#32824=CARTESIAN_POINT('Ctrl Pts',(-20.2913023607941,48.3995660736284,124.234297052958)) ;
#32825=CARTESIAN_POINT('Ctrl Pts',(-20.3188115906214,48.5894430899841,124.613917552832)) ;
#32826=CARTESIAN_POINT('Ctrl Pts',(-20.1368920377986,48.4094540096212,124.373504600187)) ;
#32827=CARTESIAN_POINT('Ctrl Pts',(-20.0965059871697,48.5994342797967,124.753554193822)) ;
#32828=CARTESIAN_POINT('Ctrl Pts',(-19.9590458940921,48.4194451994339,124.485212524752)) ;
#32829=CARTESIAN_POINT('Ctrl Pts',(-19.8542566549361,48.609386378335,124.852215716831)) ;
#32830=CARTESIAN_POINT('Ctrl Pts',(-19.7652457303651,48.4293972979721,124.5641395104)) ;
#32831=CARTESIAN_POINT('Ctrl Pts',(-19.5961577410576,48.6194326347855,124.907656726796)) ;
#32832=CARTESIAN_POINT('Ctrl Pts',(-19.5587661686804,48.4394435544226,124.608490145194)) ;
#32833=CARTESIAN_POINT('Ctrl Pts',(-19.337504837007,48.6292820821796,124.917439257159)) ;
#32834=CARTESIAN_POINT('Ctrl Pts',(-19.3518437348216,48.4492930018168,124.616313910644)) ;
#32835=CARTESIAN_POINT('Ctrl Pts',(-19.078037022272,48.6392447346748,124.882575057759)) ;
#32836=CARTESIAN_POINT('Ctrl Pts',(-19.1442698490704,48.4592556543119,124.588420320008)) ;
#32837=CARTESIAN_POINT('Ctrl Pts',(-18.8271502999389,48.6492678203169,124.802367820736)) ;
#32838=CARTESIAN_POINT('Ctrl Pts',(-18.9435612086211,48.469278739954,124.524252395797)) ;
#32839=CARTESIAN_POINT('Ctrl Pts',(-18.5961153422512,48.6591929360738,124.681264951306)) ;
#32840=CARTESIAN_POINT('Ctrl Pts',(-18.7587343441336,48.479203855711,124.427368128863)) ;
#32841=CARTESIAN_POINT('Ctrl Pts',(-18.3870750955819,48.6692454144736,124.519790373217)) ;
#32842=CARTESIAN_POINT('Ctrl Pts',(-18.5915035653785,48.4892563341108,124.298186706336)) ;
#32843=CARTESIAN_POINT('Ctrl Pts',(-18.2126444694148,48.6790969131764,124.328462267053)) ;
#32844=CARTESIAN_POINT('Ctrl Pts',(-18.4519607973613,48.4991078328135,124.14512276976)) ;
#32845=CARTESIAN_POINT('Ctrl Pts',(-18.0718445075732,48.6890686523789,124.107495060904)) ;
#32846=CARTESIAN_POINT('Ctrl Pts',(-18.339322775097,48.509079572016,123.968347874547)) ;
#32847=CARTESIAN_POINT('Ctrl Pts',(-17.9713155069276,48.6990638601446,123.86478462589)) ;
#32848=CARTESIAN_POINT('Ctrl Pts',(-18.2589016723393,48.5190747797817,123.774178726449)) ;
#32849=CARTESIAN_POINT('Ctrl Pts',(-17.9145635742469,48.7090978616136,123.607305099869)) ;
#32850=CARTESIAN_POINT('Ctrl Pts',(-18.213502337176,48.5291087812508,123.568194649321)) ;
#32851=CARTESIAN_POINT('Ctrl Pts',(-17.9031654069168,48.718953219706,123.348541528174)) ;
#32852=CARTESIAN_POINT('Ctrl Pts',(-18.2043860513762,48.5389641393431,123.361183881843)) ;
#32853=CARTESIAN_POINT('Ctrl Pts',(-17.937003026666,48.7289526952993,123.088000944887)) ;
#32854=CARTESIAN_POINT('Ctrl Pts',(-18.231458353244,48.5489636149364,123.152751774568)) ;
#32855=CARTESIAN_POINT('Ctrl Pts',(-18.0144858731634,48.7388471437944,122.839746756377)) ;
#32856=CARTESIAN_POINT('Ctrl Pts',(-18.29344667902,48.5588580634315,122.954149283923)) ;
#32857=CARTESIAN_POINT('Ctrl Pts',(-18.1359580112243,48.7489102680221,122.604899456879)) ;
#32858=CARTESIAN_POINT('Ctrl Pts',(-18.3906263763058,48.5689211876593,122.766272439426)) ;
#32859=CARTESIAN_POINT('Ctrl Pts',(-18.2926260056632,48.7587498943507,122.399136493447)) ;
#32860=CARTESIAN_POINT('Ctrl Pts',(-18.5159623218924,48.5787608139879,122.601663664949)) ;
#32861=CARTESIAN_POINT('Ctrl Pts',(-18.4866726839865,48.7688131293937,122.219522458127)) ;
#32862=CARTESIAN_POINT('Ctrl Pts',(-18.6712011734618,48.5888240490308,122.457974012859)) ;
#32863=CARTESIAN_POINT('Ctrl Pts',(-18.7053931823134,48.7787071346277,122.078888414331)) ;
#32864=CARTESIAN_POINT('Ctrl Pts',(-18.8461785372344,48.5987180542649,122.345468767959)) ;
#32865=CARTESIAN_POINT('Ctrl Pts',(-18.9460602718396,48.7886498478435,121.977234200229)) ;
#32866=CARTESIAN_POINT('Ctrl Pts',(-19.038712845065,48.6086607674806,122.264147453385)) ;
#32867=CARTESIAN_POINT('Ctrl Pts',(-19.2023805082056,48.7986555876417,121.918479266341)) ;
#32868=CARTESIAN_POINT('Ctrl Pts',(-19.2437694535632,48.6186665072788,122.217145598752)) ;
#32869=CARTESIAN_POINT('Ctrl Pts',(-19.4653884139487,48.8086764897881,121.905400360003)) ;
#32870=CARTESIAN_POINT('Ctrl Pts',(-19.4541758671944,48.6286874094252,122.206684634383)) ;
#32871=CARTESIAN_POINT('Ctrl Pts',(-19.7233301714243,48.818567259837,121.937466358609)) ;
#32872=CARTESIAN_POINT('Ctrl Pts',(-19.660528678975,48.6385781794741,122.232339509988)) ;
#32873=CARTESIAN_POINT('Ctrl Pts',(-19.9744129235702,48.8285586706167,122.014229612701)) ;
#32874=CARTESIAN_POINT('Ctrl Pts',(-19.8613941678022,48.6485695902538,122.29375209031)) ;
#32875=CARTESIAN_POINT('Ctrl Pts',(-20.2073088426993,48.8385070162812,122.13298779378)) ;
#32876=CARTESIAN_POINT('Ctrl Pts',(-20.0477097505346,48.6585179359183,122.388760413796)) ;
#32877=CARTESIAN_POINT('Ctrl Pts',(-20.4163278633967,48.8484518743424,122.289901832939)) ;
#32878=CARTESIAN_POINT('Ctrl Pts',(-20.2149235466463,48.6684627939795,122.514293137704)) ;
#32879=CARTESIAN_POINT('Ctrl Pts',(-20.5965846062851,48.8585067097353,122.483065165235)) ;
#32880=CARTESIAN_POINT('Ctrl Pts',(-20.3591274717753,48.6785176293724,122.66882529591)) ;
#32881=CARTESIAN_POINT('Ctrl Pts',(-20.7376368968491,48.8683290818368,122.699266149593)) ;
#32882=CARTESIAN_POINT('Ctrl Pts',(-20.4719672538664,48.6883400014739,122.841786671009)) ;
#32883=CARTESIAN_POINT('Ctrl Pts',(-20.8418372689003,48.8783849492805,122.942091527948)) ;
#32884=CARTESIAN_POINT('Ctrl Pts',(-20.555325764693,48.6983958689176,123.036047837099)) ;
#32885=CARTESIAN_POINT('Ctrl Pts',(-20.9011534756052,48.8883256791384,123.196510502706)) ;
#32886=CARTESIAN_POINT('Ctrl Pts',(-20.6027766814318,48.7083365987755,123.239583219455)) ;
#32887=CARTESIAN_POINT('Ctrl Pts',(-20.9161549876618,48.8982300176895,123.456358415646)) ;
#32888=CARTESIAN_POINT('Ctrl Pts',(-20.6147759351108,48.7182409373267,123.447461235112)) ;
#32889=CARTESIAN_POINT('Ctrl Pts',(-20.8852105592629,48.908276699118,123.718532273713)) ;
#32890=CARTESIAN_POINT('Ctrl Pts',(-20.5900184387417,48.7282876187551,123.657200174612)) ;
#32891=CARTESIAN_POINT('Ctrl Pts',(-20.810567540589,48.9181722065873,123.967677397249)) ;
#32892=CARTESIAN_POINT('Ctrl Pts',(-20.530302315986,48.7381831262244,123.856515274534)) ;
#32893=CARTESIAN_POINT('Ctrl Pts',(-20.6918640066937,48.9282344750859,124.203918318717)) ;
#32894=CARTESIAN_POINT('Ctrl Pts',(-20.4353377019454,48.748245394723,124.045507277748)) ;
#32895=CARTESIAN_POINT('Ctrl Pts',(-20.5374874732684,48.9380764653565,124.4114706526)) ;
#32896=CARTESIAN_POINT('Ctrl Pts',(-20.3118353640093,48.7580873849936,124.211547452761)) ;
#32897=CARTESIAN_POINT('Ctrl Pts',(-20.346982966348,48.9480698822375,124.59217583248)) ;
#32898=CARTESIAN_POINT('Ctrl Pts',(-20.1594306094742,48.7680808018746,124.356110185967)) ;
#32899=CARTESIAN_POINT('Ctrl Pts',(-20.1294622771985,48.9579943700896,124.736115686117)) ;
#32900=CARTESIAN_POINT('Ctrl Pts',(-19.9854133980772,48.7780052897268,124.471260339818)) ;
#32901=CARTESIAN_POINT('Ctrl Pts',(-19.8885974147487,48.9679940039981,124.841121711921)) ;
#32902=CARTESIAN_POINT('Ctrl Pts',(-19.7927208876813,48.7880049236352,124.555263504968)) ;
#32903=CARTESIAN_POINT('Ctrl Pts',(-19.6334469697658,48.9779801142549,124.9026502756)) ;
#32904=CARTESIAN_POINT('Ctrl Pts',(-19.5886002554755,48.797991033892,124.604484611095)) ;
#32905=CARTESIAN_POINT('Ctrl Pts',(-19.3702291570135,48.988016065442,124.918743054803)) ;
#32906=CARTESIAN_POINT('Ctrl Pts',(-19.3780258273931,48.8080269850791,124.617357030523)) ;
#32907=CARTESIAN_POINT('Ctrl Pts',(-19.1128025382839,48.9978727037768,124.889803469788)) ;
#32908=CARTESIAN_POINT('Ctrl Pts',(-19.1720854580198,48.8178836234139,124.594203711341)) ;
#32909=CARTESIAN_POINT('Ctrl Pts',(-18.8606911455665,49.0078716638548,124.815911669425)) ;
#32910=CARTESIAN_POINT('Ctrl Pts',(-18.9703969207896,48.8278825834919,124.535088685264)) ;
#32911=CARTESIAN_POINT('Ctrl Pts',(-18.6274774420179,49.0177668941686,124.700789980476)) ;
#32912=CARTESIAN_POINT('Ctrl Pts',(-18.7838272068471,48.8377778138057,124.442990132716)) ;
#32913=CARTESIAN_POINT('Ctrl Pts',(-18.4143731818113,49.0278274066372,124.544376734575)) ;
#32914=CARTESIAN_POINT('Ctrl Pts',(-18.6133446125383,48.8478383262744,124.317858101007)) ;
#32915=CARTESIAN_POINT('Ctrl Pts',(-18.2353571530203,49.0376766981834,124.357410469631)) ;
#32916=CARTESIAN_POINT('Ctrl Pts',(-18.4701335294732,48.8576876178205,124.168284578467)) ;
#32917=CARTESIAN_POINT('Ctrl Pts',(-18.0883869155088,49.0477038841156,124.13870846236)) ;
#32918=CARTESIAN_POINT('Ctrl Pts',(-18.3525585546623,48.8677148037527,123.993322118891)) ;
#32919=CARTESIAN_POINT('Ctrl Pts',(-17.9822338382996,49.0577324205749,123.89747926818)) ;
#32920=CARTESIAN_POINT('Ctrl Pts',(-18.2676375508408,48.8777433402121,123.800338060987)) ;
#32921=CARTESIAN_POINT('Ctrl Pts',(-17.9202532459207,49.0675776605399,123.646304603655)) ;
#32922=CARTESIAN_POINT('Ctrl Pts',(-18.2180547698184,48.887588580177,123.599398834632)) ;
#32923=CARTESIAN_POINT('Ctrl Pts',(-17.9018658552473,49.0775683554631,123.384397836007)) ;
#32924=CARTESIAN_POINT('Ctrl Pts',(-18.2033462475352,48.8975792751002,123.389873479783)) ;
#32925=CARTESIAN_POINT('Ctrl Pts',(-17.9299430170255,49.0876061762217,123.122114050778)) ;
#32926=CARTESIAN_POINT('Ctrl Pts',(-18.2258094796159,48.9076170958588,123.180046505559)) ;
#32927=CARTESIAN_POINT('Ctrl Pts',(-18.0013047262961,49.0974507699987,122.873439403411)) ;
#32928=CARTESIAN_POINT('Ctrl Pts',(-18.2828999451431,48.9174616896358,122.981108076686)) ;
#32929=CARTESIAN_POINT('Ctrl Pts',(-18.1158511804771,49.1074347653747,122.637421711162)) ;
#32930=CARTESIAN_POINT('Ctrl Pts',(-18.3745381797035,48.9274456850118,122.792294678741)) ;
#32931=CARTESIAN_POINT('Ctrl Pts',(-18.2691440175312,49.1173838139361,122.425609469171)) ;
#32932=CARTESIAN_POINT('Ctrl Pts',(-18.4971732750292,48.9373947335732,122.622845958059)) ;
#32933=CARTESIAN_POINT('Ctrl Pts',(-18.4576938725769,49.1273862529106,122.242453382412)) ;
#32934=CARTESIAN_POINT('Ctrl Pts',(-18.6480139645982,48.9473971725478,122.476322036241)) ;
#32935=CARTESIAN_POINT('Ctrl Pts',(-18.6757844901155,49.137407494207,122.094840814009)) ;
#32936=CARTESIAN_POINT('Ctrl Pts',(-18.8224872183678,48.9574184138441,122.358233056651)) ;
#32937=CARTESIAN_POINT('Ctrl Pts',(-18.912980073684,49.1473001726465,121.988431832938)) ;
#32938=CARTESIAN_POINT('Ctrl Pts',(-19.0122435443815,48.9673110922836,122.273107306657)) ;
#32939=CARTESIAN_POINT('Ctrl Pts',(-19.1674232251513,49.1572902265941,121.923790931797)) ;
#32940=CARTESIAN_POINT('Ctrl Pts',(-19.2157981795932,48.9773011462313,122.221395753359)) ;
#32941=CARTESIAN_POINT('Ctrl Pts',(-19.4284019621495,49.1672485877426,121.904559887262)) ;
#32942=CARTESIAN_POINT('Ctrl Pts',(-19.4245809128314,48.9872595073797,122.206012139739)) ;
#32943=CARTESIAN_POINT('Ctrl Pts',(-19.6873094646854,49.1771482146274,121.930145178779)) ;
#32944=CARTESIAN_POINT('Ctrl Pts',(-19.6317061102632,48.9971591342646,122.226481354379)) ;
#32945=CARTESIAN_POINT('Ctrl Pts',(-19.941526102593,49.1871961114308,122.001425268329)) ;
#32946=CARTESIAN_POINT('Ctrl Pts',(-19.8350792979722,49.0072070310679,122.283506510641)) ;
#32947=CARTESIAN_POINT('Ctrl Pts',(-20.1760417540059,49.1970914690668,122.113872563223)) ;
#32948=CARTESIAN_POINT('Ctrl Pts',(-20.022690714718,49.0171023887039,122.373464959482)) ;
#32949=CARTESIAN_POINT('Ctrl Pts',(-20.3909878097268,49.2071531215235,122.267804384145)) ;
#32950=CARTESIAN_POINT('Ctrl Pts',(-20.1946471758079,49.0271640411606,122.496611400077)) ;
#32951=CARTESIAN_POINT('Ctrl Pts',(-20.5720068053571,49.2169977257954,122.452644101985)) ;
#32952=CARTESIAN_POINT('Ctrl Pts',(-20.3394609075565,49.0370086454325,122.644483128646)) ;
#32953=CARTESIAN_POINT('Ctrl Pts',(-20.7206623097227,49.2269578474934,122.668068984939)) ;
#32954=CARTESIAN_POINT('Ctrl Pts',(-20.4583844503407,49.0469687671305,122.816823184735)) ;
#32955=CARTESIAN_POINT('Ctrl Pts',(-20.8300406886576,49.2369958818559,122.90810181371)) ;
#32956=CARTESIAN_POINT('Ctrl Pts',(-20.5458863746886,49.0570068014931,123.008849944546)) ;
#32957=CARTESIAN_POINT('Ctrl Pts',(-20.895474107219,49.2468701944424,123.15923667191)) ;
#32958=CARTESIAN_POINT('Ctrl Pts',(-20.5982321097899,49.0668811140795,123.209757165169)) ;
#32959=CARTESIAN_POINT('Ctrl Pts',(-20.9167021696326,49.2569396752251,123.422962968094)) ;
#32960=CARTESIAN_POINT('Ctrl Pts',(-20.6152137829838,49.0769505948622,123.420738590608)) ;
#32961=CARTESIAN_POINT('Ctrl Pts',(-20.8925309748415,49.2667740112422,123.680288852952)) ;
#32962=CARTESIAN_POINT('Ctrl Pts',(-20.5958761715019,49.0867849308793,123.626598057855)) ;
#32963=CARTESIAN_POINT('Ctrl Pts',(-20.8233682239885,49.2768069689704,123.934702843844)) ;
#32964=CARTESIAN_POINT('Ctrl Pts',(-20.5405453724813,49.0968178886076,123.830129187291)) ;
#32965=CARTESIAN_POINT('Ctrl Pts',(-20.7105597644519,49.2868273675456,124.172644633411)) ;
#32966=CARTESIAN_POINT('Ctrl Pts',(-20.4502978908563,49.1068382871827,124.020482314942)) ;
#32967=CARTESIAN_POINT('Ctrl Pts',(-20.5610300420917,49.2966929413168,124.38445939655)) ;
#32968=CARTESIAN_POINT('Ctrl Pts',(-20.3306741735145,49.116703860954,124.189932981708)) ;
#32969=CARTESIAN_POINT('Ctrl Pts',(-20.3732384290242,49.3067618159729,124.570826297004)) ;
#32970=CARTESIAN_POINT('Ctrl Pts',(-20.1804402169388,49.12677273561,124.33902629884)) ;
#32971=CARTESIAN_POINT('Ctrl Pts',(-20.1607506292362,49.3166072468784,124.718462326025)) ;
#32972=CARTESIAN_POINT('Ctrl Pts',(-20.0104505595802,49.1366181665155,124.457133981811)) ;
#32973=CARTESIAN_POINT('Ctrl Pts',(-19.9230300882037,49.3265868717491,124.829197136237)) ;
#32974=CARTESIAN_POINT('Ctrl Pts',(-19.820274187598,49.1465977913862,124.545721370372)) ;
#32975=CARTESIAN_POINT('Ctrl Pts',(-19.6685730451368,49.3366055546632,124.896756529863)) ;
#32976=CARTESIAN_POINT('Ctrl Pts',(-19.6167084117739,49.1566164743003,124.599768387045)) ;
#32977=CARTESIAN_POINT('Ctrl Pts',(-19.4098038796016,49.346488819847,124.919356964503)) ;
#32978=CARTESIAN_POINT('Ctrl Pts',(-19.4096939213468,49.1664997394842,124.617848281741)) ;
#32979=CARTESIAN_POINT('Ctrl Pts',(-19.1462832607712,49.3565571139384,124.89615090551)) ;
#32980=CARTESIAN_POINT('Ctrl Pts',(-19.1988771347697,49.1765680335755,124.599282999011)) ;
#32981=CARTESIAN_POINT('Ctrl Pts',(-18.8966752356581,49.3663872441237,124.829435060277)) ;
#32982=CARTESIAN_POINT('Ctrl Pts',(-18.999191990857,49.1863981637609,124.545910321874)) ;
#32983=CARTESIAN_POINT('Ctrl Pts',(-18.656744831752,49.3764537923389,124.718117896912)) ;
#32984=CARTESIAN_POINT('Ctrl Pts',(-18.8072474823496,49.196464711976,124.456856234754)) ;
#32985=CARTESIAN_POINT('Ctrl Pts',(-18.4436181844938,49.3863440410275,124.569306863408)) ;
#32986=CARTESIAN_POINT('Ctrl Pts',(-18.6367470167291,49.2063549606646,124.337807652728)) ;
#32987=CARTESIAN_POINT('Ctrl Pts',(-18.2572992166369,49.3963362228035,124.384299698902)) ;
#32988=CARTESIAN_POINT('Ctrl Pts',(-18.4876920638657,49.2163471424406,124.189801941018)) ;
#32989=CARTESIAN_POINT('Ctrl Pts',(-18.1065741069592,49.4062990034313,124.170232758712)) ;
#32990=CARTESIAN_POINT('Ctrl Pts',(-18.3671123543255,49.2263099230684,124.018548569717)) ;
#32991=CARTESIAN_POINT('Ctrl Pts',(-17.9953598077173,49.4162034081051,123.934891647468)) ;
#32992=CARTESIAN_POINT('Ctrl Pts',(-18.2781412702089,49.2362143277422,123.830276340777)) ;
#32993=CARTESIAN_POINT('Ctrl Pts',(-17.9258209627765,49.4262634025841,123.679859999836)) ;
#32994=CARTESIAN_POINT('Ctrl Pts',(-18.2225102077793,49.2462743222212,123.626250739129)) ;
#32995=CARTESIAN_POINT('Ctrl Pts',(-17.9019035489539,49.4361120245539,123.422136143483)) ;
#32996=CARTESIAN_POINT('Ctrl Pts',(-18.2033764111946,49.256122944191,123.42007277146)) ;
#32997=CARTESIAN_POINT('Ctrl Pts',(-17.9228967151139,49.4461424639657,123.159399391363)) ;
#32998=CARTESIAN_POINT('Ctrl Pts',(-18.2201708355214,49.2661533836029,123.209883266575)) ;
#32999=CARTESIAN_POINT('Ctrl Pts',(-17.9895783325629,49.4561521796005,122.90491683128)) ;
#33000=CARTESIAN_POINT('Ctrl Pts',(-18.2735161375883,49.2761630992376,123.006297255522)) ;
#33001=CARTESIAN_POINT('Ctrl Pts',(-18.0980952655541,49.4660629322931,122.668183285469)) ;
#33002=CARTESIAN_POINT('Ctrl Pts',(-18.3603293441848,49.2860738519302,122.816911054056)) ;
#33003=CARTESIAN_POINT('Ctrl Pts',(-18.245826326081,49.4759922052395,122.453085432562)) ;
#33004=CARTESIAN_POINT('Ctrl Pts',(-18.4785136798849,49.2960031248766,122.644833143533)) ;
#33005=CARTESIAN_POINT('Ctrl Pts',(-18.4308927790873,49.4860348966322,122.264952869192)) ;
#33006=CARTESIAN_POINT('Ctrl Pts',(-18.6265668504671,49.3060458162693,122.494326860631)) ;
#33007=CARTESIAN_POINT('Ctrl Pts',(-18.6423948660931,49.4959214298497,122.114039679069)) ;
#33008=CARTESIAN_POINT('Ctrl Pts',(-18.7957676964125,49.3159323494868,122.373596652419)) ;
#33009=CARTESIAN_POINT('Ctrl Pts',(-18.8791977037883,49.5059145747817,122.000547015104)) ;
#33010=CARTESIAN_POINT('Ctrl Pts',(-18.9852096849577,49.3259254944189,122.282802310595)) ;
#33011=CARTESIAN_POINT('Ctrl Pts',(-19.1309496466814,49.5158602556182,121.930322869947)) ;
#33012=CARTESIAN_POINT('Ctrl Pts',(-19.1866107041673,49.3358711752553,122.226622847818)) ;
#33013=CARTESIAN_POINT('Ctrl Pts',(-19.3910719340289,49.5258075127667,121.904340399635)) ;
#33014=CARTESIAN_POINT('Ctrl Pts',(-19.3947080350026,49.3458184324039,122.205836499033)) ;
#33015=CARTESIAN_POINT('Ctrl Pts',(-19.6543477211243,49.5358554166387,121.924410607122)) ;
#33016=CARTESIAN_POINT('Ctrl Pts',(-19.605328890607,49.3558663362759,122.221892336368)) ;
#33017=CARTESIAN_POINT('Ctrl Pts',(-19.9051063909627,49.5457031157367,121.988376325681)) ;
#33018=CARTESIAN_POINT('Ctrl Pts',(-19.8059348407056,49.3657140353738,122.273064246999)) ;
#33019=CARTESIAN_POINT('Ctrl Pts',(-20.1440032593785,49.5556646067154,122.095383178499)) ;
#33020=CARTESIAN_POINT('Ctrl Pts',(-19.9970522508123,49.3756755263525,122.358669026334)) ;
#33021=CARTESIAN_POINT('Ctrl Pts',(-20.3619888762732,49.5656940691293,122.243550726972)) ;
#33022=CARTESIAN_POINT('Ctrl Pts',(-20.1714411021644,49.3857049887665,122.47720268182)) ;
#33023=CARTESIAN_POINT('Ctrl Pts',(-20.5487252565727,49.5756013002292,122.424969613015)) ;
#33024=CARTESIAN_POINT('Ctrl Pts',(-20.3208300784889,49.3956122198664,122.622336896963)) ;
#33025=CARTESIAN_POINT('Ctrl Pts',(-20.7021484057419,49.5855476789066,122.636565942067)) ;
#33026=CARTESIAN_POINT('Ctrl Pts',(-20.4435688760117,49.4055585985438,122.791613175442)) ;
#33027=CARTESIAN_POINT('Ctrl Pts',(-20.817273052069,49.5955524477155,122.872960551607)) ;
#33028=CARTESIAN_POINT('Ctrl Pts',(-20.5356691966512,49.4155633673526,122.980728486746)) ;
#33029=CARTESIAN_POINT('Ctrl Pts',(-20.8894241945035,49.6055735687357,123.126222955828)) ;
#33030=CARTESIAN_POINT('Ctrl Pts',(-20.5933907246933,49.4255844883728,123.183338265928)) ;
#33031=CARTESIAN_POINT('Ctrl Pts',(-20.9164510303163,49.6154644345883,123.384745011977)) ;
#33032=CARTESIAN_POINT('Ctrl Pts',(-20.6150128120107,49.4354753542255,123.390155041313)) ;
#33033=CARTESIAN_POINT('Ctrl Pts',(-20.8983831554368,49.6254552433476,123.64665553533)) ;
#33034=CARTESIAN_POINT('Ctrl Pts',(-20.6005593184925,49.4454661629847,123.599683344797)) ;
#33035=CARTESIAN_POINT('Ctrl Pts',(-20.8353127628865,49.6354059015279,123.900441641724)) ;
#33036=CARTESIAN_POINT('Ctrl Pts',(-20.550103868979,49.4554168211651,123.802711999998)) ;
#33037=CARTESIAN_POINT('Ctrl Pts',(-20.7296226128942,49.64534211117,124.139186358957)) ;
#33038=CARTESIAN_POINT('Ctrl Pts',(-20.4655527511557,49.4653530308072,123.993707659371)) ;
#33039=CARTESIAN_POINT('Ctrl Pts',(-20.5836489640743,49.6553252778949,124.357211327668)) ;
#33040=CARTESIAN_POINT('Ctrl Pts',(-20.3487747338897,49.475336197532,124.168127991278)) ;
#33041=CARTESIAN_POINT('Ctrl Pts',(-20.4006247563479,49.6653690751052,124.547345114736)) ;
#33042=CARTESIAN_POINT('Ctrl Pts',(-20.2023558633861,49.4853799947423,124.320235708206)) ;
#33043=CARTESIAN_POINT('Ctrl Pts',(-20.1922492122206,49.6751972912734,124.70000920038)) ;
#33044=CARTESIAN_POINT('Ctrl Pts',(-20.0356569367093,49.4952082109106,124.442367083583)) ;
#33045=CARTESIAN_POINT('Ctrl Pts',(-19.9548171286621,49.6852738587427,124.817128808093)) ;
#33046=CARTESIAN_POINT('Ctrl Pts',(-19.84571140594,49.5052847783798,124.536063826559)) ;
#33047=CARTESIAN_POINT('Ctrl Pts',(-19.706248503042,49.6951259444321,124.889748332412)) ;
#33048=CARTESIAN_POINT('Ctrl Pts',(-19.646857742828,49.5151368640692,124.594160163181)) ;
#33049=CARTESIAN_POINT('Ctrl Pts',(-19.4431934347657,49.7051992118375,124.918954084388)) ;
#33050=CARTESIAN_POINT('Ctrl Pts',(-19.436413489415,49.5252101314746,124.617525881266)) ;
#33051=CARTESIAN_POINT('Ctrl Pts',(-19.1850858539182,49.7150406282611,124.902355961624)) ;
#33052=CARTESIAN_POINT('Ctrl Pts',(-19.2299283962633,49.5350515478982,124.604248517549)) ;
#33053=CARTESIAN_POINT('Ctrl Pts',(-18.93051882681,49.7250018864038,124.841407931651)) ;
#33054=CARTESIAN_POINT('Ctrl Pts',(-19.0262747888918,49.545012806041,124.555491422723)) ;
#33055=CARTESIAN_POINT('Ctrl Pts',(-18.6887821551517,49.7350385628358,124.735926054212)) ;
#33056=CARTESIAN_POINT('Ctrl Pts',(-18.8328848873509,49.5550494824729,124.471106955947)) ;
#33057=CARTESIAN_POINT('Ctrl Pts',(-18.472223638631,49.7449171706996,124.592716974689)) ;
#33058=CARTESIAN_POINT('Ctrl Pts',(-18.6596380365307,49.5649280903367,124.356541193233)) ;
#33059=CARTESIAN_POINT('Ctrl Pts',(-18.2803615486336,49.7549773993384,124.410883615209)) ;
#33060=CARTESIAN_POINT('Ctrl Pts',(-18.5061473145343,49.5749883189755,124.211075281749)) ;
#33061=CARTESIAN_POINT('Ctrl Pts',(-18.1259078276829,49.7648443834992,124.2025693445)) ;
#33062=CARTESIAN_POINT('Ctrl Pts',(-18.3825837898089,49.5848553031363,124.044425304176)) ;
#33063=CARTESIAN_POINT('Ctrl Pts',(-18.007919160607,49.7748499497519,123.967632043592)) ;
#33064=CARTESIAN_POINT('Ctrl Pts',(-18.2881916293145,49.594860869389,123.856476155528)) ;
#33065=CARTESIAN_POINT('Ctrl Pts',(-17.9327202356782,49.7848337381665,123.716228002346)) ;
#33066=CARTESIAN_POINT('Ctrl Pts',(-18.2280312110072,49.6048446578036,123.655353491718)) ;
#33067=CARTESIAN_POINT('Ctrl Pts',(-17.9024202751919,49.7948795949691,123.453999545748)) ;
#33068=CARTESIAN_POINT('Ctrl Pts',(-18.2037899069106,49.6148905146063,123.445570751579)) ;
#33069=CARTESIAN_POINT('Ctrl Pts',(-17.9174338428605,49.8047054721851,123.196221483282)) ;
#33070=CARTESIAN_POINT('Ctrl Pts',(-18.2157993021619,49.6247163918222,123.23934924798)) ;
#33071=CARTESIAN_POINT('Ctrl Pts',(-17.9771398351836,49.8146959480264,122.940561425494)) ;
#33072=CARTESIAN_POINT('Ctrl Pts',(-18.2635625340082,49.6347068676635,123.034820978752)) ;
#33073=CARTESIAN_POINT('Ctrl Pts',(-18.0815158765867,49.8247395239252,122.698141841169)) ;
#33074=CARTESIAN_POINT('Ctrl Pts',(-18.3470620957204,49.6447504435623,122.840884636504)) ;
#33075=CARTESIAN_POINT('Ctrl Pts',(-18.2227460406671,49.8345613162232,122.482103844544)) ;
#33076=CARTESIAN_POINT('Ctrl Pts',(-18.4600443913908,49.6545722358604,122.668054229687)) ;
#33077=CARTESIAN_POINT('Ctrl Pts',(-18.4027042307795,49.8445962818491,122.289342033901)) ;
#33078=CARTESIAN_POINT('Ctrl Pts',(-18.6040097854602,49.6646072014862,122.513843584762)) ;
#33079=CARTESIAN_POINT('Ctrl Pts',(-18.6136336981396,49.8546211987822,122.131496311253)) ;
#33080=CARTESIAN_POINT('Ctrl Pts',(-18.772752461505,49.6746321184193,122.38756577421)) ;
#33081=CARTESIAN_POINT('Ctrl Pts',(-18.844452425863,49.8644731371583,122.014217927815)) ;
#33082=CARTESIAN_POINT('Ctrl Pts',(-18.9574059859319,49.6844840567954,122.293741978756)) ;
#33083=CARTESIAN_POINT('Ctrl Pts',(-19.0954698169911,49.8744641131831,121.937362207403)) ;
#33084=CARTESIAN_POINT('Ctrl Pts',(-19.1582192690863,49.6944750328202,122.232255812791)) ;
#33085=CARTESIAN_POINT('Ctrl Pts',(-19.3541562238253,49.8843819339867,121.905312031361)) ;
#33086=CARTESIAN_POINT('Ctrl Pts',(-19.3651677277275,49.7043928536238,122.206614010283)) ;
#33087=CARTESIAN_POINT('Ctrl Pts',(-19.6173285205986,49.8944106545513,121.918768394832)) ;
#33088=CARTESIAN_POINT('Ctrl Pts',(-19.5757056845183,49.7144215741884,122.217377365489)) ;
#33089=CARTESIAN_POINT('Ctrl Pts',(-19.8705237928236,49.9042935811605,121.976696588945)) ;
#33090=CARTESIAN_POINT('Ctrl Pts',(-19.7782617108459,49.7243045007976,122.263718061929)) ;
#33091=CARTESIAN_POINT('Ctrl Pts',(-20.1128653758692,49.91429786628,122.078541501099)) ;
#33092=CARTESIAN_POINT('Ctrl Pts',(-19.9721356237173,49.7343087859171,122.345192269613)) ;
#33093=CARTESIAN_POINT('Ctrl Pts',(-20.3334334359267,49.9242815474878,122.22068996082)) ;
#33094=CARTESIAN_POINT('Ctrl Pts',(-20.1485909406997,49.7442924671249,122.458909422584)) ;
#33095=CARTESIAN_POINT('Ctrl Pts',(-20.5268216963565,49.9343225462177,122.400179102875)) ;
#33096=CARTESIAN_POINT('Ctrl Pts',(-20.3033028181441,49.7543334658549,122.602499480691)) ;
#33097=CARTESIAN_POINT('Ctrl Pts',(-20.683102613612,49.9441549910849,122.605949735523)) ;
#33098=CARTESIAN_POINT('Ctrl Pts',(-20.4283285548429,49.764165910722,122.767114266815)) ;
#33099=CARTESIAN_POINT('Ctrl Pts',(-20.8039177883312,49.9541499895152,122.839164524174)) ;
#33100=CARTESIAN_POINT('Ctrl Pts',(-20.5249823843959,49.7741609091523,122.953685109195)) ;
#33101=CARTESIAN_POINT('Ctrl Pts',(-20.8821585762413,49.9641815382648,123.090919199762)) ;
#33102=CARTESIAN_POINT('Ctrl Pts',(-20.5875768107398,49.7841924579019,123.155088321944)) ;
#33103=CARTESIAN_POINT('Ctrl Pts',(-20.9152659613685,49.9740469165703,123.348034537658)) ;
#33104=CARTESIAN_POINT('Ctrl Pts',(-20.6140645490356,49.7940578362074,123.3607797692)) ;
#33105=CARTESIAN_POINT('Ctrl Pts',(-20.9038469302478,49.9840087640306,123.609580354995)) ;
#33106=CARTESIAN_POINT('Ctrl Pts',(-20.6049313502839,49.8040196836677,123.57001630993)) ;
#33107=CARTESIAN_POINT('Ctrl Pts',(-20.8463577366402,49.9940437048448,123.8669305923)) ;
#33108=CARTESIAN_POINT('Ctrl Pts',(-20.5589419045982,49.814054624482,123.77589695398)) ;
#33109=CARTESIAN_POINT('Ctrl Pts',(-20.7469555508652,50.003928665862,124.106966043971)) ;
#33110=CARTESIAN_POINT('Ctrl Pts',(-20.4794221918956,49.8239395854991,123.967925670353)) ;
#33111=CARTESIAN_POINT('Ctrl Pts',(-20.6048292012254,50.0139942747808,124.330001338928)) ;
#33112=CARTESIAN_POINT('Ctrl Pts',(-20.3657227455692,49.8340051944179,124.146355087729)) ;
#33113=CARTESIAN_POINT('Ctrl Pts',(-20.4302906277304,50.0238334498225,124.520821628096)) ;
#33114=CARTESIAN_POINT('Ctrl Pts',(-20.2260937730439,49.8438443694597,124.299012279554)) ;
#33115=CARTESIAN_POINT('Ctrl Pts',(-20.2208961768224,50.0338960053224,124.682260919657)) ;
#33116=CARTESIAN_POINT('Ctrl Pts',(-20.0585794010133,49.8539069249596,124.42816542681)) ;
#33117=CARTESIAN_POINT('Ctrl Pts',(-19.990330202873,50.0437931800154,124.802645968509)) ;
#33118=CARTESIAN_POINT('Ctrl Pts',(-19.8741279016726,49.8638040996525,124.524475111746)) ;
#33119=CARTESIAN_POINT('Ctrl Pts',(-19.7418079589796,50.0537238949387,124.882264366511)) ;
#33120=CARTESIAN_POINT('Ctrl Pts',(-19.6753109887391,49.8737348145758,124.588171796186)) ;
#33121=CARTESIAN_POINT('Ctrl Pts',(-19.4802461248259,50.0637679230163,124.91762289268)) ;
#33122=CARTESIAN_POINT('Ctrl Pts',(-19.4660617807019,49.8837788426534,124.616460713011)) ;
#33123=CARTESIAN_POINT('Ctrl Pts',(-19.2206304688887,50.0736541248696,124.907397165842)) ;
#33124=CARTESIAN_POINT('Ctrl Pts',(-19.2583695113846,49.8936650445067,124.608282273323)) ;
#33125=CARTESIAN_POINT('Ctrl Pts',(-18.9639476699514,50.0836472913365,124.852050273482)) ;
#33126=CARTESIAN_POINT('Ctrl Pts',(-19.0530228963227,49.9036582109736,124.564006892753)) ;
#33127=CARTESIAN_POINT('Ctrl Pts',(-18.7219951492464,50.0935867623236,124.753556604735)) ;
#33128=CARTESIAN_POINT('Ctrl Pts',(-18.8594602370748,49.9135976819608,124.485214036914)) ;
#33129=CARTESIAN_POINT('Ctrl Pts',(-18.4991286839628,50.1036032766778,124.613546547454)) ;
#33130=CARTESIAN_POINT('Ctrl Pts',(-18.6811659438584,49.9236141963149,124.37320785353)) ;
#33131=CARTESIAN_POINT('Ctrl Pts',(-18.305447857855,50.1135333031546,124.438612238836)) ;
#33132=CARTESIAN_POINT('Ctrl Pts',(-18.5262199636435,49.9335442227918,124.233262162402)) ;
#33133=CARTESIAN_POINT('Ctrl Pts',(-18.1432330982203,50.1235858386641,124.23014085339)) ;
#33134=CARTESIAN_POINT('Ctrl Pts',(-18.396446423529,49.9435967583012,124.066486379902)) ;
#33135=CARTESIAN_POINT('Ctrl Pts',(-18.0220679537995,50.1334322418838,124.001499451881)) ;
#33136=CARTESIAN_POINT('Ctrl Pts',(-18.2995125219658,49.9534431615209,123.883574567668)) ;
#33137=CARTESIAN_POINT('Ctrl Pts',(-17.9407108291128,50.1433942847378,123.752685556883)) ;
#33138=CARTESIAN_POINT('Ctrl Pts',(-18.2344247243619,49.963405204375,123.684524241367)) ;
#33139=CARTESIAN_POINT('Ctrl Pts',(-17.903879790198,50.1534228355285,123.491714650898)) ;
#33140=CARTESIAN_POINT('Ctrl Pts',(-18.2049577020538,49.9734337551656,123.475747861428)) ;
#33141=CARTESIAN_POINT('Ctrl Pts',(-17.9127260347505,50.1633331612461,123.23144379837)) ;
#33142=CARTESIAN_POINT('Ctrl Pts',(-18.212032467387,49.9833440808833,123.267531271564)) ;
#33143=CARTESIAN_POINT('Ctrl Pts',(-17.9660995838745,50.1732680730757,122.975870378448)) ;
#33144=CARTESIAN_POINT('Ctrl Pts',(-18.2547290835788,49.9932789927128,123.063072178671)) ;
#33145=CARTESIAN_POINT('Ctrl Pts',(-18.0642927488552,50.1833090798438,122.730962183356)) ;
#33146=CARTESIAN_POINT('Ctrl Pts',(-18.3332815219319,50.0033199994809,122.867144823383)) ;
#33147=CARTESIAN_POINT('Ctrl Pts',(-18.201255664043,50.193196712676,122.510138724716)) ;
#33148=CARTESIAN_POINT('Ctrl Pts',(-18.4428498771025,50.0132076323131,122.690484981077)) ;
#33149=CARTESIAN_POINT('Ctrl Pts',(-18.3759163267486,50.203187143774,122.314146410369)) ;
#33150=CARTESIAN_POINT('Ctrl Pts',(-18.5825766919906,50.0231980634112,122.533689671197)) ;
#33151=CARTESIAN_POINT('Ctrl Pts',(-18.5813368510253,50.2131425803313,122.152125343484)) ;
#33152=CARTESIAN_POINT('Ctrl Pts',(-18.7469116404268,50.0331534999684,122.404071093068)) ;
#33153=CARTESIAN_POINT('Ctrl Pts',(-18.8104932141694,50.2230535284306,122.028377092564)) ;
#33154=CARTESIAN_POINT('Ctrl Pts',(-18.9302356832612,50.0430644480677,122.305070539431)) ;
#33155=CARTESIAN_POINT('Ctrl Pts',(-19.0601191774314,50.2330656045283,121.945157820195)) ;
#33156=CARTESIAN_POINT('Ctrl Pts',(-19.1299354530242,50.0530765241654,122.238492965492)) ;
#33157=CARTESIAN_POINT('Ctrl Pts',(-19.3208286510922,50.2430929266033,121.907019503274)) ;
#33158=CARTESIAN_POINT('Ctrl Pts',(-19.3385035281413,50.0631038462404,122.207980229758)) ;
#33159=CARTESIAN_POINT('Ctrl Pts',(-19.5798646279409,50.2529517015574,121.913948569486)) ;
#33160=CARTESIAN_POINT('Ctrl Pts',(-19.5457290400626,50.0729626211945,122.213520711451)) ;
#33161=CARTESIAN_POINT('Ctrl Pts',(-19.9254133373517,50.2663778943698,121.984759551957)) ;
#33162=CARTESIAN_POINT('Ctrl Pts',(-19.8221850711281,50.086388814007,122.270169142813)) ;
#33163=CARTESIAN_POINT('Ctrl Pts',(-20.2369013110527,50.2794619101513,122.13968280904)) ;
#33164=CARTESIAN_POINT('Ctrl Pts',(-20.0713939474092,50.0994728297884,122.394125151919)) ;
#33165=CARTESIAN_POINT('Ctrl Pts',(-20.5024950621529,50.2929353589065,122.373723117195)) ;
#33166=CARTESIAN_POINT('Ctrl Pts',(-20.2838339357162,50.1129462785436,122.581328603426)) ;
#33167=CARTESIAN_POINT('Ctrl Pts',(-20.6634968410946,50.3027683167123,122.575877232274)) ;
#33168=CARTESIAN_POINT('Ctrl Pts',(-20.4126446009124,50.1227792363495,122.743055923512)) ;
#33169=CARTESIAN_POINT('Ctrl Pts',(-20.7895391335986,50.312731590163,122.805346777483)) ;
#33170=CARTESIAN_POINT('Ctrl Pts',(-20.5134783878091,50.1327425098001,122.926629108663)) ;
#33171=CARTESIAN_POINT('Ctrl Pts',(-20.8739118055342,50.322768663981,123.05524832364)) ;
#33172=CARTESIAN_POINT('Ctrl Pts',(-20.5809791128739,50.1427795836181,123.126549935224)) ;
#33173=CARTESIAN_POINT('Ctrl Pts',(-20.9134611751376,50.3326436669926,123.311752830501)) ;
#33174=CARTESIAN_POINT('Ctrl Pts',(-20.6126206731099,50.1526545866297,123.331753172435)) ;
#33175=CARTESIAN_POINT('Ctrl Pts',(-20.9077542261225,50.3427113466188,123.576222416539)) ;
#33176=CARTESIAN_POINT('Ctrl Pts',(-20.6080572696327,50.1627222662559,123.543329200487)) ;
#33177=CARTESIAN_POINT('Ctrl Pts',(-20.857508009601,50.3525521968365,123.829932935511)) ;
#33178=CARTESIAN_POINT('Ctrl Pts',(-20.5678626302659,50.1725631164736,123.746296581769)) ;
#33179=CARTESIAN_POINT('Ctrl Pts',(-20.7314548291478,50.3658883953125,124.156910684336)) ;
#33180=CARTESIAN_POINT('Ctrl Pts',(-20.4670213805127,50.1858993149496,124.00788851066)) ;
#33181=CARTESIAN_POINT('Ctrl Pts',(-20.524653068368,50.3791059191269,124.440925618285)) ;
#33182=CARTESIAN_POINT('Ctrl Pts',(-20.3015547453208,50.199116838764,124.235123745287)) ;
#33183=CARTESIAN_POINT('Ctrl Pts',(-20.252395006723,50.3924408456182,124.66151880778)) ;
#33184=CARTESIAN_POINT('Ctrl Pts',(-20.0837839668042,50.2124517652553,124.411566257854)) ;
#33185=CARTESIAN_POINT('Ctrl Pts',(-20.0229851842833,50.4024239462128,124.788869046757)) ;
#33186=CARTESIAN_POINT('Ctrl Pts',(-19.9002502106648,50.2224348658499,124.513455083149)) ;
#33187=CARTESIAN_POINT('Ctrl Pts',(-19.7733522297728,50.4124687221124,124.874590001612)) ;
#33188=CARTESIAN_POINT('Ctrl Pts',(-19.7005468471622,50.2324796417495,124.582032094973)) ;
#33189=CARTESIAN_POINT('Ctrl Pts',(-19.5185568926512,50.4222866452983,124.915250650633)) ;
#33190=CARTESIAN_POINT('Ctrl Pts',(-19.4967086995116,50.2422975649354,124.614562632195)) ;
#33191=CARTESIAN_POINT('Ctrl Pts',(-19.2545052235582,50.4323359592536,124.911493375565)) ;
#33192=CARTESIAN_POINT('Ctrl Pts',(-19.2854717860523,50.2523468788908,124.611560855551)) ;
#33193=CARTESIAN_POINT('Ctrl Pts',(-18.9112636456039,50.4456396998762,124.845209773811)) ;
#33194=CARTESIAN_POINT('Ctrl Pts',(-19.0108574254215,50.2656506195133,124.558525723013)) ;
#33195=CARTESIAN_POINT('Ctrl Pts',(-18.5163636183236,50.4621298953529,124.654888417403)) ;
#33196=CARTESIAN_POINT('Ctrl Pts',(-18.6949672451094,50.28214081499,124.406294866323)) ;
#33197=CARTESIAN_POINT('Ctrl Pts',(-18.2061311342259,50.4788490602775,124.336917792434)) ;
#33198=CARTESIAN_POINT('Ctrl Pts',(-18.4467378517919,50.2988599799146,124.151872297986)) ;
#33199=CARTESIAN_POINT('Ctrl Pts',(-18.0368827272804,50.4920100539476,124.035219084609)) ;
#33200=CARTESIAN_POINT('Ctrl Pts',(-18.311368220634,50.3120209735847,123.910554390484)) ;
#33201=CARTESIAN_POINT('Ctrl Pts',(-17.9492027072533,50.5020062760529,123.787616040863)) ;
#33202=CARTESIAN_POINT('Ctrl Pts',(-18.2412163833771,50.32201719569,123.712463854449)) ;
#33203=CARTESIAN_POINT('Ctrl Pts',(-17.9063100733637,50.5120301155866,123.527712476807)) ;
#33204=CARTESIAN_POINT('Ctrl Pts',(-18.2069016114084,50.3320410352238,123.504545668271)) ;
#33205=CARTESIAN_POINT('Ctrl Pts',(-17.9093431973629,50.5252234375799,123.180991999699)) ;
#33206=CARTESIAN_POINT('Ctrl Pts',(-18.2093282776367,50.345234357217,123.227157652856)) ;
#33207=CARTESIAN_POINT('Ctrl Pts',(-18.027118283777,50.5418826093572,122.754212984447)) ;
#33208=CARTESIAN_POINT('Ctrl Pts',(-18.3035426189576,50.3618935289943,122.885745424795)) ;
#33209=CARTESIAN_POINT('Ctrl Pts',(-18.333937561739,50.5617927848429,122.323039035125)) ;
#33210=CARTESIAN_POINT('Ctrl Pts',(-18.5489966706976,50.38180370448,122.540800132755)) ;
#33211=CARTESIAN_POINT('Ctrl Pts',(-18.7684393921744,50.5816827726873,122.021820822919)) ;
#33212=CARTESIAN_POINT('Ctrl Pts',(-18.8965968570353,50.4016936923244,122.299823770032)) ;
#33213=CARTESIAN_POINT('Ctrl Pts',(-19.2825937715403,50.6016882207021,121.886677539595)) ;
#33214=CARTESIAN_POINT('Ctrl Pts',(-19.307919625913,50.4216991403392,122.191706067227)) ;
#33215=CARTESIAN_POINT('Ctrl Pts',(-19.8078113963263,50.6215246147294,121.934169205366)) ;
#33216=CARTESIAN_POINT('Ctrl Pts',(-19.7280952319297,50.4415355343665,122.229696987763)) ;
#33217=CARTESIAN_POINT('Ctrl Pts',(-20.2892513212485,50.6415324086261,122.159662815759)) ;
#33218=CARTESIAN_POINT('Ctrl Pts',(-20.1132481557937,50.4615433282632,122.410089630547)) ;
#33219=CARTESIAN_POINT('Ctrl Pts',(-20.6617398847741,50.66135904492,122.532541564671)) ;
#33220=CARTESIAN_POINT('Ctrl Pts',(-20.4112416638867,50.4813699645572,122.708392168977)) ;
#33221=CARTESIAN_POINT('Ctrl Pts',(-20.8871620269531,50.6813379878739,123.013304098428)) ;
#33222=CARTESIAN_POINT('Ctrl Pts',(-20.5915810553221,50.501348907511,123.093001677507)) ;
#33223=CARTESIAN_POINT('Ctrl Pts',(-20.9339369378857,50.701269789743,123.540918150504)) ;
#33224=CARTESIAN_POINT('Ctrl Pts',(-20.6290028531258,50.5212807093801,123.515093416669)) ;
#33225=CARTESIAN_POINT('Ctrl Pts',(-20.8002489892957,50.7210940902405,124.050742162796)) ;
#33226=CARTESIAN_POINT('Ctrl Pts',(-20.5220534268662,50.5411050098776,123.922954725086)) ;
#33227=CARTESIAN_POINT('Ctrl Pts',(-20.4959470937685,50.7411900915803,124.489434446394)) ;
#33228=CARTESIAN_POINT('Ctrl Pts',(-20.2786119963971,50.5612010112175,124.273908331322)) ;
#33229=CARTESIAN_POINT('Ctrl Pts',(-20.0674250455001,50.7609485076843,124.793529199864)) ;
#33230=CARTESIAN_POINT('Ctrl Pts',(-19.9357982255067,50.5809594273214,124.517186790158)) ;
#33231=CARTESIAN_POINT('Ctrl Pts',(-19.5529196248031,50.7810422005684,124.935512899744)) ;
#33232=CARTESIAN_POINT('Ctrl Pts',(-19.524171586782,50.6010531202055,124.630773511285)) ;
#33233=CARTESIAN_POINT('Ctrl Pts',(-19.2053312341041,50.7941531664751,124.907880339345)) ;
#33234=CARTESIAN_POINT('Ctrl Pts',(-19.2461441930599,50.6141640861122,124.608669210494)) ;
#33235=CARTESIAN_POINT('Ctrl Pts',(-19.035117438896,50.8008665412629,124.864312062334)) ;
#33236=CARTESIAN_POINT('Ctrl Pts',(-19.1099467513572,50.6208774609001,124.573813086965)) ;
#33237=CARTESIAN_POINT('',(-20.7227191491167,12.1498929727495,122.68753928809)) ;
#33238=CARTESIAN_POINT('',(-20.4664913274138,12.,122.732834476394)) ;
#33239=CARTESIAN_POINT('Ctrl Pts',(-20.7227191491167,12.1498929727495,122.68753928809)) ;
#33240=CARTESIAN_POINT('Ctrl Pts',(-20.7010586156241,12.1380608205066,122.687740528906)) ;
#33241=CARTESIAN_POINT('Ctrl Pts',(-20.6788750303579,12.1257316308462,122.688962697014)) ;
#33242=CARTESIAN_POINT('Ctrl Pts',(-20.6565183911447,12.1130842758946,122.691175310439)) ;
#33243=CARTESIAN_POINT('Ctrl Pts',(-20.6339362615787,12.1003093589914,122.693410240411)) ;
#33244=CARTESIAN_POINT('Ctrl Pts',(-20.6111778962031,12.0872098262344,122.696655512741)) ;
#33245=CARTESIAN_POINT('Ctrl Pts',(-20.5885827815958,12.0739700078726,122.700830016118)) ;
#33246=CARTESIAN_POINT('Ctrl Pts',(-20.5650612529886,12.0601873485781,122.705175676775)) ;
#33247=CARTESIAN_POINT('Ctrl Pts',(-20.541716986944,12.046252664071,122.710528106775)) ;
#33248=CARTESIAN_POINT('Ctrl Pts',(-20.5189045693268,12.0323738925062,122.716744901924)) ;
#33249=CARTESIAN_POINT('Ctrl Pts',(-20.5010561838023,12.021515172065,122.721608908816)) ;
#33250=CARTESIAN_POINT('Ctrl Pts',(-20.4835327586187,12.0106906783193,122.72700084837)) ;
#33251=CARTESIAN_POINT('Ctrl Pts',(-20.4664913276595,11.9999999999988,122.732834476261)) ;
#33252=CARTESIAN_POINT('',(-17.9096492507572,12.,123.379771111334)) ;
#33253=CARTESIAN_POINT('Ctrl Pts',(-20.4664913276595,11.9999999999988,122.732834476261)) ;
#33254=CARTESIAN_POINT('Ctrl Pts',(-20.4509543572035,11.9999999999989,122.704060366312)) ;
#33255=CARTESIAN_POINT('Ctrl Pts',(-20.4342538607019,12.,122.675825907815)) ;
#33256=CARTESIAN_POINT('Ctrl Pts',(-20.4164330413058,12.,122.648224859268)) ;
#33257=CARTESIAN_POINT('Ctrl Pts',(-20.3766729892274,12.,122.586644125901)) ;
#33258=CARTESIAN_POINT('Ctrl Pts',(-20.3313233976647,12.,122.528197448024)) ;
#33259=CARTESIAN_POINT('Ctrl Pts',(-20.2807728582503,12.,122.473687896805)) ;
#33260=CARTESIAN_POINT('Ctrl Pts',(-20.2341054743954,12.,122.423365621712)) ;
#33261=CARTESIAN_POINT('Ctrl Pts',(-20.1829884635469,11.9999999994,122.376380466302)) ;
#33262=CARTESIAN_POINT('Ctrl Pts',(-20.1278748005212,11.9999999999304,122.333498241347)) ;
#33263=CARTESIAN_POINT('Ctrl Pts',(-20.1234434404153,11.9999999999731,122.330050338042)) ;
#33264=CARTESIAN_POINT('Ctrl Pts',(-20.1189862610655,12.,122.32662898048)) ;
#33265=CARTESIAN_POINT('Ctrl Pts',(-20.1145035075594,12.,122.323234577862)) ;
#33266=CARTESIAN_POINT('Ctrl Pts',(-20.0669031140567,12.,122.287190905126)) ;
#33267=CARTESIAN_POINT('Ctrl Pts',(-20.0164366742931,12.0000000052168,122.254200732626)) ;
#33268=CARTESIAN_POINT('Ctrl Pts',(-19.9637911702411,12.0000000018168,122.224745622377)) ;
#33269=CARTESIAN_POINT('Ctrl Pts',(-19.9499756315567,12.0000000009246,122.217015841413)) ;
#33270=CARTESIAN_POINT('Ctrl Pts',(-19.9360102767224,12.,122.209529633199)) ;
#33271=CARTESIAN_POINT('Ctrl Pts',(-19.9219080603125,12.,122.202295954535)) ;
#33272=CARTESIAN_POINT('Ctrl Pts',(-19.8542244544787,12.,122.167577904465)) ;
#33273=CARTESIAN_POINT('Ctrl Pts',(-19.7833590089754,12.,122.138660939201)) ;
#33274=CARTESIAN_POINT('Ctrl Pts',(-19.7093663209473,12.,122.115884324254)) ;
#33275=CARTESIAN_POINT('Ctrl Pts',(-19.6563392668767,12.,122.099561403375)) ;
#33276=CARTESIAN_POINT('Ctrl Pts',(-19.6017001635138,12.0000000149114,122.086390904151)) ;
#33277=CARTESIAN_POINT('Ctrl Pts',(-19.546212003709,12.0000000073334,122.076657410532)) ;
#33278=CARTESIAN_POINT('Ctrl Pts',(-19.5244859763294,12.0000000043663,122.072846324535)) ;
#33279=CARTESIAN_POINT('Ctrl Pts',(-19.5026303315761,12.,122.069562280034)) ;
#33280=CARTESIAN_POINT('Ctrl Pts',(-19.4806930068947,12.,122.066822797438)) ;
#33281=CARTESIAN_POINT('Ctrl Pts',(-19.402879099977,12.,122.057105575911)) ;
#33282=CARTESIAN_POINT('Ctrl Pts',(-19.3241008842937,12.,122.054249810868)) ;
#33283=CARTESIAN_POINT('Ctrl Pts',(-19.2452460130912,12.,122.058247839665)) ;
#33284=CARTESIAN_POINT('Ctrl Pts',(-19.1665569481981,12.,122.062237461899)) ;
#33285=CARTESIAN_POINT('Ctrl Pts',(-19.0877130844164,12.,122.073053895301)) ;
#33286=CARTESIAN_POINT('Ctrl Pts',(-19.0093824990468,12.,122.090995385507)) ;
#33287=CARTESIAN_POINT('Ctrl Pts',(-18.9507187051536,12.,122.104432229858)) ;
#33288=CARTESIAN_POINT('Ctrl Pts',(-18.8923478250649,12.0000000102563,122.121865317184)) ;
#33289=CARTESIAN_POINT('Ctrl Pts',(-18.8351097436429,12.0000000043775,122.143167364287)) ;
#33290=CARTESIAN_POINT('Ctrl Pts',(-18.8161414792467,12.0000000024293,122.150226700512)) ;
#33291=CARTESIAN_POINT('Ctrl Pts',(-18.7972980263926,12.,122.157710808519)) ;
#33292=CARTESIAN_POINT('Ctrl Pts',(-18.7786111581444,12.,122.165614672269)) ;
#33293=CARTESIAN_POINT('Ctrl Pts',(-18.7118018157948,12.,122.193872587514)) ;
#33294=CARTESIAN_POINT('Ctrl Pts',(-18.6470553315846,12.0000000003845,122.227471732854)) ;
#33295=CARTESIAN_POINT('Ctrl Pts',(-18.5852217646428,12.0000000000663,122.265859882284)) ;
#33296=CARTESIAN_POINT('Ctrl Pts',(-18.5776852993161,12.0000000000275,122.270538748011)) ;
#33297=CARTESIAN_POINT('Ctrl Pts',(-18.5701921517252,12.,122.275288711735)) ;
#33298=CARTESIAN_POINT('Ctrl Pts',(-18.5627438981913,12.,122.280108735924)) ;
#33299=CARTESIAN_POINT('Ctrl Pts',(-18.4980309831752,12.,122.32198671635)) ;
#33300=CARTESIAN_POINT('Ctrl Pts',(-18.4366368756665,11.9999999928402,122.369197267935)) ;
#33301=CARTESIAN_POINT('Ctrl Pts',(-18.3787222199717,11.9999999993994,122.422020424971)) ;
#33302=CARTESIAN_POINT('Ctrl Pts',(-18.3753891921239,11.9999999997769,122.425060433606)) ;
#33303=CARTESIAN_POINT('Ctrl Pts',(-18.3720676802587,12.,122.428119043496)) ;
#33304=CARTESIAN_POINT('Ctrl Pts',(-18.3687577121273,12.,122.431196312548)) ;
#33305=CARTESIAN_POINT('Ctrl Pts',(-18.3264247986708,12.,122.470553115778)) ;
#33306=CARTESIAN_POINT('Ctrl Pts',(-18.2859739515088,12.0000000189751,122.512967788025)) ;
#33307=CARTESIAN_POINT('Ctrl Pts',(-18.2480707810569,12.0000000101354,122.557909386313)) ;
#33308=CARTESIAN_POINT('Ctrl Pts',(-18.2316777870941,12.0000000063122,122.577346476684)) ;
#33309=CARTESIAN_POINT('Ctrl Pts',(-18.2157618098082,12.,122.59725577119)) ;
#33310=CARTESIAN_POINT('Ctrl Pts',(-18.2003787759881,12.,122.617592113997)) ;
#33311=CARTESIAN_POINT('Ctrl Pts',(-18.1495353272504,12.,122.684807061005)) ;
#33312=CARTESIAN_POINT('Ctrl Pts',(-18.1045662126026,12.,122.756621216588)) ;
#33313=CARTESIAN_POINT('Ctrl Pts',(-18.0659377442576,12.,122.832173109989)) ;
#33314=CARTESIAN_POINT('Ctrl Pts',(-18.027387955545,12.,122.907571117009)) ;
#33315=CARTESIAN_POINT('Ctrl Pts',(-17.995114699564,12.,122.986761016303)) ;
#33316=CARTESIAN_POINT('Ctrl Pts',(-17.9698216577103,12.,123.069272641495)) ;
#33317=CARTESIAN_POINT('Ctrl Pts',(-17.9521228336151,12.,123.127010210132)) ;
#33318=CARTESIAN_POINT('Ctrl Pts',(-17.9378542916193,12.0000000080963,123.186339136655)) ;
#33319=CARTESIAN_POINT('Ctrl Pts',(-17.9272125111136,12.0000000042853,123.246300595191)) ;
#33320=CARTESIAN_POINT('Ctrl Pts',(-17.9226767295839,12.0000000026609,123.271857603811)) ;
#33321=CARTESIAN_POINT('Ctrl Pts',(-17.9187998924811,12.,123.297528881935)) ;
#33322=CARTESIAN_POINT('Ctrl Pts',(-17.915597481249,12.,123.323237316211)) ;
#33323=CARTESIAN_POINT('Ctrl Pts',(-17.9132521442838,12.,123.342065298271)) ;
#33324=CARTESIAN_POINT('Ctrl Pts',(-17.9112692183144,12.,123.360907769294)) ;
#33325=CARTESIAN_POINT('Ctrl Pts',(-17.9096492507572,12.,123.379771111334)) ;
#33326=CARTESIAN_POINT('Ctrl Pts',(-17.9096492507572,12.,123.379771111334)) ;
#33327=CARTESIAN_POINT('Ctrl Pts',(-17.9100667346536,12.0007217907825,123.36087892436)) ;
#33328=CARTESIAN_POINT('Ctrl Pts',(-17.9144060035305,12.0047464667125,123.255581124476)) ;
#33329=CARTESIAN_POINT('Ctrl Pts',(-17.9427499485555,12.0121810504321,123.062292370625)) ;
#33330=CARTESIAN_POINT('Ctrl Pts',(-18.0251977237691,12.0221110972068,122.814691316201)) ;
#33331=CARTESIAN_POINT('Ctrl Pts',(-18.1490393731302,12.0320625395439,122.584356522223)) ;
#33332=CARTESIAN_POINT('Ctrl Pts',(-18.3128249788135,12.0421093367232,122.377284739554)) ;
#33333=CARTESIAN_POINT('Ctrl Pts',(-18.5060148098008,12.0519572774033,122.205087588693)) ;
#33334=CARTESIAN_POINT('Ctrl Pts',(-18.7282729224672,12.0619189087459,122.066794754727)) ;
#33335=CARTESIAN_POINT('Ctrl Pts',(-18.9729503385559,12.0719475681218,121.968835081685)) ;
#33336=CARTESIAN_POINT('Ctrl Pts',(-19.227831787757,12.08185787101,121.915407496624)) ;
#33337=CARTESIAN_POINT('Ctrl Pts',(-19.4887612039821,12.0917927655722,121.906342273827)) ;
#33338=CARTESIAN_POINT('Ctrl Pts',(-19.7500144690061,12.1018338642391,121.943349818059)) ;
#33339=CARTESIAN_POINT('Ctrl Pts',(-19.9971083719985,12.1117211467435,122.023739879768)) ;
#33340=CARTESIAN_POINT('Ctrl Pts',(-20.2290950029525,12.121712887254,122.146694306298)) ;
#33341=CARTESIAN_POINT('Ctrl Pts',(-20.4353231818005,12.1316634364894,122.307485013012)) ;
#33342=CARTESIAN_POINT('Ctrl Pts',(-20.6005848561123,12.1410363173938,122.490103477729)) ;
#33343=CARTESIAN_POINT('Ctrl Pts',(-20.6877151581443,12.1471236046148,122.624050429204)) ;
#33344=CARTESIAN_POINT('Ctrl Pts',(-20.7227191491167,12.1498929727495,122.68753928809)) ;
#33345=CARTESIAN_POINT('Origin',(-20.3808735729049,12.,126.250122109236)) ;
#33346=CARTESIAN_POINT('',(-20.4601832664426,12.,122.734993854115)) ;
#33347=CARTESIAN_POINT('',(-20.4664913274138,12.,122.732834476394)) ;
#33348=CARTESIAN_POINT('',(-18.1640505668151,12.,123.521006833268)) ;
#33349=CARTESIAN_POINT('Origin',(-19.4092722359532,12.,123.411814366564)) ;
#33350=CARTESIAN_POINT('',(-17.9353686287936,11.9999999997025,123.599289317459)) ;
#33351=CARTESIAN_POINT('',(-18.1640505668151,12.,123.521006833268)) ;
#33352=CARTESIAN_POINT('Ctrl Pts',(-17.9096492507572,12.,123.379771111334)) ;
#33353=CARTESIAN_POINT('Ctrl Pts',(-17.9111794973639,12.,123.416636495257)) ;
#33354=CARTESIAN_POINT('Ctrl Pts',(-17.9140858729415,12.0000000000049,123.453367630287)) ;
#33355=CARTESIAN_POINT('Ctrl Pts',(-17.9226794425075,12.0000000000049,123.526662996257)) ;
#33356=CARTESIAN_POINT('Ctrl Pts',(-17.9283556505042,12.,123.563110613297)) ;
#33357=CARTESIAN_POINT('Ctrl Pts',(-17.9353686298462,12.,123.599289317255)) ;
#33358=CARTESIAN_POINT('Origin',(-19.4092722359532,16.5113612779716,123.411814366564)) ;
#33359=CARTESIAN_POINT('Ctrl Pts',(-20.5919043739536,12.7298332115048,123.006991903941)) ;
#33360=CARTESIAN_POINT('Ctrl Pts',(-20.5874582960172,12.7292023169138,122.994003648584)) ;
#33361=CARTESIAN_POINT('Ctrl Pts',(-20.5827987528111,12.7285719416166,122.981089421798)) ;
#33362=CARTESIAN_POINT('Ctrl Pts',(-20.574287862775,12.7274715784339,122.958665623562)) ;
#33363=CARTESIAN_POINT('Ctrl Pts',(-20.5705305117346,12.7270013881013,122.94912179947)) ;
#33364=CARTESIAN_POINT('Ctrl Pts',(-20.5626714838065,12.7260484071683,122.929858515579)) ;
#33365=CARTESIAN_POINT('Ctrl Pts',(-20.5585633641852,12.7255656767293,122.920142554556)) ;
#33366=CARTESIAN_POINT('Ctrl Pts',(-20.5487412627525,12.7244460890821,122.897708635331)) ;
#33367=CARTESIAN_POINT('Ctrl Pts',(-20.5429364852264,12.7238096798513,122.885031927171)) ;
#33368=CARTESIAN_POINT('Ctrl Pts',(-20.5226828266888,12.7216707323095,122.842687232925)) ;
#33369=CARTESIAN_POINT('Ctrl Pts',(-20.5072714673937,12.7201741098457,122.813494564159)) ;
#33370=CARTESIAN_POINT('Ctrl Pts',(-20.4765507937487,12.7174143135874,122.760496400936)) ;
#33371=CARTESIAN_POINT('Ctrl Pts',(-20.4615536051481,12.716148146437,122.736534761797)) ;
#33372=CARTESIAN_POINT('Ctrl Pts',(-20.4278471509029,12.7134373221124,122.686533887782)) ;
#33373=CARTESIAN_POINT('Ctrl Pts',(-20.4089225377984,12.7119923140302,122.660664676273)) ;
#33374=CARTESIAN_POINT('Ctrl Pts',(-20.3859313068839,12.7103070073287,122.631646513355)) ;
#33375=CARTESIAN_POINT('Ctrl Pts',(-20.382814149153,12.7100799261839,122.627760182863)) ;
#33376=CARTESIAN_POINT('Ctrl Pts',(-20.3774854041029,12.7096940665411,122.621197319607)) ;
#33377=CARTESIAN_POINT('Ctrl Pts',(-20.3752857428806,12.7095354497977,122.618511172157)) ;
#33378=CARTESIAN_POINT('Ctrl Pts',(-20.3711723084536,12.709240043704,122.613530471045)) ;
#33379=CARTESIAN_POINT('Ctrl Pts',(-20.3692614428512,12.7091032950564,122.611233546223)) ;
#33380=CARTESIAN_POINT('Ctrl Pts',(-20.3653693291752,12.708825721361,122.606589066027)) ;
#33381=CARTESIAN_POINT('Ctrl Pts',(-20.3633876261552,12.7086848907517,122.604241918789)) ;
#33382=CARTESIAN_POINT('Ctrl Pts',(-20.3587473404578,12.708356274068,122.598786843592)) ;
#33383=CARTESIAN_POINT('Ctrl Pts',(-20.3560821193224,12.7081683963687,122.595684614761)) ;
#33384=CARTESIAN_POINT('Ctrl Pts',(-20.3478130767288,12.7075881318747,122.586154747251)) ;
#33385=CARTESIAN_POINT('Ctrl Pts',(-20.3421586935067,12.7071950422528,122.579771355263)) ;
#33386=CARTESIAN_POINT('Ctrl Pts',(-20.3088992949423,12.7049038791851,122.542989150078)) ;
#33387=CARTESIAN_POINT('Ctrl Pts',(-20.2798755959217,12.7029855180402,122.51390804049)) ;
#33388=CARTESIAN_POINT('Ctrl Pts',(-20.2184469078676,12.6990993462048,122.458141237711)) ;
#33389=CARTESIAN_POINT('Ctrl Pts',(-20.1860224438698,12.6971407738768,122.431551495952)) ;
#33390=CARTESIAN_POINT('Ctrl Pts',(-20.1369800085691,12.6943095255758,122.395298026217)) ;
#33391=CARTESIAN_POINT('Ctrl Pts',(-20.1213787048448,12.6934261763327,122.384308426099)) ;
#33392=CARTESIAN_POINT('Ctrl Pts',(-20.0965715902114,12.6920468103064,122.367670698848)) ;
#33393=CARTESIAN_POINT('Ctrl Pts',(-20.0875338440553,12.6915493493308,122.361777417857)) ;
#33394=CARTESIAN_POINT('Ctrl Pts',(-20.0722271807047,12.6907149958544,122.352076421277)) ;
#33395=CARTESIAN_POINT('Ctrl Pts',(-20.0659990140571,12.6903777307108,122.348205551803)) ;
#33396=CARTESIAN_POINT('Ctrl Pts',(-20.0545623835731,12.6897623694749,122.341236323024)) ;
#33397=CARTESIAN_POINT('Ctrl Pts',(-20.0493647604295,12.6894841745259,122.338120610274)) ;
#33398=CARTESIAN_POINT('Ctrl Pts',(-20.0391592041141,12.688940740664,122.332103339086)) ;
#33399=CARTESIAN_POINT('Ctrl Pts',(-20.0341533674478,12.6886754879462,122.32919852184)) ;
#33400=CARTESIAN_POINT('Ctrl Pts',(-20.0226611470541,12.6880694385187,122.322636009766)) ;
#33401=CARTESIAN_POINT('Ctrl Pts',(-20.0161618837293,12.687728792848,122.319001296964)) ;
#33402=CARTESIAN_POINT('Ctrl Pts',(-19.9984421190923,12.6868055644523,122.309298351561)) ;
#33403=CARTESIAN_POINT('Ctrl Pts',(-19.9871605541439,12.6862237144543,122.303343433842)) ;
#33404=CARTESIAN_POINT('Ctrl Pts',(-19.9339037825458,12.6835033315254,122.276266173459)) ;
#33405=CARTESIAN_POINT('Ctrl Pts',(-19.8908496740945,12.681379834111,122.257348579191)) ;
#33406=CARTESIAN_POINT('Ctrl Pts',(-19.8128001830863,12.6776381537056,122.228182191831)) ;
#33407=CARTESIAN_POINT('Ctrl Pts',(-19.7782297944157,12.6760162922282,122.216954437728)) ;
#33408=CARTESIAN_POINT('Ctrl Pts',(-19.7189160196954,12.6732469844032,122.20051061311)) ;
#33409=CARTESIAN_POINT('Ctrl Pts',(-19.6944145696779,12.6721070555401,122.194510018847)) ;
#33410=CARTESIAN_POINT('Ctrl Pts',(-19.6641240256707,12.6706964537624,122.188056368476)) ;
#33411=CARTESIAN_POINT('Ctrl Pts',(-19.6584912153566,12.6704340966092,122.18689682956)) ;
#33412=CARTESIAN_POINT('Ctrl Pts',(-19.6499400281158,12.6700356924186,122.185197955526)) ;
#33413=CARTESIAN_POINT('Ctrl Pts',(-19.6470273887578,12.669899970342,122.184630071821)) ;
#33414=CARTESIAN_POINT('Ctrl Pts',(-19.6411154293813,12.6696244369637,122.183499241513)) ;
#33415=CARTESIAN_POINT('Ctrl Pts',(-19.6381160149756,12.6694846198386,122.182936896065)) ;
#33416=CARTESIAN_POINT('Ctrl Pts',(-19.6316505764505,12.6691831706065,122.181749214646)) ;
#33417=CARTESIAN_POINT('Ctrl Pts',(-19.6281839097497,12.6690214986468,122.181127532615)) ;
#33418=CARTESIAN_POINT('Ctrl Pts',(-19.6188584768404,12.6685864781895,122.179495839296)) ;
#33419=CARTESIAN_POINT('Ctrl Pts',(-19.6129950704492,12.6683128313736,122.178512963329)) ;
#33420=CARTESIAN_POINT('Ctrl Pts',(-19.5821839874874,12.6668741420245,122.173573856816)) ;
#33421=CARTESIAN_POINT('Ctrl Pts',(-19.5571279908566,12.6657014134404,122.170332720993)) ;
#33422=CARTESIAN_POINT('Ctrl Pts',(-19.4910593494478,12.6626047780172,122.163814926806)) ;
#33423=CARTESIAN_POINT('Ctrl Pts',(-19.4499531256098,12.6606726915156,122.16179964462)) ;
#33424=CARTESIAN_POINT('Ctrl Pts',(-19.3810909584357,12.6574663634508,122.161824427958)) ;
#33425=CARTESIAN_POINT('Ctrl Pts',(-19.3533672570836,12.6561833626144,122.162757243192)) ;
#33426=CARTESIAN_POINT('Ctrl Pts',(-19.3131826908954,12.6543268053868,122.165450006401)) ;
#33427=CARTESIAN_POINT('Ctrl Pts',(-19.3006813626391,12.6537496800746,122.166476925026)) ;
#33428=CARTESIAN_POINT('Ctrl Pts',(-19.2782653869539,12.6527147674379,122.168658387553)) ;
#33429=CARTESIAN_POINT('Ctrl Pts',(-19.268345111649,12.6522567364059,122.169743865703)) ;
#33430=CARTESIAN_POINT('Ctrl Pts',(-19.2470262054446,12.6512718612793,122.172335282709)) ;
#33431=CARTESIAN_POINT('Ctrl Pts',(-19.2356331903504,12.6507451913567,122.173879935112)) ;
#33432=CARTESIAN_POINT('Ctrl Pts',(-19.2018478313302,12.6491813744363,122.178936102775)) ;
#33433=CARTESIAN_POINT('Ctrl Pts',(-19.1795278985088,12.6481455987097,122.1828997066)) ;
#33434=CARTESIAN_POINT('Ctrl Pts',(-19.0840932163382,12.6436958619431,122.202538113423)) ;
#33435=CARTESIAN_POINT('Ctrl Pts',(-19.0123577181082,12.6402984837699,122.224148841466)) ;
#33436=CARTESIAN_POINT('Ctrl Pts',(-18.925032714619,12.6360191620718,122.25925787892)) ;
#33437=CARTESIAN_POINT('Ctrl Pts',(-18.9072506943902,12.6351389733826,122.266891338895)) ;
#33438=CARTESIAN_POINT('Ctrl Pts',(-18.8801150158276,12.6337789901851,122.279293896089)) ;
#33439=CARTESIAN_POINT('Ctrl Pts',(-18.8706322051877,12.6333005085761,122.283773190043)) ;
#33440=CARTESIAN_POINT('Ctrl Pts',(-18.8610038414272,12.632811123212,122.28847033258)) ;
#33441=CARTESIAN_POINT('Ctrl Pts',(-18.860800803836,12.6328008017,122.288569451474)) ;
#33442=CARTESIAN_POINT('Ctrl Pts',(-18.8604029314302,12.6327805724786,122.288763818432)) ;
#33443=CARTESIAN_POINT('Ctrl Pts',(-18.860208094397,12.6327706647844,122.288859062215)) ;
#33444=CARTESIAN_POINT('Ctrl Pts',(-18.8598261936814,12.6327512417364,122.289045873025)) ;
#33445=CARTESIAN_POINT('Ctrl Pts',(-18.85963912813,12.6327417264042,122.289137436082)) ;
#33446=CARTESIAN_POINT('Ctrl Pts',(-18.8592723663165,12.6327230678687,122.289317068785)) ;
#33447=CARTESIAN_POINT('Ctrl Pts',(-18.8590926683012,12.6327139246828,122.289405134839)) ;
#33448=CARTESIAN_POINT('Ctrl Pts',(-18.8587402609276,12.6326959913847,122.289577946927)) ;
#33449=CARTESIAN_POINT('Ctrl Pts',(-18.8585675499598,12.6326872012879,122.28966268969)) ;
#33450=CARTESIAN_POINT('Ctrl Pts',(-18.8582287580403,12.6326699562002,122.289829019171)) ;
#33451=CARTESIAN_POINT('Ctrl Pts',(-18.8580626756292,12.6326615012237,122.289910602901)) ;
#33452=CARTESIAN_POINT('Ctrl Pts',(-18.8577368028425,12.632644909431,122.290070769387)) ;
#33453=CARTESIAN_POINT('Ctrl Pts',(-18.8575770111154,12.6326367726271,122.290149349424)) ;
#33454=CARTESIAN_POINT('Ctrl Pts',(-18.8572634013213,12.6326208012057,122.290303655087)) ;
#33455=CARTESIAN_POINT('Ctrl Pts',(-18.8571095819159,12.6326129665944,122.290379378276)) ;
#33456=CARTESIAN_POINT('Ctrl Pts',(-18.8568076159666,12.6325975844553,122.290528109172)) ;
#33457=CARTESIAN_POINT('Ctrl Pts',(-18.8566594684449,12.6325900369459,122.290601114529)) ;
#33458=CARTESIAN_POINT('Ctrl Pts',(-18.8563685630119,12.63257521478,122.290744540968)) ;
#33459=CARTESIAN_POINT('Ctrl Pts',(-18.8562258041211,12.6325679401361,122.29081495994)) ;
#33460=CARTESIAN_POINT('Ctrl Pts',(-18.8559454087077,12.6325536502667,122.290953337762)) ;
#33461=CARTESIAN_POINT('Ctrl Pts',(-18.8558077712247,12.6325466350494,122.291021294708)) ;
#33462=CARTESIAN_POINT('Ctrl Pts',(-18.8555373663725,12.6325328513444,122.291154865994)) ;
#33463=CARTESIAN_POINT('Ctrl Pts',(-18.8554045981134,12.6325260828639,122.291220478591)) ;
#33464=CARTESIAN_POINT('Ctrl Pts',(-18.8551436933356,12.6325127806346,122.291349472528)) ;
#33465=CARTESIAN_POINT('Ctrl Pts',(-18.8550155560846,12.6325062468968,122.291412852225)) ;
#33466=CARTESIAN_POINT('Ctrl Pts',(-18.8547636888582,12.6324934028497,122.29153748546)) ;
#33467=CARTESIAN_POINT('Ctrl Pts',(-18.8546399580043,12.63248709254,122.291598737592)) ;
#33468=CARTESIAN_POINT('Ctrl Pts',(-18.8543966903674,12.6324746846061,122.291719215792)) ;
#33469=CARTESIAN_POINT('Ctrl Pts',(-18.854277153185,12.6324685870025,122.291778440366)) ;
#33470=CARTESIAN_POINT('Ctrl Pts',(-18.8540420728504,12.6324565943971,122.291894957549)) ;
#33471=CARTESIAN_POINT('Ctrl Pts',(-18.8539265288778,12.6324506993911,122.291952249006)) ;
#33472=CARTESIAN_POINT('Ctrl Pts',(-18.8536992450398,12.6324391024022,122.292064989514)) ;
#33473=CARTESIAN_POINT('Ctrl Pts',(-18.8535875045862,12.6324334004239,122.29212043742)) ;
#33474=CARTESIAN_POINT('Ctrl Pts',(-18.8533676479513,12.6324221804159,122.292229575811)) ;
#33475=CARTESIAN_POINT('Ctrl Pts',(-18.8532595314138,12.6324166624,122.292283265148)) ;
#33476=CARTESIAN_POINT('Ctrl Pts',(-18.8530467536773,12.6324058017891,122.292388966369)) ;
#33477=CARTESIAN_POINT('Ctrl Pts',(-18.852942091726,12.6324004591854,122.292440977404)) ;
#33478=CARTESIAN_POINT('Ctrl Pts',(-18.8527360618065,12.6323899412494,122.292543398586)) ;
#33479=CARTESIAN_POINT('Ctrl Pts',(-18.8526346936263,12.6323847659338,122.292593807709)) ;
#33480=CARTESIAN_POINT('Ctrl Pts',(-18.8524350996326,12.6323745749139,122.292693097118)) ;
#33481=CARTESIAN_POINT('Ctrl Pts',(-18.8523368733561,12.6323695592114,122.29274197659)) ;
#33482=CARTESIAN_POINT('Ctrl Pts',(-18.8521434194413,12.6323596801533,122.292838275129)) ;
#33483=CARTESIAN_POINT('Ctrl Pts',(-18.8520481912971,12.6323548167953,122.29288569348)) ;
#33484=CARTESIAN_POINT('Ctrl Pts',(-18.8518605969686,12.6323452355151,122.292979134973)) ;
#33485=CARTESIAN_POINT('Ctrl Pts',(-18.8517682305587,12.6323405176031,122.293025157332)) ;
#33486=CARTESIAN_POINT('Ctrl Pts',(-18.851586230627,12.6323312206861,122.2931158685)) ;
#33487=CARTESIAN_POINT('Ctrl Pts',(-18.8514965968201,12.6323266416867,122.293160556623)) ;
#33488=CARTESIAN_POINT('Ctrl Pts',(-18.8513199396624,12.6323176163998,122.293248657901)) ;
#33489=CARTESIAN_POINT('Ctrl Pts',(-18.851232915995,12.6323131701149,122.293292070446)) ;
#33490=CARTESIAN_POINT('Ctrl Pts',(-18.8510613633768,12.6323044043985,122.293377676028)) ;
#33491=CARTESIAN_POINT('Ctrl Pts',(-18.850976833945,12.63230008496,122.293419868591)) ;
#33492=CARTESIAN_POINT('Ctrl Pts',(-18.8508101590981,12.6322915673309,122.293503087348)) ;
#33493=CARTESIAN_POINT('Ctrl Pts',(-18.850728013559,12.6322873691502,122.293544112942)) ;
#33494=CARTESIAN_POINT('Ctrl Pts',(-18.8505660023795,12.6322790887634,122.293625047793)) ;
#33495=CARTESIAN_POINT('Ctrl Pts',(-18.8504861363609,12.632275006553,122.293664956624)) ;
#33496=CARTESIAN_POINT('Ctrl Pts',(-18.8503285846757,12.6322669530628,122.293743705865)) ;
#33497=CARTESIAN_POINT('Ctrl Pts',(-18.8502508988245,12.6322629817876,122.293782545794)) ;
#33498=CARTESIAN_POINT('Ctrl Pts',(-18.8500976136337,12.6322551454121,122.293859202448)) ;
#33499=CARTESIAN_POINT('Ctrl Pts',(-18.8500220139255,12.6322512803059,122.293897018822)) ;
#33500=CARTESIAN_POINT('Ctrl Pts',(-18.8498728106033,12.6322436516842,122.29397167201)) ;
#33501=CARTESIAN_POINT('Ctrl Pts',(-18.8497992071395,12.6322398881885,122.294008508251)) ;
#33502=CARTESIAN_POINT('Ctrl Pts',(-18.8496539118487,12.6322324585051,122.294081241963)) ;
#33503=CARTESIAN_POINT('Ctrl Pts',(-18.8495822197,12.6322287923122,122.294117139132)) ;
#33504=CARTESIAN_POINT('Ctrl Pts',(-18.8494406658337,12.6322215531152,122.294188033983)) ;
#33505=CARTESIAN_POINT('Ctrl Pts',(-18.849370803934,12.6322179801123,122.294223031324)) ;
#33506=CARTESIAN_POINT('Ctrl Pts',(-18.8492328337509,12.6322109233979,122.294292163715)) ;
#33507=CARTESIAN_POINT('Ctrl Pts',(-18.8491647251495,12.6322074396799,122.29432629852)) ;
#33508=CARTESIAN_POINT('Ctrl Pts',(-18.8490301882414,12.6322005578142,122.294393741386)) ;
#33509=CARTESIAN_POINT('Ctrl Pts',(-18.8489637597144,12.6321971596645,122.294427049179)) ;
#33510=CARTESIAN_POINT('Ctrl Pts',(-18.8488325124516,12.6321904453557,122.29449287225)) ;
#33511=CARTESIAN_POINT('Ctrl Pts',(-18.8487676938904,12.6321871292143,122.294525387087)) ;
#33512=CARTESIAN_POINT('Ctrl Pts',(-18.8486396006622,12.6321805755767,122.294589656251)) ;
#33513=CARTESIAN_POINT('Ctrl Pts',(-18.8485763257236,12.6321773380746,122.294621410384)) ;
#33514=CARTESIAN_POINT('Ctrl Pts',(-18.8484512563821,12.6321709384976,122.294684188953)) ;
#33515=CARTESIAN_POINT('Ctrl Pts',(-18.8483894617543,12.6321677764187,122.294715213192)) ;
#33516=CARTESIAN_POINT('Ctrl Pts',(-18.8482672920752,12.6321615245914,122.29477656166)) ;
#33517=CARTESIAN_POINT('Ctrl Pts',(-18.8482069170872,12.6321584348532,122.294806885566)) ;
#33518=CARTESIAN_POINT('Ctrl Pts',(-18.8480875295977,12.6321523248064,122.294866861177)) ;
#33519=CARTESIAN_POINT('Ctrl Pts',(-18.8480285167885,12.6321493044888,122.294896512765)) ;
#33520=CARTESIAN_POINT('Ctrl Pts',(-18.8479117983704,12.6321433304733,122.29495517071)) ;
#33521=CARTESIAN_POINT('Ctrl Pts',(-18.8478540926495,12.632140376776,122.294984176868)) ;
#33522=CARTESIAN_POINT('Ctrl Pts',(-18.8477399358622,12.6321345333301,122.295041569607)) ;
#33523=CARTESIAN_POINT('Ctrl Pts',(-18.8476834847199,12.6321316435834,122.295069955986)) ;
#33524=CARTESIAN_POINT('Ctrl Pts',(-18.8475717866948,12.6321259254765,122.295126133796)) ;
#33525=CARTESIAN_POINT('Ctrl Pts',(-18.847516539838,12.6321230971231,122.295153924987)) ;
#33526=CARTESIAN_POINT('Ctrl Pts',(-18.8474072027659,12.6321174993812,122.295208935705)) ;
#33527=CARTESIAN_POINT('Ctrl Pts',(-18.8473531123719,12.6321147299887,122.295236155109)) ;
#33528=CARTESIAN_POINT('Ctrl Pts',(-18.847246042138,12.6321092478244,122.295290044814)) ;
#33529=CARTESIAN_POINT('Ctrl Pts',(-18.8471930623221,12.6321065350586,122.295316714903)) ;
#33530=CARTESIAN_POINT('Ctrl Pts',(-18.847088169118,12.6321011639028,122.2953695276)) ;
#33531=CARTESIAN_POINT('Ctrl Pts',(-18.847036255879,12.6320985055249,122.295395669944)) ;
#33532=CARTESIAN_POINT('Ctrl Pts',(-18.8469334541267,12.632093241023,122.295447447592)) ;
#33533=CARTESIAN_POINT('Ctrl Pts',(-18.8468825654951,12.6320906348972,122.295473082778)) ;
#33534=CARTESIAN_POINT('Ctrl Pts',(-18.8467817731904,12.6320854728756,122.295523865619)) ;
#33535=CARTESIAN_POINT('Ctrl Pts',(-18.846731869175,12.6320829169663,122.29554901328)) ;
#33536=CARTESIAN_POINT('Ctrl Pts',(-18.8466330070026,12.6320778533874,122.295598840276)) ;
#33537=CARTESIAN_POINT('Ctrl Pts',(-18.8465840488835,12.6320753457235,122.295623519436)) ;
#33538=CARTESIAN_POINT('Ctrl Pts',(-18.846487042062,12.6320703767801,122.295672427334)) ;
#33539=CARTESIAN_POINT('Ctrl Pts',(-18.8464389931377,12.6320679154928,122.295696656037)) ;
#33540=CARTESIAN_POINT('Ctrl Pts',(-18.8463437686625,12.6320630374672,122.295744680755)) ;
#33541=CARTESIAN_POINT('Ctrl Pts',(-18.8462965932748,12.6320606207405,122.29576847655)) ;
#33542=CARTESIAN_POINT('Ctrl Pts',(-18.8462030825305,12.6320558301382,122.295815651855)) ;
#33543=CARTESIAN_POINT('Ctrl Pts',(-18.8461567469141,12.6320534562524,122.295839031365)) ;
#33544=CARTESIAN_POINT('Ctrl Pts',(-18.8460648831526,12.6320487496731,122.295885390138)) ;
#33545=CARTESIAN_POINT('Ctrl Pts',(-18.8460193549114,12.6320464169778,122.295908369325)) ;
#33546=CARTESIAN_POINT('Ctrl Pts',(-18.8459290731657,12.6320417911115,122.295953943604)) ;
#33547=CARTESIAN_POINT('Ctrl Pts',(-18.8458843203151,12.6320394979768,122.295976538248)) ;
#33548=CARTESIAN_POINT('Ctrl Pts',(-18.8457955610847,12.6320349497919,122.296021357362)) ;
#33549=CARTESIAN_POINT('Ctrl Pts',(-18.8457515541166,12.6320326947142,122.296043582017)) ;
#33550=CARTESIAN_POINT('Ctrl Pts',(-18.8456642572285,12.6320282211438,122.296087675683)) ;
#33551=CARTESIAN_POINT('Ctrl Pts',(-18.8456209671826,12.6320260026471,122.296109544651)) ;
#33552=CARTESIAN_POINT('Ctrl Pts',(-18.8455350756518,12.6320216007862,122.296152941019)) ;
#33553=CARTESIAN_POINT('Ctrl Pts',(-18.8454924744056,12.6320194174368,122.296174468199)) ;
#33554=CARTESIAN_POINT('Ctrl Pts',(-18.8454079345044,12.6320150845467,122.29621719382)) ;
#33555=CARTESIAN_POINT('Ctrl Pts',(-18.8453659955881,12.632012934995,122.296238392297)) ;
#33556=CARTESIAN_POINT('Ctrl Pts',(-18.8452827539264,12.6320086683532,122.296280473587)) ;
#33557=CARTESIAN_POINT('Ctrl Pts',(-18.8452414513663,12.6320065512747,122.296301356216)) ;
#33558=CARTESIAN_POINT('Ctrl Pts',(-18.8451112824266,12.6319998788775,122.296367178882)) ;
#33559=CARTESIAN_POINT('Ctrl Pts',(-18.8450224204141,12.6319953235254,122.296412127165)) ;
#33560=CARTESIAN_POINT('Ctrl Pts',(-18.8448453327161,12.6319862447871,122.296501728442)) ;
#33561=CARTESIAN_POINT('Ctrl Pts',(-18.8447571069507,12.6319817214013,122.296546381289)) ;
#33562=CARTESIAN_POINT('Ctrl Pts',(-18.8445812650707,12.6319727052414,122.296635404637)) ;
#33563=CARTESIAN_POINT('Ctrl Pts',(-18.8444936487542,12.6319682124613,122.296679775063)) ;
#33564=CARTESIAN_POINT('Ctrl Pts',(-18.8443189985797,12.6319592561309,122.296768246811)) ;
#33565=CARTESIAN_POINT('Ctrl Pts',(-18.8442319648159,12.6319547925897,122.296812347916)) ;
#33566=CARTESIAN_POINT('Ctrl Pts',(-18.8440584536272,12.6319458934097,122.296900293756)) ;
#33567=CARTESIAN_POINT('Ctrl Pts',(-18.8439719760347,12.6319414577663,122.296944138415)) ;
#33568=CARTESIAN_POINT('Ctrl Pts',(-18.8437995508156,12.6319326130407,122.297031584258)) ;
#33569=CARTESIAN_POINT('Ctrl Pts',(-18.8437136030792,12.6319282039566,122.297075185345)) ;
#33570=CARTESIAN_POINT('Ctrl Pts',(-18.8435422113537,12.6319194110155,122.297162156893)) ;
#33571=CARTESIAN_POINT('Ctrl Pts',(-18.8434567672829,12.6319150271577,122.297205527253)) ;
#33572=CARTESIAN_POINT('Ctrl Pts',(-18.8432863571278,12.6319062833578,122.297292049997)) ;
#33573=CARTESIAN_POINT('Ctrl Pts',(-18.8432013908638,12.6319019234098,122.297335202337)) ;
#33574=CARTESIAN_POINT('Ctrl Pts',(-18.8430319099121,12.6318932260836,122.297421302054)) ;
#33575=CARTESIAN_POINT('Ctrl Pts',(-18.8429473953669,12.631888888716,122.297464249232)) ;
#33576=CARTESIAN_POINT('Ctrl Pts',(-18.8427787924205,12.6318802352545,122.297549951172)) ;
#33577=CARTESIAN_POINT('Ctrl Pts',(-18.8426947039215,12.6318759191586,122.297592705865)) ;
#33578=CARTESIAN_POINT('Ctrl Pts',(-18.8425269269947,12.6318673069107,122.297678035739)) ;
#33579=CARTESIAN_POINT('Ctrl Pts',(-18.8424432386552,12.631863010766,122.297720610763)) ;
#33580=CARTESIAN_POINT('Ctrl Pts',(-18.8422762364909,12.6318544371166,122.297805593973)) ;
#33581=CARTESIAN_POINT('Ctrl Pts',(-18.8421929225562,12.6318501596088,122.297848002111)) ;
#33582=CARTESIAN_POINT('Ctrl Pts',(-18.8359759930584,12.6315309480047,122.301013397779)) ;
#33583=CARTESIAN_POINT('Ctrl Pts',(-18.8298682818942,12.6312157651259,122.304186977921)) ;
#33584=CARTESIAN_POINT('Ctrl Pts',(-18.8172837982111,12.6305629803702,122.310858477853)) ;
#33585=CARTESIAN_POINT('Ctrl Pts',(-18.8108110832586,12.6302253536001,122.31436348947)) ;
#33586=CARTESIAN_POINT('Ctrl Pts',(-18.7931089059569,12.6292966963258,122.32415250149)) ;
#33587=CARTESIAN_POINT('Ctrl Pts',(-18.7819449551622,12.6287051223298,122.33055303697)) ;
#33588=CARTESIAN_POINT('Ctrl Pts',(-18.739331492069,12.6264236172791,122.355866416145)) ;
#33589=CARTESIAN_POINT('Ctrl Pts',(-18.7086218185486,12.6247289117547,122.375988294816)) ;
#33590=CARTESIAN_POINT('Ctrl Pts',(-18.6666112199279,12.6223413244011,122.406239020898)) ;
#33591=CARTESIAN_POINT('Ctrl Pts',(-18.6545405745837,12.6216468710371,122.415266684362)) ;
#33592=CARTESIAN_POINT('Ctrl Pts',(-18.6391345846768,12.6207502099447,122.427229351818)) ;
#33593=CARTESIAN_POINT('Ctrl Pts',(-18.6356475495466,12.6205465592115,122.429966874391)) ;
#33594=CARTESIAN_POINT('Ctrl Pts',(-18.6299302728566,12.6202115335793,122.434504631282)) ;
#33595=CARTESIAN_POINT('Ctrl Pts',(-18.6276915315442,12.6200800595681,122.436294086583)) ;
#33596=CARTESIAN_POINT('Ctrl Pts',(-18.6245114773303,12.6198929037464,122.438853919667)) ;
#33597=CARTESIAN_POINT('Ctrl Pts',(-18.6235651061448,12.6198371560234,122.439617994593)) ;
#33598=CARTESIAN_POINT('Ctrl Pts',(-18.6212908234769,12.6197030636183,122.441459679734)) ;
#33599=CARTESIAN_POINT('Ctrl Pts',(-18.6199640046755,12.6196247339192,122.442538636595)) ;
#33600=CARTESIAN_POINT('Ctrl Pts',(-18.6148764975289,12.6193240089442,122.446693124195)) ;
#33601=CARTESIAN_POINT('Ctrl Pts',(-18.6111315416416,12.6191018553758,122.449787841994)) ;
#33602=CARTESIAN_POINT('Ctrl Pts',(-18.5953781676455,12.6181638902404,122.462961256232)) ;
#33603=CARTESIAN_POINT('Ctrl Pts',(-18.583541828003,12.6174504462069,122.473243603067)) ;
#33604=CARTESIAN_POINT('Ctrl Pts',(-18.5483328833257,12.6152953134125,122.505011650978)) ;
#33605=CARTESIAN_POINT('Ctrl Pts',(-18.5255824463411,12.6138570837495,122.527167492912)) ;
#33606=CARTESIAN_POINT('Ctrl Pts',(-18.4953990243446,12.611865868209,122.558889531879)) ;
#33607=CARTESIAN_POINT('Ctrl Pts',(-18.4872244686767,12.6113176320481,122.567733248597)) ;
#33608=CARTESIAN_POINT('Ctrl Pts',(-18.4733022493931,12.6103673277936,122.583238746288)) ;
#33609=CARTESIAN_POINT('Ctrl Pts',(-18.4674947653121,12.6099657237916,122.589845651081)) ;
#33610=CARTESIAN_POINT('Ctrl Pts',(-18.461737832456,12.6095621867674,122.596536159339)) ;
#33611=CARTESIAN_POINT('Ctrl Pts',(-18.4617181500391,12.6095608070475,122.596559035239)) ;
#33612=CARTESIAN_POINT('Ctrl Pts',(-18.461678929959,12.6095580576264,122.596604622137)) ;
#33613=CARTESIAN_POINT('Ctrl Pts',(-18.4616593920997,12.6095566879124,122.59662733334)) ;
#33614=CARTESIAN_POINT('Ctrl Pts',(-18.4616204591511,12.6095539583668,122.596672593077)) ;
#33615=CARTESIAN_POINT('Ctrl Pts',(-18.4616010640651,12.6095525985364,122.596695141584)) ;
#33616=CARTESIAN_POINT('Ctrl Pts',(-18.4615624145393,12.6095498886117,122.596740078328)) ;
#33617=CARTESIAN_POINT('Ctrl Pts',(-18.4615431602748,12.6095485385307,122.596762466339)) ;
#33618=CARTESIAN_POINT('Ctrl Pts',(-18.461504791375,12.6095458480362,122.596807083202)) ;
#33619=CARTESIAN_POINT('Ctrl Pts',(-18.4614856764583,12.609544507604,122.59682931236)) ;
#33620=CARTESIAN_POINT('Ctrl Pts',(-18.4614475841884,12.6095418362648,122.596873613853)) ;
#33621=CARTESIAN_POINT('Ctrl Pts',(-18.4614286068381,12.6095405053589,122.596895686162)) ;
#33622=CARTESIAN_POINT('Ctrl Pts',(-18.4613907879158,12.6095378529499,122.596939675966)) ;
#33623=CARTESIAN_POINT('Ctrl Pts',(-18.4613719464074,12.6095365314521,122.596961593365)) ;
#33624=CARTESIAN_POINT('Ctrl Pts',(-18.4613343977169,12.6095338977599,122.597005274973)) ;
#33625=CARTESIAN_POINT('Ctrl Pts',(-18.46131569052,12.6095325855653,122.597027039178)) ;
#33626=CARTESIAN_POINT('Ctrl Pts',(-18.461278408422,12.6095299703395,122.597070416694)) ;
#33627=CARTESIAN_POINT('Ctrl Pts',(-18.4612598338192,12.6095286673301,122.597092029637)) ;
#33628=CARTESIAN_POINT('Ctrl Pts',(-18.461222814797,12.609526070329,122.597135107026)) ;
#33629=CARTESIAN_POINT('Ctrl Pts',(-18.4612043707521,12.6095247763644,122.597156571015)) ;
#33630=CARTESIAN_POINT('Ctrl Pts',(-18.4611676131826,12.6095221974788,122.59719935004)) ;
#33631=CARTESIAN_POINT('Ctrl Pts',(-18.4611492988601,12.6095209125027,122.597220665985)) ;
#33632=CARTESIAN_POINT('Ctrl Pts',(-18.4611127976523,12.6095183513802,122.59726315245)) ;
#33633=CARTESIAN_POINT('Ctrl Pts',(-18.4610946110612,12.6095170752553,122.597284322607)) ;
#33634=CARTESIAN_POINT('Ctrl Pts',(-18.4610583638588,12.6095145317351,122.597326519134)) ;
#33635=CARTESIAN_POINT('Ctrl Pts',(-18.4610403033948,12.609513264351,122.597347545312)) ;
#33636=CARTESIAN_POINT('Ctrl Pts',(-18.4610043072333,12.6095107382297,122.597389455234)) ;
#33637=CARTESIAN_POINT('Ctrl Pts',(-18.4609863714188,12.609509479485,122.597410339095)) ;
#33638=CARTESIAN_POINT('Ctrl Pts',(-18.4609506232812,12.6095069705552,122.59745196581)) ;
#33639=CARTESIAN_POINT('Ctrl Pts',(-18.4609328107254,12.6095057203545,122.597472708916)) ;
#33640=CARTESIAN_POINT('Ctrl Pts',(-18.4608973071031,12.6095032283744,122.597514056395)) ;
#33641=CARTESIAN_POINT('Ctrl Pts',(-18.4608796160897,12.6095019865993,122.597534660688)) ;
#33642=CARTESIAN_POINT('Ctrl Pts',(-18.4608443546439,12.6094995114089,122.597575731545)) ;
#33643=CARTESIAN_POINT('Ctrl Pts',(-18.460826783901,12.6094982779724,122.597596198451)) ;
#33644=CARTESIAN_POINT('Ctrl Pts',(-18.4607917613206,12.6094958193435,122.597636996433)) ;
#33645=CARTESIAN_POINT('Ctrl Pts',(-18.4607743094319,12.6094945941482,122.597657327549)) ;
#33646=CARTESIAN_POINT('Ctrl Pts',(-18.4607395224066,12.6094921518525,122.597697856404)) ;
#33647=CARTESIAN_POINT('Ctrl Pts',(-18.460722187613,12.6094909347769,122.597718053725)) ;
#33648=CARTESIAN_POINT('Ctrl Pts',(-18.4606876341617,12.6094885086794,122.597758315657)) ;
#33649=CARTESIAN_POINT('Ctrl Pts',(-18.4606704153043,12.6094872996442,122.597778380482)) ;
#33650=CARTESIAN_POINT('Ctrl Pts',(-18.4606360920355,12.6094848895107,122.597818379339)) ;
#33651=CARTESIAN_POINT('Ctrl Pts',(-18.4606189876851,12.6094836884174,122.597838313282)) ;
#33652=CARTESIAN_POINT('Ctrl Pts',(-18.4605848914725,12.6094812940323,122.597878052607)) ;
#33653=CARTESIAN_POINT('Ctrl Pts',(-18.4605678998635,12.6094801007589,122.597897857676)) ;
#33654=CARTESIAN_POINT('Ctrl Pts',(-18.4605340293663,12.6094777220318,122.59793733893)) ;
#33655=CARTESIAN_POINT('Ctrl Pts',(-18.4605171498181,12.6094765365324,122.597957015869)) ;
#33656=CARTESIAN_POINT('Ctrl Pts',(-18.4604835004398,12.6094741731442,122.597996244315)) ;
#33657=CARTESIAN_POINT('Ctrl Pts',(-18.4604667310949,12.6094729952902,122.59801579524)) ;
#33658=CARTESIAN_POINT('Ctrl Pts',(-18.4604333012486,12.6094706471332,122.59805477263)) ;
#33659=CARTESIAN_POINT('Ctrl Pts',(-18.4604166409078,12.6094694768422,122.598074198893)) ;
#33660=CARTESIAN_POINT('Ctrl Pts',(-18.4603834273502,12.6094671436922,122.598112928916)) ;
#33661=CARTESIAN_POINT('Ctrl Pts',(-18.4603668743855,12.6094659808515,122.598132232368)) ;
#33662=CARTESIAN_POINT('Ctrl Pts',(-18.4603338755982,12.6094636626054,122.598170716702)) ;
#33663=CARTESIAN_POINT('Ctrl Pts',(-18.4603174292141,12.609462507161,122.598189898225)) ;
#33664=CARTESIAN_POINT('Ctrl Pts',(-18.460284641383,12.6094602035543,122.598228141227)) ;
#33665=CARTESIAN_POINT('Ctrl Pts',(-18.4602683000927,12.6094590554035,122.59824720251)) ;
#33666=CARTESIAN_POINT('Ctrl Pts',(-18.460235720693,12.6094567662621,122.598285207037)) ;
#33667=CARTESIAN_POINT('Ctrl Pts',(-18.4602194828837,12.6094556252932,122.598304149917)) ;
#33668=CARTESIAN_POINT('Ctrl Pts',(-18.4601871105868,12.6094533505273,122.598341917431)) ;
#33669=CARTESIAN_POINT('Ctrl Pts',(-18.4601709755477,12.609452216692,122.598360742694)) ;
#33670=CARTESIAN_POINT('Ctrl Pts',(-18.4601388064741,12.6094499560322,122.598398277636)) ;
#33671=CARTESIAN_POINT('Ctrl Pts',(-18.4601227726865,12.6094488292255,122.598416987011)) ;
#33672=CARTESIAN_POINT('Ctrl Pts',(-18.4600908048319,12.6094465825341,122.598454291634)) ;
#33673=CARTESIAN_POINT('Ctrl Pts',(-18.4600748709927,12.609445462666,122.598472886602)) ;
#33674=CARTESIAN_POINT('Ctrl Pts',(-18.4600431020616,12.6094432297849,122.598509963503)) ;
#33675=CARTESIAN_POINT('Ctrl Pts',(-18.4600272669724,12.6094421167727,122.598528445419)) ;
#33676=CARTESIAN_POINT('Ctrl Pts',(-18.4599956945988,12.6094398975388,122.598565297278)) ;
#33677=CARTESIAN_POINT('Ctrl Pts',(-18.4599799571594,12.6094387913067,122.598583667388)) ;
#33678=CARTESIAN_POINT('Ctrl Pts',(-18.459948578622,12.6094365855317,122.598620297301)) ;
#33679=CARTESIAN_POINT('Ctrl Pts',(-18.4599329375119,12.6094354859884,122.598638557106)) ;
#33680=CARTESIAN_POINT('Ctrl Pts',(-18.4599017508851,12.60943329354,122.598674967243)) ;
#33681=CARTESIAN_POINT('Ctrl Pts',(-18.4598862051093,12.6094322006171,122.598693117866)) ;
#33682=CARTESIAN_POINT('Ctrl Pts',(-18.4598552076536,12.6094300213056,122.598729311349)) ;
#33683=CARTESIAN_POINT('Ctrl Pts',(-18.4598397560122,12.6094289349202,122.598747354152)) ;
#33684=CARTESIAN_POINT('Ctrl Pts',(-18.4598089454057,12.6094267685853,122.598783333616)) ;
#33685=CARTESIAN_POINT('Ctrl Pts',(-18.4597935866557,12.6094256886514,122.598801270014)) ;
#33686=CARTESIAN_POINT('Ctrl Pts',(-18.4597629607741,12.6094235351465,122.598837037867)) ;
#33687=CARTESIAN_POINT('Ctrl Pts',(-18.4597476937627,12.6094224615845,122.598854869169)) ;
#33688=CARTESIAN_POINT('Ctrl Pts',(-18.459717250441,12.6094203207602,122.598890427866)) ;
#33689=CARTESIAN_POINT('Ctrl Pts',(-18.4597020740995,12.6094192534963,122.598908155284)) ;
#33690=CARTESIAN_POINT('Ctrl Pts',(-18.4596718109145,12.609417125185,122.598943507583)) ;
#33691=CARTESIAN_POINT('Ctrl Pts',(-18.4596567240353,12.6094160641356,122.598961132494)) ;
#33692=CARTESIAN_POINT('Ctrl Pts',(-18.4596266391364,12.6094139482099,122.598996280487)) ;
#33693=CARTESIAN_POINT('Ctrl Pts',(-18.4596116408026,12.6094128933119,122.599013803925)) ;
#33694=CARTESIAN_POINT('Ctrl Pts',(-18.4595817314313,12.6094107895803,122.599048750767)) ;
#33695=CARTESIAN_POINT('Ctrl Pts',(-18.4595668203246,12.6094097407422,122.599066174239)) ;
#33696=CARTESIAN_POINT('Ctrl Pts',(-18.4595370854242,12.6094076491331,122.599100921096)) ;
#33697=CARTESIAN_POINT('Ctrl Pts',(-18.4595222611085,12.6094066063256,122.599118245078)) ;
#33698=CARTESIAN_POINT('Ctrl Pts',(-18.4594926963092,12.6094045265341,122.59915279699)) ;
#33699=CARTESIAN_POINT('Ctrl Pts',(-18.4594779567372,12.6094034896145,122.599170023842)) ;
#33700=CARTESIAN_POINT('Ctrl Pts',(-18.4594485627125,12.6094014216904,122.599204379956)) ;
#33701=CARTESIAN_POINT('Ctrl Pts',(-18.4594339076772,12.6094003906454,122.599221509888)) ;
#33702=CARTESIAN_POINT('Ctrl Pts',(-18.4594046802912,12.6093983343003,122.599255674974)) ;
#33703=CARTESIAN_POINT('Ctrl Pts',(-18.4593901083494,12.6093973090295,122.59927270964)) ;
#33704=CARTESIAN_POINT('Ctrl Pts',(-18.4593610461059,12.6093952641605,122.599306685385)) ;
#33705=CARTESIAN_POINT('Ctrl Pts',(-18.4593465560063,12.6093942445771,122.599323626217)) ;
#33706=CARTESIAN_POINT('Ctrl Pts',(-18.4593176579707,12.6093922111209,122.599357413651)) ;
#33707=CARTESIAN_POINT('Ctrl Pts',(-18.4593032493365,12.6093911971995,122.599374261059)) ;
#33708=CARTESIAN_POINT('Ctrl Pts',(-18.4592745117047,12.6093891748908,122.599407864569)) ;
#33709=CARTESIAN_POINT('Ctrl Pts',(-18.4592601830087,12.609388166525,122.599424620308)) ;
#33710=CARTESIAN_POINT('Ctrl Pts',(-18.4592316052021,12.6093861553253,122.599458040511)) ;
#33711=CARTESIAN_POINT('Ctrl Pts',(-18.4592173558299,12.6093851524732,122.599474705271)) ;
#33712=CARTESIAN_POINT('Ctrl Pts',(-18.4591889348375,12.6093831521728,122.599507945629)) ;
#33713=CARTESIAN_POINT('Ctrl Pts',(-18.459174763505,12.6093821547452,122.599524520882)) ;
#33714=CARTESIAN_POINT('Ctrl Pts',(-18.4591464981643,12.6093801652645,122.599557582698)) ;
#33715=CARTESIAN_POINT('Ctrl Pts',(-18.4591324040815,12.6093791732067,122.599574069339)) ;
#33716=CARTESIAN_POINT('Ctrl Pts',(-18.4591042920639,12.6093771943841,122.599606955279)) ;
#33717=CARTESIAN_POINT('Ctrl Pts',(-18.4590902742304,12.6093762076268,122.599623354451)) ;
#33718=CARTESIAN_POINT('Ctrl Pts',(-18.4590623136088,12.6093742393287,122.599656066715)) ;
#33719=CARTESIAN_POINT('Ctrl Pts',(-18.459048370972,12.6093732577989,122.599672379621)) ;
#33720=CARTESIAN_POINT('Ctrl Pts',(-18.4590205603283,12.6093712999276,122.599704919812)) ;
#33721=CARTESIAN_POINT('Ctrl Pts',(-18.4590066922013,12.609370323578,122.59972114723)) ;
#33722=CARTESIAN_POINT('Ctrl Pts',(-18.4589790287884,12.6093683759421,122.59975351851)) ;
#33723=CARTESIAN_POINT('Ctrl Pts',(-18.458965233855,12.6093674046811,122.599769661951)) ;
#33724=CARTESIAN_POINT('Ctrl Pts',(-18.458937717021,12.6093654672368,122.59980186503)) ;
#33725=CARTESIAN_POINT('Ctrl Pts',(-18.4589239947938,12.609364501031,122.59981792504)) ;
#33726=CARTESIAN_POINT('Ctrl Pts',(-18.4588966214556,12.6093625735632,122.599849963474)) ;
#33727=CARTESIAN_POINT('Ctrl Pts',(-18.4588829706057,12.60936161232,122.599865941583)) ;
#33728=CARTESIAN_POINT('Ctrl Pts',(-18.4588557401595,12.6093596947882,122.599897816027)) ;
#33729=CARTESIAN_POINT('Ctrl Pts',(-18.4588421601709,12.6093587384723,122.599913712813)) ;
#33730=CARTESIAN_POINT('Ctrl Pts',(-18.4588150699696,12.6093568306919,122.599945426317)) ;
#33731=CARTESIAN_POINT('Ctrl Pts',(-18.4588015598415,12.6093558792338,122.599961242927)) ;
#33732=CARTESIAN_POINT('Ctrl Pts',(-18.4587746080911,12.6093539810804,122.59999279754)) ;
#33733=CARTESIAN_POINT('Ctrl Pts',(-18.4587611666923,12.6093530344013,122.600008535274)) ;
#33734=CARTESIAN_POINT('Ctrl Pts',(-18.4587343524859,12.609351145813,122.600039932012)) ;
#33735=CARTESIAN_POINT('Ctrl Pts',(-18.4587209792818,12.6093502038762,122.600055591471)) ;
#33736=CARTESIAN_POINT('Ctrl Pts',(-18.4586943003721,12.6093483246964,122.600086832916)) ;
#33737=CARTESIAN_POINT('Ctrl Pts',(-18.4586809946577,12.6093473874531,122.600102414904)) ;
#33738=CARTESIAN_POINT('Ctrl Pts',(-18.4586544482189,12.6093455174846,122.600133504319)) ;
#33739=CARTESIAN_POINT('Ctrl Pts',(-18.4586412083282,12.6093445848184,122.600149010763)) ;
#33740=CARTESIAN_POINT('Ctrl Pts',(-18.4586147950053,12.6093427241084,122.600179947347)) ;
#33741=CARTESIAN_POINT('Ctrl Pts',(-18.4586016208327,12.6093417960127,122.600195378348)) ;
#33742=CARTESIAN_POINT('Ctrl Pts',(-18.4585753373632,12.6093399443331,122.600226165877)) ;
#33743=CARTESIAN_POINT('Ctrl Pts',(-18.4585622279331,12.6093390207401,122.600241522555)) ;
#33744=CARTESIAN_POINT('Ctrl Pts',(-18.4585360728926,12.6093371779922,122.600272162653)) ;
#33745=CARTESIAN_POINT('Ctrl Pts',(-18.4585230273456,12.6093362588421,122.600287445993)) ;
#33746=CARTESIAN_POINT('Ctrl Pts',(-18.4584969991102,12.6093344249132,122.60031794052)) ;
#33747=CARTESIAN_POINT('Ctrl Pts',(-18.4584840165725,12.6093335101454,122.600333151524)) ;
#33748=CARTESIAN_POINT('Ctrl Pts',(-18.4584581136756,12.6093316849338,122.600363502156)) ;
#33749=CARTESIAN_POINT('Ctrl Pts',(-18.4584451933963,12.609330774496,122.600378641682)) ;
#33750=CARTESIAN_POINT('Ctrl Pts',(-18.4584194137448,12.6093289578559,122.600408850828)) ;
#33751=CARTESIAN_POINT('Ctrl Pts',(-18.4584065545495,12.6093280516663,122.600423920233)) ;
#33752=CARTESIAN_POINT('Ctrl Pts',(-18.4583808983417,12.6093262436131,122.60045398762)) ;
#33753=CARTESIAN_POINT('Ctrl Pts',(-18.4583681004896,12.6093253416907,122.600468986579)) ;
#33754=CARTESIAN_POINT('Ctrl Pts',(-18.4583425626679,12.6093235418697,122.600498918094)) ;
#33755=CARTESIAN_POINT('Ctrl Pts',(-18.4583298239715,12.6093226440611,122.600513849151)) ;
#33756=CARTESIAN_POINT('Ctrl Pts',(-18.458304406629,12.6093208526213,122.6005436423)) ;
#33757=CARTESIAN_POINT('Ctrl Pts',(-18.4582917272025,12.6093199589353,122.600558505301)) ;
#33758=CARTESIAN_POINT('Ctrl Pts',(-18.458266426828,12.6093181756307,122.600588164162)) ;
#33759=CARTESIAN_POINT('Ctrl Pts',(-18.4582538056884,12.6093172859988,122.60060296024)) ;
#33760=CARTESIAN_POINT('Ctrl Pts',(-18.4582286214437,12.6093155107718,122.600632485756)) ;
#33761=CARTESIAN_POINT('Ctrl Pts',(-18.458216058113,12.6093146251611,122.600647215453)) ;
#33762=CARTESIAN_POINT('Ctrl Pts',(-18.458190987638,12.6093128578468,122.600676610354)) ;
#33763=CARTESIAN_POINT('Ctrl Pts',(-18.4581784810713,12.6093119761842,122.600691274875)) ;
#33764=CARTESIAN_POINT('Ctrl Pts',(-18.4581535230788,12.6093102166932,122.600720540633)) ;
#33765=CARTESIAN_POINT('Ctrl Pts',(-18.4581410721763,12.609309338902,122.60073514125)) ;
#33766=CARTESIAN_POINT('Ctrl Pts',(-18.4581162264057,12.6093075872175,122.600764278134)) ;
#33767=CARTESIAN_POINT('Ctrl Pts',(-18.4581038309577,12.6093067132835,122.600778815075)) ;
#33768=CARTESIAN_POINT('Ctrl Pts',(-18.4580790947115,12.6093049692166,122.600807826213)) ;
#33769=CARTESIAN_POINT('Ctrl Pts',(-18.4580667538103,12.6093040990766,122.600822300525)) ;
#33770=CARTESIAN_POINT('Ctrl Pts',(-18.4580421260732,12.6093023625571,122.600851187072)) ;
#33771=CARTESIAN_POINT('Ctrl Pts',(-18.4580298390942,12.6093014961677,122.600865599469)) ;
#33772=CARTESIAN_POINT('Ctrl Pts',(-18.4580053181317,12.6092997670746,122.600894363426)) ;
#33773=CARTESIAN_POINT('Ctrl Pts',(-18.4579930842709,12.6092989043797,122.600908714835)) ;
#33774=CARTESIAN_POINT('Ctrl Pts',(-18.4579686688931,12.6092971826304,122.600937357563)) ;
#33775=CARTESIAN_POINT('Ctrl Pts',(-18.4579564875071,12.6092963235854,122.600951648722)) ;
#33776=CARTESIAN_POINT('Ctrl Pts',(-18.4579321755381,12.6092946090277,122.60098017274)) ;
#33777=CARTESIAN_POINT('Ctrl Pts',(-18.4579200453207,12.609293753541,122.600994405165)) ;
#33778=CARTESIAN_POINT('Ctrl Pts',(-18.4578958375331,12.6092920462307,122.601022809534)) ;
#33779=CARTESIAN_POINT('Ctrl Pts',(-18.4578837587607,12.6092911943226,122.601036982884)) ;
#33780=CARTESIAN_POINT('Ctrl Pts',(-18.4578596512629,12.6092894939864,122.601065272138)) ;
#33781=CARTESIAN_POINT('Ctrl Pts',(-18.4578476226887,12.6092886455694,122.60107938786)) ;
#33782=CARTESIAN_POINT('Ctrl Pts',(-18.4578236156322,12.6092869522193,122.601107561791)) ;
#33783=CARTESIAN_POINT('Ctrl Pts',(-18.4578116370117,12.6092861072768,122.601121620156)) ;
#33784=CARTESIAN_POINT('Ctrl Pts',(-18.457787727346,12.6092844206989,122.601149682311)) ;
#33785=CARTESIAN_POINT('Ctrl Pts',(-18.4577757971843,12.609283579126,122.601163685059)) ;
#33786=CARTESIAN_POINT('Ctrl Pts',(-18.4577519858381,12.6092818993868,122.601191634319)) ;
#33787=CARTESIAN_POINT('Ctrl Pts',(-18.4577401041467,12.6092810611849,122.601205581421)) ;
#33788=CARTESIAN_POINT('Ctrl Pts',(-18.4577163882053,12.6092793880801,122.601233421177)) ;
#33789=CARTESIAN_POINT('Ctrl Pts',(-18.4577045541045,12.6092785531878,122.60124731365)) ;
#33790=CARTESIAN_POINT('Ctrl Pts',(-18.4576809326251,12.6092768866519,122.601275044979)) ;
#33791=CARTESIAN_POINT('Ctrl Pts',(-18.4576691454202,12.6092760550207,122.601288883625)) ;
#33792=CARTESIAN_POINT('Ctrl Pts',(-18.457645616997,12.6092743949557,122.601316508148)) ;
#33793=CARTESIAN_POINT('Ctrl Pts',(-18.4576338759057,12.609273566531,122.601330293871)) ;
#33794=CARTESIAN_POINT('Ctrl Pts',(-18.4576104398768,12.6092719128912,122.601357812337)) ;
#33795=CARTESIAN_POINT('Ctrl Pts',(-18.4575987446434,12.6092710876554,122.601371545423)) ;
#33796=CARTESIAN_POINT('Ctrl Pts',(-18.4575753983673,12.6092694402556,122.601398960906)) ;
#33797=CARTESIAN_POINT('Ctrl Pts',(-18.4575637477879,12.6092686181244,122.601412642755)) ;
#33798=CARTESIAN_POINT('Ctrl Pts',(-18.4575404915852,12.6092669769882,122.601439954852)) ;
#33799=CARTESIAN_POINT('Ctrl Pts',(-18.4575288855393,12.6092661579536,122.601453585591)) ;
#33800=CARTESIAN_POINT('Ctrl Pts',(-18.4575057165708,12.6092645228817,122.601480797608)) ;
#33801=CARTESIAN_POINT('Ctrl Pts',(-18.4574941538756,12.6092637068607,122.601494378615)) ;
#33802=CARTESIAN_POINT('Ctrl Pts',(-18.4574710725384,12.6092620778821,122.60152149006)) ;
#33803=CARTESIAN_POINT('Ctrl Pts',(-18.4574595531777,12.6092612648741,122.601535021339)) ;
#33804=CARTESIAN_POINT('Ctrl Pts',(-18.4574365566691,12.6092596417921,122.601562035478)) ;
#33805=CARTESIAN_POINT('Ctrl Pts',(-18.4574250796714,12.6092588317289,122.601575518157)) ;
#33806=CARTESIAN_POINT('Ctrl Pts',(-18.4574021675679,12.6092572145145,122.601602435463)) ;
#33807=CARTESIAN_POINT('Ctrl Pts',(-18.457390732468,12.6092564073639,122.601615870077)) ;
#33808=CARTESIAN_POINT('Ctrl Pts',(-18.4573679031169,12.6092547959015,122.601642692465)) ;
#33809=CARTESIAN_POINT('Ctrl Pts',(-18.4573565091921,12.6092539916129,122.601656079851)) ;
#33810=CARTESIAN_POINT('Ctrl Pts',(-18.457333761452,12.6092523858228,122.601682808639)) ;
#33811=CARTESIAN_POINT('Ctrl Pts',(-18.4573224079669,12.6092515843448,122.601696149648)) ;
#33812=CARTESIAN_POINT('Ctrl Pts',(-18.4572997407641,12.6092499841521,122.601722786072)) ;
#33813=CARTESIAN_POINT('Ctrl Pts',(-18.4572884270274,12.6092491854363,122.601736081506)) ;
#33814=CARTESIAN_POINT('Ctrl Pts',(-18.4572658399085,12.60924759081,122.601762626076)) ;
#33815=CARTESIAN_POINT('Ctrl Pts',(-18.4572545659102,12.6092467948561,122.601775875933)) ;
#33816=CARTESIAN_POINT('Ctrl Pts',(-18.4572320558713,12.609245205585,122.601802332156)) ;
#33817=CARTESIAN_POINT('Ctrl Pts',(-18.4572208203674,12.6092444123058,122.601815537888)) ;
#33818=CARTESIAN_POINT('Ctrl Pts',(-18.4571983879089,12.609242828426,122.601841905153)) ;
#33819=CARTESIAN_POINT('Ctrl Pts',(-18.4571871907465,12.609242037811,122.601855066927)) ;
#33820=CARTESIAN_POINT('Ctrl Pts',(-18.4571648332459,12.6092404591383,122.601881348295)) ;
#33821=CARTESIAN_POINT('Ctrl Pts',(-18.4571536732682,12.6092396711063,122.601894467461)) ;
#33822=CARTESIAN_POINT('Ctrl Pts',(-18.4571313915593,12.6092380977004,122.601920661929)) ;
#33823=CARTESIAN_POINT('Ctrl Pts',(-18.4571202690711,12.6092373122732,122.601933738118)) ;
#33824=CARTESIAN_POINT('Ctrl Pts',(-18.4570980593876,12.609235743869,122.601959850092)) ;
#33825=CARTESIAN_POINT('Ctrl Pts',(-18.4570869729658,12.6092349609467,122.601972884965)) ;
#33826=CARTESIAN_POINT('Ctrl Pts',(-18.4570648359499,12.6092333975903,122.60199891367)) ;
#33827=CARTESIAN_POINT('Ctrl Pts',(-18.4570537851656,12.6092326171429,122.602011907722)) ;
#33828=CARTESIAN_POINT('Ctrl Pts',(-18.4570317199976,12.6092310587773,122.602037854101)) ;
#33829=CARTESIAN_POINT('Ctrl Pts',(-18.4570207049007,12.6092302808088,122.602050807262)) ;
#33830=CARTESIAN_POINT('Ctrl Pts',(-18.4569987083611,12.6092287272073,122.60207667508)) ;
#33831=CARTESIAN_POINT('Ctrl Pts',(-18.4569877275509,12.6092279516191,122.602089588988)) ;
#33832=CARTESIAN_POINT('Ctrl Pts',(-18.4569658004547,12.60922640284,122.602115377267)) ;
#33833=CARTESIAN_POINT('Ctrl Pts',(-18.4569548536685,12.6092256296139,122.602128252221)) ;
#33834=CARTESIAN_POINT('Ctrl Pts',(-18.4569329949719,12.6092240855844,122.602153962168)) ;
#33835=CARTESIAN_POINT('Ctrl Pts',(-18.4569220823415,12.6092233147302,122.602166798004)) ;
#33836=CARTESIAN_POINT('Ctrl Pts',(-18.4569002884575,12.6092217751975,122.60219243382)) ;
#33837=CARTESIAN_POINT('Ctrl Pts',(-18.4568894083333,12.6092210065989,122.602205232468)) ;
#33838=CARTESIAN_POINT('Ctrl Pts',(-18.4568676808509,12.609219471676,122.602230792264)) ;
#33839=CARTESIAN_POINT('Ctrl Pts',(-18.4568568332239,12.6092187053329,122.602243553726)) ;
#33840=CARTESIAN_POINT('Ctrl Pts',(-18.4568351700342,12.6092171748715,122.602269039965)) ;
#33841=CARTESIAN_POINT('Ctrl Pts',(-18.4568243544449,12.6092164107516,122.602281764772)) ;
#33842=CARTESIAN_POINT('Ctrl Pts',(-18.4568027537335,12.6092148846244,122.602307179571)) ;
#33843=CARTESIAN_POINT('Ctrl Pts',(-18.4567919690989,12.6092141226515,122.602319868988)) ;
#33844=CARTESIAN_POINT('Ctrl Pts',(-18.4567704313574,12.6092126008937,122.602345211751)) ;
#33845=CARTESIAN_POINT('Ctrl Pts',(-18.4567596776703,12.6092118410679,122.602357865778)) ;
#33846=CARTESIAN_POINT('Ctrl Pts',(-18.4567382008342,12.6092103235344,122.602383138917)) ;
#33847=CARTESIAN_POINT('Ctrl Pts',(-18.4567274776408,12.6092095658237,122.602395758079)) ;
#33848=CARTESIAN_POINT('Ctrl Pts',(-18.4567060599776,12.6092080523927,122.602420963616)) ;
#33849=CARTESIAN_POINT('Ctrl Pts',(-18.4566953662781,12.6092072967269,122.602433549082)) ;
#33850=CARTESIAN_POINT('Ctrl Pts',(-18.4566740075616,12.609205787383,122.602458687266)) ;
#33851=CARTESIAN_POINT('Ctrl Pts',(-18.4566633427467,12.6092050337193,122.602471239744)) ;
#33852=CARTESIAN_POINT('Ctrl Pts',(-18.4566420426704,12.6092035284416,122.60249631092)) ;
#33853=CARTESIAN_POINT('Ctrl Pts',(-18.4566314068469,12.6092027767879,122.602508830277)) ;
#33854=CARTESIAN_POINT('Ctrl Pts',(-18.4566101622527,12.6092012753537,122.602533838146)) ;
#33855=CARTESIAN_POINT('Ctrl Pts',(-18.4565995540587,12.609200525614,122.602546325977)) ;
#33856=CARTESIAN_POINT('Ctrl Pts',(-18.45657836624,12.6091990281154,122.602571269001)) ;
#33857=CARTESIAN_POINT('Ctrl Pts',(-18.4565677858606,12.6091982803032,122.60258372508)) ;
#33858=CARTESIAN_POINT('Ctrl Pts',(-18.456546652051,12.6091967865452,122.602608606501)) ;
#33859=CARTESIAN_POINT('Ctrl Pts',(-18.4565360986608,12.6091960406023,122.602621031793)) ;
#33860=CARTESIAN_POINT('Ctrl Pts',(-18.4565150183354,12.6091945505484,122.602645852213)) ;
#33861=CARTESIAN_POINT('Ctrl Pts',(-18.4565044913614,12.6091938064347,122.602658247385)) ;
#33862=CARTESIAN_POINT('Ctrl Pts',(-18.4564834638496,12.6091923200381,122.60268300758)) ;
#33863=CARTESIAN_POINT('Ctrl Pts',(-18.4564729630377,12.6091915777359,122.602695372923)) ;
#33864=CARTESIAN_POINT('Ctrl Pts',(-18.4564519865588,12.6091900948712,122.602720074975)) ;
#33865=CARTESIAN_POINT('Ctrl Pts',(-18.4564415111882,12.6091893543297,122.602732411333)) ;
#33866=CARTESIAN_POINT('Ctrl Pts',(-18.4564205848243,12.6091878749326,122.602757056309)) ;
#33867=CARTESIAN_POINT('Ctrl Pts',(-18.456410134092,12.6091871360954,122.602769364619)) ;
#33868=CARTESIAN_POINT('Ctrl Pts',(-18.4563892581176,12.6091856601858,122.602793952182)) ;
#33869=CARTESIAN_POINT('Ctrl Pts',(-18.4563788322551,12.6091849230696,122.602806232165)) ;
#33870=CARTESIAN_POINT('Ctrl Pts',(-18.4563580034952,12.6091834504235,122.602830766042)) ;
#33871=CARTESIAN_POINT('Ctrl Pts',(-18.456347601324,12.6091827149451,122.60284301908)) ;
#33872=CARTESIAN_POINT('Ctrl Pts',(-18.4563268202517,12.6091812455965,122.602867498701)) ;
#33873=CARTESIAN_POINT('Ctrl Pts',(-18.4563164414381,12.6091805117326,122.602879725179)) ;
#33874=CARTESIAN_POINT('Ctrl Pts',(-18.4562957065655,12.6091790455768,122.602904152283)) ;
#33875=CARTESIAN_POINT('Ctrl Pts',(-18.4562853504939,12.6091783132841,122.602916352922)) ;
#33876=CARTESIAN_POINT('Ctrl Pts',(-18.456264661426,12.6091768502936,122.602940727963)) ;
#33877=CARTESIAN_POINT('Ctrl Pts',(-18.4562543279906,12.6091761195649,122.60295290288)) ;
#33878=CARTESIAN_POINT('Ctrl Pts',(-18.4562336824289,12.6091746595776,122.602977228553)) ;
#33879=CARTESIAN_POINT('Ctrl Pts',(-18.456223370633,12.6091739303426,122.602989378918)) ;
#33880=CARTESIAN_POINT('Ctrl Pts',(-18.4562027687069,12.6091724733682,122.603013655059)) ;
#33881=CARTESIAN_POINT('Ctrl Pts',(-18.4561924782268,12.6091717456042,122.603025781246)) ;
#33882=CARTESIAN_POINT('Ctrl Pts',(-18.4561719189495,12.6091702915734,122.603050009007)) ;
#33883=CARTESIAN_POINT('Ctrl Pts',(-18.4561616496515,12.6091695652712,122.603062111169)) ;
#33884=CARTESIAN_POINT('Ctrl Pts',(-18.4561411309177,12.6091681140354,122.603086293019)) ;
#33885=CARTESIAN_POINT('Ctrl Pts',(-18.4561308819322,12.6091673891337,122.603098372174)) ;
#33886=CARTESIAN_POINT('Ctrl Pts',(-18.4561104034437,12.6091659406723,122.603122508455)) ;
#33887=CARTESIAN_POINT('Ctrl Pts',(-18.4561001742442,12.6091652171341,122.603134565219)) ;
#33888=CARTESIAN_POINT('Ctrl Pts',(-18.4560797352498,12.6091637713943,122.603158656804)) ;
#33889=CARTESIAN_POINT('Ctrl Pts',(-18.4560695255338,12.6091630491984,122.603170691529)) ;
#33890=CARTESIAN_POINT('Ctrl Pts',(-18.4560491242262,12.6091616060528,122.603194740539)) ;
#33891=CARTESIAN_POINT('Ctrl Pts',(-18.4560389330718,12.6091608851341,122.603206754306)) ;
#33892=CARTESIAN_POINT('Ctrl Pts',(-18.4560185697823,12.6091594446066,122.60323076034)) ;
#33893=CARTESIAN_POINT('Ctrl Pts',(-18.4560083971751,12.6091587249643,122.603242753161)) ;
#33894=CARTESIAN_POINT('Ctrl Pts',(-18.4559880696742,12.6091572868975,122.603266718838)) ;
#33895=CARTESIAN_POINT('Ctrl Pts',(-18.4559779148352,12.6091565684767,122.603278691627)) ;
#33896=CARTESIAN_POINT('Ctrl Pts',(-18.4559576228706,12.609155132853,122.603302617234)) ;
#33897=CARTESIAN_POINT('Ctrl Pts',(-18.4559474854854,12.6091544156318,122.603314570357)) ;
#33898=CARTESIAN_POINT('Ctrl Pts',(-18.4559272279107,12.6091529823705,122.603338457238)) ;
#33899=CARTESIAN_POINT('Ctrl Pts',(-18.4559171076743,12.6091522663273,122.60335039105)) ;
#33900=CARTESIAN_POINT('Ctrl Pts',(-18.4558968825211,12.6091508352896,122.603374241516)) ;
#33901=CARTESIAN_POINT('Ctrl Pts',(-18.4558867783399,12.6091501203472,122.603386157302)) ;
#33902=CARTESIAN_POINT('Ctrl Pts',(-18.4525865532531,12.6089166003089,122.60727823614)) ;
#33903=CARTESIAN_POINT('Ctrl Pts',(-18.4493201556422,12.6086836122397,122.611178441831)) ;
#33904=CARTESIAN_POINT('Ctrl Pts',(-18.4427860608728,12.6082137208018,122.61907787582)) ;
#33905=CARTESIAN_POINT('Ctrl Pts',(-18.4395191565058,12.6079768161092,122.623077632859)) ;
#33906=CARTESIAN_POINT('Ctrl Pts',(-18.4310030379767,12.607353995484,122.633637035963)) ;
#33907=CARTESIAN_POINT('Ctrl Pts',(-18.4257950153832,12.6069677676902,122.640229544653)) ;
#33908=CARTESIAN_POINT('Ctrl Pts',(-18.4046821908045,12.6053795869096,122.667516021047)) ;
#33909=CARTESIAN_POINT('Ctrl Pts',(-18.3893610527256,12.6041734218622,122.688653011638)) ;
#33910=CARTESIAN_POINT('Ctrl Pts',(-18.3529129052066,12.6011651823234,122.742401438485)) ;
#33911=CARTESIAN_POINT('Ctrl Pts',(-18.3326229997539,12.5993626216852,122.775547790086)) ;
#33912=CARTESIAN_POINT('Ctrl Pts',(-18.3013519866437,12.5963632708674,122.832424970965)) ;
#33913=CARTESIAN_POINT('Ctrl Pts',(-18.2895120049532,12.5951615783711,122.855652172758)) ;
#33914=CARTESIAN_POINT('Ctrl Pts',(-18.2703914513972,12.593095089258,122.89625208293)) ;
#33915=CARTESIAN_POINT('Ctrl Pts',(-18.2627613193706,12.5922298594008,122.913450412196)) ;
#33916=CARTESIAN_POINT('Ctrl Pts',(-18.2499877366282,12.5907044710171,122.944089752005)) ;
#33917=CARTESIAN_POINT('Ctrl Pts',(-18.2446827567534,12.5900441144143,122.957459646358)) ;
#33918=CARTESIAN_POINT('Ctrl Pts',(-18.2353291203443,12.5888274830707,122.982274097568)) ;
#33919=CARTESIAN_POINT('Ctrl Pts',(-18.2312141630492,12.5882711300283,122.99369182571)) ;
#33920=CARTESIAN_POINT('Ctrl Pts',(-18.2229299205174,12.5871046002402,123.017771759504)) ;
#33921=CARTESIAN_POINT('Ctrl Pts',(-18.2187955958389,12.5864945832314,123.030444419716)) ;
#33922=CARTESIAN_POINT('Ctrl Pts',(-18.2098459446753,12.5851071080092,123.059442132694)) ;
#33923=CARTESIAN_POINT('Ctrl Pts',(-18.2051597522571,12.584330175324,123.075804322379)) ;
#33924=CARTESIAN_POINT('Ctrl Pts',(-18.1854365614143,12.5808139437484,123.150391114535)) ;
#33925=CARTESIAN_POINT('Ctrl Pts',(-18.1742789802543,12.5781077443402,123.209558201588)) ;
#33926=CARTESIAN_POINT('Ctrl Pts',(-18.165247831701,12.5745318941421,123.288253428153)) ;
#33927=CARTESIAN_POINT('Ctrl Pts',(-18.16350681498,12.5736690269321,123.307255619287)) ;
#33928=CARTESIAN_POINT('Ctrl Pts',(-18.1615964095027,12.5724013181765,123.335112169401)) ;
#33929=CARTESIAN_POINT('Ctrl Pts',(-18.1610850246052,12.5719991670501,123.343940371386)) ;
#33930=CARTESIAN_POINT('Ctrl Pts',(-18.1603375499634,12.5712780638727,123.359748000308)) ;
#33931=CARTESIAN_POINT('Ctrl Pts',(-18.1600661919462,12.5709594194692,123.366725395004)) ;
#33932=CARTESIAN_POINT('Ctrl Pts',(-18.1597337725983,12.5704610579918,123.377623699465)) ;
#33933=CARTESIAN_POINT('Ctrl Pts',(-18.1596326747349,12.5702816908487,123.381543257494)) ;
#33934=CARTESIAN_POINT('Ctrl Pts',(-18.1594749622181,12.5699391371406,123.389022887593)) ;
#33935=CARTESIAN_POINT('Ctrl Pts',(-18.1594151137971,12.5697759802535,123.392582854411)) ;
#33936=CARTESIAN_POINT('Ctrl Pts',(-18.1593127468001,12.5694015118614,123.400747354398)) ;
#33937=CARTESIAN_POINT('Ctrl Pts',(-18.1592804598205,12.5691901144887,123.405351959994)) ;
#33938=CARTESIAN_POINT('Ctrl Pts',(-18.1592615668958,12.5686058998872,123.418064265863)) ;
#33939=CARTESIAN_POINT('Ctrl Pts',(-18.1593283983234,12.56823263766,123.426171796609)) ;
#33940=CARTESIAN_POINT('Ctrl Pts',(-18.1603410424638,12.5656339807923,123.482511597288)) ;
#33941=CARTESIAN_POINT('Ctrl Pts',(-18.163999479661,12.5633855848756,123.530653991032)) ;
#33942=CARTESIAN_POINT('Ctrl Pts',(-18.1725008576885,12.5604202766196,123.593851863788)) ;
#33943=CARTESIAN_POINT('Ctrl Pts',(-18.1748574905667,12.5596994256428,123.609200632076)) ;
#33944=CARTESIAN_POINT('Ctrl Pts',(-18.1785726741852,12.5586895171967,123.630717019025)) ;
#33945=CARTESIAN_POINT('Ctrl Pts',(-18.179692897117,12.5583981840394,123.636924189808)) ;
#33946=CARTESIAN_POINT('Ctrl Pts',(-18.1829555265562,12.5575847272444,123.654251083616)) ;
#33947=CARTESIAN_POINT('Ctrl Pts',(-18.1852021322485,12.5570633752392,123.665350590171)) ;
#33948=CARTESIAN_POINT('Ctrl Pts',(-18.1894573506843,12.5561392430665,123.684996896142)) ;
#33949=CARTESIAN_POINT('Ctrl Pts',(-18.1914057643807,12.5557361882895,123.693555926983)) ;
#33950=CARTESIAN_POINT('Ctrl Pts',(-18.1949804564033,12.5550299474947,123.708528437142)) ;
#33951=CARTESIAN_POINT('Ctrl Pts',(-18.1965678028148,12.5547266290454,123.714950843448)) ;
#33952=CARTESIAN_POINT('Ctrl Pts',(-18.2064236114327,12.5529027183308,123.753510660049)) ;
#33953=CARTESIAN_POINT('Ctrl Pts',(-18.2159181742257,12.5513860474914,123.785321078119)) ;
#33954=CARTESIAN_POINT('Ctrl Pts',(-18.2403913060296,12.5479301803482,123.856800295266)) ;
#33955=CARTESIAN_POINT('Ctrl Pts',(-18.256144517483,12.5459920929378,123.896160895776)) ;
#33956=CARTESIAN_POINT('Ctrl Pts',(-18.2864139935278,12.5426776230831,123.961895636907)) ;
#33957=CARTESIAN_POINT('Ctrl Pts',(-18.2999391767815,12.5413037041773,123.988685414957)) ;
#33958=CARTESIAN_POINT('Ctrl Pts',(-18.320906782015,12.5393171539216,124.026746593144)) ;
#33959=CARTESIAN_POINT('Ctrl Pts',(-18.3275883115474,12.5387028867431,124.038425005822)) ;
#33960=CARTESIAN_POINT('Ctrl Pts',(-18.3556361347127,12.536195800442,124.085662894323)) ;
#33961=CARTESIAN_POINT('Ctrl Pts',(-18.3785776511792,12.5343059321058,124.120255989233)) ;
#33962=CARTESIAN_POINT('Ctrl Pts',(-18.4101818565052,12.5318698935927,124.163117873568)) ;
#33963=CARTESIAN_POINT('Ctrl Pts',(-18.4173007033859,12.5313310269654,124.172492369061)) ;
#33964=CARTESIAN_POINT('Ctrl Pts',(-18.4313730475718,12.5302840802971,124.19049006801)) ;
#33965=CARTESIAN_POINT('Ctrl Pts',(-18.4383108759122,12.5297761075774,124.199124157621)) ;
#33966=CARTESIAN_POINT('Ctrl Pts',(-18.4533915502747,12.5286888169279,124.217389407441)) ;
#33967=CARTESIAN_POINT('Ctrl Pts',(-18.4615672703638,12.5281094294142,124.226991849584)) ;
#33968=CARTESIAN_POINT('Ctrl Pts',(-18.4845192563594,12.5265097938742,124.253137051531)) ;
#33969=CARTESIAN_POINT('Ctrl Pts',(-18.4995926633929,12.5254888445002,124.269412760923)) ;
#33970=CARTESIAN_POINT('Ctrl Pts',(-18.5195792903258,12.5241721058226,124.289873429297)) ;
#33971=CARTESIAN_POINT('Ctrl Pts',(-18.5241028558643,12.5238764342211,124.294433437138)) ;
#33972=CARTESIAN_POINT('Ctrl Pts',(-18.5405636894689,12.5228089620947,124.310773049197)) ;
#33973=CARTESIAN_POINT('Ctrl Pts',(-18.5527026030115,12.5220375731304,124.322347023014)) ;
#33974=CARTESIAN_POINT('Ctrl Pts',(-18.5700761768795,12.5209559049256,124.338257046934)) ;
#33975=CARTESIAN_POINT('Ctrl Pts',(-18.5751188771855,12.5206445121482,124.342799994797)) ;
#33976=CARTESIAN_POINT('Ctrl Pts',(-18.5843306904589,12.5200803581075,124.35096394748)) ;
#33977=CARTESIAN_POINT('Ctrl Pts',(-18.5884872763372,12.5198274973713,124.354598827182)) ;
#33978=CARTESIAN_POINT('Ctrl Pts',(-18.592727570617,12.5195712806371,124.358257611463)) ;
#33979=CARTESIAN_POINT('Ctrl Pts',(-18.5927873260139,12.5195676703064,124.358309162189)) ;
#33980=CARTESIAN_POINT('Ctrl Pts',(-18.592910094574,12.5195602535262,124.358415053825)) ;
#33981=CARTESIAN_POINT('Ctrl Pts',(-18.5929731084797,12.5195564470705,124.358469394273)) ;
#33982=CARTESIAN_POINT('Ctrl Pts',(-18.5931026313235,12.5195486238256,124.358581066583)) ;
#33983=CARTESIAN_POINT('Ctrl Pts',(-18.5931691408466,12.5195446070449,124.358638397704)) ;
#33984=CARTESIAN_POINT('Ctrl Pts',(-18.5974290272613,12.5192873625404,124.362309631823)) ;
#33985=CARTESIAN_POINT('Ctrl Pts',(-18.6016463663815,12.5190343856636,124.365895652304)) ;
#33986=CARTESIAN_POINT('Ctrl Pts',(-18.6135298933015,12.5183260590913,124.375865007776)) ;
#33987=CARTESIAN_POINT('Ctrl Pts',(-18.6212488855807,12.5178711532404,124.382184767406)) ;
#33988=CARTESIAN_POINT('Ctrl Pts',(-18.6555580665324,12.515869903977,124.409595289082)) ;
#33989=CARTESIAN_POINT('Ctrl Pts',(-18.6829251267248,12.5143270073461,124.429690436628)) ;
#33990=CARTESIAN_POINT('Ctrl Pts',(-18.7226073663886,12.5121443943146,124.456412198331)) ;
#33991=CARTESIAN_POINT('Ctrl Pts',(-18.7342675376822,12.5115094511746,124.463984470882)) ;
#33992=CARTESIAN_POINT('Ctrl Pts',(-18.7525659017382,12.5105219566522,124.475438291917)) ;
#33993=CARTESIAN_POINT('Ctrl Pts',(-18.7591177055339,12.510170121583,124.479455762419)) ;
#33994=CARTESIAN_POINT('Ctrl Pts',(-18.7723131984089,12.5094648408645,124.487380535072)) ;
#33995=CARTESIAN_POINT('Ctrl Pts',(-18.7789568118582,12.5091114085974,124.491287323184)) ;
#33996=CARTESIAN_POINT('Ctrl Pts',(-18.7928288430077,12.5083767482813,124.499273066317)) ;
#33997=CARTESIAN_POINT('Ctrl Pts',(-18.8000626144571,12.5079954898734,124.503341973614)) ;
#33998=CARTESIAN_POINT('Ctrl Pts',(-18.8178914408251,12.5070601940569,124.513138024327)) ;
#33999=CARTESIAN_POINT('Ctrl Pts',(-18.8285297648535,12.5065058464089,124.51878465749)) ;
#34000=CARTESIAN_POINT('Ctrl Pts',(-18.8636555260427,12.504687503885,124.536783051956)) ;
#34001=CARTESIAN_POINT('Ctrl Pts',(-18.8884680125031,12.5034217123461,124.548482785353)) ;
#34002=CARTESIAN_POINT('Ctrl Pts',(-18.9170795524814,12.5019848010171,124.560840196506)) ;
#34003=CARTESIAN_POINT('Ctrl Pts',(-18.9205206079246,12.5018123569094,124.562308104777)) ;
#34004=CARTESIAN_POINT('Ctrl Pts',(-18.9349243828199,12.5010921092351,124.568376278954)) ;
#34005=CARTESIAN_POINT('Ctrl Pts',(-18.9459458895193,12.5005447913997,124.572835486676)) ;
#34006=CARTESIAN_POINT('Ctrl Pts',(-18.9618279327031,12.4997619912918,124.578999051979)) ;
#34007=CARTESIAN_POINT('Ctrl Pts',(-18.9666379635638,12.4995256926901,124.580831644217)) ;
#34008=CARTESIAN_POINT('Ctrl Pts',(-18.9765575075591,12.4990399327147,124.584540929438)) ;
#34009=CARTESIAN_POINT('Ctrl Pts',(-18.9816682291636,12.4987904909948,124.586414060509)) ;
#34010=CARTESIAN_POINT('Ctrl Pts',(-18.9930455574497,12.4982368851615,124.590499870135)) ;
#34011=CARTESIAN_POINT('Ctrl Pts',(-18.9993179073584,12.4979328146393,124.592696076545)) ;
#34012=CARTESIAN_POINT('Ctrl Pts',(-19.0162415559115,12.4971151278367,124.598470649607)) ;
#34013=CARTESIAN_POINT('Ctrl Pts',(-19.0269240884848,12.496601884366,124.601955595345)) ;
#34014=CARTESIAN_POINT('Ctrl Pts',(-19.0749501033363,12.494305123,124.616909684163)) ;
#34015=CARTESIAN_POINT('Ctrl Pts',(-19.1127718729647,12.4925242973508,124.626768496694)) ;
#34016=CARTESIAN_POINT('Ctrl Pts',(-19.1589462935164,12.490364924625,124.63651963671)) ;
#34017=CARTESIAN_POINT('Ctrl Pts',(-19.1669157852112,12.4899927817394,124.638121598312)) ;
#34018=CARTESIAN_POINT('Ctrl Pts',(-19.1862628250434,12.4890904852428,124.641814615874)) ;
#34019=CARTESIAN_POINT('Ctrl Pts',(-19.1976548641831,12.4885601304442,124.643825688614)) ;
#34020=CARTESIAN_POINT('Ctrl Pts',(-19.2212395008405,12.487463705819,124.647652384872)) ;
#34021=CARTESIAN_POINT('Ctrl Pts',(-19.2334343613903,12.4868976313976,124.649446362685)) ;
#34022=CARTESIAN_POINT('Ctrl Pts',(-19.2663850521429,12.4853700324784,124.653796867446)) ;
#34023=CARTESIAN_POINT('Ctrl Pts',(-19.2871817664673,12.4844079186929,124.65601338391)) ;
#34024=CARTESIAN_POINT('Ctrl Pts',(-19.328721165881,12.4824902465458,124.6593891006)) ;
#34025=CARTESIAN_POINT('Ctrl Pts',(-19.3494568386484,12.4815349858296,124.660555057773)) ;
#34026=CARTESIAN_POINT('Ctrl Pts',(-19.3773598515602,12.4802533046945,124.661427403579)) ;
#34027=CARTESIAN_POINT('Ctrl Pts',(-19.3845095588496,12.4799252384598,124.661589527502)) ;
#34028=CARTESIAN_POINT('Ctrl Pts',(-19.3978908438063,12.4793119461118,124.661778082675)) ;
#34029=CARTESIAN_POINT('Ctrl Pts',(-19.4041219845727,12.4790266301873,124.661819287687)) ;
#34030=CARTESIAN_POINT('Ctrl Pts',(-19.4111976064019,12.4787028504042,124.661813168995)) ;
#34031=CARTESIAN_POINT('Ctrl Pts',(-19.4120420302898,12.4786642129511,124.661811583109)) ;
#34032=CARTESIAN_POINT('Ctrl Pts',(-19.413700226622,12.4785883465893,124.661806788625)) ;
#34033=CARTESIAN_POINT('Ctrl Pts',(-19.4145139988482,12.4785511174707,124.661803641011)) ;
#34034=CARTESIAN_POINT('Ctrl Pts',(-19.4167657493379,12.4784481099324,124.661792732446)) ;
#34035=CARTESIAN_POINT('Ctrl Pts',(-19.4182037184386,12.4783823375982,124.661783284793)) ;
#34036=CARTESIAN_POINT('Ctrl Pts',(-19.4312954648374,12.4777835907201,124.661674677872)) ;
#34037=CARTESIAN_POINT('Ctrl Pts',(-19.4429473575433,12.4772511677643,124.661415025728)) ;
#34038=CARTESIAN_POINT('Ctrl Pts',(-19.4947838962647,12.4748822775592,124.659534333487)) ;
#34039=CARTESIAN_POINT('Ctrl Pts',(-19.5348799973414,12.4730484851251,124.656137491742)) ;
#34040=CARTESIAN_POINT('Ctrl Pts',(-19.5855071166865,12.470710967934,124.649376168536)) ;
#34041=CARTESIAN_POINT('Ctrl Pts',(-19.5962526625424,12.4702136104057,124.647798292927)) ;
#34042=CARTESIAN_POINT('Ctrl Pts',(-19.6189267086288,12.4691611438915,124.644166377784)) ;
#34043=CARTESIAN_POINT('Ctrl Pts',(-19.6308487028074,12.4686059918,124.64207870637)) ;
#34044=CARTESIAN_POINT('Ctrl Pts',(-19.6570835676851,12.4673800285823,124.637090973545)) ;
#34045=CARTESIAN_POINT('Ctrl Pts',(-19.6713797464438,12.466709097,124.634112559026)) ;
#34046=CARTESIAN_POINT('Ctrl Pts',(-19.7036828148005,12.4651861610484,124.626789850256)) ;
#34047=CARTESIAN_POINT('Ctrl Pts',(-19.7216519587391,12.464334056648,124.62229440476)) ;
#34048=CARTESIAN_POINT('Ctrl Pts',(-19.75770732225,12.4626143365884,124.612417882623)) ;
#34049=CARTESIAN_POINT('Ctrl Pts',(-19.775784999438,12.461746942986,124.607023222533)) ;
#34050=CARTESIAN_POINT('Ctrl Pts',(-19.8008073059715,12.4605398074368,124.598935065143)) ;
#34051=CARTESIAN_POINT('Ctrl Pts',(-19.8078604000528,12.4601988218568,124.596585542749)) ;
#34052=CARTESIAN_POINT('Ctrl Pts',(-19.8205519891478,12.4595840127048,124.592231567729)) ;
#34053=CARTESIAN_POINT('Ctrl Pts',(-19.826197844593,12.45931007174,124.590249278334)) ;
#34054=CARTESIAN_POINT('Ctrl Pts',(-19.8329781494603,12.4589804475995,124.587813851763)) ;
#34055=CARTESIAN_POINT('Ctrl Pts',(-19.8341264369782,12.4589246015404,124.587399496702)) ;
#34056=CARTESIAN_POINT('Ctrl Pts',(-19.8360700331839,12.4588300375781,124.586694937977)) ;
#34057=CARTESIAN_POINT('Ctrl Pts',(-19.8368656571794,12.4587913161993,124.586405607349)) ;
#34058=CARTESIAN_POINT('Ctrl Pts',(-19.8476490265035,12.4582663595678,124.582471800163)) ;
#34059=CARTESIAN_POINT('Ctrl Pts',(-19.8575901888211,12.4577806270418,124.578700843971)) ;
#34060=CARTESIAN_POINT('Ctrl Pts',(-19.8996954286532,12.4557138785777,124.562111666141)) ;
#34061=CARTESIAN_POINT('Ctrl Pts',(-19.9313675343519,12.454135113902,124.54808690434)) ;
#34062=CARTESIAN_POINT('Ctrl Pts',(-19.9742945888471,12.4519458704999,124.526904132726)) ;
#34063=CARTESIAN_POINT('Ctrl Pts',(-19.9860787812128,12.451339609491,124.520854336017)) ;
#34064=CARTESIAN_POINT('Ctrl Pts',(-20.0079194981663,12.4502052961452,124.50919941458)) ;
#34065=CARTESIAN_POINT('Ctrl Pts',(-20.0179990712181,12.4496774589668,124.5036404183)) ;
#34066=CARTESIAN_POINT('Ctrl Pts',(-20.0392382977169,12.4485555501177,124.491541199843)) ;
#34067=CARTESIAN_POINT('Ctrl Pts',(-20.050376132214,12.4479614234722,124.484965365511)) ;
#34068=CARTESIAN_POINT('Ctrl Pts',(-20.0819285385337,12.4462612055226,124.465670125176)) ;
#34069=CARTESIAN_POINT('Ctrl Pts',(-20.1020807471657,12.4451543168983,124.452532784703)) ;
#34070=CARTESIAN_POINT('Ctrl Pts',(-20.1354694140684,12.4432847135922,124.429366719317)) ;
#34071=CARTESIAN_POINT('Ctrl Pts',(-20.1489079573111,12.4425220069596,124.419640807127)) ;
#34072=CARTESIAN_POINT('Ctrl Pts',(-20.1674306744609,12.4414569082213,124.40566524036)) ;
#34073=CARTESIAN_POINT('Ctrl Pts',(-20.1726806502959,12.4411534284501,124.401638275377)) ;
#34074=CARTESIAN_POINT('Ctrl Pts',(-20.1821686190583,12.440602129374,124.394240191788)) ;
#34075=CARTESIAN_POINT('Ctrl Pts',(-20.1864171508693,12.4403542164487,124.390882853714)) ;
#34076=CARTESIAN_POINT('Ctrl Pts',(-20.1947162523244,12.4398679201218,124.384236558636)) ;
#34077=CARTESIAN_POINT('Ctrl Pts',(-20.1987682996674,12.4396295378058,124.380949645044)) ;
#34078=CARTESIAN_POINT('Ctrl Pts',(-20.2095128408346,12.4389947417754,124.372121850109)) ;
#34079=CARTESIAN_POINT('Ctrl Pts',(-20.216168347234,12.4385986993679,124.36653639678)) ;
#34080=CARTESIAN_POINT('Ctrl Pts',(-20.2413279731527,12.4370894775508,124.344970835657)) ;
#34081=CARTESIAN_POINT('Ctrl Pts',(-20.2594200714513,12.4359787896424,124.328518466747)) ;
#34082=CARTESIAN_POINT('Ctrl Pts',(-20.2943475365323,12.4337713443,124.294832691494)) ;
#34083=CARTESIAN_POINT('Ctrl Pts',(-20.3111904638408,12.432675097936,124.277622169044)) ;
#34084=CARTESIAN_POINT('Ctrl Pts',(-20.333631552458,12.4311643786801,124.253325409506)) ;
#34085=CARTESIAN_POINT('Ctrl Pts',(-20.3396657453099,12.4307529240648,124.2466490199)) ;
#34086=CARTESIAN_POINT('Ctrl Pts',(-20.3500692061044,12.4300340589982,124.234885455946)) ;
#34087=CARTESIAN_POINT('Ctrl Pts',(-20.3544706145966,12.4297268749925,124.229827191592)) ;
#34088=CARTESIAN_POINT('Ctrl Pts',(-20.363098406707,12.4291185414802,124.219749198019)) ;
#34089=CARTESIAN_POINT('Ctrl Pts',(-20.3673263863814,12.4288174128017,124.214731112212)) ;
#34090=CARTESIAN_POINT('Ctrl Pts',(-20.3765593598748,12.4281530286161,124.203595955381)) ;
#34091=CARTESIAN_POINT('Ctrl Pts',(-20.3815462429687,12.4277896750253,124.197464237233)) ;
#34092=CARTESIAN_POINT('Ctrl Pts',(-20.3941793850878,12.4268574237199,124.18162640335)) ;
#34093=CARTESIAN_POINT('Ctrl Pts',(-20.4017404800292,12.4262880910952,124.171853475638)) ;
#34094=CARTESIAN_POINT('Ctrl Pts',(-20.4274939936011,12.4243085935446,124.137526595876)) ;
#34095=CARTESIAN_POINT('Ctrl Pts',(-20.4449300513644,12.4228956682421,124.112418870795)) ;
#34096=CARTESIAN_POINT('Ctrl Pts',(-20.469207392235,12.4208201469499,124.074570018575)) ;
#34097=CARTESIAN_POINT('Ctrl Pts',(-20.4767761285141,12.4201559539261,124.06230881979)) ;
#34098=CARTESIAN_POINT('Ctrl Pts',(-20.4887980366023,12.4190728407009,124.042058462036)) ;
#34099=CARTESIAN_POINT('Ctrl Pts',(-20.4933784570965,12.4186529411241,124.03414649349)) ;
#34100=CARTESIAN_POINT('Ctrl Pts',(-20.502492205297,12.4178020039793,124.017997899938)) ;
#34101=CARTESIAN_POINT('Ctrl Pts',(-20.5070202293992,12.4173710150697,124.009758946748)) ;
#34102=CARTESIAN_POINT('Ctrl Pts',(-20.5177380695046,12.4163299815716,123.989725179554)) ;
#34103=CARTESIAN_POINT('Ctrl Pts',(-20.5238331377591,12.4157202482998,123.97788097832)) ;
#34104=CARTESIAN_POINT('Ctrl Pts',(-20.549562384813,12.4130639262777,123.925855502576)) ;
#34105=CARTESIAN_POINT('Ctrl Pts',(-20.5672215044172,12.4110196529471,123.884734438593)) ;
#34106=CARTESIAN_POINT('Ctrl Pts',(-20.5912787219728,12.4078209736192,123.819231482994)) ;
#34107=CARTESIAN_POINT('Ctrl Pts',(-20.5992090760481,12.4066713963321,123.795452677033)) ;
#34108=CARTESIAN_POINT('Ctrl Pts',(-20.6134828954529,12.4043947279938,123.747938523882)) ;
#34109=CARTESIAN_POINT('Ctrl Pts',(-20.6198522642245,12.4032681519348,123.724222369372)) ;
#34110=CARTESIAN_POINT('Ctrl Pts',(-20.6278648432713,12.4016775444763,123.690445560328)) ;
#34111=CARTESIAN_POINT('Ctrl Pts',(-20.630089924705,12.4012122315028,123.680528817956)) ;
#34112=CARTESIAN_POINT('Ctrl Pts',(-20.6345985502187,12.4002161936719,123.659221633624)) ;
#34113=CARTESIAN_POINT('Ctrl Pts',(-20.6368447426512,12.3996857949994,123.647824269576)) ;
#34114=CARTESIAN_POINT('Ctrl Pts',(-20.6422802606537,12.398306040833,123.618063151031)) ;
#34115=CARTESIAN_POINT('Ctrl Pts',(-20.6452183096808,12.3974576105,123.599656468766)) ;
#34116=CARTESIAN_POINT('Ctrl Pts',(-20.6519275933222,12.3952029601296,123.550598591595)) ;
#34117=CARTESIAN_POINT('Ctrl Pts',(-20.6549765077723,12.3937969104405,123.51986182271)) ;
#34118=CARTESIAN_POINT('Ctrl Pts',(-20.6575153890148,12.3919190119312,123.478847204014)) ;
#34119=CARTESIAN_POINT('Ctrl Pts',(-20.6580215512615,12.3914517052291,123.468643206792)) ;
#34120=CARTESIAN_POINT('Ctrl Pts',(-20.6586924466314,12.3906279597365,123.450667248269)) ;
#34121=CARTESIAN_POINT('Ctrl Pts',(-20.6589098750464,12.3902717591962,123.442897799713)) ;
#34122=CARTESIAN_POINT('Ctrl Pts',(-20.659207098202,12.389540769035,123.426963657059)) ;
#34123=CARTESIAN_POINT('Ctrl Pts',(-20.6592793849912,12.3891659660142,123.418799189831)) ;
#34124=CARTESIAN_POINT('Ctrl Pts',(-20.6592617171154,12.3883059014497,123.400079272028)) ;
#34125=CARTESIAN_POINT('Ctrl Pts',(-20.6591180570055,12.3878204651731,123.38952449959)) ;
#34126=CARTESIAN_POINT('Ctrl Pts',(-20.6583399274576,12.3864571946517,123.359917895475)) ;
#34127=CARTESIAN_POINT('Ctrl Pts',(-20.6574033270884,12.3855785366258,123.340876944267)) ;
#34128=CARTESIAN_POINT('Ctrl Pts',(-20.6539585003184,12.3833707138074,123.293129342754)) ;
#34129=CARTESIAN_POINT('Ctrl Pts',(-20.6508924846443,12.382041487259,123.264473947319)) ;
#34130=CARTESIAN_POINT('Ctrl Pts',(-20.6459225966224,12.3804176361351,123.229500566442)) ;
#34131=CARTESIAN_POINT('Ctrl Pts',(-20.6449556855264,12.3801184788421,123.223058309291)) ;
#34132=CARTESIAN_POINT('Ctrl Pts',(-20.6430293169588,12.379552562887,123.210873175451)) ;
#34133=CARTESIAN_POINT('Ctrl Pts',(-20.642080010145,12.3792857265701,123.205128882462)) ;
#34134=CARTESIAN_POINT('Ctrl Pts',(-20.6398694252935,12.378689954479,123.192309932808)) ;
#34135=CARTESIAN_POINT('Ctrl Pts',(-20.6385872017436,12.3783611252823,123.185239094201)) ;
#34136=CARTESIAN_POINT('Ctrl Pts',(-20.6322424548513,12.3768086416373,123.151891430073)) ;
#34137=CARTESIAN_POINT('Ctrl Pts',(-20.6263979526738,12.3755875762307,123.125770518323)) ;
#34138=CARTESIAN_POINT('Ctrl Pts',(-20.6148857093288,12.3734802186777,123.081101018021)) ;
#34139=CARTESIAN_POINT('Ctrl Pts',(-20.6096165317935,12.372594938087,123.062459626244)) ;
#34140=CARTESIAN_POINT('Ctrl Pts',(-20.6001020320911,12.3711151039714,123.031561316766)) ;
#34141=CARTESIAN_POINT('Ctrl Pts',(-20.5960984489603,12.3705218271716,123.019243959999)) ;
#34142=CARTESIAN_POINT('Ctrl Pts',(-20.5919008645526,12.3699275081133,123.006981651862)) ;
#34143=CARTESIAN_POINT('Ctrl Pts',(-20.5919008187226,12.3097986802463,123.006981518046)) ;
#34144=CARTESIAN_POINT('Ctrl Pts',(-20.5959679259066,12.3103772675894,123.018862784893)) ;
#34145=CARTESIAN_POINT('Ctrl Pts',(-20.5998545754055,12.3109562954671,123.030800851875)) ;
#34146=CARTESIAN_POINT('Ctrl Pts',(-20.6035607346876,12.31153530454,123.042795421432)) ;
#34147=CARTESIAN_POINT('Ctrl Pts',(-20.6248655183692,12.3148637267982,123.111745968429)) ;
#34148=CARTESIAN_POINT('Ctrl Pts',(-20.640159292875,12.3181590011121,123.182412191089)) ;
#34149=CARTESIAN_POINT('Ctrl Pts',(-20.649270492558,12.3214523073791,123.254003328633)) ;
#34150=CARTESIAN_POINT('Ctrl Pts',(-20.6584395622931,12.3247665311775,123.326049179388)) ;
#34151=CARTESIAN_POINT('Ctrl Pts',(-20.6613122235796,12.3281113715718,123.398756812874)) ;
#34152=CARTESIAN_POINT('Ctrl Pts',(-20.6578559614911,12.331432491669,123.471301175167)) ;
#34153=CARTESIAN_POINT('Ctrl Pts',(-20.6543934482099,12.3347596185333,123.543976745329)) ;
#34154=CARTESIAN_POINT('Ctrl Pts',(-20.6445924883426,12.3380646087419,123.616209428573)) ;
#34155=CARTESIAN_POINT('Ctrl Pts',(-20.6285649359542,12.3414306615,123.687178328985)) ;
#34156=CARTESIAN_POINT('Ctrl Pts',(-20.6126520997966,12.3447726219402,123.757639273811)) ;
#34157=CARTESIAN_POINT('Ctrl Pts',(-20.590661759836,12.3480897793102,123.826588099236)) ;
#34158=CARTESIAN_POINT('Ctrl Pts',(-20.5628388308981,12.351357610961,123.893253990093)) ;
#34159=CARTESIAN_POINT('Ctrl Pts',(-20.5531745685128,12.3524926885286,123.916410310652)) ;
#34160=CARTESIAN_POINT('Ctrl Pts',(-20.5428153628591,12.3536262784784,123.939270123424)) ;
#34161=CARTESIAN_POINT('Ctrl Pts',(-20.5317752294988,12.3547689257512,123.961802575126)) ;
#34162=CARTESIAN_POINT('Ctrl Pts',(-20.5108163442102,12.3569381579818,124.0045787858)) ;
#34163=CARTESIAN_POINT('Ctrl Pts',(-20.4874304463061,12.3591457818808,124.0461201067)) ;
#34164=CARTESIAN_POINT('Ctrl Pts',(-20.4617310904093,12.3613560336666,124.086225487286)) ;
#34165=CARTESIAN_POINT('Ctrl Pts',(-20.4228614531263,12.364698984578,124.146883878986)) ;
#34166=CARTESIAN_POINT('Ctrl Pts',(-20.3788207145505,12.3679748327242,124.204068391805)) ;
#34167=CARTESIAN_POINT('Ctrl Pts',(-20.330098410005,12.3712568822117,124.257142206669)) ;
#34168=CARTESIAN_POINT('Ctrl Pts',(-20.2811120419599,12.37455671964,124.310503669202)) ;
#34169=CARTESIAN_POINT('Ctrl Pts',(-20.227580251143,12.3779005627734,124.359505786526)) ;
#34170=CARTESIAN_POINT('Ctrl Pts',(-20.1701073888366,12.3812115960284,124.403595527009)) ;
#34171=CARTESIAN_POINT('Ctrl Pts',(-20.1123795154289,12.3845373205691,124.447880896747)) ;
#34172=CARTESIAN_POINT('Ctrl Pts',(-20.0508971122197,12.3878420276153,124.487040359335)) ;
#34173=CARTESIAN_POINT('Ctrl Pts',(-19.9863588595697,12.3912102426386,124.520629512979)) ;
#34174=CARTESIAN_POINT('Ctrl Pts',(-19.9308684806042,12.3941062542349,124.549509669914)) ;
#34175=CARTESIAN_POINT('Ctrl Pts',(-19.8732884005457,12.3969908898565,124.574183755512)) ;
#34176=CARTESIAN_POINT('Ctrl Pts',(-19.814101322745,12.3998259425229,124.594444237049)) ;
#34177=CARTESIAN_POINT('Ctrl Pts',(-19.8049052026207,12.4002664353779,124.597592184691)) ;
#34178=CARTESIAN_POINT('Ctrl Pts',(-19.7956726543642,12.4007060969951,124.600632769874)) ;
#34179=CARTESIAN_POINT('Ctrl Pts',(-19.786405553344,12.4011453145424,124.603565372853)) ;
#34180=CARTESIAN_POINT('Ctrl Pts',(-19.7170359751187,12.4044331103635,124.625517591919)) ;
#34181=CARTESIAN_POINT('Ctrl Pts',(-19.645888839699,12.4077540678437,124.641369545238)) ;
#34182=CARTESIAN_POINT('Ctrl Pts',(-19.5737661106502,12.4111439811015,124.650943805026)) ;
#34183=CARTESIAN_POINT('Ctrl Pts',(-19.50230985836,12.4145025686118,124.660429590325)) ;
#34184=CARTESIAN_POINT('Ctrl Pts',(-19.430168452585,12.4177998987068,124.663716935233)) ;
#34185=CARTESIAN_POINT('Ctrl Pts',(-19.3581406945466,12.4210504446412,124.66076815496)) ;
#34186=CARTESIAN_POINT('Ctrl Pts',(-19.2854416744532,12.4243312840098,124.657791893556)) ;
#34187=CARTESIAN_POINT('Ctrl Pts',(-19.2131478831709,12.4276641706043,124.648474605693)) ;
#34188=CARTESIAN_POINT('Ctrl Pts',(-19.1420743743969,12.4310490229632,124.632922593895)) ;
#34189=CARTESIAN_POINT('Ctrl Pts',(-19.071424242274,12.4344137121492,124.617463223629)) ;
#34190=CARTESIAN_POINT('Ctrl Pts',(-19.0022480648928,12.4377416309172,124.595901484794)) ;
#34191=CARTESIAN_POINT('Ctrl Pts',(-18.9353230016292,12.4410246690359,124.568478588955)) ;
#34192=CARTESIAN_POINT('Ctrl Pts',(-18.9096039882164,12.4422863264374,124.557940088258)) ;
#34193=CARTESIAN_POINT('Ctrl Pts',(-18.8842435556656,12.4435427967642,124.546546678268)) ;
#34194=CARTESIAN_POINT('Ctrl Pts',(-18.8592840273916,12.4448018250339,124.53431736011)) ;
#34195=CARTESIAN_POINT('Ctrl Pts',(-18.75389161528,12.4501181124575,124.482678670265)) ;
#34196=CARTESIAN_POINT('Ctrl Pts',(-18.6563002355626,12.4555339951191,124.416456661723)) ;
#34197=CARTESIAN_POINT('Ctrl Pts',(-18.5693811238693,12.4609547040084,124.33760209597)) ;
#34198=CARTESIAN_POINT('Ctrl Pts',(-18.5155204329295,12.4643137250622,124.288738718141)) ;
#34199=CARTESIAN_POINT('Ctrl Pts',(-18.4660255868903,12.4676210838886,124.235267338101)) ;
#34200=CARTESIAN_POINT('Ctrl Pts',(-18.421460314933,12.4709151894271,124.177795834203)) ;
#34201=CARTESIAN_POINT('Ctrl Pts',(-18.3769039711297,12.4742086350285,124.120335844079)) ;
#34202=CARTESIAN_POINT('Ctrl Pts',(-18.3374488791071,12.477526026371,124.059101803663)) ;
#34203=CARTESIAN_POINT('Ctrl Pts',(-18.3035398956969,12.480906710666,123.994786056946)) ;
#34204=CARTESIAN_POINT('Ctrl Pts',(-18.273330930655,12.4839185076417,123.937488198125)) ;
#34205=CARTESIAN_POINT('Ctrl Pts',(-18.2476214510531,12.486897790467,123.877929793882)) ;
#34206=CARTESIAN_POINT('Ctrl Pts',(-18.2266423654683,12.4898239518789,123.816643453356)) ;
#34207=CARTESIAN_POINT('Ctrl Pts',(-18.2243056994885,12.4901498698888,123.80981733568)) ;
#34208=CARTESIAN_POINT('Ctrl Pts',(-18.2220278588499,12.4904755343012,123.802970140349)) ;
#34209=CARTESIAN_POINT('Ctrl Pts',(-18.2198098607987,12.4908011212469,123.796104957352)) ;
#34210=CARTESIAN_POINT('Ctrl Pts',(-18.1974413096866,12.4940846715785,123.72686946064)) ;
#34211=CARTESIAN_POINT('Ctrl Pts',(-18.1811618838124,12.4974253874866,123.655819011934)) ;
#34212=CARTESIAN_POINT('Ctrl Pts',(-18.1711542091949,12.5007987881958,123.58375549571)) ;
#34213=CARTESIAN_POINT('Ctrl Pts',(-18.1612141385254,12.5041494008733,123.512178783703)) ;
#34214=CARTESIAN_POINT('Ctrl Pts',(-18.1574994841532,12.5074328201644,123.439874501978)) ;
#34215=CARTESIAN_POINT('Ctrl Pts',(-18.1600525528208,12.5107289079967,123.367653486248)) ;
#34216=CARTESIAN_POINT('Ctrl Pts',(-18.1626092701643,12.5140297063784,123.295329257047)) ;
#34217=CARTESIAN_POINT('Ctrl Pts',(-18.171441973291,12.5173692988662,123.223364167744)) ;
#34218=CARTESIAN_POINT('Ctrl Pts',(-18.1864509887407,12.5206842314647,123.152568927952)) ;
#34219=CARTESIAN_POINT('Ctrl Pts',(-18.2077946755634,12.5253982570752,123.051894008153)) ;
#34220=CARTESIAN_POINT('Ctrl Pts',(-18.2414891520986,12.5300422781028,122.954240933681)) ;
#34221=CARTESIAN_POINT('Ctrl Pts',(-18.2867692424076,12.5347791480646,122.861826158003)) ;
#34222=CARTESIAN_POINT('Ctrl Pts',(-18.3053018325031,12.5367178913122,122.824001914616)) ;
#34223=CARTESIAN_POINT('Ctrl Pts',(-18.3257344508473,12.538661680911,122.787138435358)) ;
#34224=CARTESIAN_POINT('Ctrl Pts',(-18.347988906045,12.5405951669528,122.751376864801)) ;
#34225=CARTESIAN_POINT('Ctrl Pts',(-18.4246887379185,12.5472589137405,122.62812484965)) ;
#34226=CARTESIAN_POINT('Ctrl Pts',(-18.5222717230523,12.5538432931049,122.519175649303)) ;
#34227=CARTESIAN_POINT('Ctrl Pts',(-18.6363622964908,12.5605176564878,122.429414129616)) ;
#34228=CARTESIAN_POINT('Ctrl Pts',(-18.6934296541356,12.5638561293409,122.384516005324)) ;
#34229=CARTESIAN_POINT('Ctrl Pts',(-18.7543012385188,12.5671710938438,122.34467533864)) ;
#34230=CARTESIAN_POINT('Ctrl Pts',(-18.8182864537173,12.5704815138147,122.310344527998)) ;
#34231=CARTESIAN_POINT('Ctrl Pts',(-18.878035625681,12.5735727724985,122.278286536127)) ;
#34232=CARTESIAN_POINT('Ctrl Pts',(-18.9402928786006,12.5766714230685,122.251143940954)) ;
#34233=CARTESIAN_POINT('Ctrl Pts',(-19.0044431491614,12.5797954008838,122.229184496079)) ;
#34234=CARTESIAN_POINT('Ctrl Pts',(-19.0091190551512,12.5800231072746,122.227583874618)) ;
#34235=CARTESIAN_POINT('Ctrl Pts',(-19.0138047230683,12.580250794863,122.226010895838)) ;
#34236=CARTESIAN_POINT('Ctrl Pts',(-19.0184991675638,12.5804783681921,122.22446588819)) ;
#34237=CARTESIAN_POINT('Ctrl Pts',(-19.087094062903,12.5838036537943,122.201890344265)) ;
#34238=CARTESIAN_POINT('Ctrl Pts',(-19.157516417056,12.5870877342977,122.185301422084)) ;
#34239=CARTESIAN_POINT('Ctrl Pts',(-19.228976203807,12.590400895558,122.174885370676)) ;
#34240=CARTESIAN_POINT('Ctrl Pts',(-19.3005480738815,12.593719253449,122.164452981889)) ;
#34241=CARTESIAN_POINT('Ctrl Pts',(-19.3728909905207,12.5970766281283,122.160252175256)) ;
#34242=CARTESIAN_POINT('Ctrl Pts',(-19.4451903276682,12.6003730862129,122.162330516823)) ;
#34243=CARTESIAN_POINT('Ctrl Pts',(-19.5909202431352,12.6070175808509,122.166519719005)) ;
#34244=CARTESIAN_POINT('Ctrl Pts',(-19.7347890275704,12.6135840949886,122.196169604076)) ;
#34245=CARTESIAN_POINT('Ctrl Pts',(-19.8702966648422,12.6203324938027,122.249938092582)) ;
#34246=CARTESIAN_POINT('Ctrl Pts',(-19.90045071297,12.6218341917639,122.261903009267)) ;
#34247=CARTESIAN_POINT('Ctrl Pts',(-19.9301277965717,12.6233279003994,122.275037368455)) ;
#34248=CARTESIAN_POINT('Ctrl Pts',(-19.9592604445148,12.6248187332792,122.289311373019)) ;
#34249=CARTESIAN_POINT('Ctrl Pts',(-20.0602104252377,12.629984743275,122.338773422894)) ;
#34250=CARTESIAN_POINT('Ctrl Pts',(-20.1540280917424,12.6351103129767,122.401627929583)) ;
#34251=CARTESIAN_POINT('Ctrl Pts',(-20.2381746311039,12.6402255782778,122.476175109484)) ;
#34252=CARTESIAN_POINT('Ctrl Pts',(-20.3467958775309,12.6468286601993,122.572404944483)) ;
#34253=CARTESIAN_POINT('Ctrl Pts',(-20.4378292876924,12.6534583240344,122.686812124415)) ;
#34254=CARTESIAN_POINT('Ctrl Pts',(-20.5071984569157,12.6601281682878,122.814271051483)) ;
#34255=CARTESIAN_POINT('Ctrl Pts',(-20.5408008134123,12.6633590342025,122.876012028835)) ;
#34256=CARTESIAN_POINT('Ctrl Pts',(-20.5691355300788,12.6665486843384,122.940477674066)) ;
#34257=CARTESIAN_POINT('Ctrl Pts',(-20.5919010929731,12.6697683433189,123.006982319198)) ;
#34258=CARTESIAN_POINT('Ctrl Pts',(-20.5445170967909,10.1799890803629,123.023196933748)) ;
#34259=CARTESIAN_POINT('Ctrl Pts',(-20.8283303707622,9.99999999995305,122.926041870788)) ;
#34260=CARTESIAN_POINT('Ctrl Pts',(-20.5894888412031,10.186615931181,123.154521494311)) ;
#34261=CARTESIAN_POINT('Ctrl Pts',(-20.8845408160738,10.0066268507712,123.090165629839)) ;
#34262=CARTESIAN_POINT('Ctrl Pts',(-20.6334208464893,10.199846557662,123.432353270138)) ;
#34263=CARTESIAN_POINT('Ctrl Pts',(-20.9394617691535,10.0198574772522,123.437507823533)) ;
#34264=CARTESIAN_POINT('Ctrl Pts',(-20.5528814488852,10.2198221789206,123.849407494597)) ;
#34265=CARTESIAN_POINT('Ctrl Pts',(-20.8387858493865,10.0398330985108,123.958797508314)) ;
#34266=CARTESIAN_POINT('Ctrl Pts',(-20.3351890798294,10.2397395138226,124.21264452173)) ;
#34267=CARTESIAN_POINT('Ctrl Pts',(-20.5666727976471,10.0597504334128,124.41284983941)) ;
#34268=CARTESIAN_POINT('Ctrl Pts',(-20.0078940908122,10.2596127905386,124.479989674566)) ;
#34269=CARTESIAN_POINT('Ctrl Pts',(-20.157556275823,10.0796237101287,124.747029739255)) ;
#34270=CARTESIAN_POINT('Ctrl Pts',(-19.6059540280892,10.2796372807025,124.620350189469)) ;
#34271=CARTESIAN_POINT('Ctrl Pts',(-19.6551315118272,10.0996482002927,124.922482691242)) ;
#34272=CARTESIAN_POINT('Ctrl Pts',(-19.1834791470516,10.2995051218533,124.615075219233)) ;
#34273=CARTESIAN_POINT('Ctrl Pts',(-19.1270395365889,10.1195160414434,124.915890798242)) ;
#34274=CARTESIAN_POINT('Ctrl Pts',(-18.7864839057826,10.3194507727328,124.466021113069)) ;
#34275=CARTESIAN_POINT('Ctrl Pts',(-18.6307952227997,10.139461692323,124.729575809499)) ;
#34276=CARTESIAN_POINT('Ctrl Pts',(-18.4649063701951,10.3393561733498,124.190844404071)) ;
#34277=CARTESIAN_POINT('Ctrl Pts',(-18.228822407821,10.15936709294,124.385607616928)) ;
#34278=CARTESIAN_POINT('Ctrl Pts',(-18.2561330011468,10.3592304011661,123.82343533093)) ;
#34279=CARTESIAN_POINT('Ctrl Pts',(-17.9678535156375,10.1792413207563,123.926349000821)) ;
#34280=CARTESIAN_POINT('Ctrl Pts',(-18.1848402354332,10.3792161920437,123.40449567957)) ;
#34281=CARTESIAN_POINT('Ctrl Pts',(-17.8787342095081,10.1992271116339,123.402675114316)) ;
#34282=CARTESIAN_POINT('Ctrl Pts',(-18.2606699010585,10.3991104347035,122.98837126667)) ;
#34283=CARTESIAN_POINT('Ctrl Pts',(-17.9735177003611,10.2191213542937,122.882519964991)) ;
#34284=CARTESIAN_POINT('Ctrl Pts',(-18.4728612596363,10.4189891507756,122.622758653604)) ;
#34285=CARTESIAN_POINT('Ctrl Pts',(-18.2387528910192,10.2390000703658,122.425502981396)) ;
#34286=CARTESIAN_POINT('Ctrl Pts',(-18.7999520439114,10.4390286006202,122.349765919269)) ;
#34287=CARTESIAN_POINT('Ctrl Pts',(-18.6476140899653,10.2590395202104,122.084258749039)) ;
#34288=CARTESIAN_POINT('Ctrl Pts',(-19.1972003355021,10.458891762158,122.205978453982)) ;
#34289=CARTESIAN_POINT('Ctrl Pts',(-19.1441721120908,10.2789026817482,121.904520881741)) ;
#34290=CARTESIAN_POINT('Ctrl Pts',(-19.6218813508038,10.4788711301723,122.206142579944)) ;
#34291=CARTESIAN_POINT('Ctrl Pts',(-19.675023206704,10.2988820497624,121.904721686649)) ;
#34292=CARTESIAN_POINT('Ctrl Pts',(-20.0180063674985,10.4986817106951,122.349636080019)) ;
#34293=CARTESIAN_POINT('Ctrl Pts',(-20.1701799765576,10.3186926302853,122.084083785717)) ;
#34294=CARTESIAN_POINT('Ctrl Pts',(-20.3444408594761,10.5186626389807,122.621421727286)) ;
#34295=CARTESIAN_POINT('Ctrl Pts',(-20.578226084232,10.3386735585708,122.423812224516)) ;
#34296=CARTESIAN_POINT('Ctrl Pts',(-20.5574140360782,10.5385553108501,122.986919561501)) ;
#34297=CARTESIAN_POINT('Ctrl Pts',(-20.8444469589225,10.3585662304403,122.880680954071)) ;
#34298=CARTESIAN_POINT('Ctrl Pts',(-20.6337210602673,10.5584816411372,123.403677138751)) ;
#34299=CARTESIAN_POINT('Ctrl Pts',(-20.9398341758615,10.3784925607274,123.40162915944)) ;
#34300=CARTESIAN_POINT('Ctrl Pts',(-20.5626906544988,10.5784521952295,123.822322212015)) ;
#34301=CARTESIAN_POINT('Ctrl Pts',(-20.8510572231467,10.3984631148197,123.924927290917)) ;
#34302=CARTESIAN_POINT('Ctrl Pts',(-20.3894921739839,10.5949840343171,124.128174611121)) ;
#34303=CARTESIAN_POINT('Ctrl Pts',(-20.6345446352502,10.4149949539073,124.307272603932)) ;
#34304=CARTESIAN_POINT('Ctrl Pts',(-20.1931290904253,10.6083237731447,124.328455789616)) ;
#34305=CARTESIAN_POINT('Ctrl Pts',(-20.3891097553324,10.4283346927348,124.557601822234)) ;
#34306=CARTESIAN_POINT('Ctrl Pts',(-20.0213870270135,10.6183560153633,124.45086066554)) ;
#34307=CARTESIAN_POINT('Ctrl Pts',(-20.1744300570666,10.4383669349535,124.710615084661)) ;
#34308=CARTESIAN_POINT('Ctrl Pts',(-19.8344327780229,10.6282137160067,124.54030505442)) ;
#34309=CARTESIAN_POINT('Ctrl Pts',(-19.9407404802696,10.4482246355969,124.822421617956)) ;
#34310=CARTESIAN_POINT('Ctrl Pts',(-19.6321963819504,10.638205580646,124.597047913329)) ;
#34311=CARTESIAN_POINT('Ctrl Pts',(-19.6879423525452,10.4582165002362,124.893352629504)) ;
#34312=CARTESIAN_POINT('Ctrl Pts',(-19.424609722569,10.6481281304061,124.617626313307)) ;
#34313=CARTESIAN_POINT('Ctrl Pts',(-19.4284710425149,10.4681390499963,124.9190803154)) ;
#34314=CARTESIAN_POINT('Ctrl Pts',(-19.1462074516632,10.6614059038996,124.597234583046)) ;
#34315=CARTESIAN_POINT('Ctrl Pts',(-19.0804105140679,10.4814168234897,124.893583985702)) ;
#34316=CARTESIAN_POINT('Ctrl Pts',(-18.8783190629616,10.6747532428402,124.503658368855)) ;
#34317=CARTESIAN_POINT('Ctrl Pts',(-18.7455859092542,10.4947641624304,124.776616835827)) ;
#34318=CARTESIAN_POINT('Ctrl Pts',(-18.6486031256444,10.6879604746334,124.347593152274)) ;
#34319=CARTESIAN_POINT('Ctrl Pts',(-18.4584522381977,10.5079713942236,124.581549246975)) ;
#34320=CARTESIAN_POINT('Ctrl Pts',(-18.4978121198163,10.6979475907231,124.201545393376)) ;
#34321=CARTESIAN_POINT('Ctrl Pts',(-18.2699588379995,10.5179585103133,124.398989341585)) ;
#34322=CARTESIAN_POINT('Ctrl Pts',(-18.3749610360081,10.7078984963028,124.032167626381)) ;
#34323=CARTESIAN_POINT('Ctrl Pts',(-18.1163933969042,10.527909415893,124.187269395878)) ;
#34324=CARTESIAN_POINT('Ctrl Pts',(-18.2826761324805,10.7179535983103,123.842018510299)) ;
#34325=CARTESIAN_POINT('Ctrl Pts',(-18.0010345813188,10.5379645179005,123.949583784576)) ;
#34326=CARTESIAN_POINT('Ctrl Pts',(-18.2257894495901,10.7277752716314,123.643501818388)) ;
#34327=CARTESIAN_POINT('Ctrl Pts',(-17.9299233420751,10.5477861912216,123.701439503976)) ;
#34328=CARTESIAN_POINT('Ctrl Pts',(-18.2033755349775,10.7378337427063,123.433255143292)) ;
#34329=CARTESIAN_POINT('Ctrl Pts',(-17.901904058555,10.5578446622965,123.438628667081)) ;
#34330=CARTESIAN_POINT('Ctrl Pts',(-18.2179011335089,10.7477583538828,123.225094347349)) ;
#34331=CARTESIAN_POINT('Ctrl Pts',(-17.9200547530426,10.567769273473,123.1784374172)) ;
#34332=CARTESIAN_POINT('Ctrl Pts',(-18.2846726130989,10.7610356927832,122.954084571752)) ;
#34333=CARTESIAN_POINT('Ctrl Pts',(-18.0035329036583,10.5810466123734,122.839624585017)) ;
#34334=CARTESIAN_POINT('Ctrl Pts',(-18.4211117191118,10.7743345720208,122.706442666777)) ;
#34335=CARTESIAN_POINT('Ctrl Pts',(-18.1740788904205,10.5943454916109,122.530096455794)) ;
#34336=CARTESIAN_POINT('Ctrl Pts',(-18.6137282560997,10.7875734441915,122.505480302123)) ;
#34337=CARTESIAN_POINT('Ctrl Pts',(-18.414829088899,10.6075843637816,122.278909287776)) ;
#34338=CARTESIAN_POINT('Ctrl Pts',(-18.7832424185157,10.7975800623281,122.380894161506)) ;
#34339=CARTESIAN_POINT('Ctrl Pts',(-18.6267237903737,10.6175909819183,122.123170592557)) ;
#34340=CARTESIAN_POINT('Ctrl Pts',(-18.9724474720446,10.8076110073896,122.287775791708)) ;
#34341=CARTESIAN_POINT('Ctrl Pts',(-18.8632279358149,10.6276219269797,122.006771081539)) ;
#34342=CARTESIAN_POINT('Ctrl Pts',(-19.1713300500782,10.8174671807414,122.229578165669)) ;
#34343=CARTESIAN_POINT('Ctrl Pts',(-19.1118308518097,10.6374781003316,121.934021032192)) ;
#34344=CARTESIAN_POINT('Ctrl Pts',(-19.3802073449411,10.8274664517043,122.206207727251)) ;
#34345=CARTESIAN_POINT('Ctrl Pts',(-19.3729271808597,10.6474773712945,121.904805274405)) ;
#34346=CARTESIAN_POINT('Ctrl Pts',(-19.5878599933699,10.8373609034616,122.219083370884)) ;
#34347=CARTESIAN_POINT('Ctrl Pts',(-19.6324934400016,10.6573718230518,121.920897070104)) ;
#34348=CARTESIAN_POINT('Ctrl Pts',(-19.7934840277289,10.847424219271,122.268698552168)) ;
#34349=CARTESIAN_POINT('Ctrl Pts',(-19.8895240952947,10.6674351388611,121.982913347052)) ;
#34350=CARTESIAN_POINT('Ctrl Pts',(-19.9832086160557,10.8572630760106,122.351185619817)) ;
#34351=CARTESIAN_POINT('Ctrl Pts',(-20.1266813029748,10.6772739956008,122.086019825829)) ;
#34352=CARTESIAN_POINT('Ctrl Pts',(-20.1597838606521,10.8673291978282,122.467764324916)) ;
#34353=CARTESIAN_POINT('Ctrl Pts',(-20.3474018173166,10.6873401174184,122.23174090198)) ;
#34354=CARTESIAN_POINT('Ctrl Pts',(-20.3106209535211,10.8772124255524,122.610700532014)) ;
#34355=CARTESIAN_POINT('Ctrl Pts',(-20.5359503275938,10.6972233451426,122.410409425855)) ;
#34356=CARTESIAN_POINT('Ctrl Pts',(-20.4360184408181,10.8872018868312,122.779136894016)) ;
#34357=CARTESIAN_POINT('Ctrl Pts',(-20.6926994160956,10.7072128064214,122.620953380514)) ;
#34358=CARTESIAN_POINT('Ctrl Pts',(-20.5299682723289,10.8971655972577,122.966365986146)) ;
#34359=CARTESIAN_POINT('Ctrl Pts',(-20.8101391926436,10.7171765168479,122.85498870408)) ;
#34360=CARTESIAN_POINT('Ctrl Pts',(-20.5903840833054,10.9071605999886,123.167636072351)) ;
#34361=CARTESIAN_POINT('Ctrl Pts',(-20.8856615342813,10.7271715195788,123.106575647553)) ;
#34362=CARTESIAN_POINT('Ctrl Pts',(-20.6147046372521,10.9171969309989,123.377214474421)) ;
#34363=CARTESIAN_POINT('Ctrl Pts',(-20.9160649147942,10.737207850589,123.36854831693)) ;
#34364=CARTESIAN_POINT('Ctrl Pts',(-20.602840741777,10.9270431603412,123.583885830223)) ;
#34365=CARTESIAN_POINT('Ctrl Pts',(-20.9012376686418,10.7470540799313,123.626888226554)) ;
#34366=CARTESIAN_POINT('Ctrl Pts',(-20.5549910593693,10.9370286586164,123.788252345139)) ;
#34367=CARTESIAN_POINT('Ctrl Pts',(-20.8414280632278,10.7570395782066,123.882347119875)) ;
#34368=CARTESIAN_POINT('Ctrl Pts',(-20.4729131510359,10.9469635615994,123.98035400042)) ;
#34369=CARTESIAN_POINT('Ctrl Pts',(-20.7388329137616,10.7669744811896,124.122475498286)) ;
#34370=CARTESIAN_POINT('Ctrl Pts',(-20.3571965408839,10.9570210646946,124.157283328264)) ;
#34371=CARTESIAN_POINT('Ctrl Pts',(-20.5941893978565,10.7770319842848,124.343638489548)) ;
#34372=CARTESIAN_POINT('Ctrl Pts',(-20.2161055904513,10.9668427210651,124.308072643193)) ;
#34373=CARTESIAN_POINT('Ctrl Pts',(-20.4178270375078,10.7868536406553,124.532127444564)) ;
#34374=CARTESIAN_POINT('Ctrl Pts',(-20.0473038580147,10.9768987837303,124.435324360385)) ;
#34375=CARTESIAN_POINT('Ctrl Pts',(-20.2068264506129,10.7969097033205,124.691194003482)) ;
#34376=CARTESIAN_POINT('Ctrl Pts',(-19.8609387437001,10.9868394484335,124.529907956578)) ;
#34377=CARTESIAN_POINT('Ctrl Pts',(-19.9738709151532,10.8068503680237,124.809425923897)) ;
#34378=CARTESIAN_POINT('Ctrl Pts',(-19.6619073820417,10.996743852382,124.591096321842)) ;
#34379=CARTESIAN_POINT('Ctrl Pts',(-19.7250819168236,10.8167547719722,124.885913848149)) ;
#34380=CARTESIAN_POINT('Ctrl Pts',(-19.4523135812511,11.0067903373756,124.6170333815)) ;
#34381=CARTESIAN_POINT('Ctrl Pts',(-19.4630900672469,10.8268012569657,124.91833758783)) ;
#34382=CARTESIAN_POINT('Ctrl Pts',(-19.2444994497963,11.0166865651873,124.606521749711)) ;
#34383=CARTESIAN_POINT('Ctrl Pts',(-19.2033217041948,10.8366974847775,124.905200421556)) ;
#34384=CARTESIAN_POINT('Ctrl Pts',(-19.038362504801,11.0267461487508,124.559366648931)) ;
#34385=CARTESIAN_POINT('Ctrl Pts',(-18.9456501548506,10.8467570683409,124.84625892515)) ;
#34386=CARTESIAN_POINT('Ctrl Pts',(-18.8475263552642,11.0365981584196,124.478841690953)) ;
#34387=CARTESIAN_POINT('Ctrl Pts',(-18.7071032762533,10.8566090780098,124.745604613622)) ;
#34388=CARTESIAN_POINT('Ctrl Pts',(-18.6712543899711,11.0465606898592,124.365745599051)) ;
#34389=CARTESIAN_POINT('Ctrl Pts',(-18.486761846583,10.8665716094494,124.604236201888)) ;
#34390=CARTESIAN_POINT('Ctrl Pts',(-18.5164393691186,11.0565922380985,124.222526123336)) ;
#34391=CARTESIAN_POINT('Ctrl Pts',(-18.2932415519354,10.8766031576887,124.425213596777)) ;
#34392=CARTESIAN_POINT('Ctrl Pts',(-18.3904718457185,11.0664836493116,124.057073079274)) ;
#34393=CARTESIAN_POINT('Ctrl Pts',(-18.1357799385702,10.8864945689018,124.218398117889)) ;
#34394=CARTESIAN_POINT('Ctrl Pts',(-18.2936007393847,11.0764999030196,123.870096289376)) ;
#34395=CARTESIAN_POINT('Ctrl Pts',(-18.0146891208495,10.8965108226097,123.984678099448)) ;
#34396=CARTESIAN_POINT('Ctrl Pts',(-18.2310191009212,11.0865300058643,123.668736110514)) ;
#34397=CARTESIAN_POINT('Ctrl Pts',(-17.9364599064169,10.9065409254544,123.732978598367)) ;
#34398=CARTESIAN_POINT('Ctrl Pts',(-18.2044167485645,11.096386454818,123.463224365483)) ;
#34399=CARTESIAN_POINT('Ctrl Pts',(-17.9032046925238,10.9163973744082,123.476088297532)) ;
#34400=CARTESIAN_POINT('Ctrl Pts',(-18.2137726552221,11.1063854655903,123.253255515666)) ;
#34401=CARTESIAN_POINT('Ctrl Pts',(-17.9148974746838,10.9263963851804,123.213627004968)) ;
#34402=CARTESIAN_POINT('Ctrl Pts',(-18.2587594656026,11.1162806825083,123.050114933331)) ;
#34403=CARTESIAN_POINT('Ctrl Pts',(-17.9711291548573,10.9362916020984,122.959700121577)) ;
#34404=CARTESIAN_POINT('Ctrl Pts',(-18.3396629587075,11.1263411978656,122.85472528768)) ;
#34405=CARTESIAN_POINT('Ctrl Pts',(-18.0722565350831,10.9463521174558,122.715462501304)) ;
#34406=CARTESIAN_POINT('Ctrl Pts',(-18.4508021074728,11.1361904912527,122.67999776762)) ;
#34407=CARTESIAN_POINT('Ctrl Pts',(-18.2111793287359,10.9562014108428,122.497051143114)) ;
#34408=CARTESIAN_POINT('Ctrl Pts',(-18.5927075074045,11.1462176669327,122.524117766382)) ;
#34409=CARTESIAN_POINT('Ctrl Pts',(-18.3885596784698,10.9662285865229,122.302199917905)) ;
#34410=CARTESIAN_POINT('Ctrl Pts',(-18.7598974171996,11.1562462425598,122.39565716601)) ;
#34411=CARTESIAN_POINT('Ctrl Pts',(-18.5975457775066,10.97625716215,122.141622604238)) ;
#34412=CARTESIAN_POINT('Ctrl Pts',(-18.9432305176374,11.1660913361057,122.299619707887)) ;
#34413=CARTESIAN_POINT('Ctrl Pts',(-18.8267122579824,10.9861022556959,122.021573575525)) ;
#34414=CARTESIAN_POINT('Ctrl Pts',(-19.1432259259205,11.1760825775375,122.235411488495)) ;
#34415=CARTESIAN_POINT('Ctrl Pts',(-19.076706172588,10.9960934971277,121.941311591206)) ;
#34416=CARTESIAN_POINT('Ctrl Pts',(-19.3523221570473,11.1861183586808,122.207211675339)) ;
#34417=CARTESIAN_POINT('Ctrl Pts',(-19.33807608883,11.0061292782709,121.90605998594)) ;
#34418=CARTESIAN_POINT('Ctrl Pts',(-19.5592805247249,11.1959705644105,122.215313540189)) ;
#34419=CARTESIAN_POINT('Ctrl Pts',(-19.5967752495453,11.0159814840007,121.916185579001)) ;
#34420=CARTESIAN_POINT('Ctrl Pts',(-19.7640786083089,11.2059326585275,122.259120874168)) ;
#34421=CARTESIAN_POINT('Ctrl Pts',(-19.8527735772525,11.0259435781177,121.970943280824)) ;
#34422=CARTESIAN_POINT('Ctrl Pts',(-19.9592440107104,11.2159552193546,122.338540115345)) ;
#34423=CARTESIAN_POINT('Ctrl Pts',(-20.0967309230037,11.0359661389448,122.070215768885)) ;
#34424=CARTESIAN_POINT('Ctrl Pts',(-20.1360936806095,11.2258829910061,122.449415578369)) ;
#34425=CARTESIAN_POINT('Ctrl Pts',(-20.3177943873976,11.0458939105963,122.208809071597)) ;
#34426=CARTESIAN_POINT('Ctrl Pts',(-20.2927527732055,11.235925375131,122.59092205436)) ;
#34427=CARTESIAN_POINT('Ctrl Pts',(-20.5136192108406,11.0559362947211,122.385690857769)) ;
#34428=CARTESIAN_POINT('Ctrl Pts',(-20.4205680894076,11.2458145992016,122.754908938647)) ;
#34429=CARTESIAN_POINT('Ctrl Pts',(-20.6733901754155,11.0658255187918,122.590674219362)) ;
#34430=CARTESIAN_POINT('Ctrl Pts',(-20.5192928454941,11.2558038473689,122.940253974445)) ;
#34431=CARTESIAN_POINT('Ctrl Pts',(-20.7967974985827,11.0758147669591,122.82235502115)) ;
#34432=CARTESIAN_POINT('Ctrl Pts',(-20.5839847168731,11.2657624244109,123.139363117153)) ;
#34433=CARTESIAN_POINT('Ctrl Pts',(-20.877663904031,11.0857733440011,123.071241395872)) ;
#34434=CARTESIAN_POINT('Ctrl Pts',(-20.6134608095792,11.2756619935022,123.345397790749)) ;
#34435=CARTESIAN_POINT('Ctrl Pts',(-20.9145104547974,11.0956729130923,123.328785419535)) ;
#34436=CARTESIAN_POINT('Ctrl Pts',(-20.6065401284065,11.2857099055862,123.556501597487)) ;
#34437=CARTESIAN_POINT('Ctrl Pts',(-20.9058609614837,11.1057208251763,123.592665004886)) ;
#34438=CARTESIAN_POINT('Ctrl Pts',(-20.5638788823548,11.2956052598934,123.760144762529)) ;
#34439=CARTESIAN_POINT('Ctrl Pts',(-20.8525354819889,11.1156161794835,123.84722011856)) ;
#34440=CARTESIAN_POINT('Ctrl Pts',(-20.4852553344784,11.3056669103846,123.956492429052)) ;
#34441=CARTESIAN_POINT('Ctrl Pts',(-20.7542573599522,11.1256778299747,124.092654877051)) ;
#34442=CARTESIAN_POINT('Ctrl Pts',(-20.3761505871013,11.315511525847,124.132371029593)) ;
#34443=CARTESIAN_POINT('Ctrl Pts',(-20.6178768119948,11.1355224454372,124.312504919937)) ;
#34444=CARTESIAN_POINT('Ctrl Pts',(-20.237114111558,11.3254716047484,124.288935623539)) ;
#34445=CARTESIAN_POINT('Ctrl Pts',(-20.4440816601254,11.1454825243386,124.508211665925)) ;
#34446=CARTESIAN_POINT('Ctrl Pts',(-20.0714663398208,11.3355097991068,124.419675506507)) ;
#34447=CARTESIAN_POINT('Ctrl Pts',(-20.237022783302,11.155520718697,124.671637321571)) ;
#34448=CARTESIAN_POINT('Ctrl Pts',(-19.8888323535182,11.3453835145064,124.518385640457)) ;
#34449=CARTESIAN_POINT('Ctrl Pts',(-20.0087297938928,11.1653944340966,124.79502640491)) ;
#34450=CARTESIAN_POINT('Ctrl Pts',(-19.6879284940433,11.3554552240407,124.585159910392)) ;
#34451=CARTESIAN_POINT('Ctrl Pts',(-19.7576006731065,11.1754661436308,124.878495075327)) ;
#34452=CARTESIAN_POINT('Ctrl Pts',(-19.4834310386215,11.3652876644932,124.615427060217)) ;
#34453=CARTESIAN_POINT('Ctrl Pts',(-19.5019775459642,11.1852985840833,124.916330182975)) ;
#34454=CARTESIAN_POINT('Ctrl Pts',(-19.2726002542326,11.3753194854186,124.610200309681)) ;
#34455=CARTESIAN_POINT('Ctrl Pts',(-19.23843916646,11.1953304050088,124.909797495745)) ;
#34456=CARTESIAN_POINT('Ctrl Pts',(-19.0662276962164,11.3853398553042,124.567903119432)) ;
#34457=CARTESIAN_POINT('Ctrl Pts',(-18.9804733109485,11.2053507748943,124.856926970569)) ;
#34458=CARTESIAN_POINT('Ctrl Pts',(-18.8731273416045,11.3952066264379,124.492104200881)) ;
#34459=CARTESIAN_POINT('Ctrl Pts',(-18.7390964606754,11.2152175460281,124.762178595667)) ;
#34460=CARTESIAN_POINT('Ctrl Pts',(-18.6924952829997,11.4052773976273,124.381703676241)) ;
#34461=CARTESIAN_POINT('Ctrl Pts',(-18.5133063352231,11.2252883172175,124.624178813751)) ;
#34462=CARTESIAN_POINT('Ctrl Pts',(-18.5373237843845,11.4151205581489,124.244779697978)) ;
#34463=CARTESIAN_POINT('Ctrl Pts',(-18.319340401592,11.2351314777391,124.453023478545)) ;
#34464=CARTESIAN_POINT('Ctrl Pts',(-18.4059602071296,11.4251007913353,124.081184277243)) ;
#34465=CARTESIAN_POINT('Ctrl Pts',(-18.1551353492068,11.2451117109255,124.248529269584)) ;
#34466=CARTESIAN_POINT('Ctrl Pts',(-18.3049653385912,11.4351193113705,123.896363057127)) ;
#34467=CARTESIAN_POINT('Ctrl Pts',(-18.028891195505,11.2551302309607,124.017503067195)) ;
#34468=CARTESIAN_POINT('Ctrl Pts',(-18.2380760069019,11.4450026197542,123.69961958379)) ;
#34469=CARTESIAN_POINT('Ctrl Pts',(-17.9452787246737,11.2650135393444,123.771572840956)) ;
#34470=CARTESIAN_POINT('Ctrl Pts',(-18.2058712454328,11.455070903925,123.490451765677)) ;
#34471=CARTESIAN_POINT('Ctrl Pts',(-17.9050223247957,11.2750818235151,123.51011355244)) ;
#34472=CARTESIAN_POINT('Ctrl Pts',(-18.2101233464429,11.4649010305926,123.283800583045)) ;
#34473=CARTESIAN_POINT('Ctrl Pts',(-17.9103370637522,11.2849119501828,123.251798025959)) ;
#34474=CARTESIAN_POINT('Ctrl Pts',(-18.250874219467,11.4749676027992,123.076164349147)) ;
#34475=CARTESIAN_POINT('Ctrl Pts',(-17.9612752713621,11.2949785223893,122.992253063274)) ;
#34476=CARTESIAN_POINT('Ctrl Pts',(-18.3258631651741,11.4848577590399,122.882207935105)) ;
#34477=CARTESIAN_POINT('Ctrl Pts',(-18.0550114913503,11.30486867863,122.749806436383)) ;
#34478=CARTESIAN_POINT('Ctrl Pts',(-18.4340938733603,11.4948502866163,122.702175775169)) ;
#34479=CARTESIAN_POINT('Ctrl Pts',(-18.1902998279347,11.3148612062065,122.524765958855)) ;
#34480=CARTESIAN_POINT('Ctrl Pts',(-18.5716561470465,11.5048117764906,122.544271291541)) ;
#34481=CARTESIAN_POINT('Ctrl Pts',(-18.3622527777214,11.3248226960808,122.327384835922)) ;
#34482=CARTESIAN_POINT('Ctrl Pts',(-18.733397668661,11.5147209983778,122.412963329841)) ;
#34483=CARTESIAN_POINT('Ctrl Pts',(-18.5644303505111,11.334731917968,122.163249256317)) ;
#34484=CARTESIAN_POINT('Ctrl Pts',(-18.9180612846803,11.5247695781881,122.310386430444)) ;
#34485=CARTESIAN_POINT('Ctrl Pts',(-18.7952595963168,11.3447804977783,122.03502817518)) ;
#34486=CARTESIAN_POINT('Ctrl Pts',(-19.1144372305553,11.5346525526582,122.242490101265)) ;
#34487=CARTESIAN_POINT('Ctrl Pts',(-19.0407305551372,11.3546634722484,121.95015733424)) ;
#34488=CARTESIAN_POINT('Ctrl Pts',(-19.3218535876862,11.5446474638009,122.208905343626)) ;
#34489=CARTESIAN_POINT('Ctrl Pts',(-19.3000011957466,11.364658383391,121.908176470979)) ;
#34490=CARTESIAN_POINT('Ctrl Pts',(-19.5325030834212,11.5546678503745,122.212142964224)) ;
#34491=CARTESIAN_POINT('Ctrl Pts',(-19.5633130308723,11.3746787699646,121.912223489053)) ;
#34492=CARTESIAN_POINT('Ctrl Pts',(-19.7371085501306,11.5645779542315,122.251347857035)) ;
#34493=CARTESIAN_POINT('Ctrl Pts',(-19.8190707586294,11.3845888738217,121.961229817073)) ;
#34494=CARTESIAN_POINT('Ctrl Pts',(-19.9323591296137,11.5745056664414,122.325110819767)) ;
#34495=CARTESIAN_POINT('Ctrl Pts',(-20.0631345837559,11.3945165860316,122.053434027818)) ;
#34496=CARTESIAN_POINT('Ctrl Pts',(-20.1138182396832,11.5845487762087,122.433038429192)) ;
#34497=CARTESIAN_POINT('Ctrl Pts',(-20.2899581916419,11.4045596957989,122.188343592996)) ;
#34498=CARTESIAN_POINT('Ctrl Pts',(-20.2713872169236,11.5944351966642,122.568595596171)) ;
#34499=CARTESIAN_POINT('Ctrl Pts',(-20.4869200799301,11.4144461162544,122.357790944898)) ;
#34500=CARTESIAN_POINT('Ctrl Pts',(-20.4047088338096,11.6044283742699,122.730945445389)) ;
#34501=CARTESIAN_POINT('Ctrl Pts',(-20.6535719341279,11.42443929386,122.560728657127)) ;
#34502=CARTESIAN_POINT('Ctrl Pts',(-20.5072617933259,11.6143740371738,122.913157719128)) ;
#34503=CARTESIAN_POINT('Ctrl Pts',(-20.7817631202892,11.434384956764,122.788494689885)) ;
#34504=CARTESIAN_POINT('Ctrl Pts',(-20.5770363442089,11.624321333379,123.110307996559)) ;
#34505=CARTESIAN_POINT('Ctrl Pts',(-20.8689810113342,11.4443322529691,123.034933251559)) ;
#34506=CARTESIAN_POINT('Ctrl Pts',(-20.6116338746559,11.6343690989569,123.318685651132)) ;
#34507=CARTESIAN_POINT('Ctrl Pts',(-20.9122274632923,11.454380018547,123.295405142893)) ;
#34508=CARTESIAN_POINT('Ctrl Pts',(-20.6097306714455,11.6442173121745,123.525714223304)) ;
#34509=CARTESIAN_POINT('Ctrl Pts',(-20.9098479557393,11.4642282317647,123.55419225068)) ;
#34510=CARTESIAN_POINT('Ctrl Pts',(-20.5721619278645,11.6541768849686,123.731697031123)) ;
#34511=CARTESIAN_POINT('Ctrl Pts',(-20.8628861918604,11.4741878045588,123.811671085789)) ;
#34512=CARTESIAN_POINT('Ctrl Pts',(-20.4984904473743,11.6642135060011,123.92941246265)) ;
#34513=CARTESIAN_POINT('Ctrl Pts',(-20.7707963195394,11.4842244255913,124.05881501279)) ;
#34514=CARTESIAN_POINT('Ctrl Pts',(-20.3935356094815,11.6740940208114,124.108691624986)) ;
#34515=CARTESIAN_POINT('Ctrl Pts',(-20.6396015638699,11.4941049404016,124.282914554995)) ;
#34516=CARTESIAN_POINT('Ctrl Pts',(-20.2567978653035,11.6841466721185,124.269794367337)) ;
#34517=CARTESIAN_POINT('Ctrl Pts',(-20.468678971524,11.5041575917087,124.484292270333)) ;
#34518=CARTESIAN_POINT('Ctrl Pts',(-20.0967123068534,11.6940420703985,124.40270437159)) ;
#34519=CARTESIAN_POINT('Ctrl Pts',(-20.268570770948,11.5140529899886,124.650429772434)) ;
#34520=CARTESIAN_POINT('Ctrl Pts',(-19.9132571297185,11.7040921921046,124.507462775467)) ;
#34521=CARTESIAN_POINT('Ctrl Pts',(-20.0392516107157,11.5241031116947,124.781376915265)) ;
#34522=CARTESIAN_POINT('Ctrl Pts',(-19.7176472157066,11.7139764716465,124.577647205215)) ;
#34523=CARTESIAN_POINT('Ctrl Pts',(-19.7947379346561,11.5339873912366,124.869107009974)) ;
#34524=CARTESIAN_POINT('Ctrl Pts',(-19.5106395256385,11.7239712529384,124.613575520575)) ;
#34525=CARTESIAN_POINT('Ctrl Pts',(-19.535977954542,11.5439821725286,124.914016453037)) ;
#34526=CARTESIAN_POINT('Ctrl Pts',(-19.3014914963835,11.7339190981252,124.612936959039)) ;
#34527=CARTESIAN_POINT('Ctrl Pts',(-19.2745423775974,11.5539300177154,124.913217278896)) ;
#34528=CARTESIAN_POINT('Ctrl Pts',(-19.0958351736706,11.7438560615126,124.576338079464)) ;
#34529=CARTESIAN_POINT('Ctrl Pts',(-19.0174715357775,11.5638669811028,124.867467501011)) ;
#34530=CARTESIAN_POINT('Ctrl Pts',(-18.8986161272856,11.7538390262498,124.504485391709)) ;
#34531=CARTESIAN_POINT('Ctrl Pts',(-18.7709478903142,11.57384994584,124.777650445181)) ;
#34532=CARTESIAN_POINT('Ctrl Pts',(-18.7159988224537,11.7638828776654,124.398530286436)) ;
#34533=CARTESIAN_POINT('Ctrl Pts',(-18.5426769439272,11.5838937972556,124.645205762121)) ;
#34534=CARTESIAN_POINT('Ctrl Pts',(-18.5576631664198,11.7737110790002,124.265735860728)) ;
#34535=CARTESIAN_POINT('Ctrl Pts',(-18.3447570489577,11.5937219985904,124.479210868713)) ;
#34536=CARTESIAN_POINT('Ctrl Pts',(-18.4214033173466,11.7837876515982,124.103588886124)) ;
#34537=CARTESIAN_POINT('Ctrl Pts',(-18.1744334770161,11.6037985711884,124.276526674695)) ;
#34538=CARTESIAN_POINT('Ctrl Pts',(-18.3175955543511,11.7936397316058,123.92430715972)) ;
#34539=CARTESIAN_POINT('Ctrl Pts',(-18.0446742699967,11.613650651196,124.052422800999)) ;
#34540=CARTESIAN_POINT('Ctrl Pts',(-18.2447567569921,11.8037130166099,123.725492716322)) ;
#34541=CARTESIAN_POINT('Ctrl Pts',(-17.9536271836293,11.6237239362001,123.80390465871)) ;
#34542=CARTESIAN_POINT('Ctrl Pts',(-18.2084461708989,11.8135543683204,123.521791919159)) ;
#34543=CARTESIAN_POINT('Ctrl Pts',(-17.9082400348832,11.6335652879105,123.549277141693)) ;
#34544=CARTESIAN_POINT('Ctrl Pts',(-18.2072783331998,11.8235158677169,123.312385813251)) ;
#34545=CARTESIAN_POINT('Ctrl Pts',(-17.9067818388404,11.6435267873071,123.287519099371)) ;
#34546=CARTESIAN_POINT('Ctrl Pts',(-18.2431187666664,11.8335516438469,123.104460989179)) ;
#34547=CARTESIAN_POINT('Ctrl Pts',(-17.951583816613,11.653562563437,123.027613430396)) ;
#34548=CARTESIAN_POINT('Ctrl Pts',(-18.313260700151,11.8434400704844,122.908768536338)) ;
#34549=CARTESIAN_POINT('Ctrl Pts',(-18.039263006394,11.6634509900746,122.782997516974)) ;
#34550=CARTESIAN_POINT('Ctrl Pts',(-18.4172968730816,11.8534553925594,122.725703223709)) ;
#34551=CARTESIAN_POINT('Ctrl Pts',(-18.1693096864973,11.6734663121495,122.554166702765)) ;
#34552=CARTESIAN_POINT('Ctrl Pts',(-18.5521138610027,11.8634857414596,122.563558399555)) ;
#34553=CARTESIAN_POINT('Ctrl Pts',(-18.3378320340471,11.6834966610498,122.351486710927)) ;
#34554=CARTESIAN_POINT('Ctrl Pts',(-18.7097629865951,11.8733291170662,122.429511598476)) ;
#34555=CARTESIAN_POINT('Ctrl Pts',(-18.5348954405883,11.6933400366564,122.183928683916)) ;
#34556=CARTESIAN_POINT('Ctrl Pts',(-18.8914357075047,11.8833585539634,122.322486366911)) ;
#34557=CARTESIAN_POINT('Ctrl Pts',(-18.7619871989478,11.7033694735536,122.050148739799)) ;
#34558=CARTESIAN_POINT('Ctrl Pts',(-19.0891853403317,11.8933904318963,122.249153011441)) ;
#34559=CARTESIAN_POINT('Ctrl Pts',(-19.0091747228791,11.7134013514865,121.958483598084)) ;
#34560=CARTESIAN_POINT('Ctrl Pts',(-19.2923854095674,11.9032200550018,122.211622723258)) ;
#34561=CARTESIAN_POINT('Ctrl Pts',(-19.2631763810866,11.723230974592,121.911572238441)) ;
#34562=CARTESIAN_POINT('Ctrl Pts',(-19.5023882087078,11.9132095261549,122.209287327401)) ;
#34563=CARTESIAN_POINT('Ctrl Pts',(-19.5256800788835,11.733220445745,121.908654949402)) ;
#34564=CARTESIAN_POINT('Ctrl Pts',(-19.7106392401679,11.9232533749173,122.244164803758)) ;
#34565=CARTESIAN_POINT('Ctrl Pts',(-19.7859934260146,11.7432642945074,121.952253536854)) ;
#34566=CARTESIAN_POINT('Ctrl Pts',(-19.9054125620073,11.933075080449,122.312709524051)) ;
#34567=CARTESIAN_POINT('Ctrl Pts',(-20.0294606191332,11.7530860000391,122.037936667124)) ;
#34568=CARTESIAN_POINT('Ctrl Pts',(-20.0894867289459,11.9431101202768,122.415781902165)) ;
#34569=CARTESIAN_POINT('Ctrl Pts',(-20.2595522205111,11.763121039867,122.166778899323)) ;
#34570=CARTESIAN_POINT('Ctrl Pts',(-20.2523369083129,11.9531348271682,122.54956886486)) ;
#34571=CARTESIAN_POINT('Ctrl Pts',(-20.4631137172292,11.7731457467584,122.334014058128)) ;
#34572=CARTESIAN_POINT('Ctrl Pts',(-20.3874578810136,11.962987531509,122.706561960871)) ;
#34573=CARTESIAN_POINT('Ctrl Pts',(-20.6320140503792,11.7829984510992,122.53025751933)) ;
#34574=CARTESIAN_POINT('Ctrl Pts',(-20.4950292100305,11.9729756537167,122.88687951836)) ;
#34575=CARTESIAN_POINT('Ctrl Pts',(-20.7664764700505,11.7929865733069,122.755655719677)) ;
#34576=CARTESIAN_POINT('Ctrl Pts',(-20.5692290588118,11.982904123824,123.081978843733)) ;
#34577=CARTESIAN_POINT('Ctrl Pts',(-20.8592244693061,11.8029150434141,122.999531121784)) ;
#34578=CARTESIAN_POINT('Ctrl Pts',(-20.6090083992339,11.9928931009912,123.28818688241)) ;
#34579=CARTESIAN_POINT('Ctrl Pts',(-20.908946487162,11.8129040205813,123.257291767324)) ;
#34580=CARTESIAN_POINT('Ctrl Pts',(-20.6120343021104,12.0029309082709,123.499185950342)) ;
#34581=CARTESIAN_POINT('Ctrl Pts',(-20.9127267285164,11.822941827861,123.521040547075)) ;
#34582=CARTESIAN_POINT('Ctrl Pts',(-20.5793530027892,12.0127772091342,123.703591668076)) ;
#34583=CARTESIAN_POINT('Ctrl Pts',(-20.8718727621147,11.8327881287243,123.776548267518)) ;
#34584=CARTESIAN_POINT('Ctrl Pts',(-20.5108877173329,12.0228029525135,123.902937612404)) ;
#34585=CARTESIAN_POINT('Ctrl Pts',(-20.7862889532544,11.8428138721037,124.025729898037)) ;
#34586=CARTESIAN_POINT('Ctrl Pts',(-20.4083149981522,12.0328338189525,124.087198060114)) ;
#34587=CARTESIAN_POINT('Ctrl Pts',(-20.6580711492703,11.8528447385427,124.256054351239)) ;
#34588=CARTESIAN_POINT('Ctrl Pts',(-20.278204027201,12.0426711777513,124.247942559337)) ;
#34589=CARTESIAN_POINT('Ctrl Pts',(-20.4954300470344,11.8626820973415,124.456984258303)) ;
#34590=CARTESIAN_POINT('Ctrl Pts',(-20.1200700787013,12.052663138685,124.386216766339)) ;
#34591=CARTESIAN_POINT('Ctrl Pts',(-20.2977609080955,11.8726740582752,124.629825264853)) ;
#34592=CARTESIAN_POINT('Ctrl Pts',(-19.9393758024445,12.0626955012416,124.495014747097)) ;
#34593=CARTESIAN_POINT('Ctrl Pts',(-20.0718918884513,11.8827064208318,124.765820716472)) ;
#34594=CARTESIAN_POINT('Ctrl Pts',(-19.7459234684514,12.072560661816,124.569749829319)) ;
#34595=CARTESIAN_POINT('Ctrl Pts',(-19.8300749226539,11.8925715814062,124.8592375948)) ;
#34596=CARTESIAN_POINT('Ctrl Pts',(-19.5405372405183,12.0825225663937,124.610739722099)) ;
#34597=CARTESIAN_POINT('Ctrl Pts',(-19.5733413955224,11.9025334859838,124.91047253432)) ;
#34598=CARTESIAN_POINT('Ctrl Pts',(-19.3296285023073,12.0925574964694,124.615133939641)) ;
#34599=CARTESIAN_POINT('Ctrl Pts',(-19.3097054567176,11.9125684160596,124.915962853165)) ;
#34600=CARTESIAN_POINT('Ctrl Pts',(-19.12418262518,12.102442443323,124.58366381539)) ;
#34601=CARTESIAN_POINT('Ctrl Pts',(-19.052897931185,11.9224533629132,124.876622619273)) ;
#34602=CARTESIAN_POINT('Ctrl Pts',(-18.9237994034088,12.1125081196345,124.515756077525)) ;
#34603=CARTESIAN_POINT('Ctrl Pts',(-18.8024198540118,11.9325190392247,124.791735612514)) ;
#34604=CARTESIAN_POINT('Ctrl Pts',(-18.7422682640068,12.1223470392694,124.416531181598)) ;
#34605=CARTESIAN_POINT('Ctrl Pts',(-18.5755065294537,11.9423579588596,124.66770191258)) ;
#34606=CARTESIAN_POINT('Ctrl Pts',(-18.5769155643104,12.1324105490038,124.284598448374)) ;
#34607=CARTESIAN_POINT('Ctrl Pts',(-18.36881738441,11.952421468594,124.502784045041)) ;
#34608=CARTESIAN_POINT('Ctrl Pts',(-18.4394382528722,12.1423041621656,124.128483209612)) ;
#34609=CARTESIAN_POINT('Ctrl Pts',(-18.196972359284,11.9623150817557,124.307637940831)) ;
#34610=CARTESIAN_POINT('Ctrl Pts',(-18.330159277488,12.152248168979,123.950297968068)) ;
#34611=CARTESIAN_POINT('Ctrl Pts',(-18.0603757684666,11.9722590885692,124.084904760915)) ;
#34612=CARTESIAN_POINT('Ctrl Pts',(-18.2529261348415,12.1622491233333,123.754711085262)) ;
#34613=CARTESIAN_POINT('Ctrl Pts',(-17.9638367966722,11.9822600429234,123.84042009983)) ;
#34614=CARTESIAN_POINT('Ctrl Pts',(-18.2110463667562,12.1722878810256,123.547880865785)) ;
#34615=CARTESIAN_POINT('Ctrl Pts',(-17.9114896577593,11.9922988006158,123.581881819459)) ;
#34616=CARTESIAN_POINT('Ctrl Pts',(-18.2053758043967,12.1821120651956,123.341406321408)) ;
#34617=CARTESIAN_POINT('Ctrl Pts',(-17.9044041218427,12.0021229847857,123.323787975378)) ;
#34618=CARTESIAN_POINT('Ctrl Pts',(-18.2360503167514,12.192170130795,123.132209463155)) ;
#34619=CARTESIAN_POINT('Ctrl Pts',(-17.942749948479,12.0121810503852,123.062292370607)) ;
#34620=CARTESIAN_POINT('Ctrl Pts',(-18.302006424845,12.2021001775697,122.934128152636)) ;
#34621=CARTESIAN_POINT('Ctrl Pts',(-18.0251977236969,12.0221110971599,122.81469131617)) ;
#34622=CARTESIAN_POINT('Ctrl Pts',(-18.4010777311963,12.2120516199068,122.749859407281)) ;
#34623=CARTESIAN_POINT('Ctrl Pts',(-18.1490393730645,12.032062539497,122.58435652218)) ;
#34624=CARTESIAN_POINT('Ctrl Pts',(-18.5321045118858,12.2220984170861,122.584200624693)) ;
#34625=CARTESIAN_POINT('Ctrl Pts',(-18.3128249787563,12.0421093366763,122.3772847395)) ;
#34626=CARTESIAN_POINT('Ctrl Pts',(-18.6866546754837,12.2319463577662,122.446441479111)) ;
#34627=CARTESIAN_POINT('Ctrl Pts',(-18.5060148097537,12.0519572773564,122.20508758863)) ;
#34628=CARTESIAN_POINT('Ctrl Pts',(-18.8644598958187,12.2419079891088,122.335805361285)) ;
#34629=CARTESIAN_POINT('Ctrl Pts',(-18.7282729224317,12.061918908699,122.066794754657)) ;
#34630=CARTESIAN_POINT('Ctrl Pts',(-19.0602009714326,12.2519366484847,122.257435573529)) ;
#34631=CARTESIAN_POINT('Ctrl Pts',(-18.9729503385331,12.0719475680749,121.96883508161)) ;
#34632=CARTESIAN_POINT('Ctrl Pts',(-19.2641055065429,12.2618469513729,122.214691358915)) ;
#34633=CARTESIAN_POINT('Ctrl Pts',(-19.2278317877476,12.081857870963,121.915407496546)) ;
#34634=CARTESIAN_POINT('Ctrl Pts',(-19.472848854405,12.2717818459351,122.20743693277)) ;
#34635=CARTESIAN_POINT('Ctrl Pts',(-19.4887612039863,12.0917927655252,121.906342273748)) ;
#34636=CARTESIAN_POINT('Ctrl Pts',(-19.6818517454895,12.281822944602,122.237040740592)) ;
#34637=CARTESIAN_POINT('Ctrl Pts',(-19.7500144690239,12.1018338641922,121.943349817982)) ;
#34638=CARTESIAN_POINT('Ctrl Pts',(-19.8795274393584,12.2917102271064,122.301350610276)) ;
#34639=CARTESIAN_POINT('Ctrl Pts',(-19.9971083720291,12.1117211466965,122.023739879695)) ;
#34640=CARTESIAN_POINT('Ctrl Pts',(-20.0651177529335,12.3017019676169,122.399712129327)) ;
#34641=CARTESIAN_POINT('Ctrl Pts',(-20.2290950029952,12.121712887207,122.146694306232)) ;
#34642=CARTESIAN_POINT('Ctrl Pts',(-20.2301016245503,12.3116525168523,122.52834286884)) ;
#34643=CARTESIAN_POINT('Ctrl Pts',(-20.4353231818541,12.1316634364425,122.307485012955)) ;
#34644=CARTESIAN_POINT('Ctrl Pts',(-20.3702511436106,12.3215881944871,122.68320837822)) ;
#34645=CARTESIAN_POINT('Ctrl Pts',(-20.6105080303752,12.1415991140773,122.501068844244)) ;
#34646=CARTESIAN_POINT('Ctrl Pts',(-20.4821440049613,12.3315736122799,122.86084640938)) ;
#34647=CARTESIAN_POINT('Ctrl Pts',(-20.750371753323,12.15158453187,122.723117938281)) ;
#34648=CARTESIAN_POINT('Ctrl Pts',(-20.561588894867,12.3416024051504,123.056141240279)) ;
#34649=CARTESIAN_POINT('Ctrl Pts',(-20.8496752814838,12.1616133247405,122.967237619822)) ;
#34650=CARTESIAN_POINT('Ctrl Pts',(-20.605473389762,12.3514819163783,123.25914772635)) ;
#34651=CARTESIAN_POINT('Ctrl Pts',(-20.9045281451374,12.1714928359685,123.220996340635)) ;
#34652=CARTESIAN_POINT('Ctrl Pts',(-20.6140174461044,12.3614754530513,123.469077690765)) ;
#34653=CARTESIAN_POINT('Ctrl Pts',(-20.9152054114084,12.1814863726414,123.483408955601)) ;
#34654=CARTESIAN_POINT('Ctrl Pts',(-20.5854395929456,12.3715077213151,123.67803354945)) ;
#34655=CARTESIAN_POINT('Ctrl Pts',(-20.8794802828438,12.1915186409053,123.744603500806)) ;
#34656=CARTESIAN_POINT('Ctrl Pts',(-20.5225086633852,12.381371683321,123.875648773567)) ;
#34657=CARTESIAN_POINT('Ctrl Pts',(-20.8008139738613,12.2013826029112,123.991621606328)) ;
#34658=CARTESIAN_POINT('Ctrl Pts',(-20.4242612791623,12.3914417446659,124.063150375643)) ;
#34659=CARTESIAN_POINT('Ctrl Pts',(-20.6780021897342,12.2114526642561,124.225997440443)) ;
#34660=CARTESIAN_POINT('Ctrl Pts',(-20.2978479151584,12.4012841090146,124.22697472228)) ;
#34661=CARTESIAN_POINT('Ctrl Pts',(-20.5199833627417,12.2212950286048,124.430776031816)) ;
#34662=CARTESIAN_POINT('Ctrl Pts',(-20.1436024751154,12.4112447815171,124.368597953825)) ;
#34663=CARTESIAN_POINT('Ctrl Pts',(-20.3271747466949,12.2312557011072,124.607803018329)) ;
#34664=CARTESIAN_POINT('Ctrl Pts',(-19.9655160234336,12.4212828525849,124.481805478694)) ;
#34665=CARTESIAN_POINT('Ctrl Pts',(-20.1045650508994,12.2412937721751,124.749310160121)) ;
#34666=CARTESIAN_POINT('Ctrl Pts',(-19.7737887271615,12.4311564675453,124.561434581507)) ;
#34667=CARTESIAN_POINT('Ctrl Pts',(-19.8649051460095,12.2511673871355,124.848843922395)) ;
#34668=CARTESIAN_POINT('Ctrl Pts',(-19.5671291833791,12.4412287021266,124.607402354197)) ;
#34669=CARTESIAN_POINT('Ctrl Pts',(-19.6065797304147,12.2612396217167,124.906300997573)) ;
#34670=CARTESIAN_POINT('Ctrl Pts',(-19.3607684693909,12.4510527205754,124.616796315158)) ;
#34671=CARTESIAN_POINT('Ctrl Pts',(-19.3486297183274,12.2710636401655,124.918040759742)) ;
#34672=CARTESIAN_POINT('Ctrl Pts',(-19.1509428265166,12.4611176415514,124.589849021404)) ;
#34673=CARTESIAN_POINT('Ctrl Pts',(-19.0863456687307,12.2811285611415,124.884353810288)) ;
#34674=CARTESIAN_POINT('Ctrl Pts',(-18.8857365452566,12.4743279398461,124.507174456424)) ;
#34675=CARTESIAN_POINT('Ctrl Pts',(-18.7548496615418,12.2943388594363,124.781008020419)) ;
#34676=CARTESIAN_POINT('Ctrl Pts',(-18.6462382926402,12.4876433865781,124.356312359537)) ;
#34677=CARTESIAN_POINT('Ctrl Pts',(-18.4555083324541,12.3076543061683,124.592460114514)) ;
#34678=CARTESIAN_POINT('Ctrl Pts',(-18.4564387488717,12.5009336318454,124.15121232202)) ;
#34679=CARTESIAN_POINT('Ctrl Pts',(-18.218215898367,12.3209445514355,124.336043204895)) ;
#34680=CARTESIAN_POINT('Ctrl Pts',(-18.3421528810108,12.5109843814525,123.973529884011)) ;
#34681=CARTESIAN_POINT('Ctrl Pts',(-18.0753697674162,12.3309953010427,124.113946532607)) ;
#34682=CARTESIAN_POINT('Ctrl Pts',(-18.261991671417,12.5207969884347,123.783417454446)) ;
#34683=CARTESIAN_POINT('Ctrl Pts',(-17.9751686261835,12.3408079080249,123.87630326557)) ;
#34684=CARTESIAN_POINT('Ctrl Pts',(-18.2145854633708,12.530868086429,123.5770937702)) ;
#34685=CARTESIAN_POINT('Ctrl Pts',(-17.9159132712724,12.3508790060192,123.618399594221)) ;
#34686=CARTESIAN_POINT('Ctrl Pts',(-18.2041287449214,12.5407576592038,123.369434972959)) ;
#34687=CARTESIAN_POINT('Ctrl Pts',(-17.9028470179378,12.360768578794,123.35882151871)) ;
#34688=CARTESIAN_POINT('Ctrl Pts',(-18.2378495819674,12.5540277660071,123.092473664091)) ;
#34689=CARTESIAN_POINT('Ctrl Pts',(-17.944990032383,12.3740386855973,123.012644489427)) ;
#34690=CARTESIAN_POINT('Ctrl Pts',(-18.3698646515677,12.5706444529296,122.764802678493)) ;
#34691=CARTESIAN_POINT('Ctrl Pts',(-18.1100382420037,12.3906553725198,122.60301895944)) ;
#34692=CARTESIAN_POINT('Ctrl Pts',(-18.6050396672439,12.5872184962459,122.502279793378)) ;
#34693=CARTESIAN_POINT('Ctrl Pts',(-18.4039538091135,12.407229415836,122.274921978535)) ;
#34694=CARTESIAN_POINT('Ctrl Pts',(-18.8388843969827,12.6005150636777,122.349174786392)) ;
#34695=CARTESIAN_POINT('Ctrl Pts',(-18.6963080999189,12.4205259832679,122.083501484913)) ;
#34696=CARTESIAN_POINT('Ctrl Pts',(-19.032708382408,12.6105451272551,122.266104245232)) ;
#34697=CARTESIAN_POINT('Ctrl Pts',(-18.9385791928831,12.4305560468453,121.979673523447)) ;
#34698=CARTESIAN_POINT('Ctrl Pts',(-19.2351868358827,12.6204390191043,122.218590201878)) ;
#34699=CARTESIAN_POINT('Ctrl Pts',(-19.1916818709367,12.4404499386945,121.92028162813)) ;
#34700=CARTESIAN_POINT('Ctrl Pts',(-19.5133724231769,12.6336917748899,122.2020040059)) ;
#34701=CARTESIAN_POINT('Ctrl Pts',(-19.5394009792706,12.45370269448,121.899549493542)) ;
#34702=CARTESIAN_POINT('Ctrl Pts',(-19.8616244702295,12.6504198798823,122.274010765671)) ;
#34703=CARTESIAN_POINT('Ctrl Pts',(-19.9747293753449,12.4704307994725,121.989564308793)) ;
#34704=CARTESIAN_POINT('Ctrl Pts',(-20.2206924205023,12.6702507163608,122.495213042442)) ;
#34705=CARTESIAN_POINT('Ctrl Pts',(-20.4235566592419,12.490261635951,122.266069036596)) ;
#34706=CARTESIAN_POINT('Ctrl Pts',(-20.4846749217705,12.690176108251,122.826464817505)) ;
#34707=CARTESIAN_POINT('Ctrl Pts',(-20.753532722758,12.5101870278411,122.680135635445)) ;
#34708=CARTESIAN_POINT('Ctrl Pts',(-20.6197750422256,12.710101321603,123.228081726851)) ;
#34709=CARTESIAN_POINT('Ctrl Pts',(-20.9224041261866,12.5301122411931,123.182157120568)) ;
#34710=CARTESIAN_POINT('Ctrl Pts',(-20.6098235900098,12.7300263350881,123.651575664266)) ;
#34711=CARTESIAN_POINT('Ctrl Pts',(-20.9099617273898,12.5500372546782,123.711523704273)) ;
#34712=CARTESIAN_POINT('Ctrl Pts',(-20.4568446708067,12.7499028067881,124.045572962216)) ;
#34713=CARTESIAN_POINT('Ctrl Pts',(-20.7187360423288,12.5699137263783,124.204018044757)) ;
#34714=CARTESIAN_POINT('Ctrl Pts',(-20.1773211945259,12.7698821246969,124.36546202135)) ;
#34715=CARTESIAN_POINT('Ctrl Pts',(-20.369330064379,12.5898930442871,124.603877601749)) ;
#34716=CARTESIAN_POINT('Ctrl Pts',(-19.8060899945786,12.7898151282729,124.57002813045)) ;
#34717=CARTESIAN_POINT('Ctrl Pts',(-19.9052905888401,12.6098260478631,124.859582769338)) ;
#34718=CARTESIAN_POINT('Ctrl Pts',(-19.3882558614324,12.8097103983006,124.635945221289)) ;
#34719=CARTESIAN_POINT('Ctrl Pts',(-19.3829989743663,12.6297213178908,124.941977004647)) ;
#34720=CARTESIAN_POINT('Ctrl Pts',(-18.9723404365734,12.8296317362065,124.55563458962)) ;
#34721=CARTESIAN_POINT('Ctrl Pts',(-18.863106015617,12.6496426557967,124.841587523939)) ;
#34722=CARTESIAN_POINT('Ctrl Pts',(-18.6081781423476,12.8495893594727,124.337737107174)) ;
#34723=CARTESIAN_POINT('Ctrl Pts',(-18.4079042834639,12.6696002790628,124.569214869041)) ;
#34724=CARTESIAN_POINT('Ctrl Pts',(-18.3412557610278,12.8694691914299,124.010060659351)) ;
#34725=CARTESIAN_POINT('Ctrl Pts',(-18.0742532723479,12.68948011102,124.159620153189)) ;
#34726=CARTESIAN_POINT('Ctrl Pts',(-18.2010112247405,12.8893510427268,123.611173077498)) ;
#34727=CARTESIAN_POINT('Ctrl Pts',(-17.8989480656809,12.7093619623169,123.661012507465)) ;
#34728=CARTESIAN_POINT('Ctrl Pts',(-18.2061520734863,12.9094220598306,123.184494838161)) ;
#34729=CARTESIAN_POINT('Ctrl Pts',(-17.9053743363055,12.7294329794208,123.127663535491)) ;
#34730=CARTESIAN_POINT('Ctrl Pts',(-18.3545914950356,12.9292292835837,122.790282514626)) ;
#34731=CARTESIAN_POINT('Ctrl Pts',(-18.0909224032178,12.7492402031738,122.634900991588)) ;
#34732=CARTESIAN_POINT('Ctrl Pts',(-18.6302173582225,12.9492104191524,122.467021464749)) ;
#34733=CARTESIAN_POINT('Ctrl Pts',(-18.4354537166866,12.7692213387426,122.230824135061)) ;
#34734=CARTESIAN_POINT('Ctrl Pts',(-18.9990267978771,12.9691379124917,122.258503177642)) ;
#34735=CARTESIAN_POINT('Ctrl Pts',(-18.8964641845817,12.7891488320818,121.970176160886)) ;
#34736=CARTESIAN_POINT('Ctrl Pts',(-19.414525111865,12.9889585738495,122.187284802443)) ;
#34737=CARTESIAN_POINT('Ctrl Pts',(-19.4158344326454,12.8089694934396,121.881151656018)) ;
#34738=CARTESIAN_POINT('Ctrl Pts',(-19.8347816721657,13.0090557630713,122.26378936849)) ;
#34739=CARTESIAN_POINT('Ctrl Pts',(-19.941156659121,12.8290666826614,121.976780869957)) ;
#34740=CARTESIAN_POINT('Ctrl Pts',(-20.1980367737812,13.0288194420796,122.475474924502)) ;
#34741=CARTESIAN_POINT('Ctrl Pts',(-20.3952240685032,12.8488303616698,122.241384544903)) ;
#34742=CARTESIAN_POINT('Ctrl Pts',(-20.47137453339,13.0488767207527,122.802591270838)) ;
#34743=CARTESIAN_POINT('Ctrl Pts',(-20.7368987004734,12.8688876403428,122.650278782987)) ;
#34744=CARTESIAN_POINT('Ctrl Pts',(-20.6146542104524,13.0686721445001,123.198479778478)) ;
#34745=CARTESIAN_POINT('Ctrl Pts',(-20.9159999986636,12.8886830640902,123.145136393703)) ;
#34746=CARTESIAN_POINT('Ctrl Pts',(-20.6155493708649,13.0886357892277,123.622911309277)) ;
#34747=CARTESIAN_POINT('Ctrl Pts',(-20.9171224626867,12.9086467088179,123.675675466357)) ;
#34748=CARTESIAN_POINT('Ctrl Pts',(-20.4704208826885,13.1086192805018,124.022266658295)) ;
#34749=CARTESIAN_POINT('Ctrl Pts',(-20.7357148690054,12.9286302000919,124.174870580525)) ;
#34750=CARTESIAN_POINT('Ctrl Pts',(-20.2007675400314,13.1284267756511,124.345835412524)) ;
#34751=CARTESIAN_POINT('Ctrl Pts',(-20.3986521463661,12.9484376952412,124.579332558928)) ;
#34752=CARTESIAN_POINT('Ctrl Pts',(-19.834022972994,13.1484093663712,124.560193591737)) ;
#34753=CARTESIAN_POINT('Ctrl Pts',(-19.9402235763346,12.9684202859613,124.847283742943)) ;
#34754=CARTESIAN_POINT('Ctrl Pts',(-19.4180361300331,13.1682920203624,124.636116448361)) ;
#34755=CARTESIAN_POINT('Ctrl Pts',(-19.420241605384,12.9883029399526,124.942191223887)) ;
#34756=CARTESIAN_POINT('Ctrl Pts',(-18.9996554886756,13.1882502652255,124.565604893307)) ;
#34757=CARTESIAN_POINT('Ctrl Pts',(-18.897265373855,13.0082611848157,124.854056149891)) ;
#34758=CARTESIAN_POINT('Ctrl Pts',(-18.6317218676168,13.2081258522671,124.357573974673)) ;
#34759=CARTESIAN_POINT('Ctrl Pts',(-18.4373467192626,13.0281367718572,124.594021898984)) ;
#34760=CARTESIAN_POINT('Ctrl Pts',(-18.3552399068354,13.2281067404023,124.035038294504)) ;
#34761=CARTESIAN_POINT('Ctrl Pts',(-18.0917408139602,13.0481176599925,124.1908552924)) ;
#34762=CARTESIAN_POINT('Ctrl Pts',(-18.206044297576,13.2480418815133,123.638227388492)) ;
#34763=CARTESIAN_POINT('Ctrl Pts',(-17.9052414354233,13.0680528011035,123.694844185539)) ;
#34764=CARTESIAN_POINT('Ctrl Pts',(-18.2009152531286,13.2679538995244,123.214915566106)) ;
#34765=CARTESIAN_POINT('Ctrl Pts',(-17.8988271166159,13.0879648191146,123.165702838914)) ;
#34766=CARTESIAN_POINT('Ctrl Pts',(-18.3399734278226,13.287842117768,122.815536644445)) ;
#34767=CARTESIAN_POINT('Ctrl Pts',(-18.0726376302732,13.1078530373582,122.666485551937)) ;
#34768=CARTESIAN_POINT('Ctrl Pts',(-18.5625167302271,13.3044404216149,122.541702141202)) ;
#34769=CARTESIAN_POINT('Ctrl Pts',(-18.350835637743,13.1244513412051,122.324166060029)) ;
#34770=CARTESIAN_POINT('Ctrl Pts',(-18.7884633242958,13.3177130115177,122.377888779236)) ;
#34771=CARTESIAN_POINT('Ctrl Pts',(-18.6332461345366,13.1377239311079,122.119417599734)) ;
#34772=CARTESIAN_POINT('Ctrl Pts',(-18.9775497688346,13.3277204264686,122.285661961006)) ;
#34773=CARTESIAN_POINT('Ctrl Pts',(-18.8696106143379,13.1477313460587,122.004127651188)) ;
#34774=CARTESIAN_POINT('Ctrl Pts',(-19.1798541137618,13.3377277732012,122.227841226343)) ;
#34775=CARTESIAN_POINT('Ctrl Pts',(-19.1224757065686,13.1577386927914,121.9318494161)) ;
#34776=CARTESIAN_POINT('Ctrl Pts',(-19.4571882805755,13.3509941330028,122.198742528533)) ;
#34777=CARTESIAN_POINT('Ctrl Pts',(-19.4692111889478,13.171005052593,121.89547658206)) ;
#34778=CARTESIAN_POINT('Ctrl Pts',(-19.8041191619441,13.3675087906257,122.253086418136)) ;
#34779=CARTESIAN_POINT('Ctrl Pts',(-19.9027886653429,13.1875197102159,121.96339145382)) ;
#34780=CARTESIAN_POINT('Ctrl Pts',(-20.1135332813589,13.3841062238684,122.422657976203)) ;
#34781=CARTESIAN_POINT('Ctrl Pts',(-20.2896179417095,13.2041171434586,122.175375538801)) ;
#34782=CARTESIAN_POINT('Ctrl Pts',(-20.3161488488574,13.3974542210134,122.616898131359)) ;
#34783=CARTESIAN_POINT('Ctrl Pts',(-20.5428541366847,13.2174651406036,122.418153018411)) ;
#34784=CARTESIAN_POINT('Ctrl Pts',(-20.4392682471211,13.407349975365,122.78458790923)) ;
#34785=CARTESIAN_POINT('Ctrl Pts',(-20.6967627805078,13.2273608949552,122.627767557119)) ;
#34786=CARTESIAN_POINT('Ctrl Pts',(-20.5324892710804,13.4173379292963,122.972722988984)) ;
#34787=CARTESIAN_POINT('Ctrl Pts',(-20.8132896637827,13.2373488488865,122.862934128943)) ;
#34788=CARTESIAN_POINT('Ctrl Pts',(-20.5915443850433,13.4272951530011,123.173577963998)) ;
#34789=CARTESIAN_POINT('Ctrl Pts',(-20.8871117691411,13.2473060725913,123.114002366609)) ;
#34790=CARTESIAN_POINT('Ctrl Pts',(-20.6149084211195,13.4373306995577,123.383244466026)) ;
#34791=CARTESIAN_POINT('Ctrl Pts',(-20.9163194698178,13.2573416191479,123.376085199786)) ;
#34792=CARTESIAN_POINT('Ctrl Pts',(-20.6018663431854,13.4472178108339,123.590706984687)) ;
#34793=CARTESIAN_POINT('Ctrl Pts',(-20.9000197112505,13.267228730424,123.63541352092)) ;
#34794=CARTESIAN_POINT('Ctrl Pts',(-20.5528158490788,13.4572092159347,123.794940084393)) ;
#34795=CARTESIAN_POINT('Ctrl Pts',(-20.8387093067792,13.2772201355249,123.890705618854)) ;
#34796=CARTESIAN_POINT('Ctrl Pts',(-20.4693700177335,13.4671548371495,123.986654821614)) ;
#34797=CARTESIAN_POINT('Ctrl Pts',(-20.7344045825384,13.2871657567396,124.130350209197)) ;
#34798=CARTESIAN_POINT('Ctrl Pts',(-20.3542090233936,13.4771040854178,124.161276470942)) ;
#34799=CARTESIAN_POINT('Ctrl Pts',(-20.5904556481203,13.297115005008,124.34862888779)) ;
#34800=CARTESIAN_POINT('Ctrl Pts',(-20.2089077397589,13.4871505805864,124.314549867347)) ;
#34801=CARTESIAN_POINT('Ctrl Pts',(-20.40883104897,13.3071615001766,124.540222615125)) ;
#34802=CARTESIAN_POINT('Ctrl Pts',(-20.0426037732206,13.4970019233779,124.438001198331)) ;
#34803=CARTESIAN_POINT('Ctrl Pts',(-20.2009526791305,13.3170128429681,124.694539108577)) ;
#34804=CARTESIAN_POINT('Ctrl Pts',(-19.8553954660048,13.5069737035053,124.532292944024)) ;
#34805=CARTESIAN_POINT('Ctrl Pts',(-19.9669434550626,13.3269846230954,124.812406349875)) ;
#34806=CARTESIAN_POINT('Ctrl Pts',(-19.6541253092378,13.516968903483,124.592783946963)) ;
#34807=CARTESIAN_POINT('Ctrl Pts',(-19.7153564891538,13.3369798230732,124.888022808534)) ;
#34808=CARTESIAN_POINT('Ctrl Pts',(-19.444620176713,13.527002895179,124.617242515377)) ;
#34809=CARTESIAN_POINT('Ctrl Pts',(-19.4534753611661,13.3470138147692,124.91859882113)) ;
#34810=CARTESIAN_POINT('Ctrl Pts',(-19.2377415370854,13.5368583001515,124.605497638602)) ;
#34811=CARTESIAN_POINT('Ctrl Pts',(-19.1948766730109,13.3568692197417,124.903920505653)) ;
#34812=CARTESIAN_POINT('Ctrl Pts',(-19.0330890851524,13.5468575979973,124.557608984223)) ;
#34813=CARTESIAN_POINT('Ctrl Pts',(-18.9390603846548,13.3668685175874,124.844062381802)) ;
#34814=CARTESIAN_POINT('Ctrl Pts',(-18.8417203854023,13.5567527106025,124.475953276878)) ;
#34815=CARTESIAN_POINT('Ctrl Pts',(-18.6998481883224,13.3767636301927,124.741995186998)) ;
#34816=CARTESIAN_POINT('Ctrl Pts',(-18.6645864621206,13.5668133561375,124.360423798942)) ;
#34817=CARTESIAN_POINT('Ctrl Pts',(-18.4784292945403,13.3868242757276,124.597585675385)) ;
#34818=CARTESIAN_POINT('Ctrl Pts',(-18.5133398637062,13.5766622331267,124.218993175225)) ;
#34819=CARTESIAN_POINT('Ctrl Pts',(-18.2893688820631,13.3966731527169,124.420799145547)) ;
#34820=CARTESIAN_POINT('Ctrl Pts',(-18.3862631485546,13.5866909442203,124.050762009217)) ;
#34821=CARTESIAN_POINT('Ctrl Pts',(-18.1305208052828,13.4067018638104,124.210511784237)) ;
#34822=CARTESIAN_POINT('Ctrl Pts',(-18.2908283109245,13.5967203454764,123.862742118593)) ;
#34823=CARTESIAN_POINT('Ctrl Pts',(-18.0112247909558,13.4167312650665,123.975488167426)) ;
#34824=CARTESIAN_POINT('Ctrl Pts',(-18.2302062670491,13.6065605372724,123.664948493123)) ;
#34825=CARTESIAN_POINT('Ctrl Pts',(-17.9354445008445,13.4265714568625,123.728246471196)) ;
#34826=CARTESIAN_POINT('Ctrl Pts',(-18.2040444170886,13.6165639664654,123.456299673931)) ;
#34827=CARTESIAN_POINT('Ctrl Pts',(-17.9027395318293,13.4365748860555,123.467435684468)) ;
#34828=CARTESIAN_POINT('Ctrl Pts',(-18.2145600866286,13.6265494789316,123.246600447077)) ;
#34829=CARTESIAN_POINT('Ctrl Pts',(-17.9158814572938,13.4465603985218,123.205311390365)) ;
#34830=CARTESIAN_POINT('Ctrl Pts',(-18.2617823017495,13.6365905753156,123.040875922897)) ;
#34831=CARTESIAN_POINT('Ctrl Pts',(-17.9749065837084,13.4566014949057,122.948155155558)) ;
#34832=CARTESIAN_POINT('Ctrl Pts',(-18.3421364497269,13.6464337712666,122.850159429394)) ;
#34833=CARTESIAN_POINT('Ctrl Pts',(-18.075347036012,13.4664446908567,122.709757985418)) ;
#34834=CARTESIAN_POINT('Ctrl Pts',(-18.4556351281271,13.656420082321,122.67358245955)) ;
#34835=CARTESIAN_POINT('Ctrl Pts',(-18.2172182814588,13.4764310019111,122.489035231078)) ;
#34836=CARTESIAN_POINT('Ctrl Pts',(-18.5972804388859,13.6663547675787,122.520040996224)) ;
#34837=CARTESIAN_POINT('Ctrl Pts',(-18.3942732512021,13.4863656871689,122.297106419583)) ;
#34838=CARTESIAN_POINT('Ctrl Pts',(-18.7655457253041,13.6764123287957,122.392050964971)) ;
#34839=CARTESIAN_POINT('Ctrl Pts',(-18.6046031877323,13.4964232483859,122.137116873828)) ;
#34840=CARTESIAN_POINT('Ctrl Pts',(-18.948971596639,13.6862339704043,122.297188134367)) ;
#34841=CARTESIAN_POINT('Ctrl Pts',(-18.8338850494827,13.5062448899945,122.018535713122)) ;
#34842=CARTESIAN_POINT('Ctrl Pts',(-19.150630895694,13.6962900339953,122.233780317479)) ;
#34843=CARTESIAN_POINT('Ctrl Pts',(-19.0859583258677,13.5163009535855,121.939273611485)) ;
#34844=CARTESIAN_POINT('Ctrl Pts',(-19.3579055678042,13.7062307097571,122.207035465086)) ;
#34845=CARTESIAN_POINT('Ctrl Pts',(-19.3450516698188,13.5262416293473,121.905839973704)) ;
#34846=CARTESIAN_POINT('Ctrl Pts',(-19.5659365047634,13.7161350685454,122.215998316577)) ;
#34847=CARTESIAN_POINT('Ctrl Pts',(-19.6050909750298,13.5361459881356,121.917041144566)) ;
#34848=CARTESIAN_POINT('Ctrl Pts',(-19.7721240618805,13.7261817231212,122.26171766678)) ;
#34849=CARTESIAN_POINT('Ctrl Pts',(-19.8628258516087,13.5461926427114,121.974187922095)) ;
#34850=CARTESIAN_POINT('Ctrl Pts',(-19.9644220298839,13.7360773177641,122.341175721282)) ;
#34851=CARTESIAN_POINT('Ctrl Pts',(-20.1031997644219,13.5560882373542,122.073508487828)) ;
#34852=CARTESIAN_POINT('Ctrl Pts',(-20.1429187786372,13.7461392644209,122.454645564807)) ;
#34853=CARTESIAN_POINT('Ctrl Pts',(-20.3263218440841,13.5661501840111,122.215343672174)) ;
#34854=CARTESIAN_POINT('Ctrl Pts',(-20.2957594945872,13.7559888883531,122.594367289572)) ;
#34855=CARTESIAN_POINT('Ctrl Pts',(-20.517374964591,13.5759998079433,122.389994620087)) ;
#34856=CARTESIAN_POINT('Ctrl Pts',(-20.4240087228008,13.7659521273829,122.75995684231)) ;
#34857=CARTESIAN_POINT('Ctrl Pts',(-20.67768845555,13.5859630469731,122.596980439525)) ;
#34858=CARTESIAN_POINT('Ctrl Pts',(-20.5219126757159,13.7759767021588,122.946597688754)) ;
#34859=CARTESIAN_POINT('Ctrl Pts',(-20.8000704182634,13.5959876217489,122.830280403279)) ;
#34860=CARTESIAN_POINT('Ctrl Pts',(-20.5853680857787,13.7858952648465,123.145221491814)) ;
#34861=CARTESIAN_POINT('Ctrl Pts',(-20.8793920084504,13.6059061844367,123.078559981852)) ;
#34862=CARTESIAN_POINT('Ctrl Pts',(-20.6139486861192,13.7958874515705,123.353347867714)) ;
#34863=CARTESIAN_POINT('Ctrl Pts',(-20.9151199376275,13.6158983711606,123.338717822212)) ;
#34864=CARTESIAN_POINT('Ctrl Pts',(-20.6055443985715,13.8059222501547,123.564135174219)) ;
#34865=CARTESIAN_POINT('Ctrl Pts',(-20.9046168526757,13.6259331697448,123.60220196331)) ;
#34866=CARTESIAN_POINT('Ctrl Pts',(-20.5618138969041,13.8157774408283,123.766670893346)) ;
#34867=CARTESIAN_POINT('Ctrl Pts',(-20.849955662852,13.6357883604185,123.855372966765)) ;
#34868=CARTESIAN_POINT('Ctrl Pts',(-20.4827162908005,13.8257767889813,123.961402445332)) ;
#34869=CARTESIAN_POINT('Ctrl Pts',(-20.7510855574627,13.6457877085715,124.098788324471)) ;
#34870=CARTESIAN_POINT('Ctrl Pts',(-20.3723265103831,13.8356719146565,124.137764210175)) ;
#34871=CARTESIAN_POINT('Ctrl Pts',(-20.6130996724061,13.6556828342466,124.319242233536)) ;
#34872=CARTESIAN_POINT('Ctrl Pts',(-20.2306869988819,13.8457324576046,124.294801970209)) ;
#34873=CARTESIAN_POINT('Ctrl Pts',(-20.4360519660552,13.6657433771948,124.515540628951)) ;
#34874=CARTESIAN_POINT('Ctrl Pts',(-20.0674724058813,13.8555817318715,124.422248257044)) ;
#34875=CARTESIAN_POINT('Ctrl Pts',(-20.232034145729,13.6755926514616,124.674850715028)) ;
#34876=CARTESIAN_POINT('Ctrl Pts',(-19.8815742262112,13.8656089564414,124.521635316517)) ;
#34877=CARTESIAN_POINT('Ctrl Pts',(-19.9996623311439,13.6856198760316,124.799086161261)) ;
#34878=CARTESIAN_POINT('Ctrl Pts',(-19.6810321497663,13.8756373556292,124.586723666077)) ;
#34879=CARTESIAN_POINT('Ctrl Pts',(-19.7489854255022,13.6956482752193,124.880448501891)) ;
#34880=CARTESIAN_POINT('Ctrl Pts',(-19.4761166290859,13.8854831060427,124.615846164903)) ;
#34881=CARTESIAN_POINT('Ctrl Pts',(-19.4928401900541,13.7054940256328,124.916853671166)) ;
#34882=CARTESIAN_POINT('Ctrl Pts',(-19.2662085926654,13.8954718964434,124.609433443135)) ;
#34883=CARTESIAN_POINT('Ctrl Pts',(-19.2304548877746,13.7154828160336,124.908839488413)) ;
#34884=CARTESIAN_POINT('Ctrl Pts',(-19.0595750845739,13.9055168248431,124.565911416118)) ;
#34885=CARTESIAN_POINT('Ctrl Pts',(-18.9721627761569,13.7255277444333,124.85443884089)) ;
#34886=CARTESIAN_POINT('Ctrl Pts',(-18.8677390185657,13.9153413096321,124.489339185228)) ;
#34887=CARTESIAN_POINT('Ctrl Pts',(-18.7323658376194,13.7353522292223,124.758724681373)) ;
#34888=CARTESIAN_POINT('Ctrl Pts',(-18.6878125716597,13.9253987071733,124.378319657156)) ;
#34889=CARTESIAN_POINT('Ctrl Pts',(-18.507457139935,13.7454096267634,124.6199518073)) ;
#34890=CARTESIAN_POINT('Ctrl Pts',(-18.5321161135312,13.9353247987595,124.239354765055)) ;
#34891=CARTESIAN_POINT('Ctrl Pts',(-18.3128349524242,13.7553357183497,124.446246569744)) ;
#34892=CARTESIAN_POINT('Ctrl Pts',(-18.4021255349772,13.945279583904,124.075342585797)) ;
#34893=CARTESIAN_POINT('Ctrl Pts',(-18.1503452309058,13.7652905034942,124.241231958288)) ;
#34894=CARTESIAN_POINT('Ctrl Pts',(-18.3019676622171,13.9553169535617,123.889610890228)) ;
#34895=CARTESIAN_POINT('Ctrl Pts',(-18.0251465108619,13.7753278731519,124.009068223175)) ;
#34896=CARTESIAN_POINT('Ctrl Pts',(-18.2364086645203,13.9652057636833,123.692318961985)) ;
#34897=CARTESIAN_POINT('Ctrl Pts',(-17.9431959783341,13.7852166832734,123.762452941038)) ;
#34898=CARTESIAN_POINT('Ctrl Pts',(-18.2054221774035,13.9751951227343,123.484614442852)) ;
#34899=CARTESIAN_POINT('Ctrl Pts',(-17.9044614030354,13.7952060423245,123.502822293368)) ;
#34900=CARTESIAN_POINT('Ctrl Pts',(-18.2111097202979,13.9851536701904,123.275338157667)) ;
#34901=CARTESIAN_POINT('Ctrl Pts',(-17.911569338574,13.8051645897806,123.241226463724)) ;
#34902=CARTESIAN_POINT('Ctrl Pts',(-18.2523005245241,13.9950532467415,123.071321965387)) ;
#34903=CARTESIAN_POINT('Ctrl Pts',(-17.9630567197214,13.8150641663317,122.986205100585)) ;
#34904=CARTESIAN_POINT('Ctrl Pts',(-18.3294851382835,14.0051011585722,122.874712691268)) ;
#34905=CARTESIAN_POINT('Ctrl Pts',(-18.0595361492294,13.8251120781624,122.740443216443)) ;
#34906=CARTESIAN_POINT('Ctrl Pts',(-18.4378511245041,14.0149965064327,122.697097031468)) ;
#34907=CARTESIAN_POINT('Ctrl Pts',(-18.1949930035499,13.8350074260229,122.518422190222)) ;
#34908=CARTESIAN_POINT('Ctrl Pts',(-18.5776635026499,14.0250581829639,122.538393890947)) ;
#34909=CARTESIAN_POINT('Ctrl Pts',(-18.3697572977385,13.8450691025541,122.320042659878)) ;
#34910=CARTESIAN_POINT('Ctrl Pts',(-18.7393445312316,14.0349027007131,122.409181627727)) ;
#34911=CARTESIAN_POINT('Ctrl Pts',(-18.5718588198082,13.8549136203033,122.158525512857)) ;
#34912=CARTESIAN_POINT('Ctrl Pts',(-18.9227751263348,14.0448631444279,122.308189876658)) ;
#34913=CARTESIAN_POINT('Ctrl Pts',(-18.8011469810285,13.864874064018,122.032284729757)) ;
#34914=CARTESIAN_POINT('Ctrl Pts',(-19.1226020522299,14.0548999772461,122.240434925921)) ;
#34915=CARTESIAN_POINT('Ctrl Pts',(-19.0509301231039,13.8749108968362,121.947590006931)) ;
#34916=CARTESIAN_POINT('Ctrl Pts',(-19.3278464181783,14.0647787739929,122.208569582796)) ;
#34917=CARTESIAN_POINT('Ctrl Pts',(-19.3074865101941,13.884789693583,121.907757156914)) ;
#34918=CARTESIAN_POINT('Ctrl Pts',(-19.5392604494556,14.0748380901212,122.212835075085)) ;
#34919=CARTESIAN_POINT('Ctrl Pts',(-19.5717537455762,13.8948490097114,121.913088025212)) ;
#34920=CARTESIAN_POINT('Ctrl Pts',(-19.7428603551298,14.0847085368744,122.252978784912)) ;
#34921=CARTESIAN_POINT('Ctrl Pts',(-19.826254951217,13.9047194564646,121.963266910839)) ;
#34922=CARTESIAN_POINT('Ctrl Pts',(-19.9389874347738,14.0947011751325,122.328256871601)) ;
#34923=CARTESIAN_POINT('Ctrl Pts',(-20.0714142577625,13.9147120947226,122.057363864447)) ;
#34924=CARTESIAN_POINT('Ctrl Pts',(-20.1195329190691,14.1047331906804,122.437257388524)) ;
#34925=CARTESIAN_POINT('Ctrl Pts',(-20.2970965036966,13.9247441102706,122.193613633155)) ;
#34926=CARTESIAN_POINT('Ctrl Pts',(-20.2760952863307,14.114599046987,122.573331296322)) ;
#34927=CARTESIAN_POINT('Ctrl Pts',(-20.4928009018914,13.9346099665771,122.363706237524)) ;
#34928=CARTESIAN_POINT('Ctrl Pts',(-20.4093323895338,14.1246683364561,122.737799807902)) ;
#34929=CARTESIAN_POINT('Ctrl Pts',(-20.6593476165087,13.9446792560463,122.569291069307)) ;
#34930=CARTESIAN_POINT('Ctrl Pts',(-20.5097252080318,14.1345118940074,122.918773104725)) ;
#34931=CARTESIAN_POINT('Ctrl Pts',(-20.7848399903139,13.9545228135976,122.795508554564)) ;
#34932=CARTESIAN_POINT('Ctrl Pts',(-20.5787488120301,14.1444920207952,123.116900923629)) ;
#34933=CARTESIAN_POINT('Ctrl Pts',(-20.8711200645983,13.9645029403854,123.043168459395)) ;
#34934=CARTESIAN_POINT('Ctrl Pts',(-20.6120524726319,14.1545105693952,123.324867150909)) ;
#34935=CARTESIAN_POINT('Ctrl Pts',(-20.9127502837677,13.9745214889854,123.303126129529)) ;
#34936=CARTESIAN_POINT('Ctrl Pts',(-20.6092267809851,14.1643938699184,123.532651027033)) ;
#34937=CARTESIAN_POINT('Ctrl Pts',(-20.9092186327876,13.9844047895085,123.562857078082)) ;
#34938=CARTESIAN_POINT('Ctrl Pts',(-20.5695586363973,14.1744621569665,123.740532636129)) ;
#34939=CARTESIAN_POINT('Ctrl Pts',(-20.8596340363421,13.9944730765567,123.822708783232)) ;
#34940=CARTESIAN_POINT('Ctrl Pts',(-20.4963791598284,14.1842922799851,123.933839607261)) ;
#34941=CARTESIAN_POINT('Ctrl Pts',(-20.7681595372406,14.0043031995753,124.064344085661)) ;
#34942=CARTESIAN_POINT('Ctrl Pts',(-20.3884763220446,14.1943588639105,124.115856989045)) ;
#34943=CARTESIAN_POINT('Ctrl Pts',(-20.6332814623645,14.0143697835007,124.291865630692)) ;
#34944=CARTESIAN_POINT('Ctrl Pts',(-20.2528909010088,14.2042489769249,124.273525084078)) ;
#34945=CARTESIAN_POINT('Ctrl Pts',(-20.4637992773558,14.0242598965151,124.488951781999)) ;
#34946=CARTESIAN_POINT('Ctrl Pts',(-20.0906371997248,14.2142416656876,124.406937747112)) ;
#34947=CARTESIAN_POINT('Ctrl Pts',(-20.2609821100597,14.0342525852777,124.655717889256)) ;
#34948=CARTESIAN_POINT('Ctrl Pts',(-19.9081695184652,14.2242025540433,124.509708404688)) ;
#34949=CARTESIAN_POINT('Ctrl Pts',(-20.0328972096413,14.0442134736335,124.784181661486)) ;
#34950=CARTESIAN_POINT('Ctrl Pts',(-19.7116219047513,14.2341204989233,124.579266374256)) ;
#34951=CARTESIAN_POINT('Ctrl Pts',(-19.7872119389101,14.0541314185135,124.871129498616)) ;
#34952=CARTESIAN_POINT('Ctrl Pts',(-19.5041267455453,14.2441282520195,124.61419846985)) ;
#34953=CARTESIAN_POINT('Ctrl Pts',(-19.5278429325292,14.0641391716097,124.914794637659)) ;
#34954=CARTESIAN_POINT('Ctrl Pts',(-19.2932629141695,14.2541593459786,124.612140808349)) ;
#34955=CARTESIAN_POINT('Ctrl Pts',(-19.2642632651781,14.0741702655688,124.912222739692)) ;
#34956=CARTESIAN_POINT('Ctrl Pts',(-19.0896342106667,14.2640073140066,124.57465995118)) ;
#34957=CARTESIAN_POINT('Ctrl Pts',(-19.0097259981317,14.0840182335967,124.865371406534)) ;
#34958=CARTESIAN_POINT('Ctrl Pts',(-18.8913548972053,14.2740692701324,124.501004306892)) ;
#34959=CARTESIAN_POINT('Ctrl Pts',(-18.7618772163678,14.0940801897226,124.773301901486)) ;
#34960=CARTESIAN_POINT('Ctrl Pts',(-18.7119419266118,14.2839664817336,124.395611023166)) ;
#34961=CARTESIAN_POINT('Ctrl Pts',(-18.5376101428636,14.1039774013237,124.64155978923)) ;
#34962=CARTESIAN_POINT('Ctrl Pts',(-18.5525741212308,14.2938976483982,124.260736428545)) ;
#34963=CARTESIAN_POINT('Ctrl Pts',(-18.3384000135409,14.1139085679884,124.472965869056)) ;
#34964=CARTESIAN_POINT('Ctrl Pts',(-18.4177287010278,14.3039398326024,124.098297375406)) ;
#34965=CARTESIAN_POINT('Ctrl Pts',(-18.1698435133763,14.1239507521926,124.269917095333)) ;
#34966=CARTESIAN_POINT('Ctrl Pts',(-18.3146195122506,14.3138265008555,123.917815954086)) ;
#34967=CARTESIAN_POINT('Ctrl Pts',(-18.0409566998059,14.1338374204457,124.044314254014)) ;
#34968=CARTESIAN_POINT('Ctrl Pts',(-18.2433338154398,14.3238196128338,123.720204704618)) ;
#34969=CARTESIAN_POINT('Ctrl Pts',(-17.9518498697471,14.143830532424,123.797299870413)) ;
#34970=CARTESIAN_POINT('Ctrl Pts',(-18.2076886193533,14.3337652904496,123.514175880864)) ;
#34971=CARTESIAN_POINT('Ctrl Pts',(-17.9072936183919,14.1537762100398,123.539763194416)) ;
#34972=CARTESIAN_POINT('Ctrl Pts',(-18.2079318857893,14.3437125934346,123.305042620039)) ;
#34973=CARTESIAN_POINT('Ctrl Pts',(-17.9075982210939,14.1637235130248,123.278346044338)) ;
#34974=CARTESIAN_POINT('Ctrl Pts',(-18.2450800860336,14.3537603171813,123.09710524755)) ;
#34975=CARTESIAN_POINT('Ctrl Pts',(-17.9540338466966,14.1737712367715,123.018424649751)) ;
#34976=CARTESIAN_POINT('Ctrl Pts',(-18.3161751561514,14.3636086909439,122.902654315691)) ;
#34977=CARTESIAN_POINT('Ctrl Pts',(-18.0429036249904,14.183619610534,122.775359841239)) ;
#34978=CARTESIAN_POINT('Ctrl Pts',(-18.420516020689,14.3735676633896,122.72113759086)) ;
#34979=CARTESIAN_POINT('Ctrl Pts',(-18.1733306007622,14.1935785829798,122.548463907935)) ;
#34980=CARTESIAN_POINT('Ctrl Pts',(-18.5561553946168,14.3836065252707,122.559457330409)) ;
#34981=CARTESIAN_POINT('Ctrl Pts',(-18.3428801887361,14.2036174448609,122.346364098496)) ;
#34982=CARTESIAN_POINT('Ctrl Pts',(-18.7150352575607,14.3934851294425,122.425678518084)) ;
#34983=CARTESIAN_POINT('Ctrl Pts',(-18.5414813531674,14.2134960490327,122.179140432191)) ;
#34984=CARTESIAN_POINT('Ctrl Pts',(-18.8977873014348,14.4035366706458,122.319642116266)) ;
#34985=CARTESIAN_POINT('Ctrl Pts',(-18.7699215574905,14.223547590236,122.046595739421)) ;
#34986=CARTESIAN_POINT('Ctrl Pts',(-19.0931303673642,14.4134320686262,122.247993391467)) ;
#34987=CARTESIAN_POINT('Ctrl Pts',(-19.0141015690506,14.2334429882164,121.957035255703)) ;
#34988=CARTESIAN_POINT('Ctrl Pts',(-19.3010884804579,14.4234833011715,122.21067275502)) ;
#34989=CARTESIAN_POINT('Ctrl Pts',(-19.274049100191,14.2434942207616,121.910385335616)) ;
#34990=CARTESIAN_POINT('Ctrl Pts',(-19.5089481133767,14.4333694917958,122.210014197756)) ;
#34991=CARTESIAN_POINT('Ctrl Pts',(-19.5338747027571,14.253380411386,121.909562985826)) ;
#34992=CARTESIAN_POINT('Ctrl Pts',(-19.7159932801428,14.4433620311115,122.245450565557)) ;
#34993=CARTESIAN_POINT('Ctrl Pts',(-19.7926811889732,14.2633729507017,121.95385946467)) ;
#34994=CARTESIAN_POINT('Ctrl Pts',(-19.9128752055225,14.4533104770063,122.316060788436)) ;
#34995=CARTESIAN_POINT('Ctrl Pts',(-20.0387837795195,14.2733213965964,122.042123340341)) ;
#34996=CARTESIAN_POINT('Ctrl Pts',(-20.0944137100652,14.4632472795382,122.419388130175)) ;
#34997=CARTESIAN_POINT('Ctrl Pts',(-20.2657069288682,14.2832581991283,122.171283774694)) ;
#34998=CARTESIAN_POINT('Ctrl Pts',(-20.2562053966534,14.4732302869895,122.553111371439)) ;
#34999=CARTESIAN_POINT('Ctrl Pts',(-20.4679459835785,14.2932412065796,122.338438899013)) ;
#35000=CARTESIAN_POINT('Ctrl Pts',(-20.3928213225405,14.4832741284043,122.714082144546)) ;
#35001=CARTESIAN_POINT('Ctrl Pts',(-20.6387149775049,14.3032850479944,122.539652891453)) ;
#35002=CARTESIAN_POINT('Ctrl Pts',(-20.4975727490238,14.4931023270282,122.892216003962)) ;
#35003=CARTESIAN_POINT('Ctrl Pts',(-20.7696539437526,14.3131132466183,122.762322078402)) ;
#35004=CARTESIAN_POINT('Ctrl Pts',(-20.5716961928806,14.5031789204704,123.09062015157)) ;
#35005=CARTESIAN_POINT('Ctrl Pts',(-20.8623069214646,14.3231898400606,123.010327296313)) ;
#35006=CARTESIAN_POINT('Ctrl Pts',(-20.6095053348988,14.513030919812,123.29430613063)) ;
#35007=CARTESIAN_POINT('Ctrl Pts',(-20.9095673064433,14.3330418394022,123.264936220777)) ;
#35008=CARTESIAN_POINT('Ctrl Pts',(-20.6115890759441,14.5231045066358,123.506038201766)) ;
#35009=CARTESIAN_POINT('Ctrl Pts',(-20.9121706249676,14.343115426226,123.529600919864)) ;
#35010=CARTESIAN_POINT('Ctrl Pts',(-20.5776337189286,14.5329447317333,123.710123522401)) ;
#35011=CARTESIAN_POINT('Ctrl Pts',(-20.8697248958997,14.3529556513235,123.784708643361)) ;
#35012=CARTESIAN_POINT('Ctrl Pts',(-20.5085876603415,14.542910435762,123.907911470471)) ;
#35013=CARTESIAN_POINT('Ctrl Pts',(-20.7834156859523,14.3629213553522,124.031943418865)) ;
#35014=CARTESIAN_POINT('Ctrl Pts',(-20.4053409396209,14.5529370690686,124.091700513601)) ;
#35015=CARTESIAN_POINT('Ctrl Pts',(-20.6543560175657,14.3729479886588,124.261678938425)) ;
#35016=CARTESIAN_POINT('Ctrl Pts',(-20.2733679541214,14.5628513647804,124.253019570529)) ;
#35017=CARTESIAN_POINT('Ctrl Pts',(-20.489388131609,14.3828622843705,124.463327357363)) ;
#35018=CARTESIAN_POINT('Ctrl Pts',(-20.1144447570708,14.5728396534728,124.390287718717)) ;
#35019=CARTESIAN_POINT('Ctrl Pts',(-20.290732899766,14.392850573063,124.63491140998)) ;
#35020=CARTESIAN_POINT('Ctrl Pts',(-19.93300982332,14.5828783866312,124.498080446046)) ;
#35021=CARTESIAN_POINT('Ctrl Pts',(-20.0639385669917,14.4028893062214,124.769650931618)) ;
#35022=CARTESIAN_POINT('Ctrl Pts',(-19.739575472665,14.5927217184587,124.571609128069)) ;
#35023=CARTESIAN_POINT('Ctrl Pts',(-19.8221438934976,14.4127326380489,124.8615606774)) ;
#35024=CARTESIAN_POINT('Ctrl Pts',(-19.5325945345893,14.6027494443383,124.611640004367)) ;
#35025=CARTESIAN_POINT('Ctrl Pts',(-19.5634174500555,14.4227603639285,124.911597480162)) ;
#35026=CARTESIAN_POINT('Ctrl Pts',(-19.3216956220107,14.6127817807269,124.614552263941)) ;
#35027=CARTESIAN_POINT('Ctrl Pts',(-19.2997938732226,14.4327927003171,124.915236180564)) ;
#35028=CARTESIAN_POINT('Ctrl Pts',(-19.1176575039999,14.6226112810275,124.581899390616)) ;
#35029=CARTESIAN_POINT('Ctrl Pts',(-19.0447452472137,14.4426222006177,124.874418148629)) ;
#35030=CARTESIAN_POINT('Ctrl Pts',(-18.9189866148987,14.6326007849443,124.513805611947)) ;
#35031=CARTESIAN_POINT('Ctrl Pts',(-18.796407103044,14.4526117045345,124.789299015811)) ;
#35032=CARTESIAN_POINT('Ctrl Pts',(-18.7344236623876,14.6426446254567,124.411231786097)) ;
#35033=CARTESIAN_POINT('Ctrl Pts',(-18.5657044122113,14.4626555450469,124.661080239987)) ;
#35034=CARTESIAN_POINT('Ctrl Pts',(-18.5738301995033,14.6524663312247,124.281444401144)) ;
#35035=CARTESIAN_POINT('Ctrl Pts',(-18.3649628203968,14.4724772508149,124.498843726506)) ;
#35036=CARTESIAN_POINT('Ctrl Pts',(-18.4348762560386,14.6625013783571,124.122702247143)) ;
#35037=CARTESIAN_POINT('Ctrl Pts',(-18.1912720234791,14.4825122979473,124.30041474658)) ;
#35038=CARTESIAN_POINT('Ctrl Pts',(-18.3262031256769,14.672526055794,123.942122520734)) ;
#35039=CARTESIAN_POINT('Ctrl Pts',(-18.0554322543384,14.4925369753842,124.074689128033)) ;
#35040=CARTESIAN_POINT('Ctrl Pts',(-18.2514273159942,14.6823788706484,123.748954040769)) ;
#35041=CARTESIAN_POINT('Ctrl Pts',(-17.9619640242134,14.5023897902386,123.833226852774)) ;
#35042=CARTESIAN_POINT('Ctrl Pts',(-18.2104197904952,14.692366580256,123.543040108188)) ;
#35043=CARTESIAN_POINT('Ctrl Pts',(-17.9107066773587,14.5123774998462,123.575833839673)) ;
#35044=CARTESIAN_POINT('Ctrl Pts',(-18.2058049225117,14.7022965902501,123.334323737137)) ;
#35045=CARTESIAN_POINT('Ctrl Pts',(-17.9049402190557,14.5223075098402,123.314937805643)) ;
#35046=CARTESIAN_POINT('Ctrl Pts',(-18.2373702335,14.7122863454692,123.126689249675)) ;
#35047=CARTESIAN_POINT('Ctrl Pts',(-17.9443990826617,14.5322972650594,123.055394867525)) ;
#35048=CARTESIAN_POINT('Ctrl Pts',(-18.3050137193924,14.7223129541521,122.927042802694)) ;
#35049=CARTESIAN_POINT('Ctrl Pts',(-18.0289554644761,14.5423238737423,122.805837532128)) ;
#35050=CARTESIAN_POINT('Ctrl Pts',(-18.4046749189677,14.732196894174,122.744715504703)) ;
#35051=CARTESIAN_POINT('Ctrl Pts',(-18.1535342536619,14.5522078137641,122.577928818051)) ;
#35052=CARTESIAN_POINT('Ctrl Pts',(-18.5354880156566,14.7421861217125,122.580419937995)) ;
#35053=CARTESIAN_POINT('Ctrl Pts',(-18.3170525413856,14.5621970413027,122.3725606859)) ;
#35054=CARTESIAN_POINT('Ctrl Pts',(-18.6939694465223,14.7522289922362,122.44092045882)) ;
#35055=CARTESIAN_POINT('Ctrl Pts',(-18.5151557257253,14.5722399118263,122.198188061641)) ;
#35056=CARTESIAN_POINT('Ctrl Pts',(-18.8703137137284,14.7620613789916,122.333079749863)) ;
#35057=CARTESIAN_POINT('Ctrl Pts',(-18.7355880780225,14.5820722985817,122.063388638373)) ;
#35058=CARTESIAN_POINT('Ctrl Pts',(-19.0656282841589,14.7720546721632,122.255693489157)) ;
#35059=CARTESIAN_POINT('Ctrl Pts',(-18.9797323075833,14.5920655917533,121.966658037037)) ;
#35060=CARTESIAN_POINT('Ctrl Pts',(-19.2723122403626,14.7820866778116,122.213661473494)) ;
#35061=CARTESIAN_POINT('Ctrl Pts',(-19.2380876823512,14.6020975974018,121.914120317217)) ;
#35062=CARTESIAN_POINT('Ctrl Pts',(-19.4796224788741,14.7919519337806,122.207990741201)) ;
#35063=CARTESIAN_POINT('Ctrl Pts',(-19.4972262784245,14.6119628533708,121.907034280903)) ;
#35064=CARTESIAN_POINT('Ctrl Pts',(-19.686880956539,14.8019138136881,122.238115152982)) ;
#35065=CARTESIAN_POINT('Ctrl Pts',(-19.7562992627318,14.6219247332783,121.94469233049)) ;
#35066=CARTESIAN_POINT('Ctrl Pts',(-19.8870940592205,14.81194874705,122.304572113576)) ;
#35067=CARTESIAN_POINT('Ctrl Pts',(-20.0065648350641,14.6319596666402,122.027765848193)) ;
#35068=CARTESIAN_POINT('Ctrl Pts',(-20.0701544259768,14.8218337054293,122.402996415654)) ;
#35069=CARTESIAN_POINT('Ctrl Pts',(-20.2353895991696,14.6418446250194,122.15079871557)) ;
#35070=CARTESIAN_POINT('Ctrl Pts',(-20.2362472111695,14.8318993323519,122.534060407699)) ;
#35071=CARTESIAN_POINT('Ctrl Pts',(-20.4430039040202,14.6519102519421,122.314630587394)) ;
#35072=CARTESIAN_POINT('Ctrl Pts',(-20.3740932209751,14.8417384380163,122.688329422969)) ;
#35073=CARTESIAN_POINT('Ctrl Pts',(-20.6153099875451,14.6617493576065,122.507469086889)) ;
#35074=CARTESIAN_POINT('Ctrl Pts',(-20.4857432775784,14.8518012530216,122.867986014556)) ;
#35075=CARTESIAN_POINT('Ctrl Pts',(-20.754870275489,14.6718121726118,122.73204108607)) ;
#35076=CARTESIAN_POINT('Ctrl Pts',(-20.5630404308717,14.8616974590703,123.061166562861)) ;
#35077=CARTESIAN_POINT('Ctrl Pts',(-20.8514895077048,14.6817083786605,122.973518167633)) ;
#35078=CARTESIAN_POINT('Ctrl Pts',(-20.6063727048954,14.8716382820956,123.265587679795)) ;
#35079=CARTESIAN_POINT('Ctrl Pts',(-20.9056522988101,14.6916492016857,123.229045388468)) ;
#35080=CARTESIAN_POINT('Ctrl Pts',(-20.6136516344617,14.8816428650742,123.47581329813)) ;
#35081=CARTESIAN_POINT('Ctrl Pts',(-20.9147482972965,14.7016537846644,123.491827573855)) ;
#35082=CARTESIAN_POINT('Ctrl Pts',(-20.5840199308421,14.891663759519,123.684384900853)) ;
#35083=CARTESIAN_POINT('Ctrl Pts',(-20.8777060566585,14.7116746791091,123.752541737889)) ;
#35084=CARTESIAN_POINT('Ctrl Pts',(-20.5197082244626,14.9015556801084,123.882155751433)) ;
#35085=CARTESIAN_POINT('Ctrl Pts',(-20.7973137584208,14.7215665996986,123.999754867633)) ;
#35086=CARTESIAN_POINT('Ctrl Pts',(-20.4213024996246,14.9115491124538,124.067769431274)) ;
#35087=CARTESIAN_POINT('Ctrl Pts',(-20.6743041570178,14.731560032044,124.231770793008)) ;
#35088=CARTESIAN_POINT('Ctrl Pts',(-20.2927239230316,14.9214947173536,124.232648085746)) ;
#35089=CARTESIAN_POINT('Ctrl Pts',(-20.5135786632447,14.7415056369438,124.437867633148)) ;
#35090=CARTESIAN_POINT('Ctrl Pts',(-20.1377200748608,14.9314419908352,124.373043867283)) ;
#35091=CARTESIAN_POINT('Ctrl Pts',(-20.3198218573986,14.7514529104254,124.613360457507)) ;
#35092=CARTESIAN_POINT('Ctrl Pts',(-19.9587916673367,14.9414899053115,124.485309172283)) ;
#35093=CARTESIAN_POINT('Ctrl Pts',(-20.0961599099741,14.7615008249017,124.753689774918)) ;
#35094=CARTESIAN_POINT('Ctrl Pts',(-19.7670469759163,14.9513375456589,124.563382819774)) ;
#35095=CARTESIAN_POINT('Ctrl Pts',(-19.8564776376896,14.7713484652491,124.851279444963)) ;
#35096=CARTESIAN_POINT('Ctrl Pts',(-19.5624646344758,14.9612992610355,124.608121127697)) ;
#35097=CARTESIAN_POINT('Ctrl Pts',(-19.6007489896313,14.7813101806256,124.907199618472)) ;
#35098=CARTESIAN_POINT('Ctrl Pts',(-19.3517826029045,14.9713278846083,124.61644912002)) ;
#35099=CARTESIAN_POINT('Ctrl Pts',(-19.337396297839,14.7913388041985,124.917606836361)) ;
#35100=CARTESIAN_POINT('Ctrl Pts',(-19.145332332827,14.9812382466747,124.588473295284)) ;
#35101=CARTESIAN_POINT('Ctrl Pts',(-19.0793336230859,14.8012491662649,124.882634265832)) ;
#35102=CARTESIAN_POINT('Ctrl Pts',(-18.9462038692032,14.9911729403271,124.525440044832)) ;
#35103=CARTESIAN_POINT('Ctrl Pts',(-18.8304237660686,14.8111838599173,124.803839977421)) ;
#35104=CARTESIAN_POINT('Ctrl Pts',(-18.7591614865791,15.001214783455,124.427569567412)) ;
#35105=CARTESIAN_POINT('Ctrl Pts',(-18.5966220484601,14.8212257030451,124.681499373947)) ;
#35106=CARTESIAN_POINT('Ctrl Pts',(-18.5944360678556,15.0110992890254,124.300855256588)) ;
#35107=CARTESIAN_POINT('Ctrl Pts',(-18.3907168604578,14.8311102086156,124.5231041557)) ;
#35108=CARTESIAN_POINT('Ctrl Pts',(-18.4524001316479,15.0211013928106,124.145842998901)) ;
#35109=CARTESIAN_POINT('Ctrl Pts',(-18.2131739735761,14.8411123124008,124.329336878976)) ;
#35110=CARTESIAN_POINT('Ctrl Pts',(-18.3402023620306,15.0310197442256,123.970045804479)) ;
#35111=CARTESIAN_POINT('Ctrl Pts',(-18.0729290956119,14.8510306638158,124.109588770711)) ;
#35112=CARTESIAN_POINT('Ctrl Pts',(-18.2592672869496,15.0410674002465,123.774968507367)) ;
#35113=CARTESIAN_POINT('Ctrl Pts',(-17.9717628131797,14.8610783198367,123.865741080734)) ;
#35114=CARTESIAN_POINT('Ctrl Pts',(-18.2139943917343,15.0509385932747,123.572398931231)) ;
#35115=CARTESIAN_POINT('Ctrl Pts',(-17.91517451057,14.8709495128648,123.612528140346)) ;
#35116=CARTESIAN_POINT('Ctrl Pts',(-18.2043671465967,15.0610043064182,123.361053655738)) ;
#35117=CARTESIAN_POINT('Ctrl Pts',(-17.9031429830698,14.8810152260084,123.348347430976)) ;
#35118=CARTESIAN_POINT('Ctrl Pts',(-18.2307795956915,15.0708567669908,123.155558216153)) ;
#35119=CARTESIAN_POINT('Ctrl Pts',(-17.9361624248919,14.890867686581,123.091474379818)) ;
#35120=CARTESIAN_POINT('Ctrl Pts',(-18.314927021648,15.0842852297134,122.886155404172)) ;
#35121=CARTESIAN_POINT('Ctrl Pts',(-18.0413449334992,14.9042961493036,122.754742299767)) ;
#35122=CARTESIAN_POINT('Ctrl Pts',(-18.4633001207492,15.0973661772305,122.650732206668)) ;
#35123=CARTESIAN_POINT('Ctrl Pts',(-18.2267874469452,14.9173770968207,122.460483907538)) ;
#35124=CARTESIAN_POINT('Ctrl Pts',(-18.6709215131284,15.110840675465,122.458175069999)) ;
#35125=CARTESIAN_POINT('Ctrl Pts',(-18.4863543902457,14.9308515950552,122.219747666795)) ;
#35126=CARTESIAN_POINT('Ctrl Pts',(-18.8447665738617,15.1206727790745,122.346277793249)) ;
#35127=CARTESIAN_POINT('Ctrl Pts',(-18.703654434162,14.9406836986647,122.079886991897)) ;
#35128=CARTESIAN_POINT('Ctrl Pts',(-19.0375991766532,15.1306386822012,122.264426190155)) ;
#35129=CARTESIAN_POINT('Ctrl Pts',(-18.9446987350961,14.9506496017914,121.977572950956)) ;
#35130=CARTESIAN_POINT('Ctrl Pts',(-19.2431027809361,15.1406660915114,122.217314375215)) ;
#35131=CARTESIAN_POINT('Ctrl Pts',(-19.201576591091,14.9606770111016,121.918685704646)) ;
#35132=CARTESIAN_POINT('Ctrl Pts',(-19.4511603917055,15.150577122878,122.206669239406)) ;
#35133=CARTESIAN_POINT('Ctrl Pts',(-19.4616556588076,14.9705880424682,121.905384721544)) ;
#35134=CARTESIAN_POINT('Ctrl Pts',(-19.7276733496542,15.163821430499,122.240072867962)) ;
#35135=CARTESIAN_POINT('Ctrl Pts',(-19.8072618039582,14.9838323500892,121.947128778278)) ;
#35136=CARTESIAN_POINT('Ctrl Pts',(-20.0569080569754,15.1805219131702,122.372778838028)) ;
#35137=CARTESIAN_POINT('Ctrl Pts',(-20.2188550942101,15.0005328327604,122.11304531212)) ;
#35138=CARTESIAN_POINT('Ctrl Pts',(-20.3183298277955,15.197028742326,122.607156814012)) ;
#35139=CARTESIAN_POINT('Ctrl Pts',(-20.5455679442295,15.0170396619161,122.405960959444)) ;
#35140=CARTESIAN_POINT('Ctrl Pts',(-20.4717021929632,15.2103393705636,122.841112767138)) ;
#35141=CARTESIAN_POINT('Ctrl Pts',(-20.737326239263,15.0303502901537,122.698457845472)) ;
#35142=CARTESIAN_POINT('Ctrl Pts',(-20.5546889086436,15.2203319341037,123.034149268203)) ;
#35143=CARTESIAN_POINT('Ctrl Pts',(-20.8410482038523,15.0403428536938,122.939743261864)) ;
#35144=CARTESIAN_POINT('Ctrl Pts',(-20.6028117634593,15.2303620171052,123.239415681091)) ;
#35145=CARTESIAN_POINT('Ctrl Pts',(-20.9012011781756,15.0503729366954,123.196334518987)) ;
#35146=CARTESIAN_POINT('Ctrl Pts',(-20.6188231290724,15.243535621103,123.51597584994)) ;
#35147=CARTESIAN_POINT('Ctrl Pts',(-20.9212136814525,15.0635465406931,123.542009444159)) ;
#35148=CARTESIAN_POINT('Ctrl Pts',(-20.5476924046879,15.2601733263344,123.862358698214)) ;
#35149=CARTESIAN_POINT('Ctrl Pts',(-20.8322977308668,15.0801842459246,123.975012112059)) ;
#35150=CARTESIAN_POINT('Ctrl Pts',(-20.3266298052787,15.2800550889018,124.222868771879)) ;
#35151=CARTESIAN_POINT('Ctrl Pts',(-20.5559470864742,15.100066008492,124.425649304141)) ;
#35152=CARTESIAN_POINT('Ctrl Pts',(-20.0488038588937,15.2967514411183,124.443780899376)) ;
#35153=CARTESIAN_POINT('Ctrl Pts',(-20.2087222530753,15.1167623607085,124.701752625818)) ;
#35154=CARTESIAN_POINT('Ctrl Pts',(-19.7952370287234,15.3099084689074,124.554316113986)) ;
#35155=CARTESIAN_POINT('Ctrl Pts',(-19.8917080630765,15.1299193884976,124.839949683747)) ;
#35156=CARTESIAN_POINT('Ctrl Pts',(-19.5219729563658,15.3232858235509,124.620769738121)) ;
#35157=CARTESIAN_POINT('Ctrl Pts',(-19.5501536847706,15.1432967431411,124.923007742519)) ;
#35158=CARTESIAN_POINT('Ctrl Pts',(-19.1705511769297,15.3398166578097,124.612563673835)) ;
#35159=CARTESIAN_POINT('Ctrl Pts',(-19.1108554066157,15.1598275773999,124.912748434197)) ;
#35160=CARTESIAN_POINT('Ctrl Pts',(-18.7747945960682,15.3597813475528,124.459104510139)) ;
#35161=CARTESIAN_POINT('Ctrl Pts',(-18.6161685027827,15.179792267143,124.720920100974)) ;
#35162=CARTESIAN_POINT('Ctrl Pts',(-18.4561643055464,15.3796978409765,124.180149863833)) ;
#35163=CARTESIAN_POINT('Ctrl Pts',(-18.2178819294633,15.1997087605666,124.372224270665)) ;
#35164=CARTESIAN_POINT('Ctrl Pts',(-18.2513709239315,15.399587560326,123.810085056575)) ;
#35165=CARTESIAN_POINT('Ctrl Pts',(-17.9618943673674,15.2195984799162,123.909642300163)) ;
#35166=CARTESIAN_POINT('Ctrl Pts',(-18.185122044345,15.4195942899739,123.38994096914)) ;
#35167=CARTESIAN_POINT('Ctrl Pts',(-17.8790867339496,15.2396052095641,123.384461553135)) ;
#35168=CARTESIAN_POINT('Ctrl Pts',(-18.2652543652805,15.4394323436208,122.975722101847)) ;
#35169=CARTESIAN_POINT('Ctrl Pts',(-17.9792551414106,15.259443263211,122.866690154542)) ;
#35170=CARTESIAN_POINT('Ctrl Pts',(-18.4831677244092,15.4594256818344,122.610800320768)) ;
#35171=CARTESIAN_POINT('Ctrl Pts',(-18.2516493429581,15.2794366014246,122.410539526365)) ;
#35172=CARTESIAN_POINT('Ctrl Pts',(-18.8109961180814,15.479308481241,122.343735818946)) ;
#35173=CARTESIAN_POINT('Ctrl Pts',(-18.661435692943,15.2993194008312,122.076711965895)) ;
#35174=CARTESIAN_POINT('Ctrl Pts',(-19.2100433870964,15.4992006621597,122.203893854528)) ;
#35175=CARTESIAN_POINT('Ctrl Pts',(-19.1602442446261,15.3192115817499,121.901912195457)) ;
#35176=CARTESIAN_POINT('Ctrl Pts',(-19.6333249972784,15.5191028406548,122.207913004512)) ;
#35177=CARTESIAN_POINT('Ctrl Pts',(-19.6893450348299,15.3391137602449,121.906937811133)) ;
#35178=CARTESIAN_POINT('Ctrl Pts',(-20.0320344555378,15.5391401518585,122.357748545318)) ;
#35179=CARTESIAN_POINT('Ctrl Pts',(-20.1877316481342,15.3591510714487,122.094234259149)) ;
#35180=CARTESIAN_POINT('Ctrl Pts',(-20.3526586672201,15.5589525933994,122.631285692703)) ;
#35181=CARTESIAN_POINT('Ctrl Pts',(-20.5885091138789,15.3789635129896,122.43615506045)) ;
#35182=CARTESIAN_POINT('Ctrl Pts',(-20.5630361294496,15.5790178341343,123.002216406184)) ;
#35183=CARTESIAN_POINT('Ctrl Pts',(-20.851480272865,15.3990287537244,122.89981981938)) ;
#35184=CARTESIAN_POINT('Ctrl Pts',(-20.633508538707,15.5987750389901,123.416561760013)) ;
#35185=CARTESIAN_POINT('Ctrl Pts',(-20.9395694670028,15.4187859585803,123.417748054594)) ;
#35186=CARTESIAN_POINT('Ctrl Pts',(-20.5580007528934,15.6188083116358,123.835558911533)) ;
#35187=CARTESIAN_POINT('Ctrl Pts',(-20.8451846343238,15.438819231226,123.941494843155)) ;
#35188=CARTESIAN_POINT('Ctrl Pts',(-20.3461462838386,15.6386212200896,124.199911351364)) ;
#35189=CARTESIAN_POINT('Ctrl Pts',(-20.5803681949972,15.4586321396798,124.39693299142)) ;
#35190=CARTESIAN_POINT('Ctrl Pts',(-20.0203388845668,15.6586173662171,124.472784286855)) ;
#35191=CARTESIAN_POINT('Ctrl Pts',(-20.1731096406132,15.4786282858072,124.738024765077)) ;
#35192=CARTESIAN_POINT('Ctrl Pts',(-19.6233743789427,15.6784791194396,124.617449122825)) ;
#35193=CARTESIAN_POINT('Ctrl Pts',(-19.6769061894304,15.4984900390297,124.91885633034)) ;
#35194=CARTESIAN_POINT('Ctrl Pts',(-19.1967590474696,15.6985476365677,124.617705022532)) ;
#35195=CARTESIAN_POINT('Ctrl Pts',(-19.1436360481896,15.5185585561579,124.919177517844)) ;
#35196=CARTESIAN_POINT('Ctrl Pts',(-18.8003320264179,15.7183785095645,124.473760456347)) ;
#35197=CARTESIAN_POINT('Ctrl Pts',(-18.6481039856048,15.5383894291547,124.73924884154)) ;
#35198=CARTESIAN_POINT('Ctrl Pts',(-18.4747503929125,15.7383004203812,124.20293742243)) ;
#35199=CARTESIAN_POINT('Ctrl Pts',(-18.2411262733989,15.5583113399714,124.400722475614)) ;
#35200=CARTESIAN_POINT('Ctrl Pts',(-18.2610720953533,15.7582298638165,123.836921398904)) ;
#35201=CARTESIAN_POINT('Ctrl Pts',(-17.9740267389869,15.5782407834067,123.943204335261)) ;
#35202=CARTESIAN_POINT('Ctrl Pts',(-18.185068198707,15.7781395339329,123.420531358687)) ;
#35203=CARTESIAN_POINT('Ctrl Pts',(-17.8790194222821,15.5981504535231,123.422718308583)) ;
#35204=CARTESIAN_POINT('Ctrl Pts',(-18.2548638512684,15.7980128911957,123.003722761479)) ;
#35205=CARTESIAN_POINT('Ctrl Pts',(-17.9662605747909,15.6180238107859,122.901708304032)) ;
#35206=CARTESIAN_POINT('Ctrl Pts',(-18.4639568410273,15.8180044258137,122.633696412297)) ;
#35207=CARTESIAN_POINT('Ctrl Pts',(-18.2276238438955,15.6380153454039,122.439173769106)) ;
#35208=CARTESIAN_POINT('Ctrl Pts',(-18.7847146040937,15.8378700432244,122.358763046612)) ;
#35209=CARTESIAN_POINT('Ctrl Pts',(-18.6285678008825,15.6578809628146,122.095505124919)) ;
#35210=CARTESIAN_POINT('Ctrl Pts',(-19.182109206407,15.8578509730526,122.208558793697)) ;
#35211=CARTESIAN_POINT('Ctrl Pts',(-19.1253095706603,15.6778618926428,121.907746173934)) ;
#35212=CARTESIAN_POINT('Ctrl Pts',(-19.606033490729,15.8777894351358,122.203463863361)) ;
#35213=CARTESIAN_POINT('Ctrl Pts',(-19.6552143908166,15.6978003547259,121.90137366034)) ;
#35214=CARTESIAN_POINT('Ctrl Pts',(-20.0055761170638,15.8976816283575,122.342403399768)) ;
#35215=CARTESIAN_POINT('Ctrl Pts',(-20.1546433032403,15.7176925479477,122.075043824331)) ;
#35216=CARTESIAN_POINT('Ctrl Pts',(-20.3347791009066,15.9176523433929,122.61046686242)) ;
#35217=CARTESIAN_POINT('Ctrl Pts',(-20.5661496332586,15.737663262983,122.410119645755)) ;
#35218=CARTESIAN_POINT('Ctrl Pts',(-20.551706715397,15.937462015059,122.971635608473)) ;
#35219=CARTESIAN_POINT('Ctrl Pts',(-20.83731237547,15.7574729346492,122.861577302678)) ;
#35220=CARTESIAN_POINT('Ctrl Pts',(-20.6333723481961,15.9574552317502,123.388667733852)) ;
#35221=CARTESIAN_POINT('Ctrl Pts',(-20.9393997365277,15.7774661513403,123.38286609659)) ;
#35222=CARTESIAN_POINT('Ctrl Pts',(-20.5685874573327,15.9773061439465,123.805925874308)) ;
#35223=CARTESIAN_POINT('Ctrl Pts',(-20.858421608188,15.7973170635367,123.904440437754)) ;
#35224=CARTESIAN_POINT('Ctrl Pts',(-20.3629339575336,15.9973807502655,124.179831486359)) ;
#35225=CARTESIAN_POINT('Ctrl Pts',(-20.6013666269511,15.8173916698557,124.371819409612)) ;
#35226=CARTESIAN_POINT('Ctrl Pts',(-20.0986057487275,16.0138973821489,124.411216269807)) ;
#35227=CARTESIAN_POINT('Ctrl Pts',(-20.2709357009448,15.833908301739,124.661071335377)) ;
#35228=CARTESIAN_POINT('Ctrl Pts',(-19.8472305510429,16.027236089843,124.535405517903)) ;
#35229=CARTESIAN_POINT('Ctrl Pts',(-19.9567400193942,15.8472470094331,124.816295037055)) ;
#35230=CARTESIAN_POINT('Ctrl Pts',(-19.648689899929,16.0370784641513,124.593781061793)) ;
#35231=CARTESIAN_POINT('Ctrl Pts',(-19.7085577801925,15.8570893837414,124.889269258824)) ;
#35232=CARTESIAN_POINT('Ctrl Pts',(-19.4386553018546,16.047133484134,124.61748484339)) ;
#35233=CARTESIAN_POINT('Ctrl Pts',(-19.4460289923746,15.8671444037242,124.918903925126)) ;
#35234=CARTESIAN_POINT('Ctrl Pts',(-19.1610280376061,16.0603656407916,124.600218445625)) ;
#35235=CARTESIAN_POINT('Ctrl Pts',(-19.0989283678052,15.8803765603817,124.897309206235)) ;
#35236=CARTESIAN_POINT('Ctrl Pts',(-18.825889100884,16.0769806081367,124.488333617129)) ;
#35237=CARTESIAN_POINT('Ctrl Pts',(-18.680086550185,15.8969915277269,124.757481852965)) ;
#35238=CARTESIAN_POINT('Ctrl Pts',(-18.5495711916303,16.0935751951479,124.269005818189)) ;
#35239=CARTESIAN_POINT('Ctrl Pts',(-18.3346327391999,15.9135861147381,124.483293406466)) ;
#35240=CARTESIAN_POINT('Ctrl Pts',(-18.383354158807,16.1068087635033,124.045842736508)) ;
#35241=CARTESIAN_POINT('Ctrl Pts',(-18.1268897361385,15.9268196830935,124.204366870093)) ;
#35242=CARTESIAN_POINT('Ctrl Pts',(-18.2885245171761,16.1168523813119,123.857213437139)) ;
#35243=CARTESIAN_POINT('Ctrl Pts',(-18.0083439444266,15.9368633009021,123.968576154178)) ;
#35244=CARTESIAN_POINT('Ctrl Pts',(-18.2287506235429,16.1267393055468,123.658118953478)) ;
#35245=CARTESIAN_POINT('Ctrl Pts',(-17.9336253681046,15.946750225137,123.719711066809)) ;
#35246=CARTESIAN_POINT('Ctrl Pts',(-18.2038316638123,16.1367299599936,123.449583936804)) ;
#35247=CARTESIAN_POINT('Ctrl Pts',(-17.9024744065146,15.9567408795837,123.459039355826)) ;
#35248=CARTESIAN_POINT('Ctrl Pts',(-18.2155127325471,16.1466917184475,123.240472594879)) ;
#35249=CARTESIAN_POINT('Ctrl Pts',(-17.9170694040816,15.9667026380377,123.197660756738)) ;
#35250=CARTESIAN_POINT('Ctrl Pts',(-18.2792368886857,16.1600315835148,122.967353209043)) ;
#35251=CARTESIAN_POINT('Ctrl Pts',(-17.9967391762759,15.9800425031049,122.856207482252)) ;
#35252=CARTESIAN_POINT('Ctrl Pts',(-18.41302923077,16.1733403664281,122.718017566954)) ;
#35253=CARTESIAN_POINT('Ctrl Pts',(-18.1639736695268,15.9933512860182,122.544568270946)) ;
#35254=CARTESIAN_POINT('Ctrl Pts',(-18.6026009651151,16.1865361238721,122.515452306746)) ;
#35255=CARTESIAN_POINT('Ctrl Pts',(-18.4009205226465,16.0065470434623,122.291373957954)) ;
#35256=CARTESIAN_POINT('Ctrl Pts',(-18.7697316480871,16.1964980075486,122.389244608376)) ;
#35257=CARTESIAN_POINT('Ctrl Pts',(-18.6098352781677,16.0165089271388,122.133609050734)) ;
#35258=CARTESIAN_POINT('Ctrl Pts',(-18.9579132109796,16.2065411170633,122.293505577334)) ;
#35259=CARTESIAN_POINT('Ctrl Pts',(-18.8450601919875,16.0265520366534,122.013933523756)) ;
#35260=CARTESIAN_POINT('Ctrl Pts',(-19.1559583596013,16.2163933670625,122.232828073835)) ;
#35261=CARTESIAN_POINT('Ctrl Pts',(-19.092616128857,16.0364042866527,121.938083702869)) ;
#35262=CARTESIAN_POINT('Ctrl Pts',(-19.3639266023041,16.226364904013,122.20664426832)) ;
#35263=CARTESIAN_POINT('Ctrl Pts',(-19.3525761374323,16.0463758236031,121.905351203631)) ;
#35264=CARTESIAN_POINT('Ctrl Pts',(-19.5738352772956,16.2363601694905,122.217013254614)) ;
#35265=CARTESIAN_POINT('Ctrl Pts',(-19.6149622143299,16.0563710890807,121.918309627784)) ;
#35266=CARTESIAN_POINT('Ctrl Pts',(-19.7794415898056,16.2463941423641,122.264093918599)) ;
#35267=CARTESIAN_POINT('Ctrl Pts',(-19.8719707676454,16.0664050619543,121.977157725159)) ;
#35268=CARTESIAN_POINT('Ctrl Pts',(-19.9704548769762,16.2562495571265,122.344410165683)) ;
#35269=CARTESIAN_POINT('Ctrl Pts',(-20.1107386746549,16.0762604767166,122.077550542913)) ;
#35270=CARTESIAN_POINT('Ctrl Pts',(-20.1472714092236,16.2662488346353,122.458039635008)) ;
#35271=CARTESIAN_POINT('Ctrl Pts',(-20.3317609231756,16.0862597542255,122.219585083256)) ;
#35272=CARTESIAN_POINT('Ctrl Pts',(-20.3002692337498,16.2761440187983,122.599043469478)) ;
#35273=CARTESIAN_POINT('Ctrl Pts',(-20.5230102658659,16.0961549383885,122.395838020229)) ;
#35274=CARTESIAN_POINT('Ctrl Pts',(-20.4285086882037,16.2862043984391,122.767195696691)) ;
#35275=CARTESIAN_POINT('Ctrl Pts',(-20.6833117694854,16.1062153180293,122.606026601001)) ;
#35276=CARTESIAN_POINT('Ctrl Pts',(-20.5237070485476,16.2960542674472,122.951113827602)) ;
#35277=CARTESIAN_POINT('Ctrl Pts',(-20.8023123453879,16.1160651870374,122.835923343439)) ;
#35278=CARTESIAN_POINT('Ctrl Pts',(-20.5871150710927,16.3060858286551,123.152237015231)) ;
#35279=CARTESIAN_POINT('Ctrl Pts',(-20.8815749659165,16.1260967482452,123.087326542216)) ;
#35280=CARTESIAN_POINT('Ctrl Pts',(-20.6141638262457,16.3160962775374,123.360962196681)) ;
#35281=CARTESIAN_POINT('Ctrl Pts',(-20.9153886456371,16.1361071971276,123.348232716797)) ;
#35282=CARTESIAN_POINT('Ctrl Pts',(-20.6048907446535,16.3260030169544,123.569019571295)) ;
#35283=CARTESIAN_POINT('Ctrl Pts',(-20.9038000062821,16.1460139365446,123.608304860469)) ;
#35284=CARTESIAN_POINT('Ctrl Pts',(-20.5598881669259,16.3359410330228,123.773031366739)) ;
#35285=CARTESIAN_POINT('Ctrl Pts',(-20.8475493443514,16.155951952613,123.863320444471)) ;
#35286=CARTESIAN_POINT('Ctrl Pts',(-20.4797215293116,16.3459462794739,123.967521538131)) ;
#35287=CARTESIAN_POINT('Ctrl Pts',(-20.7473434746321,16.1659571990641,124.106434248702)) ;
#35288=CARTESIAN_POINT('Ctrl Pts',(-20.3663921716625,16.3559803405302,124.145428527425)) ;
#35289=CARTESIAN_POINT('Ctrl Pts',(-20.6056840714309,16.1759912601204,124.328819428223)) ;
#35290=CARTESIAN_POINT('Ctrl Pts',(-20.2268261020098,16.3658254215884,124.29828451982)) ;
#35291=CARTESIAN_POINT('Ctrl Pts',(-20.4312280688976,16.1858363411786,124.519891626443)) ;
#35292=CARTESIAN_POINT('Ctrl Pts',(-20.0607710857715,16.3758112275419,124.42667346357)) ;
#35293=CARTESIAN_POINT('Ctrl Pts',(-20.2236607635386,16.1958221471321,124.680379963882)) ;
#35294=CARTESIAN_POINT('Ctrl Pts',(-19.8759009892187,16.3857460480961,124.523947203319)) ;
#35295=CARTESIAN_POINT('Ctrl Pts',(-19.992574051782,16.2057569676862,124.801974564884)) ;
#35296=CARTESIAN_POINT('Ctrl Pts',(-19.6745001645774,16.3958035732283,124.588229437951)) ;
#35297=CARTESIAN_POINT('Ctrl Pts',(-19.740823924335,16.2158144928185,124.882329808667)) ;
#35298=CARTESIAN_POINT('Ctrl Pts',(-19.4699018787836,16.4056252238796,124.616221674398)) ;
#35299=CARTESIAN_POINT('Ctrl Pts',(-19.4850756391592,16.2256361434698,124.917322735198)) ;
#35300=CARTESIAN_POINT('Ctrl Pts',(-19.2586509012011,16.4156812873844,124.608469860798)) ;
#35301=CARTESIAN_POINT('Ctrl Pts',(-19.221011935614,16.2356922069746,124.907635447908)) ;
#35302=CARTESIAN_POINT('Ctrl Pts',(-19.0543812444969,16.4256219544483,124.56429049855)) ;
#35303=CARTESIAN_POINT('Ctrl Pts',(-18.9656740001609,16.2456328740385,124.852413667888)) ;
#35304=CARTESIAN_POINT('Ctrl Pts',(-18.861349537296,16.4355263481143,124.486210004502)) ;
#35305=CARTESIAN_POINT('Ctrl Pts',(-18.7243829673622,16.2555372677045,124.754815092922)) ;
#35306=CARTESIAN_POINT('Ctrl Pts',(-18.6823656137702,16.4455728718773,124.374110855955)) ;
#35307=CARTESIAN_POINT('Ctrl Pts',(-18.5006518514753,16.2655837914675,124.614693286705)) ;
#35308=CARTESIAN_POINT('Ctrl Pts',(-18.5277366886048,16.4554689548937,124.234866899934)) ;
#35309=CARTESIAN_POINT('Ctrl Pts',(-18.3073636532671,16.2754798744839,124.44063973377)) ;
#35310=CARTESIAN_POINT('Ctrl Pts',(-18.397512504775,16.4655356541237,124.068090149014)) ;
#35311=CARTESIAN_POINT('Ctrl Pts',(-18.1445816441947,16.2855465737139,124.232170442809)) ;
#35312=CARTESIAN_POINT('Ctrl Pts',(-18.3003784994557,16.4753592645248,123.885799724295)) ;
#35313=CARTESIAN_POINT('Ctrl Pts',(-18.0231616074264,16.2953701841149,124.004307682012)) ;
#35314=CARTESIAN_POINT('Ctrl Pts',(-18.2345231615704,16.4854151247023,123.684941160413)) ;
#35315=CARTESIAN_POINT('Ctrl Pts',(-17.9408403239872,16.3054260442924,123.753235338672)) ;
#35316=CARTESIAN_POINT('Ctrl Pts',(-18.2051689662618,16.4953482710072,123.478162940321)) ;
#35317=CARTESIAN_POINT('Ctrl Pts',(-17.9041452012384,16.3153591905974,123.494762458896)) ;
#35318=CARTESIAN_POINT('Ctrl Pts',(-18.2117436428783,16.5052935267778,123.269210161589)) ;
#35319=CARTESIAN_POINT('Ctrl Pts',(-17.9123613232578,16.325304446368,123.233570994395)) ;
#35320=CARTESIAN_POINT('Ctrl Pts',(-18.2545082390918,16.5152768252163,123.063705916951)) ;
#35321=CARTESIAN_POINT('Ctrl Pts',(-17.9658149649303,16.3352877448065,122.976690048521)) ;
#35322=CARTESIAN_POINT('Ctrl Pts',(-18.3329769113409,16.5253140053629,122.867842390834)) ;
#35323=CARTESIAN_POINT('Ctrl Pts',(-18.0638986665553,16.3453249249531,122.731859880821)) ;
#35324=CARTESIAN_POINT('Ctrl Pts',(-18.4419820599427,16.5351685580724,122.691641388023)) ;
#35325=CARTESIAN_POINT('Ctrl Pts',(-18.2001537296948,16.3551794776626,122.511606700081)) ;
#35326=CARTESIAN_POINT('Ctrl Pts',(-18.581699061968,16.5451680765197,122.534616193338)) ;
#35327=CARTESIAN_POINT('Ctrl Pts',(-18.3747984970513,16.3651789961099,122.315323705835)) ;
#35328=CARTESIAN_POINT('Ctrl Pts',(-18.7447549291817,16.5550631589818,122.405380089369)) ;
#35329=CARTESIAN_POINT('Ctrl Pts',(-18.578617637937,16.3750740785719,122.153776522229)) ;
#35330=CARTESIAN_POINT('Ctrl Pts',(-18.9307890892371,16.5651237044879,122.304812169695)) ;
#35331=CARTESIAN_POINT('Ctrl Pts',(-18.8111591522384,16.3851346240781,122.028064932937)) ;
#35332=CARTESIAN_POINT('Ctrl Pts',(-19.1272493004739,16.5749730117359,122.239351514005)) ;
#35333=CARTESIAN_POINT('Ctrl Pts',(-19.0567347651513,16.3949839313261,121.946236873257)) ;
#35334=CARTESIAN_POINT('Ctrl Pts',(-19.3356895472675,16.5850001018232,122.207921910754)) ;
#35335=CARTESIAN_POINT('Ctrl Pts',(-19.317284759462,16.4050110214134,121.906948036718)) ;
#35336=CARTESIAN_POINT('Ctrl Pts',(-19.5464580747962,16.5950290059602,122.213723078869)) ;
#35337=CARTESIAN_POINT('Ctrl Pts',(-19.5807454043867,16.4150399255504,121.914197470352)) ;
#35338=CARTESIAN_POINT('Ctrl Pts',(-19.7492714933066,16.6048728710595,122.254846303391)) ;
#35339=CARTESIAN_POINT('Ctrl Pts',(-19.8342636546969,16.4248837906497,121.965599859019)) ;
#35340=CARTESIAN_POINT('Ctrl Pts',(-19.9450340387056,16.6148686977679,122.331249053741)) ;
#35341=CARTESIAN_POINT('Ctrl Pts',(-20.0789676317577,16.4348796173581,122.06110173883)) ;
#35342=CARTESIAN_POINT('Ctrl Pts',(-20.1248865780728,16.6248939144169,122.441136839792)) ;
#35343=CARTESIAN_POINT('Ctrl Pts',(-20.3037842342036,16.4449048340071,122.198459857555)) ;
#35344=CARTESIAN_POINT('Ctrl Pts',(-20.28097718897,16.6347837465745,122.57849001676)) ;
#35345=CARTESIAN_POINT('Ctrl Pts',(-20.4988993121672,16.4547946661646,122.370150559319)) ;
#35346=CARTESIAN_POINT('Ctrl Pts',(-20.4123923595961,16.6447746026592,122.742330187419)) ;
#35347=CARTESIAN_POINT('Ctrl Pts',(-20.663169704395,16.4647855222494,122.574949866222)) ;
#35348=CARTESIAN_POINT('Ctrl Pts',(-20.5128694027826,16.6547196972521,122.925680754585)) ;
#35349=CARTESIAN_POINT('Ctrl Pts',(-20.7887677401165,16.4747306168422,122.804137700904)) ;
#35350=CARTESIAN_POINT('Ctrl Pts',(-20.5804045472884,16.6646716010202,123.12370981409)) ;
#35351=CARTESIAN_POINT('Ctrl Pts',(-20.8731883104947,16.4846825206104,123.05167397304)) ;
#35352=CARTESIAN_POINT('Ctrl Pts',(-20.6126176827345,16.6747080004896,123.332227708226)) ;
#35353=CARTESIAN_POINT('Ctrl Pts',(-20.9134563189701,16.4947189200798,123.312320962723)) ;
#35354=CARTESIAN_POINT('Ctrl Pts',(-20.6083540179915,16.6845970705783,123.540090086078)) ;
#35355=CARTESIAN_POINT('Ctrl Pts',(-20.9081282977021,16.5046079901685,123.572149884736)) ;
#35356=CARTESIAN_POINT('Ctrl Pts',(-20.5680279223368,16.6945863599492,123.746183169029)) ;
#35357=CARTESIAN_POINT('Ctrl Pts',(-20.8577220599026,16.5145972795394,123.829766727651)) ;
#35358=CARTESIAN_POINT('Ctrl Pts',(-20.4926169706463,16.7045449261589,123.941483709514)) ;
#35359=CARTESIAN_POINT('Ctrl Pts',(-20.7634596189807,16.5245558457491,124.073893349029)) ;
#35360=CARTESIAN_POINT('Ctrl Pts',(-20.3855116246943,16.7144444973757,124.119942910735)) ;
#35361=CARTESIAN_POINT('Ctrl Pts',(-20.6295786199548,16.5344554169658,124.29696878482)) ;
#35362=CARTESIAN_POINT('Ctrl Pts',(-20.2469681262543,16.7244924117899,124.279374314369)) ;
#35363=CARTESIAN_POINT('Ctrl Pts',(-20.4564004098942,16.5445033313801,124.496258761837)) ;
#35364=CARTESIAN_POINT('Ctrl Pts',(-20.0853998211911,16.7343877546505,124.410470530884)) ;
#35365=CARTESIAN_POINT('Ctrl Pts',(-20.2544401348051,16.5543986742407,124.660130610511)) ;
#35366=CARTESIAN_POINT('Ctrl Pts',(-19.9005296097113,16.7444494485979,124.513218405503)) ;
#35367=CARTESIAN_POINT('Ctrl Pts',(-20.0233532789504,16.5644603681881,124.78856641835)) ;
#35368=CARTESIAN_POINT('Ctrl Pts',(-19.7049244472247,16.7542939016821,124.580859195891)) ;
#35369=CARTESIAN_POINT('Ctrl Pts',(-19.7788459931225,16.5743048212723,124.873119039316)) ;
#35370=CARTESIAN_POINT('Ctrl Pts',(-19.4982683090675,16.7642545866405,124.614617061562)) ;
#35371=CARTESIAN_POINT('Ctrl Pts',(-19.520525537516,16.5842655062307,124.915317434052)) ;
#35372=CARTESIAN_POINT('Ctrl Pts',(-19.2872959543148,16.7742905191491,124.611604709264)) ;
#35373=CARTESIAN_POINT('Ctrl Pts',(-19.256810212926,16.5943014387393,124.911553126571)) ;
#35374=CARTESIAN_POINT('Ctrl Pts',(-19.083065641411,16.7841791348371,124.572793885594)) ;
#35375=CARTESIAN_POINT('Ctrl Pts',(-19.0015211293755,16.6041900544273,124.863040443371)) ;
#35376=CARTESIAN_POINT('Ctrl Pts',(-18.8860375470221,16.7941935439796,124.498559615146)) ;
#35377=CARTESIAN_POINT('Ctrl Pts',(-18.755235682163,16.6142044635698,124.770248444089)) ;
#35378=CARTESIAN_POINT('Ctrl Pts',(-18.7048442029777,16.8042273529374,124.390576815252)) ;
#35379=CARTESIAN_POINT('Ctrl Pts',(-18.5287435554277,16.6242382725276,124.635270964775)) ;
#35380=CARTESIAN_POINT('Ctrl Pts',(-18.5479851568458,16.8140578071936,124.255979370359)) ;
#35381=CARTESIAN_POINT('Ctrl Pts',(-18.3326680458869,16.6340687267837,124.467023867627)) ;
#35382=CARTESIAN_POINT('Ctrl Pts',(-18.4135706987232,16.8241354747718,124.092266151809)) ;
#35383=CARTESIAN_POINT('Ctrl Pts',(-18.1646495930641,16.644146394362,124.262383242849)) ;
#35384=CARTESIAN_POINT('Ctrl Pts',(-18.3118178527469,16.833987342894,123.911815748702)) ;
#35385=CARTESIAN_POINT('Ctrl Pts',(-18.0374571776765,16.6539982624842,124.036819495962)) ;
#35386=CARTESIAN_POINT('Ctrl Pts',(-18.2412580423385,16.8440603804594,123.712187854895)) ;
#35387=CARTESIAN_POINT('Ctrl Pts',(-17.9492568482379,16.6640713000495,123.787285292021)) ;
#35388=CARTESIAN_POINT('Ctrl Pts',(-18.2072505630093,16.8539029338102,123.508062557237)) ;
#35389=CARTESIAN_POINT('Ctrl Pts',(-17.9067465101857,16.6739138534004,123.532127399556)) ;
#35390=CARTESIAN_POINT('Ctrl Pts',(-18.2085239591176,16.8638833293037,123.298256187537)) ;
#35391=CARTESIAN_POINT('Ctrl Pts',(-17.9083377642427,16.6838942488938,123.269869124287)) ;
#35392=CARTESIAN_POINT('Ctrl Pts',(-18.2467556082462,16.8739018072815,123.091139951509)) ;
#35393=CARTESIAN_POINT('Ctrl Pts',(-17.9561266808108,16.6939127268717,123.01097372099)) ;
#35394=CARTESIAN_POINT('Ctrl Pts',(-18.3189697446899,16.8837851215876,122.896288022926)) ;
#35395=CARTESIAN_POINT('Ctrl Pts',(-18.0463942839959,16.7037960411777,122.767407615418)) ;
#35396=CARTESIAN_POINT('Ctrl Pts',(-18.425934681268,16.8938534241263,122.713676624745)) ;
#35397=CARTESIAN_POINT('Ctrl Pts',(-18.180099801531,16.7138643437165,122.539143460638)) ;
#35398=CARTESIAN_POINT('Ctrl Pts',(-18.5595970562926,16.9036834713997,122.556016451482)) ;
#35399=CARTESIAN_POINT('Ctrl Pts',(-18.3471784468663,16.7236943909899,122.342066798558)) ;
#35400=CARTESIAN_POINT('Ctrl Pts',(-18.722208363347,16.9137503428152,122.42061719112)) ;
#35401=CARTESIAN_POINT('Ctrl Pts',(-18.5504420735464,16.7337612624054,122.172817736583)) ;
#35402=CARTESIAN_POINT('Ctrl Pts',(-18.9027264908965,16.9236393816143,122.317430530049)) ;
#35403=CARTESIAN_POINT('Ctrl Pts',(-18.7760904676287,16.7436503012044,122.043833574467)) ;
#35404=CARTESIAN_POINT('Ctrl Pts',(-19.1003612730022,16.9336360797484,122.246020456028)) ;
#35405=CARTESIAN_POINT('Ctrl Pts',(-19.0231340622893,16.7536469993385,121.954570731794)) ;
#35406=CARTESIAN_POINT('Ctrl Pts',(-19.3065267658046,16.9435885054603,122.210251377386)) ;
#35407=CARTESIAN_POINT('Ctrl Pts',(-19.280841415143,16.7635994250505,121.909859064131)) ;
#35408=CARTESIAN_POINT('Ctrl Pts',(-19.5155081682475,16.9535298076933,122.210531944557)) ;
#35409=CARTESIAN_POINT('Ctrl Pts',(-19.5420687998033,16.7735407272835,121.910209653744)) ;
#35410=CARTESIAN_POINT('Ctrl Pts',(-19.7222133629213,16.9635130467772,122.24703377313)) ;
#35411=CARTESIAN_POINT('Ctrl Pts',(-19.8004505578653,16.7835239663674,121.955836958288)) ;
#35412=CARTESIAN_POINT('Ctrl Pts',(-19.9203861587656,16.9735518483458,122.319565863544)) ;
#35413=CARTESIAN_POINT('Ctrl Pts',(-20.0481664431419,16.793562767936,122.046501857169)) ;
#35414=CARTESIAN_POINT('Ctrl Pts',(-20.0997203161893,16.9833999544674,122.423063092642)) ;
#35415=CARTESIAN_POINT('Ctrl Pts',(-20.272335374715,16.8034108740576,122.175874105988)) ;
#35416=CARTESIAN_POINT('Ctrl Pts',(-20.2618757976447,16.9934601500428,122.558817396899)) ;
#35417=CARTESIAN_POINT('Ctrl Pts',(-20.4750293999112,16.813471069633,122.34556681789)) ;
#35418=CARTESIAN_POINT('Ctrl Pts',(-20.3956688355369,17.0033578333542,122.718192247894)) ;
#35419=CARTESIAN_POINT('Ctrl Pts',(-20.6422713391214,16.8233687529444,122.544786148039)) ;
#35420=CARTESIAN_POINT('Ctrl Pts',(-20.5006942150535,17.0132888737282,122.898630233536)) ;
#35421=CARTESIAN_POINT('Ctrl Pts',(-20.7735531877414,16.8332997933184,122.770334392625)) ;
#35422=CARTESIAN_POINT('Ctrl Pts',(-20.5733879414346,17.0233310913848,123.096836226167)) ;
#35423=CARTESIAN_POINT('Ctrl Pts',(-20.8644201008699,16.843342010975,123.018091751104)) ;
#35424=CARTESIAN_POINT('Ctrl Pts',(-20.61013604455,17.0332177521188,123.301420117355)) ;
#35425=CARTESIAN_POINT('Ctrl Pts',(-20.9103551820702,16.853228671709,123.273822727996)) ;
#35426=CARTESIAN_POINT('Ctrl Pts',(-20.6111628873651,17.0432108607212,123.511493426387)) ;
#35427=CARTESIAN_POINT('Ctrl Pts',(-20.9116383536985,16.8632217803114,123.536414570105)) ;
#35428=CARTESIAN_POINT('Ctrl Pts',(-20.5757869989794,17.0531565593595,123.717568908306)) ;
#35429=CARTESIAN_POINT('Ctrl Pts',(-20.8674180472619,16.8731674789497,123.794009449911)) ;
#35430=CARTESIAN_POINT('Ctrl Pts',(-20.5055557491606,17.0631037816305,123.91455588214)) ;
#35431=CARTESIAN_POINT('Ctrl Pts',(-20.7796283028681,16.8831147012207,124.040243534273)) ;
#35432=CARTESIAN_POINT('Ctrl Pts',(-20.400941475518,17.0731518072107,124.098065903988)) ;
#35433=CARTESIAN_POINT('Ctrl Pts',(-20.6488602157031,16.8931627268008,124.269630633143)) ;
#35434=CARTESIAN_POINT('Ctrl Pts',(-20.2688802244909,17.0829990543536,124.257492396339)) ;
#35435=CARTESIAN_POINT('Ctrl Pts',(-20.4837823786793,16.9030099739437,124.46891451259)) ;
#35436=CARTESIAN_POINT('Ctrl Pts',(-20.1097187274717,17.0929622314443,124.39364708618)) ;
#35437=CARTESIAN_POINT('Ctrl Pts',(-20.2848296698449,16.9129731510345,124.639107596635)) ;
#35438=CARTESIAN_POINT('Ctrl Pts',(-19.9279652479733,17.1029919524777,124.500535991782)) ;
#35439=CARTESIAN_POINT('Ctrl Pts',(-20.0576375878004,16.9230028720679,124.772718134016)) ;
#35440=CARTESIAN_POINT('Ctrl Pts',(-19.7329501884367,17.1128964200106,124.573568512816)) ;
#35441=CARTESIAN_POINT('Ctrl Pts',(-19.8138676647044,16.9329073396008,124.864008421911)) ;
#35442=CARTESIAN_POINT('Ctrl Pts',(-19.5257911753333,17.1229209058404,124.612154491612)) ;
#35443=CARTESIAN_POINT('Ctrl Pts',(-19.5549188176483,16.9429318254305,124.912240141171)) ;
#35444=CARTESIAN_POINT('Ctrl Pts',(-19.31756391383,17.1328247409643,124.61433347866)) ;
#35445=CARTESIAN_POINT('Ctrl Pts',(-19.2946338276939,16.9528356605544,124.914963066567)) ;
#35446=CARTESIAN_POINT('Ctrl Pts',(-19.1091090081414,17.1428759316743,124.579872920246)) ;
#35447=CARTESIAN_POINT('Ctrl Pts',(-19.0340655772847,16.9628868512645,124.871886584531)) ;
#35448=CARTESIAN_POINT('Ctrl Pts',(-18.9130563367156,17.1527603743326,124.510927123554)) ;
#35449=CARTESIAN_POINT('Ctrl Pts',(-18.7889990252693,16.9727712939228,124.785703184487)) ;
#35450=CARTESIAN_POINT('Ctrl Pts',(-18.7298067492815,17.1627533821844,124.408227429551)) ;
#35451=CARTESIAN_POINT('Ctrl Pts',(-18.5599373548678,16.9827643017746,124.657327597642)) ;
#35452=CARTESIAN_POINT('Ctrl Pts',(-18.5679203831117,17.1727017019007,124.275788607794)) ;
#35453=CARTESIAN_POINT('Ctrl Pts',(-18.3575795914543,16.9927126214909,124.491777975057)) ;
#35454=CARTESIAN_POINT('Ctrl Pts',(-18.4314404984795,17.1826385406102,124.117654900574)) ;
#35455=CARTESIAN_POINT('Ctrl Pts',(-18.1869801387972,17.0026494602004,124.294109650158)) ;
#35456=CARTESIAN_POINT('Ctrl Pts',(-18.3237434951537,17.1926215295298,123.937489058372)) ;
#35457=CARTESIAN_POINT('Ctrl Pts',(-18.0523597653878,17.0126324491199,124.068901521774)) ;
#35458=CARTESIAN_POINT('Ctrl Pts',(-18.2488910018654,17.2026654088939,123.740073906393)) ;
#35459=CARTESIAN_POINT('Ctrl Pts',(-17.9587951854012,17.022676328484,123.822132392041)) ;
#35460=CARTESIAN_POINT('Ctrl Pts',(-18.2098074279025,17.2124934742523,123.537154265796)) ;
#35461=CARTESIAN_POINT('Ctrl Pts',(-17.909941640764,17.0325043938425,123.568481191402)) ;
#35462=CARTESIAN_POINT('Ctrl Pts',(-18.2063795196312,17.2225705628072,123.325376725486)) ;
#35463=CARTESIAN_POINT('Ctrl Pts',(-17.9056580144005,17.0425814823974,123.303759681479)) ;
#35464=CARTESIAN_POINT('Ctrl Pts',(-18.2389039387934,17.2324207149635,123.120811528731)) ;
#35465=CARTESIAN_POINT('Ctrl Pts',(-17.94631501662,17.0524316345537,123.048052157432)) ;
#35466=CARTESIAN_POINT('Ctrl Pts',(-18.3079172661289,17.2425011954158,122.920496194751)) ;
#35467=CARTESIAN_POINT('Ctrl Pts',(-18.0325827863602,17.062512115006,122.797658849557)) ;
#35468=CARTESIAN_POINT('Ctrl Pts',(-18.4078418322244,17.2523156931847,122.739922505072)) ;
#35469=CARTESIAN_POINT('Ctrl Pts',(-18.1574904407199,17.0723266127749,122.571941098785)) ;
#35470=CARTESIAN_POINT('Ctrl Pts',(-18.5406376489348,17.2623839892048,122.575157598147)) ;
#35471=CARTESIAN_POINT('Ctrl Pts',(-18.3234861663254,17.082394908795,122.365986190106)) ;
#35472=CARTESIAN_POINT('Ctrl Pts',(-18.6974563857139,17.2722828216876,122.43827365892)) ;
#35473=CARTESIAN_POINT('Ctrl Pts',(-18.5195111942605,17.0922937412777,122.194881832849)) ;
#35474=CARTESIAN_POINT('Ctrl Pts',(-18.878314400253,17.2823357017021,122.329011502217)) ;
#35475=CARTESIAN_POINT('Ctrl Pts',(-18.7455842875556,17.1023466212923,122.058305557844)) ;
#35476=CARTESIAN_POINT('Ctrl Pts',(-19.0718160918219,17.2922055171983,122.253987097039)) ;
#35477=CARTESIAN_POINT('Ctrl Pts',(-18.9874629412771,17.1122164367885,121.964526142738)) ;
#35478=CARTESIAN_POINT('Ctrl Pts',(-19.2795008716947,17.3022781982811,122.212830255507)) ;
#35479=CARTESIAN_POINT('Ctrl Pts',(-19.2470688770151,17.1222891178713,121.913081725727)) ;
#35480=CARTESIAN_POINT('Ctrl Pts',(-19.4861827851385,17.312110676852,122.208383210554)) ;
#35481=CARTESIAN_POINT('Ctrl Pts',(-19.505422587491,17.1321215964422,121.907524514954)) ;
#35482=CARTESIAN_POINT('Ctrl Pts',(-19.6946785789896,17.3221413108381,122.23992020577)) ;
#35483=CARTESIAN_POINT('Ctrl Pts',(-19.7660419705,17.1421522304283,121.94694754642)) ;
#35484=CARTESIAN_POINT('Ctrl Pts',(-19.8943714717527,17.3321728680573,122.307777090262)) ;
#35485=CARTESIAN_POINT('Ctrl Pts',(-20.0156574865041,17.1521837876475,122.031770158995)) ;
#35486=CARTESIAN_POINT('Ctrl Pts',(-20.0757133418564,17.342002576929,122.406842625941)) ;
#35487=CARTESIAN_POINT('Ctrl Pts',(-20.24233509567,17.1620134965191,122.155604235023)) ;
#35488=CARTESIAN_POINT('Ctrl Pts',(-20.2401293619726,17.3519920257311,122.53751027012)) ;
#35489=CARTESIAN_POINT('Ctrl Pts',(-20.447854041674,17.1720029453212,122.318940433041)) ;
#35490=CARTESIAN_POINT('Ctrl Pts',(-20.3797110879383,17.3620358781311,122.695945873639)) ;
#35491=CARTESIAN_POINT('Ctrl Pts',(-20.6223297570002,17.1820467977213,122.51698601017)) ;
#35492=CARTESIAN_POINT('Ctrl Pts',(-20.4875963394876,17.3718575914632,122.872002282074)) ;
#35493=CARTESIAN_POINT('Ctrl Pts',(-20.7571853343679,17.1918685110533,122.737058592074)) ;
#35494=CARTESIAN_POINT('Ctrl Pts',(-20.565398754166,17.3818925964519,123.068098579527)) ;
#35495=CARTESIAN_POINT('Ctrl Pts',(-20.8544363835335,17.2019035160421,122.982179630629)) ;
#35496=CARTESIAN_POINT('Ctrl Pts',(-20.6073560537494,17.3919174348995,123.274640875661)) ;
#35497=CARTESIAN_POINT('Ctrl Pts',(-20.9068811374708,17.2119283544897,123.240357855684)) ;
#35498=CARTESIAN_POINT('Ctrl Pts',(-20.6131626095599,17.4017696478547,123.481683897343)) ;
#35499=CARTESIAN_POINT('Ctrl Pts',(-20.9141373279867,17.2217805674449,123.499162698655)) ;
#35500=CARTESIAN_POINT('Ctrl Pts',(-20.5828638631299,17.4117596040485,123.689490947812)) ;
#35501=CARTESIAN_POINT('Ctrl Pts',(-20.8762617533052,17.2317705236386,123.758921385057)) ;
#35502=CARTESIAN_POINT('Ctrl Pts',(-20.5173607069601,17.4216877143317,123.887673199299)) ;
#35503=CARTESIAN_POINT('Ctrl Pts',(-20.7943806136614,17.2416986339219,124.006649024924)) ;
#35504=CARTESIAN_POINT('Ctrl Pts',(-20.4181341555085,17.4316763144113,124.072748693797)) ;
#35505=CARTESIAN_POINT('Ctrl Pts',(-20.6703453852788,17.2516872340014,124.237992487167)) ;
#35506=CARTESIAN_POINT('Ctrl Pts',(-20.2875580116088,17.4417029063388,124.238230031649)) ;
#35507=CARTESIAN_POINT('Ctrl Pts',(-20.5071235398505,17.2617138259289,124.44484280022)) ;
#35508=CARTESIAN_POINT('Ctrl Pts',(-20.1326042864627,17.451588034403,124.376702910318)) ;
#35509=CARTESIAN_POINT('Ctrl Pts',(-20.3134293623921,17.2715989539931,124.617932747041)) ;
#35510=CARTESIAN_POINT('Ctrl Pts',(-19.9543077801982,17.4615791518765,124.487754355148)) ;
#35511=CARTESIAN_POINT('Ctrl Pts',(-20.090557366876,17.2815900714667,124.756745161421)) ;
#35512=CARTESIAN_POINT('Ctrl Pts',(-19.7583141539382,17.4716197677283,124.566132788164)) ;
#35513=CARTESIAN_POINT('Ctrl Pts',(-19.8455645964528,17.2916306873184,124.854716110679)) ;
#35514=CARTESIAN_POINT('Ctrl Pts',(-19.5560340189507,17.481452758582,124.608731196182)) ;
#35515=CARTESIAN_POINT('Ctrl Pts',(-19.5927130154579,17.3014636781722,124.90796206647)) ;
#35516=CARTESIAN_POINT('Ctrl Pts',(-19.3460857373288,17.4914458900323,124.61627350105)) ;
#35517=CARTESIAN_POINT('Ctrl Pts',(-19.3302774501978,17.3114568096224,124.917387511102)) ;
#35518=CARTESIAN_POINT('Ctrl Pts',(-19.1372544365684,17.5014779384677,124.586697623401)) ;
#35519=CARTESIAN_POINT('Ctrl Pts',(-19.0692386893075,17.3214888580579,124.880415353166)) ;
#35520=CARTESIAN_POINT('Ctrl Pts',(-18.9400052555549,17.5113431850101,124.522647715946)) ;
#35521=CARTESIAN_POINT('Ctrl Pts',(-18.8226772574824,17.3313541046003,124.800350459947)) ;
#35522=CARTESIAN_POINT('Ctrl Pts',(-18.7547863337693,17.5213050598369,124.424885268183)) ;
#35523=CARTESIAN_POINT('Ctrl Pts',(-18.5911545600196,17.3413159794271,124.678145049342)) ;
#35524=CARTESIAN_POINT('Ctrl Pts',(-18.5883681930039,17.5313400229482,124.295243637519)) ;
#35525=CARTESIAN_POINT('Ctrl Pts',(-18.3831334191365,17.3513509425383,124.516091097568)) ;
#35526=CARTESIAN_POINT('Ctrl Pts',(-18.4488134106994,17.5412248674106,124.141223324118)) ;
#35527=CARTESIAN_POINT('Ctrl Pts',(-18.2086914289876,17.3612357870008,124.323563591866)) ;
#35528=CARTESIAN_POINT('Ctrl Pts',(-18.3361743130609,17.5512909202513,123.962114608032)) ;
#35529=CARTESIAN_POINT('Ctrl Pts',(-18.0678947666069,17.3713018398415,124.099676485574)) ;
#35530=CARTESIAN_POINT('Ctrl Pts',(-18.2579149300862,17.5611284361603,123.770636276305)) ;
#35531=CARTESIAN_POINT('Ctrl Pts',(-17.9700726313158,17.3811393557505,123.860326944407)) ;
#35532=CARTESIAN_POINT('Ctrl Pts',(-18.2128572603931,17.5711971842692,123.563847910291)) ;
#35533=CARTESIAN_POINT('Ctrl Pts',(-17.9137531150226,17.3912081038593,123.601841075216)) ;
#35534=CARTESIAN_POINT('Ctrl Pts',(-18.2046218359309,17.5810777013002,123.356259866829)) ;
#35535=CARTESIAN_POINT('Ctrl Pts',(-17.9034613927267,17.4010886208904,123.342355402498)) ;
#35536=CARTESIAN_POINT('Ctrl Pts',(-18.2324382002903,17.5910688882346,123.148094680984)) ;
#35537=CARTESIAN_POINT('Ctrl Pts',(-17.938234492748,17.4110798078248,123.082149155365)) ;
#35538=CARTESIAN_POINT('Ctrl Pts',(-18.2957212303086,17.6010219545096,122.948615518676)) ;
#35539=CARTESIAN_POINT('Ctrl Pts',(-18.0173408798839,17.4210328740997,122.832800782662)) ;
#35540=CARTESIAN_POINT('Ctrl Pts',(-18.3935237813903,17.6110577920422,122.761687553403)) ;
#35541=CARTESIAN_POINT('Ctrl Pts',(-18.139596406472,17.4310687116323,122.599142062299)) ;
#35542=CARTESIAN_POINT('Ctrl Pts',(-18.5203340583895,17.6209479182536,122.596896263532)) ;
#35543=CARTESIAN_POINT('Ctrl Pts',(-18.2981116221093,17.4409588378438,122.393154239506)) ;
#35544=CARTESIAN_POINT('Ctrl Pts',(-18.6751694912199,17.6309401001616,122.454946682161)) ;
#35545=CARTESIAN_POINT('Ctrl Pts',(-18.4916578231094,17.4509510197518,122.21571919075)) ;
#35546=CARTESIAN_POINT('Ctrl Pts',(-18.8515274887847,17.6408860401002,122.342614062486)) ;
#35547=CARTESIAN_POINT('Ctrl Pts',(-18.7121069675816,17.4608969596903,122.07530556897)) ;
#35548=CARTESIAN_POINT('Ctrl Pts',(-19.0445828832562,17.6508332238642,122.262203190812)) ;
#35549=CARTESIAN_POINT('Ctrl Pts',(-18.953427454247,17.4708441434544,121.974794440386)) ;
#35550=CARTESIAN_POINT('Ctrl Pts',(-19.2507687647506,17.6608811621717,122.21630679009)) ;
#35551=CARTESIAN_POINT('Ctrl Pts',(-19.2111603866877,17.4808920817619,121.917426601143)) ;
#35552=CARTESIAN_POINT('Ctrl Pts',(-19.4575859789318,17.670728796912,122.206920104581)) ;
#35553=CARTESIAN_POINT('Ctrl Pts',(-19.4696824314126,17.4907397165021,121.905695967062)) ;
#35554=CARTESIAN_POINT('Ctrl Pts',(-19.6653420100825,17.6806905108858,122.233242738369)) ;
#35555=CARTESIAN_POINT('Ctrl Pts',(-19.7293772424128,17.500701430476,121.938602055707)) ;
#35556=CARTESIAN_POINT('Ctrl Pts',(-19.8666582474384,17.6907191456766,122.295917378937)) ;
#35557=CARTESIAN_POINT('Ctrl Pts',(-19.9810217546006,17.5107300652668,122.01694801998)) ;
#35558=CARTESIAN_POINT('Ctrl Pts',(-20.0518343532791,17.7006294642738,122.391384008924)) ;
#35559=CARTESIAN_POINT('Ctrl Pts',(-20.2124907996751,17.5206403838639,122.13628388166)) ;
#35560=CARTESIAN_POINT('Ctrl Pts',(-20.2183778744694,17.7105643205853,122.517438880118)) ;
#35561=CARTESIAN_POINT('Ctrl Pts',(-20.4206686080911,17.5305752401755,122.293854796861)) ;
#35562=CARTESIAN_POINT('Ctrl Pts',(-20.3618650760254,17.720605556546,122.672260820024)) ;
#35563=CARTESIAN_POINT('Ctrl Pts',(-20.6000255829358,17.5406164761362,122.487384162128)) ;
#35564=CARTESIAN_POINT('Ctrl Pts',(-20.4746913192289,17.730492328126,122.846848178747)) ;
#35565=CARTESIAN_POINT('Ctrl Pts',(-20.7410561134647,17.5505032477161,122.705620024143)) ;
#35566=CARTESIAN_POINT('Ctrl Pts',(-20.5566303036143,17.7404925068322,123.040424795211)) ;
#35567=CARTESIAN_POINT('Ctrl Pts',(-20.8434772707926,17.5605034264223,122.947591960543)) ;
#35568=CARTESIAN_POINT('Ctrl Pts',(-20.6035135712802,17.7504097850418,123.243613328282)) ;
#35569=CARTESIAN_POINT('Ctrl Pts',(-20.90207862794,17.5704207046319,123.20157834967)) ;
#35570=CARTESIAN_POINT('Ctrl Pts',(-20.6144792344301,17.7604570314554,123.454524019583)) ;
#35571=CARTESIAN_POINT('Ctrl Pts',(-20.9157828895286,17.5804679510456,123.465216930617)) ;
#35572=CARTESIAN_POINT('Ctrl Pts',(-20.5893156501157,17.7703309204367,123.660606188454)) ;
#35573=CARTESIAN_POINT('Ctrl Pts',(-20.8843256016214,17.5903418400269,123.722819362007)) ;
#35574=CARTESIAN_POINT('Ctrl Pts',(-20.5277259008089,17.7803929380173,123.862949653921)) ;
#35575=CARTESIAN_POINT('Ctrl Pts',(-20.8073356879099,17.6004038576075,123.975747950664)) ;
#35576=CARTESIAN_POINT('Ctrl Pts',(-20.4337117630159,17.7902639997516,124.047969554099)) ;
#35577=CARTESIAN_POINT('Ctrl Pts',(-20.6898154916365,17.6102749193418,124.207021563606)) ;
#35578=CARTESIAN_POINT('Ctrl Pts',(-20.3079243206762,17.8002580631119,124.216261726582)) ;
#35579=CARTESIAN_POINT('Ctrl Pts',(-20.5325789116927,17.620268982702,124.417385134035)) ;
#35580=CARTESIAN_POINT('Ctrl Pts',(-20.1539268427788,17.8102902211453,124.360359874933)) ;
#35581=CARTESIAN_POINT('Ctrl Pts',(-20.3400800617219,17.6303011407355,124.597505830215)) ;
#35582=CARTESIAN_POINT('Ctrl Pts',(-19.9804372227752,17.8201540973854,124.473993821074)) ;
#35583=CARTESIAN_POINT('Ctrl Pts',(-20.1232165513051,17.6401650169756,124.739545873225)) ;
#35584=CARTESIAN_POINT('Ctrl Pts',(-19.7859124945591,17.8302246120237,124.557495151561)) ;
#35585=CARTESIAN_POINT('Ctrl Pts',(-19.8800594521313,17.6502355316139,124.843920027553)) ;
#35586=CARTESIAN_POINT('Ctrl Pts',(-19.5845131324371,17.8400652489647,124.604874841152)) ;
#35587=CARTESIAN_POINT('Ctrl Pts',(-19.6283095577408,17.6600761685548,124.903141838368)) ;
#35588=CARTESIAN_POINT('Ctrl Pts',(-19.3753651784529,17.8500323778049,124.617404469325)) ;
#35589=CARTESIAN_POINT('Ctrl Pts',(-19.3668752747088,17.670043297395,124.918801259621)) ;
#35590=CARTESIAN_POINT('Ctrl Pts',(-19.1662372548247,17.8600463509294,124.593093186389)) ;
#35591=CARTESIAN_POINT('Ctrl Pts',(-19.1054626464857,17.6800572705196,124.888408905299)) ;
#35592=CARTESIAN_POINT('Ctrl Pts',(-18.8985829814894,17.8733310847927,124.513236748648)) ;
#35593=CARTESIAN_POINT('Ctrl Pts',(-18.7709105569149,17.6933420043829,124.788587304153)) ;
#35594=CARTESIAN_POINT('Ctrl Pts',(-18.6588816082281,17.8865563495074,124.366233166193)) ;
#35595=CARTESIAN_POINT('Ctrl Pts',(-18.471311575917,17.7065672690976,124.604860086417)) ;
#35596=CARTESIAN_POINT('Ctrl Pts',(-18.4660643936239,17.8998668720623,124.16345986531)) ;
#35597=CARTESIAN_POINT('Ctrl Pts',(-18.2302475347785,17.7198777916525,124.351352544066)) ;
#35598=CARTESIAN_POINT('Ctrl Pts',(-18.3496539207817,17.9098955169645,123.987675168725)) ;
#35599=CARTESIAN_POINT('Ctrl Pts',(-18.0847456432416,17.7299064365547,124.131627885485)) ;
#35600=CARTESIAN_POINT('Ctrl Pts',(-18.2666046768902,17.9197765493184,123.797265561307)) ;
#35601=CARTESIAN_POINT('Ctrl Pts',(-17.9809344251841,17.7397874689086,123.893612632068)) ;
#35602=CARTESIAN_POINT('Ctrl Pts',(-18.2169614950972,17.9297575219985,123.593391497918)) ;
#35603=CARTESIAN_POINT('Ctrl Pts',(-17.918882981317,17.7497684415886,123.638771587208)) ;
#35604=CARTESIAN_POINT('Ctrl Pts',(-18.203650414156,17.9397386495845,123.383995886292)) ;
#35605=CARTESIAN_POINT('Ctrl Pts',(-17.9022490540059,17.7597495691746,123.3770209592)) ;
#35606=CARTESIAN_POINT('Ctrl Pts',(-18.2339270986067,17.9529818398459,123.107154473442)) ;
#35607=CARTESIAN_POINT('Ctrl Pts',(-17.9400860620383,17.7729927594361,123.030998917168)) ;
#35608=CARTESIAN_POINT('Ctrl Pts',(-18.3623848961341,17.9696498352067,122.77698011445)) ;
#35609=CARTESIAN_POINT('Ctrl Pts',(-18.1006895819579,17.7896607547969,122.618237447399)) ;
#35610=CARTESIAN_POINT('Ctrl Pts',(-18.5937018814127,17.9861703352187,122.512467682985)) ;
#35611=CARTESIAN_POINT('Ctrl Pts',(-18.38978122094,17.8061812548089,122.287658244962)) ;
#35612=CARTESIAN_POINT('Ctrl Pts',(-18.8258934089198,17.9994833515347,122.356347563406)) ;
#35613=CARTESIAN_POINT('Ctrl Pts',(-18.6800705189778,17.8194942711249,122.09246633177)) ;
#35614=CARTESIAN_POINT('Ctrl Pts',(-19.0164028181987,18.0093999097677,122.271568361071)) ;
#35615=CARTESIAN_POINT('Ctrl Pts',(-18.9181973224311,17.8294108293579,121.986503440677)) ;
#35616=CARTESIAN_POINT('Ctrl Pts',(-19.2209294726659,18.0194275780706,122.220690420935)) ;
#35617=CARTESIAN_POINT('Ctrl Pts',(-19.1738622433812,17.8394384976607,121.922906470972)) ;
#35618=CARTESIAN_POINT('Ctrl Pts',(-19.4974318665862,18.0326081678152,122.200829010894)) ;
#35619=CARTESIAN_POINT('Ctrl Pts',(-19.5194723945111,17.8526190874054,121.898080551873)) ;
#35620=CARTESIAN_POINT('Ctrl Pts',(-19.8468976293333,18.0493563069346,122.268323420744)) ;
#35621=CARTESIAN_POINT('Ctrl Pts',(-19.9563231936463,17.8693672265248,121.98245538237)) ;
#35622=CARTESIAN_POINT('Ctrl Pts',(-20.208402785875,18.0691510494452,122.484267090907)) ;
#35623=CARTESIAN_POINT('Ctrl Pts',(-20.4081951552993,17.8891619690354,122.252387033686)) ;
#35624=CARTESIAN_POINT('Ctrl Pts',(-20.4779851808533,18.089195442254,122.814181391248)) ;
#35625=CARTESIAN_POINT('Ctrl Pts',(-20.7451718133563,17.9092063618442,122.664783040621)) ;
#35626=CARTESIAN_POINT('Ctrl Pts',(-20.6171002054309,18.1090346245527,123.212537767396)) ;
#35627=CARTESIAN_POINT('Ctrl Pts',(-20.9190608631241,17.9290455441429,123.162728597943)) ;
#35628=CARTESIAN_POINT('Ctrl Pts',(-20.6129501344917,18.1289599482456,123.636081201346)) ;
#35629=CARTESIAN_POINT('Ctrl Pts',(-20.9138698456781,17.9489708678357,123.692157121914)) ;
#35630=CARTESIAN_POINT('Ctrl Pts',(-20.4644170209885,18.1488835862971,124.032892736758)) ;
#35631=CARTESIAN_POINT('Ctrl Pts',(-20.7282004988174,17.9688945058873,124.188169695687)) ;
#35632=CARTESIAN_POINT('Ctrl Pts',(-20.1895488356295,18.1688084597626,124.355214759084)) ;
#35633=CARTESIAN_POINT('Ctrl Pts',(-20.3846133571134,17.9888193793528,124.591069561722)) ;
#35634=CARTESIAN_POINT('Ctrl Pts',(-19.8222522044971,18.1886870668415,124.564420794737)) ;
#35635=CARTESIAN_POINT('Ctrl Pts',(-19.9254924403146,18.0086979864317,124.852574068787)) ;
#35636=CARTESIAN_POINT('Ctrl Pts',(-19.4036094051165,18.2086645096735,124.636282835696)) ;
#35637=CARTESIAN_POINT('Ctrl Pts',(-19.4021887856864,18.0286754292637,124.9423992146)) ;
#35638=CARTESIAN_POINT('Ctrl Pts',(-18.9865333106449,18.2285963577582,124.560840820189)) ;
#35639=CARTESIAN_POINT('Ctrl Pts',(-18.8808448567096,18.0486072773484,124.848094480844)) ;
#35640=CARTESIAN_POINT('Ctrl Pts',(-18.6207574150074,18.2484916261008,124.348382771225)) ;
#35641=CARTESIAN_POINT('Ctrl Pts',(-18.423627145768,18.0685025456909,124.582520931737)) ;
#35642=CARTESIAN_POINT('Ctrl Pts',(-18.3486814493143,18.2684141245129,124.02368906418)) ;
#35643=CARTESIAN_POINT('Ctrl Pts',(-18.0835339662769,18.0884250441031,124.176653707857)) ;
#35644=CARTESIAN_POINT('Ctrl Pts',(-18.2035687666535,18.2883736063889,123.62485045441)) ;
#35645=CARTESIAN_POINT('Ctrl Pts',(-17.9021445000079,18.1083845259791,123.678105539873)) ;
#35646=CARTESIAN_POINT('Ctrl Pts',(-18.203194006856,18.3082513588482,123.202260983975)) ;
#35647=CARTESIAN_POINT('Ctrl Pts',(-17.9016770429554,18.1282622784384,123.149870596729)) ;
#35648=CARTESIAN_POINT('Ctrl Pts',(-18.3459964134725,18.3281331495828,122.804281369069)) ;
#35649=CARTESIAN_POINT('Ctrl Pts',(-18.0801792550094,18.148144069173,122.65239779118)) ;
#35650=CARTESIAN_POINT('Ctrl Pts',(-18.6191997385848,18.3482064884338,122.476442912359)) ;
#35651=CARTESIAN_POINT('Ctrl Pts',(-18.4216843161546,18.1682174080239,122.242598944776)) ;
#35652=CARTESIAN_POINT('Ctrl Pts',(-18.9830102331295,18.3680109556696,122.264221298364)) ;
#35653=CARTESIAN_POINT('Ctrl Pts',(-18.8764446817884,18.1880218752597,121.977323375749)) ;
#35654=CARTESIAN_POINT('Ctrl Pts',(-19.4008308381281,18.3879942960774,122.187305861743)) ;
#35655=CARTESIAN_POINT('Ctrl Pts',(-19.398720028265,18.2080052156676,121.881178045639)) ;
#35656=CARTESIAN_POINT('Ctrl Pts',(-19.8183304642668,18.4079092606754,122.258027106077)) ;
#35657=CARTESIAN_POINT('Ctrl Pts',(-19.9205934708434,18.2279201802656,121.969578564998)) ;
#35658=CARTESIAN_POINT('Ctrl Pts',(-20.1864288478707,18.4277777953917,122.465496330421)) ;
#35659=CARTESIAN_POINT('Ctrl Pts',(-20.380715850587,18.2477887149819,122.228912632694)) ;
#35660=CARTESIAN_POINT('Ctrl Pts',(-20.4635196115804,18.4478301796035,122.789385037709)) ;
#35661=CARTESIAN_POINT('Ctrl Pts',(-20.727080948349,18.2678410991936,122.633772923459)) ;
#35662=CARTESIAN_POINT('Ctrl Pts',(-20.6120028434724,18.4676041433927,123.182923094544)) ;
#35663=CARTESIAN_POINT('Ctrl Pts',(-20.9126860426802,18.2876150629828,123.125692137809)) ;
#35664=CARTESIAN_POINT('Ctrl Pts',(-20.6176815723447,18.487658522414,123.609124769732)) ;
#35665=CARTESIAN_POINT('Ctrl Pts',(-20.9197870561748,18.3076694420042,123.658444810711)) ;
#35666=CARTESIAN_POINT('Ctrl Pts',(-20.4791262983683,18.5074552599873,124.006731982983)) ;
#35667=CARTESIAN_POINT('Ctrl Pts',(-20.7465962163271,18.3274661795774,124.155452562242)) ;
#35668=CARTESIAN_POINT('Ctrl Pts',(-20.2119627746794,18.5274230723387,124.33658343425)) ;
#35669=CARTESIAN_POINT('Ctrl Pts',(-20.4126446943069,18.3474339919289,124.567768827169)) ;
#35670=CARTESIAN_POINT('Ctrl Pts',(-19.8479424439338,18.5473820484038,124.554891666292)) ;
#35671=CARTESIAN_POINT('Ctrl Pts',(-19.9576212451573,18.367392967994,124.840656736509)) ;
#35672=CARTESIAN_POINT('Ctrl Pts',(-19.4327602934189,18.5672769666812,124.635860460392)) ;
#35673=CARTESIAN_POINT('Ctrl Pts',(-19.4386451944318,18.3872878862713,124.941871042753)) ;
#35674=CARTESIAN_POINT('Ctrl Pts',(-19.0147820526511,18.5871732791315,124.570804620221)) ;
#35675=CARTESIAN_POINT('Ctrl Pts',(-18.9161726452975,18.4071841987217,124.860555263163)) ;
#35676=CARTESIAN_POINT('Ctrl Pts',(-18.6435903312615,18.6070812125056,124.367280330836)) ;
#35677=CARTESIAN_POINT('Ctrl Pts',(-18.4521815633457,18.4270921320958,124.606153931654)) ;
#35678=CARTESIAN_POINT('Ctrl Pts',(-18.3636220458617,18.6270311027941,124.048654042255)) ;
#35679=CARTESIAN_POINT('Ctrl Pts',(-18.1022181076318,18.4470420223842,124.207874213634)) ;
#35680=CARTESIAN_POINT('Ctrl Pts',(-18.2093224184274,18.6469083332954,123.655139111936)) ;
#35681=CARTESIAN_POINT('Ctrl Pts',(-17.9093397629679,18.4669192528855,123.71598284327)) ;
#35682=CARTESIAN_POINT('Ctrl Pts',(-18.1982991555925,18.6668910021664,123.230417623875)) ;
#35683=CARTESIAN_POINT('Ctrl Pts',(-17.8955552161012,18.4869019217566,123.185081472564)) ;
#35684=CARTESIAN_POINT('Ctrl Pts',(-18.3328317480087,18.6868238887468,122.828454448446)) ;
#35685=CARTESIAN_POINT('Ctrl Pts',(-18.0637189575334,18.5068348083369,122.682625101203)) ;
#35686=CARTESIAN_POINT('Ctrl Pts',(-18.5959241687473,18.7067366347647,122.496751886595)) ;
#35687=CARTESIAN_POINT('Ctrl Pts',(-18.3925705509658,18.5267475543548,122.267998602656)) ;
#35688=CARTESIAN_POINT('Ctrl Pts',(-18.8956709172905,18.7233063561065,122.311665038351)) ;
#35689=CARTESIAN_POINT('Ctrl Pts',(-18.7672818816645,18.5433172756967,122.036622749407)) ;
#35690=CARTESIAN_POINT('Ctrl Pts',(-19.1634796639719,18.7366063674115,122.231169175464)) ;
#35691=CARTESIAN_POINT('Ctrl Pts',(-19.1020056145129,18.5566172870017,121.936011376236)) ;
#35692=CARTESIAN_POINT('Ctrl Pts',(-19.44044901437,18.7498765551614,122.198083479457)) ;
#35693=CARTESIAN_POINT('Ctrl Pts',(-19.4482877506097,18.5698874747515,121.894651385031)) ;
#35694=CARTESIAN_POINT('Ctrl Pts',(-19.7904919604174,18.7665039375268,122.248222801517)) ;
#35695=CARTESIAN_POINT('Ctrl Pts',(-19.8857560482336,18.586514857117,121.957313792309)) ;
#35696=CARTESIAN_POINT('Ctrl Pts',(-20.1021440207609,18.783126227272,122.414835522395)) ;
#35697=CARTESIAN_POINT('Ctrl Pts',(-20.2753787251755,18.6031371468622,122.165595250292)) ;
#35698=CARTESIAN_POINT('Ctrl Pts',(-20.3055329334675,18.7963714416665,122.605057021473)) ;
#35699=CARTESIAN_POINT('Ctrl Pts',(-20.5295847929719,18.6163823612567,122.403352527165)) ;
#35700=CARTESIAN_POINT('Ctrl Pts',(-20.4311881436849,18.8062834066272,122.771300615763)) ;
#35701=CARTESIAN_POINT('Ctrl Pts',(-20.6866624263793,18.6262943262174,122.611158628131)) ;
#35702=CARTESIAN_POINT('Ctrl Pts',(-20.5272430540412,18.8163420297916,122.959664946299)) ;
#35703=CARTESIAN_POINT('Ctrl Pts',(-20.8067318368844,18.6363529493818,122.846612050216)) ;
#35704=CARTESIAN_POINT('Ctrl Pts',(-20.5880949584386,18.8261821439075,123.157414828597)) ;
#35705=CARTESIAN_POINT('Ctrl Pts',(-20.8827997470549,18.6461930634976,123.093798587246)) ;
#35706=CARTESIAN_POINT('Ctrl Pts',(-20.6144765414881,18.8362479288651,123.367346989237)) ;
#35707=CARTESIAN_POINT('Ctrl Pts',(-20.9157793857665,18.6562588484553,123.356213554675)) ;
#35708=CARTESIAN_POINT('Ctrl Pts',(-20.6041033810044,18.846131246653,123.574893561351)) ;
#35709=CARTESIAN_POINT('Ctrl Pts',(-20.9028157444031,18.6661421662431,123.61564679858)) ;
#35710=CARTESIAN_POINT('Ctrl Pts',(-20.557811278042,18.8561206845115,123.779716355101)) ;
#35711=CARTESIAN_POINT('Ctrl Pts',(-20.8449533316888,18.6761316041017,123.871675964838)) ;
#35712=CARTESIAN_POINT('Ctrl Pts',(-20.4767860972541,18.8660843985643,123.972890703501)) ;
#35713=CARTESIAN_POINT('Ctrl Pts',(-20.7436744284791,18.6860953181544,124.113145006434)) ;
#35714=CARTESIAN_POINT('Ctrl Pts',(-20.3632771377155,18.8760794102235,124.149739579038)) ;
#35715=CARTESIAN_POINT('Ctrl Pts',(-20.601790555913,18.6960903298137,124.334207674829)) ;
#35716=CARTESIAN_POINT('Ctrl Pts',(-20.2199721057436,18.8861157019177,124.304588195844)) ;
#35717=CARTESIAN_POINT('Ctrl Pts',(-20.4226612590581,18.7061266215079,124.527770408806)) ;
#35718=CARTESIAN_POINT('Ctrl Pts',(-20.0553231898177,18.8959620796112,124.430069749636)) ;
#35719=CARTESIAN_POINT('Ctrl Pts',(-20.2168518530314,18.7159729992014,124.684624557597)) ;
#35720=CARTESIAN_POINT('Ctrl Pts',(-19.8690215673185,18.9059470237619,124.526730415756)) ;
#35721=CARTESIAN_POINT('Ctrl Pts',(-19.9839760536342,18.7259579433521,124.805452933114)) ;
#35722=CARTESIAN_POINT('Ctrl Pts',(-19.6697047219603,18.9158839948918,124.589408387716)) ;
#35723=CARTESIAN_POINT('Ctrl Pts',(-19.7348307743304,18.735894914482,124.88380310373)) ;
#35724=CARTESIAN_POINT('Ctrl Pts',(-19.4602197023148,18.9259337795236,124.616715999974)) ;
#35725=CARTESIAN_POINT('Ctrl Pts',(-19.4729748038797,18.7459446991137,124.917940423266)) ;
#35726=CARTESIAN_POINT('Ctrl Pts',(-19.2533184450846,18.9357842416011,124.607579273782)) ;
#35727=CARTESIAN_POINT('Ctrl Pts',(-19.2143479954999,18.7557951611912,124.906522324795)) ;
#35728=CARTESIAN_POINT('Ctrl Pts',(-19.0485745773188,18.9457562551215,124.562644959168)) ;
#35729=CARTESIAN_POINT('Ctrl Pts',(-18.9584174462434,18.7657671747116,124.850357149064)) ;
#35730=CARTESIAN_POINT('Ctrl Pts',(-18.8542477972193,18.9557514022409,124.482609220366)) ;
#35731=CARTESIAN_POINT('Ctrl Pts',(-18.715507831181,18.7757623218311,124.750315034933)) ;
#35732=CARTESIAN_POINT('Ctrl Pts',(-18.6762610468344,18.965785371977,124.369422704143)) ;
#35733=CARTESIAN_POINT('Ctrl Pts',(-18.4930228487092,18.7857962915672,124.608834245191)) ;
#35734=CARTESIAN_POINT('Ctrl Pts',(-18.5231511574649,18.9756409176476,124.229798349696)) ;
#35735=CARTESIAN_POINT('Ctrl Pts',(-18.3016334314437,18.7956518372378,124.434305714766)) ;
#35736=CARTESIAN_POINT('Ctrl Pts',(-18.3945701733205,18.9856396746608,124.063548623651)) ;
#35737=CARTESIAN_POINT('Ctrl Pts',(-18.1409049402288,18.805650594251,124.226495189786)) ;
#35738=CARTESIAN_POINT('Ctrl Pts',(-18.2975958365009,18.995536809898,123.879424723443)) ;
#35739=CARTESIAN_POINT('Ctrl Pts',(-18.0196844553745,18.8155477294882,123.99634137888)) ;
#35740=CARTESIAN_POINT('Ctrl Pts',(-18.2330434105871,19.0055899057376,123.678199215092)) ;
#35741=CARTESIAN_POINT('Ctrl Pts',(-17.9389912916734,18.8256008253278,123.744810346015)) ;
#35742=CARTESIAN_POINT('Ctrl Pts',(-18.2048687725473,19.0154734144682,123.472321453931)) ;
#35743=CARTESIAN_POINT('Ctrl Pts',(-17.9037702161994,18.8354843340584,123.487463211665)) ;
#35744=CARTESIAN_POINT('Ctrl Pts',(-18.2124671547143,19.0254682871143,123.262341510424)) ;
#35745=CARTESIAN_POINT('Ctrl Pts',(-17.9132654844711,18.8454792067045,123.224988077214)) ;
#35746=CARTESIAN_POINT('Ctrl Pts',(-18.2568443718026,19.03548824875,123.056405743036)) ;
#35747=CARTESIAN_POINT('Ctrl Pts',(-17.9687343277872,18.8554991683402,122.967567757769)) ;
#35748=CARTESIAN_POINT('Ctrl Pts',(-18.3352281082984,19.0453936125498,122.863482475236)) ;
#35749=CARTESIAN_POINT('Ctrl Pts',(-18.0667115840273,18.86540453214,122.726412358602)) ;
#35750=CARTESIAN_POINT('Ctrl Pts',(-18.4459450487129,19.0553342001574,122.686255011705)) ;
#35751=CARTESIAN_POINT('Ctrl Pts',(-18.2051056277496,18.8753451197476,122.50487638209)) ;
#35752=CARTESIAN_POINT('Ctrl Pts',(-18.5865641592456,19.065337018258,122.529862565855)) ;
#35753=CARTESIAN_POINT('Ctrl Pts',(-18.3808775939559,18.8853479378482,122.30938398515)) ;
#35754=CARTESIAN_POINT('Ctrl Pts',(-18.7529137805727,19.0753717299822,122.400141597635)) ;
#35755=CARTESIAN_POINT('Ctrl Pts',(-18.5888129419414,18.8953826495723,122.147230647386)) ;
#35756=CARTESIAN_POINT('Ctrl Pts',(-18.9355927334257,19.0852166367195,122.302823707512)) ;
#35757=CARTESIAN_POINT('Ctrl Pts',(-18.8171608789113,18.9052275563097,122.025580673966)) ;
#35758=CARTESIAN_POINT('Ctrl Pts',(-19.135044952863,19.0952024892885,122.237424139112)) ;
#35759=CARTESIAN_POINT('Ctrl Pts',(-19.0664754950351,18.9152134088786,121.943828689827)) ;
#35760=CARTESIAN_POINT('Ctrl Pts',(-19.3418110241518,19.1051372977015,122.207643930743)) ;
#35761=CARTESIAN_POINT('Ctrl Pts',(-19.324933039813,18.9251482172917,121.906600838768)) ;
#35762=CARTESIAN_POINT('Ctrl Pts',(-19.5531110415552,19.1151948247826,122.214485106709)) ;
#35763=CARTESIAN_POINT('Ctrl Pts',(-19.5890580305802,18.9352057443728,121.915149697204)) ;
#35764=CARTESIAN_POINT('Ctrl Pts',(-19.7552767450465,19.1250164797797,122.256593308277)) ;
#35765=CARTESIAN_POINT('Ctrl Pts',(-19.8417664438669,18.9450273993699,121.967782613236)) ;
#35766=CARTESIAN_POINT('Ctrl Pts',(-19.9517461949997,19.1350725239527,122.334610066435)) ;
#35767=CARTESIAN_POINT('Ctrl Pts',(-20.0873540689594,18.9550834435429,122.065301217986)) ;
#35768=CARTESIAN_POINT('Ctrl Pts',(-20.1294455067056,19.1450132639979,122.44461757867)) ;
#35769=CARTESIAN_POINT('Ctrl Pts',(-20.3094798343404,18.965024183588,122.202808615077)) ;
#35770=CARTESIAN_POINT('Ctrl Pts',(-20.2852002013898,19.1549173850707,122.582803466189)) ;
#35771=CARTESIAN_POINT('Ctrl Pts',(-20.5041752042794,18.9749283046609,122.37553951635)) ;
#35772=CARTESIAN_POINT('Ctrl Pts',(-20.4163570695297,19.164964926225,122.748363557703)) ;
#35773=CARTESIAN_POINT('Ctrl Pts',(-20.6681231447569,18.9849758458152,122.582488035547)) ;
#35774=CARTESIAN_POINT('Ctrl Pts',(-20.5154426781397,19.1748636778254,122.931394298921)) ;
#35775=CARTESIAN_POINT('Ctrl Pts',(-20.7919825436342,18.9948745974155,122.811275811251)) ;
#35776=CARTESIAN_POINT('Ctrl Pts',(-20.5823095621663,19.1849121567912,123.13175874193)) ;
#35777=CARTESIAN_POINT('Ctrl Pts',(-20.8755683817589,19.0049230763813,123.061730492488)) ;
#35778=CARTESIAN_POINT('Ctrl Pts',(-20.6128955919429,19.1947996538749,123.337384367782)) ;
#35779=CARTESIAN_POINT('Ctrl Pts',(-20.9138033740023,19.0148105734651,123.318762800782)) ;
#35780=CARTESIAN_POINT('Ctrl Pts',(-20.6076449007628,19.204792744173,123.547386563793)) ;
#35781=CARTESIAN_POINT('Ctrl Pts',(-20.9072423075694,19.0248036637631,123.581265757215)) ;
#35782=CARTESIAN_POINT('Ctrl Pts',(-20.5661040890578,19.2147449142333,123.752459949604)) ;
#35783=CARTESIAN_POINT('Ctrl Pts',(-20.8553184944802,19.0347558338234,123.837608299637)) ;
#35784=CARTESIAN_POINT('Ctrl Pts',(-20.4899691627066,19.2246833341478,123.947015816567)) ;
#35785=CARTESIAN_POINT('Ctrl Pts',(-20.7601517685362,19.044694253738,124.080804362986)) ;
#35786=CARTESIAN_POINT('Ctrl Pts',(-20.3808817205689,19.2346684642334,124.126388705012)) ;
#35787=CARTESIAN_POINT('Ctrl Pts',(-20.6237942336124,19.0546793838236,124.305021774799)) ;
#35788=CARTESIAN_POINT('Ctrl Pts',(-20.241378136144,19.2447051536475,124.284677346866)) ;
#35789=CARTESIAN_POINT('Ctrl Pts',(-20.4494165140451,19.0647160732376,124.502884010829)) ;
#35790=CARTESIAN_POINT('Ctrl Pts',(-20.0796809670724,19.25455983764,124.414229163885)) ;
#35791=CARTESIAN_POINT('Ctrl Pts',(-20.2472957010154,19.0745707572301,124.664826057178)) ;
#35792=CARTESIAN_POINT('Ctrl Pts',(-19.8954624316429,19.2645593216878,124.515427636075)) ;
#35793=CARTESIAN_POINT('Ctrl Pts',(-20.0170234288381,19.084570241278,124.791326058975)) ;
#35794=CARTESIAN_POINT('Ctrl Pts',(-19.6985533037412,19.2744544104647,124.582628798739)) ;
#35795=CARTESIAN_POINT('Ctrl Pts',(-19.7708869846868,19.0944653300549,124.875329679464)) ;
#35796=CARTESIAN_POINT('Ctrl Pts',(-19.4895873463579,19.2845149651109,124.615123526839)) ;
#35797=CARTESIAN_POINT('Ctrl Pts',(-19.5096800897253,19.1045258847011,124.915950078739)) ;
#35798=CARTESIAN_POINT('Ctrl Pts',(-19.2825491814808,19.2943642294838,124.611047104812)) ;
#35799=CARTESIAN_POINT('Ctrl Pts',(-19.2508813050705,19.1143751490739,124.910856545267)) ;
#35800=CARTESIAN_POINT('Ctrl Pts',(-19.0756100518396,19.3043914819316,124.570889809376)) ;
#35801=CARTESIAN_POINT('Ctrl Pts',(-18.9922070756682,19.1244024015218,124.860661757926)) ;
#35802=CARTESIAN_POINT('Ctrl Pts',(-18.8789515708921,19.3144197795018,124.494880706852)) ;
#35803=CARTESIAN_POINT('Ctrl Pts',(-18.7463833098718,19.1344306990919,124.765652294149)) ;
#35804=CARTESIAN_POINT('Ctrl Pts',(-18.701566831824,19.3242659085078,124.388210448307)) ;
#35805=CARTESIAN_POINT('Ctrl Pts',(-18.5246504441737,19.1442768280979,124.63231552407)) ;
#35806=CARTESIAN_POINT('Ctrl Pts',(-18.5427028733491,19.3342598138698,124.250713710067)) ;
#35807=CARTESIAN_POINT('Ctrl Pts',(-18.3260692253039,19.15427073346,124.460445802983)) ;
#35808=CARTESIAN_POINT('Ctrl Pts',(-18.4100146534908,19.3442839115529,124.086985981103)) ;
#35809=CARTESIAN_POINT('Ctrl Pts',(-18.1602075358963,19.1642948311431,124.255787351985)) ;
#35810=CARTESIAN_POINT('Ctrl Pts',(-18.3089126305251,19.3541737394069,123.90530352091)) ;
#35811=CARTESIAN_POINT('Ctrl Pts',(-18.0338280399236,19.1741846589971,124.02868439438)) ;
#35812=CARTESIAN_POINT('Ctrl Pts',(-18.2399042502461,19.3641657208373,123.706908085251)) ;
#35813=CARTESIAN_POINT('Ctrl Pts',(-17.9475659143818,19.1841766404275,123.780690475597)) ;
#35814=CARTESIAN_POINT('Ctrl Pts',(-18.2065905895425,19.3741127256032,123.50046117222)) ;
#35815=CARTESIAN_POINT('Ctrl Pts',(-17.9059220810719,19.1941236451933,123.522631607334)) ;
#35816=CARTESIAN_POINT('Ctrl Pts',(-18.2092454060776,19.384062376993,123.291296502426)) ;
#35817=CARTESIAN_POINT('Ctrl Pts',(-17.9092390394881,19.2040732965831,123.261175270485)) ;
#35818=CARTESIAN_POINT('Ctrl Pts',(-18.2486861191594,19.3940993799704,123.084011953046)) ;
#35819=CARTESIAN_POINT('Ctrl Pts',(-17.9585383067173,19.2141102995605,123.002069407988)) ;
#35820=CARTESIAN_POINT('Ctrl Pts',(-18.3222825230277,19.4039882884054,122.889570998935)) ;
#35821=CARTESIAN_POINT('Ctrl Pts',(-18.0505326597858,19.2239992079956,122.75901679837)) ;
#35822=CARTESIAN_POINT('Ctrl Pts',(-18.4292681158825,19.4139776208829,122.708864244681)) ;
#35823=CARTESIAN_POINT('Ctrl Pts',(-18.1842635125467,19.233988540473,122.533132432026)) ;
#35824=CARTESIAN_POINT('Ctrl Pts',(-18.5657022346844,19.42393617632,122.550072619534)) ;
#35825=CARTESIAN_POINT('Ctrl Pts',(-18.3548053009727,19.2439470959102,122.334641591402)) ;
#35826=CARTESIAN_POINT('Ctrl Pts',(-18.7263649466662,19.4338357475205,122.417759602104)) ;
#35827=CARTESIAN_POINT('Ctrl Pts',(-18.5556335270532,19.2538466671106,122.169248739328)) ;
#35828=CARTESIAN_POINT('Ctrl Pts',(-18.9102833479291,19.4438836727725,122.313900274746)) ;
#35829=CARTESIAN_POINT('Ctrl Pts',(-18.7855306745669,19.2638945923626,122.039423510043)) ;
#35830=CARTESIAN_POINT('Ctrl Pts',(-19.1064125465237,19.4537789722985,122.244448286497)) ;
#35831=CARTESIAN_POINT('Ctrl Pts',(-19.0306926009138,19.2737898918887,121.952607002174)) ;
#35832=CARTESIAN_POINT('Ctrl Pts',(-19.3150144344435,19.4638408287464,122.209510718595)) ;
#35833=CARTESIAN_POINT('Ctrl Pts',(-19.2914444276043,19.2838517483366,121.908933829256)) ;
#35834=CARTESIAN_POINT('Ctrl Pts',(-19.521965316198,19.4736846751631,122.211242753843)) ;
#35835=CARTESIAN_POINT('Ctrl Pts',(-19.5501343610647,19.2936955947532,121.911097613334)) ;
#35836=CARTESIAN_POINT('Ctrl Pts',(-19.7280448443102,19.4836476242911,122.248623144845)) ;
#35837=CARTESIAN_POINT('Ctrl Pts',(-19.8077343935963,19.3036585438813,121.95782219521)) ;
#35838=CARTESIAN_POINT('Ctrl Pts',(-19.9258004100159,19.4936816607191,122.322067326375)) ;
#35839=CARTESIAN_POINT('Ctrl Pts',(-20.0549291177515,19.3136925803093,122.049626314935)) ;
#35840=CARTESIAN_POINT('Ctrl Pts',(-20.1052428274456,19.5035690876772,122.426981156448)) ;
#35841=CARTESIAN_POINT('Ctrl Pts',(-20.279233546627,19.3235800072674,122.180768204286)) ;
#35842=CARTESIAN_POINT('Ctrl Pts',(-20.2660510972554,19.5135835220135,122.562891810069)) ;
#35843=CARTESIAN_POINT('Ctrl Pts',(-20.4802444747732,19.3335944416037,122.350655841033)) ;
#35844=CARTESIAN_POINT('Ctrl Pts',(-20.4006689400157,19.5236184666485,122.725307394749)) ;
#35845=CARTESIAN_POINT('Ctrl Pts',(-20.64851754086,19.3436293862386,122.55367450977)) ;
#35846=CARTESIAN_POINT('Ctrl Pts',(-20.5034449260328,19.5334508166795,122.90468153521)) ;
#35847=CARTESIAN_POINT('Ctrl Pts',(-20.7769890299039,19.3534617362697,122.777893029289)) ;
#35848=CARTESIAN_POINT('Ctrl Pts',(-20.5752821949681,19.5435262557967,123.10390261523)) ;
#35849=CARTESIAN_POINT('Ctrl Pts',(-20.8667862747104,19.3635371753869,123.026918659829)) ;
#35850=CARTESIAN_POINT('Ctrl Pts',(-20.6107689996992,19.5533787210313,123.308014325579)) ;
#35851=CARTESIAN_POINT('Ctrl Pts',(-20.9111458115888,19.3733896406215,123.282059452488)) ;
#35852=CARTESIAN_POINT('Ctrl Pts',(-20.6104349718264,19.5634515986082,123.519742050673)) ;
#35853=CARTESIAN_POINT('Ctrl Pts',(-20.9107290325101,19.3834625181983,123.546718673393)) ;
#35854=CARTESIAN_POINT('Ctrl Pts',(-20.5741538852815,19.5732941948007,123.723476229926)) ;
#35855=CARTESIAN_POINT('Ctrl Pts',(-20.8653781809411,19.3933051143909,123.801387925584)) ;
#35856=CARTESIAN_POINT('Ctrl Pts',(-20.5027249485285,19.583274578916,123.920753137784)) ;
#35857=CARTESIAN_POINT('Ctrl Pts',(-20.7760923679228,19.4032854985061,124.047984519864)) ;
#35858=CARTESIAN_POINT('Ctrl Pts',(-20.3973703972249,19.5932930595648,124.10312422854)) ;
#35859=CARTESIAN_POINT('Ctrl Pts',(-20.64439975022,19.4133039791549,124.275948701182)) ;
#35860=CARTESIAN_POINT('Ctrl Pts',(-20.2640988385909,19.6031763745651,124.262563519958)) ;
#35861=CARTESIAN_POINT('Ctrl Pts',(-20.477809965381,19.4231872941553,124.475248963888)) ;
#35862=CARTESIAN_POINT('Ctrl Pts',(-20.1021786910339,19.6132446716556,124.398835786557)) ;
#35863=CARTESIAN_POINT('Ctrl Pts',(-20.2754104278424,19.4332555912458,124.645589428326)) ;
#35864=CARTESIAN_POINT('Ctrl Pts',(-19.923452222074,19.6230747400279,124.502661288851)) ;
#35865=CARTESIAN_POINT('Ctrl Pts',(-20.0520012191857,19.443085659618,124.775372441356)) ;
#35866=CARTESIAN_POINT('Ctrl Pts',(-19.7249017076277,19.6331415324963,124.575813941918)) ;
#35867=CARTESIAN_POINT('Ctrl Pts',(-19.8038135625344,19.4531524520865,124.866813416566)) ;
#35868=CARTESIAN_POINT('Ctrl Pts',(-19.5202469349877,19.6430308659848,124.612640504371)) ;
#35869=CARTESIAN_POINT('Ctrl Pts',(-19.5479941097324,19.463041785575,124.912847154489)) ;
#35870=CARTESIAN_POINT('Ctrl Pts',(-19.3100107554735,19.6530329974009,124.613711705916)) ;
#35871=CARTESIAN_POINT('Ctrl Pts',(-19.2851987471254,19.473043916991,124.91418637848)) ;
#35872=CARTESIAN_POINT('Ctrl Pts',(-19.1043078669417,19.6629568670219,124.578660210897)) ;
#35873=CARTESIAN_POINT('Ctrl Pts',(-19.0280693627493,19.4829677866121,124.87037205227)) ;
#35874=CARTESIAN_POINT('Ctrl Pts',(-18.9055323179189,19.6730003825391,124.507541988361)) ;
#35875=CARTESIAN_POINT('Ctrl Pts',(-18.7796000674566,19.4930113021293,124.781474531123)) ;
#35876=CARTESIAN_POINT('Ctrl Pts',(-18.7248906132605,19.6828825954274,124.404844874836)) ;
#35877=CARTESIAN_POINT('Ctrl Pts',(-18.5537969175997,19.5028935150175,124.653102677006)) ;
#35878=CARTESIAN_POINT('Ctrl Pts',(-18.5618762979718,19.6929506726468,124.269896713313)) ;
#35879=CARTESIAN_POINT('Ctrl Pts',(-18.3500292627666,19.512961592237,124.484417808862)) ;
#35880=CARTESIAN_POINT('Ctrl Pts',(-18.42770753592,19.702789177381,124.112435729889)) ;
#35881=CARTESIAN_POINT('Ctrl Pts',(-18.1823173294474,19.5228000969712,124.287590469328)) ;
#35882=CARTESIAN_POINT('Ctrl Pts',(-18.3203002755283,19.7128519458104,123.930208646522)) ;
#35883=CARTESIAN_POINT('Ctrl Pts',(-18.048058520279,19.5328628654006,124.059806890009)) ;
#35884=CARTESIAN_POINT('Ctrl Pts',(-18.2475857905658,19.7227489390931,123.735249596216)) ;
#35885=CARTESIAN_POINT('Ctrl Pts',(-17.9571650618056,19.5427598586833,123.81610713825)) ;
#35886=CARTESIAN_POINT('Ctrl Pts',(-18.2090139650098,19.7326801667279,123.530063285988)) ;
#35887=CARTESIAN_POINT('Ctrl Pts',(-17.9089504190964,19.552691086318,123.559623490834)) ;
#35888=CARTESIAN_POINT('Ctrl Pts',(-18.206860266534,19.74272232537,123.318958748455)) ;
#35889=CARTESIAN_POINT('Ctrl Pts',(-17.9062584822313,19.5627332449602,123.295743025401)) ;
#35890=CARTESIAN_POINT('Ctrl Pts',(-18.2407132566598,19.7526090349011,123.113875533513)) ;
#35891=CARTESIAN_POINT('Ctrl Pts',(-17.948575137129,19.5726199544913,123.039387974095)) ;
#35892=CARTESIAN_POINT('Ctrl Pts',(-18.3100612563688,19.7626020073297,122.915577612345)) ;
#35893=CARTESIAN_POINT('Ctrl Pts',(-18.0352605666354,19.5826129269199,122.791515506219)) ;
#35894=CARTESIAN_POINT('Ctrl Pts',(-18.4123864646547,19.7725482018663,122.733228885072)) ;
#35895=CARTESIAN_POINT('Ctrl Pts',(-18.1631676695272,19.5925591214565,122.563579250509)) ;
#35896=CARTESIAN_POINT('Ctrl Pts',(-18.544466725532,19.7824935767178,122.571123242096)) ;
#35897=CARTESIAN_POINT('Ctrl Pts',(-18.3282687770874,19.602504496308,122.360947075169)) ;
#35898=CARTESIAN_POINT('Ctrl Pts',(-18.7046124165122,19.7925484960777,122.433182725376)) ;
#35899=CARTESIAN_POINT('Ctrl Pts',(-18.5284509193159,19.6125594156678,122.188521930162)) ;
#35900=CARTESIAN_POINT('Ctrl Pts',(-18.8818996060472,19.8023700155212,122.327286077013)) ;
#35901=CARTESIAN_POINT('Ctrl Pts',(-18.7500615821666,19.6223809351113,122.056150769532)) ;
#35902=CARTESIAN_POINT('Ctrl Pts',(-19.0795285112847,19.8124357842881,122.251735177665)) ;
#35903=CARTESIAN_POINT('Ctrl Pts',(-18.9970975871785,19.6324467038783,121.961712899022)) ;
#35904=CARTESIAN_POINT('Ctrl Pts',(-19.2839777888797,19.8223377059431,122.212355081407)) ;
#35905=CARTESIAN_POINT('Ctrl Pts',(-19.2526602062973,19.6423486255333,121.912488218157)) ;
#35906=CARTESIAN_POINT('Ctrl Pts',(-19.4950664842811,19.8323807647642,122.208839746125)) ;
#35907=CARTESIAN_POINT('Ctrl Pts',(-19.5165208729991,19.6523916843543,121.908094752739)) ;
#35908=CARTESIAN_POINT('Ctrl Pts',(-19.7007200879061,19.8422867588069,122.241689755879)) ;
#35909=CARTESIAN_POINT('Ctrl Pts',(-19.7735886685329,19.662297678397,121.949158051642)) ;
#35910=CARTESIAN_POINT('Ctrl Pts',(-19.8983711923909,19.8522245318887,122.309384254829)) ;
#35911=CARTESIAN_POINT('Ctrl Pts',(-20.020652879947,19.6722354514788,122.033777229836)) ;
#35912=CARTESIAN_POINT('Ctrl Pts',(-20.0830422576944,19.862264895621,122.41160883403)) ;
#35913=CARTESIAN_POINT('Ctrl Pts',(-20.2514911587516,19.6822758152111,122.161558568132)) ;
#35914=CARTESIAN_POINT('Ctrl Pts',(-20.2447669194783,19.8721522393445,122.542209039445)) ;
#35915=CARTESIAN_POINT('Ctrl Pts',(-20.4536472526917,19.6921631589346,122.324810150198)) ;
#35916=CARTESIAN_POINT('Ctrl Pts',(-20.383052541564,19.8821444699132,122.700322050731)) ;
#35917=CARTESIAN_POINT('Ctrl Pts',(-20.6265036650204,19.7021553895033,122.522452222895)) ;
#35918=CARTESIAN_POINT('Ctrl Pts',(-20.4912730530166,19.8920929976968,122.879309922931)) ;
#35919=CARTESIAN_POINT('Ctrl Pts',(-20.7617787532514,19.712103917287,122.746188030243)) ;
#35920=CARTESIAN_POINT('Ctrl Pts',(-20.5669463250774,19.9020297814201,123.074005487427)) ;
#35921=CARTESIAN_POINT('Ctrl Pts',(-20.8563695651835,19.7220407010102,122.989558473114)) ;
#35922=CARTESIAN_POINT('Ctrl Pts',(-20.6081237683006,19.912012782217,123.279827787106)) ;
#35923=CARTESIAN_POINT('Ctrl Pts',(-20.9078402628114,19.7320237018072,123.246836830898)) ;
#35924=CARTESIAN_POINT('Ctrl Pts',(-20.6125768739177,19.9220566690578,123.490910400367)) ;
#35925=CARTESIAN_POINT('Ctrl Pts',(-20.9134056045136,19.7420675886479,123.510689929297)) ;
#35926=CARTESIAN_POINT('Ctrl Pts',(-20.5814828811847,19.9318846926323,123.695206220071)) ;
#35927=CARTESIAN_POINT('Ctrl Pts',(-20.8745366917446,19.7518956122225,123.766060949748)) ;
#35928=CARTESIAN_POINT('Ctrl Pts',(-20.5138218279158,19.941961940846,123.895916711096)) ;
#35929=CARTESIAN_POINT('Ctrl Pts',(-20.7899593278494,19.7619728604362,124.01694825061)) ;
#35930=CARTESIAN_POINT('Ctrl Pts',(-20.4147085608249,19.9518114961513,124.077785912975)) ;
#35931=CARTESIAN_POINT('Ctrl Pts',(-20.6660660069684,19.7718224157414,124.244285226942)) ;
#35932=CARTESIAN_POINT('Ctrl Pts',(-20.2825893140887,19.961894204349,124.243476019033)) ;
#35933=CARTESIAN_POINT('Ctrl Pts',(-20.5009161893585,19.7819051239392,124.451396677713)) ;
#35934=CARTESIAN_POINT('Ctrl Pts',(-20.1280154651316,19.9717067972754,124.38015779365)) ;
#35935=CARTESIAN_POINT('Ctrl Pts',(-20.3076968301649,19.7917177168656,124.622248846317)) ;
#35936=CARTESIAN_POINT('Ctrl Pts',(-19.9477519695599,19.9817739895334,124.49096411443)) ;
#35937=CARTESIAN_POINT('Ctrl Pts',(-20.0823669714387,19.8017849091236,124.760755273393)) ;
#35938=CARTESIAN_POINT('Ctrl Pts',(-19.7541568951815,19.991672818996,124.56745105753)) ;
#35939=CARTESIAN_POINT('Ctrl Pts',(-19.8403718039721,19.8116837385861,124.856362880301)) ;
#35940=CARTESIAN_POINT('Ctrl Pts',(-19.5471389116745,20.0017268101862,124.609885515152)) ;
#35941=CARTESIAN_POINT('Ctrl Pts',(-19.581599257852,19.8217377297763,124.909404420848)) ;
#35942=CARTESIAN_POINT('Ctrl Pts',(-19.3396458322229,20.0115985349694,124.615811551427)) ;
#35943=CARTESIAN_POINT('Ctrl Pts',(-19.3222318233438,19.8316094545595,124.916810422216)) ;
#35944=CARTESIAN_POINT('Ctrl Pts',(-19.1302124053593,20.0216689770996,124.585074256382)) ;
#35945=CARTESIAN_POINT('Ctrl Pts',(-19.0604406240676,19.8416798966898,124.878387276265)) ;
#35946=CARTESIAN_POINT('Ctrl Pts',(-18.9339520390974,20.0315020555299,124.520082076835)) ;
#35947=CARTESIAN_POINT('Ctrl Pts',(-18.8151144576221,19.85151297512,124.797145106949)) ;
#35948=CARTESIAN_POINT('Ctrl Pts',(-18.7480434856124,20.0415325290313,124.420574067109)) ;
#35949=CARTESIAN_POINT('Ctrl Pts',(-18.5827297026726,19.8615434486214,124.672758530755)) ;
#35950=CARTESIAN_POINT('Ctrl Pts',(-18.5825831311572,20.0515641283299,124.289788081662)) ;
#35951=CARTESIAN_POINT('Ctrl Pts',(-18.3759053293707,19.8715750479201,124.509274829731)) ;
#35952=CARTESIAN_POINT('Ctrl Pts',(-18.4448629357415,20.0613938293681,124.13573633142)) ;
#35953=CARTESIAN_POINT('Ctrl Pts',(-18.2037555510445,19.8814047489583,124.316708019018)) ;
#35954=CARTESIAN_POINT('Ctrl Pts',(-18.3336698872255,20.0713832674246,123.957571401983)) ;
#35955=CARTESIAN_POINT('Ctrl Pts',(-18.0647658072251,19.8913941870148,124.094000670372)) ;
#35956=CARTESIAN_POINT('Ctrl Pts',(-18.2551742977455,20.0814271706407,123.761552123901)) ;
#35957=CARTESIAN_POINT('Ctrl Pts',(-17.9666480382396,19.9014380902309,123.848976044815)) ;
#35958=CARTESIAN_POINT('Ctrl Pts',(-18.2124417079699,20.0912486914542,123.559542282254)) ;
#35959=CARTESIAN_POINT('Ctrl Pts',(-17.9132339250631,19.9112596110443,123.596462120668)) ;
#35960=CARTESIAN_POINT('Ctrl Pts',(-18.2047766515983,20.1012844157013,123.348703573776)) ;
#35961=CARTESIAN_POINT('Ctrl Pts',(-17.9036546812584,19.9212953352915,123.33291376826)) ;
#35962=CARTESIAN_POINT('Ctrl Pts',(-18.2343404621047,20.1113065696338,123.140074801071)) ;
#35963=CARTESIAN_POINT('Ctrl Pts',(-17.9406113336805,19.9313174892239,123.072128085438)) ;
#35964=CARTESIAN_POINT('Ctrl Pts',(-18.2983054280949,20.1211688013911,122.942870332528)) ;
#35965=CARTESIAN_POINT('Ctrl Pts',(-18.0205697572418,19.9411797209812,122.825622198573)) ;
#35966=CARTESIAN_POINT('Ctrl Pts',(-18.3959846631864,20.131127871849,122.757674344572)) ;
#35967=CARTESIAN_POINT('Ctrl Pts',(-18.1426708876465,19.9511387914392,122.59412792976)) ;
#35968=CARTESIAN_POINT('Ctrl Pts',(-18.525566423674,20.1411630442251,122.591200036149)) ;
#35969=CARTESIAN_POINT('Ctrl Pts',(-18.30464968217,19.9611739638153,122.386036390994)) ;
#35970=CARTESIAN_POINT('Ctrl Pts',(-18.6794843882295,20.1510434293834,122.45168426529)) ;
#35971=CARTESIAN_POINT('Ctrl Pts',(-18.4970491713778,19.9710543489736,122.211642765618)) ;
#35972=CARTESIAN_POINT('Ctrl Pts',(-18.8583463704345,20.1611001439773,122.33899114382)) ;
#35973=CARTESIAN_POINT('Ctrl Pts',(-18.7206276526731,19.9811110635675,122.070778322251)) ;
#35974=CARTESIAN_POINT('Ctrl Pts',(-19.0506399135892,20.1709794125494,122.260478579803)) ;
#35975=CARTESIAN_POINT('Ctrl Pts',(-18.9609961306176,19.9909903321396,121.972639347057)) ;
#35976=CARTESIAN_POINT('Ctrl Pts',(-19.2558093771799,20.1809703700351,122.21550063428)) ;
#35977=CARTESIAN_POINT('Ctrl Pts',(-19.2174586026776,20.0009812896253,121.916419162023)) ;
#35978=CARTESIAN_POINT('Ctrl Pts',(-19.466736361105,20.1910110286703,122.20725269721)) ;
#35979=CARTESIAN_POINT('Ctrl Pts',(-19.4811173295956,20.0110219482604,121.906111456717)) ;
#35980=CARTESIAN_POINT('Ctrl Pts',(-19.6716056707991,20.2008440083783,122.234820237226)) ;
#35981=CARTESIAN_POINT('Ctrl Pts',(-19.737204609292,20.0208549279685,121.940573290785)) ;
#35982=CARTESIAN_POINT('Ctrl Pts',(-19.8719676861379,20.210837141628,122.297989647427)) ;
#35983=CARTESIAN_POINT('Ctrl Pts',(-19.9876565139977,20.0308480612182,122.019537420659)) ;
#35984=CARTESIAN_POINT('Ctrl Pts',(-20.0588521291231,20.2208691940113,122.395761902795)) ;
#35985=CARTESIAN_POINT('Ctrl Pts',(-20.2212609501669,20.0408801136015,122.141754795269)) ;
#35986=CARTESIAN_POINT('Ctrl Pts',(-20.2232832799828,20.2307344229627,122.522142243572)) ;
#35987=CARTESIAN_POINT('Ctrl Pts',(-20.4267990070475,20.0507453425528,122.299732570572)) ;
#35988=CARTESIAN_POINT('Ctrl Pts',(-20.3650928807111,20.2406963642059,122.676265084852)) ;
#35989=CARTESIAN_POINT('Ctrl Pts',(-20.6040593214111,20.060707283796,122.492388017691)) ;
#35990=CARTESIAN_POINT('Ctrl Pts',(-20.4785174817246,20.2507310792426,122.854128710168)) ;
#35991=CARTESIAN_POINT('Ctrl Pts',(-20.7458379854083,20.0707419988328,122.714718839224)) ;
#35992=CARTESIAN_POINT('Ctrl Pts',(-20.5584598459099,20.2606168495867,123.045995752101)) ;
#35993=CARTESIAN_POINT('Ctrl Pts',(-20.8457638320902,20.0806277691768,122.954554133182)) ;
#35994=CARTESIAN_POINT('Ctrl Pts',(-20.6046719527906,20.2706794469754,123.252408259714)) ;
#35995=CARTESIAN_POINT('Ctrl Pts',(-20.9035264744634,20.0906903665656,123.212570178588)) ;
#35996=CARTESIAN_POINT('Ctrl Pts',(-20.6142327360248,20.2805298588107,123.459290301903)) ;
#35997=CARTESIAN_POINT('Ctrl Pts',(-20.9154749498567,20.1005407784008,123.471173528854)) ;
#35998=CARTESIAN_POINT('Ctrl Pts',(-20.5877918422668,20.2905570280966,123.668422397058)) ;
#35999=CARTESIAN_POINT('Ctrl Pts',(-20.8824212203994,20.1105679476868,123.7325883034)) ;
#36000=CARTESIAN_POINT('Ctrl Pts',(-20.5249072417576,20.3005845088108,123.869644711752)) ;
#36001=CARTESIAN_POINT('Ctrl Pts',(-20.803813048132,20.120595428401,123.984115444754)) ;
#36002=CARTESIAN_POINT('Ctrl Pts',(-20.4301831206918,20.3104275613901,124.053614638865)) ;
#36003=CARTESIAN_POINT('Ctrl Pts',(-20.6854052877138,20.1304384809802,124.214077225358)) ;
#36004=CARTESIAN_POINT('Ctrl Pts',(-20.3034580062551,20.3204214648287,124.221197227413)) ;
#36005=CARTESIAN_POINT('Ctrl Pts',(-20.5269966913831,20.1404323844189,124.423553915881)) ;
#36006=CARTESIAN_POINT('Ctrl Pts',(-20.1487806009657,20.3304485876051,124.364425720184)) ;
#36007=CARTESIAN_POINT('Ctrl Pts',(-20.3336481312911,20.1504595071953,124.602587618379)) ;
#36008=CARTESIAN_POINT('Ctrl Pts',(-19.9741372933805,20.3403392924971,124.477286085174)) ;
#36009=CARTESIAN_POINT('Ctrl Pts',(-20.1153421999281,20.1603502120873,124.743661057591)) ;
#36010=CARTESIAN_POINT('Ctrl Pts',(-19.7807153610016,20.3503313193475,124.559212631353)) ;
#36011=CARTESIAN_POINT('Ctrl Pts',(-19.8735636289023,20.1703422389376,124.846066786596)) ;
#36012=CARTESIAN_POINT('Ctrl Pts',(-19.5769304517105,20.360277300836,124.606034161387)) ;
#36013=CARTESIAN_POINT('Ctrl Pts',(-19.618831660726,20.1802882204262,124.904591118411)) ;
#36014=CARTESIAN_POINT('Ctrl Pts',(-19.3680954416651,20.3702244734579,124.617184177661)) ;
#36015=CARTESIAN_POINT('Ctrl Pts',(-19.3577875500311,20.1902353930481,124.918525903607)) ;
#36016=CARTESIAN_POINT('Ctrl Pts',(-19.1584407875054,20.3802724147841,124.591416106205)) ;
#36017=CARTESIAN_POINT('Ctrl Pts',(-19.095719576205,20.2002833343742,124.886313111821)) ;
#36018=CARTESIAN_POINT('Ctrl Pts',(-18.9604121411015,20.3901200485918,124.531032969309)) ;
#36019=CARTESIAN_POINT('Ctrl Pts',(-18.8481841830394,20.210130968182,124.810831448452)) ;
#36020=CARTESIAN_POINT('Ctrl Pts',(-18.7734517586268,20.4000817632769,124.436686230099)) ;
#36021=CARTESIAN_POINT('Ctrl Pts',(-18.6144848556616,20.2200926828671,124.692895466092)) ;
#36022=CARTESIAN_POINT('Ctrl Pts',(-18.604728389867,20.4101103961554,124.310240172556)) ;
#36023=CARTESIAN_POINT('Ctrl Pts',(-18.4035822759997,20.2301213157456,124.534835645164)) ;
#36024=CARTESIAN_POINT('Ctrl Pts',(-18.4621885899076,20.4200207216905,124.158296132863)) ;
#36025=CARTESIAN_POINT('Ctrl Pts',(-18.2254094105171,20.2400316412807,124.344903540078)) ;
#36026=CARTESIAN_POINT('Ctrl Pts',(-18.3474529168086,20.4299555521623,123.983766306947)) ;
#36027=CARTESIAN_POINT('Ctrl Pts',(-18.0819921053429,20.2499664717524,124.126739575405)) ;
#36028=CARTESIAN_POINT('Ctrl Pts',(-18.2640446601778,20.4399968845442,123.789842819283)) ;
#36029=CARTESIAN_POINT('Ctrl Pts',(-17.9777343204526,20.2600078041344,123.884334153657)) ;
#36030=CARTESIAN_POINT('Ctrl Pts',(-18.21621844815,20.4498897579831,123.587439108983)) ;
#36031=CARTESIAN_POINT('Ctrl Pts',(-17.9179543451556,20.2699006775733,123.631328380926)) ;
#36032=CARTESIAN_POINT('Ctrl Pts',(-18.203638204828,20.459858923801,123.378224162259)) ;
#36033=CARTESIAN_POINT('Ctrl Pts',(-17.9022315155995,20.2798698433911,123.369810686239)) ;
#36034=CARTESIAN_POINT('Ctrl Pts',(-18.2280625767773,20.4698876575175,123.168828358653)) ;
#36035=CARTESIAN_POINT('Ctrl Pts',(-17.9327660606948,20.2898985771077,123.108061591315)) ;
#36036=CARTESIAN_POINT('Ctrl Pts',(-18.3069889150334,20.4830801762886,122.902870280924)) ;
#36037=CARTESIAN_POINT('Ctrl Pts',(-18.0314212955399,20.3030910958788,122.775637805925)) ;
#36038=CARTESIAN_POINT('Ctrl Pts',(-18.4552942626579,20.4964400443313,122.660681326423)) ;
#36039=CARTESIAN_POINT('Ctrl Pts',(-18.2167817772331,20.3164509639215,122.472918789016)) ;
#36040=CARTESIAN_POINT('Ctrl Pts',(-18.657015951964,20.5096653814802,122.469309191778)) ;
#36041=CARTESIAN_POINT('Ctrl Pts',(-18.4689719566791,20.3296763010703,122.233665328746)) ;
#36042=CARTESIAN_POINT('Ctrl Pts',(-18.8316741273677,20.5196466073208,122.353005072726)) ;
#36043=CARTESIAN_POINT('Ctrl Pts',(-18.6872891439272,20.339657526911,122.088295732231)) ;
#36044=CARTESIAN_POINT('Ctrl Pts',(-19.0250769115555,20.5296821743037,122.268720045023)) ;
#36045=CARTESIAN_POINT('Ctrl Pts',(-18.9290457583326,20.3496930938939,121.982939786395)) ;
#36046=CARTESIAN_POINT('Ctrl Pts',(-19.2265825671295,20.5395452522658,122.219728041552)) ;
#36047=CARTESIAN_POINT('Ctrl Pts',(-19.1809279027558,20.3595561718559,121.921703115425)) ;
#36048=CARTESIAN_POINT('Ctrl Pts',(-19.4378331047405,20.5496155510669,122.206147359895)) ;
#36049=CARTESIAN_POINT('Ctrl Pts',(-19.4449915418414,20.369626470657,121.90472989406)) ;
#36050=CARTESIAN_POINT('Ctrl Pts',(-19.6434998813334,20.5594578496347,122.228940856017)) ;
#36051=CARTESIAN_POINT('Ctrl Pts',(-19.7020745055616,20.3794687692249,121.933224576269)) ;
#36052=CARTESIAN_POINT('Ctrl Pts',(-19.8446762990893,20.5694185478045,122.287051453372)) ;
#36053=CARTESIAN_POINT('Ctrl Pts',(-19.9535442297023,20.3894294673946,122.005865433009)) ;
#36054=CARTESIAN_POINT('Ctrl Pts',(-20.0339789138857,20.579456581984,122.380301038949)) ;
#36055=CARTESIAN_POINT('Ctrl Pts',(-20.1901714045635,20.3994675015741,122.122429978449)) ;
#36056=CARTESIAN_POINT('Ctrl Pts',(-20.2016869726508,20.5893303188304,122.50266789996)) ;
#36057=CARTESIAN_POINT('Ctrl Pts',(-20.3998046709524,20.4093412384206,122.275390622906)) ;
#36058=CARTESIAN_POINT('Ctrl Pts',(-20.3484287632797,20.5994021027557,122.65527287763)) ;
#36059=CARTESIAN_POINT('Ctrl Pts',(-20.5832300951719,20.4194130223459,122.466148916906)) ;
#36060=CARTESIAN_POINT('Ctrl Pts',(-20.4637684790007,20.6092342239569,122.82682741127)) ;
#36061=CARTESIAN_POINT('Ctrl Pts',(-20.7274022481796,20.429245143547,122.680593266566)) ;
#36062=CARTESIAN_POINT('Ctrl Pts',(-20.549786388294,20.6192672479823,123.019405571818)) ;
#36063=CARTESIAN_POINT('Ctrl Pts',(-20.8349222723643,20.4392781675725,122.921317142766)) ;
#36064=CARTESIAN_POINT('Ctrl Pts',(-20.600454739304,20.629283128179,123.223797814881)) ;
#36065=CARTESIAN_POINT('Ctrl Pts',(-20.8982551028601,20.4492940477692,123.176808341206)) ;
#36066=CARTESIAN_POINT('Ctrl Pts',(-20.6150583626326,20.6391666472732,123.431067002261)) ;
#36067=CARTESIAN_POINT('Ctrl Pts',(-20.9165069215873,20.4591775668633,123.435894221685)) ;
#36068=CARTESIAN_POINT('Ctrl Pts',(-20.5934884418527,20.6491570596368,123.639971139436)) ;
#36069=CARTESIAN_POINT('Ctrl Pts',(-20.8895420040993,20.469167979227,123.697025786591)) ;
#36070=CARTESIAN_POINT('Ctrl Pts',(-20.5172126026985,20.6624202228403,123.908195883155)) ;
#36071=CARTESIAN_POINT('Ctrl Pts',(-20.7941934592288,20.4824311424304,124.032297262021)) ;
#36072=CARTESIAN_POINT('Ctrl Pts',(-20.3727499039758,20.6756977930915,124.150760947289)) ;
#36073=CARTESIAN_POINT('Ctrl Pts',(-20.6136449750528,20.4957087126816,124.335469275546)) ;
#36074=CARTESIAN_POINT('Ctrl Pts',(-20.1718067412588,20.6890280955981,124.346077378148)) ;
#36075=CARTESIAN_POINT('Ctrl Pts',(-20.3624251620804,20.5090390151882,124.579659196416)) ;
#36076=CARTESIAN_POINT('Ctrl Pts',(-19.9998354457734,20.6989267774145,124.463273965374)) ;
#36077=CARTESIAN_POINT('Ctrl Pts',(-20.1474678125602,20.5189376970046,124.726143222235)) ;
#36078=CARTESIAN_POINT('Ctrl Pts',(-19.8085029004183,20.708916292462,124.549834225346)) ;
#36079=CARTESIAN_POINT('Ctrl Pts',(-19.9082988338511,20.5289272120522,124.834343756677)) ;
#36080=CARTESIAN_POINT('Ctrl Pts',(-19.6058699471084,20.718864344237,124.601638834298)) ;
#36081=CARTESIAN_POINT('Ctrl Pts',(-19.65500875944,20.5388752638272,124.899096739241)) ;
#36082=CARTESIAN_POINT('Ctrl Pts',(-19.3975069469639,20.7288057475155,124.617723893743)) ;
#36083=CARTESIAN_POINT('Ctrl Pts',(-19.3945515389807,20.5488166671057,124.91919968873)) ;
#36084=CARTESIAN_POINT('Ctrl Pts',(-19.1194310874959,20.7420924122965,124.5908661902)) ;
#36085=CARTESIAN_POINT('Ctrl Pts',(-19.0469745336925,20.5621033318866,124.885630332434)) ;
#36086=CARTESIAN_POINT('Ctrl Pts',(-18.7886547609525,20.7587028339513,124.467201444823)) ;
#36087=CARTESIAN_POINT('Ctrl Pts',(-18.6334863377583,20.5787137535414,124.731039345146)) ;
#36088=CARTESIAN_POINT('Ctrl Pts',(-18.4662665698674,20.7786140962021,124.192751228819)) ;
#36089=CARTESIAN_POINT('Ctrl Pts',(-18.2305106418052,20.5986250157922,124.387975748698)) ;
#36090=CARTESIAN_POINT('Ctrl Pts',(-18.2563995968813,20.7985582253669,123.82423191738)) ;
#36091=CARTESIAN_POINT('Ctrl Pts',(-17.9681790721331,20.6185691449571,123.927324296511)) ;
#36092=CARTESIAN_POINT('Ctrl Pts',(-18.1850241779996,20.8184813879721,123.406707624286)) ;
#36093=CARTESIAN_POINT('Ctrl Pts',(-17.8789643903476,20.6384923075623,123.405418987404)) ;
#36094=CARTESIAN_POINT('Ctrl Pts',(-18.2596109544151,20.8383715103787,122.990352378829)) ;
#36095=CARTESIAN_POINT('Ctrl Pts',(-17.9722011637848,20.6583824299688,122.884976490785)) ;
#36096=CARTESIAN_POINT('Ctrl Pts',(-18.4732404987063,20.8583764639788,122.622607393527)) ;
#36097=CARTESIAN_POINT('Ctrl Pts',(-18.2392413285388,20.678387383569,122.425297035584)) ;
#36098=CARTESIAN_POINT('Ctrl Pts',(-18.7967167999957,20.8782147209944,122.351758323974)) ;
#36099=CARTESIAN_POINT('Ctrl Pts',(-18.643587622069,20.6982256405846,122.086739272728)) ;
#36100=CARTESIAN_POINT('Ctrl Pts',(-19.1960471170997,20.8982090217809,122.206055805286)) ;
#36101=CARTESIAN_POINT('Ctrl Pts',(-19.1427514572013,20.7182199413711,121.90461393122)) ;
#36102=CARTESIAN_POINT('Ctrl Pts',(-19.6188717893715,20.9180942638254,122.205753928318)) ;
#36103=CARTESIAN_POINT('Ctrl Pts',(-19.6712810445399,20.7381051834155,121.90423957277)) ;
#36104=CARTESIAN_POINT('Ctrl Pts',(-20.0166066720332,20.9379692103013,122.348559948617)) ;
#36105=CARTESIAN_POINT('Ctrl Pts',(-20.1684474704946,20.7579801298915,122.082748587441)) ;
#36106=CARTESIAN_POINT('Ctrl Pts',(-20.3441382460836,20.9580022802424,122.620951616946)) ;
#36107=CARTESIAN_POINT('Ctrl Pts',(-20.5778609765498,20.7780131998326,122.423240113324)) ;
#36108=CARTESIAN_POINT('Ctrl Pts',(-20.5570102326951,20.9778907871428,122.986308371611)) ;
#36109=CARTESIAN_POINT('Ctrl Pts',(-20.8439482663196,20.797901706733,122.879935963117)) ;
#36110=CARTESIAN_POINT('Ctrl Pts',(-20.6337603887322,20.9977456469241,123.401507209435)) ;
#36111=CARTESIAN_POINT('Ctrl Pts',(-20.9398845190647,20.8177565665142,123.398932664503)) ;
#36112=CARTESIAN_POINT('Ctrl Pts',(-20.5628715307167,21.0177964807118,123.821804823539)) ;
#36113=CARTESIAN_POINT('Ctrl Pts',(-20.851271999308,20.837807400302,123.92430520719)) ;
#36114=CARTESIAN_POINT('Ctrl Pts',(-20.356096985501,21.037562422601,124.187831810963)) ;
#36115=CARTESIAN_POINT('Ctrl Pts',(-20.5928049105319,20.8575733421912,124.381835472943)) ;
#36116=CARTESIAN_POINT('Ctrl Pts',(-20.0335794669859,21.0575751540604,124.465226345288)) ;
#36117=CARTESIAN_POINT('Ctrl Pts',(-20.1896580437977,20.8775860736505,124.728578782412)) ;
#36118=CARTESIAN_POINT('Ctrl Pts',(-19.637720643514,21.0774679890039,124.614558860712)) ;
#36119=CARTESIAN_POINT('Ctrl Pts',(-19.6948360554423,20.8974789085941,124.91524382122)) ;
#36120=CARTESIAN_POINT('Ctrl Pts',(-19.214589507988,21.0973750123435,124.620545648609)) ;
#36121=CARTESIAN_POINT('Ctrl Pts',(-19.1659236264402,20.9173859319337,124.922728040003)) ;
#36122=CARTESIAN_POINT('Ctrl Pts',(-18.8142996405734,21.1172902772442,124.482107958723)) ;
#36123=CARTESIAN_POINT('Ctrl Pts',(-18.6655619226655,20.9373011968343,124.749682544209)) ;
#36124=CARTESIAN_POINT('Ctrl Pts',(-18.4838027384896,21.1373219694039,124.213487981599)) ;
#36125=CARTESIAN_POINT('Ctrl Pts',(-18.252439701957,20.9573328889941,124.413908184247)) ;
#36126=CARTESIAN_POINT('Ctrl Pts',(-18.2668088815555,21.1571650159769,123.851596586135)) ;
#36127=CARTESIAN_POINT('Ctrl Pts',(-17.9811972980463,20.9771759355671,123.961546540822)) ;
#36128=CARTESIAN_POINT('Ctrl Pts',(-18.1851023806558,21.1770815638767,123.436137199122)) ;
#36129=CARTESIAN_POINT('Ctrl Pts',(-17.8790621516015,20.9970924834669,123.442223784008)) ;
#36130=CARTESIAN_POINT('Ctrl Pts',(-18.2502145798426,21.197013806868,123.017317548737)) ;
#36131=CARTESIAN_POINT('Ctrl Pts',(-17.9604499278129,21.0170247264581,122.918699625123)) ;
#36132=CARTESIAN_POINT('Ctrl Pts',(-18.453820244144,21.2169176416773,122.646330539081)) ;
#36133=CARTESIAN_POINT('Ctrl Pts',(-18.2149540833388,21.0369285612675,122.454965536669)) ;
#36134=CARTESIAN_POINT('Ctrl Pts',(-18.771411200767,21.2368180418648,122.366728476114)) ;
#36135=CARTESIAN_POINT('Ctrl Pts',(-18.6119399165711,21.056828961455,122.105461255076)) ;
#36136=CARTESIAN_POINT('Ctrl Pts',(-19.1662802143597,21.2567677182441,122.211733257638)) ;
#36137=CARTESIAN_POINT('Ctrl Pts',(-19.1055245266933,21.0767786378343,121.911714229282)) ;
#36138=CARTESIAN_POINT('Ctrl Pts',(-19.5899666832492,21.2767002424645,122.200890341999)) ;
#36139=CARTESIAN_POINT('Ctrl Pts',(-19.6351319246328,21.0967111620546,121.898157077983)) ;
#36140=CARTESIAN_POINT('Ctrl Pts',(-19.9918071979918,21.2966202514507,122.334860446379)) ;
#36141=CARTESIAN_POINT('Ctrl Pts',(-20.1374331359612,21.1166311710408,122.065615887808)) ;
#36142=CARTESIAN_POINT('Ctrl Pts',(-20.3243261883736,21.3165771576268,122.598408286184)) ;
#36143=CARTESIAN_POINT('Ctrl Pts',(-20.5530840766553,21.136588077217,122.395047352142)) ;
#36144=CARTESIAN_POINT('Ctrl Pts',(-20.5465500206849,21.3364629971283,122.958223520543)) ;
#36145=CARTESIAN_POINT('Ctrl Pts',(-20.8308668600017,21.1564739167185,122.844813593055)) ;
#36146=CARTESIAN_POINT('Ctrl Pts',(-20.6329313729834,21.3564341692642,123.373889795751)) ;
#36147=CARTESIAN_POINT('Ctrl Pts',(-20.9388483134395,21.1764450888544,123.364394953385)) ;
#36148=CARTESIAN_POINT('Ctrl Pts',(-20.5733172895036,21.3762483662486,123.791020354018)) ;
#36149=CARTESIAN_POINT('Ctrl Pts',(-20.8643333248792,21.1962592858388,123.885809151941)) ;
#36150=CARTESIAN_POINT('Ctrl Pts',(-20.3738339937494,21.3962295522168,124.166047638378)) ;
#36151=CARTESIAN_POINT('Ctrl Pts',(-20.614991472528,21.216240471807,124.35458992432)) ;
#36152=CARTESIAN_POINT('Ctrl Pts',(-20.1119197884198,21.4128050576061,124.401919568806)) ;
#36153=CARTESIAN_POINT('Ctrl Pts',(-20.287577123205,21.2328159771962,124.649450004778)) ;
#36154=CARTESIAN_POINT('Ctrl Pts',(-19.8627851378671,21.4261145054697,124.529357888635)) ;
#36155=CARTESIAN_POINT('Ctrl Pts',(-19.9761906951506,21.2461254250599,124.808734121351)) ;
#36156=CARTESIAN_POINT('Ctrl Pts',(-19.5941578117551,21.4394822032463,124.611771760159)) ;
#36157=CARTESIAN_POINT('Ctrl Pts',(-19.6403422561872,21.2594931228365,124.911767929995)) ;
#36158=CARTESIAN_POINT('Ctrl Pts',(-19.2437108626746,21.4559727749122,124.6246956008)) ;
#36159=CARTESIAN_POINT('Ctrl Pts',(-19.2023540010319,21.2759836945023,124.927912591816)) ;
#36160=CARTESIAN_POINT('Ctrl Pts',(-18.8402511753296,21.475893047245,124.495996346843)) ;
#36161=CARTESIAN_POINT('Ctrl Pts',(-18.6980130161418,21.2959039668352,124.767055416111)) ;
#36162=CARTESIAN_POINT('Ctrl Pts',(-18.5605799960303,21.492510082966,124.28007609183)) ;
#36163=CARTESIAN_POINT('Ctrl Pts',(-18.3484015779362,21.3125210025561,124.497134075303)) ;
#36164=CARTESIAN_POINT('Ctrl Pts',(-18.3909714744252,21.5058009332471,124.057970104108)) ;
#36165=CARTESIAN_POINT('Ctrl Pts',(-18.1364098503335,21.3258118528373,124.219524949663)) ;
#36166=CARTESIAN_POINT('Ctrl Pts',(-18.2945586514006,21.5157699784016,123.871912739408)) ;
#36167=CARTESIAN_POINT('Ctrl Pts',(-18.015887138759,21.3357808979917,123.986950081611)) ;
#36168=CARTESIAN_POINT('Ctrl Pts',(-18.2319181244892,21.5256733690351,123.673331471138)) ;
#36169=CARTESIAN_POINT('Ctrl Pts',(-17.9375848219048,21.3456842886253,123.738726404517)) ;
#36170=CARTESIAN_POINT('Ctrl Pts',(-18.2044053248853,21.5357311551478,123.46370878248)) ;
#36171=CARTESIAN_POINT('Ctrl Pts',(-17.9031917372576,21.355742074738,123.47669498645)) ;
#36172=CARTESIAN_POINT('Ctrl Pts',(-18.213339943562,21.5455831917976,123.256751493961)) ;
#36173=CARTESIAN_POINT('Ctrl Pts',(-17.9143537184473,21.3655941113878,123.218009520756)) ;
#36174=CARTESIAN_POINT('Ctrl Pts',(-18.2735424653214,21.5589483159408,122.982353800711)) ;
#36175=CARTESIAN_POINT('Ctrl Pts',(-17.9896212280207,21.378959235531,122.874956967983)) ;
#36176=CARTESIAN_POINT('Ctrl Pts',(-18.4029674767116,21.5721743789038,122.732632420697)) ;
#36177=CARTESIAN_POINT('Ctrl Pts',(-18.1513956642549,21.392185298494,122.562838107793)) ;
#36178=CARTESIAN_POINT('Ctrl Pts',(-18.5911529593693,21.5854780271861,122.525730956398)) ;
#36179=CARTESIAN_POINT('Ctrl Pts',(-18.3866109363126,21.4054889467763,122.304222180904)) ;
#36180=CARTESIAN_POINT('Ctrl Pts',(-18.7572783870989,21.5954695583491,122.397143887496)) ;
#36181=CARTESIAN_POINT('Ctrl Pts',(-18.5942688365446,21.4154804779393,122.143483381853)) ;
#36182=CARTESIAN_POINT('Ctrl Pts',(-18.9441977840221,21.6055090061484,122.299154895599)) ;
#36183=CARTESIAN_POINT('Ctrl Pts',(-18.8279161165518,21.4255199257386,122.020995347781)) ;
#36184=CARTESIAN_POINT('Ctrl Pts',(-19.1413056725189,21.6153527816622,122.236053528025)) ;
#36185=CARTESIAN_POINT('Ctrl Pts',(-19.0743002770626,21.4353637012524,121.942115783789)) ;
#36186=CARTESIAN_POINT('Ctrl Pts',(-19.3492278326637,21.6253384230499,122.207322375982)) ;
#36187=CARTESIAN_POINT('Ctrl Pts',(-19.3342026170247,21.4453493426401,121.906199088032)) ;
#36188=CARTESIAN_POINT('Ctrl Pts',(-19.5580238062598,21.6352752074117,122.21497981521)) ;
#36189=CARTESIAN_POINT('Ctrl Pts',(-19.5951977714933,21.4552861270019,121.91576806339)) ;
#36190=CARTESIAN_POINT('Ctrl Pts',(-19.7645659584739,21.645325041879,122.259368244298)) ;
#36191=CARTESIAN_POINT('Ctrl Pts',(-19.8533761100118,21.4653359614692,121.971250859227)) ;
#36192=CARTESIAN_POINT('Ctrl Pts',(-19.9564732011589,21.6551754913822,122.337234509043)) ;
#36193=CARTESIAN_POINT('Ctrl Pts',(-20.0932613279301,21.4751864109724,122.068581121227)) ;
#36194=CARTESIAN_POINT('Ctrl Pts',(-20.1343652145138,21.6651475053643,122.448110905834)) ;
#36195=CARTESIAN_POINT('Ctrl Pts',(-20.3156279273217,21.4851584249544,122.207174295896)) ;
#36196=CARTESIAN_POINT('Ctrl Pts',(-20.2906914128935,21.6751426632114,122.588577277018)) ;
#36197=CARTESIAN_POINT('Ctrl Pts',(-20.5110376062556,21.4951535828016,122.382755229648)) ;
#36198=CARTESIAN_POINT('Ctrl Pts',(-20.4205236147211,21.6851765895751,122.754811362263)) ;
#36199=CARTESIAN_POINT('Ctrl Pts',(-20.6733301023757,21.5051875091653,122.590546133559)) ;
#36200=CARTESIAN_POINT('Ctrl Pts',(-20.5180643029118,21.6950322980075,122.937635457501)) ;
#36201=CARTESIAN_POINT('Ctrl Pts',(-20.7952585398595,21.5150432175976,122.819075138362)) ;
#36202=CARTESIAN_POINT('Ctrl Pts',(-20.5835791686227,21.7050304473461,123.137322140165)) ;
#36203=CARTESIAN_POINT('Ctrl Pts',(-20.8771547989075,21.5250413669363,123.068682710127)) ;
#36204=CARTESIAN_POINT('Ctrl Pts',(-20.6133259213828,21.7149298505197,123.343332794389)) ;
#36205=CARTESIAN_POINT('Ctrl Pts',(-20.9143410126889,21.5349407701099,123.326195883174)) ;
#36206=CARTESIAN_POINT('Ctrl Pts',(-20.6067986597741,21.7249810474082,123.554517472211)) ;
#36207=CARTESIAN_POINT('Ctrl Pts',(-20.9061847000465,21.5449919669983,123.590176807793)) ;
#36208=CARTESIAN_POINT('Ctrl Pts',(-20.5644486467122,21.734863371221,123.757928803125)) ;
#36209=CARTESIAN_POINT('Ctrl Pts',(-20.8532498235943,21.5548742908112,123.844441837928)) ;
#36210=CARTESIAN_POINT('Ctrl Pts',(-20.4869932248377,21.7448582668776,123.953249465948)) ;
#36211=CARTESIAN_POINT('Ctrl Pts',(-20.7564330307127,21.5648691864678,124.088593766692)) ;
#36212=CARTESIAN_POINT('Ctrl Pts',(-20.376239486151,21.7548793662602,124.132475484503)) ;
#36213=CARTESIAN_POINT('Ctrl Pts',(-20.6179931769502,21.5748902858503,124.312627761406)) ;
#36214=CARTESIAN_POINT('Ctrl Pts',(-20.2377724390061,21.7647866341222,124.288062190397)) ;
#36215=CARTESIAN_POINT('Ctrl Pts',(-20.4449112035146,21.5847975537124,124.507113190918)) ;
#36216=CARTESIAN_POINT('Ctrl Pts',(-20.0741502835799,21.7747249779475,124.417970243514)) ;
#36217=CARTESIAN_POINT('Ctrl Pts',(-20.2403849662949,21.5947358975377,124.669500522517)) ;
#36218=CARTESIAN_POINT('Ctrl Pts',(-19.8892850130631,21.784728397248,124.518280702167)) ;
#36219=CARTESIAN_POINT('Ctrl Pts',(-20.0093045735682,21.6047393168382,124.794890972802)) ;
#36220=CARTESIAN_POINT('Ctrl Pts',(-19.6891120590807,21.7947629479551,124.584833460336)) ;
#36221=CARTESIAN_POINT('Ctrl Pts',(-19.7590892507581,21.6147738675453,124.878084487148)) ;
#36222=CARTESIAN_POINT('Ctrl Pts',(-19.484395225653,21.8046078975607,124.615389634734)) ;
#36223=CARTESIAN_POINT('Ctrl Pts',(-19.5031930456701,21.6246188171509,124.916282417734)) ;
#36224=CARTESIAN_POINT('Ctrl Pts',(-19.2745575619711,21.8145937396736,124.610253310873)) ;
#36225=CARTESIAN_POINT('Ctrl Pts',(-19.2408957415277,21.6346046592638,124.909864611277)) ;
#36226=CARTESIAN_POINT('Ctrl Pts',(-19.0697507053397,21.8245285470427,124.569104542372)) ;
#36227=CARTESIAN_POINT('Ctrl Pts',(-18.9848863453613,21.6445394666328,124.858431106642)) ;
#36228=CARTESIAN_POINT('Ctrl Pts',(-18.8729297754626,21.834586088756,124.491928841901)) ;
#36229=CARTESIAN_POINT('Ctrl Pts',(-18.738859338047,21.6545970083461,124.761963952315)) ;
#36230=CARTESIAN_POINT('Ctrl Pts',(-18.6965214907536,21.8444076862681,124.384579575107)) ;
#36231=CARTESIAN_POINT('Ctrl Pts',(-18.5183469904229,21.6644186058583,124.62777914016)) ;
#36232=CARTESIAN_POINT('Ctrl Pts',(-18.5374995717357,21.8544639457486,124.245294446865)) ;
#36233=CARTESIAN_POINT('Ctrl Pts',(-18.3195680415118,21.6744748653387,124.453674665884)) ;
#36234=CARTESIAN_POINT('Ctrl Pts',(-18.4068771812102,21.864403882049,124.082167341671)) ;
#36235=CARTESIAN_POINT('Ctrl Pts',(-18.156287854602,21.6844148016391,124.249767117472)) ;
#36236=CARTESIAN_POINT('Ctrl Pts',(-18.3063513222259,21.8743110027934,123.899756894152)) ;
#36237=CARTESIAN_POINT('Ctrl Pts',(-18.0306281551785,21.6943219223836,124.02175476564)) ;
#36238=CARTESIAN_POINT('Ctrl Pts',(-18.2381764644266,21.8843539087187,123.699938324222)) ;
#36239=CARTESIAN_POINT('Ctrl Pts',(-17.9454073047727,21.7043648283088,123.771982422698)) ;
#36240=CARTESIAN_POINT('Ctrl Pts',(-18.2061259507257,21.8942616898179,123.494118034549)) ;
#36241=CARTESIAN_POINT('Ctrl Pts',(-17.9053416811519,21.714272609408,123.514706921446)) ;
#36242=CARTESIAN_POINT('Ctrl Pts',(-18.2099726092004,21.9042720588203,123.283696769241)) ;
#36243=CARTESIAN_POINT('Ctrl Pts',(-17.9101476584396,21.7242829784104,123.251680239074)) ;
#36244=CARTESIAN_POINT('Ctrl Pts',(-18.250799150117,21.9143028973891,123.076808306462)) ;
#36245=CARTESIAN_POINT('Ctrl Pts',(-17.9611784249109,21.7343138169792,122.993069232997)) ;
#36246=CARTESIAN_POINT('Ctrl Pts',(-18.3252324167252,21.9241557370288,122.88350173726)) ;
#36247=CARTESIAN_POINT('Ctrl Pts',(-18.0542181018734,21.7441666566189,122.751434398964)) ;
#36248=CARTESIAN_POINT('Ctrl Pts',(-18.4332250657028,21.9341437381937,122.703441071799)) ;
#36249=CARTESIAN_POINT('Ctrl Pts',(-18.189207059747,21.7541546577839,122.526357242262)) ;
#36250=CARTESIAN_POINT('Ctrl Pts',(-18.5700375225545,21.9440725571729,122.545786789656)) ;
#36251=CARTESIAN_POINT('Ctrl Pts',(-18.3602212352636,21.7640834767631,122.329287537154)) ;
#36252=CARTESIAN_POINT('Ctrl Pts',(-18.732888520769,21.9540602598952,122.413224493809)) ;
#36253=CARTESIAN_POINT('Ctrl Pts',(-18.5637837492415,21.7740711794854,122.16358286203)) ;
#36254=CARTESIAN_POINT('Ctrl Pts',(-18.9173249515201,21.9640962596979,122.31077716545)) ;
#36255=CARTESIAN_POINT('Ctrl Pts',(-18.7943281091717,21.7841071792881,122.035521757749)) ;
#36256=CARTESIAN_POINT('Ctrl Pts',(-19.1130605451374,21.9739511294993,122.242820238378)) ;
#36257=CARTESIAN_POINT('Ctrl Pts',(-19.0389977515647,21.7939620490895,121.950573238967)) ;
#36258=CARTESIAN_POINT('Ctrl Pts',(-19.3205261715052,21.9839505599228,122.209124296924)) ;
#36259=CARTESIAN_POINT('Ctrl Pts',(-19.298329579095,21.803961479513,121.908451210336)) ;
#36260=CARTESIAN_POINT('Ctrl Pts',(-19.5285708919945,21.9938456773881,122.211711498228)) ;
#36261=CARTESIAN_POINT('Ctrl Pts',(-19.5583862374027,21.8138565969783,121.911683181333)) ;
#36262=CARTESIAN_POINT('Ctrl Pts',(-19.7363587174108,22.0039061709051,122.251037909545)) ;
#36263=CARTESIAN_POINT('Ctrl Pts',(-19.8181211650705,21.8239170904953,121.960839136464)) ;
#36264=CARTESIAN_POINT('Ctrl Pts',(-19.9300913010617,22.0137556511063,122.324185172849)) ;
#36265=CARTESIAN_POINT('Ctrl Pts',(-20.0602885784537,21.8337665706965,122.052271697225)) ;
#36266=CARTESIAN_POINT('Ctrl Pts',(-20.1116425157324,22.0237821013701,122.431281071649)) ;
#36267=CARTESIAN_POINT('Ctrl Pts',(-20.2872285090302,21.8437930209603,122.18613995206)) ;
#36268=CARTESIAN_POINT('Ctrl Pts',(-20.2715450400608,22.0338133918482,122.568785511319)) ;
#36269=CARTESIAN_POINT('Ctrl Pts',(-20.4871079315914,21.8538243114383,122.358018915005)) ;
#36270=CARTESIAN_POINT('Ctrl Pts',(-20.4029602797824,22.0436547795,122.728588268752)) ;
#36271=CARTESIAN_POINT('Ctrl Pts',(-20.65137916474,21.8636656990902,122.557772038518)) ;
#36272=CARTESIAN_POINT('Ctrl Pts',(-20.5066507219347,22.0536581803912,122.911527607421)) ;
#36273=CARTESIAN_POINT('Ctrl Pts',(-20.7809938112544,21.8736690999814,122.786445434029)) ;
#36274=CARTESIAN_POINT('Ctrl Pts',(-20.5768052643418,22.0636425631824,123.109399042822)) ;
#36275=CARTESIAN_POINT('Ctrl Pts',(-20.8686887483968,21.8836534827725,123.033784325638)) ;
#36276=CARTESIAN_POINT('Ctrl Pts',(-20.6115199861339,22.0736816531958,123.317556791633)) ;
#36277=CARTESIAN_POINT('Ctrl Pts',(-20.9120839655967,21.8936925727859,123.293981073997)) ;
#36278=CARTESIAN_POINT('Ctrl Pts',(-20.6098913500393,22.0835274621049,123.524555130428)) ;
#36279=CARTESIAN_POINT('Ctrl Pts',(-20.9100499299617,21.9035383816951,123.552730180822)) ;
#36280=CARTESIAN_POINT('Ctrl Pts',(-20.5722452970051,22.0935118849239,123.731024894997)) ;
#36281=CARTESIAN_POINT('Ctrl Pts',(-20.8629939223635,21.9135228045141,123.810817924697)) ;
#36282=CARTESIAN_POINT('Ctrl Pts',(-20.4997117600218,22.1034515101651,123.927025671405)) ;
#36283=CARTESIAN_POINT('Ctrl Pts',(-20.7723283117608,21.9234624297553,124.055819959663)) ;
#36284=CARTESIAN_POINT('Ctrl Pts',(-20.3931662714284,22.1134911996838,124.109206689079)) ;
#36285=CARTESIAN_POINT('Ctrl Pts',(-20.63914792108,21.933502119274,124.283546922081)) ;
#36286=CARTESIAN_POINT('Ctrl Pts',(-20.2587285375417,22.1233793881024,124.267780927574)) ;
#36287=CARTESIAN_POINT('Ctrl Pts',(-20.4711013651506,21.9433903076926,124.48176644605)) ;
#36288=CARTESIAN_POINT('Ctrl Pts',(-20.0974265999504,22.1333689141044,124.402255862019)) ;
#36289=CARTESIAN_POINT('Ctrl Pts',(-20.269474706559,21.9533798336946,124.649861364024)) ;
#36290=CARTESIAN_POINT('Ctrl Pts',(-19.9157102403435,22.1433274154596,124.506217438115)) ;
#36291=CARTESIAN_POINT('Ctrl Pts',(-20.0423296293175,21.9633383350498,124.779814856074)) ;
#36292=CARTESIAN_POINT('Ctrl Pts',(-19.7200260725257,22.1532270094633,124.577119056446)) ;
#36293=CARTESIAN_POINT('Ctrl Pts',(-19.7977240449939,21.9732379290534,124.868443422862)) ;
#36294=CARTESIAN_POINT('Ctrl Pts',(-19.5119529377031,22.1632748975846,124.61342395275)) ;
#36295=CARTESIAN_POINT('Ctrl Pts',(-19.5376330731209,21.9832858171747,124.913825837569)) ;
#36296=CARTESIAN_POINT('Ctrl Pts',(-19.3038874510347,22.1731703228301,124.613217769104)) ;
#36297=CARTESIAN_POINT('Ctrl Pts',(-19.2775503015468,21.9931812424203,124.913569399203)) ;
#36298=CARTESIAN_POINT('Ctrl Pts',(-19.0956337768571,22.1832317135307,124.576318144067)) ;
#36299=CARTESIAN_POINT('Ctrl Pts',(-19.0172333059116,22.0032426331209,124.867446190306)) ;
#36300=CARTESIAN_POINT('Ctrl Pts',(-18.9011658613922,22.1930772972174,124.505398277424)) ;
#36301=CARTESIAN_POINT('Ctrl Pts',(-18.7741467328154,22.0130882168075,124.778797095508)) ;
#36302=CARTESIAN_POINT('Ctrl Pts',(-18.7194990589113,22.2030402705266,124.401179624215)) ;
#36303=CARTESIAN_POINT('Ctrl Pts',(-18.5470623485629,22.0230511901167,124.648524437501)) ;
#36304=CARTESIAN_POINT('Ctrl Pts',(-18.5578335683124,22.2130659373523,124.265923043721)) ;
#36305=CARTESIAN_POINT('Ctrl Pts',(-18.3449798305137,22.0330768569425,124.47945461935)) ;
#36306=CARTESIAN_POINT('Ctrl Pts',(-18.4235409053948,22.2229804152186,124.106527257626)) ;
#36307=CARTESIAN_POINT('Ctrl Pts',(-18.177112665249,22.0429913348088,124.280209964975)) ;
#36308=CARTESIAN_POINT('Ctrl Pts',(-18.3178094286118,22.2329689298936,123.925078039381)) ;
#36309=CARTESIAN_POINT('Ctrl Pts',(-18.0449474119097,22.0529798494838,124.05339871137)) ;
#36310=CARTESIAN_POINT('Ctrl Pts',(-18.2452217442394,22.2430130408091,123.726808026642)) ;
#36311=CARTESIAN_POINT('Ctrl Pts',(-17.9542118486561,22.0630239603992,123.805561752145)) ;
#36312=CARTESIAN_POINT('Ctrl Pts',(-18.2084565806548,22.2528411784036,123.523457249866)) ;
#36313=CARTESIAN_POINT('Ctrl Pts',(-17.9082542484671,22.0728520979938,123.551371969029)) ;
#36314=CARTESIAN_POINT('Ctrl Pts',(-18.2074383421507,22.2629177464626,123.311661356134)) ;
#36315=CARTESIAN_POINT('Ctrl Pts',(-17.9069805911585,22.0829286660527,123.286627562754)) ;
#36316=CARTESIAN_POINT('Ctrl Pts',(-18.2423241793869,22.2727699083667,123.107451203336)) ;
#36317=CARTESIAN_POINT('Ctrl Pts',(-17.9505873021255,22.0927808279569,123.031363437646)) ;
#36318=CARTESIAN_POINT('Ctrl Pts',(-18.3135102543039,22.2828428703236,122.908047647564)) ;
#36319=CARTESIAN_POINT('Ctrl Pts',(-18.0395690379803,22.1028537899137,122.782109150531)) ;
#36320=CARTESIAN_POINT('Ctrl Pts',(-18.4158946807527,22.2926854323265,122.728210968454)) ;
#36321=CARTESIAN_POINT('Ctrl Pts',(-18.1675496052285,22.1126963519166,122.557311692055)) ;
#36322=CARTESIAN_POINT('Ctrl Pts',(-18.549238880053,22.3026658688203,122.566223969324)) ;
#36323=CARTESIAN_POINT('Ctrl Pts',(-18.3342296704848,22.1226767884104,122.354827390297)) ;
#36324=CARTESIAN_POINT('Ctrl Pts',(-18.7095577945463,22.3126841741447,122.429637874185)) ;
#36325=CARTESIAN_POINT('Ctrl Pts',(-18.5346278830322,22.1326950937348,122.184094280937)) ;
#36326=CARTESIAN_POINT('Ctrl Pts',(-18.8885239198384,22.3225681380641,122.324009756949)) ;
#36327=CARTESIAN_POINT('Ctrl Pts',(-18.7583362356208,22.1425790576543,122.052058163441)) ;
#36328=CARTESIAN_POINT('Ctrl Pts',(-19.0866690738758,22.3326340148027,122.249785568809)) ;
#36329=CARTESIAN_POINT('Ctrl Pts',(-19.0060171333041,22.1526449343928,121.959277593411)) ;
#36330=CARTESIAN_POINT('Ctrl Pts',(-19.2900221608687,22.3424731156636,122.211822747741)) ;
#36331=CARTESIAN_POINT('Ctrl Pts',(-19.2602098520489,22.1624840352537,121.911823353311)) ;
#36332=CARTESIAN_POINT('Ctrl Pts',(-19.5009224073841,22.3525061985293,122.209172430537)) ;
#36333=CARTESIAN_POINT('Ctrl Pts',(-19.5238350449233,22.1725171181195,121.908510218205)) ;
#36334=CARTESIAN_POINT('Ctrl Pts',(-19.7087834710141,22.3625278838048,122.243664453097)) ;
#36335=CARTESIAN_POINT('Ctrl Pts',(-19.7836614016693,22.1825388033949,121.951624796593)) ;
#36336=CARTESIAN_POINT('Ctrl Pts',(-19.9045062463924,22.3723945789033,122.312314874088)) ;
#36337=CARTESIAN_POINT('Ctrl Pts',(-20.0283161574621,22.1924054984934,122.03743793613)) ;
#36338=CARTESIAN_POINT('Ctrl Pts',(-20.0873367852254,22.3823544686378,122.414394213939)) ;
#36339=CARTESIAN_POINT('Ctrl Pts',(-20.2568547841088,22.202365388228,122.165037255686)) ;
#36340=CARTESIAN_POINT('Ctrl Pts',(-20.2506677841391,22.3923894564633,122.547902606798)) ;
#36341=CARTESIAN_POINT('Ctrl Pts',(-20.4610185639065,22.2124003760535,122.331922477381)) ;
#36342=CARTESIAN_POINT('Ctrl Pts',(-20.3865916163423,22.4022761605376,122.705186554573)) ;
#36343=CARTESIAN_POINT('Ctrl Pts',(-20.6309241389178,22.2222870801277,122.528528183471)) ;
#36344=CARTESIAN_POINT('Ctrl Pts',(-20.4949858769458,22.4123413047705,122.886876646557)) ;
#36345=CARTESIAN_POINT('Ctrl Pts',(-20.7664168563428,22.2323522243607,122.755640405129)) ;
#36346=CARTESIAN_POINT('Ctrl Pts',(-20.5687197159867,22.422180595499,123.080175375466)) ;
#36347=CARTESIAN_POINT('Ctrl Pts',(-20.8585847062321,22.2421915150892,122.99726519042)) ;
#36348=CARTESIAN_POINT('Ctrl Pts',(-20.6089305970685,22.4322431529375,123.287840199753)) ;
#36349=CARTESIAN_POINT('Ctrl Pts',(-20.9088481490265,22.2522540725277,123.256845872691)) ;
#36350=CARTESIAN_POINT('Ctrl Pts',(-20.6121922591228,22.4421402041896,123.495893346216)) ;
#36351=CARTESIAN_POINT('Ctrl Pts',(-20.9129252441813,22.2621511237797,123.516913308376)) ;
#36352=CARTESIAN_POINT('Ctrl Pts',(-20.5798565032163,22.4520714109378,123.702154164007)) ;
#36353=CARTESIAN_POINT('Ctrl Pts',(-20.8725051637959,22.272082330528,123.774739999832)) ;
#36354=CARTESIAN_POINT('Ctrl Pts',(-20.5112221625243,22.4621135951567,123.901801813168)) ;
#36355=CARTESIAN_POINT('Ctrl Pts',(-20.7867121317539,22.2821245147468,124.024299304351)) ;
#36356=CARTESIAN_POINT('Ctrl Pts',(-20.4106758088328,22.4720002232676,124.083722626987)) ;
#36357=CARTESIAN_POINT('Ctrl Pts',(-20.6610284500668,22.2920111428578,124.251701155103)) ;
#36358=CARTESIAN_POINT('Ctrl Pts',(-20.278945382695,22.4819934958,124.2473690502)) ;
#36359=CARTESIAN_POINT('Ctrl Pts',(-20.4963649928886,22.3020044153902,124.456259102505)) ;
#36360=CARTESIAN_POINT('Ctrl Pts',(-20.1215083587096,22.4919385713414,124.384944915974)) ;
#36361=CARTESIAN_POINT('Ctrl Pts',(-20.2995680280864,22.3119494909316,124.628229064156)) ;
#36362=CARTESIAN_POINT('Ctrl Pts',(-19.9426983959548,22.5018881220697,124.493496277981)) ;
#36363=CARTESIAN_POINT('Ctrl Pts',(-20.0760548365221,22.3218990416599,124.763918115398)) ;
#36364=CARTESIAN_POINT('Ctrl Pts',(-19.7459427076918,22.5119274569177,124.569841858884)) ;
#36365=CARTESIAN_POINT('Ctrl Pts',(-19.8301102215501,22.3319383765079,124.859349625997)) ;
#36366=CARTESIAN_POINT('Ctrl Pts',(-19.5420901927288,22.5218135958616,124.610431047829)) ;
#36367=CARTESIAN_POINT('Ctrl Pts',(-19.5752934234481,22.3418245154518,124.910085821223)) ;
#36368=CARTESIAN_POINT('Ctrl Pts',(-19.331980404051,22.5318117088353,124.615326987992)) ;
#36369=CARTESIAN_POINT('Ctrl Pts',(-19.3126560173054,22.3518226284255,124.916205138693)) ;
#36370=CARTESIAN_POINT('Ctrl Pts',(-19.1257731714612,22.5417314711877,124.584031987848)) ;
#36371=CARTESIAN_POINT('Ctrl Pts',(-19.0548963058817,22.3617423907779,124.877085616193)) ;
#36372=CARTESIAN_POINT('Ctrl Pts',(-18.925760197074,22.5517708668004,124.51667777525)) ;
#36373=CARTESIAN_POINT('Ctrl Pts',(-18.8048804750503,22.3717817863906,124.792892259327)) ;
#36374=CARTESIAN_POINT('Ctrl Pts',(-18.7429037014523,22.5616800525887,124.416866967638)) ;
#36375=CARTESIAN_POINT('Ctrl Pts',(-18.5763093839728,22.3816909721789,124.668127742405)) ;
#36376=CARTESIAN_POINT('Ctrl Pts',(-18.579362600272,22.5716152367462,124.286939430316)) ;
#36377=CARTESIAN_POINT('Ctrl Pts',(-18.3718830460243,22.3916261563363,124.50571721687)) ;
#36378=CARTESIAN_POINT('Ctrl Pts',(-18.4395493540934,22.5816562941321,124.128790649976)) ;
#36379=CARTESIAN_POINT('Ctrl Pts',(-18.19711721559,22.4016672137223,124.308030847495)) ;
#36380=CARTESIAN_POINT('Ctrl Pts',(-18.3308735820911,22.5915434521654,123.951591507098)) ;
#36381=CARTESIAN_POINT('Ctrl Pts',(-18.0612726926849,22.4115543717555,124.086530580813)) ;
#36382=CARTESIAN_POINT('Ctrl Pts',(-18.253489695394,22.6015357318413,123.756310473585)) ;
#36383=CARTESIAN_POINT('Ctrl Pts',(-17.964543684815,22.4215466514315,123.84242873292)) ;
#36384=CARTESIAN_POINT('Ctrl Pts',(-18.2114252982926,22.6114842488863,123.551423040072)) ;
#36385=CARTESIAN_POINT('Ctrl Pts',(-17.9119640314251,22.4314951684765,123.58631871419)) ;
#36386=CARTESIAN_POINT('Ctrl Pts',(-18.2052879099196,22.6214210264567,123.342628586766)) ;
#36387=CARTESIAN_POINT('Ctrl Pts',(-17.9042933597284,22.4414319460469,123.325324977712)) ;
#36388=CARTESIAN_POINT('Ctrl Pts',(-18.2353818524349,22.6314040626037,123.134895795784)) ;
#36389=CARTESIAN_POINT('Ctrl Pts',(-17.9419119920146,22.4514149821938,123.065658904075)) ;
#36390=CARTESIAN_POINT('Ctrl Pts',(-18.3018390798526,22.6414478141974,122.934500268376)) ;
#36391=CARTESIAN_POINT('Ctrl Pts',(-18.0249844509372,22.4614587337876,122.815165001318)) ;
#36392=CARTESIAN_POINT('Ctrl Pts',(-18.3995334670519,22.65127634341,122.752393803793)) ;
#36393=CARTESIAN_POINT('Ctrl Pts',(-18.1471041894018,22.4712872630001,122.587531223325)) ;
#36394=CARTESIAN_POINT('Ctrl Pts',(-18.5304390769983,22.6613517043187,122.585924560108)) ;
#36395=CARTESIAN_POINT('Ctrl Pts',(-18.3107369255047,22.4813626239088,122.379445782513)) ;
#36396=CARTESIAN_POINT('Ctrl Pts',(-18.6848484847896,22.6712083032059,122.447668513297)) ;
#36397=CARTESIAN_POINT('Ctrl Pts',(-18.5037504475516,22.491219222796,122.206625869237)) ;
#36398=CARTESIAN_POINT('Ctrl Pts',(-18.8644168488015,22.6812712972238,122.335891874011)) ;
#36399=CARTESIAN_POINT('Ctrl Pts',(-18.7282113464364,22.5012822168139,122.066906399774)) ;
#36400=CARTESIAN_POINT('Ctrl Pts',(-19.0571331275604,22.6911492315132,122.25842835509)) ;
#36401=CARTESIAN_POINT('Ctrl Pts',(-18.9691081441107,22.5111601511034,121.97007787481)) ;
#36402=CARTESIAN_POINT('Ctrl Pts',(-19.2627566660564,22.7011498790713,122.214769477626)) ;
#36403=CARTESIAN_POINT('Ctrl Pts',(-19.2261379991783,22.5211607986615,121.915505689018)) ;
#36404=CARTESIAN_POINT('Ctrl Pts',(-19.4711669419206,22.7110677255094,122.207377365738)) ;
#36405=CARTESIAN_POINT('Ctrl Pts',(-19.486651608723,22.5310786450995,121.906267040759)) ;
#36406=CARTESIAN_POINT('Ctrl Pts',(-19.6803914078797,22.721118842515,122.236721719079)) ;
#36407=CARTESIAN_POINT('Ctrl Pts',(-19.7481817747925,22.5411297621052,121.942948938025)) ;
#36408=CARTESIAN_POINT('Ctrl Pts',(-19.8778768048327,22.7309895778256,122.300577463833)) ;
#36409=CARTESIAN_POINT('Ctrl Pts',(-19.9950390178961,22.5510004974158,122.022770439516)) ;
#36410=CARTESIAN_POINT('Ctrl Pts',(-20.0649458105329,22.7410602850686,122.39964958428)) ;
#36411=CARTESIAN_POINT('Ctrl Pts',(-20.228874215615,22.5610712046588,122.146611832899)) ;
#36412=CARTESIAN_POINT('Ctrl Pts',(-20.2281280729297,22.7508932925205,122.526586135203)) ;
#36413=CARTESIAN_POINT('Ctrl Pts',(-20.4328520597014,22.5709042121106,122.305284591609)) ;
#36414=CARTESIAN_POINT('Ctrl Pts',(-20.3700041193385,22.7609237848228,122.682583660361)) ;
#36415=CARTESIAN_POINT('Ctrl Pts',(-20.6101957114901,22.5809347044129,122.500282658212)) ;
#36416=CARTESIAN_POINT('Ctrl Pts',(-20.4821412733727,22.7709553798962,122.861209839806)) ;
#36417=CARTESIAN_POINT('Ctrl Pts',(-20.7503657378208,22.5909662994864,122.723566173328)) ;
#36418=CARTESIAN_POINT('Ctrl Pts',(-20.5603509074772,22.7807850790344,123.052474175343)) ;
#36419=CARTESIAN_POINT('Ctrl Pts',(-20.8481266307931,22.6007959986246,122.962648437227)) ;
#36420=CARTESIAN_POINT('Ctrl Pts',(-20.6054919636736,22.790774528916,123.257581426922)) ;
#36421=CARTESIAN_POINT('Ctrl Pts',(-20.904551077319,22.6107854485062,123.219033095619)) ;
#36422=CARTESIAN_POINT('Ctrl Pts',(-20.6138461179592,22.8008183867317,123.468567262756)) ;
#36423=CARTESIAN_POINT('Ctrl Pts',(-20.9149919746833,22.6208293063218,123.482765312891)) ;
#36424=CARTESIAN_POINT('Ctrl Pts',(-20.5864922399839,22.8106400773219,123.673230555573)) ;
#36425=CARTESIAN_POINT('Ctrl Pts',(-20.8807975539066,22.6306509969121,123.738595413786)) ;
#36426=CARTESIAN_POINT('Ctrl Pts',(-20.5231490604348,22.8206751678623,123.874462180045)) ;
#36427=CARTESIAN_POINT('Ctrl Pts',(-20.80161663366,22.6406860874524,123.990134218066)) ;
#36428=CARTESIAN_POINT('Ctrl Pts',(-20.4254247657349,22.830699686845,124.061198211658)) ;
#36429=CARTESIAN_POINT('Ctrl Pts',(-20.6794595799392,22.6507106064352,124.22355335811)) ;
#36430=CARTESIAN_POINT('Ctrl Pts',(-20.2991731667971,22.8405595322552,124.225579994862)) ;
#36431=CARTESIAN_POINT('Ctrl Pts',(-20.5216428900064,22.6605704518454,124.429030130097)) ;
#36432=CARTESIAN_POINT('Ctrl Pts',(-20.1451242577046,22.8505193085708,124.367400091411)) ;
#36433=CARTESIAN_POINT('Ctrl Pts',(-20.3290800370849,22.670530228161,124.606303874625)) ;
#36434=CARTESIAN_POINT('Ctrl Pts',(-19.9674278032907,22.8605475058855,124.480844125221)) ;
#36435=CARTESIAN_POINT('Ctrl Pts',(-20.1069583811312,22.6805584254756,124.748107125951)) ;
#36436=CARTESIAN_POINT('Ctrl Pts',(-19.7751521418593,22.8704550481758,124.56097363697)) ;
#36437=CARTESIAN_POINT('Ctrl Pts',(-19.8666123895731,22.690465967766,124.848267265669)) ;
#36438=CARTESIAN_POINT('Ctrl Pts',(-19.5693646949917,22.8804876987396,124.607138562997)) ;
#36439=CARTESIAN_POINT('Ctrl Pts',(-19.6093776535682,22.7004986183298,124.905971285035)) ;
#36440=CARTESIAN_POINT('Ctrl Pts',(-19.3617911177059,22.8903716551663,124.616789062193)) ;
#36441=CARTESIAN_POINT('Ctrl Pts',(-19.3499098381939,22.7103825747565,124.918032249286)) ;
#36442=CARTESIAN_POINT('Ctrl Pts',(-19.1534263144048,22.9003613565281,124.590486564837)) ;
#36443=CARTESIAN_POINT('Ctrl Pts',(-19.0894539707891,22.7203722761183,124.885151798247)) ;
#36444=CARTESIAN_POINT('Ctrl Pts',(-18.9518995245256,22.9104023518042,124.527657154102)) ;
#36445=CARTESIAN_POINT('Ctrl Pts',(-18.8375462306779,22.7304132713943,124.806612946829)) ;
#36446=CARTESIAN_POINT('Ctrl Pts',(-18.768077928406,22.9202352410725,124.433102961583)) ;
#36447=CARTESIAN_POINT('Ctrl Pts',(-18.6077694356937,22.7402461606627,124.688417721226)) ;
#36448=CARTESIAN_POINT('Ctrl Pts',(-18.6004184578311,22.93022839944,124.306510185862)) ;
#36449=CARTESIAN_POINT('Ctrl Pts',(-18.398196469038,22.7502393190301,124.530174726627)) ;
#36450=CARTESIAN_POINT('Ctrl Pts',(-18.4570423276391,22.9402604417921,124.151821923113)) ;
#36451=CARTESIAN_POINT('Ctrl Pts',(-18.2189780473495,22.7602713613823,124.336812835457)) ;
#36452=CARTESIAN_POINT('Ctrl Pts',(-18.3444002375447,22.9501256857505,123.977691444909)) ;
#36453=CARTESIAN_POINT('Ctrl Pts',(-18.0781770519716,22.7701366053407,124.119147819027)) ;
#36454=CARTESIAN_POINT('Ctrl Pts',(-18.2623606113742,22.9600875769965,123.78499218241)) ;
#36455=CARTESIAN_POINT('Ctrl Pts',(-17.9756297430065,22.7800984965867,123.878272519258)) ;
#36456=CARTESIAN_POINT('Ctrl Pts',(-18.2150170839736,22.970122477015,123.579418516963)) ;
#36457=CARTESIAN_POINT('Ctrl Pts',(-17.9164527323649,22.7901333966051,123.621304920699)) ;
#36458=CARTESIAN_POINT('Ctrl Pts',(-18.2039051887294,22.9800075574296,123.371873650446)) ;
#36459=CARTESIAN_POINT('Ctrl Pts',(-17.9025653495676,22.8000184770197,123.361873137657)) ;
#36460=CARTESIAN_POINT('Ctrl Pts',(-18.2294709369507,22.9900727295544,123.161850154122)) ;
#36461=CARTESIAN_POINT('Ctrl Pts',(-17.9345250196127,22.8100836491446,123.099344214686)) ;
#36462=CARTESIAN_POINT('Ctrl Pts',(-18.2896793781521,22.9999199642779,122.963757686704)) ;
#36463=CARTESIAN_POINT('Ctrl Pts',(-18.0097882000835,22.8199308838681,122.851728714275)) ;
#36464=CARTESIAN_POINT('Ctrl Pts',(-18.3846575460078,23.0099507755956,122.775493829682)) ;
#36465=CARTESIAN_POINT('Ctrl Pts',(-18.1285132436954,22.8299616951858,122.616400101457)) ;
#36466=CARTESIAN_POINT('Ctrl Pts',(-18.5109834152174,23.0199603915091,122.607165887845)) ;
#36467=CARTESIAN_POINT('Ctrl Pts',(-18.2864226562606,22.8399713110993,122.405991657267)) ;
#36468=CARTESIAN_POINT('Ctrl Pts',(-18.6629287718639,23.0298711709128,122.464629523893)) ;
#36469=CARTESIAN_POINT('Ctrl Pts',(-18.4763564295157,22.849882090503,122.227822802707)) ;
#36470=CARTESIAN_POINT('Ctrl Pts',(-18.8373784129168,23.0398004367019,122.349974057845)) ;
#36471=CARTESIAN_POINT('Ctrl Pts',(-18.6944202111385,22.859811356292,122.084505529284)) ;
#36472=CARTESIAN_POINT('Ctrl Pts',(-19.0313295538799,23.0498431300145,122.266578270263)) ;
#36473=CARTESIAN_POINT('Ctrl Pts',(-18.9368601501054,22.8698540496047,121.980263237203)) ;
#36474=CARTESIAN_POINT('Ctrl Pts',(-19.2336083459502,23.0597296627092,122.218742068884)) ;
#36475=CARTESIAN_POINT('Ctrl Pts',(-19.1897096706309,22.8797405822994,121.920470478076)) ;
#36476=CARTESIAN_POINT('Ctrl Pts',(-19.4433140464625,23.0697228078125,122.206271347254)) ;
#36477=CARTESIAN_POINT('Ctrl Pts',(-19.4518420605105,22.8897337274027,121.904884777568)) ;
#36478=CARTESIAN_POINT('Ctrl Pts',(-19.6510110881743,23.0796684884866,122.230368010918)) ;
#36479=CARTESIAN_POINT('Ctrl Pts',(-19.7114632832779,22.8996794080768,121.93500831667)) ;
#36480=CARTESIAN_POINT('Ctrl Pts',(-19.8515326787835,23.0896157461133,122.289763971548)) ;
#36481=CARTESIAN_POINT('Ctrl Pts',(-19.9621146838214,22.9096266657035,122.009255961529)) ;
#36482=CARTESIAN_POINT('Ctrl Pts',(-20.0404673828271,23.0996636482348,122.38422357924)) ;
#36483=CARTESIAN_POINT('Ctrl Pts',(-20.1982818352808,22.919674567825,122.127332902598)) ;
#36484=CARTESIAN_POINT('Ctrl Pts',(-20.2068601688876,23.1095113538565,122.507411205616)) ;
#36485=CARTESIAN_POINT('Ctrl Pts',(-20.4062715090899,22.9295222734466,122.281319880636)) ;
#36486=CARTESIAN_POINT('Ctrl Pts',(-20.3514553093839,23.1194728204906,122.658891921361)) ;
#36487=CARTESIAN_POINT('Ctrl Pts',(-20.587013493731,22.9394837400808,122.470672801433)) ;
#36488=CARTESIAN_POINT('Ctrl Pts',(-20.4681173020612,23.1295023737588,122.83453984717)) ;
#36489=CARTESIAN_POINT('Ctrl Pts',(-20.7328386956585,22.949513293349,122.690234279915)) ;
#36490=CARTESIAN_POINT('Ctrl Pts',(-20.5515843547797,23.1394092657862,123.025360354087)) ;
#36491=CARTESIAN_POINT('Ctrl Pts',(-20.837170043744,22.9594201853764,122.928761227123)) ;
#36492=CARTESIAN_POINT('Ctrl Pts',(-20.6012418234421,23.1493569098992,123.228492863603)) ;
#36493=CARTESIAN_POINT('Ctrl Pts',(-20.8992391771588,22.9693678294894,123.182677656163)) ;
#36494=CARTESIAN_POINT('Ctrl Pts',(-20.6150800343719,23.1593569529281,123.438296909276)) ;
#36495=CARTESIAN_POINT('Ctrl Pts',(-20.9165341377997,22.9793678725182,123.444932969308)) ;
#36496=CARTESIAN_POINT('Ctrl Pts',(-20.5918224314329,23.1693957189221,123.648041713659)) ;
#36497=CARTESIAN_POINT('Ctrl Pts',(-20.8874593438765,22.9894066385123,123.707113721917)) ;
#36498=CARTESIAN_POINT('Ctrl Pts',(-20.5341745069886,23.1792207809443,123.846402561714)) ;
#36499=CARTESIAN_POINT('Ctrl Pts',(-20.8153966816102,22.9992317005345,123.955064177267)) ;
#36500=CARTESIAN_POINT('Ctrl Pts',(-20.4411557623912,23.1892753282707,124.036199337756)) ;
#36501=CARTESIAN_POINT('Ctrl Pts',(-20.6991206974634,23.0092862478609,124.192308936978)) ;
#36502=CARTESIAN_POINT('Ctrl Pts',(-20.3176702770705,23.1992185717199,124.204874255302)) ;
#36503=CARTESIAN_POINT('Ctrl Pts',(-20.5447615014033,23.0192294913101,124.403151003518)) ;
#36504=CARTESIAN_POINT('Ctrl Pts',(-20.1678477489804,23.2091207433278,124.349412148835)) ;
#36505=CARTESIAN_POINT('Ctrl Pts',(-20.3574813482785,23.029131662918,124.583821375394)) ;
#36506=CARTESIAN_POINT('Ctrl Pts',(-19.9925143602655,23.219173578938,124.467395725293)) ;
#36507=CARTESIAN_POINT('Ctrl Pts',(-20.1383129463047,23.0391844985282,124.731298547817)) ;
#36508=CARTESIAN_POINT('Ctrl Pts',(-19.8028310164097,23.2290466366235,124.551692861004)) ;
#36509=CARTESIAN_POINT('Ctrl Pts',(-19.9012076725371,23.0490575562137,124.836667408576)) ;
#36510=CARTESIAN_POINT('Ctrl Pts',(-19.599035620592,23.2390418981492,124.602895730111)) ;
#36511=CARTESIAN_POINT('Ctrl Pts',(-19.6464624451239,23.0590528177394,124.900668231928)) ;
#36512=CARTESIAN_POINT('Ctrl Pts',(-19.3887803257811,23.2490672675697,124.617604462307)) ;
#36513=CARTESIAN_POINT('Ctrl Pts',(-19.3836439744428,23.0690781871599,124.919051527875)) ;
#36514=CARTESIAN_POINT('Ctrl Pts',(-19.1819671042923,23.2589571000963,124.596152765897)) ;
#36515=CARTESIAN_POINT('Ctrl Pts',(-19.1251242692566,23.0789680196865,124.892233416158)) ;
#36516=CARTESIAN_POINT('Ctrl Pts',(-18.9130557461595,23.2722550709057,124.5197923832)) ;
#36517=CARTESIAN_POINT('Ctrl Pts',(-18.7890035336814,23.0922659904958,124.796782825509)) ;
#36518=CARTESIAN_POINT('Ctrl Pts',(-18.6717587243513,23.2854534660148,124.376385706573)) ;
#36519=CARTESIAN_POINT('Ctrl Pts',(-18.4874072190353,23.105464385605,124.617549791565)) ;
#36520=CARTESIAN_POINT('Ctrl Pts',(-18.4752682237642,23.2988489082943,124.174730150354)) ;
#36521=CARTESIAN_POINT('Ctrl Pts',(-18.2417519025622,23.1188598278845,124.365440343036)) ;
#36522=CARTESIAN_POINT('Ctrl Pts',(-18.358218981122,23.3087247465333,124.00319866305)) ;
#36523=CARTESIAN_POINT('Ctrl Pts',(-18.0954516813819,23.1287356661234,124.151032241579)) ;
#36524=CARTESIAN_POINT('Ctrl Pts',(-18.2710692283596,23.318786149131,123.810502936059)) ;
#36525=CARTESIAN_POINT('Ctrl Pts',(-17.9865146771472,23.1387970687212,123.91015878141)) ;
#36526=CARTESIAN_POINT('Ctrl Pts',(-18.2196477196924,23.3286512060661,123.609550825009)) ;
#36527=CARTESIAN_POINT('Ctrl Pts',(-17.9222404620335,23.1486621256563,123.658970587681)) ;
#36528=CARTESIAN_POINT('Ctrl Pts',(-18.2032931252815,23.3386633020149,123.399733102314)) ;
#36529=CARTESIAN_POINT('Ctrl Pts',(-17.9018022903817,23.1586742216051,123.396691351191)) ;
#36530=CARTESIAN_POINT('Ctrl Pts',(-18.2303090879066,23.3519406111604,123.121854743172)) ;
#36531=CARTESIAN_POINT('Ctrl Pts',(-17.9355630206945,23.1719515307505,123.049376976585)) ;
#36532=CARTESIAN_POINT('Ctrl Pts',(-18.3537865412185,23.3685396366677,122.791280328664)) ;
#36533=CARTESIAN_POINT('Ctrl Pts',(-18.0899419028063,23.1885505562579,122.636110521805)) ;
#36534=CARTESIAN_POINT('Ctrl Pts',(-18.5826974213556,23.3851386847007,122.522589585536)) ;
#36535=CARTESIAN_POINT('Ctrl Pts',(-18.37602583293,23.2051496042909,122.300311520371)) ;
#36536=CARTESIAN_POINT('Ctrl Pts',(-18.8116870577227,23.3983820967316,122.364269542791)) ;
#36537=CARTESIAN_POINT('Ctrl Pts',(-18.6623130733646,23.2183930163218,122.102367993651)) ;
#36538=CARTESIAN_POINT('Ctrl Pts',(-19.0034183423248,23.4084195244201,122.276133501985)) ;
#36539=CARTESIAN_POINT('Ctrl Pts',(-18.9019676656233,23.2284304440103,121.992209381393)) ;
#36540=CARTESIAN_POINT('Ctrl Pts',(-19.2048395995662,23.4183238263757,122.223371608911)) ;
#36541=CARTESIAN_POINT('Ctrl Pts',(-19.1537511180721,23.2383347459658,121.926257438572)) ;
#36542=CARTESIAN_POINT('Ctrl Pts',(-19.4827891473364,23.4315906663508,122.19988920511)) ;
#36543=CARTESIAN_POINT('Ctrl Pts',(-19.5011668383607,23.251601585941,121.896906682968)) ;
#36544=CARTESIAN_POINT('Ctrl Pts',(-19.8307318849537,23.4482168644408,122.262263108639)) ;
#36545=CARTESIAN_POINT('Ctrl Pts',(-19.9361152833233,23.2682277840309,121.97487577289)) ;
#36546=CARTESIAN_POINT('Ctrl Pts',(-20.1971528166808,23.4681359798242,122.474678281948)) ;
#36547=CARTESIAN_POINT('Ctrl Pts',(-20.3941427128654,23.2881468994144,122.24041645657)) ;
#36548=CARTESIAN_POINT('Ctrl Pts',(-20.4241051193176,23.4847424029584,122.745236826327)) ;
#36549=CARTESIAN_POINT('Ctrl Pts',(-20.6777956763703,23.3047533225486,122.578559316813)) ;
#36550=CARTESIAN_POINT('Ctrl Pts',(-20.5421768965827,23.4980386234541,122.998554900509)) ;
#36551=CARTESIAN_POINT('Ctrl Pts',(-20.8254141686422,23.3180495430443,122.895260367397)) ;
#36552=CARTESIAN_POINT('Ctrl Pts',(-20.614959986531,23.5113074557956,123.267928258052)) ;
#36553=CARTESIAN_POINT('Ctrl Pts',(-20.9163840286482,23.3313183753857,123.231954203328)) ;
#36554=CARTESIAN_POINT('Ctrl Pts',(-20.6152647113257,23.5279987038287,123.622730942973)) ;
#36555=CARTESIAN_POINT('Ctrl Pts',(-20.9167633042125,23.3480096234189,123.675476169149)) ;
#36556=CARTESIAN_POINT('Ctrl Pts',(-20.4722994274042,23.5478084355015,124.018996186989)) ;
#36557=CARTESIAN_POINT('Ctrl Pts',(-20.7380527826881,23.3678193550916,124.170798980332)) ;
#36558=CARTESIAN_POINT('Ctrl Pts',(-20.2010981674225,23.56778604283,124.345907252259)) ;
#36559=CARTESIAN_POINT('Ctrl Pts',(-20.39904878012,23.3877969624202,124.579436972795)) ;
#36560=CARTESIAN_POINT('Ctrl Pts',(-19.8351962742171,23.5877123518879,124.559408382312)) ;
#36561=CARTESIAN_POINT('Ctrl Pts',(-19.9416700356662,23.4077232714781,124.846309372942)) ;
#36562=CARTESIAN_POINT('Ctrl Pts',(-19.4207969533748,23.6075292120526,124.636299831341)) ;
#36563=CARTESIAN_POINT('Ctrl Pts',(-19.4236722805428,23.4275401316427,124.942420637925)) ;
#36564=CARTESIAN_POINT('Ctrl Pts',(-18.9994637731957,23.6276290276466,124.565563992342)) ;
#36565=CARTESIAN_POINT('Ctrl Pts',(-18.8970052108273,23.4476399472368,124.85399762063)) ;
#36566=CARTESIAN_POINT('Ctrl Pts',(-18.6335253229913,23.6473859915291,124.358902751464)) ;
#36567=CARTESIAN_POINT('Ctrl Pts',(-18.439585873165,23.4673969111193,124.595670036083)) ;
#36568=CARTESIAN_POINT('Ctrl Pts',(-18.3557767431134,23.6674229175986,124.036039149984)) ;
#36569=CARTESIAN_POINT('Ctrl Pts',(-18.092401477784,23.4874338371887,124.192088863954)) ;
#36570=CARTESIAN_POINT('Ctrl Pts',(-18.2066700929233,23.6872924999801,123.640628669761)) ;
#36571=CARTESIAN_POINT('Ctrl Pts',(-17.9060208621078,23.5073034195703,123.697826439098)) ;
#36572=CARTESIAN_POINT('Ctrl Pts',(-18.20037309154,23.7071970717333,123.217532309015)) ;
#36573=CARTESIAN_POINT('Ctrl Pts',(-17.898151051561,23.5272079913234,123.168957382095)) ;
#36574=CARTESIAN_POINT('Ctrl Pts',(-18.3392583799834,23.7271496739318,122.816587599737)) ;
#36575=CARTESIAN_POINT('Ctrl Pts',(-18.0717585757176,23.547160593522,122.667777463701)) ;
#36576=CARTESIAN_POINT('Ctrl Pts',(-18.6060586541103,23.747059164902,122.488027614891)) ;
#36577=CARTESIAN_POINT('Ctrl Pts',(-18.405258884035,23.5670700844922,122.25707925787)) ;
#36578=CARTESIAN_POINT('Ctrl Pts',(-18.9674540788008,23.7669105336015,122.269754789477)) ;
#36579=CARTESIAN_POINT('Ctrl Pts',(-18.8570010753388,23.5869214531917,121.98423938823)) ;
#36580=CARTESIAN_POINT('Ctrl Pts',(-19.3863467957852,23.7869907297375,122.187619791407)) ;
#36581=CARTESIAN_POINT('Ctrl Pts',(-19.3806182677783,23.6070016493277,121.881570519857)) ;
#36582=CARTESIAN_POINT('Ctrl Pts',(-19.8024562321169,23.8067916733129,122.25247266476)) ;
#36583=CARTESIAN_POINT('Ctrl Pts',(-19.9007519851845,23.6268025929031,121.962636023164)) ;
#36584=CARTESIAN_POINT('Ctrl Pts',(-20.1751703809712,23.8267756498224,122.456380190659)) ;
#36585=CARTESIAN_POINT('Ctrl Pts',(-20.3666450135569,23.6467865694126,122.217519362983)) ;
#36586=CARTESIAN_POINT('Ctrl Pts',(-20.4545225997992,23.846691612798,122.774634398599)) ;
#36587=CARTESIAN_POINT('Ctrl Pts',(-20.7158350928869,23.6667025323882,122.615335633033)) ;
#36588=CARTESIAN_POINT('Ctrl Pts',(-20.6092694572912,23.8665620476199,123.167863522626)) ;
#36589=CARTESIAN_POINT('Ctrl Pts',(-20.9092697535832,23.6865729672101,123.106869748177)) ;
#36590=CARTESIAN_POINT('Ctrl Pts',(-20.6199224875745,23.886612332853,123.593929804403)) ;
#36591=CARTESIAN_POINT('Ctrl Pts',(-20.922587690432,23.7066232524431,123.639453176965)) ;
#36592=CARTESIAN_POINT('Ctrl Pts',(-20.4868864023955,23.9063863016123,123.992954670448)) ;
#36593=CARTESIAN_POINT('Ctrl Pts',(-20.7562955196526,23.7263972212025,124.138232320096)) ;
#36594=CARTESIAN_POINT('Ctrl Pts',(-20.2223831801166,23.9264427597318,124.327253105703)) ;
#36595=CARTESIAN_POINT('Ctrl Pts',(-20.4256681461697,23.746453679322,124.556107455233)) ;
#36596=CARTESIAN_POINT('Ctrl Pts',(-19.8640850949148,23.9462376427228,124.548331334748)) ;
#36597=CARTESIAN_POINT('Ctrl Pts',(-19.9777988611874,23.766248562313,124.832456311701)) ;
#36598=CARTESIAN_POINT('Ctrl Pts',(-19.448727810941,23.9662042980252,124.63574281183)) ;
#36599=CARTESIAN_POINT('Ctrl Pts',(-19.458603262155,23.7862152176154,124.941723990057)) ;
#36600=CARTESIAN_POINT('Ctrl Pts',(-19.0285651397822,23.9861632681017,124.575472295223)) ;
#36601=CARTESIAN_POINT('Ctrl Pts',(-18.9333997951167,23.8061741876918,124.866389115845)) ;
#36602=CARTESIAN_POINT('Ctrl Pts',(-18.6553168032142,24.0060593556918,124.376389568719)) ;
#36603=CARTESIAN_POINT('Ctrl Pts',(-18.4668385535569,23.826070275282,124.617539311682)) ;
#36604=CARTESIAN_POINT('Ctrl Pts',(-18.3720148561307,24.0259575256034,124.062201487962)) ;
#36605=CARTESIAN_POINT('Ctrl Pts',(-18.1127087821961,23.8459684451936,124.224807490368)) ;
#36606=CARTESIAN_POINT('Ctrl Pts',(-18.2124303919169,24.0458633609705,123.67015401321)) ;
#36607=CARTESIAN_POINT('Ctrl Pts',(-17.9132245362544,23.8658742805607,123.734750368426)) ;
#36608=CARTESIAN_POINT('Ctrl Pts',(-18.1961880168038,24.0658132859084,123.246313641307)) ;
#36609=CARTESIAN_POINT('Ctrl Pts',(-17.8929172316188,23.8858242054986,123.204950398217)) ;
#36610=CARTESIAN_POINT('Ctrl Pts',(-18.3247423088814,24.0856924758188,122.84360479257)) ;
#36611=CARTESIAN_POINT('Ctrl Pts',(-18.0536055021763,23.905703395409,122.701563670967)) ;
#36612=CARTESIAN_POINT('Ctrl Pts',(-18.5841033382921,24.1056738000994,122.507146079178)) ;
#36613=CARTESIAN_POINT('Ctrl Pts',(-18.3778029519337,23.9256847196896,122.280987362642)) ;
#36614=CARTESIAN_POINT('Ctrl Pts',(-18.942010615732,24.1256035843077,122.280096072877)) ;
#36615=CARTESIAN_POINT('Ctrl Pts',(-18.8251843464283,23.9456145038979,121.997171158649)) ;
#36616=CARTESIAN_POINT('Ctrl Pts',(-19.3555068623215,24.1455235736985,122.188809483554)) ;
#36617=CARTESIAN_POINT('Ctrl Pts',(-19.3420527237454,23.9655344932887,121.88305758852)) ;
#36618=CARTESIAN_POINT('Ctrl Pts',(-19.7742904831662,24.1653787690525,122.2430041829)) ;
#36619=CARTESIAN_POINT('Ctrl Pts',(-19.8655341730097,23.9853896886427,121.950798016856)) ;
#36620=CARTESIAN_POINT('Ctrl Pts',(-20.1526808934445,24.1854247707119,122.438992855019)) ;
#36621=CARTESIAN_POINT('Ctrl Pts',(-20.3385180584814,24.005435690302,122.195770834765)) ;
#36622=CARTESIAN_POINT('Ctrl Pts',(-20.3906070125325,24.2019245179217,122.696923893817)) ;
#36623=CARTESIAN_POINT('Ctrl Pts',(-20.6359495242744,24.0219354375118,122.518207743298)) ;
#36624=CARTESIAN_POINT('Ctrl Pts',(-20.5216768074671,24.2153131223698,122.945999721875)) ;
#36625=CARTESIAN_POINT('Ctrl Pts',(-20.7997715921417,24.0353240419599,122.829526935815)) ;
#36626=CARTESIAN_POINT('Ctrl Pts',(-20.5848955736062,24.2251749507047,123.143455647205)) ;
#36627=CARTESIAN_POINT('Ctrl Pts',(-20.8788004514972,24.0451858702949,123.07635383237)) ;
#36628=CARTESIAN_POINT('Ctrl Pts',(-20.6138199274551,24.2351410934622,123.350985731134)) ;
#36629=CARTESIAN_POINT('Ctrl Pts',(-20.9149604444561,24.0551520130524,123.335751428968)) ;
#36630=CARTESIAN_POINT('Ctrl Pts',(-20.6032002789081,24.2485028395872,123.631591883731)) ;
#36631=CARTESIAN_POINT('Ctrl Pts',(-20.9016757193744,24.0685137591774,123.686576406625)) ;
#36632=CARTESIAN_POINT('Ctrl Pts',(-20.5008787541352,24.2649571685423,123.966355059804)) ;
#36633=CARTESIAN_POINT('Ctrl Pts',(-20.7738010339996,24.0849680881324,124.104947280298)) ;
#36634=CARTESIAN_POINT('Ctrl Pts',(-20.2867198767303,24.2817244135906,124.2511417434)) ;
#36635=CARTESIAN_POINT('Ctrl Pts',(-20.5060740059502,24.1017353331807,124.46098906877)) ;
#36636=CARTESIAN_POINT('Ctrl Pts',(-20.068100156107,24.2949109788646,124.421823870107)) ;
#36637=CARTESIAN_POINT('Ctrl Pts',(-20.2328267963753,24.1149218984548,124.67431188179)) ;
#36638=CARTESIAN_POINT('Ctrl Pts',(-19.8829901974809,24.3049004376092,124.520886533694)) ;
#36639=CARTESIAN_POINT('Ctrl Pts',(-20.0014355866931,24.1249113571994,124.798149276019)) ;
#36640=CARTESIAN_POINT('Ctrl Pts',(-19.6841183586994,24.3148542100903,124.586142139234)) ;
#36641=CARTESIAN_POINT('Ctrl Pts',(-19.7528479925911,24.1348651296805,124.879719694425)) ;
#36642=CARTESIAN_POINT('Ctrl Pts',(-19.4750256631218,24.324902026623,124.61598118881)) ;
#36643=CARTESIAN_POINT('Ctrl Pts',(-19.4914820582806,24.1449129462132,124.917021763286)) ;
#36644=CARTESIAN_POINT('Ctrl Pts',(-19.2682080171776,24.3347435597455,124.609445253002)) ;
#36645=CARTESIAN_POINT('Ctrl Pts',(-19.2329600579594,24.1547544793356,124.908854524418)) ;
#36646=CARTESIAN_POINT('Ctrl Pts',(-19.0626517418926,24.3447298019652,124.566925901012)) ;
#36647=CARTESIAN_POINT('Ctrl Pts',(-18.9760140363153,24.1647407215554,124.855708116938)) ;
#36648=CARTESIAN_POINT('Ctrl Pts',(-18.8684666859137,24.3546664253901,124.489818172107)) ;
#36649=CARTESIAN_POINT('Ctrl Pts',(-18.7332816198443,24.1746773449803,124.759326036372)) ;
#36650=CARTESIAN_POINT('Ctrl Pts',(-18.688696650813,24.3647163027731,124.378854486706)) ;
#36651=CARTESIAN_POINT('Ctrl Pts',(-18.5085675409844,24.1847272223632,124.620623799744)) ;
#36652=CARTESIAN_POINT('Ctrl Pts',(-18.5339244507054,24.3745667415506,124.241242493615)) ;
#36653=CARTESIAN_POINT('Ctrl Pts',(-18.31510033538,24.1945776611408,124.448610838054)) ;
#36654=CARTESIAN_POINT('Ctrl Pts',(-18.4034080881523,24.3845387555194,124.077216087896)) ;
#36655=CARTESIAN_POINT('Ctrl Pts',(-18.1519526132977,24.2045496751095,124.243579488849)) ;
#36656=CARTESIAN_POINT('Ctrl Pts',(-18.3031188994434,24.3945339241455,123.892525344681)) ;
#36657=CARTESIAN_POINT('Ctrl Pts',(-18.0265886283388,24.2145448437356,124.012717326588)) ;
#36658=CARTESIAN_POINT('Ctrl Pts',(-18.2364182379383,24.4045678074067,123.692421879584)) ;
#36659=CARTESIAN_POINT('Ctrl Pts',(-17.943210117293,24.2245787269968,123.762588848244)) ;
#36660=CARTESIAN_POINT('Ctrl Pts',(-18.2057083821517,24.41442367747,123.487493870639)) ;
#36661=CARTESIAN_POINT('Ctrl Pts',(-17.9048199952897,24.2344345970602,123.506429025604)) ;
#36662=CARTESIAN_POINT('Ctrl Pts',(-18.2107882331578,24.4244212233872,123.277398137475)) ;
#36663=CARTESIAN_POINT('Ctrl Pts',(-17.9111670276796,24.2444321429774,123.243809194856)) ;
#36664=CARTESIAN_POINT('Ctrl Pts',(-18.2518400342972,24.4343293502864,123.073174907185)) ;
#36665=CARTESIAN_POINT('Ctrl Pts',(-17.9624791058207,24.2543402698766,122.988529382355)) ;
#36666=CARTESIAN_POINT('Ctrl Pts',(-18.3281714579042,24.4443397218086,122.877045008902)) ;
#36667=CARTESIAN_POINT('Ctrl Pts',(-18.0578908531546,24.2643506413988,122.743365948053)) ;
#36668=CARTESIAN_POINT('Ctrl Pts',(-18.438010301051,24.454370164556,122.69704745568)) ;
#36669=CARTESIAN_POINT('Ctrl Pts',(-18.1951870356192,24.2743810841462,122.518367543311)) ;
#36670=CARTESIAN_POINT('Ctrl Pts',(-18.5745495647584,24.4642181171093,122.541397741827)) ;
#36671=CARTESIAN_POINT('Ctrl Pts',(-18.3658593160334,24.2842290366995,122.323803295481)) ;
#36672=CARTESIAN_POINT('Ctrl Pts',(-18.7394306699372,24.4742807861303,122.408888682602)) ;
#36673=CARTESIAN_POINT('Ctrl Pts',(-18.5719589573897,24.2942917057204,122.158164871413)) ;
#36674=CARTESIAN_POINT('Ctrl Pts',(-18.9218207597135,24.4841751615942,122.308835807993)) ;
#36675=CARTESIAN_POINT('Ctrl Pts',(-18.7999455381044,24.3041860811844,122.033096218189)) ;
#36676=CARTESIAN_POINT('Ctrl Pts',(-19.119533784816,24.4941169599123,122.241135188269)) ;
#36677=CARTESIAN_POINT('Ctrl Pts',(-19.0470862012613,24.3141278795025,121.948467825703)) ;
#36678=CARTESIAN_POINT('Ctrl Pts',(-19.327299776132,24.5041194536396,122.208506614829)) ;
#36679=CARTESIAN_POINT('Ctrl Pts',(-19.3067933605176,24.3241303732298,121.907679467722)) ;
#36680=CARTESIAN_POINT('Ctrl Pts',(-19.5382060178291,24.5141542521466,122.212793291372)) ;
#36681=CARTESIAN_POINT('Ctrl Pts',(-19.5704262020261,24.3341651717368,121.913035104039)) ;
#36682=CARTESIAN_POINT('Ctrl Pts',(-19.741340693941,24.5239991361259,122.252526138907)) ;
#36683=CARTESIAN_POINT('Ctrl Pts',(-19.8243456091052,24.3440100557161,121.962698661927)) ;
#36684=CARTESIAN_POINT('Ctrl Pts',(-19.9373544726432,24.533984992944,122.327605162214)) ;
#36685=CARTESIAN_POINT('Ctrl Pts',(-20.0693639138085,24.3539959125342,122.056545067765)) ;
#36686=CARTESIAN_POINT('Ctrl Pts',(-20.1165728966918,24.5439198071187,122.434935896096)) ;
#36687=CARTESIAN_POINT('Ctrl Pts',(-20.293388543739,24.3639307267089,122.190706447079)) ;
#36688=CARTESIAN_POINT('Ctrl Pts',(-20.2762066027916,24.5539773069041,122.573540909043)) ;
#36689=CARTESIAN_POINT('Ctrl Pts',(-20.4929322997867,24.3739882264943,122.363960667398)) ;
#36690=CARTESIAN_POINT('Ctrl Pts',(-20.4065058320593,24.5637990653224,122.733750397852)) ;
#36691=CARTESIAN_POINT('Ctrl Pts',(-20.6558088061763,24.3838099849125,122.564221525953)) ;
#36692=CARTESIAN_POINT('Ctrl Pts',(-20.5097290699146,24.5738547231064,122.918217818253)) ;
#36693=CARTESIAN_POINT('Ctrl Pts',(-20.7848399621109,24.3938656426965,122.794804495991)) ;
#36694=CARTESIAN_POINT('Ctrl Pts',(-20.5782202375852,24.5837969052864,123.115704900593)) ;
#36695=CARTESIAN_POINT('Ctrl Pts',(-20.8704564404007,24.4038078248766,123.041662828732)) ;
#36696=CARTESIAN_POINT('Ctrl Pts',(-20.6118814894185,24.5937021139811,123.32120168517)) ;
#36697=CARTESIAN_POINT('Ctrl Pts',(-20.9125354802017,24.4137130335713,123.298533937994)) ;
#36698=CARTESIAN_POINT('Ctrl Pts',(-20.6092481539705,24.6037439049435,123.532291786237)) ;
#36699=CARTESIAN_POINT('Ctrl Pts',(-20.9092462484332,24.4237548245337,123.562396507281)) ;
#36700=CARTESIAN_POINT('Ctrl Pts',(-20.5705464706402,24.6136516794158,123.73696556278)) ;
#36701=CARTESIAN_POINT('Ctrl Pts',(-20.8608714360001,24.433662599006,123.818239689854)) ;
#36702=CARTESIAN_POINT('Ctrl Pts',(-20.4964883343986,24.6236631796434,123.933985160015)) ;
#36703=CARTESIAN_POINT('Ctrl Pts',(-20.7683009427503,24.4436740992336,124.064515066645)) ;
#36704=CARTESIAN_POINT('Ctrl Pts',(-20.388743463947,24.6336959400361,124.115308071487)) ;
#36705=CARTESIAN_POINT('Ctrl Pts',(-20.6336219826215,24.4537068596262,124.291169915727)) ;
#36706=CARTESIAN_POINT('Ctrl Pts',(-20.2539226961547,24.643546509171,124.272507133189)) ;
#36707=CARTESIAN_POINT('Ctrl Pts',(-20.4650972756189,24.4635574287611,124.487670909618)) ;
#36708=CARTESIAN_POINT('Ctrl Pts',(-20.0918811514129,24.6535351187009,124.406043156148)) ;
#36709=CARTESIAN_POINT('Ctrl Pts',(-20.2625466477775,24.4735460382911,124.65459280721)) ;
#36710=CARTESIAN_POINT('Ctrl Pts',(-19.9101907899771,24.663463774725,124.50880446125)) ;
#36711=CARTESIAN_POINT('Ctrl Pts',(-20.0354343909246,24.4834746943151,124.783046651273)) ;
#36712=CARTESIAN_POINT('Ctrl Pts',(-19.7123608153397,24.6734515209028,124.579209070927)) ;
#36713=CARTESIAN_POINT('Ctrl Pts',(-19.7881474809578,24.4934624404929,124.871054527535)) ;
#36714=CARTESIAN_POINT('Ctrl Pts',(-19.504271624768,24.6834875098385,124.614009588062)) ;
#36715=CARTESIAN_POINT('Ctrl Pts',(-19.5280364526024,24.5034984294287,124.914557400137)) ;
#36716=CARTESIAN_POINT('Ctrl Pts',(-19.2970799984549,24.6933423796521,124.612527488624)) ;
#36717=CARTESIAN_POINT('Ctrl Pts',(-19.2690459880679,24.5133532992423,124.91270694931)) ;
#36718=CARTESIAN_POINT('Ctrl Pts',(-19.090303135345,24.7033418208939,124.574834044645)) ;
#36719=CARTESIAN_POINT('Ctrl Pts',(-19.0105743992128,24.5233527404841,124.865592193669)) ;
#36720=CARTESIAN_POINT('Ctrl Pts',(-18.8951262772354,24.713236895074,124.502757695016)) ;
#36721=CARTESIAN_POINT('Ctrl Pts',(-18.7666019328794,24.5332478146641,124.775498416495)) ;
#36722=CARTESIAN_POINT('Ctrl Pts',(-18.7124871130711,24.7232975509137,124.396143715782)) ;
#36723=CARTESIAN_POINT('Ctrl Pts',(-18.5383021509455,24.5433084705038,124.642232833869)) ;
#36724=CARTESIAN_POINT('Ctrl Pts',(-18.5544214010454,24.7331464251093,124.262378682155)) ;
#36725=CARTESIAN_POINT('Ctrl Pts',(-18.3407179160903,24.5531573446995,124.475027408932)) ;
#36726=CARTESIAN_POINT('Ctrl Pts',(-18.4191678408928,24.7431751370725,124.100648450517)) ;
#36727=CARTESIAN_POINT('Ctrl Pts',(-18.1716495640593,24.5631860566627,124.272865839521)) ;
#36728=CARTESIAN_POINT('Ctrl Pts',(-18.3145372263734,24.7532045376556,123.917586468341)) ;
#36729=CARTESIAN_POINT('Ctrl Pts',(-18.0408595711502,24.5732154572458,124.044039432709)) ;
#36730=CARTESIAN_POINT('Ctrl Pts',(-18.2441926662311,24.7630447312725,123.723038994785)) ;
#36731=CARTESIAN_POINT('Ctrl Pts',(-17.9529267053287,24.5830556508627,123.800854664301)) ;
#36732=CARTESIAN_POINT('Ctrl Pts',(-18.2077279525062,24.7730481538477,123.515942344631)) ;
#36733=CARTESIAN_POINT('Ctrl Pts',(-17.9073440509862,24.5930590734379,123.541984051111)) ;
#36734=CARTESIAN_POINT('Ctrl Pts',(-18.2078442834315,24.7830336909408,123.305979629472)) ;
#36735=CARTESIAN_POINT('Ctrl Pts',(-17.9074876719924,24.6030446105309,123.27953044781)) ;
#36736=CARTESIAN_POINT('Ctrl Pts',(-18.244816810972,24.7930746954276,123.098169474309)) ;
#36737=CARTESIAN_POINT('Ctrl Pts',(-17.9537014743121,24.6130856150177,123.019767558677)) ;
#36738=CARTESIAN_POINT('Ctrl Pts',(-18.3156319158811,24.8029182343688,122.903704450163)) ;
#36739=CARTESIAN_POINT('Ctrl Pts',(-18.0422190939803,24.622929153959,122.776684574522)) ;
#36740=CARTESIAN_POINT('Ctrl Pts',(-18.4202205854455,24.8129032653596,122.721733922501)) ;
#36741=CARTESIAN_POINT('Ctrl Pts',(-18.172953642186,24.6329141849498,122.549220386066)) ;
#36742=CARTESIAN_POINT('Ctrl Pts',(-18.5541770056788,24.8228427278816,122.561322433432)) ;
#36743=CARTESIAN_POINT('Ctrl Pts',(-18.3403982887931,24.6428536474717,122.348704582973)) ;
#36744=CARTESIAN_POINT('Ctrl Pts',(-18.715558190906,24.8328824601054,122.425314061368)) ;
#36745=CARTESIAN_POINT('Ctrl Pts',(-18.5421236161381,24.6528933796956,122.178692975318)) ;
#36746=CARTESIAN_POINT('Ctrl Pts',(-18.8953205226514,24.8427706404226,122.320888321674)) ;
#36747=CARTESIAN_POINT('Ctrl Pts',(-18.7668265323495,24.6627815600127,122.048158969727)) ;
#36748=CARTESIAN_POINT('Ctrl Pts',(-19.0923303882549,24.8527601561251,122.248163396936)) ;
#36749=CARTESIAN_POINT('Ctrl Pts',(-19.0130885634248,24.6727710757152,121.957251380522)) ;
#36750=CARTESIAN_POINT('Ctrl Pts',(-19.298364039197,24.8627187067798,122.211026101757)) ;
#36751=CARTESIAN_POINT('Ctrl Pts',(-19.2706307855843,24.68272962637,121.910828202556)) ;
#36752=CARTESIAN_POINT('Ctrl Pts',(-19.5064905058478,24.8726181138848,122.209713205834)) ;
#36753=CARTESIAN_POINT('Ctrl Pts',(-19.5307897392414,24.692629033475,121.909185754138)) ;
#36754=CARTESIAN_POINT('Ctrl Pts',(-19.7147219092595,24.8826667003011,122.245162774326)) ;
#36755=CARTESIAN_POINT('Ctrl Pts',(-19.7910790035735,24.7026776198912,121.953496342131)) ;
#36756=CARTESIAN_POINT('Ctrl Pts',(-19.9106826139148,24.8925595192655,122.314960468538)) ;
#36757=CARTESIAN_POINT('Ctrl Pts',(-20.0360311857211,24.7125704388557,122.040742561754)) ;
#36758=CARTESIAN_POINT('Ctrl Pts',(-20.0946951962707,24.9026306367953,122.41960013013)) ;
#36759=CARTESIAN_POINT('Ctrl Pts',(-20.2660472328495,24.7226415563855,122.171540812084)) ;
#36760=CARTESIAN_POINT('Ctrl Pts',(-20.2538475997201,24.9124463307614,122.551014009269)) ;
#36761=CARTESIAN_POINT('Ctrl Pts',(-20.4649896869085,24.7324572503516,122.335808206384)) ;
#36762=CARTESIAN_POINT('Ctrl Pts',(-20.3913621573758,24.9225127082587,122.711814363181)) ;
#36763=CARTESIAN_POINT('Ctrl Pts',(-20.6368834830803,24.7425236278489,122.536807653751)) ;
#36764=CARTESIAN_POINT('Ctrl Pts',(-20.4970748886783,24.9324116943406,122.891133137665)) ;
#36765=CARTESIAN_POINT('Ctrl Pts',(-20.7690258159977,24.7524226139307,122.760956322178)) ;
#36766=CARTESIAN_POINT('Ctrl Pts',(-20.571232101278,24.9424658743341,123.089018879175)) ;
#36767=CARTESIAN_POINT('Ctrl Pts',(-20.8617232643384,24.7624767939243,123.008312860286)) ;
#36768=CARTESIAN_POINT('Ctrl Pts',(-20.6094160911567,24.9523366872668,123.293040667745)) ;
#36769=CARTESIAN_POINT('Ctrl Pts',(-20.909454464959,24.772347606857,123.263341038954)) ;
#36770=CARTESIAN_POINT('Ctrl Pts',(-20.6116329545151,24.9624105881206,123.504764653356)) ;
#36771=CARTESIAN_POINT('Ctrl Pts',(-20.9122265610238,24.7824215077108,123.527995577723)) ;
#36772=CARTESIAN_POINT('Ctrl Pts',(-20.5781600299015,24.9722307435072,123.708532107742)) ;
#36773=CARTESIAN_POINT('Ctrl Pts',(-20.8703860649525,24.7922416630974,123.782706579773)) ;
#36774=CARTESIAN_POINT('Ctrl Pts',(-20.508237892881,24.9823094504595,123.908493710654)) ;
#36775=CARTESIAN_POINT('Ctrl Pts',(-20.7829843523963,24.8023203700497,124.032658419527)) ;
#36776=CARTESIAN_POINT('Ctrl Pts',(-20.4070053264551,24.9921610389983,124.089234851178)) ;
#36777=CARTESIAN_POINT('Ctrl Pts',(-20.6564437175052,24.8121719585885,124.258586397177)) ;
#36778=CARTESIAN_POINT('Ctrl Pts',(-20.2731799394624,25.0022341555233,124.253310305418)) ;
#36779=CARTESIAN_POINT('Ctrl Pts',(-20.489162844456,24.8222450751134,124.463680852366)) ;
#36780=CARTESIAN_POINT('Ctrl Pts',(-20.1165044718704,25.0120766726191,124.388500704501)) ;
#36781=CARTESIAN_POINT('Ctrl Pts',(-20.2933179390666,24.8320875922093,124.63267035684)) ;
#36782=CARTESIAN_POINT('Ctrl Pts',(-19.936630039934,25.022057134173,124.496508778481)) ;
#36783=CARTESIAN_POINT('Ctrl Pts',(-20.0684748873382,24.8420680537632,124.767681031744)) ;
#36784=CARTESIAN_POINT('Ctrl Pts',(-19.7398406206067,25.0320753841638,124.571552225653)) ;
#36785=CARTESIAN_POINT('Ctrl Pts',(-19.8224883547099,24.852086303754,124.861485946941)) ;
#36786=CARTESIAN_POINT('Ctrl Pts',(-19.5358376882034,25.0419595443576,124.611179719753)) ;
#36787=CARTESIAN_POINT('Ctrl Pts',(-19.5674837085311,24.8619704639478,124.911020996761)) ;
#36788=CARTESIAN_POINT('Ctrl Pts',(-19.3242913071813,25.0520246913326,124.614802833866)) ;
#36789=CARTESIAN_POINT('Ctrl Pts',(-19.3030511329989,24.8720356109227,124.915550386489)) ;
#36790=CARTESIAN_POINT('Ctrl Pts',(-19.1199106240367,25.0618665149734,124.582483950528)) ;
#36791=CARTESIAN_POINT('Ctrl Pts',(-19.0475737608412,24.8818774345635,124.875152002787)) ;
#36792=CARTESIAN_POINT('Ctrl Pts',(-18.9203492375791,25.0718959874342,124.514427752027)) ;
#36793=CARTESIAN_POINT('Ctrl Pts',(-18.7981220481648,24.8919069070244,124.790082006615)) ;
#36794=CARTESIAN_POINT('Ctrl Pts',(-18.7359613362089,25.0819228426962,124.412260699821)) ;
#36795=CARTESIAN_POINT('Ctrl Pts',(-18.5676370264937,24.9019337622864,124.662373648664)) ;
#36796=CARTESIAN_POINT('Ctrl Pts',(-18.5748042640139,25.0917660928068,124.282445342146)) ;
#36797=CARTESIAN_POINT('Ctrl Pts',(-18.3661893963052,24.9117770123969,124.500103756248)) ;
#36798=CARTESIAN_POINT('Ctrl Pts',(-18.4355859909014,25.1018145323899,124.123567079919)) ;
#36799=CARTESIAN_POINT('Ctrl Pts',(-18.1921666069549,24.9218254519801,124.301506228966)) ;
#36800=CARTESIAN_POINT('Ctrl Pts',(-18.3274272880711,25.1117640266378,123.944530772977)) ;
#36801=CARTESIAN_POINT('Ctrl Pts',(-18.0569676781465,24.931774946228,124.07771050016)) ;
#36802=CARTESIAN_POINT('Ctrl Pts',(-18.2517272644222,25.1216718823638,123.750467023187)) ;
#36803=CARTESIAN_POINT('Ctrl Pts',(-17.9623422827385,24.941682801954,123.835129981022)) ;
#36804=CARTESIAN_POINT('Ctrl Pts',(-18.2104743970335,25.1317313590138,123.543070104516)) ;
#36805=CARTESIAN_POINT('Ctrl Pts',(-17.9107761379944,24.9517422786039,123.575884197332)) ;
#36806=CARTESIAN_POINT('Ctrl Pts',(-18.2056782190192,25.1415721684225,123.336215569633)) ;
#36807=CARTESIAN_POINT('Ctrl Pts',(-17.9047808644397,24.9615830880126,123.317314560697)) ;
#36808=CARTESIAN_POINT('Ctrl Pts',(-18.2373040930332,25.1516343187233,123.127077183961)) ;
#36809=CARTESIAN_POINT('Ctrl Pts',(-17.944313237632,24.9716452383135,123.055891956655)) ;
#36810=CARTESIAN_POINT('Ctrl Pts',(-18.3038712513499,25.1615314798458,122.929932299027)) ;
#36811=CARTESIAN_POINT('Ctrl Pts',(-18.0275225051549,24.981542399436,122.809459900644)) ;
#36812=CARTESIAN_POINT('Ctrl Pts',(-18.4033840340755,25.1714626542499,122.746394261675)) ;
#36813=CARTESIAN_POINT('Ctrl Pts',(-18.1519140706744,24.9914735738401,122.580036852165)) ;
#36814=CARTESIAN_POINT('Ctrl Pts',(-18.534887670248,25.1815048579749,122.581237562845)) ;
#36815=CARTESIAN_POINT('Ctrl Pts',(-18.3162936299814,25.0015157775651,122.373591256338)) ;
#36816=CARTESIAN_POINT('Ctrl Pts',(-18.690527647173,25.1913914404053,122.443467269935)) ;
#36817=CARTESIAN_POINT('Ctrl Pts',(-18.5108445770274,25.0114023599955,122.201377852342)) ;
#36818=CARTESIAN_POINT('Ctrl Pts',(-18.8694400895696,25.2013848761537,122.333355299341)) ;
#36819=CARTESIAN_POINT('Ctrl Pts',(-18.7344855027251,25.0213957957439,122.063738108115)) ;
#36820=CARTESIAN_POINT('Ctrl Pts',(-19.0638333349581,25.2113293445118,122.256415312659)) ;
#36821=CARTESIAN_POINT('Ctrl Pts',(-18.9774777480987,25.031340264102,121.967563231997)) ;
#36822=CARTESIAN_POINT('Ctrl Pts',(-19.2687117383254,25.2212811607574,122.213977770171)) ;
#36823=CARTESIAN_POINT('Ctrl Pts',(-19.2335763972237,25.0412920803476,121.914516693605)) ;
#36824=CARTESIAN_POINT('Ctrl Pts',(-19.4796320217027,25.2313185968719,122.207898426795)) ;
#36825=CARTESIAN_POINT('Ctrl Pts',(-19.497226599863,25.0513295164621,121.906917954513)) ;
#36826=CARTESIAN_POINT('Ctrl Pts',(-19.6852897576632,25.2412035560482,122.237873411144)) ;
#36827=CARTESIAN_POINT('Ctrl Pts',(-19.7542997604655,25.0612144756384,121.944387345467)) ;
#36828=CARTESIAN_POINT('Ctrl Pts',(-19.8849152260127,25.2512016742602,122.303598681316)) ;
#36829=CARTESIAN_POINT('Ctrl Pts',(-20.0038315528592,25.0712125938503,122.026544562905)) ;
#36830=CARTESIAN_POINT('Ctrl Pts',(-20.0687767747122,25.2611226067721,122.402114690331)) ;
#36831=CARTESIAN_POINT('Ctrl Pts',(-20.2336588621187,25.0811335263623,122.149690526429)) ;
#36832=CARTESIAN_POINT('Ctrl Pts',(-20.2347377539777,25.2711639069942,122.532559750854)) ;
#36833=CARTESIAN_POINT('Ctrl Pts',(-20.441109523497,25.0911748265844,122.312747279653)) ;
#36834=CARTESIAN_POINT('Ctrl Pts',(-20.3735985016344,25.2810708253842,122.687791031638)) ;
#36835=CARTESIAN_POINT('Ctrl Pts',(-20.6146855653085,25.1010817449744,122.506787487655)) ;
#36836=CARTESIAN_POINT('Ctrl Pts',(-20.4842246461165,25.2910066170932,122.864973861521)) ;
#36837=CARTESIAN_POINT('Ctrl Pts',(-20.7529678400748,25.1110175366834,122.728267052346)) ;
#36838=CARTESIAN_POINT('Ctrl Pts',(-20.5630324165797,25.3010475116711,123.060797396838)) ;
#36839=CARTESIAN_POINT('Ctrl Pts',(-20.8514767359584,25.1210584312613,122.973046599263)) ;
#36840=CARTESIAN_POINT('Ctrl Pts',(-20.6061255781903,25.310934713385,123.264152339049)) ;
#36841=CARTESIAN_POINT('Ctrl Pts',(-20.9053425590563,25.1309456329752,123.227241473622)) ;
#36842=CARTESIAN_POINT('Ctrl Pts',(-20.6136784836377,25.3209269811466,123.474070984614)) ;
#36843=CARTESIAN_POINT('Ctrl Pts',(-20.9147827033074,25.1409379007368,123.489640019816)) ;
#36844=CARTESIAN_POINT('Ctrl Pts',(-20.5847340091675,25.3308755021684,123.681219469277)) ;
#36845=CARTESIAN_POINT('Ctrl Pts',(-20.8786010725956,25.1508864217586,123.74857602838)) ;
#36846=CARTESIAN_POINT('Ctrl Pts',(-20.5206272668833,25.3408122757461,123.880023760585)) ;
#36847=CARTESIAN_POINT('Ctrl Pts',(-20.7984664180072,25.1608231953363,123.997081667637)) ;
#36848=CARTESIAN_POINT('Ctrl Pts',(-20.4227342551937,25.3507953238871,124.065699360491)) ;
#36849=CARTESIAN_POINT('Ctrl Pts',(-20.6760989907046,25.1708062434773,124.229175844489)) ;
#36850=CARTESIAN_POINT('Ctrl Pts',(-20.2930330978776,25.3608390314972,124.232290893968)) ;
#36851=CARTESIAN_POINT('Ctrl Pts',(-20.5139718407588,25.1808499510873,124.437414474458)) ;
#36852=CARTESIAN_POINT('Ctrl Pts',(-20.1400132496701,25.3706677246505,124.3711852769)) ;
#36853=CARTESIAN_POINT('Ctrl Pts',(-20.3226951495679,25.1906786442406,124.611032523196)) ;
#36854=CARTESIAN_POINT('Ctrl Pts',(-19.9609525577094,25.3807424737799,124.484253952446)) ;
#36855=CARTESIAN_POINT('Ctrl Pts',(-20.098868954163,25.2007533933701,124.752367074703)) ;
#36856=CARTESIAN_POINT('Ctrl Pts',(-19.7689867735879,25.3906077995755,124.56282261199)) ;
#36857=CARTESIAN_POINT('Ctrl Pts',(-19.8589101906674,25.2106187191656,124.850577176183)) ;
#36858=CARTESIAN_POINT('Ctrl Pts',(-19.5632165090055,25.4006299739324,124.608087313352)) ;
#36859=CARTESIAN_POINT('Ctrl Pts',(-19.6016970937492,25.2206408935226,124.907156637962)) ;
#36860=CARTESIAN_POINT('Ctrl Pts',(-19.3525876909076,25.4106560271393,124.616422421431)) ;
#36861=CARTESIAN_POINT('Ctrl Pts',(-19.3384110920263,25.2306669467295,124.917574265038)) ;
#36862=CARTESIAN_POINT('Ctrl Pts',(-19.147287360646,25.4205097239856,124.588883432483)) ;
#36863=CARTESIAN_POINT('Ctrl Pts',(-19.0817846505266,25.2405206435758,124.883149004146)) ;
#36864=CARTESIAN_POINT('Ctrl Pts',(-18.9475566685195,25.4304691287386,124.526036690547)) ;
#36865=CARTESIAN_POINT('Ctrl Pts',(-18.8321213569648,25.2504800483288,124.804588928361)) ;
#36866=CARTESIAN_POINT('Ctrl Pts',(-18.7604916580374,25.4405073744435,124.428375640314)) ;
#36867=CARTESIAN_POINT('Ctrl Pts',(-18.5982908950079,25.2605182940336,124.682511380087)) ;
#36868=CARTESIAN_POINT('Ctrl Pts',(-18.5957013870381,25.4503815586055,124.302092265061)) ;
#36869=CARTESIAN_POINT('Ctrl Pts',(-18.3923032184269,25.2703924781957,124.524655280028)) ;
#36870=CARTESIAN_POINT('Ctrl Pts',(-18.4526055536538,25.4604513417434,124.146119088409)) ;
#36871=CARTESIAN_POINT('Ctrl Pts',(-18.2134348353702,25.2804622613336,124.329687992467)) ;
#36872=CARTESIAN_POINT('Ctrl Pts',(-18.3413212778129,25.4702845967642,123.971882300025)) ;
#36873=CARTESIAN_POINT('Ctrl Pts',(-18.0743301698289,25.2902955163544,124.111890051022)) ;
#36874=CARTESIAN_POINT('Ctrl Pts',(-18.2598482943526,25.4803150228959,123.777393425404)) ;
#36875=CARTESIAN_POINT('Ctrl Pts',(-17.9724906535457,25.300325942486,123.868778335206)) ;
#36876=CARTESIAN_POINT('Ctrl Pts',(-18.2139714522043,25.4903466350829,123.571535696539)) ;
#36877=CARTESIAN_POINT('Ctrl Pts',(-17.91514620018,25.3103575546731,123.611455902994)) ;
#36878=CARTESIAN_POINT('Ctrl Pts',(-18.2042958256806,25.5001763319375,123.365125390913)) ;
#36879=CARTESIAN_POINT('Ctrl Pts',(-17.9030533677923,25.3201872515277,123.353441667696)) ;
#36880=CARTESIAN_POINT('Ctrl Pts',(-18.2304147172978,25.51016577384,123.156740327135)) ;
#36881=CARTESIAN_POINT('Ctrl Pts',(-17.9357039465611,25.3301766934301,123.092960405567)) ;
#36882=CARTESIAN_POINT('Ctrl Pts',(-18.2931661314917,25.5202096658556,122.955127632222)) ;
#36883=CARTESIAN_POINT('Ctrl Pts',(-18.0141448809972,25.3402205854458,122.840945210774)) ;
#36884=CARTESIAN_POINT('Ctrl Pts',(-18.3874495319765,25.5300312276249,122.771432509652)) ;
#36885=CARTESIAN_POINT('Ctrl Pts',(-18.1320014122623,25.3500421472151,122.61132607428)) ;
#36886=CARTESIAN_POINT('Ctrl Pts',(-18.5144967250623,25.5400667992491,122.60299121237)) ;
#36887=CARTESIAN_POINT('Ctrl Pts',(-18.2908120041976,25.3600777188393,122.400775785522)) ;
#36888=CARTESIAN_POINT('Ctrl Pts',(-18.669193308683,25.5500960735309,122.459723633636)) ;
#36889=CARTESIAN_POINT('Ctrl Pts',(-18.4841839837609,25.370106993121,122.221692735546)) ;
#36890=CARTESIAN_POINT('Ctrl Pts',(-18.8426660315161,25.5599299106495,122.34725013946)) ;
#36891=CARTESIAN_POINT('Ctrl Pts',(-18.7010269360749,25.3799408302397,122.081101987124)) ;
#36892=CARTESIAN_POINT('Ctrl Pts',(-19.0371487210636,25.5699823067377,122.26458450001)) ;
#36893=CARTESIAN_POINT('Ctrl Pts',(-18.9441309444013,25.3899932263279,121.977771975158)) ;
#36894=CARTESIAN_POINT('Ctrl Pts',(-19.2407432881081,25.5799190736882,122.217749926032)) ;
#36895=CARTESIAN_POINT('Ctrl Pts',(-19.1986250892974,25.3999299932784,121.919230643836)) ;
#36896=CARTESIAN_POINT('Ctrl Pts',(-19.4492836308601,25.5898533086675,122.206441411571)) ;
#36897=CARTESIAN_POINT('Ctrl Pts',(-19.4593011285886,25.4098642282577,121.905097168165)) ;
#36898=CARTESIAN_POINT('Ctrl Pts',(-19.6584731388207,25.5998770719943,122.231868584206)) ;
#36899=CARTESIAN_POINT('Ctrl Pts',(-19.7207877370462,25.4198879915845,121.936883279479)) ;
#36900=CARTESIAN_POINT('Ctrl Pts',(-19.8573510139272,25.6097634133789,122.292244191361)) ;
#36901=CARTESIAN_POINT('Ctrl Pts',(-19.96938514331,25.4297743329691,122.012355109313)) ;
#36902=CARTESIAN_POINT('Ctrl Pts',(-20.0448786077411,25.6197524621459,122.386778679778)) ;
#36903=CARTESIAN_POINT('Ctrl Pts',(-20.2037937296908,25.4397633817361,122.13052536822)) ;
#36904=CARTESIAN_POINT('Ctrl Pts',(-20.2137531182518,25.6297936828433,122.513441376923)) ;
#36905=CARTESIAN_POINT('Ctrl Pts',(-20.4148854639399,25.4498046024334,122.288855457057)) ;
#36906=CARTESIAN_POINT('Ctrl Pts',(-20.3553169833918,25.6396263230212,122.664067992544)) ;
#36907=CARTESIAN_POINT('Ctrl Pts',(-20.5918392756483,25.4596372426114,122.47714100209)) ;
#36908=CARTESIAN_POINT('Ctrl Pts',(-20.4709395710573,25.6496202523291,122.839494815761)) ;
#36909=CARTESIAN_POINT('Ctrl Pts',(-20.7363655380305,25.4696311719193,122.696425976551)) ;
#36910=CARTESIAN_POINT('Ctrl Pts',(-20.5542313166204,25.6596494600097,123.033193067616)) ;
#36911=CARTESIAN_POINT('Ctrl Pts',(-20.8404780633485,25.4796603795999,122.938549694625)) ;
#36912=CARTESIAN_POINT('Ctrl Pts',(-20.6022166705038,25.6695252717138,123.235204192602)) ;
#36913=CARTESIAN_POINT('Ctrl Pts',(-20.9004575631495,25.489536191304,123.191064817274)) ;
#36914=CARTESIAN_POINT('Ctrl Pts',(-20.6147777399099,25.6795244986852,123.445015641522)) ;
#36915=CARTESIAN_POINT('Ctrl Pts',(-20.9161564442724,25.4995354182754,123.453329386863)) ;
#36916=CARTESIAN_POINT('Ctrl Pts',(-20.5911250967984,25.6894339798409,123.652027739966)) ;
#36917=CARTESIAN_POINT('Ctrl Pts',(-20.8865881010468,25.5094448994311,123.71209469823)) ;
#36918=CARTESIAN_POINT('Ctrl Pts',(-20.531017224915,25.6994872101418,123.854627589131)) ;
#36919=CARTESIAN_POINT('Ctrl Pts',(-20.8114508926531,25.519498129732,123.965343699731)) ;
#36920=CARTESIAN_POINT('Ctrl Pts',(-20.4384325667578,25.7093578266928,124.040355450809)) ;
#36921=CARTESIAN_POINT('Ctrl Pts',(-20.6957175422726,25.529368746283,124.197502953575)) ;
#36922=CARTESIAN_POINT('Ctrl Pts',(-20.3135029459365,25.7193794884249,124.210003208649)) ;
#36923=CARTESIAN_POINT('Ctrl Pts',(-20.5395534187426,25.539390408015,124.409561109436)) ;
#36924=CARTESIAN_POINT('Ctrl Pts',(-20.1606542811385,25.729402301606,124.355058412312)) ;
#36925=CARTESIAN_POINT('Ctrl Pts',(-20.3484908449699,25.5494132211962,124.590878299878)) ;
#36926=CARTESIAN_POINT('Ctrl Pts',(-19.9878788008662,25.7392694660659,124.469843004655)) ;
#36927=CARTESIAN_POINT('Ctrl Pts',(-20.1325195803548,25.5592803856561,124.734357216865)) ;
#36928=CARTESIAN_POINT('Ctrl Pts',(-19.7955437673314,25.7492629082859,124.554394992238)) ;
#36929=CARTESIAN_POINT('Ctrl Pts',(-19.8920996177398,25.569273827876,124.840044812228)) ;
#36930=CARTESIAN_POINT('Ctrl Pts',(-19.5905777687678,25.7592945818862,124.604056660559)) ;
#36931=CARTESIAN_POINT('Ctrl Pts',(-19.6358915111291,25.5793055014764,124.902119378394)) ;
#36932=CARTESIAN_POINT('Ctrl Pts',(-19.3835799225067,25.7691610169992,124.617474520566)) ;
#36933=CARTESIAN_POINT('Ctrl Pts',(-19.3771435134403,25.5891719365894,124.918889100864)) ;
#36934=CARTESIAN_POINT('Ctrl Pts',(-19.1748644935385,25.7791484675323,124.594811648332)) ;
#36935=CARTESIAN_POINT('Ctrl Pts',(-19.1162493957919,25.5991593871224,124.890557819101)) ;
#36936=CARTESIAN_POINT('Ctrl Pts',(-18.9740276761385,25.7890933973602,124.536594188768)) ;
#36937=CARTESIAN_POINT('Ctrl Pts',(-18.8652039002505,25.6091043169504,124.817783333107)) ;
#36938=CARTESIAN_POINT('Ctrl Pts',(-18.7845612887665,25.7991382924153,124.443378041818)) ;
#36939=CARTESIAN_POINT('Ctrl Pts',(-18.6283721225414,25.6191492120055,124.701260743768)) ;
#36940=CARTESIAN_POINT('Ctrl Pts',(-18.6171242290503,25.8090003541012,124.321077049524)) ;
#36941=CARTESIAN_POINT('Ctrl Pts',(-18.4190770494623,25.6290112736914,124.5483820594)) ;
#36942=CARTESIAN_POINT('Ctrl Pts',(-18.4712964694787,25.818992076888,124.169910090686)) ;
#36943=CARTESIAN_POINT('Ctrl Pts',(-18.2367942708483,25.6390029964782,124.359421375192)) ;
#36944=CARTESIAN_POINT('Ctrl Pts',(-18.3546829235641,25.828924291128,123.996697923502)) ;
#36945=CARTESIAN_POINT('Ctrl Pts',(-18.0910294951363,25.6489352107182,124.142904444587)) ;
#36946=CARTESIAN_POINT('Ctrl Pts',(-18.269414013462,25.8388636096937,123.805925409421)) ;
#36947=CARTESIAN_POINT('Ctrl Pts',(-17.9844458362776,25.6588745292839,123.904437503989)) ;
#36948=CARTESIAN_POINT('Ctrl Pts',(-18.2182183799845,25.8489077844696,123.601068446955)) ;
#36949=CARTESIAN_POINT('Ctrl Pts',(-17.9204539830974,25.6689187040598,123.648365609481)) ;
#36950=CARTESIAN_POINT('Ctrl Pts',(-18.2035144290787,25.8587783385346,123.394080423168)) ;
#36951=CARTESIAN_POINT('Ctrl Pts',(-17.9020768057529,25.6787892581248,123.389630116783)) ;
#36952=CARTESIAN_POINT('Ctrl Pts',(-18.2245755858917,25.8687433208888,123.185646036697)) ;
#36953=CARTESIAN_POINT('Ctrl Pts',(-17.9284060680504,25.6887542404789,123.129087322385)) ;
#36954=CARTESIAN_POINT('Ctrl Pts',(-18.2821927216553,25.8787740237786,122.982799143705)) ;
#36955=CARTESIAN_POINT('Ctrl Pts',(-18.0004301996435,25.6987849433688,122.875529417098)) ;
#36956=CARTESIAN_POINT('Ctrl Pts',(-18.3726282398812,25.8886663638038,122.795495732635)) ;
#36957=CARTESIAN_POINT('Ctrl Pts',(-18.113477198808,25.708677283394,122.641401239068)) ;
#36958=CARTESIAN_POINT('Ctrl Pts',(-18.4961390189177,25.8987195969637,122.624026714153)) ;
#36959=CARTESIAN_POINT('Ctrl Pts',(-18.2678679862783,25.7187305165539,122.427066576794)) ;
#36960=CARTESIAN_POINT('Ctrl Pts',(-18.6449144456404,25.9086008414405,122.478993547401)) ;
#36961=CARTESIAN_POINT('Ctrl Pts',(-18.4538393268048,25.7286117610307,122.245777047837)) ;
#36962=CARTESIAN_POINT('Ctrl Pts',(-18.8191018734821,25.9186339623115,122.36011093306)) ;
#36963=CARTESIAN_POINT('Ctrl Pts',(-18.6715752592843,25.7386448819017,122.097176077523)) ;
#36964=CARTESIAN_POINT('Ctrl Pts',(-19.0083693285525,25.9285151725866,122.274392628594)) ;
#36965=CARTESIAN_POINT('Ctrl Pts',(-18.9081608032802,25.7485260921767,121.990030737778)) ;
#36966=CARTESIAN_POINT('Ctrl Pts',(-19.2132442732851,25.9385772483559,122.221858172896)) ;
#36967=CARTESIAN_POINT('Ctrl Pts',(-19.1642552672719,25.7585881679461,121.924365385108)) ;
#36968=CARTESIAN_POINT('Ctrl Pts',(-19.41988850403,25.9484343067377,122.205946244502)) ;
#36969=CARTESIAN_POINT('Ctrl Pts',(-19.4225607860538,25.7684452263278,121.904478285309)) ;
#36970=CARTESIAN_POINT('Ctrl Pts',(-19.6290114818218,25.9584288620267,122.226010291668)) ;
#36971=CARTESIAN_POINT('Ctrl Pts',(-19.6839642883696,25.7784397816168,121.929561151794)) ;
#36972=CARTESIAN_POINT('Ctrl Pts',(-19.8301627349406,25.9683547495622,122.281640275295)) ;
#36973=CARTESIAN_POINT('Ctrl Pts',(-19.9354025959097,25.7883656691523,121.99910133033)) ;
#36974=CARTESIAN_POINT('Ctrl Pts',(-20.0204672700362,25.9783797695574,122.372173587935)) ;
#36975=CARTESIAN_POINT('Ctrl Pts',(-20.1732821454696,25.7983906891476,122.112270545076)) ;
#36976=CARTESIAN_POINT('Ctrl Pts',(-20.1900359400144,25.9882771466611,122.492771224812)) ;
#36977=CARTESIAN_POINT('Ctrl Pts',(-20.3852412940492,25.8082880662513,122.26301982618)) ;
#36978=CARTESIAN_POINT('Ctrl Pts',(-20.3377857345997,25.998267383742,122.642047679255)) ;
#36979=CARTESIAN_POINT('Ctrl Pts',(-20.5699265940413,25.8182783033321,122.449617357503)) ;
#36980=CARTESIAN_POINT('Ctrl Pts',(-20.4575881124741,26.0083039965508,122.815736066675)) ;
#36981=CARTESIAN_POINT('Ctrl Pts',(-20.7196773405348,25.828314916141,122.66672955988)) ;
#36982=CARTESIAN_POINT('Ctrl Pts',(-20.5440893195705,26.0181538799688,123.003887825492)) ;
#36983=CARTESIAN_POINT('Ctrl Pts',(-20.8278012350938,25.838164799559,122.901920139977)) ;
#36984=CARTESIAN_POINT('Ctrl Pts',(-20.5978286138219,26.0281574968712,123.207191914562)) ;
#36985=CARTESIAN_POINT('Ctrl Pts',(-20.8949727103814,25.8481684164614,123.156051177418)) ;
#36986=CARTESIAN_POINT('Ctrl Pts',(-20.6153163617937,26.0381469086364,123.416505710601)) ;
#36987=CARTESIAN_POINT('Ctrl Pts',(-20.9168297434184,25.8581578282265,123.417692998704)) ;
#36988=CARTESIAN_POINT('Ctrl Pts',(-20.5960135788333,26.0481656699812,123.626222930686)) ;
#36989=CARTESIAN_POINT('Ctrl Pts',(-20.8926982525925,25.8681765895714,123.679841956344)) ;
#36990=CARTESIAN_POINT('Ctrl Pts',(-20.5232631932467,26.0613843453623,123.894483327193)) ;
#36991=CARTESIAN_POINT('Ctrl Pts',(-20.8017581312265,25.8813952649524,124.015153473763)) ;
#36992=CARTESIAN_POINT('Ctrl Pts',(-20.3813483402664,26.074694652607,124.13929149955)) ;
#36993=CARTESIAN_POINT('Ctrl Pts',(-20.624392002949,25.8947055721972,124.32113343049)) ;
#36994=CARTESIAN_POINT('Ctrl Pts',(-20.1842168943985,26.087932318833,124.335713981098)) ;
#36995=CARTESIAN_POINT('Ctrl Pts',(-20.3779377393068,25.9079432384232,124.566705392329)) ;
#36996=CARTESIAN_POINT('Ctrl Pts',(-20.0135494311699,26.0978520142437,124.455575991443)) ;
#36997=CARTESIAN_POINT('Ctrl Pts',(-20.164609841779,25.9178629338339,124.716521317897)) ;
#36998=CARTESIAN_POINT('Ctrl Pts',(-19.8220452045287,26.1079048812422,124.544939686849)) ;
#36999=CARTESIAN_POINT('Ctrl Pts',(-19.9252257841206,25.9279158008324,124.828226044288)) ;
#37000=CARTESIAN_POINT('Ctrl Pts',(-19.6219710853917,26.1177602895715,124.598853822715)) ;
#37001=CARTESIAN_POINT('Ctrl Pts',(-19.675135063597,25.9377712091617,124.895616007235)) ;
#37002=CARTESIAN_POINT('Ctrl Pts',(-19.4118059045154,26.1277989212481,124.617896062361)) ;
#37003=CARTESIAN_POINT('Ctrl Pts',(-19.4124225556357,25.9478098408382,124.919414322687)) ;
#37004=CARTESIAN_POINT('Ctrl Pts',(-19.1331380537758,26.1411011035151,124.594040851199)) ;
#37005=CARTESIAN_POINT('Ctrl Pts',(-19.0641152659806,25.9611120231053,124.889602890064)) ;
#37006=CARTESIAN_POINT('Ctrl Pts',(-18.8021064780862,26.157646116598,124.475037573678)) ;
#37007=CARTESIAN_POINT('Ctrl Pts',(-18.6502847526596,25.9776570361881,124.74081980976)) ;
#37008=CARTESIAN_POINT('Ctrl Pts',(-18.5297345481408,26.1742981326742,124.248799717429)) ;
#37009=CARTESIAN_POINT('Ctrl Pts',(-18.3098802866358,25.9943090522644,124.458074394321)) ;
#37010=CARTESIAN_POINT('Ctrl Pts',(-18.369098727454,26.1875212235794,124.021942776296)) ;
#37011=CARTESIAN_POINT('Ctrl Pts',(-18.1090436807986,26.0075321431696,124.174455573263)) ;
#37012=CARTESIAN_POINT('Ctrl Pts',(-18.2790691456165,26.1974821831388,123.832864887124)) ;
#37013=CARTESIAN_POINT('Ctrl Pts',(-17.9965176539115,26.0174931027289,123.938117510203)) ;
#37014=CARTESIAN_POINT('Ctrl Pts',(-18.2231373596907,26.2075069798899,123.629678729636)) ;
#37015=CARTESIAN_POINT('Ctrl Pts',(-17.9266031350855,26.0275178994801,123.684128675008)) ;
#37016=CARTESIAN_POINT('Ctrl Pts',(-18.19662185451,26.2207314272857,123.352884992182)) ;
#37017=CARTESIAN_POINT('Ctrl Pts',(-17.8934600553599,26.0407423468759,123.338151922394)) ;
#37018=CARTESIAN_POINT('Ctrl Pts',(-18.2547370627252,26.2373652119848,123.004073948381)) ;
#37019=CARTESIAN_POINT('Ctrl Pts',(-17.966109897948,26.0573761315749,122.902122581891)) ;
#37020=CARTESIAN_POINT('Ctrl Pts',(-18.4626485183739,26.2572678787097,122.635440004849)) ;
#37021=CARTESIAN_POINT('Ctrl Pts',(-18.2260016701875,26.0772787982999,122.441338078441)) ;
#37022=CARTESIAN_POINT('Ctrl Pts',(-18.7834207710504,26.2771681064916,122.359539756273)) ;
#37023=CARTESIAN_POINT('Ctrl Pts',(-18.6269689740225,26.0971790260817,122.096464789872)) ;
#37024=CARTESIAN_POINT('Ctrl Pts',(-19.1793519772945,26.2970855940231,122.209249706673)) ;
#37025=CARTESIAN_POINT('Ctrl Pts',(-19.1218834344453,26.1170965136132,121.908606135726)) ;
#37026=CARTESIAN_POINT('Ctrl Pts',(-19.60307943523,26.31701511984,122.202825724999)) ;
#37027=CARTESIAN_POINT('Ctrl Pts',(-19.6515421009245,26.1370260394302,121.900579249944)) ;
#37028=CARTESIAN_POINT('Ctrl Pts',(-20.004197714649,26.3369773877262,122.341686788595)) ;
#37029=CARTESIAN_POINT('Ctrl Pts',(-20.152938612381,26.1569883073164,122.074158377554)) ;
#37030=CARTESIAN_POINT('Ctrl Pts',(-20.3326211942537,26.3568675826784,122.608053388485)) ;
#37031=CARTESIAN_POINT('Ctrl Pts',(-20.5634651728488,26.1768785022686,122.407118082676)) ;
#37032=CARTESIAN_POINT('Ctrl Pts',(-20.5514266364284,26.3767578274247,122.970081973903)) ;
#37033=CARTESIAN_POINT('Ctrl Pts',(-20.8369695351396,26.1967687470149,122.85965377227)) ;
#37034=CARTESIAN_POINT('Ctrl Pts',(-20.6334217410706,26.3968321999872,123.388909430167)) ;
#37035=CARTESIAN_POINT('Ctrl Pts',(-20.9394612389144,26.2168431195774,123.383189522099)) ;
#37036=CARTESIAN_POINT('Ctrl Pts',(-20.5686369856693,26.4166175773475,123.804638740479)) ;
#37037=CARTESIAN_POINT('Ctrl Pts',(-20.8584786210776,26.2366284969377,123.902848054714)) ;
#37038=CARTESIAN_POINT('Ctrl Pts',(-20.3652722304398,26.4365794514146,124.177147234351)) ;
#37039=CARTESIAN_POINT('Ctrl Pts',(-20.6042720421634,26.2565903710048,124.368482650249)) ;
#37040=CARTESIAN_POINT('Ctrl Pts',(-20.0459994667024,26.4565594269051,124.457421972499)) ;
#37041=CARTESIAN_POINT('Ctrl Pts',(-20.205180240238,26.2765703464953,124.71882479519)) ;
#37042=CARTESIAN_POINT('Ctrl Pts',(-19.6538522670745,26.476371856783,124.611397902099)) ;
#37043=CARTESIAN_POINT('Ctrl Pts',(-19.7149987089406,26.2963827763732,124.911292999906)) ;
#37044=CARTESIAN_POINT('Ctrl Pts',(-19.2292568239862,26.4963519648733,124.622952036836)) ;
#37045=CARTESIAN_POINT('Ctrl Pts',(-19.1842547999706,26.3163628844635,124.925735636697)) ;
#37046=CARTESIAN_POINT('Ctrl Pts',(-18.8278291774401,26.5162463484706,124.489264756815)) ;
#37047=CARTESIAN_POINT('Ctrl Pts',(-18.6824717518565,26.3362572680608,124.758627144379)) ;
#37048=CARTESIAN_POINT('Ctrl Pts',(-18.4954865718006,26.5361732764478,124.226604674122)) ;
#37049=CARTESIAN_POINT('Ctrl Pts',(-18.267043998799,26.356184196038,124.430303289981)) ;
#37050=CARTESIAN_POINT('Ctrl Pts',(-18.2725029600721,26.556068133749,123.867014296754)) ;
#37051=CARTESIAN_POINT('Ctrl Pts',(-17.9883141682821,26.3760790533392,123.98081722358)) ;
#37052=CARTESIAN_POINT('Ctrl Pts',(-18.1854325985899,26.5761073273527,123.449960855483)) ;
#37053=CARTESIAN_POINT('Ctrl Pts',(-17.8794749234903,26.3961182469429,123.459500138787)) ;
#37054=CARTESIAN_POINT('Ctrl Pts',(-18.2454084367871,26.5959472952634,123.032350538864)) ;
#37055=CARTESIAN_POINT('Ctrl Pts',(-17.9544430375699,26.4159582148536,122.937489228137)) ;
#37056=CARTESIAN_POINT('Ctrl Pts',(-18.4440381416904,26.6158621122275,122.658424632547)) ;
#37057=CARTESIAN_POINT('Ctrl Pts',(-18.2027276436478,26.4358730318177,122.470081707815)) ;
#37058=CARTESIAN_POINT('Ctrl Pts',(-18.75897849637,26.6358043576238,122.374552553596)) ;
#37059=CARTESIAN_POINT('Ctrl Pts',(-18.5964009950836,26.455815277214,122.11524037907)) ;
#37060=CARTESIAN_POINT('Ctrl Pts',(-19.1503485290493,26.6556764057383,122.215041816388)) ;
#37061=CARTESIAN_POINT('Ctrl Pts',(-19.0856111707596,26.4756873253285,121.915849802036)) ;
#37062=CARTESIAN_POINT('Ctrl Pts',(-19.5753925439647,26.6756874706924,122.198865355149)) ;
#37063=CARTESIAN_POINT('Ctrl Pts',(-19.616916168293,26.4956983902826,121.895626311557)) ;
#37064=CARTESIAN_POINT('Ctrl Pts',(-19.9769190829482,26.695498994996,122.326876472295)) ;
#37065=CARTESIAN_POINT('Ctrl Pts',(-20.118823655728,26.5155099145862,122.055636433921)) ;
#37066=CARTESIAN_POINT('Ctrl Pts',(-20.3149929284387,26.7155942069594,122.58789233349)) ;
#37067=CARTESIAN_POINT('Ctrl Pts',(-20.5414187887215,26.5356051265496,122.381904092587)) ;
#37068=CARTESIAN_POINT('Ctrl Pts',(-20.5402392709743,26.7353749308792,122.943283604957)) ;
#37069=CARTESIAN_POINT('Ctrl Pts',(-20.8229786363096,26.5553858504693,122.826139617784)) ;
#37070=CARTESIAN_POINT('Ctrl Pts',(-20.6325355714334,26.755366006522,123.358044401428)) ;
#37071=CARTESIAN_POINT('Ctrl Pts',(-20.9383530389169,26.5753769261122,123.344589665561)) ;
#37072=CARTESIAN_POINT('Ctrl Pts',(-20.5777323731222,26.775247945565,123.777341421288)) ;
#37073=CARTESIAN_POINT('Ctrl Pts',(-20.8698532062962,26.5952588651552,123.868710610719)) ;
#37074=CARTESIAN_POINT('Ctrl Pts',(-20.3829509016501,26.7952005500682,124.154152656679)) ;
#37075=CARTESIAN_POINT('Ctrl Pts',(-20.6263804834171,26.6152114696584,124.339726432441)) ;
#37076=CARTESIAN_POINT('Ctrl Pts',(-20.0720296957647,26.8150994187989,124.441175273159)) ;
#37077=CARTESIAN_POINT('Ctrl Pts',(-20.237732360991,26.6351103383891,124.69850747848)) ;
#37078=CARTESIAN_POINT('Ctrl Pts',(-19.682246570693,26.8349928186085,124.605258451714)) ;
#37079=CARTESIAN_POINT('Ctrl Pts',(-19.7505063847468,26.6550037381987,124.90361609291)) ;
#37080=CARTESIAN_POINT('Ctrl Pts',(-19.2594063736317,26.8549019494485,124.627157490124)) ;
#37081=CARTESIAN_POINT('Ctrl Pts',(-19.2219548120754,26.6749128690387,124.930993209618)) ;
#37082=CARTESIAN_POINT('Ctrl Pts',(-18.8522665349481,26.8749340492121,124.502164719981)) ;
#37083=CARTESIAN_POINT('Ctrl Pts',(-18.7130356341948,26.6949449688022,124.774763267503)) ;
#37084=CARTESIAN_POINT('Ctrl Pts',(-18.5715001351461,26.8914661223815,124.290581364288)) ;
#37085=CARTESIAN_POINT('Ctrl Pts',(-18.362052855483,26.7114770419717,124.510268121251)) ;
#37086=CARTESIAN_POINT('Ctrl Pts',(-18.3986933822299,26.9048014629875,124.069844703011)) ;
#37087=CARTESIAN_POINT('Ctrl Pts',(-18.1460617746842,26.7248123825776,124.234367496559)) ;
#37088=CARTESIAN_POINT('Ctrl Pts',(-18.3010328118348,26.9146440215272,123.887397849221)) ;
#37089=CARTESIAN_POINT('Ctrl Pts',(-18.0239800546403,26.7346549411174,124.006303612816)) ;
#37090=CARTESIAN_POINT('Ctrl Pts',(-18.234968179349,26.9246959283771,123.68668524791)) ;
#37091=CARTESIAN_POINT('Ctrl Pts',(-17.9413973813145,26.7447068479673,123.755428033615)) ;
#37092=CARTESIAN_POINT('Ctrl Pts',(-18.1952008801186,26.937944442768,123.411026766241)) ;
#37093=CARTESIAN_POINT('Ctrl Pts',(-17.8916861491589,26.7579553623582,123.410787353361)) ;
#37094=CARTESIAN_POINT('Ctrl Pts',(-18.2364062598888,26.9545436177157,123.060472721167)) ;
#37095=CARTESIAN_POINT('Ctrl Pts',(-17.9431815126831,26.7745545373059,122.972680824435)) ;
#37096=CARTESIAN_POINT('Ctrl Pts',(-18.3945264788303,26.9711324035108,122.745229733751)) ;
#37097=CARTESIAN_POINT('Ctrl Pts',(-18.1408483241841,26.791143323101,122.578566000218)) ;
#37098=CARTESIAN_POINT('Ctrl Pts',(-18.5797786495349,26.9844082198528,122.536429267407)) ;
#37099=CARTESIAN_POINT('Ctrl Pts',(-18.37239268425,26.8044191394429,122.31759864417)) ;
#37100=CARTESIAN_POINT('Ctrl Pts',(-18.7438802886562,26.9943820706466,122.405894110244)) ;
#37101=CARTESIAN_POINT('Ctrl Pts',(-18.5775216542412,26.8143929902368,122.154420338584)) ;
#37102=CARTESIAN_POINT('Ctrl Pts',(-18.929271898675,27.004411102739,122.305482739616)) ;
#37103=CARTESIAN_POINT('Ctrl Pts',(-18.8092589677478,26.8244220223292,122.028905565385)) ;
#37104=CARTESIAN_POINT('Ctrl Pts',(-19.1264590553554,27.0143012282409,122.239497823847)) ;
#37105=CARTESIAN_POINT('Ctrl Pts',(-19.0557421895027,26.834312147831,121.946421302881)) ;
#37106=CARTESIAN_POINT('Ctrl Pts',(-19.3341576766828,27.0242937065124,122.208161049022)) ;
#37107=CARTESIAN_POINT('Ctrl Pts',(-19.3153650354492,26.8443046261026,121.907247691333)) ;
#37108=CARTESIAN_POINT('Ctrl Pts',(-19.5433352481452,27.0342449216098,122.213230891029)) ;
#37109=CARTESIAN_POINT('Ctrl Pts',(-19.5768371046755,26.8542558412,121.913582155123)) ;
#37110=CARTESIAN_POINT('Ctrl Pts',(-19.7503716423327,27.0442934233648,122.255105192578)) ;
#37111=CARTESIAN_POINT('Ctrl Pts',(-19.8356332457504,26.864304342955,121.965922317527)) ;
#37112=CARTESIAN_POINT('Ctrl Pts',(-19.9430662208723,27.0541347729816,122.330491998155)) ;
#37113=CARTESIAN_POINT('Ctrl Pts',(-20.0765024472535,26.8741456925718,122.060153189974)) ;
#37114=CARTESIAN_POINT('Ctrl Pts',(-20.1225333341149,27.0641210640018,122.439364927213)) ;
#37115=CARTESIAN_POINT('Ctrl Pts',(-20.300837872544,26.884131983592,122.196241979988)) ;
#37116=CARTESIAN_POINT('Ctrl Pts',(-20.2797057557656,27.0740576757304,122.57702448676)) ;
#37117=CARTESIAN_POINT('Ctrl Pts',(-20.4973053063257,26.8940685953206,122.368314358349)) ;
#37118=CARTESIAN_POINT('Ctrl Pts',(-20.4119625359954,27.084107551098,122.74176172172)) ;
#37119=CARTESIAN_POINT('Ctrl Pts',(-20.6626285188084,26.9041184706882,122.574234184179)) ;
#37120=CARTESIAN_POINT('Ctrl Pts',(-20.5117431177263,27.0939580096334,122.92324291587)) ;
#37121=CARTESIAN_POINT('Ctrl Pts',(-20.787356768741,26.9139689292236,122.801084418364)) ;
#37122=CARTESIAN_POINT('Ctrl Pts',(-20.579826322129,27.1039299465862,123.121493753205)) ;
#37123=CARTESIAN_POINT('Ctrl Pts',(-20.8724634669846,26.9239408661763,123.048897162367)) ;
#37124=CARTESIAN_POINT('Ctrl Pts',(-20.6125055315077,27.1139254035183,123.329105646214)) ;
#37125=CARTESIAN_POINT('Ctrl Pts',(-20.9133152578659,26.9339363231085,123.308411671267)) ;
#37126=CARTESIAN_POINT('Ctrl Pts',(-20.6083877682446,27.1239582105714,123.539972730989)) ;
#37127=CARTESIAN_POINT('Ctrl Pts',(-20.9081708679843,26.9439691301615,123.571995622516)) ;
#37128=CARTESIAN_POINT('Ctrl Pts',(-20.5686916631752,27.1338180971613,123.743433100123)) ;
#37129=CARTESIAN_POINT('Ctrl Pts',(-20.8585534427994,26.9538290167515,123.826321841981)) ;
#37130=CARTESIAN_POINT('Ctrl Pts',(-20.4936737353725,27.1438071777266,123.939559222509)) ;
#37131=CARTESIAN_POINT('Ctrl Pts',(-20.7647835916082,26.9638180973167,124.07148059007)) ;
#37132=CARTESIAN_POINT('Ctrl Pts',(-20.3863494619409,27.1537386569357,124.118661541936)) ;
#37133=CARTESIAN_POINT('Ctrl Pts',(-20.6306305350596,26.9737495765259,124.295360078416)) ;
#37134=CARTESIAN_POINT('Ctrl Pts',(-20.2490645865285,27.1637245163817,124.277504970353)) ;
#37135=CARTESIAN_POINT('Ctrl Pts',(-20.459026445873,26.9837354359718,124.493916247304)) ;
#37136=CARTESIAN_POINT('Ctrl Pts',(-20.0852193557923,27.1737626670289,124.410486117788)) ;
#37137=CARTESIAN_POINT('Ctrl Pts',(-20.2542216594621,26.993773586619,124.660144844875)) ;
#37138=CARTESIAN_POINT('Ctrl Pts',(-19.9044415797665,27.1836107575333,124.511442323854)) ;
#37139=CARTESIAN_POINT('Ctrl Pts',(-20.0282504284542,27.0036216771234,124.786342691805)) ;
#37140=CARTESIAN_POINT('Ctrl Pts',(-19.7047523070118,27.1936716660512,124.581101591854)) ;
#37141=CARTESIAN_POINT('Ctrl Pts',(-19.7786397745588,27.0136825856414,124.873419336905)) ;
#37142=CARTESIAN_POINT('Ctrl Pts',(-19.4993833052846,27.2035665132092,124.614334962714)) ;
#37143=CARTESIAN_POINT('Ctrl Pts',(-19.5219286374302,27.0235774327994,124.914963808384)) ;
#37144=CARTESIAN_POINT('Ctrl Pts',(-19.2904166566976,27.2135081852543,124.611948250234)) ;
#37145=CARTESIAN_POINT('Ctrl Pts',(-19.2607200330017,27.0335191048444,124.91198309145)) ;
#37146=CARTESIAN_POINT('Ctrl Pts',(-19.0837134685083,27.2235107123797,124.573148992734)) ;
#37147=CARTESIAN_POINT('Ctrl Pts',(-19.0023404745317,27.0435216319699,124.863486618842)) ;
#37148=CARTESIAN_POINT('Ctrl Pts',(-18.886408762246,27.2335455035672,124.49851245076)) ;
#37149=CARTESIAN_POINT('Ctrl Pts',(-18.755708647679,27.0535564231574,124.770193481256)) ;
#37150=CARTESIAN_POINT('Ctrl Pts',(-18.7082920067272,27.2433903834263,124.393076161983)) ;
#37151=CARTESIAN_POINT('Ctrl Pts',(-18.5330608652643,27.0634013030165,124.638400122034)) ;
#37152=CARTESIAN_POINT('Ctrl Pts',(-18.548717036597,27.2533762640448,124.256715634161)) ;
#37153=CARTESIAN_POINT('Ctrl Pts',(-18.3335903392145,27.073387183635,124.467951336742)) ;
#37154=CARTESIAN_POINT('Ctrl Pts',(-18.415763782662,27.263310987138,124.095588178805)) ;
#37155=CARTESIAN_POINT('Ctrl Pts',(-18.1673965821036,27.0833219067282,124.266543402292)) ;
#37156=CARTESIAN_POINT('Ctrl Pts',(-18.3117355785266,27.2733688274492,123.911537425513)) ;
#37157=CARTESIAN_POINT('Ctrl Pts',(-18.0373591120352,27.0933797470393,124.036481345852)) ;
#37158=CARTESIAN_POINT('Ctrl Pts',(-18.2425753593927,27.2831893148457,123.716980331988)) ;
#37159=CARTESIAN_POINT('Ctrl Pts',(-17.9509061763895,27.1032002344359,123.793285094088)) ;
#37160=CARTESIAN_POINT('Ctrl Pts',(-18.2070714729757,27.2932497161908,123.508505960271)) ;
#37161=CARTESIAN_POINT('Ctrl Pts',(-17.9065238900958,27.113260635781,123.532692664092)) ;
#37162=CARTESIAN_POINT('Ctrl Pts',(-18.2085717097183,27.3031806817437,123.299707474007)) ;
#37163=CARTESIAN_POINT('Ctrl Pts',(-17.9083966529468,27.1231916013339,123.271694164599)) ;
#37164=CARTESIAN_POINT('Ctrl Pts',(-18.2458677394489,27.3131195440802,123.094139009505)) ;
#37165=CARTESIAN_POINT('Ctrl Pts',(-17.955014348972,27.1331304636704,123.014732779551)) ;
#37166=CARTESIAN_POINT('Ctrl Pts',(-18.3185162099704,27.3231052750064,122.897153471792)) ;
#37167=CARTESIAN_POINT('Ctrl Pts',(-18.0458227293061,27.1431161945965,122.768499870835)) ;
#37168=CARTESIAN_POINT('Ctrl Pts',(-18.4248467767158,27.3331296604338,122.715218646708)) ;
#37169=CARTESIAN_POINT('Ctrl Pts',(-18.1787338061825,27.153140580024,122.541080100804)) ;
#37170=CARTESIAN_POINT('Ctrl Pts',(-18.5592899800235,27.3430329447871,122.556213400873)) ;
#37171=CARTESIAN_POINT('Ctrl Pts',(-18.3467863406114,27.1630438643772,122.342321572966)) ;
#37172=CARTESIAN_POINT('Ctrl Pts',(-18.7218362744338,27.3530929493651,122.42094597078)) ;
#37173=CARTESIAN_POINT('Ctrl Pts',(-18.5499675317569,27.1731038689552,122.173235543867)) ;
#37174=CARTESIAN_POINT('Ctrl Pts',(-18.9014128659292,27.3629362184342,122.3180699415)) ;
#37175=CARTESIAN_POINT('Ctrl Pts',(-18.7744378364705,27.1829471380244,122.044638016487)) ;
#37176=CARTESIAN_POINT('Ctrl Pts',(-19.0988286897178,27.3729267840419,122.246443873207)) ;
#37177=CARTESIAN_POINT('Ctrl Pts',(-19.0212070083679,27.192937703632,121.955103241805)) ;
#37178=CARTESIAN_POINT('Ctrl Pts',(-19.3044292359815,27.3828549158207,122.210437107956)) ;
#37179=CARTESIAN_POINT('Ctrl Pts',(-19.2782077784746,27.2028658354109,121.910092465448)) ;
#37180=CARTESIAN_POINT('Ctrl Pts',(-19.5144154098307,27.3928428029016,122.21031147887)) ;
#37181=CARTESIAN_POINT('Ctrl Pts',(-19.5406906769482,27.2128537224918,121.909933250566)) ;
#37182=CARTESIAN_POINT('Ctrl Pts',(-19.7221490194526,27.4028787524703,122.247173181467)) ;
#37183=CARTESIAN_POINT('Ctrl Pts',(-19.800358000924,27.2228896720605,121.956008126959)) ;
#37184=CARTESIAN_POINT('Ctrl Pts',(-19.916892573696,27.4127336388491,122.317923368138)) ;
#37185=CARTESIAN_POINT('Ctrl Pts',(-20.0437890491304,27.2327445584393,122.044444124132)) ;
#37186=CARTESIAN_POINT('Ctrl Pts',(-20.0991236220355,27.422733053197,122.422656802109)) ;
#37187=CARTESIAN_POINT('Ctrl Pts',(-20.2715790260857,27.2427439727872,122.17535915605)) ;
#37188=CARTESIAN_POINT('Ctrl Pts',(-20.2589164113812,27.4326282183875,122.555908904654)) ;
#37189=CARTESIAN_POINT('Ctrl Pts',(-20.4713218816854,27.2526391379776,122.341923187098)) ;
#37190=CARTESIAN_POINT('Ctrl Pts',(-20.3953279566597,27.4426885370794,122.71750152297)) ;
#37191=CARTESIAN_POINT('Ctrl Pts',(-20.641837725394,27.2626994566696,122.543912452702)) ;
#37192=CARTESIAN_POINT('Ctrl Pts',(-20.4995174983559,27.4525386688555,122.896483303571)) ;
#37193=CARTESIAN_POINT('Ctrl Pts',(-20.7720769169052,27.2725495884457,122.767639568981)) ;
#37194=CARTESIAN_POINT('Ctrl Pts',(-20.5728149864719,27.4625692393058,123.094198738288)) ;
#37195=CARTESIAN_POINT('Ctrl Pts',(-20.8637005069511,27.282580158896,123.014783157518)) ;
#37196=CARTESIAN_POINT('Ctrl Pts',(-20.6101494969086,27.4725833899786,123.301402871192)) ;
#37197=CARTESIAN_POINT('Ctrl Pts',(-20.9103706253092,27.2925943095687,123.273787983247)) ;
#37198=CARTESIAN_POINT('Ctrl Pts',(-20.6112662653975,27.482476323524,123.509383815082)) ;
#37199=CARTESIAN_POINT('Ctrl Pts',(-20.9117684959154,27.3024872431142,123.533764947739)) ;
#37200=CARTESIAN_POINT('Ctrl Pts',(-20.5761521288518,27.4924658375142,123.716418000998)) ;
#37201=CARTESIAN_POINT('Ctrl Pts',(-20.8678776030597,27.3124767571044,123.792558185281)) ;
#37202=CARTESIAN_POINT('Ctrl Pts',(-20.5059891635455,27.5024196081667,123.913596204343)) ;
#37203=CARTESIAN_POINT('Ctrl Pts',(-20.7801754400908,27.3224305277569,124.039031948383)) ;
#37204=CARTESIAN_POINT('Ctrl Pts',(-20.4015400398466,27.5124673768272,124.097177756809)) ;
#37205=CARTESIAN_POINT('Ctrl Pts',(-20.6496157400561,27.3324782964174,124.268509637685)) ;
#37206=CARTESIAN_POINT('Ctrl Pts',(-20.2697294375057,27.522309103267,124.256684479157)) ;
#37207=CARTESIAN_POINT('Ctrl Pts',(-20.4848531001097,27.3423200228572,124.467895083778)) ;
#37208=CARTESIAN_POINT('Ctrl Pts',(-20.1102592973178,27.5322946200898,124.393158289807)) ;
#37209=CARTESIAN_POINT('Ctrl Pts',(-20.2855162963156,27.35230553968,124.638488743921)) ;
#37210=CARTESIAN_POINT('Ctrl Pts',(-19.9303364745535,27.5422339517853,124.499474121132)) ;
#37211=CARTESIAN_POINT('Ctrl Pts',(-20.0606131128691,27.3622448713755,124.771385186878)) ;
#37212=CARTESIAN_POINT('Ctrl Pts',(-19.7327382041188,27.5522737214829,124.573617862549)) ;
#37213=CARTESIAN_POINT('Ctrl Pts',(-19.813615980086,27.3722846410731,124.864066326377)) ;
#37214=CARTESIAN_POINT('Ctrl Pts',(-19.5283912957834,27.5621618827317,124.611847447798)) ;
#37215=CARTESIAN_POINT('Ctrl Pts',(-19.5581817302903,27.3821728023218,124.91185503281)) ;
#37216=CARTESIAN_POINT('Ctrl Pts',(-19.3184025008245,27.5721514372341,124.614431043553)) ;
#37217=CARTESIAN_POINT('Ctrl Pts',(-19.2956955404855,27.3921623568242,124.915085978985)) ;
#37218=CARTESIAN_POINT('Ctrl Pts',(-19.1118246407992,27.5821098517577,124.580462400769)) ;
#37219=CARTESIAN_POINT('Ctrl Pts',(-19.0374725439627,27.4021207713479,124.872626590883)) ;
#37220=CARTESIAN_POINT('Ctrl Pts',(-18.9152594132557,27.5920097645871,124.512023957247)) ;
#37221=CARTESIAN_POINT('Ctrl Pts',(-18.7917647458392,27.4120206841773,124.787079499409)) ;
#37222=CARTESIAN_POINT('Ctrl Pts',(-18.7309264013132,27.602056464237,124.408951439022)) ;
#37223=CARTESIAN_POINT('Ctrl Pts',(-18.5613480077175,27.4220673838271,124.658240132798)) ;
#37224=CARTESIAN_POINT('Ctrl Pts',(-18.5695583676357,27.6119563245426,124.277459812412)) ;
#37225=CARTESIAN_POINT('Ctrl Pts',(-18.3596364545729,27.4319672441327,124.493876043485)) ;
#37226=CARTESIAN_POINT('Ctrl Pts',(-18.4313772500186,27.622007728748,124.117627545932)) ;
#37227=CARTESIAN_POINT('Ctrl Pts',(-18.1869092530332,27.4420186483382,124.294086730382)) ;
#37228=CARTESIAN_POINT('Ctrl Pts',(-18.3247881894919,27.6318887656692,123.939292964072)) ;
#37229=CARTESIAN_POINT('Ctrl Pts',(-18.0536713290619,27.4518996852594,124.071168267652)) ;
#37230=CARTESIAN_POINT('Ctrl Pts',(-18.2496492643862,27.6418885978467,123.742988738701)) ;
#37231=CARTESIAN_POINT('Ctrl Pts',(-17.959746551278,27.4618995174369,123.825788262649)) ;
#37232=CARTESIAN_POINT('Ctrl Pts',(-18.2098807597813,27.6518066008316,123.538271728212)) ;
#37233=CARTESIAN_POINT('Ctrl Pts',(-17.91003471053,27.4718175204217,123.569891459498)) ;
#37234=CARTESIAN_POINT('Ctrl Pts',(-18.2062837040758,27.6618579067061,123.327027887074)) ;
#37235=CARTESIAN_POINT('Ctrl Pts',(-17.9055372819879,27.4818688262963,123.305836914711)) ;
#37236=CARTESIAN_POINT('Ctrl Pts',(-18.2385839581239,27.6717277300977,123.122017781039)) ;
#37237=CARTESIAN_POINT('Ctrl Pts',(-17.9459117764605,27.4917386496878,123.049572996313)) ;
#37238=CARTESIAN_POINT('Ctrl Pts',(-18.307368702007,27.681801896148,122.921759006394)) ;
#37239=CARTESIAN_POINT('Ctrl Pts',(-18.0318915985175,27.5018128157382,122.799249602939)) ;
#37240=CARTESIAN_POINT('Ctrl Pts',(-18.4071173488075,27.6916219802896,122.74095235675)) ;
#37241=CARTESIAN_POINT('Ctrl Pts',(-18.156577349418,27.5116328998798,122.573239483778)) ;
#37242=CARTESIAN_POINT('Ctrl Pts',(-18.5399396605626,27.7017007070255,122.575930572394)) ;
#37243=CARTESIAN_POINT('Ctrl Pts',(-18.3226042807451,27.5217116266156,122.366962086678)) ;
#37244=CARTESIAN_POINT('Ctrl Pts',(-18.6958321778564,27.711552287675,122.439501623981)) ;
#37245=CARTESIAN_POINT('Ctrl Pts',(-18.5174703779917,27.5315632072652,122.196424414274)) ;
#37246=CARTESIAN_POINT('Ctrl Pts',(-18.8768591143373,27.7216254159734,122.329686829936)) ;
#37247=CARTESIAN_POINT('Ctrl Pts',(-18.7437532834389,27.5416363355635,122.05915550408)) ;
#37248=CARTESIAN_POINT('Ctrl Pts',(-19.069748360102,27.7314678938648,122.254738925638)) ;
#37249=CARTESIAN_POINT('Ctrl Pts',(-18.9848658829464,27.551478813455,121.96546939627)) ;
#37250=CARTESIAN_POINT('Ctrl Pts',(-19.275402729767,27.7414485004629,122.213172865234)) ;
#37251=CARTESIAN_POINT('Ctrl Pts',(-19.2419340497861,27.561459420053,121.913511275043)) ;
#37252=CARTESIAN_POINT('Ctrl Pts',(-19.4859500150315,27.7514662094817,122.208323768403)) ;
#37253=CARTESIAN_POINT('Ctrl Pts',(-19.50511813664,27.5714771290719,121.907449255044)) ;
#37254=CARTESIAN_POINT('Ctrl Pts',(-19.6914845982736,27.7613523885191,122.23929217762)) ;
#37255=CARTESIAN_POINT('Ctrl Pts',(-19.7620374996912,27.5813633081093,121.946159440235)) ;
#37256=CARTESIAN_POINT('Ctrl Pts',(-19.8919086335487,27.7714100010914,122.306601119756)) ;
#37257=CARTESIAN_POINT('Ctrl Pts',(-20.0125674014289,27.5914209206816,122.030295059211)) ;
#37258=CARTESIAN_POINT('Ctrl Pts',(-20.0742918881656,27.7812863944636,122.405862590949)) ;
#37259=CARTESIAN_POINT('Ctrl Pts',(-20.2405477178928,27.6012973140538,122.154372035047)) ;
#37260=CARTESIAN_POINT('Ctrl Pts',(-20.2389323043103,27.791281422614,122.536416615308)) ;
#37261=CARTESIAN_POINT('Ctrl Pts',(-20.4463485473528,27.6112923422042,122.31756446123)) ;
#37262=CARTESIAN_POINT('Ctrl Pts',(-20.3785025030073,27.80130216946,122.694229664895)) ;
#37263=CARTESIAN_POINT('Ctrl Pts',(-20.6208115760538,27.6213130890502,122.514830465303)) ;
#37264=CARTESIAN_POINT('Ctrl Pts',(-20.4874494476852,27.8112042381264,122.871614573746)) ;
#37265=CARTESIAN_POINT('Ctrl Pts',(-20.7569960330967,27.6312151577166,122.736562250917)) ;
#37266=CARTESIAN_POINT('Ctrl Pts',(-20.5649160847513,27.8211949779461,123.066844849364)) ;
#37267=CARTESIAN_POINT('Ctrl Pts',(-20.8538296012272,27.6412058975363,122.980600241096)) ;
#37268=CARTESIAN_POINT('Ctrl Pts',(-20.6070370985664,27.8311581741564,123.272013328294)) ;
#37269=CARTESIAN_POINT('Ctrl Pts',(-20.9064812124733,27.6511690937465,123.237061229653)) ;
#37270=CARTESIAN_POINT('Ctrl Pts',(-20.6133758883929,27.8410623584565,123.480152818403)) ;
#37271=CARTESIAN_POINT('Ctrl Pts',(-20.9144047818511,27.6610732780467,123.497236530686)) ;
#37272=CARTESIAN_POINT('Ctrl Pts',(-20.5828360532262,27.8511228188474,123.689412748153)) ;
#37273=CARTESIAN_POINT('Ctrl Pts',(-20.8762301627314,27.6711337384376,123.758811110932)) ;
#37274=CARTESIAN_POINT('Ctrl Pts',(-20.5181122383662,27.8609633647182,123.885935058997)) ;
#37275=CARTESIAN_POINT('Ctrl Pts',(-20.7953249519899,27.6809742843083,124.004465402218)) ;
#37276=CARTESIAN_POINT('Ctrl Pts',(-20.4183061486459,27.8710255854299,124.072424108861)) ;
#37277=CARTESIAN_POINT('Ctrl Pts',(-20.6705674371675,27.6910365050201,124.237576347418)) ;
#37278=CARTESIAN_POINT('Ctrl Pts',(-20.2895881644942,27.8809227284465,124.235913842461)) ;
#37279=CARTESIAN_POINT('Ctrl Pts',(-20.5096693379548,27.7009336480366,124.441939302663)) ;
#37280=CARTESIAN_POINT('Ctrl Pts',(-20.1343799700791,27.8908539048637,124.375554329111)) ;
#37281=CARTESIAN_POINT('Ctrl Pts',(-20.3156583736033,27.7108648244538,124.616490187183)) ;
#37282=CARTESIAN_POINT('Ctrl Pts',(-19.9551790503614,27.9008961186423,124.487164722517)) ;
#37283=CARTESIAN_POINT('Ctrl Pts',(-20.0916573040226,27.7209070382324,124.756002912792)) ;
#37284=CARTESIAN_POINT('Ctrl Pts',(-19.762401523415,27.910782658845,124.564891732212)) ;
#37285=CARTESIAN_POINT('Ctrl Pts',(-19.8506842942857,27.7307935784352,124.853161854155)) ;
#37286=CARTESIAN_POINT('Ctrl Pts',(-19.5569511425706,27.9207762534504,124.608757066638)) ;
#37287=CARTESIAN_POINT('Ctrl Pts',(-19.59387104564,27.7407871730406,124.907993194493)) ;
#37288=CARTESIAN_POINT('Ctrl Pts',(-19.3480204997779,27.930720128608,124.616215006894)) ;
#37289=CARTESIAN_POINT('Ctrl Pts',(-19.3327071093506,27.7507310481981,124.917315275417)) ;
#37290=CARTESIAN_POINT('Ctrl Pts',(-19.1406090152874,27.9406806647228,124.587509478741)) ;
#37291=CARTESIAN_POINT('Ctrl Pts',(-19.0734423500344,27.760691584313,124.881432829673)) ;
#37292=CARTESIAN_POINT('Ctrl Pts',(-18.9405381225761,27.9506772680455,124.523103824295)) ;
#37293=CARTESIAN_POINT('Ctrl Pts',(-18.8233537498005,27.7706881876357,124.800925220458)) ;
#37294=CARTESIAN_POINT('Ctrl Pts',(-18.7541744874109,27.960710351,124.424327030337)) ;
#37295=CARTESIAN_POINT('Ctrl Pts',(-18.590399518169,27.7807212705902,124.677453935448)) ;
#37296=CARTESIAN_POINT('Ctrl Pts',(-18.5906478671095,27.9705615197016,124.297248746626)) ;
#37297=CARTESIAN_POINT('Ctrl Pts',(-18.3859904695605,27.7905724392918,124.518604840419)) ;
#37298=CARTESIAN_POINT('Ctrl Pts',(-18.4496441002172,27.9805240104005,124.142390521308)) ;
#37299=CARTESIAN_POINT('Ctrl Pts',(-18.2097360022232,27.8005349299906,124.325031213383)) ;
#37300=CARTESIAN_POINT('Ctrl Pts',(-18.3371397750335,27.9905524388182,123.964073852674)) ;
#37301=CARTESIAN_POINT('Ctrl Pts',(-18.0691061955959,27.8105633584084,124.102135115814)) ;
#37302=CARTESIAN_POINT('Ctrl Pts',(-18.2581916508595,28.0004628061828,123.771274447575)) ;
#37303=CARTESIAN_POINT('Ctrl Pts',(-17.970421329577,27.8204737257729,123.861134793035)) ;
#37304=CARTESIAN_POINT('Ctrl Pts',(-18.2132715984884,28.0103976737979,123.567293786419)) ;
#37305=CARTESIAN_POINT('Ctrl Pts',(-17.9142719851426,27.8304085933881,123.606158130972)) ;
#37306=CARTESIAN_POINT('Ctrl Pts',(-18.2045541391692,28.0204388157769,123.356384171661)) ;
#37307=CARTESIAN_POINT('Ctrl Pts',(-17.9033759752312,27.8404497353671,123.342521266575)) ;
#37308=CARTESIAN_POINT('Ctrl Pts',(-18.2320173963766,28.0303259519801,123.150336225817)) ;
#37309=CARTESIAN_POINT('Ctrl Pts',(-17.9377060395353,27.8503368715702,123.084960416977)) ;
#37310=CARTESIAN_POINT('Ctrl Pts',(-18.2951662826154,28.0403182343835,122.949998669832)) ;
#37311=CARTESIAN_POINT('Ctrl Pts',(-18.0166431581051,27.8603291539736,122.834538577191)) ;
#37312=CARTESIAN_POINT('Ctrl Pts',(-18.3917805672602,28.0502667623487,122.764488512371)) ;
#37313=CARTESIAN_POINT('Ctrl Pts',(-18.1374121264596,27.8702776819389,122.602650848171)) ;
#37314=CARTESIAN_POINT('Ctrl Pts',(-18.5187344195011,28.0602034935108,122.598611319051)) ;
#37315=CARTESIAN_POINT('Ctrl Pts',(-18.2961056898264,27.880214413101,122.395304507896)) ;
#37316=CARTESIAN_POINT('Ctrl Pts',(-18.6731352153546,28.0701867043708,122.456413854557)) ;
#37317=CARTESIAN_POINT('Ctrl Pts',(-18.4891076721337,27.890197623961,122.217558370884)) ;
#37318=CARTESIAN_POINT('Ctrl Pts',(-18.8511053323271,28.0802298035207,122.342850389306)) ;
#37319=CARTESIAN_POINT('Ctrl Pts',(-18.7115707176788,27.9002407231109,122.075605016145)) ;
#37320=CARTESIAN_POINT('Ctrl Pts',(-19.0418370727349,28.0900607677956,122.26317827219)) ;
#37321=CARTESIAN_POINT('Ctrl Pts',(-18.9499871891005,27.9100716873857,121.97601543362)) ;
#37322=CARTESIAN_POINT('Ctrl Pts',(-19.2483766387023,28.1001336201815,122.216578929442)) ;
#37323=CARTESIAN_POINT('Ctrl Pts',(-19.2081615249789,27.9201445397717,121.917767583911)) ;
#37324=CARTESIAN_POINT('Ctrl Pts',(-19.4555437861215,28.1099977478933,122.206790899523)) ;
#37325=CARTESIAN_POINT('Ctrl Pts',(-19.4671216625215,27.9300086674835,121.905533740813)) ;
#37326=CARTESIAN_POINT('Ctrl Pts',(-19.6645948451265,28.1200199500282,122.233024086339)) ;
#37327=CARTESIAN_POINT('Ctrl Pts',(-19.7284352632349,27.9400308696183,121.938326646728)) ;
#37328=CARTESIAN_POINT('Ctrl Pts',(-19.8658877748029,28.1300471429966,122.295670934239)) ;
#37329=CARTESIAN_POINT('Ctrl Pts',(-19.9800509846578,27.9500580625868,122.016636385293)) ;
#37330=CARTESIAN_POINT('Ctrl Pts',(-20.0501626714237,28.1399027369636,122.39036087509)) ;
#37331=CARTESIAN_POINT('Ctrl Pts',(-20.2103950643884,27.9599136565538,122.135000592718)) ;
#37332=CARTESIAN_POINT('Ctrl Pts',(-20.2172929353047,28.1498599088289,122.516416762394)) ;
#37333=CARTESIAN_POINT('Ctrl Pts',(-20.4193072749355,27.9698708284191,122.292571980772)) ;
#37334=CARTESIAN_POINT('Ctrl Pts',(-20.36088775291,28.1598987528273,122.67106650366)) ;
#37335=CARTESIAN_POINT('Ctrl Pts',(-20.5987996284772,27.9799096724175,122.485885053501)) ;
#37336=CARTESIAN_POINT('Ctrl Pts',(-20.4738977645388,28.1697727767028,122.845224021032)) ;
#37337=CARTESIAN_POINT('Ctrl Pts',(-20.7400613605659,27.989783696293,122.703583668391)) ;
#37338=CARTESIAN_POINT('Ctrl Pts',(-20.5565305050554,28.1798426026932,123.040098786974)) ;
#37339=CARTESIAN_POINT('Ctrl Pts',(-20.8433506854112,27.9998535222834,122.947177423927)) ;
#37340=CARTESIAN_POINT('Ctrl Pts',(-20.603072347858,28.1896758465905,123.241534739974)) ;
#37341=CARTESIAN_POINT('Ctrl Pts',(-20.9015266941118,28.0096867661807,123.198973980938)) ;
#37342=CARTESIAN_POINT('Ctrl Pts',(-20.614743890259,28.1997062743635,123.452075818359)) ;
#37343=CARTESIAN_POINT('Ctrl Pts',(-20.9161142995168,28.0197171939537,123.462150342136)) ;
#37344=CARTESIAN_POINT('Ctrl Pts',(-20.5890670250738,28.2097378911087,123.661414868918)) ;
#37345=CARTESIAN_POINT('Ctrl Pts',(-20.8840166201803,28.0297488106989,123.723823875487)) ;
#37346=CARTESIAN_POINT('Ctrl Pts',(-20.5290926772713,28.2195675680894,123.859156375962)) ;
#37347=CARTESIAN_POINT('Ctrl Pts',(-20.8090466299331,28.0395784876796,123.971001465178)) ;
#37348=CARTESIAN_POINT('Ctrl Pts',(-20.4347263329766,28.2295570849293,124.046779224324)) ;
#37349=CARTESIAN_POINT('Ctrl Pts',(-20.6910868707223,28.0495680045195,124.205529304488)) ;
#37350=CARTESIAN_POINT('Ctrl Pts',(-20.308112533224,28.2396006970691,124.215750588149)) ;
#37351=CARTESIAN_POINT('Ctrl Pts',(-20.5328182780255,28.0596116166593,124.416742316219)) ;
#37352=CARTESIAN_POINT('Ctrl Pts',(-20.1577648900733,28.2494233034044,124.357312030463)) ;
#37353=CARTESIAN_POINT('Ctrl Pts',(-20.3448814895042,28.0694342229946,124.593693576186)) ;
#37354=CARTESIAN_POINT('Ctrl Pts',(-19.9816030750299,28.2594615333036,124.473500882314)) ;
#37355=CARTESIAN_POINT('Ctrl Pts',(-20.1246781855413,28.0794724528938,124.738927845649)) ;
#37356=CARTESIAN_POINT('Ctrl Pts',(-19.7882531660864,28.2694725680956,124.556669707045)) ;
#37357=CARTESIAN_POINT('Ctrl Pts',(-19.8829899980737,28.0894834876857,124.84288713183)) ;
#37358=CARTESIAN_POINT('Ctrl Pts',(-19.5858129110288,28.2793702990627,124.604775415822)) ;
#37359=CARTESIAN_POINT('Ctrl Pts',(-19.629938496845,28.0993812186529,124.903017472002)) ;
#37360=CARTESIAN_POINT('Ctrl Pts',(-19.376180880844,28.2893599269132,124.617388122946)) ;
#37361=CARTESIAN_POINT('Ctrl Pts',(-19.3678981582477,28.1093708465034,124.9187812748)) ;
#37362=CARTESIAN_POINT('Ctrl Pts',(-19.1682588404928,28.2993157173592,124.593418733339)) ;
#37363=CARTESIAN_POINT('Ctrl Pts',(-19.1079954571201,28.1193266369494,124.88881743189)) ;
#37364=CARTESIAN_POINT('Ctrl Pts',(-18.96810534998,28.3092431159212,124.534261318973)) ;
#37365=CARTESIAN_POINT('Ctrl Pts',(-18.8578037171017,28.1292540355114,124.814868421529)) ;
#37366=CARTESIAN_POINT('Ctrl Pts',(-18.7794564522439,28.3192687110311,124.440280835038)) ;
#37367=CARTESIAN_POINT('Ctrl Pts',(-18.6219935808198,28.1392796306213,124.697390886219)) ;
#37368=CARTESIAN_POINT('Ctrl Pts',(-18.6122710106145,28.3291545617007,124.31681671948)) ;
#37369=CARTESIAN_POINT('Ctrl Pts',(-18.413012494955,28.1491654812909,124.543058534204)) ;
#37370=CARTESIAN_POINT('Ctrl Pts',(-18.4672022044828,28.3391437415449,124.164964313106)) ;
#37371=CARTESIAN_POINT('Ctrl Pts',(-18.2316780605687,28.1591546611351,124.353241304925)) ;
#37372=CARTESIAN_POINT('Ctrl Pts',(-18.350468282265,28.3491849286484,123.98908060691)) ;
#37373=CARTESIAN_POINT('Ctrl Pts',(-18.08576255543,28.1691958482386,124.133385523798)) ;
#37374=CARTESIAN_POINT('Ctrl Pts',(-18.267489993905,28.3590175721244,123.799757295272)) ;
#37375=CARTESIAN_POINT('Ctrl Pts',(-17.9820414176023,28.1790284917146,123.896729581329)) ;
#37376=CARTESIAN_POINT('Ctrl Pts',(-18.2172586034104,28.3690115218339,123.595747330936)) ;
#37377=CARTESIAN_POINT('Ctrl Pts',(-17.9192545217084,28.1890224414241,123.64171642404)) ;
#37378=CARTESIAN_POINT('Ctrl Pts',(-18.2036074114145,28.3790406446104,123.385343767415)) ;
#37379=CARTESIAN_POINT('Ctrl Pts',(-17.9021928664075,28.1990515642006,123.378711840275)) ;
#37380=CARTESIAN_POINT('Ctrl Pts',(-18.2260142937554,28.3889167755291,123.178918899559)) ;
#37381=CARTESIAN_POINT('Ctrl Pts',(-17.9302039421449,28.2089276951193,123.120680343529)) ;
#37382=CARTESIAN_POINT('Ctrl Pts',(-18.2843913723889,28.3989148105461,122.977024252762)) ;
#37383=CARTESIAN_POINT('Ctrl Pts',(-18.003177692541,28.2189257301363,122.868312611981)) ;
#37384=CARTESIAN_POINT('Ctrl Pts',(-18.3760366799018,28.4088287403048,122.789803762381)) ;
#37385=CARTESIAN_POINT('Ctrl Pts',(-18.1177367767747,28.228839659895,122.634287677153)) ;
#37386=CARTESIAN_POINT('Ctrl Pts',(-18.500337734295,28.4188719280426,122.619151689602)) ;
#37387=CARTESIAN_POINT('Ctrl Pts',(-18.2731150794014,28.2388828476328,122.420974122338)) ;
#37388=CARTESIAN_POINT('Ctrl Pts',(-18.6502217855382,28.428771770183,122.474737172695)) ;
#37389=CARTESIAN_POINT('Ctrl Pts',(-18.460472242702,28.2487826897731,122.240457435549)) ;
#37390=CARTESIAN_POINT('Ctrl Pts',(-18.8242413063613,28.438763036991,122.357101788211)) ;
#37391=CARTESIAN_POINT('Ctrl Pts',(-18.6779981948362,28.2587739565812,122.093415286222)) ;
#37392=CARTESIAN_POINT('Ctrl Pts',(-19.0169763775656,28.4487951391229,122.271451770785)) ;
#37393=CARTESIAN_POINT('Ctrl Pts',(-18.9189180448154,28.2688060587131,121.986355077161)) ;
#37394=CARTESIAN_POINT('Ctrl Pts',(-19.2182110681717,28.4586620200777,122.221141613254)) ;
#37395=CARTESIAN_POINT('Ctrl Pts',(-19.170462608238,28.2786729396679,121.923469734466)) ;
#37396=CARTESIAN_POINT('Ctrl Pts',(-19.4277169110003,28.4686538113658,122.205851400272)) ;
#37397=CARTESIAN_POINT('Ctrl Pts',(-19.4323452132242,28.288664730956,121.904359612278)) ;
#37398=CARTESIAN_POINT('Ctrl Pts',(-19.6374921877922,28.4786859272774,122.227662227062)) ;
#37399=CARTESIAN_POINT('Ctrl Pts',(-19.6945640397909,28.2986968468675,121.931625723093)) ;
#37400=CARTESIAN_POINT('Ctrl Pts',(-19.8370378148064,28.4885522440774,122.284307432454)) ;
#37401=CARTESIAN_POINT('Ctrl Pts',(-19.9439958523289,28.3085631636676,122.002434913223)) ;
#37402=CARTESIAN_POINT('Ctrl Pts',(-20.0261278855234,28.498539725551,122.375526578932)) ;
#37403=CARTESIAN_POINT('Ctrl Pts',(-20.1803573810045,28.3185506451412,122.116461326089)) ;
#37404=CARTESIAN_POINT('Ctrl Pts',(-20.1958916606712,28.5084846499299,122.497612228053)) ;
#37405=CARTESIAN_POINT('Ctrl Pts',(-20.3925607131748,28.3284955695201,122.269070719358)) ;
#37406=CARTESIAN_POINT('Ctrl Pts',(-20.3432261236584,28.5185295358406,122.64887127178)) ;
#37407=CARTESIAN_POINT('Ctrl Pts',(-20.5767268497532,28.3385404554308,122.458146387044)) ;
#37408=CARTESIAN_POINT('Ctrl Pts',(-20.4600658639641,28.5283916395532,122.820164450749)) ;
#37409=CARTESIAN_POINT('Ctrl Pts',(-20.7227745276949,28.3484025591434,122.672264744805)) ;
#37410=CARTESIAN_POINT('Ctrl Pts',(-20.546882409536,28.5383832033776,123.011421338606)) ;
#37411=CARTESIAN_POINT('Ctrl Pts',(-20.831292734905,28.3583941229678,122.911337082872)) ;
#37412=CARTESIAN_POINT('Ctrl Pts',(-20.5987837541194,28.5483160114405,123.213686812683)) ;
#37413=CARTESIAN_POINT('Ctrl Pts',(-20.8961668072617,28.3683269310307,123.164169825485)) ;
#37414=CARTESIAN_POINT('Ctrl Pts',(-20.6152968104347,28.5582531136769,123.42195527368)) ;
#37415=CARTESIAN_POINT('Ctrl Pts',(-20.9168053567252,28.3782640332671,123.424505796562)) ;
#37416=CARTESIAN_POINT('Ctrl Pts',(-20.5948899082448,28.5683055599473,123.632285532663)) ;
#37417=CARTESIAN_POINT('Ctrl Pts',(-20.891293966489,28.3883164795374,123.687418366496)) ;
#37418=CARTESIAN_POINT('Ctrl Pts',(-20.5397117951602,28.5781516755289,123.831810652888)) ;
#37419=CARTESIAN_POINT('Ctrl Pts',(-20.8223185569901,28.3981625951191,123.936824298413)) ;
#37420=CARTESIAN_POINT('Ctrl Pts',(-20.4492135047243,28.5881996952438,124.022668210418)) ;
#37421=CARTESIAN_POINT('Ctrl Pts',(-20.7091931472438,28.4082106148339,124.175395051992)) ;
#37422=CARTESIAN_POINT('Ctrl Pts',(-20.3279884165152,28.5981416468727,124.192947955947)) ;
#37423=CARTESIAN_POINT('Ctrl Pts',(-20.5576594224477,28.4181525664629,124.388243230792)) ;
#37424=CARTESIAN_POINT('Ctrl Pts',(-20.1794561705445,28.6080804278718,124.339907298682)) ;
#37425=CARTESIAN_POINT('Ctrl Pts',(-20.3719920554708,28.428091347462,124.571940487543)) ;
#37426=CARTESIAN_POINT('Ctrl Pts',(-20.0060768723233,28.6181064765979,124.459748019633)) ;
#37427=CARTESIAN_POINT('Ctrl Pts',(-20.1552662552199,28.438117396188,124.72173910567)) ;
#37428=CARTESIAN_POINT('Ctrl Pts',(-19.8172567237363,28.6279933370061,124.546699844584)) ;
#37429=CARTESIAN_POINT('Ctrl Pts',(-19.9192398618571,28.4480042565963,124.830426395239)) ;
#37430=CARTESIAN_POINT('Ctrl Pts',(-19.6133539599856,28.6380246121379,124.600393761194)) ;
#37431=CARTESIAN_POINT('Ctrl Pts',(-19.6643603212946,28.4580355317281,124.897541006025)) ;
#37432=CARTESIAN_POINT('Ctrl Pts',(-19.4062711547036,28.6479075894383,124.617827169365)) ;
#37433=CARTESIAN_POINT('Ctrl Pts',(-19.4055076350618,28.4679185090285,124.919330220235)) ;
#37434=CARTESIAN_POINT('Ctrl Pts',(-19.1957631832706,28.6579644428455,124.598722627596)) ;
#37435=CARTESIAN_POINT('Ctrl Pts',(-19.1423686472361,28.4779753624356,124.895445755613)) ;
#37436=CARTESIAN_POINT('Ctrl Pts',(-18.9283731228152,28.6711326839214,124.526630695589)) ;
#37437=CARTESIAN_POINT('Ctrl Pts',(-18.8081529113216,28.4911436035116,124.805332008943)) ;
#37438=CARTESIAN_POINT('Ctrl Pts',(-18.6817983350219,28.6845337131479,124.384021538888)) ;
#37439=CARTESIAN_POINT('Ctrl Pts',(-18.4999549681537,28.5045446327381,124.627092881271)) ;
#37440=CARTESIAN_POINT('Ctrl Pts',(-18.4857344421306,28.6977466298788,124.187192207811)) ;
#37441=CARTESIAN_POINT('Ctrl Pts',(-18.254834612915,28.5177575494689,124.381018273115)) ;
#37442=CARTESIAN_POINT('Ctrl Pts',(-18.3657858162467,28.707675024332,124.016416499208)) ;
#37443=CARTESIAN_POINT('Ctrl Pts',(-18.1049098191361,28.5276859439222,124.16755417654)) ;
#37444=CARTESIAN_POINT('Ctrl Pts',(-18.2766712212058,28.7176565244601,123.826404589139)) ;
#37445=CARTESIAN_POINT('Ctrl Pts',(-17.9935167508853,28.5376674440503,123.930036177119)) ;
#37446=CARTESIAN_POINT('Ctrl Pts',(-18.2218707889986,28.7276970677302,123.622569483315)) ;
#37447=CARTESIAN_POINT('Ctrl Pts',(-17.9250194852318,28.5477079873204,123.675241990124)) ;
#37448=CARTESIAN_POINT('Ctrl Pts',(-18.2033757282844,28.7375463995133,123.416330418717)) ;
#37449=CARTESIAN_POINT('Ctrl Pts',(-17.9019033242147,28.5575573191035,123.417442838969)) ;
#37450=CARTESIAN_POINT('Ctrl Pts',(-18.2206940069242,28.747541803985,123.206912125949)) ;
#37451=CARTESIAN_POINT('Ctrl Pts',(-17.9235537435517,28.5675527235752,123.155670875164)) ;
#37452=CARTESIAN_POINT('Ctrl Pts',(-18.2745872662887,28.7575581314336,123.003350839589)) ;
#37453=CARTESIAN_POINT('Ctrl Pts',(-17.990923682681,28.5775690510238,122.901217359039)) ;
#37454=CARTESIAN_POINT('Ctrl Pts',(-18.3909335432918,28.7707817886001,122.750824717369)) ;
#37455=CARTESIAN_POINT('Ctrl Pts',(-18.1363563321202,28.5907927081903,122.585573837996)) ;
#37456=CARTESIAN_POINT('Ctrl Pts',(-18.5712652888683,28.7840760799895,122.533196711622)) ;
#37457=CARTESIAN_POINT('Ctrl Pts',(-18.3617388881424,28.6040869995797,122.313564150159)) ;
#37458=CARTESIAN_POINT('Ctrl Pts',(-18.799057046922,28.797360430921,122.371600064136)) ;
#37459=CARTESIAN_POINT('Ctrl Pts',(-18.6465253994533,28.6173713505112,122.11153161396)) ;
#37460=CARTESIAN_POINT('Ctrl Pts',(-18.9884277129976,28.8073328119828,122.281692967666)) ;
#37461=CARTESIAN_POINT('Ctrl Pts',(-18.8832307222532,28.6273437315729,121.999158080015)) ;
#37462=CARTESIAN_POINT('Ctrl Pts',(-19.1891836686621,28.8172411916084,122.226029840972)) ;
#37463=CARTESIAN_POINT('Ctrl Pts',(-19.134178804972,28.6372521111986,121.929579826064)) ;
#37464=CARTESIAN_POINT('Ctrl Pts',(-19.3995659070131,28.8272951903564,122.205875393867)) ;
#37465=CARTESIAN_POINT('Ctrl Pts',(-19.3971551455216,28.6473061099466,121.904389073362)) ;
#37466=CARTESIAN_POINT('Ctrl Pts',(-19.6062836932465,28.8371573874727,122.222079550303)) ;
#37467=CARTESIAN_POINT('Ctrl Pts',(-19.6555567772923,28.6571683070629,121.924649710888)) ;
#37468=CARTESIAN_POINT('Ctrl Pts',(-19.8780826757267,28.8505045138469,122.29182043757)) ;
#37469=CARTESIAN_POINT('Ctrl Pts',(-19.995279830665,28.6705154334371,122.01181375835)) ;
#37470=CARTESIAN_POINT('Ctrl Pts',(-20.1845000475927,28.8670414794883,122.464288153073)) ;
#37471=CARTESIAN_POINT('Ctrl Pts',(-20.3783371558537,28.6870523990785,122.227433847965)) ;
#37472=CARTESIAN_POINT('Ctrl Pts',(-20.4154369591003,28.8836760836622,122.732174044355)) ;
#37473=CARTESIAN_POINT('Ctrl Pts',(-20.6669572706625,28.7036870032524,122.562229846331)) ;
#37474=CARTESIAN_POINT('Ctrl Pts',(-20.5367399369156,28.8969658769049,122.98386445411)) ;
#37475=CARTESIAN_POINT('Ctrl Pts',(-20.8186195037405,28.7169767964951,122.876897221758)) ;
#37476=CARTESIAN_POINT('Ctrl Pts',(-20.5937434976173,28.9069185081643,123.1851719771)) ;
#37477=CARTESIAN_POINT('Ctrl Pts',(-20.8898646072513,28.7269294277544,123.128520520416)) ;
#37478=CARTESIAN_POINT('Ctrl Pts',(-20.6151704596498,28.916870475469,123.393312690541)) ;
#37479=CARTESIAN_POINT('Ctrl Pts',(-20.9166469900547,28.7368813950591,123.388702342931)) ;
#37480=CARTESIAN_POINT('Ctrl Pts',(-20.5948058201253,28.9302377339328,123.673577606172)) ;
#37481=CARTESIAN_POINT('Ctrl Pts',(-20.8911927394043,28.750248653523,123.739016958584)) ;
#37482=CARTESIAN_POINT('Ctrl Pts',(-20.4800520817175,28.9467545458819,124.005580786161)) ;
#37483=CARTESIAN_POINT('Ctrl Pts',(-20.7477418811131,28.7667654654721,124.154036877194)) ;
#37484=CARTESIAN_POINT('Ctrl Pts',(-20.2120144615373,28.9667804408883,124.336293100921)) ;
#37485=CARTESIAN_POINT('Ctrl Pts',(-20.4126932065167,28.7867913604785,124.567418944553)) ;
#37486=CARTESIAN_POINT('Ctrl Pts',(-19.8510301281953,28.9865911710184,124.553536596618)) ;
#37487=CARTESIAN_POINT('Ctrl Pts',(-19.9614615275736,28.8066020906086,124.838970603428)) ;
#37488=CARTESIAN_POINT('Ctrl Pts',(-19.4344012108349,29.0065683871483,124.636109825588)) ;
#37489=CARTESIAN_POINT('Ctrl Pts',(-19.4406750274581,28.8265793067385,124.942183198425)) ;
#37490=CARTESIAN_POINT('Ctrl Pts',(-19.0157681070412,29.0264952625436,124.57095034557)) ;
#37491=CARTESIAN_POINT('Ctrl Pts',(-18.9173848458193,28.8465061821338,124.860730356199)) ;
#37492=CARTESIAN_POINT('Ctrl Pts',(-18.6457374117665,29.0463167240198,124.369076668043)) ;
#37493=CARTESIAN_POINT('Ctrl Pts',(-18.4548495375607,28.86632764361,124.608386573035)) ;
#37494=CARTESIAN_POINT('Ctrl Pts',(-18.3635430708779,29.0663910418292,124.048922971134)) ;
#37495=CARTESIAN_POINT('Ctrl Pts',(-18.1021082198749,28.8864019614194,124.208191902882)) ;
#37496=CARTESIAN_POINT('Ctrl Pts',(-18.2096162661091,29.0862390108371,123.655849066001)) ;
#37497=CARTESIAN_POINT('Ctrl Pts',(-17.9097030413974,28.9062499304272,123.716849978501)) ;
#37498=CARTESIAN_POINT('Ctrl Pts',(-18.1981447189495,29.1061860449003,123.231968651957)) ;
#37499=CARTESIAN_POINT('Ctrl Pts',(-17.8953659111602,28.9261969644905,123.187000088167)) ;
#37500=CARTESIAN_POINT('Ctrl Pts',(-18.3318077694759,29.1260819958724,122.830562780161)) ;
#37501=CARTESIAN_POINT('Ctrl Pts',(-18.0624463344444,28.9460929154626,122.685244684146)) ;
#37502=CARTESIAN_POINT('Ctrl Pts',(-18.5938358537856,29.1459774754907,122.498483434728)) ;
#37503=CARTESIAN_POINT('Ctrl Pts',(-18.3899816867549,28.9659883950809,122.270147568278)) ;
#37504=CARTESIAN_POINT('Ctrl Pts',(-18.9545509966917,29.1659335864555,122.274963150452)) ;
#37505=CARTESIAN_POINT('Ctrl Pts',(-18.8408757371955,28.9859445060457,121.99074852876)) ;
#37506=CARTESIAN_POINT('Ctrl Pts',(-19.3687523473574,29.1858381344955,122.188317116435)) ;
#37507=CARTESIAN_POINT('Ctrl Pts',(-19.3586261760536,29.0058490540857,121.882442313801)) ;
#37508=CARTESIAN_POINT('Ctrl Pts',(-19.7873033294093,29.2057122588146,122.247090838418)) ;
#37509=CARTESIAN_POINT('Ctrl Pts',(-19.8818129365683,29.0257231784047,121.955909174204)) ;
#37510=CARTESIAN_POINT('Ctrl Pts',(-20.1636458920224,29.2257667888136,122.447434307739)) ;
#37511=CARTESIAN_POINT('Ctrl Pts',(-20.352241834532,29.0457777084038,122.206339109626)) ;
#37512=CARTESIAN_POINT('Ctrl Pts',(-20.4457143490153,29.2455743025736,122.760308780651)) ;
#37513=CARTESIAN_POINT('Ctrl Pts',(-20.7048254925802,29.0655852221637,122.59742983607)) ;
#37514=CARTESIAN_POINT('Ctrl Pts',(-20.6062625022629,29.2655576583413,123.153645694702)) ;
#37515=CARTESIAN_POINT('Ctrl Pts',(-20.9055115950316,29.0855685779315,123.089100356968)) ;
#37516=CARTESIAN_POINT('Ctrl Pts',(-20.6222571826096,29.2854759609252,123.57685578804)) ;
#37517=CARTESIAN_POINT('Ctrl Pts',(-20.9255057422974,29.1054868805154,123.618111697488)) ;
#37518=CARTESIAN_POINT('Ctrl Pts',(-20.4942524999631,29.305344176371,123.97953847386)) ;
#37519=CARTESIAN_POINT('Ctrl Pts',(-20.7655021762752,29.1253550959612,124.121463964398)) ;
#37520=CARTESIAN_POINT('Ctrl Pts',(-20.2337505644514,29.3253944931673,124.316857983923)) ;
#37521=CARTESIAN_POINT('Ctrl Pts',(-20.4398756731865,29.1454054127574,124.543114839658)) ;
#37522=CARTESIAN_POINT('Ctrl Pts',(-19.8787560188095,29.3451705550497,124.542547094781)) ;
#37523=CARTESIAN_POINT('Ctrl Pts',(-19.9961359923374,29.1651814746399,124.825226575643)) ;
#37524=CARTESIAN_POINT('Ctrl Pts',(-19.4626770517434,29.3652251607422,124.635063105545)) ;
#37525=CARTESIAN_POINT('Ctrl Pts',(-19.4760372478576,29.1852360803324,124.940874254979)) ;
#37526=CARTESIAN_POINT('Ctrl Pts',(-19.0452208405963,29.3850188498981,124.580591047788)) ;
#37527=CARTESIAN_POINT('Ctrl Pts',(-18.9542188863965,29.2050297694883,124.872787108303)) ;
#37528=CARTESIAN_POINT('Ctrl Pts',(-18.6678065643519,29.4049855414925,124.386372516553)) ;
#37529=CARTESIAN_POINT('Ctrl Pts',(-18.4824497195232,29.2249964610827,124.630017164138)) ;
#37530=CARTESIAN_POINT('Ctrl Pts',(-18.379791129464,29.4249455872434,124.074550900543)) ;
#37531=CARTESIAN_POINT('Ctrl Pts',(-18.1224282620672,29.2449565068336,124.240242602024)) ;
#37532=CARTESIAN_POINT('Ctrl Pts',(-18.2157634731263,29.4448438473937,123.684577273612)) ;
#37533=CARTESIAN_POINT('Ctrl Pts',(-17.9173907833748,29.2648547669839,123.752777846952)) ;
#37534=CARTESIAN_POINT('Ctrl Pts',(-18.1941500603982,29.4647387629429,123.262128718319)) ;
#37535=CARTESIAN_POINT('Ctrl Pts',(-17.8903701259181,29.284749682533,123.224718223143)) ;
#37536=CARTESIAN_POINT('Ctrl Pts',(-18.3177155519128,29.4846489433565,122.85722218228)) ;
#37537=CARTESIAN_POINT('Ctrl Pts',(-18.0448227790929,29.3046598629467,122.718584462638)) ;
#37538=CARTESIAN_POINT('Ctrl Pts',(-18.5722210885648,29.5045847424707,122.518222965031)) ;
#37539=CARTESIAN_POINT('Ctrl Pts',(-18.3629508948928,29.3245956620609,122.294833096164)) ;
#37540=CARTESIAN_POINT('Ctrl Pts',(-18.9271398359767,29.5245226041249,122.286384499788)) ;
#37541=CARTESIAN_POINT('Ctrl Pts',(-18.806596664507,29.3445335237151,122.005031573902)) ;
#37542=CARTESIAN_POINT('Ctrl Pts',(-19.3394465637527,29.5444416507625,122.189407632929)) ;
#37543=CARTESIAN_POINT('Ctrl Pts',(-19.3219781329288,29.3644525703527,121.88380547974)) ;
#37544=CARTESIAN_POINT('Ctrl Pts',(-19.7607048779396,29.5643905488167,122.23896191623)) ;
#37545=CARTESIAN_POINT('Ctrl Pts',(-19.8485530096287,29.3844014684068,121.945745518178)) ;
#37546=CARTESIAN_POINT('Ctrl Pts',(-20.1390238650554,29.5842963762597,122.428800132525)) ;
#37547=CARTESIAN_POINT('Ctrl Pts',(-20.3214474198528,29.4043072958499,122.183031232966)) ;
#37548=CARTESIAN_POINT('Ctrl Pts',(-20.381503088585,29.600879071625,122.684669772167)) ;
#37549=CARTESIAN_POINT('Ctrl Pts',(-20.6245684185229,29.4208899912152,122.502888255903)) ;
#37550=CARTESIAN_POINT('Ctrl Pts',(-20.5148467807965,29.6141532853487,122.929890317395)) ;
#37551=CARTESIAN_POINT('Ctrl Pts',(-20.7912341810061,29.4341642049389,122.809390920686)) ;
#37552=CARTESIAN_POINT('Ctrl Pts',(-20.5818729164079,29.624200004548,123.130156956782)) ;
#37553=CARTESIAN_POINT('Ctrl Pts',(-20.875022085284,29.4442109241382,123.059731213221)) ;
#37554=CARTESIAN_POINT('Ctrl Pts',(-20.6127109296286,29.6340440391937,123.334823989138)) ;
#37555=CARTESIAN_POINT('Ctrl Pts',(-20.9135737768824,29.4540549587838,123.315549607636)) ;
#37556=CARTESIAN_POINT('Ctrl Pts',(-20.6063479572666,29.6473784240982,123.615020683285)) ;
#37557=CARTESIAN_POINT('Ctrl Pts',(-20.9056110533452,29.4673893436884,123.665862635862)) ;
#37558=CARTESIAN_POINT('Ctrl Pts',(-20.5072137738658,29.663965641398,123.953603105851)) ;
#37559=CARTESIAN_POINT('Ctrl Pts',(-20.7817183691732,29.4839765609882,124.08900812148)) ;
#37560=CARTESIAN_POINT('Ctrl Pts',(-20.2982490380892,29.6805988534359,124.238824540592)) ;
#37561=CARTESIAN_POINT('Ctrl Pts',(-20.5204871040538,29.500609773026,124.445591168516)) ;
#37562=CARTESIAN_POINT('Ctrl Pts',(-20.0804621860381,29.6938812957081,124.413688383922)) ;
#37563=CARTESIAN_POINT('Ctrl Pts',(-20.2482786095012,29.5138922152982,124.664142759383)) ;
#37564=CARTESIAN_POINT('Ctrl Pts',(-19.8981216436981,29.7037871836223,124.514250466141)) ;
#37565=CARTESIAN_POINT('Ctrl Pts',(-20.020349611139,29.5237981032124,124.78985389597)) ;
#37566=CARTESIAN_POINT('Ctrl Pts',(-19.6995040700482,29.7137756017274,124.582447696612)) ;
#37567=CARTESIAN_POINT('Ctrl Pts',(-19.7720804978003,29.5337865213176,124.875101645532)) ;
#37568=CARTESIAN_POINT('Ctrl Pts',(-19.491307008318,29.7237990289661,124.615012952645)) ;
#37569=CARTESIAN_POINT('Ctrl Pts',(-19.5118312861941,29.5438099485563,124.915810540178)) ;
#37570=CARTESIAN_POINT('Ctrl Pts',(-19.2831262713956,29.7337034600831,124.611097510971)) ;
#37571=CARTESIAN_POINT('Ctrl Pts',(-19.2516162816034,29.5537143796733,124.910922145077)) ;
#37572=CARTESIAN_POINT('Ctrl Pts',(-19.0093558420609,29.7469666126936,124.55825582872)) ;
#37573=CARTESIAN_POINT('Ctrl Pts',(-18.9093488133152,29.5669775322837,124.844857601272)) ;
#37574=CARTESIAN_POINT('Ctrl Pts',(-18.7545952522591,29.7602915105975,124.434343951779)) ;
#37575=CARTESIAN_POINT('Ctrl Pts',(-18.5909285364319,29.5803024301876,124.68997248973)) ;
#37576=CARTESIAN_POINT('Ctrl Pts',(-18.5439553830956,29.7735472542131,124.251793494169)) ;
#37577=CARTESIAN_POINT('Ctrl Pts',(-18.327641649914,29.5935581738033,124.461801734834)) ;
#37578=CARTESIAN_POINT('Ctrl Pts',(-18.4117225992589,29.7835066276604,124.089495823393)) ;
#37579=CARTESIAN_POINT('Ctrl Pts',(-18.1623453453475,29.6035175472506,124.258928464858)) ;
#37580=CARTESIAN_POINT('Ctrl Pts',(-18.3095785405791,29.7934504515873,123.907068143892)) ;
#37581=CARTESIAN_POINT('Ctrl Pts',(-18.034663608841,29.6134613711775,124.030895956601)) ;
#37582=CARTESIAN_POINT('Ctrl Pts',(-18.2401254145393,29.8034983957346,123.707589819514)) ;
#37583=CARTESIAN_POINT('Ctrl Pts',(-17.9478442965894,29.6235093153248,123.781548712631)) ;
#37584=CARTESIAN_POINT('Ctrl Pts',(-18.2068401315693,29.8133493669528,123.503171166359)) ;
#37585=CARTESIAN_POINT('Ctrl Pts',(-17.9062349536996,29.633360286543,123.526025793522)) ;
#37586=CARTESIAN_POINT('Ctrl Pts',(-18.20904682234,29.8233211843949,123.293567779389)) ;
#37587=CARTESIAN_POINT('Ctrl Pts',(-17.9089904953262,29.6433321039851,123.264021399706)) ;
#37588=CARTESIAN_POINT('Ctrl Pts',(-18.2477491639959,29.833316606687,123.086997661394)) ;
#37589=CARTESIAN_POINT('Ctrl Pts',(-17.9573656876307,29.6533275262772,123.005808163282)) ;
#37590=CARTESIAN_POINT('Ctrl Pts',(-18.3222034367972,29.8433496718107,122.889655956978)) ;
#37591=CARTESIAN_POINT('Ctrl Pts',(-18.0504309096525,29.6633605914008,122.759129997716)) ;
#37592=CARTESIAN_POINT('Ctrl Pts',(-18.427820698995,29.8532150044759,122.711168026723)) ;
#37593=CARTESIAN_POINT('Ctrl Pts',(-18.1824501819695,29.6732259240661,122.536018472137)) ;
#37594=CARTESIAN_POINT('Ctrl Pts',(-18.5636657279792,29.8631755470735,122.551802567031)) ;
#37595=CARTESIAN_POINT('Ctrl Pts',(-18.3522544607679,29.6831864666636,122.336809733976)) ;
#37596=CARTESIAN_POINT('Ctrl Pts',(-18.7265192984171,29.8732092325752,122.41775022895)) ;
#37597=CARTESIAN_POINT('Ctrl Pts',(-18.555819664676,29.6932201521654,122.169242143803)) ;
#37598=CARTESIAN_POINT('Ctrl Pts',(-18.9073064956514,29.8830940645654,122.315216883983)) ;
#37599=CARTESIAN_POINT('Ctrl Pts',(-18.7818025396758,29.7031049841556,122.041072921701)) ;
#37600=CARTESIAN_POINT('Ctrl Pts',(-19.1067239041188,29.8931614913253,122.244413082228)) ;
#37601=CARTESIAN_POINT('Ctrl Pts',(-19.0310733363966,29.7131724109154,121.952565569441)) ;
#37602=CARTESIAN_POINT('Ctrl Pts',(-19.3106948006957,29.9029999804841,122.209895700099)) ;
#37603=CARTESIAN_POINT('Ctrl Pts',(-19.2860369019706,29.7230109000743,121.90941606454)) ;
#37604=CARTESIAN_POINT('Ctrl Pts',(-19.5222278617027,29.9130634616742,122.211069618084)) ;
#37605=CARTESIAN_POINT('Ctrl Pts',(-19.5504531994804,29.7330743812644,121.910880737609)) ;
#37606=CARTESIAN_POINT('Ctrl Pts',(-19.7268617704073,29.9229576194894,122.24850430312)) ;
#37607=CARTESIAN_POINT('Ctrl Pts',(-19.8062464008492,29.7429685390795,121.957671456144)) ;
#37608=CARTESIAN_POINT('Ctrl Pts',(-19.9229782407006,29.9328994762337,122.320699146715)) ;
#37609=CARTESIAN_POINT('Ctrl Pts',(-20.0513931602356,29.7529103958238,122.047912589634)) ;
#37610=CARTESIAN_POINT('Ctrl Pts',(-20.1047692037057,29.9429019539051,122.426450883275)) ;
#37611=CARTESIAN_POINT('Ctrl Pts',(-20.2786332742653,29.7629128734952,122.18010000286)) ;
#37612=CARTESIAN_POINT('Ctrl Pts',(-20.2657090613012,29.9529367582094,122.562825912537)) ;
#37613=CARTESIAN_POINT('Ctrl Pts',(-20.4798098359989,29.7729476777996,122.350566712066)) ;
#37614=CARTESIAN_POINT('Ctrl Pts',(-20.3982580149733,29.962781635055,122.72180138389)) ;
#37615=CARTESIAN_POINT('Ctrl Pts',(-20.6454984301045,29.7827925546452,122.549284780263)) ;
#37616=CARTESIAN_POINT('Ctrl Pts',(-20.5029831129388,29.9727675146106,122.903710362573)) ;
#37617=CARTESIAN_POINT('Ctrl Pts',(-20.7764071388817,29.7927784342008,122.776669844113)) ;
#37618=CARTESIAN_POINT('Ctrl Pts',(-20.5743335334042,29.9827022449691,123.100047335692)) ;
#37619=CARTESIAN_POINT('Ctrl Pts',(-20.8655976910144,29.8027131645593,123.022090489165)) ;
#37620=CARTESIAN_POINT('Ctrl Pts',(-20.6107482776223,29.992760057282,123.308299706397)) ;
#37621=CARTESIAN_POINT('Ctrl Pts',(-20.9111186733623,29.8127709768721,123.282405386594)) ;
#37622=CARTESIAN_POINT('Ctrl Pts',(-20.6108122645727,30.0025806494063,123.514793587701)) ;
#37623=CARTESIAN_POINT('Ctrl Pts',(-20.9112011989826,29.8225915689965,123.540523528453)) ;
#37624=CARTESIAN_POINT('Ctrl Pts',(-20.5743946708493,30.0126472350161,123.723224917904)) ;
#37625=CARTESIAN_POINT('Ctrl Pts',(-20.8656816934945,29.8326581546063,123.801062971422)) ;
#37626=CARTESIAN_POINT('Ctrl Pts',(-20.5034684423452,30.0225468155979,123.918938589695)) ;
#37627=CARTESIAN_POINT('Ctrl Pts',(-20.7770260889006,29.8425577351881,124.0457063851)) ;
#37628=CARTESIAN_POINT('Ctrl Pts',(-20.398156180313,30.0325984152762,124.102097749828)) ;
#37629=CARTESIAN_POINT('Ctrl Pts',(-20.6453879764879,29.8526093348664,124.274656477353)) ;
#37630=CARTESIAN_POINT('Ctrl Pts',(-20.2651035498594,30.0424726016932,124.261488906871)) ;
#37631=CARTESIAN_POINT('Ctrl Pts',(-20.4790736606375,29.8624835212833,124.473897491977)) ;
#37632=CARTESIAN_POINT('Ctrl Pts',(-20.1036145885846,30.0525290775741,124.397880998235)) ;
#37633=CARTESIAN_POINT('Ctrl Pts',(-20.2772141278221,29.8725399971642,124.64438938029)) ;
#37634=CARTESIAN_POINT('Ctrl Pts',(-19.9238362938821,30.0624220088767,124.502541628328)) ;
#37635=CARTESIAN_POINT('Ctrl Pts',(-20.0524919644394,29.8824329284668,124.775217544971)) ;
#37636=CARTESIAN_POINT('Ctrl Pts',(-19.7253526604774,30.0724847875893,124.575641997785)) ;
#37637=CARTESIAN_POINT('Ctrl Pts',(-19.8043884253342,29.8924957071795,124.86659520155)) ;
#37638=CARTESIAN_POINT('Ctrl Pts',(-19.5217089265332,30.0823273131705,124.612461273804)) ;
#37639=CARTESIAN_POINT('Ctrl Pts',(-19.5498333322832,29.9023382327606,124.912621791189)) ;
#37640=CARTESIAN_POINT('Ctrl Pts',(-19.3117032501177,30.0923180785953,124.613877366419)) ;
#37641=CARTESIAN_POINT('Ctrl Pts',(-19.2873260770961,29.9123289981855,124.914394172903)) ;
#37642=CARTESIAN_POINT('Ctrl Pts',(-19.1059111788541,30.1022461545934,124.578985148832)) ;
#37643=CARTESIAN_POINT('Ctrl Pts',(-19.0300851291578,29.9222570741836,124.870781057803)) ;
#37644=CARTESIAN_POINT('Ctrl Pts',(-18.9079961280173,30.1122340649804,124.508814514259)) ;
#37645=CARTESIAN_POINT('Ctrl Pts',(-18.7826904157182,29.9322449845706,124.783069756835)) ;
#37646=CARTESIAN_POINT('Ctrl Pts',(-18.7245848851423,30.1222699771053,124.404544827108)) ;
#37647=CARTESIAN_POINT('Ctrl Pts',(-18.5534253143537,29.9422808966955,124.652734665158)) ;
#37648=CARTESIAN_POINT('Ctrl Pts',(-18.5647574103382,30.132124989953,124.272686477183)) ;
#37649=CARTESIAN_POINT('Ctrl Pts',(-18.3536388770695,29.9521359095432,124.487912827433)) ;
#37650=CARTESIAN_POINT('Ctrl Pts',(-18.4280975268948,30.1421239358693,124.11300608856)) ;
#37651=CARTESIAN_POINT('Ctrl Pts',(-18.1828123336162,29.9621348554594,124.288313606245)) ;
#37652=CARTESIAN_POINT('Ctrl Pts',(-18.3221216583478,30.1520208483173,123.933916262018)) ;
#37653=CARTESIAN_POINT('Ctrl Pts',(-18.0503403718205,29.9720317679075,124.064451745959)) ;
#37654=CARTESIAN_POINT('Ctrl Pts',(-18.2476869675524,30.1620746464108,123.736121592027)) ;
#37655=CARTESIAN_POINT('Ctrl Pts',(-17.9572951647784,29.9820855660009,123.817209301513)) ;
#37656=CARTESIAN_POINT('Ctrl Pts',(-18.209328142363,30.1719555672375,123.531942530913)) ;
#37657=CARTESIAN_POINT('Ctrl Pts',(-17.9093444926805,29.9919664868276,123.561985023858)) ;
#37658=CARTESIAN_POINT('Ctrl Pts',(-18.2065963316718,30.1819600932352,123.321657997475)) ;
#37659=CARTESIAN_POINT('Ctrl Pts',(-17.9059278138012,30.0019710128254,123.299129283871)) ;
#37660=CARTESIAN_POINT('Ctrl Pts',(-18.2404207061427,30.1919440568527,123.114471153255)) ;
#37661=CARTESIAN_POINT('Ctrl Pts',(-17.9482064112009,30.0119549764429,123.040145215729)) ;
#37662=CARTESIAN_POINT('Ctrl Pts',(-18.31026366629,30.201983697404,122.915313410186)) ;
#37663=CARTESIAN_POINT('Ctrl Pts',(-18.0355081866653,30.0219946169941,122.791197498852)) ;
#37664=CARTESIAN_POINT('Ctrl Pts',(-18.4113981835528,30.2118277230187,122.734755075974)) ;
#37665=CARTESIAN_POINT('Ctrl Pts',(-18.1619252128629,30.0318386426089,122.56549765769)) ;
#37666=CARTESIAN_POINT('Ctrl Pts',(-18.5438338536838,30.221818728836,122.571724660386)) ;
#37667=CARTESIAN_POINT('Ctrl Pts',(-18.327468580518,30.0418296484262,122.361708399331)) ;
#37668=CARTESIAN_POINT('Ctrl Pts',(-18.7036229588605,30.2318565203682,122.433886669261)) ;
#37669=CARTESIAN_POINT('Ctrl Pts',(-18.5272036339807,30.0518674399584,122.189409573073)) ;
#37670=CARTESIAN_POINT('Ctrl Pts',(-18.8812446957364,30.2417009201566,122.327651393259)) ;
#37671=CARTESIAN_POINT('Ctrl Pts',(-18.7492309039636,30.0617118397468,122.056613364002)) ;
#37672=CARTESIAN_POINT('Ctrl Pts',(-19.0771915548651,30.2516857207133,122.252443734513)) ;
#37673=CARTESIAN_POINT('Ctrl Pts',(-18.9941641262514,30.0716966403035,121.962602178219)) ;
#37674=CARTESIAN_POINT('Ctrl Pts',(-19.2823241886974,30.2616252441245,122.212483119528)) ;
#37675=CARTESIAN_POINT('Ctrl Pts',(-19.2505801464845,30.0816361637147,121.912649736789)) ;
#37676=CARTESIAN_POINT('Ctrl Pts',(-19.4933414984696,30.2716649632255,122.20875992218)) ;
#37677=CARTESIAN_POINT('Ctrl Pts',(-19.5143516088837,30.0916758828157,121.907994125339)) ;
#37678=CARTESIAN_POINT('Ctrl Pts',(-19.698697204164,30.2815531351448,122.241136729093)) ;
#37679=CARTESIAN_POINT('Ctrl Pts',(-19.7710473972824,30.101564054735,121.948463714457)) ;
#37680=CARTESIAN_POINT('Ctrl Pts',(-19.8974368961156,30.2915426975618,122.308992544338)) ;
#37681=CARTESIAN_POINT('Ctrl Pts',(-20.0194726828299,30.1115536171519,122.03328218097)) ;
#37682=CARTESIAN_POINT('Ctrl Pts',(-20.0807289084001,30.3015010697565,122.410148468044)) ;
#37683=CARTESIAN_POINT('Ctrl Pts',(-20.2485888049061,30.1215119893467,122.159725978193)) ;
#37684=CARTESIAN_POINT('Ctrl Pts',(-20.2430415790186,30.3114011439872,122.540440637745)) ;
#37685=CARTESIAN_POINT('Ctrl Pts',(-20.4514811555674,30.1314120635773,122.322590700171)) ;
#37686=CARTESIAN_POINT('Ctrl Pts',(-20.3822575057102,30.3214472403608,122.699250508298)) ;
#37687=CARTESIAN_POINT('Ctrl Pts',(-20.6255019414062,30.1414581599509,122.521102011008)) ;
#37688=CARTESIAN_POINT('Ctrl Pts',(-20.4903053212277,30.3313558243579,122.877358635903)) ;
#37689=CARTESIAN_POINT('Ctrl Pts',(-20.7605632741232,30.1513667439481,122.743737177672)) ;
#37690=CARTESIAN_POINT('Ctrl Pts',(-20.56692385887,30.3413664029488,123.073373311009)) ;
#37691=CARTESIAN_POINT('Ctrl Pts',(-20.8563375787793,30.1613773225389,122.988755129696)) ;
#37692=CARTESIAN_POINT('Ctrl Pts',(-20.6080032804155,30.3513955610616,123.280185120993)) ;
#37693=CARTESIAN_POINT('Ctrl Pts',(-20.9076881588151,30.1714064806518,123.247269528935)) ;
#37694=CARTESIAN_POINT('Ctrl Pts',(-20.6127668223826,30.3612484428997,123.487255373469)) ;
#37695=CARTESIAN_POINT('Ctrl Pts',(-20.9136438599794,30.1812593624898,123.506108579088)) ;
#37696=CARTESIAN_POINT('Ctrl Pts',(-20.5818009833245,30.3712080040507,123.694340585296)) ;
#37697=CARTESIAN_POINT('Ctrl Pts',(-20.8749374875064,30.1912189236409,123.764965708025)) ;
#37698=CARTESIAN_POINT('Ctrl Pts',(-20.5144631349101,30.3812464386398,123.894334448527)) ;
#37699=CARTESIAN_POINT('Ctrl Pts',(-20.7907663165275,30.2012573582299,124.014958246579)) ;
#37700=CARTESIAN_POINT('Ctrl Pts',(-20.4154074111559,30.3911197108669,124.076778134823)) ;
#37701=CARTESIAN_POINT('Ctrl Pts',(-20.6669470046952,30.211130630457,124.243014320162)) ;
#37702=CARTESIAN_POINT('Ctrl Pts',(-20.283556385648,30.4011929528604,124.24244097245)) ;
#37703=CARTESIAN_POINT('Ctrl Pts',(-20.5021342924087,30.2212038724506,124.450093173156)) ;
#37704=CARTESIAN_POINT('Ctrl Pts',(-20.1290404897392,30.4110132843935,124.379433616432)) ;
#37705=CARTESIAN_POINT('Ctrl Pts',(-20.3089888717368,30.2310242039837,124.621335698732)) ;
#37706=CARTESIAN_POINT('Ctrl Pts',(-19.9486420914419,30.4210919456203,124.490474607517)) ;
#37707=CARTESIAN_POINT('Ctrl Pts',(-20.0834917212071,30.2411028652105,124.760137415839)) ;
#37708=CARTESIAN_POINT('Ctrl Pts',(-19.7560754413222,30.4309435409145,124.566851656652)) ;
#37709=CARTESIAN_POINT('Ctrl Pts',(-19.8427824862029,30.2509544605047,124.855609977421)) ;
#37710=CARTESIAN_POINT('Ctrl Pts',(-19.5487326187181,30.4410166761433,124.609735878305)) ;
#37711=CARTESIAN_POINT('Ctrl Pts',(-19.5836045391688,30.2610275957335,124.909215904184)) ;
#37712=CARTESIAN_POINT('Ctrl Pts',(-19.3418837703433,30.4508591116683,124.615794712703)) ;
#37713=CARTESIAN_POINT('Ctrl Pts',(-19.325042085663,30.2708700312585,124.916790254911)) ;
#37714=CARTESIAN_POINT('Ctrl Pts',(-19.1341767024053,30.4608398808017,124.586121780913)) ;
#37715=CARTESIAN_POINT('Ctrl Pts',(-19.06540787512,30.2808508003919,124.879699535885)) ;
#37716=CARTESIAN_POINT('Ctrl Pts',(-18.9341621364853,30.4708569820456,124.520222155215)) ;
#37717=CARTESIAN_POINT('Ctrl Pts',(-18.8153894690944,30.2908679016358,124.797325621864)) ;
#37718=CARTESIAN_POINT('Ctrl Pts',(-18.7508125062853,30.4807454296474,124.422211803213)) ;
#37719=CARTESIAN_POINT('Ctrl Pts',(-18.5862012534793,30.3007563492376,124.674812609877)) ;
#37720=CARTESIAN_POINT('Ctrl Pts',(-18.5845129446099,30.4908011438283,124.291721984471)) ;
#37721=CARTESIAN_POINT('Ctrl Pts',(-18.3783267486682,30.3108120634185,124.511700910581)) ;
#37722=CARTESIAN_POINT('Ctrl Pts',(-18.44588508889,30.5006763502421,124.137161226805)) ;
#37723=CARTESIAN_POINT('Ctrl Pts',(-18.2050407984667,30.3206872698323,124.318499416567)) ;
#37724=CARTESIAN_POINT('Ctrl Pts',(-18.3344500450704,30.5106714027149,123.959022928956)) ;
#37725=CARTESIAN_POINT('Ctrl Pts',(-18.0657466674759,30.330682322305,124.095826539114)) ;
#37726=CARTESIAN_POINT('Ctrl Pts',(-18.2557384460612,30.520693286677,123.763577906026)) ;
#37727=CARTESIAN_POINT('Ctrl Pts',(-17.9673568014164,30.3407042062672,123.851520456644)) ;
#37728=CARTESIAN_POINT('Ctrl Pts',(-18.2124447067718,30.5305972592063,123.559917806185)) ;
#37729=CARTESIAN_POINT('Ctrl Pts',(-17.9132391132283,30.3506081787965,123.596944459878)) ;
#37730=CARTESIAN_POINT('Ctrl Pts',(-18.204806352772,30.5405857558672,123.350065475818)) ;
#37731=CARTESIAN_POINT('Ctrl Pts',(-17.9036909634777,30.3605966754573,123.334628818857)) ;
#37732=CARTESIAN_POINT('Ctrl Pts',(-18.2337889801412,30.5505495531152,123.142620805064)) ;
#37733=CARTESIAN_POINT('Ctrl Pts',(-17.9399190540349,30.3705604727053,123.075322497825)) ;
#37734=CARTESIAN_POINT('Ctrl Pts',(-18.2974874686317,30.5604535764232,122.944369701572)) ;
#37735=CARTESIAN_POINT('Ctrl Pts',(-18.0195424014085,30.3804644960134,122.827507706728)) ;
#37736=CARTESIAN_POINT('Ctrl Pts',(-18.3963113380305,30.5705140797448,122.757403023843)) ;
#37737=CARTESIAN_POINT('Ctrl Pts',(-18.1430719622908,30.390524999335,122.593799613833)) ;
#37738=CARTESIAN_POINT('Ctrl Pts',(-18.5230838015688,30.5803546148847,122.593882778984)) ;
#37739=CARTESIAN_POINT('Ctrl Pts',(-18.3015384279118,30.4003655344749,122.389398133956)) ;
#37740=CARTESIAN_POINT('Ctrl Pts',(-18.6795561688118,30.5904168355893,122.451559837919)) ;
#37741=CARTESIAN_POINT('Ctrl Pts',(-18.4971286723623,30.4104277551794,122.211494770996)) ;
#37742=CARTESIAN_POINT('Ctrl Pts',(-18.8555743115362,30.6003139893655,122.340587366803)) ;
#37743=CARTESIAN_POINT('Ctrl Pts',(-18.7171521979326,30.4203249089557,122.072778646535)) ;
#37744=CARTESIAN_POINT('Ctrl Pts',(-19.0485703229917,30.610245122751,122.260955111829)) ;
#37745=CARTESIAN_POINT('Ctrl Pts',(-18.9583979844266,30.4302560423412,121.973238308994)) ;
#37746=CARTESIAN_POINT('Ctrl Pts',(-19.2547965608815,30.6202874978967,122.215768412004)) ;
#37747=CARTESIAN_POINT('Ctrl Pts',(-19.2161806172609,30.4402984174869,121.916755158217)) ;
#37748=CARTESIAN_POINT('Ctrl Pts',(-19.4624589820246,30.6301734356628,122.207050198295)) ;
#37749=CARTESIAN_POINT('Ctrl Pts',(-19.4757597411962,30.450184355253,121.9058575907)) ;
#37750=CARTESIAN_POINT('Ctrl Pts',(-19.6707860504758,30.6401692786477,122.234500227154)) ;
#37751=CARTESIAN_POINT('Ctrl Pts',(-19.7361687240482,30.4601801982378,121.940170526938)) ;
#37752=CARTESIAN_POINT('Ctrl Pts',(-19.8701217771489,30.6501112565263,122.297396578507)) ;
#37753=CARTESIAN_POINT('Ctrl Pts',(-19.9853388632979,30.4701221761165,122.01879150235)) ;
#37754=CARTESIAN_POINT('Ctrl Pts',(-20.0559439542631,30.6600706310073,122.393853881732)) ;
#37755=CARTESIAN_POINT('Ctrl Pts',(-20.2176167859289,30.4800815505974,122.13936377116)) ;
#37756=CARTESIAN_POINT('Ctrl Pts',(-20.2229095752647,30.6700672468411,122.521521564149)) ;
#37757=CARTESIAN_POINT('Ctrl Pts',(-20.4263236161988,30.4900781664312,122.298948878798)) ;
#37758=CARTESIAN_POINT('Ctrl Pts',(-20.3654814517331,30.6801014654146,122.676991794271)) ;
#37759=CARTESIAN_POINT('Ctrl Pts',(-20.6045380696122,30.5001123850047,122.493286837785)) ;
#37760=CARTESIAN_POINT('Ctrl Pts',(-20.4770590422529,30.6899545326252,122.851511404317)) ;
#37761=CARTESIAN_POINT('Ctrl Pts',(-20.7440103711804,30.5099654522154,122.711437778159)) ;
#37762=CARTESIAN_POINT('Ctrl Pts',(-20.5580675426808,30.6999147905028,123.044595067161)) ;
#37763=CARTESIAN_POINT('Ctrl Pts',(-20.8452704863251,30.5199257100929,122.95279307228)) ;
#37764=CARTESIAN_POINT('Ctrl Pts',(-20.6044003781511,30.7099438172084,123.250294695878)) ;
#37765=CARTESIAN_POINT('Ctrl Pts',(-20.9031858778031,30.5299547367985,123.209917654141)) ;
#37766=CARTESIAN_POINT('Ctrl Pts',(-20.6142563398137,30.7198540242428,123.458395760156)) ;
#37767=CARTESIAN_POINT('Ctrl Pts',(-20.9155052004017,30.539864943833,123.47004489255)) ;
#37768=CARTESIAN_POINT('Ctrl Pts',(-20.5883067682827,30.7297889348904,123.665646410074)) ;
#37769=CARTESIAN_POINT('Ctrl Pts',(-20.8830672768475,30.5497998544806,123.729108751016)) ;
#37770=CARTESIAN_POINT('Ctrl Pts',(-20.525923055177,30.7398300650696,123.867307187014)) ;
#37771=CARTESIAN_POINT('Ctrl Pts',(-20.8050869197555,30.5598409846598,123.981184304472)) ;
#37772=CARTESIAN_POINT('Ctrl Pts',(-20.4310732674177,30.7497172054396,124.052276123954)) ;
#37773=CARTESIAN_POINT('Ctrl Pts',(-20.686523442515,30.5697281250298,124.212396007717)) ;
#37774=CARTESIAN_POINT('Ctrl Pts',(-20.3045079136013,30.7597094829755,124.219919068454)) ;
#37775=CARTESIAN_POINT('Ctrl Pts',(-20.5283158328831,30.5797204025657,124.421949250834)) ;
#37776=CARTESIAN_POINT('Ctrl Pts',(-20.1513705963158,30.7696580262439,124.36238740214)) ;
#37777=CARTESIAN_POINT('Ctrl Pts',(-20.3368931275414,30.589668945834,124.600034326039)) ;
#37778=CARTESIAN_POINT('Ctrl Pts',(-19.97621673164,30.7795947010611,124.476202086606)) ;
#37779=CARTESIAN_POINT('Ctrl Pts',(-20.117949669765,30.5996056206513,124.742302120587)) ;
#37780=CARTESIAN_POINT('Ctrl Pts',(-19.7831216512904,30.7895781219974,124.558506793433)) ;
#37781=CARTESIAN_POINT('Ctrl Pts',(-19.8765801266948,30.6095890415876,124.845182022311)) ;
#37782=CARTESIAN_POINT('Ctrl Pts',(-19.577416346165,30.7996204371867,124.605973059919)) ;
#37783=CARTESIAN_POINT('Ctrl Pts',(-19.6194484246189,30.6196313567769,124.904513792587)) ;
#37784=CARTESIAN_POINT('Ctrl Pts',(-19.3708401231471,30.8094607546259,124.617114838702)) ;
#37785=CARTESIAN_POINT('Ctrl Pts',(-19.3612267210276,30.6294716742161,124.918439915282)) ;
#37786=CARTESIAN_POINT('Ctrl Pts',(-19.1614550331297,30.8194904586834,124.592230575313)) ;
#37787=CARTESIAN_POINT('Ctrl Pts',(-19.0994956243857,30.6395013782735,124.887333257239)) ;
#37788=CARTESIAN_POINT('Ctrl Pts',(-18.9599146448353,30.8295114154059,124.530878822072)) ;
#37789=CARTESIAN_POINT('Ctrl Pts',(-18.8475705007407,30.6495223349961,124.810642476256)) ;
#37790=CARTESIAN_POINT('Ctrl Pts',(-18.7747291699173,30.8393779577095,124.437402415365)) ;
#37791=CARTESIAN_POINT('Ctrl Pts',(-18.6160882477123,30.6593888772996,124.693795263407)) ;
#37792=CARTESIAN_POINT('Ctrl Pts',(-18.6051688450948,30.8494490576546,124.310638457262)) ;
#37793=CARTESIAN_POINT('Ctrl Pts',(-18.404138945044,30.6694599772448,124.535339469845)) ;
#37794=CARTESIAN_POINT('Ctrl Pts',(-18.4634769424933,30.8592911318322,124.159844576277)) ;
#37795=CARTESIAN_POINT('Ctrl Pts',(-18.22702415179,30.6793020514224,124.346845255136)) ;
#37796=CARTESIAN_POINT('Ctrl Pts',(-18.3481138935015,30.8692519264192,123.98508540905)) ;
#37797=CARTESIAN_POINT('Ctrl Pts',(-18.0828214570225,30.6892628460094,124.128395071052)) ;
#37798=CARTESIAN_POINT('Ctrl Pts',(-18.2645872120616,30.8792897993201,123.791299482673)) ;
#37799=CARTESIAN_POINT('Ctrl Pts',(-17.9784145005969,30.6993007189103,123.886162207507)) ;
#37800=CARTESIAN_POINT('Ctrl Pts',(-18.2163875155882,30.8891640848642,123.589358215528)) ;
#37801=CARTESIAN_POINT('Ctrl Pts',(-17.9181661939487,30.7091750044543,123.633734267032)) ;
#37802=CARTESIAN_POINT('Ctrl Pts',(-18.203753574643,30.8992338352781,123.378065938577)) ;
#37803=CARTESIAN_POINT('Ctrl Pts',(-17.902375375643,30.7192447548683,123.369619175595)) ;
#37804=CARTESIAN_POINT('Ctrl Pts',(-18.2273236827773,30.9090671198127,123.172670784879)) ;
#37805=CARTESIAN_POINT('Ctrl Pts',(-17.9318397717287,30.7290780394029,123.112874144426)) ;
#37806=CARTESIAN_POINT('Ctrl Pts',(-18.2867987026179,30.9190974606128,122.970368878916)) ;
#37807=CARTESIAN_POINT('Ctrl Pts',(-18.0061852689319,30.739108380203,122.85999735939)) ;
#37808=CARTESIAN_POINT('Ctrl Pts',(-18.3810728614528,30.9291293846124,122.781698599394)) ;
#37809=CARTESIAN_POINT('Ctrl Pts',(-18.1240293774352,30.7491403042026,122.624160309283)) ;
#37810=CARTESIAN_POINT('Ctrl Pts',(-18.50375518637,30.9389579195483,122.6154474201)) ;
#37811=CARTESIAN_POINT('Ctrl Pts',(-18.2773844644473,30.7589688391385,122.416346355299)) ;
#37812=CARTESIAN_POINT('Ctrl Pts',(-18.6555659033438,30.948951697313,122.470205569998)) ;
#37813=CARTESIAN_POINT('Ctrl Pts',(-18.4671493140106,30.7689626169032,122.23479534461)) ;
#37814=CARTESIAN_POINT('Ctrl Pts',(-18.8311197714127,30.9589794077985,122.353474256892)) ;
#37815=CARTESIAN_POINT('Ctrl Pts',(-18.6865926220437,30.7789903273887,122.088882738847)) ;
#37816=CARTESIAN_POINT('Ctrl Pts',(-19.021483587405,30.9688678186325,122.269936336135)) ;
#37817=CARTESIAN_POINT('Ctrl Pts',(-18.9245489185177,30.7888787382227,121.984461740801)) ;
#37818=CARTESIAN_POINT('Ctrl Pts',(-19.2251633873121,30.978844669168,122.219928658385)) ;
#37819=CARTESIAN_POINT('Ctrl Pts',(-19.1791493957225,30.7988555887582,121.92195402928)) ;
#37820=CARTESIAN_POINT('Ctrl Pts',(-19.4347905985392,30.9888364657185,122.206004671817)) ;
#37821=CARTESIAN_POINT('Ctrl Pts',(-19.4411836962551,30.8088473853087,121.904551040797)) ;
#37822=CARTESIAN_POINT('Ctrl Pts',(-19.6445006365015,30.9988724718122,122.229041741586)) ;
#37823=CARTESIAN_POINT('Ctrl Pts',(-19.7033209422689,30.8188833914023,121.933349289117)) ;
#37824=CARTESIAN_POINT('Ctrl Pts',(-19.8434060708219,31.008723206075,122.286751984525)) ;
#37825=CARTESIAN_POINT('Ctrl Pts',(-19.9519531581961,30.8287341256652,122.005489324645)) ;
#37826=CARTESIAN_POINT('Ctrl Pts',(-20.0320403039582,31.0187144646032,122.379080702505)) ;
#37827=CARTESIAN_POINT('Ctrl Pts',(-20.1877451627324,30.8387253841934,122.120902211043)) ;
#37828=CARTESIAN_POINT('Ctrl Pts',(-20.2006501988176,31.0286323595064,122.501784715894)) ;
#37829=CARTESIAN_POINT('Ctrl Pts',(-20.3985067246946,30.8486432790966,122.274284311922)) ;
#37830=CARTESIAN_POINT('Ctrl Pts',(-20.3470107237814,31.0386605011694,122.65350091565)) ;
#37831=CARTESIAN_POINT('Ctrl Pts',(-20.58145578964,30.8586714207596,122.463931047344)) ;
#37832=CARTESIAN_POINT('Ctrl Pts',(-20.4632104004851,31.0485456692853,122.825802329779)) ;
#37833=CARTESIAN_POINT('Ctrl Pts',(-20.7267039760268,30.8685565888754,122.679309656384)) ;
#37834=CARTESIAN_POINT('Ctrl Pts',(-20.5490845959354,31.0585350327913,123.017454794976)) ;
#37835=CARTESIAN_POINT('Ctrl Pts',(-20.8340446604861,30.8785459523814,122.918876333031)) ;
#37836=CARTESIAN_POINT('Ctrl Pts',(-20.6002096975552,31.0685761678013,123.22226668955)) ;
#37837=CARTESIAN_POINT('Ctrl Pts',(-20.8979488652551,30.8885870873915,123.17489164825)) ;
#37838=CARTESIAN_POINT('Ctrl Pts',(-20.615028805326,31.0784088359894,123.42844428818)) ;
#37839=CARTESIAN_POINT('Ctrl Pts',(-20.9164705231376,30.8984197555796,123.43261476882)) ;
#37840=CARTESIAN_POINT('Ctrl Pts',(-20.5940744638475,31.0884027389439,123.637499008543)) ;
#37841=CARTESIAN_POINT('Ctrl Pts',(-20.8902751542732,30.908413658534,123.69393304665)) ;
#37842=CARTESIAN_POINT('Ctrl Pts',(-20.5365069814263,31.0984320240284,123.840336990073)) ;
#37843=CARTESIAN_POINT('Ctrl Pts',(-20.8183135578926,30.9184429436185,123.94747986394)) ;
#37844=CARTESIAN_POINT('Ctrl Pts',(-20.446304755453,31.1083075524703,124.027344707869)) ;
#37845=CARTESIAN_POINT('Ctrl Pts',(-20.7055583075016,30.9283184720605,124.181239071711)) ;
#37846=CARTESIAN_POINT('Ctrl Pts',(-20.3236808566818,31.1183078350863,124.198085320137)) ;
#37847=CARTESIAN_POINT('Ctrl Pts',(-20.5522763631696,30.9383187546765,124.394663488977)) ;
#37848=CARTESIAN_POINT('Ctrl Pts',(-20.1746825112907,31.1282198511434,124.343800205569)) ;
#37849=CARTESIAN_POINT('Ctrl Pts',(-20.3660263502504,30.9482307707336,124.576805637023)) ;
#37850=CARTESIAN_POINT('Ctrl Pts',(-20.0004530429304,31.1382619264824,124.46299621068)) ;
#37851=CARTESIAN_POINT('Ctrl Pts',(-20.1482381590655,30.9582728460726,124.72579853176)) ;
#37852=CARTESIAN_POINT('Ctrl Pts',(-19.8108716546696,31.1481617591385,124.548900830841)) ;
#37853=CARTESIAN_POINT('Ctrl Pts',(-19.9112599341411,30.9681726787286,124.833177229077)) ;
#37854=CARTESIAN_POINT('Ctrl Pts',(-19.6074951368638,31.1581541597165,124.601515467069)) ;
#37855=CARTESIAN_POINT('Ctrl Pts',(-19.6570385216624,30.9781650793067,124.898943043769)) ;
#37856=CARTESIAN_POINT('Ctrl Pts',(-19.3971675954827,31.1681881814759,124.617712800031)) ;
#37857=CARTESIAN_POINT('Ctrl Pts',(-19.3941289164033,30.988199101066,124.919187191748)) ;
#37858=CARTESIAN_POINT('Ctrl Pts',(-19.1907487982186,31.1780527923171,124.59775750716)) ;
#37859=CARTESIAN_POINT('Ctrl Pts',(-19.1361050769599,30.9980637119073,124.894240456092)) ;
#37860=CARTESIAN_POINT('Ctrl Pts',(-18.9881977091377,31.1880451917782,124.542038359077)) ;
#37861=CARTESIAN_POINT('Ctrl Pts',(-18.8829168165826,31.0080561113684,124.824588928415)) ;
#37862=CARTESIAN_POINT('Ctrl Pts',(-18.7978278631162,31.1980771451111,124.451266994197)) ;
#37863=CARTESIAN_POINT('Ctrl Pts',(-18.6449556256529,31.0180880647013,124.711122383889)) ;
#37864=CARTESIAN_POINT('Ctrl Pts',(-18.6287533564004,31.2079435040528,124.331095273272)) ;
#37865=CARTESIAN_POINT('Ctrl Pts',(-18.4336135989421,31.027954423643,124.56090527818)) ;
#37866=CARTESIAN_POINT('Ctrl Pts',(-18.4811055178957,31.2179309795386,124.181843664757)) ;
#37867=CARTESIAN_POINT('Ctrl Pts',(-18.2490556294544,31.0379418991288,124.374338785547)) ;
#37868=CARTESIAN_POINT('Ctrl Pts',(-18.3620004505735,31.2278758857271,124.009975732587)) ;
#37869=CARTESIAN_POINT('Ctrl Pts',(-18.1001763826334,31.0478868053173,124.159502137158)) ;
#37870=CARTESIAN_POINT('Ctrl Pts',(-18.2737974644408,31.2379208503873,123.81812345337)) ;
#37871=CARTESIAN_POINT('Ctrl Pts',(-17.9899251036458,31.0579317699775,123.919685682754)) ;
#37872=CARTESIAN_POINT('Ctrl Pts',(-18.2210312867946,31.2477826572922,123.617606509006)) ;
#37873=CARTESIAN_POINT('Ctrl Pts',(-17.923969894662,31.0677935768823,123.669038395276)) ;
#37874=CARTESIAN_POINT('Ctrl Pts',(-18.2032568478729,31.2577753295979,123.408304026805)) ;
#37875=CARTESIAN_POINT('Ctrl Pts',(-17.9017545883621,31.0777862491881,123.407409964502)) ;
#37876=CARTESIAN_POINT('Ctrl Pts',(-18.222001276921,31.2677040005433,123.200401767921)) ;
#37877=CARTESIAN_POINT('Ctrl Pts',(-17.9251878867363,31.0877149201334,123.147532162206)) ;
#37878=CARTESIAN_POINT('Ctrl Pts',(-18.2763524420486,31.2776565427686,122.998365459932)) ;
#37879=CARTESIAN_POINT('Ctrl Pts',(-17.9931295755883,31.0976674623588,122.894987346487)) ;
#37880=CARTESIAN_POINT('Ctrl Pts',(-18.3653072061262,31.2876578987645,122.807825356539)) ;
#37881=CARTESIAN_POINT('Ctrl Pts',(-18.1043255908687,31.1076688183546,122.656813330309)) ;
#37882=CARTESIAN_POINT('Ctrl Pts',(-18.4865417491966,31.2976865110392,122.635347065935)) ;
#37883=CARTESIAN_POINT('Ctrl Pts',(-18.2558710625167,31.1176974306294,122.441217023583)) ;
#37884=CARTESIAN_POINT('Ctrl Pts',(-18.6332380965549,31.3075508455887,122.488744885021)) ;
#37885=CARTESIAN_POINT('Ctrl Pts',(-18.4392436559593,31.1275617651789,122.257966085738)) ;
#37886=CARTESIAN_POINT('Ctrl Pts',(-18.8051439882642,31.3175431696653,122.36805505233)) ;
#37887=CARTESIAN_POINT('Ctrl Pts',(-18.6541277020342,31.1375540892555,122.107106052704)) ;
#37888=CARTESIAN_POINT('Ctrl Pts',(-18.9941591698767,31.3274706620311,122.279486435379)) ;
#37889=CARTESIAN_POINT('Ctrl Pts',(-18.8903979931556,31.1474815816213,121.996397771836)) ;
#37890=CARTESIAN_POINT('Ctrl Pts',(-19.1976565576999,31.337498020582,122.224557944539)) ;
#37891=CARTESIAN_POINT('Ctrl Pts',(-19.1447705223737,31.1575089401722,121.927739862288)) ;
#37892=CARTESIAN_POINT('Ctrl Pts',(-19.4046860684407,31.3473844386331,122.205835676361)) ;
#37893=CARTESIAN_POINT('Ctrl Pts',(-19.4035577854677,31.1673953582233,121.904339822877)) ;
#37894=CARTESIAN_POINT('Ctrl Pts',(-19.6148093834641,31.3574161733685,122.223490530873)) ;
#37895=CARTESIAN_POINT('Ctrl Pts',(-19.6662117594047,31.1774270929587,121.926411212901)) ;
#37896=CARTESIAN_POINT('Ctrl Pts',(-19.8157458443054,31.3672977546117,122.27637611023)) ;
#37897=CARTESIAN_POINT('Ctrl Pts',(-19.9173816828767,31.1873086742019,121.992520931591)) ;
#37898=CARTESIAN_POINT('Ctrl Pts',(-20.0078493459752,31.3773597326441,122.364859285606)) ;
#37899=CARTESIAN_POINT('Ctrl Pts',(-20.1575099537051,31.1973706522342,122.103127502603)) ;
#37900=CARTESIAN_POINT('Ctrl Pts',(-20.1782249889718,31.3872168110058,122.482873113296)) ;
#37901=CARTESIAN_POINT('Ctrl Pts',(-20.3704779129066,31.207227730596,122.250647114484)) ;
#37902=CARTESIAN_POINT('Ctrl Pts',(-20.3278279199944,31.3972113841118,122.630365681166)) ;
#37903=CARTESIAN_POINT('Ctrl Pts',(-20.5574796354709,31.217222303702,122.435014859844)) ;
#37904=CARTESIAN_POINT('Ctrl Pts',(-20.4488094488748,31.4071371803994,122.800422727047)) ;
#37905=CARTESIAN_POINT('Ctrl Pts',(-20.7087042531186,31.2271480999896,122.647587798047)) ;
#37906=CARTESIAN_POINT('Ctrl Pts',(-20.5393550256187,31.4171625475691,122.990728200173)) ;
#37907=CARTESIAN_POINT('Ctrl Pts',(-20.8218837392503,31.2371734671593,122.885470873047)) ;
#37908=CARTESIAN_POINT('Ctrl Pts',(-20.5948502492867,31.427058627223,123.191245455736)) ;
#37909=CARTESIAN_POINT('Ctrl Pts',(-20.8912500206814,31.2470695468132,123.136118325627)) ;
#37910=CARTESIAN_POINT('Ctrl Pts',(-20.6153065851422,31.4370537069285,123.400378513475)) ;
#37911=CARTESIAN_POINT('Ctrl Pts',(-20.9168177978967,31.2570646265187,123.397534145114)) ;
#37912=CARTESIAN_POINT('Ctrl Pts',(-20.5987327650594,31.4470787947444,123.610482201889)) ;
#37913=CARTESIAN_POINT('Ctrl Pts',(-20.8960973228118,31.2670897143346,123.66016667256)) ;
#37914=CARTESIAN_POINT('Ctrl Pts',(-20.5297708945593,31.4602626171116,123.878943016611)) ;
#37915=CARTESIAN_POINT('Ctrl Pts',(-20.8098934767171,31.2802735367018,123.995726533584)) ;
#37916=CARTESIAN_POINT('Ctrl Pts',(-20.3913865952829,31.4735847352576,124.126114166337)) ;
#37917=CARTESIAN_POINT('Ctrl Pts',(-20.6369390480792,31.2935956548477,124.304662239596)) ;
#37918=CARTESIAN_POINT('Ctrl Pts',(-20.1945187909929,31.4869639448852,124.327003652239)) ;
#37919=CARTESIAN_POINT('Ctrl Pts',(-20.3908148582796,31.3069748644754,124.555818133177)) ;
#37920=CARTESIAN_POINT('Ctrl Pts',(-20.0266170027822,31.4968021821294,124.447815006563)) ;
#37921=CARTESIAN_POINT('Ctrl Pts',(-20.1809438415155,31.3168131017196,124.706820601869)) ;
#37922=CARTESIAN_POINT('Ctrl Pts',(-19.8359227028424,31.5068751053881,124.539840727089)) ;
#37923=CARTESIAN_POINT('Ctrl Pts',(-19.9425721440024,31.3268860249783,124.821852782607)) ;
#37924=CARTESIAN_POINT('Ctrl Pts',(-19.6364695609574,31.5167317468432,124.596111822066)) ;
#37925=CARTESIAN_POINT('Ctrl Pts',(-19.6932575438863,31.3367426664334,124.892188886097)) ;
#37926=CARTESIAN_POINT('Ctrl Pts',(-19.4276732492853,31.5267171223493,124.617725780505)) ;
#37927=CARTESIAN_POINT('Ctrl Pts',(-19.4322556852205,31.3467280419395,124.919201640544)) ;
#37928=CARTESIAN_POINT('Ctrl Pts',(-19.1491517758467,31.5400011538097,124.597557778909)) ;
#37929=CARTESIAN_POINT('Ctrl Pts',(-19.0841345591843,31.3600120733999,124.89399942422)) ;
#37930=CARTESIAN_POINT('Ctrl Pts',(-18.8168268265356,31.55651994568,124.4835998274)) ;
#37931=CARTESIAN_POINT('Ctrl Pts',(-18.6686831094872,31.3765308652702,124.751522351266)) ;
#37932=CARTESIAN_POINT('Ctrl Pts',(-18.5395236647983,31.5733056626867,124.258964597931)) ;
#37933=CARTESIAN_POINT('Ctrl Pts',(-18.3221176258068,31.3933165822769,124.470780415022)) ;
#37934=CARTESIAN_POINT('Ctrl Pts',(-18.3774782260285,31.5864188111957,124.035919217362)) ;
#37935=CARTESIAN_POINT('Ctrl Pts',(-18.11951716402,31.4064297307859,124.19192546982)) ;
#37936=CARTESIAN_POINT('Ctrl Pts',(-18.2842368170373,31.5964543602758,123.846684019974)) ;
#37937=CARTESIAN_POINT('Ctrl Pts',(-18.0029767277988,31.416465279866,123.955390640445)) ;
#37938=CARTESIAN_POINT('Ctrl Pts',(-18.2259601248409,31.6064704164553,123.644318949324)) ;
#37939=CARTESIAN_POINT('Ctrl Pts',(-17.9301311612178,31.4264813360454,123.702427282668)) ;
#37940=CARTESIAN_POINT('Ctrl Pts',(-18.1960923933868,31.6196484523213,123.368912551157)) ;
#37941=CARTESIAN_POINT('Ctrl Pts',(-17.8927981854037,31.4396593719114,123.358188928684)) ;
#37942=CARTESIAN_POINT('Ctrl Pts',(-18.2490034102453,31.6362503295084,123.019854463279)) ;
#37943=CARTESIAN_POINT('Ctrl Pts',(-17.958942776027,31.4562612490985,122.921846253588)) ;
#37944=CARTESIAN_POINT('Ctrl Pts',(-18.4541225555357,31.6563134741243,122.64582032832)) ;
#37945=CARTESIAN_POINT('Ctrl Pts',(-18.2153452936245,31.4763243937144,122.454312103311)) ;
#37946=CARTESIAN_POINT('Ctrl Pts',(-18.7702542503997,31.676114364208,122.367683074125)) ;
#37947=CARTESIAN_POINT('Ctrl Pts',(-18.6105119795109,31.4961252837982,122.106643007556)) ;
#37948=CARTESIAN_POINT('Ctrl Pts',(-19.1646379113021,31.6960574894867,122.212071616699)) ;
#37949=CARTESIAN_POINT('Ctrl Pts',(-19.1034924936839,31.5160684090769,121.912133008528)) ;
#37950=CARTESIAN_POINT('Ctrl Pts',(-19.5875617432602,31.7159555346063,122.200691268626)) ;
#37951=CARTESIAN_POINT('Ctrl Pts',(-19.632146534188,31.5359664541965,121.897911371851)) ;
#37952=CARTESIAN_POINT('Ctrl Pts',(-19.9891315337937,31.735841294233,122.333252820407)) ;
#37953=CARTESIAN_POINT('Ctrl Pts',(-20.1341066883762,31.5558522138232,122.063616102394)) ;
#37954=CARTESIAN_POINT('Ctrl Pts',(-20.3238700828937,31.7559064694129,122.597717645849)) ;
#37955=CARTESIAN_POINT('Ctrl Pts',(-20.5525283111151,31.5759173890031,122.394200252116)) ;
#37956=CARTESIAN_POINT('Ctrl Pts',(-20.5455304831707,31.7757331125157,122.956392108189)) ;
#37957=CARTESIAN_POINT('Ctrl Pts',(-20.8296000416623,31.5957440321059,122.84254361494)) ;
#37958=CARTESIAN_POINT('Ctrl Pts',(-20.6329476537698,31.7956418219641,123.370466525032)) ;
#37959=CARTESIAN_POINT('Ctrl Pts',(-20.938868749629,31.6156527415543,123.360136077139)) ;
#37960=CARTESIAN_POINT('Ctrl Pts',(-20.5737577153688,31.8155936589959,123.790666742913)) ;
#37961=CARTESIAN_POINT('Ctrl Pts',(-20.8648791196571,31.635604578586,123.885385533436)) ;
#37962=CARTESIAN_POINT('Ctrl Pts',(-20.3736372597136,31.835602133699,124.166043131573)) ;
#37963=CARTESIAN_POINT('Ctrl Pts',(-20.61472624886,31.6556130532892,124.354604941033)) ;
#37964=CARTESIAN_POINT('Ctrl Pts',(-20.0609970576513,31.8554035924605,124.448061776785)) ;
#37965=CARTESIAN_POINT('Ctrl Pts',(-20.2239265792677,31.6754145120507,124.707125000018)) ;
#37966=CARTESIAN_POINT('Ctrl Pts',(-19.6682512234286,31.8753604806964,124.608723454266)) ;
#37967=CARTESIAN_POINT('Ctrl Pts',(-19.7329944592296,31.6953714002866,124.907950847029)) ;
#37968=CARTESIAN_POINT('Ctrl Pts',(-19.2436603324159,31.8953443181105,124.624778169694)) ;
#37969=CARTESIAN_POINT('Ctrl Pts',(-19.2022559885515,31.7153552377007,124.928017723772)) ;
#37970=CARTESIAN_POINT('Ctrl Pts',(-18.8422996219988,31.9151527573315,124.496909348728)) ;
#37971=CARTESIAN_POINT('Ctrl Pts',(-18.7005580952359,31.7351636769217,124.7681819531)) ;
#37972=CARTESIAN_POINT('Ctrl Pts',(-18.5055590914568,31.9351384667117,124.237910045326)) ;
#37973=CARTESIAN_POINT('Ctrl Pts',(-18.279632753258,31.7551493863019,124.444432947337)) ;
#37974=CARTESIAN_POINT('Ctrl Pts',(-18.2784623208037,31.955007989727,123.881451590909)) ;
#37975=CARTESIAN_POINT('Ctrl Pts',(-17.9957625955385,31.7750189093172,123.998861683827)) ;
#37976=CARTESIAN_POINT('Ctrl Pts',(-18.1861815675504,31.9750287288442,123.466043557042)) ;
#37977=CARTESIAN_POINT('Ctrl Pts',(-17.8804111930081,31.7950396484344,123.479601508634)) ;
#37978=CARTESIAN_POINT('Ctrl Pts',(-18.2401047055373,31.9948327938211,123.04826047757)) ;
#37979=CARTESIAN_POINT('Ctrl Pts',(-17.9478137324898,31.8148437134113,122.957375358407)) ;
#37980=CARTESIAN_POINT('Ctrl Pts',(-18.4356159524676,32.0148947575519,122.669266623573)) ;
#37981=CARTESIAN_POINT('Ctrl Pts',(-18.1922019497026,31.8349056771421,122.483631625213)) ;
#37982=CARTESIAN_POINT('Ctrl Pts',(-18.7455928392011,32.0347279378404,122.383198650126)) ;
#37983=CARTESIAN_POINT('Ctrl Pts',(-18.5796705035048,31.8547388574305,122.126047237361)) ;
#37984=CARTESIAN_POINT('Ctrl Pts',(-19.1356511664417,32.0546471351664,122.218343920433)) ;
#37985=CARTESIAN_POINT('Ctrl Pts',(-19.0672415406951,31.8746580547566,121.919977102757)) ;
#37986=CARTESIAN_POINT('Ctrl Pts',(-19.5590376558123,32.0745851602798,122.196738769831)) ;
#37987=CARTESIAN_POINT('Ctrl Pts',(-19.5964737982828,31.8945960798699,121.892968380633)) ;
#37988=CARTESIAN_POINT('Ctrl Pts',(-19.9633771695477,32.0944632063358,122.319975235754)) ;
#37989=CARTESIAN_POINT('Ctrl Pts',(-20.101897742519,31.914474125926,122.04701086148)) ;
#37990=CARTESIAN_POINT('Ctrl Pts',(-20.3031500801308,32.1144479406239,122.575069386705)) ;
#37991=CARTESIAN_POINT('Ctrl Pts',(-20.5266155989979,31.9344588602141,122.365876034271)) ;
#37992=CARTESIAN_POINT('Ctrl Pts',(-20.5347790537855,32.1343587573024,122.929588130013)) ;
#37993=CARTESIAN_POINT('Ctrl Pts',(-20.8161540517075,31.9543696768926,122.809022005438)) ;
#37994=CARTESIAN_POINT('Ctrl Pts',(-20.6316344190319,32.1543577328211,123.343539091195)) ;
#37995=CARTESIAN_POINT('Ctrl Pts',(-20.9372264314163,31.9743686524113,123.326459903435)) ;
#37996=CARTESIAN_POINT('Ctrl Pts',(-20.5824108030896,32.1741626534663,123.761844882659)) ;
#37997=CARTESIAN_POINT('Ctrl Pts',(-20.8757007543039,31.9941735730565,123.84934083429)) ;
#37998=CARTESIAN_POINT('Ctrl Pts',(-20.3923321685515,32.1941466137575,124.141760103579)) ;
#37999=CARTESIAN_POINT('Ctrl Pts',(-20.638106149318,32.0141575333477,124.324236585246)) ;
#38000=CARTESIAN_POINT('Ctrl Pts',(-20.0852664590449,32.2140328174815,124.432569654713)) ;
#38001=CARTESIAN_POINT('Ctrl Pts',(-20.2542774845591,32.0340437370717,124.687750970739)) ;
#38002=CARTESIAN_POINT('Ctrl Pts',(-19.6964684402798,32.2339819958047,124.602063783456)) ;
#38003=CARTESIAN_POINT('Ctrl Pts',(-19.7682819396378,32.0539929153948,124.899622390198)) ;
#38004=CARTESIAN_POINT('Ctrl Pts',(-19.2741435561821,32.2538837950442,124.628548088097)) ;
#38005=CARTESIAN_POINT('Ctrl Pts',(-19.2403770539428,32.0738947146344,124.932732853873)) ;
#38006=CARTESIAN_POINT('Ctrl Pts',(-18.8683229480946,32.2737624000966,124.51031319366)) ;
#38007=CARTESIAN_POINT('Ctrl Pts',(-18.733099358732,32.0937733196867,124.784941726055)) ;
#38008=CARTESIAN_POINT('Ctrl Pts',(-18.5246822894204,32.2937947598223,124.258593479938)) ;
#38009=CARTESIAN_POINT('Ctrl Pts',(-18.3035498467092,32.1138056794125,124.470304693614)) ;
#38010=CARTESIAN_POINT('Ctrl Pts',(-18.3288903417923,32.3103764857783,123.965395680415)) ;
#38011=CARTESIAN_POINT('Ctrl Pts',(-18.0587930610625,32.1303874053685,124.103782576925)) ;
#38012=CARTESIAN_POINT('Ctrl Pts',(-18.2389994739994,32.3235706560763,123.702969811419)) ;
#38013=CARTESIAN_POINT('Ctrl Pts',(-17.9464384609931,32.1435815756664,123.775785395654)) ;
#38014=CARTESIAN_POINT('Ctrl Pts',(-18.1952099825185,32.3368828341695,123.426608876342)) ;
#38015=CARTESIAN_POINT('Ctrl Pts',(-17.8916962163373,32.1568937537597,123.430264324838)) ;
#38016=CARTESIAN_POINT('Ctrl Pts',(-18.2318513898389,32.3534490137628,123.076189005305)) ;
#38017=CARTESIAN_POINT('Ctrl Pts',(-17.9374894752917,32.173459933353,122.992325212218)) ;
#38018=CARTESIAN_POINT('Ctrl Pts',(-18.3860665926035,32.370077208623,122.758138167499)) ;
#38019=CARTESIAN_POINT('Ctrl Pts',(-18.1302718088157,32.1900881282131,122.59470355935)) ;
#38020=CARTESIAN_POINT('Ctrl Pts',(-18.5689151454784,32.3833657903327,122.546824011485)) ;
#38021=CARTESIAN_POINT('Ctrl Pts',(-18.35881410566,32.2033767099229,122.330591540725)) ;
#38022=CARTESIAN_POINT('Ctrl Pts',(-18.7313456924468,32.3933340384363,122.414447869079)) ;
#38023=CARTESIAN_POINT('Ctrl Pts',(-18.5618539277507,32.2133449580265,122.165112713806)) ;
#38024=CARTESIAN_POINT('Ctrl Pts',(-18.9132084253142,32.4032487946925,122.312590576436)) ;
#38025=CARTESIAN_POINT('Ctrl Pts',(-18.7891790717672,32.2232597142826,122.037790375952)) ;
#38026=CARTESIAN_POINT('Ctrl Pts',(-19.1118736333332,32.4132619453437,122.242954847394)) ;
#38027=CARTESIAN_POINT('Ctrl Pts',(-19.0375135912556,32.2332728649338,121.950743279244)) ;
#38028=CARTESIAN_POINT('Ctrl Pts',(-19.3196522724763,32.4232746525457,122.209207410282)) ;
#38029=CARTESIAN_POINT('Ctrl Pts',(-19.2972230251733,32.2432855721359,121.90855387345)) ;
#38030=CARTESIAN_POINT('Ctrl Pts',(-19.5975327146755,32.436493941237,122.212420867369)) ;
#38031=CARTESIAN_POINT('Ctrl Pts',(-19.6446403660518,32.2565048608272,121.912579552322)) ;
#38032=CARTESIAN_POINT('Ctrl Pts',(-19.9378232247677,32.453112622235,122.307507172536)) ;
#38033=CARTESIAN_POINT('Ctrl Pts',(-20.0699198327453,32.2731235418252,122.031411460311)) ;
#38034=CARTESIAN_POINT('Ctrl Pts',(-20.2246076543759,32.4696775300085,122.512015826499)) ;
#38035=CARTESIAN_POINT('Ctrl Pts',(-20.4284615240683,32.2896884495986,122.287076388231)) ;
#38036=CARTESIAN_POINT('Ctrl Pts',(-20.4036500534061,32.4830760016193,122.729503286316)) ;
#38037=CARTESIAN_POINT('Ctrl Pts',(-20.6522321703865,32.3030869212095,122.558907212875)) ;
#38038=CARTESIAN_POINT('Ctrl Pts',(-20.5055910328036,32.4929172571063,122.909552354167)) ;
#38039=CARTESIAN_POINT('Ctrl Pts',(-20.779667910958,32.3129281766964,122.78397239338)) ;
#38040=CARTESIAN_POINT('Ctrl Pts',(-20.5761633681093,32.5029035726945,123.10724493237)) ;
#38041=CARTESIAN_POINT('Ctrl Pts',(-20.8678841148918,32.3229144922846,123.031085830955)) ;
#38042=CARTESIAN_POINT('Ctrl Pts',(-20.6112720105989,32.5128401802809,123.313207381497)) ;
#38043=CARTESIAN_POINT('Ctrl Pts',(-20.9117732133803,32.3328510998711,123.288538866808)) ;
#38044=CARTESIAN_POINT('Ctrl Pts',(-20.6099679457665,32.5228900476492,123.524461765722)) ;
#38045=CARTESIAN_POINT('Ctrl Pts',(-20.9101458154303,32.3429009672394,123.552606824045)) ;
#38046=CARTESIAN_POINT('Ctrl Pts',(-20.5729021146074,32.532740542324,123.728221890654)) ;
#38047=CARTESIAN_POINT('Ctrl Pts',(-20.8638163143474,32.3527514619142,123.807307622457)) ;
#38048=CARTESIAN_POINT('Ctrl Pts',(-20.5006629810764,32.5427123427185,123.924992058864)) ;
#38049=CARTESIAN_POINT('Ctrl Pts',(-20.7735199835642,32.3627232623086,124.053271401058)) ;
#38050=CARTESIAN_POINT('Ctrl Pts',(-20.3950484487511,32.5527083097443,124.106711975887)) ;
#38051=CARTESIAN_POINT('Ctrl Pts',(-20.6415042016584,32.3727192293345,124.280422776286)) ;
#38052=CARTESIAN_POINT('Ctrl Pts',(-20.2587392018978,32.5627457691255,124.267771847846)) ;
#38053=CARTESIAN_POINT('Ctrl Pts',(-20.4711197707365,32.3827566887157,124.481749462208)) ;
#38054=CARTESIAN_POINT('Ctrl Pts',(-20.0999386935785,32.5725864700262,124.400395451585)) ;
#38055=CARTESIAN_POINT('Ctrl Pts',(-20.2726207382354,32.3925973896164,124.647531272465)) ;
#38056=CARTESIAN_POINT('Ctrl Pts',(-19.9169195431235,32.5826344912936,124.505860717618)) ;
#38057=CARTESIAN_POINT('Ctrl Pts',(-20.043848162919,32.4026454108838,124.779365278016)) ;
#38058=CARTESIAN_POINT('Ctrl Pts',(-19.7202317170747,32.5925818843763,124.576913026863)) ;
#38059=CARTESIAN_POINT('Ctrl Pts',(-19.797989200882,32.4125928039664,124.868183348223)) ;
#38060=CARTESIAN_POINT('Ctrl Pts',(-19.5150675447947,32.6024920304227,124.613229581171)) ;
#38061=CARTESIAN_POINT('Ctrl Pts',(-19.5415342218472,32.4225029500128,124.913581797446)) ;
#38062=CARTESIAN_POINT('Ctrl Pts',(-19.3036192781191,32.6125509442723,124.613134139564)) ;
#38063=CARTESIAN_POINT('Ctrl Pts',(-19.2772239183681,32.4325618638625,124.913465271253)) ;
#38064=CARTESIAN_POINT('Ctrl Pts',(-19.0998162930448,32.6223917145616,124.5774017769)) ;
#38065=CARTESIAN_POINT('Ctrl Pts',(-19.0224693115229,32.4424026341518,124.868802452582)) ;
#38066=CARTESIAN_POINT('Ctrl Pts',(-18.9008906926549,32.6324545841402,124.505484176666)) ;
#38067=CARTESIAN_POINT('Ctrl Pts',(-18.7738114255995,32.4524655037304,124.778908029385)) ;
#38068=CARTESIAN_POINT('Ctrl Pts',(-18.7205888208704,32.6423489072707,124.401712674565)) ;
#38069=CARTESIAN_POINT('Ctrl Pts',(-18.5484324346337,32.4623598268608,124.649195864333)) ;
#38070=CARTESIAN_POINT('Ctrl Pts',(-18.5599523550071,32.6522907143652,124.268035857057)) ;
#38071=CARTESIAN_POINT('Ctrl Pts',(-18.3476349379479,32.4723016339554,124.482101731638)) ;
#38072=CARTESIAN_POINT('Ctrl Pts',(-18.4240467284614,32.6622932253205,124.107533030312)) ;
#38073=CARTESIAN_POINT('Ctrl Pts',(-18.177750820169,32.4823041449107,124.281474853477)) ;
#38074=CARTESIAN_POINT('Ctrl Pts',(-18.3180393506076,32.6723279461389,123.925154810979)) ;
#38075=CARTESIAN_POINT('Ctrl Pts',(-18.0452392632556,32.492338865729,124.053503454167)) ;
#38076=CARTESIAN_POINT('Ctrl Pts',(-18.2463535071879,32.6821731236446,123.730976061633)) ;
#38077=CARTESIAN_POINT('Ctrl Pts',(-17.955629269533,32.5021840432348,123.810780412373)) ;
#38078=CARTESIAN_POINT('Ctrl Pts',(-18.2085503842841,32.6921578840457,123.524527153024)) ;
#38079=CARTESIAN_POINT('Ctrl Pts',(-17.9083727783056,32.5121688036358,123.552719582541)) ;
#38080=CARTESIAN_POINT('Ctrl Pts',(-18.2070734509099,32.7020967903621,123.315553842166)) ;
#38081=CARTESIAN_POINT('Ctrl Pts',(-17.9065240318063,32.5221077099522,123.291502653979)) ;
#38082=CARTESIAN_POINT('Ctrl Pts',(-18.2423288903742,32.7121390179978,123.107420822376)) ;
#38083=CARTESIAN_POINT('Ctrl Pts',(-17.9505907656903,32.532149937588,123.031335993572)) ;
#38084=CARTESIAN_POINT('Ctrl Pts',(-18.3119535046348,32.7220242295822,122.91158798625)) ;
#38085=CARTESIAN_POINT('Ctrl Pts',(-18.0376192935989,32.5420351491723,122.786543593537)) ;
#38086=CARTESIAN_POINT('Ctrl Pts',(-18.4154411859655,32.7320231597841,122.728653020651)) ;
#38087=CARTESIAN_POINT('Ctrl Pts',(-18.1669767555534,32.5520340793743,122.557873550003)) ;
#38088=CARTESIAN_POINT('Ctrl Pts',(-18.5479494903237,32.7419405826945,122.567636304584)) ;
#38089=CARTESIAN_POINT('Ctrl Pts',(-18.3326104946067,32.5619515022847,122.356600741691)) ;
#38090=CARTESIAN_POINT('Ctrl Pts',(-18.7084645463627,32.7519885147733,122.430363552934)) ;
#38091=CARTESIAN_POINT('Ctrl Pts',(-18.5332526173414,32.5719994343634,122.18500796692)) ;
#38092=CARTESIAN_POINT('Ctrl Pts',(-18.8872415852668,32.7618658905827,122.324659315536)) ;
#38093=CARTESIAN_POINT('Ctrl Pts',(-18.7567232186998,32.5818768101728,122.052875232576)) ;
#38094=CARTESIAN_POINT('Ctrl Pts',(-19.0850258483024,32.7719197837506,122.25022120339)) ;
#38095=CARTESIAN_POINT('Ctrl Pts',(-19.0039525695747,32.5919307033408,121.959825361335)) ;
#38096=CARTESIAN_POINT('Ctrl Pts',(-19.2894783129814,32.7818134070039,122.211767437767)) ;
#38097=CARTESIAN_POINT('Ctrl Pts',(-19.2595182815771,32.601824326594,121.91175567857)) ;
#38098=CARTESIAN_POINT('Ctrl Pts',(-19.5009779859704,32.7918760006269,122.209324968633)) ;
#38099=CARTESIAN_POINT('Ctrl Pts',(-19.5238926627114,32.611886920217,121.908700188331)) ;
#38100=CARTESIAN_POINT('Ctrl Pts',(-19.7051996408792,32.8017185746159,122.242795102334)) ;
#38101=CARTESIAN_POINT('Ctrl Pts',(-19.7791709674266,32.6217294942061,121.950535647237)) ;
#38102=CARTESIAN_POINT('Ctrl Pts',(-19.9035645751163,32.8117093314989,122.311756543246)) ;
#38103=CARTESIAN_POINT('Ctrl Pts',(-20.0271280441741,32.631720251089,122.036735366564)) ;
#38104=CARTESIAN_POINT('Ctrl Pts',(-20.0858058022882,32.8216373932568,122.41352070292)) ;
#38105=CARTESIAN_POINT('Ctrl Pts',(-20.2549311094076,32.641648312847,122.163938821272)) ;
#38106=CARTESIAN_POINT('Ctrl Pts',(-20.2488151784822,32.831625369146,122.545893277075)) ;
#38107=CARTESIAN_POINT('Ctrl Pts',(-20.4586943445839,32.6516362887362,122.329402962542)) ;
#38108=CARTESIAN_POINT('Ctrl Pts',(-20.3867446811956,32.8416610335024,122.705536508051)) ;
#38109=CARTESIAN_POINT('Ctrl Pts',(-20.6311078852377,32.6616719530926,122.528955452301)) ;
#38110=CARTESIAN_POINT('Ctrl Pts',(-20.4932113035389,32.8515169719221,122.883306696087)) ;
#38111=CARTESIAN_POINT('Ctrl Pts',(-20.7641935054107,32.6715278915122,122.751167847441)) ;
#38112=CARTESIAN_POINT('Ctrl Pts',(-20.5685516723176,32.861512463319,123.079449372689)) ;
#38113=CARTESIAN_POINT('Ctrl Pts',(-20.8583709771004,32.6815233829091,122.996345583819)) ;
#38114=CARTESIAN_POINT('Ctrl Pts',(-20.6084146945894,32.8714222682724,123.283945522481)) ;
#38115=CARTESIAN_POINT('Ctrl Pts',(-20.9082019159702,32.6914331878626,123.251966021341)) ;
#38116=CARTESIAN_POINT('Ctrl Pts',(-20.6125455527865,32.8814344905392,123.494398317047)) ;
#38117=CARTESIAN_POINT('Ctrl Pts',(-20.9133674663854,32.7014454101294,123.515032024861)) ;
#38118=CARTESIAN_POINT('Ctrl Pts',(-20.5796147863066,32.891462371232,123.702629937833)) ;
#38119=CARTESIAN_POINT('Ctrl Pts',(-20.8722060910086,32.7114732908222,123.775321815861)) ;
#38120=CARTESIAN_POINT('Ctrl Pts',(-20.512536676068,32.9013187672146,123.898683038546)) ;
#38121=CARTESIAN_POINT('Ctrl Pts',(-20.7883600168508,32.7213296868048,124.020389778682)) ;
#38122=CARTESIAN_POINT('Ctrl Pts',(-20.4111096637263,32.9113435643946,124.083427639594)) ;
#38123=CARTESIAN_POINT('Ctrl Pts',(-20.6615779008466,32.7313544839848,124.251321404654)) ;
#38124=CARTESIAN_POINT('Ctrl Pts',(-20.2786586384408,32.9213744943784,124.247533456191)) ;
#38125=CARTESIAN_POINT('Ctrl Pts',(-20.496015737572,32.7413854139686,124.456454889793)) ;
#38126=CARTESIAN_POINT('Ctrl Pts',(-20.1229354505894,32.931219096887,124.38384374608)) ;
#38127=CARTESIAN_POINT('Ctrl Pts',(-20.3013621684874,32.7512300164772,124.626844922509)) ;
#38128=CARTESIAN_POINT('Ctrl Pts',(-19.9435638207466,32.9412099481111,124.493133513568)) ;
#38129=CARTESIAN_POINT('Ctrl Pts',(-20.0771483651053,32.7612208677013,124.763458712238)) ;
#38130=CARTESIAN_POINT('Ctrl Pts',(-19.7468547735515,32.9512477811224,124.569535084003)) ;
#38131=CARTESIAN_POINT('Ctrl Pts',(-19.8312628601303,32.7712587007126,124.858962378783)) ;
#38132=CARTESIAN_POINT('Ctrl Pts',(-19.5439187927745,32.9610921695878,124.610185963789)) ;
#38133=CARTESIAN_POINT('Ctrl Pts',(-19.5775920832563,32.781103089178,124.90977793786)) ;
#38134=CARTESIAN_POINT('Ctrl Pts',(-19.3341011134292,32.9710769739574,124.615465585142)) ;
#38135=CARTESIAN_POINT('Ctrl Pts',(-19.3153197757282,32.7910878935475,124.916379101502)) ;
#38136=CARTESIAN_POINT('Ctrl Pts',(-19.1274257911367,32.9810164934402,124.584456615172)) ;
#38137=CARTESIAN_POINT('Ctrl Pts',(-19.0569748481589,32.8010274130304,124.87761938897)) ;
#38138=CARTESIAN_POINT('Ctrl Pts',(-18.927334989013,32.9910562244416,124.517330597724)) ;
#38139=CARTESIAN_POINT('Ctrl Pts',(-18.8068609697221,32.8110671440317,124.793713447286)) ;
#38140=CARTESIAN_POINT('Ctrl Pts',(-18.7446634407344,33.0009443526879,124.418083254216)) ;
#38141=CARTESIAN_POINT('Ctrl Pts',(-18.5785199696403,32.820955272278,124.669655218492)) ;
#38142=CARTESIAN_POINT('Ctrl Pts',(-18.5801005857967,33.0109340778964,124.28761411625)) ;
#38143=CARTESIAN_POINT('Ctrl Pts',(-18.3728153330227,32.8309449974866,124.506569798972)) ;
#38144=CARTESIAN_POINT('Ctrl Pts',(-18.4412469443852,33.0208918425979,124.130951753119)) ;
#38145=CARTESIAN_POINT('Ctrl Pts',(-18.1992468677695,32.8409027621881,124.3107425181)) ;
#38146=CARTESIAN_POINT('Ctrl Pts',(-18.3318926647563,33.0307941840099,123.9538000731)) ;
#38147=CARTESIAN_POINT('Ctrl Pts',(-18.0625524287455,32.8508051036001,124.089302873822)) ;
#38148=CARTESIAN_POINT('Ctrl Pts',(-18.2538818671851,33.0408383797163,123.757588934328)) ;
#38149=CARTESIAN_POINT('Ctrl Pts',(-17.9650377613025,32.8608492993064,123.844039624729)) ;
#38150=CARTESIAN_POINT('Ctrl Pts',(-18.2116804220347,33.0507457804755,123.553613209322)) ;
#38151=CARTESIAN_POINT('Ctrl Pts',(-17.9122844842021,32.8707567000657,123.589069438269)) ;
#38152=CARTESIAN_POINT('Ctrl Pts',(-18.2051029806548,33.0607563803499,123.343258587515)) ;
#38153=CARTESIAN_POINT('Ctrl Pts',(-17.9040614840554,32.8807672999401,123.326126151245)) ;
#38154=CARTESIAN_POINT('Ctrl Pts',(-18.2356129749223,33.0707866762621,123.134602723717)) ;
#38155=CARTESIAN_POINT('Ctrl Pts',(-17.942197627279,32.8907975958523,123.0653062275)) ;
#38156=CARTESIAN_POINT('Ctrl Pts',(-18.300450441629,33.0806414559118,122.937844780199)) ;
#38157=CARTESIAN_POINT('Ctrl Pts',(-18.0232436734784,32.900652375502,122.819357208216)) ;
#38158=CARTESIAN_POINT('Ctrl Pts',(-18.3989330999902,33.0905987841293,122.753115564655)) ;
#38159=CARTESIAN_POINT('Ctrl Pts',(-18.146346329286,32.9106097037195,122.588444800314)) ;
#38160=CARTESIAN_POINT('Ctrl Pts',(-18.5293347628917,33.1006378170362,122.587186806717)) ;
#38161=CARTESIAN_POINT('Ctrl Pts',(-18.3093474041902,32.9206487366264,122.381033273933)) ;
#38162=CARTESIAN_POINT('Ctrl Pts',(-18.6837449458525,33.1105109289255,122.44842798728)) ;
#38163=CARTESIAN_POINT('Ctrl Pts',(-18.5023603004439,32.9305218485156,122.207583253735)) ;
#38164=CARTESIAN_POINT('Ctrl Pts',(-18.8634428506156,33.1205842139526,122.336455552253)) ;
#38165=CARTESIAN_POINT('Ctrl Pts',(-18.7269817759112,32.9405951335427,122.067617063603)) ;
#38166=CARTESIAN_POINT('Ctrl Pts',(-19.0549009830223,33.1304045336893,122.259087158195)) ;
#38167=CARTESIAN_POINT('Ctrl Pts',(-18.9663055363754,32.9504154532795,121.970905134064)) ;
#38168=CARTESIAN_POINT('Ctrl Pts',(-19.2620617743464,33.1404831990678,122.214836805238)) ;
#38169=CARTESIAN_POINT('Ctrl Pts',(-19.2252558871438,32.960494118658,121.915591458539)) ;
#38170=CARTESIAN_POINT('Ctrl Pts',(-19.4690858066591,33.1503347895516,122.207323763932)) ;
#38171=CARTESIAN_POINT('Ctrl Pts',(-19.4840372151906,32.9703457091417,121.906199287726)) ;
#38172=CARTESIAN_POINT('Ctrl Pts',(-19.6788221961635,33.1604079398705,122.236318117315)) ;
#38173=CARTESIAN_POINT('Ctrl Pts',(-19.7462073717057,32.9804188594607,121.942441422223)) ;
#38174=CARTESIAN_POINT('Ctrl Pts',(-19.8757676666468,33.1702503198455,122.29984587334)) ;
#38175=CARTESIAN_POINT('Ctrl Pts',(-19.9923907934108,32.9902612394357,122.021850824129)) ;
#38176=CARTESIAN_POINT('Ctrl Pts',(-20.0615568423931,33.1802312960886,122.397340048121)) ;
#38177=CARTESIAN_POINT('Ctrl Pts',(-20.2246277641861,33.0002422156788,122.14371824194)) ;
#38178=CARTESIAN_POINT('Ctrl Pts',(-20.2279876372291,33.1902476244439,122.526364012805)) ;
#38179=CARTESIAN_POINT('Ctrl Pts',(-20.4326666594607,33.010258544034,122.304997705709)) ;
#38180=CARTESIAN_POINT('Ctrl Pts',(-20.3679958704936,33.200145421435,122.680288715959)) ;
#38181=CARTESIAN_POINT('Ctrl Pts',(-20.6076780089527,33.0201563410252,122.497403957901)) ;
#38182=CARTESIAN_POINT('Ctrl Pts',(-20.4807568430483,33.2101579781671,122.858052147058)) ;
#38183=CARTESIAN_POINT('Ctrl Pts',(-20.748629570093,33.0301688977572,122.719608055102)) ;
#38184=CARTESIAN_POINT('Ctrl Pts',(-20.5606237614743,33.2201900130135,123.053239269694)) ;
#38185=CARTESIAN_POINT('Ctrl Pts',(-20.8484637131668,33.0402009326037,122.963591613867)) ;
#38186=CARTESIAN_POINT('Ctrl Pts',(-20.6050359521563,33.230029413829,123.255287016282)) ;
#38187=CARTESIAN_POINT('Ctrl Pts',(-20.9039796444684,33.0500403334192,123.216152649284)) ;
#38188=CARTESIAN_POINT('Ctrl Pts',(-20.614049092095,33.2400951994806,123.466685199039)) ;
#38189=CARTESIAN_POINT('Ctrl Pts',(-20.915246377554,33.0601061190708,123.480399984262)) ;
#38190=CARTESIAN_POINT('Ctrl Pts',(-20.5866016199623,33.2499856545952,123.672815882505)) ;
#38191=CARTESIAN_POINT('Ctrl Pts',(-20.8809372576275,33.0699965741854,123.738064421182)) ;
#38192=CARTESIAN_POINT('Ctrl Pts',(-20.5235744358789,33.2599777732309,123.873192435292)) ;
#38193=CARTESIAN_POINT('Ctrl Pts',(-20.8021533890581,33.0799886928211,123.98853537264)) ;
#38194=CARTESIAN_POINT('Ctrl Pts',(-20.4268201921986,33.269940599994,124.058949341531)) ;
#38195=CARTESIAN_POINT('Ctrl Pts',(-20.6812106073912,33.0899515195842,124.22073203139)) ;
#38196=CARTESIAN_POINT('Ctrl Pts',(-20.3004366840512,33.2798448832669,124.224447351388)) ;
#38197=CARTESIAN_POINT('Ctrl Pts',(-20.5232306933869,33.0998558028571,124.427605321888)) ;
#38198=CARTESIAN_POINT('Ctrl Pts',(-20.1447295418141,33.289905317214,124.36754765931)) ;
#38199=CARTESIAN_POINT('Ctrl Pts',(-20.3285971107934,33.1099162368042,124.60648055999)) ;
#38200=CARTESIAN_POINT('Ctrl Pts',(-19.9705348461401,33.2997458698872,124.479200573106)) ;
#38201=CARTESIAN_POINT('Ctrl Pts',(-20.1108525131873,33.1197567894774,124.746047511575)) ;
#38202=CARTESIAN_POINT('Ctrl Pts',(-19.7754486620415,33.3098080898329,124.560937015525)) ;
#38203=CARTESIAN_POINT('Ctrl Pts',(-19.8669950901553,33.129819009423,124.848217841125)) ;
#38204=CARTESIAN_POINT('Ctrl Pts',(-19.57243885132,33.3197052291114,124.606588971433)) ;
#38205=CARTESIAN_POINT('Ctrl Pts',(-19.613231849326,33.1397161487016,124.905283007281)) ;
#38206=CARTESIAN_POINT('Ctrl Pts',(-19.3639189425878,33.3296364212465,124.61702574814)) ;
#38207=CARTESIAN_POINT('Ctrl Pts',(-19.3525812289546,33.1496473408367,124.918328736753)) ;
#38208=CARTESIAN_POINT('Ctrl Pts',(-19.1544701914488,33.3396785758916,124.5905747195)) ;
#38209=CARTESIAN_POINT('Ctrl Pts',(-19.0907705220103,33.1596894954817,124.885264797478)) ;
#38210=CARTESIAN_POINT('Ctrl Pts',(-18.9558448503062,33.3495653369109,124.529280922673)) ;
#38211=CARTESIAN_POINT('Ctrl Pts',(-18.8424878708844,33.169576256501,124.808646986512)) ;
#38212=CARTESIAN_POINT('Ctrl Pts',(-18.7686911463768,33.3595646386281,124.433610207421)) ;
#38213=CARTESIAN_POINT('Ctrl Pts',(-18.6085457634683,33.1795755582183,124.689058201109)) ;
#38214=CARTESIAN_POINT('Ctrl Pts',(-18.6021783660485,33.3694854367949,124.307970432937)) ;
#38215=CARTESIAN_POINT('Ctrl Pts',(-18.4004044123942,33.189496356385,124.532007686326)) ;
#38216=CARTESIAN_POINT('Ctrl Pts',(-18.4584063019832,33.3795194903916,124.153637802788)) ;
#38217=CARTESIAN_POINT('Ctrl Pts',(-18.2206897369565,33.1995304099818,124.339091715011)) ;
#38218=CARTESIAN_POINT('Ctrl Pts',(-18.3447487639094,33.389442607958,123.978664957015)) ;
#38219=CARTESIAN_POINT('Ctrl Pts',(-18.0786177880048,33.2094535275481,124.120374761403)) ;
#38220=CARTESIAN_POINT('Ctrl Pts',(-18.262168874499,33.3994987314571,123.784072019688)) ;
#38221=CARTESIAN_POINT('Ctrl Pts',(-17.9753934549704,33.2195096510473,123.877133689794)) ;
#38222=CARTESIAN_POINT('Ctrl Pts',(-18.2155327305873,33.4093441731119,123.582403847225)) ;
#38223=CARTESIAN_POINT('Ctrl Pts',(-17.9170984303187,33.2293550927021,123.625046988964)) ;
#38224=CARTESIAN_POINT('Ctrl Pts',(-18.203805100798,33.4193064742361,123.373306871914)) ;
#38225=CARTESIAN_POINT('Ctrl Pts',(-17.9024396208833,33.2393173938262,123.36367527573)) ;
#38226=CARTESIAN_POINT('Ctrl Pts',(-18.2290055597389,33.4293349535112,123.163973793253)) ;
#38227=CARTESIAN_POINT('Ctrl Pts',(-17.9339408231796,33.2493458731014,123.102009100118)) ;
#38228=CARTESIAN_POINT('Ctrl Pts',(-18.289374518782,33.4392453070209,122.96457571185)) ;
#38229=CARTESIAN_POINT('Ctrl Pts',(-18.0094029196339,33.2592562266111,122.852760854064)) ;
#38230=CARTESIAN_POINT('Ctrl Pts',(-18.3832010117499,33.4491801791981,122.777967476055)) ;
#38231=CARTESIAN_POINT('Ctrl Pts',(-18.1266871223005,33.2691910987883,122.619500365628)) ;
#38232=CARTESIAN_POINT('Ctrl Pts',(-18.5094881208649,33.4592213167838,122.60882144455)) ;
#38233=CARTESIAN_POINT('Ctrl Pts',(-18.2845465433312,33.2792322363739,122.408068459488)) ;
#38234=CARTESIAN_POINT('Ctrl Pts',(-18.6607816210844,33.4691084659983,122.466272054033)) ;
#38235=CARTESIAN_POINT('Ctrl Pts',(-18.4736647675595,33.2891193855885,122.229881635871)) ;
#38236=CARTESIAN_POINT('Ctrl Pts',(-18.8361603645087,33.4791007007494,122.350665197575)) ;
#38237=CARTESIAN_POINT('Ctrl Pts',(-18.6928889148364,33.2991116203396,122.085373784638)) ;
#38238=CARTESIAN_POINT('Ctrl Pts',(-19.0281558133508,33.4890494063124,122.267675696057)) ;
#38239=CARTESIAN_POINT('Ctrl Pts',(-18.9328841091026,33.3090603259026,121.981637584329)) ;
#38240=CARTESIAN_POINT('Ctrl Pts',(-19.2312903333038,33.4989854747361,122.219054749115)) ;
#38241=CARTESIAN_POINT('Ctrl Pts',(-19.1868031331722,33.3189963943262,121.920862306475)) ;
#38242=CARTESIAN_POINT('Ctrl Pts',(-19.4408438884127,33.5089711589519,122.206138288306)) ;
#38243=CARTESIAN_POINT('Ctrl Pts',(-19.4487454010875,33.328982078542,121.904717887732)) ;
#38244=CARTESIAN_POINT('Ctrl Pts',(-19.6505310611523,33.5190115855205,122.230262302281)) ;
#38245=CARTESIAN_POINT('Ctrl Pts',(-19.7108540776714,33.3390225051107,121.934873930114)) ;
#38246=CARTESIAN_POINT('Ctrl Pts',(-19.8489000133317,33.5288506989843,122.288894555747)) ;
#38247=CARTESIAN_POINT('Ctrl Pts',(-19.958816242514,33.3488616185744,122.008165761132)) ;
#38248=CARTESIAN_POINT('Ctrl Pts',(-20.0378734404374,33.5388804331601,122.382439401842)) ;
#38249=CARTESIAN_POINT('Ctrl Pts',(-20.1950323308035,33.3588913527503,122.125097981802)) ;
#38250=CARTESIAN_POINT('Ctrl Pts',(-20.2072755150805,33.548902532666,122.50771918548)) ;
#38251=CARTESIAN_POINT('Ctrl Pts',(-20.4067842186,33.3689134522561,122.281698617099)) ;
#38252=CARTESIAN_POINT('Ctrl Pts',(-20.3505163323491,33.5587709725594,122.657820476515)) ;
#38253=CARTESIAN_POINT('Ctrl Pts',(-20.5858350553215,33.3787818921496,122.469326974314)) ;
#38254=CARTESIAN_POINT('Ctrl Pts',(-20.467830910548,33.568839837245,122.833994863383)) ;
#38255=CARTESIAN_POINT('Ctrl Pts',(-20.732476955255,33.3888507568352,122.689545385332)) ;
#38256=CARTESIAN_POINT('Ctrl Pts',(-20.5508822742983,33.5786825103436,123.023527927505)) ;
#38257=CARTESIAN_POINT('Ctrl Pts',(-20.8362904560679,33.3986934299338,122.926463443112)) ;
#38258=CARTESIAN_POINT('Ctrl Pts',(-20.6010906324588,33.5886431445061,123.226819066084)) ;
#38259=CARTESIAN_POINT('Ctrl Pts',(-20.8990494416422,33.4086540640963,123.180578146972)) ;
#38260=CARTESIAN_POINT('Ctrl Pts',(-20.6149332523502,33.5986810601842,123.437385843915)) ;
#38261=CARTESIAN_POINT('Ctrl Pts',(-20.9163512491307,33.4186919797744,123.443786581485)) ;
#38262=CARTESIAN_POINT('Ctrl Pts',(-20.5927561143563,33.6085553350436,123.64381161214)) ;
#38263=CARTESIAN_POINT('Ctrl Pts',(-20.8886281344134,33.4285662546338,123.701819630234)) ;
#38264=CARTESIAN_POINT('Ctrl Pts',(-20.5339350999099,33.6186250854188,123.847144174352)) ;
#38265=CARTESIAN_POINT('Ctrl Pts',(-20.8151004365059,33.438636005009,123.955984554738)) ;
#38266=CARTESIAN_POINT('Ctrl Pts',(-20.4429721196494,33.6284583807933,124.032801166583)) ;
#38267=CARTESIAN_POINT('Ctrl Pts',(-20.7013946873049,33.4484693003834,124.188056231811)) ;
#38268=CARTESIAN_POINT('Ctrl Pts',(-20.3192120120837,33.6384886782729,124.203524561785)) ;
#38269=CARTESIAN_POINT('Ctrl Pts',(-20.546693129782,33.4584995978631,124.401459336324)) ;
#38270=CARTESIAN_POINT('Ctrl Pts',(-20.1672189301495,33.6485207647143,124.34975537749)) ;
#38271=CARTESIAN_POINT('Ctrl Pts',(-20.3567007162812,33.4685316843045,124.584246630781)) ;
#38272=CARTESIAN_POINT('Ctrl Pts',(-19.9959765672418,33.6583486932033,124.465347265226)) ;
#38273=CARTESIAN_POINT('Ctrl Pts',(-20.1426457143596,33.4783596127934,124.728735741581)) ;
#38274=CARTESIAN_POINT('Ctrl Pts',(-19.8042599262361,33.668344734314,124.551406477392)) ;
#38275=CARTESIAN_POINT('Ctrl Pts',(-19.9029989792724,33.4883556539042,124.836308043076)) ;
#38276=CARTESIAN_POINT('Ctrl Pts',(-19.5997986838968,33.6783705464153,124.602630095532)) ;
#38277=CARTESIAN_POINT('Ctrl Pts',(-19.6474220237425,33.4983814660054,124.900335793368)) ;
#38278=CARTESIAN_POINT('Ctrl Pts',(-19.3924774849365,33.6882577813101,124.617636375072)) ;
#38279=CARTESIAN_POINT('Ctrl Pts',(-19.3882695560043,33.5082687009003,124.919091810122)) ;
#38280=CARTESIAN_POINT('Ctrl Pts',(-19.1838086719246,33.6982346475211,124.59657238943)) ;
#38281=CARTESIAN_POINT('Ctrl Pts',(-19.1274334857546,33.5182455671113,124.892759807701)) ;
#38282=CARTESIAN_POINT('Ctrl Pts',(-18.9815887866603,33.7082275913929,124.539527650244)) ;
#38283=CARTESIAN_POINT('Ctrl Pts',(-18.8746590268062,33.5282385109831,124.82145190794)) ;
#38284=CARTESIAN_POINT('Ctrl Pts',(-18.7916507877663,33.7182655140643,124.447604623788)) ;
#38285=CARTESIAN_POINT('Ctrl Pts',(-18.6372374521319,33.5382764336545,124.706546424566)) ;
#38286=CARTESIAN_POINT('Ctrl Pts',(-18.6235800416685,33.728113978326,124.326664479328)) ;
#38287=CARTESIAN_POINT('Ctrl Pts',(-18.4271493677477,33.5481248979162,124.555368999673)) ;
#38288=CARTESIAN_POINT('Ctrl Pts',(-18.4767212967357,33.73810584507,124.17651438228)) ;
#38289=CARTESIAN_POINT('Ctrl Pts',(-18.2435773438857,33.5581167646602,124.367679767464)) ;
#38290=CARTESIAN_POINT('Ctrl Pts',(-18.3589139649517,33.7480235771112,124.004451145981)) ;
#38291=CARTESIAN_POINT('Ctrl Pts',(-18.0963196368505,33.5680344967013,124.152599028202)) ;
#38292=CARTESIAN_POINT('Ctrl Pts',(-18.2717798858509,33.7580517620064,123.812495005014)) ;
#38293=CARTESIAN_POINT('Ctrl Pts',(-17.9874040347647,33.5780626815966,123.91265298461)) ;
#38294=CARTESIAN_POINT('Ctrl Pts',(-18.2199583948153,33.7679369200553,123.611237430731)) ;
#38295=CARTESIAN_POINT('Ctrl Pts',(-17.9226291155183,33.5879478396455,123.661079753406)) ;
#38296=CARTESIAN_POINT('Ctrl Pts',(-18.2031899992664,33.777926280597,123.401895935145)) ;
#38297=CARTESIAN_POINT('Ctrl Pts',(-17.9016709287032,33.5979372001872,123.399402541443)) ;
#38298=CARTESIAN_POINT('Ctrl Pts',(-18.2235716353926,33.7879674375313,123.191785549963)) ;
#38299=CARTESIAN_POINT('Ctrl Pts',(-17.9271501703905,33.6079783571215,123.136764865885)) ;
#38300=CARTESIAN_POINT('Ctrl Pts',(-18.2786200114163,33.7978000209865,122.992541931651)) ;
#38301=CARTESIAN_POINT('Ctrl Pts',(-17.9959631146124,33.6178109405767,122.887710030795)) ;
#38302=CARTESIAN_POINT('Ctrl Pts',(-18.3683487595105,33.8077942409485,122.802558224902)) ;
#38303=CARTESIAN_POINT('Ctrl Pts',(-18.1081263092471,33.6278051605386,122.650231330514)) ;
#38304=CARTESIAN_POINT('Ctrl Pts',(-18.4904696258343,33.8178223427358,122.63070110739)) ;
#38305=CARTESIAN_POINT('Ctrl Pts',(-18.2607792874673,33.6378332623259,122.435411305437)) ;
#38306=CARTESIAN_POINT('Ctrl Pts',(-18.6381482308556,33.8277022873588,122.484636845884)) ;
#38307=CARTESIAN_POINT('Ctrl Pts',(-18.4453797141008,33.647713206949,122.252832221306)) ;
#38308=CARTESIAN_POINT('Ctrl Pts',(-18.8106558657306,33.8376926139159,122.364855145629)) ;
#38309=CARTESIAN_POINT('Ctrl Pts',(-18.6610157890735,33.6577035335061,122.103107051282)) ;
#38310=CARTESIAN_POINT('Ctrl Pts',(-19.0004133748142,33.8476335455702,122.277272733612)) ;
#38311=CARTESIAN_POINT('Ctrl Pts',(-18.8982140304838,33.6676444651604,121.993631136428)) ;
#38312=CARTESIAN_POINT('Ctrl Pts',(-19.2033679275045,33.8576206640731,122.223428561579)) ;
#38313=CARTESIAN_POINT('Ctrl Pts',(-19.1519080089665,33.6776315836633,121.926328336062)) ;
#38314=CARTESIAN_POINT('Ctrl Pts',(-19.413555239702,33.8676539969703,122.205893497392)) ;
#38315=CARTESIAN_POINT('Ctrl Pts',(-19.4146423301782,33.6876649165604,121.90441196927)) ;
#38316=CARTESIAN_POINT('Ctrl Pts',(-19.6201683892138,33.877520101415,122.224398460952)) ;
#38317=CARTESIAN_POINT('Ctrl Pts',(-19.6729091690193,33.6975310210052,121.927545767078)) ;
#38318=CARTESIAN_POINT('Ctrl Pts',(-19.824456202544,33.8875862152953,122.279533485596)) ;
#38319=CARTESIAN_POINT('Ctrl Pts',(-19.928268124028,33.7075971348855,121.996466980222)) ;
#38320=CARTESIAN_POINT('Ctrl Pts',(-20.0121077833752,33.8974422270637,122.367434002635)) ;
#38321=CARTESIAN_POINT('Ctrl Pts',(-20.1628320829967,33.7174531466539,122.106345209842)) ;
#38322=CARTESIAN_POINT('Ctrl Pts',(-20.1843716366312,33.9074369306951,122.487738822849)) ;
#38323=CARTESIAN_POINT('Ctrl Pts',(-20.3781604556109,33.7274478502852,122.256728476935)) ;
#38324=CARTESIAN_POINT('Ctrl Pts',(-20.3333627134761,33.9174682664199,122.63699684848)) ;
#38325=CARTESIAN_POINT('Ctrl Pts',(-20.5643974693721,33.7374791860101,122.443302838749)) ;
#38326=CARTESIAN_POINT('Ctrl Pts',(-20.4524620397036,33.9273347916236,122.806830884017)) ;
#38327=CARTESIAN_POINT('Ctrl Pts',(-20.71326976199,33.7473457112138,122.655597325684)) ;
#38328=CARTESIAN_POINT('Ctrl Pts',(-20.5416324218957,33.9373222196694,122.996895065908)) ;
#38329=CARTESIAN_POINT('Ctrl Pts',(-20.8247303533293,33.7573331392596,122.8931788086)) ;
#38330=CARTESIAN_POINT('Ctrl Pts',(-20.5963371639424,33.9472671493558,123.198716985131)) ;
#38331=CARTESIAN_POINT('Ctrl Pts',(-20.893108733767,33.767278068946,123.145457142125)) ;
#38332=CARTESIAN_POINT('Ctrl Pts',(-20.615233404167,33.9573120674643,123.409025558996)) ;
#38333=CARTESIAN_POINT('Ctrl Pts',(-20.9167263519212,33.7773229870545,123.408343079754)) ;
#38334=CARTESIAN_POINT('Ctrl Pts',(-20.5978343581406,33.9671740370782,123.615640699636)) ;
#38335=CARTESIAN_POINT('Ctrl Pts',(-20.8949748057221,33.7871849566684,123.666612207496)) ;
#38336=CARTESIAN_POINT('Ctrl Pts',(-20.5445304522243,33.9771661050995,123.818808413641)) ;
#38337=CARTESIAN_POINT('Ctrl Pts',(-20.8283422293849,33.7971770246896,123.920571241205)) ;
#38338=CARTESIAN_POINT('Ctrl Pts',(-20.4572488945019,33.987097030474,124.008482314326)) ;
#38339=CARTESIAN_POINT('Ctrl Pts',(-20.7192376865888,33.8071079500642,124.157662672226)) ;
#38340=CARTESIAN_POINT('Ctrl Pts',(-20.3384279441806,33.9970476586975,124.180637038288)) ;
#38341=CARTESIAN_POINT('Ctrl Pts',(-20.5707091130327,33.8170585782876,124.372854625931)) ;
#38342=CARTESIAN_POINT('Ctrl Pts',(-20.1908473350017,34.0070478977566,124.330400148074)) ;
#38343=CARTESIAN_POINT('Ctrl Pts',(-20.3862313186924,33.8270588173468,124.560056609372)) ;
#38344=CARTESIAN_POINT('Ctrl Pts',(-20.0188703479351,34.0170763531258,124.452341161375)) ;
#38345=CARTESIAN_POINT('Ctrl Pts',(-20.1712584195918,33.837087272716,124.712480635238)) ;
#38346=CARTESIAN_POINT('Ctrl Pts',(-19.8315368351169,34.026942387709,124.541398156012)) ;
#38347=CARTESIAN_POINT('Ctrl Pts',(-19.9370901885527,33.8469533072992,124.823799494595)) ;
#38348=CARTESIAN_POINT('Ctrl Pts',(-19.6291473919891,34.0369347094565,124.597606613349)) ;
#38349=CARTESIAN_POINT('Ctrl Pts',(-19.6841021964564,33.8569456290466,124.894057285031)) ;
#38350=CARTESIAN_POINT('Ctrl Pts',(-19.4212948778569,34.0468669991335,124.617735601843)) ;
#38351=CARTESIAN_POINT('Ctrl Pts',(-19.4242874903847,33.8668779187237,124.919216071778)) ;
#38352=CARTESIAN_POINT('Ctrl Pts',(-19.2116608547725,34.0568686441042,124.601562538898)) ;
#38353=CARTESIAN_POINT('Ctrl Pts',(-19.1622401128743,33.8768795636944,124.89899567107)) ;
#38354=CARTESIAN_POINT('Ctrl Pts',(-18.9405917318877,34.0701812775203,124.531785628182)) ;
#38355=CARTESIAN_POINT('Ctrl Pts',(-18.8234293921044,33.8901921971104,124.811777112325)) ;
#38356=CARTESIAN_POINT('Ctrl Pts',(-18.6953484784507,34.0834130269018,124.393891815293)) ;
#38357=CARTESIAN_POINT('Ctrl Pts',(-18.5168908225007,33.903423946492,124.639429121333)) ;
#38358=CARTESIAN_POINT('Ctrl Pts',(-18.4950002821873,34.0967362917189,124.198208396693)) ;
#38359=CARTESIAN_POINT('Ctrl Pts',(-18.2664169529744,33.9167472113091,124.394788919325)) ;
#38360=CARTESIAN_POINT('Ctrl Pts',(-18.3736497757206,34.1066119979366,124.029725845387)) ;
#38361=CARTESIAN_POINT('Ctrl Pts',(-18.1147393756413,33.9266229175268,124.184190734475)) ;
#38362=CARTESIAN_POINT('Ctrl Pts',(-18.2821299159748,34.1166015890366,123.840730802708)) ;
#38363=CARTESIAN_POINT('Ctrl Pts',(-18.0003398463221,33.9366125086268,123.947943873765)) ;
#38364=CARTESIAN_POINT('Ctrl Pts',(-18.2250270269363,34.126528685492,123.639969576889)) ;
#38365=CARTESIAN_POINT('Ctrl Pts',(-17.9289645287867,33.9465396050822,123.696992065045)) ;
#38366=CARTESIAN_POINT('Ctrl Pts',(-18.2034190105843,34.1365538339966,123.430338906527)) ;
#38367=CARTESIAN_POINT('Ctrl Pts',(-17.9019571310987,33.9565647535868,123.434953214905)) ;
#38368=CARTESIAN_POINT('Ctrl Pts',(-18.2182165399645,34.1464494881433,123.22280972338)) ;
#38369=CARTESIAN_POINT('Ctrl Pts',(-17.9204568678603,33.9664604077335,123.17554205704)) ;
#38370=CARTESIAN_POINT('Ctrl Pts',(-18.2690763393294,34.1564530225215,123.018767205604)) ;
#38371=CARTESIAN_POINT('Ctrl Pts',(-17.9840343131373,33.9764639421116,122.920489516551)) ;
#38372=CARTESIAN_POINT('Ctrl Pts',(-18.3544753384947,34.1664381609615,122.826969229147)) ;
#38373=CARTESIAN_POINT('Ctrl Pts',(-18.090785614711,33.9864490805517,122.680743142439)) ;
#38374=CARTESIAN_POINT('Ctrl Pts',(-18.472628068217,34.1764740855569,122.652181840679)) ;
#38375=CARTESIAN_POINT('Ctrl Pts',(-18.2384789184534,33.9964850051471,122.462260358668)) ;
#38376=CARTESIAN_POINT('Ctrl Pts',(-18.6164655673293,34.1863253609846,122.503176356432)) ;
#38377=CARTESIAN_POINT('Ctrl Pts',(-18.4182776202501,34.0063362805748,122.276005602342)) ;
#38378=CARTESIAN_POINT('Ctrl Pts',(-18.7860413391488,34.1963176221459,122.379176678945)) ;
#38379=CARTESIAN_POINT('Ctrl Pts',(-18.6302489537786,34.0163285417361,122.121008186934)) ;
#38380=CARTESIAN_POINT('Ctrl Pts',(-18.9756890039157,34.2063575061635,122.28655058311)) ;
#38381=CARTESIAN_POINT('Ctrl Pts',(-18.8673098715095,34.0263684257537,122.005227980677)) ;
#38382=CARTESIAN_POINT('Ctrl Pts',(-19.1742841833314,34.216192280666,122.228937175601)) ;
#38383=CARTESIAN_POINT('Ctrl Pts',(-19.115554348172,34.0362032002561,121.933213929696)) ;
#38384=CARTESIAN_POINT('Ctrl Pts',(-19.3848491923498,34.2262686616863,122.206064095347)) ;
#38385=CARTESIAN_POINT('Ctrl Pts',(-19.378760644143,34.0462795812764,121.904625237275)) ;
#38386=CARTESIAN_POINT('Ctrl Pts',(-19.5914235484233,34.2361149348369,122.219725589952)) ;
#38387=CARTESIAN_POINT('Ctrl Pts',(-19.6369799649449,34.0561258544271,121.921704730761)) ;
#38388=CARTESIAN_POINT('Ctrl Pts',(-19.8644290889112,34.2494794561221,122.286150104752)) ;
#38389=CARTESIAN_POINT('Ctrl Pts',(-19.9782262367298,34.0694903757123,122.004738916852)) ;
#38390=CARTESIAN_POINT('Ctrl Pts',(-20.1107333011822,34.2626857005566,122.421054667692)) ;
#38391=CARTESIAN_POINT('Ctrl Pts',(-20.2860725516043,34.0826966201467,122.173341752831)) ;
#38392=CARTESIAN_POINT('Ctrl Pts',(-20.3128900283233,34.2759506552338,122.613069418679)) ;
#38393=CARTESIAN_POINT('Ctrl Pts',(-20.5388137927401,34.095961574824,122.41339891427)) ;
#38394=CARTESIAN_POINT('Ctrl Pts',(-20.438205183774,34.2859829357855,122.782731790521)) ;
#38395=CARTESIAN_POINT('Ctrl Pts',(-20.6954462285067,34.1059938553757,122.625471146466)) ;
#38396=CARTESIAN_POINT('Ctrl Pts',(-20.5310032145783,34.2958916693034,122.96922602419)) ;
#38397=CARTESIAN_POINT('Ctrl Pts',(-20.811443835106,34.1159025888936,122.858591933843)) ;
#38398=CARTESIAN_POINT('Ctrl Pts',(-20.5907085275571,34.3058292201709,123.169440553708)) ;
#38399=CARTESIAN_POINT('Ctrl Pts',(-20.8860726330652,34.1258401397611,123.108858926541)) ;
#38400=CARTESIAN_POINT('Ctrl Pts',(-20.6147885837747,34.3158590677648,123.378897155107)) ;
#38401=CARTESIAN_POINT('Ctrl Pts',(-20.9161696355362,34.135869987355,123.370684085344)) ;
#38402=CARTESIAN_POINT('Ctrl Pts',(-20.5984660377212,34.3290942076852,123.656745178139)) ;
#38403=CARTESIAN_POINT('Ctrl Pts',(-20.8957675551439,34.1491051272754,123.717974610687)) ;
#38404=CARTESIAN_POINT('Ctrl Pts',(-20.4868736795983,34.3457626720564,123.993002939098)) ;
#38405=CARTESIAN_POINT('Ctrl Pts',(-20.7562726268959,34.1657735916466,124.138314956039)) ;
#38406=CARTESIAN_POINT('Ctrl Pts',(-20.2251415994005,34.3656336839303,124.324854114814)) ;
#38407=CARTESIAN_POINT('Ctrl Pts',(-20.429086179161,34.1856446035205,124.553127465657)) ;
#38408=CARTESIAN_POINT('Ctrl Pts',(-19.9231542481283,34.3823407683133,124.511841033235)) ;
#38409=CARTESIAN_POINT('Ctrl Pts',(-20.0516612998158,34.2023516879034,124.786832185084)) ;
#38410=CARTESIAN_POINT('Ctrl Pts',(-19.657904162901,34.3955180496239,124.591763757733)) ;
#38411=CARTESIAN_POINT('Ctrl Pts',(-19.7200431655588,34.215528969214,124.886756209317)) ;
#38412=CARTESIAN_POINT('Ctrl Pts',(-19.3810401547888,34.408785510138,124.625633782009)) ;
#38413=CARTESIAN_POINT('Ctrl Pts',(-19.3739840223189,34.2287964297281,124.929088135759)) ;
#38414=CARTESIAN_POINT('Ctrl Pts',(-19.0312401721135,34.4253994008252,124.576410369976)) ;
#38415=CARTESIAN_POINT('Ctrl Pts',(-18.9367200239934,34.2454103204153,124.867555179956)) ;
#38416=CARTESIAN_POINT('Ctrl Pts',(-18.6565409852236,34.4453482002526,124.377526322459)) ;
#38417=CARTESIAN_POINT('Ctrl Pts',(-18.4683529488441,34.2653591198428,124.618947214289)) ;
#38418=CARTESIAN_POINT('Ctrl Pts',(-18.372722975046,34.4652693117834,124.063178650212)) ;
#38419=CARTESIAN_POINT('Ctrl Pts',(-18.1135823384901,34.2852802313736,124.226010700045)) ;
#38420=CARTESIAN_POINT('Ctrl Pts',(-18.2127872385282,34.4851357599563,123.672140863886)) ;
#38421=CARTESIAN_POINT('Ctrl Pts',(-17.9136663304717,34.3051466795465,123.737213595572)) ;
#38422=CARTESIAN_POINT('Ctrl Pts',(-18.1960174572984,34.5051621065734,123.246703868946)) ;
#38423=CARTESIAN_POINT('Ctrl Pts',(-17.8927069830595,34.3251730261636,123.205416904753)) ;
#38424=CARTESIAN_POINT('Ctrl Pts',(-18.3244861075331,34.525024150963,122.844320049915)) ;
#38425=CARTESIAN_POINT('Ctrl Pts',(-18.0532950836651,34.3450350705532,122.702439446639)) ;
#38426=CARTESIAN_POINT('Ctrl Pts',(-18.5830265246617,34.5449694536441,122.508225439242)) ;
#38427=CARTESIAN_POINT('Ctrl Pts',(-18.3764719974308,34.3649803732343,122.282323158673)) ;
#38428=CARTESIAN_POINT('Ctrl Pts',(-18.9399371008137,34.564864760703,122.281121704416)) ;
#38429=CARTESIAN_POINT('Ctrl Pts',(-18.8226102498353,34.3848756802931,121.998446004873)) ;
#38430=CARTESIAN_POINT('Ctrl Pts',(-19.3527127164133,34.5847580308706,122.188711680669)) ;
#38431=CARTESIAN_POINT('Ctrl Pts',(-19.3385786404535,34.4047689504608,121.882935209687)) ;
#38432=CARTESIAN_POINT('Ctrl Pts',(-19.7737254388914,34.604723623551,122.242987808738)) ;
#38433=CARTESIAN_POINT('Ctrl Pts',(-19.8648438727178,34.4247345431412,121.950781567491)) ;
#38434=CARTESIAN_POINT('Ctrl Pts',(-20.1494199931143,34.6245989472359,122.436554500858)) ;
#38435=CARTESIAN_POINT('Ctrl Pts',(-20.3344600161098,34.444609866826,122.19273979903)) ;
#38436=CARTESIAN_POINT('Ctrl Pts',(-20.4382613496929,34.6445740098108,122.747966146561)) ;
#38437=CARTESIAN_POINT('Ctrl Pts',(-20.6955112754872,34.464584929401,122.582004291028)) ;
#38438=CARTESIAN_POINT('Ctrl Pts',(-20.6027074825129,34.6645264194419,123.139039458747)) ;
#38439=CARTESIAN_POINT('Ctrl Pts',(-20.90106819709,34.4845373390321,123.07084543129)) ;
#38440=CARTESIAN_POINT('Ctrl Pts',(-20.6245230947549,34.684362473678,123.560242571632)) ;
#38441=CARTESIAN_POINT('Ctrl Pts',(-20.9283379624116,34.5043733932682,123.597346656972)) ;
#38442=CARTESIAN_POINT('Ctrl Pts',(-20.5008638045205,34.7043403850956,123.9666287374)) ;
#38443=CARTESIAN_POINT('Ctrl Pts',(-20.7737648834349,34.5243513046858,124.105329355259)) ;
#38444=CARTESIAN_POINT('Ctrl Pts',(-20.2463289326715,34.7242584345991,124.305081206645)) ;
#38445=CARTESIAN_POINT('Ctrl Pts',(-20.4555977349915,34.5442693541892,124.528394482455)) ;
#38446=CARTESIAN_POINT('Ctrl Pts',(-19.8929765679083,34.7441265783672,124.53677216459)) ;
#38447=CARTESIAN_POINT('Ctrl Pts',(-20.0139097342073,34.5641374979573,124.818008765384)) ;
#38448=CARTESIAN_POINT('Ctrl Pts',(-19.4780285765812,34.7641774349545,124.634188159113)) ;
#38449=CARTESIAN_POINT('Ctrl Pts',(-19.4952245291037,34.5841883545447,124.939780508344)) ;
#38450=CARTESIAN_POINT('Ctrl Pts',(-19.060179710771,34.7839578714104,124.585251419341)) ;
#38451=CARTESIAN_POINT('Ctrl Pts',(-18.9729159061635,34.6039687910005,124.878612004272)) ;
#38452=CARTESIAN_POINT('Ctrl Pts',(-18.6792558296266,34.8039879270882,124.394988896057)) ;
#38453=CARTESIAN_POINT('Ctrl Pts',(-18.4967594861514,34.6239988466783,124.640786108543)) ;
#38454=CARTESIAN_POINT('Ctrl Pts',(-18.3887123278353,34.823869032263,124.087835513571)) ;
#38455=CARTESIAN_POINT('Ctrl Pts',(-18.1335792137184,34.6438799518531,124.256847057507)) ;
#38456=CARTESIAN_POINT('Ctrl Pts',(-18.2193821090019,34.8437494946307,123.70056629443)) ;
#38457=CARTESIAN_POINT('Ctrl Pts',(-17.921913909552,34.6637604142209,123.772762991372)) ;
#38458=CARTESIAN_POINT('Ctrl Pts',(-18.1923412672095,34.8637346417751,123.276475566402)) ;
#38459=CARTESIAN_POINT('Ctrl Pts',(-17.8881094854383,34.6837455613653,123.242649910953)) ;
#38460=CARTESIAN_POINT('Ctrl Pts',(-18.3111763931638,34.8836252203115,122.870576698358)) ;
#38461=CARTESIAN_POINT('Ctrl Pts',(-18.0366497414932,34.7036361399017,122.735276316427)) ;
#38462=CARTESIAN_POINT('Ctrl Pts',(-18.5608208396316,34.9035192401859,122.529106310762)) ;
#38463=CARTESIAN_POINT('Ctrl Pts',(-18.34870157791,34.7235301597761,122.30843669083)) ;
#38464=CARTESIAN_POINT('Ctrl Pts',(-18.9123762892436,34.9234406849123,122.292940920012)) ;
#38465=CARTESIAN_POINT('Ctrl Pts',(-18.7881430602203,34.7434516045024,122.013226846823)) ;
#38466=CARTESIAN_POINT('Ctrl Pts',(-19.322937407292,34.9433388229677,122.190263489512)) ;
#38467=CARTESIAN_POINT('Ctrl Pts',(-19.3013427498068,34.7633497425579,121.884875817317)) ;
#38468=CARTESIAN_POINT('Ctrl Pts',(-19.7472655180878,34.9634095781838,122.235024621243)) ;
#38469=CARTESIAN_POINT('Ctrl Pts',(-19.831753866014,34.783420497774,121.940822959817)) ;
#38470=CARTESIAN_POINT('Ctrl Pts',(-20.1256368241744,34.983195128235,122.419137958029)) ;
#38471=CARTESIAN_POINT('Ctrl Pts',(-20.304718807225,34.8032060478252,122.170959918771)) ;
#38472=CARTESIAN_POINT('Ctrl Pts',(-20.4220114238497,35.0031782031124,122.723491321835)) ;
#38473=CARTESIAN_POINT('Ctrl Pts',(-20.6751904640784,34.8231891227026,122.551398320175)) ;
#38474=CARTESIAN_POINT('Ctrl Pts',(-20.5955208583163,35.0230872857583,123.109625284551)) ;
#38475=CARTESIAN_POINT('Ctrl Pts',(-20.8920819874043,34.8430982053485,123.034062768694)) ;
#38476=CARTESIAN_POINT('Ctrl Pts',(-20.6279870536071,35.0429458448811,123.530675885179)) ;
#38477=CARTESIAN_POINT('Ctrl Pts',(-20.9326680571387,34.8629567644712,123.560377307956)) ;
#38478=CARTESIAN_POINT('Ctrl Pts',(-20.5133192729208,35.0629892887198,123.941055703616)) ;
#38479=CARTESIAN_POINT('Ctrl Pts',(-20.7893451367236,34.88300020831,124.07334538232)) ;
#38480=CARTESIAN_POINT('Ctrl Pts',(-20.3093835063598,35.079489353449,124.226623757706)) ;
#38481=CARTESIAN_POINT('Ctrl Pts',(-20.5344079581164,34.8995002730392,124.430333478013)) ;
#38482=CARTESIAN_POINT('Ctrl Pts',(-20.092268777163,35.0928790932979,124.405758678577)) ;
#38483=CARTESIAN_POINT('Ctrl Pts',(-20.2630356080209,34.912890012888,124.654232063072)) ;
#38484=CARTESIAN_POINT('Ctrl Pts',(-19.9119702886458,35.1027359945063,124.507953316112)) ;
#38485=CARTESIAN_POINT('Ctrl Pts',(-20.0376601532966,34.9227469140964,124.78198202428)) ;
#38486=CARTESIAN_POINT('Ctrl Pts',(-19.7141970013292,35.1127275203528,124.578624517524)) ;
#38487=CARTESIAN_POINT('Ctrl Pts',(-19.7904462532024,34.9327384399429,124.870322609991)) ;
#38488=CARTESIAN_POINT('Ctrl Pts',(-19.5084940721676,35.1226522008037,124.613732527868)) ;
#38489=CARTESIAN_POINT('Ctrl Pts',(-19.5333148830191,34.9426631203939,124.914209741569)) ;
#38490=CARTESIAN_POINT('Ctrl Pts',(-19.2980655867416,35.1326627908481,124.612658643822)) ;
#38491=CARTESIAN_POINT('Ctrl Pts',(-19.2702905171921,34.9526737104383,124.912873328906)) ;
#38492=CARTESIAN_POINT('Ctrl Pts',(-19.0237133873326,35.1459220515518,124.563175266845)) ;
#38493=CARTESIAN_POINT('Ctrl Pts',(-18.9272936377621,34.965932971142,124.85100643063)) ;
#38494=CARTESIAN_POINT('Ctrl Pts',(-18.7669990026085,35.1592731267021,124.442141475141)) ;
#38495=CARTESIAN_POINT('Ctrl Pts',(-18.6064360058231,34.9792840462923,124.699721053727)) ;
#38496=CARTESIAN_POINT('Ctrl Pts',(-18.5548922307535,35.1724794359369,124.262885149978)) ;
#38497=CARTESIAN_POINT('Ctrl Pts',(-18.3413122765089,34.9924903555271,124.475665673897)) ;
#38498=CARTESIAN_POINT('Ctrl Pts',(-18.4202016194479,35.1824662695272,124.101878407724)) ;
#38499=CARTESIAN_POINT('Ctrl Pts',(-18.1729444099788,35.0024771891173,124.274406568273)) ;
#38500=CARTESIAN_POINT('Ctrl Pts',(-18.3157421931826,35.1924189970233,123.920538588917)) ;
#38501=CARTESIAN_POINT('Ctrl Pts',(-18.0423683361374,35.0124299166134,124.047733829705)) ;
#38502=CARTESIAN_POINT('Ctrl Pts',(-18.243859696856,35.2024670938648,123.721927113406)) ;
#38503=CARTESIAN_POINT('Ctrl Pts',(-17.9525123754885,35.022478013455,123.799470169286)) ;
#38504=CARTESIAN_POINT('Ctrl Pts',(-18.2080532676477,35.2123085507367,123.518130094329)) ;
#38505=CARTESIAN_POINT('Ctrl Pts',(-17.9077516293332,35.0323194703268,123.544724476249)) ;
#38506=CARTESIAN_POINT('Ctrl Pts',(-18.2077298878391,35.2222948176502,123.308221872427)) ;
#38507=CARTESIAN_POINT('Ctrl Pts',(-17.9073445683003,35.0423057372403,123.28233910936)) ;
#38508=CARTESIAN_POINT('Ctrl Pts',(-18.2435874649064,35.2322314185506,123.102388357164)) ;
#38509=CARTESIAN_POINT('Ctrl Pts',(-17.9521637826458,35.0522423381408,123.025046666894)) ;
#38510=CARTESIAN_POINT('Ctrl Pts',(-18.3155310783834,35.2422813613376,122.903755486322)) ;
#38511=CARTESIAN_POINT('Ctrl Pts',(-18.0420906679153,35.0622922809278,122.776754559709)) ;
#38512=CARTESIAN_POINT('Ctrl Pts',(-18.4186601658913,35.2521315610234,122.724163217864)) ;
#38513=CARTESIAN_POINT('Ctrl Pts',(-18.1709996405976,35.0721424806135,122.552262724079)) ;
#38514=CARTESIAN_POINT('Ctrl Pts',(-18.5526102972871,35.2621044659555,122.562900255392)) ;
#38515=CARTESIAN_POINT('Ctrl Pts',(-18.3384352196135,35.0821153855456,122.350682137538)) ;
#38516=CARTESIAN_POINT('Ctrl Pts',(-18.7130161190752,35.2721028404351,122.427018538122)) ;
#38517=CARTESIAN_POINT('Ctrl Pts',(-18.5389407429499,35.0921137600253,122.180827804049)) ;
#38518=CARTESIAN_POINT('Ctrl Pts',(-18.8950233937213,35.2821230143051,122.320968913956)) ;
#38519=CARTESIAN_POINT('Ctrl Pts',(-18.7664484679587,35.1021339338953,122.048263316503)) ;
#38520=CARTESIAN_POINT('Ctrl Pts',(-19.0902785173193,35.2920240582471,122.248825467389)) ;
#38521=CARTESIAN_POINT('Ctrl Pts',(-19.0105165623508,35.1120349778372,121.958081319007)) ;
#38522=CARTESIAN_POINT('Ctrl Pts',(-19.2968437850745,35.3020128619714,122.211027115049)) ;
#38523=CARTESIAN_POINT('Ctrl Pts',(-19.2687227454452,35.1220237815616,121.91083061917)) ;
#38524=CARTESIAN_POINT('Ctrl Pts',(-19.5063361205008,35.3119783288032,122.209821899411)) ;
#38525=CARTESIAN_POINT('Ctrl Pts',(-19.5305882706749,35.1319892483934,121.909321300871)) ;
#38526=CARTESIAN_POINT('Ctrl Pts',(-19.7116863669934,35.3218818910762,122.244299443621)) ;
#38527=CARTESIAN_POINT('Ctrl Pts',(-19.7872767838553,35.1418928106663,121.952415553916)) ;
#38528=CARTESIAN_POINT('Ctrl Pts',(-19.9109411377999,35.3319425689542,122.31516138068)) ;
#38529=CARTESIAN_POINT('Ctrl Pts',(-20.0363461470048,35.1519534885443,122.040990349763)) ;
#38530=CARTESIAN_POINT('Ctrl Pts',(-20.0910169677187,35.3417828669036,122.417053554877)) ;
#38531=CARTESIAN_POINT('Ctrl Pts',(-20.2614426416731,35.1617937864938,122.168353377838)) ;
#38532=CARTESIAN_POINT('Ctrl Pts',(-20.2543967354931,35.3518458618131,122.551408724914)) ;
#38533=CARTESIAN_POINT('Ctrl Pts',(-20.4656690482837,35.1718567814032,122.336295208353)) ;
#38534=CARTESIAN_POINT('Ctrl Pts',(-20.389561216917,35.3617401559602,122.709546984576)) ;
#38535=CARTESIAN_POINT('Ctrl Pts',(-20.6346269467012,35.1817510755504,122.533966500699)) ;
#38536=CARTESIAN_POINT('Ctrl Pts',(-20.4961856714635,35.3716819536571,122.889282267769)) ;
#38537=CARTESIAN_POINT('Ctrl Pts',(-20.7679099511317,35.1916928732473,122.758634465318)) ;
#38538=CARTESIAN_POINT('Ctrl Pts',(-20.5705249428159,35.3816845311862,123.08601924968)) ;
#38539=CARTESIAN_POINT('Ctrl Pts',(-20.8608365588949,35.2016954507764,123.004554830553)) ;
#38540=CARTESIAN_POINT('Ctrl Pts',(-20.6093729379891,35.3917189951073,123.293356771096)) ;
#38541=CARTESIAN_POINT('Ctrl Pts',(-20.9093992124096,35.2117299146974,123.263726218805)) ;
#38542=CARTESIAN_POINT('Ctrl Pts',(-20.6119121965854,35.4015651336283,123.500344351237)) ;
#38543=CARTESIAN_POINT('Ctrl Pts',(-20.9125759543074,35.2215760532185,123.522461220012)) ;
#38544=CARTESIAN_POINT('Ctrl Pts',(-20.5784797869807,35.4115463068653,123.707482594867)) ;
#38545=CARTESIAN_POINT('Ctrl Pts',(-20.8707879749445,35.2315572264555,123.781384610277)) ;
#38546=CARTESIAN_POINT('Ctrl Pts',(-20.5097340551168,35.4214986008226,123.905101498051)) ;
#38547=CARTESIAN_POINT('Ctrl Pts',(-20.7848581741981,35.2415095204127,124.02840934673)) ;
#38548=CARTESIAN_POINT('Ctrl Pts',(-20.4074763823881,35.4314973959572,124.088777449656)) ;
#38549=CARTESIAN_POINT('Ctrl Pts',(-20.6570382604002,35.2515083155473,124.258005618695)) ;
#38550=CARTESIAN_POINT('Ctrl Pts',(-20.2740486464451,35.441536504218,124.252287560575)) ;
#38551=CARTESIAN_POINT('Ctrl Pts',(-20.4902556613288,35.2615474238082,124.46239487073)) ;
#38552=CARTESIAN_POINT('Ctrl Pts',(-20.1179375824698,35.4513614456571,124.387557243279)) ;
#38553=CARTESIAN_POINT('Ctrl Pts',(-20.2951179161425,35.2713723652473,124.631484396913)) ;
#38554=CARTESIAN_POINT('Ctrl Pts',(-19.9367669407761,35.4614161327315,124.496432561187)) ;
#38555=CARTESIAN_POINT('Ctrl Pts',(-20.0686559822172,35.2814270523217,124.767580615246)) ;
#38556=CARTESIAN_POINT('Ctrl Pts',(-19.7414940311369,35.4713589376717,124.571026731004)) ;
#38557=CARTESIAN_POINT('Ctrl Pts',(-19.8245654449481,35.2913698572619,124.860825828443)) ;
#38558=CARTESIAN_POINT('Ctrl Pts',(-19.5371642498936,35.4812627236682,124.611053711609)) ;
#38559=CARTESIAN_POINT('Ctrl Pts',(-19.569153162575,35.3012736432584,124.910862029664)) ;
#38560=CARTESIAN_POINT('Ctrl Pts',(-19.3260021505189,35.491309540233,124.614922626693)) ;
#38561=CARTESIAN_POINT('Ctrl Pts',(-19.3052006854383,35.3113204598231,124.915700617932)) ;
#38562=CARTESIAN_POINT('Ctrl Pts',(-19.1204374563193,35.5012050597117,124.582740242867)) ;
#38563=CARTESIAN_POINT('Ctrl Pts',(-19.0482438727932,35.3212159793018,124.875474923226)) ;
#38564=CARTESIAN_POINT('Ctrl Pts',(-18.9203301984494,35.5112671450361,124.514241085289)) ;
#38565=CARTESIAN_POINT('Ctrl Pts',(-18.7981091918195,35.3312780646263,124.78985331279)) ;
#38566=CARTESIAN_POINT('Ctrl Pts',(-18.7390904234207,35.521109855994,124.414343573593)) ;
#38567=CARTESIAN_POINT('Ctrl Pts',(-18.5715575696293,35.3411207755842,124.664983089967)) ;
#38568=CARTESIAN_POINT('Ctrl Pts',(-18.575252732091,35.5311005733001,124.282960921875)) ;
#38569=CARTESIAN_POINT('Ctrl Pts',(-18.3667589019596,35.3511114928903,124.500756432861)) ;
#38570=CARTESIAN_POINT('Ctrl Pts',(-18.4375879398549,35.5410286563966,124.126065100434)) ;
#38571=CARTESIAN_POINT('Ctrl Pts',(-18.1946758846968,35.3610395759868,124.304637787701)) ;
#38572=CARTESIAN_POINT('Ctrl Pts',(-18.3282912493656,35.5510165865084,123.94676509158)) ;
#38573=CARTESIAN_POINT('Ctrl Pts',(-18.0580530663617,35.3710275060986,124.080513755033)) ;
#38574=CARTESIAN_POINT('Ctrl Pts',(-18.2517565825726,35.5610524126357,123.750158377981)) ;
#38575=CARTESIAN_POINT('Ctrl Pts',(-17.9623826479832,35.3810633322259,123.834756266212)) ;
#38576=CARTESIAN_POINT('Ctrl Pts',(-18.2109351619,35.5709077497493,123.547017923555)) ;
#38577=CARTESIAN_POINT('Ctrl Pts',(-17.9113535513551,35.3909186693395,123.580830234508)) ;
#38578=CARTESIAN_POINT('Ctrl Pts',(-18.2056029932862,35.5809054845995,123.336924382834)) ;
#38579=CARTESIAN_POINT('Ctrl Pts',(-17.9046862414438,35.4009164041897,123.318213209576)) ;
#38580=CARTESIAN_POINT('Ctrl Pts',(-18.2364854342571,35.5908133885839,123.130921758617)) ;
#38581=CARTESIAN_POINT('Ctrl Pts',(-17.9432873404419,35.4108243081741,123.060708970224)) ;
#38582=CARTESIAN_POINT('Ctrl Pts',(-18.3030212952615,35.6008244631324,122.931244855466)) ;
#38583=CARTESIAN_POINT('Ctrl Pts',(-18.0264553067541,35.4208353827226,122.811112169796)) ;
#38584=CARTESIAN_POINT('Ctrl Pts',(-18.4037616999809,35.610852318668,122.746053058714)) ;
#38585=CARTESIAN_POINT('Ctrl Pts',(-18.152378938914,35.4308632382582,122.579621476775)) ;
#38586=CARTESIAN_POINT('Ctrl Pts',(-18.532602474964,35.6207099125732,122.583737923954)) ;
#38587=CARTESIAN_POINT('Ctrl Pts',(-18.3134289649953,35.4407208321634,122.376725539673)) ;
#38588=CARTESIAN_POINT('Ctrl Pts',(-18.6900489868914,35.6307365994113,122.443575063873)) ;
#38589=CARTESIAN_POINT('Ctrl Pts',(-18.5102358432647,35.4507475190015,122.201520587854)) ;
#38590=CARTESIAN_POINT('Ctrl Pts',(-18.8697550672844,35.6407652685651,122.333303125857)) ;
#38591=CARTESIAN_POINT('Ctrl Pts',(-18.7348673255347,35.4607761881552,122.063678979637)) ;
#38592=CARTESIAN_POINT('Ctrl Pts',(-19.0621320904684,35.6506104768465,122.256973154102)) ;
#38593=CARTESIAN_POINT('Ctrl Pts',(-18.9753389391847,35.4706213964366,121.968264330537)) ;
#38594=CARTESIAN_POINT('Ctrl Pts',(-19.2677365853568,35.6606011658096,122.214031607131)) ;
#38595=CARTESIAN_POINT('Ctrl Pts',(-19.2323443952297,35.4806120853998,121.914585661978)) ;
#38596=CARTESIAN_POINT('Ctrl Pts',(-19.4786728867515,35.6706390420919,122.207881553144)) ;
#38597=CARTESIAN_POINT('Ctrl Pts',(-19.4960145845465,35.4906499616821,121.906896220125)) ;
#38598=CARTESIAN_POINT('Ctrl Pts',(-19.6835091491884,35.6804834197341,122.237505000338)) ;
#38599=CARTESIAN_POINT('Ctrl Pts',(-19.7520613231503,35.5004943393243,121.943923950891)) ;
#38600=CARTESIAN_POINT('Ctrl Pts',(-19.8829904576665,35.6904682241255,122.302762495252)) ;
#38601=CARTESIAN_POINT('Ctrl Pts',(-20.0014137030145,35.5104791437157,122.025494346752)) ;
#38602=CARTESIAN_POINT('Ctrl Pts',(-20.0673637367163,35.7004077543441,122.401163727744)) ;
#38603=CARTESIAN_POINT('Ctrl Pts',(-20.2318815339164,35.5204186739343,122.148494733282)) ;
#38604=CARTESIAN_POINT('Ctrl Pts',(-20.2334425789832,35.710447442381,122.531393346306)) ;
#38605=CARTESIAN_POINT('Ctrl Pts',(-20.4394809697668,35.5304583619711,122.311280393295)) ;
#38606=CARTESIAN_POINT('Ctrl Pts',(-20.3723559056366,35.7203357317493,122.686064760268)) ;
#38607=CARTESIAN_POINT('Ctrl Pts',(-20.6131244207702,35.5403466513395,122.504619288764)) ;
#38608=CARTESIAN_POINT('Ctrl Pts',(-20.4837508188583,35.7303248554341,122.864079606437)) ;
#38609=CARTESIAN_POINT('Ctrl Pts',(-20.7523694042622,35.5503357750242,122.727137258845)) ;
#38610=CARTESIAN_POINT('Ctrl Pts',(-20.5621646542934,35.7402848651087,123.058229679049)) ;
#38611=CARTESIAN_POINT('Ctrl Pts',(-20.850388256129,35.5602957846989,122.969824688624)) ;
#38612=CARTESIAN_POINT('Ctrl Pts',(-20.6059033424676,35.7501852948129,123.261726613465)) ;
#38613=CARTESIAN_POINT('Ctrl Pts',(-20.9050630990468,35.5701962144031,123.224196430438)) ;
#38614=CARTESIAN_POINT('Ctrl Pts',(-20.6137449772283,35.7602283762197,123.472709317713)) ;
#38615=CARTESIAN_POINT('Ctrl Pts',(-20.9148664710667,35.5802392958098,123.487924566712)) ;
#38616=CARTESIAN_POINT('Ctrl Pts',(-20.5852260061574,35.7701357701273,123.67904320518)) ;
#38617=CARTESIAN_POINT('Ctrl Pts',(-20.8792189655505,35.5901466897175,123.745842918038)) ;
#38618=CARTESIAN_POINT('Ctrl Pts',(-20.5210141564566,35.7801475011165,123.879489186249)) ;
#38619=CARTESIAN_POINT('Ctrl Pts',(-20.7989552796093,35.6001584207067,123.996400804907)) ;
#38620=CARTESIAN_POINT('Ctrl Pts',(-20.4224008662751,35.7901797188313,124.06593183367)) ;
#38621=CARTESIAN_POINT('Ctrl Pts',(-20.6756899073962,35.6101906384214,124.229454654576)) ;
#38622=CARTESIAN_POINT('Ctrl Pts',(-20.2954649937383,35.8000322280774,124.229594024067)) ;
#38623=CARTESIAN_POINT('Ctrl Pts',(-20.5170202760373,35.6200431476676,124.434034154128)) ;
#38624=CARTESIAN_POINT('Ctrl Pts',(-20.1408226833668,35.8099901646204,124.370712894289)) ;
#38625=CARTESIAN_POINT('Ctrl Pts',(-20.3237177194056,35.6300010842106,124.610433802468)) ;
#38626=CARTESIAN_POINT('Ctrl Pts',(-19.9624034194556,35.8200290346287,124.483417161163)) ;
#38627=CARTESIAN_POINT('Ctrl Pts',(-20.1006943915222,35.6400399542189,124.751315017592)) ;
#38628=CARTESIAN_POINT('Ctrl Pts',(-19.7704532057316,35.829902189787,124.56248627394)) ;
#38629=CARTESIAN_POINT('Ctrl Pts',(-19.8607559657589,35.6499131093772,124.850152762087)) ;
#38630=CARTESIAN_POINT('Ctrl Pts',(-19.5636408193586,35.8399754646367,124.607848543225)) ;
#38631=CARTESIAN_POINT('Ctrl Pts',(-19.6022411196916,35.6599863842269,124.906856510857)) ;
#38632=CARTESIAN_POINT('Ctrl Pts',(-19.3573296065172,35.8497957818141,124.616666849155)) ;
#38633=CARTESIAN_POINT('Ctrl Pts',(-19.3443505908439,35.6698067014042,124.917880380805)) ;
#38634=CARTESIAN_POINT('Ctrl Pts',(-19.1473070231254,35.8598744676076,124.58902082137)) ;
#38635=CARTESIAN_POINT('Ctrl Pts',(-19.0818227173848,35.6798853871977,124.883323751805)) ;
#38636=CARTESIAN_POINT('Ctrl Pts',(-18.9497113689918,35.8697259789907,124.526804413324)) ;
#38637=CARTESIAN_POINT('Ctrl Pts',(-18.8348266453124,35.6897368985808,124.805553629487)) ;
#38638=CARTESIAN_POINT('Ctrl Pts',(-18.7617765756378,35.8797994252973,124.429271647714)) ;
#38639=CARTESIAN_POINT('Ctrl Pts',(-18.5999081950483,35.6998103448875,124.683638544775)) ;
#38640=CARTESIAN_POINT('Ctrl Pts',(-18.597467101793,35.889640700422,124.303505365942)) ;
#38641=CARTESIAN_POINT('Ctrl Pts',(-18.3945197611564,35.7096516200122,124.526430434766)) ;
#38642=CARTESIAN_POINT('Ctrl Pts',(-18.4549920931084,35.8996258000788,124.149368497595)) ;
#38643=CARTESIAN_POINT('Ctrl Pts',(-18.2164254320206,35.7196367196689,124.333759479589)) ;
#38644=CARTESIAN_POINT('Ctrl Pts',(-18.3414173666157,35.9096332762131,123.972250384681)) ;
#38645=CARTESIAN_POINT('Ctrl Pts',(-18.0744564632935,35.7296441958033,124.11236211311)) ;
#38646=CARTESIAN_POINT('Ctrl Pts',(-18.2608430560108,35.919555863922,123.779847146659)) ;
#38647=CARTESIAN_POINT('Ctrl Pts',(-17.9737377683904,35.7395667835122,123.871857563542)) ;
#38648=CARTESIAN_POINT('Ctrl Pts',(-18.2142645919712,35.9295424681954,123.575109420464)) ;
#38649=CARTESIAN_POINT('Ctrl Pts',(-17.9155142333491,35.7495533877855,123.615935266931)) ;
#38650=CARTESIAN_POINT('Ctrl Pts',(-18.2042845382939,35.9395825965295,123.364287204911)) ;
#38651=CARTESIAN_POINT('Ctrl Pts',(-17.9030386019391,35.7595935161196,123.352407710943)) ;
#38652=CARTESIAN_POINT('Ctrl Pts',(-18.2300836682839,35.9494220310629,123.159025741679)) ;
#38653=CARTESIAN_POINT('Ctrl Pts',(-17.9352873093069,35.7694329506531,123.095829360988)) ;
#38654=CARTESIAN_POINT('Ctrl Pts',(-18.2923429640459,35.9594860855539,122.956842133847)) ;
#38655=CARTESIAN_POINT('Ctrl Pts',(-18.0131110082293,35.779497005144,122.843100123042)) ;
#38656=CARTESIAN_POINT('Ctrl Pts',(-18.3872080620054,35.969377004791,122.771780131143)) ;
#38657=CARTESIAN_POINT('Ctrl Pts',(-18.1316925351678,35.7893879243812,122.61177152467)) ;
#38658=CARTESIAN_POINT('Ctrl Pts',(-18.5136711614344,35.9793689980971,122.604062443733)) ;
#38659=CARTESIAN_POINT('Ctrl Pts',(-18.2897713916433,35.7993799176872,122.402124132934)) ;
#38660=CARTESIAN_POINT('Ctrl Pts',(-18.6670229740416,35.9893318620564,122.461407293779)) ;
#38661=CARTESIAN_POINT('Ctrl Pts',(-18.4814613117937,35.8093427816465,122.2238046921)) ;
#38662=CARTESIAN_POINT('Ctrl Pts',(-18.8415130358515,35.9992361218741,122.347760866079)) ;
#38663=CARTESIAN_POINT('Ctrl Pts',(-18.6995746479516,35.8192470414643,122.081746101309)) ;
#38664=CARTESIAN_POINT('Ctrl Pts',(-19.0361390397703,36.0092966124456,122.26503638611)) ;
#38665=CARTESIAN_POINT('Ctrl Pts',(-18.9428567780689,35.8293075320357,121.978340523803)) ;
#38666=CARTESIAN_POINT('Ctrl Pts',(-19.2376557259542,36.0191369620766,122.218129994328)) ;
#38667=CARTESIAN_POINT('Ctrl Pts',(-19.1947540651951,35.8391478816668,121.919707183681)) ;
#38668=CARTESIAN_POINT('Ctrl Pts',(-19.4488594057997,36.0291999375666,122.206420949229)) ;
#38669=CARTESIAN_POINT('Ctrl Pts',(-19.4587582959339,35.8492108571568,121.905070980608)) ;
#38670=CARTESIAN_POINT('Ctrl Pts',(-19.6553963029658,36.03909425771,122.231316246705)) ;
#38671=CARTESIAN_POINT('Ctrl Pts',(-19.716930430741,35.8591051773002,121.936190237878)) ;
#38672=CARTESIAN_POINT('Ctrl Pts',(-19.8555419191766,36.0490359708416,122.291429452583)) ;
#38673=CARTESIAN_POINT('Ctrl Pts',(-19.9671129942115,35.8690468904317,122.011332156025)) ;
#38674=CARTESIAN_POINT('Ctrl Pts',(-20.0434534803591,36.0590388606357,122.385905221195)) ;
#38675=CARTESIAN_POINT('Ctrl Pts',(-20.2020024297715,35.8790497802259,122.129427167132)) ;
#38676=CARTESIAN_POINT('Ctrl Pts',(-20.2124564475029,36.0690787177962,122.512316557016)) ;
#38677=CARTESIAN_POINT('Ctrl Pts',(-20.4132559197918,35.8890896373864,122.287441324551)) ;
#38678=CARTESIAN_POINT('Ctrl Pts',(-20.3542066989014,36.0789028986338,122.662550738687)) ;
#38679=CARTESIAN_POINT('Ctrl Pts',(-20.5904446049979,35.898913818224,122.475235421975)) ;
#38680=CARTESIAN_POINT('Ctrl Pts',(-20.4706332696789,36.088959872137,122.839015977808)) ;
#38681=CARTESIAN_POINT('Ctrl Pts',(-20.7359772784727,35.9089707917272,122.695816923805)) ;
#38682=CARTESIAN_POINT('Ctrl Pts',(-20.5533425088199,36.0988879963241,123.030662056921)) ;
#38683=CARTESIAN_POINT('Ctrl Pts',(-20.8393638310025,35.9188989159142,122.935375322658)) ;
#38684=CARTESIAN_POINT('Ctrl Pts',(-20.6021853906492,36.1088416913975,123.234141443748)) ;
#38685=CARTESIAN_POINT('Ctrl Pts',(-20.9004170384747,35.9288526109877,123.189725205671)) ;
#38686=CARTESIAN_POINT('Ctrl Pts',(-20.6147732903502,36.1188878849728,123.444966785403)) ;
#38687=CARTESIAN_POINT('Ctrl Pts',(-20.9161514804583,35.9388988045629,123.453256665998)) ;
#38688=CARTESIAN_POINT('Ctrl Pts',(-20.5912389874168,36.1287359873327,123.65066140107)) ;
#38689=CARTESIAN_POINT('Ctrl Pts',(-20.8867329497479,35.9487469069229,123.710376268583)) ;
#38690=CARTESIAN_POINT('Ctrl Pts',(-20.5322920817203,36.1386975755603,123.851608665551)) ;
#38691=CARTESIAN_POINT('Ctrl Pts',(-20.8130484687253,35.9587084951504,123.961560575072)) ;
#38692=CARTESIAN_POINT('Ctrl Pts',(-20.4384766708263,36.1487262457165,124.040434185181)) ;
#38693=CARTESIAN_POINT('Ctrl Pts',(-20.6957786699468,35.9687371653067,124.19759210039)) ;
#38694=CARTESIAN_POINT('Ctrl Pts',(-20.3148448154568,36.1586365485983,124.208121309133)) ;
#38695=CARTESIAN_POINT('Ctrl Pts',(-20.5412377893626,35.9786474681884,124.407201312271)) ;
#38696=CARTESIAN_POINT('Ctrl Pts',(-20.1639673049378,36.1685714324062,124.352558297041)) ;
#38697=CARTESIAN_POINT('Ctrl Pts',(-20.3526398125577,35.9885823519964,124.587747365934)) ;
#38698=CARTESIAN_POINT('Ctrl Pts',(-19.9883464931502,36.1786125740968,124.4696744726)) ;
#38699=CARTESIAN_POINT('Ctrl Pts',(-20.1331135059833,35.998623493687,124.734141809711)) ;
#38700=CARTESIAN_POINT('Ctrl Pts',(-19.7980654386768,36.1884996952608,124.553357993941)) ;
#38701=CARTESIAN_POINT('Ctrl Pts',(-19.8952608882238,36.008510614851,124.83874584046)) ;
#38702=CARTESIAN_POINT('Ctrl Pts',(-19.5941039539844,36.1984920381093,124.603590833534)) ;
#38703=CARTESIAN_POINT('Ctrl Pts',(-19.6403085962597,36.0185029576995,124.901535971486)) ;
#38704=CARTESIAN_POINT('Ctrl Pts',(-19.3854139464057,36.2084403393333,124.617526696654)) ;
#38705=CARTESIAN_POINT('Ctrl Pts',(-19.3794454821453,36.0284512589234,124.918954868262)) ;
#38706=CARTESIAN_POINT('Ctrl Pts',(-19.1776885830865,36.2183779170154,124.595344537768)) ;
#38707=CARTESIAN_POINT('Ctrl Pts',(-19.1197882532183,36.0383888366056,124.891226019477)) ;
#38708=CARTESIAN_POINT('Ctrl Pts',(-18.9758949839322,36.228364491466,124.537343966283)) ;
#38709=CARTESIAN_POINT('Ctrl Pts',(-18.8675463523615,36.0483754110561,124.818724120337)) ;
#38710=CARTESIAN_POINT('Ctrl Pts',(-18.7865605948736,36.2383933013744,124.444585421192)) ;
#38711=CARTESIAN_POINT('Ctrl Pts',(-18.6308789215962,36.0584042209646,124.702775017939)) ;
#38712=CARTESIAN_POINT('Ctrl Pts',(-18.6186460163788,36.2482716226812,124.322389246568)) ;
#38713=CARTESIAN_POINT('Ctrl Pts',(-18.4209855121362,36.0682825422714,124.550028242174)) ;
#38714=CARTESIAN_POINT('Ctrl Pts',(-18.4724839475725,36.2582632700286,124.171514768616)) ;
#38715=CARTESIAN_POINT('Ctrl Pts',(-18.2382837455573,36.0782741896188,124.361434085775)) ;
#38716=CARTESIAN_POINT('Ctrl Pts',(-18.3546005152364,36.2682977934664,123.996579143374)) ;
#38717=CARTESIAN_POINT('Ctrl Pts',(-18.0909304836931,36.0883087130566,124.14276398916)) ;
#38718=CARTESIAN_POINT('Ctrl Pts',(-18.2699376189153,36.278161150345,123.80726784102)) ;
#38719=CARTESIAN_POINT('Ctrl Pts',(-17.985102604673,36.0981720699351,123.906123266349)) ;
#38720=CARTESIAN_POINT('Ctrl Pts',(-18.2183426275422,36.2882313770253,123.601966412164)) ;
#38721=CARTESIAN_POINT('Ctrl Pts',(-17.9206102594322,36.1082422966155,123.649496524014)) ;
#38722=CARTESIAN_POINT('Ctrl Pts',(-18.2035300755518,36.2980736851599,123.395572554759)) ;
#38723=CARTESIAN_POINT('Ctrl Pts',(-17.9020958098303,36.1180846047501,123.391502808903)) ;
#38724=CARTESIAN_POINT('Ctrl Pts',(-18.2242647172834,36.3080344171834,123.187200743274)) ;
#38725=CARTESIAN_POINT('Ctrl Pts',(-17.9280157513934,36.1280453367736,123.13103779863)) ;
#38726=CARTESIAN_POINT('Ctrl Pts',(-18.2817044009816,36.3180723063815,122.984147670972)) ;
#38727=CARTESIAN_POINT('Ctrl Pts',(-17.9998167260215,36.1380832259716,122.877221984958)) ;
#38728=CARTESIAN_POINT('Ctrl Pts',(-18.3716994134048,36.3279465893003,122.797053220826)) ;
#38729=CARTESIAN_POINT('Ctrl Pts',(-18.1123123668166,36.1479575088905,122.643353698626)) ;
#38730=CARTESIAN_POINT('Ctrl Pts',(-18.4951890966193,36.3380163339178,122.625139380423)) ;
#38731=CARTESIAN_POINT('Ctrl Pts',(-18.2666755577788,36.158027253508,122.428462610137)) ;
#38732=CARTESIAN_POINT('Ctrl Pts',(-18.6430502592492,36.3478496442634,122.480641003559)) ;
#38733=CARTESIAN_POINT('Ctrl Pts',(-18.4515040640522,36.1678605638536,122.247839904788)) ;
#38734=CARTESIAN_POINT('Ctrl Pts',(-18.8168167962975,36.3578798876161,122.361190643597)) ;
#38735=CARTESIAN_POINT('Ctrl Pts',(-18.6687131962047,36.1778908072062,122.098528505447)) ;
#38736=CARTESIAN_POINT('Ctrl Pts',(-19.0089931407264,36.3679121755945,122.274279269825)) ;
#38737=CARTESIAN_POINT('Ctrl Pts',(-18.9089342116868,36.1879230951846,121.989890796005)) ;
#38738=CARTESIAN_POINT('Ctrl Pts',(-19.2090377913951,36.3777393520626,122.222649776035)) ;
#38739=CARTESIAN_POINT('Ctrl Pts',(-19.1589917224772,36.1977502716528,121.925355327171)) ;
#38740=CARTESIAN_POINT('Ctrl Pts',(-19.4186819898018,36.3877447349294,122.205814654101)) ;
#38741=CARTESIAN_POINT('Ctrl Pts',(-19.4210472098024,36.2077556545196,121.904313326914)) ;
#38742=CARTESIAN_POINT('Ctrl Pts',(-19.6276479448215,36.3977273739222,122.225666562334)) ;
#38743=CARTESIAN_POINT('Ctrl Pts',(-19.6822546897999,36.2177382935123,121.929130109928)) ;
#38744=CARTESIAN_POINT('Ctrl Pts',(-19.831109521622,36.4077714410588,122.282077039624)) ;
#38745=CARTESIAN_POINT('Ctrl Pts',(-19.9365810272127,36.2277823606489,121.99964491067)) ;
#38746=CARTESIAN_POINT('Ctrl Pts',(-20.0176363662993,36.4175926598628,122.370629532132)) ;
#38747=CARTESIAN_POINT('Ctrl Pts',(-20.1697398906733,36.237603579453,122.110337795511)) ;
#38748=CARTESIAN_POINT('Ctrl Pts',(-20.1899535608722,36.4276294988008,122.49240362926)) ;
#38749=CARTESIAN_POINT('Ctrl Pts',(-20.3851350978056,36.247640418391,122.262557053021)) ;
#38750=CARTESIAN_POINT('Ctrl Pts',(-20.3379053809418,36.4376539108986,122.642492380833)) ;
#38751=CARTESIAN_POINT('Ctrl Pts',(-20.57007350028,36.2576648304888,122.450169309944)) ;
#38752=CARTESIAN_POINT('Ctrl Pts',(-20.4558677797191,36.4475059953039,122.812743968213)) ;
#38753=CARTESIAN_POINT('Ctrl Pts',(-20.7175254013576,36.267516914894,122.662985785886)) ;
#38754=CARTESIAN_POINT('Ctrl Pts',(-20.5439760773838,36.457496892047,123.003382833653)) ;
#38755=CARTESIAN_POINT('Ctrl Pts',(-20.827658912921,36.2775078116372,122.901285416347)) ;
#38756=CARTESIAN_POINT('Ctrl Pts',(-20.5973974591388,36.467414883948,123.20495630849)) ;
#38757=CARTESIAN_POINT('Ctrl Pts',(-20.8944336982195,36.2874258035382,123.153253367659)) ;
#38758=CARTESIAN_POINT('Ctrl Pts',(-20.6152498950623,36.477442999405,123.415005149614)) ;
#38759=CARTESIAN_POINT('Ctrl Pts',(-20.9167470715242,36.2974539189952,123.415814568148)) ;
#38760=CARTESIAN_POINT('Ctrl Pts',(-20.5967150299844,36.4873281753471,123.621999291059)) ;
#38761=CARTESIAN_POINT('Ctrl Pts',(-20.8935762348369,36.3073390949373,123.674557784491)) ;
#38762=CARTESIAN_POINT('Ctrl Pts',(-20.5424427129043,36.497317533754,123.824877571005)) ;
#38763=CARTESIAN_POINT('Ctrl Pts',(-20.8257335493315,36.3173284533442,123.928155184721)) ;
#38764=CARTESIAN_POINT('Ctrl Pts',(-20.4529063543909,36.5073586813343,124.016044649924)) ;
#38765=CARTESIAN_POINT('Ctrl Pts',(-20.7138111339089,36.3273696009244,124.167113009854)) ;
#38766=CARTESIAN_POINT('Ctrl Pts',(-20.3343398025796,36.5171913043407,124.185369576253)) ;
#38767=CARTESIAN_POINT('Ctrl Pts',(-20.5656005076425,36.3372022239309,124.378768633735)) ;
#38768=CARTESIAN_POINT('Ctrl Pts',(-20.1861956020173,36.5271853754515,124.334353336419)) ;
#38769=CARTESIAN_POINT('Ctrl Pts',(-20.3804184421246,36.3471962950417,124.564996698396)) ;
#38770=CARTESIAN_POINT('Ctrl Pts',(-20.013585956424,36.5372140330923,124.455438892729)) ;
#38771=CARTESIAN_POINT('Ctrl Pts',(-20.1646550508687,36.3572249526825,124.716351716275)) ;
#38772=CARTESIAN_POINT('Ctrl Pts',(-19.8254390215131,36.5470983592851,124.543627316343)) ;
#38773=CARTESIAN_POINT('Ctrl Pts',(-19.9294697799038,36.3671092788753,124.826585348524)) ;
#38774=CARTESIAN_POINT('Ctrl Pts',(-19.6233034874049,36.5570641027758,124.598757212987)) ;
#38775=CARTESIAN_POINT('Ctrl Pts',(-19.6767994745844,36.3770750223659,124.895495364901)) ;
#38776=CARTESIAN_POINT('Ctrl Pts',(-19.4133432163963,36.567092481907,124.617767958151)) ;
#38777=CARTESIAN_POINT('Ctrl Pts',(-19.4143489319627,36.3871034014971,124.919256362249)) ;
#38778=CARTESIAN_POINT('Ctrl Pts',(-19.2058808015427,36.5769933281139,124.600571301318)) ;
#38779=CARTESIAN_POINT('Ctrl Pts',(-19.1550206095312,36.397004247704,124.897758003424)) ;
#38780=CARTESIAN_POINT('Ctrl Pts',(-19.0014191299385,36.587051985531,124.546729537717)) ;
#38781=CARTESIAN_POINT('Ctrl Pts',(-18.8994442732489,36.4070629051212,124.830453416139)) ;
#38782=CARTESIAN_POINT('Ctrl Pts',(-18.813096638073,36.5969095483129,124.460143866391)) ;
#38783=CARTESIAN_POINT('Ctrl Pts',(-18.664041621049,36.416920467903,124.722218749331)) ;
#38784=CARTESIAN_POINT('Ctrl Pts',(-18.6390013358373,36.6069779508661,124.339804591474)) ;
#38785=CARTESIAN_POINT('Ctrl Pts',(-18.446424079418,36.4269888704563,124.571792635171)) ;
#38786=CARTESIAN_POINT('Ctrl Pts',(-18.4916105941839,36.6168333496057,124.194162637956)) ;
#38787=CARTESIAN_POINT('Ctrl Pts',(-18.2621870023976,36.4368442691958,124.389737932102)) ;
#38788=CARTESIAN_POINT('Ctrl Pts',(-18.3695504756262,36.6268282166796,124.023135375574)) ;
#38789=CARTESIAN_POINT('Ctrl Pts',(-18.109613965784,36.4468391362698,124.175952224947)) ;
#38790=CARTESIAN_POINT('Ctrl Pts',(-18.2791165716848,36.636859511663,123.832615497264)) ;
#38791=CARTESIAN_POINT('Ctrl Pts',(-17.9965739247964,36.4568704312532,123.937801266172)) ;
#38792=CARTESIAN_POINT('Ctrl Pts',(-18.2237360833858,36.6467260363896,123.632712396887)) ;
#38793=CARTESIAN_POINT('Ctrl Pts',(-17.9273507222651,36.4667369559798,123.687921184564)) ;
#38794=CARTESIAN_POINT('Ctrl Pts',(-18.2033310226805,36.6567135070853,123.423763661605)) ;
#38795=CARTESIAN_POINT('Ctrl Pts',(-17.9018470653367,36.4767244266755,123.426734881174)) ;
#38796=CARTESIAN_POINT('Ctrl Pts',(-18.2193352845113,36.6666582666492,123.215274762374)) ;
#38797=CARTESIAN_POINT('Ctrl Pts',(-17.9218551057962,36.4866691862394,123.166123729033)) ;
#38798=CARTESIAN_POINT('Ctrl Pts',(-18.2719370323567,36.676703822598,123.010765439361)) ;
#38799=CARTESIAN_POINT('Ctrl Pts',(-17.9876098910879,36.4967147421882,122.910487765903)) ;
#38800=CARTESIAN_POINT('Ctrl Pts',(-18.3574522060071,36.6865634109731,122.82192143973)) ;
#38801=CARTESIAN_POINT('Ctrl Pts',(-18.0945065088877,36.5065743305633,122.674433491179)) ;
#38802=CARTESIAN_POINT('Ctrl Pts',(-18.4758403465642,36.6965643661092,122.648211025078)) ;
#38803=CARTESIAN_POINT('Ctrl Pts',(-18.2424940101629,36.5165752856994,122.457296954306)) ;
#38804=CARTESIAN_POINT('Ctrl Pts',(-18.6211027599908,36.7064685933867,122.49899007134)) ;
#38805=CARTESIAN_POINT('Ctrl Pts',(-18.4240741922452,36.5264795129769,122.270772499989)) ;
#38806=CARTESIAN_POINT('Ctrl Pts',(-18.7923364863628,36.7165106702819,122.37555164078)) ;
#38807=CARTESIAN_POINT('Ctrl Pts',(-18.6381179776892,36.5365215898721,122.116476705883)) ;
#38808=CARTESIAN_POINT('Ctrl Pts',(-18.9798717838469,36.726418282968,122.28482859885)) ;
#38809=CARTESIAN_POINT('Ctrl Pts',(-18.8725385168202,36.5464292025582,122.003075302524)) ;
#38810=CARTESIAN_POINT('Ctrl Pts',(-19.1832128493394,36.7364728135838,122.227207958605)) ;
#38811=CARTESIAN_POINT('Ctrl Pts',(-19.1267156102727,36.556483733174,121.931052177894)) ;
#38812=CARTESIAN_POINT('Ctrl Pts',(-19.3894625931079,36.7463336001326,122.206055828831)) ;
#38813=CARTESIAN_POINT('Ctrl Pts',(-19.3845283469654,36.5663445197228,121.904614760516)) ;
#38814=CARTESIAN_POINT('Ctrl Pts',(-19.5990077419193,36.7563273552037,122.220846428092)) ;
#38815=CARTESIAN_POINT('Ctrl Pts',(-19.6464596606134,36.5763382747939,121.923105823605)) ;
#38816=CARTESIAN_POINT('Ctrl Pts',(-19.8014959540694,36.7662527154437,122.271364787942)) ;
#38817=CARTESIAN_POINT('Ctrl Pts',(-19.8995693751414,36.5862636350339,121.9862565339)) ;
#38818=CARTESIAN_POINT('Ctrl Pts',(-19.9940544316431,36.776280644839,122.357120402506)) ;
#38819=CARTESIAN_POINT('Ctrl Pts',(-20.1402663825866,36.5962915644292,122.093453651189)) ;
#38820=CARTESIAN_POINT('Ctrl Pts',(-20.1664982335649,36.7861669116383,122.473197134529)) ;
#38821=CARTESIAN_POINT('Ctrl Pts',(-20.3558196617757,36.6061778312285,122.238551973219)) ;
#38822=CARTESIAN_POINT('Ctrl Pts',(-20.3183982755101,36.7961986805365,122.619450743956)) ;
#38823=CARTESIAN_POINT('Ctrl Pts',(-20.5456928031765,36.6162096001267,122.421371062142)) ;
#38824=CARTESIAN_POINT('Ctrl Pts',(-20.4409436536401,36.8060802763801,122.787245264454)) ;
#38825=CARTESIAN_POINT('Ctrl Pts',(-20.6988722846578,36.6260911959703,122.631115950186)) ;
#38826=CARTESIAN_POINT('Ctrl Pts',(-20.5341804059787,36.8161421618481,122.977086052336)) ;
#38827=CARTESIAN_POINT('Ctrl Pts',(-20.8154157384353,36.6361530814383,122.868418182674)) ;
#38828=CARTESIAN_POINT('Ctrl Pts',(-20.5919244424178,36.825999595867,123.176140531021)) ;
#38829=CARTESIAN_POINT('Ctrl Pts',(-20.8875930299572,36.6460105154571,123.117237354215)) ;
#38830=CARTESIAN_POINT('Ctrl Pts',(-20.6149712049277,36.8359928389089,123.384935530242)) ;
#38831=CARTESIAN_POINT('Ctrl Pts',(-20.9163988743964,36.6560037584991,123.378230437878)) ;
#38832=CARTESIAN_POINT('Ctrl Pts',(-20.6015124206239,36.8459235997953,123.593287168939)) ;
#38833=CARTESIAN_POINT('Ctrl Pts',(-20.8995719079285,36.6659345193854,123.638673612043)) ;
#38834=CARTESIAN_POINT('Ctrl Pts',(-20.5353308402502,36.8592725919925,123.866051377186)) ;
#38835=CARTESIAN_POINT('Ctrl Pts',(-20.816844696695,36.6792835115826,123.979609103894)) ;
#38836=CARTESIAN_POINT('Ctrl Pts',(-20.3999609319661,36.8725409648089,124.11357862058)) ;
#38837=CARTESIAN_POINT('Ctrl Pts',(-20.6476556409082,36.6925518843991,124.288994177513)) ;
#38838=CARTESIAN_POINT('Ctrl Pts',(-20.2075188150344,36.8858239061933,124.315902403528)) ;
#38839=CARTESIAN_POINT('Ctrl Pts',(-20.4070652076919,36.7058348257834,124.541941671603)) ;
#38840=CARTESIAN_POINT('Ctrl Pts',(-20.0375727801162,36.8958666920355,124.441171046121)) ;
#38841=CARTESIAN_POINT('Ctrl Pts',(-20.1946380685307,36.7158776116257,124.698516250098)) ;
#38842=CARTESIAN_POINT('Ctrl Pts',(-19.8521787979742,36.9057166345876,124.533432305183)) ;
#38843=CARTESIAN_POINT('Ctrl Pts',(-19.9628921815121,36.7257275541777,124.813842499305)) ;
#38844=CARTESIAN_POINT('Ctrl Pts',(-19.6507731123258,36.9157138675065,124.593480412264)) ;
#38845=CARTESIAN_POINT('Ctrl Pts',(-19.711136668814,36.7357247870967,124.888900023819)) ;
#38846=CARTESIAN_POINT('Ctrl Pts',(-19.4415809415258,36.9257287628411,124.617367629168)) ;
#38847=CARTESIAN_POINT('Ctrl Pts',(-19.4496388355462,36.7457396824312,124.918754107252)) ;
#38848=CARTESIAN_POINT('Ctrl Pts',(-19.1637149095619,36.9389684394793,124.600711262707)) ;
#38849=CARTESIAN_POINT('Ctrl Pts',(-19.1023419164325,36.7589793590695,124.897941856182)) ;
#38850=CARTESIAN_POINT('Ctrl Pts',(-18.8297170296114,36.9555156638846,124.490312279794)) ;
#38851=CARTESIAN_POINT('Ctrl Pts',(-18.6847931249535,36.7755265834747,124.759912522022)) ;
#38852=CARTESIAN_POINT('Ctrl Pts',(-18.5515569849989,36.9721631010157,124.271299498721)) ;
#38853=CARTESIAN_POINT('Ctrl Pts',(-18.3371603329955,36.7921740206059,124.486198909342)) ;
#38854=CARTESIAN_POINT('Ctrl Pts',(-18.3844875359923,36.9854525984939,124.047410122767)) ;
#38855=CARTESIAN_POINT('Ctrl Pts',(-18.12827768874,36.8054635180841,124.206288377177)) ;
#38856=CARTESIAN_POINT('Ctrl Pts',(-18.2905524045651,36.9953260063163,123.862298699992)) ;
#38857=CARTESIAN_POINT('Ctrl Pts',(-18.0108710101384,36.8153369259064,123.974907927286)) ;
#38858=CARTESIAN_POINT('Ctrl Pts',(-18.2290667315247,37.005378383909,123.660120832007)) ;
#38859=CARTESIAN_POINT('Ctrl Pts',(-17.9340138083653,36.8253893034992,123.722181735782)) ;
#38860=CARTESIAN_POINT('Ctrl Pts',(-18.2040801154488,37.0152820374499,123.45340205248)) ;
#38861=CARTESIAN_POINT('Ctrl Pts',(-17.9027830694493,36.8352929570401,123.463785283057)) ;
#38862=CARTESIAN_POINT('Ctrl Pts',(-18.214904553946,37.0252263064452,123.244652571559)) ;
#38863=CARTESIAN_POINT('Ctrl Pts',(-17.9163185740289,36.8452372260354,123.20284412537)) ;
#38864=CARTESIAN_POINT('Ctrl Pts',(-18.2776834319682,37.0385573147779,122.97143393021)) ;
#38865=CARTESIAN_POINT('Ctrl Pts',(-17.9947816308902,36.858568234368,122.861344091151)) ;
#38866=CARTESIAN_POINT('Ctrl Pts',(-18.4435275534842,37.0551788953021,122.659444683358)) ;
#38867=CARTESIAN_POINT('Ctrl Pts',(-18.2021201495305,36.8751898148923,122.471324046432)) ;
#38868=CARTESIAN_POINT('Ctrl Pts',(-18.704290384894,37.0717215660005,122.423272162924)) ;
#38869=CARTESIAN_POINT('Ctrl Pts',(-18.5280140337885,36.8917324855907,122.176159129559)) ;
#38870=CARTESIAN_POINT('Ctrl Pts',(-18.9539020590981,37.0850707255635,122.295120923871)) ;
#38871=CARTESIAN_POINT('Ctrl Pts',(-18.8400831149199,36.9050816451537,122.015936356895)) ;
#38872=CARTESIAN_POINT('Ctrl Pts',(-19.2195445907984,37.098298875723,122.212649877143)) ;
#38873=CARTESIAN_POINT('Ctrl Pts',(-19.1721122727265,36.9183097953132,121.912858361349)) ;
#38874=CARTESIAN_POINT('Ctrl Pts',(-19.5728022237674,37.1149295528605,122.198387297674)) ;
#38875=CARTESIAN_POINT('Ctrl Pts',(-19.6137036972976,36.9349404724507,121.895030598784)) ;
#38876=CARTESIAN_POINT('Ctrl Pts',(-19.9761409789066,37.1348324921486,122.326670598827)) ;
#38877=CARTESIAN_POINT('Ctrl Pts',(-20.1178689308349,36.9548434117388,122.055389405925)) ;
#38878=CARTESIAN_POINT('Ctrl Pts',(-20.3116476022959,37.1547353587518,122.584460179412)) ;
#38879=CARTESIAN_POINT('Ctrl Pts',(-20.5372508618849,36.974746278342,122.377628584665)) ;
#38880=CARTESIAN_POINT('Ctrl Pts',(-20.539804233534,37.1746485238567,122.941249904607)) ;
#38881=CARTESIAN_POINT('Ctrl Pts',(-20.8224429653255,36.9946594434469,122.823616943163)) ;
#38882=CARTESIAN_POINT('Ctrl Pts',(-20.6323994014347,37.194684352998,123.35701958835)) ;
#38883=CARTESIAN_POINT('Ctrl Pts',(-20.9381837030193,37.0146952725882,123.343330198134)) ;
#38884=CARTESIAN_POINT('Ctrl Pts',(-20.5783831690263,37.2145029278761,123.775043446031)) ;
#38885=CARTESIAN_POINT('Ctrl Pts',(-20.8706604307742,37.0345138474663,123.86585779173)) ;
#38886=CARTESIAN_POINT('Ctrl Pts',(-20.3841900567002,37.2344732289181,124.152499639715)) ;
#38887=CARTESIAN_POINT('Ctrl Pts',(-20.6279168053661,37.0544841485082,124.337676429596)) ;
#38888=CARTESIAN_POINT('Ctrl Pts',(-20.0739514395831,37.2543647612826,124.440192864302)) ;
#38889=CARTESIAN_POINT('Ctrl Pts',(-20.2401177850966,37.0743756808728,124.6972903502)) ;
#38890=CARTESIAN_POINT('Ctrl Pts',(-19.6816910451499,37.2743878590991,124.605446609559)) ;
#38891=CARTESIAN_POINT('Ctrl Pts',(-19.7497910668665,37.0943987786893,124.903855399338)) ;
#38892=CARTESIAN_POINT('Ctrl Pts',(-19.2612575086077,37.2941846120191,124.626987367423)) ;
#38893=CARTESIAN_POINT('Ctrl Pts',(-19.2242516782376,37.1141955316092,124.930779156433)) ;
#38894=CARTESIAN_POINT('Ctrl Pts',(-18.8551235164096,37.3141457005079,124.503854762639)) ;
#38895=CARTESIAN_POINT('Ctrl Pts',(-18.7165851062423,37.134156620098,124.776862536651)) ;
#38896=CARTESIAN_POINT('Ctrl Pts',(-18.5155691321444,37.33412396944,124.248549659237)) ;
#38897=CARTESIAN_POINT('Ctrl Pts',(-18.2921431805253,37.1541348890302,124.457730120123)) ;
#38898=CARTESIAN_POINT('Ctrl Pts',(-18.2848840893229,37.353943984231,123.895912818502)) ;
#38899=CARTESIAN_POINT('Ctrl Pts',(-18.0037890981004,37.1739549038212,124.016935959748)) ;
#38900=CARTESIAN_POINT('Ctrl Pts',(-18.1867266757181,37.3738823934829,123.483465881593)) ;
#38901=CARTESIAN_POINT('Ctrl Pts',(-17.8810922819459,37.193893313073,123.501378325244)) ;
#38902=CARTESIAN_POINT('Ctrl Pts',(-18.2364290835758,37.3939295108753,123.060063699983)) ;
#38903=CARTESIAN_POINT('Ctrl Pts',(-17.9432206010294,37.2139404304655,122.972124751347)) ;
#38904=CARTESIAN_POINT('Ctrl Pts',(-18.425848548575,37.4137757567091,122.683031202947)) ;
#38905=CARTESIAN_POINT('Ctrl Pts',(-18.1799938361584,37.2337866762993,122.50083649183)) ;
#38906=CARTESIAN_POINT('Ctrl Pts',(-18.7315064002048,37.4336247252212,122.391977885503)) ;
#38907=CARTESIAN_POINT('Ctrl Pts',(-18.5620635940809,37.2536356448114,122.137020325859)) ;
#38908=CARTESIAN_POINT('Ctrl Pts',(-19.1222176535589,37.4536750275325,122.221508253603)) ;
#38909=CARTESIAN_POINT('Ctrl Pts',(-19.0504528465685,37.2736859471226,121.923931865061)) ;
#38910=CARTESIAN_POINT('Ctrl Pts',(-19.5432296563708,37.4735099499637,122.194969642124)) ;
#38911=CARTESIAN_POINT('Ctrl Pts',(-19.5767155011181,37.2935208695539,121.890757345923)) ;
#38912=CARTESIAN_POINT('Ctrl Pts',(-19.9499494548822,37.4934403511896,122.313396694246)) ;
#38913=CARTESIAN_POINT('Ctrl Pts',(-20.0851149441252,37.3134512707798,122.038788804376)) ;
#38914=CARTESIAN_POINT('Ctrl Pts',(-20.2916433860762,37.5133252965484,122.562694249305)) ;
#38915=CARTESIAN_POINT('Ctrl Pts',(-20.5122328950724,37.3333362161386,122.350407887825)) ;
#38916=CARTESIAN_POINT('Ctrl Pts',(-20.5292680047328,37.5333979046998,122.917125700607)) ;
#38917=CARTESIAN_POINT('Ctrl Pts',(-20.8092661803388,37.35340882429,122.793446550303)) ;
#38918=CARTESIAN_POINT('Ctrl Pts',(-20.6303478789093,37.5531892210279,123.325688691572)) ;
#38919=CARTESIAN_POINT('Ctrl Pts',(-20.9356180405514,37.3732001406181,123.304147384371)) ;
#38920=CARTESIAN_POINT('Ctrl Pts',(-20.5868633210281,37.5731540107952,123.747925395275)) ;
#38921=CARTESIAN_POINT('Ctrl Pts',(-20.8812658706994,37.3931649303854,123.831943312422)) ;
#38922=CARTESIAN_POINT('Ctrl Pts',(-20.400758322157,37.5931369665455,124.129898349839)) ;
#38923=CARTESIAN_POINT('Ctrl Pts',(-20.6486375256377,37.4131478861357,124.309410738595)) ;
#38924=CARTESIAN_POINT('Ctrl Pts',(-20.0987238949301,37.6129454885216,124.423499457933)) ;
#38925=CARTESIAN_POINT('Ctrl Pts',(-20.2710983170849,37.4329564081118,124.676413569075)) ;
#38926=CARTESIAN_POINT('Ctrl Pts',(-19.7115115108839,37.6329310632575,124.598340112043)) ;
#38927=CARTESIAN_POINT('Ctrl Pts',(-19.7870846026181,37.4529419828477,124.894968051446)) ;
#38928=CARTESIAN_POINT('Ctrl Pts',(-19.2898630183284,37.6528137033259,124.630311193854)) ;
#38929=CARTESIAN_POINT('Ctrl Pts',(-19.2600251516801,37.4728246229161,124.934935958252)) ;
#38930=CARTESIAN_POINT('Ctrl Pts',(-18.8812143689227,37.6727690154578,124.516434264361)) ;
#38931=CARTESIAN_POINT('Ctrl Pts',(-18.7492134555488,37.492779935048,124.792594096321)) ;
#38932=CARTESIAN_POINT('Ctrl Pts',(-18.5370718720123,37.6926433720656,124.271071448135)) ;
#38933=CARTESIAN_POINT('Ctrl Pts',(-18.3190332544941,37.5126542916557,124.485894779844)) ;
#38934=CARTESIAN_POINT('Ctrl Pts',(-18.295856749821,37.7126255789266,123.921365626854)) ;
#38935=CARTESIAN_POINT('Ctrl Pts',(-18.0175106059338,37.5326364985168,124.048765115421)) ;
#38936=CARTESIAN_POINT('Ctrl Pts',(-18.1889170459794,37.7325566568766,123.511199159604)) ;
#38937=CARTESIAN_POINT('Ctrl Pts',(-17.8838308617146,37.5525675764668,123.536059048155)) ;
#38938=CARTESIAN_POINT('Ctrl Pts',(-18.2282802535352,37.7524836317316,123.089417927906)) ;
#38939=CARTESIAN_POINT('Ctrl Pts',(-17.9330320753594,37.5724945513218,123.008830581994)) ;
#38940=CARTESIAN_POINT('Ctrl Pts',(-18.4076686429173,37.7723160906805,122.707716966432)) ;
#38941=CARTESIAN_POINT('Ctrl Pts',(-18.1572546227827,37.5923270102706,122.5317096236)) ;
#38942=CARTESIAN_POINT('Ctrl Pts',(-18.6583803627313,37.7889737748557,122.457695839393)) ;
#38943=CARTESIAN_POINT('Ctrl Pts',(-18.4706659457607,37.6089846944459,122.219158783992)) ;
#38944=CARTESIAN_POINT('Ctrl Pts',(-18.8998510224225,37.8022229987628,122.318670298478)) ;
#38945=CARTESIAN_POINT('Ctrl Pts',(-18.7724796761742,37.622233918353,122.045392670277)) ;
#38946=CARTESIAN_POINT('Ctrl Pts',(-19.0983967328829,37.812272020214,122.246576703272)) ;
#38947=CARTESIAN_POINT('Ctrl Pts',(-19.0206690088964,37.6322829398042,121.955269929657)) ;
#38948=CARTESIAN_POINT('Ctrl Pts',(-19.3025665370279,37.8221320284445,122.210682156202)) ;
#38949=CARTESIAN_POINT('Ctrl Pts',(-19.2758657648951,37.6421429480347,121.910397904095)) ;
#38950=CARTESIAN_POINT('Ctrl Pts',(-19.5818034711638,37.8354155416691,122.209888694931)) ;
#38951=CARTESIAN_POINT('Ctrl Pts',(-19.6249794284408,37.6554264612593,121.909413584205)) ;
#38952=CARTESIAN_POINT('Ctrl Pts',(-19.9238580353541,37.8520614606699,122.300927522182)) ;
#38953=CARTESIAN_POINT('Ctrl Pts',(-20.0524638778984,37.6720723802601,122.023188295544)) ;
#38954=CARTESIAN_POINT('Ctrl Pts',(-20.2129442647701,37.868615438486,122.501691868279)) ;
#38955=CARTESIAN_POINT('Ctrl Pts',(-20.4138807769964,37.6886263580762,122.274169668355)) ;
#38956=CARTESIAN_POINT('Ctrl Pts',(-20.3943636779236,37.8819751674576,122.716138212852)) ;
#38957=CARTESIAN_POINT('Ctrl Pts',(-20.6406243713775,37.7019860870478,122.542201540459)) ;
#38958=CARTESIAN_POINT('Ctrl Pts',(-20.4992200878676,37.8918682192543,122.895764414402)) ;
#38959=CARTESIAN_POINT('Ctrl Pts',(-20.7717039791491,37.7118791388445,122.766737576654)) ;
#38960=CARTESIAN_POINT('Ctrl Pts',(-20.5722587350757,37.9018581845353,123.092651468805)) ;
#38961=CARTESIAN_POINT('Ctrl Pts',(-20.863003128302,37.7218691041255,123.012844193448)) ;
#38962=CARTESIAN_POINT('Ctrl Pts',(-20.6099889776979,37.9118100653962,123.298474001835)) ;
#38963=CARTESIAN_POINT('Ctrl Pts',(-20.9101691765869,37.7318209849863,123.270122215442)) ;
#38964=CARTESIAN_POINT('Ctrl Pts',(-20.6112435236213,37.921858417088,123.509695858603)) ;
#38965=CARTESIAN_POINT('Ctrl Pts',(-20.9117400295887,37.7418693366781,123.534149528091)) ;
#38966=CARTESIAN_POINT('Ctrl Pts',(-20.5767689441837,37.9316997011942,123.713719442)) ;
#38967=CARTESIAN_POINT('Ctrl Pts',(-20.8686496158708,37.7517106207844,123.789179451351)) ;
#38968=CARTESIAN_POINT('Ctrl Pts',(-20.5068028273446,37.9416864043198,123.911631328625)) ;
#38969=CARTESIAN_POINT('Ctrl Pts',(-20.7811945959471,37.76169732391,124.036570320632)) ;
#38970=CARTESIAN_POINT('Ctrl Pts',(-20.4041443174755,37.9516214331373,124.093573751061)) ;
#38971=CARTESIAN_POINT('Ctrl Pts',(-20.6528738764456,37.7716323527274,124.263999794923)) ;
#38972=CARTESIAN_POINT('Ctrl Pts',(-20.2697516088806,37.9616772280442,124.256720400925)) ;
#38973=CARTESIAN_POINT('Ctrl Pts',(-20.4848851322736,37.7816881476343,124.467934944168)) ;
#38974=CARTESIAN_POINT('Ctrl Pts',(-20.112868940614,37.9715055913335,124.391230410189)) ;
#38975=CARTESIAN_POINT('Ctrl Pts',(-20.2887835293131,37.7915165109236,124.636074676851)) ;
#38976=CARTESIAN_POINT('Ctrl Pts',(-19.9310077930652,37.9815665612314,124.499176168369)) ;
#38977=CARTESIAN_POINT('Ctrl Pts',(-20.0614584856312,37.8015774808215,124.771009318102)) ;
#38978=CARTESIAN_POINT('Ctrl Pts',(-19.7359423603849,37.9914808401212,124.572672275179)) ;
#38979=CARTESIAN_POINT('Ctrl Pts',(-19.8176275658796,37.8114917597113,124.862882128351)) ;
#38980=CARTESIAN_POINT('Ctrl Pts',(-19.5292180654532,38.0014898345894,124.611953243679)) ;
#38981=CARTESIAN_POINT('Ctrl Pts',(-19.5592226441378,37.8215007541796,124.911986102297)) ;
#38982=CARTESIAN_POINT('Ctrl Pts',(-19.3183758075429,38.0115196691532,124.614317888065)) ;
#38983=CARTESIAN_POINT('Ctrl Pts',(-19.2956698137469,37.8315305887433,124.914944725323)) ;
#38984=CARTESIAN_POINT('Ctrl Pts',(-19.1138048120896,38.0213778992254,124.581009867866)) ;
#38985=CARTESIAN_POINT('Ctrl Pts',(-19.039955392314,37.8413888188156,124.873312424848)) ;
#38986=CARTESIAN_POINT('Ctrl Pts',(-18.9152985830758,38.0313766049678,124.51196923972)) ;
#38987=CARTESIAN_POINT('Ctrl Pts',(-18.7918216048149,37.851387524558,124.787014243673)) ;
#38988=CARTESIAN_POINT('Ctrl Pts',(-18.7335213440721,38.0412712608866,124.410757402581)) ;
#38989=CARTESIAN_POINT('Ctrl Pts',(-18.5645984860239,37.8612821804768,124.660501733437)) ;
#38990=CARTESIAN_POINT('Ctrl Pts',(-18.5694307222782,38.0513343252705,124.27728255479)) ;
#38991=CARTESIAN_POINT('Ctrl Pts',(-18.3594834847506,37.8713452448607,124.493660346737)) ;
#38992=CARTESIAN_POINT('Ctrl Pts',(-18.4338627813113,38.0611739835504,124.120992090027)) ;
#38993=CARTESIAN_POINT('Ctrl Pts',(-18.190021216124,37.8811849031406,124.298298757622)) ;
#38994=CARTESIAN_POINT('Ctrl Pts',(-18.3248772146404,38.0712371506323,123.939698712811)) ;
#38995=CARTESIAN_POINT('Ctrl Pts',(-18.0537869453048,37.8912480702225,124.071683477149)) ;
#38996=CARTESIAN_POINT('Ctrl Pts',(-18.2504447417178,38.0811313957594,123.745439174698)) ;
#38997=CARTESIAN_POINT('Ctrl Pts',(-17.960743677064,37.9011423153496,123.828859729591)) ;
#38998=CARTESIAN_POINT('Ctrl Pts',(-18.2101341066762,38.091073217364,123.54038139259)) ;
#38999=CARTESIAN_POINT('Ctrl Pts',(-17.9103527061802,37.9110841369542,123.572537760111)) ;
#39000=CARTESIAN_POINT('Ctrl Pts',(-18.2059368471232,38.1010757482821,123.330110491768)) ;
#39001=CARTESIAN_POINT('Ctrl Pts',(-17.9051034698684,37.9210866678723,123.309699103463)) ;
#39002=CARTESIAN_POINT('Ctrl Pts',(-18.238734440385,38.1111103747396,123.12172723179)) ;
#39003=CARTESIAN_POINT('Ctrl Pts',(-17.9460977833977,37.9311212943298,123.049219622121)) ;
#39004=CARTESIAN_POINT('Ctrl Pts',(-18.305619068495,38.120955909726,122.925840042337)) ;
#39005=CARTESIAN_POINT('Ctrl Pts',(-18.0297012300199,37.9409668293162,122.804359246447)) ;
#39006=CARTESIAN_POINT('Ctrl Pts',(-18.4064882596098,38.130939334565,122.74180463094)) ;
#39007=CARTESIAN_POINT('Ctrl Pts',(-18.155785528009,37.9509502541552,122.574313582094)) ;
#39008=CARTESIAN_POINT('Ctrl Pts',(-18.537392601509,38.1408897249301,122.578629160492)) ;
#39009=CARTESIAN_POINT('Ctrl Pts',(-18.3194140987467,37.9609006445203,122.370342409451)) ;
#39010=CARTESIAN_POINT('Ctrl Pts',(-18.6952097088462,38.1508873652272,122.439785210272)) ;
#39011=CARTESIAN_POINT('Ctrl Pts',(-18.5166838775073,37.9708982848174,122.196785487639)) ;
#39012=CARTESIAN_POINT('Ctrl Pts',(-18.8756765943063,38.1609264457904,122.330377777602)) ;
#39013=CARTESIAN_POINT('Ctrl Pts',(-18.7422660731798,37.9809373653805,122.060023983212)) ;
#39014=CARTESIAN_POINT('Ctrl Pts',(-19.0680799590173,38.1707525965595,122.255148656096)) ;
#39015=CARTESIAN_POINT('Ctrl Pts',(-18.9827700674424,37.9907635161496,121.965984935023)) ;
#39016=CARTESIAN_POINT('Ctrl Pts',(-19.2752831931946,38.1808091714886,122.213190167837)) ;
#39017=CARTESIAN_POINT('Ctrl Pts',(-19.2417735141218,38.0008200910788,121.913534414726)) ;
#39018=CARTESIAN_POINT('Ctrl Pts',(-19.4842136350837,38.1907497108689,122.208272468333)) ;
#39019=CARTESIAN_POINT('Ctrl Pts',(-19.5029368385438,38.010760630459,121.907384733484)) ;
#39020=CARTESIAN_POINT('Ctrl Pts',(-19.6901672000189,38.2006541038453,122.238947693484)) ;
#39021=CARTESIAN_POINT('Ctrl Pts',(-19.7603796759011,38.0206650234355,121.945726450794)) ;
#39022=CARTESIAN_POINT('Ctrl Pts',(-19.8904397603091,38.2107007580502,122.305985318567)) ;
#39023=CARTESIAN_POINT('Ctrl Pts',(-20.0107210558976,38.0307116776404,122.029521129551)) ;
#39024=CARTESIAN_POINT('Ctrl Pts',(-20.073374575685,38.2205963199886,122.405120062079)) ;
#39025=CARTESIAN_POINT('Ctrl Pts',(-20.2393912303879,38.0406072395788,122.153437721964)) ;
#39026=CARTESIAN_POINT('Ctrl Pts',(-20.239009195266,38.2306583978341,122.536650134801)) ;
#39027=CARTESIAN_POINT('Ctrl Pts',(-20.4464358605155,38.0506693174243,122.317848314832)) ;
#39028=CARTESIAN_POINT('Ctrl Pts',(-20.3763552173519,38.2405010962479,122.691451330782)) ;
#39029=CARTESIAN_POINT('Ctrl Pts',(-20.6181207396149,38.0605120158381,122.511348876355)) ;
#39030=CARTESIAN_POINT('Ctrl Pts',(-20.4867630860936,38.2504918712094,122.870097720652)) ;
#39031=CARTESIAN_POINT('Ctrl Pts',(-20.7561325944184,38.0705027907995,122.734655821547)) ;
#39032=CARTESIAN_POINT('Ctrl Pts',(-20.5639707241842,38.2604197362285,123.064019607399)) ;
#39033=CARTESIAN_POINT('Ctrl Pts',(-20.8526444302955,38.0804306558186,122.97705779297)) ;
#39034=CARTESIAN_POINT('Ctrl Pts',(-20.606936524891,38.2704084809947,123.269576207478)) ;
#39035=CARTESIAN_POINT('Ctrl Pts',(-20.9063538532472,38.0904194005849,123.234003272372)) ;
#39036=CARTESIAN_POINT('Ctrl Pts',(-20.6132774081827,38.2804412665816,123.480405040988)) ;
#39037=CARTESIAN_POINT('Ctrl Pts',(-20.9142822163388,38.1004521861718,123.497539173059)) ;
#39038=CARTESIAN_POINT('Ctrl Pts',(-20.5836278378137,38.2903079512023,123.685696146507)) ;
#39039=CARTESIAN_POINT('Ctrl Pts',(-20.8772223147978,38.1103188707925,123.754154223946)) ;
#39040=CARTESIAN_POINT('Ctrl Pts',(-20.5187275010846,38.3002698433654,123.884820325634)) ;
#39041=CARTESIAN_POINT('Ctrl Pts',(-20.796098729083,38.1202807629555,124.00306041156)) ;
#39042=CARTESIAN_POINT('Ctrl Pts',(-20.4192419119231,38.310303320278,124.070811287122)) ;
#39043=CARTESIAN_POINT('Ctrl Pts',(-20.6717436693402,38.1303142398682,124.235550043446)) ;
#39044=CARTESIAN_POINT('Ctrl Pts',(-20.2911476331738,38.3201876615263,124.234467456338)) ;
#39045=CARTESIAN_POINT('Ctrl Pts',(-20.5116269404507,38.1401985811165,124.440122137417)) ;
#39046=CARTESIAN_POINT('Ctrl Pts',(-20.1338310125617,38.3302506036474,124.375873737008)) ;
#39047=CARTESIAN_POINT('Ctrl Pts',(-20.314982722804,38.1502615232376,124.616881340086)) ;
#39048=CARTESIAN_POINT('Ctrl Pts',(-19.9581597878484,38.340101005267,124.485559805927)) ;
#39049=CARTESIAN_POINT('Ctrl Pts',(-20.0953938753125,38.1601119248572,124.75399118934)) ;
#39050=CARTESIAN_POINT('Ctrl Pts',(-19.7628910644464,38.3501278940566,124.564952690496)) ;
#39051=CARTESIAN_POINT('Ctrl Pts',(-19.8513087068657,38.1701388136468,124.853234002118)) ;
#39052=CARTESIAN_POINT('Ctrl Pts',(-19.5566368100917,38.3601565090128,124.608705273283)) ;
#39053=CARTESIAN_POINT('Ctrl Pts',(-19.5934913762966,38.180167428603,124.907926696721)) ;
#39054=CARTESIAN_POINT('Ctrl Pts',(-19.3498081641325,38.3700017321329,124.616238591243)) ;
#39055=CARTESIAN_POINT('Ctrl Pts',(-19.3349545228512,38.1900126517231,124.917345289644)) ;
#39056=CARTESIAN_POINT('Ctrl Pts',(-19.1416901454092,38.3799924159389,124.587880295423)) ;
#39057=CARTESIAN_POINT('Ctrl Pts',(-19.0748065717791,38.200003335529,124.881899109287)) ;
#39058=CARTESIAN_POINT('Ctrl Pts',(-18.9408634995236,38.3900302980113,124.52306847004)) ;
#39059=CARTESIAN_POINT('Ctrl Pts',(-18.8237728136587,38.2100412176015,124.800886156502)) ;
#39060=CARTESIAN_POINT('Ctrl Pts',(-18.7577593662331,38.3998746576501,124.426589014127)) ;
#39061=CARTESIAN_POINT('Ctrl Pts',(-18.5948907895903,38.2198855772403,124.680287851549)) ;
#39062=CARTESIAN_POINT('Ctrl Pts',(-18.5916294729954,38.4098595282649,124.298321906934)) ;
#39063=CARTESIAN_POINT('Ctrl Pts',(-18.3872272286313,38.2298704478551,124.519955106636)) ;
#39064=CARTESIAN_POINT('Ctrl Pts',(-18.4508291327248,38.4197988115935,124.14388654102)) ;
#39065=CARTESIAN_POINT('Ctrl Pts',(-18.2112252563258,38.2398097311837,124.326911572876)) ;
#39066=CARTESIAN_POINT('Ctrl Pts',(-18.3379263587694,38.4298394209667,123.965558708293)) ;
#39067=CARTESIAN_POINT('Ctrl Pts',(-18.0700954991663,38.2498503405568,124.104002776389)) ;
#39068=CARTESIAN_POINT('Ctrl Pts',(-18.2587866795904,38.4397242718799,123.77338134412)) ;
#39069=CARTESIAN_POINT('Ctrl Pts',(-17.9711690913836,38.2597351914701,123.863780801311)) ;
#39070=CARTESIAN_POINT('Ctrl Pts',(-18.2134543934735,38.4497262280487,123.568085773831)) ;
#39071=CARTESIAN_POINT('Ctrl Pts',(-17.9145022539085,38.2697371476389,123.607161518805)) ;
#39072=CARTESIAN_POINT('Ctrl Pts',(-18.2043619080485,38.4596448247692,123.359731016795)) ;
#39073=CARTESIAN_POINT('Ctrl Pts',(-17.9031351939058,38.2796557443593,123.346717419447)) ;
#39074=CARTESIAN_POINT('Ctrl Pts',(-18.2319694185159,38.469691646845,123.150356999405)) ;
#39075=CARTESIAN_POINT('Ctrl Pts',(-17.9376431227028,38.2897025664352,123.084999919359)) ;
#39076=CARTESIAN_POINT('Ctrl Pts',(-18.2942537247054,38.4795659279577,122.952295745254)) ;
#39077=CARTESIAN_POINT('Ctrl Pts',(-18.0154975115809,38.2995768475479,122.837421943635)) ;
#39078=CARTESIAN_POINT('Ctrl Pts',(-18.3915795652772,38.4896201280023,122.764705800279)) ;
#39079=CARTESIAN_POINT('Ctrl Pts',(-18.137153510748,38.3096310475925,122.6029341291)) ;
#39080=CARTESIAN_POINT('Ctrl Pts',(-18.517948341089,38.4995155576375,122.599403244728)) ;
#39081=CARTESIAN_POINT('Ctrl Pts',(-18.295114007529,38.3195264772277,122.396304412865)) ;
#39082=CARTESIAN_POINT('Ctrl Pts',(-18.6735897291934,38.5095771859549,122.456195028724)) ;
#39083=CARTESIAN_POINT('Ctrl Pts',(-18.489664633959,38.329588105545,122.217293421635)) ;
#39084=CARTESIAN_POINT('Ctrl Pts',(-18.8479034008404,38.5194218147848,122.344605396143)) ;
#39085=CARTESIAN_POINT('Ctrl Pts',(-18.7075571482526,38.3394327343749,122.077804596449)) ;
#39086=CARTESIAN_POINT('Ctrl Pts',(-19.0408840506454,38.5293818623904,122.263352848004)) ;
#39087=CARTESIAN_POINT('Ctrl Pts',(-18.9487829946341,38.3493927819806,121.976237815582)) ;
#39088=CARTESIAN_POINT('Ctrl Pts',(-19.2467307026046,38.5394201685644,122.216882947286)) ;
#39089=CARTESIAN_POINT('Ctrl Pts',(-19.2060908983503,38.3594310881546,121.918149353358)) ;
#39090=CARTESIAN_POINT('Ctrl Pts',(-19.4540764654965,38.5492934679971,122.206624033393)) ;
#39091=CARTESIAN_POINT('Ctrl Pts',(-19.4652741750453,38.3693043875873,121.905324657116)) ;
#39092=CARTESIAN_POINT('Ctrl Pts',(-19.6641424754752,38.5593667295834,122.233106532609)) ;
#39093=CARTESIAN_POINT('Ctrl Pts',(-19.727856392787,38.3793776491735,121.938426707884)) ;
#39094=CARTESIAN_POINT('Ctrl Pts',(-19.8615036156616,38.5691869555401,122.293853612687)) ;
#39095=CARTESIAN_POINT('Ctrl Pts',(-19.9745595743233,38.3891978751303,122.014360134758)) ;
#39096=CARTESIAN_POINT('Ctrl Pts',(-20.0501587943975,38.5792660194796,122.390213788691)) ;
#39097=CARTESIAN_POINT('Ctrl Pts',(-20.2103785147043,38.3992769390698,122.13480937885)) ;
#39098=CARTESIAN_POINT('Ctrl Pts',(-20.2155221291384,38.5891161094994,122.514954133078)) ;
#39099=CARTESIAN_POINT('Ctrl Pts',(-20.4170842341613,38.4091270290896,122.290734959932)) ;
#39100=CARTESIAN_POINT('Ctrl Pts',(-20.3599977542973,38.5991948631132,122.669874910187)) ;
#39101=CARTESIAN_POINT('Ctrl Pts',(-20.5976790050337,38.4192057827034,122.484385049219)) ;
#39102=CARTESIAN_POINT('Ctrl Pts',(-20.4726208048676,38.6090163303726,122.842988026387)) ;
#39103=CARTESIAN_POINT('Ctrl Pts',(-20.7384592822056,38.4290272499628,122.700777392745)) ;
#39104=CARTESIAN_POINT('Ctrl Pts',(-20.5557471903728,38.6190819287303,123.037535696826)) ;
#39105=CARTESIAN_POINT('Ctrl Pts',(-20.8423676550526,38.4390928483204,122.943961403753)) ;
#39106=CARTESIAN_POINT('Ctrl Pts',(-20.6030203243983,38.628984584505,123.240335099083)) ;
#39107=CARTESIAN_POINT('Ctrl Pts',(-20.9014598752685,38.4489955040952,123.197461404654)) ;
#39108=CARTESIAN_POINT('Ctrl Pts',(-20.6145926696744,38.6390354103346,123.451275235179)) ;
#39109=CARTESIAN_POINT('Ctrl Pts',(-20.9159258762497,38.4590463299248,123.461136272489)) ;
#39110=CARTESIAN_POINT('Ctrl Pts',(-20.5899961792857,38.6489096146735,123.657445196275)) ;
#39111=CARTESIAN_POINT('Ctrl Pts',(-20.8851806309727,38.4689205342637,123.718849938171)) ;
#39112=CARTESIAN_POINT('Ctrl Pts',(-20.5288093864204,38.6589820647126,123.860120703039)) ;
#39113=CARTESIAN_POINT('Ctrl Pts',(-20.808697747112,38.4789929843028,123.972194060063)) ;
#39114=CARTESIAN_POINT('Ctrl Pts',(-20.4358076287803,38.6688110814861,124.044689523101)) ;
#39115=CARTESIAN_POINT('Ctrl Pts',(-20.6924452330698,38.4888220010763,124.202906653786)) ;
#39116=CARTESIAN_POINT('Ctrl Pts',(-20.3094581014981,38.6788779274009,124.214427563999)) ;
#39117=CARTESIAN_POINT('Ctrl Pts',(-20.5345088117852,38.4988888469911,124.415079071693)) ;
#39118=CARTESIAN_POINT('Ctrl Pts',(-20.1581204946843,38.6887680987027,124.357044093307)) ;
#39119=CARTESIAN_POINT('Ctrl Pts',(-20.3453362910771,38.5087790182928,124.593350718239)) ;
#39120=CARTESIAN_POINT('Ctrl Pts',(-19.9828118483022,38.6987602923265,124.472759650499)) ;
#39121=CARTESIAN_POINT('Ctrl Pts',(-20.1262004053529,38.5187712119167,124.737995435584)) ;
#39122=CARTESIAN_POINT('Ctrl Pts',(-19.7905552310231,38.7087231029499,124.555852659848)) ;
#39123=CARTESIAN_POINT('Ctrl Pts',(-19.8858793197605,38.5287340225401,124.841862120284)) ;
#39124=CARTESIAN_POINT('Ctrl Pts',(-19.5880898351678,38.7186273757934,124.604536143381)) ;
#39125=CARTESIAN_POINT('Ctrl Pts',(-19.6327966736639,38.5386382953835,124.902716744678)) ;
#39126=CARTESIAN_POINT('Ctrl Pts',(-19.3770005006573,38.728687867598,124.617340881454)) ;
#39127=CARTESIAN_POINT('Ctrl Pts',(-19.3689353661854,38.5486987871882,124.918722771534)) ;
#39128=CARTESIAN_POINT('Ctrl Pts',(-19.1714080286777,38.7385281992703,124.594087546926)) ;
#39129=CARTESIAN_POINT('Ctrl Pts',(-19.111943312049,38.5585391188605,124.889655955277)) ;
#39130=CARTESIAN_POINT('Ctrl Pts',(-18.9684668170041,38.7485912453621,124.53442387862)) ;
#39131=CARTESIAN_POINT('Ctrl Pts',(-18.8582671795693,38.5686021649523,124.81507639537)) ;
#39132=CARTESIAN_POINT('Ctrl Pts',(-18.7821841412429,38.7584853010572,124.441832669131)) ;
#39133=CARTESIAN_POINT('Ctrl Pts',(-18.6254129262144,38.5784962206474,124.699336919399)) ;
#39134=CARTESIAN_POINT('Ctrl Pts',(-18.613681541493,38.7684280013801,124.318182967995)) ;
#39135=CARTESIAN_POINT('Ctrl Pts',(-18.4147842987737,38.5884389209703,124.544774213957)) ;
#39136=CARTESIAN_POINT('Ctrl Pts',(-18.4682304496749,38.7784337423077,124.166191909922)) ;
#39137=CARTESIAN_POINT('Ctrl Pts',(-18.2329705622682,38.5984446618979,124.354785151185)) ;
#39138=CARTESIAN_POINT('Ctrl Pts',(-18.3514150571057,38.7884546528233,123.990879578772)) ;
#39139=CARTESIAN_POINT('Ctrl Pts',(-18.086951476035,38.6084655724134,124.135644682237)) ;
#39140=CARTESIAN_POINT('Ctrl Pts',(-18.2676887679517,38.7983453882732,123.800540045983)) ;
#39141=CARTESIAN_POINT('Ctrl Pts',(-17.9822934308171,38.6183563078634,123.89771920694)) ;
#39142=CARTESIAN_POINT('Ctrl Pts',(-18.2174815072807,38.8083369290021,123.596583556656)) ;
#39143=CARTESIAN_POINT('Ctrl Pts',(-17.919534669745,38.6283478485923,123.642773296605)) ;
#39144=CARTESIAN_POINT('Ctrl Pts',(-18.2035708832846,38.8182847894237,123.387913191954)) ;
#39145=CARTESIAN_POINT('Ctrl Pts',(-17.9021467019561,38.6382957090139,123.381934725882)) ;
#39146=CARTESIAN_POINT('Ctrl Pts',(-18.2256918881132,38.8282314586101,123.17996466364)) ;
#39147=CARTESIAN_POINT('Ctrl Pts',(-17.9297985345698,38.6482423782002,123.121998548206)) ;
#39148=CARTESIAN_POINT('Ctrl Pts',(-18.2843906460259,38.8382795347457,122.977049468211)) ;
#39149=CARTESIAN_POINT('Ctrl Pts',(-18.0031723205418,38.6582904543359,122.868354913006)) ;
#39150=CARTESIAN_POINT('Ctrl Pts',(-18.3754224094433,38.8481271327513,122.79110855479)) ;
#39151=CARTESIAN_POINT('Ctrl Pts',(-18.1169630845175,38.6681380523415,122.635927730697)) ;
#39152=CARTESIAN_POINT('Ctrl Pts',(-18.4982316363328,38.8580888558358,122.621481919964)) ;
#39153=CARTESIAN_POINT('Ctrl Pts',(-18.2704754939208,38.6780997754259,122.423894509183)) ;
#39154=CARTESIAN_POINT('Ctrl Pts',(-18.6498412742199,38.8681174909188,122.474952850286)) ;
#39155=CARTESIAN_POINT('Ctrl Pts',(-18.4599879202385,38.6881284105089,122.240733703657)) ;
#39156=CARTESIAN_POINT('Ctrl Pts',(-18.822471332867,38.8780277992368,122.358322296909)) ;
#39157=CARTESIAN_POINT('Ctrl Pts',(-18.6757765964576,38.698038718827,122.094945578036)) ;
#39158=CARTESIAN_POINT('Ctrl Pts',(-19.0129931752722,38.8879626963727,122.272721130062)) ;
#39159=CARTESIAN_POINT('Ctrl Pts',(-18.9139298646376,38.7079736159628,121.987944654612)) ;
#39160=CARTESIAN_POINT('Ctrl Pts',(-19.2176845439249,38.8980037793153,122.221146163374)) ;
#39161=CARTESIAN_POINT('Ctrl Pts',(-19.1697940908781,38.7180146989054,121.923476774972)) ;
#39162=CARTESIAN_POINT('Ctrl Pts',(-19.4250041735291,38.9078911221435,122.205985759555)) ;
#39163=CARTESIAN_POINT('Ctrl Pts',(-19.4289447281895,38.7279020417337,121.904527054384)) ;
#39164=CARTESIAN_POINT('Ctrl Pts',(-19.6340005528841,38.9178826370828,122.22691350164)) ;
#39165=CARTESIAN_POINT('Ctrl Pts',(-19.6901903067316,38.737893556673,121.930687744882)) ;
#39166=CARTESIAN_POINT('Ctrl Pts',(-19.8353682152375,38.9278340282793,122.283672510292)) ;
#39167=CARTESIAN_POINT('Ctrl Pts',(-19.9419001392647,38.7478449478695,122.001637581094)) ;
#39168=CARTESIAN_POINT('Ctrl Pts',(-20.0236163341247,38.9377665616119,122.374032890848)) ;
#39169=CARTESIAN_POINT('Ctrl Pts',(-20.1772104092454,38.7577774812021,122.114589337073)) ;
#39170=CARTESIAN_POINT('Ctrl Pts',(-20.1944626039504,38.9477637195114,122.496427038679)) ;
#39171=CARTESIAN_POINT('Ctrl Pts',(-20.3907677133097,38.7677746391016,122.267583026832)) ;
#39172=CARTESIAN_POINT('Ctrl Pts',(-20.3413685794426,38.9577487296749,122.646417878081)) ;
#39173=CARTESIAN_POINT('Ctrl Pts',(-20.5743995161531,38.7777596492651,122.455072551168)) ;
#39174=CARTESIAN_POINT('Ctrl Pts',(-20.46039600103,38.9677915562447,122.820765432393)) ;
#39175=CARTESIAN_POINT('Ctrl Pts',(-20.723182830776,38.7878024758349,122.673007430782)) ;
#39176=CARTESIAN_POINT('Ctrl Pts',(-20.5459597437265,38.9776217905496,123.00891851305)) ;
#39177=CARTESIAN_POINT('Ctrl Pts',(-20.830136998743,38.7976327101398,122.908200598541)) ;
#39178=CARTESIAN_POINT('Ctrl Pts',(-20.5989170245634,38.9876978157843,123.213977187539)) ;
#39179=CARTESIAN_POINT('Ctrl Pts',(-20.8963322765034,38.8077087353745,123.164523836738)) ;
#39180=CARTESIAN_POINT('Ctrl Pts',(-20.6152120888322,38.9975500522752,123.42050479598)) ;
#39181=CARTESIAN_POINT('Ctrl Pts',(-20.9166999185625,38.8175609718654,123.422684680524)) ;
#39182=CARTESIAN_POINT('Ctrl Pts',(-20.5951407332866,39.0076232587093,123.631287792169)) ;
#39183=CARTESIAN_POINT('Ctrl Pts',(-20.8916094133679,38.8276341782995,123.686162896896)) ;
#39184=CARTESIAN_POINT('Ctrl Pts',(-20.5400039210857,39.0174647682165,123.830719200316)) ;
#39185=CARTESIAN_POINT('Ctrl Pts',(-20.8226867660567,38.8374756878066,123.935453060499)) ;
#39186=CARTESIAN_POINT('Ctrl Pts',(-20.4507189099979,39.0274257149963,124.020134101284)) ;
#39187=CARTESIAN_POINT('Ctrl Pts',(-20.711078874203,38.8474366345865,124.172221368171)) ;
#39188=CARTESIAN_POINT('Ctrl Pts',(-20.3286238637453,39.0374635437963,124.192245807622)) ;
#39189=CARTESIAN_POINT('Ctrl Pts',(-20.558458951946,38.8574744633865,124.387360046593)) ;
#39190=CARTESIAN_POINT('Ctrl Pts',(-20.1811938017144,39.0473378535508,124.338423480837)) ;
#39191=CARTESIAN_POINT('Ctrl Pts',(-20.3741695323941,38.867348773141,124.570081721037)) ;
#39192=CARTESIAN_POINT('Ctrl Pts',(-20.0072836350948,39.0574075512239,124.45908427213)) ;
#39193=CARTESIAN_POINT('Ctrl Pts',(-20.1567812055982,38.8774184708141,124.720906204258)) ;
#39194=CARTESIAN_POINT('Ctrl Pts',(-19.8195805182457,39.0672410225113,124.545752922959)) ;
#39195=CARTESIAN_POINT('Ctrl Pts',(-19.9221504639086,38.8872519421015,124.829241080154)) ;
#39196=CARTESIAN_POINT('Ctrl Pts',(-19.6158666766055,39.0772706690413,124.600148476529)) ;
#39197=CARTESIAN_POINT('Ctrl Pts',(-19.6675077755465,38.8972815886314,124.897233739446)) ;
#39198=CARTESIAN_POINT('Ctrl Pts',(-19.4056375158977,39.0873051833686,124.617714671404)) ;
#39199=CARTESIAN_POINT('Ctrl Pts',(-19.4047212779263,38.9073161029588,124.919189866016)) ;
#39200=CARTESIAN_POINT('Ctrl Pts',(-19.1998910206002,39.0971304688395,124.599407552797)) ;
#39201=CARTESIAN_POINT('Ctrl Pts',(-19.1475370274875,38.9171413884297,124.896304082201)) ;
#39202=CARTESIAN_POINT('Ctrl Pts',(-18.9967244321837,39.1071347103881,124.545112550832)) ;
#39203=CARTESIAN_POINT('Ctrl Pts',(-18.8935792031273,38.9271456299783,124.828433457383)) ;
#39204=CARTESIAN_POINT('Ctrl Pts',(-18.8064617759764,39.1171173554672,124.456450033526)) ;
#39205=CARTESIAN_POINT('Ctrl Pts',(-18.6557514840538,38.9371282750574,124.717603510454)) ;
#39206=CARTESIAN_POINT('Ctrl Pts',(-18.6335954547731,39.1271625525587,124.335184104469)) ;
#39207=CARTESIAN_POINT('Ctrl Pts',(-18.4396697499404,38.9471734721488,124.566019705059)) ;
#39208=CARTESIAN_POINT('Ctrl Pts',(-18.4874417294713,39.1369856683188,124.189274410091)) ;
#39209=CARTESIAN_POINT('Ctrl Pts',(-18.2569780632048,38.956996587909,124.383630345481)) ;
#39210=CARTESIAN_POINT('Ctrl Pts',(-18.3658597551784,39.1470202801191,124.016878296206)) ;
#39211=CARTESIAN_POINT('Ctrl Pts',(-18.105002354756,38.9670311997093,124.16813409238)) ;
#39212=CARTESIAN_POINT('Ctrl Pts',(-18.2766733676231,39.1570452888922,123.825914539901)) ;
#39213=CARTESIAN_POINT('Ctrl Pts',(-17.9935211047734,38.9770562084824,123.929428614869)) ;
#39214=CARTESIAN_POINT('Ctrl Pts',(-18.2225068331294,39.1668972137338,123.626000802301)) ;
#39215=CARTESIAN_POINT('Ctrl Pts',(-17.9258146374258,38.986908133324,123.679534933415)) ;
#39216=CARTESIAN_POINT('Ctrl Pts',(-18.2032934378515,39.1768881520565,123.416865948046)) ;
#39217=CARTESIAN_POINT('Ctrl Pts',(-17.9017999975466,38.9968990716467,123.418116000194)) ;
#39218=CARTESIAN_POINT('Ctrl Pts',(-18.2204270850265,39.186806137203,123.209038883101)) ;
#39219=CARTESIAN_POINT('Ctrl Pts',(-17.9232192571751,39.0068170567931,123.158331775169)) ;
#39220=CARTESIAN_POINT('Ctrl Pts',(-18.2739141189626,39.1968342380985,123.005131243804)) ;
#39221=CARTESIAN_POINT('Ctrl Pts',(-17.9900801458931,39.0168451576887,122.903447812463)) ;
#39222=CARTESIAN_POINT('Ctrl Pts',(-18.3606686893931,39.2067194790411,122.816282003128)) ;
#39223=CARTESIAN_POINT('Ctrl Pts',(-18.0985256645182,39.0267303986312,122.667386508151)) ;
#39224=CARTESIAN_POINT('Ctrl Pts',(-18.4797149154803,39.2167085920077,122.643274137874)) ;
#39225=CARTESIAN_POINT('Ctrl Pts',(-18.2473354546327,39.0367195115979,122.451127866557)) ;
#39226=CARTESIAN_POINT('Ctrl Pts',(-18.6280950699641,39.2267506563485,122.493104045599)) ;
#39227=CARTESIAN_POINT('Ctrl Pts',(-18.4328121554454,39.0467615759387,122.263416874348)) ;
#39228=CARTESIAN_POINT('Ctrl Pts',(-18.7964289728388,39.236579857753,122.37324034441)) ;
#39229=CARTESIAN_POINT('Ctrl Pts',(-18.6432316642318,39.0565907773432,122.1135885661)) ;
#39230=CARTESIAN_POINT('Ctrl Pts',(-18.9861633069281,39.2465866985112,122.282419196658)) ;
#39231=CARTESIAN_POINT('Ctrl Pts',(-18.8804006959782,39.0665976181013,122.000064282173)) ;
#39232=CARTESIAN_POINT('Ctrl Pts',(-19.1884846108807,39.2565742227031,122.226135721448)) ;
#39233=CARTESIAN_POINT('Ctrl Pts',(-19.1333031196134,39.0765851422933,121.929712194774)) ;
#39234=CARTESIAN_POINT('Ctrl Pts',(-19.3983474426324,39.2666038685117,122.205902107928)) ;
#39235=CARTESIAN_POINT('Ctrl Pts',(-19.3956318554849,39.0866147881019,121.904422523762)) ;
#39236=CARTESIAN_POINT('Ctrl Pts',(-19.6053336272935,39.2764778992504,122.221912828081)) ;
#39237=CARTESIAN_POINT('Ctrl Pts',(-19.6543650766662,39.0964888188406,121.924438378647)) ;
#39238=CARTESIAN_POINT('Ctrl Pts',(-19.8089581741731,39.2864772221145,122.274010548513)) ;
#39239=CARTESIAN_POINT('Ctrl Pts',(-19.908895255935,39.1064881417047,121.989562946807)) ;
#39240=CARTESIAN_POINT('Ctrl Pts',(-19.9988971817539,39.2963880576901,122.359747483072)) ;
#39241=CARTESIAN_POINT('Ctrl Pts',(-20.1463184204501,39.1163989772803,122.096736593736)) ;
#39242=CARTESIAN_POINT('Ctrl Pts',(-20.173454632489,39.3064423056642,122.478884560245)) ;
#39243=CARTESIAN_POINT('Ctrl Pts',(-20.3645137351281,39.1264532252543,122.245659936817)) ;
#39244=CARTESIAN_POINT('Ctrl Pts',(-20.321953767156,39.3163010499269,122.623523272663)) ;
#39245=CARTESIAN_POINT('Ctrl Pts',(-20.5501363523846,39.136311969517,122.426460600521)) ;
#39246=CARTESIAN_POINT('Ctrl Pts',(-20.4457184725392,39.3263691359999,122.79519306141)) ;
#39247=CARTESIAN_POINT('Ctrl Pts',(-20.7048400637397,39.1463800555901,122.641049209718)) ;
#39248=CARTESIAN_POINT('Ctrl Pts',(-20.5358574260446,39.3362246191794,122.981770543194)) ;
#39249=CARTESIAN_POINT('Ctrl Pts',(-20.8175117264018,39.1562355387696,122.874272740712)) ;
#39250=CARTESIAN_POINT('Ctrl Pts',(-20.593627567202,39.3462194649736,123.183789054105)) ;
#39251=CARTESIAN_POINT('Ctrl Pts',(-20.8897218677833,39.1662303845638,123.126796707749)) ;
#39252=CARTESIAN_POINT('Ctrl Pts',(-20.6150717947813,39.3562507606361,123.393589597854)) ;
#39253=CARTESIAN_POINT('Ctrl Pts',(-20.9165245763785,39.1762616802263,123.38904765132)) ;
#39254=CARTESIAN_POINT('Ctrl Pts',(-20.6003432400617,39.366117303926,123.600498782211)) ;
#39255=CARTESIAN_POINT('Ctrl Pts',(-20.8981112103202,39.1861282235162,123.647684462336)) ;
#39256=CARTESIAN_POINT('Ctrl Pts',(-20.5496307755805,39.3761046996894,123.804223422372)) ;
#39257=CARTESIAN_POINT('Ctrl Pts',(-20.8347179860478,39.1961156192796,123.902339731303)) ;
#39258=CARTESIAN_POINT('Ctrl Pts',(-20.4647567854182,39.3860497404194,123.995331104397)) ;
#39259=CARTESIAN_POINT('Ctrl Pts',(-20.7286229324539,39.2060606600095,124.141223452018)) ;
#39260=CARTESIAN_POINT('Ctrl Pts',(-20.3467526330684,39.3960942466361,124.170424565575)) ;
#39261=CARTESIAN_POINT('Ctrl Pts',(-20.5811155220778,39.2161051662263,124.360088757651)) ;
#39262=CARTESIAN_POINT('Ctrl Pts',(-20.2028876578197,39.4059577527734,124.31979097255)) ;
#39263=CARTESIAN_POINT('Ctrl Pts',(-20.4012820502174,39.2259686723636,124.546795194505)) ;
#39264=CARTESIAN_POINT('Ctrl Pts',(-20.0333359133557,39.4159506136095,124.443780975724)) ;
#39265=CARTESIAN_POINT('Ctrl Pts',(-20.1893406640015,39.2359615331996,124.701780528512)) ;
#39266=CARTESIAN_POINT('Ctrl Pts',(-19.8460776642137,39.4258768073284,124.535944097192)) ;
#39267=CARTESIAN_POINT('Ctrl Pts',(-19.9552664329301,39.2458877269186,124.81698205313)) ;
#39268=CARTESIAN_POINT('Ctrl Pts',(-19.6438526109254,39.435895733361,124.594760442334)) ;
#39269=CARTESIAN_POINT('Ctrl Pts',(-19.7024842949492,39.2559066529511,124.890499840272)) ;
#39270=CARTESIAN_POINT('Ctrl Pts',(-19.4366243471817,39.4458107327286,124.617535468965)) ;
#39271=CARTESIAN_POINT('Ctrl Pts',(-19.4434484431306,39.2658216523187,124.918965884145)) ;
#39272=CARTESIAN_POINT('Ctrl Pts',(-19.2257177733582,39.4558655042859,124.603751642872)) ;
#39273=CARTESIAN_POINT('Ctrl Pts',(-19.1798154010416,39.275876423876,124.901733325826)) ;
#39274=CARTESIAN_POINT('Ctrl Pts',(-19.024324659477,39.4657244665834,124.554651862093)) ;
#39275=CARTESIAN_POINT('Ctrl Pts',(-18.9280744033363,39.2857353861736,124.840355827258)) ;
#39276=CARTESIAN_POINT('Ctrl Pts',(-18.8318078658274,39.4757187104213,124.47057126686)) ;
#39277=CARTESIAN_POINT('Ctrl Pts',(-18.6874294683432,39.2957296300115,124.73525247238)) ;
#39278=CARTESIAN_POINT('Ctrl Pts',(-18.6579134178425,39.4856439398455,124.355188357993)) ;
#39279=CARTESIAN_POINT('Ctrl Pts',(-18.4700628512776,39.3056548594357,124.591021419494)) ;
#39280=CARTESIAN_POINT('Ctrl Pts',(-18.505167355136,39.495671903737,124.209924117878)) ;
#39281=CARTESIAN_POINT('Ctrl Pts',(-18.2791321697384,39.3156828233272,124.409439034556)) ;
#39282=CARTESIAN_POINT('Ctrl Pts',(-18.3815260589152,39.5055581633674,124.042821017598)) ;
#39283=CARTESIAN_POINT('Ctrl Pts',(-18.1245827426847,39.3255690829575,124.200558385434)) ;
#39284=CARTESIAN_POINT('Ctrl Pts',(-18.2873441788241,39.5155899264452,123.854158630485)) ;
#39285=CARTESIAN_POINT('Ctrl Pts',(-18.0068578912932,39.3356008460354,123.96472907927)) ;
#39286=CARTESIAN_POINT('Ctrl Pts',(-18.2280346546859,39.5254715527393,123.655023225739)) ;
#39287=CARTESIAN_POINT('Ctrl Pts',(-17.9327236697007,39.3454824723295,123.715808953647)) ;
#39288=CARTESIAN_POINT('Ctrl Pts',(-18.2037205041182,39.5355333222255,123.444926394971)) ;
#39289=CARTESIAN_POINT('Ctrl Pts',(-17.9023337792081,39.3555442418157,123.453187507277)) ;
#39290=CARTESIAN_POINT('Ctrl Pts',(-18.2159436021786,39.545391189721,123.238018443075)) ;
#39291=CARTESIAN_POINT('Ctrl Pts',(-17.9176154684793,39.3654021093111,123.194552719104)) ;
#39292=CARTESIAN_POINT('Ctrl Pts',(-18.2640935145991,39.5553828148383,123.033581530344)) ;
#39293=CARTESIAN_POINT('Ctrl Pts',(-17.977805608363,39.3753937344285,122.939007178542)) ;
#39294=CARTESIAN_POINT('Ctrl Pts',(-18.346604236998,39.5653196139466,122.841649932194)) ;
#39295=CARTESIAN_POINT('Ctrl Pts',(-18.080946592247,39.3853305335367,122.699093789384)) ;
#39296=CARTESIAN_POINT('Ctrl Pts',(-18.4615503978526,39.5753104435039,122.665852839243)) ;
#39297=CARTESIAN_POINT('Ctrl Pts',(-18.2246316582035,39.3953213630941,122.479348914354)) ;
#39298=CARTESIAN_POINT('Ctrl Pts',(-18.6059214023956,39.5853336792171,122.512353088395)) ;
#39299=CARTESIAN_POINT('Ctrl Pts',(-18.4050975253552,39.4053445988073,122.287476075937)) ;
#39300=CARTESIAN_POINT('Ctrl Pts',(-18.7725024087154,39.5952300272463,122.38771377753)) ;
#39301=CARTESIAN_POINT('Ctrl Pts',(-18.6133254066548,39.4152409468365,122.131679228694)) ;
#39302=CARTESIAN_POINT('Ctrl Pts',(-18.9597546314449,39.6052195897488,122.292601295741)) ;
#39303=CARTESIAN_POINT('Ctrl Pts',(-18.847391914281,39.4252305093389,122.012791074243)) ;
#39304=CARTESIAN_POINT('Ctrl Pts',(-19.1618012116734,39.6152598974333,122.231549580434)) ;
#39305=CARTESIAN_POINT('Ctrl Pts',(-19.0999512728401,39.4352708170235,121.936479082137)) ;
#39306=CARTESIAN_POINT('Ctrl Pts',(-19.367227076232,39.6251022007805,122.206604242828)) ;
#39307=CARTESIAN_POINT('Ctrl Pts',(-19.3567329848068,39.4451131203707,121.905300141078)) ;
#39308=CARTESIAN_POINT('Ctrl Pts',(-19.5776342598679,39.6351259090596,122.217627035733)) ;
#39309=CARTESIAN_POINT('Ctrl Pts',(-19.6197445019945,39.4551368286498,121.919081532406)) ;
#39310=CARTESIAN_POINT('Ctrl Pts',(-19.8485635991152,39.6483480865273,122.280050363964)) ;
#39311=CARTESIAN_POINT('Ctrl Pts',(-19.9583923044569,39.4683590061174,121.997113385138)) ;
#39312=CARTESIAN_POINT('Ctrl Pts',(-20.0983757230061,39.6616406715866,122.4121455033)) ;
#39313=CARTESIAN_POINT('Ctrl Pts',(-20.2706261181755,39.4816515911767,122.162206025438)) ;
#39314=CARTESIAN_POINT('Ctrl Pts',(-20.3030677190675,39.6749255275082,122.602175666116)) ;
#39315=CARTESIAN_POINT('Ctrl Pts',(-20.5265366200898,39.4949364470983,122.399782063026)) ;
#39316=CARTESIAN_POINT('Ctrl Pts',(-20.4297258307919,39.684897754681,122.76921101663)) ;
#39317=CARTESIAN_POINT('Ctrl Pts',(-20.6848475062814,39.5049086742711,122.608570519068)) ;
#39318=CARTESIAN_POINT('Ctrl Pts',(-20.5251856164806,39.69480637112,122.95438797765)) ;
#39319=CARTESIAN_POINT('Ctrl Pts',(-20.8041722375958,39.5148172907101,122.8400449268)) ;
#39320=CARTESIAN_POINT('Ctrl Pts',(-20.587851626912,39.7048595765037,123.156213626947)) ;
#39321=CARTESIAN_POINT('Ctrl Pts',(-20.8825021975675,39.5248704960938,123.092326029343)) ;
#39322=CARTESIAN_POINT('Ctrl Pts',(-20.6141617899061,39.714724710264,123.361949025928)) ;
#39323=CARTESIAN_POINT('Ctrl Pts',(-20.9153854641388,39.5347356298541,123.349500706132)) ;
#39324=CARTESIAN_POINT('Ctrl Pts',(-20.6014061829563,39.7280637678903,123.642094545317)) ;
#39325=CARTESIAN_POINT('Ctrl Pts',(-20.8994475639115,39.5480746874805,123.699654940687)) ;
#39326=CARTESIAN_POINT('Ctrl Pts',(-20.4948803150655,39.7446329552234,123.977922234663)) ;
#39327=CARTESIAN_POINT('Ctrl Pts',(-20.766262621046,39.5646438748136,124.119481950591)) ;
#39328=CARTESIAN_POINT('Ctrl Pts',(-20.279368944222,39.7612780950745,124.258669320355)) ;
#39329=CARTESIAN_POINT('Ctrl Pts',(-20.4969232973437,39.5812890146646,124.4703529915)) ;
#39330=CARTESIAN_POINT('Ctrl Pts',(-20.057952056873,39.7745503975479,124.428460036515)) ;
#39331=CARTESIAN_POINT('Ctrl Pts',(-20.220105563722,39.5945613171381,124.682635504539)) ;
#39332=CARTESIAN_POINT('Ctrl Pts',(-19.8719346516173,39.7845313609955,124.525525802343)) ;
#39333=CARTESIAN_POINT('Ctrl Pts',(-19.987592650646,39.6045422805857,124.803956293418)) ;
#39334=CARTESIAN_POINT('Ctrl Pts',(-19.6726840160093,39.7944731930648,124.588696431075)) ;
#39335=CARTESIAN_POINT('Ctrl Pts',(-19.7385233068457,39.614484112655,124.882919421842)) ;
#39336=CARTESIAN_POINT('Ctrl Pts',(-19.3951538397195,39.8077927622802,124.625793701431)) ;
#39337=CARTESIAN_POINT('Ctrl Pts',(-19.3916274184832,39.6278036818704,124.929289096375)) ;
#39338=CARTESIAN_POINT('Ctrl Pts',(-19.0464383279096,39.824322917213,124.581253491284)) ;
#39339=CARTESIAN_POINT('Ctrl Pts',(-18.9557155359745,39.6443338368031,124.87360860491)) ;
#39340=CARTESIAN_POINT('Ctrl Pts',(-18.668086969949,39.8443446427051,124.386327800272)) ;
#39341=CARTESIAN_POINT('Ctrl Pts',(-18.4827841914454,39.6643555622952,124.629948165765)) ;
#39342=CARTESIAN_POINT('Ctrl Pts',(-18.3816863058028,39.8641560393119,124.077284990008)) ;
#39343=CARTESIAN_POINT('Ctrl Pts',(-18.1247857375312,39.6841669589021,124.243642886359)) ;
#39344=CARTESIAN_POINT('Ctrl Pts',(-18.2159257669221,39.8841412880207,123.686114821925)) ;
#39345=CARTESIAN_POINT('Ctrl Pts',(-17.9175888920775,39.7041522076109,123.754678947972)) ;
#39346=CARTESIAN_POINT('Ctrl Pts',(-18.1939835367103,39.9040353506567,123.263614550275)) ;
#39347=CARTESIAN_POINT('Ctrl Pts',(-17.8901646193541,39.7240462702468,123.226554358743)) ;
#39348=CARTESIAN_POINT('Ctrl Pts',(-18.317143757237,39.9239670298303,122.858111488064)) ;
#39349=CARTESIAN_POINT('Ctrl Pts',(-18.04411771938,39.7439779494204,122.719677099865)) ;
#39350=CARTESIAN_POINT('Ctrl Pts',(-18.5719284249735,39.9439310843023,122.518586193573)) ;
#39351=CARTESIAN_POINT('Ctrl Pts',(-18.3626008286058,39.7639420038924,122.295272619699)) ;
#39352=CARTESIAN_POINT('Ctrl Pts',(-18.9256419898356,39.9638119860652,122.287076377155)) ;
#39353=CARTESIAN_POINT('Ctrl Pts',(-18.8047431637994,39.7838229056553,122.005888410371)) ;
#39354=CARTESIAN_POINT('Ctrl Pts',(-19.3381892305123,39.9837506476736,122.189510079094)) ;
#39355=CARTESIAN_POINT('Ctrl Pts',(-19.3204270314269,39.8037615672637,121.883932996497)) ;
#39356=CARTESIAN_POINT('Ctrl Pts',(-19.7583997067115,40.0036471729289,122.23841409713)) ;
#39357=CARTESIAN_POINT('Ctrl Pts',(-19.8456885699693,39.8236580925191,121.945064977798)) ;
#39358=CARTESIAN_POINT('Ctrl Pts',(-20.1370001314726,40.0235422113832,122.427152769696)) ;
#39359=CARTESIAN_POINT('Ctrl Pts',(-20.3189371294042,39.8435531309734,122.180988955617)) ;
#39360=CARTESIAN_POINT('Ctrl Pts',(-20.4293996902846,40.0435060346893,122.734826780891)) ;
#39361=CARTESIAN_POINT('Ctrl Pts',(-20.6844353023525,39.8635169542794,122.565581974884)) ;
#39362=CARTESIAN_POINT('Ctrl Pts',(-20.598804014177,40.0633801588183,123.121996946429)) ;
#39363=CARTESIAN_POINT('Ctrl Pts',(-20.896189201181,39.8833910784085,123.049543285413)) ;
#39364=CARTESIAN_POINT('Ctrl Pts',(-20.6264486511241,40.0833552345456,123.545839265876)) ;
#39365=CARTESIAN_POINT('Ctrl Pts',(-20.9307446999829,39.9033661541358,123.579345858912)) ;
#39366=CARTESIAN_POINT('Ctrl Pts',(-20.5073509704462,40.1033088039022,123.953040176851)) ;
#39367=CARTESIAN_POINT('Ctrl Pts',(-20.7818723369442,39.9233197234924,124.088346140081)) ;
#39368=CARTESIAN_POINT('Ctrl Pts',(-20.2585393963816,40.12314671409,124.293652583633)) ;
#39369=CARTESIAN_POINT('Ctrl Pts',(-20.4708597449385,39.9431576336802,124.514109737986)) ;
#39370=CARTESIAN_POINT('Ctrl Pts',(-19.9062499760645,40.143122542661,124.530920991778)) ;
#39371=CARTESIAN_POINT('Ctrl Pts',(-20.0304987771177,39.9631334622511,124.810695893645)) ;
#39372=CARTESIAN_POINT('Ctrl Pts',(-19.4952472081866,40.1630405873712,124.63297354376)) ;
#39373=CARTESIAN_POINT('Ctrl Pts',(-19.5167467255033,39.9830515069614,124.938262136375)) ;
#39374=CARTESIAN_POINT('Ctrl Pts',(-19.0748749833404,40.1829108331589,124.58981024594)) ;
#39375=CARTESIAN_POINT('Ctrl Pts',(-18.9912829799655,40.0029217527491,124.884310017426)) ;
#39376=CARTESIAN_POINT('Ctrl Pts',(-18.6914968706604,40.2029598362585,124.403647517381)) ;
#39377=CARTESIAN_POINT('Ctrl Pts',(-18.5120590676542,40.0229707558487,124.651607827886)) ;
#39378=CARTESIAN_POINT('Ctrl Pts',(-18.3981552231749,40.2227390774993,124.10210693945)) ;
#39379=CARTESIAN_POINT('Ctrl Pts',(-18.1453823899239,40.0427499970895,124.274685535376)) ;
#39380=CARTESIAN_POINT('Ctrl Pts',(-18.2226350296879,40.2427691412082,123.714169214818)) ;
#39381=CARTESIAN_POINT('Ctrl Pts',(-17.9259795061212,40.0627800607984,123.789764142182)) ;
#39382=CARTESIAN_POINT('Ctrl Pts',(-18.1909445920671,40.2626514261102,123.292541082987)) ;
#39383=CARTESIAN_POINT('Ctrl Pts',(-17.8863640755037,40.0826623457003,123.262730489932)) ;
#39384=CARTESIAN_POINT('Ctrl Pts',(-18.3038777435817,40.2825337270031,122.885191709277)) ;
#39385=CARTESIAN_POINT('Ctrl Pts',(-18.0275270007158,40.1025446465933,122.753544083074)) ;
#39386=CARTESIAN_POINT('Ctrl Pts',(-18.5504210038991,40.3025168366215,122.539129314307)) ;
#39387=CARTESIAN_POINT('Ctrl Pts',(-18.3357032517793,40.1225277562117,122.320964219428)) ;
#39388=CARTESIAN_POINT('Ctrl Pts',(-18.8986806428871,40.3224072319994,122.29912255241)) ;
#39389=CARTESIAN_POINT('Ctrl Pts',(-18.7710249751716,40.1424181515896,122.02095345069)) ;
#39390=CARTESIAN_POINT('Ctrl Pts',(-19.3078266805979,40.3423040220336,122.191737778741)) ;
#39391=CARTESIAN_POINT('Ctrl Pts',(-19.2824556627303,40.1623149416238,121.886718883262)) ;
#39392=CARTESIAN_POINT('Ctrl Pts',(-19.7296085524883,40.3622210759752,122.230003374302)) ;
#39393=CARTESIAN_POINT('Ctrl Pts',(-19.8096827929728,40.1822319955654,121.934546603933)) ;
#39394=CARTESIAN_POINT('Ctrl Pts',(-20.1146489811739,40.3822246241788,122.410827144587)) ;
#39395=CARTESIAN_POINT('Ctrl Pts',(-20.290985297795,40.2022355437689,122.160572440188)) ;
#39396=CARTESIAN_POINT('Ctrl Pts',(-20.4133927271247,40.4021629178314,122.711596083807)) ;
#39397=CARTESIAN_POINT('Ctrl Pts',(-20.6644175476842,40.2221738374216,122.536530476468)) ;
#39398=CARTESIAN_POINT('Ctrl Pts',(-20.5914685302538,40.4219844052643,123.093592798811)) ;
#39399=CARTESIAN_POINT('Ctrl Pts',(-20.887016493454,40.2419953248545,123.014022848791)) ;
#39400=CARTESIAN_POINT('Ctrl Pts',(-20.6292190379642,40.4419627982552,123.516656820411)) ;
#39401=CARTESIAN_POINT('Ctrl Pts',(-20.9342078754109,40.2619737178453,123.542854403197)) ;
#39402=CARTESIAN_POINT('Ctrl Pts',(-20.5204888317716,40.4618611798689,123.925614309865)) ;
#39403=CARTESIAN_POINT('Ctrl Pts',(-20.7983060144044,40.2818720994591,124.054044528047)) ;
#39404=CARTESIAN_POINT('Ctrl Pts',(-20.3195216622248,40.4784441105988,124.215207938259)) ;
#39405=CARTESIAN_POINT('Ctrl Pts',(-20.5470819881122,40.2984550301889,124.4160621592)) ;
#39406=CARTESIAN_POINT('Ctrl Pts',(-20.1066630617855,40.4917183461876,124.395787910796)) ;
#39407=CARTESIAN_POINT('Ctrl Pts',(-20.2810284413274,40.3117292657778,124.641768863656)) ;
#39408=CARTESIAN_POINT('Ctrl Pts',(-19.9242973164539,40.5017647636438,124.502269830301)) ;
#39409=CARTESIAN_POINT('Ctrl Pts',(-20.0530654837858,40.321775683234,124.774877815185)) ;
#39410=CARTESIAN_POINT('Ctrl Pts',(-19.7302037187856,40.5116099888631,124.57423387795)) ;
#39411=CARTESIAN_POINT('Ctrl Pts',(-19.8104644040159,40.3316209084532,124.864833820597)) ;
#39412=CARTESIAN_POINT('Ctrl Pts',(-19.4546005991835,40.5249449599025,124.625166757655)) ;
#39413=CARTESIAN_POINT('Ctrl Pts',(-19.4658929191253,40.3449558794926,124.928504806304)) ;
#39414=CARTESIAN_POINT('Ctrl Pts',(-19.102968767351,40.5415278166951,124.597279021719)) ;
#39415=CARTESIAN_POINT('Ctrl Pts',(-19.0264390688112,40.3615387362853,124.893652813631)) ;
#39416=CARTESIAN_POINT('Ctrl Pts',(-18.7810021390429,40.5581708190445,124.450732297002)) ;
#39417=CARTESIAN_POINT('Ctrl Pts',(-18.6239205040099,40.3781817386347,124.710456066607)) ;
#39418=CARTESIAN_POINT('Ctrl Pts',(-18.5658420171576,40.5714145500762,124.273876479058)) ;
#39419=CARTESIAN_POINT('Ctrl Pts',(-18.3550031410249,40.3914254696664,124.489405088458)) ;
#39420=CARTESIAN_POINT('Ctrl Pts',(-18.428371398618,40.5814689447508,124.113372164029)) ;
#39421=CARTESIAN_POINT('Ctrl Pts',(-18.1831556506219,40.401479864341,124.288773158627)) ;
#39422=CARTESIAN_POINT('Ctrl Pts',(-18.322862621758,40.5913100061393,123.935361777761)) ;
#39423=CARTESIAN_POINT('Ctrl Pts',(-18.051269318921,40.4113209257295,124.066262657629)) ;
#39424=CARTESIAN_POINT('Ctrl Pts',(-18.2480294467794,40.6013762304958,123.737449279801)) ;
#39425=CARTESIAN_POINT('Ctrl Pts',(-17.9577246776694,40.421387150086,123.81887262292)) ;
#39426=CARTESIAN_POINT('Ctrl Pts',(-18.2094701938353,40.6112568434155,123.533303511753)) ;
#39427=CARTESIAN_POINT('Ctrl Pts',(-17.9095230456685,40.4312677630057,123.563691114029)) ;
#39428=CARTESIAN_POINT('Ctrl Pts',(-18.206516541867,40.6212501365751,123.323267667439)) ;
#39429=CARTESIAN_POINT('Ctrl Pts',(-17.9058281377945,40.4412610561653,123.301146268744)) ;
#39430=CARTESIAN_POINT('Ctrl Pts',(-18.2398673386455,40.6312011447987,123.11670429861)) ;
#39431=CARTESIAN_POINT('Ctrl Pts',(-17.9475138798417,40.4512120643889,123.042941598597)) ;
#39432=CARTESIAN_POINT('Ctrl Pts',(-18.3093839574438,40.6412496591607,122.917243416711)) ;
#39433=CARTESIAN_POINT('Ctrl Pts',(-18.0344070396887,40.4612605787509,122.79361447851)) ;
#39434=CARTESIAN_POINT('Ctrl Pts',(-18.4101694123091,40.6510911652234,122.736528533016)) ;
#39435=CARTESIAN_POINT('Ctrl Pts',(-18.1603863835786,40.4711020848136,122.567719550019)) ;
#39436=CARTESIAN_POINT('Ctrl Pts',(-18.542325109746,40.6610768178531,122.573458997662)) ;
#39437=CARTESIAN_POINT('Ctrl Pts',(-18.3255788629678,40.4810877374433,122.363880789435)) ;
#39438=CARTESIAN_POINT('Ctrl Pts',(-18.7000440263116,40.671015826698,122.436353330348)) ;
#39439=CARTESIAN_POINT('Ctrl Pts',(-18.5227257140417,40.4910267462881,122.192496536493)) ;
#39440=CARTESIAN_POINT('Ctrl Pts',(-18.8809941836839,40.681056751991,122.327685783444)) ;
#39441=CARTESIAN_POINT('Ctrl Pts',(-18.7489120153054,40.5010676715811,122.056659651351)) ;
#39442=CARTESIAN_POINT('Ctrl Pts',(-19.0750989997885,40.6909470737459,122.253093211541)) ;
#39443=CARTESIAN_POINT('Ctrl Pts',(-18.9915421154264,40.510957993336,121.963416273377)) ;
#39444=CARTESIAN_POINT('Ctrl Pts',(-19.2812929576741,40.7009430470793,122.212614380291)) ;
#39445=CARTESIAN_POINT('Ctrl Pts',(-19.2492841014226,40.5209539666695,121.912814957427)) ;
#39446=CARTESIAN_POINT('Ctrl Pts',(-19.4900519469436,40.7108744466613,122.208562124172)) ;
#39447=CARTESIAN_POINT('Ctrl Pts',(-19.5102329048688,40.5308853662515,121.907746825815)) ;
#39448=CARTESIAN_POINT('Ctrl Pts',(-19.6979309739298,40.7208799871384,122.240764687343)) ;
#39449=CARTESIAN_POINT('Ctrl Pts',(-19.7700821946182,40.5408909067286,121.947997275282)) ;
#39450=CARTESIAN_POINT('Ctrl Pts',(-19.8974653853249,40.7309129710697,122.30911862514)) ;
#39451=CARTESIAN_POINT('Ctrl Pts',(-20.0195011591116,40.5509238906599,122.033437044864)) ;
#39452=CARTESIAN_POINT('Ctrl Pts',(-20.0790342263548,40.7407686018965,122.40896792997)) ;
#39453=CARTESIAN_POINT('Ctrl Pts',(-20.2464637604677,40.5607795214867,122.158246335516)) ;
#39454=CARTESIAN_POINT('Ctrl Pts',(-20.2429931194927,40.7507680040897,122.540475873946)) ;
#39455=CARTESIAN_POINT('Ctrl Pts',(-20.4514141920233,40.5707789236799,122.322629146691)) ;
#39456=CARTESIAN_POINT('Ctrl Pts',(-20.3804016988981,40.7606624734508,122.696694794566)) ;
#39457=CARTESIAN_POINT('Ctrl Pts',(-20.6231771610024,40.5806733930409,122.517901168741)) ;
#39458=CARTESIAN_POINT('Ctrl Pts',(-20.4903492131892,40.770725587615,122.877396553859)) ;
#39459=CARTESIAN_POINT('Ctrl Pts',(-20.7606139058303,40.5907365072052,122.74377689725)) ;
#39460=CARTESIAN_POINT('Ctrl Pts',(-20.565781026169,40.7805652333314,123.070050005765)) ;
#39461=CARTESIAN_POINT('Ctrl Pts',(-20.8549063787126,40.6005761529215,122.984593090439)) ;
#39462=CARTESIAN_POINT('Ctrl Pts',(-20.6077950411033,40.7906284008871,123.277366104284)) ;
#39463=CARTESIAN_POINT('Ctrl Pts',(-20.9074265588259,40.6106393204773,123.243737629729)) ;
#39464=CARTESIAN_POINT('Ctrl Pts',(-20.6129087024178,40.800522656682,123.485334552873)) ;
#39465=CARTESIAN_POINT('Ctrl Pts',(-20.9138213840981,40.6205335762722,123.503698450434)) ;
#39466=CARTESIAN_POINT('Ctrl Pts',(-20.5822552704826,40.8104644351417,123.692055896881)) ;
#39467=CARTESIAN_POINT('Ctrl Pts',(-20.8755072032349,40.6304753547318,123.762100783277)) ;
#39468=CARTESIAN_POINT('Ctrl Pts',(-20.5158234904619,40.8204671279719,123.891604227127)) ;
#39469=CARTESIAN_POINT('Ctrl Pts',(-20.7924699763018,40.640478047562,124.011537115985)) ;
#39470=CARTESIAN_POINT('Ctrl Pts',(-20.4151748597048,40.8305011499257,124.076979654914)) ;
#39471=CARTESIAN_POINT('Ctrl Pts',(-20.6666615752948,40.6505120695159,124.24325767995)) ;
#39472=CARTESIAN_POINT('Ctrl Pts',(-20.2865434555371,40.8403489410147,124.239210149898)) ;
#39473=CARTESIAN_POINT('Ctrl Pts',(-20.5058740591631,40.6603598606049,124.446047890663)) ;
#39474=CARTESIAN_POINT('Ctrl Pts',(-20.1299205089068,40.8503304655638,124.378837643327)) ;
#39475=CARTESIAN_POINT('Ctrl Pts',(-20.3100969714377,40.6703413851539,124.620584309746)) ;
#39476=CARTESIAN_POINT('Ctrl Pts',(-19.951972487446,40.8602796890547,124.488778577698)) ;
#39477=CARTESIAN_POINT('Ctrl Pts',(-20.0876630799847,40.6802906086448,124.75801282766)) ;
#39478=CARTESIAN_POINT('Ctrl Pts',(-19.7567802099133,40.8702773452713,124.566778486158)) ;
#39479=CARTESIAN_POINT('Ctrl Pts',(-19.8436735817006,40.6902882648614,124.855515120225)) ;
#39480=CARTESIAN_POINT('Ctrl Pts',(-19.5500818247868,40.8803175583263,124.609481079621)) ;
#39481=CARTESIAN_POINT('Ctrl Pts',(-19.5853011891649,40.7003284779165,124.908895920556)) ;
#39482=CARTESIAN_POINT('Ctrl Pts',(-19.3435554371878,40.8901456056026,124.615967681651)) ;
#39483=CARTESIAN_POINT('Ctrl Pts',(-19.3271425182184,40.7101565251927,124.917006738084)) ;
#39484=CARTESIAN_POINT('Ctrl Pts',(-19.1343072045349,40.9001999526349,124.586146876164)) ;
#39485=CARTESIAN_POINT('Ctrl Pts',(-19.0655819825026,40.7202108722251,124.879733201106)) ;
#39486=CARTESIAN_POINT('Ctrl Pts',(-18.9357705406544,40.9101410889635,124.520845573056)) ;
#39487=CARTESIAN_POINT('Ctrl Pts',(-18.8174100403861,40.7301520085537,124.798108890676)) ;
#39488=CARTESIAN_POINT('Ctrl Pts',(-18.7519690818306,40.9200453220432,124.423000581694)) ;
#39489=CARTESIAN_POINT('Ctrl Pts',(-18.5876566118976,40.7400562416334,124.675804537105)) ;
#39490=CARTESIAN_POINT('Ctrl Pts',(-18.585688282195,40.9300920188868,124.292792552293)) ;
#39491=CARTESIAN_POINT('Ctrl Pts',(-18.3798041844337,40.750102938477,124.513046489753)) ;
#39492=CARTESIAN_POINT('Ctrl Pts',(-18.4464901568893,40.9399875701671,124.138142420818)) ;
#39493=CARTESIAN_POINT('Ctrl Pts',(-18.2058043531238,40.7599984897572,124.319735002342)) ;
#39494=CARTESIAN_POINT('Ctrl Pts',(-18.3344376414912,40.9500496480066,123.958756744201)) ;
#39495=CARTESIAN_POINT('Ctrl Pts',(-18.0657367626223,40.7700605675967,124.095504335567)) ;
#39496=CARTESIAN_POINT('Ctrl Pts',(-18.2568316622771,40.9598923571026,123.766911195192)) ;
#39497=CARTESIAN_POINT('Ctrl Pts',(-17.9687267603037,40.7799032766928,123.85569749179)) ;
#39498=CARTESIAN_POINT('Ctrl Pts',(-18.2125910584586,40.9698830893411,123.561614077019)) ;
#39499=CARTESIAN_POINT('Ctrl Pts',(-17.9134237542837,40.7898940089313,123.599076400328)) ;
#39500=CARTESIAN_POINT('Ctrl Pts',(-18.204750664211,40.9798111145698,123.353032026553)) ;
#39501=CARTESIAN_POINT('Ctrl Pts',(-17.9036209756427,40.79982203416,123.338348435946)) ;
#39502=CARTESIAN_POINT('Ctrl Pts',(-18.2330639112473,40.9897992612204,123.14496244916)) ;
#39503=CARTESIAN_POINT('Ctrl Pts',(-17.9390103971516,40.8098101808106,123.078260992333)) ;
#39504=CARTESIAN_POINT('Ctrl Pts',(-18.297681746232,40.9998342790604,122.944131359391)) ;
#39505=CARTESIAN_POINT('Ctrl Pts',(-18.0197805146049,40.8198451986505,122.827221506628)) ;
#39506=CARTESIAN_POINT('Ctrl Pts',(-18.3943201381265,41.0096990761655,122.760643431724)) ;
#39507=CARTESIAN_POINT('Ctrl Pts',(-18.1405769535564,40.8297099957557,122.597859805784)) ;
#39508=CARTESIAN_POINT('Ctrl Pts',(-18.5221077214792,41.0196598085217,122.594742227815)) ;
#39509=CARTESIAN_POINT('Ctrl Pts',(-18.3003100261573,40.8396707281118,122.3904817787)) ;
#39510=CARTESIAN_POINT('Ctrl Pts',(-18.6781171729852,41.0296932709187,122.452788170327)) ;
#39511=CARTESIAN_POINT('Ctrl Pts',(-18.4953203364259,40.8497041905088,122.213037685438)) ;
#39512=CARTESIAN_POINT('Ctrl Pts',(-18.8536177054508,41.0395788051301,122.341428905828)) ;
#39513=CARTESIAN_POINT('Ctrl Pts',(-18.7146955767599,40.8595897247203,122.073836456168)) ;
#39514=CARTESIAN_POINT('Ctrl Pts',(-19.0492301850846,41.0496436458101,122.260823818413)) ;
#39515=CARTESIAN_POINT('Ctrl Pts',(-18.959210160501,40.8696545654002,121.97307830108)) ;
#39516=CARTESIAN_POINT('Ctrl Pts',(-19.2514386207072,41.0594917775389,122.216286024392)) ;
#39517=CARTESIAN_POINT('Ctrl Pts',(-19.2119712899372,40.8795026971291,121.917403865037)) ;
#39518=CARTESIAN_POINT('Ctrl Pts',(-19.4620301676676,41.0695192745291,122.206830853245)) ;
#39519=CARTESIAN_POINT('Ctrl Pts',(-19.4752106016356,40.8895301941192,121.905583046099)) ;
#39520=CARTESIAN_POINT('Ctrl Pts',(-19.6710285196364,41.0795477265741,122.234643377154)) ;
#39521=CARTESIAN_POINT('Ctrl Pts',(-19.7364587404742,40.8995586461643,121.940346685174)) ;
#39522=CARTESIAN_POINT('Ctrl Pts',(-19.8684484239612,41.0893929931382,122.29677641338)) ;
#39523=CARTESIAN_POINT('Ctrl Pts',(-19.9832352577445,40.9094039127284,122.018011497332)) ;
#39524=CARTESIAN_POINT('Ctrl Pts',(-20.05506817094,41.0993836660792,122.39316265703)) ;
#39525=CARTESIAN_POINT('Ctrl Pts',(-20.216510909968,40.9193945856693,122.138492853091)) ;
#39526=CARTESIAN_POINT('Ctrl Pts',(-20.2226153017789,41.1094215481676,122.521458694971)) ;
#39527=CARTESIAN_POINT('Ctrl Pts',(-20.4259458604825,40.9294324677578,122.298861327962)) ;
#39528=CARTESIAN_POINT('Ctrl Pts',(-20.3628619913098,41.1192659186073,122.673663617627)) ;
#39529=CARTESIAN_POINT('Ctrl Pts',(-20.6012563124349,40.9392768381975,122.489117146643)) ;
#39530=CARTESIAN_POINT('Ctrl Pts',(-20.4764734479912,41.1292507460027,122.850139489613)) ;
#39531=CARTESIAN_POINT('Ctrl Pts',(-20.7432721400765,40.9492616655929,122.709711313063)) ;
#39532=CARTESIAN_POINT('Ctrl Pts',(-20.5574566491448,41.139190191408,123.042799763275)) ;
#39533=CARTESIAN_POINT('Ctrl Pts',(-20.8445028247559,40.9592011109982,122.950536538192)) ;
#39534=CARTESIAN_POINT('Ctrl Pts',(-20.6041559807991,41.1492301956939,123.248619953668)) ;
#39535=CARTESIAN_POINT('Ctrl Pts',(-20.9028785374185,40.9692411152841,123.20781127081)) ;
#39536=CARTESIAN_POINT('Ctrl Pts',(-20.6143967382331,41.1591173048795,123.456249137288)) ;
#39537=CARTESIAN_POINT('Ctrl Pts',(-20.9156810986657,40.9791282244697,123.467348610192)) ;
#39538=CARTESIAN_POINT('Ctrl Pts',(-20.5883994319064,41.169117364782,123.664835776685)) ;
#39539=CARTESIAN_POINT('Ctrl Pts',(-20.8831859203431,40.9891282843722,123.728082234678)) ;
#39540=CARTESIAN_POINT('Ctrl Pts',(-20.5272409128475,41.1790347806967,123.864195390867)) ;
#39541=CARTESIAN_POINT('Ctrl Pts',(-20.8067389221257,40.9990457002868,123.977282854294)) ;
#39542=CARTESIAN_POINT('Ctrl Pts',(-20.4311340846493,41.1890815954375,124.052246102088)) ;
#39543=CARTESIAN_POINT('Ctrl Pts',(-20.6866067691322,41.0090925150276,124.212346711467)) ;
#39544=CARTESIAN_POINT('Ctrl Pts',(-20.3061390393343,41.1989570726341,124.218058301868)) ;
#39545=CARTESIAN_POINT('Ctrl Pts',(-20.5303634280542,41.0189679922243,124.419613620492)) ;
#39546=CARTESIAN_POINT('Ctrl Pts',(-20.1516052416653,41.2090131683554,124.362275980325)) ;
#39547=CARTESIAN_POINT('Ctrl Pts',(-20.337197279219,41.0290240879456,124.59988651574)) ;
#39548=CARTESIAN_POINT('Ctrl Pts',(-19.977229302393,41.2189063303704,124.475710615594)) ;
#39549=CARTESIAN_POINT('Ctrl Pts',(-20.1192272912167,41.0389172499606,124.741681401937)) ;
#39550=CARTESIAN_POINT('Ctrl Pts',(-19.782620580465,41.228968566393,124.558568223159)) ;
#39551=CARTESIAN_POINT('Ctrl Pts',(-19.8759671921911,41.0489794859832,124.845254462192)) ;
#39552=CARTESIAN_POINT('Ctrl Pts',(-19.5810123835409,41.238813032022,124.605369966311)) ;
#39553=CARTESIAN_POINT('Ctrl Pts',(-19.6239559484713,41.0588239516122,124.903758180458)) ;
#39554=CARTESIAN_POINT('Ctrl Pts',(-19.3719656317782,41.2487731247261,124.617339157751)) ;
#39555=CARTESIAN_POINT('Ctrl Pts',(-19.3626471098538,41.0687840443163,124.918720690841)) ;
#39556=CARTESIAN_POINT('Ctrl Pts',(-19.1624388090685,41.2588114137072,124.592224884282)) ;
#39557=CARTESIAN_POINT('Ctrl Pts',(-19.1007386053402,41.0788223332973,124.887329010264)) ;
#39558=CARTESIAN_POINT('Ctrl Pts',(-18.9636200217074,41.2686847368134,124.532486383853)) ;
#39559=CARTESIAN_POINT('Ctrl Pts',(-18.8522137572245,41.0886956564036,124.812656518807)) ;
#39560=CARTESIAN_POINT('Ctrl Pts',(-18.7745367667636,41.2787579208985,124.437217363327)) ;
#39561=CARTESIAN_POINT('Ctrl Pts',(-18.6158596069145,41.0987688404886,124.693571352433)) ;
#39562=CARTESIAN_POINT('Ctrl Pts',(-18.6088938849064,41.2885784331864,124.313905580801)) ;
#39563=CARTESIAN_POINT('Ctrl Pts',(-18.4088042083413,41.1085893527766,124.539431437852)) ;
#39564=CARTESIAN_POINT('Ctrl Pts',(-18.4633794200554,41.2986564293022,124.159977351109)) ;
#39565=CARTESIAN_POINT('Ctrl Pts',(-18.2269108302381,41.1186673488924,124.34702207149)) ;
#39566=CARTESIAN_POINT('Ctrl Pts',(-18.34929862132,41.3085105042855,123.986997787861)) ;
#39567=CARTESIAN_POINT('Ctrl Pts',(-18.0843084262806,41.1285214238756,124.130796993376)) ;
#39568=CARTESIAN_POINT('Ctrl Pts',(-18.2650562986397,41.3185743858692,123.79296185912)) ;
#39569=CARTESIAN_POINT('Ctrl Pts',(-17.9790049811193,41.1385853054594,123.888252695301)) ;
#39570=CARTESIAN_POINT('Ctrl Pts',(-18.2166879254847,41.3284578118429,123.590852828316)) ;
#39571=CARTESIAN_POINT('Ctrl Pts',(-17.9185435300632,41.1484687314331,123.635615538462)) ;
#39572=CARTESIAN_POINT('Ctrl Pts',(-18.2036681221716,41.338458415764,123.381049020955)) ;
#39573=CARTESIAN_POINT('Ctrl Pts',(-17.9022681371012,41.1584693353541,123.373360677128)) ;
#39574=CARTESIAN_POINT('Ctrl Pts',(-18.2269611110855,41.3483782001018,123.173770725139)) ;
#39575=CARTESIAN_POINT('Ctrl Pts',(-17.9313838879789,41.168389119692,123.114261971912)) ;
#39576=CARTESIAN_POINT('Ctrl Pts',(-18.2866756180986,41.3584255504587,122.971196494413)) ;
#39577=CARTESIAN_POINT('Ctrl Pts',(-18.006026378471,41.1784364700489,122.861044240418)) ;
#39578=CARTESIAN_POINT('Ctrl Pts',(-18.3788795710986,41.368302892693,122.785091205517)) ;
#39579=CARTESIAN_POINT('Ctrl Pts',(-18.1212813811311,41.1883138122831,122.628411371789)) ;
#39580=CARTESIAN_POINT('Ctrl Pts',(-18.5043585823623,41.3783727737676,122.614637642039)) ;
#39581=CARTESIAN_POINT('Ctrl Pts',(-18.2781294850694,41.1983836933578,122.415344458244)) ;
#39582=CARTESIAN_POINT('Ctrl Pts',(-18.6537818292948,41.3882024789693,122.471833456278)) ;
#39583=CARTESIAN_POINT('Ctrl Pts',(-18.464909367622,41.2082133985595,122.236837854642)) ;
#39584=CARTESIAN_POINT('Ctrl Pts',(-18.8296579695578,41.3982691401357,122.35418375427)) ;
#39585=CARTESIAN_POINT('Ctrl Pts',(-18.6847540386552,41.2182800597259,122.089775689202)) ;
#39586=CARTESIAN_POINT('Ctrl Pts',(-19.0200041203782,41.408159362003,122.270450878119)) ;
#39587=CARTESIAN_POINT('Ctrl Pts',(-18.9226875395076,41.2281702815932,121.985108837404)) ;
#39588=CARTESIAN_POINT('Ctrl Pts',(-19.2239333482095,41.4181515381132,122.220092117685)) ;
#39589=CARTESIAN_POINT('Ctrl Pts',(-19.1775992382412,41.2381624577033,121.922160157679)) ;
#39590=CARTESIAN_POINT('Ctrl Pts',(-19.432913401362,41.4281143682258,122.206147099919)) ;
#39591=CARTESIAN_POINT('Ctrl Pts',(-19.4388247420812,41.248125287816,121.904728591828)) ;
#39592=CARTESIAN_POINT('Ctrl Pts',(-19.6399945794,41.4380185806261,122.228042536446)) ;
#39593=CARTESIAN_POINT('Ctrl Pts',(-19.6976771545736,41.2580295002163,121.932097935287)) ;
#39594=CARTESIAN_POINT('Ctrl Pts',(-19.84319524037,41.448079294714,122.286638879611)) ;
#39595=CARTESIAN_POINT('Ctrl Pts',(-19.9516776747538,41.2680902143041,122.005343143333)) ;
#39596=CARTESIAN_POINT('Ctrl Pts',(-20.0291359735094,41.4579187976968,122.377353855789)) ;
#39597=CARTESIAN_POINT('Ctrl Pts',(-20.1841049253303,41.277929717287,122.118737500437)) ;
#39598=CARTESIAN_POINT('Ctrl Pts',(-20.2004294013988,41.4679849362632,122.501563731977)) ;
#39599=CARTESIAN_POINT('Ctrl Pts',(-20.398221343626,41.2879958558534,122.273999666792)) ;
#39600=CARTESIAN_POINT('Ctrl Pts',(-20.3448588998162,41.4778674507492,122.650955267273)) ;
#39601=CARTESIAN_POINT('Ctrl Pts',(-20.5787589736022,41.2978783703394,122.460739928053)) ;
#39602=CARTESIAN_POINT('Ctrl Pts',(-20.4627539040108,41.4878597501047,122.824784252551)) ;
#39603=CARTESIAN_POINT('Ctrl Pts',(-20.726127681702,41.3078706696949,122.678026456286)) ;
#39604=CARTESIAN_POINT('Ctrl Pts',(-20.5484123348916,41.4978128170581,123.01572690911)) ;
#39605=CARTESIAN_POINT('Ctrl Pts',(-20.8332007283989,41.3178237366483,122.916705335821)) ;
#39606=CARTESIAN_POINT('Ctrl Pts',(-20.5999387117747,41.5078475252634,123.220282510794)) ;
#39607=CARTESIAN_POINT('Ctrl Pts',(-20.8976084793922,41.3278584448536,123.172399737511)) ;
#39608=CARTESIAN_POINT('Ctrl Pts',(-20.6150963668154,41.5177357461675,123.42762288197)) ;
#39609=CARTESIAN_POINT('Ctrl Pts',(-20.9165553817882,41.3377466657577,123.431576287924)) ;
#39610=CARTESIAN_POINT('Ctrl Pts',(-20.5941420991674,41.527730169198,123.636678083396)) ;
#39611=CARTESIAN_POINT('Ctrl Pts',(-20.8903621465551,41.3477410887881,123.692895458751)) ;
#39612=CARTESIAN_POINT('Ctrl Pts',(-20.5374038460003,41.5376755086441,123.837915099807)) ;
#39613=CARTESIAN_POINT('Ctrl Pts',(-20.8194388312566,41.3576864282343,123.944442205992)) ;
#39614=CARTESIAN_POINT('Ctrl Pts',(-20.4469513423603,41.5476228532555,124.026477171833)) ;
#39615=CARTESIAN_POINT('Ctrl Pts',(-20.7063724849258,41.3676337728457,124.180145089971)) ;
#39616=CARTESIAN_POINT('Ctrl Pts',(-20.3237166893896,41.5576707486665,124.198034788354)) ;
#39617=CARTESIAN_POINT('Ctrl Pts',(-20.5523289699453,41.3776816682566,124.394591659051)) ;
#39618=CARTESIAN_POINT('Ctrl Pts',(-20.1756958626887,41.5675183941458,124.342779195868)) ;
#39619=CARTESIAN_POINT('Ctrl Pts',(-20.3673015896702,41.387529313736,124.575522794195)) ;
#39620=CARTESIAN_POINT('Ctrl Pts',(-20.0031915988338,41.5774801080598,124.461512163313)) ;
#39621=CARTESIAN_POINT('Ctrl Pts',(-20.1516704587089,41.39749102765,124.72393864251)) ;
#39622=CARTESIAN_POINT('Ctrl Pts',(-19.8112800553437,41.5875087323508,124.548840187101)) ;
#39623=CARTESIAN_POINT('Ctrl Pts',(-19.9117808501252,41.407519651941,124.833098044419)) ;
#39624=CARTESIAN_POINT('Ctrl Pts',(-19.6095677146579,41.5974190930075,124.600957112613)) ;
#39625=CARTESIAN_POINT('Ctrl Pts',(-19.6596394073154,41.4174300125977,124.898243770092)) ;
#39626=CARTESIAN_POINT('Ctrl Pts',(-19.4013858198479,41.6073537915808,124.617849546448)) ;
#39627=CARTESIAN_POINT('Ctrl Pts',(-19.3994113076563,41.4273647111709,124.919358484118)) ;
#39628=CARTESIAN_POINT('Ctrl Pts',(-19.1912280423145,41.617395616435,124.597921301321)) ;
#39629=CARTESIAN_POINT('Ctrl Pts',(-19.1367143515036,41.4374065360251,124.894447395095)) ;
#39630=CARTESIAN_POINT('Ctrl Pts',(-18.990832747362,41.6272801901794,124.542852864692)) ;
#39631=CARTESIAN_POINT('Ctrl Pts',(-18.8862194476492,41.4472911097696,124.825610729132)) ;
#39632=CARTESIAN_POINT('Ctrl Pts',(-18.8007506253046,41.6372820395426,124.453017154148)) ;
#39633=CARTESIAN_POINT('Ctrl Pts',(-18.6486170761849,41.4572929591327,124.713315149786)) ;
#39634=CARTESIAN_POINT('Ctrl Pts',(-18.6304363747329,41.6472013411166,124.332637276004)) ;
#39635=CARTESIAN_POINT('Ctrl Pts',(-18.4357242322811,41.4672122607068,124.562839022711)) ;
#39636=CARTESIAN_POINT('Ctrl Pts',(-18.4817919543754,41.6572454494619,124.182685192246)) ;
#39637=CARTESIAN_POINT('Ctrl Pts',(-18.2499195837337,41.4772563690521,124.375398347037)) ;
#39638=CARTESIAN_POINT('Ctrl Pts',(-18.3632889695078,41.6671298729041,124.011973794938)) ;
#39639=CARTESIAN_POINT('Ctrl Pts',(-18.101791128682,41.4871407924943,124.162007655871)) ;
#39640=CARTESIAN_POINT('Ctrl Pts',(-18.2746407632442,41.6771462348136,123.820958583722)) ;
#39641=CARTESIAN_POINT('Ctrl Pts',(-17.9909819761394,41.4971571544038,123.923238127111)) ;
#39642=CARTESIAN_POINT('Ctrl Pts',(-18.2209377342613,41.687182890319,123.616916772057)) ;
#39643=CARTESIAN_POINT('Ctrl Pts',(-17.923854202781,41.5071938099091,123.668185724593)) ;
#39644=CARTESIAN_POINT('Ctrl Pts',(-18.2032737429254,41.6970130205083,123.410988166114)) ;
#39645=CARTESIAN_POINT('Ctrl Pts',(-17.9017753133352,41.5170239400985,123.410773438911)) ;
#39646=CARTESIAN_POINT('Ctrl Pts',(-18.2220155993058,41.7070890735982,123.200029060193)) ;
#39647=CARTESIAN_POINT('Ctrl Pts',(-17.9252038428082,41.5270999931883,123.147075094829)) ;
#39648=CARTESIAN_POINT('Ctrl Pts',(-18.2757906963554,41.716941302784,122.999961670963)) ;
#39649=CARTESIAN_POINT('Ctrl Pts',(-17.9924242808848,41.5369522223742,122.896990000654)) ;
#39650=CARTESIAN_POINT('Ctrl Pts',(-18.3652603008448,41.7270145105833,122.808056320445)) ;
#39651=CARTESIAN_POINT('Ctrl Pts',(-18.104262344417,41.5470254301734,122.657109249367)) ;
#39652=CARTESIAN_POINT('Ctrl Pts',(-18.4839724624689,41.7368560219347,122.638585553312)) ;
#39653=CARTESIAN_POINT('Ctrl Pts',(-18.2526543868077,41.5568669415249,122.445270485512)) ;
#39654=CARTESIAN_POINT('Ctrl Pts',(-18.6315099791709,41.7468169599722,122.489983799293)) ;
#39655=CARTESIAN_POINT('Ctrl Pts',(-18.4370777101602,41.5668278795624,122.259519138092)) ;
#39656=CARTESIAN_POINT('Ctrl Pts',(-18.8041736856207,41.7568548218972,122.368670001095)) ;
#39657=CARTESIAN_POINT('Ctrl Pts',(-18.6529080737504,41.5768657414874,122.107878162764)) ;
#39658=CARTESIAN_POINT('Ctrl Pts',(-18.9920269431984,41.7667290078943,122.280273355514)) ;
#39659=CARTESIAN_POINT('Ctrl Pts',(-18.8877262423415,41.5867399274844,121.997383365616)) ;
#39660=CARTESIAN_POINT('Ctrl Pts',(-19.1963027713809,41.7767991674721,122.224790072043)) ;
#39661=CARTESIAN_POINT('Ctrl Pts',(-19.1430711045698,41.5968100870623,121.928030886466)) ;
#39662=CARTESIAN_POINT('Ctrl Pts',(-19.4021553537775,41.786630914898,122.205937341071)) ;
#39663=CARTESIAN_POINT('Ctrl Pts',(-19.4003882644738,41.6066418344882,121.90446647736)) ;
#39664=CARTESIAN_POINT('Ctrl Pts',(-19.6124500007053,41.7966669949693,122.222921105174)) ;
#39665=CARTESIAN_POINT('Ctrl Pts',(-19.6632563157886,41.6166779145595,121.925697979443)) ;
#39666=CARTESIAN_POINT('Ctrl Pts',(-19.8161003455475,41.8066840418218,122.27657994795)) ;
#39667=CARTESIAN_POINT('Ctrl Pts',(-19.9178188413612,41.626694961412,121.992773118828)) ;
#39668=CARTESIAN_POINT('Ctrl Pts',(-20.004923629097,41.8165662999884,122.363238250864)) ;
#39669=CARTESIAN_POINT('Ctrl Pts',(-20.1538480382327,41.6365772195785,122.101097977742)) ;
#39670=CARTESIAN_POINT('Ctrl Pts',(-20.1777719329602,41.8265539827847,122.482413681147)) ;
#39671=CARTESIAN_POINT('Ctrl Pts',(-20.3699075386574,41.6465649023749,122.250068895557)) ;
#39672=CARTESIAN_POINT('Ctrl Pts',(-20.326844928488,41.8365006395015,122.629102840794)) ;
#39673=CARTESIAN_POINT('Ctrl Pts',(-20.5562477856128,41.6565115590916,122.433432011436)) ;
#39674=CARTESIAN_POINT('Ctrl Pts',(-20.4493206526294,41.8465576975816,122.801419365625)) ;
#39675=CARTESIAN_POINT('Ctrl Pts',(-20.70934082782,41.6665686171718,122.648828544802)) ;
#39676=CARTESIAN_POINT('Ctrl Pts',(-20.5381348768749,41.8563758771311,122.98775540366)) ;
#39677=CARTESIAN_POINT('Ctrl Pts',(-20.8203574276799,41.6763867967212,122.8817505594)) ;
#39678=CARTESIAN_POINT('Ctrl Pts',(-20.5950148919747,41.86641181157,123.190925085264)) ;
#39679=CARTESIAN_POINT('Ctrl Pts',(-20.8914554134342,41.6864227311602,123.135713115913)) ;
#39680=CARTESIAN_POINT('Ctrl Pts',(-20.615129903165,41.876436465999,123.400720653862)) ;
#39681=CARTESIAN_POINT('Ctrl Pts',(-20.9165972821223,41.6964473855892,123.397957733957)) ;
#39682=CARTESIAN_POINT('Ctrl Pts',(-20.5992555683587,41.8862884855786,123.607234834638)) ;
#39683=CARTESIAN_POINT('Ctrl Pts',(-20.8967522554503,41.7062994051687,123.656101312772)) ;
#39684=CARTESIAN_POINT('Ctrl Pts',(-20.5473561444667,41.8962793992935,123.810736345392)) ;
#39685=CARTESIAN_POINT('Ctrl Pts',(-20.8318758705057,41.7162903188837,123.910477841252)) ;
#39686=CARTESIAN_POINT('Ctrl Pts',(-20.4616446993946,41.9061973881331,124.000839502752)) ;
#39687=CARTESIAN_POINT('Ctrl Pts',(-20.7247343586045,41.7262083077233,124.14810642243)) ;
#39688=CARTESIAN_POINT('Ctrl Pts',(-20.3429884977472,41.9162254988639,124.175080591613)) ;
#39689=CARTESIAN_POINT('Ctrl Pts',(-20.576412327472,41.7362364184541,124.365906529222)) ;
#39690=CARTESIAN_POINT('Ctrl Pts',(-20.1980255650348,41.9261106967723,124.323996156688)) ;
#39691=CARTESIAN_POINT('Ctrl Pts',(-20.3952065715185,41.7461216163624,124.552049981511)) ;
#39692=CARTESIAN_POINT('Ctrl Pts',(-20.0279320557978,41.9360999720403,124.447175593972)) ;
#39693=CARTESIAN_POINT('Ctrl Pts',(-20.1825881915895,41.7561108916304,124.706022484773)) ;
#39694=CARTESIAN_POINT('Ctrl Pts',(-19.837857448319,41.9461414302098,124.539013945011)) ;
#39695=CARTESIAN_POINT('Ctrl Pts',(-19.9449940548439,41.7661523498,124.820818389539)) ;
#39696=CARTESIAN_POINT('Ctrl Pts',(-19.6390644945786,41.9559728939981,124.595621547206)) ;
#39697=CARTESIAN_POINT('Ctrl Pts',(-19.6965012965353,41.7759838135883,124.8915759365)) ;
#39698=CARTESIAN_POINT('Ctrl Pts',(-19.4299150619604,41.965977826302,124.617688613248)) ;
#39699=CARTESIAN_POINT('Ctrl Pts',(-19.4350641759106,41.7859887458922,124.919157369888)) ;
#39700=CARTESIAN_POINT('Ctrl Pts',(-19.2204473086949,41.9759641901967,124.603013545437)) ;
#39701=CARTESIAN_POINT('Ctrl Pts',(-19.173229491633,41.7959751097869,124.900811143263)) ;
#39702=CARTESIAN_POINT('Ctrl Pts',(-19.0159203877433,41.9859938190826,124.551823701844)) ;
#39703=CARTESIAN_POINT('Ctrl Pts',(-18.9175714408516,41.8060047386728,124.836821562525)) ;
#39704=CARTESIAN_POINT('Ctrl Pts',(-18.8262081647961,41.995869041191,124.467451255716)) ;
#39705=CARTESIAN_POINT('Ctrl Pts',(-18.6804315219081,41.8158799607811,124.731353527427)) ;
#39706=CARTESIAN_POINT('Ctrl Pts',(-18.6517356024177,42.0058702535881,124.350176231649)) ;
#39707=CARTESIAN_POINT('Ctrl Pts',(-18.4623421035924,41.8258811731783,124.58475763756)) ;
#39708=CARTESIAN_POINT('Ctrl Pts',(-18.5014918306554,42.0157788328236,124.205833220851)) ;
#39709=CARTESIAN_POINT('Ctrl Pts',(-18.2745387789703,41.8357897524138,124.40432673796)) ;
#39710=CARTESIAN_POINT('Ctrl Pts',(-18.376872413352,42.0258336853796,124.035131663706)) ;
#39711=CARTESIAN_POINT('Ctrl Pts',(-18.1187665880274,41.8458446049698,124.190948411638)) ;
#39712=CARTESIAN_POINT('Ctrl Pts',(-18.285357700117,42.0356922676544,123.849131188738)) ;
#39713=CARTESIAN_POINT('Ctrl Pts',(-18.0043751833933,41.8557031872446,123.958446111425)) ;
#39714=CARTESIAN_POINT('Ctrl Pts',(-18.2261951447151,42.0457603970971,123.645935941914)) ;
#39715=CARTESIAN_POINT('Ctrl Pts',(-17.9304244939929,41.8657713166872,123.704451485335)) ;
#39716=CARTESIAN_POINT('Ctrl Pts',(-18.2037096295155,42.0556158687862,123.439949227679)) ;
#39717=CARTESIAN_POINT('Ctrl Pts',(-17.9023200740901,41.8756267883763,123.446967189867)) ;
#39718=CARTESIAN_POINT('Ctrl Pts',(-18.2168940215252,42.0656107171724,123.230246957662)) ;
#39719=CARTESIAN_POINT('Ctrl Pts',(-17.9188032302144,41.8856216367626,123.184839420301)) ;
#39720=CARTESIAN_POINT('Ctrl Pts',(-18.2669137943528,42.0756420139569,123.025370929616)) ;
#39721=CARTESIAN_POINT('Ctrl Pts',(-17.9813304618854,41.8956529335471,122.928744998812)) ;
#39722=CARTESIAN_POINT('Ctrl Pts',(-18.3500517364716,42.085508550167,122.835328127626)) ;
#39723=CARTESIAN_POINT('Ctrl Pts',(-18.085255518592,41.9055194697571,122.691192079441)) ;
#39724=CARTESIAN_POINT('Ctrl Pts',(-18.4660321364788,42.0954959731278,122.660329302149)) ;
#39725=CARTESIAN_POINT('Ctrl Pts',(-18.2302333322314,41.915506892718,122.472444933133)) ;
#39726=CARTESIAN_POINT('Ctrl Pts',(-18.6099789814412,42.1054409121476,122.508661371675)) ;
#39727=CARTESIAN_POINT('Ctrl Pts',(-18.4101690100721,41.9254518317378,122.282861709765)) ;
#39728=CARTESIAN_POINT('Ctrl Pts',(-18.7797885338698,42.1154857980076,122.383148139199)) ;
#39729=CARTESIAN_POINT('Ctrl Pts',(-18.6224325373826,41.9354967175978,122.125972345767)) ;
#39730=CARTESIAN_POINT('Ctrl Pts',(-18.9654610961427,42.1253543330938,122.290568762634)) ;
#39731=CARTESIAN_POINT('Ctrl Pts',(-18.8545248231333,41.945365252684,122.010250360276)) ;
#39732=CARTESIAN_POINT('Ctrl Pts',(-19.1661696006187,42.1353202011005,122.230497998175)) ;
#39733=CARTESIAN_POINT('Ctrl Pts',(-19.1054113849809,41.9553311206907,121.935164518656)) ;
#39734=CARTESIAN_POINT('Ctrl Pts',(-19.3754959713858,42.145342848553,122.206283829226)) ;
#39735=CARTESIAN_POINT('Ctrl Pts',(-19.3670697024501,41.9653537681432,121.904899528169)) ;
#39736=CARTESIAN_POINT('Ctrl Pts',(-19.5837472933625,42.1552664875606,122.218600651272)) ;
#39737=CARTESIAN_POINT('Ctrl Pts',(-19.6273839317771,41.9752774071507,121.920298317291)) ;
#39738=CARTESIAN_POINT('Ctrl Pts',(-19.7872248880091,42.1652092125663,122.266499710306)) ;
#39739=CARTESIAN_POINT('Ctrl Pts',(-19.8817304497054,41.9852201321565,121.980174899342)) ;
#39740=CARTESIAN_POINT('Ctrl Pts',(-19.98116015884,42.1752548186182,122.350078644094)) ;
#39741=CARTESIAN_POINT('Ctrl Pts',(-20.1241484577125,41.9952657382084,122.084651122063)) ;
#39742=CARTESIAN_POINT('Ctrl Pts',(-20.1545514692075,42.1851162411393,122.463760650406)) ;
#39743=CARTESIAN_POINT('Ctrl Pts',(-20.3408862917472,42.0051271607295,122.226756112428)) ;
#39744=CARTESIAN_POINT('Ctrl Pts',(-20.3078045675298,42.1951098095885,122.607431591005)) ;
#39745=CARTESIAN_POINT('Ctrl Pts',(-20.5324507968352,42.0151207291787,122.406346888333)) ;
#39746=CARTESIAN_POINT('Ctrl Pts',(-20.4330485966864,42.2050352803438,122.774367875557)) ;
#39747=CARTESIAN_POINT('Ctrl Pts',(-20.689003659768,42.025046199934,122.61501906144)) ;
#39748=CARTESIAN_POINT('Ctrl Pts',(-20.528359134433,42.2150629542996,122.96237648736)) ;
#39749=CARTESIAN_POINT('Ctrl Pts',(-20.808139363891,42.0350738738898,122.850031069937)) ;
#39750=CARTESIAN_POINT('Ctrl Pts',(-20.5889282022475,42.2249501323413,123.161244468246)) ;
#39751=CARTESIAN_POINT('Ctrl Pts',(-20.8838479742396,42.0449610519315,123.098617303738)) ;
#39752=CARTESIAN_POINT('Ctrl Pts',(-20.6145455202288,42.2349785117095,123.370482821943)) ;
#39753=CARTESIAN_POINT('Ctrl Pts',(-20.9158670632357,42.0549894312997,123.360164459765)) ;
#39754=CARTESIAN_POINT('Ctrl Pts',(-20.6037026584376,42.244872754431,123.57823145244)) ;
#39755=CARTESIAN_POINT('Ctrl Pts',(-20.9023097752642,42.0648836740212,123.619854631493)) ;
#39756=CARTESIAN_POINT('Ctrl Pts',(-20.5408518696117,42.2582256710819,123.851819040007)) ;
#39757=CARTESIAN_POINT('Ctrl Pts',(-20.8237470249791,42.078236590672,123.961816174776)) ;
#39758=CARTESIAN_POINT('Ctrl Pts',(-20.4095172303577,42.2714281888286,124.099989933585)) ;
#39759=CARTESIAN_POINT('Ctrl Pts',(-20.6595997815487,42.0914391084188,124.272009590698)) ;
#39760=CARTESIAN_POINT('Ctrl Pts',(-20.2186534632653,42.2847840941096,124.305832996325)) ;
#39761=CARTESIAN_POINT('Ctrl Pts',(-20.4209837963246,42.1047950136997,124.529355053703)) ;
#39762=CARTESIAN_POINT('Ctrl Pts',(-20.0529351292621,42.2946807427474,124.431692913237)) ;
#39763=CARTESIAN_POINT('Ctrl Pts',(-20.2138409515124,42.1146916623376,124.686668821031)) ;
#39764=CARTESIAN_POINT('Ctrl Pts',(-19.8651277354385,42.3047288807999,124.528356903845)) ;
#39765=CARTESIAN_POINT('Ctrl Pts',(-19.9790784983031,42.12473980039,124.807498749115)) ;
#39766=CARTESIAN_POINT('Ctrl Pts',(-19.6665158493402,42.3146198409776,124.58996703809)) ;
#39767=CARTESIAN_POINT('Ctrl Pts',(-19.7308134332354,42.1346307605678,124.884508093011)) ;
#39768=CARTESIAN_POINT('Ctrl Pts',(-19.4581683197363,42.3246126768544,124.616948547445)) ;
#39769=CARTESIAN_POINT('Ctrl Pts',(-19.4703782998124,42.1446235964446,124.918232356499)) ;
#39770=CARTESIAN_POINT('Ctrl Pts',(-19.2473681600248,42.334651771856,124.606814985885)) ;
#39771=CARTESIAN_POINT('Ctrl Pts',(-19.2068788945303,42.1546626914461,124.905562766007)) ;
#39772=CARTESIAN_POINT('Ctrl Pts',(-19.0455307327722,42.3444891277071,124.561634051858)) ;
#39773=CARTESIAN_POINT('Ctrl Pts',(-18.9545800921751,42.1645000472973,124.849083179749)) ;
#39774=CARTESIAN_POINT('Ctrl Pts',(-18.7855849758638,42.3578820756379,124.453519111834)) ;
#39775=CARTESIAN_POINT('Ctrl Pts',(-18.6296634518403,42.177892995228,124.713940021427)) ;
#39776=CARTESIAN_POINT('Ctrl Pts',(-18.5635083695273,42.3710487520648,124.282885771656)) ;
#39777=CARTESIAN_POINT('Ctrl Pts',(-18.3520925364805,42.191059671655,124.500678451759)) ;
#39778=CARTESIAN_POINT('Ctrl Pts',(-18.392149943478,42.3844335334716,124.059804324477)) ;
#39779=CARTESIAN_POINT('Ctrl Pts',(-18.1378563759375,42.2044444530618,124.221781306331)) ;
#39780=CARTESIAN_POINT('Ctrl Pts',(-18.2962255678194,42.3942953161154,123.875955923581)) ;
#39781=CARTESIAN_POINT('Ctrl Pts',(-18.0179616237047,42.2143062357056,123.991978653558)) ;
#39782=CARTESIAN_POINT('Ctrl Pts',(-18.2325120769393,42.4042944640685,123.675676595792)) ;
#39783=CARTESIAN_POINT('Ctrl Pts',(-17.9383202715921,42.2243053836587,123.741625973952)) ;
#39784=CARTESIAN_POINT('Ctrl Pts',(-18.2046075101168,42.4141972566856,123.469320833634)) ;
#39785=CARTESIAN_POINT('Ctrl Pts',(-17.9034419631951,42.2342081762757,123.483683307467)) ;
#39786=CARTESIAN_POINT('Ctrl Pts',(-18.2131324921205,42.4242468365765,123.258275057059)) ;
#39787=CARTESIAN_POINT('Ctrl Pts',(-17.9141036163892,42.2442577561667,123.21987047092)) ;
#39788=CARTESIAN_POINT('Ctrl Pts',(-18.271742279274,42.437433910386,122.987181315059)) ;
#39789=CARTESIAN_POINT('Ctrl Pts',(-17.9873542557703,42.2574448299761,122.881031053138)) ;
#39790=CARTESIAN_POINT('Ctrl Pts',(-18.4346521343874,42.4541867003572,122.670610361465)) ;
#39791=CARTESIAN_POINT('Ctrl Pts',(-18.1910268971843,42.2741976199474,122.485278257372)) ;
#39792=CARTESIAN_POINT('Ctrl Pts',(-18.6920409930995,42.4706753524519,122.432258546102)) ;
#39793=CARTESIAN_POINT('Ctrl Pts',(-18.5127023286891,42.2906862720421,122.187393477303)) ;
#39794=CARTESIAN_POINT('Ctrl Pts',(-18.9400618332129,42.4840321786353,122.300845882537)) ;
#39795=CARTESIAN_POINT('Ctrl Pts',(-18.8227825349373,42.3040430982254,122.02309131617)) ;
#39796=CARTESIAN_POINT('Ctrl Pts',(-19.1380453310715,42.4939285635132,122.236723926044)) ;
#39797=CARTESIAN_POINT('Ctrl Pts',(-19.0702507618839,42.3139394831034,121.942948929618)) ;
#39798=CARTESIAN_POINT('Ctrl Pts',(-19.346318954824,42.5039350780337,122.2075435774)) ;
#39799=CARTESIAN_POINT('Ctrl Pts',(-19.3305991664971,42.3239459976239,121.906474651772)) ;
#39800=CARTESIAN_POINT('Ctrl Pts',(-19.623580125889,42.5171252015501,122.216652416966)) ;
#39801=CARTESIAN_POINT('Ctrl Pts',(-19.6771578660566,42.3371361211402,121.917859655093)) ;
#39802=CARTESIAN_POINT('Ctrl Pts',(-19.9644761073968,42.5338917626996,122.32049383106)) ;
#39803=CARTESIAN_POINT('Ctrl Pts',(-20.1032957575769,42.3539026822898,122.047670197604)) ;
#39804=CARTESIAN_POINT('Ctrl Pts',(-20.3009572251947,42.5536762514077,122.573177848514)) ;
#39805=CARTESIAN_POINT('Ctrl Pts',(-20.5238873611749,42.3736871709978,122.363526340952)) ;
#39806=CARTESIAN_POINT('Ctrl Pts',(-20.5338536920251,42.5736216990041,122.927472083475)) ;
#39807=CARTESIAN_POINT('Ctrl Pts',(-20.8150059841299,42.3936326185943,122.806396279315)) ;
#39808=CARTESIAN_POINT('Ctrl Pts',(-20.6313376491033,42.5935333611601,123.339481760479)) ;
#39809=CARTESIAN_POINT('Ctrl Pts',(-20.936856534069,42.4135442807503,123.321408446945)) ;
#39810=CARTESIAN_POINT('Ctrl Pts',(-20.5833429972544,42.6134255531789,123.75977761235)) ;
#39811=CARTESIAN_POINT('Ctrl Pts',(-20.8768601174768,42.4334364727691,123.846776921261)) ;
#39812=CARTESIAN_POINT('Ctrl Pts',(-20.3928775516324,42.6334666837336,124.140904242147)) ;
#39813=CARTESIAN_POINT('Ctrl Pts',(-20.6387749465304,42.4534776033238,124.323184054262)) ;
#39814=CARTESIAN_POINT('Ctrl Pts',(-20.0872595412336,42.6532850183492,124.431171962633)) ;
#39815=CARTESIAN_POINT('Ctrl Pts',(-20.2567515624384,42.4732959379394,124.686015098772)) ;
#39816=CARTESIAN_POINT('Ctrl Pts',(-19.6984277741902,42.6732575835688,124.601563615224)) ;
#39817=CARTESIAN_POINT('Ctrl Pts',(-19.7707111217322,42.4932685031589,124.899002007954)) ;
#39818=CARTESIAN_POINT('Ctrl Pts',(-19.2762631710593,42.6931467997404,124.629052850656)) ;
#39819=CARTESIAN_POINT('Ctrl Pts',(-19.2430064355519,42.5131577193306,124.933361057045)) ;
#39820=CARTESIAN_POINT('Ctrl Pts',(-18.8676531896362,42.7131703740631,124.5098269493)) ;
#39821=CARTESIAN_POINT('Ctrl Pts',(-18.7322443545609,42.5331812936533,124.784326245824)) ;
#39822=CARTESIAN_POINT('Ctrl Pts',(-18.5278123839697,42.7329675371513,124.26130431907)) ;
#39823=CARTESIAN_POINT('Ctrl Pts',(-18.3074466868531,42.5529784567415,124.473672881687)) ;
#39824=CARTESIAN_POINT('Ctrl Pts',(-18.2904261749242,42.7529330309751,123.909466884417)) ;
#39825=CARTESIAN_POINT('Ctrl Pts',(-18.0107152100322,42.5729439505653,124.033875901422)) ;
#39826=CARTESIAN_POINT('Ctrl Pts',(-18.187872486649,42.7728867387165,123.49766130319)) ;
#39827=CARTESIAN_POINT('Ctrl Pts',(-17.8825244705075,42.5928976583067,123.519119143686)) ;
#39828=CARTESIAN_POINT('Ctrl Pts',(-18.2318581554824,42.7927941154431,123.076763552661)) ;
#39829=CARTESIAN_POINT('Ctrl Pts',(-17.937507467377,42.6128050350333,122.992998485327)) ;
#39830=CARTESIAN_POINT('Ctrl Pts',(-18.4153780545509,42.8126463269917,122.696553693905)) ;
#39831=CARTESIAN_POINT('Ctrl Pts',(-18.1669062691419,42.6326572465818,122.517738273544)) ;
#39832=CARTESIAN_POINT('Ctrl Pts',(-18.7212077898556,42.8327187139374,122.398884993394)) ;
#39833=CARTESIAN_POINT('Ctrl Pts',(-18.5491943142901,42.6527296335276,122.145651577416)) ;
#39834=CARTESIAN_POINT('Ctrl Pts',(-19.1059608983857,42.8525565835777,122.225998547386)) ;
#39835=CARTESIAN_POINT('Ctrl Pts',(-19.030133332195,42.6725675031678,121.929544757025)) ;
#39836=CARTESIAN_POINT('Ctrl Pts',(-19.526741490911,42.8724072381308,122.192939772244)) ;
#39837=CARTESIAN_POINT('Ctrl Pts',(-19.5561067931741,42.692418157721,121.888220022681)) ;
#39838=CARTESIAN_POINT('Ctrl Pts',(-19.9374721598721,42.8924591724712,122.307188454904)) ;
#39839=CARTESIAN_POINT('Ctrl Pts',(-20.0695211678487,42.7124700920614,122.031029897326)) ;
#39840=CARTESIAN_POINT('Ctrl Pts',(-20.2808472333612,42.9122923600373,122.552162407161)) ;
#39841=CARTESIAN_POINT('Ctrl Pts',(-20.4987389792861,42.7323032796275,122.337244880604)) ;
#39842=CARTESIAN_POINT('Ctrl Pts',(-20.5217209474624,42.932221572268,122.90060218186)) ;
#39843=CARTESIAN_POINT('Ctrl Pts',(-20.7998323715724,42.7522324918582,122.772792578449)) ;
#39844=CARTESIAN_POINT('Ctrl Pts',(-20.6295592118292,42.9521065374824,123.309594803802)) ;
#39845=CARTESIAN_POINT('Ctrl Pts',(-20.9346324232029,42.7721174570725,123.284031475308)) ;
#39846=CARTESIAN_POINT('Ctrl Pts',(-20.5903609500711,42.972180278627,123.734525663825)) ;
#39847=CARTESIAN_POINT('Ctrl Pts',(-20.8856369562463,42.7921911982171,123.815196128972)) ;
#39848=CARTESIAN_POINT('Ctrl Pts',(-20.4110322867297,42.9919734604074,124.115338189697)) ;
#39849=CARTESIAN_POINT('Ctrl Pts',(-20.6614795251778,42.8119843799976,124.29121080534)) ;
#39850=CARTESIAN_POINT('Ctrl Pts',(-20.1109437575518,43.0119361684101,124.415478901693)) ;
#39851=CARTESIAN_POINT('Ctrl Pts',(-20.2863715696401,42.8319470880002,124.66638895846)) ;
#39852=CARTESIAN_POINT('Ctrl Pts',(-19.7255846738428,43.0319191201525,124.594466908089)) ;
#39853=CARTESIAN_POINT('Ctrl Pts',(-19.8046741907644,42.8519300397427,124.89012675408)) ;
#39854=CARTESIAN_POINT('Ctrl Pts',(-19.3059710828873,43.0517297399247,124.631722413805)) ;
#39855=CARTESIAN_POINT('Ctrl Pts',(-19.2801592562406,42.8717406595148,124.936699673611)) ;
#39856=CARTESIAN_POINT('Ctrl Pts',(-18.8952733972345,43.0717134559576,124.523123476909)) ;
#39857=CARTESIAN_POINT('Ctrl Pts',(-18.7667862152557,42.8917243755477,124.800954951292)) ;
#39858=CARTESIAN_POINT('Ctrl Pts',(-18.547948160276,43.0915949198549,124.281962291053)) ;
#39859=CARTESIAN_POINT('Ctrl Pts',(-18.3326279856104,42.9116058394451,124.499507379854)) ;
#39860=CARTESIAN_POINT('Ctrl Pts',(-18.3027271825646,43.1115502496993,123.935800002761)) ;
#39861=CARTESIAN_POINT('Ctrl Pts',(-18.0260984755264,42.9315611692895,124.06680718518)) ;
#39862=CARTESIAN_POINT('Ctrl Pts',(-18.1904651269619,43.1314257105047,123.528307608364)) ;
#39863=CARTESIAN_POINT('Ctrl Pts',(-17.8857662259609,42.9514366300949,123.557444062355)) ;
#39864=CARTESIAN_POINT('Ctrl Pts',(-18.2239197601607,43.1514100305563,123.104753802092)) ;
#39865=CARTESIAN_POINT('Ctrl Pts',(-17.9275815085421,42.9714209501464,123.027999899629)) ;
#39866=CARTESIAN_POINT('Ctrl Pts',(-18.3996847638181,43.1713380633459,122.719094804955)) ;
#39867=CARTESIAN_POINT('Ctrl Pts',(-18.1472767537008,42.9913489829361,122.545930346228)) ;
#39868=CARTESIAN_POINT('Ctrl Pts',(-18.646890943322,43.1879468252857,122.467036487721)) ;
#39869=CARTESIAN_POINT('Ctrl Pts',(-18.4563016259039,43.0079577448759,122.230836526312)) ;
#39870=CARTESIAN_POINT('Ctrl Pts',(-18.8854093868125,43.2011344639758,122.325626761766)) ;
#39871=CARTESIAN_POINT('Ctrl Pts',(-18.754428778719,43.021145383566,122.054087877061)) ;
#39872=CARTESIAN_POINT('Ctrl Pts',(-19.0816631258239,43.2111208983359,122.25109404408)) ;
#39873=CARTESIAN_POINT('Ctrl Pts',(-18.9997521034585,43.0311318179261,121.960916807057)) ;
#39874=CARTESIAN_POINT('Ctrl Pts',(-19.2884287473412,43.2211302722953,122.211885729769)) ;
#39875=CARTESIAN_POINT('Ctrl Pts',(-19.2581944108734,43.0411411918854,121.911902702799)) ;
#39876=CARTESIAN_POINT('Ctrl Pts',(-19.5677559979308,43.2344203058605,122.208091123803)) ;
#39877=CARTESIAN_POINT('Ctrl Pts',(-19.6074202778516,43.0544312254507,121.907165841885)) ;
#39878=CARTESIAN_POINT('Ctrl Pts',(-19.9099408495608,43.251014293523,122.294450351363)) ;
#39879=CARTESIAN_POINT('Ctrl Pts',(-20.035068776761,43.0710252131132,122.015093622718)) ;
#39880=CARTESIAN_POINT('Ctrl Pts',(-20.2026638187543,43.2676465487985,122.492780810066)) ;
#39881=CARTESIAN_POINT('Ctrl Pts',(-20.4010277794192,43.0876574683887,122.26302842481)) ;
#39882=CARTESIAN_POINT('Ctrl Pts',(-20.3849853860425,43.2808889324664,122.703218028358)) ;
#39883=CARTESIAN_POINT('Ctrl Pts',(-20.6289019817708,43.1008998520566,122.526052209326)) ;
#39884=CARTESIAN_POINT('Ctrl Pts',(-20.4925880976511,43.2908031406938,122.881725152075)) ;
#39885=CARTESIAN_POINT('Ctrl Pts',(-20.7634137016277,43.110814060284,122.74918883152)) ;
#39886=CARTESIAN_POINT('Ctrl Pts',(-20.5684111030146,43.3008597799655,123.079068387712)) ;
#39887=CARTESIAN_POINT('Ctrl Pts',(-20.8581936478077,43.1208706995557,122.995865179675)) ;
#39888=CARTESIAN_POINT('Ctrl Pts',(-20.6082199665284,43.3107055863856,123.282209920598)) ;
#39889=CARTESIAN_POINT('Ctrl Pts',(-20.9079570488716,43.1307165059758,123.249794573019)) ;
#39890=CARTESIAN_POINT('Ctrl Pts',(-20.6125910585015,43.3207505860188,123.493341268355)) ;
#39891=CARTESIAN_POINT('Ctrl Pts',(-20.9134264775724,43.140761505609,123.513697714183)) ;
#39892=CARTESIAN_POINT('Ctrl Pts',(-20.569416287465,43.3340316083915,123.769136883137)) ;
#39893=CARTESIAN_POINT('Ctrl Pts',(-20.8594473357506,43.1540425279817,123.858497845356)) ;
#39894=CARTESIAN_POINT('Ctrl Pts',(-20.4566616002104,43.3472290549162,124.026134355986)) ;
#39895=CARTESIAN_POINT('Ctrl Pts',(-20.7185081963273,43.1672399745064,124.17971260663)) ;
#39896=CARTESIAN_POINT('Ctrl Pts',(-20.2801208783856,43.3606433527231,124.246084172849)) ;
#39897=CARTESIAN_POINT('Ctrl Pts',(-20.4978485963145,43.1806542723133,124.454637161289)) ;
#39898=CARTESIAN_POINT('Ctrl Pts',(-20.1246767207839,43.3704824181259,124.382563644853)) ;
#39899=CARTESIAN_POINT('Ctrl Pts',(-20.3035425807925,43.1904933377161,124.625241624107)) ;
#39900=CARTESIAN_POINT('Ctrl Pts',(-19.9456198245211,43.3804656244036,124.492010358693)) ;
#39901=CARTESIAN_POINT('Ctrl Pts',(-20.0797235876793,43.2004765439937,124.762051652088)) ;
#39902=CARTESIAN_POINT('Ctrl Pts',(-19.7508481450483,43.3904168593164,124.568404517536)) ;
#39903=CARTESIAN_POINT('Ctrl Pts',(-19.8362597617157,43.2104277789065,124.857547214576)) ;
#39904=CARTESIAN_POINT('Ctrl Pts',(-19.5447971219931,43.400417859018,124.610275376094)) ;
#39905=CARTESIAN_POINT('Ctrl Pts',(-19.5786965198852,43.2204287786082,124.909888505261)) ;
#39906=CARTESIAN_POINT('Ctrl Pts',(-19.3339717832248,43.4104492048053,124.615418235309)) ;
#39907=CARTESIAN_POINT('Ctrl Pts',(-19.3151648430012,43.2304601243955,124.916319914213)) ;
#39908=CARTESIAN_POINT('Ctrl Pts',(-19.1290970717957,43.4203029695104,124.584716305653)) ;
#39909=CARTESIAN_POINT('Ctrl Pts',(-19.0590709276803,43.2403138891005,124.877945266939)) ;
#39910=CARTESIAN_POINT('Ctrl Pts',(-18.9302029392523,43.4302736231787,124.518609768227)) ;
#39911=CARTESIAN_POINT('Ctrl Pts',(-18.8104522662842,43.2502845427688,124.795314724082)) ;
#39912=CARTESIAN_POINT('Ctrl Pts',(-18.7452726680142,43.4402708668359,124.418674434814)) ;
#39913=CARTESIAN_POINT('Ctrl Pts',(-18.579288025875,43.2602817864261,124.670397983548)) ;
#39914=CARTESIAN_POINT('Ctrl Pts',(-18.5801137359114,43.4503043227801,124.28749236113)) ;
#39915=CARTESIAN_POINT('Ctrl Pts',(-18.3728375783014,43.2703152423702,124.506422572579)) ;
#39916=CARTESIAN_POINT('Ctrl Pts',(-18.4424457993828,43.4601598270805,124.132620980022)) ;
#39917=CARTESIAN_POINT('Ctrl Pts',(-18.2007504133427,43.2801707466707,124.312835032827)) ;
#39918=CARTESIAN_POINT('Ctrl Pts',(-18.3319639426538,43.4701592633666,123.953818397867)) ;
#39919=CARTESIAN_POINT('Ctrl Pts',(-18.0626456728445,43.2901701829567,124.089333194089)) ;
#39920=CARTESIAN_POINT('Ctrl Pts',(-18.2547737206712,43.4800537228825,123.760615819088)) ;
#39921=CARTESIAN_POINT('Ctrl Pts',(-17.9661552349322,43.3000646424727,123.847830754012)) ;
#39922=CARTESIAN_POINT('Ctrl Pts',(-18.2116553133487,43.4901168423341,123.553535266331)) ;
#39923=CARTESIAN_POINT('Ctrl Pts',(-17.912254517231,43.3101277619243,123.58898066156)) ;
#39924=CARTESIAN_POINT('Ctrl Pts',(-18.2050619663453,43.4999564767461,123.346745963906)) ;
#39925=CARTESIAN_POINT('Ctrl Pts',(-17.9040100748789,43.3199673963363,123.330493713349)) ;
#39926=CARTESIAN_POINT('Ctrl Pts',(-18.23486765756,43.5100196842319,123.137325469672)) ;
#39927=CARTESIAN_POINT('Ctrl Pts',(-17.9412644854558,43.3300306038221,123.068717754893)) ;
#39928=CARTESIAN_POINT('Ctrl Pts',(-18.2996597954055,43.5199137916111,122.939643533093)) ;
#39929=CARTESIAN_POINT('Ctrl Pts',(-18.0222521550485,43.3399247112013,122.821614169034)) ;
#39930=CARTESIAN_POINT('Ctrl Pts',(-18.3977518129424,43.5298561238035,122.755103321263)) ;
#39931=CARTESIAN_POINT('Ctrl Pts',(-18.1448649356919,43.3498670433936,122.590937416145)) ;
#39932=CARTESIAN_POINT('Ctrl Pts',(-18.5271067731501,43.5398567501185,122.589320233305)) ;
#39933=CARTESIAN_POINT('Ctrl Pts',(-18.3065565945631,43.3598676697087,122.383706851655)) ;
#39934=CARTESIAN_POINT('Ctrl Pts',(-18.6841488510847,43.5498984844004,122.448264779539)) ;
#39935=CARTESIAN_POINT('Ctrl Pts',(-18.5028573530052,43.3699094039905,122.207385535519)) ;
#39936=CARTESIAN_POINT('Ctrl Pts',(-18.8592239504986,43.5597239103495,122.33861707734)) ;
#39937=CARTESIAN_POINT('Ctrl Pts',(-18.7217003533582,43.3797348299397,122.070323331538)) ;
#39938=CARTESIAN_POINT('Ctrl Pts',(-19.0550398152044,43.5697807368771,122.258927424476)) ;
#39939=CARTESIAN_POINT('Ctrl Pts',(-18.9664691272674,43.3897916564673,121.9707088847)) ;
#39940=CARTESIAN_POINT('Ctrl Pts',(-19.2591461901148,43.5797081699987,122.215302018421)) ;
#39941=CARTESIAN_POINT('Ctrl Pts',(-19.221601860933,43.3997190895889,121.916174469937)) ;
#39942=CARTESIAN_POINT('Ctrl Pts',(-19.4681756382475,43.5896581624049,122.207163663793)) ;
#39943=CARTESIAN_POINT('Ctrl Pts',(-19.482888856262,43.4096690819951,121.905998966788)) ;
#39944=CARTESIAN_POINT('Ctrl Pts',(-19.6775616742312,43.5997133634789,122.236109466576)) ;
#39945=CARTESIAN_POINT('Ctrl Pts',(-19.7446216548222,43.4197242830691,121.94217861372)) ;
#39946=CARTESIAN_POINT('Ctrl Pts',(-19.874223881596,43.6095356375312,122.299123887037)) ;
#39947=CARTESIAN_POINT('Ctrl Pts',(-19.990450932251,43.4295465571214,122.020944452107)) ;
#39948=CARTESIAN_POINT('Ctrl Pts',(-20.0614519230175,43.6195915314905,122.397267586826)) ;
#39949=CARTESIAN_POINT('Ctrl Pts',(-20.2244870381209,43.4396024510806,122.1436218314)) ;
#39950=CARTESIAN_POINT('Ctrl Pts',(-20.2266685259505,43.6295322533356,122.525258130833)) ;
#39951=CARTESIAN_POINT('Ctrl Pts',(-20.4310096168691,43.4495431729258,122.303608199014)) ;
#39952=CARTESIAN_POINT('Ctrl Pts',(-20.3671176125788,43.6394365974222,122.678983059671)) ;
#39953=CARTESIAN_POINT('Ctrl Pts',(-20.6065731184641,43.4594475170124,122.495763120435)) ;
#39954=CARTESIAN_POINT('Ctrl Pts',(-20.4802208408433,43.6494832647217,122.857339300403)) ;
#39955=CARTESIAN_POINT('Ctrl Pts',(-20.7479541653206,43.4694941843119,122.718707024685)) ;
#39956=CARTESIAN_POINT('Ctrl Pts',(-20.5596229425746,43.6593788231716,123.049662217343)) ;
#39957=CARTESIAN_POINT('Ctrl Pts',(-20.8472092356636,43.4793897427618,122.959110289746)) ;
#39958=CARTESIAN_POINT('Ctrl Pts',(-20.6051653987093,43.6694409018763,123.256207404328)) ;
#39959=CARTESIAN_POINT('Ctrl Pts',(-20.904139618106,43.4894518214665,123.217291078414)) ;
#39960=CARTESIAN_POINT('Ctrl Pts',(-20.614077706757,43.6792836003421,123.462962817774)) ;
#39961=CARTESIAN_POINT('Ctrl Pts',(-20.9152824167308,43.4992945199322,123.475736104281)) ;
#39962=CARTESIAN_POINT('Ctrl Pts',(-20.587046897207,43.6892743742365,123.671227339976)) ;
#39963=CARTESIAN_POINT('Ctrl Pts',(-20.8814961281011,43.5092852938267,123.736067222358)) ;
#39964=CARTESIAN_POINT('Ctrl Pts',(-20.5246153399661,43.6992022434715,123.870395640026)) ;
#39965=CARTESIAN_POINT('Ctrl Pts',(-20.8034587033773,43.5192131630616,123.985028739418)) ;
#39966=CARTESIAN_POINT('Ctrl Pts',(-20.4282901507528,43.7091909724413,124.0570066794)) ;
#39967=CARTESIAN_POINT('Ctrl Pts',(-20.6830540647479,43.5292018920315,124.218293703529)) ;
#39968=CARTESIAN_POINT('Ctrl Pts',(-20.300083088921,43.7192303744251,124.224651641945)) ;
#39969=CARTESIAN_POINT('Ctrl Pts',(-20.5227971111526,43.5392412940152,124.427851205547)) ;
#39970=CARTESIAN_POINT('Ctrl Pts',(-20.1480587442798,43.7290705421618,124.364969335422)) ;
#39971=CARTESIAN_POINT('Ctrl Pts',(-20.3327674227831,43.549081461752,124.603250592151)) ;
#39972=CARTESIAN_POINT('Ctrl Pts',(-19.9704841404498,43.7391187525363,124.479372090359)) ;
#39973=CARTESIAN_POINT('Ctrl Pts',(-20.1108004287788,43.5591296721265,124.746255706774)) ;
#39974=CARTESIAN_POINT('Ctrl Pts',(-19.7775615457972,43.7490659228241,124.560080673461)) ;
#39975=CARTESIAN_POINT('Ctrl Pts',(-19.8696476489061,43.5690768424143,124.847143607125)) ;
#39976=CARTESIAN_POINT('Ctrl Pts',(-19.5744358323149,43.7589767710792,124.606507407475)) ;
#39977=CARTESIAN_POINT('Ctrl Pts',(-19.6157403076498,43.5789876906694,124.905179129391)) ;
#39978=CARTESIAN_POINT('Ctrl Pts',(-19.3632888752703,43.7690330987569,124.616913341482)) ;
#39979=CARTESIAN_POINT('Ctrl Pts',(-19.3518069355722,43.5890440183471,124.918188595458)) ;
#39980=CARTESIAN_POINT('Ctrl Pts',(-19.1577934192907,43.7788835115255,124.591215482131)) ;
#39981=CARTESIAN_POINT('Ctrl Pts',(-19.0949363387269,43.5988944311156,124.886068138091)) ;
#39982=CARTESIAN_POINT('Ctrl Pts',(-18.9561968908211,43.7889103973592,124.529628376844)) ;
#39983=CARTESIAN_POINT('Ctrl Pts',(-18.8429401698884,43.6089213169493,124.809086046487)) ;
#39984=CARTESIAN_POINT('Ctrl Pts',(-18.7685615510423,43.79893901299,124.433463237905)) ;
#39985=CARTESIAN_POINT('Ctrl Pts',(-18.6083951336162,43.6189499325802,124.688881455455)) ;
#39986=CARTESIAN_POINT('Ctrl Pts',(-18.6033288718835,43.8087842363675,124.30883132978)) ;
#39987=CARTESIAN_POINT('Ctrl Pts',(-18.4018522456161,43.6287951559577,124.533092420039)) ;
#39988=CARTESIAN_POINT('Ctrl Pts',(-18.4597378892454,43.8187749184691,124.155537858628)) ;
#39989=CARTESIAN_POINT('Ctrl Pts',(-18.222362119769,43.6387858380593,124.341476622119)) ;
#39990=CARTESIAN_POINT('Ctrl Pts',(-18.3448008532577,43.8288128071015,123.978559187435)) ;
#39991=CARTESIAN_POINT('Ctrl Pts',(-18.0786893212489,43.6488237266917,124.120254417856)) ;
#39992=CARTESIAN_POINT('Ctrl Pts',(-18.2635921715876,43.8386571422047,123.78819018194)) ;
#39993=CARTESIAN_POINT('Ctrl Pts',(-17.9771763876503,43.6586680617949,123.882292776762)) ;
#39994=CARTESIAN_POINT('Ctrl Pts',(-18.2156072803135,43.8486421044022,123.583862375105)) ;
#39995=CARTESIAN_POINT('Ctrl Pts',(-17.9171936283301,43.6686530239924,123.626883148395)) ;
#39996=CARTESIAN_POINT('Ctrl Pts',(-18.2037829776996,43.8585810459356,123.375218987753)) ;
#39997=CARTESIAN_POINT('Ctrl Pts',(-17.9024116243898,43.6785919655257,123.366078461574)) ;
#39998=CARTESIAN_POINT('Ctrl Pts',(-18.2286806326614,43.868622930907,123.165600430253)) ;
#39999=CARTESIAN_POINT('Ctrl Pts',(-17.9335320665927,43.6886338504972,123.104055220475)) ;
#40000=CARTESIAN_POINT('Ctrl Pts',(-18.2885381500914,43.8785094788153,122.96653880576)) ;
#40001=CARTESIAN_POINT('Ctrl Pts',(-18.008352723636,43.6985203984054,122.855226846707)) ;
#40002=CARTESIAN_POINT('Ctrl Pts',(-18.3827677761836,43.8885034043153,122.778780845212)) ;
#40003=CARTESIAN_POINT('Ctrl Pts',(-18.1261385187885,43.7085143239054,122.62052857553)) ;
#40004=CARTESIAN_POINT('Ctrl Pts',(-18.507397260208,43.8984394954417,122.611106118602)) ;
#40005=CARTESIAN_POINT('Ctrl Pts',(-18.2819245676368,43.7184504150319,122.410933845999)) ;
#40006=CARTESIAN_POINT('Ctrl Pts',(-18.6606561201383,43.9084687644217,122.466343302757)) ;
#40007=CARTESIAN_POINT('Ctrl Pts',(-18.4734970875325,43.7284796840119,122.229979319917)) ;
#40008=CARTESIAN_POINT('Ctrl Pts',(-18.8340470507955,43.918351146981,122.351835718989)) ;
#40009=CARTESIAN_POINT('Ctrl Pts',(-18.690235843168,43.7383620665712,122.08684314791)) ;
#40010=CARTESIAN_POINT('Ctrl Pts',(-19.0278824329128,43.9284036640689,122.267711760247)) ;
#40011=CARTESIAN_POINT('Ctrl Pts',(-18.9325293092755,43.748414583659,121.981687073704)) ;
#40012=CARTESIAN_POINT('Ctrl Pts',(-19.2301849856646,43.9382977848928,122.219177390576)) ;
#40013=CARTESIAN_POINT('Ctrl Pts',(-19.1854080916238,43.7583087044829,121.92101763461)) ;
#40014=CARTESIAN_POINT('Ctrl Pts',(-19.441298301709,43.9483597643132,122.206244667768)) ;
#40015=CARTESIAN_POINT('Ctrl Pts',(-19.4492993318435,43.7683706839034,121.904850471497)) ;
#40016=CARTESIAN_POINT('Ctrl Pts',(-19.6469435683342,43.9582042975421,122.229626514128)) ;
#40017=CARTESIAN_POINT('Ctrl Pts',(-19.7063573702786,43.7782152171323,121.934076662978)) ;
#40018=CARTESIAN_POINT('Ctrl Pts',(-19.8479372841435,43.9681643764484,122.288322728641)) ;
#40019=CARTESIAN_POINT('Ctrl Pts',(-19.9576002327709,43.7881752960385,122.007446102403)) ;
#40020=CARTESIAN_POINT('Ctrl Pts',(-20.0369708079469,43.978202653021,122.38212312448)) ;
#40021=CARTESIAN_POINT('Ctrl Pts',(-20.1938925037077,43.7982135726111,122.124695495062)) ;
#40022=CARTESIAN_POINT('Ctrl Pts',(-20.2043238205213,43.9880760395588,122.504967849574)) ;
#40023=CARTESIAN_POINT('Ctrl Pts',(-20.4030852669938,43.808086959149,122.27825126005)) ;
#40024=CARTESIAN_POINT('Ctrl Pts',(-20.3506106823668,43.9981489823259,122.658028324524)) ;
#40025=CARTESIAN_POINT('Ctrl Pts',(-20.5859442922176,43.8181599019161,122.469575837345)) ;
#40026=CARTESIAN_POINT('Ctrl Pts',(-20.465419038605,44.0079703964542,122.82969122843)) ;
#40027=CARTESIAN_POINT('Ctrl Pts',(-20.7294563689263,43.8279813160444,122.684155238278)) ;
#40028=CARTESIAN_POINT('Ctrl Pts',(-20.5510249351871,44.0180450265265,123.023378752783)) ;
#40029=CARTESIAN_POINT('Ctrl Pts',(-20.836464323358,43.8380559461167,122.926263897457)) ;
#40030=CARTESIAN_POINT('Ctrl Pts',(-20.6005844279953,44.0279116638434,123.224825343159)) ;
#40031=CARTESIAN_POINT('Ctrl Pts',(-20.8984148213761,43.8479225834336,123.178073112057)) ;
#40032=CARTESIAN_POINT('Ctrl Pts',(-20.6151706977744,44.0379352092152,123.435036739168)) ;
#40033=CARTESIAN_POINT('Ctrl Pts',(-20.9166483133652,43.8579461288053,123.440837266539)) ;
#40034=CARTESIAN_POINT('Ctrl Pts',(-20.5925229977775,44.0479609607324,123.644602262895)) ;
#40035=CARTESIAN_POINT('Ctrl Pts',(-20.8883395524588,43.8679718803225,123.702794177779)) ;
#40036=CARTESIAN_POINT('Ctrl Pts',(-20.5351790535078,44.0578145477417,123.843648615532)) ;
#40037=CARTESIAN_POINT('Ctrl Pts',(-20.8166599480238,43.8778254673319,123.951603594753)) ;
#40038=CARTESIAN_POINT('Ctrl Pts',(-20.4434995838773,44.0677915079697,124.032303037785)) ;
#40039=CARTESIAN_POINT('Ctrl Pts',(-20.7020609237205,43.8878024275598,124.187422142882)) ;
#40040=CARTESIAN_POINT('Ctrl Pts',(-20.3196315257472,44.0778126509981,124.202704231129)) ;
#40041=CARTESIAN_POINT('Ctrl Pts',(-20.5472263848323,43.8978235705883,124.400424003593)) ;
#40042=CARTESIAN_POINT('Ctrl Pts',(-20.1704166426939,44.0876952570181,124.347313905858)) ;
#40043=CARTESIAN_POINT('Ctrl Pts',(-20.3607073266123,43.9077061766083,124.581187205832)) ;
#40044=CARTESIAN_POINT('Ctrl Pts',(-19.9951290913081,44.0977637276508,124.465904961827)) ;
#40045=CARTESIAN_POINT('Ctrl Pts',(-20.1415985165623,43.9177746472409,124.729426223208)) ;
#40046=CARTESIAN_POINT('Ctrl Pts',(-19.8065219734023,44.1075938108345,124.550461991308)) ;
#40047=CARTESIAN_POINT('Ctrl Pts',(-19.9058383855196,43.9276047304247,124.835123522577)) ;
#40048=CARTESIAN_POINT('Ctrl Pts',(-19.6014110884651,44.1176603705148,124.602451546472)) ;
#40049=CARTESIAN_POINT('Ctrl Pts',(-19.6494502413874,43.937671290105,124.900110672146)) ;
#40050=CARTESIAN_POINT('Ctrl Pts',(-19.3940171097119,44.1275506203441,124.617639758843)) ;
#40051=CARTESIAN_POINT('Ctrl Pts',(-19.3902067493434,43.9475615399342,124.919096378377)) ;
#40052=CARTESIAN_POINT('Ctrl Pts',(-19.1849952546928,44.1375427860929,124.596831802444)) ;
#40053=CARTESIAN_POINT('Ctrl Pts',(-19.1289291993342,43.957553705683,124.893086594039)) ;
#40054=CARTESIAN_POINT('Ctrl Pts',(-18.9834025895948,44.147505629689,124.540019916616)) ;
#40055=CARTESIAN_POINT('Ctrl Pts',(-18.8769378575114,43.9675165492791,124.822071867024)) ;
#40056=CARTESIAN_POINT('Ctrl Pts',(-18.7955966982782,44.1574097985167,124.450071701931)) ;
#40057=CARTESIAN_POINT('Ctrl Pts',(-18.6421796236428,43.9774207181069,124.709636239005)) ;
#40058=CARTESIAN_POINT('Ctrl Pts',(-18.6237306354897,44.1674706734111,124.326834768521)) ;
#40059=CARTESIAN_POINT('Ctrl Pts',(-18.427347259584,43.9874815930013,124.555590382831)) ;
#40060=CARTESIAN_POINT('Ctrl Pts',(-18.4788866563946,44.1773095767404,124.179124043168)) ;
#40061=CARTESIAN_POINT('Ctrl Pts',(-18.246291241733,43.9973204963306,124.370950929474)) ;
#40062=CARTESIAN_POINT('Ctrl Pts',(-18.3590318669185,44.1873779531143,124.004699120229)) ;
#40063=CARTESIAN_POINT('Ctrl Pts',(-18.0964730403445,44.0073888727045,124.152920066844)) ;
#40064=CARTESIAN_POINT('Ctrl Pts',(-18.2729573990922,44.197258569747,123.815617005926)) ;
#40065=CARTESIAN_POINT('Ctrl Pts',(-17.9888795242081,44.0172694893372,123.916566377158)) ;
#40066=CARTESIAN_POINT('Ctrl Pts',(-18.2200454094595,44.207249729976,123.612376766819)) ;
#40067=CARTESIAN_POINT('Ctrl Pts',(-17.9227396808908,44.0272606495662,123.662515814655)) ;
#40068=CARTESIAN_POINT('Ctrl Pts',(-18.2032518304312,44.2172028034081,123.403775478978)) ;
#40069=CARTESIAN_POINT('Ctrl Pts',(-17.901747886527,44.0372137229982,123.40176367561)) ;
#40070=CARTESIAN_POINT('Ctrl Pts',(-18.2231612060629,44.2272386390207,123.19374932302)) ;
#40071=CARTESIAN_POINT('Ctrl Pts',(-17.9266347799098,44.0472495586109,123.139231148723)) ;
#40072=CARTESIAN_POINT('Ctrl Pts',(-18.2782926365655,44.2371287657509,122.993256824972)) ;
#40073=CARTESIAN_POINT('Ctrl Pts',(-17.9955495885847,44.0571396853411,122.888614558042)) ;
#40074=CARTESIAN_POINT('Ctrl Pts',(-18.368002893643,44.2471209475202,122.803320931818)) ;
#40075=CARTESIAN_POINT('Ctrl Pts',(-18.1076878439649,44.0671318671104,122.651194666608)) ;
#40076=CARTESIAN_POINT('Ctrl Pts',(-18.4888319440295,44.2570668874946,122.632672480447)) ;
#40077=CARTESIAN_POINT('Ctrl Pts',(-18.2587247866169,44.0770778070848,122.437883820096)) ;
#40078=CARTESIAN_POINT('Ctrl Pts',(-18.6371833756394,44.2670140712541,122.485268515715)) ;
#40079=CARTESIAN_POINT('Ctrl Pts',(-18.4441648499468,44.0870249908443,122.253628827134)) ;
#40080=CARTESIAN_POINT('Ctrl Pts',(-18.810735082372,44.2770620095444,122.364857154366)) ;
#40081=CARTESIAN_POINT('Ctrl Pts',(-18.6611045195104,44.0970729291346,122.1031151175)) ;
#40082=CARTESIAN_POINT('Ctrl Pts',(-18.9986676053786,44.286909644358,122.278010090229)) ;
#40083=CARTESIAN_POINT('Ctrl Pts',(-18.8960216519276,44.1069205639482,121.994556148526)) ;
#40084=CARTESIAN_POINT('Ctrl Pts',(-19.2009643648431,44.296871358056,122.223868979964)) ;
#40085=CARTESIAN_POINT('Ctrl Pts',(-19.1488932353509,44.1168822776461,121.92688036903)) ;
#40086=CARTESIAN_POINT('Ctrl Pts',(-19.4110368321455,44.3068999938771,122.205817721847)) ;
#40087=CARTESIAN_POINT('Ctrl Pts',(-19.4114837782063,44.1269109134673,121.90431694798)) ;
#40088=CARTESIAN_POINT('Ctrl Pts',(-19.6185576126464,44.3168103086289,122.224226084689)) ;
#40089=CARTESIAN_POINT('Ctrl Pts',(-19.6708855677845,44.1368212282191,121.927328148296)) ;
#40090=CARTESIAN_POINT('Ctrl Pts',(-19.8203871123028,44.3267451792916,122.277995841482)) ;
#40091=CARTESIAN_POINT('Ctrl Pts',(-19.9231728540548,44.1467560988817,121.994541369451)) ;
#40092=CARTESIAN_POINT('Ctrl Pts',(-20.0117417687553,44.3367863616933,122.367111250582)) ;
#40093=CARTESIAN_POINT('Ctrl Pts',(-20.1623656623035,44.1567972812835,122.105936279565)) ;
#40094=CARTESIAN_POINT('Ctrl Pts',(-20.182178194294,44.3466733331581,122.48611803753)) ;
#40095=CARTESIAN_POINT('Ctrl Pts',(-20.3754115588307,44.1666842527482,122.254696080768)) ;
#40096=CARTESIAN_POINT('Ctrl Pts',(-20.3311931711049,44.3566727654207,122.634359060664)) ;
#40097=CARTESIAN_POINT('Ctrl Pts',(-20.5616797006855,44.1766836850109,122.439998156189)) ;
#40098=CARTESIAN_POINT('Ctrl Pts',(-20.4513895888392,44.3665928306773,122.804819406772)) ;
#40099=CARTESIAN_POINT('Ctrl Pts',(-20.7119248210621,44.1866037502675,122.653074789984)) ;
#40100=CARTESIAN_POINT('Ctrl Pts',(-20.5412304164301,44.3766296832615,122.995731464311)) ;
#40101=CARTESIAN_POINT('Ctrl Pts',(-20.8242248480823,44.1966406028516,122.891715161763)) ;
#40102=CARTESIAN_POINT('Ctrl Pts',(-20.5958716500195,44.3865423426014,123.196839523156)) ;
#40103=CARTESIAN_POINT('Ctrl Pts',(-20.8925256089118,44.2065532621916,123.143101297564)) ;
#40104=CARTESIAN_POINT('Ctrl Pts',(-20.6153694128764,44.3965335545164,123.405991946571)) ;
#40105=CARTESIAN_POINT('Ctrl Pts',(-20.9168966358172,44.2165444741065,123.404542148438)) ;
#40106=CARTESIAN_POINT('Ctrl Pts',(-20.5976979683511,44.4065751959195,123.616341273831)) ;
#40107=CARTESIAN_POINT('Ctrl Pts',(-20.8948063198031,44.2265861155096,123.667478543091)) ;
#40108=CARTESIAN_POINT('Ctrl Pts',(-20.54540602134,44.4164039901265,123.816275966712)) ;
#40109=CARTESIAN_POINT('Ctrl Pts',(-20.8294398408102,44.2364149097167,123.917397996008)) ;
#40110=CARTESIAN_POINT('Ctrl Pts',(-20.4571322193429,44.4264804012478,124.008799381337)) ;
#40111=CARTESIAN_POINT('Ctrl Pts',(-20.7190966285522,44.2464913208379,124.158051348359)) ;
#40112=CARTESIAN_POINT('Ctrl Pts',(-20.3394898621036,44.4363325342902,124.179323371872)) ;
#40113=CARTESIAN_POINT('Ctrl Pts',(-20.5720419187285,44.2563434538804,124.371206621311)) ;
#40114=CARTESIAN_POINT('Ctrl Pts',(-20.1909447204641,44.4464057686315,124.330210550994)) ;
#40115=CARTESIAN_POINT('Ctrl Pts',(-20.3863598083337,44.2664166882217,124.559814357992)) ;
#40116=CARTESIAN_POINT('Ctrl Pts',(-20.0223534222565,44.4562472699582,124.450168274092)) ;
#40117=CARTESIAN_POINT('Ctrl Pts',(-20.1756188493181,44.2762581895484,124.709761183262)) ;
#40118=CARTESIAN_POINT('Ctrl Pts',(-19.8335848822427,44.466208221553,124.540812132209)) ;
#40119=CARTESIAN_POINT('Ctrl Pts',(-19.9396571120526,44.2862191411431,124.823064731711)) ;
#40120=CARTESIAN_POINT('Ctrl Pts',(-19.6302748014164,44.4762460392736,124.597332076024)) ;
#40121=CARTESIAN_POINT('Ctrl Pts',(-19.6855192485498,44.2962569588638,124.893713217943)) ;
#40122=CARTESIAN_POINT('Ctrl Pts',(-19.4236658402343,44.4861203885307,124.617747552604)) ;
#40123=CARTESIAN_POINT('Ctrl Pts',(-19.4272568805924,44.3061313081208,124.919231077628)) ;
#40124=CARTESIAN_POINT('Ctrl Pts',(-19.2126136916866,44.4961899392729,124.601657803566)) ;
#40125=CARTESIAN_POINT('Ctrl Pts',(-19.163442166299,44.316200858863,124.899117334213)) ;
#40126=CARTESIAN_POINT('Ctrl Pts',(-19.0122816584332,44.5060239587815,124.550498030164)) ;
#40127=CARTESIAN_POINT('Ctrl Pts',(-18.9130262792638,44.3260348783717,124.835165719993)) ;
#40128=CARTESIAN_POINT('Ctrl Pts',(-18.8198408604291,44.516058113361,124.464118183293)) ;
#40129=CARTESIAN_POINT('Ctrl Pts',(-18.6724761255708,44.3360690329512,124.727189304503)) ;
#40130=CARTESIAN_POINT('Ctrl Pts',(-18.6459125382961,44.5260740391835,124.345407050209)) ;
#40131=CARTESIAN_POINT('Ctrl Pts',(-18.4550666358209,44.3460849587737,124.578799029754)) ;
#40132=CARTESIAN_POINT('Ctrl Pts',(-18.4969953236926,44.5359562943777,124.200536328678)) ;
#40133=CARTESIAN_POINT('Ctrl Pts',(-18.2689206933838,44.3559672139679,124.397708730876)) ;
#40134=CARTESIAN_POINT('Ctrl Pts',(-18.3739888329453,44.5459451008887,124.030365635577)) ;
#40135=CARTESIAN_POINT('Ctrl Pts',(-18.1151639541636,44.3659560204788,124.184994122612)) ;
#40136=CARTESIAN_POINT('Ctrl Pts',(-18.2825994603111,44.5558936681514,123.842202089097)) ;
#40137=CARTESIAN_POINT('Ctrl Pts',(-18.0009287363938,44.3759045877415,123.949788453005)) ;
#40138=CARTESIAN_POINT('Ctrl Pts',(-18.2248894304791,44.5659484734534,123.638872201841)) ;
#40139=CARTESIAN_POINT('Ctrl Pts',(-17.9287930123435,44.3859593930436,123.695625807399)) ;
#40140=CARTESIAN_POINT('Ctrl Pts',(-18.2035656681982,44.575767256717,123.433544830677)) ;
#40141=CARTESIAN_POINT('Ctrl Pts',(-17.9021400803731,44.3957781763071,123.438965134923)) ;
#40142=CARTESIAN_POINT('Ctrl Pts',(-18.2179757066852,44.5858030290775,123.223058832807)) ;
#40143=CARTESIAN_POINT('Ctrl Pts',(-17.9201546964338,44.4058139486677,123.175857889866)) ;
#40144=CARTESIAN_POINT('Ctrl Pts',(-18.2692459499617,44.5958277281062,123.018631696878)) ;
#40145=CARTESIAN_POINT('Ctrl Pts',(-17.9842443391472,44.4158386476964,122.920324456144)) ;
#40146=CARTESIAN_POINT('Ctrl Pts',(-18.3533314311282,44.6056797313652,122.829344467355)) ;
#40147=CARTESIAN_POINT('Ctrl Pts',(-18.0893534626568,44.4256906509554,122.683715321266)) ;
#40148=CARTESIAN_POINT('Ctrl Pts',(-18.4703557315628,44.6156706657625,122.65495463514)) ;
#40149=CARTESIAN_POINT('Ctrl Pts',(-18.2356357012521,44.4356815853526,122.465729074821)) ;
#40150=CARTESIAN_POINT('Ctrl Pts',(-18.6147549951052,44.6255885881936,122.504508089155)) ;
#40151=CARTESIAN_POINT('Ctrl Pts',(-18.4161367370382,44.4455995077838,122.27767197509)) ;
#40152=CARTESIAN_POINT('Ctrl Pts',(-18.7848954850902,44.6356169438759,122.380036959605)) ;
#40153=CARTESIAN_POINT('Ctrl Pts',(-18.6288136046969,44.4556278634661,122.122084840431)) ;
#40154=CARTESIAN_POINT('Ctrl Pts',(-18.9713236852492,44.6455012283865,122.288233366533)) ;
#40155=CARTESIAN_POINT('Ctrl Pts',(-18.8618504935947,44.4655121479767,122.00733199544)) ;
#40156=CARTESIAN_POINT('Ctrl Pts',(-19.1729084480282,44.6554939122944,122.229103541019)) ;
#40157=CARTESIAN_POINT('Ctrl Pts',(-19.1138322342579,44.4755048318845,121.93342190107)) ;
#40158=CARTESIAN_POINT('Ctrl Pts',(-19.382493485015,44.6655226493021,122.206156839358)) ;
#40159=CARTESIAN_POINT('Ctrl Pts',(-19.3758137501486,44.4855335688923,121.904740742788)) ;
#40160=CARTESIAN_POINT('Ctrl Pts',(-19.5898954585969,44.675408045931,122.219478540037)) ;
#40161=CARTESIAN_POINT('Ctrl Pts',(-19.635066763445,44.4954189655212,121.921395205992)) ;
#40162=CARTESIAN_POINT('Ctrl Pts',(-19.793970597842,44.6853959313449,122.268821405339)) ;
#40163=CARTESIAN_POINT('Ctrl Pts',(-19.8901602888194,44.505406850935,121.983076126972)) ;
#40164=CARTESIAN_POINT('Ctrl Pts',(-19.9857471745296,44.6953466340055,122.352468749605)) ;
#40165=CARTESIAN_POINT('Ctrl Pts',(-20.1298803582972,44.5153575535956,122.08763762812)) ;
#40166=CARTESIAN_POINT('Ctrl Pts',(-20.1615504334524,44.7053869521029,122.469253001426)) ;
#40167=CARTESIAN_POINT('Ctrl Pts',(-20.3496330624208,44.525397871693,122.233619868596)) ;
#40168=CARTESIAN_POINT('Ctrl Pts',(-20.3120561281735,44.7152615174361,122.612267502799)) ;
#40169=CARTESIAN_POINT('Ctrl Pts',(-20.5377640234827,44.5352724370263,122.412390214777)) ;
#40170=CARTESIAN_POINT('Ctrl Pts',(-20.4371874370457,44.7252611774972,122.78115208881)) ;
#40171=CARTESIAN_POINT('Ctrl Pts',(-20.6941762400881,44.5452720970874,122.623497503529)) ;
#40172=CARTESIAN_POINT('Ctrl Pts',(-20.5304535414409,44.7351701726649,122.967466993672)) ;
#40173=CARTESIAN_POINT('Ctrl Pts',(-20.8107568463989,44.5551810922551,122.856392682667)) ;
#40174=CARTESIAN_POINT('Ctrl Pts',(-20.5907433449701,44.7452249138281,123.170033529265)) ;
#40175=CARTESIAN_POINT('Ctrl Pts',(-20.8861166780626,44.5652358334183,123.109601455846)) ;
#40176=CARTESIAN_POINT('Ctrl Pts',(-20.6147190095158,44.7550835257419,123.375937676543)) ;
#40177=CARTESIAN_POINT('Ctrl Pts',(-20.9160838152845,44.5750944453321,123.366982582958)) ;
#40178=CARTESIAN_POINT('Ctrl Pts',(-20.60245263379,44.7651516480213,123.587214744072)) ;
#40179=CARTESIAN_POINT('Ctrl Pts',(-20.9007482952773,44.5851625676115,123.631078613725)) ;
#40180=CARTESIAN_POINT('Ctrl Pts',(-20.5546908139825,44.7750071187245,123.788845425538)) ;
#40181=CARTESIAN_POINT('Ctrl Pts',(-20.8410433869933,44.5950180383147,123.883116988004)) ;
#40182=CARTESIAN_POINT('Ctrl Pts',(-20.4720727117349,44.7850019782178,123.9820375159)) ;
#40183=CARTESIAN_POINT('Ctrl Pts',(-20.7377682696153,44.605012897808,124.124606144485)) ;
#40184=CARTESIAN_POINT('Ctrl Pts',(-20.3563607572283,44.7950332315598,124.158351468293)) ;
#40185=CARTESIAN_POINT('Ctrl Pts',(-20.593126161349,44.61504415115,124.34499716475)) ;
#40186=CARTESIAN_POINT('Ctrl Pts',(-20.2144020973158,44.8048999304329,124.309603441992)) ;
#40187=CARTESIAN_POINT('Ctrl Pts',(-20.4156755542351,44.624910850023,124.534060702325)) ;
#40188=CARTESIAN_POINT('Ctrl Pts',(-20.0465467747764,44.8148867461841,124.435681086058)) ;
#40189=CARTESIAN_POINT('Ctrl Pts',(-20.2058546847312,44.6348976657742,124.691655677505)) ;
#40190=CARTESIAN_POINT('Ctrl Pts',(-19.8600899400834,44.8248339513795,124.530430266587)) ;
#40191=CARTESIAN_POINT('Ctrl Pts',(-19.9727822075315,44.6448448709697,124.810089850154)) ;
#40192=CARTESIAN_POINT('Ctrl Pts',(-19.6581014765466,44.8348769395058,124.591850093754)) ;
#40193=CARTESIAN_POINT('Ctrl Pts',(-19.7202958616574,44.654887859096,124.886862052419)) ;
#40194=CARTESIAN_POINT('Ctrl Pts',(-19.4521749099809,44.8447442941273,124.616945312236)) ;
#40195=CARTESIAN_POINT('Ctrl Pts',(-19.4628869098963,44.6647552137175,124.918228439738)) ;
#40196=CARTESIAN_POINT('Ctrl Pts',(-19.242936933169,44.8547101874254,124.606358445387)) ;
#40197=CARTESIAN_POINT('Ctrl Pts',(-19.2013394365001,44.6747211070155,124.904992081286)) ;
#40198=CARTESIAN_POINT('Ctrl Pts',(-19.0375566117157,44.8647339648015,124.559112347747)) ;
#40199=CARTESIAN_POINT('Ctrl Pts',(-18.9446146116766,44.6847448843916,124.845931776664)) ;
#40200=CARTESIAN_POINT('Ctrl Pts',(-18.8454040569223,44.8746595127332,124.477781348015)) ;
#40201=CARTESIAN_POINT('Ctrl Pts',(-18.7044247703593,44.6946704323233,124.744265398485)) ;
#40202=CARTESIAN_POINT('Ctrl Pts',(-18.6697413624025,44.8845999891542,124.364553604711)) ;
#40203=CARTESIAN_POINT('Ctrl Pts',(-18.4848477731796,44.7046109087444,124.602728280035)) ;
#40204=CARTESIAN_POINT('Ctrl Pts',(-18.5149584063942,44.8946461988171,124.220874734381)) ;
#40205=CARTESIAN_POINT('Ctrl Pts',(-18.2913709520565,44.7146571184072,124.423127645195)) ;
#40206=CARTESIAN_POINT('Ctrl Pts',(-18.3896255165691,44.9045074554789,124.055712470621)) ;
#40207=CARTESIAN_POINT('Ctrl Pts',(-18.1347068985663,44.7245183750691,124.216672914179)) ;
#40208=CARTESIAN_POINT('Ctrl Pts',(-18.2933036607311,44.9145010837542,123.869030082729)) ;
#40209=CARTESIAN_POINT('Ctrl Pts',(-18.014307045051,44.7345120033443,123.983318570119)) ;
#40210=CARTESIAN_POINT('Ctrl Pts',(-18.2311629194592,44.9244264810644,123.669801758037)) ;
#40211=CARTESIAN_POINT('Ctrl Pts',(-17.9366337629122,44.7444374006545,123.734282199361)) ;
#40212=CARTESIAN_POINT('Ctrl Pts',(-18.2042856489682,44.9344543889746,123.46073131352)) ;
#40213=CARTESIAN_POINT('Ctrl Pts',(-17.9030399616873,44.7544653085648,123.472943722702)) ;
#40214=CARTESIAN_POINT('Ctrl Pts',(-18.2137679240456,44.9443407046438,123.253075539075)) ;
#40215=CARTESIAN_POINT('Ctrl Pts',(-17.9148956262802,44.764351624234,123.213374011932)) ;
#40216=CARTESIAN_POINT('Ctrl Pts',(-18.2597049737886,44.9543722995476,123.047278072271)) ;
#40217=CARTESIAN_POINT('Ctrl Pts',(-17.9723197113406,44.7743832191377,122.956127728826)) ;
#40218=CARTESIAN_POINT('Ctrl Pts',(-18.339321156955,44.9642545424993,122.855346311805)) ;
#40219=CARTESIAN_POINT('Ctrl Pts',(-18.0718425713176,44.7842654620895,122.716214046149)) ;
#40220=CARTESIAN_POINT('Ctrl Pts',(-18.4529511231331,44.9743140135291,122.677012970206)) ;
#40221=CARTESIAN_POINT('Ctrl Pts',(-18.2138824565309,44.7943249331193,122.493298818383)) ;
#40222=CARTESIAN_POINT('Ctrl Pts',(-18.5931221037197,44.9841804581923,122.524103073492)) ;
#40223=CARTESIAN_POINT('Ctrl Pts',(-18.3890982743492,44.8041913777825,122.302163339067)) ;
#40224=CARTESIAN_POINT('Ctrl Pts',(-18.7589604520614,44.994146582641,122.3960648915)) ;
#40225=CARTESIAN_POINT('Ctrl Pts',(-18.5963979569231,44.8141575022311,122.142117824545)) ;
#40226=CARTESIAN_POINT('Ctrl Pts',(-18.9458650964473,45.0041768260321,122.298439068355)) ;
#40227=CARTESIAN_POINT('Ctrl Pts',(-18.8300300927148,44.8241877456223,122.020087986047)) ;
#40228=CARTESIAN_POINT('Ctrl Pts',(-19.1440629077566,45.0140698609852,122.235330723378)) ;
#40229=CARTESIAN_POINT('Ctrl Pts',(-19.0777784030941,44.8340807805753,121.941205272845)) ;
#40230=CARTESIAN_POINT('Ctrl Pts',(-19.3534531145185,45.024120775222,122.207100463021)) ;
#40231=CARTESIAN_POINT('Ctrl Pts',(-19.3395157430268,44.8441316948122,121.905920090601)) ;
#40232=CARTESIAN_POINT('Ctrl Pts',(-19.5612049836232,45.0340106014466,122.215495999718)) ;
#40233=CARTESIAN_POINT('Ctrl Pts',(-19.5992088007516,44.8540215210367,121.916417743539)) ;
#40234=CARTESIAN_POINT('Ctrl Pts',(-19.8352568409963,45.0473454164935,122.274745540189)) ;
#40235=CARTESIAN_POINT('Ctrl Pts',(-19.9417558495627,44.8673563360837,121.990481112077)) ;
#40236=CARTESIAN_POINT('Ctrl Pts',(-20.0861970248156,45.060622507665,122.404050574181)) ;
#40237=CARTESIAN_POINT('Ctrl Pts',(-20.2554040576393,44.8806334272551,122.152088557829)) ;
#40238=CARTESIAN_POINT('Ctrl Pts',(-20.2927670242742,45.0738707962633,122.590851363296)) ;
#40239=CARTESIAN_POINT('Ctrl Pts',(-20.5136611156459,44.8938817158535,122.385626670175)) ;
#40240=CARTESIAN_POINT('Ctrl Pts',(-20.4224319151714,45.0839256377574,122.757766119149)) ;
#40241=CARTESIAN_POINT('Ctrl Pts',(-20.6757307464125,44.9039365573475,122.594264917547)) ;
#40242=CARTESIAN_POINT('Ctrl Pts',(-20.5192820589709,45.0937566270649,122.940386196395)) ;
#40243=CARTESIAN_POINT('Ctrl Pts',(-20.7967932246685,44.9137675466551,122.822543238492)) ;
#40244=CARTESIAN_POINT('Ctrl Pts',(-20.584670046844,45.1038331913881,123.141847213542)) ;
#40245=CARTESIAN_POINT('Ctrl Pts',(-20.8785256179564,44.9238441109783,123.07436836546)) ;
#40246=CARTESIAN_POINT('Ctrl Pts',(-20.6134250008506,45.1136825165221,123.34692196347)) ;
#40247=CARTESIAN_POINT('Ctrl Pts',(-20.9144646605094,44.9336934361122,123.330718388818)) ;
#40248=CARTESIAN_POINT('Ctrl Pts',(-20.6042179421268,45.1270305161593,123.627426871071)) ;
#40249=CARTESIAN_POINT('Ctrl Pts',(-20.9029627809531,44.9470414357495,123.681317025958)) ;
#40250=CARTESIAN_POINT('Ctrl Pts',(-20.501477245052,45.1436152756959,123.964696954444)) ;
#40251=CARTESIAN_POINT('Ctrl Pts',(-20.7745082952535,44.9636261952861,124.102953255056)) ;
#40252=CARTESIAN_POINT('Ctrl Pts',(-20.2906509977138,45.160183827044,124.247002494003)) ;
#40253=CARTESIAN_POINT('Ctrl Pts',(-20.5110259010541,44.9801947466342,124.455768261857)) ;
#40254=CARTESIAN_POINT('Ctrl Pts',(-20.0699761701848,45.173543651863,124.420705346495)) ;
#40255=CARTESIAN_POINT('Ctrl Pts',(-20.2351348039326,44.9935545714532,124.672943272152)) ;
#40256=CARTESIAN_POINT('Ctrl Pts',(-19.8865323634229,45.1834490606937,124.519294728282)) ;
#40257=CARTESIAN_POINT('Ctrl Pts',(-20.0058393288529,45.0034599802838,124.796167835436)) ;
#40258=CARTESIAN_POINT('Ctrl Pts',(-19.6878012033677,45.1934090872777,124.585169308581)) ;
#40259=CARTESIAN_POINT('Ctrl Pts',(-19.7574184008702,45.0134200068679,124.878510971873)) ;
#40260=CARTESIAN_POINT('Ctrl Pts',(-19.4120405401479,45.206666671463,124.625957687893)) ;
#40261=CARTESIAN_POINT('Ctrl Pts',(-19.4127381950799,45.0266775910532,124.929494089097)) ;
#40262=CARTESIAN_POINT('Ctrl Pts',(-19.0603261711488,45.2233178829577,124.585513512105)) ;
#40263=CARTESIAN_POINT('Ctrl Pts',(-18.9730728854601,45.0433288025479,124.87893348785)) ;
#40264=CARTESIAN_POINT('Ctrl Pts',(-18.6814904591991,45.243236097068,124.396215063051)) ;
#40265=CARTESIAN_POINT('Ctrl Pts',(-18.4995381186074,45.0632470166581,124.642306903912)) ;
#40266=CARTESIAN_POINT('Ctrl Pts',(-18.3898754544286,45.2631138602888,124.090194523484)) ;
#40267=CARTESIAN_POINT('Ctrl Pts',(-18.1350210819203,45.083124779879,124.259778759183)) ;
#40268=CARTESIAN_POINT('Ctrl Pts',(-18.2194472690857,45.283126528076,123.70037612657)) ;
#40269=CARTESIAN_POINT('Ctrl Pts',(-17.9219902773801,45.1031374476661,123.772503946096)) ;
#40270=CARTESIAN_POINT('Ctrl Pts',(-18.1921410054773,45.3029390507426,123.279913832054)) ;
#40271=CARTESIAN_POINT('Ctrl Pts',(-17.8878614142663,45.1229499703327,123.246927329165)) ;
#40272=CARTESIAN_POINT('Ctrl Pts',(-18.3102817888919,45.3229223507425,122.871855648759)) ;
#40273=CARTESIAN_POINT('Ctrl Pts',(-18.0355408684249,45.1429332703326,122.736855760761)) ;
#40274=CARTESIAN_POINT('Ctrl Pts',(-18.5597996288413,45.3428166278438,122.530199318799)) ;
#40275=CARTESIAN_POINT('Ctrl Pts',(-18.3474404946202,45.162827547434,122.30978822878)) ;
#40276=CARTESIAN_POINT('Ctrl Pts',(-18.9111760068349,45.3627493896015,122.293234594438)) ;
#40277=CARTESIAN_POINT('Ctrl Pts',(-18.7866621497905,45.1827603091917,122.013585300627)) ;
#40278=CARTESIAN_POINT('Ctrl Pts',(-19.3230940340298,45.3827153953663,122.190513539357)) ;
#40279=CARTESIAN_POINT('Ctrl Pts',(-19.301560104668,45.2027263149564,121.885187082608)) ;
#40280=CARTESIAN_POINT('Ctrl Pts',(-19.7435470242779,45.4025939275311,122.234031106994)) ;
#40281=CARTESIAN_POINT('Ctrl Pts',(-19.8271247058166,45.2226048471213,121.939586650909)) ;
#40282=CARTESIAN_POINT('Ctrl Pts',(-20.1251936183417,45.4225335941915,122.418585683632)) ;
#40283=CARTESIAN_POINT('Ctrl Pts',(-20.3041812490241,45.2425445137817,122.170281678223)) ;
#40284=CARTESIAN_POINT('Ctrl Pts',(-20.4204383603451,45.4424284688368,122.721592637798)) ;
#40285=CARTESIAN_POINT('Ctrl Pts',(-20.673234757287,45.262439388427,122.549040856851)) ;
#40286=CARTESIAN_POINT('Ctrl Pts',(-20.5949902534563,45.4623356081302,123.107099332329)) ;
#40287=CARTESIAN_POINT('Ctrl Pts',(-20.8914226003614,45.2823465277204,123.03092366851)) ;
#40288=CARTESIAN_POINT('Ctrl Pts',(-20.6282585414511,45.4822461562087,123.529280154733)) ;
#40289=CARTESIAN_POINT('Ctrl Pts',(-20.9330069949025,45.3022570757988,123.558648564274)) ;
#40290=CARTESIAN_POINT('Ctrl Pts',(-20.5136884964889,45.5023147415659,123.940226483196)) ;
#40291=CARTESIAN_POINT('Ctrl Pts',(-20.7897928711764,45.322325661156,124.072332126793)) ;
#40292=CARTESIAN_POINT('Ctrl Pts',(-20.2695153225536,45.5220965388806,124.282881980283)) ;
#40293=CARTESIAN_POINT('Ctrl Pts',(-20.4845776582098,45.3421074584708,124.500648372622)) ;
#40294=CARTESIAN_POINT('Ctrl Pts',(-19.9197219519249,45.5421040858251,124.52470903084)) ;
#40295=CARTESIAN_POINT('Ctrl Pts',(-20.0473359397497,45.3621150054153,124.802932073831)) ;
#40296=CARTESIAN_POINT('Ctrl Pts',(-19.5119563590964,45.561925824128,124.631740685911)) ;
#40297=CARTESIAN_POINT('Ctrl Pts',(-19.5376317009482,45.3819367437181,124.936721152297)) ;
#40298=CARTESIAN_POINT('Ctrl Pts',(-19.0888978513631,45.5819058440321,124.593677351388)) ;
#40299=CARTESIAN_POINT('Ctrl Pts',(-19.008808761564,45.4019167636223,124.889143040462)) ;
#40300=CARTESIAN_POINT('Ctrl Pts',(-18.7055922778892,45.6018232952944,124.413561871822)) ;
#40301=CARTESIAN_POINT('Ctrl Pts',(-18.5296775435037,45.4218342148845,124.664000015281)) ;
#40302=CARTESIAN_POINT('Ctrl Pts',(-18.4066895135121,45.6216982164671,124.114786478611)) ;
#40303=CARTESIAN_POINT('Ctrl Pts',(-18.1560490204871,45.4417091360573,124.290533223546)) ;
#40304=CARTESIAN_POINT('Ctrl Pts',(-18.2266120856884,45.6417225850179,123.729001322783)) ;
#40305=CARTESIAN_POINT('Ctrl Pts',(-17.9309504550063,45.4617335046081,123.808302209961)) ;
#40306=CARTESIAN_POINT('Ctrl Pts',(-18.1894029579917,45.6615892693914,123.308154855926)) ;
#40307=CARTESIAN_POINT('Ctrl Pts',(-17.8844372684627,45.4816001889816,123.282245957204)) ;
#40308=CARTESIAN_POINT('Ctrl Pts',(-18.2977756961196,45.6815330912376,122.898226280014)) ;
#40309=CARTESIAN_POINT('Ctrl Pts',(-18.0199005694617,45.5015440108278,122.769835234254)) ;
#40310=CARTESIAN_POINT('Ctrl Pts',(-18.5392315029753,45.7014404604891,122.55056181091)) ;
#40311=CARTESIAN_POINT('Ctrl Pts',(-18.3217175474318,45.5214513800793,122.335254029411)) ;
#40312=CARTESIAN_POINT('Ctrl Pts',(-18.8838051537408,45.7213151582358,122.30592410139)) ;
#40313=CARTESIAN_POINT('Ctrl Pts',(-18.7524316861254,45.541326077826,122.029454998102)) ;
#40314=CARTESIAN_POINT('Ctrl Pts',(-19.2933757524993,45.7412971007575,122.192842071119)) ;
#40315=CARTESIAN_POINT('Ctrl Pts',(-19.2643939100307,45.5613080203477,121.888099189158)) ;
#40316=CARTESIAN_POINT('Ctrl Pts',(-19.7151717006801,45.7611997676684,122.226529361424)) ;
#40317=CARTESIAN_POINT('Ctrl Pts',(-19.7916381676722,45.5812106872585,121.930204794617)) ;
#40318=CARTESIAN_POINT('Ctrl Pts',(-20.0998523433655,45.7810551252071,122.400620470514)) ;
#40319=CARTESIAN_POINT('Ctrl Pts',(-20.2724895989513,45.6010660447972,122.14781446257)) ;
#40320=CARTESIAN_POINT('Ctrl Pts',(-20.4047844549801,45.8011191639231,122.698883119931)) ;
#40321=CARTESIAN_POINT('Ctrl Pts',(-20.6536580200365,45.6211300835133,122.520640262286)) ;
#40322=CARTESIAN_POINT('Ctrl Pts',(-20.5876495556406,45.8209743436481,123.079572690105)) ;
#40323=CARTESIAN_POINT('Ctrl Pts',(-20.8822424651836,45.6409852632383,122.996499598283)) ;
#40324=CARTESIAN_POINT('Ctrl Pts',(-20.6301960454336,45.8409544483126,123.502103273831)) ;
#40325=CARTESIAN_POINT('Ctrl Pts',(-20.9354305274522,45.6609653679027,123.524661889093)) ;
#40326=CARTESIAN_POINT('Ctrl Pts',(-20.5273174567824,45.8607635534824,123.910665052776)) ;
#40327=CARTESIAN_POINT('Ctrl Pts',(-20.8068347568446,45.6807744730725,124.035365380698)) ;
#40328=CARTESIAN_POINT('Ctrl Pts',(-20.2894986913643,45.8807561738231,124.262859185796)) ;
#40329=CARTESIAN_POINT('Ctrl Pts',(-20.509573914599,45.7007670934133,124.475605981079)) ;
#40330=CARTESIAN_POINT('Ctrl Pts',(-20.0050296007185,45.8972956563272,124.469758288625)) ;
#40331=CARTESIAN_POINT('Ctrl Pts',(-20.1539637829623,45.7173065759173,124.734247767435)) ;
#40332=CARTESIAN_POINT('Ctrl Pts',(-19.7428533033287,45.9106599743914,124.570733072106)) ;
#40333=CARTESIAN_POINT('Ctrl Pts',(-19.8262766968498,45.7306708939816,124.860455779967)) ;
#40334=CARTESIAN_POINT('Ctrl Pts',(-19.4702042971827,45.9238775768929,124.624395490945)) ;
#40335=CARTESIAN_POINT('Ctrl Pts',(-19.4853999049145,45.7438884964831,124.927543476364)) ;
#40336=CARTESIAN_POINT('Ctrl Pts',(-19.1168393550171,45.9405351711707,124.600762737389)) ;
#40337=CARTESIAN_POINT('Ctrl Pts',(-19.0437646821561,45.7605460907609,124.897999792961)) ;
#40338=CARTESIAN_POINT('Ctrl Pts',(-18.7301975068277,45.9604008732124,124.430507653493)) ;
#40339=CARTESIAN_POINT('Ctrl Pts',(-18.5604443553071,45.7804117928026,124.685196121314)) ;
#40340=CARTESIAN_POINT('Ctrl Pts',(-18.4743625889817,45.9770305999024,124.186562575314)) ;
#40341=CARTESIAN_POINT('Ctrl Pts',(-18.24063059039,45.7970415194926,124.380241225742)) ;
#40342=CARTESIAN_POINT('Ctrl Pts',(-18.3289929824002,45.9903197150403,123.947896155844)) ;
#40343=CARTESIAN_POINT('Ctrl Pts',(-18.0589348453774,45.8103306346304,124.081934291381)) ;
#40344=CARTESIAN_POINT('Ctrl Pts',(-18.2525232753599,46.0002840620174,123.752891385966)) ;
#40345=CARTESIAN_POINT('Ctrl Pts',(-17.9633418368629,45.8202949816076,123.838171148534)) ;
#40346=CARTESIAN_POINT('Ctrl Pts',(-18.2110838319254,46.0102124300189,123.548318215047)) ;
#40347=CARTESIAN_POINT('Ctrl Pts',(-17.9115389080793,45.8302233496091,123.582470100108)) ;
#40348=CARTESIAN_POINT('Ctrl Pts',(-18.2034517091304,46.0234958631076,123.269181346863)) ;
#40349=CARTESIAN_POINT('Ctrl Pts',(-17.9020047413627,45.8435067826978,123.233481404812)) ;
#40350=CARTESIAN_POINT('Ctrl Pts',(-18.2859373810871,46.0401479408479,122.924806830037)) ;
#40351=CARTESIAN_POINT('Ctrl Pts',(-18.0050894428753,45.8601588604381,122.803097863818)) ;
#40352=CARTESIAN_POINT('Ctrl Pts',(-18.479608382182,46.0566993101488,122.631034753051)) ;
#40353=CARTESIAN_POINT('Ctrl Pts',(-18.247204245024,45.8767102297389,122.43582128981)) ;
#40354=CARTESIAN_POINT('Ctrl Pts',(-18.6881326465127,46.0699867382977,122.445080340454)) ;
#40355=CARTESIAN_POINT('Ctrl Pts',(-18.5078328375025,45.8899976578879,122.203411111206)) ;
#40356=CARTESIAN_POINT('Ctrl Pts',(-18.8678435030827,46.0800312779978,122.334231053414)) ;
#40357=CARTESIAN_POINT('Ctrl Pts',(-18.7324749006749,45.900042197588,122.064839903959)) ;
#40358=CARTESIAN_POINT('Ctrl Pts',(-19.060066473483,46.0898741198217,122.257583029304)) ;
#40359=CARTESIAN_POINT('Ctrl Pts',(-18.9727512213938,45.9098850394119,121.969029204028)) ;
#40360=CARTESIAN_POINT('Ctrl Pts',(-19.2654570004802,46.0998584040686,122.214404145467)) ;
#40361=CARTESIAN_POINT('Ctrl Pts',(-19.2294892302729,45.9198693236588,121.915052304712)) ;
#40362=CARTESIAN_POINT('Ctrl Pts',(-19.474529222648,46.1098080494678,122.207609739844)) ;
#40363=CARTESIAN_POINT('Ctrl Pts',(-19.4908293876559,45.9298189690579,121.906556619417)) ;
#40364=CARTESIAN_POINT('Ctrl Pts',(-19.6826867659275,46.1198078111562,122.237114286998)) ;
#40365=CARTESIAN_POINT('Ctrl Pts',(-19.7510268140422,45.9398187307464,121.943434488451)) ;
#40366=CARTESIAN_POINT('Ctrl Pts',(-19.8830689863678,46.1298391571151,122.30284594859)) ;
#40367=CARTESIAN_POINT('Ctrl Pts',(-20.0015055167164,45.9498500767053,122.025596415267)) ;
#40368=CARTESIAN_POINT('Ctrl Pts',(-20.0658738233849,46.1396941115922,122.400357303943)) ;
#40369=CARTESIAN_POINT('Ctrl Pts',(-20.2300129909118,45.9597050311824,122.147483174529)) ;
#40370=CARTESIAN_POINT('Ctrl Pts',(-20.2311978485199,46.1496666495927,122.529251790254)) ;
#40371=CARTESIAN_POINT('Ctrl Pts',(-20.436669839149,45.9696775691829,122.308599139471)) ;
#40372=CARTESIAN_POINT('Ctrl Pts',(-20.371971249445,46.1596616433277,122.68529494029)) ;
#40373=CARTESIAN_POINT('Ctrl Pts',(-20.6126387230333,45.9796725629179,122.503651259924)) ;
#40374=CARTESIAN_POINT('Ctrl Pts',(-20.4837019140822,46.1696957021218,122.864201377535)) ;
#40375=CARTESIAN_POINT('Ctrl Pts',(-20.7523044635287,45.989706621712,122.727282847783)) ;
#40376=CARTESIAN_POINT('Ctrl Pts',(-20.5615851923955,46.1795510449448,123.056218498459)) ;
#40377=CARTESIAN_POINT('Ctrl Pts',(-20.8496612408274,45.999561964535,122.967303410846)) ;
#40378=CARTESIAN_POINT('Ctrl Pts',(-20.6058435319962,46.1895505242904,123.261688930267)) ;
#40379=CARTESIAN_POINT('Ctrl Pts',(-20.9049869102636,46.0095614438806,123.224140951686)) ;
#40380=CARTESIAN_POINT('Ctrl Pts',(-20.613909648338,46.1994449730457,123.469584195291)) ;
#40381=CARTESIAN_POINT('Ctrl Pts',(-20.9150723248819,46.0194558926359,123.484010185293)) ;
#40382=CARTESIAN_POINT('Ctrl Pts',(-20.5852243576683,46.2095080924802,123.679152099285)) ;
#40383=CARTESIAN_POINT('Ctrl Pts',(-20.8792184641812,46.0295190120704,123.745970407951)) ;
#40384=CARTESIAN_POINT('Ctrl Pts',(-20.5222181496825,46.2193477377214,123.87621952154)) ;
#40385=CARTESIAN_POINT('Ctrl Pts',(-20.8004631964892,46.0393586573116,123.992305910874)) ;
#40386=CARTESIAN_POINT('Ctrl Pts',(-20.4240329883721,46.2294109019075,124.06358200029)) ;
#40387=CARTESIAN_POINT('Ctrl Pts',(-20.6777341783053,46.0494218214976,124.22651023524)) ;
#40388=CARTESIAN_POINT('Ctrl Pts',(-20.2968048807207,46.2393051716563,124.228173665467)) ;
#40389=CARTESIAN_POINT('Ctrl Pts',(-20.5187010120896,46.0593160912465,124.432251752414)) ;
#40390=CARTESIAN_POINT('Ctrl Pts',(-20.1426117795388,46.2492468976701,124.369228950053)) ;
#40391=CARTESIAN_POINT('Ctrl Pts',(-20.3259612494257,46.0692578172603,124.608573010478)) ;
#40392=CARTESIAN_POINT('Ctrl Pts',(-19.9651819070724,46.2592497863295,124.482167683482)) ;
#40393=CARTESIAN_POINT('Ctrl Pts',(-20.1041752621222,46.0792607059197,124.749748717366)) ;
#40394=CARTESIAN_POINT('Ctrl Pts',(-19.7700203195679,46.2692896351235,124.562503209581)) ;
#40395=CARTESIAN_POINT('Ctrl Pts',(-19.8602243414152,46.0893005547136,124.850170623669)) ;
#40396=CARTESIAN_POINT('Ctrl Pts',(-19.5683677612482,46.2791138505843,124.607227073809)) ;
#40397=CARTESIAN_POINT('Ctrl Pts',(-19.6081586045718,46.0991247701745,124.906078173835)) ;
#40398=CARTESIAN_POINT('Ctrl Pts',(-19.3571724462641,46.2891706940779,124.61676513193)) ;
#40399=CARTESIAN_POINT('Ctrl Pts',(-19.3441646598622,46.109181613668,124.91800334369)) ;
#40400=CARTESIAN_POINT('Ctrl Pts',(-19.1502130268079,46.2990993034739,124.589560068272)) ;
#40401=CARTESIAN_POINT('Ctrl Pts',(-19.0854647176611,46.119110223064,124.883999596973)) ;
#40402=CARTESIAN_POINT('Ctrl Pts',(-18.9504791865377,46.3090511875118,124.527247497498)) ;
#40403=CARTESIAN_POINT('Ctrl Pts',(-18.8357963857366,46.129062107102,124.806111234184)) ;
#40404=CARTESIAN_POINT('Ctrl Pts',(-18.7629062407361,46.3191041403194,124.429897592764)) ;
#40405=CARTESIAN_POINT('Ctrl Pts',(-18.6013290922815,46.1391150599095,124.684426224034)) ;
#40406=CARTESIAN_POINT('Ctrl Pts',(-18.5986696134654,46.3289270167856,124.304685324782)) ;
#40407=CARTESIAN_POINT('Ctrl Pts',(-18.3960311453645,46.1489379363757,124.527912442019)) ;
#40408=CARTESIAN_POINT('Ctrl Pts',(-18.4550971880899,46.3389827493557,124.149533035185)) ;
#40409=CARTESIAN_POINT('Ctrl Pts',(-18.2165638687555,46.1589936689459,124.333973843057)) ;
#40410=CARTESIAN_POINT('Ctrl Pts',(-18.34225300586,46.3489235143433,123.973622295558)) ;
#40411=CARTESIAN_POINT('Ctrl Pts',(-18.0755063144971,46.1689344339335,124.114086515465)) ;
#40412=CARTESIAN_POINT('Ctrl Pts',(-18.2613628141207,46.358827847249,123.78175251306)) ;
#40413=CARTESIAN_POINT('Ctrl Pts',(-17.9743911402147,46.1788387668392,123.874249738022)) ;
#40414=CARTESIAN_POINT('Ctrl Pts',(-18.2144855602519,46.3688745161297,123.575825795225)) ;
#40415=CARTESIAN_POINT('Ctrl Pts',(-17.915792209874,46.1888854357199,123.616841983507)) ;
#40416=CARTESIAN_POINT('Ctrl Pts',(-18.2040405773316,46.3787700794355,123.368018792122)) ;
#40417=CARTESIAN_POINT('Ctrl Pts',(-17.9027335514431,46.1987809990257,123.357082770934)) ;
#40418=CARTESIAN_POINT('Ctrl Pts',(-18.2302623333417,46.3888321371358,123.158144461646)) ;
#40419=CARTESIAN_POINT('Ctrl Pts',(-17.9355083347954,46.2088430567259,123.094739738862)) ;
#40420=CARTESIAN_POINT('Ctrl Pts',(-18.2910726090505,46.3986749147633,122.960331021879)) ;
#40421=CARTESIAN_POINT('Ctrl Pts',(-18.0115191596007,46.2186858343534,122.84747141581)) ;
#40422=CARTESIAN_POINT('Ctrl Pts',(-18.3862537401612,46.4086653930151,122.773135377991)) ;
#40423=CARTESIAN_POINT('Ctrl Pts',(-18.1304936326188,46.2286763126053,122.613475678905)) ;
#40424=CARTESIAN_POINT('Ctrl Pts',(-18.5117634998611,46.4185943656587,122.606329099744)) ;
#40425=CARTESIAN_POINT('Ctrl Pts',(-18.2873793151944,46.2386052852488,122.404966075786)) ;
#40426=CARTESIAN_POINT('Ctrl Pts',(-18.6650531697513,46.4285855025382,122.462726172881)) ;
#40427=CARTESIAN_POINT('Ctrl Pts',(-18.4789900283412,46.2485964221284,122.225460708886)) ;
#40428=CARTESIAN_POINT('Ctrl Pts',(-18.8416348523983,46.4386076200272,122.347776529069)) ;
#40429=CARTESIAN_POINT('Ctrl Pts',(-18.6997158872506,46.2586185396174,122.081771774916)) ;
#40430=CARTESIAN_POINT('Ctrl Pts',(-19.033062714252,46.4485081304294,122.266054468037)) ;
#40431=CARTESIAN_POINT('Ctrl Pts',(-18.9390004515554,46.2685190500195,121.979616917405)) ;
#40432=CARTESIAN_POINT('Ctrl Pts',(-19.2375063165582,46.4584971231755,122.218070769825)) ;
#40433=CARTESIAN_POINT('Ctrl Pts',(-19.1945546489637,46.2785080427657,121.919635191625)) ;
#40434=CARTESIAN_POINT('Ctrl Pts',(-19.4466780664343,46.4684623672261,122.206487877889)) ;
#40435=CARTESIAN_POINT('Ctrl Pts',(-19.4560195398853,46.2884732868162,121.905154403396)) ;
#40436=CARTESIAN_POINT('Ctrl Pts',(-19.6534929917255,46.4783666317393,122.230762789135)) ;
#40437=CARTESIAN_POINT('Ctrl Pts',(-19.7145391120735,46.2983775513295,121.935496118743)) ;
#40438=CARTESIAN_POINT('Ctrl Pts',(-19.8559786184111,46.4884247234375,122.291626495888)) ;
#40439=CARTESIAN_POINT('Ctrl Pts',(-19.9676465194211,46.3084356430277,122.01157371518)) ;
#40440=CARTESIAN_POINT('Ctrl Pts',(-20.0410082512781,46.4982746638659,122.384630025382)) ;
#40441=CARTESIAN_POINT('Ctrl Pts',(-20.1989353902654,46.3182855834561,122.127826794812)) ;
#40442=CARTESIAN_POINT('Ctrl Pts',(-20.2103627890321,46.5083016750394,122.510144547104)) ;
#40443=CARTESIAN_POINT('Ctrl Pts',(-20.4106296401111,46.3283125946296,122.28471843049)) ;
#40444=CARTESIAN_POINT('Ctrl Pts',(-20.354983799268,46.5183302616515,122.66357001132)) ;
#40445=CARTESIAN_POINT('Ctrl Pts',(-20.5914073283371,46.3383411812416,122.476498822168)) ;
#40446=CARTESIAN_POINT('Ctrl Pts',(-20.4689669278839,46.5281754757642,122.836320633626)) ;
#40447=CARTESIAN_POINT('Ctrl Pts',(-20.7338884448632,46.3481863953544,122.692436981953)) ;
#40448=CARTESIAN_POINT('Ctrl Pts',(-20.5529614777016,46.5381662239437,123.028836720587)) ;
#40449=CARTESIAN_POINT('Ctrl Pts',(-20.8388832978075,46.3581771435339,122.933081577191)) ;
#40450=CARTESIAN_POINT('Ctrl Pts',(-20.6020311758152,46.5482038575292,123.234075060244)) ;
#40451=CARTESIAN_POINT('Ctrl Pts',(-20.9002222160661,46.3682147771194,123.189628936888)) ;
#40452=CARTESIAN_POINT('Ctrl Pts',(-20.6148200501619,46.5580491467421,123.440660845129)) ;
#40453=CARTESIAN_POINT('Ctrl Pts',(-20.9162101456028,46.3780600663322,123.447862222643)) ;
#40454=CARTESIAN_POINT('Ctrl Pts',(-20.5916887931145,46.568030547548,123.649206343481)) ;
#40455=CARTESIAN_POINT('Ctrl Pts',(-20.8872976540817,46.3880414671381,123.708544539152)) ;
#40456=CARTESIAN_POINT('Ctrl Pts',(-20.5328161463453,46.5779827805379,123.849986028359)) ;
#40457=CARTESIAN_POINT('Ctrl Pts',(-20.8137082786471,46.3979937001281,123.959520057997)) ;
#40458=CARTESIAN_POINT('Ctrl Pts',(-20.4397820483577,46.5879815919945,124.038501912924)) ;
#40459=CARTESIAN_POINT('Ctrl Pts',(-20.6974169784286,46.4079925115847,124.195165716558)) ;
#40460=CARTESIAN_POINT('Ctrl Pts',(-20.3146171869605,46.5980206959252,124.208420179491)) ;
#40461=CARTESIAN_POINT('Ctrl Pts',(-20.5409623496544,46.4180316155154,124.407564420315)) ;
#40462=CARTESIAN_POINT('Ctrl Pts',(-20.1653985323656,46.6078456383445,124.351256112857)) ;
#40463=CARTESIAN_POINT('Ctrl Pts',(-20.3544390960166,46.4278565579347,124.586111387975)) ;
#40464=CARTESIAN_POINT('Ctrl Pts',(-19.989843192052,46.6179003258204,124.468971674532)) ;
#40465=CARTESIAN_POINT('Ctrl Pts',(-20.1349959199088,46.4379112454106,124.733256870645)) ;
#40466=CARTESIAN_POINT('Ctrl Pts',(-19.7985051156906,46.6278431281773,124.553146705472)) ;
#40467=CARTESIAN_POINT('Ctrl Pts',(-19.8958234362886,46.4478540477674,124.838477290349)) ;
#40468=CARTESIAN_POINT('Ctrl Pts',(-19.5964092228832,46.637746924117,124.603245253759)) ;
#40469=CARTESIAN_POINT('Ctrl Pts',(-19.6432030628743,46.4577578437072,124.901101950922)) ;
#40470=CARTESIAN_POINT('Ctrl Pts',(-19.3856978448509,46.6477937034921,124.617570281629)) ;
#40471=CARTESIAN_POINT('Ctrl Pts',(-19.3798141419752,46.4678046230822,124.919009575236)) ;
#40472=CARTESIAN_POINT('Ctrl Pts',(-19.1787922985653,46.6576893617867,124.595604702868)) ;
#40473=CARTESIAN_POINT('Ctrl Pts',(-19.1211811679107,46.4777002813768,124.891553789265)) ;
#40474=CARTESIAN_POINT('Ctrl Pts',(-18.9755356634845,46.6677509290373,124.537120494577)) ;
#40475=CARTESIAN_POINT('Ctrl Pts',(-18.8671103311034,46.4877618486275,124.818449853057)) ;
#40476=CARTESIAN_POINT('Ctrl Pts',(-18.7895780705822,46.6775955734746,124.446252644844)) ;
#40477=CARTESIAN_POINT('Ctrl Pts',(-18.6346615957994,46.4976064930648,124.704865605412)) ;
#40478=CARTESIAN_POINT('Ctrl Pts',(-18.6198270026623,46.6875556197173,124.323663154049)) ;
#40479=CARTESIAN_POINT('Ctrl Pts',(-18.4224718069729,46.5075665393075,124.551629282705)) ;
#40480=CARTESIAN_POINT('Ctrl Pts',(-18.4730960397559,46.6975939157357,124.171998085648)) ;
#40481=CARTESIAN_POINT('Ctrl Pts',(-18.2390573894133,46.5176048353258,124.362048863157)) ;
#40482=CARTESIAN_POINT('Ctrl Pts',(-18.3565170418454,46.707467257154,124.0002223481)) ;
#40483=CARTESIAN_POINT('Ctrl Pts',(-18.0933321835111,46.5274781767442,124.147328823176)) ;
#40484=CARTESIAN_POINT('Ctrl Pts',(-18.2699035021467,46.7175403609533,123.807021171241)) ;
#40485=CARTESIAN_POINT('Ctrl Pts',(-17.9850644965826,46.5375512805435,123.90582815991)) ;
#40486=CARTESIAN_POINT('Ctrl Pts',(-18.2191778694931,46.7273611760722,123.606843477145)) ;
#40487=CARTESIAN_POINT('Ctrl Pts',(-17.9216561766036,46.5473720956623,123.655604769704)) ;
#40488=CARTESIAN_POINT('Ctrl Pts',(-18.2033482281936,46.7374380411502,123.395627154277)) ;
#40489=CARTESIAN_POINT('Ctrl Pts',(-17.9018683249847,46.5574489607404,123.391584873683)) ;
#40490=CARTESIAN_POINT('Ctrl Pts',(-18.2240747598041,46.7473027808054,123.189252605334)) ;
#40491=CARTESIAN_POINT('Ctrl Pts',(-17.9277757498325,46.5673137003956,123.133615388433)) ;
#40492=CARTESIAN_POINT('Ctrl Pts',(-18.2806784571676,46.7573251840468,122.986304105928)) ;
#40493=CARTESIAN_POINT('Ctrl Pts',(-17.9985297243312,46.5773361036369,122.879929630488)) ;
#40494=CARTESIAN_POINT('Ctrl Pts',(-18.3721757227985,46.7673509083353,122.796412957651)) ;
#40495=CARTESIAN_POINT('Ctrl Pts',(-18.112900494446,46.5873618279254,122.642565399485)) ;
#40496=CARTESIAN_POINT('Ctrl Pts',(-18.4928445279093,46.7772056913566,122.628018609058)) ;
#40497=CARTESIAN_POINT('Ctrl Pts',(-18.263736687569,46.5972166109468,122.432070963877)) ;
#40498=CARTESIAN_POINT('Ctrl Pts',(-18.6424131075352,46.7871845350798,122.480907272402)) ;
#40499=CARTESIAN_POINT('Ctrl Pts',(-18.4506972916497,46.60719545467,122.2481811978)) ;
#40500=CARTESIAN_POINT('Ctrl Pts',(-18.8161403685394,46.7972034273165,122.361831711629)) ;
#40501=CARTESIAN_POINT('Ctrl Pts',(-18.6678559884492,46.6172143469067,122.099336220599)) ;
#40502=CARTESIAN_POINT('Ctrl Pts',(-19.0051621248725,46.8070866363575,122.275502154482)) ;
#40503=CARTESIAN_POINT('Ctrl Pts',(-18.9041339832158,46.6270975559476,121.991423381357)) ;
#40504=CARTESIAN_POINT('Ctrl Pts',(-19.210031702073,46.8171549456977,122.222428926557)) ;
#40505=CARTESIAN_POINT('Ctrl Pts',(-19.1602204279104,46.6371658652879,121.925081449828)) ;
#40506=CARTESIAN_POINT('Ctrl Pts',(-19.4160633040709,46.8269850710304,122.205881850251)) ;
#40507=CARTESIAN_POINT('Ctrl Pts',(-19.4177614318247,46.6469959906205,121.904397063285)) ;
#40508=CARTESIAN_POINT('Ctrl Pts',(-19.6267444353502,46.8370516234074,122.22554880192)) ;
#40509=CARTESIAN_POINT('Ctrl Pts',(-19.681112479363,46.6570625429976,121.928980404432)) ;
#40510=CARTESIAN_POINT('Ctrl Pts',(-19.8272585672866,46.8469418603011,122.280657735595)) ;
#40511=CARTESIAN_POINT('Ctrl Pts',(-19.9317562516672,46.6669527798912,121.997866497252)) ;
#40512=CARTESIAN_POINT('Ctrl Pts',(-20.0172576560397,46.8569340850951,122.370232887069)) ;
#40513=CARTESIAN_POINT('Ctrl Pts',(-20.1692553844412,46.6769450046852,122.109835361728)) ;
#40514=CARTESIAN_POINT('Ctrl Pts',(-20.1882040593248,46.866896705446,122.491242308474)) ;
#40515=CARTESIAN_POINT('Ctrl Pts',(-20.3829389131925,46.6869076250362,122.261097188101)) ;
#40516=CARTESIAN_POINT('Ctrl Pts',(-20.3350687567512,46.8768017082092,122.638883740388)) ;
#40517=CARTESIAN_POINT('Ctrl Pts',(-20.5665204840061,46.6968126277993,122.445649602408)) ;
#40518=CARTESIAN_POINT('Ctrl Pts',(-20.4557645798383,46.8868594706073,122.812475638472)) ;
#40519=CARTESIAN_POINT('Ctrl Pts',(-20.717390165257,46.7068703901975,122.662639131552)) ;
#40520=CARTESIAN_POINT('Ctrl Pts',(-20.5428264939987,46.8967099899861,123.000391779581)) ;
#40521=CARTESIAN_POINT('Ctrl Pts',(-20.8262181895513,46.7167209095763,122.897535565363)) ;
#40522=CARTESIAN_POINT('Ctrl Pts',(-20.5973539637941,46.9067415669843,123.204102169364)) ;
#40523=CARTESIAN_POINT('Ctrl Pts',(-20.8943773618828,46.7267524865744,123.152173475016)) ;
#40524=CARTESIAN_POINT('Ctrl Pts',(-20.6152416325616,46.9167513020892,123.413800001265)) ;
#40525=CARTESIAN_POINT('Ctrl Pts',(-20.9167369791309,46.7367622216794,123.414295804395)) ;
#40526=CARTESIAN_POINT('Ctrl Pts',(-20.5968220041765,46.9266608787155,123.621296181329)) ;
#40527=CARTESIAN_POINT('Ctrl Pts',(-20.8937123153828,46.7466717983056,123.673666920651)) ;
#40528=CARTESIAN_POINT('Ctrl Pts',(-20.5430662397492,46.9365882645721,123.822968750851)) ;
#40529=CARTESIAN_POINT('Ctrl Pts',(-20.8265171674888,46.7565991841623,123.925758286635)) ;
#40530=CARTESIAN_POINT('Ctrl Pts',(-20.4539206450829,46.9466331990624,124.014396648142)) ;
#40531=CARTESIAN_POINT('Ctrl Pts',(-20.7150850922939,46.7666441186526,124.165042884017)) ;
#40532=CARTESIAN_POINT('Ctrl Pts',(-20.3348959674513,46.9565191312504,124.184787009017)) ;
#40533=CARTESIAN_POINT('Ctrl Pts',(-20.5663034238084,46.7765300508405,124.378031588632)) ;
#40534=CARTESIAN_POINT('Ctrl Pts',(-20.1867731077761,46.9665124372034,124.333759281434)) ;
#40535=CARTESIAN_POINT('Ctrl Pts',(-20.3811494336944,46.7865233567936,124.56424680327)) ;
#40536=CARTESIAN_POINT('Ctrl Pts',(-20.0157955120954,46.9764580749853,124.454112395529)) ;
#40537=CARTESIAN_POINT('Ctrl Pts',(-20.1674267507565,46.7964689945755,124.714688252235)) ;
#40538=CARTESIAN_POINT('Ctrl Pts',(-19.8266604007549,46.9864053433312,124.543356690271)) ;
#40539=CARTESIAN_POINT('Ctrl Pts',(-19.9310071201498,46.8064162629214,124.826243396282)) ;
#40540=CARTESIAN_POINT('Ctrl Pts',(-19.6228151224958,46.9964532454683,124.598728489148)) ;
#40541=CARTESIAN_POINT('Ctrl Pts',(-19.6762006528728,46.8164641650585,124.895457669086)) ;
#40542=CARTESIAN_POINT('Ctrl Pts',(-19.4166526981356,47.0063009403085,124.617657767281)) ;
#40543=CARTESIAN_POINT('Ctrl Pts',(-19.4184961828362,46.8263118598987,124.919118902968)) ;
#40544=CARTESIAN_POINT('Ctrl Pts',(-19.2079050762096,47.0162624500529,124.600964149911)) ;
#40545=CARTESIAN_POINT('Ctrl Pts',(-19.1575612606984,46.8362733696431,124.898251094287)) ;
#40546=CARTESIAN_POINT('Ctrl Pts',(-19.0039009099091,47.0262918416617,124.54764239375)) ;
#40547=CARTESIAN_POINT('Ctrl Pts',(-18.9025563129706,46.8463027612519,124.83159830442)) ;
#40548=CARTESIAN_POINT('Ctrl Pts',(-18.8145419924307,47.0361993372165,124.460883485285)) ;
#40549=CARTESIAN_POINT('Ctrl Pts',(-18.6658571373516,46.8562102568067,124.723148672064)) ;
#40550=CARTESIAN_POINT('Ctrl Pts',(-18.642246189298,47.0461447288795,124.342465094977)) ;
#40551=CARTESIAN_POINT('Ctrl Pts',(-18.4504873824493,46.8661556484697,124.575124657346)) ;
#40552=CARTESIAN_POINT('Ctrl Pts',(-18.4921614871914,47.0561466464769,124.1951532533)) ;
#40553=CARTESIAN_POINT('Ctrl Pts',(-18.2628820412351,46.876157566067,124.390984128051)) ;
#40554=CARTESIAN_POINT('Ctrl Pts',(-18.3698136381604,47.0661867140291,124.023179183361)) ;
#40555=CARTESIAN_POINT('Ctrl Pts',(-18.1099479380349,46.8861976336192,124.176016249367)) ;
#40556=CARTESIAN_POINT('Ctrl Pts',(-18.2806928887342,47.0760110254689,123.836839708192)) ;
#40557=CARTESIAN_POINT('Ctrl Pts',(-17.9985471751424,46.896021945059,123.943090129872)) ;
#40558=CARTESIAN_POINT('Ctrl Pts',(-18.2237020979738,47.086067266625,123.633273731581)) ;
#40559=CARTESIAN_POINT('Ctrl Pts',(-17.9273097684418,46.9060781862152,123.688632681339)) ;
#40560=CARTESIAN_POINT('Ctrl Pts',(-18.203421628533,47.0959981883606,123.425458332389)) ;
#40561=CARTESIAN_POINT('Ctrl Pts',(-17.9019600483901,46.9160091079508,123.428862667501)) ;
#40562=CARTESIAN_POINT('Ctrl Pts',(-18.2191232760878,47.1059414244368,123.217037662918)) ;
#40563=CARTESIAN_POINT('Ctrl Pts',(-17.92158824873,46.925952344027,123.168336310524)) ;
#40564=CARTESIAN_POINT('Ctrl Pts',(-18.2707913644975,47.1159227084493,123.013627488194)) ;
#40565=CARTESIAN_POINT('Ctrl Pts',(-17.9861745622981,46.9359336280395,122.914073624289)) ;
#40566=CARTESIAN_POINT('Ctrl Pts',(-18.3578456878256,47.125967010075,122.821273166394)) ;
#40567=CARTESIAN_POINT('Ctrl Pts',(-18.094993333607,46.9459779296651,122.67363132512)) ;
#40568=CARTESIAN_POINT('Ctrl Pts',(-18.4740478321358,47.1357950912944,122.650390408871)) ;
#40569=CARTESIAN_POINT('Ctrl Pts',(-18.2402478329173,46.9558060108846,122.460027367122)) ;
#40570=CARTESIAN_POINT('Ctrl Pts',(-18.6216725538285,47.1458716941436,122.498517159224)) ;
#40571=CARTESIAN_POINT('Ctrl Pts',(-18.4247793330905,46.9658826137337,122.270186990545)) ;
#40572=CARTESIAN_POINT('Ctrl Pts',(-18.789608451275,47.1557237732621,122.377209771896)) ;
#40573=CARTESIAN_POINT('Ctrl Pts',(-18.6347009617325,46.9757346928523,122.118553077967)) ;
#40574=CARTESIAN_POINT('Ctrl Pts',(-18.980091407923,47.165797031571,122.284749398737)) ;
#40575=CARTESIAN_POINT('Ctrl Pts',(-18.8728048872748,46.9858079511612,122.002979006132)) ;
#40576=CARTESIAN_POINT('Ctrl Pts',(-19.1791102852178,47.1756384909513,122.228144087822)) ;
#40577=CARTESIAN_POINT('Ctrl Pts',(-19.1215801045006,46.9956494105415,121.932223291973)) ;
#40578=CARTESIAN_POINT('Ctrl Pts',(-19.3873332175923,47.1855995863637,122.205917819797)) ;
#40579=CARTESIAN_POINT('Ctrl Pts',(-19.3818593433925,47.0056105059539,121.904442012437)) ;
#40580=CARTESIAN_POINT('Ctrl Pts',(-19.5978250311267,47.1956368707604,122.220705841968)) ;
#40581=CARTESIAN_POINT('Ctrl Pts',(-19.6449738783017,47.0156477903506,121.922928491148)) ;
#40582=CARTESIAN_POINT('Ctrl Pts',(-19.7993828425593,47.2055132094957,122.270652196407)) ;
#40583=CARTESIAN_POINT('Ctrl Pts',(-19.8969217299494,47.0255241290858,121.985363214228)) ;
#40584=CARTESIAN_POINT('Ctrl Pts',(-19.9927485786675,47.2155753356489,122.356364369119)) ;
#40585=CARTESIAN_POINT('Ctrl Pts',(-20.1386279884398,47.0355862552391,122.092504779717)) ;
#40586=CARTESIAN_POINT('Ctrl Pts',(-20.1649812697198,47.2254435096255,122.472061623222)) ;
#40587=CARTESIAN_POINT('Ctrl Pts',(-20.353918813109,47.0454544292157,122.237128269976)) ;
#40588=CARTESIAN_POINT('Ctrl Pts',(-20.3168466409141,47.2354490581293,122.61756598711)) ;
#40589=CARTESIAN_POINT('Ctrl Pts',(-20.5437493741257,47.0554599777195,122.419010050807)) ;
#40590=CARTESIAN_POINT('Ctrl Pts',(-20.4408371920724,47.2454316900249,122.7869363998)) ;
#40591=CARTESIAN_POINT('Ctrl Pts',(-20.698736298612,47.065442609615,122.63072426996)) ;
#40592=CARTESIAN_POINT('Ctrl Pts',(-20.5338834735868,47.2554756324466,122.976466219455)) ;
#40593=CARTESIAN_POINT('Ctrl Pts',(-20.8150425910065,47.0754865520368,122.867637130204)) ;
#40594=CARTESIAN_POINT('Ctrl Pts',(-20.5916167588128,47.2653037804738,123.17485450326)) ;
#40595=CARTESIAN_POINT('Ctrl Pts',(-20.8872078792665,47.085314700064,123.115624213274)) ;
#40596=CARTESIAN_POINT('Ctrl Pts',(-20.6150653225155,47.2752936478482,123.383560571913)) ;
#40597=CARTESIAN_POINT('Ctrl Pts',(-20.9165166535545,47.0953045674384,123.376507189918)) ;
#40598=CARTESIAN_POINT('Ctrl Pts',(-20.601300740418,47.2853373868037,123.594262445601)) ;
#40599=CARTESIAN_POINT('Ctrl Pts',(-20.89930914947,47.1053483063939,123.639884268213)) ;
#40600=CARTESIAN_POINT('Ctrl Pts',(-20.552687444503,47.2951591353416,123.794940800993)) ;
#40601=CARTESIAN_POINT('Ctrl Pts',(-20.8385403651115,47.1151700549318,123.890732974472)) ;
#40602=CARTESIAN_POINT('Ctrl Pts',(-20.4686462395042,47.3051941129514,123.988445576631)) ;
#40603=CARTESIAN_POINT('Ctrl Pts',(-20.7334869966669,47.1252050325415,124.132613019334)) ;
#40604=CARTESIAN_POINT('Ctrl Pts',(-20.3519069360569,47.3152190257091,124.163922378538)) ;
#40605=CARTESIAN_POINT('Ctrl Pts',(-20.5875612970063,47.1352299452993,124.351957946724)) ;
#40606=CARTESIAN_POINT('Ctrl Pts',(-20.2093112218679,47.3250709688029,124.314143088258)) ;
#40607=CARTESIAN_POINT('Ctrl Pts',(-20.4093144806354,47.1450818883931,124.539733166046)) ;
#40608=CARTESIAN_POINT('Ctrl Pts',(-20.0406636984681,47.335061930132,124.439301449808)) ;
#40609=CARTESIAN_POINT('Ctrl Pts',(-20.198503670169,47.1550728497222,124.696179510647)) ;
#40610=CARTESIAN_POINT('Ctrl Pts',(-19.8542359453285,47.3449798050004,124.532734343896)) ;
#40611=CARTESIAN_POINT('Ctrl Pts',(-19.9654674976821,47.1649907245906,124.812968953149)) ;
#40612=CARTESIAN_POINT('Ctrl Pts',(-19.6522424998238,47.3550083240017,124.593072966075)) ;
#40613=CARTESIAN_POINT('Ctrl Pts',(-19.7129751029458,47.1750192435918,124.888390135927)) ;
#40614=CARTESIAN_POINT('Ctrl Pts',(-19.4458515602898,47.3648920027995,124.617180149755)) ;
#40615=CARTESIAN_POINT('Ctrl Pts',(-19.4549854354242,47.1849029223897,124.918522015766)) ;
#40616=CARTESIAN_POINT('Ctrl Pts',(-19.2360564520279,47.3748869462393,124.605411359256)) ;
#40617=CARTESIAN_POINT('Ctrl Pts',(-19.1927415406331,47.1948978658294,124.903808702295)) ;
#40618=CARTESIAN_POINT('Ctrl Pts',(-19.0309200127824,47.3849138000617,124.556888090555)) ;
#40619=CARTESIAN_POINT('Ctrl Pts',(-18.9363215273334,47.2049247196518,124.843152452607)) ;
#40620=CARTESIAN_POINT('Ctrl Pts',(-18.8399600132762,47.3947979644006,124.474930121574)) ;
#40621=CARTESIAN_POINT('Ctrl Pts',(-18.6976217950218,47.2148088839908,124.740702605939)) ;
#40622=CARTESIAN_POINT('Ctrl Pts',(-18.6641751096275,47.404786062443,124.360112233341)) ;
#40623=CARTESIAN_POINT('Ctrl Pts',(-18.4778918250727,47.2247969820332,124.597178175562)) ;
#40624=CARTESIAN_POINT('Ctrl Pts',(-18.5114500487226,47.4147371689001,124.217101265402)) ;
#40625=CARTESIAN_POINT('Ctrl Pts',(-18.2869868869879,47.2347480884902,124.41841249346)) ;
#40626=CARTESIAN_POINT('Ctrl Pts',(-18.3848081572941,47.4247822200682,124.048124629567)) ;
#40627=CARTESIAN_POINT('Ctrl Pts',(-18.1286864682483,47.2447931396584,124.207190353559)) ;
#40628=CARTESIAN_POINT('Ctrl Pts',(-18.2910618402465,47.4346439804265,123.86320370385)) ;
#40629=CARTESIAN_POINT('Ctrl Pts',(-18.0115053674307,47.2546549000167,123.976037450249)) ;
#40630=CARTESIAN_POINT('Ctrl Pts',(-18.2296126467464,47.4446067972569,123.662969790822)) ;
#40631=CARTESIAN_POINT('Ctrl Pts',(-17.9346962186419,47.2646177168471,123.725744078464)) ;
#40632=CARTESIAN_POINT('Ctrl Pts',(-18.2040389740413,47.4546414785377,123.45357433271)) ;
#40633=CARTESIAN_POINT('Ctrl Pts',(-17.9027315658583,47.2746523981279,123.4639994927)) ;
#40634=CARTESIAN_POINT('Ctrl Pts',(-18.2146920724958,47.4645265083184,123.246004580245)) ;
#40635=CARTESIAN_POINT('Ctrl Pts',(-17.9160504866388,47.2845374279086,123.204536864784)) ;
#40636=CARTESIAN_POINT('Ctrl Pts',(-18.2621069746344,47.4745921017164,123.039809498366)) ;
#40637=CARTESIAN_POINT('Ctrl Pts',(-17.9753215325258,47.2946030213066,122.946793722873)) ;
#40638=CARTESIAN_POINT('Ctrl Pts',(-18.3425816794122,47.4844312700779,122.849220328905)) ;
#40639=CARTESIAN_POINT('Ctrl Pts',(-18.0759175401619,47.3044421896681,122.708557598434)) ;
#40640=CARTESIAN_POINT('Ctrl Pts',(-18.457201944164,47.4944938678194,122.671444955583)) ;
#40641=CARTESIAN_POINT('Ctrl Pts',(-18.2191949883695,47.3145047874096,122.486339905926)) ;
#40642=CARTESIAN_POINT('Ctrl Pts',(-18.5987718864396,47.5043908802264,122.518950167232)) ;
#40643=CARTESIAN_POINT('Ctrl Pts',(-18.3961596154612,47.3244017998165,122.295722821645)) ;
#40644=CARTESIAN_POINT('Ctrl Pts',(-18.7648105631557,47.514322202052,122.392374159236)) ;
#40645=CARTESIAN_POINT('Ctrl Pts',(-18.6037098264128,47.3343331216421,122.137504758637)) ;
#40646=CARTESIAN_POINT('Ctrl Pts',(-18.9524743880465,47.5243639648065,122.295687498941)) ;
#40647=CARTESIAN_POINT('Ctrl Pts',(-18.8382907890094,47.3443748843966,122.016648795415)) ;
#40648=CARTESIAN_POINT('Ctrl Pts',(-19.1509626646768,47.5342521636972,122.233865751707)) ;
#40649=CARTESIAN_POINT('Ctrl Pts',(-19.0864023365474,47.3542630832873,121.939374027892)) ;
#40650=CARTESIAN_POINT('Ctrl Pts',(-19.3593042021687,47.544246102297,122.206837954189)) ;
#40651=CARTESIAN_POINT('Ctrl Pts',(-19.3468297085814,47.3642570218872,121.905591956096)) ;
#40652=CARTESIAN_POINT('Ctrl Pts',(-19.5680879347369,47.5541869233339,122.216359937286)) ;
#40653=CARTESIAN_POINT('Ctrl Pts',(-19.6078094898801,47.3741978429241,121.917497147555)) ;
#40654=CARTESIAN_POINT('Ctrl Pts',(-19.7724614957895,47.5641463056221,122.26180879175)) ;
#40655=CARTESIAN_POINT('Ctrl Pts',(-19.8632760201086,47.3841572252123,121.974310927334)) ;
#40656=CARTESIAN_POINT('Ctrl Pts',(-19.966662779158,47.5741440652745,122.342257817906)) ;
#40657=CARTESIAN_POINT('Ctrl Pts',(-20.106026651874,47.3941549848646,122.074874782369)) ;
#40658=CARTESIAN_POINT('Ctrl Pts',(-20.1444477349424,47.5841802014768,122.455869269298)) ;
#40659=CARTESIAN_POINT('Ctrl Pts',(-20.3282563986767,47.4041911210669,122.21689139883)) ;
#40660=CARTESIAN_POINT('Ctrl Pts',(-20.2971040279646,47.5940309989677,122.595810595244)) ;
#40661=CARTESIAN_POINT('Ctrl Pts',(-20.5190752000147,47.4140419185579,122.391820347665)) ;
#40662=CARTESIAN_POINT('Ctrl Pts',(-20.425042108738,47.603991864044,122.761583938118)) ;
#40663=CARTESIAN_POINT('Ctrl Pts',(-20.6789956607741,47.4240027836341,122.599038838979)) ;
#40664=CARTESIAN_POINT('Ctrl Pts',(-20.5226996631887,47.6140207316744,122.948455189612)) ;
#40665=CARTESIAN_POINT('Ctrl Pts',(-20.8010651624345,47.4340316512646,122.832629226819)) ;
#40666=CARTESIAN_POINT('Ctrl Pts',(-20.5857281504088,47.6239309678108,123.147028040722)) ;
#40667=CARTESIAN_POINT('Ctrl Pts',(-20.8798481804422,47.443941887401,123.080846336927)) ;
#40668=CARTESIAN_POINT('Ctrl Pts',(-20.6139336283943,47.6338659211253,123.353984814139)) ;
#40669=CARTESIAN_POINT('Ctrl Pts',(-20.9151022555058,47.4538768407155,123.339542816452)) ;
#40670=CARTESIAN_POINT('Ctrl Pts',(-20.605496943485,47.6439068515349,123.564903134672)) ;
#40671=CARTESIAN_POINT('Ctrl Pts',(-20.9045535939889,47.4639177711251,123.603190650001)) ;
#40672=CARTESIAN_POINT('Ctrl Pts',(-20.5613779871071,47.6537947483165,123.768050424334)) ;
#40673=CARTESIAN_POINT('Ctrl Pts',(-20.8494021157821,47.4738056679067,123.85712432545)) ;
#40674=CARTESIAN_POINT('Ctrl Pts',(-20.4822143423052,47.6637841999752,123.962563095657)) ;
#40675=CARTESIAN_POINT('Ctrl Pts',(-20.7504449184819,47.4837951195654,124.100264163636)) ;
#40676=CARTESIAN_POINT('Ctrl Pts',(-20.370678012507,47.6737432903405,124.139744915088)) ;
#40677=CARTESIAN_POINT('Ctrl Pts',(-20.6110220669894,47.4937542099307,124.321740017051)) ;
#40678=CARTESIAN_POINT('Ctrl Pts',(-20.2313246232406,47.6836406026468,124.294278132182)) ;
#40679=CARTESIAN_POINT('Ctrl Pts',(-20.4368281965644,47.503651522237,124.514904688162)) ;
#40680=CARTESIAN_POINT('Ctrl Pts',(-20.0645809253998,47.6936970285471,124.424226886793)) ;
#40681=CARTESIAN_POINT('Ctrl Pts',(-20.2283967744632,47.5137079481373,124.677338457661)) ;
#40682=CARTESIAN_POINT('Ctrl Pts',(-19.8812864921283,47.7035670311368,124.521524514142)) ;
#40683=CARTESIAN_POINT('Ctrl Pts',(-19.9992773799841,47.523577950727,124.798958001581)) ;
#40684=CARTESIAN_POINT('Ctrl Pts',(-19.6813729094116,47.7135709643141,124.586772503536)) ;
#40685=CARTESIAN_POINT('Ctrl Pts',(-19.7493845402338,47.5335818839042,124.880515352812)) ;
#40686=CARTESIAN_POINT('Ctrl Pts',(-19.4734437265146,47.723558224778,124.616166289177)) ;
#40687=CARTESIAN_POINT('Ctrl Pts',(-19.489472364039,47.5435691443681,124.917254732938)) ;
#40688=CARTESIAN_POINT('Ctrl Pts',(-19.2627853496724,47.7335852763637,124.608859964159)) ;
#40689=CARTESIAN_POINT('Ctrl Pts',(-19.2261503134939,47.5535961959539,124.908119290027)) ;
#40690=CARTESIAN_POINT('Ctrl Pts',(-19.0593193011781,47.7434763661898,124.565875611357)) ;
#40691=CARTESIAN_POINT('Ctrl Pts',(-18.9718149570736,47.5634872857799,124.854385043572)) ;
#40692=CARTESIAN_POINT('Ctrl Pts',(-18.7998791514015,47.7567741209708,124.46180634869)) ;
#40693=CARTESIAN_POINT('Ctrl Pts',(-18.6475331408363,47.576785040561,124.72430028687)) ;
#40694=CARTESIAN_POINT('Ctrl Pts',(-18.5749055156603,47.769972180579,124.293953042302)) ;
#40695=CARTESIAN_POINT('Ctrl Pts',(-18.3663382798693,47.5899831001692,124.514511431448)) ;
#40696=CARTESIAN_POINT('Ctrl Pts',(-18.4005844763,47.7833689211482,124.072822952987)) ;
#40697=CARTESIAN_POINT('Ctrl Pts',(-18.1483991887815,47.6033798407383,124.23805464201)) ;
#40698=CARTESIAN_POINT('Ctrl Pts',(-18.3021342969201,47.7932398332216,123.890089252221)) ;
#40699=CARTESIAN_POINT('Ctrl Pts',(-18.0253471436318,47.6132507528118,124.009644853033)) ;
#40700=CARTESIAN_POINT('Ctrl Pts',(-18.2356106700847,47.8033133949897,123.689082460906)) ;
#40701=CARTESIAN_POINT('Ctrl Pts',(-17.9421929510955,47.6233243145799,123.758382877835)) ;
#40702=CARTESIAN_POINT('Ctrl Pts',(-18.2055029737511,47.8131348075781,123.484761908509)) ;
#40703=CARTESIAN_POINT('Ctrl Pts',(-17.9045616883092,47.6331457271682,123.502983370992)) ;
#40704=CARTESIAN_POINT('Ctrl Pts',(-18.2112771538204,47.8232088248091,123.273106955294)) ;
#40705=CARTESIAN_POINT('Ctrl Pts',(-17.9117818429639,47.6432197443993,123.238412336135)) ;
#40706=CARTESIAN_POINT('Ctrl Pts',(-18.2665340735366,47.8363676117737,123.001975829454)) ;
#40707=CARTESIAN_POINT('Ctrl Pts',(-17.9808569614188,47.6563785313638,122.899509564603)) ;
#40708=CARTESIAN_POINT('Ctrl Pts',(-18.3927847313785,47.8497337148678,122.747421002799)) ;
#40709=CARTESIAN_POINT('Ctrl Pts',(-18.138643663301,47.669744634458,122.581350825169)) ;
#40710=CARTESIAN_POINT('Ctrl Pts',(-18.5783616406369,47.8630476497569,122.537834672679)) ;
#40711=CARTESIAN_POINT('Ctrl Pts',(-18.3706523157878,47.6830585693471,122.319320691022)) ;
#40712=CARTESIAN_POINT('Ctrl Pts',(-18.7409869953793,47.8729476892044,122.407978701696)) ;
#40713=CARTESIAN_POINT('Ctrl Pts',(-18.5739282398192,47.6929586087946,122.157012936073)) ;
#40714=CARTESIAN_POINT('Ctrl Pts',(-18.924736336014,47.8829120923389,122.307361857159)) ;
#40715=CARTESIAN_POINT('Ctrl Pts',(-18.803618171693,47.7029230119291,122.031241515274)) ;
#40716=CARTESIAN_POINT('Ctrl Pts',(-19.124525129965,47.89294205946,122.239917422604)) ;
#40717=CARTESIAN_POINT('Ctrl Pts',(-19.053353575871,47.7129529790502,121.946938831244)) ;
#40718=CARTESIAN_POINT('Ctrl Pts',(-19.3303060797298,47.9028443360691,122.20850438304)) ;
#40719=CARTESIAN_POINT('Ctrl Pts',(-19.310583887986,47.7228552556593,121.907675661844)) ;
#40720=CARTESIAN_POINT('Ctrl Pts',(-19.6091875472562,47.9161102652382,122.214220010693)) ;
#40721=CARTESIAN_POINT('Ctrl Pts',(-19.6591650885783,47.7361211848284,121.914819682734)) ;
#40722=CARTESIAN_POINT('Ctrl Pts',(-19.9485239198388,47.9327317963447,122.312705470027)) ;
#40723=CARTESIAN_POINT('Ctrl Pts',(-20.0833550247986,47.7527427159348,122.03793050963)) ;
#40724=CARTESIAN_POINT('Ctrl Pts',(-20.2902037781463,47.9526066249893,122.561462918073)) ;
#40725=CARTESIAN_POINT('Ctrl Pts',(-20.5104537296024,47.7726175445795,122.348898696979)) ;
#40726=CARTESIAN_POINT('Ctrl Pts',(-20.4884640691053,47.9692798330912,122.855376240776)) ;
#40727=CARTESIAN_POINT('Ctrl Pts',(-20.7582479358971,47.7892907526814,122.716231896323)) ;
#40728=CARTESIAN_POINT('Ctrl Pts',(-20.5789910924744,47.9825309580725,123.118806998675)) ;
#40729=CARTESIAN_POINT('Ctrl Pts',(-20.8714295869676,47.8025418776626,123.045575912821)) ;
#40730=CARTESIAN_POINT('Ctrl Pts',(-20.6233964771784,47.9957732768933,123.393706926206)) ;
#40731=CARTESIAN_POINT('Ctrl Pts',(-20.9269298435313,47.8157841964835,123.38917831621)) ;
#40732=CARTESIAN_POINT('Ctrl Pts',(-20.5867718231029,48.0125065172328,123.747531507057)) ;
#40733=CARTESIAN_POINT('Ctrl Pts',(-20.8811455204018,47.8325174368229,123.83147612068)) ;
#40734=CARTESIAN_POINT('Ctrl Pts',(-20.4028036698389,48.0323356654207,124.126994342041)) ;
#40735=CARTESIAN_POINT('Ctrl Pts',(-20.6511822087016,47.8523465850109,124.305796219688)) ;
#40736=CARTESIAN_POINT('Ctrl Pts',(-20.0997742547527,48.0522603605214,124.422927439283)) ;
#40737=CARTESIAN_POINT('Ctrl Pts',(-20.2723934902677,47.8722712801115,124.67571100162)) ;
#40738=CARTESIAN_POINT('Ctrl Pts',(-19.7138146747958,48.0721835891048,124.597703149849)) ;
#40739=CARTESIAN_POINT('Ctrl Pts',(-19.789943257648,47.892194508695,124.894176873647)) ;
#40740=CARTESIAN_POINT('Ctrl Pts',(-19.2914240334227,48.0921107282309,124.630406193651)) ;
#40741=CARTESIAN_POINT('Ctrl Pts',(-19.2619554888024,47.9121216478211,124.935052545487)) ;
#40742=CARTESIAN_POINT('Ctrl Pts',(-18.8840463674362,48.1119871908466,124.517801066557)) ;
#40743=CARTESIAN_POINT('Ctrl Pts',(-18.7527354696234,47.9319981104368,124.794293876261)) ;
#40744=CARTESIAN_POINT('Ctrl Pts',(-18.5376979877752,48.1319644194519,124.271899046843)) ;
#40745=CARTESIAN_POINT('Ctrl Pts',(-18.3198015892521,47.9519753390421,124.486914551097)) ;
#40746=CARTESIAN_POINT('Ctrl Pts',(-18.2968188645784,48.1518992774256,123.923081812922)) ;
#40747=CARTESIAN_POINT('Ctrl Pts',(-18.0187050937589,47.9719101970158,124.050892286843)) ;
#40748=CARTESIAN_POINT('Ctrl Pts',(-18.1892385120565,48.1717957263564,123.513969714441)) ;
#40749=CARTESIAN_POINT('Ctrl Pts',(-17.8842318765128,47.9918066459466,123.539502996673)) ;
#40750=CARTESIAN_POINT('Ctrl Pts',(-18.2273051805781,48.191717010423,123.092084857011)) ;
#40751=CARTESIAN_POINT('Ctrl Pts',(-17.931816529744,48.0117279300131,123.01214812022)) ;
#40752=CARTESIAN_POINT('Ctrl Pts',(-18.4074959386059,48.2116736600939,122.707887148316)) ;
#40753=CARTESIAN_POINT('Ctrl Pts',(-18.1570558911113,48.0316845796841,122.531902035384)) ;
#40754=CARTESIAN_POINT('Ctrl Pts',(-18.7066336703321,48.2315509532055,122.409391624937)) ;
#40755=CARTESIAN_POINT('Ctrl Pts',(-18.5309774064704,48.0515618727957,122.158784664418)) ;
#40756=CARTESIAN_POINT('Ctrl Pts',(-19.0894690754,48.251437425434,122.229752123671)) ;
#40757=CARTESIAN_POINT('Ctrl Pts',(-19.0095199143014,48.0714483450242,121.934235959728)) ;
#40758=CARTESIAN_POINT('Ctrl Pts',(-19.5143590700572,48.271498991358,122.191844649005)) ;
#40759=CARTESIAN_POINT('Ctrl Pts',(-19.5406334938979,48.0915099109482,121.886851609372)) ;
#40760=CARTESIAN_POINT('Ctrl Pts',(-19.9220000869853,48.2913393988987,122.300380775824)) ;
#40761=CARTESIAN_POINT('Ctrl Pts',(-20.0501821768605,48.1113503184889,122.022521216155)) ;
#40762=CARTESIAN_POINT('Ctrl Pts',(-20.2693591113835,48.3111907228717,122.540208509566)) ;
#40763=CARTESIAN_POINT('Ctrl Pts',(-20.484379980263,48.1312016424618,122.322303458177)) ;
#40764=CARTESIAN_POINT('Ctrl Pts',(-20.515946924029,48.3312439928231,122.887990451022)) ;
#40765=CARTESIAN_POINT('Ctrl Pts',(-20.7926161665068,48.1512549124133,122.757030819411)) ;
#40766=CARTESIAN_POINT('Ctrl Pts',(-20.6278740447954,48.3510646502064,123.29441743572)) ;
#40767=CARTESIAN_POINT('Ctrl Pts',(-20.9325258350394,48.1710755697966,123.265061844728)) ;
#40768=CARTESIAN_POINT('Ctrl Pts',(-20.594840913384,48.3710360715369,123.717637162342)) ;
#40769=CARTESIAN_POINT('Ctrl Pts',(-20.8912365983852,48.1910469911271,123.794086280591)) ;
#40770=CARTESIAN_POINT('Ctrl Pts',(-20.4200275936189,48.3909295639006,124.102979449163)) ;
#40771=CARTESIAN_POINT('Ctrl Pts',(-20.6727225903165,48.2109404834908,124.275764014149)) ;
#40772=CARTESIAN_POINT('Ctrl Pts',(-20.1222338289871,48.4109536501417,124.407148329069)) ;
#40773=CARTESIAN_POINT('Ctrl Pts',(-20.3004819425232,48.2309645697319,124.655976968118)) ;
#40774=CARTESIAN_POINT('Ctrl Pts',(-19.7426972067717,48.4307585292546,124.589684508702)) ;
#40775=CARTESIAN_POINT('Ctrl Pts',(-19.8260643109715,48.2507694488447,124.884148701438)) ;
#40776=CARTESIAN_POINT('Ctrl Pts',(-19.3205665484207,48.4507175449524,124.633213336041)) ;
#40777=CARTESIAN_POINT('Ctrl Pts',(-19.2984016894082,48.2707284645426,124.938563164656)) ;
#40778=CARTESIAN_POINT('Ctrl Pts',(-18.9085978348677,48.4707035685815,124.528976750497)) ;
#40779=CARTESIAN_POINT('Ctrl Pts',(-18.7834401752253,48.2907144881717,124.808270536244)) ;
#40780=CARTESIAN_POINT('Ctrl Pts',(-18.5595521592662,48.490512064342,124.293192736646)) ;
#40781=CARTESIAN_POINT('Ctrl Pts',(-18.347132448287,48.3105229839322,124.513544556364)) ;
#40782=CARTESIAN_POINT('Ctrl Pts',(-18.3093912570992,48.5104947034476,123.949871011709)) ;
#40783=CARTESIAN_POINT('Ctrl Pts',(-18.0344280932118,48.3305056230378,124.084394876758)) ;
#40784=CARTESIAN_POINT('Ctrl Pts',(-18.1920511017376,48.5303761512416,123.543638375906)) ;
#40785=CARTESIAN_POINT('Ctrl Pts',(-17.8877491678814,48.3503870708318,123.576606049557)) ;
#40786=CARTESIAN_POINT('Ctrl Pts',(-18.2201380169056,48.5503326179791,123.120331661826)) ;
#40787=CARTESIAN_POINT('Ctrl Pts',(-17.9228534216477,48.3703435375693,123.047472668658)) ;
#40788=CARTESIAN_POINT('Ctrl Pts',(-18.3901149333137,48.5702100149347,122.733295429989)) ;
#40789=CARTESIAN_POINT('Ctrl Pts',(-18.135320026782,48.3902209345249,122.563676201038)) ;
#40790=CARTESIAN_POINT('Ctrl Pts',(-18.6832494392057,48.59019196111,122.425805232135)) ;
#40791=CARTESIAN_POINT('Ctrl Pts',(-18.5017348374679,48.4102028807002,122.179310317694)) ;
#40792=CARTESIAN_POINT('Ctrl Pts',(-19.0629244099466,48.6101210601467,122.237437305555)) ;
#40793=CARTESIAN_POINT('Ctrl Pts',(-18.9763255338621,48.4301319797369,121.943845821866)) ;
#40794=CARTESIAN_POINT('Ctrl Pts',(-19.483901793505,48.6300496833594,122.189890024133)) ;
#40795=CARTESIAN_POINT('Ctrl Pts',(-19.5025485758223,48.4500606029495,121.88440856262)) ;
#40796=CARTESIAN_POINT('Ctrl Pts',(-19.8941924839498,48.6498840074658,122.2876543526)) ;
#40797=CARTESIAN_POINT('Ctrl Pts',(-20.0154041734729,48.469894927056,122.006602474258)) ;
#40798=CARTESIAN_POINT('Ctrl Pts',(-20.1900657132766,48.6665362948492,122.481970833508)) ;
#40799=CARTESIAN_POINT('Ctrl Pts',(-20.3852740340887,48.4865472144393,122.249514009175)) ;
#40800=CARTESIAN_POINT('Ctrl Pts',(-20.375507427574,48.6797967958714,122.690222552236)) ;
#40801=CARTESIAN_POINT('Ctrl Pts',(-20.6170557320591,48.4998077154616,122.509808729573)) ;
#40802=CARTESIAN_POINT('Ctrl Pts',(-20.4862754015006,48.6897982730727,122.868932780703)) ;
#40803=CARTESIAN_POINT('Ctrl Pts',(-20.7555225669934,48.5098091926629,122.733198872914)) ;
#40804=CARTESIAN_POINT('Ctrl Pts',(-20.5642475378503,48.6998302939322,123.064902655755)) ;
#40805=CARTESIAN_POINT('Ctrl Pts',(-20.8529891979542,48.5198412135224,122.978158629143)) ;
#40806=CARTESIAN_POINT('Ctrl Pts',(-20.6065360548538,48.7096938376577,123.267899186555)) ;
#40807=CARTESIAN_POINT('Ctrl Pts',(-20.905851938362,48.5297047572479,123.231906669107)) ;
#40808=CARTESIAN_POINT('Ctrl Pts',(-20.6135560240591,48.7196625513279,123.477368148513)) ;
#40809=CARTESIAN_POINT('Ctrl Pts',(-20.9146324102644,48.539673470918,123.493731289985)) ;
#40810=CARTESIAN_POINT('Ctrl Pts',(-20.5737423786962,48.7330082987316,123.755033330118)) ;
#40811=CARTESIAN_POINT('Ctrl Pts',(-20.8648547232343,48.5530192183217,123.840870176968)) ;
#40812=CARTESIAN_POINT('Ctrl Pts',(-20.4644055794944,48.7461588538042,124.012444095883)) ;
#40813=CARTESIAN_POINT('Ctrl Pts',(-20.7281894338914,48.5661697733944,124.16259745945)) ;
#40814=CARTESIAN_POINT('Ctrl Pts',(-20.2913023971137,48.7595442343541,124.234297005858)) ;
#40815=CARTESIAN_POINT('Ctrl Pts',(-20.5118249049467,48.5795551539443,124.43990359673)) ;
#40816=CARTESIAN_POINT('Ctrl Pts',(-20.1368920609285,48.7694321703469,124.373504586034)) ;
#40817=CARTESIAN_POINT('Ctrl Pts',(-20.3188115906688,48.5894430899371,124.613917552895)) ;
#40818=CARTESIAN_POINT('Ctrl Pts',(-19.9590459239484,48.7794233601596,124.485212508452)) ;
#40819=CARTESIAN_POINT('Ctrl Pts',(-20.0965059872055,48.5994342797498,124.753554193892)) ;
#40820=CARTESIAN_POINT('Ctrl Pts',(-19.7652457599506,48.7893754586979,124.564139501548)) ;
#40821=CARTESIAN_POINT('Ctrl Pts',(-19.8542566549594,48.6093863782881,124.852215716906)) ;
#40822=CARTESIAN_POINT('Ctrl Pts',(-19.5587662011907,48.7994217151483,124.608490141116)) ;
#40823=CARTESIAN_POINT('Ctrl Pts',(-19.5961577410674,48.6194326347385,124.907656726874)) ;
#40824=CARTESIAN_POINT('Ctrl Pts',(-19.3518437628438,48.8092711625425,124.616313912249)) ;
#40825=CARTESIAN_POINT('Ctrl Pts',(-19.3375048370033,48.6292820821327,124.917439257237)) ;
#40826=CARTESIAN_POINT('Ctrl Pts',(-19.1442698754285,48.8192338150376,124.588420325865)) ;
#40827=CARTESIAN_POINT('Ctrl Pts',(-19.0780370222547,48.6392447346278,124.882575057836)) ;
#40828=CARTESIAN_POINT('Ctrl Pts',(-18.9435612342431,48.8292569006798,124.52425240661)) ;
#40829=CARTESIAN_POINT('Ctrl Pts',(-18.8271502999085,48.64926782027,124.802367820809)) ;
#40830=CARTESIAN_POINT('Ctrl Pts',(-18.7587343657275,48.8391820164367,124.427368142674)) ;
#40831=CARTESIAN_POINT('Ctrl Pts',(-18.5961153422088,48.6591929360269,124.681264951372)) ;
#40832=CARTESIAN_POINT('Ctrl Pts',(-18.5915035853904,48.8492344948365,124.298186724899)) ;
#40833=CARTESIAN_POINT('Ctrl Pts',(-18.3870750955286,48.6692454144267,124.519790373275)) ;
#40834=CARTESIAN_POINT('Ctrl Pts',(-18.4519608110317,48.8590859935392,124.14512278795)) ;
#40835=CARTESIAN_POINT('Ctrl Pts',(-18.2126444693524,48.6790969131294,124.328462267101)) ;
#40836=CARTESIAN_POINT('Ctrl Pts',(-18.3393227852187,48.8690577327418,123.968347894014)) ;
#40837=CARTESIAN_POINT('Ctrl Pts',(-18.0718445075034,48.6890686523319,124.107495060941)) ;
#40838=CARTESIAN_POINT('Ctrl Pts',(-18.2589016789919,48.8790529405074,123.774178747308)) ;
#40839=CARTESIAN_POINT('Ctrl Pts',(-17.9713155068526,48.6990638600976,123.864784625914)) ;
#40840=CARTESIAN_POINT('Ctrl Pts',(-18.2135023400313,48.8890869419765,123.568194672117)) ;
#40841=CARTESIAN_POINT('Ctrl Pts',(-17.9145635741689,48.7090978615667,123.60730509988)) ;
#40842=CARTESIAN_POINT('Ctrl Pts',(-18.2043860504649,48.8989423000689,123.361183900461)) ;
#40843=CARTESIAN_POINT('Ctrl Pts',(-17.9031654068382,48.7189532196591,123.348541528171)) ;
#40844=CARTESIAN_POINT('Ctrl Pts',(-18.2314583491406,48.9089417756622,123.152751792762)) ;
#40845=CARTESIAN_POINT('Ctrl Pts',(-17.9370030265892,48.7289526952524,123.08800094487)) ;
#40846=CARTESIAN_POINT('Ctrl Pts',(-18.2934466731116,48.9188362241573,122.954149298326)) ;
#40847=CARTESIAN_POINT('Ctrl Pts',(-18.0144858730906,48.7388471437475,122.839746756347)) ;
#40848=CARTESIAN_POINT('Ctrl Pts',(-18.3906263668652,48.928899348385,122.766272454152)) ;
#40849=CARTESIAN_POINT('Ctrl Pts',(-18.1359580111579,48.7489102679752,122.604899456837)) ;
#40850=CARTESIAN_POINT('Ctrl Pts',(-18.5159623132325,48.9387389747136,122.601663674346)) ;
#40851=CARTESIAN_POINT('Ctrl Pts',(-18.2926260056049,48.7587498943038,122.399136493394)) ;
#40852=CARTESIAN_POINT('Ctrl Pts',(-18.6712011618515,48.9488022097566,122.457974021879)) ;
#40853=CARTESIAN_POINT('Ctrl Pts',(-18.4866726839384,48.7688131293468,122.219522458064)) ;
#40854=CARTESIAN_POINT('Ctrl Pts',(-18.8461785268419,48.9586962149906,122.345468773217)) ;
#40855=CARTESIAN_POINT('Ctrl Pts',(-18.7053931822767,48.7787071345808,122.078888414261)) ;
#40856=CARTESIAN_POINT('Ctrl Pts',(-19.038712835581,48.9686389282064,122.264147456417)) ;
#40857=CARTESIAN_POINT('Ctrl Pts',(-18.9460602718155,48.7886498477966,121.977234200154)) ;
#40858=CARTESIAN_POINT('Ctrl Pts',(-19.2437694434536,48.9786446680046,122.217145600225)) ;
#40859=CARTESIAN_POINT('Ctrl Pts',(-19.2023805081948,48.7986555875947,121.918479266263)) ;
#40860=CARTESIAN_POINT('Ctrl Pts',(-19.4541758562915,48.988665570151,122.206684633886)) ;
#40861=CARTESIAN_POINT('Ctrl Pts',(-19.4653884139516,48.8086764897411,121.905400359925)) ;
#40862=CARTESIAN_POINT('Ctrl Pts',(-19.6605286713295,48.9985563401998,122.232339508242)) ;
#40863=CARTESIAN_POINT('Ctrl Pts',(-19.7233301714407,48.81856725979,121.937466358533)) ;
#40864=CARTESIAN_POINT('Ctrl Pts',(-19.8613941607014,49.0085477509796,122.29375208743)) ;
#40865=CARTESIAN_POINT('Ctrl Pts',(-19.9744129235996,48.8285586705698,122.014229612628)) ;
#40866=CARTESIAN_POINT('Ctrl Pts',(-20.0477097453618,49.0184960966441,122.388760410401)) ;
#40867=CARTESIAN_POINT('Ctrl Pts',(-20.207308842741,48.8385070162342,122.132987793713)) ;
#40868=CARTESIAN_POINT('Ctrl Pts',(-20.2149235430791,49.0284409547052,122.514293134598)) ;
#40869=CARTESIAN_POINT('Ctrl Pts',(-20.4163278634492,48.8484518742954,122.28990183288)) ;
#40870=CARTESIAN_POINT('Ctrl Pts',(-20.3591274679965,49.0384957900982,122.668825290875)) ;
#40871=CARTESIAN_POINT('Ctrl Pts',(-20.596584606347,48.8585067096884,122.483065165186)) ;
#40872=CARTESIAN_POINT('Ctrl Pts',(-20.4719672533018,49.0483181621996,122.841786669687)) ;
#40873=CARTESIAN_POINT('Ctrl Pts',(-20.7376368969184,48.8683290817898,122.699266149555)) ;
#40874=CARTESIAN_POINT('Ctrl Pts',(-20.5553257636715,49.0583740296434,123.036047834246)) ;
#40875=CARTESIAN_POINT('Ctrl Pts',(-20.841837268975,48.8783849492335,122.942091527924)) ;
#40876=CARTESIAN_POINT('Ctrl Pts',(-20.6027766814193,49.0683147595013,123.239583217983)) ;
#40877=CARTESIAN_POINT('Ctrl Pts',(-20.901153475683,48.8883256790915,123.196510502695)) ;
#40878=CARTESIAN_POINT('Ctrl Pts',(-20.6147759350692,49.0782190980524,123.447461236143)) ;
#40879=CARTESIAN_POINT('Ctrl Pts',(-20.9161549877404,48.8982300176426,123.456358415648)) ;
#40880=CARTESIAN_POINT('Ctrl Pts',(-20.5900184388483,49.0882657794809,123.657200174385)) ;
#40881=CARTESIAN_POINT('Ctrl Pts',(-20.8852105593399,48.9082766990711,123.718532273729)) ;
#40882=CARTESIAN_POINT('Ctrl Pts',(-20.5303023151086,49.0981612869501,123.856515276786)) ;
#40883=CARTESIAN_POINT('Ctrl Pts',(-20.8105675406621,48.9181722065403,123.967677397278)) ;
#40884=CARTESIAN_POINT('Ctrl Pts',(-20.4353377015861,49.1082235554488,124.045507278438)) ;
#40885=CARTESIAN_POINT('Ctrl Pts',(-20.6918640067606,48.9282344750389,124.203918318758)) ;
#40886=CARTESIAN_POINT('Ctrl Pts',(-20.3118353609742,49.1180655457194,124.211547456422)) ;
#40887=CARTESIAN_POINT('Ctrl Pts',(-20.5374874733273,48.9380764653096,124.411470652652)) ;
#40888=CARTESIAN_POINT('Ctrl Pts',(-20.1594306056428,49.1280589626003,124.356110189049)) ;
#40889=CARTESIAN_POINT('Ctrl Pts',(-20.3469829663969,48.9480698821905,124.592175832541)) ;
#40890=CARTESIAN_POINT('Ctrl Pts',(-19.9854133922224,49.1379834504525,124.471260343078)) ;
#40891=CARTESIAN_POINT('Ctrl Pts',(-20.1294622772361,48.9579943700427,124.736115686186)) ;
#40892=CARTESIAN_POINT('Ctrl Pts',(-19.7927208813877,49.147983084361,124.555263507083)) ;
#40893=CARTESIAN_POINT('Ctrl Pts',(-19.8885974147737,48.9679940039512,124.841121711995)) ;
#40894=CARTESIAN_POINT('Ctrl Pts',(-19.5886002486788,49.1579691946177,124.604484612063)) ;
#40895=CARTESIAN_POINT('Ctrl Pts',(-19.6334469697775,48.9779801142079,124.902650275678)) ;
#40896=CARTESIAN_POINT('Ctrl Pts',(-19.3780258214189,49.1680051458049,124.617357030462)) ;
#40897=CARTESIAN_POINT('Ctrl Pts',(-19.3702291570115,48.9880160653951,124.918743054882)) ;
#40898=CARTESIAN_POINT('Ctrl Pts',(-19.1720854488287,49.1778617841397,124.594203709604)) ;
#40899=CARTESIAN_POINT('Ctrl Pts',(-19.1128025382684,48.9978727037298,124.889803469865)) ;
#40900=CARTESIAN_POINT('Ctrl Pts',(-18.9703969120688,49.1878607442177,124.535088681931)) ;
#40901=CARTESIAN_POINT('Ctrl Pts',(-18.8606911455378,49.0078716638079,124.815911669499)) ;
#40902=CARTESIAN_POINT('Ctrl Pts',(-18.7838271969103,49.1977559745315,124.442990126703)) ;
#40903=CARTESIAN_POINT('Ctrl Pts',(-18.6274774419771,49.0177668941216,124.700789980543)) ;
#40904=CARTESIAN_POINT('Ctrl Pts',(-18.6133446048038,49.2078164870001,124.317858094273)) ;
#40905=CARTESIAN_POINT('Ctrl Pts',(-18.4143731817595,49.0278274065903,124.544376734634)) ;
#40906=CARTESIAN_POINT('Ctrl Pts',(-18.470133520923,49.2176657785463,124.168284568055)) ;
#40907=CARTESIAN_POINT('Ctrl Pts',(-18.235357152959,49.0376766981364,124.35741046968)) ;
#40908=CARTESIAN_POINT('Ctrl Pts',(-18.3525585485733,49.2276929644785,123.993322107595)) ;
#40909=CARTESIAN_POINT('Ctrl Pts',(-18.0883869154399,49.0477038840687,124.138708462397)) ;
#40910=CARTESIAN_POINT('Ctrl Pts',(-18.2676375468135,49.2377215009378,123.800338049473)) ;
#40911=CARTESIAN_POINT('Ctrl Pts',(-17.9822338382252,49.057732420528,123.897479268206)) ;
#40912=CARTESIAN_POINT('Ctrl Pts',(-18.2180547672955,49.2475667409028,123.599398819481)) ;
#40913=CARTESIAN_POINT('Ctrl Pts',(-17.920253245843,49.067577660493,123.646304603667)) ;
#40914=CARTESIAN_POINT('Ctrl Pts',(-18.2033462478986,49.257557435826,123.389873464327)) ;
#40915=CARTESIAN_POINT('Ctrl Pts',(-17.9018658551687,49.0775683554161,123.384397836006)) ;
#40916=CARTESIAN_POINT('Ctrl Pts',(-18.2258094823577,49.2675952565846,123.180046491113)) ;
#40917=CARTESIAN_POINT('Ctrl Pts',(-17.9299430169483,49.0876061761748,123.122114050763)) ;
#40918=CARTESIAN_POINT('Ctrl Pts',(-18.282899951332,49.2774398503615,122.981108060184)) ;
#40919=CARTESIAN_POINT('Ctrl Pts',(-18.0013047262226,49.0974507699517,122.873439403383)) ;
#40920=CARTESIAN_POINT('Ctrl Pts',(-18.3745381888825,49.2874238457376,122.792294663389)) ;
#40921=CARTESIAN_POINT('Ctrl Pts',(-18.1158511804097,49.1074347653277,122.637421711122)) ;
#40922=CARTESIAN_POINT('Ctrl Pts',(-18.4971732872616,49.297372894299,122.622845943854)) ;
#40923=CARTESIAN_POINT('Ctrl Pts',(-18.2691440174717,49.1173838138892,122.42560946912)) ;
#40924=CARTESIAN_POINT('Ctrl Pts',(-18.6480139790816,49.3073753332735,122.476322024514)) ;
#40925=CARTESIAN_POINT('Ctrl Pts',(-18.4576938725273,49.1273862528637,122.242453382351)) ;
#40926=CARTESIAN_POINT('Ctrl Pts',(-18.8224872342568,49.3173965745699,122.358233047741)) ;
#40927=CARTESIAN_POINT('Ctrl Pts',(-18.6757844900772,49.1374074941601,122.09484081394)) ;
#40928=CARTESIAN_POINT('Ctrl Pts',(-19.0122435632454,49.3272892530094,122.273107300004)) ;
#40929=CARTESIAN_POINT('Ctrl Pts',(-18.9129800736581,49.1473001725995,121.988431832864)) ;
#40930=CARTESIAN_POINT('Ctrl Pts',(-19.2157981994734,49.337279306957,122.221395750134)) ;
#40931=CARTESIAN_POINT('Ctrl Pts',(-19.1674232251386,49.1572902265472,121.92379093172)) ;
#40932=CARTESIAN_POINT('Ctrl Pts',(-19.4245809336143,49.3472376681055,122.206012139912)) ;
#40933=CARTESIAN_POINT('Ctrl Pts',(-19.4284019621505,49.1672485876957,121.904559887183)) ;
#40934=CARTESIAN_POINT('Ctrl Pts',(-19.6317061321161,49.3571372949903,122.226481358477)) ;
#40935=CARTESIAN_POINT('Ctrl Pts',(-19.6873094647,49.1771482145805,121.930145178701)) ;
#40936=CARTESIAN_POINT('Ctrl Pts',(-19.8350793181158,49.3671851917937,122.283506518214)) ;
#40937=CARTESIAN_POINT('Ctrl Pts',(-19.9415261026208,49.1871961113839,122.001425268256)) ;
#40938=CARTESIAN_POINT('Ctrl Pts',(-20.0226907344885,49.3770805494297,122.373464971147)) ;
#40939=CARTESIAN_POINT('Ctrl Pts',(-20.1760417540459,49.1970914690199,122.113872563155)) ;
#40940=CARTESIAN_POINT('Ctrl Pts',(-20.1946471925884,49.3871422018863,122.496611414451)) ;
#40941=CARTESIAN_POINT('Ctrl Pts',(-20.390987809778,49.2071531214765,122.267804384086)) ;
#40942=CARTESIAN_POINT('Ctrl Pts',(-20.3394609229976,49.3969868061583,122.644483147191)) ;
#40943=CARTESIAN_POINT('Ctrl Pts',(-20.5720068054178,49.2169977257485,122.452644101935)) ;
#40944=CARTESIAN_POINT('Ctrl Pts',(-20.4583844624104,49.4069469278563,122.816823206098)) ;
#40945=CARTESIAN_POINT('Ctrl Pts',(-20.7206623097911,49.2269578474465,122.668068984901)) ;
#40946=CARTESIAN_POINT('Ctrl Pts',(-20.5458863827844,49.4169849622188,123.008849967238)) ;
#40947=CARTESIAN_POINT('Ctrl Pts',(-20.8300406887317,49.236995881809,122.908101813683)) ;
#40948=CARTESIAN_POINT('Ctrl Pts',(-20.5982321140661,49.4268592748053,123.209757190274)) ;
#40949=CARTESIAN_POINT('Ctrl Pts',(-20.8954741072966,49.2468701943954,123.159236671897)) ;
#40950=CARTESIAN_POINT('Ctrl Pts',(-20.6152137828225,49.436928755588,123.420738615319)) ;
#40951=CARTESIAN_POINT('Ctrl Pts',(-20.9167021697112,49.2569396751782,123.422962968095)) ;
#40952=CARTESIAN_POINT('Ctrl Pts',(-20.5958761668654,49.4467630916051,123.62659808383)) ;
#40953=CARTESIAN_POINT('Ctrl Pts',(-20.8925309749188,49.2667740111952,123.680288852966)) ;
#40954=CARTESIAN_POINT('Ctrl Pts',(-20.540545363407,49.4567960493333,123.83012921168)) ;
#40955=CARTESIAN_POINT('Ctrl Pts',(-20.8233682240622,49.2768069689235,123.934702843871)) ;
#40956=CARTESIAN_POINT('Ctrl Pts',(-20.4502978778667,49.4668164479085,124.020482337261)) ;
#40957=CARTESIAN_POINT('Ctrl Pts',(-20.7105597645197,49.2868273674987,124.17264463345)) ;
#40958=CARTESIAN_POINT('Ctrl Pts',(-20.3306741561224,49.4766820216797,124.189933002317)) ;
#40959=CARTESIAN_POINT('Ctrl Pts',(-20.5610300421518,49.2966929412699,124.3844593966)) ;
#40960=CARTESIAN_POINT('Ctrl Pts',(-20.1804401966572,49.4867508963358,124.339026315722)) ;
#40961=CARTESIAN_POINT('Ctrl Pts',(-20.3732384290745,49.306761815926,124.570826297065)) ;
#40962=CARTESIAN_POINT('Ctrl Pts',(-20.0104505357021,49.4965963272413,124.45713399561)) ;
#40963=CARTESIAN_POINT('Ctrl Pts',(-20.1607506292754,49.3166072468315,124.718462326093)) ;
#40964=CARTESIAN_POINT('Ctrl Pts',(-19.8202741615974,49.506575952112,124.545721379773)) ;
#40965=CARTESIAN_POINT('Ctrl Pts',(-19.9230300882305,49.3265868717022,124.82919713631)) ;
#40966=CARTESIAN_POINT('Ctrl Pts',(-19.6167083846425,49.5165946350261,124.599768391812)) ;
#40967=CARTESIAN_POINT('Ctrl Pts',(-19.6685730451503,49.3366055546162,124.896756529941)) ;
#40968=CARTESIAN_POINT('Ctrl Pts',(-19.4096938931667,49.5264779002099,124.617848281754)) ;
#40969=CARTESIAN_POINT('Ctrl Pts',(-19.4098038796016,49.3464888198001,124.919356964581)) ;
#40970=CARTESIAN_POINT('Ctrl Pts',(-19.198877107358,49.5365461943013,124.599282994167)) ;
#40971=CARTESIAN_POINT('Ctrl Pts',(-19.1462832607575,49.3565571138914,124.896150905587)) ;
#40972=CARTESIAN_POINT('Ctrl Pts',(-18.9991919639653,49.5463763244866,124.54591031217)) ;
#40973=CARTESIAN_POINT('Ctrl Pts',(-18.8966752356314,49.3663872440768,124.829435060351)) ;
#40974=CARTESIAN_POINT('Ctrl Pts',(-18.8072474578189,49.5564428727018,124.456856220617)) ;
#40975=CARTESIAN_POINT('Ctrl Pts',(-18.6567448317127,49.3764537922919,124.71811789698)) ;
#40976=CARTESIAN_POINT('Ctrl Pts',(-18.6367469946914,49.5663331213904,124.337807634366)) ;
#40977=CARTESIAN_POINT('Ctrl Pts',(-18.4436181844435,49.3863440409805,124.569306863468)) ;
#40978=CARTESIAN_POINT('Ctrl Pts',(-18.4876920453678,49.5763253031664,124.189801919102)) ;
#40979=CARTESIAN_POINT('Ctrl Pts',(-18.2572992165768,49.3963362227566,124.384299698953)) ;
#40980=CARTESIAN_POINT('Ctrl Pts',(-18.3671123398386,49.5862880837942,124.018548544852)) ;
#40981=CARTESIAN_POINT('Ctrl Pts',(-18.1065741068912,49.4062990033844,124.170232758751)) ;
#40982=CARTESIAN_POINT('Ctrl Pts',(-18.2781412601889,49.5961924884679,123.830276313694)) ;
#40983=CARTESIAN_POINT('Ctrl Pts',(-17.9953598076436,49.4162034080581,123.934891647495)) ;
#40984=CARTESIAN_POINT('Ctrl Pts',(-18.222510202651,49.606252482947,123.626250710745)) ;
#40985=CARTESIAN_POINT('Ctrl Pts',(-17.9258209626991,49.4262634025372,123.67985999985)) ;
#40986=CARTESIAN_POINT('Ctrl Pts',(-18.203376410996,49.6161011049168,123.420072742586)) ;
#40987=CARTESIAN_POINT('Ctrl Pts',(-17.9019035488752,49.436112024507,123.422136143484)) ;
#40988=CARTESIAN_POINT('Ctrl Pts',(-18.2201708403545,49.6261315443286,123.209883238116)) ;
#40989=CARTESIAN_POINT('Ctrl Pts',(-17.9228967150364,49.4461424639188,123.159399391349)) ;
#40990=CARTESIAN_POINT('Ctrl Pts',(-18.2735161472999,49.6361412599634,123.00629722832)) ;
#40991=CARTESIAN_POINT('Ctrl Pts',(-17.9895783324889,49.4561521795535,122.904916831254)) ;
#40992=CARTESIAN_POINT('Ctrl Pts',(-18.3603293584098,49.646052012656,122.816911028997)) ;
#40993=CARTESIAN_POINT('Ctrl Pts',(-18.0980952654857,49.4660629322462,122.66818328543)) ;
#40994=CARTESIAN_POINT('Ctrl Pts',(-18.4785136980993,49.6559812856024,122.644833121426)) ;
#40995=CARTESIAN_POINT('Ctrl Pts',(-18.2458263260203,49.4759922051926,122.453085432512)) ;
#40996=CARTESIAN_POINT('Ctrl Pts',(-18.6265668723548,49.666023976995,122.494326841967)) ;
#40997=CARTESIAN_POINT('Ctrl Pts',(-18.4308927790362,49.4860348965852,122.264952869132)) ;
#40998=CARTESIAN_POINT('Ctrl Pts',(-18.7957677209067,49.6759105102126,122.373596637961)) ;
#40999=CARTESIAN_POINT('Ctrl Pts',(-18.6423948660531,49.4959214298028,122.114039679002)) ;
#41000=CARTESIAN_POINT('Ctrl Pts',(-18.985209711551,49.6859036551446,122.282802300609)) ;
#41001=CARTESIAN_POINT('Ctrl Pts',(-18.8791977037607,49.5059145747348,122.00054701503)) ;
#41002=CARTESIAN_POINT('Ctrl Pts',(-19.1866107318813,49.6958493359811,122.226622842635)) ;
#41003=CARTESIAN_POINT('Ctrl Pts',(-19.1309496466669,49.5158602555713,121.93032286987)) ;
#41004=CARTESIAN_POINT('Ctrl Pts',(-19.3947080629283,49.7057965931296,122.205836498686)) ;
#41005=CARTESIAN_POINT('Ctrl Pts',(-19.391071934028,49.5258075127198,121.904340399556)) ;
#41006=CARTESIAN_POINT('Ctrl Pts',(-19.6053289184389,49.7158444970016,122.221892340969)) ;
#41007=CARTESIAN_POINT('Ctrl Pts',(-19.6543477211371,49.5358554165918,121.924410607044)) ;
#41008=CARTESIAN_POINT('Ctrl Pts',(-19.8059348665026,49.7256921960996,122.273064256038)) ;
#41009=CARTESIAN_POINT('Ctrl Pts',(-19.9051063909885,49.5457031156897,121.988376325606)) ;
#41010=CARTESIAN_POINT('Ctrl Pts',(-19.9970522744167,49.7356536870782,122.358669039494)) ;
#41011=CARTESIAN_POINT('Ctrl Pts',(-20.1440032594168,49.5556646066684,122.09538317843)) ;
#41012=CARTESIAN_POINT('Ctrl Pts',(-20.1714411232963,49.7456831494922,122.477202699067)) ;
#41013=CARTESIAN_POINT('Ctrl Pts',(-20.3619888763229,49.5656940690824,122.243550726911)) ;
#41014=CARTESIAN_POINT('Ctrl Pts',(-20.3208300958534,49.7555903805921,122.622336917083)) ;
#41015=CARTESIAN_POINT('Ctrl Pts',(-20.5487252566321,49.5756013001823,122.424969612964)) ;
#41016=CARTESIAN_POINT('Ctrl Pts',(-20.4435688894129,49.7655367592695,122.791613197818)) ;
#41017=CARTESIAN_POINT('Ctrl Pts',(-20.7021484058093,49.5855476788597,122.636565942027)) ;
#41018=CARTESIAN_POINT('Ctrl Pts',(-20.5356692060204,49.7755415280784,122.980728511161)) ;
#41019=CARTESIAN_POINT('Ctrl Pts',(-20.8172730521425,49.5955524476686,122.872960551579)) ;
#41020=CARTESIAN_POINT('Ctrl Pts',(-20.5933907296624,49.7855626490986,123.183338291841)) ;
#41021=CARTESIAN_POINT('Ctrl Pts',(-20.8894241945807,49.6055735686887,123.126222955813)) ;
#41022=CARTESIAN_POINT('Ctrl Pts',(-20.615012812427,49.7954535149512,123.390155066676)) ;
#41023=CARTESIAN_POINT('Ctrl Pts',(-20.9164510303949,49.6154644345414,123.384745011976)) ;
#41024=CARTESIAN_POINT('Ctrl Pts',(-20.6005593145487,49.8054443237105,123.599683369761)) ;
#41025=CARTESIAN_POINT('Ctrl Pts',(-20.8983831555145,49.6254552433007,123.646655535342)) ;
#41026=CARTESIAN_POINT('Ctrl Pts',(-20.5501038609146,49.8153949818908,123.802712023402)) ;
#41027=CARTESIAN_POINT('Ctrl Pts',(-20.8353127629609,49.635405901481,123.900441641749)) ;
#41028=CARTESIAN_POINT('Ctrl Pts',(-20.4655527395291,49.8253311915329,123.993707680392)) ;
#41029=CARTESIAN_POINT('Ctrl Pts',(-20.729622612963,49.6453421111231,124.139186358995)) ;
#41030=CARTESIAN_POINT('Ctrl Pts',(-20.3487747189752,49.8353143582578,124.168128009877)) ;
#41031=CARTESIAN_POINT('Ctrl Pts',(-20.5836489641355,49.655325277848,124.357211327717)) ;
#41032=CARTESIAN_POINT('Ctrl Pts',(-20.2023558449378,49.8453581554681,124.320235724213)) ;
#41033=CARTESIAN_POINT('Ctrl Pts',(-20.4006247563996,49.6653690750583,124.547345114795)) ;
#41034=CARTESIAN_POINT('Ctrl Pts',(-20.0356569177011,49.8551863716364,124.442367095108)) ;
#41035=CARTESIAN_POINT('Ctrl Pts',(-20.1922492122614,49.6751972912265,124.700009200447)) ;
#41036=CARTESIAN_POINT('Ctrl Pts',(-19.8457113842319,49.8652629391056,124.536063834955)) ;
#41037=CARTESIAN_POINT('Ctrl Pts',(-19.9548171286906,49.6852738586958,124.817128808166)) ;
#41038=CARTESIAN_POINT('Ctrl Pts',(-19.6468577220022,49.875115024795,124.594160167334)) ;
#41039=CARTESIAN_POINT('Ctrl Pts',(-19.7062485030575,49.6951259443852,124.889748332489)) ;
#41040=CARTESIAN_POINT('Ctrl Pts',(-19.4364134670954,49.8851882922004,124.617525881756)) ;
#41041=CARTESIAN_POINT('Ctrl Pts',(-19.4431934347675,49.7051992117906,124.918954084467)) ;
#41042=CARTESIAN_POINT('Ctrl Pts',(-19.2299283765432,49.895029708624,124.604248514442)) ;
#41043=CARTESIAN_POINT('Ctrl Pts',(-19.1850858539065,49.7150406282141,124.902355961702)) ;
#41044=CARTESIAN_POINT('Ctrl Pts',(-19.0262747705676,49.9049909667667,124.55549141664)) ;
#41045=CARTESIAN_POINT('Ctrl Pts',(-18.930518826785,49.7250018863569,124.841407931726)) ;
#41046=CARTESIAN_POINT('Ctrl Pts',(-18.8328848698317,49.9150276431986,124.471106946337)) ;
#41047=CARTESIAN_POINT('Ctrl Pts',(-18.6887821551141,49.7350385627888,124.735926054281)) ;
#41048=CARTESIAN_POINT('Ctrl Pts',(-18.6596380225063,49.9249062510625,124.35654118208)) ;
#41049=CARTESIAN_POINT('Ctrl Pts',(-18.4722236385822,49.7449171706527,124.592716974751)) ;
#41050=CARTESIAN_POINT('Ctrl Pts',(-18.5061473019625,49.9349664797013,124.211075267504)) ;
#41051=CARTESIAN_POINT('Ctrl Pts',(-18.2803615485747,49.7549773992915,124.410883615261)) ;
#41052=CARTESIAN_POINT('Ctrl Pts',(-18.3825837811286,49.9448334638621,124.044425289918)) ;
#41053=CARTESIAN_POINT('Ctrl Pts',(-18.1259078276159,49.7648443834522,124.202569344541)) ;
#41054=CARTESIAN_POINT('Ctrl Pts',(-18.2881916231086,49.9548390301148,123.856476139896)) ;
#41055=CARTESIAN_POINT('Ctrl Pts',(-18.0079191605339,49.774849949705,123.967632043621)) ;
#41056=CARTESIAN_POINT('Ctrl Pts',(-18.2280312076151,49.9648228185294,123.655353475487)) ;
#41057=CARTESIAN_POINT('Ctrl Pts',(-17.9327202356011,49.7848337381195,123.716228002362)) ;
#41058=CARTESIAN_POINT('Ctrl Pts',(-18.2037899064989,49.974868675332,123.445570734123)) ;
#41059=CARTESIAN_POINT('Ctrl Pts',(-17.9024202751132,49.7948795949222,123.45399954575)) ;
#41060=CARTESIAN_POINT('Ctrl Pts',(-18.2157993043397,49.984694552548,123.239349234005)) ;
#41061=CARTESIAN_POINT('Ctrl Pts',(-17.9174338427827,49.8047054721381,123.196221483271)) ;
#41062=CARTESIAN_POINT('Ctrl Pts',(-18.2635625382729,49.9946850283893,123.034820965476)) ;
#41063=CARTESIAN_POINT('Ctrl Pts',(-17.9771398351089,49.8146959479795,122.94056142547)) ;
#41064=CARTESIAN_POINT('Ctrl Pts',(-18.3470621028792,50.0047286042881,122.840884623417)) ;
#41065=CARTESIAN_POINT('Ctrl Pts',(-18.0815158765175,49.8247395238783,122.698141841132)) ;
#41066=CARTESIAN_POINT('Ctrl Pts',(-18.4600443984035,50.0145503965861,122.668054220945)) ;
#41067=CARTESIAN_POINT('Ctrl Pts',(-18.2227460406052,49.8345613161763,122.482103844495)) ;
#41068=CARTESIAN_POINT('Ctrl Pts',(-18.604009794299,50.024585362212,122.513843576675)) ;
#41069=CARTESIAN_POINT('Ctrl Pts',(-18.402704230727,49.8445962818022,122.289342033842)) ;
#41070=CARTESIAN_POINT('Ctrl Pts',(-18.7727524722638,50.034610279145,122.387565767662)) ;
#41071=CARTESIAN_POINT('Ctrl Pts',(-18.6136336980981,49.8546211987352,122.131496311186)) ;
#41072=CARTESIAN_POINT('Ctrl Pts',(-18.957405994649,50.0444622175212,122.293741975346)) ;
#41073=CARTESIAN_POINT('Ctrl Pts',(-18.8444524258335,49.8644731371114,122.014217927742)) ;
#41074=CARTESIAN_POINT('Ctrl Pts',(-19.1582192780616,50.0544531935459,122.23225581094)) ;
#41075=CARTESIAN_POINT('Ctrl Pts',(-19.0954698169748,49.8744641131361,121.937362207326)) ;
#41076=CARTESIAN_POINT('Ctrl Pts',(-19.3651677350279,50.0643710143496,122.206614010036)) ;
#41077=CARTESIAN_POINT('Ctrl Pts',(-19.3541562238225,49.8843819339398,121.905312031282)) ;
#41078=CARTESIAN_POINT('Ctrl Pts',(-19.5757056924692,50.0743997349142,122.217377366657)) ;
#41079=CARTESIAN_POINT('Ctrl Pts',(-19.6173285206094,49.8944106545043,121.918768394754)) ;
#41080=CARTESIAN_POINT('Ctrl Pts',(-19.7782617157918,50.0842826615234,122.263718063625)) ;
#41081=CARTESIAN_POINT('Ctrl Pts',(-19.8705237928477,49.9042935811135,121.97669658887)) ;
#41082=CARTESIAN_POINT('Ctrl Pts',(-19.9721356284537,50.0942869466428,122.345192272109)) ;
#41083=CARTESIAN_POINT('Ctrl Pts',(-20.1128653759059,49.914297866233,122.07854150103)) ;
#41084=CARTESIAN_POINT('Ctrl Pts',(-20.1485909447356,50.1042706278507,122.458909425641)) ;
#41085=CARTESIAN_POINT('Ctrl Pts',(-20.3334334359749,49.9242815474409,122.220689960758)) ;
#41086=CARTESIAN_POINT('Ctrl Pts',(-20.3033028222086,50.1143116265806,122.602499485329)) ;
#41087=CARTESIAN_POINT('Ctrl Pts',(-20.5268216964148,49.9343225461708,122.400179102823)) ;
#41088=CARTESIAN_POINT('Ctrl Pts',(-20.4283285557546,50.1241440714477,122.767114268604)) ;
#41089=CARTESIAN_POINT('Ctrl Pts',(-20.6831026136784,49.9441549910379,122.605949735481)) ;
#41090=CARTESIAN_POINT('Ctrl Pts',(-20.5249823851883,50.1341390698781,122.95368511086)) ;
#41091=CARTESIAN_POINT('Ctrl Pts',(-20.803917788404,49.9541499894682,122.839164524144)) ;
#41092=CARTESIAN_POINT('Ctrl Pts',(-20.5875768112403,50.1441706186277,123.155088324659)) ;
#41093=CARTESIAN_POINT('Ctrl Pts',(-20.8821585763182,49.9641815382179,123.090919199745)) ;
#41094=CARTESIAN_POINT('Ctrl Pts',(-20.6140645488152,50.1540359969332,123.360779768465)) ;
#41095=CARTESIAN_POINT('Ctrl Pts',(-20.915265961447,49.9740469165233,123.348034537655)) ;
#41096=CARTESIAN_POINT('Ctrl Pts',(-20.6049313505838,50.1639978443934,123.570016308224)) ;
#41097=CARTESIAN_POINT('Ctrl Pts',(-20.9038469303257,49.9840087639836,123.609580355005)) ;
#41098=CARTESIAN_POINT('Ctrl Pts',(-20.5589419047173,50.1740327852077,123.775896953256)) ;
#41099=CARTESIAN_POINT('Ctrl Pts',(-20.8463577367152,49.9940437047979,123.866930592324)) ;
#41100=CARTESIAN_POINT('Ctrl Pts',(-20.4794221936391,50.1839177462248,123.967925666986)) ;
#41101=CARTESIAN_POINT('Ctrl Pts',(-20.746955550935,50.003928665815,124.106966044007)) ;
#41102=CARTESIAN_POINT('Ctrl Pts',(-20.3657227466916,50.1939833551437,124.146355086132)) ;
#41103=CARTESIAN_POINT('Ctrl Pts',(-20.6048292012877,50.0139942747339,124.330001338976)) ;
#41104=CARTESIAN_POINT('Ctrl Pts',(-20.2260937776423,50.2038225301854,124.299012275186)) ;
#41105=CARTESIAN_POINT('Ctrl Pts',(-20.4302906277836,50.0238334497756,124.520821628154)) ;
#41106=CARTESIAN_POINT('Ctrl Pts',(-20.0585794048684,50.2138850856853,124.428165424389)) ;
#41107=CARTESIAN_POINT('Ctrl Pts',(-20.2208961768648,50.0338960052755,124.682260919723)) ;
#41108=CARTESIAN_POINT('Ctrl Pts',(-19.8741279084005,50.2237822603782,124.524475108692)) ;
#41109=CARTESIAN_POINT('Ctrl Pts',(-19.9903302029033,50.0437931799684,124.802645968582)) ;
#41110=CARTESIAN_POINT('Ctrl Pts',(-19.675310997847,50.2337129753016,124.588171794171)) ;
#41111=CARTESIAN_POINT('Ctrl Pts',(-19.741807958997,50.0537238948917,124.882264366588)) ;
#41112=CARTESIAN_POINT('Ctrl Pts',(-19.4660617887297,50.2437570033792,124.616460712568)) ;
#41113=CARTESIAN_POINT('Ctrl Pts',(-19.4802461248296,50.0637679229693,124.917622892758)) ;
#41114=CARTESIAN_POINT('Ctrl Pts',(-19.2583695225843,50.2536432052325,124.608282274617)) ;
#41115=CARTESIAN_POINT('Ctrl Pts',(-19.2206304688788,50.0736541248226,124.90739716592)) ;
#41116=CARTESIAN_POINT('Ctrl Pts',(-19.0530229072309,50.2636363716993,124.564006896081)) ;
#41117=CARTESIAN_POINT('Ctrl Pts',(-18.9639476699282,50.0836472912895,124.852050273557)) ;
#41118=CARTESIAN_POINT('Ctrl Pts',(-18.8594602487142,50.2735758426865,124.485214042851)) ;
#41119=CARTESIAN_POINT('Ctrl Pts',(-18.7219951492105,50.0935867622767,124.753556604805)) ;
#41120=CARTESIAN_POINT('Ctrl Pts',(-18.6811659538875,50.2835923570407,124.373207861046)) ;
#41121=CARTESIAN_POINT('Ctrl Pts',(-18.4991286839154,50.1036032766309,124.613546547517)) ;
#41122=CARTESIAN_POINT('Ctrl Pts',(-18.5262199735624,50.2935223835175,124.233262173088)) ;
#41123=CARTESIAN_POINT('Ctrl Pts',(-18.3054478577974,50.1135333031077,124.438612238889)) ;
#41124=CARTESIAN_POINT('Ctrl Pts',(-18.3964464306137,50.303574919027,124.066486390739)) ;
#41125=CARTESIAN_POINT('Ctrl Pts',(-18.1432330981543,50.1235858386171,124.230140853432)) ;
#41126=CARTESIAN_POINT('Ctrl Pts',(-18.2995125290276,50.3134213222466,123.883574583666)) ;
#41127=CARTESIAN_POINT('Ctrl Pts',(-18.0220679537271,50.1334322418368,124.001499451912)) ;
#41128=CARTESIAN_POINT('Ctrl Pts',(-18.2344247285052,50.3233833651007,123.684524259499)) ;
#41129=CARTESIAN_POINT('Ctrl Pts',(-17.9407108290362,50.1433942846909,123.752685556901)) ;
#41130=CARTESIAN_POINT('Ctrl Pts',(-18.204957703029,50.3334119158914,123.475747879046)) ;
#41131=CARTESIAN_POINT('Ctrl Pts',(-17.9038797901194,50.1534228354815,123.491714650902)) ;
#41132=CARTESIAN_POINT('Ctrl Pts',(-18.2120324651509,50.343322241609,123.267531291762)) ;
#41133=CARTESIAN_POINT('Ctrl Pts',(-17.9127260346725,50.1633331611992,123.23144379836)) ;
#41134=CARTESIAN_POINT('Ctrl Pts',(-18.2547290771079,50.3532571534386,123.063072199955)) ;
#41135=CARTESIAN_POINT('Ctrl Pts',(-17.9660995837992,50.1732680730287,122.975870378425)) ;
#41136=CARTESIAN_POINT('Ctrl Pts',(-18.3332815125372,50.3632981602067,122.867144842082)) ;
#41137=CARTESIAN_POINT('Ctrl Pts',(-18.064292748785,50.1833090797968,122.730962183321)) ;
#41138=CARTESIAN_POINT('Ctrl Pts',(-18.4428498626735,50.3731857930389,122.69048500063)) ;
#41139=CARTESIAN_POINT('Ctrl Pts',(-18.2012556639799,50.193196712629,122.510138724669)) ;
#41140=CARTESIAN_POINT('Ctrl Pts',(-18.5825766741435,50.3831762241369,122.533689688026)) ;
#41141=CARTESIAN_POINT('Ctrl Pts',(-18.3759163266947,50.2031871437271,122.314146410312)) ;
#41142=CARTESIAN_POINT('Ctrl Pts',(-18.7469116188207,50.3931316606941,122.404071107336)) ;
#41143=CARTESIAN_POINT('Ctrl Pts',(-18.5813368509821,50.2131425802843,122.152125343419)) ;
#41144=CARTESIAN_POINT('Ctrl Pts',(-18.930235657484,50.4030426087935,122.305070551018)) ;
#41145=CARTESIAN_POINT('Ctrl Pts',(-18.8104932141382,50.2230535283836,122.028377092492)) ;
#41146=CARTESIAN_POINT('Ctrl Pts',(-19.1299354241263,50.4130546848912,122.238492971298)) ;
#41147=CARTESIAN_POINT('Ctrl Pts',(-19.0601191774132,50.2330656044813,121.945157820118)) ;
#41148=CARTESIAN_POINT('Ctrl Pts',(-19.3385035067007,50.4230820069661,122.207980233689)) ;
#41149=CARTESIAN_POINT('Ctrl Pts',(-19.3208286510876,50.2430929265563,121.907019503195)) ;
#41150=CARTESIAN_POINT('Ctrl Pts',(-19.5457289876827,50.4329407819203,122.213520699819)) ;
#41151=CARTESIAN_POINT('Ctrl Pts',(-19.5798646279498,50.2529517015105,121.913948569408)) ;
#41152=CARTESIAN_POINT('Ctrl Pts',(-19.822185156653,50.4463669747327,122.270169175991)) ;
#41153=CARTESIAN_POINT('Ctrl Pts',(-19.9254133373787,50.2663778943229,121.984759551883)) ;
#41154=CARTESIAN_POINT('Ctrl Pts',(-20.0713938613618,50.4594509905141,122.394125106127)) ;
#41155=CARTESIAN_POINT('Ctrl Pts',(-20.2369013110958,50.2794619101043,122.139682808974)) ;
#41156=CARTESIAN_POINT('Ctrl Pts',(-20.2838339244026,50.4729244392694,122.581328585295)) ;
#41157=CARTESIAN_POINT('Ctrl Pts',(-20.5024950622099,50.2929353588595,122.373723117141)) ;
#41158=CARTESIAN_POINT('Ctrl Pts',(-20.4126445774875,50.4827573970752,122.743055891855)) ;
#41159=CARTESIAN_POINT('Ctrl Pts',(-20.66349684116,50.3027683166654,122.575877232231)) ;
#41160=CARTESIAN_POINT('Ctrl Pts',(-20.5134783735398,50.4927206705259,122.926629074294)) ;
#41161=CARTESIAN_POINT('Ctrl Pts',(-20.7895391336707,50.3127315901161,122.805346777451)) ;
#41162=CARTESIAN_POINT('Ctrl Pts',(-20.5809791036652,50.5027577443438,123.126549900042)) ;
#41163=CARTESIAN_POINT('Ctrl Pts',(-20.8739118056106,50.322768663934,123.055248323622)) ;
#41164=CARTESIAN_POINT('Ctrl Pts',(-20.6126206713393,50.5126327473555,123.331753130747)) ;
#41165=CARTESIAN_POINT('Ctrl Pts',(-20.913461175216,50.3326436669457,123.311752830496)) ;
#41166=CARTESIAN_POINT('Ctrl Pts',(-20.608057270493,50.5227004269817,123.543329168377)) ;
#41167=CARTESIAN_POINT('Ctrl Pts',(-20.9077542262007,50.3427113465718,123.576222416547)) ;
#41168=CARTESIAN_POINT('Ctrl Pts',(-20.5678626540345,50.5325412771994,123.746296518726)) ;
#41169=CARTESIAN_POINT('Ctrl Pts',(-20.8575080096766,50.3525521967896,123.829932935533)) ;
#41170=CARTESIAN_POINT('Ctrl Pts',(-20.4670213376231,50.5458774756753,124.007888589382)) ;
#41171=CARTESIAN_POINT('Ctrl Pts',(-20.7314548292168,50.3658883952655,124.156910684375)) ;
#41172=CARTESIAN_POINT('Ctrl Pts',(-20.3015547858526,50.5590949994898,124.235123685654)) ;
#41173=CARTESIAN_POINT('Ctrl Pts',(-20.5246530684262,50.3791059190799,124.440925618339)) ;
#41174=CARTESIAN_POINT('Ctrl Pts',(-20.0837840031638,50.572429925981,124.411566237074)) ;
#41175=CARTESIAN_POINT('Ctrl Pts',(-20.252395006767,50.3924408455712,124.661518807846)) ;
#41176=CARTESIAN_POINT('Ctrl Pts',(-19.9002502528585,50.5824130265756,124.513455062962)) ;
#41177=CARTESIAN_POINT('Ctrl Pts',(-20.0229851843153,50.4024239461658,124.788869046828)) ;
#41178=CARTESIAN_POINT('Ctrl Pts',(-19.7005468923068,50.5924578024753,124.582032085012)) ;
#41179=CARTESIAN_POINT('Ctrl Pts',(-19.7733522297918,50.4124687220654,124.874590001688)) ;
#41180=CARTESIAN_POINT('Ctrl Pts',(-19.4967087425705,50.6022757256612,124.614562625887)) ;
#41181=CARTESIAN_POINT('Ctrl Pts',(-19.5185568926569,50.4222866452513,124.915250650711)) ;
#41182=CARTESIAN_POINT('Ctrl Pts',(-19.2854718592234,50.6123250396165,124.611560869832)) ;
#41183=CARTESIAN_POINT('Ctrl Pts',(-19.2545052235501,50.4323359592067,124.911493375644)) ;
#41184=CARTESIAN_POINT('Ctrl Pts',(-19.0108573397302,50.6256287802391,124.558525690301)) ;
#41185=CARTESIAN_POINT('Ctrl Pts',(-18.9112636455779,50.4456396998293,124.845209773886)) ;
#41186=CARTESIAN_POINT('Ctrl Pts',(-18.6949673472923,50.6421189757157,124.406294928456)) ;
#41187=CARTESIAN_POINT('Ctrl Pts',(-18.516363618277,50.4621298953059,124.654888417468)) ;
#41188=CARTESIAN_POINT('Ctrl Pts',(-18.4467378433555,50.6588381406404,124.151872297138)) ;
#41189=CARTESIAN_POINT('Ctrl Pts',(-18.2061311341632,50.4788490602306,124.336917792482)) ;
#41190=CARTESIAN_POINT('Ctrl Pts',(-18.311368251597,50.6719991343105,123.910554451692)) ;
#41191=CARTESIAN_POINT('Ctrl Pts',(-18.0368827272088,50.4920100539007,124.035219084642)) ;
#41192=CARTESIAN_POINT('Ctrl Pts',(-18.2412163964924,50.6819953564158,123.7124638999)) ;
#41193=CARTESIAN_POINT('Ctrl Pts',(-17.9492027071772,50.502006276006,123.787616040882)) ;
#41194=CARTESIAN_POINT('Ctrl Pts',(-18.2069016120642,50.6920191959495,123.504545752087)) ;
#41195=CARTESIAN_POINT('Ctrl Pts',(-17.9063100732853,50.5120301155397,123.527712476813)) ;
#41196=CARTESIAN_POINT('Ctrl Pts',(-18.209328291179,50.7052125179428,123.227157565911)) ;
#41197=CARTESIAN_POINT('Ctrl Pts',(-17.9093431972847,50.5252234375329,123.180991999686)) ;
#41198=CARTESIAN_POINT('Ctrl Pts',(-18.3035425854847,50.7218716897201,122.88574552881)) ;
#41199=CARTESIAN_POINT('Ctrl Pts',(-18.0271182837049,50.5418826093103,122.754212984413)) ;
#41200=CARTESIAN_POINT('Ctrl Pts',(-18.5489966287471,50.7417818652058,122.540800163354)) ;
#41201=CARTESIAN_POINT('Ctrl Pts',(-18.3339375616829,50.561792784796,122.323039035069)) ;
#41202=CARTESIAN_POINT('Ctrl Pts',(-18.8965967981805,50.7616718530502,122.299823800529)) ;
#41203=CARTESIAN_POINT('Ctrl Pts',(-18.768439392141,50.5816827726403,122.021820822847)) ;
#41204=CARTESIAN_POINT('Ctrl Pts',(-19.3079195621711,50.781677301065,122.191706071761)) ;
#41205=CARTESIAN_POINT('Ctrl Pts',(-19.2825937715337,50.6016882206552,121.886677539516)) ;
#41206=CARTESIAN_POINT('Ctrl Pts',(-19.728095167199,50.8015136950923,122.229696970735)) ;
#41207=CARTESIAN_POINT('Ctrl Pts',(-19.8078113963471,50.6215246146825,121.934169205289)) ;
#41208=CARTESIAN_POINT('Ctrl Pts',(-20.1132481010553,50.821521488989,122.410089592141)) ;
#41209=CARTESIAN_POINT('Ctrl Pts',(-20.2892513212944,50.6415324085791,122.159662815693)) ;
#41210=CARTESIAN_POINT('Ctrl Pts',(-20.4112416238867,50.8413481252829,122.708392112376)) ;
#41211=CARTESIAN_POINT('Ctrl Pts',(-20.6617398848394,50.6613590448731,122.532541564625)) ;
#41212=CARTESIAN_POINT('Ctrl Pts',(-20.5915810372585,50.8613270682368,123.093001610394)) ;
#41213=CARTESIAN_POINT('Ctrl Pts',(-20.8871620270303,50.6813379878269,123.013304098407)) ;
#41214=CARTESIAN_POINT('Ctrl Pts',(-20.6290028587678,50.8812588701058,123.51509334654)) ;
#41215=CARTESIAN_POINT('Ctrl Pts',(-20.9339369379652,50.701269789696,123.540918150511)) ;
#41216=CARTESIAN_POINT('Ctrl Pts',(-20.5220534572003,50.9010831706034,123.922954659986)) ;
#41217=CARTESIAN_POINT('Ctrl Pts',(-20.8002489893683,50.7210940901936,124.050742162829)) ;
#41218=CARTESIAN_POINT('Ctrl Pts',(-20.2786120446289,50.9211791719433,124.273908281155)) ;
#41219=CARTESIAN_POINT('Ctrl Pts',(-20.4959470938252,50.7411900915334,124.48943444645)) ;
#41220=CARTESIAN_POINT('Ctrl Pts',(-19.9357982920383,50.9409375880472,124.517186763173)) ;
#41221=CARTESIAN_POINT('Ctrl Pts',(-20.0674250455344,50.7609485076374,124.793529199936)) ;
#41222=CARTESIAN_POINT('Ctrl Pts',(-19.5241716085477,50.9610312809313,124.630773509642)) ;
#41223=CARTESIAN_POINT('Ctrl Pts',(-19.5529196248106,50.7810422005214,124.935512899824)) ;
#41224=CARTESIAN_POINT('Ctrl Pts',(-19.2461442415946,50.9741422468379,124.608669218602)) ;
#41225=CARTESIAN_POINT('Ctrl Pts',(-19.2053312340935,50.7941531664281,124.907880339423)) ;
#41226=CARTESIAN_POINT('Ctrl Pts',(-19.1099467513572,50.9808556216258,124.573813086965)) ;
#41227=CARTESIAN_POINT('Ctrl Pts',(-19.0351174388764,50.800866541216,124.86431206241)) ;
#41228=CARTESIAN_POINT('',(-20.8890752031254,12.1693713464509,123.166987767337)) ;
#41229=CARTESIAN_POINT('Ctrl Pts',(-20.8890752032057,12.1693713464047,123.166987767343)) ;
#41230=CARTESIAN_POINT('Ctrl Pts',(-20.8610687220169,12.1854956519226,123.164917450078)) ;
#41231=CARTESIAN_POINT('Ctrl Pts',(-20.8327633568022,12.2014611086523,123.160624756444)) ;
#41232=CARTESIAN_POINT('Ctrl Pts',(-20.7745996966326,12.2331206623017,123.145633809153)) ;
#41233=CARTESIAN_POINT('Ctrl Pts',(-20.7441110801631,12.24905051571,123.134145565635)) ;
#41234=CARTESIAN_POINT('Ctrl Pts',(-20.6955669569155,12.272204921772,123.1064423772)) ;
#41235=CARTESIAN_POINT('Ctrl Pts',(-20.6762675979802,12.2807112212954,123.092474606893)) ;
#41236=CARTESIAN_POINT('Ctrl Pts',(-20.6467890442397,12.2917621876962,123.063862344896)) ;
#41237=CARTESIAN_POINT('Ctrl Pts',(-20.635672579296,12.295300396613,123.050723734153)) ;
#41238=CARTESIAN_POINT('Ctrl Pts',(-20.619631838715,12.2989553934292,123.026534454028)) ;
#41239=CARTESIAN_POINT('Ctrl Pts',(-20.6139434300127,12.2998015796369,123.016333414216)) ;
#41240=CARTESIAN_POINT('Ctrl Pts',(-20.6070335810964,12.3000406423084,123.001098589481)) ;
#41241=CARTESIAN_POINT('Ctrl Pts',(-20.6051280525899,12.2999881147679,122.996469969497)) ;
#41242=CARTESIAN_POINT('Ctrl Pts',(-20.6030890986318,12.2997791002204,122.990964267602)) ;
#41243=CARTESIAN_POINT('Ctrl Pts',(-20.6027932190504,12.2997444866016,122.990149815383)) ;
#41244=CARTESIAN_POINT('Ctrl Pts',(-20.6024894319963,12.2997043922845,122.989297097151)) ;
#41245=CARTESIAN_POINT('Ctrl Pts',(-20.6024764105458,12.2997026647784,122.989260514172)) ;
#41246=CARTESIAN_POINT('Ctrl Pts',(-20.6024544471701,12.2996997359228,122.989198754854)) ;
#41247=CARTESIAN_POINT('Ctrl Pts',(-20.6024454997488,12.2996985385416,122.989173580088)) ;
#41248=CARTESIAN_POINT('Ctrl Pts',(-20.6024308468241,12.2996965706967,122.989132327026)) ;
#41249=CARTESIAN_POINT('Ctrl Pts',(-20.6024251384176,12.2996958023491,122.989116249634)) ;
#41250=CARTESIAN_POINT('Ctrl Pts',(-20.6024162524072,12.2996946036105,122.989091212972)) ;
#41251=CARTESIAN_POINT('Ctrl Pts',(-20.6024130734271,12.2996941742243,122.989082254137)) ;
#41252=CARTESIAN_POINT('Ctrl Pts',(-20.6024072279404,12.299693383686,122.989065777121)) ;
#41253=CARTESIAN_POINT('Ctrl Pts',(-20.6024045612302,12.2996930226649,122.989058258941)) ;
#41254=CARTESIAN_POINT('Ctrl Pts',(-20.6023987642738,12.2996922370477,122.989041912772)) ;
#41255=CARTESIAN_POINT('Ctrl Pts',(-20.6023956342093,12.2996918123332,122.989033084778)) ;
#41256=CARTESIAN_POINT('Ctrl Pts',(-20.6023869166592,12.2996906280087,122.989008492654)) ;
#41257=CARTESIAN_POINT('Ctrl Pts',(-20.6023813304886,12.2996898674372,122.988992728105)) ;
#41258=CARTESIAN_POINT('Ctrl Pts',(-20.6023507307001,12.299685692091,122.988906340457)) ;
#41259=CARTESIAN_POINT('Ctrl Pts',(-20.602325753627,12.2996822506058,122.988835705718)) ;
#41260=CARTESIAN_POINT('Ctrl Pts',(-20.6022559538207,12.2996725396693,122.988637974298)) ;
#41261=CARTESIAN_POINT('Ctrl Pts',(-20.6022112171852,12.2996662073738,122.988510850483)) ;
#41262=CARTESIAN_POINT('Ctrl Pts',(-20.5998442084474,12.2993254047404,122.981763874573)) ;
#41263=CARTESIAN_POINT('Ctrl Pts',(-20.5978658821419,12.2987454066201,122.975055792179)) ;
#41264=CARTESIAN_POINT('Ctrl Pts',(-20.5933548407168,12.2964747990813,122.956304836256)) ;
#41265=CARTESIAN_POINT('Ctrl Pts',(-20.5915905482467,12.2942918311834,122.944252818362)) ;
#41266=CARTESIAN_POINT('Ctrl Pts',(-20.5898591383132,12.2873891660181,122.914933679065)) ;
#41267=CARTESIAN_POINT('Ctrl Pts',(-20.5910205314854,12.2820577513669,122.8979913349)) ;
#41268=CARTESIAN_POINT('Ctrl Pts',(-20.5980947263798,12.2670202296296,122.858409784169)) ;
#41269=CARTESIAN_POINT('Ctrl Pts',(-20.6057336956224,12.2565042285035,122.83652182479)) ;
#41270=CARTESIAN_POINT('Ctrl Pts',(-20.6376705328441,12.2199530300488,122.770754536439)) ;
#41271=CARTESIAN_POINT('Ctrl Pts',(-20.673969475726,12.1873876374,122.72708632587)) ;
#41272=CARTESIAN_POINT('Ctrl Pts',(-20.7227191491784,12.149892972702,122.68753928804)) ;
#41273=CARTESIAN_POINT('Ctrl Pts',(-17.9353686288931,11.9999999994367,123.599289317261)) ;
#41274=CARTESIAN_POINT('Ctrl Pts',(-17.9738189265565,12.0242028233619,123.58612699736)) ;
#41275=CARTESIAN_POINT('Ctrl Pts',(-18.0134459580924,12.0487813737637,123.575656459509)) ;
#41276=CARTESIAN_POINT('Ctrl Pts',(-18.0909257937832,12.0961326415371,123.561717397006)) ;
#41277=CARTESIAN_POINT('Ctrl Pts',(-18.129448015999,12.1193588332732,123.557760132541)) ;
#41278=CARTESIAN_POINT('Ctrl Pts',(-18.1677926267253,12.1420303856096,123.557513873554)) ;
#41279=CARTESIAN_POINT('Ctrl Pts',(-20.8890752031254,12.1693713464509,123.166987767337)) ;
#41280=CARTESIAN_POINT('Ctrl Pts',(-20.8921168691093,12.1700845612802,123.185411053998)) ;
#41281=CARTESIAN_POINT('Ctrl Pts',(-20.9073190645084,12.174105036101,123.289588099265)) ;
#41282=CARTESIAN_POINT('Ctrl Pts',(-20.9152054113298,12.1814863726884,123.483408955597)) ;
#41283=CARTESIAN_POINT('Ctrl Pts',(-20.8794802827671,12.1915186409522,123.744603500789)) ;
#41284=CARTESIAN_POINT('Ctrl Pts',(-20.8008139737887,12.2013826029581,123.991621606298)) ;
#41285=CARTESIAN_POINT('Ctrl Pts',(-20.678002189668,12.211452664303,124.225997440401)) ;
#41286=CARTESIAN_POINT('Ctrl Pts',(-20.5199833626838,12.2212950286517,124.430776031763)) ;
#41287=CARTESIAN_POINT('Ctrl Pts',(-20.327174746647,12.2312557011542,124.607803018266)) ;
#41288=CARTESIAN_POINT('Ctrl Pts',(-20.1045650508631,12.241293772222,124.749310160051)) ;
#41289=CARTESIAN_POINT('Ctrl Pts',(-19.8649051459857,12.2511673871824,124.84884392232)) ;
#41290=CARTESIAN_POINT('Ctrl Pts',(-19.6065797304044,12.2612396217637,124.906300997495)) ;
#41291=CARTESIAN_POINT('Ctrl Pts',(-19.3486297183306,12.2710636402125,124.918040759663)) ;
#41292=CARTESIAN_POINT('Ctrl Pts',(-19.0863456687476,12.2811285611885,124.884353810211)) ;
#41293=CARTESIAN_POINT('Ctrl Pts',(-18.7548496615759,12.2943388594833,124.781008020348)) ;
#41294=CARTESIAN_POINT('Ctrl Pts',(-18.4555083325038,12.3076543062152,124.592460114452)) ;
#41295=CARTESIAN_POINT('Ctrl Pts',(-18.2182158984291,12.3209445514825,124.336043204847)) ;
#41296=CARTESIAN_POINT('Ctrl Pts',(-18.0753697674858,12.3309953010896,124.113946532571)) ;
#41297=CARTESIAN_POINT('Ctrl Pts',(-17.9751686262583,12.3408079080718,123.876303265546)) ;
#41298=CARTESIAN_POINT('Ctrl Pts',(-17.9159132713503,12.3508790060661,123.61839959421)) ;
#41299=CARTESIAN_POINT('Ctrl Pts',(-17.9028470180164,12.360768578841,123.358821518713)) ;
#41300=CARTESIAN_POINT('Ctrl Pts',(-17.9449900324593,12.3740386856443,123.012644489447)) ;
#41301=CARTESIAN_POINT('Ctrl Pts',(-18.1100382420715,12.3906553725668,122.603018959482)) ;
#41302=CARTESIAN_POINT('Ctrl Pts',(-18.403953809166,12.407229415883,122.274921978595)) ;
#41303=CARTESIAN_POINT('Ctrl Pts',(-18.6963080999561,12.4205259833148,122.083501484983)) ;
#41304=CARTESIAN_POINT('Ctrl Pts',(-18.9385791929077,12.4305560468922,121.979673523522)) ;
#41305=CARTESIAN_POINT('Ctrl Pts',(-19.1916818709481,12.4404499387415,121.920281628208)) ;
#41306=CARTESIAN_POINT('Ctrl Pts',(-19.5394009792638,12.453702694527,121.899549493621)) ;
#41307=CARTESIAN_POINT('Ctrl Pts',(-19.9747293753154,12.4704307995194,121.989564308867)) ;
#41308=CARTESIAN_POINT('Ctrl Pts',(-20.423556659189,12.4902616359979,122.266069036656)) ;
#41309=CARTESIAN_POINT('Ctrl Pts',(-20.7535327226879,12.5101870278881,122.680135635484)) ;
#41310=CARTESIAN_POINT('Ctrl Pts',(-20.9224041261076,12.5301122412401,123.18215712058)) ;
#41311=CARTESIAN_POINT('Ctrl Pts',(-20.9099617273115,12.5500372547252,123.711523704258)) ;
#41312=CARTESIAN_POINT('Ctrl Pts',(-20.7187360422604,12.5699137264252,124.204018044716)) ;
#41313=CARTESIAN_POINT('Ctrl Pts',(-20.3693300643289,12.5898930443341,124.603877601687)) ;
#41314=CARTESIAN_POINT('Ctrl Pts',(-19.9052905888142,12.6098260479101,124.859582769263)) ;
#41315=CARTESIAN_POINT('Ctrl Pts',(-19.3829989743676,12.6297213179378,124.941977004567)) ;
#41316=CARTESIAN_POINT('Ctrl Pts',(-18.8631060156455,12.6496426558436,124.841587523865)) ;
#41317=CARTESIAN_POINT('Ctrl Pts',(-18.4079042835162,12.6696002791098,124.569214868981)) ;
#41318=CARTESIAN_POINT('Ctrl Pts',(-18.0742532724176,12.689480111067,124.15962015315)) ;
#41319=CARTESIAN_POINT('Ctrl Pts',(-17.8989480657597,12.7093619623639,123.661012507451)) ;
#41320=CARTESIAN_POINT('Ctrl Pts',(-17.9053743363839,12.7294329794677,123.127663535506)) ;
#41321=CARTESIAN_POINT('Ctrl Pts',(-18.0909224032866,12.7492402032208,122.634900991628)) ;
#41322=CARTESIAN_POINT('Ctrl Pts',(-18.4354537167374,12.7692213387896,122.230824135122)) ;
#41323=CARTESIAN_POINT('Ctrl Pts',(-18.8964641846084,12.7891488321288,121.970176160961)) ;
#41324=CARTESIAN_POINT('Ctrl Pts',(-19.415834432645,12.8089694934866,121.881151656097)) ;
#41325=CARTESIAN_POINT('Ctrl Pts',(-19.9411566590932,12.8290666827084,121.976780870031)) ;
#41326=CARTESIAN_POINT('Ctrl Pts',(-20.3952240684518,12.8488303617167,122.241384544964)) ;
#41327=CARTESIAN_POINT('Ctrl Pts',(-20.7368987004041,12.8688876403898,122.650278783027)) ;
#41328=CARTESIAN_POINT('Ctrl Pts',(-20.915999998585,12.8886830641372,123.145136393717)) ;
#41329=CARTESIAN_POINT('Ctrl Pts',(-20.9171224626081,12.9086467088648,123.675675466344)) ;
#41330=CARTESIAN_POINT('Ctrl Pts',(-20.7357148689362,12.9286302001389,124.174870580485)) ;
#41331=CARTESIAN_POINT('Ctrl Pts',(-20.3986521463145,12.9484376952882,124.579332558867)) ;
#41332=CARTESIAN_POINT('Ctrl Pts',(-19.9402235763069,12.9684202860083,124.847283742868)) ;
#41333=CARTESIAN_POINT('Ctrl Pts',(-19.4202416053834,12.9883029399995,124.942191223807)) ;
#41334=CARTESIAN_POINT('Ctrl Pts',(-18.8972653738817,13.0082611848626,124.854056149815)) ;
#41335=CARTESIAN_POINT('Ctrl Pts',(-18.4373467193133,13.0281367719042,124.594021898923)) ;
#41336=CARTESIAN_POINT('Ctrl Pts',(-18.0917408140289,13.0481176600395,124.190855292359)) ;
#41337=CARTESIAN_POINT('Ctrl Pts',(-17.9052414355018,13.0680528011505,123.694844185524)) ;
#41338=CARTESIAN_POINT('Ctrl Pts',(-17.8988271166947,13.0879648191615,123.165702838927)) ;
#41339=CARTESIAN_POINT('Ctrl Pts',(-18.072637630343,13.1078530374051,122.666485551976)) ;
#41340=CARTESIAN_POINT('Ctrl Pts',(-18.3508356377982,13.124451341252,122.324166060085)) ;
#41341=CARTESIAN_POINT('Ctrl Pts',(-18.6332461345771,13.1377239311548,122.119417599801)) ;
#41342=CARTESIAN_POINT('Ctrl Pts',(-18.8696106143661,13.1477313461057,122.004127651261)) ;
#41343=CARTESIAN_POINT('Ctrl Pts',(-19.1224757065835,13.1577386928383,121.931849416177)) ;
#41344=CARTESIAN_POINT('Ctrl Pts',(-19.4692111889447,13.1710050526399,121.895476582139)) ;
#41345=CARTESIAN_POINT('Ctrl Pts',(-19.9027886653172,13.1875197102629,121.963391453896)) ;
#41346=CARTESIAN_POINT('Ctrl Pts',(-20.2896179416635,13.2041171435055,122.175375538865)) ;
#41347=CARTESIAN_POINT('Ctrl Pts',(-20.5428541366256,13.2174651406505,122.418153018463)) ;
#41348=CARTESIAN_POINT('Ctrl Pts',(-20.6967627804406,13.2273608950021,122.62776755716)) ;
#41349=CARTESIAN_POINT('Ctrl Pts',(-20.8132896637095,13.2373488489335,122.862934128972)) ;
#41350=CARTESIAN_POINT('Ctrl Pts',(-20.8871117690639,13.2473060726382,123.114002366625)) ;
#41351=CARTESIAN_POINT('Ctrl Pts',(-20.9163194697392,13.2573416191949,123.376085199788)) ;
#41352=CARTESIAN_POINT('Ctrl Pts',(-20.9000197111728,13.267228730471,123.635413520908)) ;
#41353=CARTESIAN_POINT('Ctrl Pts',(-20.8387093067046,13.2772201355718,123.890705618829)) ;
#41354=CARTESIAN_POINT('Ctrl Pts',(-20.7344045824693,13.2871657567866,124.130350209159)) ;
#41355=CARTESIAN_POINT('Ctrl Pts',(-20.5904556480587,13.2971150050549,124.348628887742)) ;
#41356=CARTESIAN_POINT('Ctrl Pts',(-20.4088310489179,13.3071615002235,124.540222615066)) ;
#41357=CARTESIAN_POINT('Ctrl Pts',(-20.2009526790891,13.3170128430151,124.69453910851)) ;
#41358=CARTESIAN_POINT('Ctrl Pts',(-19.9669434550335,13.3269846231424,124.812406349802)) ;
#41359=CARTESIAN_POINT('Ctrl Pts',(-19.7153564891379,13.3369798231201,124.888022808457)) ;
#41360=CARTESIAN_POINT('Ctrl Pts',(-19.4534753611638,13.3470138148161,124.918598821052)) ;
#41361=CARTESIAN_POINT('Ctrl Pts',(-19.1948766730221,13.3568692197886,124.903920505576)) ;
#41362=CARTESIAN_POINT('Ctrl Pts',(-18.9390603846793,13.3668685176344,124.844062381727)) ;
#41363=CARTESIAN_POINT('Ctrl Pts',(-18.6998481883594,13.3767636302396,124.741995186928)) ;
#41364=CARTESIAN_POINT('Ctrl Pts',(-18.4784292945889,13.3868242757746,124.597585675323)) ;
#41365=CARTESIAN_POINT('Ctrl Pts',(-18.2893688821215,13.3966731527638,124.420799145494)) ;
#41366=CARTESIAN_POINT('Ctrl Pts',(-18.1305208053495,13.4067018638574,124.210511784196)) ;
#41367=CARTESIAN_POINT('Ctrl Pts',(-18.0112247910287,13.4167312651135,123.975488167396)) ;
#41368=CARTESIAN_POINT('Ctrl Pts',(-17.9354445009214,13.4265714569095,123.72824647118)) ;
#41369=CARTESIAN_POINT('Ctrl Pts',(-17.9027395319079,13.4365748861025,123.467435684465)) ;
#41370=CARTESIAN_POINT('Ctrl Pts',(-17.9158814573718,13.4465603985687,123.205311390375)) ;
#41371=CARTESIAN_POINT('Ctrl Pts',(-17.9749065837832,13.4566014949527,122.948155155583)) ;
#41372=CARTESIAN_POINT('Ctrl Pts',(-18.0753470360815,13.4664446909037,122.709757985454)) ;
#41373=CARTESIAN_POINT('Ctrl Pts',(-18.217218281521,13.4764310019581,122.489035231126)) ;
#41374=CARTESIAN_POINT('Ctrl Pts',(-18.3942732512551,13.4863656872158,122.297106419642)) ;
#41375=CARTESIAN_POINT('Ctrl Pts',(-18.6046031877743,13.4964232484328,122.137116873894)) ;
#41376=CARTESIAN_POINT('Ctrl Pts',(-18.8338850495127,13.5062448900415,122.018535713195)) ;
#41377=CARTESIAN_POINT('Ctrl Pts',(-19.0859583258846,13.5163009536324,121.939273611562)) ;
#41378=CARTESIAN_POINT('Ctrl Pts',(-19.3450516698222,13.5262416293942,121.905839973782)) ;
#41379=CARTESIAN_POINT('Ctrl Pts',(-19.6050909750196,13.5361459881825,121.917041144644)) ;
#41380=CARTESIAN_POINT('Ctrl Pts',(-19.862825851585,13.5461926427583,121.97418792217)) ;
#41381=CARTESIAN_POINT('Ctrl Pts',(-20.1031997643857,13.5560882374012,122.073508487898)) ;
#41382=CARTESIAN_POINT('Ctrl Pts',(-20.3263218440362,13.5661501840581,122.215343672236)) ;
#41383=CARTESIAN_POINT('Ctrl Pts',(-20.5173749645332,13.5759998079902,122.38999462014)) ;
#41384=CARTESIAN_POINT('Ctrl Pts',(-20.6776884554839,13.5859630470201,122.596980439567)) ;
#41385=CARTESIAN_POINT('Ctrl Pts',(-20.8000704181908,13.5959876217959,122.830280403309)) ;
#41386=CARTESIAN_POINT('Ctrl Pts',(-20.8793920083737,13.6059061844836,123.07855998187)) ;
#41387=CARTESIAN_POINT('Ctrl Pts',(-20.9151199375489,13.6158983712076,123.338717822216)) ;
#41388=CARTESIAN_POINT('Ctrl Pts',(-20.9046168525977,13.6259331697918,123.6022019633)) ;
#41389=CARTESIAN_POINT('Ctrl Pts',(-20.8499556627768,13.6357883604655,123.855372966742)) ;
#41390=CARTESIAN_POINT('Ctrl Pts',(-20.7510855573927,13.6457877086185,124.098788324435)) ;
#41391=CARTESIAN_POINT('Ctrl Pts',(-20.6130996723433,13.6556828342936,124.319242233489)) ;
#41392=CARTESIAN_POINT('Ctrl Pts',(-20.4360519660016,13.6657433772417,124.515540628893)) ;
#41393=CARTESIAN_POINT('Ctrl Pts',(-20.232034145686,13.6755926515086,124.674850714962)) ;
#41394=CARTESIAN_POINT('Ctrl Pts',(-19.9996623311131,13.6856198760785,124.799086161189)) ;
#41395=CARTESIAN_POINT('Ctrl Pts',(-19.7489854254844,13.6956482752663,124.880448501815)) ;
#41396=CARTESIAN_POINT('Ctrl Pts',(-19.4928401900497,13.7054940256798,124.916853671087)) ;
#41397=CARTESIAN_POINT('Ctrl Pts',(-19.230454887784,13.7154828160805,124.908839488335)) ;
#41398=CARTESIAN_POINT('Ctrl Pts',(-18.9721627761797,13.7255277444802,124.854438840815)) ;
#41399=CARTESIAN_POINT('Ctrl Pts',(-18.7323658376547,13.7353522292692,124.758724681303)) ;
#41400=CARTESIAN_POINT('Ctrl Pts',(-18.507457139982,13.7454096268104,124.619951807237)) ;
#41401=CARTESIAN_POINT('Ctrl Pts',(-18.3128349524813,13.7553357183966,124.44624656969)) ;
#41402=CARTESIAN_POINT('Ctrl Pts',(-18.1503452309715,13.7652905035412,124.241231958245)) ;
#41403=CARTESIAN_POINT('Ctrl Pts',(-18.0251465109341,13.7753278731988,124.009068223143)) ;
#41404=CARTESIAN_POINT('Ctrl Pts',(-17.9431959784106,13.7852166833204,123.762452941019)) ;
#41405=CARTESIAN_POINT('Ctrl Pts',(-17.9044614031139,13.7952060423715,123.502822293364)) ;
#41406=CARTESIAN_POINT('Ctrl Pts',(-17.9115693386521,13.8051645898276,123.241226463732)) ;
#41407=CARTESIAN_POINT('Ctrl Pts',(-17.9630567197968,13.8150641663786,122.986205100608)) ;
#41408=CARTESIAN_POINT('Ctrl Pts',(-18.0595361492998,13.8251120782093,122.740443216478)) ;
#41409=CARTESIAN_POINT('Ctrl Pts',(-18.1949930036132,13.8350074260699,122.518422190268)) ;
#41410=CARTESIAN_POINT('Ctrl Pts',(-18.3697572977927,13.845069102601,122.320042659935)) ;
#41411=CARTESIAN_POINT('Ctrl Pts',(-18.5718588198519,13.8549136203502,122.158525512922)) ;
#41412=CARTESIAN_POINT('Ctrl Pts',(-18.8011469810602,13.864874064065,122.032284729829)) ;
#41413=CARTESIAN_POINT('Ctrl Pts',(-19.0509301231226,13.8749108968832,121.947590007007)) ;
#41414=CARTESIAN_POINT('Ctrl Pts',(-19.3074865101994,13.88478969363,121.907757156992)) ;
#41415=CARTESIAN_POINT('Ctrl Pts',(-19.5717537455678,13.8948490097584,121.91308802529)) ;
#41416=CARTESIAN_POINT('Ctrl Pts',(-19.8262549511952,13.9047194565116,121.963266910915)) ;
#41417=CARTESIAN_POINT('Ctrl Pts',(-20.0714142577279,13.9147120947696,122.057363864517)) ;
#41418=CARTESIAN_POINT('Ctrl Pts',(-20.2970965036502,13.9247441103175,122.193613633218)) ;
#41419=CARTESIAN_POINT('Ctrl Pts',(-20.4928009018349,13.9346099666241,122.363706237578)) ;
#41420=CARTESIAN_POINT('Ctrl Pts',(-20.6593476164435,13.9446792560932,122.569291069351)) ;
#41421=CARTESIAN_POINT('Ctrl Pts',(-20.7848399902421,13.9545228136445,122.795508554596)) ;
#41422=CARTESIAN_POINT('Ctrl Pts',(-20.871120064522,13.9645029404323,123.043168459414)) ;
#41423=CARTESIAN_POINT('Ctrl Pts',(-20.9127502836893,13.9745214890323,123.303126129535)) ;
#41424=CARTESIAN_POINT('Ctrl Pts',(-20.9092186327094,13.9844047895555,123.562857078074)) ;
#41425=CARTESIAN_POINT('Ctrl Pts',(-20.8668755026365,13.9930026771793,123.784759348932)) ;
#41426=CARTESIAN_POINT('Ctrl Pts',(-20.8240292246658,13.9981476378102,123.912638068403)) ;
#41427=CARTESIAN_POINT('Ctrl Pts',(-20.8063667317783,14.0000000000496,123.957804304199)) ;
#41428=CARTESIAN_POINT('Origin',(-20.3808735729049,12.,126.250122109236)) ;
#41429=CARTESIAN_POINT('',(-18.3583806245238,12.,124.088665030377)) ;
#41430=CARTESIAN_POINT('',(-18.1677493372133,12.,124.153922001841)) ;
#41431=CARTESIAN_POINT('Origin',(-19.4092722359532,12.,123.411814366564)) ;
#41432=CARTESIAN_POINT('Origin',(-19.4092722359532,-13.9601742359176,123.411814366564)) ;
#41433=CARTESIAN_POINT('',(-20.5919010016347,-12.5498814819081,123.006982052377)) ;
#41434=CARTESIAN_POINT('Ctrl Pts',(-18.2266423654683,-12.3699164408135,
123.816643453356)) ;
#41435=CARTESIAN_POINT('Ctrl Pts',(-18.2493742613449,-12.3731350315633,
123.883050290101)) ;
#41436=CARTESIAN_POINT('Ctrl Pts',(-18.2776599920336,-12.3763218616224,
123.947414117214)) ;
#41437=CARTESIAN_POINT('Ctrl Pts',(-18.3111475606552,-12.3795367049563,
124.008992897305)) ;
#41438=CARTESIAN_POINT('Ctrl Pts',(-18.3133023878075,-12.3797435707274,
124.012955311801)) ;
#41439=CARTESIAN_POINT('Ctrl Pts',(-18.3154787380571,-12.3799505524888,
124.016906203678)) ;
#41440=CARTESIAN_POINT('Ctrl Pts',(-18.3176765111433,-12.3801576661661,
124.020845378626)) ;
#41441=CARTESIAN_POINT('Ctrl Pts',(-18.3624711373787,-12.3843790208745,
124.101132952698)) ;
#41442=CARTESIAN_POINT('Ctrl Pts',(-18.4158874627463,-12.3885782982683,
124.176062257801)) ;
#41443=CARTESIAN_POINT('Ctrl Pts',(-18.4768889137241,-12.3927747089667,
124.244377481592)) ;
#41444=CARTESIAN_POINT('Ctrl Pts',(-18.5122948246434,-12.3952103517423,
124.284028386435)) ;
#41445=CARTESIAN_POINT('Ctrl Pts',(-18.5502576072234,-12.3976450287944,
124.321452073109)) ;
#41446=CARTESIAN_POINT('Ctrl Pts',(-18.5905771630734,-12.4000824963187,
124.356398072605)) ;
#41447=CARTESIAN_POINT('Ctrl Pts',(-18.6720599780286,-12.4050084363757,
124.42702133098)) ;
#41448=CARTESIAN_POINT('Ctrl Pts',(-18.762391466541,-12.4099534088704,124.486846557586)) ;
#41449=CARTESIAN_POINT('Ctrl Pts',(-18.8593143846845,-12.4148934429917,
124.53433223364)) ;
#41450=CARTESIAN_POINT('Ctrl Pts',(-18.8925082975444,-12.4165852932299,
124.5505950064)) ;
#41451=CARTESIAN_POINT('Ctrl Pts',(-18.9264384731065,-12.4182785416309,
124.565389349838)) ;
#41452=CARTESIAN_POINT('Ctrl Pts',(-18.9609092505901,-12.4199790179757,
124.578635104052)) ;
#41453=CARTESIAN_POINT('Ctrl Pts',(-19.0479270417047,-12.4242716886425,
124.612072593934)) ;
#41454=CARTESIAN_POINT('Ctrl Pts',(-19.1382300374287,-12.428523931692,124.635603002896)) ;
#41455=CARTESIAN_POINT('Ctrl Pts',(-19.2301289024319,-12.4327743159446,
124.64891083254)) ;
#41456=CARTESIAN_POINT('Ctrl Pts',(-19.2817154738864,-12.4351602295351,
124.656381058694)) ;
#41457=CARTESIAN_POINT('Ctrl Pts',(-19.3338065523741,-12.4375455574124,
124.660630085422)) ;
#41458=CARTESIAN_POINT('Ctrl Pts',(-19.3861021450717,-12.4399371216425,
124.661599606901)) ;
#41459=CARTESIAN_POINT('Ctrl Pts',(-19.5313727356904,-12.4465805868045,
124.664292815845)) ;
#41460=CARTESIAN_POINT('Ctrl Pts',(-19.6760004365552,-12.4532079500155,
124.64163824834)) ;
#41461=CARTESIAN_POINT('Ctrl Pts',(-19.8134891857048,-12.4598668438148,
124.594653602306)) ;
#41462=CARTESIAN_POINT('Ctrl Pts',(-19.8136929095394,-12.4598767106249,
124.594583982847)) ;
#41463=CARTESIAN_POINT('Ctrl Pts',(-19.8138971253372,-12.4598866034866,
124.594514136294)) ;
#41464=CARTESIAN_POINT('Ctrl Pts',(-19.8141008161599,-12.4598964712907,
124.594444410459)) ;
#41465=CARTESIAN_POINT('Ctrl Pts',(-19.9512603591532,-12.4665411667972,
124.547493038525)) ;
#41466=CARTESIAN_POINT('Ctrl Pts',(-20.079206290757,-12.4731348095734,124.47703975085)) ;
#41467=CARTESIAN_POINT('Ctrl Pts',(-20.1922170357684,-12.4797820389184,
124.386235959366)) ;
#41468=CARTESIAN_POINT('Ctrl Pts',(-20.2724857565317,-12.4845034005562,
124.321740285241)) ;
#41469=CARTESIAN_POINT('Ctrl Pts',(-20.3443508215252,-12.4891911037781,
124.247678939301)) ;
#41470=CARTESIAN_POINT('Ctrl Pts',(-20.4062803455442,-12.4938975845992,
124.165787064668)) ;
#41471=CARTESIAN_POINT('Ctrl Pts',(-20.4317492598245,-12.4958331550479,
124.132108505558)) ;
#41472=CARTESIAN_POINT('Ctrl Pts',(-20.4555379658399,-12.4977719013865,
124.097104804527)) ;
#41473=CARTESIAN_POINT('Ctrl Pts',(-20.477537722934,-12.4997174708836,124.060897450153)) ;
#41474=CARTESIAN_POINT('Ctrl Pts',(-20.4970770533415,-12.5014454502005,
124.02873948326)) ;
#41475=CARTESIAN_POINT('Ctrl Pts',(-20.5151876206594,-12.5031867191234,
123.995654919809)) ;
#41476=CARTESIAN_POINT('Ctrl Pts',(-20.5317606313249,-12.5049236383535,
123.961832368389)) ;
#41477=CARTESIAN_POINT('Ctrl Pts',(-20.5790398477391,-12.5098786934024,
123.865343941481)) ;
#41478=CARTESIAN_POINT('Ctrl Pts',(-20.6136630444319,-12.5147321491143,
123.76319238016)) ;
#41479=CARTESIAN_POINT('Ctrl Pts',(-20.6348005037812,-12.5196443197352,
123.657945357767)) ;
#41480=CARTESIAN_POINT('Ctrl Pts',(-20.6530044812983,-12.5238747734556,
123.567304642735)) ;
#41481=CARTESIAN_POINT('Ctrl Pts',(-20.6610621663733,-12.5281007098675,
123.475112747438)) ;
#41482=CARTESIAN_POINT('Ctrl Pts',(-20.6589406533506,-12.5323257106508,
123.383024669876)) ;
#41483=CARTESIAN_POINT('Ctrl Pts',(-20.6577323804436,-12.5347319904727,
123.330577417381)) ;
#41484=CARTESIAN_POINT('Ctrl Pts',(-20.6532216458869,-12.5371379668062,
123.278162196879)) ;
#41485=CARTESIAN_POINT('Ctrl Pts',(-20.6453973814328,-12.5395443013262,
123.2260870805)) ;
#41486=CARTESIAN_POINT('Ctrl Pts',(-20.6348831474355,-12.5427779297865,
123.156108622811)) ;
#41487=CARTESIAN_POINT('Ctrl Pts',(-20.6184302716024,-12.5460210114688,
123.087076547404)) ;
#41488=CARTESIAN_POINT('Ctrl Pts',(-20.5962158993244,-12.5492621658114,
123.019813422613)) ;
#41489=CARTESIAN_POINT('Ctrl Pts',(-20.5948009399898,-12.5494686133101,
123.015529052787)) ;
#41490=CARTESIAN_POINT('Ctrl Pts',(-20.5933626230645,-12.5496750529894,
123.011251858573)) ;
#41491=CARTESIAN_POINT('Ctrl Pts',(-20.5919010016528,-12.5498814819081,
123.00698205237)) ;
#41492=CARTESIAN_POINT('Ctrl Pts',(-20.591901001653,-12.5498814819195,123.006982052371)) ;
#41493=CARTESIAN_POINT('Ctrl Pts',(-20.5823589431143,-12.5512291337733,
122.979107022349)) ;
#41494=CARTESIAN_POINT('Ctrl Pts',(-20.5718380184699,-12.5525754721182,
122.951587396436)) ;
#41495=CARTESIAN_POINT('Ctrl Pts',(-20.5566068789105,-12.554364799924,122.915613370786)) ;
#41496=CARTESIAN_POINT('Ctrl Pts',(-20.5527611641633,-12.5548048764859,
122.906814087733)) ;
#41497=CARTESIAN_POINT('Ctrl Pts',(-20.5450459304218,-12.5556659701827,
122.889701173019)) ;
#41498=CARTESIAN_POINT('Ctrl Pts',(-20.5411855614764,-12.5560869246646,
122.881384074547)) ;
#41499=CARTESIAN_POINT('Ctrl Pts',(-20.5325850560412,-12.5570042627748,
122.863375967916)) ;
#41500=CARTESIAN_POINT('Ctrl Pts',(-20.5278102677573,-12.5575008059757,
122.853702336013)) ;
#41501=CARTESIAN_POINT('Ctrl Pts',(-20.5099171526103,-12.5593178066816,
122.818603391076)) ;
#41502=CARTESIAN_POINT('Ctrl Pts',(-20.4960524227534,-12.5606460879697,
122.793569051698)) ;
#41503=CARTESIAN_POINT('Ctrl Pts',(-20.4689003040132,-12.563103295292,122.748283142712)) ;
#41504=CARTESIAN_POINT('Ctrl Pts',(-20.4558595340843,-12.5642297729607,
122.727898901248)) ;
#41505=CARTESIAN_POINT('Ctrl Pts',(-20.4302918678698,-12.5663368883533,
122.690379167524)) ;
#41506=CARTESIAN_POINT('Ctrl Pts',(-20.4179041026958,-12.5673180750482,
122.67315909667)) ;
#41507=CARTESIAN_POINT('Ctrl Pts',(-20.4021421413916,-12.5685190263038,
122.652384948628)) ;
#41508=CARTESIAN_POINT('Ctrl Pts',(-20.399177560185,-12.5687429472497,122.648524684188)) ;
#41509=CARTESIAN_POINT('Ctrl Pts',(-20.3938451328287,-12.5691422581575,
122.641664500751)) ;
#41510=CARTESIAN_POINT('Ctrl Pts',(-20.3914859348972,-12.5693177379361,
122.638657943332)) ;
#41511=CARTESIAN_POINT('Ctrl Pts',(-20.3866874495288,-12.5696722825805,
122.632600172743)) ;
#41512=CARTESIAN_POINT('Ctrl Pts',(-20.3842475723445,-12.56985133876,122.629549479762)) ;
#41513=CARTESIAN_POINT('Ctrl Pts',(-20.3793277569038,-12.5702099774409,
122.623456776567)) ;
#41514=CARTESIAN_POINT('Ctrl Pts',(-20.3768477118311,-12.5703895564525,
122.620414908624)) ;
#41515=CARTESIAN_POINT('Ctrl Pts',(-20.3697971849743,-12.5708967125171,
122.611849857049)) ;
#41516=CARTESIAN_POINT('Ctrl Pts',(-20.3651934473058,-12.5712239111852,
122.606354229413)) ;
#41517=CARTESIAN_POINT('Ctrl Pts',(-20.3398192354273,-12.5730063449014,
122.57658821007)) ;
#41518=CARTESIAN_POINT('Ctrl Pts',(-20.3181713921682,-12.5744508679129,
122.553081106076)) ;
#41519=CARTESIAN_POINT('Ctrl Pts',(-20.2713672340028,-12.5774452618565,
122.506012022865)) ;
#41520=CARTESIAN_POINT('Ctrl Pts',(-20.2460895006122,-12.5789942678939,
122.482609041878)) ;
#41521=CARTESIAN_POINT('Ctrl Pts',(-20.205190152754,-12.5814291326774,122.447767194467)) ;
#41522=CARTESIAN_POINT('Ctrl Pts',(-20.1902149311921,-12.5823059052257,
122.435596778385)) ;
#41523=CARTESIAN_POINT('Ctrl Pts',(-20.1638910135029,-12.5838226693699,
122.415196710945)) ;
#41524=CARTESIAN_POINT('Ctrl Pts',(-20.1526744831753,-12.5844616261347,
122.406802253454)) ;
#41525=CARTESIAN_POINT('Ctrl Pts',(-20.1314495042424,-12.5856575004875,
122.391467241805)) ;
#41526=CARTESIAN_POINT('Ctrl Pts',(-20.1214760949646,-12.5862141527252,
122.384480962141)) ;
#41527=CARTESIAN_POINT('Ctrl Pts',(-20.1011791499057,-12.587336753662,122.37070077624)) ;
#41528=CARTESIAN_POINT('Ctrl Pts',(-20.0908537279533,-12.5879026562735,
122.363912007451)) ;
#41529=CARTESIAN_POINT('Ctrl Pts',(-20.0670701829121,-12.5891948400098,
122.3487750351)) ;
#41530=CARTESIAN_POINT('Ctrl Pts',(-20.0535506550379,-12.5899212991964,
122.340527254705)) ;
#41531=CARTESIAN_POINT('Ctrl Pts',(-20.019016799078,-12.5917579196349,122.320349601424)) ;
#41532=CARTESIAN_POINT('Ctrl Pts',(-19.9978065224073,-12.5928685898015,
122.308768060688)) ;
#41533=CARTESIAN_POINT('Ctrl Pts',(-19.93325379259,-12.5962035556881,122.275912295499)) ;
#41534=CARTESIAN_POINT('Ctrl Pts',(-19.8890016377507,-12.5984314623645,
122.25652660003)) ;
#41535=CARTESIAN_POINT('Ctrl Pts',(-19.8175637829835,-12.6019633799019,
122.230045627904)) ;
#41536=CARTESIAN_POINT('Ctrl Pts',(-19.7910698527825,-12.6032577175856,
122.221222105843)) ;
#41537=CARTESIAN_POINT('Ctrl Pts',(-19.7479684467081,-12.6053351370545,
122.208454446933)) ;
#41538=CARTESIAN_POINT('Ctrl Pts',(-19.7315369229615,-12.6061207124371,
122.203950261288)) ;
#41539=CARTESIAN_POINT('Ctrl Pts',(-19.7147727171071,-12.6069159056836,
122.199721333712)) ;
#41540=CARTESIAN_POINT('Ctrl Pts',(-19.7145270194464,-12.6069275587511,
122.199659433633)) ;
#41541=CARTESIAN_POINT('Ctrl Pts',(-19.7140600882535,-12.6069497020197,
122.19954194784)) ;
#41542=CARTESIAN_POINT('Ctrl Pts',(-19.7138388583028,-12.6069601923071,
122.199486347973)) ;
#41543=CARTESIAN_POINT('Ctrl Pts',(-19.7134183934058,-12.6069801278413,
122.199380798416)) ;
#41544=CARTESIAN_POINT('Ctrl Pts',(-19.7132191613582,-12.6069895731578,
122.199330837273)) ;
#41545=CARTESIAN_POINT('Ctrl Pts',(-19.7128404665971,-12.6070075248681,
122.19923597172)) ;
#41546=CARTESIAN_POINT('Ctrl Pts',(-19.7126610062194,-12.6070160313187,
122.19919105804)) ;
#41547=CARTESIAN_POINT('Ctrl Pts',(-19.7123198520826,-12.607032200713,122.199105757619)) ;
#41548=CARTESIAN_POINT('Ctrl Pts',(-19.7121581602287,-12.6070398637017,
122.199065363379)) ;
#41549=CARTESIAN_POINT('Ctrl Pts',(-19.7118507434955,-12.6070544318554,
122.198988629121)) ;
#41550=CARTESIAN_POINT('Ctrl Pts',(-19.7117050201375,-12.6070613370577,
122.198952283027)) ;
#41551=CARTESIAN_POINT('Ctrl Pts',(-19.7114279248196,-12.6070744665121,
122.198883223387)) ;
#41552=CARTESIAN_POINT('Ctrl Pts',(-19.7112965539404,-12.6070806908015,
122.198850504881)) ;
#41553=CARTESIAN_POINT('Ctrl Pts',(-19.7110467140566,-12.6070925273652,
122.198788324245)) ;
#41554=CARTESIAN_POINT('Ctrl Pts',(-19.7109282459476,-12.6070981396689,
122.198758858101)) ;
#41555=CARTESIAN_POINT('Ctrl Pts',(-19.710702911402,-12.6071088140654,122.198702846505)) ;
#41556=CARTESIAN_POINT('Ctrl Pts',(-19.7105960459328,-12.6071138761706,
122.19867629786)) ;
#41557=CARTESIAN_POINT('Ctrl Pts',(-19.7103927509742,-12.6071235055567,
122.198625821704)) ;
#41558=CARTESIAN_POINT('Ctrl Pts',(-19.7102963222004,-12.6071280728509,
122.198601891585)) ;
#41559=CARTESIAN_POINT('Ctrl Pts',(-19.7101128553429,-12.6071367622617,
122.198556384995)) ;
#41560=CARTESIAN_POINT('Ctrl Pts',(-19.7100258179597,-12.6071408843834,
122.198534806435)) ;
#41561=CARTESIAN_POINT('Ctrl Pts',(-19.709860196494,-12.6071487279555,122.198493764)) ;
#41562=CARTESIAN_POINT('Ctrl Pts',(-19.709781612976,-12.6071524494102,122.198474298425)) ;
#41563=CARTESIAN_POINT('Ctrl Pts',(-19.7096320586394,-12.6071595315467,
122.198437268405)) ;
#41564=CARTESIAN_POINT('Ctrl Pts',(-19.7095610879269,-12.6071628922488,
122.198419702491)) ;
#41565=CARTESIAN_POINT('Ctrl Pts',(-19.7094260047425,-12.6071692886795,
122.198386280719)) ;
#41566=CARTESIAN_POINT('Ctrl Pts',(-19.7093618923431,-12.6071723244254,
122.198370423662)) ;
#41567=CARTESIAN_POINT('Ctrl Pts',(-19.7092398482187,-12.6071781030863,
122.198340248493)) ;
#41568=CARTESIAN_POINT('Ctrl Pts',(-19.7091819168212,-12.6071808460027,
122.198325929471)) ;
#41569=CARTESIAN_POINT('Ctrl Pts',(-19.7090716261686,-12.607186067866,122.198298677086)) ;
#41570=CARTESIAN_POINT('Ctrl Pts',(-19.7090192673479,-12.6071885468059,
122.198285743023)) ;
#41571=CARTESIAN_POINT('Ctrl Pts',(-19.7089195754003,-12.6071932666276,
122.198261123227)) ;
#41572=CARTESIAN_POINT('Ctrl Pts',(-19.7088722423718,-12.6071955075157,
122.198249436861)) ;
#41573=CARTESIAN_POINT('Ctrl Pts',(-19.7086621076391,-12.6072054557069,
122.198197568342)) ;
#41574=CARTESIAN_POINT('Ctrl Pts',(-19.7084992986925,-12.6072131628154,
122.19815741622)) ;
#41575=CARTESIAN_POINT('Ctrl Pts',(-19.708179391157,-12.6072283055615,122.198078588555)) ;
#41576=CARTESIAN_POINT('Ctrl Pts',(-19.7080222928393,-12.6072357412268,
122.198039910678)) ;
#41577=CARTESIAN_POINT('Ctrl Pts',(-19.7077135496704,-12.6072503533658,
122.197963961149)) ;
#41578=CARTESIAN_POINT('Ctrl Pts',(-19.7075619055399,-12.6072575298429,
122.197926687461)) ;
#41579=CARTESIAN_POINT('Ctrl Pts',(-19.7072638259343,-12.6072716353024,
122.197853479587)) ;
#41580=CARTESIAN_POINT('Ctrl Pts',(-19.7071173905713,-12.6072785643139,
122.197817543388)) ;
#41581=CARTESIAN_POINT('Ctrl Pts',(-19.7042389243756,-12.6074147579478,
122.197111701068)) ;
#41582=CARTESIAN_POINT('Ctrl Pts',(-19.7015046439169,-12.6075439648712,
122.196450991845)) ;
#41583=CARTESIAN_POINT('Ctrl Pts',(-19.6987043805034,-12.607676123953,122.195784334832)) ;
#41584=CARTESIAN_POINT('Ctrl Pts',(-19.6986406059296,-12.6076791337209,
122.195769157359)) ;
#41585=CARTESIAN_POINT('Ctrl Pts',(-19.698514362601,-12.6076850914561,122.195739123674)) ;
#41586=CARTESIAN_POINT('Ctrl Pts',(-19.6984518936512,-12.6076880394362,
122.1957242672)) ;
#41587=CARTESIAN_POINT('Ctrl Pts',(-19.6983282031066,-12.6076938763653,
122.195694860969)) ;
#41588=CARTESIAN_POINT('Ctrl Pts',(-19.6982669812627,-12.6076967653295,
122.195680310952)) ;
#41589=CARTESIAN_POINT('Ctrl Pts',(-19.6981457281189,-12.6077024869176,
122.195651503537)) ;
#41590=CARTESIAN_POINT('Ctrl Pts',(-19.6980856973534,-12.6077053195195,
122.195637246077)) ;
#41591=CARTESIAN_POINT('Ctrl Pts',(-19.6979667723343,-12.6077109309419,
122.195609010383)) ;
#41592=CARTESIAN_POINT('Ctrl Pts',(-19.6979078780992,-12.6077137097645,
122.195595031978)) ;
#41593=CARTESIAN_POINT('Ctrl Pts',(-19.6977911743134,-12.6077192160826,
122.195567341568)) ;
#41594=CARTESIAN_POINT('Ctrl Pts',(-19.6977333646325,-12.6077219435868,
122.195553629367)) ;
#41595=CARTESIAN_POINT('Ctrl Pts',(-19.6976187794936,-12.6077273496572,
122.195526458909)) ;
#41596=CARTESIAN_POINT('Ctrl Pts',(-19.6975620044722,-12.6077300282052,
122.1955130006)) ;
#41597=CARTESIAN_POINT('Ctrl Pts',(-19.697449440663,-12.6077353386347,122.195486326088)) ;
#41598=CARTESIAN_POINT('Ctrl Pts',(-19.6973936515213,-12.6077379705353,
122.195473109657)) ;
#41599=CARTESIAN_POINT('Ctrl Pts',(-19.6972830127344,-12.607743189882,122.195446907401)) ;
#41600=CARTESIAN_POINT('Ctrl Pts',(-19.6972281633212,-12.6077457773194,
122.195433921495)) ;
#41601=CARTESIAN_POINT('Ctrl Pts',(-19.6971193589717,-12.6077509098701,
122.195408169227)) ;
#41602=CARTESIAN_POINT('Ctrl Pts',(-19.6970654040202,-12.6077534549862,
122.195395402735)) ;
#41603=CARTESIAN_POINT('Ctrl Pts',(-19.6969583450318,-12.6077585049555,
122.19537007861)) ;
#41604=CARTESIAN_POINT('Ctrl Pts',(-19.6969052412423,-12.607761009799,122.195357520917)) ;
#41605=CARTESIAN_POINT('Ctrl Pts',(-19.6967998427331,-12.6077659812027,
122.195332604143)) ;
#41606=CARTESIAN_POINT('Ctrl Pts',(-19.6967475478354,-12.6077684477731,
122.195320244909)) ;
#41607=CARTESIAN_POINT('Ctrl Pts',(-19.6966437264461,-12.6077733445542,
122.195295715112)) ;
#41608=CARTESIAN_POINT('Ctrl Pts',(-19.6965921998974,-12.6077757747692,
122.195283544432)) ;
#41609=CARTESIAN_POINT('Ctrl Pts',(-19.6964898757104,-12.6077806007074,
122.195259382105)) ;
#41610=CARTESIAN_POINT('Ctrl Pts',(-19.6964390779954,-12.6077829964357,
122.195247390343)) ;
#41611=CARTESIAN_POINT('Ctrl Pts',(-19.6963381731068,-12.6077877552149,
122.195223576507)) ;
#41612=CARTESIAN_POINT('Ctrl Pts',(-19.6962880659664,-12.6077901182656,
122.195211754349)) ;
#41613=CARTESIAN_POINT('Ctrl Pts',(-19.6961885047292,-12.6077948134625,
122.195188270605)) ;
#41614=CARTESIAN_POINT('Ctrl Pts',(-19.6961390510113,-12.6077971455921,
122.195176609023)) ;
#41615=CARTESIAN_POINT('Ctrl Pts',(-19.6960407609794,-12.6078017806316,
122.195153437773)) ;
#41616=CARTESIAN_POINT('Ctrl Pts',(-19.6959919240049,-12.6078040835739,
122.195141927871)) ;
#41617=CARTESIAN_POINT('Ctrl Pts',(-19.6958948320165,-12.6078086619139,
122.195119051393)) ;
#41618=CARTESIAN_POINT('Ctrl Pts',(-19.6958465770502,-12.6078109373106,
122.195107684755)) ;
#41619=CARTESIAN_POINT('Ctrl Pts',(-19.6957506146551,-12.6078154621864,
122.19508508648)) ;
#41620=CARTESIAN_POINT('Ctrl Pts',(-19.6957029068916,-12.6078177116823,
122.195073854695)) ;
#41621=CARTESIAN_POINT('Ctrl Pts',(-19.6956080047544,-12.6078221863699,
122.195051517883)) ;
#41622=CARTESIAN_POINT('Ctrl Pts',(-19.6955608109201,-12.6078244115372,
122.195040412919)) ;
#41623=CARTESIAN_POINT('Ctrl Pts',(-19.6903983371163,-12.6080678145502,
122.193825971945)) ;
#41624=CARTESIAN_POINT('Ctrl Pts',(-19.6852755117442,-12.6083087869214,
122.192654899501)) ;
#41625=CARTESIAN_POINT('Ctrl Pts',(-19.6750393244738,-12.6087892085501,
122.190382742671)) ;
#41626=CARTESIAN_POINT('Ctrl Pts',(-19.6699261315132,-12.6090286549086,
122.189281379645)) ;
#41627=CARTESIAN_POINT('Ctrl Pts',(-19.6576159234169,-12.609603906466,122.186710547548)) ;
#41628=CARTESIAN_POINT('Ctrl Pts',(-19.6504125670521,-12.6099395127285,
122.185272359259)) ;
#41629=CARTESIAN_POINT('Ctrl Pts',(-19.6186345223002,-12.6114160073915,
122.179218471343)) ;
#41630=CARTESIAN_POINT('Ctrl Pts',(-19.5939371351516,-12.612552702159,122.175277227788)) ;
#41631=CARTESIAN_POINT('Ctrl Pts',(-19.5429227890274,-12.6148881231595,
122.168698845769)) ;
#41632=CARTESIAN_POINT('Ctrl Pts',(-19.5166069563132,-12.6160860748548,
122.166150720282)) ;
#41633=CARTESIAN_POINT('Ctrl Pts',(-19.4774895783422,-12.617868798666,122.163611898003)) ;
#41634=CARTESIAN_POINT('Ctrl Pts',(-19.4647370547848,-12.6184503341318,
122.162980246681)) ;
#41635=CARTESIAN_POINT('Ctrl Pts',(-19.4481949718653,-12.6192065964796,
122.162414773797)) ;
#41636=CARTESIAN_POINT('Ctrl Pts',(-19.4444122264889,-12.6193796709886,
122.162302660851)) ;
#41637=CARTESIAN_POINT('Ctrl Pts',(-19.4370994027916,-12.6197145334933,
122.162119157728)) ;
#41638=CARTESIAN_POINT('Ctrl Pts',(-19.4335694201136,-12.6198762945393,
122.162045542757)) ;
#41639=CARTESIAN_POINT('Ctrl Pts',(-19.4273966833207,-12.6201593496691,
122.161942977503)) ;
#41640=CARTESIAN_POINT('Ctrl Pts',(-19.4247540579576,-12.6202805900396,
122.161907450853)) ;
#41641=CARTESIAN_POINT('Ctrl Pts',(-19.4158363722518,-12.620689914162,122.161815849925)) ;
#41642=CARTESIAN_POINT('Ctrl Pts',(-19.4095610187109,-12.6209782745147,
122.161798648365)) ;
#41643=CARTESIAN_POINT('Ctrl Pts',(-19.3763857784635,-12.6225041419926,
122.161957530909)) ;
#41644=CARTESIAN_POINT('Ctrl Pts',(-19.3494969871598,-12.6237456414186,
122.162954670679)) ;
#41645=CARTESIAN_POINT('Ctrl Pts',(-19.3030391145788,-12.6258943829398,
122.16618142812)) ;
#41646=CARTESIAN_POINT('Ctrl Pts',(-19.2834516409819,-12.6268015222898,
122.16800727749)) ;
#41647=CARTESIAN_POINT('Ctrl Pts',(-19.2535954058591,-12.6281856795908,
122.17150283852)) ;
#41648=CARTESIAN_POINT('Ctrl Pts',(-19.2432908679898,-12.6286636822435,
122.172839730654)) ;
#41649=CARTESIAN_POINT('Ctrl Pts',(-19.2328541455855,-12.6291481394445,
122.174326313922)) ;
#41650=CARTESIAN_POINT('Ctrl Pts',(-19.2327041180626,-12.6291551035688,
122.174347711342)) ;
#41651=CARTESIAN_POINT('Ctrl Pts',(-19.2320853257231,-12.6291838275611,
122.17443608037)) ;
#41652=CARTESIAN_POINT('Ctrl Pts',(-19.2316165951017,-12.6292055864462,
122.174503291056)) ;
#41653=CARTESIAN_POINT('Ctrl Pts',(-19.2307133962872,-12.6292475150354,
122.174633323401)) ;
#41654=CARTESIAN_POINT('Ctrl Pts',(-19.2302789227293,-12.6292676848928,
122.174696107623)) ;
#41655=CARTESIAN_POINT('Ctrl Pts',(-19.2294408644839,-12.6293065917713,
122.174817663155)) ;
#41656=CARTESIAN_POINT('Ctrl Pts',(-19.229037275287,-12.6293253289209,122.174876403138)) ;
#41657=CARTESIAN_POINT('Ctrl Pts',(-19.2282579490958,-12.6293615111381,
122.174990218902)) ;
#41658=CARTESIAN_POINT('Ctrl Pts',(-19.2278822083674,-12.6293789563107,
122.175045268398)) ;
#41659=CARTESIAN_POINT('Ctrl Pts',(-19.2271558456986,-12.6294126812908,
122.175152025387)) ;
#41660=CARTESIAN_POINT('Ctrl Pts',(-19.2268052205377,-12.6294289611899,
122.175203710792)) ;
#41661=CARTESIAN_POINT('Ctrl Pts',(-19.2261266277404,-12.6294604697388,
122.175304036564)) ;
#41662=CARTESIAN_POINT('Ctrl Pts',(-19.2257986573805,-12.6294756984659,
122.175352658314)) ;
#41663=CARTESIAN_POINT('Ctrl Pts',(-19.2251631568053,-12.6295052074923,
122.175447129968)) ;
#41664=CARTESIAN_POINT('Ctrl Pts',(-19.224855624276,-12.629519487857,122.175492964141)) ;
#41665=CARTESIAN_POINT('Ctrl Pts',(-19.2242590000135,-12.6295471928808,
122.175582111665)) ;
#41666=CARTESIAN_POINT('Ctrl Pts',(-19.2239699064247,-12.6295606175903,
122.175625411672)) ;
#41667=CARTESIAN_POINT('Ctrl Pts',(-19.2234083555449,-12.6295866949983,
122.175709721338)) ;
#41668=CARTESIAN_POINT('Ctrl Pts',(-19.2231358964744,-12.629599347749,122.175750719693)) ;
#41669=CARTESIAN_POINT('Ctrl Pts',(-19.2226059834077,-12.6296239569056,
122.175830637693)) ;
#41670=CARTESIAN_POINT('Ctrl Pts',(-19.2223485279447,-12.6296359133535,
122.175869547708)) ;
#41671=CARTESIAN_POINT('Ctrl Pts',(-19.2218471448554,-12.6296591984346,
122.175945483481)) ;
#41672=CARTESIAN_POINT('Ctrl Pts',(-19.2216032160826,-12.6296705270986,
122.175982501006)) ;
#41673=CARTESIAN_POINT('Ctrl Pts',(-19.2211275459536,-12.6296926188009,
122.17605483063)) ;
#41674=CARTESIAN_POINT('Ctrl Pts',(-19.2208958034993,-12.6297033818708,
122.176090135709)) ;
#41675=CARTESIAN_POINT('Ctrl Pts',(-19.2204432864389,-12.629724398972,122.17615920521)) ;
#41676=CARTESIAN_POINT('Ctrl Pts',(-19.2202225108943,-12.6297346530301,
122.176192963621)) ;
#41677=CARTESIAN_POINT('Ctrl Pts',(-19.2197908145895,-12.6297547037577,
122.176259091973)) ;
#41678=CARTESIAN_POINT('Ctrl Pts',(-19.2195798930826,-12.6297645004474,
122.176291456753)) ;
#41679=CARTESIAN_POINT('Ctrl Pts',(-19.219166885471,-12.6297836837448,122.176354938821)) ;
#41680=CARTESIAN_POINT('Ctrl Pts',(-19.2189647987147,-12.6297930703704,
122.176386051681)) ;
#41681=CARTESIAN_POINT('Ctrl Pts',(-19.2185685230648,-12.6298114770519,
122.176447161003)) ;
#41682=CARTESIAN_POINT('Ctrl Pts',(-19.2183743335841,-12.6298204971244,
122.176477153672)) ;
#41683=CARTESIAN_POINT('Ctrl Pts',(-19.2179929859661,-12.6298382109194,
122.176536145082)) ;
#41684=CARTESIAN_POINT('Ctrl Pts',(-19.2178058273476,-12.6298469046551,
122.17656514057)) ;
#41685=CARTESIAN_POINT('Ctrl Pts',(-19.2174377361236,-12.6298640031592,
122.176622252649)) ;
#41686=CARTESIAN_POINT('Ctrl Pts',(-19.217256803013,-12.6298724079432,122.176650366475)) ;
#41687=CARTESIAN_POINT('Ctrl Pts',(-19.21690040926,-12.6298889635257,122.176705824004)) ;
#41688=CARTESIAN_POINT('Ctrl Pts',(-19.2167249482493,-12.6298971143347,
122.176733165344)) ;
#41689=CARTESIAN_POINT('Ctrl Pts',(-19.2163787882633,-12.6299131949506,
122.176787181534)) ;
#41690=CARTESIAN_POINT('Ctrl Pts',(-19.2162080890678,-12.6299211247621,
122.176813854373)) ;
#41691=CARTESIAN_POINT('Ctrl Pts',(-19.2158707773977,-12.6299367947389,
122.176866633117)) ;
#41692=CARTESIAN_POINT('Ctrl Pts',(-19.2157041645138,-12.6299445349184,
122.176892737376)) ;
#41693=CARTESIAN_POINT('Ctrl Pts',(-19.215374376648,-12.6299598557597,122.176944475638)) ;
#41694=CARTESIAN_POINT('Ctrl Pts',(-19.2152112016524,-12.6299674364181,
122.176970108237)) ;
#41695=CARTESIAN_POINT('Ctrl Pts',(-19.214887659885,-12.6299824674594,122.177020998013)) ;
#41696=CARTESIAN_POINT('Ctrl Pts',(-19.2147272926278,-12.6299899178617,
122.177046254141)) ;
#41697=CARTESIAN_POINT('Ctrl Pts',(-19.2144087467008,-12.6300047171697,
122.177096485315)) ;
#41698=CARTESIAN_POINT('Ctrl Pts',(-19.2142505681731,-12.6300120660663,
122.177121459475)) ;
#41699=CARTESIAN_POINT('Ctrl Pts',(-19.2139357821194,-12.6300266910494,
122.177171221757)) ;
#41700=CARTESIAN_POINT('Ctrl Pts',(-19.2137791745908,-12.6300339671342,
122.177196009267)) ;
#41701=CARTESIAN_POINT('Ctrl Pts',(-19.2134669057242,-12.6300484755186,
122.177245495431)) ;
#41702=CARTESIAN_POINT('Ctrl Pts',(-19.2133112441929,-12.6300557078261,
122.177270193752)) ;
#41703=CARTESIAN_POINT('Ctrl Pts',(-19.2057079430292,-12.6304089747836,
122.178478059654)) ;
#41704=CARTESIAN_POINT('Ctrl Pts',(-19.1982711444168,-12.6307547041646,
122.179728571221)) ;
#41705=CARTESIAN_POINT('Ctrl Pts',(-19.1834408532855,-12.6314446406511,
122.182360523757)) ;
#41706=CARTESIAN_POINT('Ctrl Pts',(-19.1760476010201,-12.6317888352755,
122.183741553141)) ;
#41707=CARTESIAN_POINT('Ctrl Pts',(-19.1551189992639,-12.6327640416747,
122.187846740422)) ;
#41708=CARTESIAN_POINT('Ctrl Pts',(-19.1416156682069,-12.6333942802176,
122.190728545803)) ;
#41709=CARTESIAN_POINT('Ctrl Pts',(-19.0661340313394,-12.636925871898,122.208149672345)) ;
#41710=CARTESIAN_POINT('Ctrl Pts',(-19.0052893743557,-12.6398087058573,
122.227183451971)) ;
#41711=CARTESIAN_POINT('Ctrl Pts',(-18.9149366045977,-12.6442413311643,
122.263222930508)) ;
#41712=CARTESIAN_POINT('Ctrl Pts',(-18.8842284343812,-12.6457738995312,
122.27693155338)) ;
#41713=CARTESIAN_POINT('Ctrl Pts',(-18.8391459719155,-12.6480717008126,
122.299278974222)) ;
#41714=CARTESIAN_POINT('Ctrl Pts',(-18.824331823361,-12.6488348427199,122.30699597971)) ;
#41715=CARTESIAN_POINT('Ctrl Pts',(-18.7999530658644,-12.6501057378032,
122.32032320454)) ;
#41716=CARTESIAN_POINT('Ctrl Pts',(-18.7903004680454,-12.6506129655805,
122.32576797826)) ;
#41717=CARTESIAN_POINT('Ctrl Pts',(-18.7783091002417,-12.6512485272351,
122.33274378916)) ;
#41718=CARTESIAN_POINT('Ctrl Pts',(-18.7759013432938,-12.6513764198403,
122.33415528227)) ;
#41719=CARTESIAN_POINT('Ctrl Pts',(-18.7670487639839,-12.6518476839976,
122.339384823345)) ;
#41720=CARTESIAN_POINT('Ctrl Pts',(-18.7606335807206,-12.6521912364205,
122.343252712879)) ;
#41721=CARTESIAN_POINT('Ctrl Pts',(-18.7464048898659,-12.6529580188698,
122.352006930493)) ;
#41722=CARTESIAN_POINT('Ctrl Pts',(-18.7386098729769,-12.6533813616417,
122.356922469633)) ;
#41723=CARTESIAN_POINT('Ctrl Pts',(-18.7182237799422,-12.6544976850978,
122.370095243963)) ;
#41724=CARTESIAN_POINT('Ctrl Pts',(-18.7057263480336,-12.655191387144,122.378494532999)) ;
#41725=CARTESIAN_POINT('Ctrl Pts',(-18.661383944203,-12.6576898506211,122.409473661028)) ;
#41726=CARTESIAN_POINT('Ctrl Pts',(-18.630449572009,-12.6595074050684,122.433316059771)) ;
#41727=CARTESIAN_POINT('Ctrl Pts',(-18.5761658949485,-12.6628381702742,
122.479362045516)) ;
#41728=CARTESIAN_POINT('Ctrl Pts',(-18.5524608573029,-12.6643427238562,
122.501096074152)) ;
#41729=CARTESIAN_POINT('Ctrl Pts',(-18.5214989868315,-12.6663677019011,
122.531763624268)) ;
#41730=CARTESIAN_POINT('Ctrl Pts',(-18.5134887348652,-12.6668974640506,
122.539918401899)) ;
#41731=CARTESIAN_POINT('Ctrl Pts',(-18.5014977361161,-12.667699428476,122.552465447875)) ;
#41732=CARTESIAN_POINT('Ctrl Pts',(-18.4974345599665,-12.6679727817489,
122.556778016611)) ;
#41733=CARTESIAN_POINT('Ctrl Pts',(-18.4901635195785,-12.668464873343,122.564606119295)) ;
#41734=CARTESIAN_POINT('Ctrl Pts',(-18.4869447827434,-12.6686837672033,
122.56811138798)) ;
#41735=CARTESIAN_POINT('Ctrl Pts',(-18.4815131203139,-12.6690549693455,
122.574094806925)) ;
#41736=CARTESIAN_POINT('Ctrl Pts',(-18.4792899194231,-12.6692074283339,
122.576563548974)) ;
#41737=CARTESIAN_POINT('Ctrl Pts',(-18.4750700222158,-12.6694978250517,
122.581287247649)) ;
#41738=CARTESIAN_POINT('Ctrl Pts',(-18.4730715829044,-12.6696357878119,
122.583540614292)) ;
#41739=CARTESIAN_POINT('Ctrl Pts',(-18.4684621772687,-12.6699550260662,
122.588776006018)) ;
#41740=CARTESIAN_POINT('Ctrl Pts',(-18.4658572084882,-12.6701362118605,
122.591763273304)) ;
#41741=CARTESIAN_POINT('Ctrl Pts',(-18.4577135960731,-12.6707050992548,
122.601192182458)) ;
#41742=CARTESIAN_POINT('Ctrl Pts',(-18.4522263678402,-12.6710920427928,
122.607677948871)) ;
#41743=CARTESIAN_POINT('Ctrl Pts',(-18.42261589974,-12.6732008171969,122.643409215233)) ;
#41744=CARTESIAN_POINT('Ctrl Pts',(-18.3997664505841,-12.6749032551716,
122.673684744541)) ;
#41745=CARTESIAN_POINT('Ctrl Pts',(-18.3538817853352,-12.6785388722717,
122.740606617841)) ;
#41746=CARTESIAN_POINT('Ctrl Pts',(-18.3313019093948,-12.6804754585744,
122.77750466779)) ;
#41747=CARTESIAN_POINT('Ctrl Pts',(-18.3014044680669,-12.6833092522263,
122.832584729281)) ;
#41748=CARTESIAN_POINT('Ctrl Pts',(-18.2925298800675,-12.6841907254495,
122.849885131158)) ;
#41749=CARTESIAN_POINT('Ctrl Pts',(-18.2792955763098,-12.6855724906585,
122.877237398557)) ;
#41750=CARTESIAN_POINT('Ctrl Pts',(-18.2746583098953,-12.6860709525609,
122.887151595537)) ;
#41751=CARTESIAN_POINT('Ctrl Pts',(-18.267106157034,-12.6869076388084,122.903866177355)) ;
#41752=CARTESIAN_POINT('Ctrl Pts',(-18.2641203595118,-12.6872454130824,
122.910633865986)) ;
#41753=CARTESIAN_POINT('Ctrl Pts',(-18.2587962826136,-12.6878607690106,
122.922997572714)) ;
#41754=CARTESIAN_POINT('Ctrl Pts',(-18.2564383210447,-12.6881382245845,
122.92858487498)) ;
#41755=CARTESIAN_POINT('Ctrl Pts',(-18.251730558928,-12.6887024069194,122.93997073982)) ;
#41756=CARTESIAN_POINT('Ctrl Pts',(-18.2493834459303,-12.6889891411828,
122.945770230628)) ;
#41757=CARTESIAN_POINT('Ctrl Pts',(-18.2443071692216,-12.6896215946021,
122.958589135016)) ;
#41758=CARTESIAN_POINT('Ctrl Pts',(-18.2415977053822,-12.6899674154144,
122.965616083993)) ;
#41759=CARTESIAN_POINT('Ctrl Pts',(-18.2343375333888,-12.6909173795375,
122.984964323006)) ;
#41760=CARTESIAN_POINT('Ctrl Pts',(-18.2299172780155,-12.6915222193984,
122.997333491861)) ;
#41761=CARTESIAN_POINT('Ctrl Pts',(-18.2093085207767,-12.694478434943,123.058003660494)) ;
#41762=CARTESIAN_POINT('Ctrl Pts',(-18.1958882779016,-12.6968431854278,
123.107193023935)) ;
#41763=CARTESIAN_POINT('Ctrl Pts',(-18.1774542858308,-12.7010750666826,
123.195745579125)) ;
#41764=CARTESIAN_POINT('Ctrl Pts',(-18.1712402661295,-12.7029291714922,
123.23478869457)) ;
#41765=CARTESIAN_POINT('Ctrl Pts',(-18.1654539819847,-12.7053718894351,
123.286974583963)) ;
#41766=CARTESIAN_POINT('Ctrl Pts',(-18.1642235341705,-12.7059746615582,
123.299910144494)) ;
#41767=CARTESIAN_POINT('Ctrl Pts',(-18.1626765950558,-12.7068782140379,
123.319390404262)) ;
#41768=CARTESIAN_POINT('Ctrl Pts',(-18.1622095214984,-12.7071804742072,
123.325922180861)) ;
#41769=CARTESIAN_POINT('Ctrl Pts',(-18.1615327254344,-12.7076716790464,
123.336561296873)) ;
#41770=CARTESIAN_POINT('Ctrl Pts',(-18.1612919099343,-12.7078609439941,
123.340666516006)) ;
#41771=CARTESIAN_POINT('Ctrl Pts',(-18.1608750310765,-12.7082182780589,
123.34842810391)) ;
#41772=CARTESIAN_POINT('Ctrl Pts',(-18.1606947626094,-12.7083863898857,
123.352084201567)) ;
#41773=CARTESIAN_POINT('Ctrl Pts',(-18.1603887097239,-12.7086994042937,
123.35889993839)) ;
#41774=CARTESIAN_POINT('Ctrl Pts',(-18.1602588499147,-12.7088443489854,
123.362059363132)) ;
#41775=CARTESIAN_POINT('Ctrl Pts',(-18.1600049796484,-12.7091562594369,
123.368865168655)) ;
#41776=CARTESIAN_POINT('Ctrl Pts',(-18.1598849423355,-12.7093231816509,
123.372511670275)) ;
#41777=CARTESIAN_POINT('Ctrl Pts',(-18.1596045888525,-12.709772398752,123.382336161789)) ;
#41778=CARTESIAN_POINT('Ctrl Pts',(-18.159474120741,-12.7100543749281,123.38851491354)) ;
#41779=CARTESIAN_POINT('Ctrl Pts',(-18.1590117737733,-12.7115921273386,
123.422269624332)) ;
#41780=CARTESIAN_POINT('Ctrl Pts',(-18.1595467225219,-12.7128384326479,
123.449850025637)) ;
#41781=CARTESIAN_POINT('Ctrl Pts',(-18.1611750874062,-12.7142357117041,
123.480846876769)) ;
#41782=CARTESIAN_POINT('Ctrl Pts',(-18.1613710178504,-12.7143914426241,
123.484302500605)) ;
#41783=CARTESIAN_POINT('Ctrl Pts',(-18.1617139215948,-12.7146452921126,
123.489936179065)) ;
#41784=CARTESIAN_POINT('Ctrl Pts',(-18.1618522523349,-12.7147434473181,
123.492114738866)) ;
#41785=CARTESIAN_POINT('Ctrl Pts',(-18.1644289779936,-12.7164990055125,
123.531081082994)) ;
#41786=CARTESIAN_POINT('Ctrl Pts',(-18.1684880122812,-12.7181494619589,
123.567743186609)) ;
#41787=CARTESIAN_POINT('Ctrl Pts',(-18.1769816217963,-12.7206445999397,
123.622279720628)) ;
#41788=CARTESIAN_POINT('Ctrl Pts',(-18.1801994938702,-12.7214758827103,
123.640322592031)) ;
#41789=CARTESIAN_POINT('Ctrl Pts',(-18.1862202536776,-12.7228648724916,
123.670257618892)) ;
#41790=CARTESIAN_POINT('Ctrl Pts',(-18.1888028923239,-12.7234212188363,
123.682191224482)) ;
#41791=CARTESIAN_POINT('Ctrl Pts',(-18.1937585235136,-12.7244227162455,
123.703569758564)) ;
#41792=CARTESIAN_POINT('Ctrl Pts',(-18.196067855581,-12.724867531529,123.713028450735)) ;
#41793=CARTESIAN_POINT('Ctrl Pts',(-18.2009245696807,-12.7257612735697,
123.731958223253)) ;
#41794=CARTESIAN_POINT('Ctrl Pts',(-18.2034733879766,-12.7262101759464,
123.741428245317)) ;
#41795=CARTESIAN_POINT('Ctrl Pts',(-18.208547693183,-12.7270672430795,123.759434561359)) ;
#41796=CARTESIAN_POINT('Ctrl Pts',(-18.2110534508749,-12.7274753170839,
123.767975804784)) ;
#41797=CARTESIAN_POINT('Ctrl Pts',(-18.2177465313335,-12.7285278005071,
123.78991970147)) ;
#41798=CARTESIAN_POINT('Ctrl Pts',(-18.222068836222,-12.729172528345,123.803279863462)) ;
#41799=CARTESIAN_POINT('Ctrl Pts',(-18.226624312154,-12.7298190838978,123.816590711209)) ;
#41800=CARTESIAN_POINT('Ctrl Pts',(-18.2266333383706,-12.7298203648599,
123.816617082436)) ;
#41801=CARTESIAN_POINT('Ctrl Pts',(-18.2266423654683,-12.7298216458232,
123.816643453356)) ;
#41802=CARTESIAN_POINT('',(-20.5919009558702,-12.4898128815389,123.006981918687)) ;
#41803=CARTESIAN_POINT('Ctrl Pts',(-18.2266423654705,-12.6697781342469,
123.816643453362)) ;
#41804=CARTESIAN_POINT('Ctrl Pts',(-18.2222198725711,-12.6691526626378,
123.803723995805)) ;
#41805=CARTESIAN_POINT('Ctrl Pts',(-18.2180093556767,-12.6685278300723,
123.790732860964)) ;
#41806=CARTESIAN_POINT('Ctrl Pts',(-18.2086322522418,-12.6670628909818,
123.760098065799)) ;
#41807=CARTESIAN_POINT('Ctrl Pts',(-18.2036403657761,-12.6662233326266,
123.742404295056)) ;
#41808=CARTESIAN_POINT('Ctrl Pts',(-18.19298079256,-12.6642778060177,123.701161126861)) ;
#41809=CARTESIAN_POINT('Ctrl Pts',(-18.1876036952942,-12.6631723117401,
123.677544292641)) ;
#41810=CARTESIAN_POINT('Ctrl Pts',(-18.1816338847035,-12.6617606659644,
123.647288244401)) ;
#41811=CARTESIAN_POINT('Ctrl Pts',(-18.1804034253215,-12.6614572806127,
123.640780116299)) ;
#41812=CARTESIAN_POINT('Ctrl Pts',(-18.1792049658555,-12.6611485008418,
123.634153124928)) ;
#41813=CARTESIAN_POINT('Ctrl Pts',(-18.1791851952805,-12.6611434031646,
123.634043718373)) ;
#41814=CARTESIAN_POINT('Ctrl Pts',(-18.1791518820801,-12.6611348071483,
123.633859228886)) ;
#41815=CARTESIAN_POINT('Ctrl Pts',(-18.1791383317286,-12.6611313088524,
123.633784147331)) ;
#41816=CARTESIAN_POINT('Ctrl Pts',(-18.1791126313361,-12.6611246703369,
123.633641668613)) ;
#41817=CARTESIAN_POINT('Ctrl Pts',(-18.1791004799697,-12.6611215301275,
123.633574271746)) ;
#41818=CARTESIAN_POINT('Ctrl Pts',(-18.1790774318414,-12.6611155711528,
123.633446376416)) ;
#41819=CARTESIAN_POINT('Ctrl Pts',(-18.1790665339962,-12.6611127523918,
123.633385878106)) ;
#41820=CARTESIAN_POINT('Ctrl Pts',(-18.1790458624592,-12.6611074033964,
123.633271073575)) ;
#41821=CARTESIAN_POINT('Ctrl Pts',(-18.1790360878958,-12.6611048731659,
123.633216767484)) ;
#41822=CARTESIAN_POINT('Ctrl Pts',(-18.179017546121,-12.661100071661,123.633113712869)) ;
#41823=CARTESIAN_POINT('Ctrl Pts',(-18.1790087782331,-12.6610978003963,
123.633064964592)) ;
#41824=CARTESIAN_POINT('Ctrl Pts',(-18.1789928277888,-12.6610936671406,
123.632976252003)) ;
#41825=CARTESIAN_POINT('Ctrl Pts',(-18.1789856442511,-12.661091805147,123.632936287691)) ;
#41826=CARTESIAN_POINT('Ctrl Pts',(-18.1789714724399,-12.6610881307546,
123.632857423312)) ;
#41827=CARTESIAN_POINT('Ctrl Pts',(-18.1789644840787,-12.6610863183602,
123.632818523347)) ;
#41828=CARTESIAN_POINT('Ctrl Pts',(-18.1789506970924,-12.6610827418132,
123.632741758643)) ;
#41829=CARTESIAN_POINT('Ctrl Pts',(-18.1789438983696,-12.661080977661,123.632703893917)) ;
#41830=CARTESIAN_POINT('Ctrl Pts',(-18.1789304853164,-12.6610774962882,
123.632629171589)) ;
#41831=CARTESIAN_POINT('Ctrl Pts',(-18.1789238708723,-12.6610757790624,
123.63259231388)) ;
#41832=CARTESIAN_POINT('Ctrl Pts',(-18.1789108211518,-12.6610723902585,
123.63251957804)) ;
#41833=CARTESIAN_POINT('Ctrl Pts',(-18.1789043858028,-12.6610707186845,
123.632483700004)) ;
#41834=CARTESIAN_POINT('Ctrl Pts',(-18.1788916892156,-12.6610674199392,
123.632412896805)) ;
#41835=CARTESIAN_POINT('Ctrl Pts',(-18.1788854278926,-12.6610657927677,
123.632377971642)) ;
#41836=CARTESIAN_POINT('Ctrl Pts',(-18.1788730744341,-12.6610625816129,
123.632309048137)) ;
#41837=CARTESIAN_POINT('Ctrl Pts',(-18.1788669822482,-12.6610609976372,
123.632275049961)) ;
#41838=CARTESIAN_POINT('Ctrl Pts',(-18.1788549623318,-12.6610578717051,
123.632207955356)) ;
#41839=CARTESIAN_POINT('Ctrl Pts',(-18.1788490344895,-12.6610563297393,
123.632174858727)) ;
#41840=CARTESIAN_POINT('Ctrl Pts',(-18.1788373386141,-12.6610532866768,
123.632109542538)) ;
#41841=CARTESIAN_POINT('Ctrl Pts',(-18.1788315705353,-12.6610517855868,
123.632077323125)) ;
#41842=CARTESIAN_POINT('Ctrl Pts',(-18.178820189713,-12.6610488231668,123.632013737577)) ;
#41843=CARTESIAN_POINT('Ctrl Pts',(-18.1788145768701,-12.6610473618286,
123.631982371267)) ;
#41844=CARTESIAN_POINT('Ctrl Pts',(-18.1788035021421,-12.6610444778248,
123.631920468596)) ;
#41845=CARTESIAN_POINT('Ctrl Pts',(-18.178798040216,-12.6610430551653,123.631889932366)) ;
#41846=CARTESIAN_POINT('Ctrl Pts',(-18.1787872630764,-12.6610402474628,
123.631829667196)) ;
#41847=CARTESIAN_POINT('Ctrl Pts',(-18.1787819478163,-12.6610388624234,
123.631799938338)) ;
#41848=CARTESIAN_POINT('Ctrl Pts',(-18.1787714599335,-12.6610361289464,
123.631741266135)) ;
#41849=CARTESIAN_POINT('Ctrl Pts',(-18.1787662872217,-12.6610347805005,
123.631712322618)) ;
#41850=CARTESIAN_POINT('Ctrl Pts',(-18.1787560804207,-12.6610321192082,
123.631655199598)) ;
#41851=CARTESIAN_POINT('Ctrl Pts',(-18.1787510463077,-12.6610308063697,
123.631627020268)) ;
#41852=CARTESIAN_POINT('Ctrl Pts',(-18.1787411128303,-12.6610282153243,
123.631571404855)) ;
#41853=CARTESIAN_POINT('Ctrl Pts',(-18.1787362134164,-12.6610269371179,
123.631543968784)) ;
#41854=CARTESIAN_POINT('Ctrl Pts',(-18.1787265455952,-12.6610244144002,
123.631489819798)) ;
#41855=CARTESIAN_POINT('Ctrl Pts',(-18.178721777131,-12.6610231698868,123.631463106839)) ;
#41856=CARTESIAN_POINT('Ctrl Pts',(-18.1787123675407,-12.6610207136356,
123.631410384348)) ;
#41857=CARTESIAN_POINT('Ctrl Pts',(-18.1787077263944,-12.6610195019045,
123.631384374963)) ;
#41858=CARTESIAN_POINT('Ctrl Pts',(-18.1786985679346,-12.6610171103388,
123.631333040751)) ;
#41859=CARTESIAN_POINT('Ctrl Pts',(-18.1786940505312,-12.6610159304921,
123.631307715668)) ;
#41860=CARTESIAN_POINT('Ctrl Pts',(-18.1786851360851,-12.6610136018221,
123.631257731334)) ;
#41861=CARTESIAN_POINT('Ctrl Pts',(-18.1786807390407,-12.6610124530092,
123.631233072307)) ;
#41862=CARTESIAN_POINT('Ctrl Pts',(-18.1786720619454,-12.6610101855594,
123.631184401898)) ;
#41863=CARTESIAN_POINT('Ctrl Pts',(-18.1786677818952,-12.6610090669329,
123.631160390743)) ;
#41864=CARTESIAN_POINT('Ctrl Pts',(-18.1786593355864,-12.6610068590496,
123.631112998777)) ;
#41865=CARTESIAN_POINT('Ctrl Pts',(-18.1786551692717,-12.6610057697879,
123.631089617863)) ;
#41866=CARTESIAN_POINT('Ctrl Pts',(-18.1786474529009,-12.6610037520521,
123.631046307264)) ;
#41867=CARTESIAN_POINT('Ctrl Pts',(-18.1786439026348,-12.6610028235718,
123.631026377457)) ;
#41868=CARTESIAN_POINT('Ctrl Pts',(-18.1786368277849,-12.6610009730697,
123.630986656424)) ;
#41869=CARTESIAN_POINT('Ctrl Pts',(-18.1786333031354,-12.6610000510325,
123.630966864868)) ;
#41870=CARTESIAN_POINT('Ctrl Pts',(-18.1786262792059,-12.6609982133402,
123.630927418699)) ;
#41871=CARTESIAN_POINT('Ctrl Pts',(-18.1786227800154,-12.6609972977102,
123.630907764626)) ;
#41872=CARTESIAN_POINT('Ctrl Pts',(-18.1786158068435,-12.6609954727955,
123.630868592636)) ;
#41873=CARTESIAN_POINT('Ctrl Pts',(-18.1786123327889,-12.6609945634934,
123.630849074345)) ;
#41874=CARTESIAN_POINT('Ctrl Pts',(-18.1786054096866,-12.6609927511868,
123.630810172895)) ;
#41875=CARTESIAN_POINT('Ctrl Pts',(-18.1786019606267,-12.6609918481809,
123.630790789704)) ;
#41876=CARTESIAN_POINT('Ctrl Pts',(-18.1785950872891,-12.6609900484128,
123.630752157304)) ;
#41877=CARTESIAN_POINT('Ctrl Pts',(-18.1785916629856,-12.6609891516457,
123.630732907986)) ;
#41878=CARTESIAN_POINT('Ctrl Pts',(-18.1785848389233,-12.6609873642982,
123.630694542104)) ;
#41879=CARTESIAN_POINT('Ctrl Pts',(-18.1785814391846,-12.6609864737247,
123.63067542569)) ;
#41880=CARTESIAN_POINT('Ctrl Pts',(-18.1785746640443,-12.6609846987152,
123.630637324558)) ;
#41881=CARTESIAN_POINT('Ctrl Pts',(-18.1785712886371,-12.6609838142793,
123.630618339843)) ;
#41882=CARTESIAN_POINT('Ctrl Pts',(-18.1785645619599,-12.6609820514973,
123.630580501093)) ;
#41883=CARTESIAN_POINT('Ctrl Pts',(-18.1785612106855,-12.6609811731517,
123.630561647066)) ;
#41884=CARTESIAN_POINT('Ctrl Pts',(-18.1785545320595,-12.6609794224991,
123.63052406859)) ;
#41885=CARTESIAN_POINT('Ctrl Pts',(-18.178551204716,-12.6609785501958,123.63050534422)) ;
#41886=CARTESIAN_POINT('Ctrl Pts',(-18.1785445737538,-12.6609768115805,
123.630468024045)) ;
#41887=CARTESIAN_POINT('Ctrl Pts',(-18.1785412701285,-12.6609759452684,
123.630449428237)) ;
#41888=CARTESIAN_POINT('Ctrl Pts',(-18.178534686392,-12.660974218585,123.630412364102)) ;
#41889=CARTESIAN_POINT('Ctrl Pts',(-18.178531406295,-12.660973358219,123.630393895889)) ;
#41890=CARTESIAN_POINT('Ctrl Pts',(-18.1785248694447,-12.6609716433877,
123.630357086084)) ;
#41891=CARTESIAN_POINT('Ctrl Pts',(-18.1785216126508,-12.6609707889133,
123.630338744297)) ;
#41892=CARTESIAN_POINT('Ctrl Pts',(-18.1785151221673,-12.660969085807,123.630302186095)) ;
#41893=CARTESIAN_POINT('Ctrl Pts',(-18.1785118885266,-12.6609682371894,
123.630283969988)) ;
#41894=CARTESIAN_POINT('Ctrl Pts',(-18.1785054441989,-12.6609665457617,
123.630247662396)) ;
#41895=CARTESIAN_POINT('Ctrl Pts',(-18.1785022334477,-12.6609657029363,
123.630229570582)) ;
#41896=CARTESIAN_POINT('Ctrl Pts',(-18.1784958346946,-12.6609640230436,
123.630193510517)) ;
#41897=CARTESIAN_POINT('Ctrl Pts',(-18.1784926467002,-12.6609631859798,
123.630175542342)) ;
#41898=CARTESIAN_POINT('Ctrl Pts',(-18.1784862932401,-12.6609615175568,
123.630139728408)) ;
#41899=CARTESIAN_POINT('Ctrl Pts',(-18.1784831277879,-12.6609606862027,
123.630121882756)) ;
#41900=CARTESIAN_POINT('Ctrl Pts',(-18.1784768192196,-12.6609590291528,
123.630086312877)) ;
#41901=CARTESIAN_POINT('Ctrl Pts',(-18.1784736761173,-12.6609582034621,
123.630068588759)) ;
#41902=CARTESIAN_POINT('Ctrl Pts',(-18.1784674120955,-12.660956557703,123.630033261172)) ;
#41903=CARTESIAN_POINT('Ctrl Pts',(-18.1784642911362,-12.6609557376256,
123.630015657511)) ;
#41904=CARTESIAN_POINT('Ctrl Pts',(-18.1784580712099,-12.6609541030473,
123.629980569855)) ;
#41905=CARTESIAN_POINT('Ctrl Pts',(-18.1784549722345,-12.6609532885455,
123.629963085843)) ;
#41906=CARTESIAN_POINT('Ctrl Pts',(-18.1784487960732,-12.6609516650692,
123.629928236432)) ;
#41907=CARTESIAN_POINT('Ctrl Pts',(-18.1784457188897,-12.6609508560967,
123.629910871075)) ;
#41908=CARTESIAN_POINT('Ctrl Pts',(-18.1784395861508,-12.6609492436407,
123.629876258152)) ;
#41909=CARTESIAN_POINT('Ctrl Pts',(-18.1784365305591,-12.6609484401489,
123.629859010409)) ;
#41910=CARTESIAN_POINT('Ctrl Pts',(-18.1784304408045,-12.6609468386058,
123.629824631675)) ;
#41911=CARTESIAN_POINT('Ctrl Pts',(-18.1784274066506,-12.6609460405582,
123.629807500762)) ;
#41912=CARTESIAN_POINT('Ctrl Pts',(-18.1784213595656,-12.6609444498532,
123.629773354611)) ;
#41913=CARTESIAN_POINT('Ctrl Pts',(-18.1784183466596,-12.6609436572038,
123.629756339541)) ;
#41914=CARTESIAN_POINT('Ctrl Pts',(-18.178412341923,-12.6609420772603,123.629722424328)) ;
#41915=CARTESIAN_POINT('Ctrl Pts',(-18.1784093500629,-12.6609412899597,
123.629705524045)) ;
#41916=CARTESIAN_POINT('Ctrl Pts',(-18.178403387222,-12.6609397206661,123.629671837378)) ;
#41917=CARTESIAN_POINT('Ctrl Pts',(-18.178400416268,-12.6609389386814,123.629655051174)) ;
#41918=CARTESIAN_POINT('Ctrl Pts',(-18.1783944951202,-12.6609373799921,
123.629621592074)) ;
#41919=CARTESIAN_POINT('Ctrl Pts',(-18.1783915448412,-12.6609366032662,
123.629604918724)) ;
#41920=CARTESIAN_POINT('Ctrl Pts',(-18.1783856648063,-12.6609350550358,
123.629571684074)) ;
#41921=CARTESIAN_POINT('Ctrl Pts',(-18.178382735116,-12.6609342835497,123.62955512317)) ;
#41922=CARTESIAN_POINT('Ctrl Pts',(-18.1783768960917,-12.6609327457586,
123.629522112549)) ;
#41923=CARTESIAN_POINT('Ctrl Pts',(-18.1783739867411,-12.6609319794504,
123.629505662764)) ;
#41924=CARTESIAN_POINT('Ctrl Pts',(-18.1783681882437,-12.6609304519784,
123.629472873596)) ;
#41925=CARTESIAN_POINT('Ctrl Pts',(-18.1783652990943,-12.6609296908152,
123.629456534224)) ;
#41926=CARTESIAN_POINT('Ctrl Pts',(-18.1783595408339,-12.6609281735932,
123.629423965023)) ;
#41927=CARTESIAN_POINT('Ctrl Pts',(-18.1783566717088,-12.6609274175319,
123.62940773514)) ;
#41928=CARTESIAN_POINT('Ctrl Pts',(-18.1783509532808,-12.6609259104603,
123.629375383771)) ;
#41929=CARTESIAN_POINT('Ctrl Pts',(-18.1783481040431,-12.6609251594683,
123.629359262678)) ;
#41930=CARTESIAN_POINT('Ctrl Pts',(-18.1783424252856,-12.6609236625113,
123.629327128374)) ;
#41931=CARTESIAN_POINT('Ctrl Pts',(-18.1783395957,-12.6609229165301,123.629311114814)) ;
#41932=CARTESIAN_POINT('Ctrl Pts',(-18.1783339560997,-12.6609214295592,
123.629279194819)) ;
#41933=CARTESIAN_POINT('Ctrl Pts',(-18.178331146059,-12.6609206885638,123.62926328826)) ;
#41934=CARTESIAN_POINT('Ctrl Pts',(-18.1783255453141,-12.6609192115063,
123.629231581011)) ;
#41935=CARTESIAN_POINT('Ctrl Pts',(-18.1783227546722,-12.6609184754616,
123.629215780698)) ;
#41936=CARTESIAN_POINT('Ctrl Pts',(-18.1783171926251,-12.6609170082824,
123.629184285446)) ;
#41937=CARTESIAN_POINT('Ctrl Pts',(-18.178314421147,-12.6609162771297,123.629168590119)) ;
#41938=CARTESIAN_POINT('Ctrl Pts',(-18.1783088972574,-12.6609148196929,
123.629137303948)) ;
#41939=CARTESIAN_POINT('Ctrl Pts',(-18.1783061448562,-12.6609140934126,
123.629121713186)) ;
#41940=CARTESIAN_POINT('Ctrl Pts',(-18.1783006589467,-12.6609126456778,
123.62909063523)) ;
#41941=CARTESIAN_POINT('Ctrl Pts',(-18.1782979254317,-12.6609119242227,
123.629075148021)) ;
#41942=CARTESIAN_POINT('Ctrl Pts',(-18.1782924771045,-12.6609104860913,
123.629044276164)) ;
#41943=CARTESIAN_POINT('Ctrl Pts',(-18.178289762344,-12.6609097694297,123.629028891831)) ;
#41944=CARTESIAN_POINT('Ctrl Pts',(-18.1782843514437,-12.660908340867,123.628998225328)) ;
#41945=CARTESIAN_POINT('Ctrl Pts',(-18.1782816552182,-12.6609076289442,
123.628982942694)) ;
#41946=CARTESIAN_POINT('Ctrl Pts',(-18.1782762811695,-12.6609062098044,
123.628952478418)) ;
#41947=CARTESIAN_POINT('Ctrl Pts',(-18.1782736034264,-12.6609055026096,
123.628937297252)) ;
#41948=CARTESIAN_POINT('Ctrl Pts',(-18.1782682662141,-12.6609040928948,
123.628907035249)) ;
#41949=CARTESIAN_POINT('Ctrl Pts',(-18.178265606707,-12.6609033903658,123.628891954219)) ;
#41950=CARTESIAN_POINT('Ctrl Pts',(-18.1782603058577,-12.660901989957,123.628861891935)) ;
#41951=CARTESIAN_POINT('Ctrl Pts',(-18.1782576644744,-12.6609012920673,
123.628846910469)) ;
#41952=CARTESIAN_POINT('Ctrl Pts',(-18.178252399662,-12.6608999008842,123.628817046183)) ;
#41953=CARTESIAN_POINT('Ctrl Pts',(-18.178249776286,-12.6608992076058,123.628802163684)) ;
#41954=CARTESIAN_POINT('Ctrl Pts',(-18.1782445473528,-12.6608978256126,
123.628772496627)) ;
#41955=CARTESIAN_POINT('Ctrl Pts',(-18.178241941783,-12.6608971368954,123.628757712017)) ;
#41956=CARTESIAN_POINT('Ctrl Pts',(-18.1782367483339,-12.6608957639934,
123.628728240072)) ;
#41957=CARTESIAN_POINT('Ctrl Pts',(-18.1782341604485,-12.660895079808,123.628713552721)) ;
#41958=CARTESIAN_POINT('Ctrl Pts',(-18.1782290022397,-12.6608937159384,
123.628684274628)) ;
#41959=CARTESIAN_POINT('Ctrl Pts',(-18.178226431882,-12.6608930362462,123.628669683709)) ;
#41960=CARTESIAN_POINT('Ctrl Pts',(-18.1782213085765,-12.6608916813255,
123.628640597674)) ;
#41961=CARTESIAN_POINT('Ctrl Pts',(-18.1782187556213,-12.6608910060961,
123.628626102536)) ;
#41962=CARTESIAN_POINT('Ctrl Pts',(-18.17821366697,-12.660889660064,123.628597207265)) ;
#41963=CARTESIAN_POINT('Ctrl Pts',(-18.1782111312665,-12.6608889892603,
123.628582807111)) ;
#41964=CARTESIAN_POINT('Ctrl Pts',(-18.1782060769312,-12.6608876520327,
123.628554100802)) ;
#41965=CARTESIAN_POINT('Ctrl Pts',(-18.1782035583615,-12.6608869856262,
123.62853979502)) ;
#41966=CARTESIAN_POINT('Ctrl Pts',(-18.1781985381848,-12.6608856571668,
123.628511276895)) ;
#41967=CARTESIAN_POINT('Ctrl Pts',(-18.1781960365599,-12.6608849951101,
123.628497064469)) ;
#41968=CARTESIAN_POINT('Ctrl Pts',(-18.1781910501952,-12.6608836753326,
123.628468732673)) ;
#41969=CARTESIAN_POINT('Ctrl Pts',(-18.1781885653864,-12.6608830175943,
123.628454612929)) ;
#41970=CARTESIAN_POINT('Ctrl Pts',(-18.1781836124378,-12.660881706399,123.628426465325)) ;
#41971=CARTESIAN_POINT('Ctrl Pts',(-18.1781811443734,-12.6608810529627,
123.628412437911)) ;
#41972=CARTESIAN_POINT('Ctrl Pts',(-18.1781762247696,-12.6608797503358,
123.628384474206)) ;
#41973=CARTESIAN_POINT('Ctrl Pts',(-18.178173773246,-12.6608791011502,123.628370538021)) ;
#41974=CARTESIAN_POINT('Ctrl Pts',(-18.1781688866781,-12.660877807015,123.628342756566)) ;
#41975=CARTESIAN_POINT('Ctrl Pts',(-18.1781664515469,-12.6608771620433,
123.628328910821)) ;
#41976=CARTESIAN_POINT('Ctrl Pts',(-18.178161597596,-12.6608758762939,123.628301309345)) ;
#41977=CARTESIAN_POINT('Ctrl Pts',(-18.1781591787926,-12.6608752355213,
123.628287553725)) ;
#41978=CARTESIAN_POINT('Ctrl Pts',(-18.178154357366,-12.6608739581381,123.628260131806)) ;
#41979=CARTESIAN_POINT('Ctrl Pts',(-18.1781519547067,-12.6608733215186,
123.62824646532)) ;
#41980=CARTESIAN_POINT('Ctrl Pts',(-18.1781471654095,-12.6608720524017,
123.628219220818)) ;
#41981=CARTESIAN_POINT('Ctrl Pts',(-18.1781447788043,-12.6608714199138,
123.628205643005)) ;
#41982=CARTESIAN_POINT('Ctrl Pts',(-18.1781400214645,-12.6608701590224,
123.628178575045)) ;
#41983=CARTESIAN_POINT('Ctrl Pts',(-18.1781376507604,-12.6608695306279,
123.628165085087)) ;
#41984=CARTESIAN_POINT('Ctrl Pts',(-18.1781329251248,-12.6608682778998,
123.62813819233)) ;
#41985=CARTESIAN_POINT('Ctrl Pts',(-18.1781305701799,-12.6608676535634,
123.62812478947)) ;
#41986=CARTESIAN_POINT('Ctrl Pts',(-18.1781258759642,-12.6608664089277,
123.628098070399)) ;
#41987=CARTESIAN_POINT('Ctrl Pts',(-18.1781235366593,-12.6608657886201,
123.628084754009)) ;
#41988=CARTESIAN_POINT('Ctrl Pts',(-18.1781188735632,-12.6608645520018,
123.628058207013)) ;
#41989=CARTESIAN_POINT('Ctrl Pts',(-18.1781165498001,-12.6608639356993,
123.628044976583)) ;
#41990=CARTESIAN_POINT('Ctrl Pts',(-18.1781119176568,-12.6608627070587,
123.628018600811)) ;
#41991=CARTESIAN_POINT('Ctrl Pts',(-18.178109609283,-12.6608620947231,123.628005455521)) ;
#41992=CARTESIAN_POINT('Ctrl Pts',(-18.178105007843,-12.6608608739985,123.627979249649)) ;
#41993=CARTESIAN_POINT('Ctrl Pts',(-18.1781027147224,-12.6608602655959,
123.627966188772)) ;
#41994=CARTESIAN_POINT('Ctrl Pts',(-18.1780981436022,-12.6608590526899,
123.627940150711)) ;
#41995=CARTESIAN_POINT('Ctrl Pts',(-18.1780958656748,-12.6608584482065,
123.627927173953)) ;
#41996=CARTESIAN_POINT('Ctrl Pts',(-18.1780913248799,-12.660857243125,123.627901303827)) ;
#41997=CARTESIAN_POINT('Ctrl Pts',(-18.1780890619314,-12.6608566425061,
123.627888410014)) ;
#41998=CARTESIAN_POINT('Ctrl Pts',(-18.1780845509411,-12.6608554451151,
123.627862704951)) ;
#41999=CARTESIAN_POINT('Ctrl Pts',(-18.178082302945,-12.6608548483559,123.627849893976)) ;
#42000=CARTESIAN_POINT('Ctrl Pts',(-18.1780778217311,-12.6608536586521,
123.627824353905)) ;
#42001=CARTESIAN_POINT('Ctrl Pts',(-18.1780755885098,-12.6608530657074,
123.627811624803)) ;
#42002=CARTESIAN_POINT('Ctrl Pts',(-18.1780711367808,-12.6608518836177,
123.627786248154)) ;
#42003=CARTESIAN_POINT('Ctrl Pts',(-18.1780689182151,-12.660851294458,123.62777360029)) ;
#42004=CARTESIAN_POINT('Ctrl Pts',(-18.1780644956893,-12.6608501199116,
123.627748385544)) ;
#42005=CARTESIAN_POINT('Ctrl Pts',(-18.1780622916852,-12.6608495345139,
123.627735818426)) ;
#42006=CARTESIAN_POINT('Ctrl Pts',(-18.1780578980972,-12.6608483674444,
123.627710764159)) ;
#42007=CARTESIAN_POINT('Ctrl Pts',(-18.178055708567,-12.6608477857875,123.62769827733)) ;
#42008=CARTESIAN_POINT('Ctrl Pts',(-18.1780513438163,-12.6608466261721,
123.627673383054)) ;
#42009=CARTESIAN_POINT('Ctrl Pts',(-18.1780491685949,-12.6608460482141,
123.627660975616)) ;
#42010=CARTESIAN_POINT('Ctrl Pts',(-18.1780448323125,-12.6608448959588,
123.627636239312)) ;
#42011=CARTESIAN_POINT('Ctrl Pts',(-18.178042671332,-12.6608443216836,123.62762391092)) ;
#42012=CARTESIAN_POINT('Ctrl Pts',(-18.1770321734612,-12.660575760822,123.621858511994)) ;
#42013=CARTESIAN_POINT('Ctrl Pts',(-18.1760641746186,-12.6603075266588,
123.61609846262)) ;
#42014=CARTESIAN_POINT('Ctrl Pts',(-18.1729267270412,-12.6593992151072,
123.596593701384)) ;
#42015=CARTESIAN_POINT('Ctrl Pts',(-18.1709464297291,-12.6587578392535,
123.582819672376)) ;
#42016=CARTESIAN_POINT('Ctrl Pts',(-18.1654378014235,-12.6567363410127,
123.539365052685)) ;
#42017=CARTESIAN_POINT('Ctrl Pts',(-18.1627437207223,-12.6553542485752,
123.509589316382)) ;
#42018=CARTESIAN_POINT('Ctrl Pts',(-18.1600304775297,-12.6530499804726,
123.459736882306)) ;
#42019=CARTESIAN_POINT('Ctrl Pts',(-18.1594227751612,-12.6521265907355,
123.439704698591)) ;
#42020=CARTESIAN_POINT('Ctrl Pts',(-18.1592419010343,-12.6508028087505,
123.410911485108)) ;
#42021=CARTESIAN_POINT('Ctrl Pts',(-18.1592788870681,-12.6504007243802,
123.402156113199)) ;
#42022=CARTESIAN_POINT('Ctrl Pts',(-18.1594169997785,-12.6499705901163,
123.392780859932)) ;
#42023=CARTESIAN_POINT('Ctrl Pts',(-18.1594266105133,-12.6499421022534,
123.39215989285)) ;
#42024=CARTESIAN_POINT('Ctrl Pts',(-18.159457427645,-12.649854958374,123.390260236952)) ;
#42025=CARTESIAN_POINT('Ctrl Pts',(-18.1594801335978,-12.6497963097356,
123.388981573)) ;
#42026=CARTESIAN_POINT('Ctrl Pts',(-18.1595662437714,-12.649591616403,123.384518223812)) ;
#42027=CARTESIAN_POINT('Ctrl Pts',(-18.1596398587758,-12.6494456224759,
123.381333745682)) ;
#42028=CARTESIAN_POINT('Ctrl Pts',(-18.1597277541691,-12.6492961005507,
123.378071304311)) ;
#42029=CARTESIAN_POINT('Ctrl Pts',(-18.1597298704669,-12.6492925129913,
123.37799302622)) ;
#42030=CARTESIAN_POINT('Ctrl Pts',(-18.1597339708883,-12.6492855860819,
123.377841884647)) ;
#42031=CARTESIAN_POINT('Ctrl Pts',(-18.1597359540301,-12.6492822467258,
123.377769021115)) ;
#42032=CARTESIAN_POINT('Ctrl Pts',(-18.159739795121,-12.6492757996023,123.377628346238)) ;
#42033=CARTESIAN_POINT('Ctrl Pts',(-18.1597416522171,-12.6492726918304,
123.377560534866)) ;
#42034=CARTESIAN_POINT('Ctrl Pts',(-18.1599289759344,-12.648960145286,123.370740745807)) ;
#42035=CARTESIAN_POINT('Ctrl Pts',(-18.1601691619896,-12.6486509823074,
123.363990370268)) ;
#42036=CARTESIAN_POINT('Ctrl Pts',(-18.160973701865,-12.6478082050313,123.345579572654)) ;
#42037=CARTESIAN_POINT('Ctrl Pts',(-18.1616467078773,-12.6472751536992,
123.333924563584)) ;
#42038=CARTESIAN_POINT('Ctrl Pts',(-18.1635496623423,-12.6460635503773,
123.307425231623)) ;
#42039=CARTESIAN_POINT('Ctrl Pts',(-18.1648818716474,-12.6453855231187,
123.292590016733)) ;
#42040=CARTESIAN_POINT('Ctrl Pts',(-18.171704422704,-12.6424917283109,123.229328964051)) ;
#42041=CARTESIAN_POINT('Ctrl Pts',(-18.1797590550159,-12.6402830294978,
123.181223074307)) ;
#42042=CARTESIAN_POINT('Ctrl Pts',(-18.1973603972008,-12.6366730949746,
123.10409276087)) ;
#42043=CARTESIAN_POINT('Ctrl Pts',(-18.2051966899157,-12.6352846790454,
123.074731348285)) ;
#42044=CARTESIAN_POINT('Ctrl Pts',(-18.2251424619583,-12.6321693056675,
123.009621247692)) ;
#42045=CARTESIAN_POINT('Ctrl Pts',(-18.2378167241948,-12.6304432995783,
122.974076317143)) ;
#42046=CARTESIAN_POINT('Ctrl Pts',(-18.2592454496299,-12.6278460495146,
122.921612747141)) ;
#42047=CARTESIAN_POINT('Ctrl Pts',(-18.2668103838277,-12.626977019358,122.904231712306)) ;
#42048=CARTESIAN_POINT('Ctrl Pts',(-18.2749152773553,-12.626090811094,122.886710172793)) ;
#42049=CARTESIAN_POINT('Ctrl Pts',(-18.2750631056821,-12.6260746616098,
122.886390944318)) ;
#42050=CARTESIAN_POINT('Ctrl Pts',(-18.2753392722442,-12.6260445186976,
122.885795234971)) ;
#42051=CARTESIAN_POINT('Ctrl Pts',(-18.2754675768948,-12.626030525351,122.885518738532)) ;
#42052=CARTESIAN_POINT('Ctrl Pts',(-18.2757073049846,-12.6260043999089,
122.885002619174)) ;
#42053=CARTESIAN_POINT('Ctrl Pts',(-18.2758187033151,-12.6259922678738,
122.884762984572)) ;
#42054=CARTESIAN_POINT('Ctrl Pts',(-18.2760268735667,-12.625969611822,122.884315550214)) ;
#42055=CARTESIAN_POINT('Ctrl Pts',(-18.2761236266551,-12.6259590878539,
122.884107741756)) ;
#42056=CARTESIAN_POINT('Ctrl Pts',(-18.27630445493,-12.625939430258,122.88371963376)) ;
#42057=CARTESIAN_POINT('Ctrl Pts',(-18.276388516012,-12.6259302966649,122.883539327646)) ;
#42058=CARTESIAN_POINT('Ctrl Pts',(-18.2765456444916,-12.6259132325251,
122.88320250621)) ;
#42059=CARTESIAN_POINT('Ctrl Pts',(-18.2766187013132,-12.6259053020029,
122.883045985911)) ;
#42060=CARTESIAN_POINT('Ctrl Pts',(-18.2767552776296,-12.6258904826902,
122.8827535367)) ;
#42061=CARTESIAN_POINT('Ctrl Pts',(-18.2768187891567,-12.6258835939199,
122.882617604078)) ;
#42062=CARTESIAN_POINT('Ctrl Pts',(-18.2770372670083,-12.6258599056609,
122.882150219157)) ;
#42063=CARTESIAN_POINT('Ctrl Pts',(-18.2771923543361,-12.6258431058732,
122.881818823575)) ;
#42064=CARTESIAN_POINT('Ctrl Pts',(-18.2774970413321,-12.6258101309488,
122.881168502537)) ;
#42065=CARTESIAN_POINT('Ctrl Pts',(-18.2776466303692,-12.6257939558394,
122.880849572104)) ;
#42066=CARTESIAN_POINT('Ctrl Pts',(-18.2779405767708,-12.6257621992555,
122.880223553862)) ;
#42067=CARTESIAN_POINT('Ctrl Pts',(-18.2780849243952,-12.6257466178078,
122.879916461522)) ;
#42068=CARTESIAN_POINT('Ctrl Pts',(-18.2783686310298,-12.6257160192645,
122.879313527701)) ;
#42069=CARTESIAN_POINT('Ctrl Pts',(-18.2785079811195,-12.6257010021941,
122.879017682069)) ;
#42070=CARTESIAN_POINT('Ctrl Pts',(-18.2787819233553,-12.6256715047635,
122.878436683655)) ;
#42071=CARTESIAN_POINT('Ctrl Pts',(-18.2789165073475,-12.6256570244245,
122.878151527019)) ;
#42072=CARTESIAN_POINT('Ctrl Pts',(-18.2791811363385,-12.6256285743533,
122.877591380183)) ;
#42073=CARTESIAN_POINT('Ctrl Pts',(-18.2793111738436,-12.6256146046422,
122.877316386472)) ;
#42074=CARTESIAN_POINT('Ctrl Pts',(-18.2795669175777,-12.625587151181,122.876776068955)) ;
#42075=CARTESIAN_POINT('Ctrl Pts',(-18.2796926169244,-12.6255736674509,
122.876510741928)) ;
#42076=CARTESIAN_POINT('Ctrl Pts',(-18.2799398813877,-12.6255471626783,
122.875989289337)) ;
#42077=CARTESIAN_POINT('Ctrl Pts',(-18.2800614401804,-12.6255341416544,
122.875733160809)) ;
#42078=CARTESIAN_POINT('Ctrl Pts',(-18.2803006103763,-12.6255085403208,
122.875229663333)) ;
#42079=CARTESIAN_POINT('Ctrl Pts',(-18.2804182159959,-12.6254959600249,
122.874982291586)) ;
#42080=CARTESIAN_POINT('Ctrl Pts',(-18.2806496571411,-12.6254712193825,
122.874495890458)) ;
#42081=CARTESIAN_POINT('Ctrl Pts',(-18.2807634873175,-12.6254590590515,
122.87425685855)) ;
#42082=CARTESIAN_POINT('Ctrl Pts',(-18.2809875457193,-12.6254351387228,
122.873786743287)) ;
#42083=CARTESIAN_POINT('Ctrl Pts',(-18.2810977690084,-12.6254233787403,
122.873555657615)) ;
#42084=CARTESIAN_POINT('Ctrl Pts',(-18.287541854932,-12.6247362749384,122.860056157743)) ;
#42085=CARTESIAN_POINT('Ctrl Pts',(-18.2941092361412,-12.6240603376009,
122.84690052324)) ;
#42086=CARTESIAN_POINT('Ctrl Pts',(-18.307827305343,-12.6226942650302,122.820592684519)) ;
#42087=CARTESIAN_POINT('Ctrl Pts',(-18.3149852471551,-12.6220042033772,
122.807446932521)) ;
#42088=CARTESIAN_POINT('Ctrl Pts',(-18.3326564680827,-12.6203511428849,
122.776336898223)) ;
#42089=CARTESIAN_POINT('Ctrl Pts',(-18.3433856903454,-12.6193862658968,
122.758500518981)) ;
#42090=CARTESIAN_POINT('Ctrl Pts',(-18.3737759357875,-12.6167585607486,
122.710722371413)) ;
#42091=CARTESIAN_POINT('Ctrl Pts',(-18.3942867137277,-12.6150971782096,
122.681343962543)) ;
#42092=CARTESIAN_POINT('Ctrl Pts',(-18.4210320278047,-12.6130671201886,
122.646341214415)) ;
#42093=CARTESIAN_POINT('Ctrl Pts',(-18.4260979258935,-12.612688079985,122.639845369389)) ;
#42094=CARTESIAN_POINT('Ctrl Pts',(-18.4342773663973,-12.6120846646705,
122.629568249464)) ;
#42095=CARTESIAN_POINT('Ctrl Pts',(-18.4373495517714,-12.6118599016483,
122.625754394585)) ;
#42096=CARTESIAN_POINT('Ctrl Pts',(-18.4428707377722,-12.611459276532,122.618982169492)) ;
#42097=CARTESIAN_POINT('Ctrl Pts',(-18.4453111066451,-12.6112833318287,
122.616016848548)) ;
#42098=CARTESIAN_POINT('Ctrl Pts',(-18.4511895629447,-12.610862188603,122.608940583543)) ;
#42099=CARTESIAN_POINT('Ctrl Pts',(-18.4546405013989,-12.6106171233224,
122.604840406996)) ;
#42100=CARTESIAN_POINT('Ctrl Pts',(-18.4619338508133,-12.610103649682,122.596287189935)) ;
#42101=CARTESIAN_POINT('Ctrl Pts',(-18.4657815404245,-12.6098353009703,
122.591838818415)) ;
#42102=CARTESIAN_POINT('Ctrl Pts',(-18.4760797110779,-12.6091236568087,
122.580101407085)) ;
#42103=CARTESIAN_POINT('Ctrl Pts',(-18.4825841873557,-12.6086809075479,
122.572860257337)) ;
#42104=CARTESIAN_POINT('Ctrl Pts',(-18.5038720921853,-12.6072525757861,
122.54971102731)) ;
#42105=CARTESIAN_POINT('Ctrl Pts',(-18.5189856960247,-12.6062701096431,
122.534111983459)) ;
#42106=CARTESIAN_POINT('Ctrl Pts',(-18.5552211526755,-12.6039773765129,
122.498612098717)) ;
#42107=CARTESIAN_POINT('Ctrl Pts',(-18.5766446136048,-12.6026687430557,
122.479037407174)) ;
#42108=CARTESIAN_POINT('Ctrl Pts',(-18.606038714761,-12.6009154462183,122.454000138348)) ;
#42109=CARTESIAN_POINT('Ctrl Pts',(-18.613419321866,-12.6004784952232,122.44785880551)) ;
#42110=CARTESIAN_POINT('Ctrl Pts',(-18.6244298596054,-12.5998307587984,
122.438909700844)) ;
#42111=CARTESIAN_POINT('Ctrl Pts',(-18.6280056131143,-12.5996210589038,
122.436035955186)) ;
#42112=CARTESIAN_POINT('Ctrl Pts',(-18.6344379685612,-12.5992450517586,
122.4309244517)) ;
#42113=CARTESIAN_POINT('Ctrl Pts',(-18.6372886534297,-12.5990788369211,
122.428679322317)) ;
#42114=CARTESIAN_POINT('Ctrl Pts',(-18.6432681697942,-12.5987310973486,
122.424012044864)) ;
#42115=CARTESIAN_POINT('Ctrl Pts',(-18.6463988080334,-12.5985495493898,
122.42159227582)) ;
#42116=CARTESIAN_POINT('Ctrl Pts',(-18.6495510876864,-12.5983672760887,
122.419179601347)) ;
#42117=CARTESIAN_POINT('Ctrl Pts',(-18.649561298306,-12.5983666856887,122.419171786649)) ;
#42118=CARTESIAN_POINT('Ctrl Pts',(-18.6495817299632,-12.5983655042975,
122.41915614978)) ;
#42119=CARTESIAN_POINT('Ctrl Pts',(-18.6495919552914,-12.5983649130582,
122.419148324325)) ;
#42120=CARTESIAN_POINT('Ctrl Pts',(-18.6496124246755,-12.5983637295078,
122.419132659585)) ;
#42121=CARTESIAN_POINT('Ctrl Pts',(-18.6496226676214,-12.598363137261,122.41912482115)) ;
#42122=CARTESIAN_POINT('Ctrl Pts',(-18.6496431684722,-12.5983619519136,
122.419109133335)) ;
#42123=CARTESIAN_POINT('Ctrl Pts',(-18.6496534279312,-12.5983613587232,
122.419101282767)) ;
#42124=CARTESIAN_POINT('Ctrl Pts',(-18.649673963113,-12.5983601714132,122.419085569691)) ;
#42125=CARTESIAN_POINT('Ctrl Pts',(-18.6496842391464,-12.5983595772757,
122.419077706946)) ;
#42126=CARTESIAN_POINT('Ctrl Pts',(-18.649704810932,-12.5983583878719,122.419061966874)) ;
#42127=CARTESIAN_POINT('Ctrl Pts',(-18.6497151053305,-12.5983577926839,
122.419054090584)) ;
#42128=CARTESIAN_POINT('Ctrl Pts',(-18.6497357091842,-12.5983566014486,
122.419038326992)) ;
#42129=CARTESIAN_POINT('Ctrl Pts',(-18.6497460203609,-12.5983560053018,
122.419030438374)) ;
#42130=CARTESIAN_POINT('Ctrl Pts',(-18.6497666613134,-12.5983548119443,
122.419014647418)) ;
#42131=CARTESIAN_POINT('Ctrl Pts',(-18.6497769905191,-12.5983542147666,
122.419006745518)) ;
#42132=CARTESIAN_POINT('Ctrl Pts',(-18.6497976667056,-12.5983530193947,
122.41899092863)) ;
#42133=CARTESIAN_POINT('Ctrl Pts',(-18.6498080139681,-12.5983524211844,
122.418983013428)) ;
#42134=CARTESIAN_POINT('Ctrl Pts',(-18.6498287254617,-12.5983512237942,
122.418967170558)) ;
#42135=CARTESIAN_POINT('Ctrl Pts',(-18.6498390902779,-12.5983506245805,
122.418959242442)) ;
#42136=CARTESIAN_POINT('Ctrl Pts',(-18.6498598401011,-12.5983494249973,
122.418943371282)) ;
#42137=CARTESIAN_POINT('Ctrl Pts',(-18.6498702238716,-12.5983488246992,
122.418935429184)) ;
#42138=CARTESIAN_POINT('Ctrl Pts',(-18.6498910091217,-12.5983476230909,
122.41891953196)) ;
#42139=CARTESIAN_POINT('Ctrl Pts',(-18.6499014111075,-12.5983470217514,
122.418911576448)) ;
#42140=CARTESIAN_POINT('Ctrl Pts',(-18.6499222350237,-12.5983458179308,
122.418895650689)) ;
#42141=CARTESIAN_POINT('Ctrl Pts',(-18.6499326563795,-12.598345215483,122.418887680882)) ;
#42142=CARTESIAN_POINT('Ctrl Pts',(-18.6499535161522,-12.5983440096128,
122.418871728741)) ;
#42143=CARTESIAN_POINT('Ctrl Pts',(-18.6499639557221,-12.5983434061237,
122.418863745526)) ;
#42144=CARTESIAN_POINT('Ctrl Pts',(-18.6499848560941,-12.5983421979297,
122.418847763382)) ;
#42145=CARTESIAN_POINT('Ctrl Pts',(-18.6499953156951,-12.5983415932943,
122.418839765372)) ;
#42146=CARTESIAN_POINT('Ctrl Pts',(-18.6500162525731,-12.5983403830134,
122.418823756361)) ;
#42147=CARTESIAN_POINT('Ctrl Pts',(-18.6500267310911,-12.5983397772962,
122.418815744412)) ;
#42148=CARTESIAN_POINT('Ctrl Pts',(-18.6500477077048,-12.5983385647417,
122.41879970607)) ;
#42149=CARTESIAN_POINT('Ctrl Pts',(-18.650058205517,-12.5983379579209,122.418791679895)) ;
#42150=CARTESIAN_POINT('Ctrl Pts',(-18.6500792232105,-12.5983367430153,
122.418775611201)) ;
#42151=CARTESIAN_POINT('Ctrl Pts',(-18.6500897417746,-12.5983361350067,
122.418767569689)) ;
#42152=CARTESIAN_POINT('Ctrl Pts',(-18.6501107971926,-12.5983349179441,
122.418751473213)) ;
#42153=CARTESIAN_POINT('Ctrl Pts',(-18.6501213353978,-12.598334308812,122.418743417217)) ;
#42154=CARTESIAN_POINT('Ctrl Pts',(-18.6501424318548,-12.598333089401,122.418727290432)) ;
#42155=CARTESIAN_POINT('Ctrl Pts',(-18.6501529901725,-12.5983324791182,
122.418719219593)) ;
#42156=CARTESIAN_POINT('Ctrl Pts',(-18.6501741276519,-12.5983312573597,
122.418703062517)) ;
#42157=CARTESIAN_POINT('Ctrl Pts',(-18.650184706356,-12.5983306459105,122.41869497663)) ;
#42158=CARTESIAN_POINT('Ctrl Pts',(-18.6502058856374,-12.5983294217598,
122.418678788674)) ;
#42159=CARTESIAN_POINT('Ctrl Pts',(-18.6502164853907,-12.5983288091059,
122.418670687235)) ;
#42160=CARTESIAN_POINT('Ctrl Pts',(-18.6502377059149,-12.5983275825953,
122.418654468832)) ;
#42161=CARTESIAN_POINT('Ctrl Pts',(-18.6502483268186,-12.598326968731,122.418646351767)) ;
#42162=CARTESIAN_POINT('Ctrl Pts',(-18.6502695889701,-12.5983257398385,
122.418630102629)) ;
#42163=CARTESIAN_POINT('Ctrl Pts',(-18.6502802309545,-12.5983251247678,
122.418621969995)) ;
#42164=CARTESIAN_POINT('Ctrl Pts',(-18.6503015350622,-12.5983238934745,
122.418605689878)) ;
#42165=CARTESIAN_POINT('Ctrl Pts',(-18.650312197665,-12.5983232772243,122.41859754203)) ;
#42166=CARTESIAN_POINT('Ctrl Pts',(-18.6503335468897,-12.5983220433477,
122.418581228525)) ;
#42167=CARTESIAN_POINT('Ctrl Pts',(-18.6503442316723,-12.5983214258277,
122.418573064274)) ;
#42168=CARTESIAN_POINT('Ctrl Pts',(-18.6503656234731,-12.5983201895148,
122.418556719329)) ;
#42169=CARTESIAN_POINT('Ctrl Pts',(-18.6503763303433,-12.5983195707305,
122.418548538749)) ;
#42170=CARTESIAN_POINT('Ctrl Pts',(-18.6503977654965,-12.5983183319365,
122.418532161777)) ;
#42171=CARTESIAN_POINT('Ctrl Pts',(-18.6504084943738,-12.5983177118926,
122.418523964932)) ;
#42172=CARTESIAN_POINT('Ctrl Pts',(-18.6504299741154,-12.5983164705463,
122.418507554996)) ;
#42173=CARTESIAN_POINT('Ctrl Pts',(-18.6504407253918,-12.5983158492202,
122.418499341591)) ;
#42174=CARTESIAN_POINT('Ctrl Pts',(-18.6504622492835,-12.5983146053472,
122.418482899032)) ;
#42175=CARTESIAN_POINT('Ctrl Pts',(-18.6504730226356,-12.5983139827576,
122.418474669317)) ;
#42176=CARTESIAN_POINT('Ctrl Pts',(-18.6504945928455,-12.5983127362326,
122.418458192486)) ;
#42177=CARTESIAN_POINT('Ctrl Pts',(-18.6505053891011,-12.5983121123319,
122.418449945831)) ;
#42178=CARTESIAN_POINT('Ctrl Pts',(-18.6505270049518,-12.5983108631942,
122.418433435253)) ;
#42179=CARTESIAN_POINT('Ctrl Pts',(-18.6505378244112,-12.598310237965,122.418425171433)) ;
#42180=CARTESIAN_POINT('Ctrl Pts',(-18.6505594853712,-12.5983089862455,
122.41840862752)) ;
#42181=CARTESIAN_POINT('Ctrl Pts',(-18.6505703273927,-12.5983083597251,
122.418400347029)) ;
#42182=CARTESIAN_POINT('Ctrl Pts',(-18.6505920369108,-12.5983071052247,
122.418383767155)) ;
#42183=CARTESIAN_POINT('Ctrl Pts',(-18.6506029029903,-12.5983064773266,
122.418375468854)) ;
#42184=CARTESIAN_POINT('Ctrl Pts',(-18.6506246587612,-12.5983052201786,
122.418358854785)) ;
#42185=CARTESIAN_POINT('Ctrl Pts',(-18.6506355488577,-12.5983045909054,
122.418350538709)) ;
#42186=CARTESIAN_POINT('Ctrl Pts',(-18.650657350895,-12.5983033311092,122.418333890444)) ;
#42187=CARTESIAN_POINT('Ctrl Pts',(-18.6506682642414,-12.5983027005051,
122.418325557182)) ;
#42188=CARTESIAN_POINT('Ctrl Pts',(-18.6506901160332,-12.5983014378594,
122.418308872064)) ;
#42189=CARTESIAN_POINT('Ctrl Pts',(-18.6507010539031,-12.5983008058511,
122.418300520648)) ;
#42190=CARTESIAN_POINT('Ctrl Pts',(-18.6507229529526,-12.5982995405003,
122.41828380059)) ;
#42191=CARTESIAN_POINT('Ctrl Pts',(-18.6507339146566,-12.5982989071275,
122.418275431549)) ;
#42192=CARTESIAN_POINT('Ctrl Pts',(-18.6507558643608,-12.5982976388755,
122.418258673967)) ;
#42193=CARTESIAN_POINT('Ctrl Pts',(-18.650766851228,-12.5982970040617,122.418250286291)) ;
#42194=CARTESIAN_POINT('Ctrl Pts',(-18.6507888495272,-12.5982957330276,
122.418233492763)) ;
#42195=CARTESIAN_POINT('Ctrl Pts',(-18.6507998614117,-12.5982950967812,
122.418225086567)) ;
#42196=CARTESIAN_POINT('Ctrl Pts',(-18.6508219084853,-12.5982938229549,
122.418208256965)) ;
#42197=CARTESIAN_POINT('Ctrl Pts',(-18.6508329445605,-12.5982931853238,
122.418199832884)) ;
#42198=CARTESIAN_POINT('Ctrl Pts',(-18.6508550450937,-12.5982919084347,
122.41818296364)) ;
#42199=CARTESIAN_POINT('Ctrl Pts',(-18.6508661076924,-12.5982912692842,
122.418174519897)) ;
#42200=CARTESIAN_POINT('Ctrl Pts',(-18.6508882565901,-12.5982899896269,
122.418157614906)) ;
#42201=CARTESIAN_POINT('Ctrl Pts',(-18.6508993445044,-12.5982893490269,
122.418149152427)) ;
#42202=CARTESIAN_POINT('Ctrl Pts',(-18.6509215447641,-12.5982880664284,
122.418132209411)) ;
#42203=CARTESIAN_POINT('Ctrl Pts',(-18.6509326578662,-12.5982874243863,
122.418123728298)) ;
#42204=CARTESIAN_POINT('Ctrl Pts',(-18.6509549114128,-12.5982861387356,
122.418106745795)) ;
#42205=CARTESIAN_POINT('Ctrl Pts',(-18.6509660506469,-12.598285495197,122.418098245331)) ;
#42206=CARTESIAN_POINT('Ctrl Pts',(-18.6509883572059,-12.5982842065101,
122.41808122356)) ;
#42207=CARTESIAN_POINT('Ctrl Pts',(-18.650999523427,-12.5982835614257,122.418072703097)) ;
#42208=CARTESIAN_POINT('Ctrl Pts',(-18.6510218813851,-12.598282269796,122.418055643296)) ;
#42209=CARTESIAN_POINT('Ctrl Pts',(-18.6510330739266,-12.5982816232044,
122.418047103347)) ;
#42210=CARTESIAN_POINT('Ctrl Pts',(-18.6510554860335,-12.5982803284733,
122.418030003427)) ;
#42211=CARTESIAN_POINT('Ctrl Pts',(-18.6510667055843,-12.5982796803347,
122.41802144347)) ;
#42212=CARTESIAN_POINT('Ctrl Pts',(-18.6510891711257,-12.5982783825436,
122.418004303985)) ;
#42213=CARTESIAN_POINT('Ctrl Pts',(-18.6511004175758,-12.5982777328646,
122.417995724108)) ;
#42214=CARTESIAN_POINT('Ctrl Pts',(-18.6511229378347,-12.5982764319395,
122.417978544087)) ;
#42215=CARTESIAN_POINT('Ctrl Pts',(-18.6511342115148,-12.5982757807011,
122.417969944043)) ;
#42216=CARTESIAN_POINT('Ctrl Pts',(-18.6511567874916,-12.5982744765845,
122.417952722732)) ;
#42217=CARTESIAN_POINT('Ctrl Pts',(-18.6511680892582,-12.5982738237372,
122.417944101871)) ;
#42218=CARTESIAN_POINT('Ctrl Pts',(-18.6511907192162,-12.5982725165297,
122.417926840603)) ;
#42219=CARTESIAN_POINT('Ctrl Pts',(-18.6512020482939,-12.5982718621184,
122.417918199522)) ;
#42220=CARTESIAN_POINT('Ctrl Pts',(-18.6512247359857,-12.5982705516034,
122.417900895445)) ;
#42221=CARTESIAN_POINT('Ctrl Pts',(-18.651236093824,-12.5982698955445,122.417892233042)) ;
#42222=CARTESIAN_POINT('Ctrl Pts',(-18.6512588361687,-12.5982685819001,
122.417874888513)) ;
#42223=CARTESIAN_POINT('Ctrl Pts',(-18.6512702217627,-12.5982679242518,
122.41786620556)) ;
#42224=CARTESIAN_POINT('Ctrl Pts',(-18.6512930227638,-12.5982666072469,
122.417848817536)) ;
#42225=CARTESIAN_POINT('Ctrl Pts',(-18.6513044373569,-12.5982659479374,
122.417840113088)) ;
#42226=CARTESIAN_POINT('Ctrl Pts',(-18.6513272951699,-12.5982646276789,
122.417822682985)) ;
#42227=CARTESIAN_POINT('Ctrl Pts',(-18.6513387386052,-12.5982639667175,
122.417813957168)) ;
#42228=CARTESIAN_POINT('Ctrl Pts',(-18.6513616545633,-12.5982626431285,
122.417796483978)) ;
#42229=CARTESIAN_POINT('Ctrl Pts',(-18.6513731270605,-12.5982619805025,
122.417787736627)) ;
#42230=CARTESIAN_POINT('Ctrl Pts',(-18.65139610204,-12.5982606535327,122.417770219693)) ;
#42231=CARTESIAN_POINT('Ctrl Pts',(-18.6514076041197,-12.5982599892121,
122.417761450417)) ;
#42232=CARTESIAN_POINT('Ctrl Pts',(-18.6514306381346,-12.5982586588609,
122.417743889736)) ;
#42233=CARTESIAN_POINT('Ctrl Pts',(-18.6514421700625,-12.5982579928306,
122.417735098338)) ;
#42234=CARTESIAN_POINT('Ctrl Pts',(-18.6514652635442,-12.5982566590731,
122.417717493591)) ;
#42235=CARTESIAN_POINT('Ctrl Pts',(-18.6514768254377,-12.5982559913264,
122.417708679985)) ;
#42236=CARTESIAN_POINT('Ctrl Pts',(-18.6514999788699,-12.5982546541351,
122.417691030814)) ;
#42237=CARTESIAN_POINT('Ctrl Pts',(-18.6515115706694,-12.5982539846755,
122.417682195051)) ;
#42238=CARTESIAN_POINT('Ctrl Pts',(-18.6515347860698,-12.598252643934,122.417664499928)) ;
#42239=CARTESIAN_POINT('Ctrl Pts',(-18.6515464088379,-12.5982519727003,
122.417655641203)) ;
#42240=CARTESIAN_POINT('Ctrl Pts',(-18.651569684921,-12.5982506284831,122.417637901117)) ;
#42241=CARTESIAN_POINT('Ctrl Pts',(-18.6515813386761,-12.5982499554743,
122.417629019421)) ;
#42242=CARTESIAN_POINT('Ctrl Pts',(-18.6516046756774,-12.5982486077681,
122.417611234203)) ;
#42243=CARTESIAN_POINT('Ctrl Pts',(-18.6516163598529,-12.598247933017,122.417602329973)) ;
#42244=CARTESIAN_POINT('Ctrl Pts',(-18.6516397613945,-12.5982465816127,
122.417584496873)) ;
#42245=CARTESIAN_POINT('Ctrl Pts',(-18.6516514776689,-12.5982459050226,
122.417575568835)) ;
#42246=CARTESIAN_POINT('Ctrl Pts',(-18.6516749400284,-12.5982445501355,
122.4175576907)) ;
#42247=CARTESIAN_POINT('Ctrl Pts',(-18.6516866871725,-12.5982438717775,
122.417548739796)) ;
#42248=CARTESIAN_POINT('Ctrl Pts',(-18.6517102155907,-12.5982425131052,
122.417530812642)) ;
#42249=CARTESIAN_POINT('Ctrl Pts',(-18.651721995559,-12.5982418328664,122.417521837389)) ;
#42250=CARTESIAN_POINT('Ctrl Pts',(-18.6517455858715,-12.5982404706496,
122.417503864401)) ;
#42251=CARTESIAN_POINT('Ctrl Pts',(-18.6517573975375,-12.5982397885953,
122.417494865661)) ;
#42252=CARTESIAN_POINT('Ctrl Pts',(-18.6517810536065,-12.5982384226112,
122.417476843907)) ;
#42253=CARTESIAN_POINT('Ctrl Pts',(-18.6517928977279,-12.5982377386978,
122.417467821109)) ;
#42254=CARTESIAN_POINT('Ctrl Pts',(-18.6518166193069,-12.5982363689609,
122.417449750787)) ;
#42255=CARTESIAN_POINT('Ctrl Pts',(-18.6518284963018,-12.5982356831643,
122.417440703618)) ;
#42256=CARTESIAN_POINT('Ctrl Pts',(-18.6518522838537,-12.5982343096481,
122.417422584387)) ;
#42257=CARTESIAN_POINT('Ctrl Pts',(-18.6518641941415,-12.5982336219442,
122.417413512533)) ;
#42258=CARTESIAN_POINT('Ctrl Pts',(-18.6518880474834,-12.5982322446596,
122.417395344543)) ;
#42259=CARTESIAN_POINT('Ctrl Pts',(-18.651899990836,-12.5982315550617,122.417386248183)) ;
#42260=CARTESIAN_POINT('Ctrl Pts',(-18.6519239126945,-12.5982301738515,
122.41736802937)) ;
#42261=CARTESIAN_POINT('Ctrl Pts',(-18.6519358905298,-12.5982294822779,
122.417358907429)) ;
#42262=CARTESIAN_POINT('Ctrl Pts',(-18.6519598771807,-12.5982280973573,
122.41734064064)) ;
#42263=CARTESIAN_POINT('Ctrl Pts',(-18.6519718876903,-12.5982274039125,
122.417331494502)) ;
#42264=CARTESIAN_POINT('Ctrl Pts',(-18.6519959460754,-12.598226014881,122.417313174461)) ;
#42265=CARTESIAN_POINT('Ctrl Pts',(-18.6520079917256,-12.5982253194228,
122.417304002255)) ;
#42266=CARTESIAN_POINT('Ctrl Pts',(-18.6520321171906,-12.5982239265495,
122.417285632518)) ;
#42267=CARTESIAN_POINT('Ctrl Pts',(-18.6520441973327,-12.5982232291154,
122.417276434742)) ;
#42268=CARTESIAN_POINT('Ctrl Pts',(-18.6520683923358,-12.5982218322585,
122.417258013451)) ;
#42269=CARTESIAN_POINT('Ctrl Pts',(-18.6520805072433,-12.5982211328329,
122.417248789902)) ;
#42270=CARTESIAN_POINT('Ctrl Pts',(-18.6521047732719,-12.5982197319068,
122.417230315935)) ;
#42271=CARTESIAN_POINT('Ctrl Pts',(-18.6521169240576,-12.5982190304257,
122.417221065774)) ;
#42272=CARTESIAN_POINT('Ctrl Pts',(-18.6521412587488,-12.5982176255671,
122.417202540942)) ;
#42273=CARTESIAN_POINT('Ctrl Pts',(-18.6521534443566,-12.5982169220914,
122.417193264978)) ;
#42274=CARTESIAN_POINT('Ctrl Pts',(-18.652177851847,-12.5982155130618,122.417174686144)) ;
#42275=CARTESIAN_POINT('Ctrl Pts',(-18.6521900733948,-12.5982148075273,
122.417165383532)) ;
#42276=CARTESIAN_POINT('Ctrl Pts',(-18.6522145527332,-12.5982133943819,
122.417146751433)) ;
#42277=CARTESIAN_POINT('Ctrl Pts',(-18.6522268105489,-12.5982126867697,
122.41713742193)) ;
#42278=CARTESIAN_POINT('Ctrl Pts',(-18.6522513615862,-12.5982112695173,
122.417118736692)) ;
#42279=CARTESIAN_POINT('Ctrl Pts',(-18.6522636552575,-12.5982105598513,
122.417109380617)) ;
#42280=CARTESIAN_POINT('Ctrl Pts',(-18.6522882813838,-12.5982091382967,
122.417090639673)) ;
#42281=CARTESIAN_POINT('Ctrl Pts',(-18.6523006125482,-12.5982084264826,
122.417081255788)) ;
#42282=CARTESIAN_POINT('Ctrl Pts',(-18.6523253102834,-12.5982070008268,
122.417062461798)) ;
#42283=CARTESIAN_POINT('Ctrl Pts',(-18.6523376777531,-12.5982062869333,
122.417053051012)) ;
#42284=CARTESIAN_POINT('Ctrl Pts',(-18.6523624522966,-12.5982048568765,
122.417034200033)) ;
#42285=CARTESIAN_POINT('Ctrl Pts',(-18.6523748579617,-12.5982041407946,
122.417024760915)) ;
#42286=CARTESIAN_POINT('Ctrl Pts',(-18.6523997055566,-12.598202706554,122.417005855819)) ;
#42287=CARTESIAN_POINT('Ctrl Pts',(-18.6524121484581,-12.5982019883392,
122.416996389105)) ;
#42288=CARTESIAN_POINT('Ctrl Pts',(-18.652437073206,-12.5982005496783,122.416977426784)) ;
#42289=CARTESIAN_POINT('Ctrl Pts',(-18.6524495545654,-12.5981998292603,
122.416967931551)) ;
#42290=CARTESIAN_POINT('Ctrl Pts',(-18.6567934521444,-12.597949104504,122.413663426948)) ;
#42291=CARTESIAN_POINT('Ctrl Pts',(-18.6611463339235,-12.5976988627779,
122.41039674497)) ;
#42292=CARTESIAN_POINT('Ctrl Pts',(-18.6734340244622,-12.5969953609926,
122.401300104429)) ;
#42293=CARTESIAN_POINT('Ctrl Pts',(-18.6814165759149,-12.5965417064587,
122.395535327698)) ;
#42294=CARTESIAN_POINT('Ctrl Pts',(-18.7188613552968,-12.5944301126438,
122.369161238339)) ;
#42295=CARTESIAN_POINT('Ctrl Pts',(-18.7491360860425,-12.5927700185484,
122.349734795158)) ;
#42296=CARTESIAN_POINT('Ctrl Pts',(-18.7857313605827,-12.5908238242757,
122.328422627866)) ;
#42297=CARTESIAN_POINT('Ctrl Pts',(-18.7912812474141,-12.590530242542,122.325247285693)) ;
#42298=CARTESIAN_POINT('Ctrl Pts',(-18.8028525912613,-12.5899213713806,
122.318744129597)) ;
#42299=CARTESIAN_POINT('Ctrl Pts',(-18.8088776479493,-12.5896061159434,
122.315423164743)) ;
#42300=CARTESIAN_POINT('Ctrl Pts',(-18.8357079027558,-12.5882093979238,
122.300922022959)) ;
#42301=CARTESIAN_POINT('Ctrl Pts',(-18.8568001232337,-12.5871301699246,
122.290283086876)) ;
#42302=CARTESIAN_POINT('Ctrl Pts',(-18.8910698359654,-12.5853981641484,
122.274198884258)) ;
#42303=CARTESIAN_POINT('Ctrl Pts',(-18.9040609666328,-12.5847464256436,
122.26837032123)) ;
#42304=CARTESIAN_POINT('Ctrl Pts',(-18.9257845822485,-12.5836632697075,
122.259066369322)) ;
#42305=CARTESIAN_POINT('Ctrl Pts',(-18.9344617697248,-12.5832323614048,
122.255465251041)) ;
#42306=CARTESIAN_POINT('Ctrl Pts',(-18.9546147311477,-12.5822352048693,
122.247366662356)) ;
#42307=CARTESIAN_POINT('Ctrl Pts',(-18.9661180654133,-12.5816687171091,
122.242940428904)) ;
#42308=CARTESIAN_POINT('Ctrl Pts',(-18.991440956753,-12.5804270281306,122.233624287929)) ;
#42309=CARTESIAN_POINT('Ctrl Pts',(-19.0052848873552,-12.5797514602395,
122.228805888461)) ;
#42310=CARTESIAN_POINT('Ctrl Pts',(-19.036454196692,-12.5782395924792,122.218568314961)) ;
#42311=CARTESIAN_POINT('Ctrl Pts',(-19.0538194611561,-12.5774037391161,
122.213280779272)) ;
#42312=CARTESIAN_POINT('Ctrl Pts',(-19.0782936512719,-12.5762358103298,
122.206407364857)) ;
#42313=CARTESIAN_POINT('Ctrl Pts',(-19.0853105791302,-12.5759020884391,
122.204502597124)) ;
#42314=CARTESIAN_POINT('Ctrl Pts',(-19.0951918284113,-12.5754336967082,
122.201912648842)) ;
#42315=CARTESIAN_POINT('Ctrl Pts',(-19.0980425471548,-12.5752987474402,
122.201176208488)) ;
#42316=CARTESIAN_POINT('Ctrl Pts',(-19.1015729348443,-12.5751318427742,
122.200277479658)) ;
#42317=CARTESIAN_POINT('Ctrl Pts',(-19.1022501704758,-12.5750998353516,
122.200105680638)) ;
#42318=CARTESIAN_POINT('Ctrl Pts',(-19.1093955983175,-12.5747622335787,
122.198299425895)) ;
#42319=CARTESIAN_POINT('Ctrl Pts',(-19.1158766436932,-12.5744569275915,
122.196716207647)) ;
#42320=CARTESIAN_POINT('Ctrl Pts',(-19.1299808509378,-12.5737943389088,
122.19339019267)) ;
#42321=CARTESIAN_POINT('Ctrl Pts',(-19.1376083219823,-12.5734371685362,
122.19166689041)) ;
#42322=CARTESIAN_POINT('Ctrl Pts',(-19.1598876430185,-12.5723968088264,
122.186852511924)) ;
#42323=CARTESIAN_POINT('Ctrl Pts',(-19.1745794660451,-12.5717144545339,
122.18395300421)) ;
#42324=CARTESIAN_POINT('Ctrl Pts',(-19.2168706178744,-12.5697561605352,
122.176393419967)) ;
#42325=CARTESIAN_POINT('Ctrl Pts',(-19.2445789193188,-12.5684789041517,
122.17239539015)) ;
#42326=CARTESIAN_POINT('Ctrl Pts',(-19.2929290543277,-12.5662551913537,
122.16706904809)) ;
#42327=CARTESIAN_POINT('Ctrl Pts',(-19.313513071246,-12.5653101695494,122.165316543651)) ;
#42328=CARTESIAN_POINT('Ctrl Pts',(-19.3465686699224,-12.5637932141276,
122.163325872459)) ;
#42329=CARTESIAN_POINT('Ctrl Pts',(-19.3590168401675,-12.5632220935145,
122.162762865888)) ;
#42330=CARTESIAN_POINT('Ctrl Pts',(-19.374320526249,-12.5625197120779,122.162299859459)) ;
#42331=CARTESIAN_POINT('Ctrl Pts',(-19.3771700169683,-12.5623889203638,
122.162223404289)) ;
#42332=CARTESIAN_POINT('Ctrl Pts',(-19.3805399956548,-12.5622342201541,
122.162144518463)) ;
#42333=CARTESIAN_POINT('Ctrl Pts',(-19.3810602557747,-12.5622103368968,
122.162132665065)) ;
#42334=CARTESIAN_POINT('Ctrl Pts',(-19.3826507720328,-12.5621373204145,
122.16209742112)) ;
#42335=CARTESIAN_POINT('Ctrl Pts',(-19.3837210507941,-12.5620881844143,
122.16207508055)) ;
#42336=CARTESIAN_POINT('Ctrl Pts',(-19.3856611977276,-12.5619991086109,
122.162037076059)) ;
#42337=CARTESIAN_POINT('Ctrl Pts',(-19.3865310561313,-12.5619591701102,
122.162020945343)) ;
#42338=CARTESIAN_POINT('Ctrl Pts',(-19.3881164518054,-12.5618863753109,
122.161993201357)) ;
#42339=CARTESIAN_POINT('Ctrl Pts',(-19.3888319836274,-12.5618535198421,
122.161981294395)) ;
#42340=CARTESIAN_POINT('Ctrl Pts',(-19.3901421788481,-12.5617933565315,
122.161960617243)) ;
#42341=CARTESIAN_POINT('Ctrl Pts',(-19.3907368390446,-12.5617660492346,
122.161951656968)) ;
#42342=CARTESIAN_POINT('Ctrl Pts',(-19.3918300580083,-12.5617158459883,
122.161935964835)) ;
#42343=CARTESIAN_POINT('Ctrl Pts',(-19.3923286148623,-12.5616929504034,
122.161929106876)) ;
#42344=CARTESIAN_POINT('Ctrl Pts',(-19.3932483021518,-12.5616507136896,
122.161917006378)) ;
#42345=CARTESIAN_POINT('Ctrl Pts',(-19.3936694313873,-12.5616313728104,
122.161911678375)) ;
#42346=CARTESIAN_POINT('Ctrl Pts',(-19.4113900891808,-12.5608175087271,
122.161696439116)) ;
#42347=CARTESIAN_POINT('Ctrl Pts',(-19.4286920506294,-12.5600218326315,
122.161845492945)) ;
#42348=CARTESIAN_POINT('Ctrl Pts',(-19.4630088294997,-12.5584411133718,
122.162853826808)) ;
#42349=CARTESIAN_POINT('Ctrl Pts',(-19.4800203654697,-12.5576564426578,
122.163701890469)) ;
#42350=CARTESIAN_POINT('Ctrl Pts',(-19.5262482463775,-12.5555216647514,
122.166954629337)) ;
#42351=CARTESIAN_POINT('Ctrl Pts',(-19.555405934401,-12.5541726197496,122.170039787513)) ;
#42352=CARTESIAN_POINT('Ctrl Pts',(-19.59792318565,-12.5522000013078,122.176056873907)) ;
#42353=CARTESIAN_POINT('Ctrl Pts',(-19.6113860357677,-12.5515745361261,
122.178187285577)) ;
#42354=CARTESIAN_POINT('Ctrl Pts',(-19.6374693193354,-12.5503604965431,
122.182753251485)) ;
#42355=CARTESIAN_POINT('Ctrl Pts',(-19.6500923643258,-12.5497719283014,
122.185164130982)) ;
#42356=CARTESIAN_POINT('Ctrl Pts',(-19.6916144804534,-12.5478313074489,
122.19376010551)) ;
#42357=CARTESIAN_POINT('Ctrl Pts',(-19.7203314428175,-12.5464819532277,
122.200775348978)) ;
#42358=CARTESIAN_POINT('Ctrl Pts',(-19.7690137598523,-12.544171420534,122.214513918643)) ;
#42359=CARTESIAN_POINT('Ctrl Pts',(-19.7891073189696,-12.543210809444,122.220736018034)) ;
#42360=CARTESIAN_POINT('Ctrl Pts',(-19.8138279735893,-12.5420166036866,
122.229080138977)) ;
#42361=CARTESIAN_POINT('Ctrl Pts',(-19.8186118233225,-12.5417849199917,
122.230727282536)) ;
#42362=CARTESIAN_POINT('Ctrl Pts',(-19.8286646732417,-12.5412967228836,
122.234257026657)) ;
#42363=CARTESIAN_POINT('Ctrl Pts',(-19.8339312982787,-12.5410401833435,
122.236146052025)) ;
#42364=CARTESIAN_POINT('Ctrl Pts',(-19.8393751002482,-12.5407741391536,
122.238139979367)) ;
#42365=CARTESIAN_POINT('Ctrl Pts',(-19.8395651295574,-12.5407648511191,
122.238209634658)) ;
#42366=CARTESIAN_POINT('Ctrl Pts',(-19.8399251962172,-12.5407472500901,
122.238341716392)) ;
#42367=CARTESIAN_POINT('Ctrl Pts',(-19.8400952369567,-12.5407389371509,
122.238404133657)) ;
#42368=CARTESIAN_POINT('Ctrl Pts',(-19.8404178425076,-12.5407231639424,
122.238522632831)) ;
#42369=CARTESIAN_POINT('Ctrl Pts',(-19.8405704099801,-12.5407157037166,
122.238578707552)) ;
#42370=CARTESIAN_POINT('Ctrl Pts',(-19.8408602071454,-12.5407015318824,
122.238685283905)) ;
#42371=CARTESIAN_POINT('Ctrl Pts',(-19.8409974388453,-12.5406948203131,
122.238735779834)) ;
#42372=CARTESIAN_POINT('Ctrl Pts',(-19.8412583897215,-12.540682056919,122.2388318516)) ;
#42373=CARTESIAN_POINT('Ctrl Pts',(-19.8413821105724,-12.5406760051216,
122.238877422941)) ;
#42374=CARTESIAN_POINT('Ctrl Pts',(-19.8416176052147,-12.5406644850109,
122.23896420736)) ;
#42375=CARTESIAN_POINT('Ctrl Pts',(-19.8417293804722,-12.5406590167133,
122.239005416896)) ;
#42376=CARTESIAN_POINT('Ctrl Pts',(-19.8419423331497,-12.540648597847,122.239083963318)) ;
#42377=CARTESIAN_POINT('Ctrl Pts',(-19.8420435116101,-12.5406436472977,
122.239121297312)) ;
#42378=CARTESIAN_POINT('Ctrl Pts',(-19.8422364385473,-12.5406342069886,
122.239192514084)) ;
#42379=CARTESIAN_POINT('Ctrl Pts',(-19.8423281876774,-12.5406297172537,
122.239226394463)) ;
#42380=CARTESIAN_POINT('Ctrl Pts',(-19.8425032697084,-12.5406211491292,
122.239291070693)) ;
#42381=CARTESIAN_POINT('Ctrl Pts',(-19.8425866035672,-12.5406170707389,
122.23932186476)) ;
#42382=CARTESIAN_POINT('Ctrl Pts',(-19.8427457408515,-12.5406092820854,
122.239380689481)) ;
#42383=CARTESIAN_POINT('Ctrl Pts',(-19.8428215446682,-12.5406055718406,
122.239408718539)) ;
#42384=CARTESIAN_POINT('Ctrl Pts',(-19.8429663967868,-12.540598481658,122.239462294721)) ;
#42385=CARTESIAN_POINT('Ctrl Pts',(-19.8430354455828,-12.5405951017267,
122.239487840605)) ;
#42386=CARTESIAN_POINT('Ctrl Pts',(-19.8431674686224,-12.5405886389267,
122.23953669824)) ;
#42387=CARTESIAN_POINT('Ctrl Pts',(-19.8432304433881,-12.5405855560577,
122.239560009019)) ;
#42388=CARTESIAN_POINT('Ctrl Pts',(-19.8487290245072,-12.5403163674425,
122.241595871051)) ;
#42389=CARTESIAN_POINT('Ctrl Pts',(-19.8541505595263,-12.5400500239687,
122.243646196633)) ;
#42390=CARTESIAN_POINT('Ctrl Pts',(-19.8644764810031,-12.5395410404277,
122.24763358236)) ;
#42391=CARTESIAN_POINT('Ctrl Pts',(-19.869383260888,-12.5392984364597,122.249564114839)) ;
#42392=CARTESIAN_POINT('Ctrl Pts',(-19.8910811647693,-12.5382224562978,
122.25825991873)) ;
#42393=CARTESIAN_POINT('Ctrl Pts',(-19.9077363657536,-12.5373881047342,
122.265358428475)) ;
#42394=CARTESIAN_POINT('Ctrl Pts',(-19.948165803999,-12.5353435195757,122.283637221976)) ;
#42395=CARTESIAN_POINT('Ctrl Pts',(-19.9717531705136,-12.5341340752103,
122.295210069937)) ;
#42396=CARTESIAN_POINT('Ctrl Pts',(-20.0038506164595,-12.5324650231041,
122.312233600051)) ;
#42397=CARTESIAN_POINT('Ctrl Pts',(-20.0126855108448,-12.532003078948,122.317056981037)) ;
#42398=CARTESIAN_POINT('Ctrl Pts',(-20.0283729895442,-12.5311781174807,
122.325869108256)) ;
#42399=CARTESIAN_POINT('Ctrl Pts',(-20.035247696484,-12.5308149452415,122.329817337744)) ;
#42400=CARTESIAN_POINT('Ctrl Pts',(-20.052174639553,-12.5299164678722,122.339754014594)) ;
#42401=CARTESIAN_POINT('Ctrl Pts',(-20.0621812477939,-12.5293815441596,
122.345818718191)) ;
#42402=CARTESIAN_POINT('Ctrl Pts',(-20.0839274480615,-12.5282100720115,
122.359419520616)) ;
#42403=CARTESIAN_POINT('Ctrl Pts',(-20.0956290266402,-12.5275738342157,
122.36701346472)) ;
#42404=CARTESIAN_POINT('Ctrl Pts',(-20.1371995564869,-12.5252898670514,
122.39499120492)) ;
#42405=CARTESIAN_POINT('Ctrl Pts',(-20.1663077450611,-12.5236463313578,
122.416472843222)) ;
#42406=CARTESIAN_POINT('Ctrl Pts',(-20.2002484428382,-12.5216543243005,
122.443872066418)) ;
#42407=CARTESIAN_POINT('Ctrl Pts',(-20.206011247099,-12.5213133141225,122.448610024873)) ;
#42408=CARTESIAN_POINT('Ctrl Pts',(-20.2150684731054,-12.5207726138369,
122.456193433105)) ;
#42409=CARTESIAN_POINT('Ctrl Pts',(-20.2183910409297,-12.5205732262521,
122.459004992359)) ;
#42410=CARTESIAN_POINT('Ctrl Pts',(-20.2256882974061,-12.5201330076515,
122.465245631297)) ;
#42411=CARTESIAN_POINT('Ctrl Pts',(-20.2296562007776,-12.5198921200652,
122.468682506186)) ;
#42412=CARTESIAN_POINT('Ctrl Pts',(-20.2390746949293,-12.5193167913841,
122.47694492528)) ;
#42413=CARTESIAN_POINT('Ctrl Pts',(-20.244505011187,-12.5189822124506,122.481793289362)) ;
#42414=CARTESIAN_POINT('Ctrl Pts',(-20.2632234434634,-12.517819201591,122.498801895604)) ;
#42415=CARTESIAN_POINT('Ctrl Pts',(-20.2762908516892,-12.5169901071281,
122.511201710088)) ;
#42416=CARTESIAN_POINT('Ctrl Pts',(-20.2987081723119,-12.5155386848456,
122.533413995483)) ;
#42417=CARTESIAN_POINT('Ctrl Pts',(-20.3081750123101,-12.514916140234,122.543104232447)) ;
#42418=CARTESIAN_POINT('Ctrl Pts',(-20.3231299535994,-12.5139171839564,
122.558918341652)) ;
#42419=CARTESIAN_POINT('Ctrl Pts',(-20.3287183775611,-12.5135402701681,
122.564945810877)) ;
#42420=CARTESIAN_POINT('Ctrl Pts',(-20.3394589780795,-12.5128087217969,
122.576761872617)) ;
#42421=CARTESIAN_POINT('Ctrl Pts',(-20.3446175793769,-12.5124540628249,
122.582544125998)) ;
#42422=CARTESIAN_POINT('Ctrl Pts',(-20.35317908599,-12.5118597788923,122.592322208077)) ;
#42423=CARTESIAN_POINT('Ctrl Pts',(-20.3566111861844,-12.511619976883,122.59629217012)) ;
#42424=CARTESIAN_POINT('Ctrl Pts',(-20.3664643869393,-12.5109269031389,
122.60783565252)) ;
#42425=CARTESIAN_POINT('Ctrl Pts',(-20.3728203742093,-12.5104741101781,
122.615464209613)) ;
#42426=CARTESIAN_POINT('Ctrl Pts',(-20.3964459859189,-12.5087676513948,
122.644517037307)) ;
#42427=CARTESIAN_POINT('Ctrl Pts',(-20.4130973853529,-12.5075157518028,
122.666433746619)) ;
#42428=CARTESIAN_POINT('Ctrl Pts',(-20.4328063780566,-12.5059581201874,
122.694234471175)) ;
#42429=CARTESIAN_POINT('Ctrl Pts',(-20.436558676165,-12.5056579513954,122.699616630187)) ;
#42430=CARTESIAN_POINT('Ctrl Pts',(-20.4430090363465,-12.5051354306199,
122.709025834574)) ;
#42431=CARTESIAN_POINT('Ctrl Pts',(-20.4457263725472,-12.5049132399226,
122.713039498848)) ;
#42432=CARTESIAN_POINT('Ctrl Pts',(-20.4515086819168,-12.5044358910012,
122.721688242119)) ;
#42433=CARTESIAN_POINT('Ctrl Pts',(-20.4545662293466,-12.5041806747331,
122.726328156609)) ;
#42434=CARTESIAN_POINT('Ctrl Pts',(-20.4608144196517,-12.5036532090433,
122.735948977861)) ;
#42435=CARTESIAN_POINT('Ctrl Pts',(-20.464000849022,-12.5033809292519,122.740932454319)) ;
#42436=CARTESIAN_POINT('Ctrl Pts',(-20.4720224206811,-12.502686954097,122.753676353063)) ;
#42437=CARTESIAN_POINT('Ctrl Pts',(-20.4768079952114,-12.5022648338344,
122.76146753493)) ;
#42438=CARTESIAN_POINT('Ctrl Pts',(-20.4874017674507,-12.501311673866,122.779146833229)) ;
#42439=CARTESIAN_POINT('Ctrl Pts',(-20.4931602188682,-12.5007801590533,
122.789063748253)) ;
#42440=CARTESIAN_POINT('Ctrl Pts',(-20.5113092029293,-12.4990619699213,
122.821333505918)) ;
#42441=CARTESIAN_POINT('Ctrl Pts',(-20.5231511539718,-12.4978751115754,
122.84398788179)) ;
#42442=CARTESIAN_POINT('Ctrl Pts',(-20.5364386895791,-12.4964705762957,
122.87142554464)) ;
#42443=CARTESIAN_POINT('Ctrl Pts',(-20.5385607013546,-12.4962438242242,
122.875874206416)) ;
#42444=CARTESIAN_POINT('Ctrl Pts',(-20.5418174161854,-12.4958919850364,
122.882806926424)) ;
#42445=CARTESIAN_POINT('Ctrl Pts',(-20.5429703787687,-12.4957666572122,
122.885282337128)) ;
#42446=CARTESIAN_POINT('Ctrl Pts',(-20.5452527984745,-12.4955170149904,
122.890224945431)) ;
#42447=CARTESIAN_POINT('Ctrl Pts',(-20.5463823520393,-12.4953926998991,
122.892692081729)) ;
#42448=CARTESIAN_POINT('Ctrl Pts',(-20.548615950219,-12.4951453312416,122.897612907794)) ;
#42449=CARTESIAN_POINT('Ctrl Pts',(-20.5497201233433,-12.4950222765312,
122.90006652276)) ;
#42450=CARTESIAN_POINT('Ctrl Pts',(-20.5522251138042,-12.4947413310105,
122.90568130678)) ;
#42451=CARTESIAN_POINT('Ctrl Pts',(-20.5536207551637,-12.4945835107433,
122.908844763223)) ;
#42452=CARTESIAN_POINT('Ctrl Pts',(-20.5574141688876,-12.494150938545,122.917540698383)) ;
#42453=CARTESIAN_POINT('Ctrl Pts',(-20.559785068028,-12.4938765422664,122.923084808435)) ;
#42454=CARTESIAN_POINT('Ctrl Pts',(-20.5729182539762,-12.4923329668888,
122.954420685885)) ;
#42455=CARTESIAN_POINT('Ctrl Pts',(-20.5828498748888,-12.4910752987972,
122.980541181549)) ;
#42456=CARTESIAN_POINT('Ctrl Pts',(-20.5919009558887,-12.4898128815271,
123.00698191868)) ;
#42457=CARTESIAN_POINT('Ctrl Pts',(-20.5919009558702,-12.4898128815389,
123.006981918687)) ;
#42458=CARTESIAN_POINT('Ctrl Pts',(-20.612879600018,-12.4868868188589,123.068266969564)) ;
#42459=CARTESIAN_POINT('Ctrl Pts',(-20.6290608408633,-12.4839078358475,
123.131081843711)) ;
#42460=CARTESIAN_POINT('Ctrl Pts',(-20.6403019341679,-12.4808963918362,
123.194867639949)) ;
#42461=CARTESIAN_POINT('Ctrl Pts',(-20.6529209728128,-12.4775158017703,
123.266472367879)) ;
#42462=CARTESIAN_POINT('Ctrl Pts',(-20.6592686579283,-12.4741985571895,
123.339040698344)) ;
#42463=CARTESIAN_POINT('Ctrl Pts',(-20.6592722344714,-12.4709053075509,
123.411752881973)) ;
#42464=CARTESIAN_POINT('Ctrl Pts',(-20.6592758117281,-12.4676114008349,
123.484479573319)) ;
#42465=CARTESIAN_POINT('Ctrl Pts',(-20.6529324105397,-12.4643042891385,
123.557066247848)) ;
#42466=CARTESIAN_POINT('Ctrl Pts',(-20.6403149806974,-12.4609455594289,
123.628687049695)) ;
#42467=CARTESIAN_POINT('Ctrl Pts',(-20.6199530079514,-12.4555252508826,
123.744268498017)) ;
#42468=CARTESIAN_POINT('Ctrl Pts',(-20.5834152479651,-12.4501098853957,
123.856407451353)) ;
#42469=CARTESIAN_POINT('Ctrl Pts',(-20.5317752294988,-12.444794208555,123.961802575126)) ;
#42470=CARTESIAN_POINT('Ctrl Pts',(-20.5195465431204,-12.4435354223093,
123.986760813963)) ;
#42471=CARTESIAN_POINT('Ctrl Pts',(-20.5064888790875,-12.442279198336,124.011304221324)) ;
#42472=CARTESIAN_POINT('Ctrl Pts',(-20.4926240347142,-12.4410177925474,
124.035391851884)) ;
#42473=CARTESIAN_POINT('Ctrl Pts',(-20.4565432913977,-12.4377352127181,
124.098075542512)) ;
#42474=CARTESIAN_POINT('Ctrl Pts',(-20.4150917468142,-12.4344077824959,
124.157507085578)) ;
#42475=CARTESIAN_POINT('Ctrl Pts',(-20.3687357231582,-12.4310436061992,
124.213019594203)) ;
#42476=CARTESIAN_POINT('Ctrl Pts',(-20.3221020045676,-12.4276592768643,
124.268864649523)) ;
#42477=CARTESIAN_POINT('Ctrl Pts',(-20.2706831796546,-12.4243269367417,
124.320530635347)) ;
#42478=CARTESIAN_POINT('Ctrl Pts',(-20.2150581879501,-12.4210466606148,
124.367434060606)) ;
#42479=CARTESIAN_POINT('Ctrl Pts',(-20.1599469320555,-12.4177966801385,
124.413904299838)) ;
#42480=CARTESIAN_POINT('Ctrl Pts',(-20.100924231773,-12.4144999293209,124.455516207877)) ;
#42481=CARTESIAN_POINT('Ctrl Pts',(-20.0386444222632,-12.4111419282649,
124.491810038396)) ;
#42482=CARTESIAN_POINT('Ctrl Pts',(-19.9757838743836,-12.4077526149735,
124.528442296731)) ;
#42483=CARTESIAN_POINT('Ctrl Pts',(-19.9098471799391,-12.4044322628923,
124.559515887026)) ;
#42484=CARTESIAN_POINT('Ctrl Pts',(-19.841576804616,-12.401145070914,124.584679559154)) ;
#42485=CARTESIAN_POINT('Ctrl Pts',(-19.8324565589139,-12.4007059346361,
124.588041176422)) ;
#42486=CARTESIAN_POINT('Ctrl Pts',(-19.8232974443718,-12.4002663542339,
124.591296288893)) ;
#42487=CARTESIAN_POINT('Ctrl Pts',(-19.814101322745,-12.3998259425229,124.594444237049)) ;
#42488=CARTESIAN_POINT('Ctrl Pts',(-19.7549143065903,-12.3969914155221,
124.614704697484)) ;
#42489=CARTESIAN_POINT('Ctrl Pts',(-19.6942924538234,-12.39410730187,124.630492631303)) ;
#42490=CARTESIAN_POINT('Ctrl Pts',(-19.6327443861755,-12.3912118041499,
124.641676227974)) ;
#42491=CARTESIAN_POINT('Ctrl Pts',(-19.5611608795202,-12.3878441942762,
124.654683314912)) ;
#42492=CARTESIAN_POINT('Ctrl Pts',(-19.4885786093359,-12.3845400790549,
124.661415969366)) ;
#42493=CARTESIAN_POINT('Ctrl Pts',(-19.4158220208586,-12.3812149268458,
124.661797206604)) ;
#42494=CARTESIAN_POINT('Ctrl Pts',(-19.343386996428,-12.377904470892,124.662176758878)) ;
#42495=CARTESIAN_POINT('Ctrl Pts',(-19.2710559139747,-12.3745611835623,
124.656259343137)) ;
#42496=CARTESIAN_POINT('Ctrl Pts',(-19.1996452414557,-12.3712618741336,
124.644111620985)) ;
#42497=CARTESIAN_POINT('Ctrl Pts',(-19.1286196590726,-12.3679803566045,
124.6320294068)) ;
#42498=CARTESIAN_POINT('Ctrl Pts',(-19.0587744373215,-12.3647050110643,
124.613829966515)) ;
#42499=CARTESIAN_POINT('Ctrl Pts',(-18.990886651944,-12.3613625287099,124.589716528532)) ;
#42500=CARTESIAN_POINT('Ctrl Pts',(-18.9459998958675,-12.3591525112628,
124.573772953368)) ;
#42501=CARTESIAN_POINT('Ctrl Pts',(-18.9020613678976,-12.3569451070035,
124.555276798977)) ;
#42502=CARTESIAN_POINT('Ctrl Pts',(-18.8592840273916,-12.3547760794749,
124.53431736011)) ;
#42503=CARTESIAN_POINT('Ctrl Pts',(-18.8367533302812,-12.3536336591727,
124.52327808644)) ;
#42504=CARTESIAN_POINT('Ctrl Pts',(-18.8145600542151,-12.3525002895855,
124.511562945122)) ;
#42505=CARTESIAN_POINT('Ctrl Pts',(-18.7927341753271,-12.3513654274978,
124.49918772465)) ;
#42506=CARTESIAN_POINT('Ctrl Pts',(-18.7298943652711,-12.3480979981127,
124.463557704534)) ;
#42507=CARTESIAN_POINT('Ctrl Pts',(-18.6702644990938,-12.3447812010954,
124.422549451139)) ;
#42508=CARTESIAN_POINT('Ctrl Pts',(-18.6145104587646,-12.3414395552883,
124.376621973083)) ;
#42509=CARTESIAN_POINT('Ctrl Pts',(-18.5583545546135,-12.3380738235755,
124.330363459073)) ;
#42510=CARTESIAN_POINT('Ctrl Pts',(-18.5063444574012,-12.3347691056417,
124.279290603724)) ;
#42511=CARTESIAN_POINT('Ctrl Pts',(-18.4590716004823,-12.3314422012028,
124.223983531472)) ;
#42512=CARTESIAN_POINT('Ctrl Pts',(-18.4118841285253,-12.3281213058699,
124.168776355704)) ;
#42513=CARTESIAN_POINT('Ctrl Pts',(-18.3695977095774,-12.3247766394425,
124.109561752482)) ;
#42514=CARTESIAN_POINT('Ctrl Pts',(-18.3326922444195,-12.3214625370788,
124.047011597277)) ;
#42515=CARTESIAN_POINT('Ctrl Pts',(-18.2960197209067,-12.3181693528218,
123.984856249073)) ;
#42516=CARTESIAN_POINT('Ctrl Pts',(-18.2647994434423,-12.3148741484591,
123.919643033231)) ;
#42517=CARTESIAN_POINT('Ctrl Pts',(-18.239380419725,-12.3115457444478,123.852101929866)) ;
#42518=CARTESIAN_POINT('Ctrl Pts',(-18.2349565077231,-12.3109664709628,
123.840347115789)) ;
#42519=CARTESIAN_POINT('Ctrl Pts',(-18.2307100075446,-12.3103871771171,
123.828526282873)) ;
#42520=CARTESIAN_POINT('Ctrl Pts',(-18.2266423654683,-12.3098085062256,
123.816643453356)) ;
#42521=CARTESIAN_POINT('Origin',(-19.4092722359532,-13.9601742359176,123.411814366564)) ;
#42522=CARTESIAN_POINT('',(-18.3578548015691,-12.0237683560339,124.087847855652)) ;
#42523=CARTESIAN_POINT('',(-18.2266508223232,-11.7,123.81666815758)) ;
#42524=CARTESIAN_POINT('Ctrl Pts',(-18.3578549773983,-12.0237683877577,
124.087848203357)) ;
#42525=CARTESIAN_POINT('Ctrl Pts',(-18.3582088223246,-12.0157754186098,
124.088398528862)) ;
#42526=CARTESIAN_POINT('Ctrl Pts',(-18.3583806245238,-12.007835083744,124.088665030377)) ;
#42527=CARTESIAN_POINT('Ctrl Pts',(-18.3583806245238,-12.,124.088665030376)) ;
#42528=CARTESIAN_POINT('Ctrl Pts',(-18.3583806245238,-11.9621695797156,
124.088665030376)) ;
#42529=CARTESIAN_POINT('Ctrl Pts',(-18.3540742080748,-11.9219235159019,
124.082116008719)) ;
#42530=CARTESIAN_POINT('Ctrl Pts',(-18.3375495990129,-11.8480564696762,
124.055365260225)) ;
#42531=CARTESIAN_POINT('Ctrl Pts',(-18.3254377303918,-11.8144220247009,
124.035135143544)) ;
#42532=CARTESIAN_POINT('Ctrl Pts',(-18.2995859960063,-11.761317155029,123.987854560826)) ;
#42533=CARTESIAN_POINT('Ctrl Pts',(-18.2841086594605,-11.7382522587826,
123.957600803974)) ;
#42534=CARTESIAN_POINT('Ctrl Pts',(-18.2537250256192,-11.7075896772134,
123.889921628303)) ;
#42535=CARTESIAN_POINT('Ctrl Pts',(-18.2389020196221,-11.7,123.852455220934)) ;
#42536=CARTESIAN_POINT('Ctrl Pts',(-18.2266508223232,-11.7,123.81666815758)) ;
#42537=CARTESIAN_POINT('',(-20.6477480580335,-12.1788369205275,123.242469634735)) ;
#42538=CARTESIAN_POINT('Ctrl Pts',(-18.3578547670581,-12.0237683857362,
124.08784787622)) ;
#42539=CARTESIAN_POINT('Ctrl Pts',(-18.3612709689585,-12.0240583399856,
124.093161006863)) ;
#42540=CARTESIAN_POINT('Ctrl Pts',(-18.3647221587456,-12.0243476810626,
124.09844020082)) ;
#42541=CARTESIAN_POINT('Ctrl Pts',(-18.3720326190228,-12.0249532474956,
124.109439954333)) ;
#42542=CARTESIAN_POINT('Ctrl Pts',(-18.3758941530953,-12.0252689942272,
124.115147304605)) ;
#42543=CARTESIAN_POINT('Ctrl Pts',(-18.3962392787662,-12.0269117251184,
124.144688135181)) ;
#42544=CARTESIAN_POINT('Ctrl Pts',(-18.413500777637,-12.0282350907313,124.167975020533)) ;
#42545=CARTESIAN_POINT('Ctrl Pts',(-18.4355734167998,-12.0298564993528,
124.195684372511)) ;
#42546=CARTESIAN_POINT('Ctrl Pts',(-18.4396298675406,-12.0301517584363,
124.200696647887)) ;
#42547=CARTESIAN_POINT('Ctrl Pts',(-18.4472060060469,-12.030698480577,124.209911236339)) ;
#42548=CARTESIAN_POINT('Ctrl Pts',(-18.4507149053608,-12.0309498672555,
124.214122217716)) ;
#42549=CARTESIAN_POINT('Ctrl Pts',(-18.4585324561556,-12.0315061313412,
124.223379458499)) ;
#42550=CARTESIAN_POINT('Ctrl Pts',(-18.4628538019447,-12.0318111676068,
124.228414742769)) ;
#42551=CARTESIAN_POINT('Ctrl Pts',(-18.4806423513383,-12.033056668807,124.248811299113)) ;
#42552=CARTESIAN_POINT('Ctrl Pts',(-18.4944450745935,-12.0339992029702,
124.263875745673)) ;
#42553=CARTESIAN_POINT('Ctrl Pts',(-18.5141829230335,-12.0353100504372,
124.284385105258)) ;
#42554=CARTESIAN_POINT('Ctrl Pts',(-18.5198107691195,-12.035679840316,124.290121187478)) ;
#42555=CARTESIAN_POINT('Ctrl Pts',(-18.5293205336302,-12.0362979726219,
124.299628697603)) ;
#42556=CARTESIAN_POINT('Ctrl Pts',(-18.53317233433,-12.0365465344298,124.303429893235)) ;
#42557=CARTESIAN_POINT('Ctrl Pts',(-18.5406782615933,-12.0370274103583,
124.310741606244)) ;
#42558=CARTESIAN_POINT('Ctrl Pts',(-18.5443292894376,-12.0372597469713,
124.314255153538)) ;
#42559=CARTESIAN_POINT('Ctrl Pts',(-18.5515137068691,-12.0377138829511,
124.321085387555)) ;
#42560=CARTESIAN_POINT('Ctrl Pts',(-18.5550452201474,-12.0379356960937,
124.324403918043)) ;
#42561=CARTESIAN_POINT('Ctrl Pts',(-18.5636048377083,-12.0384699476098,
124.332354090901)) ;
#42562=CARTESIAN_POINT('Ctrl Pts',(-18.5686518180992,-12.038782184171,124.336965189997)) ;
#42563=CARTESIAN_POINT('Ctrl Pts',(-18.5914463314759,-12.0401803146378,
124.357450526429)) ;
#42564=CARTESIAN_POINT('Ctrl Pts',(-18.6096074102078,-12.0412612739329,
124.372857097527)) ;
#42565=CARTESIAN_POINT('Ctrl Pts',(-18.6402319121722,-12.0430413302621,
124.397367295236)) ;
#42566=CARTESIAN_POINT('Ctrl Pts',(-18.6524433750215,-12.0437409093724,
124.406775505422)) ;
#42567=CARTESIAN_POINT('Ctrl Pts',(-18.672791183876,-12.0448937163516,124.421860892095)) ;
#42568=CARTESIAN_POINT('Ctrl Pts',(-18.6808266487049,-12.0453457458803,
124.427671319415)) ;
#42569=CARTESIAN_POINT('Ctrl Pts',(-18.6926060729012,-12.0460043095135,
124.435977361085)) ;
#42570=CARTESIAN_POINT('Ctrl Pts',(-18.6962957325594,-12.0462100160739,
124.438549353814)) ;
#42571=CARTESIAN_POINT('Ctrl Pts',(-18.7030476176529,-12.0465854497209,
124.443202021255)) ;
#42572=CARTESIAN_POINT('Ctrl Pts',(-18.706105361161,-12.0467551034372,124.445289113152)) ;
#42573=CARTESIAN_POINT('Ctrl Pts',(-18.7122417299274,-12.0470948522912,
124.44943770917)) ;
#42574=CARTESIAN_POINT('Ctrl Pts',(-18.7153203387539,-12.0472649459507,
124.451499170589)) ;
#42575=CARTESIAN_POINT('Ctrl Pts',(-18.7240874100868,-12.0477483350986,
124.457313384164)) ;
#42576=CARTESIAN_POINT('Ctrl Pts',(-18.7297974432447,-12.0480619910566,
124.461033336482)) ;
#42577=CARTESIAN_POINT('Ctrl Pts',(-18.7632486650801,-12.0498927564979,
124.482438424913)) ;
#42578=CARTESIAN_POINT('Ctrl Pts',(-18.7916487038095,-12.0514225918069,
124.499069364155)) ;
#42579=CARTESIAN_POINT('Ctrl Pts',(-18.8309632392298,-12.0534908001967,
124.520053878567)) ;
#42580=CARTESIAN_POINT('Ctrl Pts',(-18.8413320036948,-12.0540314147734,
124.525403162818)) ;
#42581=CARTESIAN_POINT('Ctrl Pts',(-18.8568201622614,-12.0548308889698,
124.533120966241)) ;
#42582=CARTESIAN_POINT('Ctrl Pts',(-18.8618830985897,-12.0550909775863,
124.535601231108)) ;
#42583=CARTESIAN_POINT('Ctrl Pts',(-18.8701791912078,-12.0555150752811,
124.539596009511)) ;
#42584=CARTESIAN_POINT('Ctrl Pts',(-18.8734023498748,-12.0556793348499,
124.541131067215)) ;
#42585=CARTESIAN_POINT('Ctrl Pts',(-18.8791665832693,-12.0559721852485,
124.543846100261)) ;
#42586=CARTESIAN_POINT('Ctrl Pts',(-18.8817051288494,-12.0561008427538,
124.54503137873)) ;
#42587=CARTESIAN_POINT('Ctrl Pts',(-18.8868594141117,-12.056361440124,124.547416905385)) ;
#42588=CARTESIAN_POINT('Ctrl Pts',(-18.8894753568765,-12.0564933731153,
124.548616674428)) ;
#42589=CARTESIAN_POINT('Ctrl Pts',(-18.8947406895689,-12.0567582758437,
124.551009578329)) ;
#42590=CARTESIAN_POINT('Ctrl Pts',(-18.8973901424193,-12.0568912425011,
124.552202530793)) ;
#42591=CARTESIAN_POINT('Ctrl Pts',(-18.9050072965419,-12.0572725923696,
124.555600365016)) ;
#42592=CARTESIAN_POINT('Ctrl Pts',(-18.9099852587864,-12.0575206812022,
124.557782103541)) ;
#42593=CARTESIAN_POINT('Ctrl Pts',(-18.9360113871106,-12.058812156449,124.568987044983)) ;
#42594=CARTESIAN_POINT('Ctrl Pts',(-18.9572904285564,-12.0598484571019,
124.577463066214)) ;
#42595=CARTESIAN_POINT('Ctrl Pts',(-18.9943522547517,-12.0616349119909,
124.59105826424)) ;
#42596=CARTESIAN_POINT('Ctrl Pts',(-19.0100260955046,-12.0623856386635,
124.596456623542)) ;
#42597=CARTESIAN_POINT('Ctrl Pts',(-19.033332479642,-12.0634986553714,124.603968672123)) ;
#42598=CARTESIAN_POINT('Ctrl Pts',(-19.0408851478688,-12.0638587898761,
124.606324115848)) ;
#42599=CARTESIAN_POINT('Ctrl Pts',(-19.0532910983399,-12.0644496650562,
124.610064296411)) ;
#42600=CARTESIAN_POINT('Ctrl Pts',(-19.0581313172037,-12.0646800274288,
124.611491623022)) ;
#42601=CARTESIAN_POINT('Ctrl Pts',(-19.0631991562815,-12.0649210690279,
124.612952774745)) ;
#42602=CARTESIAN_POINT('Ctrl Pts',(-19.0634182941461,-12.0649314915787,
124.613015891296)) ;
#42603=CARTESIAN_POINT('Ctrl Pts',(-19.0638422009522,-12.0649516526898,
124.613137860212)) ;
#42604=CARTESIAN_POINT('Ctrl Pts',(-19.0640469678079,-12.0649613911891,
124.613196720232)) ;
#42605=CARTESIAN_POINT('Ctrl Pts',(-19.0644433009267,-12.064980239876,124.61331053608)) ;
#42606=CARTESIAN_POINT('Ctrl Pts',(-19.0646348651881,-12.0649893500009,
124.613365498421)) ;
#42607=CARTESIAN_POINT('Ctrl Pts',(-19.0650058714959,-12.0650069933203,
124.613471849052)) ;
#42608=CARTESIAN_POINT('Ctrl Pts',(-19.0651853119072,-12.0650155264649,
124.613523242963)) ;
#42609=CARTESIAN_POINT('Ctrl Pts',(-19.0655330645158,-12.0650320631757,
124.613622759254)) ;
#42610=CARTESIAN_POINT('Ctrl Pts',(-19.065701375233,-12.0650400666954,124.613670886447)) ;
#42611=CARTESIAN_POINT('Ctrl Pts',(-19.0660277823305,-12.0650555876845,
124.61376414595)) ;
#42612=CARTESIAN_POINT('Ctrl Pts',(-19.066185877715,-12.065063105127,124.613809282484)) ;
#42613=CARTESIAN_POINT('Ctrl Pts',(-19.0664926942241,-12.0650776939686,
124.613896813721)) ;
#42614=CARTESIAN_POINT('Ctrl Pts',(-19.0666414144139,-12.0650847653407,
124.613939212045)) ;
#42615=CARTESIAN_POINT('Ctrl Pts',(-19.066930251874,-12.0650984987698,124.61402149815)) ;
#42616=CARTESIAN_POINT('Ctrl Pts',(-19.0670703681084,-12.0651051607926,
124.614061388995)) ;
#42617=CARTESIAN_POINT('Ctrl Pts',(-19.0673427049197,-12.065118109196,124.614138871338)) ;
#42618=CARTESIAN_POINT('Ctrl Pts',(-19.0674749246114,-12.0651243955475,
124.614176465489)) ;
#42619=CARTESIAN_POINT('Ctrl Pts',(-19.0677321165733,-12.0651366234674,
124.614249547273)) ;
#42620=CARTESIAN_POINT('Ctrl Pts',(-19.0678570882186,-12.0651425650173,
124.614285037246)) ;
#42621=CARTESIAN_POINT('Ctrl Pts',(-19.0681003787338,-12.0651541316391,
124.614354086924)) ;
#42622=CARTESIAN_POINT('Ctrl Pts',(-19.0682186969636,-12.0651597566903,
124.614387648632)) ;
#42623=CARTESIAN_POINT('Ctrl Pts',(-19.0684492260406,-12.0651707162727,
124.614453002893)) ;
#42624=CARTESIAN_POINT('Ctrl Pts',(-19.0685614362341,-12.0651760507812,
124.614484797161)) ;
#42625=CARTESIAN_POINT('Ctrl Pts',(-19.068780248515,-12.0651864530393,124.614546763584)) ;
#42626=CARTESIAN_POINT('Ctrl Pts',(-19.0688868504596,-12.0651915207894,
124.614576937354)) ;
#42627=CARTESIAN_POINT('Ctrl Pts',(-19.0690949059344,-12.0652014114058,
124.614635797755)) ;
#42628=CARTESIAN_POINT('Ctrl Pts',(-19.0691963589123,-12.0652062342523,
124.614664485676)) ;
#42629=CARTESIAN_POINT('Ctrl Pts',(-19.0693945370095,-12.065215655073,124.61472049754)) ;
#42630=CARTESIAN_POINT('Ctrl Pts',(-19.0694912621768,-12.0652202530551,
124.614747822761)) ;
#42631=CARTESIAN_POINT('Ctrl Pts',(-19.0696803731708,-12.0652292426324,
124.614801222695)) ;
#42632=CARTESIAN_POINT('Ctrl Pts',(-19.0697727584279,-12.0652336342055,
124.614827298353)) ;
#42633=CARTESIAN_POINT('Ctrl Pts',(-19.0699535460676,-12.0652422279242,
124.614878303023)) ;
#42634=CARTESIAN_POINT('Ctrl Pts',(-19.0700419482321,-12.0652464300637,
124.614903232943)) ;
#42635=CARTESIAN_POINT('Ctrl Pts',(-19.0702150979003,-12.0652546605296,
124.614952041547)) ;
#42636=CARTESIAN_POINT('Ctrl Pts',(-19.0702998455832,-12.0652586888682,
124.614975921134)) ;
#42637=CARTESIAN_POINT('Ctrl Pts',(-19.0704659909973,-12.0652665862273,
124.615022717435)) ;
#42638=CARTESIAN_POINT('Ctrl Pts',(-19.0705473882328,-12.0652704552275,
124.61504563476)) ;
#42639=CARTESIAN_POINT('Ctrl Pts',(-19.0707071138598,-12.0652780472812,
124.615090587886)) ;
#42640=CARTESIAN_POINT('Ctrl Pts',(-19.0707854418161,-12.065281770317,124.615112624226)) ;
#42641=CARTESIAN_POINT('Ctrl Pts',(-19.0709392895052,-12.0652890828384,
124.615155890645)) ;
#42642=CARTESIAN_POINT('Ctrl Pts',(-19.0710148090141,-12.0652926723158,
124.615177121244)) ;
#42643=CARTESIAN_POINT('Ctrl Pts',(-19.0711632813639,-12.0652997292093,
124.6152188458)) ;
#42644=CARTESIAN_POINT('Ctrl Pts',(-19.0712362345037,-12.0653031966418,
124.615239340354)) ;
#42645=CARTESIAN_POINT('Ctrl Pts',(-19.0713798009225,-12.0653100202322,
124.615279658047)) ;
#42646=CARTESIAN_POINT('Ctrl Pts',(-19.0714504139388,-12.0653133763796,
124.615299481564)) ;
#42647=CARTESIAN_POINT('Ctrl Pts',(-19.0715895118707,-12.0653199874703,
124.615338517959)) ;
#42648=CARTESIAN_POINT('Ctrl Pts',(-19.0716579964576,-12.0653232423998,
124.615357731144)) ;
#42649=CARTESIAN_POINT('Ctrl Pts',(-19.0717930352878,-12.065329660459,124.615395603528)) ;
#42650=CARTESIAN_POINT('Ctrl Pts',(-19.0718595897204,-12.0653328235992,
124.615414263131)) ;
#42651=CARTESIAN_POINT('Ctrl Pts',(-19.0719909564925,-12.0653390670313,
124.615451082161)) ;
#42652=CARTESIAN_POINT('Ctrl Pts',(-19.0720557684534,-12.0653421473066,
124.615469241789)) ;
#42653=CARTESIAN_POINT('Ctrl Pts',(-19.0721838265998,-12.0653482333928,
124.615505111178)) ;
#42654=CARTESIAN_POINT('Ctrl Pts',(-19.0722470731097,-12.0653512392202,
124.615522821299)) ;
#42655=CARTESIAN_POINT('Ctrl Pts',(-19.0762301485984,-12.0655405357329,
124.616637813054)) ;
#42656=CARTESIAN_POINT('Ctrl Pts',(-19.0801553049901,-12.0657269895376,
124.617715944138)) ;
#42657=CARTESIAN_POINT('Ctrl Pts',(-19.088639114193,-12.0661298023783,124.620001703209)) ;
#42658=CARTESIAN_POINT('Ctrl Pts',(-19.0931994742278,-12.066346212982,124.621202744347)) ;
#42659=CARTESIAN_POINT('Ctrl Pts',(-19.1058204566635,-12.0669448117018,
124.624450412063)) ;
#42660=CARTESIAN_POINT('Ctrl Pts',(-19.1138948552431,-12.0673274084469,
124.626442442691)) ;
#42661=CARTESIAN_POINT('Ctrl Pts',(-19.1433593517,-12.0687219818445,124.633400433995)) ;
#42662=CARTESIAN_POINT('Ctrl Pts',(-19.1648594142534,-12.0697368347804,
124.637883103475)) ;
#42663=CARTESIAN_POINT('Ctrl Pts',(-19.1965346659422,-12.0712225840397,
124.643620936463)) ;
#42664=CARTESIAN_POINT('Ctrl Pts',(-19.2066251032401,-12.0716943379384,
124.64532109144)) ;
#42665=CARTESIAN_POINT('Ctrl Pts',(-19.2240995537892,-12.0725084127209,
124.648045181434)) ;
#42666=CARTESIAN_POINT('Ctrl Pts',(-19.2314739172003,-12.0728511124802,
124.649127305228)) ;
#42667=CARTESIAN_POINT('Ctrl Pts',(-19.246018295573,-12.0735255157969,124.651128853948)) ;
#42668=CARTESIAN_POINT('Ctrl Pts',(-19.2531874837964,-12.0738572263652,
124.652052165627)) ;
#42669=CARTESIAN_POINT('Ctrl Pts',(-19.2652503094854,-12.0744143195046,
124.653499472226)) ;
#42670=CARTESIAN_POINT('Ctrl Pts',(-19.2701397533147,-12.0746398406192,
124.654056842615)) ;
#42671=CARTESIAN_POINT('Ctrl Pts',(-19.3003609648911,-12.0760322130973,
124.657321234559)) ;
#42672=CARTESIAN_POINT('Ctrl Pts',(-19.3257672984041,-12.0771958162629,
124.659282182534)) ;
#42673=CARTESIAN_POINT('Ctrl Pts',(-19.3569476665447,-12.0786231564571,
124.660731923813)) ;
#42674=CARTESIAN_POINT('Ctrl Pts',(-19.3626812935453,-12.0788856044457,
124.660958957615)) ;
#42675=CARTESIAN_POINT('Ctrl Pts',(-19.3705669119841,-12.0792466520045,
124.661216835009)) ;
#42676=CARTESIAN_POINT('Ctrl Pts',(-19.3727177257002,-12.0793451380621,
124.661281612246)) ;
#42677=CARTESIAN_POINT('Ctrl Pts',(-19.3760108183361,-12.0794959517665,
124.661372281832)) ;
#42678=CARTESIAN_POINT('Ctrl Pts',(-19.3771529839349,-12.0795482636559,
124.661402162263)) ;
#42679=CARTESIAN_POINT('Ctrl Pts',(-19.3794827977797,-12.0796549805596,
124.661459916603)) ;
#42680=CARTESIAN_POINT('Ctrl Pts',(-19.3806704480149,-12.0797093860621,
124.661487663504)) ;
#42681=CARTESIAN_POINT('Ctrl Pts',(-19.3872243507252,-12.0800096500864,
124.66163143356)) ;
#42682=CARTESIAN_POINT('Ctrl Pts',(-19.3925912598122,-12.0802556576475,
124.6617145846)) ;
#42683=CARTESIAN_POINT('Ctrl Pts',(-19.4033303867848,-12.0807483282119,
124.661811788053)) ;
#42684=CARTESIAN_POINT('Ctrl Pts',(-19.4087024912663,-12.0809949863761,
124.661825780289)) ;
#42685=CARTESIAN_POINT('Ctrl Pts',(-19.4355377146454,-12.0822285714519,
124.661722683523)) ;
#42686=CARTESIAN_POINT('Ctrl Pts',(-19.4569951615066,-12.0832196122376,
124.661087432713)) ;
#42687=CARTESIAN_POINT('Ctrl Pts',(-19.4878060683474,-12.0846422148189,
124.659380277275)) ;
#42688=CARTESIAN_POINT('Ctrl Pts',(-19.4971804512169,-12.0850750365897,
124.658754786505)) ;
#42689=CARTESIAN_POINT('Ctrl Pts',(-19.5121411979591,-12.0857654490284,
124.657587003704)) ;
#42690=CARTESIAN_POINT('Ctrl Pts',(-19.5177324896768,-12.0860234049652,
124.657112668334)) ;
#42691=CARTESIAN_POINT('Ctrl Pts',(-19.5278088525537,-12.0864881156827,
124.656189465094)) ;
#42692=CARTESIAN_POINT('Ctrl Pts',(-19.5322950464282,-12.0866949551186,
124.65575395656)) ;
#42693=CARTESIAN_POINT('Ctrl Pts',(-19.5405634575249,-12.0870760643871,
124.654906112773)) ;
#42694=CARTESIAN_POINT('Ctrl Pts',(-19.5443463344156,-12.0872503822523,
124.654500755951)) ;
#42695=CARTESIAN_POINT('Ctrl Pts',(-19.5536894535107,-12.0876808202606,
124.653456421)) ;
#42696=CARTESIAN_POINT('Ctrl Pts',(-19.5592473726583,-12.0879367854468,
124.652797357071)) ;
#42697=CARTESIAN_POINT('Ctrl Pts',(-19.575734040739,-12.0886958706214,124.650729975241)) ;
#42698=CARTESIAN_POINT('Ctrl Pts',(-19.5866488193571,-12.0891981431688,
124.649214450418)) ;
#42699=CARTESIAN_POINT('Ctrl Pts',(-19.6260165305145,-12.0910101146941,
124.643216623814)) ;
#42700=CARTESIAN_POINT('Ctrl Pts',(-19.6543322905931,-12.0923132982599,
124.637895593769)) ;
#42701=CARTESIAN_POINT('Ctrl Pts',(-19.6913845279926,-12.0940384591645,
124.629597882083)) ;
#42702=CARTESIAN_POINT('Ctrl Pts',(-19.700307724554,-12.0944554785715,124.627496224327)) ;
#42703=CARTESIAN_POINT('Ctrl Pts',(-19.7142309322125,-12.0951091842482,
124.624054844294)) ;
#42704=CARTESIAN_POINT('Ctrl Pts',(-19.7192471231918,-12.0953453120366,
124.622781893504)) ;
#42705=CARTESIAN_POINT('Ctrl Pts',(-19.7274820049232,-12.0957340472592,
124.620637621175)) ;
#42706=CARTESIAN_POINT('Ctrl Pts',(-19.7307053761778,-12.0958864857901,
124.619784504543)) ;
#42707=CARTESIAN_POINT('Ctrl Pts',(-19.7339524604594,-12.0960403357193,
124.618911194777)) ;
#42708=CARTESIAN_POINT('Ctrl Pts',(-19.7339796304271,-12.0960416230786,
124.618903886377)) ;
#42709=CARTESIAN_POINT('Ctrl Pts',(-19.7340336567299,-12.0960441829775,
124.618889351983)) ;
#42710=CARTESIAN_POINT('Ctrl Pts',(-19.7340605132027,-12.0960454555231,
124.618882125976)) ;
#42711=CARTESIAN_POINT('Ctrl Pts',(-19.7341139201516,-12.0960479861552,
124.618867754381)) ;
#42712=CARTESIAN_POINT('Ctrl Pts',(-19.7341404706024,-12.0960492442399,
124.618860608822)) ;
#42713=CARTESIAN_POINT('Ctrl Pts',(-19.7341932732528,-12.0960517463157,
124.618846396104)) ;
#42714=CARTESIAN_POINT('Ctrl Pts',(-19.7342195251464,-12.0960529902919,
124.618839329049)) ;
#42715=CARTESIAN_POINT('Ctrl Pts',(-19.7342717382947,-12.0960554645101,
124.618825271352)) ;
#42716=CARTESIAN_POINT('Ctrl Pts',(-19.734297699264,-12.0960566947381,124.618818280807)) ;
#42717=CARTESIAN_POINT('Ctrl Pts',(-19.7343493355344,-12.0960591416944,
124.618804374854)) ;
#42718=CARTESIAN_POINT('Ctrl Pts',(-19.7343750118,-12.0960603584679,124.618797459205)) ;
#42719=CARTESIAN_POINT('Ctrl Pts',(-19.734426088005,-12.0960627789565,124.618783700584)) ;
#42720=CARTESIAN_POINT('Ctrl Pts',(-19.7344514874982,-12.09606398265,124.618776857751)) ;
#42721=CARTESIAN_POINT('Ctrl Pts',(-19.7345020142175,-12.09606637717,124.618763243726)) ;
#42722=CARTESIAN_POINT('Ctrl Pts',(-19.7345271425784,-12.0960675680498,
124.618756472247)) ;
#42723=CARTESIAN_POINT('Ctrl Pts',(-19.7345771369075,-12.0960699374091,
124.618742998321)) ;
#42724=CARTESIAN_POINT('Ctrl Pts',(-19.7346020019772,-12.0960711158457,
124.618736296135)) ;
#42725=CARTESIAN_POINT('Ctrl Pts',(-19.7346514742387,-12.0960734605313,
124.618722959631)) ;
#42726=CARTESIAN_POINT('Ctrl Pts',(-19.7346760819729,-12.0960746268057,
124.618716325184)) ;
#42727=CARTESIAN_POINT('Ctrl Pts',(-19.7347250463702,-12.0960769474887,
124.618703122376)) ;
#42728=CARTESIAN_POINT('Ctrl Pts',(-19.7347494031223,-12.0960781019012,
124.618696554006)) ;
#42729=CARTESIAN_POINT('Ctrl Pts',(-19.7347978734309,-12.0960803992325,
124.618683481276)) ;
#42730=CARTESIAN_POINT('Ctrl Pts',(-19.7348219863018,-12.0960815421184,
124.618676977116)) ;
#42731=CARTESIAN_POINT('Ctrl Pts',(-19.7348699724547,-12.0960838165668,
124.61866403188)) ;
#42732=CARTESIAN_POINT('Ctrl Pts',(-19.7348938465724,-12.0960849481685,
124.618657590593)) ;
#42733=CARTESIAN_POINT('Ctrl Pts',(-19.7349413640165,-12.0960872004641,
124.618644768776)) ;
#42734=CARTESIAN_POINT('Ctrl Pts',(-19.7349650063444,-12.0960883211106,
124.618638388529)) ;
#42735=CARTESIAN_POINT('Ctrl Pts',(-19.7350120654982,-12.0960905517456,
124.618625687406)) ;
#42736=CARTESIAN_POINT('Ctrl Pts',(-19.7350354820297,-12.09609166172,124.618619366624)) ;
#42737=CARTESIAN_POINT('Ctrl Pts',(-19.7350820945787,-12.0960938712465,
124.618606783128)) ;
#42738=CARTESIAN_POINT('Ctrl Pts',(-19.7351052909254,-12.096094970814,124.618600520338)) ;
#42739=CARTESIAN_POINT('Ctrl Pts',(-19.7351514696571,-12.0960971598365,
124.618588051098)) ;
#42740=CARTESIAN_POINT('Ctrl Pts',(-19.7351744520568,-12.0960982492919,
124.618581844657)) ;
#42741=CARTESIAN_POINT('Ctrl Pts',(-19.7352202067037,-12.0961004182701,
124.618569487123)) ;
#42742=CARTESIAN_POINT('Ctrl Pts',(-19.7352429798793,-12.0961014978365,
124.618563335794)) ;
#42743=CARTESIAN_POINT('Ctrl Pts',(-19.7352883253059,-12.0961036474734,
124.618551086029)) ;
#42744=CARTESIAN_POINT('Ctrl Pts',(-19.7353108963806,-12.0961047174877,
124.618544987925)) ;
#42745=CARTESIAN_POINT('Ctrl Pts',(-19.7353558390246,-12.096106848087,124.618532844263)) ;
#42746=CARTESIAN_POINT('Ctrl Pts',(-19.7353782117894,-12.0961079087283,
124.618526798396)) ;
#42747=CARTESIAN_POINT('Ctrl Pts',(-19.7354227680478,-12.0961100210658,
124.618514756478)) ;
#42748=CARTESIAN_POINT('Ctrl Pts',(-19.7354449497628,-12.0961110726774,
124.61850876092)) ;
#42749=CARTESIAN_POINT('Ctrl Pts',(-19.7354891260055,-12.0961131670537,
124.618496819092)) ;
#42750=CARTESIAN_POINT('Ctrl Pts',(-19.7355111212321,-12.0961142098513,
124.618490872645)) ;
#42751=CARTESIAN_POINT('Ctrl Pts',(-19.7355549297109,-12.0961162868459,
124.618479027661)) ;
#42752=CARTESIAN_POINT('Ctrl Pts',(-19.7355767436234,-12.096117321074,124.618473128958)) ;
#42753=CARTESIAN_POINT('Ctrl Pts',(-19.7356201949731,-12.0961193811898,
124.618461378006)) ;
#42754=CARTESIAN_POINT('Ctrl Pts',(-19.7356418326082,-12.0961204070867,
124.618455525715)) ;
#42755=CARTESIAN_POINT('Ctrl Pts',(-19.7356849384307,-12.0961224508725,
124.61844386572)) ;
#42756=CARTESIAN_POINT('Ctrl Pts',(-19.7357064057764,-12.0961234687213,
124.618438058252)) ;
#42757=CARTESIAN_POINT('Ctrl Pts',(-19.735749173782,-12.0961254965414,124.618426487185)) ;
#42758=CARTESIAN_POINT('Ctrl Pts',(-19.7357704750478,-12.0961265065413,
124.618420723431)) ;
#42759=CARTESIAN_POINT('Ctrl Pts',(-19.7358129177099,-12.096128518986,124.618409237974)) ;
#42760=CARTESIAN_POINT('Ctrl Pts',(-19.7358340584645,-12.0961295214003,
124.618403516455)) ;
#42761=CARTESIAN_POINT('Ctrl Pts',(-19.7358761852192,-12.0961315189159,
124.61839211411)) ;
#42762=CARTESIAN_POINT('Ctrl Pts',(-19.7358971709611,-12.0961325140047,
124.618386433363)) ;
#42763=CARTESIAN_POINT('Ctrl Pts',(-19.7359389890441,-12.0961344969332,
124.618375112224)) ;
#42764=CARTESIAN_POINT('Ctrl Pts',(-19.7359598231085,-12.0961354848543,
124.618369471373)) ;
#42765=CARTESIAN_POINT('Ctrl Pts',(-19.7360013467242,-12.0961374538682,
124.618358227644)) ;
#42766=CARTESIAN_POINT('Ctrl Pts',(-19.7360220352338,-12.0961384349113,
124.618352625056)) ;
#42767=CARTESIAN_POINT('Ctrl Pts',(-19.7360632710443,-12.0961403903255,
124.618341456982)) ;
#42768=CARTESIAN_POINT('Ctrl Pts',(-19.7360838183628,-12.0961413646971,
124.618335891499)) ;
#42769=CARTESIAN_POINT('Ctrl Pts',(-19.7361247769421,-12.096143307012,124.618324796263)) ;
#42770=CARTESIAN_POINT('Ctrl Pts',(-19.7361451879543,-12.0961442749433,
124.618319266585)) ;
#42771=CARTESIAN_POINT('Ctrl Pts',(-19.7361858788676,-12.0961462046116,
124.618308241639)) ;
#42772=CARTESIAN_POINT('Ctrl Pts',(-19.7362061586647,-12.0961471663435,
124.618302746408)) ;
#42773=CARTESIAN_POINT('Ctrl Pts',(-19.7362465895581,-12.0961490837269,
124.618291789725)) ;
#42774=CARTESIAN_POINT('Ctrl Pts',(-19.7362667418648,-12.0961500394356,
124.618286327952)) ;
#42775=CARTESIAN_POINT('Ctrl Pts',(-19.7363069243786,-12.0961519450853,
124.618275436418)) ;
#42776=CARTESIAN_POINT('Ctrl Pts',(-19.7363269542645,-12.0961528950109,
124.61827000675)) ;
#42777=CARTESIAN_POINT('Ctrl Pts',(-19.7363668968152,-12.0961547893252,
124.618259178123)) ;
#42778=CARTESIAN_POINT('Ctrl Pts',(-19.7363868090088,-12.0961557336915,
124.618253779297)) ;
#42779=CARTESIAN_POINT('Ctrl Pts',(-19.7364265203621,-12.0961576170853,
124.618243011238)) ;
#42780=CARTESIAN_POINT('Ctrl Pts',(-19.7364463193167,-12.0961585561031,
124.618237642066)) ;
#42781=CARTESIAN_POINT('Ctrl Pts',(-19.7364858091557,-12.0961604290351,
124.618226931985)) ;
#42782=CARTESIAN_POINT('Ctrl Pts',(-19.7365054998218,-12.0961613629388,
124.618221591141)) ;
#42783=CARTESIAN_POINT('Ctrl Pts',(-19.7365447752037,-12.0961632257428,
124.618210937158)) ;
#42784=CARTESIAN_POINT('Ctrl Pts',(-19.7365643610092,-12.0961641546947,
124.618205623729)) ;
#42785=CARTESIAN_POINT('Ctrl Pts',(-19.7366034337662,-12.0961660079312,
124.618195022668)) ;
#42786=CARTESIAN_POINT('Ctrl Pts',(-19.7366229198876,-12.0961669321765,
124.618189735266)) ;
#42787=CARTESIAN_POINT('Ctrl Pts',(-19.7366617980166,-12.0961687762243,
124.618179184988)) ;
#42788=CARTESIAN_POINT('Ctrl Pts',(-19.7366811894335,-12.0961696959988,
124.618173922277)) ;
#42789=CARTESIAN_POINT('Ctrl Pts',(-19.7367198795494,-12.0961715311709,
124.618163421017)) ;
#42790=CARTESIAN_POINT('Ctrl Pts',(-19.7367391795114,-12.0961724466285,
124.618158182129)) ;
#42791=CARTESIAN_POINT('Ctrl Pts',(-19.7367776930937,-12.0961742734689,
124.618147726799)) ;
#42792=CARTESIAN_POINT('Ctrl Pts',(-19.7367969062961,-12.096175184832,124.618142510474)) ;
#42793=CARTESIAN_POINT('Ctrl Pts',(-19.7368352525188,-12.0961770037753,
124.61813209861)) ;
#42794=CARTESIAN_POINT('Ctrl Pts',(-19.7368543842842,-12.0961779112961,
124.618126903415)) ;
#42795=CARTESIAN_POINT('Ctrl Pts',(-19.7368925691138,-12.0961797226248,
124.618116533422)) ;
#42796=CARTESIAN_POINT('Ctrl Pts',(-19.736911622872,-12.0961806264657,124.618111358439)) ;
#42797=CARTESIAN_POINT('Ctrl Pts',(-19.7369496578063,-12.0961824307248,
124.618101027218)) ;
#42798=CARTESIAN_POINT('Ctrl Pts',(-19.736968638743,-12.0961833311315,124.618095871049)) ;
#42799=CARTESIAN_POINT('Ctrl Pts',(-19.7370065299704,-12.096185128614,124.618085576941)) ;
#42800=CARTESIAN_POINT('Ctrl Pts',(-19.7370254414852,-12.0961860257477,
124.618080438674)) ;
#42801=CARTESIAN_POINT('Ctrl Pts',(-19.7370632004219,-12.0961878169947,
124.6180701786)) ;
#42802=CARTESIAN_POINT('Ctrl Pts',(-19.7370820475637,-12.0961887110947,
124.618065056872)) ;
#42803=CARTESIAN_POINT('Ctrl Pts',(-19.7371196814388,-12.0961904964487,
124.618054828886)) ;
#42804=CARTESIAN_POINT('Ctrl Pts',(-19.7371384683679,-12.0961913877121,
124.618049722578)) ;
#42805=CARTESIAN_POINT('Ctrl Pts',(-19.7371759864669,-12.0961931676134,
124.618039524174)) ;
#42806=CARTESIAN_POINT('Ctrl Pts',(-19.7371947176093,-12.0961940562499,
124.61803443209)) ;
#42807=CARTESIAN_POINT('Ctrl Pts',(-19.7405997366698,-12.0963555978143,
124.61710868825)) ;
#42808=CARTESIAN_POINT('Ctrl Pts',(-19.7439821260536,-12.0965163884945,
124.616173783017)) ;
#42809=CARTESIAN_POINT('Ctrl Pts',(-19.7507141210482,-12.0968370742468,
124.614282483996)) ;
#42810=CARTESIAN_POINT('Ctrl Pts',(-19.7540637548073,-12.0969969657835,
124.613326306902)) ;
#42811=CARTESIAN_POINT('Ctrl Pts',(-19.7632557265596,-12.0974366574562,
124.610660788293)) ;
#42812=CARTESIAN_POINT('Ctrl Pts',(-19.7690896284843,-12.0977167451546,
124.608922756839)) ;
#42813=CARTESIAN_POINT('Ctrl Pts',(-19.7976899585334,-12.09909500957,124.600174213327)) ;
#42814=CARTESIAN_POINT('Ctrl Pts',(-19.820265196321,-12.1001994120349,124.59255657963)) ;
#42815=CARTESIAN_POINT('Ctrl Pts',(-19.8693189595106,-12.102631156938,124.574426899797)) ;
#42816=CARTESIAN_POINT('Ctrl Pts',(-19.8956853775682,-12.1039568944303,
124.563644756999)) ;
#42817=CARTESIAN_POINT('Ctrl Pts',(-19.9260897669721,-12.1054933812914,
124.549980969834)) ;
#42818=CARTESIAN_POINT('Ctrl Pts',(-19.9305070847157,-12.1057168492066,
124.547964801112)) ;
#42819=CARTESIAN_POINT('Ctrl Pts',(-19.9375200061838,-12.1060719953755,
124.544714429497)) ;
#42820=CARTESIAN_POINT('Ctrl Pts',(-19.940123282688,-12.1062039114271,124.543496930535)) ;
#42821=CARTESIAN_POINT('Ctrl Pts',(-19.9448507101916,-12.1064436155215,
124.541266108199)) ;
#42822=CARTESIAN_POINT('Ctrl Pts',(-19.9469762401277,-12.106551446171,124.540255744165)) ;
#42823=CARTESIAN_POINT('Ctrl Pts',(-19.9515370033646,-12.1067829421594,
124.538071987723)) ;
#42824=CARTESIAN_POINT('Ctrl Pts',(-19.9539713101389,-12.1069065787527,
124.536896686145)) ;
#42825=CARTESIAN_POINT('Ctrl Pts',(-19.9593114539544,-12.1071779750773,
124.534297030684)) ;
#42826=CARTESIAN_POINT('Ctrl Pts',(-19.9622156120695,-12.1073256838582,
124.532869269544)) ;
#42827=CARTESIAN_POINT('Ctrl Pts',(-19.9697149510113,-12.1077074274355,
124.529146164705)) ;
#42828=CARTESIAN_POINT('Ctrl Pts',(-19.9743015930968,-12.1079412141059,
124.526833743045)) ;
#42829=CARTESIAN_POINT('Ctrl Pts',(-19.9881406320803,-12.1086477046893,
124.519749273)) ;
#42830=CARTESIAN_POINT('Ctrl Pts',(-19.9973478087975,-12.1091192102228,
124.514889839884)) ;
#42831=CARTESIAN_POINT('Ctrl Pts',(-20.0215044949151,-12.1103619976979,
124.501751819312)) ;
#42832=CARTESIAN_POINT('Ctrl Pts',(-20.036346753028,-12.1111313842965,124.493280751154)) ;
#42833=CARTESIAN_POINT('Ctrl Pts',(-20.0704202612595,-12.1129222911441,
124.472896292557)) ;
#42834=CARTESIAN_POINT('Ctrl Pts',(-20.0895109091983,-12.1139449510268,
124.460759978135)) ;
#42835=CARTESIAN_POINT('Ctrl Pts',(-20.1122599797971,-12.1151956220572,
124.445415591473)) ;
#42836=CARTESIAN_POINT('Ctrl Pts',(-20.1162426664637,-12.1154157779529,
124.442695577085)) ;
#42837=CARTESIAN_POINT('Ctrl Pts',(-20.1223874124323,-12.1157573627394,
124.438446606678)) ;
#42838=CARTESIAN_POINT('Ctrl Pts',(-20.1245605299186,-12.1158785394931,
124.436933709777)) ;
#42839=CARTESIAN_POINT('Ctrl Pts',(-20.128885892467,-12.1161204830641,124.433901997012)) ;
#42840=CARTESIAN_POINT('Ctrl Pts',(-20.1310381760492,-12.1162412481258,
124.432383260182)) ;
#42841=CARTESIAN_POINT('Ctrl Pts',(-20.1356334093656,-12.1164998962648,
124.429118874098)) ;
#42842=CARTESIAN_POINT('Ctrl Pts',(-20.1380749010505,-12.1166378106526,
124.427371204245)) ;
#42843=CARTESIAN_POINT('Ctrl Pts',(-20.1454431368342,-12.1170555231082,
124.422056614904)) ;
#42844=CARTESIAN_POINT('Ctrl Pts',(-20.1503501471911,-12.1173357443812,
124.418462529776)) ;
#42845=CARTESIAN_POINT('Ctrl Pts',(-20.1616290016971,-12.1179845456639,
124.410074291885)) ;
#42846=CARTESIAN_POINT('Ctrl Pts',(-20.1679815775983,-12.1183534923118,
124.405254709584)) ;
#42847=CARTESIAN_POINT('Ctrl Pts',(-20.1911329294585,-12.1197107080698,
124.387338616034)) ;
#42848=CARTESIAN_POINT('Ctrl Pts',(-20.2076422078547,-12.1207035885708,
124.373874177019)) ;
#42849=CARTESIAN_POINT('Ctrl Pts',(-20.226468669525,-12.1218594738387,124.357701449505)) ;
#42850=CARTESIAN_POINT('Ctrl Pts',(-20.2291284303065,-12.1220233308964,
124.35539701018)) ;
#42851=CARTESIAN_POINT('Ctrl Pts',(-20.2351020664319,-12.1223925389384,
124.350177075046)) ;
#42852=CARTESIAN_POINT('Ctrl Pts',(-20.2384103054665,-12.122597846561,124.347255194933)) ;
#42853=CARTESIAN_POINT('Ctrl Pts',(-20.2538281340221,-12.1235584006917,
124.333491919365)) ;
#42854=CARTESIAN_POINT('Ctrl Pts',(-20.2657410907948,-12.1243113136328,
124.322432446614)) ;
#42855=CARTESIAN_POINT('Ctrl Pts',(-20.2807229564756,-12.1252707928341,
124.307969780083)) ;
#42856=CARTESIAN_POINT('Ctrl Pts',(-20.2839933661764,-12.1254810421141,
124.304777875385)) ;
#42857=CARTESIAN_POINT('Ctrl Pts',(-20.2890828848724,-12.1258095053345,
124.299755738583)) ;
#42858=CARTESIAN_POINT('Ctrl Pts',(-20.2909139468366,-12.1259279365625,
124.297937694196)) ;
#42859=CARTESIAN_POINT('Ctrl Pts',(-20.294493721387,-12.1261599871198,124.294361289684)) ;
#42860=CARTESIAN_POINT('Ctrl Pts',(-20.2962428562168,-12.1262736137381,
124.292603370023)) ;
#42861=CARTESIAN_POINT('Ctrl Pts',(-20.3002646019119,-12.1265354409871,
124.288537296624)) ;
#42862=CARTESIAN_POINT('Ctrl Pts',(-20.3025334969575,-12.1266835740991,
124.286225489534)) ;
#42863=CARTESIAN_POINT('Ctrl Pts',(-20.3072886687628,-12.1269949406869,
124.281342559565)) ;
#42864=CARTESIAN_POINT('Ctrl Pts',(-20.3097729484632,-12.1271581382706,
124.27876953202)) ;
#42865=CARTESIAN_POINT('Ctrl Pts',(-20.3163458878405,-12.1275913780223,
124.271903048324)) ;
#42866=CARTESIAN_POINT('Ctrl Pts',(-20.3204151091899,-12.1278610948475,
124.267591098832)) ;
#42867=CARTESIAN_POINT('Ctrl Pts',(-20.3333135961762,-12.1287211710195,
124.253726928046)) ;
#42868=CARTESIAN_POINT('Ctrl Pts',(-20.3420245192357,-12.1293097712817,
124.244065757561)) ;
#42869=CARTESIAN_POINT('Ctrl Pts',(-20.3780491128386,-12.1317834919378,
124.202835171555)) ;
#42870=CARTESIAN_POINT('Ctrl Pts',(-20.4039229951881,-12.133665496402,124.170044161355)) ;
#42871=CARTESIAN_POINT('Ctrl Pts',(-20.4326409014067,-12.1359244306395,
124.129642890673)) ;
#42872=CARTESIAN_POINT('Ctrl Pts',(-20.4371138748614,-12.1362815412584,
124.123223376887)) ;
#42873=CARTESIAN_POINT('Ctrl Pts',(-20.4441998734258,-12.1368559876269,
124.112847361706)) ;
#42874=CARTESIAN_POINT('Ctrl Pts',(-20.4468511773194,-12.1370729431233,
124.108917239409)) ;
#42875=CARTESIAN_POINT('Ctrl Pts',(-20.4517921004877,-12.1374811144328,
124.101502496155)) ;
#42876=CARTESIAN_POINT('Ctrl Pts',(-20.4540867686813,-12.1376722784924,
124.098021315029)) ;
#42877=CARTESIAN_POINT('Ctrl Pts',(-20.4590218714978,-12.1380869241402,
124.09045225585)) ;
#42878=CARTESIAN_POINT('Ctrl Pts',(-20.4616559365253,-12.1383104623465,
124.08636030916)) ;
#42879=CARTESIAN_POINT('Ctrl Pts',(-20.4697727866498,-12.1390063025262,
124.073587737718)) ;
#42880=CARTESIAN_POINT('Ctrl Pts',(-20.4751725450949,-12.1394793418457,
124.064854902847)) ;
#42881=CARTESIAN_POINT('Ctrl Pts',(-20.4878462015155,-12.140614400604,124.043782211095)) ;
#42882=CARTESIAN_POINT('Ctrl Pts',(-20.4950167610676,-12.141277231621,124.031381939984)) ;
#42883=CARTESIAN_POINT('Ctrl Pts',(-20.5231955639474,-12.1439664058702,
123.980659351967)) ;
#42884=CARTESIAN_POINT('Ctrl Pts',(-20.5424007538072,-12.145996522205,123.941370420517)) ;
#42885=CARTESIAN_POINT('Ctrl Pts',(-20.564422676239,-12.1485928190175,123.889606177248)) ;
#42886=CARTESIAN_POINT('Ctrl Pts',(-20.5691622386565,-12.1491710437647,
123.877982510394)) ;
#42887=CARTESIAN_POINT('Ctrl Pts',(-20.5760254615005,-12.1500388375457,
123.86039759376)) ;
#42888=CARTESIAN_POINT('Ctrl Pts',(-20.5782802270883,-12.1503292795052,
123.854488420545)) ;
#42889=CARTESIAN_POINT('Ctrl Pts',(-20.5819280882339,-12.1508082164861,
123.844706029162)) ;
#42890=CARTESIAN_POINT('Ctrl Pts',(-20.5833470702858,-12.1509968864711,
123.840842597478)) ;
#42891=CARTESIAN_POINT('Ctrl Pts',(-20.5859593480778,-12.1513487156225,
123.83362018246)) ;
#42892=CARTESIAN_POINT('Ctrl Pts',(-20.5871574063013,-12.1515119057973,
123.830262967591)) ;
#42893=CARTESIAN_POINT('Ctrl Pts',(-20.590848318402,-12.1520204575482,123.819778787641)) ;
#42894=CARTESIAN_POINT('Ctrl Pts',(-20.5932909752033,-12.1523654705896,
123.812634317626)) ;
#42895=CARTESIAN_POINT('Ctrl Pts',(-20.5984366744584,-12.1531112297016,
123.797126172777)) ;
#42896=CARTESIAN_POINT('Ctrl Pts',(-20.6011165377074,-12.1535118105786,
123.788755225348)) ;
#42897=CARTESIAN_POINT('Ctrl Pts',(-20.608761404753,-12.1546921825679,123.763978418761)) ;
#42898=CARTESIAN_POINT('Ctrl Pts',(-20.6134775192506,-12.1554704922135,
123.74749788668)) ;
#42899=CARTESIAN_POINT('Ctrl Pts',(-20.624572344293,-12.1574417129196,123.705478063161)) ;
#42900=CARTESIAN_POINT('Ctrl Pts',(-20.6304860336949,-12.1586328222597,
123.679824771)) ;
#42901=CARTESIAN_POINT('Ctrl Pts',(-20.6358819592532,-12.1598967441597,
123.652502812988)) ;
#42902=CARTESIAN_POINT('Ctrl Pts',(-20.6361756779736,-12.1599662005072,
123.651001083359)) ;
#42903=CARTESIAN_POINT('Ctrl Pts',(-20.6397192990144,-12.1608122642352,
123.632704926981)) ;
#42904=CARTESIAN_POINT('Ctrl Pts',(-20.6426268591874,-12.1615906171343,
123.615846181314)) ;
#42905=CARTESIAN_POINT('Ctrl Pts',(-20.6463000445998,-12.1627107943247,
123.591584874177)) ;
#42906=CARTESIAN_POINT('Ctrl Pts',(-20.6473470189309,-12.1630504902502,
123.584226854407)) ;
#42907=CARTESIAN_POINT('Ctrl Pts',(-20.6490766126,-12.1636499543836,123.571242178131)) ;
#42908=CARTESIAN_POINT('Ctrl Pts',(-20.6497866997148,-12.1639095431914,
123.565619387327)) ;
#42909=CARTESIAN_POINT('Ctrl Pts',(-20.651100729922,-12.1644177267814,123.554612621106)) ;
#42910=CARTESIAN_POINT('Ctrl Pts',(-20.6517079583086,-12.1646662964126,
123.549229160334)) ;
#42911=CARTESIAN_POINT('Ctrl Pts',(-20.6529406274532,-12.1652022033277,
123.537623875316)) ;
#42912=CARTESIAN_POINT('Ctrl Pts',(-20.653554417112,-12.1654895998622,123.531400962233)) ;
#42913=CARTESIAN_POINT('Ctrl Pts',(-20.6558242437937,-12.1666409855252,
123.506474990045)) ;
#42914=CARTESIAN_POINT('Ctrl Pts',(-20.6571054691004,-12.1675068697634,
123.487740364236)) ;
#42915=CARTESIAN_POINT('Ctrl Pts',(-20.659178980782,-12.1696022439032,123.442451062891)) ;
#42916=CARTESIAN_POINT('Ctrl Pts',(-20.6595477573357,-12.1708338511469,
123.415886147478)) ;
#42917=CARTESIAN_POINT('Ctrl Pts',(-20.6587145982682,-12.1729824755116,
123.36957490034)) ;
#42918=CARTESIAN_POINT('Ctrl Pts',(-20.6578908525933,-12.1738977522582,
123.349830879059)) ;
#42919=CARTESIAN_POINT('Ctrl Pts',(-20.6562081118598,-12.1750843629603,
123.32414015327)) ;
#42920=CARTESIAN_POINT('Ctrl Pts',(-20.655773871485,-12.1753598923354,123.318168654451)) ;
#42921=CARTESIAN_POINT('Ctrl Pts',(-20.6550167088993,-12.175796418416,123.308697653849)) ;
#42922=CARTESIAN_POINT('Ctrl Pts',(-20.6547219037851,-12.1759577096709,
123.305196013)) ;
#42923=CARTESIAN_POINT('Ctrl Pts',(-20.6541429130458,-12.1762590772131,
123.298649218436)) ;
#42924=CARTESIAN_POINT('Ctrl Pts',(-20.6538623099325,-12.1763991912635,
123.295603776444)) ;
#42925=CARTESIAN_POINT('Ctrl Pts',(-20.6532787278679,-12.1766791884981,
123.289514721006)) ;
#42926=CARTESIAN_POINT('Ctrl Pts',(-20.6529757488871,-12.1768190706846,
123.286471128958)) ;
#42927=CARTESIAN_POINT('Ctrl Pts',(-20.6520888008697,-12.1772136655272,
123.277881217506)) ;
#42928=CARTESIAN_POINT('Ctrl Pts',(-20.6514788797325,-12.1774680913652,
123.272337640915)) ;
#42929=CARTESIAN_POINT('Ctrl Pts',(-20.6498835175878,-12.1780945119676,
123.258678896268)) ;
#42930=CARTESIAN_POINT('Ctrl Pts',(-20.648855529304,-12.1784660504912,123.250568950122)) ;
#42931=CARTESIAN_POINT('Ctrl Pts',(-20.6477480580335,-12.1788369205275,
123.242469634735)) ;
#42932=CARTESIAN_POINT('',(-20.6521256561948,-12.1170419242982,123.278341262904)) ;
#42933=CARTESIAN_POINT('Ctrl Pts',(-20.652125778092,-12.1170429607118,123.278341249912)) ;
#42934=CARTESIAN_POINT('Ctrl Pts',(-20.6511064564272,-12.1390146862922,
123.268849694058)) ;
#42935=CARTESIAN_POINT('Ctrl Pts',(-20.6497041626644,-12.1597501137876,
123.256775377451)) ;
#42936=CARTESIAN_POINT('Ctrl Pts',(-20.6477481882033,-12.178832505456,123.242470586714)) ;
#42937=CARTESIAN_POINT('',(-18.9628485264954,-11.9999999945477,124.57937843518)) ;
#42938=CARTESIAN_POINT('Ctrl Pts',(-20.6521257750101,-12.1170412970773,
123.278341221215)) ;
#42939=CARTESIAN_POINT('Ctrl Pts',(-20.6530685080591,-12.1166364163469,
123.287119609581)) ;
#42940=CARTESIAN_POINT('Ctrl Pts',(-20.6539182121897,-12.1162318136361,
123.295907752301)) ;
#42941=CARTESIAN_POINT('Ctrl Pts',(-20.6554930910976,-12.1153901623278,
123.314219343693)) ;
#42942=CARTESIAN_POINT('Ctrl Pts',(-20.6562023658464,-12.1149531919745,
123.323743599029)) ;
#42943=CARTESIAN_POINT('Ctrl Pts',(-20.6580408657703,-12.1136154895481,
123.352946609739)) ;
#42944=CARTESIAN_POINT('Ctrl Pts',(-20.658813852262,-12.1127162276281,123.372644757154)) ;
#42945=CARTESIAN_POINT('Ctrl Pts',(-20.65955069476,-12.1105596121518,123.419966285538)) ;
#42946=CARTESIAN_POINT('Ctrl Pts',(-20.6590654399524,-12.1093028384769,
123.447586137842)) ;
#42947=CARTESIAN_POINT('Ctrl Pts',(-20.6573711131328,-12.1077750330124,
123.480973558669)) ;
#42948=CARTESIAN_POINT('Ctrl Pts',(-20.6570359486246,-12.10750913202,123.486777812164)) ;
#42949=CARTESIAN_POINT('Ctrl Pts',(-20.6563183775252,-12.1070007389935,
123.497860435606)) ;
#42950=CARTESIAN_POINT('Ctrl Pts',(-20.6559429191866,-12.1067582934322,
123.503139130868)) ;
#42951=CARTESIAN_POINT('Ctrl Pts',(-20.6551380630678,-12.1062807300479,
123.513522691455)) ;
#42952=CARTESIAN_POINT('Ctrl Pts',(-20.6547107818719,-12.1060456304326,
123.518627617948)) ;
#42953=CARTESIAN_POINT('Ctrl Pts',(-20.6536312738023,-12.1054917832732,
123.530636384154)) ;
#42954=CARTESIAN_POINT('Ctrl Pts',(-20.6529529546488,-12.1051728677302,
123.537537699275)) ;
#42955=CARTESIAN_POINT('Ctrl Pts',(-20.6501177575175,-12.1039423214097,
123.564110090908)) ;
#42956=CARTESIAN_POINT('Ctrl Pts',(-20.6475513238575,-12.1030278748426,
123.583734369519)) ;
#42957=CARTESIAN_POINT('Ctrl Pts',(-20.6416060284001,-12.1012290557006,
123.622088791108)) ;
#42958=CARTESIAN_POINT('Ctrl Pts',(-20.6382631350108,-12.1003459094887,
123.640819360478)) ;
#42959=CARTESIAN_POINT('Ctrl Pts',(-20.6330494195697,-12.0991289732489,
123.66661344932)) ;
#42960=CARTESIAN_POINT('Ctrl Pts',(-20.6315422800174,-12.0987922689256,
123.673747770058)) ;
#42961=CARTESIAN_POINT('Ctrl Pts',(-20.6292059866973,-12.0982919947271,
123.684347548924)) ;
#42962=CARTESIAN_POINT('Ctrl Pts',(-20.6284243051366,-12.0981279475955,
123.687823286711)) ;
#42963=CARTESIAN_POINT('Ctrl Pts',(-20.6274174392802,-12.0979207859479,
123.69221256319)) ;
#42964=CARTESIAN_POINT('Ctrl Pts',(-20.6272060697273,-12.0978775211649,
123.693129246387)) ;
#42965=CARTESIAN_POINT('Ctrl Pts',(-20.6268298072623,-12.0978009002881,
123.694752676629)) ;
#42966=CARTESIAN_POINT('Ctrl Pts',(-20.6266653333704,-12.0977675395721,
123.695459520086)) ;
#42967=CARTESIAN_POINT('Ctrl Pts',(-20.6258378225337,-12.0976003535137,
123.699001854537)) ;
#42968=CARTESIAN_POINT('Ctrl Pts',(-20.62516549329,-12.0974666328674,123.701835170169)) ;
#42969=CARTESIAN_POINT('Ctrl Pts',(-20.6237885965282,-12.0971969823739,
123.707548710003)) ;
#42970=CARTESIAN_POINT('Ctrl Pts',(-20.6230836691423,-12.0970610576193,
123.710428828233)) ;
#42971=CARTESIAN_POINT('Ctrl Pts',(-20.6216508844303,-12.0967889840116,
123.716193841872)) ;
#42972=CARTESIAN_POINT('Ctrl Pts',(-20.6209229617056,-12.0966528368838,
123.719078700845)) ;
#42973=CARTESIAN_POINT('Ctrl Pts',(-20.6188249099563,-12.0962662424827,
123.727270173304)) ;
#42974=CARTESIAN_POINT('Ctrl Pts',(-20.6174301686541,-12.0960160896464,
123.732570422232)) ;
#42975=CARTESIAN_POINT('Ctrl Pts',(-20.6081874718496,-12.0944012715098,
123.766778451028)) ;
#42976=CARTESIAN_POINT('Ctrl Pts',(-20.599337539341,-12.0930500252769,123.795405064408)) ;
#42977=CARTESIAN_POINT('Ctrl Pts',(-20.584436332981,-12.0910067668295,123.838103604677)) ;
#42978=CARTESIAN_POINT('Ctrl Pts',(-20.5791412110244,-12.0903160981055,
123.852427288074)) ;
#42979=CARTESIAN_POINT('Ctrl Pts',(-20.5711241175557,-12.0893156046617,
123.872949862714)) ;
#42980=CARTESIAN_POINT('Ctrl Pts',(-20.5686121347261,-12.0890079948117,
123.879229320365)) ;
#42981=CARTESIAN_POINT('Ctrl Pts',(-20.5639925258408,-12.0884524307241,
123.890511048196)) ;
#42982=CARTESIAN_POINT('Ctrl Pts',(-20.5619030411288,-12.0882046967968,
123.895520566085)) ;
#42983=CARTESIAN_POINT('Ctrl Pts',(-20.5586835861007,-12.0878282262319,
123.903099851064)) ;
#42984=CARTESIAN_POINT('Ctrl Pts',(-20.5575774736087,-12.0876997907368,
123.905679692584)) ;
#42985=CARTESIAN_POINT('Ctrl Pts',(-20.5554046494442,-12.0874492439976,
123.910700714292)) ;
#42986=CARTESIAN_POINT('Ctrl Pts',(-20.5543388047405,-12.0873271443661,
123.913142253482)) ;
#42987=CARTESIAN_POINT('Ctrl Pts',(-20.5518769810121,-12.0870469457384,
123.918732763676)) ;
#42988=CARTESIAN_POINT('Ctrl Pts',(-20.550475776245,-12.0868887811144,123.921879405832)) ;
#42989=CARTESIAN_POINT('Ctrl Pts',(-20.5465582576679,-12.0864501870359,
123.930579902941)) ;
#42990=CARTESIAN_POINT('Ctrl Pts',(-20.5440142944134,-12.0861694120203,
123.936121182391)) ;
#42991=CARTESIAN_POINT('Ctrl Pts',(-20.5281920721199,-12.0844475026756,
123.969930660639)) ;
#42992=CARTESIAN_POINT('Ctrl Pts',(-20.5138989204612,-12.0829932142455,
123.997711305277)) ;
#42993=CARTESIAN_POINT('Ctrl Pts',(-20.4917812341337,-12.0808966370568,
124.037007491188)) ;
#42994=CARTESIAN_POINT('Ctrl Pts',(-20.4847811940601,-12.0802530730777,
124.048974205351)) ;
#42995=CARTESIAN_POINT('Ctrl Pts',(-20.4743313470192,-12.0793221287414,
124.066175371041)) ;
#42996=CARTESIAN_POINT('Ctrl Pts',(-20.471038983326,-12.0790328822455,124.071504148972)) ;
#42997=CARTESIAN_POINT('Ctrl Pts',(-20.4653210836285,-12.0785374876542,
124.080605021455)) ;
#42998=CARTESIAN_POINT('Ctrl Pts',(-20.4629150540793,-12.0783310795398,
124.084389210572)) ;
#42999=CARTESIAN_POINT('Ctrl Pts',(-20.459024363397,-12.0780005639255,124.090436349207)) ;
#43000=CARTESIAN_POINT('Ctrl Pts',(-20.4575526308465,-12.0778762734332,
124.092707557993)) ;
#43001=CARTESIAN_POINT('Ctrl Pts',(-20.4545688850919,-12.0776257600917,
124.097279533397)) ;
#43002=CARTESIAN_POINT('Ctrl Pts',(-20.4530566237068,-12.0774995416619,
124.099580119985)) ;
#43003=CARTESIAN_POINT('Ctrl Pts',(-20.4497822550268,-12.0772278527464,
124.104525707)) ;
#43004=CARTESIAN_POINT('Ctrl Pts',(-20.4480176351474,-12.0770824197811,
124.1071690219)) ;
#43005=CARTESIAN_POINT('Ctrl Pts',(-20.4432268762233,-12.0766902095232,
124.114286413317)) ;
#43006=CARTESIAN_POINT('Ctrl Pts',(-20.440181782998,-12.0764437074837,124.118747659604)) ;
#43007=CARTESIAN_POINT('Ctrl Pts',(-20.4231600012997,-12.0750808141701,
124.143341722488)) ;
#43008=CARTESIAN_POINT('Ctrl Pts',(-20.4086224061265,-12.0739729147259,
124.163079910862)) ;
#43009=CARTESIAN_POINT('Ctrl Pts',(-20.3827342658463,-12.0720740657774,
124.196146860031)) ;
#43010=CARTESIAN_POINT('Ctrl Pts',(-20.3716669023115,-12.0712826312124,
124.20968796889)) ;
#43011=CARTESIAN_POINT('Ctrl Pts',(-20.3550700481116,-12.0701207228053,
124.229146566824)) ;
#43012=CARTESIAN_POINT('Ctrl Pts',(-20.3497613598008,-12.069752667848,124.235249630609)) ;
#43013=CARTESIAN_POINT('Ctrl Pts',(-20.3410677171123,-12.0691554422604,
124.24505041029)) ;
#43014=CARTESIAN_POINT('Ctrl Pts',(-20.337719091561,-12.0689266956642,124.248780052448)) ;
#43015=CARTESIAN_POINT('Ctrl Pts',(-20.334271918944,-12.0686925060229,124.252573309059)) ;
#43016=CARTESIAN_POINT('Ctrl Pts',(-20.3341956945753,-12.0686873282287,
124.252657163172)) ;
#43017=CARTESIAN_POINT('Ctrl Pts',(-20.3339595696124,-12.0686712906362,
124.252916852313)) ;
#43018=CARTESIAN_POINT('Ctrl Pts',(-20.3337996301731,-12.0686604303742,
124.25309265221)) ;
#43019=CARTESIAN_POINT('Ctrl Pts',(-20.333492784064,-12.0686396001985,124.253429733652)) ;
#43020=CARTESIAN_POINT('Ctrl Pts',(-20.3333458853265,-12.0686296303806,
124.253591022336)) ;
#43021=CARTESIAN_POINT('Ctrl Pts',(-20.3330642130737,-12.0686105182027,
124.253900124131)) ;
#43022=CARTESIAN_POINT('Ctrl Pts',(-20.3329294463048,-12.0686013759237,
124.254047943343)) ;
#43023=CARTESIAN_POINT('Ctrl Pts',(-20.332671168294,-12.0685838587225,124.254331099572)) ;
#43024=CARTESIAN_POINT('Ctrl Pts',(-20.3325476627452,-12.0685754838667,
124.254466441818)) ;
#43025=CARTESIAN_POINT('Ctrl Pts',(-20.3323110779287,-12.0685594443458,
124.254725586322)) ;
#43026=CARTESIAN_POINT('Ctrl Pts',(-20.3321980034844,-12.0685517797371,
124.254849393011)) ;
#43027=CARTESIAN_POINT('Ctrl Pts',(-20.331981493834,-12.0685371065704,124.255086356494)) ;
#43028=CARTESIAN_POINT('Ctrl Pts',(-20.3318780627405,-12.0685300980628,
124.255199516989)) ;
#43029=CARTESIAN_POINT('Ctrl Pts',(-20.331680096091,-12.0685166860376,124.255416025672)) ;
#43030=CARTESIAN_POINT('Ctrl Pts',(-20.3315855639849,-12.0685102825614,
124.255519376997)) ;
#43031=CARTESIAN_POINT('Ctrl Pts',(-20.3314046954537,-12.0684980326301,
124.255717052638)) ;
#43032=CARTESIAN_POINT('Ctrl Pts',(-20.3313183618313,-12.0684921862032,
124.255811379699)) ;
#43033=CARTESIAN_POINT('Ctrl Pts',(-20.3311532334888,-12.0684810054224,
124.255991741332)) ;
#43034=CARTESIAN_POINT('Ctrl Pts',(-20.3310744412592,-12.0684756711016,
124.256077778053)) ;
#43035=CARTESIAN_POINT('Ctrl Pts',(-20.3309237821305,-12.0684654725984,
124.256242243189)) ;
#43036=CARTESIAN_POINT('Ctrl Pts',(-20.3308519172403,-12.0684606084385,
124.256320673486)) ;
#43037=CARTESIAN_POINT('Ctrl Pts',(-20.3307145406868,-12.0684513112035,
124.25647056202)) ;
#43038=CARTESIAN_POINT('Ctrl Pts',(-20.3306490307995,-12.068446878154,124.256542021725)) ;
#43039=CARTESIAN_POINT('Ctrl Pts',(-20.3305238328676,-12.068438406905,124.256678558643)) ;
#43040=CARTESIAN_POINT('Ctrl Pts',(-20.3304641462319,-12.0684343687219,
124.256743637161)) ;
#43041=CARTESIAN_POINT('Ctrl Pts',(-20.3303501020326,-12.0684266536365,
124.256867957267)) ;
#43042=CARTESIAN_POINT('Ctrl Pts',(-20.3302957456573,-12.0684229767488,
124.256927199926)) ;
#43043=CARTESIAN_POINT('Ctrl Pts',(-20.3301919066605,-12.068415953263,124.257040351455)) ;
#43044=CARTESIAN_POINT('Ctrl Pts',(-20.330142424839,-12.0684126066642,124.257094261423)) ;
#43045=CARTESIAN_POINT('Ctrl Pts',(-20.3275942274742,-12.0682402782955,
124.259870008572)) ;
#43046=CARTESIAN_POINT('Ctrl Pts',(-20.3250834654456,-12.0680711542442,
124.262580752766)) ;
#43047=CARTESIAN_POINT('Ctrl Pts',(-20.3198780452649,-12.0677218897207,
124.2681510398)) ;
#43048=CARTESIAN_POINT('Ctrl Pts',(-20.3171818495613,-12.0675417325455,
124.27100908913)) ;
#43049=CARTESIAN_POINT('Ctrl Pts',(-20.3108023467093,-12.0671172050382,
124.27770799624)) ;
#43050=CARTESIAN_POINT('Ctrl Pts',(-20.307107903323,-12.0668727084403,124.281538134576)) ;
#43051=CARTESIAN_POINT('Ctrl Pts',(-20.2943345101222,-12.066031994209,124.294612561432)) ;
#43052=CARTESIAN_POINT('Ctrl Pts',(-20.2851363904559,-12.0654344961369,
124.303739173765)) ;
#43053=CARTESIAN_POINT('Ctrl Pts',(-20.2574822667929,-12.0636620930152,
124.330337946274)) ;
#43054=CARTESIAN_POINT('Ctrl Pts',(-20.2386334803495,-12.0624846856754,
124.347392129637)) ;
#43055=CARTESIAN_POINT('Ctrl Pts',(-20.2119556078083,-12.0608669657171,
124.37008981392)) ;
#43056=CARTESIAN_POINT('Ctrl Pts',(-20.2045616104589,-12.0604234921339,
124.376235042615)) ;
#43057=CARTESIAN_POINT('Ctrl Pts',(-20.1924866005343,-12.0597072178838,
124.386037405299)) ;
#43058=CARTESIAN_POINT('Ctrl Pts',(-20.1878491418317,-12.0594339856606,
124.389747529939)) ;
#43059=CARTESIAN_POINT('Ctrl Pts',(-20.1794767341394,-12.0589439914911,
124.396348436506)) ;
#43060=CARTESIAN_POINT('Ctrl Pts',(-20.1757515128087,-12.0587271273454,
124.399251363141)) ;
#43061=CARTESIAN_POINT('Ctrl Pts',(-20.1683540435549,-12.0582987269334,
124.404948850542)) ;
#43062=CARTESIAN_POINT('Ctrl Pts',(-20.1646825945398,-12.05808718572,124.407744326043)) ;
#43063=CARTESIAN_POINT('Ctrl Pts',(-20.1608157665465,-12.0578654925939,
124.410654880582)) ;
#43064=CARTESIAN_POINT('Ctrl Pts',(-20.1606357528137,-12.0578551745396,
124.410790300384)) ;
#43065=CARTESIAN_POINT('Ctrl Pts',(-20.1602984200065,-12.0578358439238,
124.411043924606)) ;
#43066=CARTESIAN_POINT('Ctrl Pts',(-20.1601411095926,-12.0578268312673,
124.411162140563)) ;
#43067=CARTESIAN_POINT('Ctrl Pts',(-20.1598434801329,-12.0578097830254,
124.41138569382)) ;
#43068=CARTESIAN_POINT('Ctrl Pts',(-20.1597031667895,-12.0578017473767,
124.411491038747)) ;
#43069=CARTESIAN_POINT('Ctrl Pts',(-20.1594356387402,-12.057786429109,124.411691806296)) ;
#43070=CARTESIAN_POINT('Ctrl Pts',(-20.1593084281031,-12.0577791464533,
124.411787234111)) ;
#43071=CARTESIAN_POINT('Ctrl Pts',(-20.1590643237101,-12.0577651741489,
124.411970277687)) ;
#43072=CARTESIAN_POINT('Ctrl Pts',(-20.1589474327491,-12.0577584844668,
124.412057897273)) ;
#43073=CARTESIAN_POINT('Ctrl Pts',(-20.1587219056403,-12.057745579542,124.41222688703)) ;
#43074=CARTESIAN_POINT('Ctrl Pts',(-20.1586132717365,-12.0577393642849,
124.412308259894)) ;
#43075=CARTESIAN_POINT('Ctrl Pts',(-20.1584026835164,-12.0577273176757,
124.412465948699)) ;
#43076=CARTESIAN_POINT('Ctrl Pts',(-20.1583007306745,-12.0577214863002,
124.41254226684)) ;
#43077=CARTESIAN_POINT('Ctrl Pts',(-20.1581022696193,-12.057710136507,124.412690780155)) ;
#43078=CARTESIAN_POINT('Ctrl Pts',(-20.1580057625742,-12.0577046180735,
124.412762976991)) ;
#43079=CARTESIAN_POINT('Ctrl Pts',(-20.1578172025761,-12.0576938372846,
124.412903996033)) ;
#43080=CARTESIAN_POINT('Ctrl Pts',(-20.1577251505985,-12.0576885749206,
124.41297281948)) ;
#43081=CARTESIAN_POINT('Ctrl Pts',(-20.1575446897698,-12.0576782597237,
124.413107703761)) ;
#43082=CARTESIAN_POINT('Ctrl Pts',(-20.157456281808,-12.0576732068914,124.413173765474)) ;
#43083=CARTESIAN_POINT('Ctrl Pts',(-20.1572824323929,-12.0576632719408,
124.413303636337)) ;
#43084=CARTESIAN_POINT('Ctrl Pts',(-20.1571969916154,-12.0576583898217,
124.413367446194)) ;
#43085=CARTESIAN_POINT('Ctrl Pts',(-20.1570285018939,-12.057648763346,124.413493246027)) ;
#43086=CARTESIAN_POINT('Ctrl Pts',(-20.1569454531689,-12.0576440189712,
124.413555236787)) ;
#43087=CARTESIAN_POINT('Ctrl Pts',(-20.1567812503429,-12.0576346394902,
124.413677772291)) ;
#43088=CARTESIAN_POINT('Ctrl Pts',(-20.1567000966792,-12.0576300043853,
124.41373831744)) ;
#43089=CARTESIAN_POINT('Ctrl Pts',(-20.1565392466497,-12.0576208183974,
124.413858290094)) ;
#43090=CARTESIAN_POINT('Ctrl Pts',(-20.156459550551,-12.0576162675118,124.413917717952)) ;
#43091=CARTESIAN_POINT('Ctrl Pts',(-20.1563012245518,-12.0576072275777,
124.414035749237)) ;
#43092=CARTESIAN_POINT('Ctrl Pts',(-20.156222594731,-12.0576027385209,124.414094353002)) ;
#43093=CARTESIAN_POINT('Ctrl Pts',(-20.1560660452786,-12.0575938018824,
124.414211002567)) ;
#43094=CARTESIAN_POINT('Ctrl Pts',(-20.1559881258435,-12.0575893543035,
124.414269048484)) ;
#43095=CARTESIAN_POINT('Ctrl Pts',(-20.1558326679136,-12.0575804818033,
124.414384828354)) ;
#43096=CARTESIAN_POINT('Ctrl Pts',(-20.1557551293923,-12.0575760568759,
124.414442562469)) ;
#43097=CARTESIAN_POINT('Ctrl Pts',(-20.1556001235508,-12.0575672119902,
124.414557949737)) ;
#43098=CARTESIAN_POINT('Ctrl Pts',(-20.1555226562434,-12.0575627920317,
124.41461560291)) ;
#43099=CARTESIAN_POINT('Ctrl Pts',(-20.1553674967905,-12.0575539401913,
124.414731048651)) ;
#43100=CARTESIAN_POINT('Ctrl Pts',(-20.1552898045009,-12.0575495083037,
124.414788841249)) ;
#43101=CARTESIAN_POINT('Ctrl Pts',(-20.1551339073804,-12.0575406162019,
124.414904779572)) ;
#43102=CARTESIAN_POINT('Ctrl Pts',(-20.155055702674,-12.0575361560007,124.414962925023)) ;
#43103=CARTESIAN_POINT('Ctrl Pts',(-20.1548984973455,-12.0575271911289,
124.415079779147)) ;
#43104=CARTESIAN_POINT('Ctrl Pts',(-20.1548194964674,-12.0575226864529,
124.415138487725)) ;
#43105=CARTESIAN_POINT('Ctrl Pts',(-20.1546604153098,-12.057513616496,124.415256677862)) ;
#43106=CARTESIAN_POINT('Ctrl Pts',(-20.1545803348686,-12.0575090512186,
124.415316159148)) ;
#43107=CARTESIAN_POINT('Ctrl Pts',(-20.1544188072179,-12.0574998437157,
124.415436106912)) ;
#43108=CARTESIAN_POINT('Ctrl Pts',(-20.1543373597396,-12.0574952014913,
124.415496573083)) ;
#43109=CARTESIAN_POINT('Ctrl Pts',(-20.1541728031628,-12.0574858233395,
124.415618707936)) ;
#43110=CARTESIAN_POINT('Ctrl Pts',(-20.1540896936947,-12.0574810874112,
124.415680376264)) ;
#43111=CARTESIAN_POINT('Ctrl Pts',(-20.1539215070125,-12.0574715044696,
124.415805140628)) ;
#43112=CARTESIAN_POINT('Ctrl Pts',(-20.1538364294899,-12.0574666574632,
124.415868236134)) ;
#43113=CARTESIAN_POINT('Ctrl Pts',(-20.1536639857806,-12.0574568341573,
124.415996090502)) ;
#43114=CARTESIAN_POINT('Ctrl Pts',(-20.1535766191235,-12.0574518578602,
124.416060848806)) ;
#43115=CARTESIAN_POINT('Ctrl Pts',(-20.1533992573629,-12.0574417567091,
124.416192277825)) ;
#43116=CARTESIAN_POINT('Ctrl Pts',(-20.1533092619858,-12.0574366318741,
124.41625894767)) ;
#43117=CARTESIAN_POINT('Ctrl Pts',(-20.1531262805519,-12.057426213125,124.416394464812)) ;
#43118=CARTESIAN_POINT('Ctrl Pts',(-20.1530332937176,-12.0574209192072,
124.416463311428)) ;
#43119=CARTESIAN_POINT('Ctrl Pts',(-20.1528439398439,-12.0574101402404,
124.416603466635)) ;
#43120=CARTESIAN_POINT('Ctrl Pts',(-20.1527475721204,-12.0574046551997,
124.416674774262)) ;
#43121=CARTESIAN_POINT('Ctrl Pts',(-20.152551034916,-12.0573934701379,124.416820158891)) ;
#43122=CARTESIAN_POINT('Ctrl Pts',(-20.1524508647029,-12.0573877701304,
124.416894234717)) ;
#43123=CARTESIAN_POINT('Ctrl Pts',(-20.1522462639951,-12.0573761292124,
124.417045489537)) ;
#43124=CARTESIAN_POINT('Ctrl Pts',(-20.1521418324939,-12.057370188309,124.417122667273)) ;
#43125=CARTESIAN_POINT('Ctrl Pts',(-20.1519282076745,-12.0573580372646,
124.417280490394)) ;
#43126=CARTESIAN_POINT('Ctrl Pts',(-20.1518190132248,-12.0573518271342,
124.417361134281)) ;
#43127=CARTESIAN_POINT('Ctrl Pts',(-20.1515953113498,-12.0573391065198,
124.417526289564)) ;
#43128=CARTESIAN_POINT('Ctrl Pts',(-20.1514808026935,-12.0573325960531,
124.417610799143)) ;
#43129=CARTESIAN_POINT('Ctrl Pts',(-20.1512458645269,-12.0573192404725,
124.417784126035)) ;
#43130=CARTESIAN_POINT('Ctrl Pts',(-20.1511254334448,-12.0573123953713,
124.41787294132)) ;
#43131=CARTESIAN_POINT('Ctrl Pts',(-20.150877977331,-12.057298332577,124.418055366191)) ;
#43132=CARTESIAN_POINT('Ctrl Pts',(-20.150750950563,-12.0572911149049,124.41814897332)) ;
#43133=CARTESIAN_POINT('Ctrl Pts',(-20.150489555502,-12.0572762648578,124.418341521251)) ;
#43134=CARTESIAN_POINT('Ctrl Pts',(-20.1503551850694,-12.0572686325019,
124.418440459237)) ;
#43135=CARTESIAN_POINT('Ctrl Pts',(-20.1500782699442,-12.0572529062177,
124.418644268482)) ;
#43136=CARTESIAN_POINT('Ctrl Pts',(-20.1499357226919,-12.0572448123094,
124.41874913645)) ;
#43137=CARTESIAN_POINT('Ctrl Pts',(-20.1496415237164,-12.0572281106098,
124.418965474014)) ;
#43138=CARTESIAN_POINT('Ctrl Pts',(-20.1494898692096,-12.0572195028557,
124.419076939539)) ;
#43139=CARTESIAN_POINT('Ctrl Pts',(-20.1443685394988,-12.0569288782317,
124.422839317504)) ;
#43140=CARTESIAN_POINT('Ctrl Pts',(-20.1393719328144,-12.0566471386495,
124.426453445166)) ;
#43141=CARTESIAN_POINT('Ctrl Pts',(-20.1255185054637,-12.055870715307,124.436318536948)) ;
#43142=CARTESIAN_POINT('Ctrl Pts',(-20.1166067945575,-12.0553765247343,
124.442491491923)) ;
#43143=CARTESIAN_POINT('Ctrl Pts',(-20.0914470099835,-12.0539941350989,
124.459439124179)) ;
#43144=CARTESIAN_POINT('Ctrl Pts',(-20.0750255514472,-12.0531066090487,
124.469950736286)) ;
#43145=CARTESIAN_POINT('Ctrl Pts',(-20.0525191720812,-12.0519027342167,
124.483625996374)) ;
#43146=CARTESIAN_POINT('Ctrl Pts',(-20.0466442997958,-12.0515896710104,
124.487129967897)) ;
#43147=CARTESIAN_POINT('Ctrl Pts',(-20.032676899066,-12.0508483209912,124.495305915879)) ;
#43148=CARTESIAN_POINT('Ctrl Pts',(-20.0245601602005,-12.0504198260218,
124.499935720589)) ;
#43149=CARTESIAN_POINT('Ctrl Pts',(-20.0044213265263,-12.0493626881266,
124.511125562891)) ;
#43150=CARTESIAN_POINT('Ctrl Pts',(-19.99234186859,-12.0487338290955,124.517579870373)) ;
#43151=CARTESIAN_POINT('Ctrl Pts',(-19.9652252818033,-12.0473342758816,
124.531500928543)) ;
#43152=CARTESIAN_POINT('Ctrl Pts',(-19.9501388118741,-12.0465637667119,
124.538865889378)) ;
#43153=CARTESIAN_POINT('Ctrl Pts',(-19.9252376540814,-12.0453053509998,
124.550407052698)) ;
#43154=CARTESIAN_POINT('Ctrl Pts',(-19.9155097758157,-12.0448169927548,
124.554765446727)) ;
#43155=CARTESIAN_POINT('Ctrl Pts',(-19.8946295993106,-12.0437755254986,
124.563801543125)) ;
#43156=CARTESIAN_POINT('Ctrl Pts',(-19.8834627402678,-12.0432225964147,
124.568442911964)) ;
#43157=CARTESIAN_POINT('Ctrl Pts',(-19.8591075566196,-12.0420248983349,
124.578153839921)) ;
#43158=CARTESIAN_POINT('Ctrl Pts',(-19.8458970696197,-12.0413804432317,
124.583163306072)) ;
#43159=CARTESIAN_POINT('Ctrl Pts',(-19.8158088678918,-12.0399210477339,
124.593993120661)) ;
#43160=CARTESIAN_POINT('Ctrl Pts',(-19.7988857140135,-12.0391060622872,
124.599677984354)) ;
#43161=CARTESIAN_POINT('Ctrl Pts',(-19.7740746841145,-12.037916823148,124.607425284482)) ;
#43162=CARTESIAN_POINT('Ctrl Pts',(-19.7662791928372,-12.037543982045,124.609776104457)) ;
#43163=CARTESIAN_POINT('Ctrl Pts',(-19.7511429703411,-12.0368214058152,
124.614179740467)) ;
#43164=CARTESIAN_POINT('Ctrl Pts',(-19.7438053291909,-12.0364717322552,
124.616241907134)) ;
#43165=CARTESIAN_POINT('Ctrl Pts',(-19.7285968277276,-12.0357481327927,
124.620366393384)) ;
#43166=CARTESIAN_POINT('Ctrl Pts',(-19.7207237653236,-12.0353741796058,
124.622419232244)) ;
#43167=CARTESIAN_POINT('Ctrl Pts',(-19.7001251584904,-12.0343974086205,
124.627575913835)) ;
#43168=CARTESIAN_POINT('Ctrl Pts',(-19.6873698948791,-12.0337941495709,
124.630556854992)) ;
#43169=CARTESIAN_POINT('Ctrl Pts',(-19.6501716827793,-12.032040031368,124.638635797085)) ;
#43170=CARTESIAN_POINT('Ctrl Pts',(-19.6256197994497,-12.0308890095939,
124.64320265141)) ;
#43171=CARTESIAN_POINT('Ctrl Pts',(-19.5931551337363,-12.0293793022699,
124.648240370936)) ;
#43172=CARTESIAN_POINT('Ctrl Pts',(-19.585351408933,-12.0290172890477,124.649375803324)) ;
#43173=CARTESIAN_POINT('Ctrl Pts',(-19.5718896897063,-12.0283942530006,
124.651204559206)) ;
#43174=CARTESIAN_POINT('Ctrl Pts',(-19.566236744264,-12.0281330610235,124.651933162974)) ;
#43175=CARTESIAN_POINT('Ctrl Pts',(-19.5523692417059,-12.0274933054995,
124.653624194782)) ;
#43176=CARTESIAN_POINT('Ctrl Pts',(-19.5441497319452,-12.0271149612263,
124.654543807795)) ;
#43177=CARTESIAN_POINT('Ctrl Pts',(-19.5246868080321,-12.0262206937252,
124.656525983081)) ;
#43178=CARTESIAN_POINT('Ctrl Pts',(-19.5134369276591,-12.0257050709966,
124.657517882401)) ;
#43179=CARTESIAN_POINT('Ctrl Pts',(-19.4853015009001,-12.0244171121581,
124.659614772145)) ;
#43180=CARTESIAN_POINT('Ctrl Pts',(-19.4684041245786,-12.0236450813739,
124.660529593175)) ;
#43181=CARTESIAN_POINT('Ctrl Pts',(-19.4466484370546,-12.0226489006946,
124.661264854053)) ;
#43182=CARTESIAN_POINT('Ctrl Pts',(-19.4418025291007,-12.022426842339,124.661400410368)) ;
#43183=CARTESIAN_POINT('Ctrl Pts',(-19.4307285636967,-12.0219190179987,
124.661645725414)) ;
#43184=CARTESIAN_POINT('Ctrl Pts',(-19.4245002340791,-12.021633153557,124.661737127126)) ;
#43185=CARTESIAN_POINT('Ctrl Pts',(-19.4090200919699,-12.0209222484223,
124.661848577842)) ;
#43186=CARTESIAN_POINT('Ctrl Pts',(-19.3997682456536,-12.0204970125023,
124.661812473261)) ;
#43187=CARTESIAN_POINT('Ctrl Pts',(-19.3687712433552,-12.0190718561693,
124.661347352535)) ;
#43188=CARTESIAN_POINT('Ctrl Pts',(-19.3470369751362,-12.0180719687089,
124.660453542271)) ;
#43189=CARTESIAN_POINT('Ctrl Pts',(-19.3172112971142,-12.0167006665855,
124.658446273279)) ;
#43190=CARTESIAN_POINT('Ctrl Pts',(-19.3090910499798,-12.0163273817509,
124.657820007713)) ;
#43191=CARTESIAN_POINT('Ctrl Pts',(-19.2923975866369,-12.0155600723983,
124.656368297838)) ;
#43192=CARTESIAN_POINT('Ctrl Pts',(-19.2838256084633,-12.0151661101584,
124.65553351323)) ;
#43193=CARTESIAN_POINT('Ctrl Pts',(-19.2703192963284,-12.0145453108416,
124.654077142413)) ;
#43194=CARTESIAN_POINT('Ctrl Pts',(-19.2653788878238,-12.0143182181916,
124.653514583271)) ;
#43195=CARTESIAN_POINT('Ctrl Pts',(-19.2538264463011,-12.0137871040584,
124.652129246321)) ;
#43196=CARTESIAN_POINT('Ctrl Pts',(-19.2472173711565,-12.0134831886539,
124.65128304931)) ;
#43197=CARTESIAN_POINT('Ctrl Pts',(-19.2191352127577,-12.0121912127168,
124.647459082904)) ;
#43198=CARTESIAN_POINT('Ctrl Pts',(-19.1977348075048,-12.0112052787082,
124.643975828618)) ;
#43199=CARTESIAN_POINT('Ctrl Pts',(-19.1647917789404,-12.0096765760457,
124.637730254132)) ;
#43200=CARTESIAN_POINT('Ctrl Pts',(-19.1531797584936,-12.0091356193974,
124.635357213597)) ;
#43201=CARTESIAN_POINT('Ctrl Pts',(-19.1355291313851,-12.0083092609858,
124.631487839693)) ;
#43202=CARTESIAN_POINT('Ctrl Pts',(-19.1294650249487,-12.0080246193139,
124.630110961285)) ;
#43203=CARTESIAN_POINT('Ctrl Pts',(-19.1181604698532,-12.0074925317238,
124.627455363806)) ;
#43204=CARTESIAN_POINT('Ctrl Pts',(-19.1129175323337,-12.0072451636844,
124.626187860992)) ;
#43205=CARTESIAN_POINT('Ctrl Pts',(-19.1022175780253,-12.0067390810999,
124.623527679998)) ;
#43206=CARTESIAN_POINT('Ctrl Pts',(-19.0967614396839,-12.0064803529673,
124.622131977315)) ;
#43207=CARTESIAN_POINT('Ctrl Pts',(-19.0836511005747,-12.005857049312,124.618683735493)) ;
#43208=CARTESIAN_POINT('Ctrl Pts',(-19.0760066315201,-12.0054922749296,
124.616595190539)) ;
#43209=CARTESIAN_POINT('Ctrl Pts',(-19.0526500235282,-12.0043737799839,
124.609974621791)) ;
#43210=CARTESIAN_POINT('Ctrl Pts',(-19.0370065431197,-12.0036190387041,
124.6052068633)) ;
#43211=CARTESIAN_POINT('Ctrl Pts',(-19.0087145905505,-12.002245856984,124.595973710673)) ;
#43212=CARTESIAN_POINT('Ctrl Pts',(-18.9960357541656,-12.0016275452273,
124.591609006089)) ;
#43213=CARTESIAN_POINT('Ctrl Pts',(-18.9765469245285,-12.0006731551457,
124.584547241213)) ;
#43214=CARTESIAN_POINT('Ctrl Pts',(-18.9696863143,-12.0003364032899,124.581992903515)) ;
#43215=CARTESIAN_POINT('Ctrl Pts',(-18.9628485243969,-11.9999999855698,
124.579378441824)) ;
#43216=CARTESIAN_POINT('',(-20.654497037415,-12.,123.302657626506)) ;
#43217=CARTESIAN_POINT('Origin',(-19.4092722359532,-12.,123.411814366564)) ;
#43218=CARTESIAN_POINT('',(-20.591904925275,-11.7,123.006993514553)) ;
#43219=CARTESIAN_POINT('Ctrl Pts',(-20.591904925275,-11.7,123.006993514553)) ;
#43220=CARTESIAN_POINT('Ctrl Pts',(-20.6041551258135,-11.7,123.042780919119)) ;
#43221=CARTESIAN_POINT('Ctrl Pts',(-20.6154021887201,-11.7075896772134,
123.081471444624)) ;
#43222=CARTESIAN_POINT('Ctrl Pts',(-20.6328682032119,-11.7382522587826,
123.15357258444)) ;
#43223=CARTESIAN_POINT('Ctrl Pts',(-20.6391780918807,-11.761317155029,123.186964545377)) ;
#43224=CARTESIAN_POINT('Ctrl Pts',(-20.6477244677879,-11.8144220247009,
123.24016910469)) ;
#43225=CARTESIAN_POINT('Ctrl Pts',(-20.6505510417636,-11.8480564696762,
123.263577766805)) ;
#43226=CARTESIAN_POINT('Ctrl Pts',(-20.6538866180434,-11.9219235159019,
123.294843389787)) ;
#43227=CARTESIAN_POINT('Ctrl Pts',(-20.654497037415,-11.9621695797156,123.302657626506)) ;
#43228=CARTESIAN_POINT('Ctrl Pts',(-20.654497037415,-12.,123.302657626506)) ;
#43229=CARTESIAN_POINT('',(-20.4601832664426,-12.,122.734993854115)) ;
#43230=CARTESIAN_POINT('Ctrl Pts',(-20.4601832664426,-12.,122.734993854115)) ;
#43231=CARTESIAN_POINT('Ctrl Pts',(-20.4601832664426,-11.9621695923928,
122.734993854115)) ;
#43232=CARTESIAN_POINT('Ctrl Pts',(-20.464489460108,-11.9219235188397,122.741542946412)) ;
#43233=CARTESIAN_POINT('Ctrl Pts',(-20.4810132149992,-11.8480564142548,
122.76829402158)) ;
#43234=CARTESIAN_POINT('Ctrl Pts',(-20.4931244558124,-11.8144219229966,
122.788524394775)) ;
#43235=CARTESIAN_POINT('Ctrl Pts',(-20.5189747646632,-11.7613170365764,
122.835805557673)) ;
#43236=CARTESIAN_POINT('Ctrl Pts',(-20.5344511925933,-11.7382521626639,
122.86605964457)) ;
#43237=CARTESIAN_POINT('Ctrl Pts',(-20.5648328354891,-11.7075896412594,
122.933739475197)) ;
#43238=CARTESIAN_POINT('Ctrl Pts',(-20.5796547571477,-11.7,122.971206204672)) ;
#43239=CARTESIAN_POINT('Ctrl Pts',(-20.591904925275,-11.7,123.006993514553)) ;
#43240=CARTESIAN_POINT('',(-18.1640505668151,-12.,123.521006833268)) ;
#43241=CARTESIAN_POINT('Origin',(-19.4092722359532,-12.,123.411814366564)) ;
#43242=CARTESIAN_POINT('Ctrl Pts',(-18.2266423653438,-11.7000000011364,
123.816643452992)) ;
#43243=CARTESIAN_POINT('Ctrl Pts',(-18.2143944061214,-11.700003292843,123.780863409226)) ;
#43244=CARTESIAN_POINT('Ctrl Pts',(-18.2031495305491,-11.7075931690383,
123.742182778096)) ;
#43245=CARTESIAN_POINT('Ctrl Pts',(-18.1856835511285,-11.7382521626639,
123.670090636116)) ;
#43246=CARTESIAN_POINT('Ctrl Pts',(-18.1793727421957,-11.7613170365764,
123.636698971197)) ;
#43247=CARTESIAN_POINT('Ctrl Pts',(-18.1708248842569,-11.8144219229966,
123.583494827023)) ;
#43248=CARTESIAN_POINT('Ctrl Pts',(-18.1679976569785,-11.8480564142548,
123.560086346945)) ;
#43249=CARTESIAN_POINT('Ctrl Pts',(-18.1646612055237,-11.9219235188397,
123.528820989278)) ;
#43250=CARTESIAN_POINT('Ctrl Pts',(-18.1640505668151,-11.9621695923928,
123.521006833268)) ;
#43251=CARTESIAN_POINT('Ctrl Pts',(-18.1640505668151,-12.,123.521006833268)) ;
#43252=CARTESIAN_POINT('',(-18.2266423654683,-13.9601742359176,123.816643453356)) ;
#43253=CARTESIAN_POINT('Ctrl Pts',(-18.2740109056134,-10.1799890803629,
123.800437437226)) ;
#43254=CARTESIAN_POINT('Ctrl Pts',(-17.9901976317162,-10.,123.897592500161)) ;
#43255=CARTESIAN_POINT('Ctrl Pts',(-18.3189528014318,-10.186615931181,123.93177221557)) ;
#43256=CARTESIAN_POINT('Ctrl Pts',(-18.0463587734884,-10.0066268508181,
124.061733136808)) ;
#43257=CARTESIAN_POINT('Ctrl Pts',(-18.4544999825326,-10.199846557662,124.178242251159)) ;
#43258=CARTESIAN_POINT('Ctrl Pts',(-18.2158202083151,-10.0198574772991,
124.369865791197)) ;
#43259=CARTESIAN_POINT('Ctrl Pts',(-18.7737258963307,-10.2198221789206,
124.458448669119)) ;
#43260=CARTESIAN_POINT('Ctrl Pts',(-18.6148367045085,-10.0398330985578,
124.72010058675)) ;
#43261=CARTESIAN_POINT('Ctrl Pts',(-19.1683517049307,-10.2397395138226,
124.612076715426)) ;
#43262=CARTESIAN_POINT('Ctrl Pts',(-19.1081207670208,-10.0597504334597,
124.912141899864)) ;
#43263=CARTESIAN_POINT('Ctrl Pts',(-19.5908221387894,-10.2596127905386,
124.622761896565)) ;
#43264=CARTESIAN_POINT('Ctrl Pts',(-19.636206114934,-10.0796237101757,124.92549851548)) ;
#43265=CARTESIAN_POINT('Ctrl Pts',(-19.9944586595383,-10.2796372807025,
124.487357143018)) ;
#43266=CARTESIAN_POINT('Ctrl Pts',(-20.1407529320189,-10.0996482003397,
124.756244590335)) ;
#43267=CARTESIAN_POINT('Ctrl Pts',(-20.3250726893908,-10.2995051218533,
124.224284503461)) ;
#43268=CARTESIAN_POINT('Ctrl Pts',(-20.5540202995955,-10.1195160414904,
124.427406225433)) ;
#43269=CARTESIAN_POINT('Ctrl Pts',(-20.5474404603406,-10.3194507727328,
123.863209826147)) ;
#43270=CARTESIAN_POINT('Ctrl Pts',(-20.8319818407582,-10.1394616923699,
123.976064807431)) ;
#43271=CARTESIAN_POINT('Ctrl Pts',(-20.6329204930996,-10.3393561733498,
123.448689022605)) ;
#43272=CARTESIAN_POINT('Ctrl Pts',(-20.9388342400949,-10.1593670929869,
123.457915382835)) ;
#43273=CARTESIAN_POINT('Ctrl Pts',(-20.5727382583942,-10.3592304011661,
123.030414178423)) ;
#43274=CARTESIAN_POINT('Ctrl Pts',(-20.8636098402301,-10.1792413208033,
122.935072644727)) ;
#43275=CARTESIAN_POINT('Ctrl Pts',(-20.3723372035374,-10.3792161920437,
122.655670923463)) ;
#43276=CARTESIAN_POINT('Ctrl Pts',(-20.6131115834081,-10.1992271116809,
122.466642059227)) ;
#43277=CARTESIAN_POINT('Ctrl Pts',(-20.0574028124706,-10.3991104347035,
122.373313004285)) ;
#43278=CARTESIAN_POINT('Ctrl Pts',(-20.219446657189,-10.2191213543406,122.11369274935)) ;
#43279=CARTESIAN_POINT('Ctrl Pts',(-19.6656681691958,-10.4189891507756,
122.214436559376)) ;
#43280=CARTESIAN_POINT('Ctrl Pts',(-19.729780773993,-10.2390000704127,121.915093775378)) ;
#43281=CARTESIAN_POINT('Ctrl Pts',(-19.2398981074651,-10.4390286006202,
122.199163423108)) ;
#43282=CARTESIAN_POINT('Ctrl Pts',(-19.1975679684769,-10.2590395202573,
121.895998337816)) ;
#43283=CARTESIAN_POINT('Ctrl Pts',(-18.8378689724914,-10.458891762158,122.328984896592)) ;
#43284=CARTESIAN_POINT('Ctrl Pts',(-18.6950312339923,-10.2789026817952,
122.058270950238)) ;
#43285=CARTESIAN_POINT('Ctrl Pts',(-18.5023795521869,-10.4788711301723,
122.589370841986)) ;
#43286=CARTESIAN_POINT('Ctrl Pts',(-18.2756669291778,-10.2988820498094,
122.383749835563)) ;
#43287=CARTESIAN_POINT('Ctrl Pts',(-18.2772917542457,-10.4986817106951,
122.945518138246)) ;
#43288=CARTESIAN_POINT('Ctrl Pts',(-17.9943038605785,-10.3186926303322,
122.828930487561)) ;
#43289=CARTESIAN_POINT('Ctrl Pts',(-18.1858955375249,-10.5186626389807,
123.360335745372)) ;
#43290=CARTESIAN_POINT('Ctrl Pts',(-17.8800540061898,-10.3386735586178,
123.347451469643)) ;
#43291=CARTESIAN_POINT('Ctrl Pts',(-18.2415877544767,-10.5385553108501,
123.779674054783)) ;
#43292=CARTESIAN_POINT('Ctrl Pts',(-17.949663613675,-10.3585662304872,123.871624239523)) ;
#43293=CARTESIAN_POINT('Ctrl Pts',(-18.4366892236376,-10.5584816411372,
124.155765874511)) ;
#43294=CARTESIAN_POINT('Ctrl Pts',(-18.1935384904851,-10.3784925607743,
124.34174209524)) ;
#43295=CARTESIAN_POINT('Ctrl Pts',(-18.7493758900079,-10.5784521952295,
124.443056780365)) ;
#43296=CARTESIAN_POINT('Ctrl Pts',(-18.5843830566034,-10.3984631148666,
124.700856014279)) ;
#43297=CARTESIAN_POINT('Ctrl Pts',(-19.0736750036282,-10.5949840343171,
124.578605622473)) ;
#43298=CARTESIAN_POINT('Ctrl Pts',(-18.9897866675992,-10.4149949539542,
124.870306748339)) ;
#43299=CARTESIAN_POINT('Ctrl Pts',(-19.3515822133367,-10.6083237731447,
124.616534422033)) ;
#43300=CARTESIAN_POINT('Ctrl Pts',(-19.3371420473607,-10.4283346927818,
124.917711789777)) ;
#43301=CARTESIAN_POINT('Ctrl Pts',(-19.5623087353055,-10.6183560153633,
124.608012512987)) ;
#43302=CARTESIAN_POINT('Ctrl Pts',(-19.6005562667331,-10.4383669350004,
124.907063768782)) ;
#43303=CARTESIAN_POINT('Ctrl Pts',(-19.7648570829155,-10.6282137160067,
124.564122231623)) ;
#43304=CARTESIAN_POINT('Ctrl Pts',(-19.8537397870735,-10.4482246356439,
124.852203726746)) ;
#43305=CARTESIAN_POINT('Ctrl Pts',(-19.9594412369529,-10.638205580646,124.485025335786)) ;
#43306=CARTESIAN_POINT('Ctrl Pts',(-20.0969735539785,-10.4582165002831,
124.753332920083)) ;
#43307=CARTESIAN_POINT('Ctrl Pts',(-20.1360906792147,-10.6481281304061,
124.374071893985)) ;
#43308=CARTESIAN_POINT('Ctrl Pts',(-20.3177787346395,-10.4681390500432,
124.614652183365)) ;
#43309=CARTESIAN_POINT('Ctrl Pts',(-20.3435921685771,-10.6614059038996,
124.187345412144)) ;
#43310=CARTESIAN_POINT('Ctrl Pts',(-20.5771970981362,-10.4814168235367,
124.381203458891)) ;
#43311=CARTESIAN_POINT('Ctrl Pts',(-20.4979359412099,-10.6747532428402,
123.949230531229)) ;
#43312=CARTESIAN_POINT('Ctrl Pts',(-20.7701003708174,-10.4947641624773,
124.083584310457)) ;
#43313=CARTESIAN_POINT('Ctrl Pts',(-20.5838202221108,-10.6879604746334,
123.685128933396)) ;
#43314=CARTESIAN_POINT('Ctrl Pts',(-20.8774553693723,-10.5079713942705,
123.753475217054)) ;
#43315=CARTESIAN_POINT('Ctrl Pts',(-20.6134756841563,-10.6979475907231,
123.477310674119)) ;
#43316=CARTESIAN_POINT('Ctrl Pts',(-20.9145282391216,-10.5179585103602,
123.493699384276)) ;
#43317=CARTESIAN_POINT('Ctrl Pts',(-20.6067552821165,-10.7078984963028,
123.26817900999)) ;
#43318=CARTESIAN_POINT('Ctrl Pts',(-20.9061303769722,-10.52790941594,123.232285620267)) ;
#43319=CARTESIAN_POINT('Ctrl Pts',(-20.5631517199141,-10.7179535983103,
123.061365279476)) ;
#43320=CARTESIAN_POINT('Ctrl Pts',(-20.8516285272166,-10.5379645179474,
122.973767430347)) ;
#43321=CARTESIAN_POINT('Ctrl Pts',(-20.4864480135789,-10.7277752716314,
122.869632358223)) ;
#43322=CARTESIAN_POINT('Ctrl Pts',(-20.755752145473,-10.5477861912685,122.734100762332)) ;
#43323=CARTESIAN_POINT('Ctrl Pts',(-20.3753148949047,-10.7378337427063,
122.689756073264)) ;
#43324=CARTESIAN_POINT('Ctrl Pts',(-20.6168357130529,-10.5578446623434,
122.509252277714)) ;
#43325=CARTESIAN_POINT('Ctrl Pts',(-20.2362698429268,-10.7477583538828,
122.534165638144)) ;
#43326=CARTESIAN_POINT('Ctrl Pts',(-20.4430403513938,-10.5677692735199,
122.314768071456)) ;
#43327=CARTESIAN_POINT('Ctrl Pts',(-20.0174236370264,-10.7610356927832,
122.360928612314)) ;
#43328=CARTESIAN_POINT('Ctrl Pts',(-20.1694406712993,-10.5810466124203,
122.098190251904)) ;
#43329=CARTESIAN_POINT('Ctrl Pts',(-19.7578453903065,-10.7743345720208,
122.248851511266)) ;
#43330=CARTESIAN_POINT('Ctrl Pts',(-19.8449850134819,-10.5943454916579,
121.958111265335)) ;
#43331=CARTESIAN_POINT('Ctrl Pts',(-19.4824813143237,-10.7875734441915,
122.208088439905)) ;
#43332=CARTESIAN_POINT('Ctrl Pts',(-19.5008057716341,-10.6075843638286,
121.907157355648)) ;
#43333=CARTESIAN_POINT('Ctrl Pts',(-19.2721785775522,-10.7975800623281,
122.213521358078)) ;
#43334=CARTESIAN_POINT('Ctrl Pts',(-19.2379220825872,-10.6175909819652,
121.913944971404)) ;
#43335=CARTESIAN_POINT('Ctrl Pts',(-19.0656000898289,-10.8076110073896,
122.255887753777)) ;
#43336=CARTESIAN_POINT('Ctrl Pts',(-18.9796997397484,-10.6276219270267,
121.966900411424)) ;
#43337=CARTESIAN_POINT('Ctrl Pts',(-18.8727746571245,-10.8174671807414,
122.33177975615)) ;
#43338=CARTESIAN_POINT('Ctrl Pts',(-18.7386663423424,-10.6374781003785,
122.061762842601)) ;
#43339=CARTESIAN_POINT('Ctrl Pts',(-18.6933942950045,-10.8274664517043,
122.441317819794)) ;
#43340=CARTESIAN_POINT('Ctrl Pts',(-18.5144394578762,-10.6474773713414,
122.198683103417)) ;
#43341=CARTESIAN_POINT('Ctrl Pts',(-18.5371942685893,-10.8373609034616,
122.578747643145)) ;
#43342=CARTESIAN_POINT('Ctrl Pts',(-18.3191873796767,-10.6573718230987,
122.370468477432)) ;
#43343=CARTESIAN_POINT('Ctrl Pts',(-18.4051122896899,-10.847424219271,122.743966469464)) ;
#43344=CARTESIAN_POINT('Ctrl Pts',(-18.1540827677519,-10.6674351389081,
122.576990252266)) ;
#43345=CARTESIAN_POINT('Ctrl Pts',(-18.3057391169289,-10.8572630760106,
122.925417587621)) ;
#43346=CARTESIAN_POINT('Ctrl Pts',(-18.0298636947034,-10.6772739956477,
122.80380319062)) ;
#43347=CARTESIAN_POINT('Ctrl Pts',(-18.2376490708675,-10.8673291978282,
123.125750203822)) ;
#43348=CARTESIAN_POINT('Ctrl Pts',(-17.9447485718205,-10.6873401174653,
123.054218033102)) ;
#43349=CARTESIAN_POINT('Ctrl Pts',(-18.2060503452321,-10.8772124255524,
123.331137906529)) ;
#43350=CARTESIAN_POINT('Ctrl Pts',(-17.9052474071487,-10.6972233451896,
123.310952604467)) ;
#43351=CARTESIAN_POINT('Ctrl Pts',(-18.2101816179164,-10.8872018868312,
123.541086163132)) ;
#43352=CARTESIAN_POINT('Ctrl Pts',(-17.9104088183902,-10.7072128064683,
123.573388107812)) ;
#43353=CARTESIAN_POINT('Ctrl Pts',(-18.2506800550467,-10.8971655972577,
123.746612755988)) ;
#43354=CARTESIAN_POINT('Ctrl Pts',(-17.9610292610865,-10.7171765168948,
123.830297049982)) ;
#43355=CARTESIAN_POINT('Ctrl Pts',(-18.3262823417106,-10.9071605999886,
123.942684202324)) ;
#43356=CARTESIAN_POINT('Ctrl Pts',(-18.055529675207,-10.7271715196257,124.075387412779)) ;
#43357=CARTESIAN_POINT('Ctrl Pts',(-18.4354992661144,-10.9171969309989,
124.123200848044)) ;
#43358=CARTESIAN_POINT('Ctrl Pts',(-18.1920485023394,-10.737207850636,124.30103460394)) ;
#43359=CARTESIAN_POINT('Ctrl Pts',(-18.5715282260324,-10.9270431603412,
124.279245467908)) ;
#43360=CARTESIAN_POINT('Ctrl Pts',(-18.3620830674316,-10.7470540799783,
124.496092551227)) ;
#43361=CARTESIAN_POINT('Ctrl Pts',(-18.734581283145,-10.9370286586164,124.411415680481)) ;
#43362=CARTESIAN_POINT('Ctrl Pts',(-18.5658978745921,-10.7570395782535,
124.661307439936)) ;
#43363=CARTESIAN_POINT('Ctrl Pts',(-18.9171658090595,-10.9469635615994,
124.512917995207)) ;
#43364=CARTESIAN_POINT('Ctrl Pts',(-18.7941275674691,-10.7669744812365,
124.788187738228)) ;
#43365=CARTESIAN_POINT('Ctrl Pts',(-19.1170341754858,-10.9570210646946,
124.581816159323)) ;
#43366=CARTESIAN_POINT('Ctrl Pts',(-19.0439620659958,-10.7770319843317,
124.874312872399)) ;
#43367=CARTESIAN_POINT('Ctrl Pts',(-19.3209344460454,-10.9668427210651,
124.614507954261)) ;
#43368=CARTESIAN_POINT('Ctrl Pts',(-19.2988377714799,-10.7868536407023,
124.915180256188)) ;
#43369=CARTESIAN_POINT('Ctrl Pts',(-19.5323077477126,-10.9768987837303,
124.611618015789)) ;
#43370=CARTESIAN_POINT('Ctrl Pts',(-19.5630543230624,-10.7969097033674,
124.911570311771)) ;
#43371=CARTESIAN_POINT('Ctrl Pts',(-19.7375399994228,-10.9868394484335,
124.572149859508)) ;
#43372=CARTESIAN_POINT('Ctrl Pts',(-19.819595446342,-10.8068503680706,124.862237558294)) ;
#43373=CARTESIAN_POINT('Ctrl Pts',(-19.932315810984,-10.996743852382,124.498530010297)) ;
#43374=CARTESIAN_POINT('Ctrl Pts',(-20.0630665620373,-10.8167547720191,
124.77021482164)) ;
#43375=CARTESIAN_POINT('Ctrl Pts',(-20.1138352643569,-11.0067903373756,
124.39058103883)) ;
#43376=CARTESIAN_POINT('Ctrl Pts',(-20.2899670415844,-10.8268012570127,
124.635280761768)) ;
#43377=CARTESIAN_POINT('Ctrl Pts',(-20.271611629066,-11.0166865651873,124.254920335698)) ;
#43378=CARTESIAN_POINT('Ctrl Pts',(-20.4871895041345,-10.8366974848244,
124.465706330208)) ;
#43379=CARTESIAN_POINT('Ctrl Pts',(-20.4056065237285,-11.0267461487508,
124.09133118011)) ;
#43380=CARTESIAN_POINT('Ctrl Pts',(-20.6546848715982,-10.8467570683879,
124.261221540526)) ;
#43381=CARTESIAN_POINT('Ctrl Pts',(-20.5070605056192,-11.0365981584196,
123.910749358251)) ;
#43382=CARTESIAN_POINT('Ctrl Pts',(-20.7815048415044,-10.8566090780567,
124.035494716813)) ;
#43383=CARTESIAN_POINT('Ctrl Pts',(-20.5770451368418,-11.0465606898592,
123.713354618847)) ;
#43384=CARTESIAN_POINT('Ctrl Pts',(-20.8689878382938,-10.8665716094963,
123.788751735695)) ;
#43385=CARTESIAN_POINT('Ctrl Pts',(-20.6116136924991,-11.0565922380985,
123.505305288482)) ;
#43386=CARTESIAN_POINT('Ctrl Pts',(-20.912200798905,-10.8766031577357,123.528690516731)) ;
#43387=CARTESIAN_POINT('Ctrl Pts',(-20.6097611314172,-11.0664836493116,
123.297365165469)) ;
#43388=CARTESIAN_POINT('Ctrl Pts',(-20.9098873495447,-10.8864945689487,
123.268764662041)) ;
#43389=CARTESIAN_POINT('Ctrl Pts',(-20.5717257520097,-11.0764999030196,
123.090247708174)) ;
#43390=CARTESIAN_POINT('Ctrl Pts',(-20.8623452479891,-10.8965108226567,
123.009867420401)) ;
#43391=CARTESIAN_POINT('Ctrl Pts',(-20.4977797269794,-11.0865300058643,
122.892777790247)) ;
#43392=CARTESIAN_POINT('Ctrl Pts',(-20.7699148713601,-10.9065409255014,
122.763029266333)) ;
#43393=CARTESIAN_POINT('Ctrl Pts',(-20.3928580773295,-11.096386454818,122.714076335493)) ;
#43394=CARTESIAN_POINT('Ctrl Pts',(-20.6387642261451,-10.9163973744551,
122.539650565094)) ;
#43395=CARTESIAN_POINT('Ctrl Pts',(-20.2567901765193,-11.1063854655903,
122.553889016232)) ;
#43396=CARTESIAN_POINT('Ctrl Pts',(-20.4686808693851,-10.9263963852274,
122.339414946397)) ;
#43397=CARTESIAN_POINT('Ctrl Pts',(-20.0967506938251,-11.1162806825083,
122.420933108959)) ;
#43398=CARTESIAN_POINT('Ctrl Pts',(-20.2686322562331,-10.9362916021454,
122.17321802605)) ;
#43399=CARTESIAN_POINT('Ctrl Pts',(-19.9130792390864,-11.1263411978656,
122.316112855486)) ;
#43400=CARTESIAN_POINT('Ctrl Pts',(-20.0390441621644,-10.9463521175027,
122.042191046987)) ;
#43401=CARTESIAN_POINT('Ctrl Pts',(-19.7181773873714,-11.1361904912527,
122.246149401792)) ;
#43402=CARTESIAN_POINT('Ctrl Pts',(-19.7954165502139,-10.9562014108898,
121.954734482504)) ;
#43403=CARTESIAN_POINT('Ctrl Pts',(-19.5105138121636,-11.1462176669327,
122.209933979005)) ;
#43404=CARTESIAN_POINT('Ctrl Pts',(-19.5358374377705,-10.9662285865698,
121.909463378996)) ;
#43405=CARTESIAN_POINT('Ctrl Pts',(-19.2996733625681,-11.1562462425598,
122.210880868471)) ;
#43406=CARTESIAN_POINT('Ctrl Pts',(-19.2722869357793,-10.976257162197,121.910644966112)) ;
#43407=CARTESIAN_POINT('Ctrl Pts',(-19.0959460919219,-11.1660913361057,
122.247342057068)) ;
#43408=CARTESIAN_POINT('Ctrl Pts',(-19.0176264126342,-10.9861022557429,
121.956219772892)) ;
#43409=CARTESIAN_POINT('Ctrl Pts',(-18.8985578247058,-11.1760825775375,
122.319166361709)) ;
#43410=CARTESIAN_POINT('Ctrl Pts',(-18.7708903038592,-10.9960934971746,
122.045998590472)) ;
#43411=CARTESIAN_POINT('Ctrl Pts',(-18.7160448813455,-11.1861183586808,
122.425022343304)) ;
#43412=CARTESIAN_POINT('Ctrl Pts',(-18.5427482922778,-11.0061292783179,
122.178316886012)) ;
#43413=CARTESIAN_POINT('Ctrl Pts',(-18.5574679836989,-11.1959705644105,
122.558254372856)) ;
#43414=CARTESIAN_POINT('Ctrl Pts',(-18.3445251559911,-11.0159814840476,
122.344856285624)) ;
#43415=CARTESIAN_POINT('Ctrl Pts',(-18.4224794756724,-11.2059326585275,
122.718377576205)) ;
#43416=CARTESIAN_POINT('Ctrl Pts',(-18.1757880512695,-11.0259435781646,
122.545009574833)) ;
#43417=CARTESIAN_POINT('Ctrl Pts',(-18.3169268323872,-11.2159552193546,
122.900738727932)) ;
#43418=CARTESIAN_POINT('Ctrl Pts',(-18.0438458206682,-11.0359661389917,
122.7729601423)) ;
#43419=CARTESIAN_POINT('Ctrl Pts',(-18.2451248266948,-11.2258829910061,
123.096732722796)) ;
#43420=CARTESIAN_POINT('Ctrl Pts',(-17.9540915966108,-11.0458939106433,
123.017952668927)) ;
#43421=CARTESIAN_POINT('Ctrl Pts',(-18.2080492813558,-11.235925375131,123.304558510364)) ;
#43422=CARTESIAN_POINT('Ctrl Pts',(-17.9077456060715,-11.0559362947681,
123.277734456028)) ;
#43423=CARTESIAN_POINT('Ctrl Pts',(-18.2075431826477,-11.2458145992016,
123.512472427979)) ;
#43424=CARTESIAN_POINT('Ctrl Pts',(-17.9071113956414,-11.0658255188387,
123.537627775337)) ;
#43425=CARTESIAN_POINT('Ctrl Pts',(-18.2431137932323,-11.2558038473689,
123.719436413788)) ;
#43426=CARTESIAN_POINT('Ctrl Pts',(-17.9515732678051,-11.075814767006,123.796333212552)) ;
#43427=CARTESIAN_POINT('Ctrl Pts',(-18.3140127800185,-11.2657624244109,
123.916420734498)) ;
#43428=CARTESIAN_POINT('Ctrl Pts',(-18.0401957307403,-11.085773344048,124.042564530846)) ;
#43429=CARTESIAN_POINT('Ctrl Pts',(-18.4169840173117,-11.2756619935022,
124.097296523522)) ;
#43430=CARTESIAN_POINT('Ctrl Pts',(-18.168909061226,-11.0956729131393,124.268660685117)) ;
#43431=CARTESIAN_POINT('Ctrl Pts',(-18.5518230953768,-11.2857099055862,
124.259873078024)) ;
#43432=CARTESIAN_POINT('Ctrl Pts',(-18.337456729501,-11.1057208252233,124.471882073783)) ;
#43433=CARTESIAN_POINT('Ctrl Pts',(-18.7103328750192,-11.2956052598934,
124.394651304533)) ;
#43434=CARTESIAN_POINT('Ctrl Pts',(-18.5355938114042,-11.1156161795305,
124.640356432155)) ;
#43435=CARTESIAN_POINT('Ctrl Pts',(-18.8927897807584,-11.3056669103846,
124.50162581541)) ;
#43436=CARTESIAN_POINT('Ctrl Pts',(-18.7636640136148,-11.1256778300217,
124.774075513825)) ;
#43437=CARTESIAN_POINT('Ctrl Pts',(-19.0867894285585,-11.315511525847,124.573745609378)) ;
#43438=CARTESIAN_POINT('Ctrl Pts',(-19.006164366436,-11.1355224454842,124.864226909227)) ;
#43439=CARTESIAN_POINT('Ctrl Pts',(-19.2926054693123,-11.3254716047484,
124.612260164776)) ;
#43440=CARTESIAN_POINT('Ctrl Pts',(-19.2634346826531,-11.1454825243856,
124.912371167711)) ;
#43441=CARTESIAN_POINT('Ctrl Pts',(-19.5036241030656,-11.3355097991068,
124.6140594671)) ;
#43442=CARTESIAN_POINT('Ctrl Pts',(-19.527207804198,-11.1555207187439,124.914621442776)) ;
#43443=CARTESIAN_POINT('Ctrl Pts',(-19.7084368116268,-11.3453835145064,
124.580138707835)) ;
#43444=CARTESIAN_POINT('Ctrl Pts',(-19.7832249578582,-11.1653944341435,
124.872221302149)) ;
#43445=CARTESIAN_POINT('Ctrl Pts',(-19.9081154986966,-11.3554552240407,
124.509785415039)) ;
#43446=CARTESIAN_POINT('Ctrl Pts',(-20.0328232712046,-11.1754661436778,
124.784280775567)) ;
#43447=CARTESIAN_POINT('Ctrl Pts',(-20.0882613339957,-11.3652876644932,
124.408381333972)) ;
#43448=CARTESIAN_POINT('Ctrl Pts',(-20.2580073160466,-11.1852985841303,
124.657525797588)) ;
#43449=CARTESIAN_POINT('Ctrl Pts',(-20.251660229155,-11.3753194854186,124.275048143701)) ;
#43450=CARTESIAN_POINT('Ctrl Pts',(-20.4622563153842,-11.1953304050557,
124.490859965048)) ;
#43451=CARTESIAN_POINT('Ctrl Pts',(-20.388818370831,-11.3853398553042,124.115153399644)) ;
#43452=CARTESIAN_POINT('Ctrl Pts',(-20.6337047072471,-11.2053507749413,
124.290992198856)) ;
#43453=CARTESIAN_POINT('Ctrl Pts',(-20.4949578126602,-11.3952066264379,
123.936918605361)) ;
#43454=CARTESIAN_POINT('Ctrl Pts',(-20.7663802888455,-11.215217546075,124.068198059716)) ;
#43455=CARTESIAN_POINT('Ctrl Pts',(-20.5700397801666,-11.4052773976273,
123.738981962488)) ;
#43456=CARTESIAN_POINT('Ctrl Pts',(-20.8602333250101,-11.2252883172644,
123.820777914708)) ;
#43457=CARTESIAN_POINT('Ctrl Pts',(-20.608748085118,-11.4151205581489,123.535688979496)) ;
#43458=CARTESIAN_POINT('Ctrl Pts',(-20.9086197171465,-11.235131477786,123.566660443392)) ;
#43459=CARTESIAN_POINT('Ctrl Pts',(-20.6122979783934,-11.4251007913353,
123.32590993056)) ;
#43460=CARTESIAN_POINT('Ctrl Pts',(-20.9130575837451,-11.2451117109724,
123.304436329207)) ;
#43461=CARTESIAN_POINT('Ctrl Pts',(-20.5788422571338,-11.4351193113705,
123.117968685033)) ;
#43462=CARTESIAN_POINT('Ctrl Pts',(-20.871238578832,-11.2551302310076,123.044509679255)) ;
#43463=CARTESIAN_POINT('Ctrl Pts',(-20.5111294875309,-11.4450026197542,
122.921507091262)) ;
#43464=CARTESIAN_POINT('Ctrl Pts',(-20.7865977118334,-11.2650135393913,
122.798931493979)) ;
#43465=CARTESIAN_POINT('Ctrl Pts',(-20.4083944122188,-11.455070903925,122.736483235784)) ;
#43466=CARTESIAN_POINT('Ctrl Pts',(-20.6581795184354,-11.2750818235621,
122.567651782636)) ;
#43467=CARTESIAN_POINT('Ctrl Pts',(-20.278392781555,-11.4649010305926,122.575789839308)) ;
#43468=CARTESIAN_POINT('Ctrl Pts',(-20.4956768373956,-11.2849119502298,
122.366783576293)) ;
#43469=CARTESIAN_POINT('Ctrl Pts',(-20.1189455476198,-11.4749676027992,
122.43668549405)) ;
#43470=CARTESIAN_POINT('Ctrl Pts',(-20.2963683002106,-11.2949785224363,
122.192903170129)) ;
#43471=CARTESIAN_POINT('Ctrl Pts',(-19.9408261904973,-11.4848577590399,
122.329373206102)) ;
#43472=CARTESIAN_POINT('Ctrl Pts',(-20.0737183940731,-11.304868678677,122.058761956782)) ;
#43473=CARTESIAN_POINT('Ctrl Pts',(-19.7449718071379,-11.4948502866163,
122.253435565076)) ;
#43474=CARTESIAN_POINT('Ctrl Pts',(-19.8289002832035,-11.3148612062534,
121.963839656321)) ;
#43475=CARTESIAN_POINT('Ctrl Pts',(-19.5394995838217,-11.5048117764906,
122.212958774971)) ;
#43476=CARTESIAN_POINT('Ctrl Pts',(-19.5720596012938,-11.3248226961277,
121.913243325035)) ;
#43477=CARTESIAN_POINT('Ctrl Pts',(-19.3312195995513,-11.5147209983778,
122.208316709471)) ;
#43478=CARTESIAN_POINT('Ctrl Pts',(-19.3117087063765,-11.3347319180149,
121.907440658381)) ;
#43479=CARTESIAN_POINT('Ctrl Pts',(-19.1224333832175,-11.5247695781881,
122.240425699493)) ;
#43480=CARTESIAN_POINT('Ctrl Pts',(-19.0507261790839,-11.3447804978252,
121.947576761925)) ;
#43481=CARTESIAN_POINT('Ctrl Pts',(-18.9256450998965,-11.5346525526582,
122.307117491957)) ;
#43482=CARTESIAN_POINT('Ctrl Pts',(-18.8047397506185,-11.3546634722953,
122.030941792183)) ;
#43483=CARTESIAN_POINT('Ctrl Pts',(-18.7411595782649,-11.5446474638009,
122.407688727702)) ;
#43484=CARTESIAN_POINT('Ctrl Pts',(-18.5741327464813,-11.364658383438,122.156656022076)) ;
#43485=CARTESIAN_POINT('Ctrl Pts',(-18.5766849466755,-11.5546678503745,
122.539338975724)) ;
#43486=CARTESIAN_POINT('Ctrl Pts',(-18.3685394795987,-11.3746787700116,
122.321218804861)) ;
#43487=CARTESIAN_POINT('Ctrl Pts',(-18.4390281447,-11.5645779542315,122.69570721258)) ;
#43488=CARTESIAN_POINT('Ctrl Pts',(-18.1964679003152,-11.3845888738687,
122.516679816547)) ;
#43489=CARTESIAN_POINT('Ctrl Pts',(-18.3299418694843,-11.5745056664414,
122.873650877876)) ;
#43490=CARTESIAN_POINT('Ctrl Pts',(-18.0601098924679,-11.3945165860786,
122.739110167226)) ;
#43491=CARTESIAN_POINT('Ctrl Pts',(-18.2526908814426,-11.5845487762087,
123.070140221989)) ;
#43492=CARTESIAN_POINT('Ctrl Pts',(-17.9635464111682,-11.4045596958458,
122.984721718142)) ;
#43493=CARTESIAN_POINT('Ctrl Pts',(-18.2112504293198,-11.5944351966642,
123.273822369061)) ;
#43494=CARTESIAN_POINT('Ctrl Pts',(-17.9117458665147,-11.4144461163014,
123.239325516368)) ;
#43495=CARTESIAN_POINT('Ctrl Pts',(-18.2053899399513,-11.6044283742699,
123.48381708741)) ;
#43496=CARTESIAN_POINT('Ctrl Pts',(-17.9044206322636,-11.424439293907,123.501819128649)) ;
#43497=CARTESIAN_POINT('Ctrl Pts',(-18.2360155974427,-11.6143740371738,
123.690651541286)) ;
#43498=CARTESIAN_POINT('Ctrl Pts',(-17.9427031377925,-11.4343849568109,
123.760362733581)) ;
#43499=CARTESIAN_POINT('Ctrl Pts',(-18.3016977196334,-11.624321333379,123.889202740392)) ;
#43500=CARTESIAN_POINT('Ctrl Pts',(-18.0248064637638,-11.4443322530161,
124.008552115012)) ;
#43501=CARTESIAN_POINT('Ctrl Pts',(-18.4020577550734,-11.6343690989569,
124.075068550386)) ;
#43502=CARTESIAN_POINT('Ctrl Pts',(-18.1502567640289,-11.454380018594,124.240883955143)) ;
#43503=CARTESIAN_POINT('Ctrl Pts',(-18.53043452236,-11.6442173121745,124.237499635771)) ;
#43504=CARTESIAN_POINT('Ctrl Pts',(-18.31072897444,-11.4642282318116,124.443923603713)) ;
#43505=CARTESIAN_POINT('Ctrl Pts',(-18.6863539195395,-11.6541768849686,
124.377247513015)) ;
#43506=CARTESIAN_POINT('Ctrl Pts',(-18.5056290796381,-11.4741878046057,
124.618608195999)) ;
#43507=CARTESIAN_POINT('Ctrl Pts',(-18.8657358234262,-11.6642135060011,
124.488337618152)) ;
#43508=CARTESIAN_POINT('Ctrl Pts',(-18.7298566496538,-11.4842244256382,
124.757470221316)) ;
#43509=CARTESIAN_POINT('Ctrl Pts',(-19.0585401018813,-11.6740940208114,
124.565687771704)) ;
#43510=CARTESIAN_POINT('Ctrl Pts',(-18.9708633136617,-11.4941049404486,
124.854157638432)) ;
#43511=CARTESIAN_POINT('Ctrl Pts',(-19.2653207495063,-11.6841466721185,
124.609197173488)) ;
#43512=CARTESIAN_POINT('Ctrl Pts',(-19.2293390121453,-11.5041575917556,
124.90854357499)) ;
#43513=CARTESIAN_POINT('Ctrl Pts',(-19.4732739400485,-11.6940420703985,
124.616120019601)) ;
#43514=CARTESIAN_POINT('Ctrl Pts',(-19.4892814880954,-11.5140529900356,
124.917196362515)) ;
#43515=CARTESIAN_POINT('Ctrl Pts',(-19.6824421140478,-11.7040921921046,
124.586475455409)) ;
#43516=CARTESIAN_POINT('Ctrl Pts',(-19.7507413265183,-11.5241031117417,
124.880139860388)) ;
#43517=CARTESIAN_POINT('Ctrl Pts',(-19.8800272774462,-11.7139764716465,
124.522061203542)) ;
#43518=CARTESIAN_POINT('Ctrl Pts',(-19.9977235238706,-11.5339873912836,
124.799620909315)) ;
#43519=CARTESIAN_POINT('Ctrl Pts',(-20.0656260604384,-11.7239712529384,
124.423592328542)) ;
#43520=CARTESIAN_POINT('Ctrl Pts',(-20.2297217101426,-11.5439821725755,
124.676533838734)) ;
#43521=CARTESIAN_POINT('Ctrl Pts',(-20.2305069833902,-11.7339190981252,
124.294916040327)) ;
#43522=CARTESIAN_POINT('Ctrl Pts',(-20.4358226950316,-11.5539300177623,
124.515687379052)) ;
#43523=CARTESIAN_POINT('Ctrl Pts',(-20.3705912261117,-11.7438560615126,
124.139963124901)) ;
#43524=CARTESIAN_POINT('Ctrl Pts',(-20.6109276227123,-11.5638669811497,
124.321995034894)) ;
#43525=CARTESIAN_POINT('Ctrl Pts',(-20.482403685854,-11.7538390262498,123.962322659801)) ;
#43526=CARTESIAN_POINT('Ctrl Pts',(-20.7506923359331,-11.5738499458869,
124.099943607919)) ;
#43527=CARTESIAN_POINT('Ctrl Pts',(-20.5617787036582,-11.7638828776654,
123.766682247549)) ;
#43528=CARTESIAN_POINT('Ctrl Pts',(-20.8499100759965,-11.5838937973026,
123.855392878857)) ;
#43529=CARTESIAN_POINT('Ctrl Pts',(-20.6055180822358,-11.7737110790002,
123.564713422646)) ;
#43530=CARTESIAN_POINT('Ctrl Pts',(-20.9045834153395,-11.5937219986373,
123.60293017781)) ;
#43531=CARTESIAN_POINT('Ctrl Pts',(-20.6138247387092,-11.7837876515982,
123.353078389392)) ;
#43532=CARTESIAN_POINT('Ctrl Pts',(-20.9149654649752,-11.6037985712354,
123.338386769837)) ;
#43533=CARTESIAN_POINT('Ctrl Pts',(-20.5859865681062,-11.7936397316058,
123.147790724545)) ;
#43534=CARTESIAN_POINT('Ctrl Pts',(-20.8801663077808,-11.6136506512429,
123.081776137432)) ;
#43535=CARTESIAN_POINT('Ctrl Pts',(-20.5217060175956,-11.8037130166099,
122.94604661898)) ;
#43536=CARTESIAN_POINT('Ctrl Pts',(-20.7998144512249,-11.623723936247,122.829596800206)) ;
#43537=CARTESIAN_POINT('Ctrl Pts',(-20.4255657745516,-11.8135543683204,
122.7628267317)) ;
#43538=CARTESIAN_POINT('Ctrl Pts',(-20.6796373590905,-11.6335652879575,
122.60057140377)) ;
#43539=CARTESIAN_POINT('Ctrl Pts',(-20.2981587765571,-11.8235158677169,
122.596634860964)) ;
#43540=CARTESIAN_POINT('Ctrl Pts',(-20.5203770951846,-11.643526787354,122.39283222261)) ;
#43541=CARTESIAN_POINT('Ctrl Pts',(-20.1424149976007,-11.8335516438469,
122.454293214028)) ;
#43542=CARTESIAN_POINT('Ctrl Pts',(-20.3256964580967,-11.653562563484,122.21490632929)) ;
#43543=CARTESIAN_POINT('Ctrl Pts',(-19.9670619376452,-11.8434400704844,
122.342638696447)) ;
#43544=CARTESIAN_POINT('Ctrl Pts',(-20.1065035192901,-11.6634509901216,
122.07533899432)) ;
#43545=CARTESIAN_POINT('Ctrl Pts',(-19.7726633460982,-11.8534553925594,
122.261733680716)) ;
#43546=CARTESIAN_POINT('Ctrl Pts',(-19.8635046295888,-11.6734663121965,
121.974209274979)) ;
#43547=CARTESIAN_POINT('Ctrl Pts',(-19.5667618955136,-11.8634857414596,
122.216223716099)) ;
#43548=CARTESIAN_POINT('Ctrl Pts',(-19.6061275734712,-11.6834966610967,
121.917323321599)) ;
#43549=CARTESIAN_POINT('Ctrl Pts',(-19.3600373542584,-11.8733291170662,
122.206909440911)) ;
#43550=CARTESIAN_POINT('Ctrl Pts',(-19.3477206075241,-11.6933400367034,
121.905682077823)) ;
#43551=CARTESIAN_POINT('Ctrl Pts',(-19.150888532225,-11.8833585539634,122.233670381781)) ;
#43552=CARTESIAN_POINT('Ctrl Pts',(-19.0862848802727,-11.7033694736005,
121.939135039902)) ;
#43553=CARTESIAN_POINT('Ctrl Pts',(-18.9496827788183,-11.8933904318963,
122.296907578933)) ;
#43554=CARTESIAN_POINT('Ctrl Pts',(-18.834778258423,-11.7134013515334,122.018183059179)) ;
#43555=CARTESIAN_POINT('Ctrl Pts',(-18.7661111079611,-11.9032200550018,
122.391777133203)) ;
#43556=CARTESIAN_POINT('Ctrl Pts',(-18.6053133475109,-11.7232309746389,
122.136772150957)) ;
#43557=CARTESIAN_POINT('Ctrl Pts',(-18.5987322084384,-11.9132095261549,
122.518627177409)) ;
#43558=CARTESIAN_POINT('Ctrl Pts',(-18.3960907645237,-11.733220445792,122.295336373572)) ;
#43559=CARTESIAN_POINT('Ctrl Pts',(-18.4555426602971,-11.9232533749173,
122.673809920536)) ;
#43560=CARTESIAN_POINT('Ctrl Pts',(-18.2171052463347,-11.7432642945544,
122.489315908043)) ;
#43561=CARTESIAN_POINT('Ctrl Pts',(-18.3436356389824,-11.933075080449,122.847337567212)) ;
#43562=CARTESIAN_POINT('Ctrl Pts',(-18.0772224088806,-11.7530860000861,
122.706227559913)) ;
#43563=CARTESIAN_POINT('Ctrl Pts',(-18.2613427697256,-11.9431101202768,
123.041592805838)) ;
#43564=CARTESIAN_POINT('Ctrl Pts',(-17.974358275623,-11.7631210399139,122.949047320032)) ;
#43565=CARTESIAN_POINT('Ctrl Pts',(-18.2146441937951,-11.9531348271682,
123.247112574505)) ;
#43566=CARTESIAN_POINT('Ctrl Pts',(-17.9159869176276,-11.7731457468054,
123.205947428722)) ;
#43567=CARTESIAN_POINT('Ctrl Pts',(-18.2040790572873,-11.962987531509,123.453976992299)) ;
#43568=CARTESIAN_POINT('Ctrl Pts',(-17.9027824760765,-11.7829984511461,
123.464529062484)) ;
#43569=CARTESIAN_POINT('Ctrl Pts',(-18.2295779813126,-11.9729756537167,
123.662389605254)) ;
#43570=CARTESIAN_POINT('Ctrl Pts',(-17.9346582755181,-11.7929865733538,
123.72504475189)) ;
#43571=CARTESIAN_POINT('Ctrl Pts',(-18.2905062794645,-11.982904123824,123.862032052655)) ;
#43572=CARTESIAN_POINT('Ctrl Pts',(-18.0108208430666,-11.8029150434611,
123.974597684985)) ;
#43573=CARTESIAN_POINT('Ctrl Pts',(-18.3854419619658,-11.9928931009912,
124.049358952293)) ;
#43574=CARTESIAN_POINT('Ctrl Pts',(-18.129492517191,-11.8129040206283,124.20875545915)) ;
#43575=CARTESIAN_POINT('Ctrl Pts',(-18.51235689706,-12.0029309082709,124.217948281748)) ;
#43576=CARTESIAN_POINT('Ctrl Pts',(-18.2881378411285,-11.822941827908,124.419490767607)) ;
#43577=CARTESIAN_POINT('Ctrl Pts',(-18.6634476701596,-12.0127772091342,
124.359445076949)) ;
#43578=CARTESIAN_POINT('Ctrl Pts',(-18.4770035096972,-11.8327881287713,
124.596360779214)) ;
#43579=CARTESIAN_POINT('Ctrl Pts',(-18.8397147754035,-12.0228029525135,
124.475014140463)) ;
#43580=CARTESIAN_POINT('Ctrl Pts',(-18.6973386411338,-11.8428138721506,
124.740820127041)) ;
#43581=CARTESIAN_POINT('Ctrl Pts',(-19.03368933323,-12.0328338189525,124.557760416671)) ;
#43582=CARTESIAN_POINT('Ctrl Pts',(-18.9398076657194,-11.8528447385896,
124.844250930531)) ;
#43583=CARTESIAN_POINT('Ctrl Pts',(-19.2350138531615,-12.0426711777513,
124.605047798355)) ;
#43584=CARTESIAN_POINT('Ctrl Pts',(-19.1914647637144,-11.8626820973884,
124.903358127309)) ;
#43585=CARTESIAN_POINT('Ctrl Pts',(-19.4447121805973,-12.052663138685,124.61740552715)) ;
#43586=CARTESIAN_POINT('Ctrl Pts',(-19.4535879451844,-11.8726740583222,
124.918802859843)) ;
#43587=CARTESIAN_POINT('Ctrl Pts',(-19.654174209039,-12.0626955012416,124.59264506007)) ;
#43588=CARTESIAN_POINT('Ctrl Pts',(-19.7154151681285,-11.8827064208787,
124.887849956679)) ;
#43589=CARTESIAN_POINT('Ctrl Pts',(-19.8528431822894,-12.072560661816,124.53314903407)) ;
#43590=CARTESIAN_POINT('Ctrl Pts',(-19.9637513981786,-11.8925715814531,
124.813477415096)) ;
#43591=CARTESIAN_POINT('Ctrl Pts',(-20.0402625333132,-12.0825225663937,
124.439673578487)) ;
#43592=CARTESIAN_POINT('Ctrl Pts',(-20.1980246864583,-11.9025334860308,
124.696630723348)) ;
#43593=CARTESIAN_POINT('Ctrl Pts',(-20.2096190237234,-12.0925574964694,
124.313895264945)) ;
#43594=CARTESIAN_POINT('Ctrl Pts',(-20.4097188088187,-11.9125684161065,
124.539405883131)) ;
#43595=CARTESIAN_POINT('Ctrl Pts',(-20.3526800116948,-12.102442443323,124.163124144137)) ;
#43596=CARTESIAN_POINT('Ctrl Pts',(-20.5885436050965,-11.9224533629601,
124.350939834724)) ;
#43597=CARTESIAN_POINT('Ctrl Pts',(-20.4694104296519,-12.1125081196345,
123.986661950019)) ;
#43598=CARTESIAN_POINT('Ctrl Pts',(-20.7344544461953,-11.9325190392716,
124.130360829596)) ;
#43599=CARTESIAN_POINT('Ctrl Pts',(-20.5520515995571,-12.1223470392694,
123.797005493285)) ;
#43600=CARTESIAN_POINT('Ctrl Pts',(-20.8377538535721,-11.9423579589065,
123.89328858742)) ;
#43601=CARTESIAN_POINT('Ctrl Pts',(-20.6018640316816,-12.1324105490038,
123.591417354039)) ;
#43602=CARTESIAN_POINT('Ctrl Pts',(-20.9000168313516,-11.9524214686409,
123.636302931589)) ;
#43603=CARTESIAN_POINT('Ctrl Pts',(-20.6148291614051,-12.1423041621656,
123.383802604213)) ;
#43604=CARTESIAN_POINT('Ctrl Pts',(-20.9162207081352,-11.9623150818027,
123.376783859036)) ;
#43605=CARTESIAN_POINT('Ctrl Pts',(-20.5919863900176,-12.152248168979,123.176028489943)) ;
#43606=CARTESIAN_POINT('Ctrl Pts',(-20.8876645643203,-11.9722590886161,
123.117066234101)) ;
#43607=CARTESIAN_POINT('Ctrl Pts',(-20.5331562624697,-12.1622491233333,
122.974141880329)) ;
#43608=CARTESIAN_POINT('Ctrl Pts',(-20.8141243155986,-11.9822600429704,
122.8647086418)) ;
#43609=CARTESIAN_POINT('Ctrl Pts',(-20.4394990832698,-12.1722878810256,
122.785036123018)) ;
#43610=CARTESIAN_POINT('Ctrl Pts',(-20.6970504996991,-11.9922988006627,
122.628327621003)) ;
#43611=CARTESIAN_POINT('Ctrl Pts',(-20.3174467550257,-12.1821120651956,
122.618401426981)) ;
#43612=CARTESIAN_POINT('Ctrl Pts',(-20.5444825751892,-12.0021229848327,
122.420035361004)) ;
#43613=CARTESIAN_POINT('Ctrl Pts',(-20.1650056351834,-12.192170130795,122.471888778406)) ;
#43614=CARTESIAN_POINT('Ctrl Pts',(-20.3539293395536,-12.0121810504321,
122.236896566325)) ;
#43615=CARTESIAN_POINT('Ctrl Pts',(-19.9914963261328,-12.2021001775697,
122.355781356402)) ;
#43616=CARTESIAN_POINT('Ctrl Pts',(-20.1370409747147,-12.0221110972068,
122.091764368012)) ;
#43617=CARTESIAN_POINT('Ctrl Pts',(-19.8002835579305,-12.2120516199068,
122.270882760811)) ;
#43618=CARTESIAN_POINT('Ctrl Pts',(-19.8980237231667,-12.0320625395439,
121.985643564698)) ;
#43619=CARTESIAN_POINT('Ctrl Pts',(-19.5952237413981,-12.2220984170861,
122.220273264171)) ;
#43620=CARTESIAN_POINT('Ctrl Pts',(-19.6416983085707,-12.0421093367232,
121.922384338977)) ;
#43621=CARTESIAN_POINT('Ctrl Pts',(-19.388673024252,-12.2319463577662,122.206126303153)) ;
#43622=CARTESIAN_POINT('Ctrl Pts',(-19.3835093232675,-12.0519572774033,
121.904703348343)) ;
#43623=CARTESIAN_POINT('Ctrl Pts',(-19.180367514707,-12.2419079891088,122.227663750523)) ;
#43624=CARTESIAN_POINT('Ctrl Pts',(-19.1231275997313,-12.0619189087459,
121.931627958287)) ;
#43625=CARTESIAN_POINT('Ctrl Pts',(-18.9776624918692,-12.2519366484847,
122.285690175812)) ;
#43626=CARTESIAN_POINT('Ctrl Pts',(-18.8697470442625,-12.0719475681218,
122.004163670847)) ;
#43627=CARTESIAN_POINT('Ctrl Pts',(-18.7903389023048,-12.2618469513729,
122.376871314838)) ;
#43628=CARTESIAN_POINT('Ctrl Pts',(-18.6355935850335,-12.08185787101,122.118142693142)) ;
#43629=CARTESIAN_POINT('Ctrl Pts',(-18.6209407245683,-12.2717818459351,
122.499062432989)) ;
#43630=CARTESIAN_POINT('Ctrl Pts',(-18.4238474019827,-12.0917927655722,
122.270883953054)) ;
#43631=CARTESIAN_POINT('Ctrl Pts',(-18.4739251947791,-12.281822944602,122.650538595866)) ;
#43632=CARTESIAN_POINT('Ctrl Pts',(-18.2400799717895,-12.1018338642391,
122.460231143199)) ;
#43633=CARTESIAN_POINT('Ctrl Pts',(-18.3571294374524,-12.2917102271064,
122.822498446866)) ;
#43634=CARTESIAN_POINT('Ctrl Pts',(-18.0940875093298,-12.1117211467435,
122.675182672206)) ;
#43635=CARTESIAN_POINT('Ctrl Pts',(-18.270751539422,-12.3017019676169,123.013960222828)) ;
#43636=CARTESIAN_POINT('Ctrl Pts',(-17.9861176823212,-12.121712887254,122.914511116819)) ;
#43637=CARTESIAN_POINT('Ctrl Pts',(-18.2192070084759,-12.3116525168523,
123.216713043698)) ;
#43638=CARTESIAN_POINT('Ctrl Pts',(-17.921689729601,-12.1316634364894,123.16795292873)) ;
#43639=CARTESIAN_POINT('Ctrl Pts',(-18.203364387181,-12.3215881944871,123.424977839185)) ;
#43640=CARTESIAN_POINT('Ctrl Pts',(-17.9018892648507,-12.1415991141242,
123.428284203218)) ;
#43641=CARTESIAN_POINT('Ctrl Pts',(-18.2238062767761,-12.3315736122799,
123.63392140019)) ;
#43642=CARTESIAN_POINT('Ctrl Pts',(-17.9274444398076,-12.151584531917,123.689463440879)) ;
#43643=CARTESIAN_POINT('Ctrl Pts',(-18.2807096673845,-12.3416024051504,
123.83693264531)) ;
#43644=CARTESIAN_POINT('Ctrl Pts',(-17.9985764205707,-12.1616133247875,
123.943226816736)) ;
#43645=CARTESIAN_POINT('Ctrl Pts',(-18.3704393887249,-12.3514819163783,
124.024245376824)) ;
#43646=CARTESIAN_POINT('Ctrl Pts',(-18.1107411250608,-12.1714928360155,
124.177366527378)) ;
#43647=CARTESIAN_POINT('Ctrl Pts',(-18.4923386110279,-12.3614754530513,
124.195371559684)) ;
#43648=CARTESIAN_POINT('Ctrl Pts',(-18.263117466536,-12.1814863726884,124.391272663474)) ;
#43649=CARTESIAN_POINT('Ctrl Pts',(-18.6429752247149,-12.3715077213151,
124.342978657029)) ;
#43650=CARTESIAN_POINT('Ctrl Pts',(-18.4514152853576,-12.1915186409522,
124.575779592005)) ;
#43651=CARTESIAN_POINT('Ctrl Pts',(-18.8138083567616,-12.381371683321,124.460571682728)) ;
#43652=CARTESIAN_POINT('Ctrl Pts',(-18.6649582254987,-12.2013826029581,
124.722768521293)) ;
#43653=CARTESIAN_POINT('Ctrl Pts',(-19.0063512318433,-12.3914417446659,
124.548529857693)) ;
#43654=CARTESIAN_POINT('Ctrl Pts',(-18.9056381213548,-12.211452664303,124.832713751572)) ;
#43655=CARTESIAN_POINT('Ctrl Pts',(-19.2066412567903,-12.4012841090146,
124.600516981642)) ;
#43656=CARTESIAN_POINT('Ctrl Pts',(-19.1560012005742,-12.2212950286517,
124.897694900574)) ;
#43657=CARTESIAN_POINT('Ctrl Pts',(-19.4153191948693,-12.4112447815171,
124.61790415066)) ;
#43658=CARTESIAN_POINT('Ctrl Pts',(-19.4168488001017,-12.2312557011542,
124.919426126704)) ;
#43659=CARTESIAN_POINT('Ctrl Pts',(-19.6254227673264,-12.4212828525849,
124.598226325567)) ;
#43660=CARTESIAN_POINT('Ctrl Pts',(-19.6794781670334,-12.241293772222,124.894826056415)) ;
#43661=CARTESIAN_POINT('Ctrl Pts',(-19.8257277780076,-12.4311564675453,
124.54365478677)) ;
#43662=CARTESIAN_POINT('Ctrl Pts',(-19.9298584470305,-12.2511673871824,
124.826609084731)) ;
#43663=CARTESIAN_POINT('Ctrl Pts',(-20.0172039066253,-12.4412287021266,
124.453332611574)) ;
#43664=CARTESIAN_POINT('Ctrl Pts',(-20.1692027685541,-12.2612396217637,
124.713703674863)) ;
#43665=CARTESIAN_POINT('Ctrl Pts',(-20.1860304534501,-12.4510527205754,
124.334292333234)) ;
#43666=CARTESIAN_POINT('Ctrl Pts',(-20.3802336084559,-12.2710636402125,
124.56490174156)) ;
#43667=CARTESIAN_POINT('Ctrl Pts',(-20.3353241205461,-12.4611176415514,
124.184411186943)) ;
#43668=CARTESIAN_POINT('Ctrl Pts',(-20.5668505339034,-12.2811285611885,
124.3775468474)) ;
#43669=CARTESIAN_POINT('Ctrl Pts',(-20.4942292788694,-12.4743279398461,
123.956554640027)) ;
#43670=CARTESIAN_POINT('Ctrl Pts',(-20.7654710388387,-12.2943388594833,
124.092731380698)) ;
#43671=CARTESIAN_POINT('Ctrl Pts',(-20.5910323234022,-12.4876433865781,
123.690569761034)) ;
#43672=CARTESIAN_POINT('Ctrl Pts',(-20.8864681734945,-12.3076543062152,
123.760293059331)) ;
#43673=CARTESIAN_POINT('Ctrl Pts',(-20.6153241142933,-12.5009336318454,
123.412181900129)) ;
#43674=CARTESIAN_POINT('Ctrl Pts',(-20.9168412402485,-12.3209445514825,
123.412248798329)) ;
#43675=CARTESIAN_POINT('Ctrl Pts',(-20.5967460044986,-12.5109843814525,
123.20173674764)) ;
#43676=CARTESIAN_POINT('Ctrl Pts',(-20.8936136564304,-12.3309953010896,
123.149204261583)) ;
#43677=CARTESIAN_POINT('Ctrl Pts',(-20.5435845802291,-12.5207969884347,
123.002381741764)) ;
#43678=CARTESIAN_POINT('Ctrl Pts',(-20.8271599100472,-12.3408079080718,
122.900008574106)) ;
#43679=CARTESIAN_POINT('Ctrl Pts',(-20.4546049045706,-12.530868086429,122.81028950204)) ;
#43680=CARTESIAN_POINT('Ctrl Pts',(-20.7159339872492,-12.3508790060661,
122.659895486434)) ;
#43681=CARTESIAN_POINT('Ctrl Pts',(-20.3356089336191,-12.5407576592038,
122.639785901111)) ;
#43682=CARTESIAN_POINT('Ctrl Pts',(-20.5671825471141,-12.360768578841,122.446765213332)) ;
#43683=CARTESIAN_POINT('Ctrl Pts',(-20.1392326312349,-12.5540277660071,
122.441591528531)) ;
#43684=CARTESIAN_POINT('Ctrl Pts',(-20.3217335957846,-12.3740386856443,
122.199036770175)) ;
#43685=CARTESIAN_POINT('Ctrl Pts',(-19.8341063016993,-12.5706444529296,
122.263562945351)) ;
#43686=CARTESIAN_POINT('Ctrl Pts',(-19.9402799223287,-12.3906553725668,
121.976489963183)) ;
#43687=CARTESIAN_POINT('Ctrl Pts',(-19.4873858216236,-12.5872184962459,
122.20023473755)) ;
#43688=CARTESIAN_POINT('Ctrl Pts',(-19.5069560654083,-12.407229415883,121.897341845887)) ;
#43689=CARTESIAN_POINT('Ctrl Pts',(-19.208770852032,-12.6005150636777,122.222555120843)) ;
#43690=CARTESIAN_POINT('Ctrl Pts',(-19.1586250796142,-12.4205259833148,
121.925240968701)) ;
#43691=CARTESIAN_POINT('Ctrl Pts',(-19.004699994285,-12.6105451272551,122.27569208682)) ;
#43692=CARTESIAN_POINT('Ctrl Pts',(-18.9035497915594,-12.4305560468922,
121.991664800906)) ;
#43693=CARTESIAN_POINT('Ctrl Pts',(-18.8155802354143,-12.6204390191043,
122.362230085653)) ;
#43694=CARTESIAN_POINT('Ctrl Pts',(-18.6671468529052,-12.4404499387414,
122.099840645972)) ;
#43695=CARTESIAN_POINT('Ctrl Pts',(-18.5855888789982,-12.6336917748899,
122.519603205496)) ;
#43696=CARTESIAN_POINT('Ctrl Pts',(-18.3796682061191,-12.453702694527,122.296549637466)) ;
#43697=CARTESIAN_POINT('Ctrl Pts',(-18.354522049861,-12.6504198798823,122.789922613237)) ;
#43698=CARTESIAN_POINT('Ctrl Pts',(-18.0908280313655,-12.4704307995194,
122.634462100718)) ;
#43699=CARTESIAN_POINT('Ctrl Pts',(-18.2063394457701,-12.6702507163608,
123.184767083892)) ;
#43700=CARTESIAN_POINT('Ctrl Pts',(-17.9056069777788,-12.4902616359979,
123.128014485523)) ;
#43701=CARTESIAN_POINT('Ctrl Pts',(-18.2007363155492,-12.690176108251,123.608303510177)) ;
#43702=CARTESIAN_POINT('Ctrl Pts',(-17.8986058474029,-12.5101870278881,
123.65743523967)) ;
#43703=CARTESIAN_POINT('Ctrl Pts',(-18.3400998829644,-12.710101321603,124.008460954811)) ;
#43704=CARTESIAN_POINT('Ctrl Pts',(-18.0728134812496,-12.5301122412401,
124.157630024429)) ;
#43705=CARTESIAN_POINT('Ctrl Pts',(-18.6074924622381,-12.7300263350881,
124.337014382701)) ;
#43706=CARTESIAN_POINT('Ctrl Pts',(-18.4070561283902,-12.5500372547252,
124.568319257347)) ;
#43707=CARTESIAN_POINT('Ctrl Pts',(-18.9698313696597,-12.7499028067881,
124.554607895198)) ;
#43708=CARTESIAN_POINT('Ctrl Pts',(-18.8599799731256,-12.5699137264252,
124.840308096966)) ;
#43709=CARTESIAN_POINT('Ctrl Pts',(-19.3867523160162,-12.7698821246969,
124.636089846791)) ;
#43710=CARTESIAN_POINT('Ctrl Pts',(-19.3811313633293,-12.5898930443341,
124.942158139695)) ;
#43711=CARTESIAN_POINT('Ctrl Pts',(-19.8054691433214,-12.7898151282729,
124.570240660478)) ;
#43712=CARTESIAN_POINT('Ctrl Pts',(-19.9045262603243,-12.6098260479101,
124.859844414469)) ;
#43713=CARTESIAN_POINT('Ctrl Pts',(-20.1760444374323,-12.8097103983006,
124.366269150013)) ;
#43714=CARTESIAN_POINT('Ctrl Pts',(-20.3677432424192,-12.6297213179378,
124.6048789893)) ;
#43715=CARTESIAN_POINT('Ctrl Pts',(-20.4554911510886,-12.8296317362065,
124.047921898696)) ;
#43716=CARTESIAN_POINT('Ctrl Pts',(-20.7170498595964,-12.6496426558436,
124.206944794287)) ;
#43717=CARTESIAN_POINT('Ctrl Pts',(-20.6097246596929,-12.8495893594727,
123.652566976865)) ;
#43718=CARTESIAN_POINT('Ctrl Pts',(-20.9098403565593,-12.6696002791098,
123.712751204342)) ;
#43719=CARTESIAN_POINT('Ctrl Pts',(-20.6198419912611,-12.8694691914299,
123.23005419397)) ;
#43720=CARTESIAN_POINT('Ctrl Pts',(-20.922485985003,-12.689480111067,123.18461209717)) ;
#43721=CARTESIAN_POINT('Ctrl Pts',(-20.4862162340303,-12.8893510427268,
122.828900869269)) ;
#43722=CARTESIAN_POINT('Ctrl Pts',(-20.7554545445051,-12.7093619623639,
122.683172172836)) ;
#43723=CARTESIAN_POINT('Ctrl Pts',(-20.2206736454974,-12.9094220598306,
122.494883082429)) ;
#43724=CARTESIAN_POINT('Ctrl Pts',(-20.4235254244291,-12.7294329794677,
122.265649141046)) ;
#43725=CARTESIAN_POINT('Ctrl Pts',(-19.8617901510047,-12.9292292835837,
122.274337723655)) ;
#43726=CARTESIAN_POINT('Ctrl Pts',(-19.9749237655201,-12.7492402032208,
121.989968961482)) ;
#43727=CARTESIAN_POINT('Ctrl Pts',(-19.4458827143192,-12.9492104191524,
122.187802603992)) ;
#43728=CARTESIAN_POINT('Ctrl Pts',(-19.4550399386783,-12.7692213387896,
121.881799009553)) ;
#43729=CARTESIAN_POINT('Ctrl Pts',(-19.0266575984833,-12.9691379124917,
122.249044591949)) ;
#43730=CARTESIAN_POINT('Ctrl Pts',(-18.9310095255676,-12.7891488321288,
121.958350587305)) ;
#43731=CARTESIAN_POINT('Ctrl Pts',(-18.6546793341104,-12.9889585738495,
122.447395484881)) ;
#43732=CARTESIAN_POINT('Ctrl Pts',(-18.4660378435683,-12.8089694934866,
122.206286369213)) ;
#43733=CARTESIAN_POINT('Ctrl Pts',(-18.3694697209431,-13.0090557630713,
122.765395487489)) ;
#43734=CARTESIAN_POINT('Ctrl Pts',(-18.1095237058468,-12.8290666827084,
122.603786127405)) ;
#43735=CARTESIAN_POINT('Ctrl Pts',(-18.2121462510153,-13.0288194420796,
123.155285689063)) ;
#43736=CARTESIAN_POINT('Ctrl Pts',(-17.9128685242105,-12.8488303617167,
123.091145395877)) ;
#43737=CARTESIAN_POINT('Ctrl Pts',(-18.1966161351743,-13.0488767207527,
123.581287391373)) ;
#43738=CARTESIAN_POINT('Ctrl Pts',(-17.8934532250118,-12.8688876403898,
123.623648070234)) ;
#43739=CARTESIAN_POINT('Ctrl Pts',(-18.3260055582142,-13.0686721445001,
123.981930815811)) ;
#43740=CARTESIAN_POINT('Ctrl Pts',(-18.0551868058746,-12.8886830641372,
124.124451004221)) ;
#43741=CARTESIAN_POINT('Ctrl Pts',(-18.585401546907,-13.0886357892277,124.317872249246)) ;
#43742=CARTESIAN_POINT('Ctrl Pts',(-18.3794288064129,-12.9086467088648,
124.544379679826)) ;
#43743=CARTESIAN_POINT('Ctrl Pts',(-18.9448204747835,-13.1086192805018,
124.544510743668)) ;
#43744=CARTESIAN_POINT('Ctrl Pts',(-18.8287006511552,-12.9286302001389,
124.827680379695)) ;
#43745=CARTESIAN_POINT('Ctrl Pts',(-19.3561968961379,-13.1284267756511,
124.634949141891)) ;
#43746=CARTESIAN_POINT('Ctrl Pts',(-19.3429186866301,-12.9484376952882,
124.94073161998)) ;
#43747=CARTESIAN_POINT('Ctrl Pts',(-19.7773691623945,-13.1484093663712,
124.579587344744)) ;
#43748=CARTESIAN_POINT('Ctrl Pts',(-19.8693844497185,-12.9684202860083,
124.871533418394)) ;
#43749=CARTESIAN_POINT('Ctrl Pts',(-20.1526165065807,-13.1682920203624,
124.384654627234)) ;
#43750=CARTESIAN_POINT('Ctrl Pts',(-20.3384447754671,-12.9883029399995,
124.627871581349)) ;
#43751=CARTESIAN_POINT('Ctrl Pts',(-20.4400164199857,-13.1882502652255,
124.072540016501)) ;
#43752=CARTESIAN_POINT('Ctrl Pts',(-20.6976976848122,-13.0082611848626,
124.237731507644)) ;
#43753=CARTESIAN_POINT('Ctrl Pts',(-20.6032765964651,-13.2081258522671,
123.682670644288)) ;
#43754=CARTESIAN_POINT('Ctrl Pts',(-20.9017768869257,-13.0281367719042,
123.750397269444)) ;
#43755=CARTESIAN_POINT('Ctrl Pts',(-20.6240984710499,-13.2281067404023,
123.258361807286)) ;
#43756=CARTESIAN_POINT('Ctrl Pts',(-20.9278087943981,-13.0481176600395,
123.220011471926)) ;
#43757=CARTESIAN_POINT('Ctrl Pts',(-20.498818644834,-13.2480418815133,122.853364041742)) ;
#43758=CARTESIAN_POINT('Ctrl Pts',(-20.7712144053819,-13.0680528011505,
122.713763278227)) ;
#43759=CARTESIAN_POINT('Ctrl Pts',(-20.2434545299471,-13.2679538995244,
122.515712779495)) ;
#43760=CARTESIAN_POINT('Ctrl Pts',(-20.4520106816014,-13.0879648191615,
122.291696114272)) ;
#43761=CARTESIAN_POINT('Ctrl Pts',(-19.8888180187742,-13.287842117768,122.285335601894)) ;
#43762=CARTESIAN_POINT('Ctrl Pts',(-20.0087285877316,-13.1078530374051,
122.003722192709)) ;
#43763=CARTESIAN_POINT('Ctrl Pts',(-19.5451472567373,-13.3044404216149,
122.205327702706)) ;
#43764=CARTESIAN_POINT('Ctrl Pts',(-19.5791090604564,-13.124451341252,121.903703056221)) ;
#43765=CARTESIAN_POINT('Ctrl Pts',(-19.2662111497509,-13.3177130115177,
122.214345970221)) ;
#43766=CARTESIAN_POINT('Ctrl Pts',(-19.2304680801455,-13.1377239311548,
121.914976366624)) ;
#43767=CARTESIAN_POINT('Ctrl Pts',(-19.0602727562378,-13.3277204264686,
122.257344197933)) ;
#43768=CARTESIAN_POINT('Ctrl Pts',(-18.9730360739325,-13.1477313461057,
121.968723010403)) ;
#43769=CARTESIAN_POINT('Ctrl Pts',(-18.8649743558658,-13.3377277732012,
122.335630979356)) ;
#43770=CARTESIAN_POINT('Ctrl Pts',(-18.7289237747832,-13.1577386928383,
122.066570256317)) ;
#43771=CARTESIAN_POINT('Ctrl Pts',(-18.6279877995192,-13.3509941330028,
122.482594738179)) ;
#43772=CARTESIAN_POINT('Ctrl Pts',(-18.4326373531694,-13.1710050526399,
122.250316913842)) ;
#43773=CARTESIAN_POINT('Ctrl Pts',(-18.38714068302,-13.3675087906257,122.738147005354)) ;
#43774=CARTESIAN_POINT('Ctrl Pts',(-18.1316373287835,-13.1875197102629,
122.569692622284)) ;
#43775=CARTESIAN_POINT('Ctrl Pts',(-18.2465546320846,-13.3841062238684,
123.06176278507)) ;
#43776=CARTESIAN_POINT('Ctrl Pts',(-17.9558681007045,-13.2041171435055,
122.974265631492)) ;
#43777=CARTESIAN_POINT('Ctrl Pts',(-18.2054801703779,-13.3974542210134,
123.339422999475)) ;
#43778=CARTESIAN_POINT('Ctrl Pts',(-17.9045373896821,-13.2174651406505,
123.321302564893)) ;
#43779=CARTESIAN_POINT('Ctrl Pts',(-18.2109540995371,-13.407349975365,123.547385217031)) ;
#43780=CARTESIAN_POINT('Ctrl Pts',(-17.9113737957956,-13.2273608950021,
123.581262925382)) ;
#43781=CARTESIAN_POINT('Ctrl Pts',(-18.2525836667426,-13.4173379292963,
123.753181102987)) ;
#43782=CARTESIAN_POINT('Ctrl Pts',(-17.9634088821012,-13.2373488489335,
123.838506352538)) ;
#43783=CARTESIAN_POINT('Ctrl Pts',(-18.3290068072186,-13.4272951530011,
123.948090648861)) ;
#43784=CARTESIAN_POINT('Ctrl Pts',(-18.0589349739684,-13.2473060726382,
124.082144873651)) ;
#43785=CARTESIAN_POINT('Ctrl Pts',(-18.4390335780382,-13.4373306995577,
124.128090732076)) ;
#43786=CARTESIAN_POINT('Ctrl Pts',(-18.1964661586106,-13.2573416191949,
124.307146372465)) ;
#43787=CARTESIAN_POINT('Ctrl Pts',(-18.576478403772,-13.4472178108339,124.284038519252)) ;
#43788=CARTESIAN_POINT('Ctrl Pts',(-18.3682700533626,-13.267228730471,124.502082982706)) ;
#43789=CARTESIAN_POINT('Ctrl Pts',(-18.7403986017361,-13.4572092159347,
124.415367414347)) ;
#43790=CARTESIAN_POINT('Ctrl Pts',(-18.573168600081,-13.2772201355718,124.666246335832)) ;
#43791=CARTESIAN_POINT('Ctrl Pts',(-18.9238269690954,-13.4671548371495,
124.515725679001)) ;
#43792=CARTESIAN_POINT('Ctrl Pts',(-18.8024527486924,-13.2871657567866,
124.791696662128)) ;
#43793=CARTESIAN_POINT('Ctrl Pts',(-19.1218420695638,-13.4771040854178,
124.583140773883)) ;
#43794=CARTESIAN_POINT('Ctrl Pts',(-19.0499707909462,-13.2971150050549,
124.87596822317)) ;
#43795=CARTESIAN_POINT('Ctrl Pts',(-19.3305917291493,-13.4871505805864,
124.615215322897)) ;
#43796=CARTESIAN_POINT('Ctrl Pts',(-19.3109074952385,-13.3071615002235,
124.91606420447)) ;
#43797=CARTESIAN_POINT('Ctrl Pts',(-19.5376622730773,-13.4970019233779,
124.610852955936)) ;
#43798=CARTESIAN_POINT('Ctrl Pts',(-19.5697458477253,-13.3170128430151,
124.910614060128)) ;
#43799=CARTESIAN_POINT('Ctrl Pts',(-19.7433819757979,-13.5069737035053,
124.570637442649)) ;
#43800=CARTESIAN_POINT('Ctrl Pts',(-19.8268961278364,-13.3269846231424,
124.86034740168)) ;
#43801=CARTESIAN_POINT('Ctrl Pts',(-19.9394995576033,-13.516968903483,124.495094530682)) ;
#43802=CARTESIAN_POINT('Ctrl Pts',(-20.0720441858723,-13.3369798231201,
124.765921346646)) ;
#43803=CARTESIAN_POINT('Ctrl Pts',(-20.1200428835865,-13.527002895179,124.386031569206)) ;
#43804=CARTESIAN_POINT('Ctrl Pts',(-20.2977248332106,-13.3470138148161,
124.629595035348)) ;
#43805=CARTESIAN_POINT('Ctrl Pts',(-20.2763242405218,-13.5368583001515,
124.249969630593)) ;
#43806=CARTESIAN_POINT('Ctrl Pts',(-20.4930785404264,-13.3568692197886,
124.459519571124)) ;
#43807=CARTESIAN_POINT('Ctrl Pts',(-20.4086965221813,-13.5468575979973,
124.086710547082)) ;
#43808=CARTESIAN_POINT('Ctrl Pts',(-20.6585461151986,-13.3668685176344,
124.255447402342)) ;
#43809=CARTESIAN_POINT('Ctrl Pts',(-20.5098783796781,-13.5567527106025,
123.904908826794)) ;
#43810=CARTESIAN_POINT('Ctrl Pts',(-20.7850259763668,-13.3767636302396,
124.028196369691)) ;
#43811=CARTESIAN_POINT('Ctrl Pts',(-20.5790528982995,-13.5668133561375,
123.705062953625)) ;
#43812=CARTESIAN_POINT('Ctrl Pts',(-20.8714967332555,-13.3868242757746,
123.778389961119)) ;
#43813=CARTESIAN_POINT('Ctrl Pts',(-20.6118978850877,-13.5766622331267,
123.500614031643)) ;
#43814=CARTESIAN_POINT('Ctrl Pts',(-20.9125557494614,-13.3966731527638,
123.522828864941)) ;
#43815=CARTESIAN_POINT('Ctrl Pts',(-20.6092193159514,-13.5866909442203,
123.289798847138)) ;
#43816=CARTESIAN_POINT('Ctrl Pts',(-20.9092102411542,-13.4067018638574,
123.259309807964)) ;
#43817=CARTESIAN_POINT('Ctrl Pts',(-20.5694097322058,-13.5967203454764,
123.082737299415)) ;
#43818=CARTESIAN_POINT('Ctrl Pts',(-20.8594509750379,-13.4167312651135,
123.00048234628)) ;
#43819=CARTESIAN_POINT('Ctrl Pts',(-20.4961008853216,-13.6065605372724,
122.889286624956)) ;
#43820=CARTESIAN_POINT('Ctrl Pts',(-20.7678172835609,-13.4265714569095,
122.758667592175)) ;
#43821=CARTESIAN_POINT('Ctrl Pts',(-20.3889086577013,-13.6165639664654,
122.708376154055)) ;
#43822=CARTESIAN_POINT('Ctrl Pts',(-20.6338292437046,-13.4365748861025,
122.532528063033)) ;
#43823=CARTESIAN_POINT('Ctrl Pts',(-20.2520895253684,-13.6265494789316,
122.549112630056)) ;
#43824=CARTESIAN_POINT('Ctrl Pts',(-20.4628072717642,-13.4465603985687,
122.333446821148)) ;
#43825=CARTESIAN_POINT('Ctrl Pts',(-20.0887000777735,-13.6365905753156,
122.415484766701)) ;
#43826=CARTESIAN_POINT('Ctrl Pts',(-20.258572195235,-13.4566014949527,122.16640991458)) ;
#43827=CARTESIAN_POINT('Ctrl Pts',(-19.9083265613386,-13.6464337712666,
122.314020661915)) ;
#43828=CARTESIAN_POINT('Ctrl Pts',(-20.0331061121126,-13.4664446909037,
122.03957718795)) ;
#43829=CARTESIAN_POINT('Ctrl Pts',(-19.7104267761794,-13.656420082321,122.244041727144)) ;
#43830=CARTESIAN_POINT('Ctrl Pts',(-19.7857320971472,-13.4764310019581,
121.952101012445)) ;
#43831=CARTESIAN_POINT('Ctrl Pts',(-19.5044018483537,-13.6663547675787,
122.209514866081)) ;
#43832=CARTESIAN_POINT('Ctrl Pts',(-19.5282010411868,-13.4863656872158,
121.908939847016)) ;
#43833=CARTESIAN_POINT('Ctrl Pts',(-19.2929999960134,-13.6764123287957,
122.211492627575)) ;
#43834=CARTESIAN_POINT('Ctrl Pts',(-19.2639488168614,-13.4964232484328,
121.911409438826)) ;
#43835=CARTESIAN_POINT('Ctrl Pts',(-19.0899192604328,-13.6862339704043,
122.248938878938)) ;
#43836=CARTESIAN_POINT('Ctrl Pts',(-19.0100966675528,-13.5062448900414,
121.958214888149)) ;
#43837=CARTESIAN_POINT('Ctrl Pts',(-18.8917066678072,-13.6962900339953,
122.32241535315)) ;
#43838=CARTESIAN_POINT('Ctrl Pts',(-18.7623301682284,-13.5163009536324,
122.050058119956)) ;
#43839=CARTESIAN_POINT('Ctrl Pts',(-18.711524790799,-13.7062307097571,122.428304767284)) ;
#43840=CARTESIAN_POINT('Ctrl Pts',(-18.5371012425962,-13.5262416293942,
122.182417857288)) ;
#43841=CARTESIAN_POINT('Ctrl Pts',(-18.5526279674509,-13.7161350685454,
122.562874462865)) ;
#43842=CARTESIAN_POINT('Ctrl Pts',(-18.338478245611,-13.5361459881825,122.350628473911)) ;
#43843=CARTESIAN_POINT('Ctrl Pts',(-18.4177132106572,-13.7261817231212,
122.725360080974)) ;
#43844=CARTESIAN_POINT('Ctrl Pts',(-18.1698329826385,-13.5461926427583,
122.553733855565)) ;
#43845=CARTESIAN_POINT('Ctrl Pts',(-18.3144502475993,-13.7360773177641,
122.905994660676)) ;
#43846=CARTESIAN_POINT('Ctrl Pts',(-18.0407519036657,-13.5560882374012,
122.779526388176)) ;
#43847=CARTESIAN_POINT('Ctrl Pts',(-18.2429366007976,-13.7461392644209,
123.105048153552)) ;
#43848=CARTESIAN_POINT('Ctrl Pts',(-17.9513576421501,-13.5661501840581,
123.028342279855)) ;
#43849=CARTESIAN_POINT('Ctrl Pts',(-18.2077846553653,-13.7559888883531,
123.309123594396)) ;
#43850=CARTESIAN_POINT('Ctrl Pts',(-17.9074152113575,-13.5759998079902,
123.283436990171)) ;
#43851=CARTESIAN_POINT('Ctrl Pts',(-18.2079178316408,-13.7659521273829,
123.518569880535)) ;
#43852=CARTESIAN_POINT('Ctrl Pts',(-17.9075794490051,-13.5859630470201,
123.545245160118)) ;
#43853=CARTESIAN_POINT('Ctrl Pts',(-18.2449311630796,-13.7759767021588,
123.726054826624)) ;
#43854=CARTESIAN_POINT('Ctrl Pts',(-17.9538438452054,-13.5959876217959,
123.804601716854)) ;
#43855=CARTESIAN_POINT('Ctrl Pts',(-18.3165097926261,-13.7858952648465,
123.921897886242)) ;
#43856=CARTESIAN_POINT('Ctrl Pts',(-18.0433151854202,-13.6059061844836,
124.0494068293)) ;
#43857=CARTESIAN_POINT('Ctrl Pts',(-18.4214705157971,-13.7958874515705,
124.103877790771)) ;
#43858=CARTESIAN_POINT('Ctrl Pts',(-18.1745142883211,-13.6158983712076,
124.276882942804)) ;
#43859=CARTESIAN_POINT('Ctrl Pts',(-18.5572880042135,-13.8059222501547,
124.265295046581)) ;
#43860=CARTESIAN_POINT('Ctrl Pts',(-18.3442843563806,-13.6259331697918,
124.478655912716)) ;
#43861=CARTESIAN_POINT('Ctrl Pts',(-18.7159640539968,-13.8157774408283,
124.398542881549)) ;
#43862=CARTESIAN_POINT('Ctrl Pts',(-18.5426287178468,-13.6357883604655,
124.645217964009)) ;
#43863=CARTESIAN_POINT('Ctrl Pts',(-18.8978051688274,-13.8257767889813,
124.503949795873)) ;
#43864=CARTESIAN_POINT('Ctrl Pts',(-18.7699291705974,-13.6457877086185,
124.776978497853)) ;
#43865=CARTESIAN_POINT('Ctrl Pts',(-19.0931163675303,-13.8356719146565,
124.575663890585)) ;
#43866=CARTESIAN_POINT('Ctrl Pts',(-19.0140681533579,-13.6556828342936,
124.86662328346)) ;
#43867=CARTESIAN_POINT('Ctrl Pts',(-19.3012793398308,-13.8457324576046,
124.612957137398)) ;
#43868=CARTESIAN_POINT('Ctrl Pts',(-19.2742712713222,-13.6657433772417,
124.913241817981)) ;
#43869=CARTESIAN_POINT('Ctrl Pts',(-19.5083568286429,-13.8555817318715,
124.613644904383)) ;
#43870=CARTESIAN_POINT('Ctrl Pts',(-19.5331191647968,-13.6755926515086,
124.914103544901)) ;
#43871=CARTESIAN_POINT('Ctrl Pts',(-19.7161637957389,-13.8656089564414,
124.578258675114)) ;
#43872=CARTESIAN_POINT('Ctrl Pts',(-19.792878148494,-13.6856198760785,124.869872597639)) ;
#43873=CARTESIAN_POINT('Ctrl Pts',(-19.9145234172926,-13.8756373556292,
124.506794850628)) ;
#43874=CARTESIAN_POINT('Ctrl Pts',(-20.0408282968694,-13.6956482752663,
124.780544744153)) ;
#43875=CARTESIAN_POINT('Ctrl Pts',(-20.0942981409798,-13.8854831060427,
124.404230045374)) ;
#43876=CARTESIAN_POINT('Ctrl Pts',(-20.2655486146661,-13.7054940256798,
124.652339842706)) ;
#43877=CARTESIAN_POINT('Ctrl Pts',(-20.2562410694359,-13.8954718964434,
124.27052516634)) ;
#43878=CARTESIAN_POINT('Ctrl Pts',(-20.4679785318478,-13.7154828160805,
124.485209945321)) ;
#43879=CARTESIAN_POINT('Ctrl Pts',(-20.3928548044161,-13.9055168248431,
124.109502618488)) ;
#43880=CARTESIAN_POINT('Ctrl Pts',(-20.6387470354959,-13.7255277444802,
124.283933112254)) ;
#43881=CARTESIAN_POINT('Ctrl Pts',(-20.4975212772136,-13.9153413096321,
123.931431530893)) ;
#43882=CARTESIAN_POINT('Ctrl Pts',(-20.7695822850911,-13.7353522292692,
124.061344007578)) ;
#43883=CARTESIAN_POINT('Ctrl Pts',(-20.5716663162285,-13.9253987071733,
123.733438159543)) ;
#43884=CARTESIAN_POINT('Ctrl Pts',(-20.8622650301573,-13.7454096268104,
123.813853115559)) ;
#43885=CARTESIAN_POINT('Ctrl Pts',(-20.6095387245746,-13.9353247987595,
123.528210702811)) ;
#43886=CARTESIAN_POINT('Ctrl Pts',(-20.9096073544687,-13.7553357183966,
123.557318498504)) ;
#43887=CARTESIAN_POINT('Ctrl Pts',(-20.6117482503137,-13.945279583904,123.318943735867)) ;
#43888=CARTESIAN_POINT('Ctrl Pts',(-20.9123708210729,-13.7652905035412,
123.295734355723)) ;
#43889=CARTESIAN_POINT('Ctrl Pts',(-20.5770731565774,-13.9553169535617,
123.110795951615)) ;
#43890=CARTESIAN_POINT('Ctrl Pts',(-20.8690285856397,-13.7753278731988,
123.035549479101)) ;
#43891=CARTESIAN_POINT('Ctrl Pts',(-20.5079730266207,-13.9652057636833,
122.914716225052)) ;
#43892=CARTESIAN_POINT('Ctrl Pts',(-20.7826546061871,-13.7852166833204,
122.790448432935)) ;
#43893=CARTESIAN_POINT('Ctrl Pts',(-20.4051720006662,-13.9751951227343,
122.731595284921)) ;
#43894=CARTESIAN_POINT('Ctrl Pts',(-20.6541544832906,-13.7952060423715,
122.561546360115)) ;
#43895=CARTESIAN_POINT('Ctrl Pts',(-20.2724273246368,-13.9851536701904,
122.569707167163)) ;
#43896=CARTESIAN_POINT('Ctrl Pts',(-20.4882245281512,-13.8051645898276,
122.359184924028)) ;
#43897=CARTESIAN_POINT('Ctrl Pts',(-20.1148509111908,-13.9950532467415,
122.433733040983)) ;
#43898=CARTESIAN_POINT('Ctrl Pts',(-20.2912542115885,-13.8150641663786,
122.189215690163)) ;
#43899=CARTESIAN_POINT('Ctrl Pts',(-19.9333707547642,-14.0051011585722,
122.32566998488)) ;
#43900=CARTESIAN_POINT('Ctrl Pts',(-20.0644048944981,-13.8251120782093,
122.054135819925)) ;
#43901=CARTESIAN_POINT('Ctrl Pts',(-19.738890370448,-14.0149965064327,122.251724804565)) ;
#43902=CARTESIAN_POINT('Ctrl Pts',(-19.8213040212289,-13.8350074260699,
121.961702812424)) ;
#43903=CARTESIAN_POINT('Ctrl Pts',(-19.5311506381738,-14.0250581829639,
122.211995828632)) ;
#43904=CARTESIAN_POINT('Ctrl Pts',(-19.5616299165928,-13.845069102601,121.912040392459)) ;
#43905=CARTESIAN_POINT('Ctrl Pts',(-19.3242027583877,-14.0349027007131,
122.208972747124)) ;
#43906=CARTESIAN_POINT('Ctrl Pts',(-19.302943765994,-13.8549136203502,121.908260248801)) ;
#43907=CARTESIAN_POINT('Ctrl Pts',(-19.1173623183453,-14.0448631444279,
122.241578718461)) ;
#43908=CARTESIAN_POINT('Ctrl Pts',(-19.0443926106772,-13.864874064065,121.949016797608)) ;
#43909=CARTESIAN_POINT('Ctrl Pts',(-18.917933653831,-14.0548999772461,122.310497086348)) ;
#43910=CARTESIAN_POINT('Ctrl Pts',(-18.7951065533296,-13.8749108968832,
122.035163624274)) ;
#43911=CARTESIAN_POINT('Ctrl Pts',(-18.7362181804366,-14.0647787739929,
122.41109597588)) ;
#43912=CARTESIAN_POINT('Ctrl Pts',(-18.5679607592807,-13.88478969363,122.160911880469)) ;
#43913=CARTESIAN_POINT('Ctrl Pts',(-18.5717693082948,-14.0748380901212,
122.544026993693)) ;
#43914=CARTESIAN_POINT('Ctrl Pts',(-18.3623992980865,-13.8948490097584,
122.327074678705)) ;
#43915=CARTESIAN_POINT('Ctrl Pts',(-18.4354824503582,-14.0847085368744,
122.700520863806)) ;
#43916=CARTESIAN_POINT('Ctrl Pts',(-18.1920392191495,-13.9047194565116,
122.522692233472)) ;
#43917=CARTESIAN_POINT('Ctrl Pts',(-18.3266320599271,-14.0947011751325,
122.880198948747)) ;
#43918=CARTESIAN_POINT('Ctrl Pts',(-18.0559754687445,-13.9147120947696,
122.747289602296)) ;
#43919=CARTESIAN_POINT('Ctrl Pts',(-18.2507605415013,-14.1047331906804,
123.076976227112)) ;
#43920=CARTESIAN_POINT('Ctrl Pts',(-17.9611352243635,-13.9247441103175,
122.993260746216)) ;
#43921=CARTESIAN_POINT('Ctrl Pts',(-18.2104322023642,-14.114599046987,123.280449832988)) ;
#43922=CARTESIAN_POINT('Ctrl Pts',(-17.9107237978205,-13.9346099666241,
123.247603809028)) ;
#43923=CARTESIAN_POINT('Ctrl Pts',(-18.2059368718994,-14.1246683364561,
123.492066961254)) ;
#43924=CARTESIAN_POINT('Ctrl Pts',(-17.9051038745564,-13.9446792560932,
123.512124786768)) ;
#43925=CARTESIAN_POINT('Ctrl Pts',(-18.2375102294898,-14.1345118940074,
123.696598560914)) ;
#43926=CARTESIAN_POINT('Ctrl Pts',(-17.9445700338335,-13.9545228136445,
123.767790796992)) ;
#43927=CARTESIAN_POINT('Ctrl Pts',(-18.3043848267997,-14.1444920207952,
123.895462028567)) ;
#43928=CARTESIAN_POINT('Ctrl Pts',(-18.0281629110103,-13.9645029404324,
124.016370584098)) ;
#43929=CARTESIAN_POINT('Ctrl Pts',(-18.4055151657071,-14.1545105693952,
124.080209802711)) ;
#43930=CARTESIAN_POINT('Ctrl Pts',(-18.1545752563571,-13.9745214890323,
124.247305606012)) ;
#43931=CARTESIAN_POINT('Ctrl Pts',(-18.5350837698109,-14.1643938699184,
124.242672415459)) ;
#43932=CARTESIAN_POINT('Ctrl Pts',(-18.3165363213439,-13.9844047895555,
124.450385027953)) ;
#43933=CARTESIAN_POINT('Ctrl Pts',(-18.6938257864244,-14.1744621569665,
124.382634186157)) ;
#43934=CARTESIAN_POINT('Ctrl Pts',(-18.5149631927261,-13.9944730766036,
124.625337357405)) ;
#43935=CARTESIAN_POINT('Ctrl Pts',(-18.8701172743958,-14.1842922799851,
124.490542166158)) ;
#43936=CARTESIAN_POINT('Ctrl Pts',(-18.7353286473751,-14.0043031996223,
124.760223493667)) ;
#43937=CARTESIAN_POINT('Ctrl Pts',(-19.0669291678649,-14.1943588639105,
124.568249490539)) ;
#43938=CARTESIAN_POINT('Ctrl Pts',(-18.9813430292803,-14.0143697835476,
124.857357794633)) ;
#43939=CARTESIAN_POINT('Ctrl Pts',(-19.2706943838824,-14.2042489769249,
124.609750952324)) ;
#43940=CARTESIAN_POINT('Ctrl Pts',(-19.2360505050157,-14.0242598965621,
124.909235187301)) ;
#43941=CARTESIAN_POINT('Ctrl Pts',(-19.4806689201278,-14.2142416656876,
124.615742309981)) ;
#43942=CARTESIAN_POINT('Ctrl Pts',(-19.4985188781141,-14.0342525853247,
124.916724579482)) ;
#43943=CARTESIAN_POINT('Ctrl Pts',(-19.6878386126546,-14.2242025540433,
124.585132160337)) ;
#43944=CARTESIAN_POINT('Ctrl Pts',(-19.7574815058424,-14.0442134736805,
124.878462065094)) ;
#43945=CARTESIAN_POINT('Ctrl Pts',(-19.8857808498602,-14.2341204989233,
124.519648220953)) ;
#43946=CARTESIAN_POINT('Ctrl Pts',(-20.0049101277491,-14.0541314185605,
124.796606975513)) ;
#43947=CARTESIAN_POINT('Ctrl Pts',(-20.0711543280967,-14.2441282520195,
124.42009338198)) ;
#43948=CARTESIAN_POINT('Ctrl Pts',(-20.2366270328514,-14.0641391716567,
124.672163407092)) ;
#43949=CARTESIAN_POINT('Ctrl Pts',(-20.2365214427845,-14.2541593459786,
124.289244206464)) ;
#43950=CARTESIAN_POINT('Ctrl Pts',(-20.4433359395377,-14.0741702656157,
124.508602153767)) ;
#43951=CARTESIAN_POINT('Ctrl Pts',(-20.3744629268658,-14.2640073140066,
124.134836918703)) ;
#43952=CARTESIAN_POINT('Ctrl Pts',(-20.6157637308144,-14.0840182336437,
124.315591986878)) ;
#43953=CARTESIAN_POINT('Ctrl Pts',(-20.4860083257482,-14.2740692701324,
123.95512196643)) ;
#43954=CARTESIAN_POINT('Ctrl Pts',(-20.7551952257147,-14.0940801897696,
124.090948556963)) ;
#43955=CARTESIAN_POINT('Ctrl Pts',(-20.5631955250995,-14.2839664817336,
123.761889219392)) ;
#43956=CARTESIAN_POINT('Ctrl Pts',(-20.8516795936219,-14.1039774013707,
123.849406694872)) ;
#43957=CARTESIAN_POINT('Ctrl Pts',(-20.6064757403202,-14.2938976483982,
123.557644080804)) ;
#43958=CARTESIAN_POINT('Ctrl Pts',(-20.9057797422551,-14.1139085680353,
123.594099508417)) ;
#43959=CARTESIAN_POINT('Ctrl Pts',(-20.6134856977865,-14.3039398326024,
123.346645043293)) ;
#43960=CARTESIAN_POINT('Ctrl Pts',(-20.9145419978762,-14.1239507522395,
123.330350913867)) ;
#43961=CARTESIAN_POINT('Ctrl Pts',(-20.5843602960543,-14.3138265008555,
123.140837465138)) ;
#43962=CARTESIAN_POINT('Ctrl Pts',(-20.878134852128,-14.1338374204927,123.073090399106)) ;
#43963=CARTESIAN_POINT('Ctrl Pts',(-20.5195898101172,-14.3238196128338,
122.940995926319)) ;
#43964=CARTESIAN_POINT('Ctrl Pts',(-20.797171317607,-14.1438305324709,122.823288399636)) ;
#43965=CARTESIAN_POINT('Ctrl Pts',(-20.4214970858592,-14.3337652904496,
122.756344163075)) ;
#43966=CARTESIAN_POINT('Ctrl Pts',(-20.6745548235997,-14.1537762100867,
122.592473334251)) ;
#43967=CARTESIAN_POINT('Ctrl Pts',(-20.2931422169085,-14.3437125934346,
122.591232662632)) ;
#43968=CARTESIAN_POINT('Ctrl Pts',(-20.5141104749864,-14.1637235130717,
122.386083823547)) ;
#43969=CARTESIAN_POINT('Ctrl Pts',(-20.1363573288779,-14.3537603171813,
122.449682535313)) ;
#43970=CARTESIAN_POINT('Ctrl Pts',(-20.3181292651246,-14.1737712368185,
122.209146648077)) ;
#43971=CARTESIAN_POINT('Ctrl Pts',(-19.9610119228354,-14.3636086909439,
122.339593196702)) ;
#43972=CARTESIAN_POINT('Ctrl Pts',(-20.098946063385,-14.183619610581,122.071534647514)) ;
#43973=CARTESIAN_POINT('Ctrl Pts',(-19.7673215762674,-14.3735676633896,
122.260098624231)) ;
#43974=CARTESIAN_POINT('Ctrl Pts',(-19.8568324061559,-14.1935785830267,
121.972166958928)) ;
#43975=CARTESIAN_POINT('Ctrl Pts',(-19.5610549600458,-14.3836065252707,
122.215459746428)) ;
#43976=CARTESIAN_POINT('Ctrl Pts',(-19.5989991593622,-14.2036174449079,
121.916368996619)) ;
#43977=CARTESIAN_POINT('Ctrl Pts',(-19.3535221005735,-14.3934851294425,
122.207111470236)) ;
#43978=CARTESIAN_POINT('Ctrl Pts',(-19.339581937027,-14.2134960490797,121.905934350721)) ;
#43979=CARTESIAN_POINT('Ctrl Pts',(-19.1441263617507,-14.4035366706458,
122.235315239726)) ;
#43980=CARTESIAN_POINT('Ctrl Pts',(-19.0778376414756,-14.223547590283,121.941189793871)) ;
#43981=CARTESIAN_POINT('Ctrl Pts',(-18.9458547057129,-14.4134320686262,
122.298408849419)) ;
#43982=CARTESIAN_POINT('Ctrl Pts',(-18.8299973984445,-14.2334429882633,
122.020057862292)) ;
#43983=CARTESIAN_POINT('Ctrl Pts',(-18.7586516298394,-14.4234833011715,
122.396359934609)) ;
#43984=CARTESIAN_POINT('Ctrl Pts',(-18.5959941772312,-14.2434942208086,
122.142497343035)) ;
#43985=CARTESIAN_POINT('Ctrl Pts',(-18.5939939088903,-14.4333694917958,
122.523221653132)) ;
#43986=CARTESIAN_POINT('Ctrl Pts',(-18.3901717062413,-14.2533804114329,
122.301075810793)) ;
#43987=CARTESIAN_POINT('Ctrl Pts',(-18.4520997591911,-14.4433620311115,
122.678107054398)) ;
#43988=CARTESIAN_POINT('Ctrl Pts',(-18.2128046217201,-14.2633729507487,
122.494683384681)) ;
#43989=CARTESIAN_POINT('Ctrl Pts',(-18.3397922812975,-14.4533104770063,
122.854559106031)) ;
#43990=CARTESIAN_POINT('Ctrl Pts',(-18.0724208014174,-14.2733213966434,
122.715249428786)) ;
#43991=CARTESIAN_POINT('Ctrl Pts',(-18.2596593833855,-14.4632472795382,
123.047461897236)) ;
#43992=CARTESIAN_POINT('Ctrl Pts',(-17.9722554347127,-14.2832581991753,
122.956378922665)) ;
#43993=CARTESIAN_POINT('Ctrl Pts',(-18.2137581958001,-14.4732302869895,
123.252282638572)) ;
#43994=CARTESIAN_POINT('Ctrl Pts',(-17.9148800450432,-14.2932412066266,
123.212405357803)) ;
#43995=CARTESIAN_POINT('Ctrl Pts',(-18.2044493527583,-14.4832741284043,
123.463206431544)) ;
#43996=CARTESIAN_POINT('Ctrl Pts',(-17.9032450354326,-14.3032850480414,
123.476059954926)) ;
#43997=CARTESIAN_POINT('Ctrl Pts',(-18.2308383801991,-14.4931023270282,
123.668165335843)) ;
#43998=CARTESIAN_POINT('Ctrl Pts',(-17.9362327116183,-14.3131132466653,
123.732259863028)) ;
#43999=CARTESIAN_POINT('Ctrl Pts',(-18.2938523410951,-14.5031789204704,
123.870372485691)) ;
#44000=CARTESIAN_POINT('Ctrl Pts',(-18.0150012319065,-14.3231898401075,
123.985018013429)) ;
#44001=CARTESIAN_POINT('Ctrl Pts',(-18.3887993193818,-14.513030919812,124.0544990199)) ;
#44002=CARTESIAN_POINT('Ctrl Pts',(-18.1336866675862,-14.3330418394491,
124.215176688599)) ;
#44003=CARTESIAN_POINT('Ctrl Pts',(-18.516907971024,-14.5231045066358,124.223090197898)) ;
#44004=CARTESIAN_POINT('Ctrl Pts',(-18.2938233161721,-14.343115426273,124.425914520946)) ;
#44005=CARTESIAN_POINT('Ctrl Pts',(-18.6688091775145,-14.5329447317333,
124.363553032254)) ;
#44006=CARTESIAN_POINT('Ctrl Pts',(-18.4837016929012,-14.3529556513705,
124.601492972209)) ;
#44007=CARTESIAN_POINT('Ctrl Pts',(-18.8445804362272,-14.542910435762,124.477535027406)) ;
#44008=CARTESIAN_POINT('Ctrl Pts',(-18.703416961841,-14.3629213553991,124.743969337012)) ;
#44009=CARTESIAN_POINT('Ctrl Pts',(-19.0387987115393,-14.5529370690686,
124.559495745125)) ;
#44010=CARTESIAN_POINT('Ctrl Pts',(-18.946190326884,-14.3729479887057,124.846418837597)) ;
#44011=CARTESIAN_POINT('Ctrl Pts',(-19.2419467311579,-14.5628513647804,
124.606096057943)) ;
#44012=CARTESIAN_POINT('Ctrl Pts',(-19.2001264119849,-14.3828622844175,
124.904667897107)) ;
#44013=CARTESIAN_POINT('Ctrl Pts',(-19.4516521953088,-14.5728396534728,
124.61717510903)) ;
#44014=CARTESIAN_POINT('Ctrl Pts',(-19.4622585243968,-14.39285057311,124.918515058784)) ;
#44015=CARTESIAN_POINT('Ctrl Pts',(-19.6610834565671,-14.5828783866312,
124.591166378612)) ;
#44016=CARTESIAN_POINT('Ctrl Pts',(-19.7240472766002,-14.4028893062683,
124.886002641431)) ;
#44017=CARTESIAN_POINT('Ctrl Pts',(-19.858998903738,-14.5927217184587,124.530728055798)) ;
#44018=CARTESIAN_POINT('Ctrl Pts',(-19.9714422784701,-14.4127326380959,
124.810452799983)) ;
#44019=CARTESIAN_POINT('Ctrl Pts',(-20.0470907094626,-14.6027494443383,
124.43551748704)) ;
#44020=CARTESIAN_POINT('Ctrl Pts',(-20.2065561510804,-14.4227603639755,
124.691438006509)) ;
#44021=CARTESIAN_POINT('Ctrl Pts',(-20.215531250739,-14.6127817807269,124.308574127084)) ;
#44022=CARTESIAN_POINT('Ctrl Pts',(-20.4171057819061,-14.432792700364,124.532757562362)) ;
#44023=CARTESIAN_POINT('Ctrl Pts',(-20.3567549827595,-14.6226112810275,
124.157731091938)) ;
#44024=CARTESIAN_POINT('Ctrl Pts',(-20.5936350310893,-14.4426222006646,
124.34420163555)) ;
#44025=CARTESIAN_POINT('Ctrl Pts',(-20.4720182760222,-14.6326007849443,
123.982171250015)) ;
#44026=CARTESIAN_POINT('Ctrl Pts',(-20.7377126082824,-14.4526117045814,
124.124750610571)) ;
#44027=CARTESIAN_POINT('Ctrl Pts',(-20.5550029183584,-14.6426446254567,
123.788010434387)) ;
#44028=CARTESIAN_POINT('Ctrl Pts',(-20.8414417058682,-14.4626555450938,
123.882049023559)) ;
#44029=CARTESIAN_POINT('Ctrl Pts',(-20.6023692510491,-14.6524663312247,
123.587034176731)) ;
#44030=CARTESIAN_POINT('Ctrl Pts',(-20.900648035962,-14.4724772508619,123.63082704311)) ;
#44031=CARTESIAN_POINT('Ctrl Pts',(-20.614891393778,-14.6625013783571,123.376438673923)) ;
#44032=CARTESIAN_POINT('Ctrl Pts',(-20.9162986354435,-14.4825122979942,
123.367582647658)) ;
#44033=CARTESIAN_POINT('Ctrl Pts',(-20.5901024671484,-14.672526055794,123.167143676446)) ;
#44034=CARTESIAN_POINT('Ctrl Pts',(-20.8853105895479,-14.4925369754311,
123.105964149167)) ;
#44035=CARTESIAN_POINT('Ctrl Pts',(-20.5308125782497,-14.6823788706484,
122.968674050456)) ;
#44036=CARTESIAN_POINT('Ctrl Pts',(-20.8111959911623,-14.5023897902856,
122.85787673168)) ;
#44037=CARTESIAN_POINT('Ctrl Pts',(-20.4370276643577,-14.692366580256,122.780826892626)) ;
#44038=CARTESIAN_POINT('Ctrl Pts',(-20.6939628548545,-14.5123774998931,
122.623068574786)) ;
#44039=CARTESIAN_POINT('Ctrl Pts',(-20.3127672555841,-14.7022965902501,
122.613067626526)) ;
#44040=CARTESIAN_POINT('Ctrl Pts',(-20.5386353139162,-14.5223075098872,
122.413370344863)) ;
#44041=CARTESIAN_POINT('Ctrl Pts',(-20.1605796757999,-14.7122863454692,
122.468335495329)) ;
#44042=CARTESIAN_POINT('Ctrl Pts',(-20.3483991859879,-14.5322972651064,
122.232456679631)) ;
#44043=CARTESIAN_POINT('Ctrl Pts',(-19.9847778139171,-14.7223129541521,
122.352025348161)) ;
#44044=CARTESIAN_POINT('Ctrl Pts',(-20.1286457021689,-14.5423238737893,
122.087070807904)) ;
#44045=CARTESIAN_POINT('Ctrl Pts',(-19.7942886748206,-14.732196894174,122.269022419418)) ;
#44046=CARTESIAN_POINT('Ctrl Pts',(-19.8905327192245,-14.5522078138111,
121.983318872916)) ;
#44047=CARTESIAN_POINT('Ctrl Pts',(-19.5902331312652,-14.7421861217125,
122.219359207184)) ;
#44048=CARTESIAN_POINT('Ctrl Pts',(-19.635462587809,-14.5621970413496,121.921242080345)) ;
#44049=CARTESIAN_POINT('Ctrl Pts',(-19.3795093368715,-14.7522289922362,
122.206246194729)) ;
#44050=CARTESIAN_POINT('Ctrl Pts',(-19.3720577988296,-14.5722399118733,
121.904853033029)) ;
#44051=CARTESIAN_POINT('Ctrl Pts',(-19.1740714005142,-14.7620613789916,
122.229097308269)) ;
#44052=CARTESIAN_POINT('Ctrl Pts',(-19.1152596800331,-14.5820722986287,
121.933419317847)) ;
#44053=CARTESIAN_POINT('Ctrl Pts',(-18.9723061416938,-14.7720546721632,
122.287639558838)) ;
#44054=CARTESIAN_POINT('Ctrl Pts',(-18.8630536665113,-14.5920655918003,
122.006599511882)) ;
#44055=CARTESIAN_POINT('Ctrl Pts',(-18.7832226625352,-14.7820866778116,
122.381086795298)) ;
#44056=CARTESIAN_POINT('Ctrl Pts',(-18.6267003875226,-14.6020975974487,
122.123410637976)) ;
#44057=CARTESIAN_POINT('Ctrl Pts',(-18.6159274829548,-14.7919519337806,
122.503651125695)) ;
#44058=CARTESIAN_POINT('Ctrl Pts',(-18.4175822404663,-14.6119628534177,
122.276618419926)) ;
#44059=CARTESIAN_POINT('Ctrl Pts',(-18.4706094581403,-14.8019138136881,
122.654469653778)) ;
#44060=CARTESIAN_POINT('Ctrl Pts',(-18.2359363520061,-14.6219247333252,
122.465143513999)) ;
#44061=CARTESIAN_POINT('Ctrl Pts',(-18.3531243947538,-14.81194874705,122.829681165894)) ;
#44062=CARTESIAN_POINT('Ctrl Pts',(-18.0890820796082,-14.6319596666871,
122.684159241081)) ;
#44063=CARTESIAN_POINT('Ctrl Pts',(-18.2687841779479,-14.8218337054293,
123.019642132794)) ;
#44064=CARTESIAN_POINT('Ctrl Pts',(-17.9836588830903,-14.6418446250664,
122.921611991648)) ;
#44065=CARTESIAN_POINT('Ctrl Pts',(-18.2178545293784,-14.8318993323519,
123.224997323136)) ;
#44066=CARTESIAN_POINT('Ctrl Pts',(-17.91999930049,-14.6519102519891,123.178306439075)) ;
#44067=CARTESIAN_POINT('Ctrl Pts',(-18.2034666313483,-14.8417384380163,
123.431379104992)) ;
#44068=CARTESIAN_POINT('Ctrl Pts',(-17.9020169238166,-14.6617493576534,
123.43628455332)) ;
#44069=CARTESIAN_POINT('Ctrl Pts',(-18.2253374188485,-14.8518012530216,
123.641768968564)) ;
#44070=CARTESIAN_POINT('Ctrl Pts',(-17.9293579840825,-14.6718121726588,
123.699271479237)) ;
#44071=CARTESIAN_POINT('Ctrl Pts',(-18.2826422959049,-14.8616974590703,
123.841793280128)) ;
#44072=CARTESIAN_POINT('Ctrl Pts',(-18.0009916819233,-14.6817083787074,
123.949301617982)) ;
#44073=CARTESIAN_POINT('Ctrl Pts',(-18.3736753162085,-14.8716382820956,
124.029885460281)) ;
#44074=CARTESIAN_POINT('Ctrl Pts',(-18.1147854788541,-14.6916492017327,
124.184415931245)) ;
#44075=CARTESIAN_POINT('Ctrl Pts',(-18.4967554476146,-14.8816428650742,
124.200469969171)) ;
#44076=CARTESIAN_POINT('Ctrl Pts',(-18.2686378473878,-14.7016537847114,
124.397645063482)) ;
#44077=CARTESIAN_POINT('Ctrl Pts',(-18.6479893488011,-14.891663759519,124.347127592409)) ;
#44078=CARTESIAN_POINT('Ctrl Pts',(-18.4576820792314,-14.7116746791561,
124.580965224182)) ;
#44079=CARTESIAN_POINT('Ctrl Pts',(-18.8200089658471,-14.9015556801084,
124.463997418573)) ;
#44080=CARTESIAN_POINT('Ctrl Pts',(-18.6727084410143,-14.7215665997455,
124.72705053099)) ;
#44081=CARTESIAN_POINT('Ctrl Pts',(-19.0115199934511,-14.9115491124538,
124.550366690489)) ;
#44082=CARTESIAN_POINT('Ctrl Pts',(-18.9120984381462,-14.7315600320909,
124.835009694246)) ;
#44083=CARTESIAN_POINT('Ctrl Pts',(-19.2141671143431,-14.9214947173536,
124.601860043974)) ;
#44084=CARTESIAN_POINT('Ctrl Pts',(-19.1654082297074,-14.7415056369908,
124.899373825222)) ;
#44085=CARTESIAN_POINT('Ctrl Pts',(-19.422692143887,-14.9314419908352,124.617812488144)) ;
#44086=CARTESIAN_POINT('Ctrl Pts',(-19.4260649276626,-14.7514529104723,
124.919311654018)) ;
#44087=CARTESIAN_POINT('Ctrl Pts',(-19.6328836255055,-14.9414899053115,
124.596874131456)) ;
#44088=CARTESIAN_POINT('Ctrl Pts',(-19.6888039980346,-14.7615008249487,
124.893135998467)) ;
#44089=CARTESIAN_POINT('Ctrl Pts',(-19.8322491561593,-14.9513375456589,
124.541062785767)) ;
#44090=CARTESIAN_POINT('Ctrl Pts',(-19.9380105597305,-14.771348465296,124.823369065413)) ;
#44091=CARTESIAN_POINT('Ctrl Pts',(-20.0213303949895,-14.9612992610355,
124.451042034006)) ;
#44092=CARTESIAN_POINT('Ctrl Pts',(-20.1743610165879,-14.7813101806726,
124.710840541122)) ;
#44093=CARTESIAN_POINT('Ctrl Pts',(-20.1929184638276,-14.9713278846083,
124.328511186806)) ;
#44094=CARTESIAN_POINT('Ctrl Pts',(-20.3888445239229,-14.7913388042454,
124.557674697892)) ;
#44095=CARTESIAN_POINT('Ctrl Pts',(-20.3389145430226,-14.9812382466747,
124.179885799862)) ;
#44096=CARTESIAN_POINT('Ctrl Pts',(-20.5713377846761,-14.8012491663118,
124.371890859621)) ;
#44097=CARTESIAN_POINT('Ctrl Pts',(-20.4576406506801,-14.9911729403271,
124.008044457199)) ;
#44098=CARTESIAN_POINT('Ctrl Pts',(-20.7197431781313,-14.8111838599642,
124.157087470465)) ;
#44099=CARTESIAN_POINT('Ctrl Pts',(-20.5454669216902,-15.001214783455,123.816080842499)) ;
#44100=CARTESIAN_POINT('Ctrl Pts',(-20.8295234845104,-14.8212257030921,
123.917131743842)) ;
#44101=CARTESIAN_POINT('Ctrl Pts',(-20.5979816592684,-15.0110992890254,
123.615000802519)) ;
#44102=CARTESIAN_POINT('Ctrl Pts',(-20.8951642259537,-14.8311102086625,
123.665780824477)) ;
#44103=CARTESIAN_POINT('Ctrl Pts',(-20.6152250273524,-15.0211013928106,
123.405463995573)) ;
#44104=CARTESIAN_POINT('Ctrl Pts',(-20.9167156314067,-14.8411123124477,
123.40385951735)) ;
#44105=CARTESIAN_POINT('Ctrl Pts',(-20.5961521969141,-15.0310197442256,
123.197788238171)) ;
#44106=CARTESIAN_POINT('Ctrl Pts',(-20.8928717590869,-14.8510306638627,
123.144264974598)) ;
#44107=CARTESIAN_POINT('Ctrl Pts',(-20.5405596861251,-15.0410674002465,
122.994035665252)) ;
#44108=CARTESIAN_POINT('Ctrl Pts',(-20.8233784416685,-14.8610783198836,
122.889574983756)) ;
#44109=CARTESIAN_POINT('Ctrl Pts',(-20.4521948522776,-15.0509385932747,
122.806217337189)) ;
#44110=CARTESIAN_POINT('Ctrl Pts',(-20.7129195792152,-14.8709495129118,
122.65480303298)) ;
#44111=CARTESIAN_POINT('Ctrl Pts',(-20.330284242075,-15.0610043064182,122.633308943981)) ;
#44112=CARTESIAN_POINT('Ctrl Pts',(-20.5605298604237,-14.8810152260553,
122.438669790613)) ;
#44113=CARTESIAN_POINT('Ctrl Pts',(-20.1834794070481,-15.0708567669908,
122.487109307967)) ;
#44114=CARTESIAN_POINT('Ctrl Pts',(-20.3770184511198,-14.890867686628,122.255919659017)) ;
#44115=CARTESIAN_POINT('Ctrl Pts',(-19.9518872310143,-15.0842852297134,
122.325790591143)) ;
#44116=CARTESIAN_POINT('Ctrl Pts',(-20.087542768723,-14.9042961493505,122.054287114174)) ;
#44117=CARTESIAN_POINT('Ctrl Pts',(-19.6903665057396,-15.0973661772305,
122.230682396376)) ;
#44118=CARTESIAN_POINT('Ctrl Pts',(-19.7606733441546,-14.9173770968676,
121.935403530529)) ;
#44119=CARTESIAN_POINT('Ctrl Pts',(-19.4082962992305,-15.110840675465,122.205756665579)) ;
#44120=CARTESIAN_POINT('Ctrl Pts',(-19.4080294143569,-14.9308515951022,
121.904239538084)) ;
#44121=CARTESIAN_POINT('Ctrl Pts',(-19.2023473006596,-15.1206727790745,
122.223870629062)) ;
#44122=CARTESIAN_POINT('Ctrl Pts',(-19.1506048230124,-14.9406836987116,
121.926886772641)) ;
#44123=CARTESIAN_POINT('Ctrl Pts',(-18.9998068488561,-15.1306386822012,
122.277363273524)) ;
#44124=CARTESIAN_POINT('Ctrl Pts',(-18.8974267387151,-14.9506496018383,
121.993755117999)) ;
#44125=CARTESIAN_POINT('Ctrl Pts',(-18.8085430621808,-15.1406660915114,
122.366073015869)) ;
#44126=CARTESIAN_POINT('Ctrl Pts',(-18.6583498545096,-14.9606770111485,
122.104643278367)) ;
#44127=CARTESIAN_POINT('Ctrl Pts',(-18.6376088448104,-15.150577122878,122.48516450023)) ;
#44128=CARTESIAN_POINT('Ctrl Pts',(-18.4446798401524,-14.9705880425151,
122.253516252991)) ;
#44129=CARTESIAN_POINT('Ctrl Pts',(-18.4395743724625,-15.163821430499,122.681015377369)) ;
#44130=CARTESIAN_POINT('Ctrl Pts',(-18.1971580268326,-14.9838323501362,
122.498300087744)) ;
#44131=CARTESIAN_POINT('Ctrl Pts',(-18.2607335132502,-15.1805219131702,
122.987645959784)) ;
#44132=CARTESIAN_POINT('Ctrl Pts',(-17.9735883960073,-15.0005328328073,
122.881645823256)) ;
#44133=CARTESIAN_POINT('Ctrl Pts',(-18.1977869763505,-15.197028742326,123.333061812602)) ;
#44134=CARTESIAN_POINT('Ctrl Pts',(-17.8949212635065,-15.0170396619631,
123.313331293313)) ;
#44135=CARTESIAN_POINT('Ctrl Pts',(-18.2199642495241,-15.2103393705636,
123.611928517238)) ;
#44136=CARTESIAN_POINT('Ctrl Pts',(-17.9226408363166,-15.0303502902007,
123.661981974254)) ;
#44137=CARTESIAN_POINT('Ctrl Pts',(-18.2726848636332,-15.2203319341037,
123.815325721179)) ;
#44138=CARTESIAN_POINT('Ctrl Pts',(-17.9885443792014,-15.0403428537408,
123.916213406476)) ;
#44139=CARTESIAN_POINT('Ctrl Pts',(-18.3604503080189,-15.2303620171052,
124.007021668416)) ;
#44140=CARTESIAN_POINT('Ctrl Pts',(-18.0982567045418,-15.0503729367423,
124.155839488556)) ;
#44141=CARTESIAN_POINT('Ctrl Pts',(-18.5172815670806,-15.243535621103,124.235376320227)) ;
#44142=CARTESIAN_POINT('Ctrl Pts',(-18.294281628791,-15.0635465407401,124.441261777876)) ;
#44143=CARTESIAN_POINT('Ctrl Pts',(-18.785763220475,-15.2601733263344,124.465502936072)) ;
#44144=CARTESIAN_POINT('Ctrl Pts',(-18.6299004804778,-15.0801842459715,
124.72893753815)) ;
#44145=CARTESIAN_POINT('Ctrl Pts',(-19.1813810887829,-15.2800550889018,
124.614910728195)) ;
#44146=CARTESIAN_POINT('Ctrl Pts',(-19.1244402677115,-15.1000660085389,
124.915683237853)) ;
#44147=CARTESIAN_POINT('Ctrl Pts',(-19.536304822624,-15.2967514411183,124.619219755491)) ;
#44148=CARTESIAN_POINT('Ctrl Pts',(-19.5680268436857,-15.1167623607554,
124.921075710828)) ;
#44149=CARTESIAN_POINT('Ctrl Pts',(-19.8044165799873,-15.3099084689074,
124.551173766666)) ;
#44150=CARTESIAN_POINT('Ctrl Pts',(-19.9032277012158,-15.1299193885445,
124.836006276955)) ;
#44151=CARTESIAN_POINT('Ctrl Pts',(-20.0610790101127,-15.3232858235509,
124.436222758126)) ;
#44152=CARTESIAN_POINT('Ctrl Pts',(-20.2240299227746,-15.1432967431881,
124.692326184051)) ;
#44153=CARTESIAN_POINT('Ctrl Pts',(-20.3337494420324,-15.3398166578097,
124.214377221525)) ;
#44154=CARTESIAN_POINT('Ctrl Pts',(-20.5648835408221,-15.1598275774469,
124.415004995461)) ;
#44155=CARTESIAN_POINT('Ctrl Pts',(-20.552438862062,-15.3597813475528,123.850580679781)) ;
#44156=CARTESIAN_POINT('Ctrl Pts',(-20.8382356610329,-15.17979226719,123.960261264776)) ;
#44157=CARTESIAN_POINT('Ctrl Pts',(-20.6332747084739,-15.3796978409765,
123.434880640488)) ;
#44158=CARTESIAN_POINT('Ctrl Pts',(-20.9392779039823,-15.1997087606136,
123.440635012867)) ;
#44159=CARTESIAN_POINT('Ctrl Pts',(-20.5683199143235,-15.399587560326,123.016946237213)) ;
#44160=CARTESIAN_POINT('Ctrl Pts',(-20.8580805309166,-15.2195984799632,
122.918218801443)) ;
#44161=CARTESIAN_POINT('Ctrl Pts',(-20.3631949850862,-15.4195942899739,
122.644342249502)) ;
#44162=CARTESIAN_POINT('Ctrl Pts',(-20.6016712396196,-15.239605209611,122.45246543698)) ;
#44163=CARTESIAN_POINT('Ctrl Pts',(-20.0460283351885,-15.4394323436208,
122.366126910109)) ;
#44164=CARTESIAN_POINT('Ctrl Pts',(-20.2052118909962,-15.2594432632579,
122.104699832134)) ;
#44165=CARTESIAN_POINT('Ctrl Pts',(-19.6501954328286,-15.4594256818344,
122.211302972032)) ;
#44166=CARTESIAN_POINT('Ctrl Pts',(-19.7104197648505,-15.2794366014715,
121.911172706133)) ;
#44167=CARTESIAN_POINT('Ctrl Pts',(-19.22747548443,-15.479308481241,122.20116645109)) ;
#44168=CARTESIAN_POINT('Ctrl Pts',(-19.1820210308814,-15.2993194008781,
121.898505004141)) ;
#44169=CARTESIAN_POINT('Ctrl Pts',(-18.8264426794319,-15.4992006621597,
122.335208188009)) ;
#44170=CARTESIAN_POINT('Ctrl Pts',(-18.6807320925926,-15.3192115817968,
122.06605896947)) ;
#44171=CARTESIAN_POINT('Ctrl Pts',(-18.4944215574731,-15.5191028406548,
122.597782843408)) ;
#44172=CARTESIAN_POINT('Ctrl Pts',(-18.2657076846686,-15.3391137602919,
122.394277865644)) ;
#44173=CARTESIAN_POINT('Ctrl Pts',(-18.2711780684696,-15.5391401518585,
122.960525542868)) ;
#44174=CARTESIAN_POINT('Ctrl Pts',(-17.9866547281374,-15.3591510714956,
122.847707709371)) ;
#44175=CARTESIAN_POINT('Ctrl Pts',(-18.1854465994955,-15.5589525933994,
123.373166514348)) ;
#44176=CARTESIAN_POINT('Ctrl Pts',(-17.8794922157529,-15.3789635130365,
123.363506708324)) ;
#44177=CARTESIAN_POINT('Ctrl Pts',(-18.2465194115136,-15.5790178341343,
123.795207249882)) ;
#44178=CARTESIAN_POINT('Ctrl Pts',(-17.955834597053,-15.3990287537714,123.891058298143)) ;
#44179=CARTESIAN_POINT('Ctrl Pts',(-18.4447532133238,-15.5987750389901,
124.16581727744)) ;
#44180=CARTESIAN_POINT('Ctrl Pts',(-18.2036257717715,-15.4187859586272,
124.35431729337)) ;
#44181=CARTESIAN_POINT('Ctrl Pts',(-18.7611937431446,-15.6188083116358,
124.450642539288)) ;
#44182=CARTESIAN_POINT('Ctrl Pts',(-18.5991767273495,-15.4388192312729,
124.710349085039)) ;
#44183=CARTESIAN_POINT('Ctrl Pts',(-19.1518899017671,-15.6386212200896,
124.608729629548)) ;
#44184=CARTESIAN_POINT('Ctrl Pts',(-19.0875441524019,-15.4586321397268,
124.907957059452)) ;
#44185=CARTESIAN_POINT('Ctrl Pts',(-19.5765723952849,-15.6586173662171,
124.624694592537)) ;
#44186=CARTESIAN_POINT('Ctrl Pts',(-19.6183970906308,-15.4786282858542,
124.927914166445)) ;
#44187=CARTESIAN_POINT('Ctrl Pts',(-19.9789149548444,-15.6784791194396,
124.495740343834)) ;
#44188=CARTESIAN_POINT('Ctrl Pts',(-20.1213238855666,-15.4984900390767,
124.766723103207)) ;
#44189=CARTESIAN_POINT('Ctrl Pts',(-20.3161903072829,-15.6985476365677,
124.234500907358)) ;
#44190=CARTESIAN_POINT('Ctrl Pts',(-20.5429196526182,-15.5185585562048,
124.440174246411)) ;
#44191=CARTESIAN_POINT('Ctrl Pts',(-20.5412403283249,-15.7183785095645,
123.877812094549)) ;
#44192=CARTESIAN_POINT('Ctrl Pts',(-20.8242320696034,-15.5383894292016,
123.994315885912)) ;
#44193=CARTESIAN_POINT('Ctrl Pts',(-20.6325525181329,-15.7383004203812,
123.464277815718)) ;
#44194=CARTESIAN_POINT('Ctrl Pts',(-20.9383743235662,-15.5583113400183,
123.477399544044)) ;
#44195=CARTESIAN_POINT('Ctrl Pts',(-20.5770999387733,-15.7582298638165,
123.044097906908)) ;
#44196=CARTESIAN_POINT('Ctrl Pts',(-20.8690610707405,-15.5782407834536,
122.952175132017)) ;
#44197=CARTESIAN_POINT('Ctrl Pts',(-20.3819841700265,-15.7781395339329,
122.668482285981)) ;
#44198=CARTESIAN_POINT('Ctrl Pts',(-20.6251692263084,-15.59815045357,122.482655310939)) ;
#44199=CARTESIAN_POINT('Ctrl Pts',(-20.071398669403,-15.7980128911957,122.381885903197)) ;
#44200=CARTESIAN_POINT('Ctrl Pts',(-20.2369405024036,-15.6180238108329,
122.124408327086)) ;
#44201=CARTESIAN_POINT('Ctrl Pts',(-19.6794075493568,-15.8180044258137,
122.217622884656)) ;
#44202=CARTESIAN_POINT('Ctrl Pts',(-19.7469529682357,-15.6380153454508,
121.919076471871)) ;
#44203=CARTESIAN_POINT('Ctrl Pts',(-19.2574526738448,-15.8378700432244,
122.196935178988)) ;
#44204=CARTESIAN_POINT('Ctrl Pts',(-19.2195107524883,-15.6578809628615,
121.893213319316)) ;
#44205=CARTESIAN_POINT('Ctrl Pts',(-18.8513755370978,-15.8578509730526,
122.321775663419)) ;
#44206=CARTESIAN_POINT('Ctrl Pts',(-18.7119132760314,-15.6778618926898,
122.049260143643)) ;
#44207=CARTESIAN_POINT('Ctrl Pts',(-18.5132612033128,-15.8777894351358,
122.577542069427)) ;
#44208=CARTESIAN_POINT('Ctrl Pts',(-18.2892684219833,-15.6978003547729,
122.368964780256)) ;
#44209=CARTESIAN_POINT('Ctrl Pts',(-18.2826819587382,-15.8976816283575,
122.932185153396)) ;
#44210=CARTESIAN_POINT('Ctrl Pts',(-18.0010412603232,-15.7176925479946,
122.812265657401)) ;
#44211=CARTESIAN_POINT('Ctrl Pts',(-18.1868169762122,-15.9176523433929,
123.34575803658)) ;
#44212=CARTESIAN_POINT('Ctrl Pts',(-17.8812058283193,-15.73766326303,123.329230583634)) ;
#44213=CARTESIAN_POINT('Ctrl Pts',(-18.2367313458389,-15.937462015059,123.764098817235)) ;
#44214=CARTESIAN_POINT('Ctrl Pts',(-17.9435942352086,-15.7574729346961,
123.852155946774)) ;
#44215=CARTESIAN_POINT('Ctrl Pts',(-18.4277666040295,-15.9574552317502,
124.143691492752)) ;
#44216=CARTESIAN_POINT('Ctrl Pts',(-18.1823832687672,-15.7774661513873,
124.326648974509)) ;
#44217=CARTESIAN_POINT('Ctrl Pts',(-18.7346680099378,-15.9773061439465,
124.433713845188)) ;
#44218=CARTESIAN_POINT('Ctrl Pts',(-18.5660086878683,-15.7973170635836,
124.689180060652)) ;
#44219=CARTESIAN_POINT('Ctrl Pts',(-19.1263185071962,-15.9973807502655,
124.603150136167)) ;
#44220=CARTESIAN_POINT('Ctrl Pts',(-19.0555605460036,-15.8173916699027,
124.900980308244)) ;
#44221=CARTESIAN_POINT('Ctrl Pts',(-19.4769940370043,-16.0138973821489,
124.624006616587)) ;
#44222=CARTESIAN_POINT('Ctrl Pts',(-19.493934124633,-15.833908301786,124.927054796924)) ;
#44223=CARTESIAN_POINT('Ctrl Pts',(-19.7517414985942,-16.027236089843,124.568093364996)) ;
#44224=CARTESIAN_POINT('Ctrl Pts',(-19.837342147255,-15.8472470094801,124.8571673599)) ;
#44225=CARTESIAN_POINT('Ctrl Pts',(-19.9444057679308,-16.0370784641513,
124.492551498524)) ;
#44226=CARTESIAN_POINT('Ctrl Pts',(-20.0781804979122,-15.8570893837884,
124.762739875852)) ;
#44227=CARTESIAN_POINT('Ctrl Pts',(-20.1249049321985,-16.047133484134,124.382567620846)) ;
#44228=CARTESIAN_POINT('Ctrl Pts',(-20.303796053823,-15.8671444037711,124.625272793233)) ;
#44229=CARTESIAN_POINT('Ctrl Pts',(-20.3337092884455,-16.0603656407916,
124.198785774196)) ;
#44230=CARTESIAN_POINT('Ctrl Pts',(-20.5648469001253,-15.8803765604287,
124.395495442102)) ;
#44231=CARTESIAN_POINT('Ctrl Pts',(-20.5299755382867,-16.0769806081367,
123.904990129354)) ;
#44232=CARTESIAN_POINT('Ctrl Pts',(-20.8101326079248,-15.8969915277738,
124.02832371329)) ;
#44233=CARTESIAN_POINT('Ctrl Pts',(-20.6139164154991,-16.0935751951479,
123.562338411869)) ;
#44234=CARTESIAN_POINT('Ctrl Pts',(-20.9150857051299,-15.913586114785,123.599951810518)) ;
#44235=CARTESIAN_POINT('Ctrl Pts',(-20.6085033819079,-16.1068087635033,
123.284128846805)) ;
#44236=CARTESIAN_POINT('Ctrl Pts',(-20.9083137993507,-15.9268196831404,
123.252228775196)) ;
#44237=CARTESIAN_POINT('Ctrl Pts',(-20.5678420997152,-16.1168523813119,
123.076956614971)) ;
#44238=CARTESIAN_POINT('Ctrl Pts',(-20.8574915953394,-15.9368633009491,
122.993254896173)) ;
#44239=CARTESIAN_POINT('Ctrl Pts',(-20.4930658285917,-16.1267393055468,
122.882997750619)) ;
#44240=CARTESIAN_POINT('Ctrl Pts',(-20.7640240610611,-15.9467502251839,
122.750807958911)) ;
#44241=CARTESIAN_POINT('Ctrl Pts',(-20.3849611897659,-16.1367299599936,
122.702938885806)) ;
#44242=CARTESIAN_POINT('Ctrl Pts',(-20.6288932481491,-15.9567408796307,
122.525730668388)) ;
#44243=CARTESIAN_POINT('Ctrl Pts',(-20.2475814117215,-16.1466917184475,
122.544854107054)) ;
#44244=CARTESIAN_POINT('Ctrl Pts',(-20.4571800169588,-15.9667026380847,
122.328129169805)) ;
#44245=CARTESIAN_POINT('Ctrl Pts',(-20.0298504240982,-16.1600315835148,
122.368082548189)) ;
#44246=CARTESIAN_POINT('Ctrl Pts',(-20.1849716448928,-15.9800425031519,
122.107130949398)) ;
#44247=CARTESIAN_POINT('Ctrl Pts',(-19.7713257253914,-16.1733403664281,
122.253045017901)) ;
#44248=CARTESIAN_POINT('Ctrl Pts',(-19.8618390549407,-15.9933512860652,
121.963354376013)) ;
#44249=CARTESIAN_POINT('Ctrl Pts',(-19.4973854044494,-16.1865361238721,
122.209149372698)) ;
#44250=CARTESIAN_POINT('Ctrl Pts',(-19.5194352459976,-16.0065470435093,
121.908483591951)) ;
#44251=CARTESIAN_POINT('Ctrl Pts',(-19.2879723974171,-16.1964980075486,
122.211840246962)) ;
#44252=CARTESIAN_POINT('Ctrl Pts',(-19.2576646411518,-16.0165089271858,
121.911843868139)) ;
#44253=CARTESIAN_POINT('Ctrl Pts',(-19.0805966754575,-16.2065411170633,
122.251508529244)) ;
#44254=CARTESIAN_POINT('Ctrl Pts',(-18.9984455353945,-16.0265520367004,
121.961426597411)) ;
#44255=CARTESIAN_POINT('Ctrl Pts',(-18.8869132560321,-16.2163933670625,
122.324927691343)) ;
#44256=CARTESIAN_POINT('Ctrl Pts',(-18.7563398527303,-16.0364042866996,
122.053197919852)) ;
#44257=CARTESIAN_POINT('Ctrl Pts',(-18.7065271330224,-16.226364904013,122.431685493257)) ;
#44258=CARTESIAN_POINT('Ctrl Pts',(-18.5308557513542,-16.0463758236501,
122.186642824529)) ;
#44259=CARTESIAN_POINT('Ctrl Pts',(-18.5470082080786,-16.2363601694905,
122.56851706965)) ;
#44260=CARTESIAN_POINT('Ctrl Pts',(-18.331455189681,-16.0563710891276,122.357680218404)) ;
#44261=CARTESIAN_POINT('Ctrl Pts',(-18.413387011108,-16.2463941423641,122.731722217809)) ;
#44262=CARTESIAN_POINT('Ctrl Pts',(-18.164426495201,-16.0664050620013,122.561684900348)) ;
#44263=CARTESIAN_POINT('Ctrl Pts',(-18.3116651483155,-16.2562495571265,
122.91224766768)) ;
#44264=CARTESIAN_POINT('Ctrl Pts',(-18.037271614364,-16.0762604767636,122.787340539645)) ;
#44265=CARTESIAN_POINT('Ctrl Pts',(-18.2415770596379,-16.2662488346353,
123.110397616458)) ;
#44266=CARTESIAN_POINT('Ctrl Pts',(-17.9496588451974,-16.0862597542724,
123.035027131255)) ;
#44267=CARTESIAN_POINT('Ctrl Pts',(-18.2070866766184,-16.2761440187983,
123.315582482187)) ;
#44268=CARTESIAN_POINT('Ctrl Pts',(-17.9065430994945,-16.0961549384354,
123.291508010341)) ;
#44269=CARTESIAN_POINT('Ctrl Pts',(-18.2087980539472,-16.2862043984391,
123.527047846686)) ;
#44270=CARTESIAN_POINT('Ctrl Pts',(-17.908679550301,-16.1062153180762,123.555839709386)) ;
#44271=CARTESIAN_POINT('Ctrl Pts',(-18.2462808343881,-16.2960542674472,
123.730723195858)) ;
#44272=CARTESIAN_POINT('Ctrl Pts',(-17.9555303866204,-16.1160651870843,
123.810434776852)) ;
#44273=CARTESIAN_POINT('Ctrl Pts',(-18.3194286022039,-16.3060858286551,
123.928512270352)) ;
#44274=CARTESIAN_POINT('Ctrl Pts',(-18.0469625663343,-16.1260967482922,
124.057672087697)) ;
#44275=CARTESIAN_POINT('Ctrl Pts',(-18.425966779491,-16.3160962775374,124.110026603965)) ;
#44276=CARTESIAN_POINT('Ctrl Pts',(-18.1801329408613,-16.1361071971745,
124.284566442434)) ;
#44277=CARTESIAN_POINT('Ctrl Pts',(-18.560797825782,-16.3260030169544,124.268754201217)) ;
#44278=CARTESIAN_POINT('Ctrl Pts',(-18.3486698658472,-16.1460139365915,
124.482977937529)) ;
#44279=CARTESIAN_POINT('Ctrl Pts',(-18.7213836715412,-16.3359410330228,
124.402388892912)) ;
#44280=CARTESIAN_POINT('Ctrl Pts',(-18.5494006644894,-16.1559519526599,
124.65002353466)) ;
#44281=CARTESIAN_POINT('Ctrl Pts',(-18.9039216281586,-16.3459462794739,
124.506949932254)) ;
#44282=CARTESIAN_POINT('Ctrl Pts',(-18.7775718601343,-16.1659571991111,
124.780727182674)) ;
#44283=CARTESIAN_POINT('Ctrl Pts',(-19.1025026858816,-16.3559803405302,
124.578083634945)) ;
#44284=CARTESIAN_POINT('Ctrl Pts',(-19.0257972538791,-16.1759912601674,
124.869646856981)) ;
#44285=CARTESIAN_POINT('Ctrl Pts',(-19.3064644872942,-16.3658254215884,
124.613343041828)) ;
#44286=CARTESIAN_POINT('Ctrl Pts',(-19.2807496064641,-16.1858363412255,
124.913723831211)) ;
#44287=CARTESIAN_POINT('Ctrl Pts',(-19.5163642119704,-16.3758112275419,
124.61303502221)) ;
#44288=CARTESIAN_POINT('Ctrl Pts',(-19.5431244270057,-16.195822147179,124.913341409534)) ;
#44289=CARTESIAN_POINT('Ctrl Pts',(-19.7220636700193,-16.3857460480961,
124.576608850265)) ;
#44290=CARTESIAN_POINT('Ctrl Pts',(-19.8002495182117,-16.2057569677332,
124.86781116894)) ;
#44291=CARTESIAN_POINT('Ctrl Pts',(-19.9206078791978,-16.3958035732283,
124.503981755754)) ;
#44292=CARTESIAN_POINT('Ctrl Pts',(-20.0484305675557,-16.2158144928654,
124.777029790826)) ;
#44293=CARTESIAN_POINT('Ctrl Pts',(-20.0994392626122,-16.4056252238796,
124.400718208666)) ;
#44294=CARTESIAN_POINT('Ctrl Pts',(-20.2719717473046,-16.2256361435168,
124.647952173762)) ;
#44295=CARTESIAN_POINT('Ctrl Pts',(-20.2616227730663,-16.4156812873844,
124.265132165577)) ;
#44296=CARTESIAN_POINT('Ctrl Pts',(-20.4747026404309,-16.2356922070215,
124.478471590715)) ;
#44297=CARTESIAN_POINT('Ctrl Pts',(-20.3959657201901,-16.4256219544483,
124.105038813883)) ;
#44298=CARTESIAN_POINT('Ctrl Pts',(-20.6426334922787,-16.2456328740854,
124.278356285801)) ;
#44299=CARTESIAN_POINT('Ctrl Pts',(-20.5006527032414,-16.4355263481143,
123.925043149726)) ;
#44300=CARTESIAN_POINT('Ctrl Pts',(-20.7734945781979,-16.2555372677514,
124.053362462488)) ;
#44301=CARTESIAN_POINT('Ctrl Pts',(-20.5733913233739,-16.4455728718773,
123.726774248668)) ;
#44302=CARTESIAN_POINT('Ctrl Pts',(-20.8644201156856,-16.2655837915144,
123.805527276489)) ;
#44303=CARTESIAN_POINT('Ctrl Pts',(-20.6102491313444,-16.4554689548937,
123.521980484657)) ;
#44304=CARTESIAN_POINT('Ctrl Pts',(-20.9104948421842,-16.2754798745308,
123.549534920301)) ;
#44305=CARTESIAN_POINT('Ctrl Pts',(-20.6109490500216,-16.4655356541237,
123.310385747446)) ;
#44306=CARTESIAN_POINT('Ctrl Pts',(-20.9113721563004,-16.2855465737608,
123.285041710437)) ;
#44307=CARTESIAN_POINT('Ctrl Pts',(-20.5759933517223,-16.4753592645248,
123.106810422099)) ;
#44308=CARTESIAN_POINT('Ctrl Pts',(-20.8676796982969,-16.2953701841619,
123.030571216678)) ;
#44309=CARTESIAN_POINT('Ctrl Pts',(-20.504941661928,-16.4854151247023,122.907730675288)) ;
#44310=CARTESIAN_POINT('Ctrl Pts',(-20.7788672822299,-16.3054260443394,
122.78172092023)) ;
#44311=CARTESIAN_POINT('Ctrl Pts',(-20.4014184334642,-16.4953482710072,
122.726342025547)) ;
#44312=CARTESIAN_POINT('Ctrl Pts',(-20.6494650621371,-16.3153591906443,
122.554983567681)) ;
#44313=CARTESIAN_POINT('Ctrl Pts',(-20.2681709832991,-16.5052935267778,
122.565253208005)) ;
#44314=CARTESIAN_POINT('Ctrl Pts',(-20.482907205734,-16.3253044464149,122.353620794924)) ;
#44315=CARTESIAN_POINT('Ctrl Pts',(-20.1084390136851,-16.5152768252163,
122.429067661281)) ;
#44316=CARTESIAN_POINT('Ctrl Pts',(-20.2832435137654,-16.3352877448534,
122.183387066587)) ;
#44317=CARTESIAN_POINT('Ctrl Pts',(-19.9264011878482,-16.5253140053629,
122.322380814143)) ;
#44318=CARTESIAN_POINT('Ctrl Pts',(-20.0556974557247,-16.345324925,122.050026596419)) ;
#44319=CARTESIAN_POINT('Ctrl Pts',(-19.7322826676452,-16.5351685580724,
122.24994521566)) ;
#44320=CARTESIAN_POINT('Ctrl Pts',(-19.8130492090875,-16.3551794777095,
121.959479734219)) ;
#44321=CARTESIAN_POINT('Ctrl Pts',(-19.5256465946988,-16.5451680765197,
122.211483731313)) ;
#44322=CARTESIAN_POINT('Ctrl Pts',(-19.5547543717417,-16.3651789961568,
121.911400782604)) ;
#44323=CARTESIAN_POINT('Ctrl Pts',(-19.3175976842918,-16.5550631589818,
122.209284349518)) ;
#44324=CARTESIAN_POINT('Ctrl Pts',(-19.2946925229401,-16.3750740786189,
121.908649507765)) ;
#44325=CARTESIAN_POINT('Ctrl Pts',(-19.1089595995031,-16.5651237044879,
122.243820775951)) ;
#44326=CARTESIAN_POINT('Ctrl Pts',(-19.0338948184868,-16.385134624125,121.951817978904)) ;
#44327=CARTESIAN_POINT('Ctrl Pts',(-18.9135973762475,-16.5749730117359,
122.312488918254)) ;
#44328=CARTESIAN_POINT('Ctrl Pts',(-18.7896903909749,-16.394983931373,122.037651600435)) ;
#44329=CARTESIAN_POINT('Ctrl Pts',(-18.7296234980827,-16.5850001018232,
122.415390660692)) ;
#44330=CARTESIAN_POINT('Ctrl Pts',(-18.5597221685601,-16.4050110214604,
122.166277137884)) ;
#44331=CARTESIAN_POINT('Ctrl Pts',(-18.5666258182799,-16.5950290059602,
122.549139612565)) ;
#44332=CARTESIAN_POINT('Ctrl Pts',(-18.3559738383633,-16.4150399255973,
122.333461717457)) ;
#44333=CARTESIAN_POINT('Ctrl Pts',(-18.4315607292266,-16.6048728710595,
122.705925530433)) ;
#44334=CARTESIAN_POINT('Ctrl Pts',(-18.1871403035161,-16.4248837906966,
122.529443722511)) ;
#44335=CARTESIAN_POINT('Ctrl Pts',(-18.3236876247588,-16.6148686977679,
122.886268946656)) ;
#44336=CARTESIAN_POINT('Ctrl Pts',(-18.0522973396058,-16.434879617405,122.754872248908)) ;
#44337=CARTESIAN_POINT('Ctrl Pts',(-18.2489074259559,-16.6248939144169,
123.083322704059)) ;
#44338=CARTESIAN_POINT('Ctrl Pts',(-17.9588203685943,-16.444904834054,123.001188739217)) ;
#44339=CARTESIAN_POINT('Ctrl Pts',(-18.2097358480084,-16.6347837465745,
123.287518104386)) ;
#44340=CARTESIAN_POINT('Ctrl Pts',(-17.909853990901,-16.4547946662116,123.256433493462)) ;
#44341=CARTESIAN_POINT('Ctrl Pts',(-18.2062951743029,-16.6447746026592,
123.497522176624)) ;
#44342=CARTESIAN_POINT('Ctrl Pts',(-17.9055514641145,-16.4647855222963,
123.518938743175)) ;
#44343=CARTESIAN_POINT('Ctrl Pts',(-18.2392588330395,-16.6547196972521,
123.70398395006)) ;
#44344=CARTESIAN_POINT('Ctrl Pts',(-17.9467544397181,-16.4747306168892,
123.777016725455)) ;
#44345=CARTESIAN_POINT('Ctrl Pts',(-18.3072491133093,-16.6646716010202,
123.901857207325)) ;
#44346=CARTESIAN_POINT('Ctrl Pts',(-18.0317409622789,-16.4846825206573,
124.02435926062)) ;
#44347=CARTESIAN_POINT('Ctrl Pts',(-18.4095792800101,-16.6747080004896,
124.086372613872)) ;
#44348=CARTESIAN_POINT('Ctrl Pts',(-18.1596521832206,-16.4947189201267,
124.255004193986)) ;
#44349=CARTESIAN_POINT('Ctrl Pts',(-18.5403323023959,-16.6845970705783,
124.24801603038)) ;
#44350=CARTESIAN_POINT('Ctrl Pts',(-18.3230928107259,-16.5046079902154,
124.45706017088)) ;
#44351=CARTESIAN_POINT('Ctrl Pts',(-18.6984981846878,-16.6945863599492,
124.386161267394)) ;
#44352=CARTESIAN_POINT('Ctrl Pts',(-18.5207993714946,-16.5145972795863,
124.62974295052)) ;
#44353=CARTESIAN_POINT('Ctrl Pts',(-18.8777747357484,-16.7045449261589,
124.494277089496)) ;
#44354=CARTESIAN_POINT('Ctrl Pts',(-18.7448946531672,-16.524555845796,124.764889240736)) ;
#44355=CARTESIAN_POINT('Ctrl Pts',(-19.071775886629,-16.7144444973757,124.569661405429)) ;
#44356=CARTESIAN_POINT('Ctrl Pts',(-18.9873964306672,-16.5344554170128,
124.859121187844)) ;
#44357=CARTESIAN_POINT('Ctrl Pts',(-19.2789592287976,-16.7244924117899,
124.6107434715)) ;
#44358=CARTESIAN_POINT('Ctrl Pts',(-19.2463751321028,-16.5445033314271,
124.910475054052)) ;
#44359=CARTESIAN_POINT('Ctrl Pts',(-19.4869725711741,-16.7343877546505,
124.615324364318)) ;
#44360=CARTESIAN_POINT('Ctrl Pts',(-19.5063926931676,-16.5543986742876,
124.916202482167)) ;
#44361=CARTESIAN_POINT('Ctrl Pts',(-19.6960268210127,-16.7444494485979,
124.583223874358)) ;
#44362=CARTESIAN_POINT('Ctrl Pts',(-19.7677103786567,-16.5644603682351,
124.876078188685)) ;
#44363=CARTESIAN_POINT('Ctrl Pts',(-19.8920494172545,-16.7542939016821,
124.51680250823)) ;
#44364=CARTESIAN_POINT('Ctrl Pts',(-20.0127402827111,-16.5743048213192,
124.793052261125)) ;
#44365=CARTESIAN_POINT('Ctrl Pts',(-20.0760402865908,-16.7642545866405,
124.416833948505)) ;
#44366=CARTESIAN_POINT('Ctrl Pts',(-20.2427297441495,-16.5842655062777,
124.668092227822)) ;
#44367=CARTESIAN_POINT('Ctrl Pts',(-20.2409080973794,-16.7742905191491,
124.285163854322)) ;
#44368=CARTESIAN_POINT('Ctrl Pts',(-20.4488151079738,-16.5943014387862,
124.503505578167)) ;
#44369=CARTESIAN_POINT('Ctrl Pts',(-20.3785099430271,-16.7841791348371,
124.129336922064)) ;
#44370=CARTESIAN_POINT('Ctrl Pts',(-20.6208188759846,-16.6041900544743,
124.308721850935)) ;
#44371=CARTESIAN_POINT('Ctrl Pts',(-20.4887120097041,-16.7941935439796,
123.949931511366)) ;
#44372=CARTESIAN_POINT('Ctrl Pts',(-20.7585722335098,-16.6142044636167,
124.084465548632)) ;
#44373=CARTESIAN_POINT('Ctrl Pts',(-20.5657191627696,-16.8042273529374,
123.753561423584)) ;
#44374=CARTESIAN_POINT('Ctrl Pts',(-20.8548321532337,-16.6242382725745,
123.839003471637)) ;
#44375=CARTESIAN_POINT('Ctrl Pts',(-20.6071867597122,-16.8140578071936,
123.551072730248)) ;
#44376=CARTESIAN_POINT('Ctrl Pts',(-20.9066678159083,-16.6340687268307,
123.585891332046)) ;
#44377=CARTESIAN_POINT('Ctrl Pts',(-20.6130753200358,-16.8241354747718,
123.339330931498)) ;
#44378=CARTESIAN_POINT('Ctrl Pts',(-20.9140293672991,-16.6441463944089,
123.321214560583)) ;
#44379=CARTESIAN_POINT('Ctrl Pts',(-20.582897122482,-16.833987342894,123.134379068764)) ;
#44380=CARTESIAN_POINT('Ctrl Pts',(-20.8763072380744,-16.6539982625311,
123.065023312876)) ;
#44381=CARTESIAN_POINT('Ctrl Pts',(-20.5163171737132,-16.8440603804594,
122.933388787276)) ;
#44382=CARTESIAN_POINT('Ctrl Pts',(-20.7930831562176,-16.6640713000965,
122.81378563807)) ;
#44383=CARTESIAN_POINT('Ctrl Pts',(-20.4180968317784,-16.8539029338102,
122.751244860052)) ;
#44384=CARTESIAN_POINT('Ctrl Pts',(-20.6703077317123,-16.6739138534474,
122.586104119148)) ;
#44385=CARTESIAN_POINT('Ctrl Pts',(-20.2885154375274,-16.8638833293037,
122.586232749684)) ;
#44386=CARTESIAN_POINT('Ctrl Pts',(-20.5083311850613,-16.6838942489408,
122.3798384328)) ;
#44387=CARTESIAN_POINT('Ctrl Pts',(-20.1313776052616,-16.8739018072815,
122.445995465439)) ;
#44388=CARTESIAN_POINT('Ctrl Pts',(-20.3119093379596,-16.6939127269186,
122.204541346776)) ;
#44389=CARTESIAN_POINT('Ctrl Pts',(-19.9549021525347,-16.8837851215876,
122.336275047287)) ;
#44390=CARTESIAN_POINT('Ctrl Pts',(-20.0913143430655,-16.7037960412247,
122.067389838621)) ;
#44391=CARTESIAN_POINT('Ctrl Pts',(-19.7584673745493,-16.8938534241263,
122.257523549518)) ;
#44392=CARTESIAN_POINT('Ctrl Pts',(-19.8457714437164,-16.7138643437634,
121.968950139572)) ;
#44393=CARTESIAN_POINT('Ctrl Pts',(-19.5562266361521,-16.9036834713997,
122.214849851963)) ;
#44394=CARTESIAN_POINT('Ctrl Pts',(-19.5929691002655,-16.7236943910368,
121.915607289983)) ;
#44395=CARTESIAN_POINT('Ctrl Pts',(-19.3447520721929,-16.9137503428152,
122.207507802747)) ;
#44396=CARTESIAN_POINT('Ctrl Pts',(-19.3286263043383,-16.7337612624523,
121.906429428325)) ;
#44397=CARTESIAN_POINT('Ctrl Pts',(-19.1388680110044,-16.9236393816143,
122.236594479174)) ;
#44398=CARTESIAN_POINT('Ctrl Pts',(-19.0712701351498,-16.7436503012514,
121.942787563624)) ;
#44399=CARTESIAN_POINT('Ctrl Pts',(-18.9389316545158,-16.9336360797484,
122.301281101622)) ;
#44400=CARTESIAN_POINT('Ctrl Pts',(-18.8213494437771,-16.7536469993855,
122.023645715726)) ;
#44401=CARTESIAN_POINT('Ctrl Pts',(-18.7540959744669,-16.9435885054603,
122.39935968639)) ;
#44402=CARTESIAN_POINT('Ctrl Pts',(-18.5903042632975,-16.7635994250975,
122.146243992672)) ;
#44403=CARTESIAN_POINT('Ctrl Pts',(-18.5891273339633,-16.9535298076933,
122.527650967993)) ;
#44404=CARTESIAN_POINT('Ctrl Pts',(-18.3840928904313,-16.7735407273304,
122.306608387421)) ;
#44405=CARTESIAN_POINT('Ctrl Pts',(-18.4481547796409,-16.9635130467772,
122.683169969797)) ;
#44406=CARTESIAN_POINT('Ctrl Pts',(-18.2078769998902,-16.7835239664143,
122.501007316772)) ;
#44407=CARTESIAN_POINT('Ctrl Pts',(-18.3360050079193,-16.9735518483458,
122.861931794176)) ;
#44408=CARTESIAN_POINT('Ctrl Pts',(-18.0676897405683,-16.7935627679829,
122.724459360897)) ;
#44409=CARTESIAN_POINT('Ctrl Pts',(-18.2577181334253,-16.9833999544674,
123.053617948428)) ;
#44410=CARTESIAN_POINT('Ctrl Pts',(-17.9698306083083,-16.8034108741046,
122.964068373402)) ;
#44411=CARTESIAN_POINT('Ctrl Pts',(-18.2127741605597,-16.9934601500428,
123.260266613058)) ;
#44412=CARTESIAN_POINT('Ctrl Pts',(-17.91365079712,-16.8134710696799,123.222378870925)) ;
#44413=CARTESIAN_POINT('Ctrl Pts',(-18.2047179854304,-17.0033578333542,
123.468199338141)) ;
#44414=CARTESIAN_POINT('Ctrl Pts',(-17.9035805406861,-16.8233687529913,
123.482295776231)) ;
#44415=CARTESIAN_POINT('Ctrl Pts',(-18.232302562789,-17.0132888737282,123.675146887286)) ;
#44416=CARTESIAN_POINT('Ctrl Pts',(-17.938061631521,-16.8332997933653,123.740980891344)) ;
#44417=CARTESIAN_POINT('Ctrl Pts',(-18.2963248753717,-17.0233310913848,
123.876321281435)) ;
#44418=CARTESIAN_POINT('Ctrl Pts',(-18.018089634645,-16.8433420110219,123.992448629415)) ;
#44419=CARTESIAN_POINT('Ctrl Pts',(-18.3926605695863,-17.0332177521188,
124.06050712681)) ;
#44420=CARTESIAN_POINT('Ctrl Pts',(-18.1385099721154,-16.8532286717559,
124.222681786331)) ;
#44421=CARTESIAN_POINT('Ctrl Pts',(-18.5205878645769,-17.0432108607212,
124.227139826993)) ;
#44422=CARTESIAN_POINT('Ctrl Pts',(-18.2984195187527,-16.8632217803584,
124.430972590157)) ;
#44423=CARTESIAN_POINT('Ctrl Pts',(-18.674831224359,-17.0531565593595,124.368304779055)) ;
#44424=CARTESIAN_POINT('Ctrl Pts',(-18.4912243940808,-16.8731674789966,
124.607428923697)) ;
#44425=CARTESIAN_POINT('Ctrl Pts',(-18.8510481817693,-17.0631037816305,
124.480927513138)) ;
#44426=CARTESIAN_POINT('Ctrl Pts',(-18.7114963548054,-16.8831147012677,
124.748207213336)) ;
#44427=CARTESIAN_POINT('Ctrl Pts',(-19.0461761282001,-17.0731518072107,
124.561829669415)) ;
#44428=CARTESIAN_POINT('Ctrl Pts',(-18.9554062189626,-16.8931627268478,
124.849334419905)) ;
#44429=CARTESIAN_POINT('Ctrl Pts',(-19.2482340808857,-17.0829990543536,
124.606880354677)) ;
#44430=CARTESIAN_POINT('Ctrl Pts',(-19.2079801341472,-16.9030099739907,
124.905647599935)) ;
#44431=CARTESIAN_POINT('Ctrl Pts',(-19.4574454956206,-17.0929622314443,
124.616933495659)) ;
#44432=CARTESIAN_POINT('Ctrl Pts',(-19.4694948938835,-16.9129731510814,
124.918213293)) ;
#44433=CARTESIAN_POINT('Ctrl Pts',(-19.6665745901204,-17.1029919524777,
124.590015336654)) ;
#44434=CARTESIAN_POINT('Ctrl Pts',(-19.7309060814548,-16.9230028721148,
124.884564981777)) ;
#44435=CARTESIAN_POINT('Ctrl Pts',(-19.8654350785867,-17.1128964200106,
124.528216237133)) ;
#44436=CARTESIAN_POINT('Ctrl Pts',(-19.9794823375165,-16.9329073396477,
124.807315146919)) ;
#44437=CARTESIAN_POINT('Ctrl Pts',(-20.0527821290814,-17.1229209058404,
124.431754757046)) ;
#44438=CARTESIAN_POINT('Ctrl Pts',(-20.2136657521584,-16.9429318254775,
124.686737651366)) ;
#44439=CARTESIAN_POINT('Ctrl Pts',(-20.2186621175981,-17.1328247409643,
124.305869214479)) ;
#44440=CARTESIAN_POINT('Ctrl Pts',(-20.421015963903,-16.9528356606014,124.529379524787)) ;
#44441=CARTESIAN_POINT('Ctrl Pts',(-20.362268269371,-17.1428759316743,124.150890987089)) ;
#44442=CARTESIAN_POINT('Ctrl Pts',(-20.6005228715144,-16.9628868513114,
124.335656354932)) ;
#44443=CARTESIAN_POINT('Ctrl Pts',(-20.4749404633162,-17.1527603743326,
123.976262382427)) ;
#44444=CARTESIAN_POINT('Ctrl Pts',(-20.7413629698391,-16.9727712939697,
124.117369250282)) ;
#44445=CARTESIAN_POINT('Ctrl Pts',(-20.5568101272468,-17.1627533821844,
123.782806970068)) ;
#44446=CARTESIAN_POINT('Ctrl Pts',(-20.8436992076654,-16.9827643018216,
123.875549411217)) ;
#44447=CARTESIAN_POINT('Ctrl Pts',(-20.6035732599445,-17.1727017019007,
123.578943176126)) ;
#44448=CARTESIAN_POINT('Ctrl Pts',(-20.9021522987122,-16.9927126215379,
123.62071892228)) ;
#44449=CARTESIAN_POINT('Ctrl Pts',(-20.6145132332225,-17.1826385406102,
123.370344649638)) ;
#44450=CARTESIAN_POINT('Ctrl Pts',(-20.9158262169464,-17.0026494602473,
123.359970070186)) ;
#44451=CARTESIAN_POINT('Ctrl Pts',(-20.589206594443,-17.1926215295298,123.16197490794)) ;
#44452=CARTESIAN_POINT('Ctrl Pts',(-20.884191716522,-17.0126324491669,123.099507780396)) ;
#44453=CARTESIAN_POINT('Ctrl Pts',(-20.5273748243571,-17.2026654088939,
122.960102497268)) ;
#44454=CARTESIAN_POINT('Ctrl Pts',(-20.8069010684721,-17.022676328531,122.84716775239)) ;
#44455=CARTESIAN_POINT('Ctrl Pts',(-20.4339045567548,-17.2124934742523,
122.775800529378)) ;
#44456=CARTESIAN_POINT('Ctrl Pts',(-20.6900614936507,-17.0325043938894,
122.616789554295)) ;
#44457=CARTESIAN_POINT('Ctrl Pts',(-20.3068302236449,-17.2225705628072,
122.606349678098)) ;
#44458=CARTESIAN_POINT('Ctrl Pts',(-20.5312178370155,-17.0425814824443,
122.404977090048)) ;
#44459=CARTESIAN_POINT('Ctrl Pts',(-20.1557656867094,-17.2324207149635,
122.464630719431)) ;
#44460=CARTESIAN_POINT('Ctrl Pts',(-20.3423853676555,-17.0524316346006,
122.227828485222)) ;
#44461=CARTESIAN_POINT('Ctrl Pts',(-19.9784714409174,-17.2425011954158,
122.348631483285)) ;
#44462=CARTESIAN_POINT('Ctrl Pts',(-20.1207672096215,-17.062512115053,122.082830799905)) ;
#44463=CARTESIAN_POINT('Ctrl Pts',(-19.7888488448021,-17.2523156931847,
122.267175683269)) ;
#44464=CARTESIAN_POINT('Ctrl Pts',(-19.883737034747,-17.0723266128218,121.981011738217)) ;
#44465=CARTESIAN_POINT('Ctrl Pts',(-19.582938898268,-17.2623839892048,122.218356656156)) ;
#44466=CARTESIAN_POINT('Ctrl Pts',(-19.6263495978592,-17.0823949088419,
121.919989507403)) ;
#44467=CARTESIAN_POINT('Ctrl Pts',(-19.3751318674818,-17.2722828216876,
122.206291542029)) ;
#44468=CARTESIAN_POINT('Ctrl Pts',(-19.3665898868783,-17.0922937413247,
121.904909547411)) ;
#44469=CARTESIAN_POINT('Ctrl Pts',(-19.1652559904925,-17.2823357017021,
122.230785552897)) ;
#44470=CARTESIAN_POINT('Ctrl Pts',(-19.1042454569356,-17.1023466213392,
121.935528536243)) ;
#44471=CARTESIAN_POINT('Ctrl Pts',(-18.9663707089697,-17.2922055171983,
122.29008319877)) ;
#44472=CARTESIAN_POINT('Ctrl Pts',(-18.855638307516,-17.1122164368354,122.009652399298)) ;
#44473=CARTESIAN_POINT('Ctrl Pts',(-18.7770326931717,-17.3022781982811,
122.384835344758)) ;
#44474=CARTESIAN_POINT('Ctrl Pts',(-18.6189668205951,-17.1222891179182,
122.128093849741)) ;
#44475=CARTESIAN_POINT('Ctrl Pts',(-18.6109839358936,-17.312110676852,122.507981598294)) ;
#44476=CARTESIAN_POINT('Ctrl Pts',(-18.4114058096886,-17.1321215964892,
122.282028735497)) ;
#44477=CARTESIAN_POINT('Ctrl Pts',(-18.4655538333765,-17.3221413108381,
122.660674634817)) ;
#44478=CARTESIAN_POINT('Ctrl Pts',(-18.2296195608768,-17.1421522304753,
122.472896223419)) ;
#44479=CARTESIAN_POINT('Ctrl Pts',(-18.349337760532,-17.3321728680573,122.83667359108)) ;
#44480=CARTESIAN_POINT('Ctrl Pts',(-18.0843508674256,-17.1521837876944,
122.692895741896)) ;
#44481=CARTESIAN_POINT('Ctrl Pts',(-18.2667484940145,-17.342002576929,123.026088129245)) ;
#44482=CARTESIAN_POINT('Ctrl Pts',(-17.9811153912308,-17.1620134965661,
122.92966578504)) ;
#44483=CARTESIAN_POINT('Ctrl Pts',(-18.2169009601804,-17.3519920257311,
123.230102550982)) ;
#44484=CARTESIAN_POINT('Ctrl Pts',(-17.9188078334472,-17.1720029453682,
123.184684449035)) ;
#44485=CARTESIAN_POINT('Ctrl Pts',(-18.20369487068,-17.3620358781311,123.440840534949)) ;
#44486=CARTESIAN_POINT('Ctrl Pts',(-17.9023020185663,-17.1820467977682,
123.44810689289)) ;
#44487=CARTESIAN_POINT('Ctrl Pts',(-18.2263343781215,-17.3718575914632,
123.646078297448)) ;
#44488=CARTESIAN_POINT('Ctrl Pts',(-17.9306034522518,-17.1918685111003,
123.704655127921)) ;
#44489=CARTESIAN_POINT('Ctrl Pts',(-18.2850268408009,-17.3818925964519,
123.848716320605)) ;
#44490=CARTESIAN_POINT('Ctrl Pts',(-18.0039709952741,-17.201903516089,123.957951976954)) ;
#44491=CARTESIAN_POINT('Ctrl Pts',(-18.3784463059481,-17.3919174348995,
124.037642069545)) ;
#44492=CARTESIAN_POINT('Ctrl Pts',(-18.1207470223198,-17.2119283545366,
124.194108297233)) ;
#44493=CARTESIAN_POINT('Ctrl Pts',(-18.5007395484921,-17.4017696478547,
124.204809326343)) ;
#44494=CARTESIAN_POINT('Ctrl Pts',(-18.2736158124755,-17.2217805674918,
124.40306698223)) ;
#44495=CARTESIAN_POINT('Ctrl Pts',(-18.6520320192726,-17.4117596040485,
124.350454005425)) ;
#44496=CARTESIAN_POINT('Ctrl Pts',(-18.4627330156681,-17.2317705236856,
124.585121418507)) ;
#44497=CARTESIAN_POINT('Ctrl Pts',(-18.8252452575916,-17.4216877143317,
124.466918774105)) ;
#44498=CARTESIAN_POINT('Ctrl Pts',(-18.6792511906987,-17.2416986339689,
124.730700896654)) ;
#44499=CARTESIAN_POINT('Ctrl Pts',(-19.0170751012007,-17.4316763144113,
124.552359737803)) ;
#44500=CARTESIAN_POINT('Ctrl Pts',(-18.9190395513556,-17.2516872340484,
124.837500135833)) ;
#44501=CARTESIAN_POINT('Ctrl Pts',(-19.2216700740144,-17.4417029063388,
124.603105177326)) ;
#44502=CARTESIAN_POINT('Ctrl Pts',(-19.174783750514,-17.2617138259759,124.900929840425)) ;
#44503=CARTESIAN_POINT('Ctrl Pts',(-19.4289770875473,-17.451588034403,124.617568828443)) ;
#44504=CARTESIAN_POINT('Ctrl Pts',(-19.4339184087845,-17.2715989540401,
124.919007255833)) ;
#44505=CARTESIAN_POINT('Ctrl Pts',(-19.6379253432582,-17.4615791518765,
124.596058505797)) ;
#44506=CARTESIAN_POINT('Ctrl Pts',(-19.6951036459662,-17.2815900715136,
124.892117022616)) ;
#44507=CARTESIAN_POINT('Ctrl Pts',(-19.8408352338707,-17.4716197677283,
124.537884142129)) ;
#44508=CARTESIAN_POINT('Ctrl Pts',(-19.9487403100385,-17.2916306873654,
124.819396962872)) ;
#44509=CARTESIAN_POINT('Ctrl Pts',(-20.0267858411353,-17.481452758582,124.447583261545)) ;
#44510=CARTESIAN_POINT('Ctrl Pts',(-20.1811784262085,-17.3014636782191,
124.706518373388)) ;
#44511=CARTESIAN_POINT('Ctrl Pts',(-20.1973125975978,-17.4914458900323,
124.324881213278)) ;
#44512=CARTESIAN_POINT('Ctrl Pts',(-20.3943355471498,-17.3114568096694,
124.553138757061)) ;
#44513=CARTESIAN_POINT('Ctrl Pts',(-20.3442096502401,-17.5014779384677,
124.173532276575)) ;
#44514=CARTESIAN_POINT('Ctrl Pts',(-20.5779551582987,-17.3214888581048,
124.36395098382)) ;
#44515=CARTESIAN_POINT('Ctrl Pts',(-20.460827682046,-17.5113431850101,124.002039230905)) ;
#44516=CARTESIAN_POINT('Ctrl Pts',(-20.7237261254064,-17.3313541046472,
124.149582721403)) ;
#44517=CARTESIAN_POINT('Ctrl Pts',(-20.5472792275311,-17.5213050598369,
123.811278450178)) ;
#44518=CARTESIAN_POINT('Ctrl Pts',(-20.831788362086,-17.341315979474,123.911130472896)) ;
#44519=CARTESIAN_POINT('Ctrl Pts',(-20.5993376398069,-17.5313400229482,
123.606847846578)) ;
#44520=CARTESIAN_POINT('Ctrl Pts',(-20.8968589917748,-17.3513509425853,
123.655591647109)) ;
#44521=CARTESIAN_POINT('Ctrl Pts',(-20.615228249655,-17.5412248674106,123.399615410114)) ;
#44522=CARTESIAN_POINT('Ctrl Pts',(-20.9167197829666,-17.3612357870477,
123.396550342786)) ;
#44523=CARTESIAN_POINT('Ctrl Pts',(-20.5944747720619,-17.5512909202513,
123.189052375223)) ;
#44524=CARTESIAN_POINT('Ctrl Pts',(-20.8907754476135,-17.3713018398884,
123.133346946234)) ;
#44525=CARTESIAN_POINT('Ctrl Pts',(-20.5389734302153,-17.5611284361603,
122.989783502597)) ;
#44526=CARTESIAN_POINT('Ctrl Pts',(-20.8213961192781,-17.3811393557974,
122.88426085308)) ;
#44527=CARTESIAN_POINT('Ctrl Pts',(-20.4478531306755,-17.5711971842692,
122.798763312751)) ;
#44528=CARTESIAN_POINT('Ctrl Pts',(-20.7074934610674,-17.3912081039063,
122.645486865945)) ;
#44529=CARTESIAN_POINT('Ctrl Pts',(-20.3271452161414,-17.5810777013002,
122.629676892913)) ;
#44530=CARTESIAN_POINT('Ctrl Pts',(-20.5566061673441,-17.4010886209373,
122.434129920283)) ;
#44531=CARTESIAN_POINT('Ctrl Pts',(-20.1775948897127,-17.5910688882346,
122.482227937037)) ;
#44532=CARTESIAN_POINT('Ctrl Pts',(-20.3696663136538,-17.4110798078718,
122.249820531952)) ;
#44533=CARTESIAN_POINT('Ctrl Pts',(-20.0053412492469,-17.6010219545096,
122.363377773261)) ;
#44534=CARTESIAN_POINT('Ctrl Pts',(-20.1543475643769,-17.4210328741467,
122.101259878823)) ;
#44535=CARTESIAN_POINT('Ctrl Pts',(-19.8135014291807,-17.6110577920422,
122.275600289609)) ;
#44536=CARTESIAN_POINT('Ctrl Pts',(-19.9145466995836,-17.4310687116793,
121.991540433781)) ;
#44537=CARTESIAN_POINT('Ctrl Pts',(-19.6123051874755,-17.6209479182536,
122.223092310276)) ;
#44538=CARTESIAN_POINT('Ctrl Pts',(-19.6630503154042,-17.4409588378907,
121.925907930665)) ;
#44539=CARTESIAN_POINT('Ctrl Pts',(-19.4029610311012,-17.6309401001616,
122.205808818066)) ;
#44540=CARTESIAN_POINT('Ctrl Pts',(-19.4013697921715,-17.4509510197987,
121.904306259386)) ;
#44541=CARTESIAN_POINT('Ctrl Pts',(-19.1947594778902,-17.6408860401002,
122.225118763395)) ;
#44542=CARTESIAN_POINT('Ctrl Pts',(-19.1411178680801,-17.4608969597373,
121.928446401877)) ;
#44543=CARTESIAN_POINT('Ctrl Pts',(-18.9929258923836,-17.6508332238642,
122.279886430677)) ;
#44544=CARTESIAN_POINT('Ctrl Pts',(-18.88882641169,-17.4708441435014,121.996908692805)) ;
#44545=CARTESIAN_POINT('Ctrl Pts',(-18.8018677982958,-17.6608811621717,
122.369974731862)) ;
#44546=CARTESIAN_POINT('Ctrl Pts',(-18.6500049664529,-17.4808920818088,
122.109521528359)) ;
#44547=CARTESIAN_POINT('Ctrl Pts',(-18.6326849760237,-17.670728796912,122.489300515306)) ;
#44548=CARTESIAN_POINT('Ctrl Pts',(-18.4385276907917,-17.4907397165491,
122.258681232222)) ;
#44549=CARTESIAN_POINT('Ctrl Pts',(-18.48464394166,-17.6806905108858,122.637419729703)) ;
#44550=CARTESIAN_POINT('Ctrl Pts',(-18.2534782916843,-17.5007014305229,
122.443832320291)) ;
#44551=CARTESIAN_POINT('Ctrl Pts',(-18.3639692527773,-17.6907191456766,
122.810318421013)) ;
#44552=CARTESIAN_POINT('Ctrl Pts',(-18.1026371828242,-17.5107300653138,
122.659957308441)) ;
#44553=CARTESIAN_POINT('Ctrl Pts',(-18.2761446006497,-17.7006294642738,
122.999238769557)) ;
#44554=CARTESIAN_POINT('Ctrl Pts',(-17.9928588043532,-17.5206403839109,
122.896109111999)) ;
#44555=CARTESIAN_POINT('Ctrl Pts',(-18.2217890454544,-17.7105643205853,
123.200911892758)) ;
#44556=CARTESIAN_POINT('Ctrl Pts',(-17.9249170447996,-17.5305752402224,
123.148201377917)) ;
#44557=CARTESIAN_POINT('Ctrl Pts',(-18.2032822313656,-17.720605556546,123.411187682898)) ;
#44558=CARTESIAN_POINT('Ctrl Pts',(-17.9017863181592,-17.5406164761831,
123.41104640664)) ;
#44559=CARTESIAN_POINT('Ctrl Pts',(-18.2211170108079,-17.730492328126,123.618292553974)) ;
#44560=CARTESIAN_POINT('Ctrl Pts',(-17.9240826085059,-17.5505032477631,
123.669927416836)) ;
#44561=CARTESIAN_POINT('Ctrl Pts',(-18.2749965572381,-17.7404925068322,
123.821474487423)) ;
#44562=CARTESIAN_POINT('Ctrl Pts',(-17.991434789336,-17.5605034264693,123.923904177985)) ;
#44563=CARTESIAN_POINT('Ctrl Pts',(-18.36246816189,-17.7504097850418,124.010768806246)) ;
#44564=CARTESIAN_POINT('Ctrl Pts',(-18.1007768933539,-17.5704207046789,
124.160520976212)) ;
#44565=CARTESIAN_POINT('Ctrl Pts',(-18.48305480673,-17.7604570314554,124.184154003306)) ;
#44566=CARTESIAN_POINT('Ctrl Pts',(-18.2515125585857,-17.5804679510926,
124.377250917313)) ;
#44567=CARTESIAN_POINT('Ctrl Pts',(-18.629232331941,-17.7703309204367,124.331582621373)) ;
#44568=CARTESIAN_POINT('Ctrl Pts',(-18.4342365122274,-17.5903418400739,
124.561534748343)) ;
#44569=CARTESIAN_POINT('Ctrl Pts',(-18.8019032378778,-17.7803929380173,
124.453733894309)) ;
#44570=CARTESIAN_POINT('Ctrl Pts',(-18.6500768441802,-17.6004038576544,
124.714221581004)) ;
#44571=CARTESIAN_POINT('Ctrl Pts',(-18.9895800757917,-17.7902639997516,
124.542325237439)) ;
#44572=CARTESIAN_POINT('Ctrl Pts',(-18.8846741125319,-17.6102749193887,
124.82495821564)) ;
#44573=CARTESIAN_POINT('Ctrl Pts',(-19.1921134940513,-17.8002580631119,
124.598226493753)) ;
#44574=CARTESIAN_POINT('Ctrl Pts',(-19.1378416764729,-17.620268982749,124.894832090563)) ;
#44575=CARTESIAN_POINT('Ctrl Pts',(-19.4021121856622,-17.8102902211453,
124.617721341239)) ;
#44576=CARTESIAN_POINT('Ctrl Pts',(-19.4003404043878,-17.6303011407824,
124.919197850728)) ;
#44577=CARTESIAN_POINT('Ctrl Pts',(-19.608844588004,-17.8201540973854,124.601197546684)) ;
#44578=CARTESIAN_POINT('Ctrl Pts',(-19.6587556166457,-17.6401650170226,
124.898540308878)) ;
#44579=CARTESIAN_POINT('Ctrl Pts',(-19.8137331839509,-17.8302246120237,
124.54797156307)) ;
#44580=CARTESIAN_POINT('Ctrl Pts',(-19.9148657636072,-17.6502355316608,
124.832005118292)) ;
#44581=CARTESIAN_POINT('Ctrl Pts',(-20.0019178911935,-17.8400652489647,
124.461988692631)) ;
#44582=CARTESIAN_POINT('Ctrl Pts',(-20.150095477634,-17.6600761686018,124.724523892798)) ;
#44583=CARTESIAN_POINT('Ctrl Pts',(-20.1748685848524,-17.8500323778049,
124.343718173055)) ;
#44584=CARTESIAN_POINT('Ctrl Pts',(-20.3662817216806,-17.670043297442,124.576684081866)) ;
#44585=CARTESIAN_POINT('Ctrl Pts',(-20.3252263227975,-17.8600463509294,
124.196347627969)) ;
#44586=CARTESIAN_POINT('Ctrl Pts',(-20.5542290543161,-17.6800572705665,
124.392466662647)) ;
#44587=CARTESIAN_POINT('Ctrl Pts',(-20.4877929513438,-17.8733310847927,
123.96921781494)) ;
#44588=CARTESIAN_POINT('Ctrl Pts',(-20.7574242465171,-17.6933420044298,
124.108563216833)) ;
#44589=CARTESIAN_POINT('Ctrl Pts',(-20.5871211093539,-17.8865563495074,
123.706157520284)) ;
#44590=CARTESIAN_POINT('Ctrl Pts',(-20.8815792327918,-17.7065672691446,
123.779776387227)) ;
#44591=CARTESIAN_POINT('Ctrl Pts',(-20.6152234023706,-17.8998668720623,
123.427758973367)) ;
#44592=CARTESIAN_POINT('Ctrl Pts',(-20.9167156267444,-17.7198777916994,
123.431719811702)) ;
#44593=CARTESIAN_POINT('Ctrl Pts',(-20.5994871791015,-17.9098955169645,
123.217511431126)) ;
#44594=CARTESIAN_POINT('Ctrl Pts',(-20.8970403045933,-17.7299064366016,
123.168922156233)) ;
#44595=CARTESIAN_POINT('Ctrl Pts',(-20.5484258087731,-17.9197765493184,
123.01615172322)) ;
#44596=CARTESIAN_POINT('Ctrl Pts',(-20.833211337434,-17.7397874689555,122.917220164191)) ;
#44597=CARTESIAN_POINT('Ctrl Pts',(-20.462715022261,-17.9297575219985,122.82462433537)) ;
#44598=CARTESIAN_POINT('Ctrl Pts',(-20.7260717926928,-17.7497684416356,
122.677813694401)) ;
#44599=CARTESIAN_POINT('Ctrl Pts',(-20.3449102482183,-17.9397386495845,
122.650999042694)) ;
#44600=CARTESIAN_POINT('Ctrl Pts',(-20.5788081877206,-17.7597495692216,
122.460780265078)) ;
#44601=CARTESIAN_POINT('Ctrl Pts',(-20.1513290480844,-17.9529818398459,
122.450788742147)) ;
#44602=CARTESIAN_POINT('Ctrl Pts',(-20.3368568947388,-17.772992759483,122.21053545582)) ;
#44603=CARTESIAN_POINT('Ctrl Pts',(-19.8474795977767,-17.9696498352067,
122.268601957147)) ;
#44604=CARTESIAN_POINT('Ctrl Pts',(-19.9569936985326,-17.7896607548438,
121.982786748505)) ;
#44605=CARTESIAN_POINT('Ctrl Pts',(-19.5025885485555,-17.9861703352187,
122.201337269194)) ;
#44606=CARTESIAN_POINT('Ctrl Pts',(-19.5259606159641,-17.8061812548558,
121.898720902141)) ;
#44607=CARTESIAN_POINT('Ctrl Pts',(-19.2234322226272,-17.9994833515347,
122.220261932405)) ;
#44608=CARTESIAN_POINT('Ctrl Pts',(-19.1769501917683,-17.8194942711718,
121.922374301912)) ;
#44609=CARTESIAN_POINT('Ctrl Pts',(-19.0209334833378,-18.0093999097677,
122.270017422137)) ;
#44610=CARTESIAN_POINT('Ctrl Pts',(-18.9238414463951,-17.8294108294048,
121.984571342196)) ;
#44611=CARTESIAN_POINT('Ctrl Pts',(-18.8281337131634,-18.0194275780706,
122.355152407899)) ;
#44612=CARTESIAN_POINT('Ctrl Pts',(-18.6828367951169,-17.8394384977077,
122.090994480729)) ;
#44613=CARTESIAN_POINT('Ctrl Pts',(-18.5974653025486,-18.0326081678152,
122.508905891752)) ;
#44614=CARTESIAN_POINT('Ctrl Pts',(-18.394515897223,-17.8526190874524,122.283176068422)) ;
#44615=CARTESIAN_POINT('Ctrl Pts',(-18.3626740824795,-18.0493563069346,
122.776403364024)) ;
#44616=CARTESIAN_POINT('Ctrl Pts',(-18.1010163558912,-17.8693672265717,
122.617564692546)) ;
#44617=CARTESIAN_POINT('Ctrl Pts',(-18.2093429381581,-18.0691510494452,
123.168585983566)) ;
#44618=CARTESIAN_POINT('Ctrl Pts',(-17.909361184572,-17.8891619690823,123.107788785577)) ;
#44619=CARTESIAN_POINT('Ctrl Pts',(-18.1984950373618,-18.089195442254,123.594497284543)) ;
#44620=CARTESIAN_POINT('Ctrl Pts',(-17.8958042831171,-17.9092063618911,
123.640179567808)) ;
#44621=CARTESIAN_POINT('Ctrl Pts',(-18.3326878160101,-18.1090346245527,
123.994538645704)) ;
#44622=CARTESIAN_POINT('Ctrl Pts',(-18.0635490482974,-17.9290455441898,
124.140228438831)) ;
#44623=CARTESIAN_POINT('Ctrl Pts',(-18.595526380158,-18.1289599482456,124.326686433183)) ;
#44624=CARTESIAN_POINT('Ctrl Pts',(-18.3920994920008,-17.9489708678827,
124.555410464658)) ;
#44625=CARTESIAN_POINT('Ctrl Pts',(-18.9560767803861,-18.1488835862971,
124.549228315396)) ;
#44626=CARTESIAN_POINT('Ctrl Pts',(-18.842788696369,-17.9688945059342,124.833584548175)) ;
#44627=CARTESIAN_POINT('Ctrl Pts',(-19.3708100254435,-18.1688084597626,
124.63548572576)) ;
#44628=CARTESIAN_POINT('Ctrl Pts',(-19.3612051307133,-17.9888193793997,
124.941403037166)) ;
#44629=CARTESIAN_POINT('Ctrl Pts',(-19.7892611661208,-18.1886870668415,
124.575714298968)) ;
#44630=CARTESIAN_POINT('Ctrl Pts',(-19.8842672961237,-18.0086979864787,
124.866686275026)) ;
#44631=CARTESIAN_POINT('Ctrl Pts',(-20.1641187112948,-18.2086645096735,
124.375945013966)) ;
#44632=CARTESIAN_POINT('Ctrl Pts',(-20.3528378762813,-18.0286754293106,
124.616972672775)) ;
#44633=CARTESIAN_POINT('Ctrl Pts',(-20.4474662277744,-18.2285963577582,
124.06073373373)) ;
#44634=CARTESIAN_POINT('Ctrl Pts',(-20.7070199751766,-18.0486072773953,
124.222957551387)) ;
#44635=CARTESIAN_POINT('Ctrl Pts',(-20.6063082660546,-18.2484916261008,
123.668688283209)) ;
#44636=CARTESIAN_POINT('Ctrl Pts',(-20.9055702118375,-18.0685025457379,
123.732901280458)) ;
#44637=CARTESIAN_POINT('Ctrl Pts',(-20.6223259515978,-18.2684141245129,
123.245374252905)) ;
#44638=CARTESIAN_POINT('Ctrl Pts',(-20.9255908588565,-18.08842504415,123.203759760806)) ;
#44639=CARTESIAN_POINT('Ctrl Pts',(-20.4925770960382,-18.2883736063889,
122.841276292266)) ;
#44640=CARTESIAN_POINT('Ctrl Pts',(-20.7634037510858,-18.108384526026,122.69863823452)) ;
#44641=CARTESIAN_POINT('Ctrl Pts',(-20.2338987435689,-18.3082513588482,
122.507109401429)) ;
#44642=CARTESIAN_POINT('Ctrl Pts',(-20.4400561873198,-18.1282622784854,
122.280931726728)) ;
#44643=CARTESIAN_POINT('Ctrl Pts',(-19.8771610118705,-18.3281331495828,
122.280132547987)) ;
#44644=CARTESIAN_POINT('Ctrl Pts',(-19.9941357017279,-18.1481440692199,
121.997211525704)) ;
#44645=CARTESIAN_POINT('Ctrl Pts',(-19.4603627437856,-18.3482064884338,
122.188495687106)) ;
#44646=CARTESIAN_POINT('Ctrl Pts',(-19.473136676439,-18.1682174080709,121.882665391242)) ;
#44647=CARTESIAN_POINT('Ctrl Pts',(-19.0428183765593,-18.3680109556696,
122.243747752997)) ;
#44648=CARTESIAN_POINT('Ctrl Pts',(-18.9512092802025,-18.1880218753067,
121.951729931367)) ;
#44649=CARTESIAN_POINT('Ctrl Pts',(-18.6655136826897,-18.3879942960774,
122.439019897287)) ;
#44650=CARTESIAN_POINT('Ctrl Pts',(-18.4795781028299,-18.2080052157145,
122.195819043251)) ;
#44651=CARTESIAN_POINT('Ctrl Pts',(-18.3789384655421,-18.4079092606754,
122.750760297529)) ;
#44652=CARTESIAN_POINT('Ctrl Pts',(-18.1213593079001,-18.2279201803125,
122.585493056781)) ;
#44653=CARTESIAN_POINT('Ctrl Pts',(-18.2152038691917,-18.4277777953917,
123.140286780608)) ;
#44654=CARTESIAN_POINT('Ctrl Pts',(-17.9166900271828,-18.2477887150289,
123.072398846961)) ;
#44655=CARTESIAN_POINT('Ctrl Pts',(-18.1947300807791,-18.4478301796035,
123.566037893384)) ;
#44656=CARTESIAN_POINT('Ctrl Pts',(-17.891096129626,-18.2678410992406,123.604588275985)) ;
#44657=CARTESIAN_POINT('Ctrl Pts',(-18.3185671471098,-18.4676041433927,
123.96801283456)) ;
#44658=CARTESIAN_POINT('Ctrl Pts',(-18.0458895721995,-18.2876150630298,
124.107054946119)) ;
#44659=CARTESIAN_POINT('Ctrl Pts',(-18.5752678737993,-18.487658522414,124.308284568343)) ;
#44660=CARTESIAN_POINT('Ctrl Pts',(-18.3667637788578,-18.3076694420512,
124.53239666562)) ;
#44661=CARTESIAN_POINT('Ctrl Pts',(-18.9284212326359,-18.5074552599873,
124.537569903936)) ;
#44662=CARTESIAN_POINT('Ctrl Pts',(-18.8082021318572,-18.3274661796244,
124.819004328744)) ;
#44663=CARTESIAN_POINT('Ctrl Pts',(-19.3416803678244,-18.5274230723387,
124.634498823647)) ;
#44664=CARTESIAN_POINT('Ctrl Pts',(-19.3247749684746,-18.3474339919759,
124.940168786496)) ;
#44665=CARTESIAN_POINT('Ctrl Pts',(-19.7631205986786,-18.5473820484038,
124.583927911147)) ;
#44666=CARTESIAN_POINT('Ctrl Pts',(-19.8515753099783,-18.3673929680409,
124.876958419446)) ;
#44667=CARTESIAN_POINT('Ctrl Pts',(-20.1408243512989,-18.5672769666812,
124.393475715096)) ;
#44668=CARTESIAN_POINT('Ctrl Pts',(-20.323705737491,-18.3872878863183,124.638896796326)) ;
#44669=CARTESIAN_POINT('Ctrl Pts',(-20.4312496937618,-18.5871732791315,
124.085918903188)) ;
#44670=CARTESIAN_POINT('Ctrl Pts',(-20.6867396805035,-18.4071841987686,
124.254454112951)) ;
#44671=CARTESIAN_POINT('Ctrl Pts',(-20.5998462621265,-18.6070812125056,
123.69761409053)) ;
#44672=CARTESIAN_POINT('Ctrl Pts',(-20.8974889909594,-18.4270921321427,
123.769075405427)) ;
#44673=CARTESIAN_POINT('Ctrl Pts',(-20.6258188714983,-18.6270311027941,
123.274258003805)) ;
#44674=CARTESIAN_POINT('Ctrl Pts',(-20.9299591274622,-18.4470420224312,
123.239880881336)) ;
#44675=CARTESIAN_POINT('Ctrl Pts',(-20.5065921902261,-18.6469083332954,
122.868736889825)) ;
#44676=CARTESIAN_POINT('Ctrl Pts',(-20.7809301918273,-18.4669192529325,
122.732978965387)) ;
#44677=CARTESIAN_POINT('Ctrl Pts',(-20.2550219026943,-18.6668910021664,
122.526359546569)) ;
#44678=CARTESIAN_POINT('Ctrl Pts',(-20.4664719534886,-18.4869019218035,
122.305004321908)) ;
#44679=CARTESIAN_POINT('Ctrl Pts',(-19.9023778798508,-18.6868238887468,
122.291166846904)) ;
#44680=CARTESIAN_POINT('Ctrl Pts',(-20.0256670326121,-18.5068348083839,
122.011010324086)) ;
#44681=CARTESIAN_POINT('Ctrl Pts',(-19.4912013862512,-18.7067366347647,
122.190280264544)) ;
#44682=CARTESIAN_POINT('Ctrl Pts',(-19.5117084694408,-18.5267475544018,
121.884894904274)) ;
#44683=CARTESIAN_POINT('Ctrl Pts',(-19.1409101901299,-18.7233063561065,
122.227714641459)) ;
#44684=CARTESIAN_POINT('Ctrl Pts',(-19.0738118336098,-18.5433172757436,
121.93169130508)) ;
#44685=CARTESIAN_POINT('Ctrl Pts',(-18.8799531775115,-18.7366063674115,
122.328226065219)) ;
#44686=CARTESIAN_POINT('Ctrl Pts',(-18.7476501460358,-18.5566172870486,
122.057314468906)) ;
#44687=CARTESIAN_POINT('Ctrl Pts',(-18.6408115625997,-18.7498765551614,
122.471815662188)) ;
#44688=CARTESIAN_POINT('Ctrl Pts',(-18.4486656986035,-18.5698874747985,
122.23684236878)) ;
#44689=CARTESIAN_POINT('Ctrl Pts',(-18.3949285657691,-18.7665039375268,
122.725952569314)) ;
#44690=CARTESIAN_POINT('Ctrl Pts',(-18.1413722273347,-18.5865148571639,
122.554451895096)) ;
#44691=CARTESIAN_POINT('Ctrl Pts',(-18.2507607995782,-18.783126227272,123.048601698657)) ;
#44692=CARTESIAN_POINT('Ctrl Pts',(-17.9611265356219,-18.6031371469091,
122.957810899862)) ;
#44693=CARTESIAN_POINT('Ctrl Pts',(-18.2066124842382,-18.7963714416665,
123.323560231487)) ;
#44694=CARTESIAN_POINT('Ctrl Pts',(-17.9059528961361,-18.6163823613036,
123.301475150408)) ;
#44695=CARTESIAN_POINT('Ctrl Pts',(-18.2091963113951,-18.8062834066272,
123.531933666297)) ;
#44696=CARTESIAN_POINT('Ctrl Pts',(-17.9091768534027,-18.6262943262643,
123.561948497621)) ;
#44697=CARTESIAN_POINT('Ctrl Pts',(-18.2487269856474,-18.8163420297916,
123.739647393853)) ;
#44698=CARTESIAN_POINT('Ctrl Pts',(-17.9585883655337,-18.6363529494288,
123.821589557109)) ;
#44699=CARTESIAN_POINT('Ctrl Pts',(-18.3218273859011,-18.8261821439075,
123.933204366604)) ;
#44700=CARTESIAN_POINT('Ctrl Pts',(-18.0499609717764,-18.6461930635446,
124.06353698501)) ;
#44701=CARTESIAN_POINT('Ctrl Pts',(-18.4296324438484,-18.8362479288651,
124.115263613763)) ;
#44702=CARTESIAN_POINT('Ctrl Pts',(-18.1847150492908,-18.6562588485022,
124.291112489594)) ;
#44703=CARTESIAN_POINT('Ctrl Pts',(-18.5650197569021,-18.846131246653,124.27291340767)) ;
#44704=CARTESIAN_POINT('Ctrl Pts',(-18.3539469883158,-18.6661421662901,
124.488176476276)) ;
#44705=CARTESIAN_POINT('Ctrl Pts',(-18.7271216090986,-18.8561206845115,
124.40639870705)) ;
#44706=CARTESIAN_POINT('Ctrl Pts',(-18.5565725704209,-18.6761316041487,
124.655035297587)) ;
#44707=CARTESIAN_POINT('Ctrl Pts',(-18.9095316281554,-18.8660843985643,
124.509393822221)) ;
#44708=CARTESIAN_POINT('Ctrl Pts',(-18.7845837390266,-18.6860953182014,
124.783781642268)) ;
#44709=CARTESIAN_POINT('Ctrl Pts',(-19.1076061689565,-18.8760794102235,
124.579581320828)) ;
#44710=CARTESIAN_POINT('Ctrl Pts',(-19.0321760408685,-18.6960903298606,
124.871518685265)) ;
#44711=CARTESIAN_POINT('Ctrl Pts',(-19.3157436958266,-18.8861157019177,
124.61412399333)) ;
#44712=CARTESIAN_POINT('Ctrl Pts',(-19.2923475774158,-18.7061266215549,
124.914699798494)) ;
#44713=CARTESIAN_POINT('Ctrl Pts',(-19.5227505678203,-18.8959620796112,
124.612380202904)) ;
#44714=CARTESIAN_POINT('Ctrl Pts',(-19.5511061455371,-18.7159729992483,
124.912522869748)) ;
#44715=CARTESIAN_POINT('Ctrl Pts',(-19.7292055330348,-18.9059470237619,
124.57459229136)) ;
#44716=CARTESIAN_POINT('Ctrl Pts',(-19.8091754394204,-18.725957943399,124.865290742735)) ;
#44717=CARTESIAN_POINT('Ctrl Pts',(-19.9251198106704,-18.9158839948918,
124.501974601842)) ;
#44718=CARTESIAN_POINT('Ctrl Pts',(-20.0540693302501,-18.735894914529,124.774521245313)) ;
#44719=CARTESIAN_POINT('Ctrl Pts',(-20.1073932158431,-18.9259337795236,
124.395175327921)) ;
#44720=CARTESIAN_POINT('Ctrl Pts',(-20.2819125648932,-18.7459446991607,
124.64102455522)) ;
#44721=CARTESIAN_POINT('Ctrl Pts',(-20.2652907922645,-18.9357842416011,
124.261160532584)) ;
#44722=CARTESIAN_POINT('Ctrl Pts',(-20.4792864441643,-18.7557951612382,
124.473508135846)) ;
#44723=CARTESIAN_POINT('Ctrl Pts',(-20.3995458132042,-18.9457562551215,
124.100179995345)) ;
#44724=CARTESIAN_POINT('Ctrl Pts',(-20.6471074503595,-18.7657671747586,
124.272284173853)) ;
#44725=CARTESIAN_POINT('Ctrl Pts',(-20.5040579564351,-18.9557514022409,
123.91784560784)) ;
#44726=CARTESIAN_POINT('Ctrl Pts',(-20.7777500986428,-18.775762321878,124.044367513356)) ;
#44727=CARTESIAN_POINT('Ctrl Pts',(-20.5753422248365,-18.965785371977,123.71932854599)) ;
#44728=CARTESIAN_POINT('Ctrl Pts',(-20.86685809816,-18.7857962916141,123.796222100934)) ;
#44729=CARTESIAN_POINT('Ctrl Pts',(-20.6107665468007,-18.9756409176476,
123.515165091888)) ;
#44730=CARTESIAN_POINT('Ctrl Pts',(-20.9111412970602,-18.7956518372847,
123.541018035015)) ;
#44731=CARTESIAN_POINT('Ctrl Pts',(-20.6104909571507,-18.9856396746608,
123.304993816628)) ;
#44732=CARTESIAN_POINT('Ctrl Pts',(-20.9107995971931,-18.8056505942979,
123.278303845419)) ;
#44733=CARTESIAN_POINT('Ctrl Pts',(-20.5742854817518,-18.995536809898,123.100067497722)) ;
#44734=CARTESIAN_POINT('Ctrl Pts',(-20.8655454311932,-18.8155477295351,
123.022145216685)) ;
#44735=CARTESIAN_POINT('Ctrl Pts',(-20.5019793355474,-19.0055899057376,
122.901496245715)) ;
#44736=CARTESIAN_POINT('Ctrl Pts',(-20.7751653502272,-18.8256008253747,
122.773930212868)) ;
#44737=CARTESIAN_POINT('Ctrl Pts',(-20.3980758274042,-19.0154734144682,
122.721542018855)) ;
#44738=CARTESIAN_POINT('Ctrl Pts',(-20.6452882013384,-18.8354843341053,
122.54898577994)) ;
#44739=CARTESIAN_POINT('Ctrl Pts',(-20.2633899531571,-19.0254682871143,
122.560268873648)) ;
#44740=CARTESIAN_POINT('Ctrl Pts',(-20.4769328739096,-18.8454792067514,
122.347392525977)) ;
#44741=CARTESIAN_POINT('Ctrl Pts',(-20.1021192146536,-19.03548824875,122.424730589061)) ;
#44742=CARTESIAN_POINT('Ctrl Pts',(-20.2753461930725,-18.8554991683871,
122.177967546874)) ;
#44743=CARTESIAN_POINT('Ctrl Pts',(-19.9219503779301,-19.0453936125498,
122.320315131971)) ;
#44744=CARTESIAN_POINT('Ctrl Pts',(-20.0501362495513,-18.865404532187,122.047445707246)) ;
#44745=CARTESIAN_POINT('Ctrl Pts',(-19.725850127901,-19.0553342001574,122.248117440437)) ;
#44746=CARTESIAN_POINT('Ctrl Pts',(-19.8050116122211,-18.8753451197945,
121.957195984845)) ;
#44747=CARTESIAN_POINT('Ctrl Pts',(-19.5188889597631,-19.065337018258,122.21070880174)) ;
#44748=CARTESIAN_POINT('Ctrl Pts',(-19.5463105434524,-18.8853479378952,
121.910432554943)) ;
#44749=CARTESIAN_POINT('Ctrl Pts',(-19.3079401318783,-19.0753717299822,
122.210144775601)) ;
#44750=CARTESIAN_POINT('Ctrl Pts',(-19.2826245313416,-18.8953826496193,
121.909724812354)) ;
#44751=CARTESIAN_POINT('Ctrl Pts',(-19.1039450954541,-19.0852166367195,
122.245193265837)) ;
#44752=CARTESIAN_POINT('Ctrl Pts',(-19.0276297317745,-18.9052275563566,
121.953532899944)) ;
#44753=CARTESIAN_POINT('Ctrl Pts',(-18.9062559735361,-19.0952024892885,
122.315743265558)) ;
#44754=CARTESIAN_POINT('Ctrl Pts',(-18.7805173029334,-18.9152134089256,
122.041718002023)) ;
#44755=CARTESIAN_POINT('Ctrl Pts',(-18.7246158514163,-19.1051372977015,
122.418922406294)) ;
#44756=CARTESIAN_POINT('Ctrl Pts',(-18.5534655977386,-18.9251482173387,
122.170689853634)) ;
#44757=CARTESIAN_POINT('Ctrl Pts',(-18.5618355249981,-19.1151948247826,
122.553818901335)) ;
#44758=CARTESIAN_POINT('Ctrl Pts',(-18.3499886138001,-18.9352057444197,
122.33930838977)) ;
#44759=CARTESIAN_POINT('Ctrl Pts',(-18.4278858922511,-19.1250164797797,
122.710986226802)) ;
#44760=CARTESIAN_POINT('Ctrl Pts',(-18.1825491267777,-18.9450273994168,
122.535766487528)) ;
#44761=CARTESIAN_POINT('Ctrl Pts',(-18.3204432885905,-19.1350725239527,
122.893038269463)) ;
#44762=CARTESIAN_POINT('Ctrl Pts',(-18.0482437942149,-18.9550834435898,
122.76333018742)) ;
#44763=CARTESIAN_POINT('Ctrl Pts',(-18.2474379776068,-19.1450132639979,
123.088867079134)) ;
#44764=CARTESIAN_POINT('Ctrl Pts',(-17.9569846493071,-18.965024183635,123.008115620737)) ;
#44765=CARTESIAN_POINT('Ctrl Pts',(-18.2090421542517,-19.1549173850707,
123.293514642458)) ;
#44766=CARTESIAN_POINT('Ctrl Pts',(-17.9089873948513,-18.9749283047079,
123.26392514927)) ;
#44767=CARTESIAN_POINT('Ctrl Pts',(-18.2068596104492,-19.164964926225,123.504719529866)) ;
#44768=CARTESIAN_POINT('Ctrl Pts',(-17.9062567714271,-18.9849758458621,
123.527931134947)) ;
#44769=CARTESIAN_POINT('Ctrl Pts',(-18.2407268057589,-19.1748636778254,
123.710075861997)) ;
#44770=CARTESIAN_POINT('Ctrl Pts',(-17.9485884795945,-18.9948745974625,
123.784627499312)) ;
#44771=CARTESIAN_POINT('Ctrl Pts',(-18.3106763440572,-19.1849121567912,
123.909385049677)) ;
#44772=CARTESIAN_POINT('Ctrl Pts',(-18.0360231031298,-19.0049230764283,
124.033764662916)) ;
#44773=CARTESIAN_POINT('Ctrl Pts',(-18.4125198148673,-19.1947996538749,
124.09061780245)) ;
#44774=CARTESIAN_POINT('Ctrl Pts',(-18.163325670764,-19.014810573512,124.260307326459)) ;
#44775=CARTESIAN_POINT('Ctrl Pts',(-18.5453641416013,-19.204792744173,124.253347261805)) ;
#44776=CARTESIAN_POINT('Ctrl Pts',(-18.3293793931802,-19.0248036638101,
124.463720725707)) ;
#44777=CARTESIAN_POINT('Ctrl Pts',(-18.70386501416,-19.2147449142333,124.389942305651)) ;
#44778=CARTESIAN_POINT('Ctrl Pts',(-18.5275042406602,-19.0347558338704,
124.634466519872)) ;
#44779=CARTESIAN_POINT('Ctrl Pts',(-18.8832573055452,-19.2246833341478,
124.497026002691)) ;
#44780=CARTESIAN_POINT('Ctrl Pts',(-18.7517438317463,-19.0446942537849,
124.768323296831)) ;
#44781=CARTESIAN_POINT('Ctrl Pts',(-19.0793846745513,-19.2346684642334,
124.571917646202)) ;
#44782=CARTESIAN_POINT('Ctrl Pts',(-18.9969024435329,-19.0546793838705,
124.861939962815)) ;
#44783=CARTESIAN_POINT('Ctrl Pts',(-19.2866263766652,-19.2447051536475,
124.611508315712)) ;
#44784=CARTESIAN_POINT('Ctrl Pts',(-19.2559540582378,-19.0647160732846,
124.91143051181)) ;
#44785=CARTESIAN_POINT('Ctrl Pts',(-19.4937950988768,-19.25455983764,124.614789826941)) ;
#44786=CARTESIAN_POINT('Ctrl Pts',(-19.5149158429124,-19.0745707572771,
124.915534595951)) ;
#44787=CARTESIAN_POINT('Ctrl Pts',(-19.7013848668796,-19.2645593216878,
124.581864338488)) ;
#44788=CARTESIAN_POINT('Ctrl Pts',(-19.774403515448,-19.0845702413249,124.874379795706)) ;
#44789=CARTESIAN_POINT('Ctrl Pts',(-19.8981684622734,-19.2744544104647,
124.514296465217)) ;
#44790=CARTESIAN_POINT('Ctrl Pts',(-20.0203843648563,-19.0944653301018,
124.789921645643)) ;
#44791=CARTESIAN_POINT('Ctrl Pts',(-20.0832105036019,-19.2845149651109,
124.411914232186)) ;
#44792=CARTESIAN_POINT('Ctrl Pts',(-20.2516876994953,-19.104525884748,124.66194576436)) ;
#44793=CARTESIAN_POINT('Ctrl Pts',(-20.2443173608154,-19.2943642294838,
124.281814272574)) ;
#44794=CARTESIAN_POINT('Ctrl Pts',(-20.4530733453116,-19.1143751491209,
124.499321729623)) ;
#44795=CARTESIAN_POINT('Ctrl Pts',(-20.383234603429,-19.3043914819316,124.123263298254)) ;
#44796=CARTESIAN_POINT('Ctrl Pts',(-20.6267212720183,-19.1244024015687,
124.301134264892)) ;
#44797=CARTESIAN_POINT('Ctrl Pts',(-20.4920569293237,-19.3144197795018,
123.942681895053)) ;
#44798=CARTESIAN_POINT('Ctrl Pts',(-20.7627508777503,-19.1344306991389,
124.075408616383)) ;
#44799=CARTESIAN_POINT('Ctrl Pts',(-20.5668588209695,-19.3242659085078,
123.749683017547)) ;
#44800=CARTESIAN_POINT('Ctrl Pts',(-20.8562554221649,-19.1442768281449,
123.834159661665)) ;
#44801=CARTESIAN_POINT('Ctrl Pts',(-20.608133965986,-19.3342598138698,123.543674588756)) ;
#44802=CARTESIAN_POINT('Ctrl Pts',(-20.9078510940648,-19.154270733507,123.576649296537)) ;
#44803=CARTESIAN_POINT('Ctrl Pts',(-20.6126495317417,-19.3442839115529,
123.332979210101)) ;
#44804=CARTESIAN_POINT('Ctrl Pts',(-20.9134974107354,-19.16429483119,123.313280162661)) ;
#44805=CARTESIAN_POINT('Ctrl Pts',(-20.5812020044249,-19.3541737394069,
123.127452597675)) ;
#44806=CARTESIAN_POINT('Ctrl Pts',(-20.8741896282484,-19.174184659044,123.056370784505)) ;
#44807=CARTESIAN_POINT('Ctrl Pts',(-20.5141513741435,-19.3641657208373,
122.928386984327)) ;
#44808=CARTESIAN_POINT('Ctrl Pts',(-20.7903778747057,-19.1841766404745,
122.807538053505)) ;
#44809=CARTESIAN_POINT('Ctrl Pts',(-20.4139600151984,-19.3741127256032,
122.744833669231)) ;
#44810=CARTESIAN_POINT('Ctrl Pts',(-20.665139925686,-19.1941236452403,122.578095153288)) ;
#44811=CARTESIAN_POINT('Ctrl Pts',(-20.2836802509689,-19.384062376993,122.581175213375)) ;
#44812=CARTESIAN_POINT('Ctrl Pts',(-20.5022911487532,-19.2040732966301,
122.373520731289)) ;
#44813=CARTESIAN_POINT('Ctrl Pts',(-20.1254838491908,-19.3940993799704,
122.441545872889)) ;
#44814=CARTESIAN_POINT('Ctrl Pts',(-20.3045468222314,-19.2141102996075,
122.198982921485)) ;
#44815=CARTESIAN_POINT('Ctrl Pts',(-19.9481679622584,-19.4039882884054,
122.332997305238)) ;
#44816=CARTESIAN_POINT('Ctrl Pts',(-20.0829020053588,-19.2239992080425,
122.063295386373)) ;
#44817=CARTESIAN_POINT('Ctrl Pts',(-19.7528840797197,-19.4139776208829,
122.255763547514)) ;
#44818=CARTESIAN_POINT('Ctrl Pts',(-19.8387974857453,-19.23398854052,121.96675176185)) ;
#44819=CARTESIAN_POINT('Ctrl Pts',(-19.5477596783419,-19.42393617632,122.213894358969)) ;
#44820=CARTESIAN_POINT('Ctrl Pts',(-19.5823918613755,-19.2439470959571,
121.91441371455)) ;
#44821=CARTESIAN_POINT('Ctrl Pts',(-19.339716261487,-19.4338357475205,122.20779695739)) ;
#44822=CARTESIAN_POINT('Ctrl Pts',(-19.3223367513905,-19.2538466671576,
121.906790613366)) ;
#44823=CARTESIAN_POINT('Ctrl Pts',(-19.1307330189891,-19.4438836727725,
122.238435863334)) ;
#44824=CARTESIAN_POINT('Ctrl Pts',(-19.0611077173987,-19.2638945924096,
121.945087876798)) ;
#44825=CARTESIAN_POINT('Ctrl Pts',(-18.9331863686477,-19.4537789722985,
122.303747134582)) ;
#44826=CARTESIAN_POINT('Ctrl Pts',(-18.814173133126,-19.2737898919356,122.026726025059)) ;
#44827=CARTESIAN_POINT('Ctrl Pts',(-18.7469349813943,-19.4638408287464,
122.403975883156)) ;
#44828=CARTESIAN_POINT('Ctrl Pts',(-18.5813585770366,-19.2838517483836,
122.152010675439)) ;
#44829=CARTESIAN_POINT('Ctrl Pts',(-18.5844603918164,-19.4736846751631,
122.532169779838)) ;
#44830=CARTESIAN_POINT('Ctrl Pts',(-18.3782635159342,-19.2936955948002,
122.312252866463)) ;
#44831=CARTESIAN_POINT('Ctrl Pts',(-18.444520656928,-19.4836476242911,122.687999610544)) ;
#44832=CARTESIAN_POINT('Ctrl Pts',(-18.203337799749,-19.3036585439283,122.507039819624)) ;
#44833=CARTESIAN_POINT('Ctrl Pts',(-18.3332595420171,-19.4936816607191,
122.867226494345)) ;
#44834=CARTESIAN_POINT('Ctrl Pts',(-18.0642605165968,-19.3136925803563,
122.731072713085)) ;
#44835=CARTESIAN_POINT('Ctrl Pts',(-18.2557552508508,-19.5035690876772,
123.060098414967)) ;
#44836=CARTESIAN_POINT('Ctrl Pts',(-17.9673787966871,-19.3235800073143,
122.972163161456)) ;
#44837=CARTESIAN_POINT('Ctrl Pts',(-18.2119716822401,-19.5135835220135,
123.266045020976)) ;
#44838=CARTESIAN_POINT('Ctrl Pts',(-17.9126484521056,-19.3335944416507,
123.229596243496)) ;
#44839=CARTESIAN_POINT('Ctrl Pts',(-18.2051271781336,-19.5236184666485,
123.476886047581)) ;
#44840=CARTESIAN_POINT('Ctrl Pts',(-17.9040917216401,-19.3436293862856,
123.493147352358)) ;
#44841=CARTESIAN_POINT('Ctrl Pts',(-18.2338373099495,-19.5334508166795,
123.681614438135)) ;
#44842=CARTESIAN_POINT('Ctrl Pts',(-17.9399787131204,-19.3534617363166,
123.749059430674)) ;
#44843=CARTESIAN_POINT('Ctrl Pts',(-18.2991584830252,-19.5435262557967,
123.883066110455)) ;
#44844=CARTESIAN_POINT('Ctrl Pts',(-18.0216292180747,-19.3635371754338,
124.000873856143)) ;
#44845=CARTESIAN_POINT('Ctrl Pts',(-18.3962015107462,-19.5533787210313,
124.066105872207)) ;
#44846=CARTESIAN_POINT('Ctrl Pts',(-18.1429328956799,-19.3733896406684,
124.229675102606)) ;
#44847=CARTESIAN_POINT('Ctrl Pts',(-18.5262180602235,-19.5634515986082,
124.233211940351)) ;
#44848=CARTESIAN_POINT('Ctrl Pts',(-18.3054527184388,-19.3834625182453,
124.438557806816)) ;
#44849=CARTESIAN_POINT('Ctrl Pts',(-18.6797419077355,-19.5732941948007,
124.371972025685)) ;
#44850=CARTESIAN_POINT('Ctrl Pts',(-18.497358063962,-19.3933051144378,124.61200943149)) ;
#44851=CARTESIAN_POINT('Ctrl Pts',(-18.8570829768545,-19.583274578916,124.484089894838)) ;
#44852=CARTESIAN_POINT('Ctrl Pts',(-18.7190343990807,-19.4032854985531,
124.75215735034)) ;
#44853=CARTESIAN_POINT('Ctrl Pts',(-19.0520979345884,-19.5932930595648,
124.563638386236)) ;
#44854=CARTESIAN_POINT('Ctrl Pts',(-18.9628028394866,-19.4133039792019,
124.851593565958)) ;
#44855=CARTESIAN_POINT('Ctrl Pts',(-19.2551201360957,-19.6031763745651,
124.60795747562)) ;
#44856=CARTESIAN_POINT('Ctrl Pts',(-19.2165815610938,-19.4231872942023,
124.906993128951)) ;
#44857=CARTESIAN_POINT('Ctrl Pts',(-19.4665835366487,-19.6132446716556,
124.616412950505)) ;
#44858=CARTESIAN_POINT('Ctrl Pts',(-19.48091038097,-19.4332555912927,124.917562972667)) ;
#44859=CARTESIAN_POINT('Ctrl Pts',(-19.6714432989599,-19.6230747400279,
124.588929074882)) ;
#44860=CARTESIAN_POINT('Ctrl Pts',(-19.7369866664886,-19.443085659665,124.883208337292)) ;
#44861=CARTESIAN_POINT('Ctrl Pts',(-19.8731711829206,-19.6331415324963,
124.525058281319)) ;
#44862=CARTESIAN_POINT('Ctrl Pts',(-19.9891462344239,-19.4531524521334,
124.803370268973)) ;
#44863=CARTESIAN_POINT('Ctrl Pts',(-20.0574611220455,-19.6430308659848,
124.428741148867)) ;
#44864=CARTESIAN_POINT('Ctrl Pts',(-20.2195097660386,-19.4630417856219,
124.682973671205)) ;
#44865=CARTESIAN_POINT('Ctrl Pts',(-20.2242497094466,-19.6530329974009,
124.300749095355)) ;
#44866=CARTESIAN_POINT('Ctrl Pts',(-20.4279957455821,-19.473043917038,124.522983695097)) ;
#44867=CARTESIAN_POINT('Ctrl Pts',(-20.3653190292274,-19.6629568670219,
124.146990412121)) ;
#44868=CARTESIAN_POINT('Ctrl Pts',(-20.6043330327823,-19.482967786659,124.330784900546)) ;
#44869=CARTESIAN_POINT('Ctrl Pts',(-20.4788115638029,-19.6730003825391,
123.968976465865)) ;
#44870=CARTESIAN_POINT('Ctrl Pts',(-20.7461987470963,-19.4930113021762,
124.108267757242)) ;
#44871=CARTESIAN_POINT('Ctrl Pts',(-20.5586220167799,-19.6828825954274,
123.777121275203)) ;
#44872=CARTESIAN_POINT('Ctrl Pts',(-20.8459623353145,-19.5028935150645,
123.868447779189)) ;
#44873=CARTESIAN_POINT('Ctrl Pts',(-20.6047386809469,-19.6929506726468,
123.570583320886)) ;
#44874=CARTESIAN_POINT('Ctrl Pts',(-20.9036081809755,-19.5129615922839,
123.610275746684)) ;
#44875=CARTESIAN_POINT('Ctrl Pts',(-20.6142646304395,-19.702789177381,123.36393271165)) ;
#44876=CARTESIAN_POINT('Ctrl Pts',(-20.9155157124554,-19.5228000970181,
123.351961006778)) ;
#44877=CARTESIAN_POINT('Ctrl Pts',(-20.5874658464836,-19.7128519458104,
123.154111705371)) ;
#44878=CARTESIAN_POINT('Ctrl Pts',(-20.8820171905211,-19.5328628654475,
123.089685129375)) ;
#44879=CARTESIAN_POINT('Ctrl Pts',(-20.5254497535726,-19.7227489390931,
122.955490377615)) ;
#44880=CARTESIAN_POINT('Ctrl Pts',(-20.8044967773862,-19.5427598587302,
122.841407511896)) ;
#44881=CARTESIAN_POINT('Ctrl Pts',(-20.4301860161421,-19.7326801667279,
122.769710863237)) ;
#44882=CARTESIAN_POINT('Ctrl Pts',(-20.6854165300552,-19.552691086365,122.609182603989)) ;
#44883=CARTESIAN_POINT('Ctrl Pts',(-20.3025172159415,-19.74272232537,122.601572700884)) ;
#44884=CARTESIAN_POINT('Ctrl Pts',(-20.5258305091892,-19.5627332450072,
122.399010178353)) ;
#44885=CARTESIAN_POINT('Ctrl Pts',(-20.1500853642892,-19.7526090349011,
122.460258580595)) ;
#44886=CARTESIAN_POINT('Ctrl Pts',(-20.3352897321001,-19.5726199545382,
122.222366967696)) ;
#44887=CARTESIAN_POINT('Ctrl Pts',(-19.973762981087,-19.7626020073297,122.346058634074)) ;
#44888=CARTESIAN_POINT('Ctrl Pts',(-20.1148863727174,-19.5826129269668,
122.079617245507)) ;
#44889=CARTESIAN_POINT('Ctrl Pts',(-19.7811555655468,-19.7725482018663,
122.26467134964)) ;
#44890=CARTESIAN_POINT('Ctrl Pts',(-19.8741264226561,-19.5925591215034,
121.977883229186)) ;
#44891=CARTESIAN_POINT('Ctrl Pts',(-19.577440733495,-19.7824935767178,122.217515204757)) ;
#44892=CARTESIAN_POINT('Ctrl Pts',(-19.6194821905471,-19.6025044963549,
121.918938430882)) ;
#44893=CARTESIAN_POINT('Ctrl Pts',(-19.3663571883107,-19.7925484960777,
122.206654014904)) ;
#44894=CARTESIAN_POINT('Ctrl Pts',(-19.3556280435181,-19.6125594157148,
121.905362356848)) ;
#44895=CARTESIAN_POINT('Ctrl Pts',(-19.1613655130489,-19.8023700155212,
122.231619206292)) ;
#44896=CARTESIAN_POINT('Ctrl Pts',(-19.0993869105069,-19.6223809351583,
121.936569596424)) ;
#44897=CARTESIAN_POINT('Ctrl Pts',(-18.9588961884829,-19.8124357842881,
122.293030078192)) ;
#44898=CARTESIAN_POINT('Ctrl Pts',(-18.8463008166757,-19.6324467039252,
122.013333704317)) ;
#44899=CARTESIAN_POINT('Ctrl Pts',(-18.7732037589491,-19.8223377059431,
122.387203432726)) ;
#44900=CARTESIAN_POINT('Ctrl Pts',(-18.6141847413824,-19.6423486255803,
122.131051371132)) ;
#44901=CARTESIAN_POINT('Ctrl Pts',(-18.6042436666865,-19.8323807647642,
122.513786536381)) ;
#44902=CARTESIAN_POINT('Ctrl Pts',(-18.4029852173609,-19.6523916844013,
122.289280682628)) ;
#44903=CARTESIAN_POINT('Ctrl Pts',(-18.4618641617122,-19.8422867588069,
122.665775366195)) ;
#44904=CARTESIAN_POINT('Ctrl Pts',(-18.2250106932067,-19.662297678444,122.479267826305)) ;
#44905=CARTESIAN_POINT('Ctrl Pts',(-18.347162029579,-19.8522245318887,122.840394738477)) ;
#44906=CARTESIAN_POINT('Ctrl Pts',(-18.0816334128682,-19.6722354515258,
122.697543077663)) ;
#44907=CARTESIAN_POINT('Ctrl Pts',(-18.2638779267283,-19.862264895621,123.034345828099)) ;
#44908=CARTESIAN_POINT('Ctrl Pts',(-17.9775290976188,-19.6822758152581,
122.939982086318)) ;
#44909=CARTESIAN_POINT('Ctrl Pts',(-18.2161158206728,-19.8721522393445,
123.236657619917)) ;
#44910=CARTESIAN_POINT('Ctrl Pts',(-17.9178270664722,-19.6921631589816,
123.192873036797)) ;
#44911=CARTESIAN_POINT('Ctrl Pts',(-18.2037362405876,-19.8821444699132,
123.446346397897)) ;
#44912=CARTESIAN_POINT('Ctrl Pts',(-17.9023535730957,-19.7021553895503,
123.454984271159)) ;
#44913=CARTESIAN_POINT('Ctrl Pts',(-18.2279073020014,-19.8920929976968,
123.65410610834)) ;
#44914=CARTESIAN_POINT('Ctrl Pts',(-17.9325684280021,-19.7121039173339,
123.714684335697)) ;
#44915=CARTESIAN_POINT('Ctrl Pts',(-18.2874238407614,-19.9020297814201,
123.854332451644)) ;
#44916=CARTESIAN_POINT('Ctrl Pts',(-18.0069653213655,-19.7220407010572,
123.964967568088)) ;
#44917=CARTESIAN_POINT('Ctrl Pts',(-18.3810183276697,-19.912012782217,124.042211329903)) ;
#44918=CARTESIAN_POINT('Ctrl Pts',(-18.1239596004005,-19.7320237018542,
124.199815869688)) ;
#44919=CARTESIAN_POINT('Ctrl Pts',(-18.5068566623067,-19.9220566690578,
124.211741307508)) ;
#44920=CARTESIAN_POINT('Ctrl Pts',(-18.2812582377019,-19.7420675886949,
124.411727571249)) ;
#44921=CARTESIAN_POINT('Ctrl Pts',(-18.656625770795,-19.9318846926323,124.354124004755)) ;
#44922=CARTESIAN_POINT('Ctrl Pts',(-18.4684715103472,-19.7518956122695,
124.589706055916)) ;
#44923=CARTESIAN_POINT('Ctrl Pts',(-18.8330935902759,-19.941961940846,124.47126421145)) ;
#44924=CARTESIAN_POINT('Ctrl Pts',(-18.6890566141087,-19.7619728604831,
124.736130030075)) ;
#44925=CARTESIAN_POINT('Ctrl Pts',(-19.0228690100662,-19.9518114961513,
124.55424093318)) ;
#44926=CARTESIAN_POINT('Ctrl Pts',(-18.9262775519246,-19.7718224157884,
124.839850242289)) ;
#44927=CARTESIAN_POINT('Ctrl Pts',(-19.2288113073246,-19.961894204349,124.604205688793)) ;
#44928=CARTESIAN_POINT('Ctrl Pts',(-19.1837052991682,-19.7819051239861,
124.902304787671)) ;
#44929=CARTESIAN_POINT('Ctrl Pts',(-19.434720498365,-19.9717067972754,124.617486778315)) ;
#44930=CARTESIAN_POINT('Ctrl Pts',(-19.4410933758794,-19.7917177169126,
124.918904855256)) ;
#44931=CARTESIAN_POINT('Ctrl Pts',(-19.645072882955,-19.9817739895334,124.594577329218)) ;
#44932=CARTESIAN_POINT('Ctrl Pts',(-19.7040333399795,-19.8017849091705,
124.890266579354)) ;
#44933=CARTESIAN_POINT('Ctrl Pts',(-19.8449282407417,-19.991672818996,124.536378177571)) ;
#44934=CARTESIAN_POINT('Ctrl Pts',(-19.9538529269052,-19.8116837386331,
124.817515981026)) ;
#44935=CARTESIAN_POINT('Ctrl Pts',(-20.0345223013733,-20.0017268101862,
124.443044256288)) ;
#44936=CARTESIAN_POINT('Ctrl Pts',(-20.1908446168851,-19.8217377298233,
124.700847328328)) ;
#44937=CARTESIAN_POINT('Ctrl Pts',(-20.2021184222333,-20.0115985349694,
124.320569621367)) ;
#44938=CARTESIAN_POINT('Ctrl Pts',(-20.4003396792968,-19.8316094546065,
124.547752149574)) ;
#44939=CARTESIAN_POINT('Ctrl Pts',(-20.3487795362929,-20.0216689770996,
124.167933913824)) ;
#44940=CARTESIAN_POINT('Ctrl Pts',(-20.5836646742585,-19.8416798967367,
124.356956666456)) ;
#44941=CARTESIAN_POINT('Ctrl Pts',(-20.4640387398854,-20.0315020555299,
123.996302242053)) ;
#44942=CARTESIAN_POINT('Ctrl Pts',(-20.7277380468266,-19.851512975167,124.142415105616)) ;
#44943=CARTESIAN_POINT('Ctrl Pts',(-20.5499655152487,-20.0415325290313,
123.803739463889)) ;
#44944=CARTESIAN_POINT('Ctrl Pts',(-20.8351448171807,-19.8615434486684,
123.901710971158)) ;
#44945=CARTESIAN_POINT('Ctrl Pts',(-20.6005657766499,-20.0515641283299,
123.59899153)) ;
#44946=CARTESIAN_POINT('Ctrl Pts',(-20.8983935514118,-19.8715750479671,
123.645775745948)) ;
#44947=CARTESIAN_POINT('Ctrl Pts',(-20.6149874000634,-20.0613938293681,
123.392858537114)) ;
#44948=CARTESIAN_POINT('Ctrl Pts',(-20.9164189115037,-19.8814047490052,
123.388108112838)) ;
#44949=CARTESIAN_POINT('Ctrl Pts',(-20.593669608918,-20.0713832674246,123.183927476953)) ;
#44950=CARTESIAN_POINT('Ctrl Pts',(-20.889769707107,-19.8913941870617,123.126944309975)) ;
#44951=CARTESIAN_POINT('Ctrl Pts',(-20.5355721040913,-20.0814271706407,
122.980925519128)) ;
#44952=CARTESIAN_POINT('Ctrl Pts',(-20.817146145048,-19.9014380902778,122.873192498264)) ;
#44953=CARTESIAN_POINT('Ctrl Pts',(-20.445542899385,-20.0912486914542,122.795106271871)) ;
#44954=CARTESIAN_POINT('Ctrl Pts',(-20.7046073617645,-19.9112596110913,
122.640918152662)) ;
#44955=CARTESIAN_POINT('Ctrl Pts',(-20.3223921732371,-20.1012844157013,
122.623800659788)) ;
#44956=CARTESIAN_POINT('Ctrl Pts',(-20.5506673334166,-19.9212953353384,
122.426787436432)) ;
#44957=CARTESIAN_POINT('Ctrl Pts',(-20.1711768869751,-20.1113065696338,
122.477056253106)) ;
#44958=CARTESIAN_POINT('Ctrl Pts',(-20.3616469061169,-19.9313174892709,
122.243358309574)) ;
#44959=CARTESIAN_POINT('Ctrl Pts',(-19.9997783644996,-20.1211688013911,
122.360421499363)) ;
#44960=CARTESIAN_POINT('Ctrl Pts',(-20.1473968172802,-19.9411797210282,
122.097565987472)) ;
#44961=CARTESIAN_POINT('Ctrl Pts',(-19.8090973942944,-20.131127871849,122.273937081549)) ;
#44962=CARTESIAN_POINT('Ctrl Pts',(-19.9090443945828,-19.9511387914861,
121.989462309799)) ;
#44963=CARTESIAN_POINT('Ctrl Pts',(-19.6046796800119,-20.1411630442251,
122.221797594559)) ;
#44964=CARTESIAN_POINT('Ctrl Pts',(-19.653521817539,-19.9611739638623,121.924289992094)) ;
#44965=CARTESIAN_POINT('Ctrl Pts',(-19.3975520285983,-20.1510434293834,
122.205875090006)) ;
#44966=CARTESIAN_POINT('Ctrl Pts',(-19.3946113132475,-19.9710543490205,
121.904388967509)) ;
#44967=CARTESIAN_POINT('Ctrl Pts',(-19.1871508596279,-20.1611001439773,
122.226434671735)) ;
#44968=CARTESIAN_POINT('Ctrl Pts',(-19.1316102592397,-19.9811110636145,
121.930090607281)) ;
#44969=CARTESIAN_POINT('Ctrl Pts',(-18.9870826370418,-20.1709794125494,
122.28223552978)) ;
#44970=CARTESIAN_POINT('Ctrl Pts',(-18.8815248170591,-19.9909903321865,
121.999843996043)) ;
#44971=CARTESIAN_POINT('Ctrl Pts',(-18.7973905879869,-20.1809703700351,
122.372426720586)) ;
#44972=CARTESIAN_POINT('Ctrl Pts',(-18.6444106249268,-20.0009812896722,
122.112585153845)) ;
#44973=CARTESIAN_POINT('Ctrl Pts',(-18.6256580137942,-20.1910110286703,
122.495170942343)) ;
#44974=CARTESIAN_POINT('Ctrl Pts',(-18.4297462676032,-20.0110219483074,
122.266017180346)) ;
#44975=CARTESIAN_POINT('Ctrl Pts',(-18.4806610276397,-20.2008440083783,
122.642504839744)) ;
#44976=CARTESIAN_POINT('Ctrl Pts',(-18.2485010034738,-20.0208549280154,
122.450186849546)) ;
#44977=CARTESIAN_POINT('Ctrl Pts',(-18.3610435893545,-20.210837141628,122.81520973265)) ;
#44978=CARTESIAN_POINT('Ctrl Pts',(-18.0989811418267,-20.0308480612651,
122.666069459646)) ;
#44979=CARTESIAN_POINT('Ctrl Pts',(-18.2732819316886,-20.2208691940113,
123.00699894088)) ;
#44980=CARTESIAN_POINT('Ctrl Pts',(-17.9892812124725,-20.0408801136485,
122.905806909259)) ;
#44981=CARTESIAN_POINT('Ctrl Pts',(-18.2207950634058,-20.2307344229627,
123.207634736704)) ;
#44982=CARTESIAN_POINT('Ctrl Pts',(-17.9236747635864,-20.0507453425998,
123.15660297018)) ;
#44983=CARTESIAN_POINT('Ctrl Pts',(-18.2031854904533,-20.2406963642059,
123.416330007382)) ;
#44984=CARTESIAN_POINT('Ctrl Pts',(-17.9016652917606,-20.060707283843,123.417472522822)) ;
#44985=CARTESIAN_POINT('Ctrl Pts',(-18.2225552242185,-20.2507310792426,
123.626390528993)) ;
#44986=CARTESIAN_POINT('Ctrl Pts',(-17.9258798988399,-20.0707419988798,
123.680047914976)) ;
#44987=CARTESIAN_POINT('Ctrl Pts',(-18.2769648586683,-20.2606168495867,
123.826997944236)) ;
#44988=CARTESIAN_POINT('Ctrl Pts',(-17.9938945221677,-20.0806277692238,
123.930807070481)) ;
#44989=CARTESIAN_POINT('Ctrl Pts',(-18.3669425663381,-20.2706794469754,
124.018428595502)) ;
#44990=CARTESIAN_POINT('Ctrl Pts',(-18.1063688771636,-20.0906903666126,
124.17009418255)) ;
#44991=CARTESIAN_POINT('Ctrl Pts',(-18.4861705032572,-20.2805298588107,
124.187769337836)) ;
#44992=CARTESIAN_POINT('Ctrl Pts',(-18.2554062654784,-20.1005407784478,
124.381769206372)) ;
#44993=CARTESIAN_POINT('Ctrl Pts',(-18.6352264586599,-20.2905570280966,
124.336825287887)) ;
#44994=CARTESIAN_POINT('Ctrl Pts',(-18.4417280629167,-20.1105679477337,
124.568087270912)) ;
#44995=CARTESIAN_POINT('Ctrl Pts',(-18.8082335054071,-20.3005845088108,
124.457297088272)) ;
#44996=CARTESIAN_POINT('Ctrl Pts',(-18.6579883240975,-20.1205954284479,
124.71867494309)) ;
#44997=CARTESIAN_POINT('Ctrl Pts',(-18.9958279314293,-20.3104275613901,
124.544623627874)) ;
#44998=CARTESIAN_POINT('Ctrl Pts',(-18.8924830333248,-20.1304384810272,
124.827831022184)) ;
#44999=CARTESIAN_POINT('Ctrl Pts',(-19.19866746115,-20.3204214648287,124.599389527813)) ;
#45000=CARTESIAN_POINT('Ctrl Pts',(-19.1460332396166,-20.1404323844658,
124.896285825858)) ;
#45001=CARTESIAN_POINT('Ctrl Pts',(-19.4086704937467,-20.3304485876051,
124.617780480722)) ;
#45002=CARTESIAN_POINT('Ctrl Pts',(-19.408537282864,-20.1504595072422,124.919271899717)) ;
#45003=CARTESIAN_POINT('Ctrl Pts',(-19.6158404873169,-20.3403392924971,
124.599938377875)) ;
#45004=CARTESIAN_POINT('Ctrl Pts',(-19.6674999586504,-20.1603502121343,
124.896966576094)) ;
#45005=CARTESIAN_POINT('Ctrl Pts',(-19.8188925643533,-20.3503313193475,
124.546143797245)) ;
#45006=CARTESIAN_POINT('Ctrl Pts',(-19.9213144643627,-20.1703422389846,
124.829720703187)) ;
#45007=CARTESIAN_POINT('Ctrl Pts',(-20.0086203150577,-20.360277300836,124.458257930678)) ;
#45008=CARTESIAN_POINT('Ctrl Pts',(-20.158473228304,-20.1802882204731,124.719860821045)) ;
#45009=CARTESIAN_POINT('Ctrl Pts',(-20.1804782509526,-20.3702244734579,
124.339088999519)) ;
#45010=CARTESIAN_POINT('Ctrl Pts',(-20.3732942470927,-20.190235393095,124.570897282398)) ;
#45011=CARTESIAN_POINT('Ctrl Pts',(-20.3303594599015,-20.3802724147841,
124.190244480905)) ;
#45012=CARTESIAN_POINT('Ctrl Pts',(-20.5606438303885,-20.2002833344212,
124.384839709342)) ;
#45013=CARTESIAN_POINT('Ctrl Pts',(-20.4498405364493,-20.3901200485918,
124.021171300404)) ;
#45014=CARTESIAN_POINT('Ctrl Pts',(-20.7099931677264,-20.210130968229,124.17349632098)) ;
#45015=CARTESIAN_POINT('Ctrl Pts',(-20.5397614536319,-20.4000817632769,
123.832042454196)) ;
#45016=CARTESIAN_POINT('Ctrl Pts',(-20.8223918370586,-20.220092682914,123.937083946774)) ;
#45017=CARTESIAN_POINT('Ctrl Pts',(-20.5955998308358,-20.4101103961554,
123.628724338267)) ;
#45018=CARTESIAN_POINT('Ctrl Pts',(-20.8921871412405,-20.2301213157925,
123.682935524378)) ;
#45019=CARTESIAN_POINT('Ctrl Pts',(-20.6151216491279,-20.4200207216905,
123.421303306592)) ;
#45020=CARTESIAN_POINT('Ctrl Pts',(-20.9165866653184,-20.2400316413277,
123.423658765384)) ;
#45021=CARTESIAN_POINT('Ctrl Pts',(-20.5988309906371,-20.4299555521623,
123.213073747542)) ;
#45022=CARTESIAN_POINT('Ctrl Pts',(-20.8962205046669,-20.2499664717994,
123.163371888268)) ;
#45023=CARTESIAN_POINT('Ctrl Pts',(-20.5458999153234,-20.4399968845442,
123.008717300108)) ;
#45024=CARTESIAN_POINT('Ctrl Pts',(-20.8300540056933,-20.2600078041814,
122.907927043714)) ;
#45025=CARTESIAN_POINT('Ctrl Pts',(-20.4596544020495,-20.4498897579831,
122.819465298956)) ;
#45026=CARTESIAN_POINT('Ctrl Pts',(-20.7222442141385,-20.2699006776202,
122.671362855132)) ;
#45027=CARTESIAN_POINT('Ctrl Pts',(-20.3413828244053,-20.459858923801,122.646430648159)) ;
#45028=CARTESIAN_POINT('Ctrl Pts',(-20.574403392537,-20.2798698434381,122.45507183945)) ;
#45029=CARTESIAN_POINT('Ctrl Pts',(-20.1937587502541,-20.4698876575175,
122.49593053107)) ;
#45030=CARTESIAN_POINT('Ctrl Pts',(-20.389867415721,-20.2898985771546,122.266945763663)) ;
#45031=CARTESIAN_POINT('Ctrl Pts',(-19.9684033928012,-20.4830801762886,
122.334134273859)) ;
#45032=CARTESIAN_POINT('Ctrl Pts',(-20.108189935514,-20.3030910959258,122.064717611353)) ;
#45033=CARTESIAN_POINT('Ctrl Pts',(-19.7027899632007,-20.4964400443313,
122.233638145416)) ;
#45034=CARTESIAN_POINT('Ctrl Pts',(-19.776200429425,-20.3164509639684,121.939098030054)) ;
#45035=CARTESIAN_POINT('Ctrl Pts',(-19.4261080021341,-20.5096653814802,
122.206033322011)) ;
#45036=CARTESIAN_POINT('Ctrl Pts',(-19.4302944299176,-20.3296763011173,
121.904585070859)) ;
#45037=CARTESIAN_POINT('Ctrl Pts',(-19.2168158322053,-20.5196466073208,
122.221163224534)) ;
#45038=CARTESIAN_POINT('Ctrl Pts',(-19.1686900557449,-20.3396575269579,
121.923502397448)) ;
#45039=CARTESIAN_POINT('Ctrl Pts',(-19.0123335437991,-20.5296821743037,
122.273082359298)) ;
#45040=CARTESIAN_POINT('Ctrl Pts',(-18.9130849261984,-20.3496930939408,
121.988403504327)) ;
#45041=CARTESIAN_POINT('Ctrl Pts',(-18.8230767712462,-20.5395452522658,
122.357856292057)) ;
#45042=CARTESIAN_POINT('Ctrl Pts',(-18.6765159440695,-20.3595561719029,
122.094373600289)) ;
#45043=CARTESIAN_POINT('Ctrl Pts',(-18.6478204664462,-20.5496155510669,
122.476584772983)) ;
#45044=CARTESIAN_POINT('Ctrl Pts',(-18.4574468061617,-20.369626470704,122.2427865665)) ;
#45045=CARTESIAN_POINT('Ctrl Pts',(-18.4992676427898,-20.5594578496347,
122.620634851231)) ;
#45046=CARTESIAN_POINT('Ctrl Pts',(-18.2717579005638,-20.3794687692718,
122.422851075719)) ;
#45047=CARTESIAN_POINT('Ctrl Pts',(-18.3759064700005,-20.5694185478045,
122.789841274378)) ;
#45048=CARTESIAN_POINT('Ctrl Pts',(-18.1175586647282,-20.3894294674416,
122.634360678073)) ;
#45049=CARTESIAN_POINT('Ctrl Pts',(-18.283462315847,-20.579456581984,122.979538516165)) ;
#45050=CARTESIAN_POINT('Ctrl Pts',(-18.0020059072157,-20.3994675016211,
122.871483585782)) ;
#45051=CARTESIAN_POINT('Ctrl Pts',(-18.2259264092377,-20.5893303188304,
123.179010973159)) ;
#45052=CARTESIAN_POINT('Ctrl Pts',(-17.9300887193781,-20.4093412384676,
123.12082468391)) ;
#45053=CARTESIAN_POINT('Ctrl Pts',(-18.203489149074,-20.5994021027557,123.389529384903)) ;
#45054=CARTESIAN_POINT('Ctrl Pts',(-17.9020448474058,-20.4194130223928,
123.383973224126)) ;
#45055=CARTESIAN_POINT('Ctrl Pts',(-18.217479141793,-20.6092342239569,123.595777992507)) ;
#45056=CARTESIAN_POINT('Ctrl Pts',(-17.9195350319781,-20.429245143594,123.641783391188)) ;
#45057=CARTESIAN_POINT('Ctrl Pts',(-18.2675235725742,-20.6192672479823,
123.800670607276)) ;
#45058=CARTESIAN_POINT('Ctrl Pts',(-17.9820931576725,-20.4392781676194,
123.897898640785)) ;
#45059=CARTESIAN_POINT('Ctrl Pts',(-18.3527418081313,-20.629283128179,123.993235721321)) ;
#45060=CARTESIAN_POINT('Ctrl Pts',(-18.0886185614509,-20.4492940478161,
124.138604141846)) ;
#45061=CARTESIAN_POINT('Ctrl Pts',(-18.4682220622006,-20.6391666472732,
124.165972783851)) ;
#45062=CARTESIAN_POINT('Ctrl Pts',(-18.2329706508674,-20.4591775669103,
124.354523331879)) ;
#45063=CARTESIAN_POINT('Ctrl Pts',(-18.6132891948029,-20.6491570596368,
124.317833664429)) ;
#45064=CARTESIAN_POINT('Ctrl Pts',(-18.4143074091382,-20.469167979274,124.54434899152)) ;
#45065=CARTESIAN_POINT('Ctrl Pts',(-18.8379391592786,-20.6624202228403,
124.483045377824)) ;
#45066=CARTESIAN_POINT('Ctrl Pts',(-18.6951170310066,-20.4824311424774,
124.750853866765)) ;
#45067=CARTESIAN_POINT('Ctrl Pts',(-19.1007465541756,-20.6756977930915,
124.586193595685)) ;
#45068=CARTESIAN_POINT('Ctrl Pts',(-19.0235816254603,-20.4957087127286,
124.879780338446)) ;
#45069=CARTESIAN_POINT('Ctrl Pts',(-19.3792304841943,-20.6890280955981,
124.617392370144)) ;
#45070=CARTESIAN_POINT('Ctrl Pts',(-19.3717460245778,-20.5090390152352,
124.918788838269)) ;
#45071=CARTESIAN_POINT('Ctrl Pts',(-19.5869463660609,-20.6989267774145,
124.604614305006)) ;
#45072=CARTESIAN_POINT('Ctrl Pts',(-19.631378352144,-20.5189376970516,124.902811153565)) ;
#45073=CARTESIAN_POINT('Ctrl Pts',(-19.7911870424571,-20.708916292462,124.555761796128)) ;
#45074=CARTESIAN_POINT('Ctrl Pts',(-19.886681931356,-20.5289272120991,124.841743662503)) ;
#45075=CARTESIAN_POINT('Ctrl Pts',(-19.9830582667155,-20.718864344237,124.472519591824)) ;
#45076=CARTESIAN_POINT('Ctrl Pts',(-20.1265183759964,-20.5388752638742,
124.737689396078)) ;
#45077=CARTESIAN_POINT('Ctrl Pts',(-20.1575675432332,-20.7288057475155,
124.357539674552)) ;
#45078=CARTESIAN_POINT('Ctrl Pts',(-20.3446556457236,-20.5488166671527,
124.593959705977)) ;
#45079=CARTESIAN_POINT('Ctrl Pts',(-20.3608485699155,-20.7420924122965,
124.165903707027)) ;
#45080=CARTESIAN_POINT('Ctrl Pts',(-20.5987445476078,-20.5621033319336,
124.354427857962)) ;
#45081=CARTESIAN_POINT('Ctrl Pts',(-20.5464483543658,-20.7587028339513,
123.865472903908)) ;
#45082=CARTESIAN_POINT('Ctrl Pts',(-20.8307521720102,-20.5787137535884,
123.97887050718)) ;
#45083=CARTESIAN_POINT('Ctrl Pts',(-20.6330141955444,-20.7786140962021,
123.451029395144)) ;
#45084=CARTESIAN_POINT('Ctrl Pts',(-20.9389514260489,-20.5986250158392,
123.460821316337)) ;
#45085=CARTESIAN_POINT('Ctrl Pts',(-20.5730157601791,-20.7985582253669,
123.03120703151)) ;
#45086=CARTESIAN_POINT('Ctrl Pts',(-20.8639502681966,-20.6185691450041,
122.93604284961)) ;
#45087=CARTESIAN_POINT('Ctrl Pts',(-20.3735473898492,-20.8184813879721,
122.657531564048)) ;
#45088=CARTESIAN_POINT('Ctrl Pts',(-20.614611211859,-20.6384923076093,122.468951374548)) ;
#45089=CARTESIAN_POINT('Ctrl Pts',(-20.0594536899428,-20.8383715103787,
122.374229560323)) ;
#45090=CARTESIAN_POINT('Ctrl Pts',(-20.2219924331107,-20.6583824300158,
122.114827126927)) ;
#45091=CARTESIAN_POINT('Ctrl Pts',(-19.6652757918242,-20.8583764639788,
122.21454943932)) ;
#45092=CARTESIAN_POINT('Ctrl Pts',(-19.7292685932625,-20.6783873836159,
121.915230361568)) ;
#45093=CARTESIAN_POINT('Ctrl Pts',(-19.2436756516205,-20.8782147209944,
122.198755207655)) ;
#45094=CARTESIAN_POINT('Ctrl Pts',(-19.2022698837694,-20.6982256406315,
121.895490958203)) ;
#45095=CARTESIAN_POINT('Ctrl Pts',(-18.8388276678669,-20.8982090217809,
122.328339296805)) ;
#45096=CARTESIAN_POINT('Ctrl Pts',(-18.6962108824023,-20.718219941418,122.057473862947)) ;
#45097=CARTESIAN_POINT('Ctrl Pts',(-18.5045195812377,-20.9180942638254,
122.587219380678)) ;
#45098=CARTESIAN_POINT('Ctrl Pts',(-18.2783285952611,-20.7381051834625,
122.381075560874)) ;
#45099=CARTESIAN_POINT('Ctrl Pts',(-18.2777383338491,-20.9379692103013,
122.943809989293)) ;
#45100=CARTESIAN_POINT('Ctrl Pts',(-17.994854669319,-20.7579801299384,122.826813664133)) ;
#45101=CARTESIAN_POINT('Ctrl Pts',(-18.1858465710656,-20.9580022802424,
123.359778806522)) ;
#45102=CARTESIAN_POINT('Ctrl Pts',(-17.8799919148202,-20.7780131998795,
123.346775629798)) ;
#45103=CARTESIAN_POINT('Ctrl Pts',(-18.2415322925881,-20.9778907871428,
123.778943620506)) ;
#45104=CARTESIAN_POINT('Ctrl Pts',(-17.9496011378404,-20.7979017067799,
123.870729922687)) ;
#45105=CARTESIAN_POINT('Ctrl Pts',(-18.4353283530407,-20.9977456469241,
124.154075261847)) ;
#45106=CARTESIAN_POINT('Ctrl Pts',(-18.1918462219095,-20.8177565665612,
124.3396421318)) ;
#45107=CARTESIAN_POINT('Ctrl Pts',(-18.7489158886705,-21.0177964807118,
124.442758777326)) ;
#45108=CARTESIAN_POINT('Ctrl Pts',(-18.5838321068267,-20.8378074003489,
124.700496054133)) ;
#45109=CARTESIAN_POINT('Ctrl Pts',(-19.136624015985,-21.037562422601,124.605282240514)) ;
#45110=CARTESIAN_POINT('Ctrl Pts',(-19.068464276831,-20.8575733422382,124.903648311882)) ;
#45111=CARTESIAN_POINT('Ctrl Pts',(-19.5614777516072,-21.0575751540604,
124.626836375853)) ;
#45112=CARTESIAN_POINT('Ctrl Pts',(-19.5995315082648,-20.8775860736975,
124.930591112169)) ;
#45113=CARTESIAN_POINT('Ctrl Pts',(-19.9658070655714,-21.0774679890039,
124.50224819763)) ;
#45114=CARTESIAN_POINT('Ctrl Pts',(-20.1049415619315,-20.8974789086411,
124.774856355301)) ;
#45115=CARTESIAN_POINT('Ctrl Pts',(-20.3038411949213,-21.0973750123435,
124.247672615778)) ;
#45116=CARTESIAN_POINT('Ctrl Pts',(-20.5274834956155,-20.9173859319806,
124.456638371314)) ;
#45117=CARTESIAN_POINT('Ctrl Pts',(-20.5353184672274,-21.1172902772442,
123.892968169314)) ;
#45118=CARTESIAN_POINT('Ctrl Pts',(-20.816830578431,-20.9373011968813,124.013259477076)) ;
#45119=CARTESIAN_POINT('Ctrl Pts',(-20.6318648780347,-21.1373219694039,
123.478162570319)) ;
#45120=CARTESIAN_POINT('Ctrl Pts',(-20.9375148304315,-20.957332889041,123.494752291647)) ;
#45121=CARTESIAN_POINT('Ctrl Pts',(-20.5815599947794,-21.1571650159769,
123.059210144883)) ;
#45122=CARTESIAN_POINT('Ctrl Pts',(-20.8746353856575,-20.977175935614,122.971063764451)) ;
#45123=CARTESIAN_POINT('Ctrl Pts',(-20.3915208487305,-21.1770815638767,
122.680835228278)) ;
#45124=CARTESIAN_POINT('Ctrl Pts',(-20.6370889547164,-20.9970924835138,
122.498095047724)) ;
#45125=CARTESIAN_POINT('Ctrl Pts',(-20.083403861949,-21.197013806868,122.389779528303)) ;
#45126=CARTESIAN_POINT('Ctrl Pts',(-20.2519449229263,-21.0170247265051,
122.134274226715)) ;
#45127=CARTESIAN_POINT('Ctrl Pts',(-19.69516019848,-21.2169176416773,122.221394595349)) ;
#45128=CARTESIAN_POINT('Ctrl Pts',(-19.7666424548644,-21.0369285613144,
121.923791010191)) ;
#45129=CARTESIAN_POINT('Ctrl Pts',(-19.2728466795046,-21.2368180418648,
122.195076901029)) ;
#45130=CARTESIAN_POINT('Ctrl Pts',(-19.2387517746297,-21.0568289615019,
121.890890792397)) ;
#45131=CARTESIAN_POINT('Ctrl Pts',(-18.8658292690085,-21.2567677182441,
122.314583734304)) ;
#45132=CARTESIAN_POINT('Ctrl Pts',(-18.7299794806847,-21.0767786378812,
122.040270945825)) ;
#45133=CARTESIAN_POINT('Ctrl Pts',(-18.5243803368553,-21.2767002424645,
122.565662246867)) ;
#45134=CARTESIAN_POINT('Ctrl Pts',(-18.303166710287,-21.0967111621016,122.354115893689)) ;
#45135=CARTESIAN_POINT('Ctrl Pts',(-18.288939857507,-21.2966202514507,122.917786612455)) ;
#45136=CARTESIAN_POINT('Ctrl Pts',(-18.0088633209534,-21.1166311710878,
122.794268679534)) ;
#45137=CARTESIAN_POINT('Ctrl Pts',(-18.1876872131217,-21.3165771576268,
123.329823315717)) ;
#45138=CARTESIAN_POINT('Ctrl Pts',(-17.8822937308164,-21.136588077264,123.309313272766)) ;
#45139=CARTESIAN_POINT('Ctrl Pts',(-18.2325869540117,-21.3364629971283,
123.750340197414)) ;
#45140=CARTESIAN_POINT('Ctrl Pts',(-17.9384143246764,-21.1564739167655,
123.834958994811)) ;
#45141=CARTESIAN_POINT('Ctrl Pts',(-18.4190587415346,-21.3564341692642,
124.131743478507)) ;
#45142=CARTESIAN_POINT('Ctrl Pts',(-18.1714993859742,-21.1764450889013,
124.31171484266)) ;
#45143=CARTESIAN_POINT('Ctrl Pts',(-18.721795903564,-21.3762483662486,124.42483382689)) ;
#45144=CARTESIAN_POINT('Ctrl Pts',(-18.5499193847217,-21.1962592858857,
124.678080171936)) ;
#45145=CARTESIAN_POINT('Ctrl Pts',(-19.109257994725,-21.3962295522168,124.59893775336)) ;
#45146=CARTESIAN_POINT('Ctrl Pts',(-19.0342352621923,-21.2162404718539,
124.89571496393)) ;
#45147=CARTESIAN_POINT('Ctrl Pts',(-19.460775786385,-21.4128050576061,124.624819419925)) ;
#45148=CARTESIAN_POINT('Ctrl Pts',(-19.4736619237772,-21.2328159772432,
124.928069751188)) ;
#45149=CARTESIAN_POINT('Ctrl Pts',(-19.7357438512233,-21.4261145054697,
124.572846707991)) ;
#45150=CARTESIAN_POINT('Ctrl Pts',(-19.8173383619088,-21.2461254251068,
124.863112509641)) ;
#45151=CARTESIAN_POINT('Ctrl Pts',(-19.9985231275647,-21.4394822032463,
124.473349278481)) ;
#45152=CARTESIAN_POINT('Ctrl Pts',(-20.1458733462935,-21.2594931228834,
124.738714343657)) ;
#45153=CARTESIAN_POINT('Ctrl Pts',(-20.2833722213967,-21.4559727749122,
124.268798347122)) ;
#45154=CARTESIAN_POINT('Ctrl Pts',(-20.5018728442166,-21.2759836945493,
124.483060829662)) ;
#45155=CARTESIAN_POINT('Ctrl Pts',(-20.5233223205152,-21.475893047245,123.919846821527)) ;
#45156=CARTESIAN_POINT('Ctrl Pts',(-20.8018337601815,-21.2959039668821,
124.04687473534)) ;
#45157=CARTESIAN_POINT('Ctrl Pts',(-20.6120012444767,-21.492510082966,123.577832825468)) ;
#45158=CARTESIAN_POINT('Ctrl Pts',(-20.9126872837308,-21.3125210026031,
123.619326861712)) ;
#45159=CARTESIAN_POINT('Ctrl Pts',(-20.6099160380865,-21.5058009332471,
123.298380195676)) ;
#45160=CARTESIAN_POINT('Ctrl Pts',(-20.9100801364126,-21.3258118528842,
123.270041130568)) ;
#45161=CARTESIAN_POINT('Ctrl Pts',(-20.5720819647299,-21.5157699784016,
123.092270132128)) ;
#45162=CARTESIAN_POINT('Ctrl Pts',(-20.8627908877047,-21.3357808980387,
123.01239695694)) ;
#45163=CARTESIAN_POINT('Ctrl Pts',(-20.499885467458,-21.5256733690351,122.8969600671)) ;
#45164=CARTESIAN_POINT('Ctrl Pts',(-20.7725483587208,-21.3456842886722,
122.768260657611)) ;
#45165=CARTESIAN_POINT('Ctrl Pts',(-20.3931639686196,-21.5357311551478,
122.714452129114)) ;
#45166=CARTESIAN_POINT('Ctrl Pts',(-20.6391462593297,-21.355742074785,122.540122041422)) ;
#45167=CARTESIAN_POINT('Ctrl Pts',(-20.2592745444822,-21.5455831917976,
122.556386418772)) ;
#45168=CARTESIAN_POINT('Ctrl Pts',(-20.471796281269,-21.3655941114347,122.342544854426)) ;
#45169=CARTESIAN_POINT('Ctrl Pts',(-20.0435430288408,-21.5589483159408,
122.376446565359)) ;
#45170=CARTESIAN_POINT('Ctrl Pts',(-20.202086568455,-21.3789592355779,122.117585029651)) ;
#45171=CARTESIAN_POINT('Ctrl Pts',(-19.7882330766326,-21.5721743789038,
122.25842779773)) ;
#45172=CARTESIAN_POINT('Ctrl Pts',(-19.8829746642869,-21.3921852985409,
121.970083356066)) ;
#45173=CARTESIAN_POINT('Ctrl Pts',(-19.512730849252,-21.5854780271861,122.210256078633)) ;
#45174=CARTESIAN_POINT('Ctrl Pts',(-19.5386166648269,-21.4054889468232,
121.909867161857)) ;
#45175=CARTESIAN_POINT('Ctrl Pts',(-19.3026540676817,-21.5954695583491,
122.210450686566)) ;
#45176=CARTESIAN_POINT('Ctrl Pts',(-19.2760167649195,-21.4154804779862,
121.910107183642)) ;
#45177=CARTESIAN_POINT('Ctrl Pts',(-19.0948968921359,-21.6055090061484,
122.247567522211)) ;
#45178=CARTESIAN_POINT('Ctrl Pts',(-19.0163207496462,-21.4255199257855,
121.956500605478)) ;
#45179=CARTESIAN_POINT('Ctrl Pts',(-18.9004687004283,-21.6153527816622,
122.318496927726)) ;
#45180=CARTESIAN_POINT('Ctrl Pts',(-18.7732843139319,-21.4353637012994,
122.045159677628)) ;
#45181=CARTESIAN_POINT('Ctrl Pts',(-18.7185579083454,-21.6253384230499,
122.423213533386)) ;
#45182=CARTESIAN_POINT('Ctrl Pts',(-18.5458944197202,-21.445349342687,122.176053036341)) ;
#45183=CARTESIAN_POINT('Ctrl Pts',(-18.5582565476501,-21.6352752074117,
122.557220506057)) ;
#45184=CARTESIAN_POINT('Ctrl Pts',(-18.3455158402902,-21.4552861270488,
122.343559635745)) ;
#45185=CARTESIAN_POINT('Ctrl Pts',(-18.4222459587121,-21.645325041879,122.718871713832)) ;
#45186=CARTESIAN_POINT('Ctrl Pts',(-18.1755004123989,-21.4653359615162,
122.545621877111)) ;
#45187=CARTESIAN_POINT('Ctrl Pts',(-18.3183162605906,-21.6551754913822,
122.898008987532)) ;
#45188=CARTESIAN_POINT('Ctrl Pts',(-18.0455857951863,-21.4751864110193,
122.769542152888)) ;
#45189=CARTESIAN_POINT('Ctrl Pts',(-18.2456911500029,-21.6651475053643,
123.09464249712)) ;
#45190=CARTESIAN_POINT('Ctrl Pts',(-17.9548017337126,-21.4851584250014,
123.015333175436)) ;
#45191=CARTESIAN_POINT('Ctrl Pts',(-18.2082412582699,-21.6751426632114,
123.301442369805)) ;
#45192=CARTESIAN_POINT('Ctrl Pts',(-17.9079865989931,-21.4951535828485,
123.273832595304)) ;
#45193=CARTESIAN_POINT('Ctrl Pts',(-18.2075185297832,-21.6851765895751,
123.512368066183)) ;
#45194=CARTESIAN_POINT('Ctrl Pts',(-17.9070803718407,-21.5051875092122,
123.537489745388)) ;
#45195=CARTESIAN_POINT('Ctrl Pts',(-18.2424799085402,-21.6950322980075,
123.716614333339)) ;
#45196=CARTESIAN_POINT('Ctrl Pts',(-17.9507793758627,-21.5150432176446,
123.792798278233)) ;
#45197=CARTESIAN_POINT('Ctrl Pts',(-18.3130824839469,-21.7050304473461,
123.914559389374)) ;
#45198=CARTESIAN_POINT('Ctrl Pts',(-18.0390300008137,-21.5250413669833,
124.040230621142)) ;
#45199=CARTESIAN_POINT('Ctrl Pts',(-18.4158251214299,-21.7149298505197,
124.095582065844)) ;
#45200=CARTESIAN_POINT('Ctrl Pts',(-18.1674560178269,-21.5349407701568,
124.266510551616)) ;
#45201=CARTESIAN_POINT('Ctrl Pts',(-18.5504028728454,-21.7249810474082,
124.258463624392)) ;
#45202=CARTESIAN_POINT('Ctrl Pts',(-18.3356760700349,-21.5449919670453,
124.470114254987)) ;
#45203=CARTESIAN_POINT('Ctrl Pts',(-18.7085246366495,-21.734863371221,124.393249383885)) ;
#45204=CARTESIAN_POINT('Ctrl Pts',(-18.5333267197165,-21.5548742908582,
124.63859875685)) ;
#45205=CARTESIAN_POINT('Ctrl Pts',(-18.8894290935753,-21.7448582668776,
124.500128199222)) ;
#45206=CARTESIAN_POINT('Ctrl Pts',(-18.7594560018533,-21.5648691865148,
124.772199667984)) ;
#45207=CARTESIAN_POINT('Ctrl Pts',(-19.0867831919036,-21.7548793662602,
124.573882631177)) ;
#45208=CARTESIAN_POINT('Ctrl Pts',(-19.0061476935566,-21.5748902858973,
124.864395292257)) ;
#45209=CARTESIAN_POINT('Ctrl Pts',(-19.2915499840716,-21.7647866341222,
124.611973404616)) ;
#45210=CARTESIAN_POINT('Ctrl Pts',(-19.2621059878606,-21.5847975537594,
124.912011501582)) ;
#45211=CARTESIAN_POINT('Ctrl Pts',(-19.5004581738309,-21.7747249779475,
124.614356734753)) ;
#45212=CARTESIAN_POINT('Ctrl Pts',(-19.523241461829,-21.5947358975846,124.914993347183)) ;
#45213=CARTESIAN_POINT('Ctrl Pts',(-19.7080148034449,-21.784728397248,124.580333186118)) ;
#45214=CARTESIAN_POINT('Ctrl Pts',(-19.7826877608653,-21.6047393168851,
124.872466522298)) ;
#45215=CARTESIAN_POINT('Ctrl Pts',(-19.9069801683133,-21.7947629479551,
124.510252770105)) ;
#45216=CARTESIAN_POINT('Ctrl Pts',(-20.0313953526163,-21.6147738675922,
124.784868563439)) ;
#45217=CARTESIAN_POINT('Ctrl Pts',(-20.0874764819987,-21.8046078975607,
124.408942640164)) ;
#45218=CARTESIAN_POINT('Ctrl Pts',(-20.2570175361055,-21.6246188171978,
124.658232944476)) ;
#45219=CARTESIAN_POINT('Ctrl Pts',(-20.2501460126216,-21.8145937396736,
124.276289518342)) ;
#45220=CARTESIAN_POINT('Ctrl Pts',(-20.4603562191612,-21.6346046593107,
124.492418457877)) ;
#45221=CARTESIAN_POINT('Ctrl Pts',(-20.3867706955757,-21.8245285470427,
124.118261781283)) ;
#45222=CARTESIAN_POINT('Ctrl Pts',(-20.6311392301702,-21.6445394666798,
124.294885221514)) ;
#45223=CARTESIAN_POINT('Ctrl Pts',(-20.4950064678875,-21.834586088756,123.936658959793)) ;
#45224=CARTESIAN_POINT('Ctrl Pts',(-20.7664361277187,-21.6545970083931,
124.067883129677)) ;
#45225=CARTESIAN_POINT('Ctrl Pts',(-20.568620634059,-21.8444076862681,123.743721916865)) ;
#45226=CARTESIAN_POINT('Ctrl Pts',(-20.8584564948569,-21.6644186059052,
123.826712005177)) ;
#45227=CARTESIAN_POINT('Ctrl Pts',(-20.6089246273583,-21.8544639457486,
123.53620346997)) ;
#45228=CARTESIAN_POINT('Ctrl Pts',(-20.9088388978743,-21.6744748653857,
123.567314526484)) ;
#45229=CARTESIAN_POINT('Ctrl Pts',(-20.6121758192455,-21.864403882049,123.327248711453)) ;
#45230=CARTESIAN_POINT('Ctrl Pts',(-20.912905442173,-21.6844148016861,123.306120784318)) ;
#45231=CARTESIAN_POINT('Ctrl Pts',(-20.5798268668381,-21.8743110027934,
123.121499920529)) ;
#45232=CARTESIAN_POINT('Ctrl Pts',(-20.8724715625939,-21.6943219224305,
123.048933898916)) ;
#45233=CARTESIAN_POINT('Ctrl Pts',(-20.5112454372603,-21.8843539087187,
122.921820528397)) ;
#45234=CARTESIAN_POINT('Ctrl Pts',(-20.7867471086995,-21.7043648283558,
122.799333949718)) ;
#45235=CARTESIAN_POINT('Ctrl Pts',(-20.4104399306398,-21.8942616898179,
122.739536472857)) ;
#45236=CARTESIAN_POINT('Ctrl Pts',(-20.6607421010669,-21.714272609455,122.571477249608)) ;
#45237=CARTESIAN_POINT('Ctrl Pts',(-20.2784482766661,-21.9042720588203,
122.57561542797)) ;
#45238=CARTESIAN_POINT('Ctrl Pts',(-20.4957543255686,-21.7242829784574,
122.366574426333)) ;
#45239=CARTESIAN_POINT('Ctrl Pts',(-20.1193995034889,-21.9143028973891,
122.437148355259)) ;
#45240=CARTESIAN_POINT('Ctrl Pts',(-20.2969450012254,-21.7343138170262,
122.19348877084)) ;
#45241=CARTESIAN_POINT('Ctrl Pts',(-19.9421174960905,-21.9241557370288,
122.33000905002)) ;
#45242=CARTESIAN_POINT('Ctrl Pts',(-20.0753430040453,-21.7441666566659,
122.059562188914)) ;
#45243=CARTESIAN_POINT('Ctrl Pts',(-19.7464337621037,-21.9341437381937,
122.253902994198)) ;
#45244=CARTESIAN_POINT('Ctrl Pts',(-19.8307389892015,-21.7541546578309,
121.964427436421)) ;
#45245=CARTESIAN_POINT('Ctrl Pts',(-19.5417073868984,-21.9440725571729,
122.213164409012)) ;
#45246=CARTESIAN_POINT('Ctrl Pts',(-19.5748309877734,-21.76408347681,121.913501885889)) ;
#45247=CARTESIAN_POINT('Ctrl Pts',(-19.3317819851724,-21.9540602598952,
122.208211065697)) ;
#45248=CARTESIAN_POINT('Ctrl Pts',(-19.3124241042443,-21.7740711795323,
121.907308024055)) ;
#45249=CARTESIAN_POINT('Ctrl Pts',(-19.1232546991255,-21.9640962596979,
122.240283219505)) ;
#45250=CARTESIAN_POINT('Ctrl Pts',(-19.0517647367421,-21.784107179335,121.947395958042)) ;
#45251=CARTESIAN_POINT('Ctrl Pts',(-18.9269352967466,-21.9739511294993,
122.306534700964)) ;
#45252=CARTESIAN_POINT('Ctrl Pts',(-18.8063639187183,-21.7939620491364,
122.030208537148)) ;
#45253=CARTESIAN_POINT('Ctrl Pts',(-18.7423427052336,-21.9839505599228,
122.407048270959)) ;
#45254=CARTESIAN_POINT('Ctrl Pts',(-18.5756220536227,-21.80396147956,122.155848712853)) ;
#45255=CARTESIAN_POINT('Ctrl Pts',(-18.5795278154634,-21.9938456773881,
122.536588268655)) ;
#45256=CARTESIAN_POINT('Ctrl Pts',(-18.3721015982493,-21.8138565970253,
122.317772569663)) ;
#45257=CARTESIAN_POINT('Ctrl Pts',(-18.4394307306069,-22.0039061709051,
122.695002768727)) ;
#45258=CARTESIAN_POINT('Ctrl Pts',(-18.1969788650756,-21.8239170905422,
122.515789157084)) ;
#45259=CARTESIAN_POINT('Ctrl Pts',(-18.3311666833367,-22.0137556511063,
122.871529628342)) ;
#45260=CARTESIAN_POINT('Ctrl Pts',(-18.0616465449145,-21.8337665707434,
122.736447563643)) ;
#45261=CARTESIAN_POINT('Ctrl Pts',(-18.253333217475,-22.0237821013701,123.067418185129)) ;
#45262=CARTESIAN_POINT('Ctrl Pts',(-17.9643529997641,-21.8437930210072,
122.981307539562)) ;
#45263=CARTESIAN_POINT('Ctrl Pts',(-18.2112421000978,-22.0338133918482,
123.274069161545)) ;
#45264=CARTESIAN_POINT('Ctrl Pts',(-17.911737129383,-21.8538243114853,123.239620782822)) ;
#45265=CARTESIAN_POINT('Ctrl Pts',(-18.2053271335064,-22.0436547795,123.480882845049)) ;
#45266=CARTESIAN_POINT('Ctrl Pts',(-17.9043414975955,-21.8636656991371,
123.498138969836)) ;
#45267=CARTESIAN_POINT('Ctrl Pts',(-18.235499498762,-22.0536581803912,123.688988918486)) ;
#45268=CARTESIAN_POINT('Ctrl Pts',(-17.9420552180239,-21.8736691000283,
123.758271923707)) ;
#45269=CARTESIAN_POINT('Ctrl Pts',(-18.3013232908441,-22.0636425631824,
123.88834285791)) ;
#45270=CARTESIAN_POINT('Ctrl Pts',(-18.0243333212748,-21.8836534828195,
124.007465107845)) ;
#45271=CARTESIAN_POINT('Ctrl Pts',(-18.4014559554124,-22.0736816531958,
124.074106712805)) ;
#45272=CARTESIAN_POINT('Ctrl Pts',(-18.1494974495607,-21.8936925728329,
124.239670692868)) ;
#45273=CARTESIAN_POINT('Ctrl Pts',(-18.5295972273494,-22.0835274621049,
124.236682169581)) ;
#45274=CARTESIAN_POINT('Ctrl Pts',(-18.3096733742783,-21.9035383817421,
124.442892027175)) ;
#45275=CARTESIAN_POINT('Ctrl Pts',(-18.6858761362846,-22.0935118849239,
124.376767470781)) ;
#45276=CARTESIAN_POINT('Ctrl Pts',(-18.5050211085327,-21.9135228045611,
124.618000034142)) ;
#45277=CARTESIAN_POINT('Ctrl Pts',(-18.8633080302938,-22.1034515101651,
124.487199990123)) ;
#45278=CARTESIAN_POINT('Ctrl Pts',(-18.7268105926817,-21.9234624298023,
124.756042327652)) ;
#45279=CARTESIAN_POINT('Ctrl Pts',(-19.0591476044493,-22.1134911996838,
124.565868443362)) ;
#45280=CARTESIAN_POINT('Ctrl Pts',(-18.9716093217471,-21.9335021193209,
124.854379340595)) ;
#45281=CARTESIAN_POINT('Ctrl Pts',(-19.2625612087232,-22.1233793881024,
124.608789289149)) ;
#45282=CARTESIAN_POINT('Ctrl Pts',(-19.2258769015638,-21.9433903077395,
124.908032136323)) ;
#45283=CARTESIAN_POINT('Ctrl Pts',(-19.4724346347167,-22.1333689141044,
124.616203338408)) ;
#45284=CARTESIAN_POINT('Ctrl Pts',(-19.4882188467763,-21.9533798337416,
124.917301153433)) ;
#45285=CARTESIAN_POINT('Ctrl Pts',(-19.6797404481245,-22.1433274154596,
124.586994703036)) ;
#45286=CARTESIAN_POINT('Ctrl Pts',(-19.7473517520323,-21.9633383350968,
124.88079179001)) ;
#45287=CARTESIAN_POINT('Ctrl Pts',(-19.8778238010788,-22.1532270094633,
124.523101680733)) ;
#45288=CARTESIAN_POINT('Ctrl Pts',(-19.9949571853173,-21.9732379291004,
124.800926502595)) ;
#45289=CARTESIAN_POINT('Ctrl Pts',(-20.0644952954339,-22.1632748975846,
124.424277452298)) ;
#45290=CARTESIAN_POINT('Ctrl Pts',(-20.2282969934944,-21.9832858172217,
124.67739751358)) ;
#45291=CARTESIAN_POINT('Ctrl Pts',(-20.2287857483374,-22.1731703228301,
124.296606248266)) ;
#45292=CARTESIAN_POINT('Ctrl Pts',(-20.4336615725465,-21.9931812424672,
124.51780896921)) ;
#45293=CARTESIAN_POINT('Ctrl Pts',(-20.3707381562611,-22.1832317135307,
124.139823950091)) ;
#45294=CARTESIAN_POINT('Ctrl Pts',(-20.6111028161255,-22.0032426331678,
124.321832200981)) ;
#45295=CARTESIAN_POINT('Ctrl Pts',(-20.4809482851262,-22.1930772972174,
123.964606584726)) ;
#45296=CARTESIAN_POINT('Ctrl Pts',(-20.7488672563639,-22.0130882168545,
124.102810049072)) ;
#45297=CARTESIAN_POINT('Ctrl Pts',(-20.5606363459277,-22.2030402705266,
123.770920839856)) ;
#45298=CARTESIAN_POINT('Ctrl Pts',(-20.8484784322108,-22.0230511901637,
123.860702848364)) ;
#45299=CARTESIAN_POINT('Ctrl Pts',(-20.605498138732,-22.2130659373523,123.564965764745)) ;
#45300=CARTESIAN_POINT('Ctrl Pts',(-20.9045567467684,-22.0330768569895,
123.603259320304)) ;
#45301=CARTESIAN_POINT('Ctrl Pts',(-20.6139362962588,-22.2229804152186,
123.356710312389)) ;
#45302=CARTESIAN_POINT('Ctrl Pts',(-20.9151055478435,-22.0429913348558,
123.342939247587)) ;
#45303=CARTESIAN_POINT('Ctrl Pts',(-20.5862899774463,-22.2329689298936,
123.148530954525)) ;
#45304=CARTESIAN_POINT('Ctrl Pts',(-20.8805485313156,-22.0529798495308,
123.082714706942)) ;
#45305=CARTESIAN_POINT('Ctrl Pts',(-20.5221446354155,-22.2430130408091,
122.947370956092)) ;
#45306=CARTESIAN_POINT('Ctrl Pts',(-20.8003679518013,-22.0630239604462,
122.831264561867)) ;
#45307=CARTESIAN_POINT('Ctrl Pts',(-20.4265781092213,-22.2528411784036,
122.764149083107)) ;
#45308=CARTESIAN_POINT('Ctrl Pts',(-20.6809098953037,-22.0728520980408,
122.602235481647)) ;
#45309=CARTESIAN_POINT('Ctrl Pts',(-20.2975883675018,-22.2629177464626,
122.596160440805)) ;
#45310=CARTESIAN_POINT('Ctrl Pts',(-20.5196736795458,-22.0829286660997,
122.392249516455)) ;
#45311=CARTESIAN_POINT('Ctrl Pts',(-20.1448753794696,-22.2727699083667,
122.456169185964)) ;
#45312=CARTESIAN_POINT('Ctrl Pts',(-20.328782028387,-22.0927808280039,122.217258955797)) ;
#45313=CARTESIAN_POINT('Ctrl Pts',(-19.9664229552607,-22.2828428703236,
122.342221971823)) ;
#45314=CARTESIAN_POINT('Ctrl Pts',(-20.1057172725599,-22.1028537899607,
122.074824536988)) ;
#45315=CARTESIAN_POINT('Ctrl Pts',(-19.7753081970072,-22.2926854323265,
122.26285604015)) ;
#45316=CARTESIAN_POINT('Ctrl Pts',(-19.8668228113398,-22.1126963519636,
121.975615871429)) ;
#45317=CARTESIAN_POINT('Ctrl Pts',(-19.5706672880173,-22.3026658688203,
122.216568225967)) ;
#45318=CARTESIAN_POINT('Ctrl Pts',(-19.6110214816132,-22.1226767884574,
121.917755554155)) ;
#45319=CARTESIAN_POINT('Ctrl Pts',(-19.3602768856682,-22.3126841741447,
122.206883478724)) ;
#45320=CARTESIAN_POINT('Ctrl Pts',(-19.3480335183811,-22.1326950937818,
121.905648968687)) ;
#45321=CARTESIAN_POINT('Ctrl Pts',(-19.1541230507367,-22.3225681380641,
122.233089766057)) ;
#45322=CARTESIAN_POINT('Ctrl Pts',(-19.090340079734,-22.1425790577013,121.938406487101)) ;
#45323=CARTESIAN_POINT('Ctrl Pts',(-18.9520588230378,-22.3326340148027,
122.295865398734)) ;
#45324=CARTESIAN_POINT('Ctrl Pts',(-18.8377600204759,-22.1526449344398,
122.016875429429)) ;
#45325=CARTESIAN_POINT('Ctrl Pts',(-18.7681011669116,-22.3424731156636,
122.390486931831)) ;
#45326=CARTESIAN_POINT('Ctrl Pts',(-18.6078114382176,-22.1624840353007,
122.135152615212)) ;
#45327=CARTESIAN_POINT('Ctrl Pts',(-18.5998200970519,-22.3525061985293,
122.517638100478)) ;
#45328=CARTESIAN_POINT('Ctrl Pts',(-18.3974600457705,-22.1725171181664,
122.294091316826)) ;
#45329=CARTESIAN_POINT('Ctrl Pts',(-18.4567024912476,-22.3625278838048,
122.672277268552)) ;
#45330=CARTESIAN_POINT('Ctrl Pts',(-18.2185627413665,-22.1825388034419,
122.487389938133)) ;
#45331=CARTESIAN_POINT('Ctrl Pts',(-18.3441099722616,-22.3723945789033,
122.846470293017)) ;
#45332=CARTESIAN_POINT('Ctrl Pts',(-18.0778211454052,-22.1924054985404,
122.70513209668)) ;
#45333=CARTESIAN_POINT('Ctrl Pts',(-18.2621912773549,-22.3823544686378,
123.039178686657)) ;
#45334=CARTESIAN_POINT('Ctrl Pts',(-17.9754225074273,-22.2023653882749,
122.946017980769)) ;
#45335=CARTESIAN_POINT('Ctrl Pts',(-18.214942034536,-22.3923894564633,123.2447729843)) ;
#45336=CARTESIAN_POINT('Ctrl Pts',(-17.9163607642041,-22.2124003761004,
123.203010659034)) ;
#45337=CARTESIAN_POINT('Ctrl Pts',(-18.2039207070877,-22.4022761605376,
123.452359252462)) ;
#45338=CARTESIAN_POINT('Ctrl Pts',(-17.9025839574836,-22.2222870801747,
123.462494584695)) ;
#45339=CARTESIAN_POINT('Ctrl Pts',(-18.2296104639163,-22.4123413047705,
123.662360780197)) ;
#45340=CARTESIAN_POINT('Ctrl Pts',(-17.9346959980839,-22.2323522244076,
123.724996117154)) ;
#45341=CARTESIAN_POINT('Ctrl Pts',(-18.2898035554938,-22.422180595499,123.860294782693)) ;
#45342=CARTESIAN_POINT('Ctrl Pts',(-18.0099377691919,-22.2421915151362,
123.972415043862)) ;
#45343=CARTESIAN_POINT('Ctrl Pts',(-18.3852909858274,-22.4322431529375,
124.049037318576)) ;
#45344=CARTESIAN_POINT('Ctrl Pts',(-18.1292969690806,-22.2522540725746,
124.208342841471)) ;
#45345=CARTESIAN_POINT('Ctrl Pts',(-18.5102142780944,-22.4421402041896,
124.215443211625)) ;
#45346=CARTESIAN_POINT('Ctrl Pts',(-18.2854516849338,-22.2621511238267,
124.416351010826)) ;
#45347=CARTESIAN_POINT('Ctrl Pts',(-18.6621688535695,-22.4520714109378,
124.358617696287)) ;
#45348=CARTESIAN_POINT('Ctrl Pts',(-18.4753956190122,-22.272082330575,124.595319409224)) ;
#45349=CARTESIAN_POINT('Ctrl Pts',(-18.8387544421233,-22.4621135951567,
124.474321570263)) ;
#45350=CARTESIAN_POINT('Ctrl Pts',(-18.6961275311406,-22.2821245147938,
124.739948983585)) ;
#45351=CARTESIAN_POINT('Ctrl Pts',(-19.0296939400006,-22.4720002232676,
124.556460841573)) ;
#45352=CARTESIAN_POINT('Ctrl Pts',(-18.9348029986765,-22.2920111429047,
124.842623278117)) ;
#45353=CARTESIAN_POINT('Ctrl Pts',(-19.234076559489,-22.4819934958,124.605048925011)) ;
#45354=CARTESIAN_POINT('Ctrl Pts',(-19.190281558459,-22.3020044154371,124.903358057767)) ;
#45355=CARTESIAN_POINT('Ctrl Pts',(-19.4427962027987,-22.4919385713414,
124.617281907534)) ;
#45356=CARTESIAN_POINT('Ctrl Pts',(-19.4511817330596,-22.3119494909786,
124.918648968524)) ;
#45357=CARTESIAN_POINT('Ctrl Pts',(-19.6506180805942,-22.5018881220697,
124.593481317551)) ;
#45358=CARTESIAN_POINT('Ctrl Pts',(-19.7109595708651,-22.3218990417068,
124.888897659172)) ;
#45359=CARTESIAN_POINT('Ctrl Pts',(-19.8528843773795,-22.5119274569177,
124.5332335477)) ;
#45360=CARTESIAN_POINT('Ctrl Pts',(-19.963792160214,-22.3319383765548,124.813587576149)) ;
#45361=CARTESIAN_POINT('Ctrl Pts',(-20.0388462005348,-22.5218135958616,
124.440381350932)) ;
#45362=CARTESIAN_POINT('Ctrl Pts',(-20.196245173065,-22.3418245154987,124.697521392829)) ;
#45363=CARTESIAN_POINT('Ctrl Pts',(-20.2078788172091,-22.5318117088353,
124.315489125279)) ;
#45364=CARTESIAN_POINT('Ctrl Pts',(-20.4075357060316,-22.3518226284724,
124.541405526169)) ;
#45365=CARTESIAN_POINT('Ctrl Pts',(-20.3516487618174,-22.5417314711877,
124.164389810808)) ;
#45366=CARTESIAN_POINT('Ctrl Pts',(-20.5872481934702,-22.3617423908249,
124.352530361773)) ;
#45367=CARTESIAN_POINT('Ctrl Pts',(-20.4684258196986,-22.5517708668004,
123.98859191938)) ;
#45368=CARTESIAN_POINT('Ctrl Pts',(-20.7332188476262,-22.3717817864375,
124.132782767646)) ;
#45369=CARTESIAN_POINT('Ctrl Pts',(-20.5517552452748,-22.5616800525887,
123.797660250607)) ;
#45370=CARTESIAN_POINT('Ctrl Pts',(-20.8373803848515,-22.3816909722258,
123.894117096644)) ;
#45371=CARTESIAN_POINT('Ctrl Pts',(-20.6013649615286,-22.5716152367462,
123.594766848094)) ;
#45372=CARTESIAN_POINT('Ctrl Pts',(-20.8993918232317,-22.3916261563833,
123.640499494821)) ;
#45373=CARTESIAN_POINT('Ctrl Pts',(-20.6149297753148,-22.5816562941321,
123.384113634597)) ;
#45374=CARTESIAN_POINT('Ctrl Pts',(-20.9163470243233,-22.4016672137692,
123.377183112359)) ;
#45375=CARTESIAN_POINT('Ctrl Pts',(-20.5922146510685,-22.5915434521654,
123.177488411578)) ;
#45376=CARTESIAN_POINT('Ctrl Pts',(-20.8879521472035,-22.4115543718025,
123.118900643946)) ;
#45377=CARTESIAN_POINT('Ctrl Pts',(-20.5336910768669,-22.6015357318413,
122.975751109046)) ;
#45378=CARTESIAN_POINT('Ctrl Pts',(-20.8147966666412,-22.4215466514784,
122.866729097642)) ;
#45379=CARTESIAN_POINT('Ctrl Pts',(-20.4413703874593,-22.6114842488863,
122.788067427756)) ;
#45380=CARTESIAN_POINT('Ctrl Pts',(-20.6993946933195,-22.4314951685235,
122.632124438289)) ;
#45381=CARTESIAN_POINT('Ctrl Pts',(-20.3182652486574,-22.6214210264567,
122.619313417233)) ;
#45382=CARTESIAN_POINT('Ctrl Pts',(-20.5455120187168,-22.4414319460939,
122.421182047729)) ;
#45383=CARTESIAN_POINT('Ctrl Pts',(-20.1671801256002,-22.6314040626037,
122.473601909739)) ;
#45384=CARTESIAN_POINT('Ctrl Pts',(-20.3566546113368,-22.4514149822408,
122.239043334206)) ;
#45385=CARTESIAN_POINT('Ctrl Pts',(-19.991856607727,-22.6414478141974,122.355972854816)) ;
#45386=CARTESIAN_POINT('Ctrl Pts',(-20.1374997937318,-22.4614587338345,
122.092007982459)) ;
#45387=CARTESIAN_POINT('Ctrl Pts',(-19.8030570092897,-22.65127634341,122.271939115384)) ;
#45388=CARTESIAN_POINT('Ctrl Pts',(-19.9014984819869,-22.4712872630471,
121.986966332369)) ;
#45389=CARTESIAN_POINT('Ctrl Pts',(-19.5975962709593,-22.6613517043187,
122.220614922131)) ;
#45390=CARTESIAN_POINT('Ctrl Pts',(-19.644672669795,-22.4813626239558,121.922812414429)) ;
#45391=CARTESIAN_POINT('Ctrl Pts',(-19.3908522666017,-22.6712083032059,
122.205989042453)) ;
#45392=CARTESIAN_POINT('Ctrl Pts',(-19.3862413607618,-22.491219222843,121.904531259593)) ;
#45393=CARTESIAN_POINT('Ctrl Pts',(-19.1804545485629,-22.6812712972238,
122.227705733918)) ;
#45394=CARTESIAN_POINT('Ctrl Pts',(-19.1232446773172,-22.5012822168609,
121.931678446646)) ;
#45395=CARTESIAN_POINT('Ctrl Pts',(-18.9806951570671,-22.6911492315132,
122.284594628893)) ;
#45396=CARTESIAN_POINT('Ctrl Pts',(-18.8735448281778,-22.5111601511503,
122.002791143889)) ;
#45397=CARTESIAN_POINT('Ctrl Pts',(-18.7914526517928,-22.7011498790713,
122.376106438856)) ;
#45398=CARTESIAN_POINT('Ctrl Pts',(-18.6369922199882,-22.5211607987084,
122.117182286071)) ;
#45399=CARTESIAN_POINT('Ctrl Pts',(-18.6222332954635,-22.7110677255094,
122.497984639726)) ;
#45400=CARTESIAN_POINT('Ctrl Pts',(-18.4254683343915,-22.5310786451465,
122.269531684477)) ;
#45401=CARTESIAN_POINT('Ctrl Pts',(-18.474883672655,-22.721118842515,122.649391564558)) ;
#45402=CARTESIAN_POINT('Ctrl Pts',(-18.2412825269459,-22.5411297621521,
122.45879123557)) ;
#45403=CARTESIAN_POINT('Ctrl Pts',(-18.3579599908217,-22.7309895778256,
122.820875939281)) ;
#45404=CARTESIAN_POINT('Ctrl Pts',(-18.0951286476762,-22.5510004974627,
122.673148447113)) ;
#45405=CARTESIAN_POINT('Ctrl Pts',(-18.270849081835,-22.7410602850686,123.013805427642)) ;
#45406=CARTESIAN_POINT('Ctrl Pts',(-17.986241610246,-22.5610712047057,122.914310640418)) ;
#45407=CARTESIAN_POINT('Ctrl Pts',(-18.2196899669182,-22.7508932925205,
123.214115396645)) ;
#45408=CARTESIAN_POINT('Ctrl Pts',(-17.9222939724761,-22.5709042121576,
123.164699747312)) ;
#45409=CARTESIAN_POINT('Ctrl Pts',(-18.203176745519,-22.7609237848228,123.42433279345)) ;
#45410=CARTESIAN_POINT('Ctrl Pts',(-17.9016542679233,-22.5809347044599,
123.427471548306)) ;
#45411=CARTESIAN_POINT('Ctrl Pts',(-18.2240311555207,-22.7709553798962,
123.634206914964)) ;
#45412=CARTESIAN_POINT('Ctrl Pts',(-17.927723884169,-22.5909662995333,123.689813957202)) ;
#45413=CARTESIAN_POINT('Ctrl Pts',(-18.2794406669794,-22.7807850790344,
123.83327619676)) ;
#45414=CARTESIAN_POINT('Ctrl Pts',(-17.9969878123147,-22.6007959986715,
123.93865131243)) ;
#45415=CARTESIAN_POINT('Ctrl Pts',(-18.3694648397809,-22.790774528916,124.023019043572)) ;
#45416=CARTESIAN_POINT('Ctrl Pts',(-18.1095198729244,-22.6107854485531,
124.175829191989)) ;
#45417=CARTESIAN_POINT('Ctrl Pts',(-18.4921611930021,-22.8008183867317,
124.194863216364)) ;
#45418=CARTESIAN_POINT('Ctrl Pts',(-18.2628916857644,-22.6208293063688,
124.390633246382)) ;
#45419=CARTESIAN_POINT('Ctrl Pts',(-18.6391999982746,-22.8106400773219,
124.339828342554)) ;
#45420=CARTESIAN_POINT('Ctrl Pts',(-18.446692434265,-22.630650996959,124.571839161793)) ;
#45421=CARTESIAN_POINT('Ctrl Pts',(-18.8125751270944,-22.8206751678623,
124.460026469785)) ;
#45422=CARTESIAN_POINT('Ctrl Pts',(-18.6634124377873,-22.6406860874994,
124.722085054435)) ;
#45423=CARTESIAN_POINT('Ctrl Pts',(-19.0042354854205,-22.830699686845,124.547700241937)) ;
#45424=CARTESIAN_POINT('Ctrl Pts',(-18.9029886662497,-22.6507106064821,
124.831675526016)) ;
#45425=CARTESIAN_POINT('Ctrl Pts',(-19.2047392934395,-22.8405595322552,
124.600226995631)) ;
#45426=CARTESIAN_POINT('Ctrl Pts',(-19.1536198777574,-22.6605704518923,
124.897332264122)) ;
#45427=CARTESIAN_POINT('Ctrl Pts',(-19.4133825738018,-22.8505193085708,
124.617890170241)) ;
#45428=CARTESIAN_POINT('Ctrl Pts',(-19.4144244913002,-22.670530228208,124.919409092967)) ;
#45429=CARTESIAN_POINT('Ctrl Pts',(-19.6233229031397,-22.8605475058855,
124.598638239538)) ;
#45430=CARTESIAN_POINT('Ctrl Pts',(-19.6768496651292,-22.6805584255226,
124.895342097645)) ;
#45431=CARTESIAN_POINT('Ctrl Pts',(-19.8243679055007,-22.8704550481758,
124.544126078897)) ;
#45432=CARTESIAN_POINT('Ctrl Pts',(-19.9281559636117,-22.6904659678129,
124.827199646983)) ;
#45433=CARTESIAN_POINT('Ctrl Pts',(-20.0152757096399,-22.8804876987396,
124.454494142613)) ;
#45434=CARTESIAN_POINT('Ctrl Pts',(-20.1667897461997,-22.7004986183768,
124.715157775083)) ;
#45435=CARTESIAN_POINT('Ctrl Pts',(-20.1852178949266,-22.8903716551663,
124.33491330894)) ;
#45436=CARTESIAN_POINT('Ctrl Pts',(-20.3792168210052,-22.7103825748034,
124.56567950925)) ;
#45437=CARTESIAN_POINT('Ctrl Pts',(-20.3337523313298,-22.9003613565281,
124.186436934306)) ;
#45438=CARTESIAN_POINT('Ctrl Pts',(-20.5648833309736,-22.7203722761653,
124.380082284069)) ;
#45439=CARTESIAN_POINT('Ctrl Pts',(-20.4544985548872,-22.9104023518042,
124.013286908638)) ;
#45440=CARTESIAN_POINT('Ctrl Pts',(-20.7158142403492,-22.7304132714413,
124.163643559951)) ;
#45441=CARTESIAN_POINT('Ctrl Pts',(-20.5418120177757,-22.9202352410725,
123.825917664307)) ;
#45442=CARTESIAN_POINT('Ctrl Pts',(-20.8249543879318,-22.7402461607097,
123.929430163563)) ;
#45443=CARTESIAN_POINT('Ctrl Pts',(-20.5967197719903,-22.93022839944,123.623135595412)) ;
#45444=CARTESIAN_POINT('Ctrl Pts',(-20.8935867559205,-22.7502393190771,
123.675951817842)) ;
#45445=CARTESIAN_POINT('Ctrl Pts',(-20.6152207366922,-22.9402604417921,
123.413033506782)) ;
#45446=CARTESIAN_POINT('Ctrl Pts',(-20.9167106283028,-22.7602713614292,
123.413324039136)) ;
#45447=CARTESIAN_POINT('Ctrl Pts',(-20.5975204253957,-22.9501256857505,
123.2064025244)) ;
#45448=CARTESIAN_POINT('Ctrl Pts',(-20.8945827853963,-22.7701366053876,
123.155034786092)) ;
#45449=CARTESIAN_POINT('Ctrl Pts',(-20.5442580745083,-22.9600875769965,
123.003852214581)) ;
#45450=CARTESIAN_POINT('Ctrl Pts',(-20.82800234089,-22.7800984966336,122.901847296241)) ;
#45451=CARTESIAN_POINT('Ctrl Pts',(-20.4556884997879,-22.970122477015,122.812391064617)) ;
#45452=CARTESIAN_POINT('Ctrl Pts',(-20.7172881603951,-22.7901333966521,
122.662521920387)) ;
#45453=CARTESIAN_POINT('Ctrl Pts',(-20.3372800803288,-22.9800075574296,
122.641575983214)) ;
#45454=CARTESIAN_POINT('Ctrl Pts',(-20.5692752424808,-22.8000184770667,
122.449004039222)) ;
#45455=CARTESIAN_POINT('Ctrl Pts',(-20.1883694042385,-22.9900727295544,
122.491279319789)) ;
#45456=CARTESIAN_POINT('Ctrl Pts',(-20.3831352080727,-22.8100836491915,
122.261135086256)) ;
#45457=CARTESIAN_POINT('Ctrl Pts',(-20.0193951599007,-22.9999199642779,
122.37164075247)) ;
#45458=CARTESIAN_POINT('Ctrl Pts',(-20.1719153765991,-22.819930883915,122.111588554488)) ;
#45459=CARTESIAN_POINT('Ctrl Pts',(-19.8289685430891,-23.0099507755956,
122.281076764927)) ;
#45460=CARTESIAN_POINT('Ctrl Pts',(-19.9338810019722,-22.8299616952328,
121.998385955222)) ;
#45461=CARTESIAN_POINT('Ctrl Pts',(-19.6259877305142,-23.0199603915091,
122.225477205925)) ;
#45462=CARTESIAN_POINT('Ctrl Pts',(-19.6801542546242,-22.8399713111463,
121.928888950712)) ;
#45463=CARTESIAN_POINT('Ctrl Pts',(-19.4185677638405,-23.0298711709128,
122.205958909889)) ;
#45464=CARTESIAN_POINT('Ctrl Pts',(-19.4208786354196,-22.84988209055,121.904493618432)) ;
#45465=CARTESIAN_POINT('Ctrl Pts',(-19.2104507212989,-23.0398004367019,
122.222263809827)) ;
#45466=CARTESIAN_POINT('Ctrl Pts',(-19.1607322268354,-22.859811356339,121.924877430898)) ;
#45467=CARTESIAN_POINT('Ctrl Pts',(-19.0060800631454,-23.0498431300145,
122.275221685096)) ;
#45468=CARTESIAN_POINT('Ctrl Pts',(-18.9052696006217,-22.8698540496516,
121.991077325652)) ;
#45469=CARTESIAN_POINT('Ctrl Pts',(-18.816920652705,-23.0597296627092,122.361382751279)) ;
#45470=CARTESIAN_POINT('Ctrl Pts',(-18.6688210508467,-22.8797405823464,
122.098781259546)) ;
#45471=CARTESIAN_POINT('Ctrl Pts',(-18.6435653180198,-23.0697228078125,
122.480041622256)) ;
#45472=CARTESIAN_POINT('Ctrl Pts',(-18.4521283292672,-22.8897337274496,
122.247107144986)) ;
#45473=CARTESIAN_POINT('Ctrl Pts',(-18.4942067621472,-23.0796684884866,
122.626365687683)) ;
#45474=CARTESIAN_POINT('Ctrl Pts',(-18.2654318576276,-22.8996794081237,
122.430014319229)) ;
#45475=CARTESIAN_POINT('Ctrl Pts',(-18.3721507507593,-23.0896157461133,
122.796186530113)) ;
#45476=CARTESIAN_POINT('Ctrl Pts',(-18.1128639588266,-22.9096266657504,
122.642292140986)) ;
#45477=CARTESIAN_POINT('Ctrl Pts',(-18.280738860759,-23.0996636482348,122.986614485634)) ;
#45478=CARTESIAN_POINT('Ctrl Pts',(-17.9986015572507,-22.9196745678719,
122.880328253833)) ;
#45479=CARTESIAN_POINT('Ctrl Pts',(-18.2247452921894,-23.1095113538565,
123.185929489645)) ;
#45480=CARTESIAN_POINT('Ctrl Pts',(-17.9286121291567,-22.9295222734936,
123.129473138919)) ;
#45481=CARTESIAN_POINT('Ctrl Pts',(-18.203315371917,-23.1194728204906,123.394243964455)) ;
#45482=CARTESIAN_POINT('Ctrl Pts',(-17.9018275042711,-22.9394837401277,
123.389866644002)) ;
#45483=CARTESIAN_POINT('Ctrl Pts',(-18.2187690231212,-23.1295023737588,
123.604537566451)) ;
#45484=CARTESIAN_POINT('Ctrl Pts',(-17.9211473399048,-22.9495132933959,
123.652733485376)) ;
#45485=CARTESIAN_POINT('Ctrl Pts',(-18.2697520445231,-23.1394092657862,
123.806478018759)) ;
#45486=CARTESIAN_POINT('Ctrl Pts',(-17.9848788717473,-22.9594201854233,
123.905158576402)) ;
#45487=CARTESIAN_POINT('Ctrl Pts',(-18.3549970966278,-23.1493569098992,
123.997428173794)) ;
#45488=CARTESIAN_POINT('Ctrl Pts',(-18.0914378078134,-22.9693678295363,
124.143845240036)) ;
#45489=CARTESIAN_POINT('Ctrl Pts',(-18.4726356234465,-23.1593569529281,
124.171699257656)) ;
#45490=CARTESIAN_POINT('Ctrl Pts',(-18.2384883382395,-22.9793678725652,
124.361682579422)) ;
#45491=CARTESIAN_POINT('Ctrl Pts',(-18.6195515746322,-23.1693957189221,
124.323190189224)) ;
#45492=CARTESIAN_POINT('Ctrl Pts',(-18.4221353271476,-22.9894066385592,
124.551044334108)) ;
#45493=CARTESIAN_POINT('Ctrl Pts',(-18.7866669271075,-23.1792207809443,
124.444609990743)) ;
#45494=CARTESIAN_POINT('Ctrl Pts',(-18.6310313255418,-22.9992317005814,
124.702816918751)) ;
#45495=CARTESIAN_POINT('Ctrl Pts',(-18.9764845901678,-23.1892753282707,
124.537586105056)) ;
#45496=CARTESIAN_POINT('Ctrl Pts',(-18.8683046803637,-23.0092862479078,
124.81903454041)) ;
#45497=CARTESIAN_POINT('Ctrl Pts',(-19.1774335204479,-23.1992185717199,
124.595200515695)) ;
#45498=CARTESIAN_POINT('Ctrl Pts',(-19.1194917233323,-23.019229491357,124.891049871198)) ;
#45499=CARTESIAN_POINT('Ctrl Pts',(-19.3844025852747,-23.2091207433278,
124.617601381638)) ;
#45500=CARTESIAN_POINT('Ctrl Pts',(-19.3782034066478,-23.0291316629649,
124.919048155738)) ;
#45501=CARTESIAN_POINT('Ctrl Pts',(-19.5952575378545,-23.219173578938,124.603384824931)) ;
#45502=CARTESIAN_POINT('Ctrl Pts',(-19.6417720055539,-23.0391844985751,
124.9012746228)) ;
#45503=CARTESIAN_POINT('Ctrl Pts',(-19.796808082773,-23.2290466366235,124.553754633832)) ;
#45504=CARTESIAN_POINT('Ctrl Pts',(-19.8937094829923,-23.0490575562606,
124.839234191459)) ;
#45505=CARTESIAN_POINT('Ctrl Pts',(-19.9892291256445,-23.2390418981492,
124.469324547835)) ;
#45506=CARTESIAN_POINT('Ctrl Pts',(-20.1342348698061,-23.0590528177863,
124.733693798384)) ;
#45507=CARTESIAN_POINT('Ctrl Pts',(-20.1643902735447,-23.2490672675697,
124.352097383469)) ;
#45508=CARTESIAN_POINT('Ctrl Pts',(-20.3531841875638,-23.0690781872068,
124.587158170132)) ;
#45509=CARTESIAN_POINT('Ctrl Pts',(-20.3146713289308,-23.2589571000963,
124.208405044587)) ;
#45510=CARTESIAN_POINT('Ctrl Pts',(-20.5410358788454,-23.0789680197334,
124.407538039965)) ;
#45511=CARTESIAN_POINT('Ctrl Pts',(-20.4803738058375,-23.2722550709057,
123.98326749613)) ;
#45512=CARTESIAN_POINT('Ctrl Pts',(-20.74814931711,-23.0922659905428,124.126127329763)) ;
#45513=CARTESIAN_POINT('Ctrl Pts',(-20.5831671550575,-23.2854534660148,
123.722071678799)) ;
#45514=CARTESIAN_POINT('Ctrl Pts',(-20.87663678955,-23.105464385652,123.799667857733)) ;
#45515=CARTESIAN_POINT('Ctrl Pts',(-20.6148571245368,-23.2988489082943,
123.442305301246)) ;
#45516=CARTESIAN_POINT('Ctrl Pts',(-20.9162580761209,-23.1188598279314,
123.449902418922)) ;
#45517=CARTESIAN_POINT('Ctrl Pts',(-20.6022321518531,-23.3087247465333,
123.235027259948)) ;
#45518=CARTESIAN_POINT('Ctrl Pts',(-20.9004717403109,-23.1287356661704,
123.190816756868)) ;
#45519=CARTESIAN_POINT('Ctrl Pts',(-20.5530100746428,-23.318786149131,123.029348117295)) ;
#45520=CARTESIAN_POINT('Ctrl Pts',(-20.8389416666321,-23.1387970687681,
122.933714939038)) ;
#45521=CARTESIAN_POINT('Ctrl Pts',(-20.470495204662,-23.3286512060661,122.839039896976)) ;
#45522=CARTESIAN_POINT('Ctrl Pts',(-20.7357971607144,-23.1486621257033,
122.69583283738)) ;
#45523=CARTESIAN_POINT('Ctrl Pts',(-20.3548367842642,-23.3386633020149,
122.663215896037)) ;
#45524=CARTESIAN_POINT('Ctrl Pts',(-20.5912157870178,-23.1586742216521,
122.476050346887)) ;
#45525=CARTESIAN_POINT('Ctrl Pts',(-20.1631967914319,-23.3519406111604,
122.460187922931)) ;
#45526=CARTESIAN_POINT('Ctrl Pts',(-20.3516936594044,-23.1719515307975,
122.222286259416)) ;
#45527=CARTESIAN_POINT('Ctrl Pts',(-19.8630377268875,-23.3685396366677,
122.274632914981)) ;
#45528=CARTESIAN_POINT('Ctrl Pts',(-19.9764398067608,-23.1885505563048,
121.990323874655)) ;
#45529=CARTESIAN_POINT('Ctrl Pts',(-19.517487437228,-23.3851386847007,122.202591928007)) ;
#45530=CARTESIAN_POINT('Ctrl Pts',(-19.5445846288261,-23.2051496043378,
121.900290049291)) ;
#45531=CARTESIAN_POINT('Ctrl Pts',(-19.23951312528,-23.3983820967316,122.217815968059)) ;
#45532=CARTESIAN_POINT('Ctrl Pts',(-19.197050432373,-23.2183930163688,121.919316506906)) ;
#45533=CARTESIAN_POINT('Ctrl Pts',(-19.0339916765018,-23.4084195244201,
122.265667627133)) ;
#45534=CARTESIAN_POINT('Ctrl Pts',(-18.9401631491161,-23.2284304440572,
121.979134289703)) ;
#45535=CARTESIAN_POINT('Ctrl Pts',(-18.8424913044911,-23.4183238263757,
122.347410808801)) ;
#45536=CARTESIAN_POINT('Ctrl Pts',(-18.7007825062615,-23.2383347460128,
122.08131781826)) ;
#45537=CARTESIAN_POINT('Ctrl Pts',(-18.6084602838952,-23.4315906663508,
122.499189778994)) ;
#45538=CARTESIAN_POINT('Ctrl Pts',(-18.4082618728628,-23.251601585988,122.271030307521)) ;
#45539=CARTESIAN_POINT('Ctrl Pts',(-18.3717345959788,-23.4482168644408,
122.761707590166)) ;
#45540=CARTESIAN_POINT('Ctrl Pts',(-18.1123399887699,-23.2682277840779,
122.599191193754)) ;
#45541=CARTESIAN_POINT('Ctrl Pts',(-18.2123565640676,-23.4681359798242,
123.154114455554)) ;
#45542=CARTESIAN_POINT('Ctrl Pts',(-17.9131297581632,-23.2881468994613,
123.089717711788)) ;
#45543=CARTESIAN_POINT('Ctrl Pts',(-18.1988208253406,-23.4847424029584,
123.506996953541)) ;
#45544=CARTESIAN_POINT('Ctrl Pts',(-17.8962057487813,-23.3047533225956,
123.530754190466)) ;
#45545=CARTESIAN_POINT('Ctrl Pts',(-18.2607588524776,-23.4980386234541,
123.779530753442)) ;
#45546=CARTESIAN_POINT('Ctrl Pts',(-17.9736383080703,-23.3180495430913,
123.871481315084)) ;
#45547=CARTESIAN_POINT('Ctrl Pts',(-18.3683238744161,-23.5113074557956,
124.036997547401)) ;
#45548=CARTESIAN_POINT('Ctrl Pts',(-18.1080876895051,-23.3313183754327,
124.193291225439)) ;
#45549=CARTESIAN_POINT('Ctrl Pts',(-18.585515956159,-23.5279987038287,124.31755527357)) ;
#45550=CARTESIAN_POINT('Ctrl Pts',(-18.3795904845808,-23.3480096234658,
124.544002089629)) ;
#45551=CARTESIAN_POINT('Ctrl Pts',(-18.9413317824027,-23.5478084355015,
124.543077586913)) ;
#45552=CARTESIAN_POINT('Ctrl Pts',(-18.8243580038784,-23.3678193551386,
124.825895671555)) ;
#45553=CARTESIAN_POINT('Ctrl Pts',(-19.3559796542478,-23.56778604283,124.635208528437)) ;
#45554=CARTESIAN_POINT('Ctrl Pts',(-19.3426692477421,-23.3877969624672,
124.941057197669)) ;
#45555=CARTESIAN_POINT('Ctrl Pts',(-19.7759608022422,-23.5877123518879,
124.579685890579)) ;
#45556=CARTESIAN_POINT('Ctrl Pts',(-19.8676443126626,-23.407723271525,124.871649885225)) ;
#45557=CARTESIAN_POINT('Ctrl Pts',(-20.1505472402133,-23.6075292120526,
124.386491448277)) ;
#45558=CARTESIAN_POINT('Ctrl Pts',(-20.3358743901566,-23.4275401316897,
124.630155280585)) ;
#45559=CARTESIAN_POINT('Ctrl Pts',(-20.4401428515061,-23.6276290276466,
124.072390207339)) ;
#45560=CARTESIAN_POINT('Ctrl Pts',(-20.6978674016167,-23.4476399472837,
124.237525821763)) ;
#45561=CARTESIAN_POINT('Ctrl Pts',(-20.6026657871358,-23.6473859915291,
123.684825873049)) ;
#45562=CARTESIAN_POINT('Ctrl Pts',(-20.9010174941863,-23.4673969111663,
123.753071870117)) ;
#45563=CARTESIAN_POINT('Ctrl Pts',(-20.6242876059637,-23.6674229175986,
123.259481688023)) ;
#45564=CARTESIAN_POINT('Ctrl Pts',(-20.9280426935608,-23.4874338372357,
123.221391133714)) ;
#45565=CARTESIAN_POINT('Ctrl Pts',(-20.4997957023964,-23.6872924999801,
122.855645078802)) ;
#45566=CARTESIAN_POINT('Ctrl Pts',(-20.772426096765,-23.5073034196172,122.716597558778)) ;
#45567=CARTESIAN_POINT('Ctrl Pts',(-20.2454865673464,-23.7071970717333,
122.517448321673)) ;
#45568=CARTESIAN_POINT('Ctrl Pts',(-20.4545393933605,-23.5272079913704,
122.293853597091)) ;
#45569=CARTESIAN_POINT('Ctrl Pts',(-19.8900271158853,-23.7271496739318,
122.285727883188)) ;
#45570=CARTESIAN_POINT('Ctrl Pts',(-20.0102149504557,-23.5471605935689,
122.004204373971)) ;
#45571=CARTESIAN_POINT('Ctrl Pts',(-19.4778464728188,-23.747059164902,122.189596892363)) ;
#45572=CARTESIAN_POINT('Ctrl Pts',(-19.4949902616942,-23.5670700845392,
121.884042017214)) ;
#45573=CARTESIAN_POINT('Ctrl Pts',(-19.0585021845433,-23.7669105336015,
122.238587168872)) ;
#45574=CARTESIAN_POINT('Ctrl Pts',(-18.9708122647659,-23.5869214532386,
121.94527950064)) ;
#45575=CARTESIAN_POINT('Ctrl Pts',(-18.6771515985997,-23.7869907297375,
122.43039174872)) ;
#45576=CARTESIAN_POINT('Ctrl Pts',(-18.4941229340544,-23.6070016493746,
122.185035924344)) ;
#45577=CARTESIAN_POINT('Ctrl Pts',(-18.3880786328134,-23.8067916733129,
122.736642917923)) ;
#45578=CARTESIAN_POINT('Ctrl Pts',(-18.1327837985555,-23.62680259295,122.567847534588)) ;
#45579=CARTESIAN_POINT('Ctrl Pts',(-18.2185138748618,-23.8267756498224,
123.126183556028)) ;
#45580=CARTESIAN_POINT('Ctrl Pts',(-17.9208269264055,-23.6467865694595,
123.054772698368)) ;
#45581=CARTESIAN_POINT('Ctrl Pts',(-18.1928000702527,-23.846691612798,123.54886807584)) ;
#45582=CARTESIAN_POINT('Ctrl Pts',(-17.8886839110732,-23.6667025324351,
123.583127051767)) ;
#45583=CARTESIAN_POINT('Ctrl Pts',(-18.3114981929088,-23.8665620476199,
123.954437415859)) ;
#45584=CARTESIAN_POINT('Ctrl Pts',(-18.0370543006657,-23.686572967257,124.090087584522)) ;
#45585=CARTESIAN_POINT('Ctrl Pts',(-18.5641851710754,-23.886612332853,124.297650548748)) ;
#45586=CARTESIAN_POINT('Ctrl Pts',(-18.3529120736301,-23.7066232524901,
124.519105466772)) ;
#45587=CARTESIAN_POINT('Ctrl Pts',(-18.9138459519034,-23.9063863016123,
124.531438448419)) ;
#45588=CARTESIAN_POINT('Ctrl Pts',(-18.789984541274,-23.7263972212494,124.811340607854)) ;
#45589=CARTESIAN_POINT('Ctrl Pts',(-19.327728107229,-23.9264427597318,124.633511754983)) ;
#45590=CARTESIAN_POINT('Ctrl Pts',(-19.3073372095614,-23.746453679369,124.93893490729)) ;
#45591=CARTESIAN_POINT('Ctrl Pts',(-19.7463440551213,-23.9462376427228,
124.588636490226)) ;
#45592=CARTESIAN_POINT('Ctrl Pts',(-19.8306051755044,-23.76624856236,124.882843707526)) ;
#45593=CARTESIAN_POINT('Ctrl Pts',(-20.128134455108,-23.9662042980252,124.403168082798)) ;
#45594=CARTESIAN_POINT('Ctrl Pts',(-20.3078444224997,-23.7862152176623,
124.651011447722)) ;
#45595=CARTESIAN_POINT('Ctrl Pts',(-20.4232185491835,-23.9861632681017,
124.098054033906)) ;
#45596=CARTESIAN_POINT('Ctrl Pts',(-20.6767016461882,-23.8061741877388,
124.269621393362)) ;
#45597=CARTESIAN_POINT('Ctrl Pts',(-20.5961622014183,-24.0060593556918,
123.711998667547)) ;
#45598=CARTESIAN_POINT('Ctrl Pts',(-20.892884068729,-23.8260702753289,123.787054530312)) ;
#45599=CARTESIAN_POINT('Ctrl Pts',(-20.6274889819743,-24.0259575256034,
123.290106766545)) ;
#45600=CARTESIAN_POINT('Ctrl Pts',(-20.9320464014087,-23.8459684452405,
123.259690813219)) ;
#45601=CARTESIAN_POINT('Ctrl Pts',(-20.513337763902,-24.0458633609705,122.882506566483)) ;
#45602=CARTESIAN_POINT('Ctrl Pts',(-20.7893616368976,-23.8658742806076,
122.750190072207)) ;
#45603=CARTESIAN_POINT('Ctrl Pts',(-20.266431677999,-24.0658132859084,122.537627079781)) ;
#45604=CARTESIAN_POINT('Ctrl Pts',(-20.4807327588592,-23.8858242055455,
122.319088447684)) ;
#45605=CARTESIAN_POINT('Ctrl Pts',(-19.9180548383199,-24.0856924758188,
122.298181469176)) ;
#45606=CARTESIAN_POINT('Ctrl Pts',(-20.0452649316201,-23.9057033954559,
122.019778092239)) ;
#45607=CARTESIAN_POINT('Ctrl Pts',(-19.5069122512383,-24.1056738000994,
122.191249797151)) ;
#45608=CARTESIAN_POINT('Ctrl Pts',(-19.5313379424967,-23.9256847197365,
121.886108846057)) ;
#45609=CARTESIAN_POINT('Ctrl Pts',(-19.0849454561733,-24.1256035843077,
122.231166566416)) ;
#45610=CARTESIAN_POINT('Ctrl Pts',(-19.0038793190178,-23.9456145039448,
121.936000230857)) ;
#45611=CARTESIAN_POINT('Ctrl Pts',(-18.7022509031181,-24.1455235736985,
122.412432300618)) ;
#45612=CARTESIAN_POINT('Ctrl Pts',(-18.5255093850671,-23.9655344933356,
122.162577000674)) ;
#45613=CARTESIAN_POINT('Ctrl Pts',(-18.4045331289834,-24.1653787690525,
122.711900017558)) ;
#45614=CARTESIAN_POINT('Ctrl Pts',(-18.1533588423712,-23.9853896886896,
122.536910497568)) ;
#45615=CARTESIAN_POINT('Ctrl Pts',(-18.2256300026401,-24.1854247707119,
123.098661615411)) ;
#45616=CARTESIAN_POINT('Ctrl Pts',(-17.9297252155865,-24.005435690349,123.020349675099)) ;
#45617=CARTESIAN_POINT('Ctrl Pts',(-18.1956840876194,-24.2019245179217,
123.448290706154)) ;
#45618=CARTESIAN_POINT('Ctrl Pts',(-17.8922881637436,-24.0219354375588,
123.457418896112)) ;
#45619=CARTESIAN_POINT('Ctrl Pts',(-18.244751099481,-24.2153131223698,123.725437756677)) ;
#45620=CARTESIAN_POINT('Ctrl Pts',(-17.9536182369137,-24.0353240420069,
123.803823185436)) ;
#45621=CARTESIAN_POINT('Ctrl Pts',(-18.3158010212771,-24.2251749507047,
123.92021291796)) ;
#45622=CARTESIAN_POINT('Ctrl Pts',(-18.0424306542549,-24.0451858703418,
124.047300970856)) ;
#45623=CARTESIAN_POINT('Ctrl Pts',(-18.4201246805275,-24.2351410934622,
124.101932284297)) ;
#45624=CARTESIAN_POINT('Ctrl Pts',(-18.1728224348044,-24.0551520130994,
124.274441107709)) ;
#45625=CARTESIAN_POINT('Ctrl Pts',(-18.600479700421,-24.2485028395872,124.317163919076)) ;
#45626=CARTESIAN_POINT('Ctrl Pts',(-18.398315477012,-24.0685137592243,124.543527593381)) ;
#45627=CARTESIAN_POINT('Ctrl Pts',(-18.8864879871126,-24.2649571685423,
124.518993893139)) ;
#45628=CARTESIAN_POINT('Ctrl Pts',(-18.7557534014151,-24.0849680881794,
124.795766078304)) ;
#45629=CARTESIAN_POINT('Ctrl Pts',(-19.2302450355489,-24.2817244135906,
124.612794594497)) ;
#45630=CARTESIAN_POINT('Ctrl Pts',(-19.1855079887731,-24.1017353332277,
124.913045707015)) ;
#45631=CARTESIAN_POINT('Ctrl Pts',(-19.5076006939437,-24.2949109788646,
124.613694249436)) ;
#45632=CARTESIAN_POINT('Ctrl Pts',(-19.5321625871901,-24.1149218985017,
124.914163508115)) ;
#45633=CARTESIAN_POINT('Ctrl Pts',(-19.714585996907,-24.3049004376092,124.57853472076)) ;
#45634=CARTESIAN_POINT('Ctrl Pts',(-19.7909027433267,-24.1249113572463,
124.870218955293)) ;
#45635=CARTESIAN_POINT('Ctrl Pts',(-19.9117282679633,-24.3148542100903,
124.508226632481)) ;
#45636=CARTESIAN_POINT('Ctrl Pts',(-20.0373293987813,-24.1348651297274,
124.782335916118)) ;
#45637=CARTESIAN_POINT('Ctrl Pts',(-20.0952429868065,-24.324902026623,124.40366816945)) ;
#45638=CARTESIAN_POINT('Ctrl Pts',(-20.2667248444726,-24.1449129462601,
124.651640371251)) ;
#45639=CARTESIAN_POINT('Ctrl Pts',(-20.2546683283464,-24.3347435597455,
124.271759801232)) ;
#45640=CARTESIAN_POINT('Ctrl Pts',(-20.4660081191832,-24.1547544793826,
124.486757064472)) ;
#45641=CARTESIAN_POINT('Ctrl Pts',(-20.3910452829839,-24.3447298019652,
124.112189741865)) ;
#45642=CARTESIAN_POINT('Ctrl Pts',(-20.6364815530708,-24.1647407216023,
124.287296273843)) ;
#45643=CARTESIAN_POINT('Ctrl Pts',(-20.4972397987561,-24.3546664253901,
123.932255968931)) ;
#45644=CARTESIAN_POINT('Ctrl Pts',(-20.7692271456916,-24.1746773450272,
124.062380424929)) ;
#45645=CARTESIAN_POINT('Ctrl Pts',(-20.5712954604918,-24.3647163027731,
123.73440257886)) ;
#45646=CARTESIAN_POINT('Ctrl Pts',(-20.8617993883025,-24.1847272224102,
123.815064619583)) ;
#45647=CARTESIAN_POINT('Ctrl Pts',(-20.6092665986412,-24.3745667415506,
123.530810616257)) ;
#45648=CARTESIAN_POINT('Ctrl Pts',(-20.9092661000716,-24.1945776611878,
123.560575071859)) ;
#45649=CARTESIAN_POINT('Ctrl Pts',(-20.6118828892727,-24.3845387555194,
123.321210192378)) ;
#45650=CARTESIAN_POINT('Ctrl Pts',(-20.9125392723098,-24.2045496751565,
123.298574461719)) ;
#45651=CARTESIAN_POINT('Ctrl Pts',(-20.5779494879227,-24.3945339241455,
123.113804511949)) ;
#45652=CARTESIAN_POINT('Ctrl Pts',(-20.8701252717379,-24.2145448437826,
123.039316830709)) ;
#45653=CARTESIAN_POINT('Ctrl Pts',(-20.5080285322928,-24.4045678074067,
122.914803419106)) ;
#45654=CARTESIAN_POINT('Ctrl Pts',(-20.7827267210347,-24.2245787270438,
122.790564493814)) ;
#45655=CARTESIAN_POINT('Ctrl Pts',(-20.4067104297543,-24.41442367747,122.734046050817)) ;
#45656=CARTESIAN_POINT('Ctrl Pts',(-20.6560814228119,-24.2344345971071,
122.564616215145)) ;
#45657=CARTESIAN_POINT('Ctrl Pts',(-20.2739437816179,-24.4244212233872,
122.571137981273)) ;
#45658=CARTESIAN_POINT('Ctrl Pts',(-20.4901252098502,-24.2444321430243,
122.3609792939)) ;
#45659=CARTESIAN_POINT('Ctrl Pts',(-20.1163503321144,-24.4343293502864,
122.434915065284)) ;
#45660=CARTESIAN_POINT('Ctrl Pts',(-20.293135035734,-24.2543402699236,122.190698398529)) ;
#45661=CARTESIAN_POINT('Ctrl Pts',(-19.9358381554827,-24.4443397218086,
122.326707961461)) ;
#45662=CARTESIAN_POINT('Ctrl Pts',(-20.0674961654377,-24.2643506414457,
122.055437128195)) ;
#45663=CARTESIAN_POINT('Ctrl Pts',(-19.7387342050816,-24.454370164556,122.251783176735)) ;
#45664=CARTESIAN_POINT('Ctrl Pts',(-19.8211172047256,-24.2743810841931,
121.961778537735)) ;
#45665=CARTESIAN_POINT('Ctrl Pts',(-19.5354521664302,-24.4642181171093,
122.212461214448)) ;
#45666=CARTESIAN_POINT('Ctrl Pts',(-19.5670147878812,-24.2842290367464,
121.912623318456)) ;
#45667=CARTESIAN_POINT('Ctrl Pts',(-19.3239551652899,-24.4742807861303,
122.208794045191)) ;
#45668=CARTESIAN_POINT('Ctrl Pts',(-19.3026436245788,-24.2942917057674,
121.908036631008)) ;
#45669=CARTESIAN_POINT('Ctrl Pts',(-19.1185123192759,-24.4841751615942,
122.241504281932)) ;
#45670=CARTESIAN_POINT('Ctrl Pts',(-19.0458393133714,-24.3041860812313,
121.948921771872)) ;
#45671=CARTESIAN_POINT('Ctrl Pts',(-18.9207873898694,-24.4941169599123,
122.309170126325)) ;
#45672=CARTESIAN_POINT('Ctrl Pts',(-18.7986820358757,-24.3141278795495,
122.033501629842)) ;
#45673=CARTESIAN_POINT('Ctrl Pts',(-18.7366115575641,-24.5041194536396,
122.410711220208)) ;
#45674=CARTESIAN_POINT('Ctrl Pts',(-18.5684608876012,-24.3241303732768,
122.160425707919)) ;
#45675=CARTESIAN_POINT('Ctrl Pts',(-18.5725769314898,-24.5141542521466,
122.543347790697)) ;
#45676=CARTESIAN_POINT('Ctrl Pts',(-18.3634159135229,-24.3341651717837,
122.326219304177)) ;
#45677=CARTESIAN_POINT('Ctrl Pts',(-18.4364059179355,-24.5239991361259,
122.699231885075)) ;
#45678=CARTESIAN_POINT('Ctrl Pts',(-18.1931997744196,-24.3440100557631,
122.521073096174)) ;
#45679=CARTESIAN_POINT('Ctrl Pts',(-18.3275230682562,-24.533984992944,122.878683232876)) ;
#45680=CARTESIAN_POINT('Ctrl Pts',(-18.0570939034257,-24.3539959125811,
122.745386068162)) ;
#45681=CARTESIAN_POINT('Ctrl Pts',(-18.2516769257629,-24.5439198071187,
123.073327761756)) ;
#45682=CARTESIAN_POINT('Ctrl Pts',(-17.9622837121039,-24.3639307267559,
122.988691099202)) ;
#45683=CARTESIAN_POINT('Ctrl Pts',(-18.2104726947077,-24.5539773069041,
123.280683690247)) ;
#45684=CARTESIAN_POINT('Ctrl Pts',(-17.9107758866694,-24.3739882265412,
123.247885388004)) ;
#45685=CARTESIAN_POINT('Ctrl Pts',(-18.2056888743538,-24.5637990653224,
123.487134857633)) ;
#45686=CARTESIAN_POINT('Ctrl Pts',(-17.904793545213,-24.3838099849595,123.505950068629)) ;
#45687=CARTESIAN_POINT('Ctrl Pts',(-18.2371668828863,-24.5738547231064,
123.696162130977)) ;
#45688=CARTESIAN_POINT('Ctrl Pts',(-17.9441385895894,-24.3938656427435,
123.767234420915)) ;
#45689=CARTESIAN_POINT('Ctrl Pts',(-18.3040695591823,-24.5837969052864,
123.894192986261)) ;
#45690=CARTESIAN_POINT('Ctrl Pts',(-18.0277646258523,-24.4038078249235,
124.014774122479)) ;
#45691=CARTESIAN_POINT('Ctrl Pts',(-18.4034039808886,-24.5937021139811,
124.07720850749)) ;
#45692=CARTESIAN_POINT('Ctrl Pts',(-18.1519307759585,-24.4137130336182,
124.243545142332)) ;
#45693=CARTESIAN_POINT('Ctrl Pts',(-18.5348467278453,-24.6037439049435,
124.242401635363)) ;
#45694=CARTESIAN_POINT('Ctrl Pts',(-18.3162322484998,-24.4237548245807,
124.450038000876)) ;
#45695=CARTESIAN_POINT('Ctrl Pts',(-18.6908591823526,-24.6136516794158,
124.380420797567)) ;
#45696=CARTESIAN_POINT('Ctrl Pts',(-18.5112465951366,-24.4336625990529,
124.622564118162)) ;
#45697=CARTESIAN_POINT('Ctrl Pts',(-18.8701202015806,-24.6236631796434,
124.490724089556)) ;
#45698=CARTESIAN_POINT('Ctrl Pts',(-18.7353216882572,-24.4436740992805,
124.760445262885)) ;
#45699=CARTESIAN_POINT('Ctrl Pts',(-19.0663816760572,-24.6336959400361,
124.567979438688)) ;
#45700=CARTESIAN_POINT('Ctrl Pts',(-18.9806475911732,-24.4537068596732,
124.857016709312)) ;
#45701=CARTESIAN_POINT('Ctrl Pts',(-19.2692552137906,-24.643546509171,124.609578863151)) ;
#45702=CARTESIAN_POINT('Ctrl Pts',(-19.2342398512447,-24.4635574288081,
124.909018469813)) ;
#45703=CARTESIAN_POINT('Ctrl Pts',(-19.4791376987757,-24.6535351187009,
124.615797717259)) ;
#45704=CARTESIAN_POINT('Ctrl Pts',(-19.496593073052,-24.473546038338,124.916794312844)) ;
#45705=CARTESIAN_POINT('Ctrl Pts',(-19.6856874087961,-24.663463774725,124.585656540183)) ;
#45706=CARTESIAN_POINT('Ctrl Pts',(-19.7547810174037,-24.4834746943621,
124.879120015881)) ;
#45707=CARTESIAN_POINT('Ctrl Pts',(-19.8851618333618,-24.6734515209028,
124.520055763717)) ;
#45708=CARTESIAN_POINT('Ctrl Pts',(-20.0041249025158,-24.4934624405399,
124.797121058112)) ;
#45709=CARTESIAN_POINT('Ctrl Pts',(-20.0709240901513,-24.6834875098385,
124.420032910437)) ;
#45710=CARTESIAN_POINT('Ctrl Pts',(-20.2363287243684,-24.5034984294756,
124.672094532501)) ;
#45711=CARTESIAN_POINT('Ctrl Pts',(-20.2337420876468,-24.6933423796521,
124.291888982276)) ;
#45712=CARTESIAN_POINT('Ctrl Pts',(-20.4398532893897,-24.5133532992892,
124.511915768883)) ;
#45713=CARTESIAN_POINT('Ctrl Pts',(-20.3740410207416,-24.7033418208939,
124.135384425764)) ;
#45714=CARTESIAN_POINT('Ctrl Pts',(-20.6152286146219,-24.523352740531,124.316286380148)) ;
#45715=CARTESIAN_POINT('Ctrl Pts',(-20.4841026431737,-24.713236895074,123.958818728685)) ;
#45716=CARTESIAN_POINT('Ctrl Pts',(-20.7528077611867,-24.5332478147111,
124.095579716367)) ;
#45717=CARTESIAN_POINT('Ctrl Pts',(-20.5630911584333,-24.7232975509137,
123.762644267269)) ;
#45718=CARTESIAN_POINT('Ctrl Pts',(-20.8515452176625,-24.5433084705508,
123.850362627596)) ;
#45719=CARTESIAN_POINT('Ctrl Pts',(-20.6060224074376,-24.7331464251093,
123.560073880987)) ;
#45720=CARTESIAN_POINT('Ctrl Pts',(-20.90521146566,-24.5531573447464,123.597149046186)) ;
#45721=CARTESIAN_POINT('Ctrl Pts',(-20.6137892692649,-24.7431751370725,
123.349384846586)) ;
#45722=CARTESIAN_POINT('Ctrl Pts',(-20.9149218984342,-24.5631860567097,
123.333787858284)) ;
#45723=CARTESIAN_POINT('Ctrl Pts',(-20.5842846845228,-24.7532045376556,
123.140605694628)) ;
#45724=CARTESIAN_POINT('Ctrl Pts',(-20.8780431867244,-24.5732154572928,
123.072813707619)) ;
#45725=CARTESIAN_POINT('Ctrl Pts',(-20.5206480631986,-24.7630447312725,
122.943761957022)) ;
#45726=CARTESIAN_POINT('Ctrl Pts',(-20.7984988600526,-24.5830556509096,
122.826757371458)) ;
#45727=CARTESIAN_POINT('Ctrl Pts',(-20.4225485419105,-24.7730481538477,
122.757764156564)) ;
#45728=CARTESIAN_POINT('Ctrl Pts',(-20.675875973219,-24.5930590734848,122.594259198633)) ;
#45729=CARTESIAN_POINT('Ctrl Pts',(-20.2937856669965,-24.7830336909408,
122.591919417926)) ;
#45730=CARTESIAN_POINT('Ctrl Pts',(-20.5149236678703,-24.6030446105779,
122.386952011327)) ;
#45731=CARTESIAN_POINT('Ctrl Pts',(-20.1372175607481,-24.7930746954276,
122.450362162771)) ;
#45732=CARTESIAN_POINT('Ctrl Pts',(-20.319214882974,-24.6130856150647,122.210004150072)) ;
#45733=CARTESIAN_POINT('Ctrl Pts',(-19.9620847517272,-24.8029182343688,
122.340090117792)) ;
#45734=CARTESIAN_POINT('Ctrl Pts',(-20.100298824301,-24.6229291540059,122.072161974285)) ;
#45735=CARTESIAN_POINT('Ctrl Pts',(-19.7679204826026,-24.8129032653596,
122.260388804538)) ;
#45736=CARTESIAN_POINT('Ctrl Pts',(-19.8575938757749,-24.6329141849967,
121.972533729906)) ;
#45737=CARTESIAN_POINT('Ctrl Pts',(-19.5637613025099,-24.8228427278816,
122.215721170497)) ;
#45738=CARTESIAN_POINT('Ctrl Pts',(-19.6023947114749,-24.6428536475187,
121.916697509575)) ;
#45739=CARTESIAN_POINT('Ctrl Pts',(-19.3528855208101,-24.8328824601054,
122.207143938468)) ;
#45740=CARTESIAN_POINT('Ctrl Pts',(-19.3388001962216,-24.6528933797425,
121.905974359338)) ;
#45741=CARTESIAN_POINT('Ctrl Pts',(-19.1468393604488,-24.8427706404226,
122.234788301827)) ;
#45742=CARTESIAN_POINT('Ctrl Pts',(-19.0812413725031,-24.6627815600597,
121.940528367606)) ;
#45743=CARTESIAN_POINT('Ctrl Pts',(-18.9465910465543,-24.8527601561251,
122.298052941285)) ;
#45744=CARTESIAN_POINT('Ctrl Pts',(-18.830930339593,-24.6727710757622,122.019607849904)) ;
#45745=CARTESIAN_POINT('Ctrl Pts',(-18.7610210692701,-24.8627187067798,
122.394969542259)) ;
#45746=CARTESIAN_POINT('Ctrl Pts',(-18.5989667873706,-24.6827296264169,
122.140752466296)) ;
#45747=CARTESIAN_POINT('Ctrl Pts',(-18.5957514950734,-24.8726181138848,
122.521477714569)) ;
#45748=CARTESIAN_POINT('Ctrl Pts',(-18.3923783177254,-24.6926290335219,
122.298887165231)) ;
#45749=CARTESIAN_POINT('Ctrl Pts',(-18.4529280511965,-24.8826667003011,
122.677100505805)) ;
#45750=CARTESIAN_POINT('Ctrl Pts',(-18.2138481637525,-24.7026776199382,
122.493414575767)) ;
#45751=CARTESIAN_POINT('Ctrl Pts',(-18.3408505972411,-24.8925595192655,
122.85234593428)) ;
#45752=CARTESIAN_POINT('Ctrl Pts',(-18.0737497675781,-24.7125704389027,
122.712471449112)) ;
#45753=CARTESIAN_POINT('Ctrl Pts',(-18.2595668677293,-24.9026306367953,
123.047801925644)) ;
#45754=CARTESIAN_POINT('Ctrl Pts',(-17.9721440404555,-24.7226415564325,
122.95679058556)) ;
#45755=CARTESIAN_POINT('Ctrl Pts',(-18.2143360447103,-24.9124463307614,
123.249180345051)) ;
#45756=CARTESIAN_POINT('Ctrl Pts',(-17.9156039987701,-24.7324572503985,
123.208514840523)) ;
#45757=CARTESIAN_POINT('Ctrl Pts',(-18.2042126503118,-24.9225127082587,
123.460520176297)) ;
#45758=CARTESIAN_POINT('Ctrl Pts',(-17.9029486725744,-24.7425236278958,
123.472689210429)) ;
#45759=CARTESIAN_POINT('Ctrl Pts',(-18.2305681873623,-24.9324116943406,
123.667004534321)) ;
#45760=CARTESIAN_POINT('Ctrl Pts',(-17.935892095498,-24.7524226139777,123.730795685717)) ;
#45761=CARTESIAN_POINT('Ctrl Pts',(-18.2932377700678,-24.9424658743341,
123.868822725467)) ;
#45762=CARTESIAN_POINT('Ctrl Pts',(-18.0142279454651,-24.7624767939712,
123.983068491379)) ;
#45763=CARTESIAN_POINT('Ctrl Pts',(-18.3880943306794,-24.9523366872668,
124.053444339054)) ;
#45764=CARTESIAN_POINT('Ctrl Pts',(-18.1327982653444,-24.7723476069039,
124.213846997016)) ;
#45765=CARTESIAN_POINT('Ctrl Pts',(-18.5160928318226,-24.9624105881206,
124.222110708763)) ;
#45766=CARTESIAN_POINT('Ctrl Pts',(-18.2927953165878,-24.7824215077577,
124.424680232047)) ;
#45767=CARTESIAN_POINT('Ctrl Pts',(-18.6674180149936,-24.9722307435072,
124.362618007818)) ;
#45768=CARTESIAN_POINT('Ctrl Pts',(-18.4819523062821,-24.7922416631444,
124.600316090913)) ;
#45769=CARTESIAN_POINT('Ctrl Pts',(-18.8452136411496,-24.9823094504595,
124.477780776126)) ;
#45770=CARTESIAN_POINT('Ctrl Pts',(-18.7041959809352,-24.8023203700966,
124.744270009316)) ;
#45771=CARTESIAN_POINT('Ctrl Pts',(-19.0359724593799,-24.9921610389983,
124.558567319872)) ;
#45772=CARTESIAN_POINT('Ctrl Pts',(-18.9426453970189,-24.8121719586354,
124.845254460228)) ;
#45773=CARTESIAN_POINT('Ctrl Pts',(-19.2422734738344,-25.0022341555233,
124.606210580914)) ;
#45774=CARTESIAN_POINT('Ctrl Pts',(-19.200521069137,-24.8222450751604,124.904809172551)) ;
#45775=CARTESIAN_POINT('Ctrl Pts',(-19.4489294427733,-25.0120766726191,
124.617025230768)) ;
#45776=CARTESIAN_POINT('Ctrl Pts',(-19.4588424041164,-24.8320875922562,
124.91832832477)) ;
#45777=CARTESIAN_POINT('Ctrl Pts',(-19.6572595399181,-25.022057134173,124.592142989449)) ;
#45778=CARTESIAN_POINT('Ctrl Pts',(-19.7192553917927,-24.8420680538102,
124.887225976131)) ;
#45779=CARTESIAN_POINT('Ctrl Pts',(-19.858754508053,-25.0320753841638,124.530845580541)) ;
#45780=CARTESIAN_POINT('Ctrl Pts',(-19.9711242826029,-24.8520863038009,
124.810604842072)) ;
#45781=CARTESIAN_POINT('Ctrl Pts',(-20.0442458404208,-25.0419595443576,
124.437141256552)) ;
#45782=CARTESIAN_POINT('Ctrl Pts',(-20.2029896410635,-24.8619704639947,
124.693474375189)) ;
#45783=CARTESIAN_POINT('Ctrl Pts',(-20.2136336533158,-25.0520246913326,
124.310362839137)) ;
#45784=CARTESIAN_POINT('Ctrl Pts',(-20.4147243951242,-24.8720356109697,
124.535001991824)) ;
#45785=CARTESIAN_POINT('Ctrl Pts',(-20.3553327642867,-25.0618665149734,
124.159573795063)) ;
#45786=CARTESIAN_POINT('Ctrl Pts',(-20.5918496186671,-24.8818774346105,
124.346514930548)) ;
#45787=CARTESIAN_POINT('Ctrl Pts',(-20.4713227735349,-25.0718959874342,
123.98349792825)) ;
#45788=CARTESIAN_POINT('Ctrl Pts',(-20.7368372685072,-24.8919069070713,
124.126420308641)) ;
#45789=CARTESIAN_POINT('Ctrl Pts',(-20.5544183696664,-25.0819228426962,
123.789765828092)) ;
#45790=CARTESIAN_POINT('Ctrl Pts',(-20.8407071584653,-24.9019337623334,
123.884255455993)) ;
#45791=CARTESIAN_POINT('Ctrl Pts',(-20.6022129333517,-25.0917660928068,
123.58842207058)) ;
#45792=CARTESIAN_POINT('Ctrl Pts',(-20.9004509562917,-24.9117770124439,
123.632574419147)) ;
#45793=CARTESIAN_POINT('Ctrl Pts',(-20.6148605428865,-25.1018145323899,
123.377557024283)) ;
#45794=CARTESIAN_POINT('Ctrl Pts',(-20.916260611242,-24.9218254520271,123.368993380643)) ;
#45795=CARTESIAN_POINT('Ctrl Pts',(-20.590610957124,-25.1117640266378,123.16979691793)) ;
#45796=CARTESIAN_POINT('Ctrl Pts',(-20.8859488523691,-24.931774946275,123.109292637768)) ;
#45797=CARTESIAN_POINT('Ctrl Pts',(-20.5315027514083,-25.1216718823638,
122.970053451003)) ;
#45798=CARTESIAN_POINT('Ctrl Pts',(-20.812063374515,-24.941682802001,122.85961242254)) ;
#45799=CARTESIAN_POINT('Ctrl Pts',(-20.4370028959412,-25.1317313590138,
122.780884060618)) ;
#45800=CARTESIAN_POINT('Ctrl Pts',(-20.6939388264685,-24.9517422786509,
122.623150935641)) ;
#45801=CARTESIAN_POINT('Ctrl Pts',(-20.3140267459724,-25.1415721684225,
122.614484936629)) ;
#45802=CARTESIAN_POINT('Ctrl Pts',(-20.5402177796958,-24.9615830880596,
122.415150839327)) ;
#45803=CARTESIAN_POINT('Ctrl Pts',(-20.1608696779371,-25.1516343187233,
122.46860151475)) ;
#45804=CARTESIAN_POINT('Ctrl Pts',(-20.3487716521003,-24.9716452383604,
122.232796879525)) ;
#45805=CARTESIAN_POINT('Ctrl Pts',(-19.9874513742878,-25.1615314798458,
122.353608540262)) ;
#45806=CARTESIAN_POINT('Ctrl Pts',(-20.1319979378848,-24.981542399483,122.089055106717)) ;
#45807=CARTESIAN_POINT('Ctrl Pts',(-19.7963375421497,-25.1714626542499,
122.269557911198)) ;
#45808=CARTESIAN_POINT('Ctrl Pts',(-19.8931048762682,-24.991473573887,121.983991783669)) ;
#45809=CARTESIAN_POINT('Ctrl Pts',(-19.5912085972719,-25.1815048579749,
122.219637399699)) ;
#45810=CARTESIAN_POINT('Ctrl Pts',(-19.6366938542377,-25.001515777612,121.921591372385)) ;
#45811=CARTESIAN_POINT('Ctrl Pts',(-19.3837898601191,-25.1913914404053,
122.206149497569)) ;
#45812=CARTESIAN_POINT('Ctrl Pts',(-19.3774193320319,-25.0114023600425,
121.904731667752)) ;
#45813=CARTESIAN_POINT('Ctrl Pts',(-19.174930617181,-25.2013848761537,122.228779671047)) ;
#45814=CARTESIAN_POINT('Ctrl Pts',(-19.116345118076,-25.0213957957908,121.933019786069)) ;
#45815=CARTESIAN_POINT('Ctrl Pts',(-18.9741668937736,-25.2113293445118,
122.287109961351)) ;
#45816=CARTESIAN_POINT('Ctrl Pts',(-18.8653899853733,-25.031340264149,122.0059331557)) ;
#45817=CARTESIAN_POINT('Ctrl Pts',(-18.7862616744613,-25.2212811607574,
122.379130251146)) ;
#45818=CARTESIAN_POINT('Ctrl Pts',(-18.6305081904514,-25.0412920803945,
122.120959221121)) ;
#45819=CARTESIAN_POINT('Ctrl Pts',(-18.6158633692364,-25.2313185968719,
122.503584025425)) ;
#45820=CARTESIAN_POINT('Ctrl Pts',(-18.4175106984375,-25.051329516509,122.276526693865)) ;
#45821=CARTESIAN_POINT('Ctrl Pts',(-18.4717187038832,-25.2412035560482,
122.653303494758)) ;
#45822=CARTESIAN_POINT('Ctrl Pts',(-18.2373294887089,-25.0612144756854,
122.463677159572)) ;
#45823=CARTESIAN_POINT('Ctrl Pts',(-18.3542495988289,-25.2512016742602,
122.827576694392)) ;
#45824=CARTESIAN_POINT('Ctrl Pts',(-18.0904935273236,-25.0712125938973,
122.681519130343)) ;
#45825=CARTESIAN_POINT('Ctrl Pts',(-18.2693324752695,-25.2611226067721,
123.018101116052)) ;
#45826=CARTESIAN_POINT('Ctrl Pts',(-17.9843474113932,-25.0811335264093,
122.919675638714)) ;
#45827=CARTESIAN_POINT('Ctrl Pts',(-18.2181276836119,-25.2711639069942,
123.2228864421)) ;
#45828=CARTESIAN_POINT('Ctrl Pts',(-17.9203421285094,-25.0911748266313,
123.175657289294)) ;
#45829=CARTESIAN_POINT('Ctrl Pts',(-18.203527625728,-25.2810708253842,123.430650481538)) ;
#45830=CARTESIAN_POINT('Ctrl Pts',(-17.9020926498255,-25.1010817450213,
123.435363279085)) ;
#45831=CARTESIAN_POINT('Ctrl Pts',(-18.2246915361504,-25.2910066170932,
123.638458055856)) ;
#45832=CARTESIAN_POINT('Ctrl Pts',(-17.9285484881312,-25.1110175367304,
123.69512331008)) ;
#45833=CARTESIAN_POINT('Ctrl Pts',(-18.2824223938012,-25.3010475116711,
123.841496647617)) ;
#45834=CARTESIAN_POINT('Ctrl Pts',(-18.0007127842541,-25.1210584313083,
123.948921149935)) ;
#45835=CARTESIAN_POINT('Ctrl Pts',(-18.3729909834067,-25.310934713385,124.028599784085)) ;
#45836=CARTESIAN_POINT('Ctrl Pts',(-18.1139247515408,-25.1309456330221,
124.18280063066)) ;
#45837=CARTESIAN_POINT('Ctrl Pts',(-18.4956664931269,-25.3209269811466,
124.19910961797)) ;
#45838=CARTESIAN_POINT('Ctrl Pts',(-18.2672700656794,-25.1409379007837,
124.395937506852)) ;
#45839=CARTESIAN_POINT('Ctrl Pts',(-18.6454852083747,-25.3308755021684,
124.345063822644)) ;
#45840=CARTESIAN_POINT('Ctrl Pts',(-18.4545445264848,-25.1508864218055,
124.578379945049)) ;
#45841=CARTESIAN_POINT('Ctrl Pts',(-18.8179761803924,-25.3408122757461,
124.462875898515)) ;
#45842=CARTESIAN_POINT('Ctrl Pts',(-18.6701593794825,-25.1608231953832,
124.72564450551)) ;
#45843=CARTESIAN_POINT('Ctrl Pts',(-19.0091199998643,-25.3507953238871,
124.549608305468)) ;
#45844=CARTESIAN_POINT('Ctrl Pts',(-18.9090898746252,-25.1708062435242,
124.834059046402)) ;
#45845=CARTESIAN_POINT('Ctrl Pts',(-19.2137039022557,-25.3608390314972,
124.601767255972)) ;
#45846=CARTESIAN_POINT('Ctrl Pts',(-19.1648198261409,-25.1808499511343,
124.899256681723)) ;
#45847=CARTESIAN_POINT('Ctrl Pts',(-19.4197410435178,-25.3706677246505,
124.617749119944)) ;
#45848=CARTESIAN_POINT('Ctrl Pts',(-19.4223677819913,-25.1906786442876,
124.919232914373)) ;
#45849=CARTESIAN_POINT('Ctrl Pts',(-19.6305293861476,-25.3807424737799,
124.597364532467)) ;
#45850=CARTESIAN_POINT('Ctrl Pts',(-19.6858526790546,-25.200753393417,124.893750955826)) ;
#45851=CARTESIAN_POINT('Ctrl Pts',(-19.8303729849827,-25.3906077995755,
124.541808861825)) ;
#45852=CARTESIAN_POINT('Ctrl Pts',(-19.9356579462158,-25.2106187192126,
124.824304856564)) ;
#45853=CARTESIAN_POINT('Ctrl Pts',(-20.0207155288672,-25.4006299739324,
124.451476082817)) ;
#45854=CARTESIAN_POINT('Ctrl Pts',(-20.173585469303,-25.2206408935695,124.711387601586)) ;
#45855=CARTESIAN_POINT('Ctrl Pts',(-20.1922659082655,-25.4106560271393,
124.328983469291)) ;
#45856=CARTESIAN_POINT('Ctrl Pts',(-20.3880226560733,-25.2306669467765,
124.558270853384)) ;
#45857=CARTESIAN_POINT('Ctrl Pts',(-20.3376209909237,-25.4205097239856,
124.181407992117)) ;
#45858=CARTESIAN_POINT('Ctrl Pts',(-20.5697163878782,-25.2405206436227,
124.373799671678)) ;
#45859=CARTESIAN_POINT('Ctrl Pts',(-20.4569372871272,-25.4304691287386,
124.009344969333)) ;
#45860=CARTESIAN_POINT('Ctrl Pts',(-20.7188606913848,-25.2504800483757,
124.15871963452)) ;
#45861=CARTESIAN_POINT('Ctrl Pts',(-20.5449097818086,-25.4405073744435,
123.817532980503)) ;
#45862=CARTESIAN_POINT('Ctrl Pts',(-20.8288249195141,-25.2605182940806,
123.91895416316)) ;
#45863=CARTESIAN_POINT('Ctrl Pts',(-20.5977398559491,-25.4503815586055,
123.616753729714)) ;
#45864=CARTESIAN_POINT('Ctrl Pts',(-20.8948612313139,-25.2703924782426,
123.667978712676)) ;
#45865=CARTESIAN_POINT('Ctrl Pts',(-20.6152318947396,-25.4604513417434,
123.405808054371)) ;
#45866=CARTESIAN_POINT('Ctrl Pts',(-20.9167246661195,-25.2804622613806,
123.404296836379)) ;
#45867=CARTESIAN_POINT('Ctrl Pts',(-20.5963934662247,-25.4702845967642,
123.199925169976)) ;
#45868=CARTESIAN_POINT('Ctrl Pts',(-20.8931748950452,-25.2902955164013,
123.146942101532)) ;
#45869=CARTESIAN_POINT('Ctrl Pts',(-20.5415866211297,-25.4803150228959,
122.99630793319)) ;
#45870=CARTESIAN_POINT('Ctrl Pts',(-20.824664603496,-25.300325942533,122.892421113422)) ;
#45871=CARTESIAN_POINT('Ctrl Pts',(-20.4516839654255,-25.4903466350829,
122.805521136802)) ;
#45872=CARTESIAN_POINT('Ctrl Pts',(-20.7122848539056,-25.31035755472,122.653938383803)) ;
#45873=CARTESIAN_POINT('Ctrl Pts',(-20.3328358727724,-25.5001763319375,
122.636482789407)) ;
#45874=CARTESIAN_POINT('Ctrl Pts',(-20.5637225648046,-25.3201872515746,
122.442640422475)) ;
#45875=CARTESIAN_POINT('Ctrl Pts',(-20.1844921702679,-25.51016577384,122.487819824173)) ;
#45876=CARTESIAN_POINT('Ctrl Pts',(-20.3782914259255,-25.3301766934771,
122.2568129731)) ;
#45877=CARTESIAN_POINT('Ctrl Pts',(-20.0113511337868,-25.5202096658556,
122.366957918595)) ;
#45878=CARTESIAN_POINT('Ctrl Pts',(-20.1618642262399,-25.3402205854928,
122.105737145019)) ;
#45879=CARTESIAN_POINT('Ctrl Pts',(-19.8242733803076,-25.5300312276249,
122.279578448375)) ;
#45880=CARTESIAN_POINT('Ctrl Pts',(-19.9280150892264,-25.350042147262,121.996514020556)) ;
#45881=CARTESIAN_POINT('Ctrl Pts',(-19.6206530982633,-25.5400667992491,
122.2243313612)) ;
#45882=CARTESIAN_POINT('Ctrl Pts',(-19.6734892886853,-25.3600777188862,
121.927457195706)) ;
#45883=CARTESIAN_POINT('Ctrl Pts',(-19.4106109576734,-25.5500960735309,
122.205921274925)) ;
#45884=CARTESIAN_POINT('Ctrl Pts',(-19.4109364974854,-25.370106993168,121.904446478748)) ;
#45885=CARTESIAN_POINT('Ctrl Pts',(-19.2046030647571,-25.5599299106495,
122.22335172287)) ;
#45886=CARTESIAN_POINT('Ctrl Pts',(-19.153425698316,-25.3799408302867,121.92623667871)) ;
#45887=CARTESIAN_POINT('Ctrl Pts',(-19.000259823004,-25.5699823067377,122.277212320983)) ;
#45888=CARTESIAN_POINT('Ctrl Pts',(-18.8979973838901,-25.3899932263748,
121.99356443242)) ;
#45889=CARTESIAN_POINT('Ctrl Pts',(-18.8106744902198,-25.5799190736882,
122.364971233025)) ;
#45890=CARTESIAN_POINT('Ctrl Pts',(-18.6610161340933,-25.3999299933253,
122.103265136597)) ;
#45891=CARTESIAN_POINT('Ctrl Pts',(-18.6389522732557,-25.5898533086675,
122.483834336028)) ;
#45892=CARTESIAN_POINT('Ctrl Pts',(-18.4463642084405,-25.4098642283046,
122.251846102408)) ;
#45893=CARTESIAN_POINT('Ctrl Pts',(-18.4892297183612,-25.5998770719943,
122.632124416292)) ;
#45894=CARTESIAN_POINT('Ctrl Pts',(-18.2592125481551,-25.4198879916314,
122.437210228712)) ;
#45895=CARTESIAN_POINT('Ctrl Pts',(-18.3690729527359,-25.6097634133789,
122.801712077461)) ;
#45896=CARTESIAN_POINT('Ctrl Pts',(-18.1090179641426,-25.429774333016,122.649196677396)) ;
#45897=CARTESIAN_POINT('Ctrl Pts',(-18.2788188736161,-25.6197524621459,
122.991336888981)) ;
#45898=CARTESIAN_POINT('Ctrl Pts',(-17.9962023976865,-25.439763381783,122.886228834323)) ;
#45899=CARTESIAN_POINT('Ctrl Pts',(-18.2229938244163,-25.6297936828433,
123.194918820965)) ;
#45900=CARTESIAN_POINT('Ctrl Pts',(-17.92642324804,-25.4498046024804,123.140706746069)) ;
#45901=CARTESIAN_POINT('Ctrl Pts',(-18.2034358522084,-25.6396263230212,
123.400700722428)) ;
#45902=CARTESIAN_POINT('Ctrl Pts',(-17.9019779830715,-25.4596372426583,
123.397935296118)) ;
#45903=CARTESIAN_POINT('Ctrl Pts',(-18.2195753607672,-25.6496202523291,
123.610182629394)) ;
#45904=CARTESIAN_POINT('Ctrl Pts',(-17.9221548130397,-25.4696311719663,
123.659787613403)) ;
#45905=CARTESIAN_POINT('Ctrl Pts',(-18.2724604743426,-25.6596494600097,
123.814289690547)) ;
#45906=CARTESIAN_POINT('Ctrl Pts',(-17.9882634627547,-25.4796603796468,
123.914920831953)) ;
#45907=CARTESIAN_POINT('Ctrl Pts',(-18.358339643957,-25.6695252717138,124.003328990778)) ;
#45908=CARTESIAN_POINT('Ctrl Pts',(-18.095614902813,-25.4895361913509,124.151219574805)) ;
#45909=CARTESIAN_POINT('Ctrl Pts',(-18.4769919261622,-25.6795244986852,
124.176823257226)) ;
#45910=CARTESIAN_POINT('Ctrl Pts',(-18.243932354423,-25.4995354183223,124.368086107195)) ;
#45911=CARTESIAN_POINT('Ctrl Pts',(-18.6225453670208,-25.6894339798409,
124.325912667589)) ;
#45912=CARTESIAN_POINT('Ctrl Pts',(-18.4258762775159,-25.509444899478,124.554446462771)) ;
#45913=CARTESIAN_POINT('Ctrl Pts',(-18.7942023877807,-25.6994872101418,
124.449174674582)) ;
#45914=CARTESIAN_POINT('Ctrl Pts',(-18.6404489287507,-25.5194981297789,
124.708521879958)) ;
#45915=CARTESIAN_POINT('Ctrl Pts',(-18.9811834854639,-25.7093578266928,
124.539201485248)) ;
#45916=CARTESIAN_POINT('Ctrl Pts',(-18.8741769469546,-25.52936874633,124.821053391255)) ;
#45917=CARTESIAN_POINT('Ctrl Pts',(-19.1838697790237,-25.7193794884249,
124.596699644364)) ;
#45918=CARTESIAN_POINT('Ctrl Pts',(-19.127535526737,-25.539390408062,124.892923586668)) ;
#45919=CARTESIAN_POINT('Ctrl Pts',(-19.3935471693339,-25.729402301606,124.617654797258)) ;
#45920=CARTESIAN_POINT('Ctrl Pts',(-19.3896325300281,-25.5494132212431,
124.919115026202)) ;
#45921=CARTESIAN_POINT('Ctrl Pts',(-19.6004203943415,-25.7392694660659,
124.60247790701)) ;
#45922=CARTESIAN_POINT('Ctrl Pts',(-19.6482244565105,-25.5592803857031,
124.900141299359)) ;
#45923=CARTESIAN_POINT('Ctrl Pts',(-19.804222528808,-25.7492629082859,124.551424075459)) ;
#45924=CARTESIAN_POINT('Ctrl Pts',(-19.902976585568,-25.569273827923,124.83632140457)) ;
#45925=CARTESIAN_POINT('Ctrl Pts',(-19.9966241110481,-25.7592945818862,
124.465058729289)) ;
#45926=CARTESIAN_POINT('Ctrl Pts',(-20.1434775002714,-25.5793055015233,
124.728362358273)) ;
#45927=CARTESIAN_POINT('Ctrl Pts',(-20.1684200868147,-25.7691610169992,
124.348807750651)) ;
#45928=CARTESIAN_POINT('Ctrl Pts',(-20.3582214202011,-25.5891719366363,
124.583046155646)) ;
#45929=CARTESIAN_POINT('Ctrl Pts',(-20.3194620562051,-25.7791484675323,
124.202992595232)) ;
#45930=CARTESIAN_POINT('Ctrl Pts',(-20.5470220993217,-25.5991593871694,
124.400775187836)) ;
#45931=CARTESIAN_POINT('Ctrl Pts',(-20.4424893830337,-25.7890933973602,
124.033909844264)) ;
#45932=CARTESIAN_POINT('Ctrl Pts',(-20.7008042109663,-25.6091043169973,
124.189419968421)) ;
#45933=CARTESIAN_POINT('Ctrl Pts',(-20.5350834451132,-25.7991382924153,
123.844138661879)) ;
#45934=CARTESIAN_POINT('Ctrl Pts',(-20.8165443609091,-25.6191492120525,
123.952204828847)) ;
#45935=CARTESIAN_POINT('Ctrl Pts',(-20.5924455699357,-25.8090003541012,
123.64488433114)) ;
#45936=CARTESIAN_POINT('Ctrl Pts',(-20.8882445301737,-25.6290112737383,
123.70313575114)) ;
#45937=CARTESIAN_POINT('Ctrl Pts',(-20.6150418051958,-25.818992076888,123.436062409259)) ;
#45938=CARTESIAN_POINT('Ctrl Pts',(-20.9164870894924,-25.6390029965252,
123.442107956851)) ;
#45939=CARTESIAN_POINT('Ctrl Pts',(-20.6010425706833,-25.828924291128,123.22772327375)) ;
#45940=CARTESIAN_POINT('Ctrl Pts',(-20.8989852870473,-25.6489352107651,
123.181683998695)) ;
#45941=CARTESIAN_POINT('Ctrl Pts',(-20.5515128182878,-25.8388636096937,
123.024716518231)) ;
#45942=CARTESIAN_POINT('Ctrl Pts',(-20.8370703423436,-25.6588745293309,
122.927926047669)) ;
#45943=CARTESIAN_POINT('Ctrl Pts',(-20.4664264572267,-25.8489077844696,
122.831461041933)) ;
#45944=CARTESIAN_POINT('Ctrl Pts',(-20.7307098426691,-25.6689187041067,
122.686357803622)) ;
#45945=CARTESIAN_POINT('Ctrl Pts',(-20.3511977884892,-25.8587783385346,
122.658884676041)) ;
#45946=CARTESIAN_POINT('Ctrl Pts',(-20.5866715410215,-25.6787892581717,
122.47063867262)) ;
#45947=CARTESIAN_POINT('Ctrl Pts',(-20.2068205658345,-25.8687433208888,
122.507083215677)) ;
#45948=CARTESIAN_POINT('Ctrl Pts',(-20.4061979028758,-25.6887542405259,
122.280888722177)) ;
#45949=CARTESIAN_POINT('Ctrl Pts',(-20.0369803709032,-25.8787740237786,
122.382099598688)) ;
#45950=CARTESIAN_POINT('Ctrl Pts',(-20.1938959519348,-25.6987849434157,
122.124661424676)) ;
#45951=CARTESIAN_POINT('Ctrl Pts',(-19.8507320191725,-25.8886663638038,
122.289510710408)) ;
#45952=CARTESIAN_POINT('Ctrl Pts',(-19.9610841220414,-25.7086772834409,
122.008927766554)) ;
#45953=CARTESIAN_POINT('Ctrl Pts',(-19.6480507991876,-25.8987195969637,
122.229703855428)) ;
#45954=CARTESIAN_POINT('Ctrl Pts',(-19.7077317559287,-25.7187305166009,
121.934171888619)) ;
#45955=CARTESIAN_POINT('Ctrl Pts',(-19.4416056541742,-25.9086008414405,
122.206269923725)) ;
#45956=CARTESIAN_POINT('Ctrl Pts',(-19.4496748815431,-25.7286117610776,
121.904882259363)) ;
#45957=CARTESIAN_POINT('Ctrl Pts',(-19.2311053037005,-25.9186339623115,
122.219073769285)) ;
#45958=CARTESIAN_POINT('Ctrl Pts',(-19.1865495494831,-25.7386448819486,
121.920889891667)) ;
#45959=CARTESIAN_POINT('Ctrl Pts',(-19.0290124695695,-25.9285151725866,
122.267326061068)) ;
#45960=CARTESIAN_POINT('Ctrl Pts',(-18.933934095788,-25.7485260922237,121.981208015015)) ;
#45961=CARTESIAN_POINT('Ctrl Pts',(-18.8349223161673,-25.9385772483559,
122.351365482574)) ;
#45962=CARTESIAN_POINT('Ctrl Pts',(-18.6913224502721,-25.758588167993,122.086259918764)) ;
#45963=CARTESIAN_POINT('Ctrl Pts',(-18.6618773393018,-25.9484343067377,
122.465428901543)) ;
#45964=CARTESIAN_POINT('Ctrl Pts',(-18.4750177696445,-25.7684452263748,
122.228841554689)) ;
#45965=CARTESIAN_POINT('Ctrl Pts',(-18.508920686306,-25.9584288620267,122.609440179343)) ;
#45966=CARTESIAN_POINT('Ctrl Pts',(-18.2838238477272,-25.7784397816638,
122.408857735709)) ;
#45967=CARTESIAN_POINT('Ctrl Pts',(-18.3840592104564,-25.9683547495622,
122.776670958682)) ;
#45968=CARTESIAN_POINT('Ctrl Pts',(-18.1277492566093,-25.7883656691993,
122.617897877619)) ;
#45969=CARTESIAN_POINT('Ctrl Pts',(-18.2891587151755,-25.9783797695574,
122.964835760839)) ;
#45970=CARTESIAN_POINT('Ctrl Pts',(-18.0091260993972,-25.7983906891946,
122.853105228335)) ;
#45971=CARTESIAN_POINT('Ctrl Pts',(-18.2290682932492,-25.9882771466611,
123.164050381415)) ;
#45972=CARTESIAN_POINT('Ctrl Pts',(-17.9340157762588,-25.8082880662982,
123.102124235181)) ;
#45973=CARTESIAN_POINT('Ctrl Pts',(-18.2037946806714,-25.998267383742,123.3725562714)) ;
#45974=CARTESIAN_POINT('Ctrl Pts',(-17.9024264992633,-25.8182783033791,
123.362756958186)) ;
#45975=CARTESIAN_POINT('Ctrl Pts',(-18.2155658880432,-26.0083039965508,
123.583225928318)) ;
#45976=CARTESIAN_POINT('Ctrl Pts',(-17.9171433202812,-25.8283149161879,
123.62609402293)) ;
#45977=CARTESIAN_POINT('Ctrl Pts',(-18.2625157876823,-26.0181538799688,
123.784916905059)) ;
#45978=CARTESIAN_POINT('Ctrl Pts',(-17.9758333009536,-25.8381647996059,
123.878206838358)) ;
#45979=CARTESIAN_POINT('Ctrl Pts',(-18.3446404620089,-26.0281574968712,
123.978504100519)) ;
#45980=CARTESIAN_POINT('Ctrl Pts',(-18.0784917995666,-25.8481684165084,
124.120189945079)) ;
#45981=CARTESIAN_POINT('Ctrl Pts',(-18.4590946254507,-26.0381469086364,
124.154624318019)) ;
#45982=CARTESIAN_POINT('Ctrl Pts',(-18.2215613397651,-25.8581578282735,
124.340338256903)) ;
#45983=CARTESIAN_POINT('Ctrl Pts',(-18.6028685076964,-26.0481656699812,
124.308517074879)) ;
#45984=CARTESIAN_POINT('Ctrl Pts',(-18.4012825635189,-25.8681765896183,
124.532704279284)) ;
#45985=CARTESIAN_POINT('Ctrl Pts',(-18.8247544491437,-26.0613843453623,
124.475917456974)) ;
#45986=CARTESIAN_POINT('Ctrl Pts',(-18.6786331146531,-25.8813952649994,
124.7419424)) ;
#45987=CARTESIAN_POINT('Ctrl Pts',(-19.0869231326057,-26.074694652607,124.582399606467)) ;
#45988=CARTESIAN_POINT('Ctrl Pts',(-19.0063037436624,-25.8947055722441,
124.875037990649)) ;
#45989=CARTESIAN_POINT('Ctrl Pts',(-19.363072798974,-26.087932318833,124.616808325891)) ;
#45990=CARTESIAN_POINT('Ctrl Pts',(-19.3515492793032,-25.9079432384701,
124.918059062423)) ;
#45991=CARTESIAN_POINT('Ctrl Pts',(-19.5713918157783,-26.0978520142437,
124.606935546831)) ;
#45992=CARTESIAN_POINT('Ctrl Pts',(-19.6119358669547,-25.9178629338808,
124.905712873478)) ;
#45993=CARTESIAN_POINT('Ctrl Pts',(-19.7774861802108,-26.1079048812422,
124.560193148227)) ;
#45994=CARTESIAN_POINT('Ctrl Pts',(-19.8695568706956,-25.9279158008794,
124.847282646854)) ;
#45995=CARTESIAN_POINT('Ctrl Pts',(-19.9686281474796,-26.1177602895715,
124.480186051397)) ;
#45996=CARTESIAN_POINT('Ctrl Pts',(-20.1084811470634,-25.9377712092086,
124.747272818571)) ;
#45997=CARTESIAN_POINT('Ctrl Pts',(-20.14637377885,-26.1277989212481,124.366438520996)) ;
#45998=CARTESIAN_POINT('Ctrl Pts',(-20.3306652047621,-25.9478098408852,
124.60508116567)) ;
#45999=CARTESIAN_POINT('Ctrl Pts',(-20.3519626171017,-26.1411011035151,
124.176812384291)) ;
#46000=CARTESIAN_POINT('Ctrl Pts',(-20.5876341488702,-25.9611120231522,
124.368071353018)) ;
#46001=CARTESIAN_POINT('Ctrl Pts',(-20.5406207798638,-26.157646116598,123.879908726874)) ;
#46002=CARTESIAN_POINT('Ctrl Pts',(-20.8234715239028,-25.9776570362351,
123.996893725382)) ;
#46003=CARTESIAN_POINT('Ctrl Pts',(-20.6172088047157,-26.1742981326742,
123.534214772238)) ;
#46004=CARTESIAN_POINT('Ctrl Pts',(-20.9191905979447,-25.9943090523113,
123.56485434143)) ;
#46005=CARTESIAN_POINT('Ctrl Pts',(-20.6051217054238,-26.1875212235794,
123.256506578879)) ;
#46006=CARTESIAN_POINT('Ctrl Pts',(-20.9040855806235,-26.0075321432166,
123.217655815596)) ;
#46007=CARTESIAN_POINT('Ctrl Pts',(-20.5603924279369,-26.1974821831388,
123.05192147308)) ;
#46008=CARTESIAN_POINT('Ctrl Pts',(-20.8481710288913,-26.0174931027759,
122.961938491828)) ;
#46009=CARTESIAN_POINT('Ctrl Pts',(-20.4800725687243,-26.2075069798899,
122.857083849691)) ;
#46010=CARTESIAN_POINT('Ctrl Pts',(-20.7477672743641,-26.027517899527,122.718386742879)) ;
#46011=CARTESIAN_POINT('Ctrl Pts',(-20.3313987181556,-26.2207314272857,
122.62210740137)) ;
#46012=CARTESIAN_POINT('Ctrl Pts',(-20.561933381812,-26.0407423469228,122.424679164752)) ;
#46013=CARTESIAN_POINT('Ctrl Pts',(-20.0717140768469,-26.2373652119848,
122.382085717408)) ;
#46014=CARTESIAN_POINT('Ctrl Pts',(-20.2373134506599,-26.0573761316219,
122.124643357412)) ;
#46015=CARTESIAN_POINT('Ctrl Pts',(-19.6815099293272,-26.2572678787097,
122.218198924247)) ;
#46016=CARTESIAN_POINT('Ctrl Pts',(-19.7495611853889,-26.0772787983468,
121.919792632271)) ;
#46017=CARTESIAN_POINT('Ctrl Pts',(-19.2589510713564,-26.2771681064916,
122.196756051272)) ;
#46018=CARTESIAN_POINT('Ctrl Pts',(-19.22136228124,-26.0971790261287,121.892991857284)) ;
#46019=CARTESIAN_POINT('Ctrl Pts',(-18.8539777559444,-26.2970855940231,
122.320631928225)) ;
#46020=CARTESIAN_POINT('Ctrl Pts',(-18.715147674176,-26.1170965136602,122.047840068895)) ;
#46021=CARTESIAN_POINT('Ctrl Pts',(-18.5152044782925,-26.31701511984,122.575227475119)) ;
#46022=CARTESIAN_POINT('Ctrl Pts',(-18.2916834899083,-26.1370260394771,
122.366086543322)) ;
#46023=CARTESIAN_POINT('Ctrl Pts',(-18.2833320361407,-26.3369773877262,
122.930774152276)) ;
#46024=CARTESIAN_POINT('Ctrl Pts',(-18.0018457091614,-26.1569883073634,
122.810521281011)) ;
#46025=CARTESIAN_POINT('Ctrl Pts',(-18.187043146482,-26.3568675826784,123.342528444568)) ;
#46026=CARTESIAN_POINT('Ctrl Pts',(-17.8814876928622,-26.1768785023156,
123.325213587121)) ;
#46027=CARTESIAN_POINT('Ctrl Pts',(-18.2360005587426,-26.3767578274247,
123.762699469235)) ;
#46028=CARTESIAN_POINT('Ctrl Pts',(-17.942686360803,-26.1967687470618,123.850425839036)) ;
#46029=CARTESIAN_POINT('Ctrl Pts',(-18.4278756911333,-26.3968321999872,
124.143912754518)) ;
#46030=CARTESIAN_POINT('Ctrl Pts',(-18.182532872639,-26.2168431196243,124.326942241085)) ;
#46031=CARTESIAN_POINT('Ctrl Pts',(-18.7338400806782,-26.4166175773475,
124.432727082962)) ;
#46032=CARTESIAN_POINT('Ctrl Pts',(-18.5649877790472,-26.2366284969846,
124.687956672163)) ;
#46033=CARTESIAN_POINT('Ctrl Pts',(-19.1228257813227,-26.4365794514146,
124.602461953777)) ;
#46034=CARTESIAN_POINT('Ctrl Pts',(-19.0512197803277,-26.2565903710517,
124.900124064153)) ;
#46035=CARTESIAN_POINT('Ctrl Pts',(-19.5468805261724,-26.4565594269051,
124.628280549384)) ;
#46036=CARTESIAN_POINT('Ctrl Pts',(-19.5812880978387,-26.2765703465422,
124.932395779744)) ;
#46037=CARTESIAN_POINT('Ctrl Pts',(-19.9511224656437,-26.476371856783,124.509636259826)) ;
#46038=CARTESIAN_POINT('Ctrl Pts',(-20.0865875254388,-26.2963827764202,
124.784090581285)) ;
#46039=CARTESIAN_POINT('Ctrl Pts',(-20.2937255390238,-26.4963519648733,
124.258562719939)) ;
#46040=CARTESIAN_POINT('Ctrl Pts',(-20.5148410357087,-26.3163628845105,
124.470248873448)) ;
#46041=CARTESIAN_POINT('Ctrl Pts',(-20.5290130856317,-26.5162463484706,
123.906914863893)) ;
#46042=CARTESIAN_POINT('Ctrl Pts',(-20.8089496480924,-26.3362572681077,
124.030690459046)) ;
#46043=CARTESIAN_POINT('Ctrl Pts',(-20.6306703899268,-26.5361732764478,
123.495687774504)) ;
#46044=CARTESIAN_POINT('Ctrl Pts',(-20.9360216455939,-26.3561841960849,
123.516657893152)) ;
#46045=CARTESIAN_POINT('Ctrl Pts',(-20.58650883794,-26.556068133749,123.074882964739)) ;
#46046=CARTESIAN_POINT('Ctrl Pts',(-20.8808211228342,-26.3760790533862,
122.990653193015)) ;
#46047=CARTESIAN_POINT('Ctrl Pts',(-20.3997314232741,-26.5761073273527,
122.691961278104)) ;
#46048=CARTESIAN_POINT('Ctrl Pts',(-20.647350202661,-26.3961182469898,122.512000068605)) ;
#46049=CARTESIAN_POINT('Ctrl Pts',(-20.0964143874877,-26.5959472952634,
122.39871350997)) ;
#46050=CARTESIAN_POINT('Ctrl Pts',(-20.2682064549475,-26.4159582149006,
122.145440895336)) ;
#46051=CARTESIAN_POINT('Ctrl Pts',(-19.7103017728837,-26.6158621122275,
122.224956806707)) ;
#46052=CARTESIAN_POINT('Ctrl Pts',(-19.7855675978371,-26.4358730318646,
121.928243360252)) ;
#46053=CARTESIAN_POINT('Ctrl Pts',(-19.2874660199691,-26.6358043576238,
122.193640512695)) ;
#46054=CARTESIAN_POINT('Ctrl Pts',(-19.2570238059739,-26.4558152772609,
121.889095738746)) ;
#46055=CARTESIAN_POINT('Ctrl Pts',(-18.8804463278445,-26.6556764057383,
122.30743483587)) ;
#46056=CARTESIAN_POINT('Ctrl Pts',(-18.748249738879,-26.4756873253754,122.031335489932)) ;
#46057=CARTESIAN_POINT('Ctrl Pts',(-18.534656096257,-26.6756874706924,122.555130633679)) ;
#46058=CARTESIAN_POINT('Ctrl Pts',(-18.3160101803626,-26.4956983903295,
122.340952921604)) ;
#46059=CARTESIAN_POINT('Ctrl Pts',(-18.2958118938891,-26.695498994996,122.902353695436)) ;
#46060=CARTESIAN_POINT('Ctrl Pts',(-18.0174531568864,-26.5155099146331,
122.774978345867)) ;
#46061=CARTESIAN_POINT('Ctrl Pts',(-18.1886180442207,-26.7155942069594,
123.315793755655)) ;
#46062=CARTESIAN_POINT('Ctrl Pts',(-17.883457283048,-26.5356051265965,123.29177843999)) ;
#46063=CARTESIAN_POINT('Ctrl Pts',(-18.2284182206714,-26.7353749308792,
123.734667026007)) ;
#46064=CARTESIAN_POINT('Ctrl Pts',(-17.9332038026506,-26.5553858505163,
123.815368387734)) ;
#46065=CARTESIAN_POINT('Ctrl Pts',(-18.4096610154177,-26.755366006522,124.118979626269)) ;
#46066=CARTESIAN_POINT('Ctrl Pts',(-18.1597535329976,-26.5753769261591,
124.295760856938)) ;
#46067=CARTESIAN_POINT('Ctrl Pts',(-18.7099242034501,-26.775247945565,124.416730191879)) ;
#46068=CARTESIAN_POINT('Ctrl Pts',(-18.5350790245251,-26.5952588652021,
124.667951356014)) ;
#46069=CARTESIAN_POINT('Ctrl Pts',(-19.0947640893078,-26.7952005500682,
124.595125233846)) ;
#46070=CARTESIAN_POINT('Ctrl Pts',(-19.0161267182173,-26.6152114697054,
124.89094908574)) ;
#46071=CARTESIAN_POINT('Ctrl Pts',(-19.5163545803771,-26.8150994187989,
124.631394180349)) ;
#46072=CARTESIAN_POINT('Ctrl Pts',(-19.5431138580635,-26.635110338436,124.936289536443)) ;
#46073=CARTESIAN_POINT('Ctrl Pts',(-19.9249223900067,-26.8349928186085,
124.522185577163)) ;
#46074=CARTESIAN_POINT('Ctrl Pts',(-20.0538241489415,-26.6550037382456,
124.799784245693)) ;
#46075=CARTESIAN_POINT('Ctrl Pts',(-20.2724780813472,-26.8549019494485,
124.28036241543)) ;
#46076=CARTESIAN_POINT('Ctrl Pts',(-20.4882718449817,-26.6749128690856,
124.497507103209)) ;
#46077=CARTESIAN_POINT('Ctrl Pts',(-20.5176077328645,-26.8749340492121,
123.93208451665)) ;
#46078=CARTESIAN_POINT('Ctrl Pts',(-20.7946862216762,-26.6949449688492,
124.062171882771)) ;
#46079=CARTESIAN_POINT('Ctrl Pts',(-20.6098098899142,-26.8914661223815,
123.592826429201)) ;
#46080=CARTESIAN_POINT('Ctrl Pts',(-20.9099487231253,-26.7114770420187,
123.638071483004)) ;
#46081=CARTESIAN_POINT('Ctrl Pts',(-20.6110911401444,-26.9048014629875,
123.312495899499)) ;
#46082=CARTESIAN_POINT('Ctrl Pts',(-20.9115489477632,-26.7248123826246,
123.287684923675)) ;
#46083=CARTESIAN_POINT('Ctrl Pts',(-20.5764556782728,-26.9146440215272,
123.108474267684)) ;
#46084=CARTESIAN_POINT('Ctrl Pts',(-20.8682561091955,-26.7346549411643,
123.032650001442)) ;
#46085=CARTESIAN_POINT('Ctrl Pts',(-20.505658826445,-26.9246959283771,122.909381601415)) ;
#46086=CARTESIAN_POINT('Ctrl Pts',(-20.77977083026,-26.7447068480142,122.78379500435)) ;
#46087=CARTESIAN_POINT('Ctrl Pts',(-20.3681524800132,-26.937944442768,122.66718118586)) ;
#46088=CARTESIAN_POINT('Ctrl Pts',(-20.6078481493321,-26.7579553624051,
122.480989791618)) ;
#46089=CARTESIAN_POINT('Ctrl Pts',(-20.1207621070725,-26.9545436177157,
122.415419343604)) ;
#46090=CARTESIAN_POINT('Ctrl Pts',(-20.2986718809481,-26.7745545373529,
122.166348506659)) ;
#46091=CARTESIAN_POINT('Ctrl Pts',(-19.8026232747545,-26.9711324035108,
122.26320952748)) ;
#46092=CARTESIAN_POINT('Ctrl Pts',(-19.9009478345017,-26.7911433231479,
121.976048097058)) ;
#46093=CARTESIAN_POINT('Ctrl Pts',(-19.5282752383854,-26.9844082198528,
122.211739570841)) ;
#46094=CARTESIAN_POINT('Ctrl Pts',(-19.5580496300445,-26.8044191394899,
121.911724128209)) ;
#46095=CARTESIAN_POINT('Ctrl Pts',(-19.318603845964,-26.9943820706466,122.209154533502)) ;
#46096=CARTESIAN_POINT('Ctrl Pts',(-19.2959531359205,-26.8143929902837,
121.908486613091)) ;
#46097=CARTESIAN_POINT('Ctrl Pts',(-19.1105694524777,-27.004411102739,122.243420895193)) ;
#46098=CARTESIAN_POINT('Ctrl Pts',(-19.0359115386452,-26.8244220223761,
121.951317775132)) ;
#46099=CARTESIAN_POINT('Ctrl Pts',(-18.9143115037935,-27.0143012282409,
122.3121202507)) ;
#46100=CARTESIAN_POINT('Ctrl Pts',(-18.7905877643252,-26.834312147878,122.037189062032)) ;
#46101=CARTESIAN_POINT('Ctrl Pts',(-18.730980558228,-27.0242937065124,122.414640859144)) ;
#46102=CARTESIAN_POINT('Ctrl Pts',(-18.5614228030226,-26.8443046261495,
122.165337470072)) ;
#46103=CARTESIAN_POINT('Ctrl Pts',(-18.5687919015397,-27.0342449216098,
122.546836923164)) ;
#46104=CARTESIAN_POINT('Ctrl Pts',(-18.3586851596353,-26.8542558412469,
122.330580371171)) ;
#46105=CARTESIAN_POINT('Ctrl Pts',(-18.4308500276103,-27.0442934233648,
122.706804310669)) ;
#46106=CARTESIAN_POINT('Ctrl Pts',(-18.1862556413636,-26.8643043430019,
122.530537857795)) ;
#46107=CARTESIAN_POINT('Ctrl Pts',(-18.324778682574,-27.0541347729816,122.884464775646)) ;
#46108=CARTESIAN_POINT('Ctrl Pts',(-18.0536640724743,-26.8741456926187,
122.752611956706)) ;
#46109=CARTESIAN_POINT('Ctrl Pts',(-18.2496811215229,-27.0641210640018,
123.080480376407)) ;
#46110=CARTESIAN_POINT('Ctrl Pts',(-17.9597894559771,-26.8841319836389,
122.997630523713)) ;
#46111=CARTESIAN_POINT('Ctrl Pts',(-18.2098424384287,-27.0740576757304,
123.285580848838)) ;
#46112=CARTESIAN_POINT('Ctrl Pts',(-17.9099883261813,-26.8940685953675,
123.254005646133)) ;
#46113=CARTESIAN_POINT('Ctrl Pts',(-18.206286456587,-27.084107551098,123.496809557806)) ;
#46114=CARTESIAN_POINT('Ctrl Pts',(-17.9055405282516,-26.9041184707351,
123.518041545854)) ;
#46115=CARTESIAN_POINT('Ctrl Pts',(-18.2386548673565,-27.0939580096334,
123.701367310787)) ;
#46116=CARTESIAN_POINT('Ctrl Pts',(-17.9459982769325,-26.9139689292705,
123.7737392886)) ;
#46117=CARTESIAN_POINT('Ctrl Pts',(-18.3063479731576,-27.1039299465862,
123.899751686817)) ;
#46118=CARTESIAN_POINT('Ctrl Pts',(-18.0306120394359,-26.9239408662233,
124.021720774531)) ;
#46119=CARTESIAN_POINT('Ctrl Pts',(-18.4077546179831,-27.1139254035183,
124.083836779179)) ;
#46120=CARTESIAN_POINT('Ctrl Pts',(-18.1573679303231,-26.9339363231554,
124.251828560722)) ;
#46121=CARTESIAN_POINT('Ctrl Pts',(-18.5402337139463,-27.1239582105714,
124.247943977524)) ;
#46122=CARTESIAN_POINT('Ctrl Pts',(-18.3229646348335,-26.9439691302085,
124.456964358552)) ;
#46123=CARTESIAN_POINT('Ctrl Pts',(-18.696288367492,-27.1338180971613,124.384394875918)) ;
#46124=CARTESIAN_POINT('Ctrl Pts',(-18.5180312778613,-26.9538290167985,
124.627530238962)) ;
#46125=CARTESIAN_POINT('Ctrl Pts',(-18.8757602839204,-27.1438071777266,
124.493403942456)) ;
#46126=CARTESIAN_POINT('Ctrl Pts',(-18.7423698226788,-26.9638180973637,
124.763794005457)) ;
#46127=CARTESIAN_POINT('Ctrl Pts',(-19.0703285555277,-27.1537386569357,
124.569162296289)) ;
#46128=CARTESIAN_POINT('Ctrl Pts',(-18.9855793301611,-26.9737495765729,
124.858494603905)) ;
#46129=CARTESIAN_POINT('Ctrl Pts',(-19.2761569854026,-27.1637245163817,
124.610551053502)) ;
#46130=CARTESIAN_POINT('Ctrl Pts',(-19.2428644372235,-26.9837354360188,
124.910233267454)) ;
#46131=CARTESIAN_POINT('Ctrl Pts',(-19.4871247300181,-27.1737626670289,
124.61522608717)) ;
#46132=CARTESIAN_POINT('Ctrl Pts',(-19.5065740592286,-26.993773586666,124.916079842677)) ;
#46133=CARTESIAN_POINT('Ctrl Pts',(-19.6918470853474,-27.1836107575333,
124.584217748348)) ;
#46134=CARTESIAN_POINT('Ctrl Pts',(-19.7624778086568,-27.0036216771704,
124.877322071397)) ;
#46135=CARTESIAN_POINT('Ctrl Pts',(-19.8923339922519,-27.1936716660512,
124.516888561277)) ;
#46136=CARTESIAN_POINT('Ctrl Pts',(-20.0130872707028,-27.0136825856884,
124.793163184846)) ;
#46137=CARTESIAN_POINT('Ctrl Pts',(-20.0749863200746,-27.2035665132092,
124.417294329767)) ;
#46138=CARTESIAN_POINT('Ctrl Pts',(-20.2414042796906,-27.0235774328464,
124.668672645301)) ;
#46139=CARTESIAN_POINT('Ctrl Pts',(-20.2386525978464,-27.2135081852543,
124.287347778684)) ;
#46140=CARTESIAN_POINT('Ctrl Pts',(-20.4459889974729,-27.0335191048914,
124.506241389245)) ;
#46141=CARTESIAN_POINT('Ctrl Pts',(-20.3782156387396,-27.2235107123797,
124.130014539962)) ;
#46142=CARTESIAN_POINT('Ctrl Pts',(-20.6204448444618,-27.0435216320169,
124.309576543544)) ;
#46143=CARTESIAN_POINT('Ctrl Pts',(-20.4883897656227,-27.2335455035672,
123.950121732222)) ;
#46144=CARTESIAN_POINT('Ctrl Pts',(-20.758164805552,-27.0535564232043,124.084711962413)) ;
#46145=CARTESIAN_POINT('Ctrl Pts',(-20.5645263195821,-27.2433903834263,
123.757649358259)) ;
#46146=CARTESIAN_POINT('Ctrl Pts',(-20.8533381771542,-27.0634013030634,
123.8441219504)) ;
#46147=CARTESIAN_POINT('Ctrl Pts',(-20.6070596189447,-27.2533762640448,
123.552103054265)) ;
#46148=CARTESIAN_POINT('Ctrl Pts',(-20.9065073830601,-27.0733871836819,
123.587189440378)) ;
#46149=CARTESIAN_POINT('Ctrl Pts',(-20.6133781384881,-27.263310987138,123.343300034861)) ;
#46150=CARTESIAN_POINT('Ctrl Pts',(-20.9144081114304,-27.0833219067751,
123.326185418482)) ;
#46151=CARTESIAN_POINT('Ctrl Pts',(-20.5827915728053,-27.2733688274492,
123.134108713238)) ;
#46152=CARTESIAN_POINT('Ctrl Pts',(-20.8761775034525,-27.0933797470863,
123.064696003703)) ;
#46153=CARTESIAN_POINT('Ctrl Pts',(-20.5182131701365,-27.2831893148457,
122.937983170637)) ;
#46154=CARTESIAN_POINT('Ctrl Pts',(-20.7954566740253,-27.1032002344828,
122.819537535272)) ;
#46155=CARTESIAN_POINT('Ctrl Pts',(-20.4185100813219,-27.2932497161908,
122.751485493187)) ;
#46156=CARTESIAN_POINT('Ctrl Pts',(-20.6708300595228,-27.1132606358279,
122.586414372848)) ;
#46157=CARTESIAN_POINT('Ctrl Pts',(-20.2893670926231,-27.3031806817437,
122.587408843276)) ;
#46158=CARTESIAN_POINT('Ctrl Pts',(-20.5094030853154,-27.1231916013808,
122.381316698631)) ;
#46159=CARTESIAN_POINT('Ctrl Pts',(-20.1339171194866,-27.3131195440802,
122.447821260435)) ;
#46160=CARTESIAN_POINT('Ctrl Pts',(-20.3150919759397,-27.1331304637173,
122.206830149708)) ;
#46161=CARTESIAN_POINT('Ctrl Pts',(-19.9557909141703,-27.3231052750064,
122.336681000777)) ;
#46162=CARTESIAN_POINT('Ctrl Pts',(-20.0924353593602,-27.1431161946435,
122.067902692524)) ;
#46163=CARTESIAN_POINT('Ctrl Pts',(-19.7602720484493,-27.3331296604338,
122.258075382976)) ;
#46164=CARTESIAN_POINT('Ctrl Pts',(-19.8480377025175,-27.1531405800709,
121.969643385179)) ;
#46165=CARTESIAN_POINT('Ctrl Pts',(-19.5565899889511,-27.3430329447871,
122.214817299832)) ;
#46166=CARTESIAN_POINT('Ctrl Pts',(-19.59343508194,-27.1630438644242,121.915568323419)) ;
#46167=CARTESIAN_POINT('Ctrl Pts',(-19.3452475882926,-27.3530929493651,
122.207539583544)) ;
#46168=CARTESIAN_POINT('Ctrl Pts',(-19.3292573389903,-27.1731038690022,
121.90646877428)) ;
#46169=CARTESIAN_POINT('Ctrl Pts',(-19.1402979082901,-27.3629362184342,
122.236294727092)) ;
#46170=CARTESIAN_POINT('Ctrl Pts',(-19.0730690560541,-27.1829471380713,
121.942410469089)) ;
#46171=CARTESIAN_POINT('Ctrl Pts',(-18.9404022090521,-27.3729267840419,
122.300676483571)) ;
#46172=CARTESIAN_POINT('Ctrl Pts',(-18.8231985706705,-27.192937703679,122.02288556215)) ;
#46173=CARTESIAN_POINT('Ctrl Pts',(-18.7558672982378,-27.3828549158207,
122.398221029593)) ;
#46174=CARTESIAN_POINT('Ctrl Pts',(-18.5925284415636,-27.2028658354578,
122.144814465017)) ;
#46175=CARTESIAN_POINT('Ctrl Pts',(-18.5898557423788,-27.3928428029016,
122.526807079815)) ;
#46176=CARTESIAN_POINT('Ctrl Pts',(-18.3850125185332,-27.2128537225387,
122.305545417301)) ;
#46177=CARTESIAN_POINT('Ctrl Pts',(-18.4482910581977,-27.4028787524703,
122.68324070113)) ;
#46178=CARTESIAN_POINT('Ctrl Pts',(-18.2080550368114,-27.2228896721074,
122.501085855653)) ;
#46179=CARTESIAN_POINT('Ctrl Pts',(-18.3377591304148,-27.4127336388491,
122.858492901612)) ;
#46180=CARTESIAN_POINT('Ctrl Pts',(-18.0698877945043,-27.2327445584862,
122.720150718132)) ;
#46181=CARTESIAN_POINT('Ctrl Pts',(-18.2579406650141,-27.422733053197,123.052931220241)) ;
#46182=CARTESIAN_POINT('Ctrl Pts',(-17.9701127120356,-27.2427439728341,
122.963197940076)) ;
#46183=CARTESIAN_POINT('Ctrl Pts',(-18.2133303124607,-27.4326282183875,
123.256154680513)) ;
#46184=CARTESIAN_POINT('Ctrl Pts',(-17.9143476221429,-27.2526391380246,
123.217227543753)) ;
#46185=CARTESIAN_POINT('Ctrl Pts',(-18.204564058286,-27.4426885370794,123.467444615832)) ;
#46186=CARTESIAN_POINT('Ctrl Pts',(-17.9033877648429,-27.2626994567166,
123.481339637183)) ;
#46187=CARTESIAN_POINT('Ctrl Pts',(-18.2319167259409,-27.4525386688555,
123.672729223044)) ;
#46188=CARTESIAN_POINT('Ctrl Pts',(-17.937576742963,-27.2725495884926,123.737946697359)) ;
#46189=CARTESIAN_POINT('Ctrl Pts',(-18.2951613085268,-27.4625692393058,
123.87388597203)) ;
#46190=CARTESIAN_POINT('Ctrl Pts',(-18.0166306722375,-27.2825801589429,
123.989393136718)) ;
#46191=CARTESIAN_POINT('Ctrl Pts',(-18.392639370384,-27.4725833899786,124.060501742582)) ;
#46192=CARTESIAN_POINT('Ctrl Pts',(-18.1384764760697,-27.2925943096157,
124.222663794495)) ;
#46193=CARTESIAN_POINT('Ctrl Pts',(-18.5192133454885,-27.482476323524,124.225536129967)) ;
#46194=CARTESIAN_POINT('Ctrl Pts',(-18.2966929164752,-27.3024872431611,
124.428958569241)) ;
#46195=CARTESIAN_POINT('Ctrl Pts',(-18.6738373848897,-27.4924658375142,
124.367619074625)) ;
#46196=CARTESIAN_POINT('Ctrl Pts',(-18.4899718704159,-27.3124767571514,
124.60656373873)) ;
#46197=CARTESIAN_POINT('Ctrl Pts',(-18.8501175734663,-27.5024196081667,
124.480434768082)) ;
#46198=CARTESIAN_POINT('Ctrl Pts',(-18.7103215045909,-27.3224305278038,
124.74758509881)) ;
#46199=CARTESIAN_POINT('Ctrl Pts',(-19.0451588516024,-27.5124673768272,
124.561494657488)) ;
#46200=CARTESIAN_POINT('Ctrl Pts',(-18.9541222140896,-27.3324782964644,
124.848911596832)) ;
#46201=CARTESIAN_POINT('Ctrl Pts',(-19.2470679046849,-27.522309103267,124.606762346263)) ;
#46202=CARTESIAN_POINT('Ctrl Pts',(-19.2065092981465,-27.3423200229042,
124.905498197986)) ;
#46203=CARTESIAN_POINT('Ctrl Pts',(-19.4567187804264,-27.5322946200898,
124.616878516761)) ;
#46204=CARTESIAN_POINT('Ctrl Pts',(-19.4685730601993,-27.3523055397269,
124.918145048951)) ;
#46205=CARTESIAN_POINT('Ctrl Pts',(-19.6640500637913,-27.5422339517853,
124.590629381917)) ;
#46206=CARTESIAN_POINT('Ctrl Pts',(-19.727737905255,-27.3622448714225,124.885335148688)) ;
#46207=CARTESIAN_POINT('Ctrl Pts',(-19.8656328349993,-27.5522737214829,
124.52812532427)) ;
#46208=CARTESIAN_POINT('Ctrl Pts',(-19.9797167083431,-27.37228464112,124.807206664709)) ;
#46209=CARTESIAN_POINT('Ctrl Pts',(-20.050539305733,-27.5621618827317,124.433105551511)) ;
#46210=CARTESIAN_POINT('Ctrl Pts',(-20.210851339288,-27.3821728023688,124.688432935281)) ;
#46211=CARTESIAN_POINT('Ctrl Pts',(-20.2180592426687,-27.5721514372341,
124.306460221141)) ;
#46212=CARTESIAN_POINT('Ctrl Pts',(-20.4202523049205,-27.3921623568712,
124.530127299133)) ;
#46213=CARTESIAN_POINT('Ctrl Pts',(-20.3604835812191,-27.5821098517577,
124.153021019065)) ;
#46214=CARTESIAN_POINT('Ctrl Pts',(-20.5982841261054,-27.4021207713948,
124.338329003495)) ;
#46215=CARTESIAN_POINT('Ctrl Pts',(-20.473871725562,-27.5920097645871,123.978479224777)) ;
#46216=CARTESIAN_POINT('Ctrl Pts',(-20.7400208952278,-27.4120206842242,
124.120151747141)) ;
#46217=CARTESIAN_POINT('Ctrl Pts',(-20.5563690525815,-27.602056464237,123.784065248068)) ;
#46218=CARTESIAN_POINT('Ctrl Pts',(-20.8431437130591,-27.4220673838741,
123.877134998684)) ;
#46219=CARTESIAN_POINT('Ctrl Pts',(-20.6033030576586,-27.6119563245426,
123.581267591945)) ;
#46220=CARTESIAN_POINT('Ctrl Pts',(-20.9018126855217,-27.4319672441797,
123.623637353348)) ;
#46221=CARTESIAN_POINT('Ctrl Pts',(-20.6145464495285,-27.622007728748,123.370284273142)) ;
#46222=CARTESIAN_POINT('Ctrl Pts',(-20.9158681861848,-27.4420186483852,
123.359908517845)) ;
#46223=CARTESIAN_POINT('Ctrl Pts',(-20.5894865428159,-27.6318887656692,
123.164040601756)) ;
#46224=CARTESIAN_POINT('Ctrl Pts',(-20.8845444215458,-27.4518996853063,
123.102102763115)) ;
#46225=CARTESIAN_POINT('Ctrl Pts',(-20.5285619224102,-27.6418885978467,
122.96287053044)) ;
#46226=CARTESIAN_POINT('Ctrl Pts',(-20.8083897017697,-27.4618995174838,
122.850639705419)) ;
#46227=CARTESIAN_POINT('Ctrl Pts',(-20.4345314205031,-27.6518066008316,
122.776728506564)) ;
#46228=CARTESIAN_POINT('Ctrl Pts',(-20.6908521995959,-27.4718175204687,
122.61796100732)) ;
#46229=CARTESIAN_POINT('Ctrl Pts',(-20.307917816095,-27.6618579067061,122.607595735028)) ;
#46230=CARTESIAN_POINT('Ctrl Pts',(-20.5325862276468,-27.4818688263432,
122.406544566139)) ;
#46231=CARTESIAN_POINT('Ctrl Pts',(-20.1567577654715,-27.6717277300977,
122.465387827078)) ;
#46232=CARTESIAN_POINT('Ctrl Pts',(-20.3436360267876,-27.4917386497348,
122.228783160696)) ;
#46233=CARTESIAN_POINT('Ctrl Pts',(-19.979678811247,-27.681801896148,122.349293202809)) ;
#46234=CARTESIAN_POINT('Ctrl Pts',(-20.1222882553386,-27.5018128157851,
122.083664260692)) ;
#46235=CARTESIAN_POINT('Ctrl Pts',(-19.7900524651862,-27.6916219802896,
122.267545505754)) ;
#46236=CARTESIAN_POINT('Ctrl Pts',(-19.8852542608473,-27.5116328999267,
121.981478176074)) ;
#46237=CARTESIAN_POINT('Ctrl Pts',(-19.5839641602467,-27.7017007070255,
122.218539726718)) ;
#46238=CARTESIAN_POINT('Ctrl Pts',(-19.6276445348726,-27.5217116266626,
121.920220233275)) ;
#46239=CARTESIAN_POINT('Ctrl Pts',(-19.3771678744328,-27.711552287675,122.206266541028)) ;
#46240=CARTESIAN_POINT('Ctrl Pts',(-19.3691479103184,-27.5315632073121,
121.904877852358)) ;
#46241=CARTESIAN_POINT('Ctrl Pts',(-19.1668198410956,-27.7216254159734,
122.230427368706)) ;
#46242=CARTESIAN_POINT('Ctrl Pts',(-19.1062132173581,-27.5416363356105,
121.935078088023)) ;
#46243=CARTESIAN_POINT('Ctrl Pts',(-18.9684654062851,-27.7314678938648,
122.289410143151)) ;
#46244=CARTESIAN_POINT('Ctrl Pts',(-18.8582685980059,-27.5514788135019,
122.008806224884)) ;
#46245=CARTESIAN_POINT('Ctrl Pts',(-18.7804810737789,-27.7414485004629,
122.382594626151)) ;
#46246=CARTESIAN_POINT('Ctrl Pts',(-18.6232876861483,-27.5614594201,122.125286522871)) ;
#46247=CARTESIAN_POINT('Ctrl Pts',(-18.6111314469125,-27.7514662094817,
122.50779197817)) ;
#46248=CARTESIAN_POINT('Ctrl Pts',(-18.4116002704639,-27.5714771291188,
122.281782687979)) ;
#46249=CARTESIAN_POINT('Ctrl Pts',(-18.46769289707,-27.7613523885191,122.65822099697)) ;
#46250=CARTESIAN_POINT('Ctrl Pts',(-18.2323009870814,-27.5813633081562,
122.469819398542)) ;
#46251=CARTESIAN_POINT('Ctrl Pts',(-18.3505632690495,-27.7714100010914,
122.834235024386)) ;
#46252=CARTESIAN_POINT('Ctrl Pts',(-18.0858887221731,-27.5914209207286,
122.689836404072)) ;
#46253=CARTESIAN_POINT('Ctrl Pts',(-18.2672711578626,-27.7812863944636,
123.024442583232)) ;
#46254=CARTESIAN_POINT('Ctrl Pts',(-17.981772680714,-27.6012973141007,122.927596725681)) ;
#46255=CARTESIAN_POINT('Ctrl Pts',(-18.2171766731924,-27.791281422614,123.228504736778)) ;
#46256=CARTESIAN_POINT('Ctrl Pts',(-17.9191542665853,-27.6112923422511,
123.182674524743)) ;
#46257=CARTESIAN_POINT('Ctrl Pts',(-18.2035981744951,-27.80130216946,123.438743704045)) ;
#46258=CARTESIAN_POINT('Ctrl Pts',(-17.9021807329972,-27.6213130890971,
123.445473162291)) ;
#46259=CARTESIAN_POINT('Ctrl Pts',(-18.2262128560997,-27.8112042381264,
123.645681904527)) ;
#46260=CARTESIAN_POINT('Ctrl Pts',(-17.930448869701,-27.6312151577635,123.704146901839)) ;
#46261=CARTESIAN_POINT('Ctrl Pts',(-18.284639933744,-27.8211949779461,123.847429809037)) ;
#46262=CARTESIAN_POINT('Ctrl Pts',(-18.0034825912362,-27.6412058975832,
123.956332064129)) ;
#46263=CARTESIAN_POINT('Ctrl Pts',(-18.3770881160731,-27.8311581741564,
124.035370273374)) ;
#46264=CARTESIAN_POINT('Ctrl Pts',(-18.1190427862629,-27.6511690937935,
124.191258163438)) ;
#46265=CARTESIAN_POINT('Ctrl Pts',(-18.4996327245681,-27.8410623584565,
124.203730145458)) ;
#46266=CARTESIAN_POINT('Ctrl Pts',(-18.2722240570765,-27.6610732780936,
124.401708795378)) ;
#46267=CARTESIAN_POINT('Ctrl Pts',(-18.652006072211,-27.8511228188474,124.350375168077)) ;
#46268=CARTESIAN_POINT('Ctrl Pts',(-18.4626904000373,-27.6711337384845,
124.585014918484)) ;
#46269=CARTESIAN_POINT('Ctrl Pts',(-18.8235862046144,-27.8609633647182,
124.466005825925)) ;
#46270=CARTESIAN_POINT('Ctrl Pts',(-18.6771667745688,-27.6809742843553,
124.729554078274)) ;
#46271=CARTESIAN_POINT('Ctrl Pts',(-19.0167402747536,-27.8710255854299,
124.552208647531)) ;
#46272=CARTESIAN_POINT('Ctrl Pts',(-18.9186090603338,-27.6910365050671,
124.83730737481)) ;
#46273=CARTESIAN_POINT('Ctrl Pts',(-19.2186463887635,-27.8809227284465,
124.602519019844)) ;
#46274=CARTESIAN_POINT('Ctrl Pts',(-19.1709926750529,-27.7009336480836,
124.900195583727)) ;
#46275=CARTESIAN_POINT('Ctrl Pts',(-19.4268700305496,-27.8908539048637,
124.617749388412)) ;
#46276=CARTESIAN_POINT('Ctrl Pts',(-19.4312729665485,-27.7108648245008,
124.919233320648)) ;
#46277=CARTESIAN_POINT('Ctrl Pts',(-19.6368755079311,-27.9008961186423,
124.596126506695)) ;
#46278=CARTESIAN_POINT('Ctrl Pts',(-19.6937795868889,-27.7209070382794,
124.892204557255)) ;
#46279=CARTESIAN_POINT('Ctrl Pts',(-19.8368447731837,-27.910782658845,124.539408291931)) ;
#46280=CARTESIAN_POINT('Ctrl Pts',(-19.9437421483585,-27.7307935784821,
124.821306255689)) ;
#46281=CARTESIAN_POINT('Ctrl Pts',(-20.026076968928,-27.9207762534504,124.448165743483)) ;
#46282=CARTESIAN_POINT('Ctrl Pts',(-20.180282407611,-27.7407871730876,124.707252644134)) ;
#46283=CARTESIAN_POINT('Ctrl Pts',(-20.1957478692997,-27.930720128608,124.326020666064)) ;
#46284=CARTESIAN_POINT('Ctrl Pts',(-20.3923713220577,-27.7507310482451,
124.554570637425)) ;
#46285=CARTESIAN_POINT('Ctrl Pts',(-20.3420563337105,-27.9406806647228,
124.176229596615)) ;
#46286=CARTESIAN_POINT('Ctrl Pts',(-20.5752568933734,-27.7606915843599,
124.367331130021)) ;
#46287=CARTESIAN_POINT('Ctrl Pts',(-20.4606861174511,-27.9506772680455,
124.002726210929)) ;
#46288=CARTESIAN_POINT('Ctrl Pts',(-20.7235437790341,-27.7706881876827,
124.150451479886)) ;
#46289=CARTESIAN_POINT('Ctrl Pts',(-20.5474206151358,-27.960710351,123.810462365008)) ;
#46290=CARTESIAN_POINT('Ctrl Pts',(-20.8319614750394,-27.7807212706372,
123.910121632712)) ;
#46291=CARTESIAN_POINT('Ctrl Pts',(-20.5987649896307,-27.9705615197016,
123.609829364369)) ;
#46292=CARTESIAN_POINT('Ctrl Pts',(-20.8961417940296,-27.7905724393387,
123.65932892789)) ;
#46293=CARTESIAN_POINT('Ctrl Pts',(-20.6152871156439,-27.9805240104005,
123.401046818215)) ;
#46294=CARTESIAN_POINT('Ctrl Pts',(-20.9167937428057,-27.8005349300376,
123.398350225034)) ;
#46295=CARTESIAN_POINT('Ctrl Pts',(-20.5949125271602,-27.9905524388182,
123.191192264674)) ;
#46296=CARTESIAN_POINT('Ctrl Pts',(-20.8913248727649,-27.8105633584554,
123.136032193867)) ;
#46297=CARTESIAN_POINT('Ctrl Pts',(-20.53914584983,-28.0004628061828,122.990457378277)) ;
#46298=CARTESIAN_POINT('Ctrl Pts',(-20.8216156440544,-27.8204737258199,
122.885112920422)) ;
#46299=CARTESIAN_POINT('Ctrl Pts',(-20.4496374418431,-28.0103976737979,
122.801740219199)) ;
#46300=CARTESIAN_POINT('Ctrl Pts',(-20.7097290522174,-27.830408593435,122.649216253135)) ;
#46301=CARTESIAN_POINT('Ctrl Pts',(-20.3272748886815,-28.0204388157769,
122.629733634215)) ;
#46302=CARTESIAN_POINT('Ctrl Pts',(-20.5567753117552,-27.840449735414,122.434208642636)) ;
#46303=CARTESIAN_POINT('Ctrl Pts',(-20.1793010965195,-28.0303259519801,
122.483741362788)) ;
#46304=CARTESIAN_POINT('Ctrl Pts',(-20.371806724897,-27.8503368716172,122.251718186914)) ;
#46305=CARTESIAN_POINT('Ctrl Pts',(-20.0066274113567,-28.0403182343835,
122.364130675041)) ;
#46306=CARTESIAN_POINT('Ctrl Pts',(-20.1559638841929,-27.8603291540206,
122.102205529793)) ;
#46307=CARTESIAN_POINT('Ctrl Pts',(-19.8165954509597,-28.0502667623487,
122.276745364225)) ;
#46308=CARTESIAN_POINT('Ctrl Pts',(-19.9184230348256,-27.8702776819858,
121.99297454764)) ;
#46309=CARTESIAN_POINT('Ctrl Pts',(-19.6146202820985,-28.0602034935108,
122.223467272798)) ;
#46310=CARTESIAN_POINT('Ctrl Pts',(-19.665953180287,-27.8802144131479,121.926377817828)) ;
#46311=CARTESIAN_POINT('Ctrl Pts',(-19.4054676734705,-28.0701867043708,
122.205721541684)) ;
#46312=CARTESIAN_POINT('Ctrl Pts',(-19.4045120642448,-27.8901976240079,
121.904196807196)) ;
#46313=CARTESIAN_POINT('Ctrl Pts',(-19.1952379005433,-28.0802298035207,
122.225046803646)) ;
#46314=CARTESIAN_POINT('Ctrl Pts',(-19.1417251311674,-27.9002407231578,
121.92835440127)) ;
#46315=CARTESIAN_POINT('Ctrl Pts',(-18.9956932343111,-28.0900607677956,
122.278974247708)) ;
#46316=CARTESIAN_POINT('Ctrl Pts',(-18.892293224786,-27.9100716874327,121.995765252508)) ;
#46317=CARTESIAN_POINT('Ctrl Pts',(-18.8039248705908,-28.1001336201815,
122.368723820022)) ;
#46318=CARTESIAN_POINT('Ctrl Pts',(-18.6525836805033,-27.9201445398186,
122.107953193368)) ;
#46319=CARTESIAN_POINT('Ctrl Pts',(-18.6342195703199,-28.1099977478933,
122.487946903188)) ;
#46320=CARTESIAN_POINT('Ctrl Pts',(-18.4404518362338,-27.9300086675304,
122.256983728471)) ;
#46321=CARTESIAN_POINT('Ctrl Pts',(-18.4851003678343,-28.1200199500282,
122.636789063921)) ;
#46322=CARTESIAN_POINT('Ctrl Pts',(-18.2540538810711,-27.9400308696653,
122.44303741669)) ;
#46323=CARTESIAN_POINT('Ctrl Pts',(-18.3644270649533,-28.1300471429966,
122.809651509413)) ;
#46324=CARTESIAN_POINT('Ctrl Pts',(-18.1032133230383,-27.9500580626337,
122.659116134907)) ;
#46325=CARTESIAN_POINT('Ctrl Pts',(-18.2768385867952,-28.1399027369636,
122.997405819395)) ;
#46326=CARTESIAN_POINT('Ctrl Pts',(-17.9937284543403,-27.9599136566007,
122.893810711294)) ;
#46327=CARTESIAN_POINT('Ctrl Pts',(-18.2220200004676,-28.1498599088289,
123.199439317662)) ;
#46328=CARTESIAN_POINT('Ctrl Pts',(-17.9252066477856,-27.969870828466,123.146353412769)) ;
#46329=CARTESIAN_POINT('Ctrl Pts',(-18.2033226183059,-28.1598987528273,
123.409644983658)) ;
#46330=CARTESIAN_POINT('Ctrl Pts',(-17.9018363926086,-27.9799096724644,
123.409110487333)) ;
#46331=CARTESIAN_POINT('Ctrl Pts',(-18.2207487622362,-28.1697727767028,
123.616522805315)) ;
#46332=CARTESIAN_POINT('Ctrl Pts',(-17.9236207437678,-27.98978369634,123.667708642615)) ;
#46333=CARTESIAN_POINT('Ctrl Pts',(-18.2748756328717,-28.1798426026932,
123.821155710981)) ;
#46334=CARTESIAN_POINT('Ctrl Pts',(-17.9912807797275,-27.9998535223304,
123.923499029241)) ;
#46335=CARTESIAN_POINT('Ctrl Pts',(-18.3615430076775,-28.1896758465905,
124.008855877301)) ;
#46336=CARTESIAN_POINT('Ctrl Pts',(-18.0996170115864,-28.0096867662276,
124.158124720439)) ;
#46337=CARTESIAN_POINT('Ctrl Pts',(-18.4813453459947,-28.1997062743635,
124.18238158238)) ;
#46338=CARTESIAN_POINT('Ctrl Pts',(-18.249371382821,-28.0197171940007,124.375030745284)) ;
#46339=CARTESIAN_POINT('Ctrl Pts',(-18.6299243812976,-28.2097378911087,
124.332069289836)) ;
#46340=CARTESIAN_POINT('Ctrl Pts',(-18.4350962680924,-28.0297488107458,
124.562139179243)) ;
#46341=CARTESIAN_POINT('Ctrl Pts',(-18.7984985629321,-28.2195675680894,
124.451573981328)) ;
#46342=CARTESIAN_POINT('Ctrl Pts',(-18.6458160519967,-28.0395784877265,
124.711519341739)) ;
#46343=CARTESIAN_POINT('Ctrl Pts',(-18.9880488787878,-28.2295570849293,
124.542006375535)) ;
#46344=CARTESIAN_POINT('Ctrl Pts',(-18.8827549500496,-28.0495680045665,
124.824558143869)) ;
#46345=CARTESIAN_POINT('Ctrl Pts',(-19.1916515256229,-28.2396006970691,
124.597937925507)) ;
#46346=CARTESIAN_POINT('Ctrl Pts',(-19.1372585887124,-28.0596116167062,
124.894470815532)) ;
#46347=CARTESIAN_POINT('Ctrl Pts',(-19.3972114936263,-28.2494233034044,
124.617664945189)) ;
#46348=CARTESIAN_POINT('Ctrl Pts',(-19.3942099817878,-28.0694342230415,
124.91912779169)) ;
#46349=CARTESIAN_POINT('Ctrl Pts',(-19.6076212256826,-28.2594615333036,
124.601522484725)) ;
#46350=CARTESIAN_POINT('Ctrl Pts',(-19.6572218646034,-28.0794724529408,
124.898947663021)) ;
#46351=CARTESIAN_POINT('Ctrl Pts',(-19.8113776911949,-28.2694725680956,
124.548753711217)) ;
#46352=CARTESIAN_POINT('Ctrl Pts',(-19.9119170104515,-28.0894834877327,
124.832984826371)) ;
#46353=CARTESIAN_POINT('Ctrl Pts',(-20.0008298539462,-28.2793702990627,
124.462706665286)) ;
#46354=CARTESIAN_POINT('Ctrl Pts',(-20.1487320477206,-28.0993812186998,
124.725423875281)) ;
#46355=CARTESIAN_POINT('Ctrl Pts',(-20.1742139857442,-28.2893599269132,
124.344205140818)) ;
#46356=CARTESIAN_POINT('Ctrl Pts',(-20.3654611748462,-28.1093708465503,
124.5772951408)) ;
#46357=CARTESIAN_POINT('Ctrl Pts',(-20.3238283363393,-28.2993157173592,
124.19784376409)) ;
#46358=CARTESIAN_POINT('Ctrl Pts',(-20.5524779416027,-28.1193266369963,
124.394341663434)) ;
#46359=CARTESIAN_POINT('Ctrl Pts',(-20.4457396566452,-28.3092431159212,
124.028437006786)) ;
#46360=CARTESIAN_POINT('Ctrl Pts',(-20.7048656204767,-28.1292540355584,
124.182581520283)) ;
#46361=CARTESIAN_POINT('Ctrl Pts',(-20.5372193180134,-28.3192687110311,
123.838562812821)) ;
#46362=CARTESIAN_POINT('Ctrl Pts',(-20.8192132351186,-28.1392796306682,
123.945237856592)) ;
#46363=CARTESIAN_POINT('Ctrl Pts',(-20.5936698159923,-28.3291545617007,
123.638543561245)) ;
#46364=CARTESIAN_POINT('Ctrl Pts',(-20.8897744387993,-28.1491654813378,
123.695212486568)) ;
#46365=CARTESIAN_POINT('Ctrl Pts',(-20.6152462524492,-28.3391437415449,
123.429645094941)) ;
#46366=CARTESIAN_POINT('Ctrl Pts',(-20.9167426862714,-28.159154661182,123.434089007642)) ;
#46367=CARTESIAN_POINT('Ctrl Pts',(-20.5997049484337,-28.3491849286484,
123.219121094953)) ;
#46368=CARTESIAN_POINT('Ctrl Pts',(-20.8973138529512,-28.1691958482856,
123.170934263122)) ;
#46369=CARTESIAN_POINT('Ctrl Pts',(-20.5492532199071,-28.3590175721244,
123.018663279547)) ;
#46370=CARTESIAN_POINT('Ctrl Pts',(-20.8342467261708,-28.1790284917615,
122.920361624849)) ;
#46371=CARTESIAN_POINT('Ctrl Pts',(-20.4639239618416,-28.3690115218339,
122.826668029978)) ;
#46372=CARTESIAN_POINT('Ctrl Pts',(-20.7275828726051,-28.189022441471,122.680368443651)) ;
#46373=CARTESIAN_POINT('Ctrl Pts',(-20.3457702484628,-28.3790406446104,
122.652037807507)) ;
#46374=CARTESIAN_POINT('Ctrl Pts',(-20.5798888066981,-28.1990515642475,
122.462081994114)) ;
#46375=CARTESIAN_POINT('Ctrl Pts',(-20.2015610995993,-28.3889167755291,
122.502648999928)) ;
#46376=CARTESIAN_POINT('Ctrl Pts',(-20.3996251641318,-28.2089276951662,
122.275347174546)) ;
#46377=CARTESIAN_POINT('Ctrl Pts',(-20.0317039479304,-28.3989148105461,
122.37888357769)) ;
#46378=CARTESIAN_POINT('Ctrl Pts',(-20.1873021799441,-28.2189257301832,
122.120642324747)) ;
#46379=CARTESIAN_POINT('Ctrl Pts',(-19.8445504166726,-28.4088287403048,
122.287101606991)) ;
#46380=CARTESIAN_POINT('Ctrl Pts',(-19.9533587455655,-28.2288396599419,
122.005916898594)) ;
#46381=CARTESIAN_POINT('Ctrl Pts',(-19.6417453548372,-28.4188719280426,
122.228424618647)) ;
#46382=CARTESIAN_POINT('Ctrl Pts',(-19.6998517913933,-28.2388828476797,
121.932573093305)) ;
#46383=CARTESIAN_POINT('Ctrl Pts',(-19.4348032819945,-28.428771770183,122.206158950053)) ;
#46384=CARTESIAN_POINT('Ctrl Pts',(-19.4411734358199,-28.2487826898201,
121.904743447238)) ;
#46385=CARTESIAN_POINT('Ctrl Pts',(-19.225199951328,-28.438763036991,122.219845479332)) ;
#46386=CARTESIAN_POINT('Ctrl Pts',(-19.1791693222562,-28.2587739566281,
121.921854204058)) ;
#46387=CARTESIAN_POINT('Ctrl Pts',(-19.0204087974407,-28.4487951391229,
122.270276783567)) ;
#46388=CARTESIAN_POINT('Ctrl Pts',(-18.923180998322,-28.2688060587601,121.984895781452)) ;
#46389=CARTESIAN_POINT('Ctrl Pts',(-18.8305583447142,-28.4586620200777,
122.353843034253)) ;
#46390=CARTESIAN_POINT('Ctrl Pts',(-18.6858684267657,-28.2786729397148,
122.08935619064)) ;
#46391=CARTESIAN_POINT('Ctrl Pts',(-18.6556330787561,-28.4686538113658,
122.470151417965)) ;
#46392=CARTESIAN_POINT('Ctrl Pts',(-18.4672132264588,-28.288664731003,122.234743944374)) ;
#46393=CARTESIAN_POINT('Ctrl Pts',(-18.5032314430184,-28.4786859272774,
122.61594277691)) ;
#46394=CARTESIAN_POINT('Ctrl Pts',(-18.276712974157,-28.2986968469145,122.416985014583)) ;
#46395=CARTESIAN_POINT('Ctrl Pts',(-18.380260915545,-28.4885522440774,122.782991829368)) ;
#46396=CARTESIAN_POINT('Ctrl Pts',(-18.1230016340979,-28.3085631637145,
122.625798315029)) ;
#46397=CARTESIAN_POINT('Ctrl Pts',(-18.286740408124,-28.498539725551,122.970954331532)) ;
#46398=CARTESIAN_POINT('Ctrl Pts',(-18.0061033569078,-28.3185506451881,
122.86075275285)) ;
#46399=CARTESIAN_POINT('Ctrl Pts',(-18.2274077058308,-28.5084846499299,
123.171464369965)) ;
#46400=CARTESIAN_POINT('Ctrl Pts',(-17.931940003922,-28.328495569567,123.111391293711)) ;
#46401=CARTESIAN_POINT('Ctrl Pts',(-18.2036772806348,-28.5185295358406,
123.381282408305)) ;
#46402=CARTESIAN_POINT('Ctrl Pts',(-17.902279648867,-28.3385404554777,123.373664123611)) ;
#46403=CARTESIAN_POINT('Ctrl Pts',(-18.2163217636226,-28.5283916395532,
123.588243745579)) ;
#46404=CARTESIAN_POINT('Ctrl Pts',(-17.9180879856087,-28.3484025591903,
123.632366059909)) ;
#46405=CARTESIAN_POINT('Ctrl Pts',(-18.2649253863527,-28.5383832033776,
123.792581695052)) ;
#46406=CARTESIAN_POINT('Ctrl Pts',(-17.978845222314,-28.3583941230148,123.887787950721)) ;
#46407=CARTESIAN_POINT('Ctrl Pts',(-18.3478659471332,-28.5483160114405,
123.984221813374)) ;
#46408=CARTESIAN_POINT('Ctrl Pts',(-18.0825235360191,-28.3683269310777,
124.127337211337)) ;
#46409=CARTESIAN_POINT('Ctrl Pts',(-18.4624497179601,-28.5582531136769,
124.158918671784)) ;
#46410=CARTESIAN_POINT('Ctrl Pts',(-18.2257556811439,-28.378264033314,124.345706898237)) ;
#46411=CARTESIAN_POINT('Ctrl Pts',(-18.6074717807451,-28.5683055599473,
124.312619227432)) ;
#46412=CARTESIAN_POINT('Ctrl Pts',(-18.4070352870554,-28.3883164795844,
124.537830699298)) ;
#46413=CARTESIAN_POINT('Ctrl Pts',(-18.7733489453358,-28.5781516755289,
124.436472624767)) ;
#46414=CARTESIAN_POINT('Ctrl Pts',(-18.6143836431893,-28.398162595166,124.692645379455)) ;
#46415=CARTESIAN_POINT('Ctrl Pts',(-18.9618249797804,-28.5881996952438,
124.531831590146)) ;
#46416=CARTESIAN_POINT('Ctrl Pts',(-18.8499799673712,-28.4082106148809,
124.811841582492)) ;
#46417=CARTESIAN_POINT('Ctrl Pts',(-19.1619711895627,-28.5981416468727,
124.592099396301)) ;
#46418=CARTESIAN_POINT('Ctrl Pts',(-19.1001636769322,-28.4181525665098,
124.887173703346)) ;
#46419=CARTESIAN_POINT('Ctrl Pts',(-19.36940458292,-28.6080804278718,124.617204452178)) ;
#46420=CARTESIAN_POINT('Ctrl Pts',(-19.3594558684256,-28.4280913475089,
124.91855224253)) ;
#46421=CARTESIAN_POINT('Ctrl Pts',(-19.5798534901081,-28.6181064765979,
124.605652962537)) ;
#46422=CARTESIAN_POINT('Ctrl Pts',(-19.6225169288426,-28.438117396235,124.904110048364)) ;
#46423=CARTESIAN_POINT('Ctrl Pts',(-19.7823487906233,-28.6279933370061,
124.558649540917)) ;
#46424=CARTESIAN_POINT('Ctrl Pts',(-19.8756354818284,-28.4480042566432,
124.845353062354)) ;
#46425=CARTESIAN_POINT('Ctrl Pts',(-19.9763812601013,-28.6380246121379,
124.476122124052)) ;
#46426=CARTESIAN_POINT('Ctrl Pts',(-20.1181752200281,-28.458035531775,124.742190925089)) ;
#46427=CARTESIAN_POINT('Ctrl Pts',(-20.1507052106711,-28.6479075894383,
124.362992233123)) ;
#46428=CARTESIAN_POINT('Ctrl Pts',(-20.3360779496977,-28.4679185090754,
124.600777052286)) ;
#46429=CARTESIAN_POINT('Ctrl Pts',(-20.3053443200726,-28.6579644428455,
124.218890410107)) ;
#46430=CARTESIAN_POINT('Ctrl Pts',(-20.5293776948737,-28.4779753624826,
124.420644314917)) ;
#46431=CARTESIAN_POINT('Ctrl Pts',(-20.4724604666755,-28.6711326839214,
123.998058155589)) ;
#46432=CARTESIAN_POINT('Ctrl Pts',(-20.7382563360483,-28.4911436035585,
124.144618303968)) ;
#46433=CARTESIAN_POINT('Ctrl Pts',(-20.5799131365806,-28.6845337131479,
123.73425819107)) ;
#46434=CARTESIAN_POINT('Ctrl Pts',(-20.8725696183407,-28.504544632785,123.814898572995)) ;
#46435=CARTESIAN_POINT('Ctrl Pts',(-20.6142236375671,-28.6977466298788,
123.458567013862)) ;
#46436=CARTESIAN_POINT('Ctrl Pts',(-20.9154664864313,-28.5177575495159,
123.470229804426)) ;
#46437=CARTESIAN_POINT('Ctrl Pts',(-20.604352967794,-28.707675024332,123.250109379369)) ;
#46438=CARTESIAN_POINT('Ctrl Pts',(-20.9031228604222,-28.5276859439691,
123.209668872578)) ;
#46439=CARTESIAN_POINT('Ctrl Pts',(-20.5583282587321,-28.7176565244601,
123.045346923892)) ;
#46440=CARTESIAN_POINT('Ctrl Pts',(-20.8455899283561,-28.5376674440972,
122.953713451803)) ;
#46441=CARTESIAN_POINT('Ctrl Pts',(-20.4767166915395,-28.7276970677302,
122.850689815527)) ;
#46442=CARTESIAN_POINT('Ctrl Pts',(-20.7435726949857,-28.5477079873673,
122.710393832338)) ;
#46443=CARTESIAN_POINT('Ctrl Pts',(-20.3649428036905,-28.7375463995133,
122.676381992891)) ;
#46444=CARTESIAN_POINT('Ctrl Pts',(-20.6038530329981,-28.5575573191504,
122.492510433972)) ;
#46445=CARTESIAN_POINT('Ctrl Pts',(-20.2229203006753,-28.747541803985,122.521509294334)) ;
#46446=CARTESIAN_POINT('Ctrl Pts',(-20.4263234254277,-28.5675527236221,
122.298921849287)) ;
#46447=CARTESIAN_POINT('Ctrl Pts',(-20.0555849748291,-28.7575581314336,
122.393679057562)) ;
#46448=CARTESIAN_POINT('Ctrl Pts',(-20.2171504397288,-28.5775690510707,
122.139134607576)) ;
#46449=CARTESIAN_POINT('Ctrl Pts',(-19.8088912325934,-28.7707817886001,
122.265428926498)) ;
#46450=CARTESIAN_POINT('Ctrl Pts',(-19.9087920777924,-28.5907927082372,
121.978832990271)) ;
#46451=CARTESIAN_POINT('Ctrl Pts',(-19.5330216381452,-28.7840760799895,
122.203967929054)) ;
#46452=CARTESIAN_POINT('Ctrl Pts',(-19.5639959876032,-28.6040869996266,
121.90200706357)) ;
#46453=CARTESIAN_POINT('Ctrl Pts',(-19.2539859157199,-28.797360430921,122.215868648645)) ;
#46454=CARTESIAN_POINT('Ctrl Pts',(-19.2151418343695,-28.6173713505581,
121.916882629654)) ;
#46455=CARTESIAN_POINT('Ctrl Pts',(-19.0492445151565,-28.8073328119828,
122.260874137876)) ;
#46456=CARTESIAN_POINT('Ctrl Pts',(-18.9592277477311,-28.6273437316199,
121.973142750752)) ;
#46457=CARTESIAN_POINT('Ctrl Pts',(-18.8564919194603,-28.8172411916084,
122.339917001314)) ;
#46458=CARTESIAN_POINT('Ctrl Pts',(-18.7182849243588,-28.6372521112455,
122.071948770313)) ;
#46459=CARTESIAN_POINT('Ctrl Pts',(-18.6778931742279,-28.8272951903564,
122.452918665696)) ;
#46460=CARTESIAN_POINT('Ctrl Pts',(-18.4950390577731,-28.6473061099936,
122.213201780035)) ;
#46461=CARTESIAN_POINT('Ctrl Pts',(-18.524471696003,-28.8371573874727,122.592405825859)) ;
#46462=CARTESIAN_POINT('Ctrl Pts',(-18.3032620688519,-28.6571683071099,
122.38756772639)) ;
#46463=CARTESIAN_POINT('Ctrl Pts',(-18.3524307607685,-28.8505045138469,
122.814082154856)) ;
#46464=CARTESIAN_POINT('Ctrl Pts',(-18.0882237967221,-28.670515433484,122.664637872146)) ;
#46465=CARTESIAN_POINT('Ctrl Pts',(-18.2159876348167,-28.8670414794883,
123.138150036716)) ;
#46466=CARTESIAN_POINT('Ctrl Pts',(-17.9176634712148,-28.6870523991254,
123.069772556873)) ;
#46467=CARTESIAN_POINT('Ctrl Pts',(-18.1976653162901,-28.8836760836622,
123.491362438096)) ;
#46468=CARTESIAN_POINT('Ctrl Pts',(-17.8947632869084,-28.7036870032994,
123.511208297081)) ;
#46469=CARTESIAN_POINT('Ctrl Pts',(-18.2560525173173,-28.8969658769049,
123.764590199396)) ;
#46470=CARTESIAN_POINT('Ctrl Pts',(-17.9677541226804,-28.716976796542,123.852806493769)) ;
#46471=CARTESIAN_POINT('Ctrl Pts',(-18.3343741631932,-28.9069185081643,
123.958600107731)) ;
#46472=CARTESIAN_POINT('Ctrl Pts',(-18.0656567609654,-28.7269294278014,
124.095304375433)) ;
#46473=CARTESIAN_POINT('Ctrl Pts',(-18.4449965967694,-28.916870475469,124.136207394979)) ;
#46474=CARTESIAN_POINT('Ctrl Pts',(-18.2039394803118,-28.7368813951061,
124.317317362258)) ;
#46475=CARTESIAN_POINT('Ctrl Pts',(-18.6328431511708,-28.9302377339328,
124.345197379133)) ;
#46476=CARTESIAN_POINT('Ctrl Pts',(-18.4387363200913,-28.7502486535699,
124.578542730155)) ;
#46477=CARTESIAN_POINT('Ctrl Pts',(-18.9269841780433,-28.9467545458819,
124.537227554656)) ;
#46478=CARTESIAN_POINT('Ctrl Pts',(-18.8064292376097,-28.7667654655191,
124.818587725884)) ;
#46479=CARTESIAN_POINT('Ctrl Pts',(-19.3414615997305,-28.9667804408883,
124.634301072555)) ;
#46480=CARTESIAN_POINT('Ctrl Pts',(-19.3245222155934,-28.7867913605254,
124.939922033055)) ;
#46481=CARTESIAN_POINT('Ctrl Pts',(-19.759850235118,-28.9865911710184,124.584749330712)) ;
#46482=CARTESIAN_POINT('Ctrl Pts',(-19.8475073460439,-28.8066020906556,
124.877979440127)) ;
#46483=CARTESIAN_POINT('Ctrl Pts',(-20.1396804889429,-29.0065683871483,
124.394678367115)) ;
#46484=CARTESIAN_POINT('Ctrl Pts',(-20.3222930272887,-28.8265793067854,
124.640387404646)) ;
#46485=CARTESIAN_POINT('Ctrl Pts',(-20.4305598017003,-29.0264952625436,
124.086638339135)) ;
#46486=CARTESIAN_POINT('Ctrl Pts',(-20.6858890813368,-28.8465061821807,
124.255335344324)) ;
#46487=CARTESIAN_POINT('Ctrl Pts',(-20.5992504484349,-29.0463167240198,
123.700349376274)) ;
#46488=CARTESIAN_POINT('Ctrl Pts',(-20.896748937638,-28.866327643657,123.772474684031)) ;
#46489=CARTESIAN_POINT('Ctrl Pts',(-20.626046085885,-29.0663910418292,123.274422117827)) ;
#46490=CARTESIAN_POINT('Ctrl Pts',(-20.930240651337,-28.8864019614663,123.240064582413)) ;
#46491=CARTESIAN_POINT('Ctrl Pts',(-20.506795066352,-29.0862390108371,122.869477985307)) ;
#46492=CARTESIAN_POINT('Ctrl Pts',(-20.7811745275789,-28.9062499304742,
122.733886817119)) ;
#46493=CARTESIAN_POINT('Ctrl Pts',(-20.2560944539261,-29.1061860449003,
122.527490551716)) ;
#46494=CARTESIAN_POINT('Ctrl Pts',(-20.4677973260097,-28.9261969645374,
122.306404432572)) ;
#46495=CARTESIAN_POINT('Ctrl Pts',(-19.9044790885967,-29.1260819958724,
122.292205363375)) ;
#46496=CARTESIAN_POINT('Ctrl Pts',(-20.0282780332881,-28.9460929155096,
122.012300463532)) ;
#46497=CARTESIAN_POINT('Ctrl Pts',(-19.493912747964,-29.1459774754907,122.190368785616)) ;
#46498=CARTESIAN_POINT('Ctrl Pts',(-19.5150711784553,-28.9659883951278,
121.885006525189)) ;
#46499=CARTESIAN_POINT('Ctrl Pts',(-19.0718902420119,-29.1659335864555,
122.234795537404)) ;
#46500=CARTESIAN_POINT('Ctrl Pts',(-18.987543756163,-28.9859445060926,121.940541079356)) ;
#46501=CARTESIAN_POINT('Ctrl Pts',(-18.6914823643913,-29.1858381344955,
122.420160422829)) ;
#46502=CARTESIAN_POINT('Ctrl Pts',(-18.5120357100849,-29.0058490541326,
122.172247469475)) ;
#46503=CARTESIAN_POINT('Ctrl Pts',(-18.3967545767849,-29.2057122588146,
122.723103992137)) ;
#46504=CARTESIAN_POINT('Ctrl Pts',(-18.1436273509991,-29.0257231784517,
122.550925494824)) ;
#46505=CARTESIAN_POINT('Ctrl Pts',(-18.2221384336728,-29.2257667888136,
123.11205184558)) ;
#46506=CARTESIAN_POINT('Ctrl Pts',(-17.9253569901024,-29.0457777084507,
123.037111210492)) ;
#46507=CARTESIAN_POINT('Ctrl Pts',(-18.190981362348,-29.2455743025736,123.532149795036)) ;
#46508=CARTESIAN_POINT('Ctrl Pts',(-17.8864107136343,-29.0655852222107,
123.562230606204)) ;
#46509=CARTESIAN_POINT('Ctrl Pts',(-18.3051612613185,-29.2655576583413,
123.941359506721)) ;
#46510=CARTESIAN_POINT('Ctrl Pts',(-18.0291344865639,-29.0855685779784,
124.073742812752)) ;
#46511=CARTESIAN_POINT('Ctrl Pts',(-18.5518768276411,-29.2854759609252,
124.285589142629)) ;
#46512=CARTESIAN_POINT('Ctrl Pts',(-18.3375275327191,-29.1054868805624,
124.504029337498)) ;
#46513=CARTESIAN_POINT('Ctrl Pts',(-18.8998033234493,-29.305344176371,124.525350894694)) ;
#46514=CARTESIAN_POINT('Ctrl Pts',(-18.7724331767996,-29.1253550960081,
124.803732067651)) ;
#46515=CARTESIAN_POINT('Ctrl Pts',(-19.3123749934706,-29.3253944931673,
124.632263603809)) ;
#46516=CARTESIAN_POINT('Ctrl Pts',(-19.2881479519155,-29.1454054128044,
124.937374691163)) ;
#46517=CARTESIAN_POINT('Ctrl Pts',(-19.7312061051285,-29.3451705550497,
124.593056434788)) ;
#46518=CARTESIAN_POINT('Ctrl Pts',(-19.8116842876558,-29.1651814746869,
124.888368150055)) ;
#46519=CARTESIAN_POINT('Ctrl Pts',(-20.1166949902579,-29.3652251607422,
124.411179447447)) ;
#46520=CARTESIAN_POINT('Ctrl Pts',(-20.2935470559368,-29.1852360803793,
124.661024000669)) ;
#46521=CARTESIAN_POINT('Ctrl Pts',(-20.413193850282,-29.3850188498981,124.112306030586)) ;
#46522=CARTESIAN_POINT('Ctrl Pts',(-20.6641709204212,-29.2050297695352,
124.287435707295)) ;
#46523=CARTESIAN_POINT('Ctrl Pts',(-20.5924104104792,-29.4049855414925,
123.727541429383)) ;
#46524=CARTESIAN_POINT('Ctrl Pts',(-20.8881946382118,-29.2249964611296,
123.806481690324)) ;
#46525=CARTESIAN_POINT('Ctrl Pts',(-20.6289121024175,-29.4249455872434,
123.304630992729)) ;
#46526=CARTESIAN_POINT('Ctrl Pts',(-20.9338249693073,-29.2449565068806,
123.277844260743)) ;
#46527=CARTESIAN_POINT('Ctrl Pts',(-20.5195428798539,-29.4448438473937,
122.895946670909)) ;
#46528=CARTESIAN_POINT('Ctrl Pts',(-20.7971171356574,-29.2648547670308,
122.766988876807)) ;
#46529=CARTESIAN_POINT('Ctrl Pts',(-20.2777340208433,-29.4647387629429,
122.548875500711)) ;
#46530=CARTESIAN_POINT('Ctrl Pts',(-20.4948597929885,-29.28474968258,122.33314837501)) ;
#46531=CARTESIAN_POINT('Ctrl Pts',(-19.9319526108886,-29.4846489433565,
122.30463596634)) ;
#46532=CARTESIAN_POINT('Ctrl Pts',(-20.0626359964947,-29.3046598629936,
122.027845909722)) ;
#46533=CARTESIAN_POINT('Ctrl Pts',(-19.5230900240382,-29.5045847424707,
122.192721165908)) ;
#46534=CARTESIAN_POINT('Ctrl Pts',(-19.5515593327172,-29.3245956621079,
121.887948224382)) ;
#46535=CARTESIAN_POINT('Ctrl Pts',(-19.1005503152697,-29.5245226041249,
122.227022561574)) ;
#46536=CARTESIAN_POINT('Ctrl Pts',(-19.0233846938744,-29.344533523762,121.930820617086)) ;
#46537=CARTESIAN_POINT('Ctrl Pts',(-18.7153085805982,-29.5444416507625,
122.403062773862)) ;
#46538=CARTESIAN_POINT('Ctrl Pts',(-18.5418309889796,-29.3644525703997,
122.150865733304)) ;
#46539=CARTESIAN_POINT('Ctrl Pts',(-18.4127914875677,-29.5643905488167,
122.700380117268)) ;
#46540=CARTESIAN_POINT('Ctrl Pts',(-18.1636813294162,-29.3844014684538,
122.522511403366)) ;
#46541=CARTESIAN_POINT('Ctrl Pts',(-18.2301756318706,-29.5842963762597,
123.082237752554)) ;
#46542=CARTESIAN_POINT('Ctrl Pts',(-17.9354075384507,-29.4043072958969,
122.999821271264)) ;
#46543=CARTESIAN_POINT('Ctrl Pts',(-18.1953684956847,-29.600879071625,123.433028159498)) ;
#46544=CARTESIAN_POINT('Ctrl Pts',(-17.8918934979895,-29.4208899912622,
123.438338526591)) ;
#46545=CARTESIAN_POINT('Ctrl Pts',(-18.24027601235,-29.6141532853487,123.708522208439)) ;
#46546=CARTESIAN_POINT('Ctrl Pts',(-17.9480247352152,-29.4341642049858,
123.782679410161)) ;
#46547=CARTESIAN_POINT('Ctrl Pts',(-18.3100397706379,-29.624200004548,123.907851703837)) ;
#46548=CARTESIAN_POINT('Ctrl Pts',(-18.0352295821613,-29.4442109241851,
124.031850013628)) ;
#46549=CARTESIAN_POINT('Ctrl Pts',(-18.4110966673818,-29.6340440391937,
124.088481382499)) ;
#46550=CARTESIAN_POINT('Ctrl Pts',(-18.1615379687603,-29.4540549588308,
124.257627504343)) ;
#46551=CARTESIAN_POINT('Ctrl Pts',(-18.5878370635189,-29.6473784240982,
124.305998065082)) ;
#46552=CARTESIAN_POINT('Ctrl Pts',(-18.3825117400926,-29.4673893437353,
124.529570908532)) ;
#46553=CARTESIAN_POINT('Ctrl Pts',(-18.8736671997377,-29.663965641398,124.512799362027)) ;
#46554=CARTESIAN_POINT('Ctrl Pts',(-18.7397290349317,-29.4839765610351,
124.788022651488)) ;
#46555=CARTESIAN_POINT('Ctrl Pts',(-19.2135861785788,-29.6805988534359,
124.610126724355)) ;
#46556=CARTESIAN_POINT('Ctrl Pts',(-19.1646822605817,-29.500609773073,124.90971077457)) ;
#46557=CARTESIAN_POINT('Ctrl Pts',(-19.4928463617671,-29.6938812957081,
124.61484124617)) ;
#46558=CARTESIAN_POINT('Ctrl Pts',(-19.5137203885275,-29.5138922153452,
124.915596996125)) ;
#46559=CARTESIAN_POINT('Ctrl Pts',(-19.6985621110543,-29.7037871836223,
124.582563757789)) ;
#46560=CARTESIAN_POINT('Ctrl Pts',(-19.7708729287446,-29.5237981032594,
124.875254844356)) ;
#46561=CARTESIAN_POINT('Ctrl Pts',(-19.8973061665422,-29.7137756017274,
124.514736011145)) ;
#46562=CARTESIAN_POINT('Ctrl Pts',(-20.0193014854552,-29.5337865213645,
124.790472867222)) ;
#46563=CARTESIAN_POINT('Ctrl Pts',(-20.0817838352029,-29.7237990289661,
124.412880710944)) ;
#46564=CARTESIAN_POINT('Ctrl Pts',(-20.2499022751864,-29.5438099486033,
124.663153811252)) ;
#46565=CARTESIAN_POINT('Ctrl Pts',(-20.2438922250525,-29.7337034600831,
124.282207760991)) ;
#46566=CARTESIAN_POINT('Ctrl Pts',(-20.4525327560064,-29.5537143797203,
124.499823981593)) ;
#46567=CARTESIAN_POINT('Ctrl Pts',(-20.4278473297483,-29.7469666126936,
124.072677307792)) ;
#46568=CARTESIAN_POINT('Ctrl Pts',(-20.6825120254526,-29.5669775323307,
124.237867726831)) ;
#46569=CARTESIAN_POINT('Ctrl Pts',(-20.5532267657517,-29.7602915105975,
123.81863575924)) ;
#46570=CARTESIAN_POINT('Ctrl Pts',(-20.8392151516731,-29.5803024302346,
123.9203381995)) ;
#46571=CARTESIAN_POINT('Ctrl Pts',(-20.607805933461,-29.7735472542131,123.545295424663)) ;
#46572=CARTESIAN_POINT('Ctrl Pts',(-20.9074394904579,-29.5935581738502,
123.578684401647)) ;
#46573=CARTESIAN_POINT('Ctrl Pts',(-20.6128379852353,-29.7835066276604,
123.336009205538)) ;
#46574=CARTESIAN_POINT('Ctrl Pts',(-20.9137330388378,-29.6035175472975,
123.317072430943)) ;
#46575=CARTESIAN_POINT('Ctrl Pts',(-20.5817572009049,-29.7934504515873,
123.129255120168)) ;
#46576=CARTESIAN_POINT('Ctrl Pts',(-20.8748846541773,-29.6134613712245,
123.058630457453)) ;
#46577=CARTESIAN_POINT('Ctrl Pts',(-20.5143943920179,-29.8034983957346,
122.929061237664)) ;
#46578=CARTESIAN_POINT('Ctrl Pts',(-20.7906838438031,-29.6235093153718,
122.808386846984)) ;
#46579=CARTESIAN_POINT('Ctrl Pts',(-20.4154235821622,-29.8133493669528,
122.747128077914)) ;
#46580=CARTESIAN_POINT('Ctrl Pts',(-20.666972739531,-29.6333602865899,122.580969032646)) ;
#46581=CARTESIAN_POINT('Ctrl Pts',(-20.2852290763675,-29.8233211843949,
122.582848316609)) ;
#46582=CARTESIAN_POINT('Ctrl Pts',(-20.504231739043,-29.643332104032,122.37561747521)) ;
#46583=CARTESIAN_POINT('Ctrl Pts',(-20.128053971246,-29.833316606687,122.443331037292)) ;
#46584=CARTESIAN_POINT('Ctrl Pts',(-20.3077646577954,-29.6533275263241,
122.20121873475)) ;
#46585=CARTESIAN_POINT('Ctrl Pts',(-19.9482825221474,-29.8433496718107,
122.333015974272)) ;
#46586=CARTESIAN_POINT('Ctrl Pts',(-20.0830517816903,-29.6633605914478,
122.063322483088)) ;
#46587=CARTESIAN_POINT('Ctrl Pts',(-19.7554396738521,-29.8532150044759,
122.25669701737)) ;
#46588=CARTESIAN_POINT('Ctrl Pts',(-19.8419990547799,-29.673225924113,121.967921099706)) ;
#46589=CARTESIAN_POINT('Ctrl Pts',(-19.5504291193949,-29.8631755470735,
122.214013364722)) ;
#46590=CARTESIAN_POINT('Ctrl Pts',(-19.5857362753535,-29.6831864667106,
121.914563791572)) ;
#46591=CARTESIAN_POINT('Ctrl Pts',(-19.3395885460387,-29.8732092325752,
122.207884141582)) ;
#46592=CARTESIAN_POINT('Ctrl Pts',(-19.3221856204255,-29.6932201522123,
121.906899471747)) ;
#46593=CARTESIAN_POINT('Ctrl Pts',(-19.1338922316553,-29.8830940645654,
122.237651972592)) ;
#46594=CARTESIAN_POINT('Ctrl Pts',(-19.0650645565921,-29.7031049842026,
121.944106565339)) ;
#46595=CARTESIAN_POINT('Ctrl Pts',(-18.93291875455,-29.8931614913253,122.303910124113)) ;
#46596=CARTESIAN_POINT('Ctrl Pts',(-18.8138468784926,-29.7131724109624,
122.026926609439)) ;
#46597=CARTESIAN_POINT('Ctrl Pts',(-18.7505843551157,-29.9029999804841,
122.40163291113)) ;
#46598=CARTESIAN_POINT('Ctrl Pts',(-18.5859272208204,-29.7230109001213,
122.149077864787)) ;
#46599=CARTESIAN_POINT('Ctrl Pts',(-18.5841468216196,-29.9130634616742,
122.532193860216)) ;
#46600=CARTESIAN_POINT('Ctrl Pts',(-18.3778786570836,-29.7330743813114,
122.312276880641)) ;
#46601=CARTESIAN_POINT('Ctrl Pts',(-18.445382712112,-29.9229576194894,122.687180679488)) ;
#46602=CARTESIAN_POINT('Ctrl Pts',(-18.2044212593036,-29.7429685391265,
122.506008820073)) ;
#46603=CARTESIAN_POINT('Ctrl Pts',(-18.3346512088788,-29.9328994762337,
122.864415832755)) ;
#46604=CARTESIAN_POINT('Ctrl Pts',(-18.0660044708574,-29.7529103958708,
122.727551566468)) ;
#46605=CARTESIAN_POINT('Ctrl Pts',(-18.2558045501675,-29.9429019539051,
123.059389134583)) ;
#46606=CARTESIAN_POINT('Ctrl Pts',(-17.9674436496093,-29.7629128735422,
122.971267274101)) ;
#46607=CARTESIAN_POINT('Ctrl Pts',(-18.2122015809126,-29.9529367582094,
123.265783338575)) ;
#46608=CARTESIAN_POINT('Ctrl Pts',(-17.9129372902024,-29.7729476778465,
123.229259453664)) ;
#46609=CARTESIAN_POINT('Ctrl Pts',(-18.204883750954,-29.962781635055,123.472638058067)) ;
#46610=CARTESIAN_POINT('Ctrl Pts',(-17.9037873257415,-29.7827925546922,
123.487828320676)) ;
#46611=CARTESIAN_POINT('Ctrl Pts',(-18.2336070809338,-29.9727675146106,
123.680563989553)) ;
#46612=CARTESIAN_POINT('Ctrl Pts',(-17.9396889314393,-29.7927784342477,
123.747736250522)) ;
#46613=CARTESIAN_POINT('Ctrl Pts',(-18.2975455094374,-29.9827022449691,
123.879438238451)) ;
#46614=CARTESIAN_POINT('Ctrl Pts',(-18.0196096204046,-29.8027131646062,
123.996330158484)) ;
#46615=CARTESIAN_POINT('Ctrl Pts',(-18.3963927749203,-29.992760057282,124.066318685816)) ;
#46616=CARTESIAN_POINT('Ctrl Pts',(-18.1431663387283,-29.8127709769191,
124.229931834435)) ;
#46617=CARTESIAN_POINT('Ctrl Pts',(-18.5228873624992,-30.0025806494063,
124.229532798022)) ;
#46618=CARTESIAN_POINT('Ctrl Pts',(-18.3012830487912,-29.8225915690435,
124.433951656902)) ;
#46619=CARTESIAN_POINT('Ctrl Pts',(-18.6793976240298,-30.0126472350161,
124.371920994788)) ;
#46620=CARTESIAN_POINT('Ctrl Pts',(-18.4969190824133,-29.8326581546532,
124.611938648179)) ;
#46621=CARTESIAN_POINT('Ctrl Pts',(-18.8553834505121,-30.0225468155979,
124.483111642296)) ;
#46622=CARTESIAN_POINT('Ctrl Pts',(-18.7169004533599,-29.8425577352351,
124.750929340355)) ;
#46623=CARTESIAN_POINT('Ctrl Pts',(-19.0508479412311,-30.0325984152762,
124.563308795256)) ;
#46624=CARTESIAN_POINT('Ctrl Pts',(-18.9612300162177,-29.8526093349133,
124.851178041536)) ;
#46625=CARTESIAN_POINT('Ctrl Pts',(-19.2536676439756,-30.0424726016932,
124.607724013289)) ;
#46626=CARTESIAN_POINT('Ctrl Pts',(-19.2147547487882,-29.8624835213303,
124.90669960071)) ;
#46627=CARTESIAN_POINT('Ctrl Pts',(-19.4648637458808,-30.0525290775741,
124.616538418553)) ;
#46628=CARTESIAN_POINT('Ctrl Pts',(-19.4787496446823,-29.8725399972112,
124.917720031893)) ;
#46629=CARTESIAN_POINT('Ctrl Pts',(-19.6710664677573,-30.0624220088767,
124.589069886953)) ;
#46630=CARTESIAN_POINT('Ctrl Pts',(-19.7365039466463,-29.8824329285138,
124.883386677831)) ;
#46631=CARTESIAN_POINT('Ctrl Pts',(-19.8727094603673,-30.0724847875893,
124.525198764561)) ;
#46632=CARTESIAN_POINT('Ctrl Pts',(-19.9885582400929,-29.8924957072264,
124.803550123632)) ;
#46633=CARTESIAN_POINT('Ctrl Pts',(-20.0561959945725,-30.0823273131705,
124.429495466673)) ;
#46634=CARTESIAN_POINT('Ctrl Pts',(-20.2179182729383,-29.9023382328076,
124.683922711731)) ;
#46635=CARTESIAN_POINT('Ctrl Pts',(-20.2230137933602,-30.0923180785953,
124.301917210482)) ;
#46636=CARTESIAN_POINT('Ctrl Pts',(-20.4264420362186,-29.9123289982325,
124.524451584241)) ;
#46637=CARTESIAN_POINT('Ctrl Pts',(-20.364251196426,-30.1022461545934,124.148229737283)) ;
#46638=CARTESIAN_POINT('Ctrl Pts',(-20.6029907905239,-29.9222570742305,
124.332343420825)) ;
#46639=CARTESIAN_POINT('Ctrl Pts',(-20.4776444590878,-30.1122340649804,
123.971491927839)) ;
#46640=CARTESIAN_POINT('Ctrl Pts',(-20.7447343008597,-29.9322449846175,
124.11142218186)) ;
#46641=CARTESIAN_POINT('Ctrl Pts',(-20.5586797306925,-30.1222699771053,
123.776696813867)) ;
#46642=CARTESIAN_POINT('Ctrl Pts',(-20.8460304545597,-29.9422808967425,
123.867929241378)) ;
#46643=CARTESIAN_POINT('Ctrl Pts',(-20.6041716223551,-30.132124989953,123.57455346389)) ;
#46644=CARTESIAN_POINT('Ctrl Pts',(-20.9028976475888,-29.9521359095901,
123.61524963978)) ;
#46645=CARTESIAN_POINT('Ctrl Pts',(-20.6143059846248,-30.1421239358693,
123.364622415793)) ;
#46646=CARTESIAN_POINT('Ctrl Pts',(-20.9155677101948,-29.9621348555064,
123.352835793816)) ;
#46647=CARTESIAN_POINT('Ctrl Pts',(-20.5882986886202,-30.1520208483173,
123.158157718472)) ;
#46648=CARTESIAN_POINT('Ctrl Pts',(-20.8830605294398,-29.9720317679544,
123.094753953415)) ;
#46649=CARTESIAN_POINT('Ctrl Pts',(-20.5259041849406,-30.1620746464108,
122.956241447257)) ;
#46650=CARTESIAN_POINT('Ctrl Pts',(-20.805069403928,-29.9820855660479,122.84235819033)) ;
#46651=CARTESIAN_POINT('Ctrl Pts',(-20.4310894011429,-30.1719555672375,
122.771388410386)) ;
#46652=CARTESIAN_POINT('Ctrl Pts',(-20.6865523391872,-29.9919664868746,
122.611290225832)) ;
#46653=CARTESIAN_POINT('Ctrl Pts',(-20.3043799559765,-30.1819600932352,
122.603543945781)) ;
#46654=CARTESIAN_POINT('Ctrl Pts',(-20.5281670015566,-30.0019710128723,
122.40148341337)) ;
#46655=CARTESIAN_POINT('Ctrl Pts',(-20.1506815547945,-30.1919440568527,
122.460549966187)) ;
#46656=CARTESIAN_POINT('Ctrl Pts',(-20.3360451640396,-30.0119549764898,
122.222739387201)) ;
#46657=CARTESIAN_POINT('Ctrl Pts',(-19.9734411230241,-30.201983697404,122.345973899521)) ;
#46658=CARTESIAN_POINT('Ctrl Pts',(-20.1144958155581,-30.0219946170411,
122.079517699187)) ;
#46659=CARTESIAN_POINT('Ctrl Pts',(-19.782871813628,-30.2118277230187,122.26527172513)) ;
#46660=CARTESIAN_POINT('Ctrl Pts',(-19.8762838854574,-30.0318386426558,
121.978637774701)) ;
#46661=CARTESIAN_POINT('Ctrl Pts',(-19.5783094050863,-30.221818728836,122.217602614152)) ;
#46662=CARTESIAN_POINT('Ctrl Pts',(-19.6205810796489,-30.0418296484732,
121.919049659348)) ;
#46663=CARTESIAN_POINT('Ctrl Pts',(-19.3675704704491,-30.2318565203682,
122.206603916104)) ;
#46664=CARTESIAN_POINT('Ctrl Pts',(-19.3571576412147,-30.0518674400053,
121.905299416152)) ;
#46665=CARTESIAN_POINT('Ctrl Pts',(-19.1621069099491,-30.2417009201566,
122.231506538147)) ;
#46666=CARTESIAN_POINT('Ctrl Pts',(-19.1003268169004,-30.0617118397937,
121.936426083733)) ;
#46667=CARTESIAN_POINT('Ctrl Pts',(-18.9611771135097,-30.2516857207133,
122.292157840187)) ;
#46668=CARTESIAN_POINT('Ctrl Pts',(-18.8491638611297,-30.0716966403505,
122.012238721689)) ;
#46669=CARTESIAN_POINT('Ctrl Pts',(-18.7745889266096,-30.2616252441245,
122.386291238736)) ;
#46670=CARTESIAN_POINT('Ctrl Pts',(-18.6159274223169,-30.0816361637616,
122.129904287764)) ;
#46671=CARTESIAN_POINT('Ctrl Pts',(-18.6055578608464,-30.2716649632255,
122.512666339246)) ;
#46672=CARTESIAN_POINT('Ctrl Pts',(-18.4046377386934,-30.0916758828626,
122.287871780247)) ;
#46673=CARTESIAN_POINT('Ctrl Pts',(-18.4631237680064,-30.2815531351448,
122.664098676228)) ;
#46674=CARTESIAN_POINT('Ctrl Pts',(-18.2265933390173,-30.1015640547819,
122.477161788335)) ;
#46675=CARTESIAN_POINT('Ctrl Pts',(-18.3476602750316,-30.2915426975618,
122.839512639782)) ;
#46676=CARTESIAN_POINT('Ctrl Pts',(-18.0822626446461,-30.1115536171989,
122.696428624441)) ;
#46677=CARTESIAN_POINT('Ctrl Pts',(-18.264811021222,-30.3015010697565,123.031774138297)) ;
#46678=CARTESIAN_POINT('Ctrl Pts',(-17.9786995241896,-30.1215119893936,
122.936755300708)) ;
#46679=CARTESIAN_POINT('Ctrl Pts',(-18.2163954880168,-30.3114011439872,
123.234202863219)) ;
#46680=CARTESIAN_POINT('Ctrl Pts',(-17.9181786121953,-30.1314120636243,
123.189791746356)) ;
#46681=CARTESIAN_POINT('Ctrl Pts',(-18.2037078203567,-30.3214472403608,
123.445012427325)) ;
#46682=CARTESIAN_POINT('Ctrl Pts',(-17.9023177046355,-30.1414581599979,
123.453303427384)) ;
#46683=CARTESIAN_POINT('Ctrl Pts',(-18.2274762171961,-30.3313558243579,
123.651971116123)) ;
#46684=CARTESIAN_POINT('Ctrl Pts',(-17.9320269697077,-30.151366743995,123.712002752069)) ;
#46685=CARTESIAN_POINT('Ctrl Pts',(-18.2870541787712,-30.3413664029488,
123.853819127414)) ;
#46686=CARTESIAN_POINT('Ctrl Pts',(-18.0064982865296,-30.1613773225859,
123.964313150607)) ;
#46687=CARTESIAN_POINT('Ctrl Pts',(-18.3813325232713,-30.3513955610616,
124.042419862782)) ;
#46688=CARTESIAN_POINT('Ctrl Pts',(-18.1243449648106,-30.1714064806987,
124.200064581345)) ;
#46689=CARTESIAN_POINT('Ctrl Pts',(-18.5044666604839,-30.3612484428997,
124.20896945013)) ;
#46690=CARTESIAN_POINT('Ctrl Pts',(-18.2782623863857,-30.1812593625368,
124.408253321648)) ;
#46691=CARTESIAN_POINT('Ctrl Pts',(-18.6558439163059,-30.3712080040507,
124.353634907533)) ;
#46692=CARTESIAN_POINT('Ctrl Pts',(-18.4674836005063,-30.1912189236878,
124.589086196399)) ;
#46693=CARTESIAN_POINT('Ctrl Pts',(-18.8316171646393,-30.3812464386398,
124.470406891884)) ;
#46694=CARTESIAN_POINT('Ctrl Pts',(-18.687199388826,-30.2012573582769,124.735052040734)) ;
#46695=CARTESIAN_POINT('Ctrl Pts',(-19.0216991726386,-30.3911197108669,
124.553872844899)) ;
#46696=CARTESIAN_POINT('Ctrl Pts',(-18.9248025261078,-30.211130630504,124.839385850343)) ;
#46697=CARTESIAN_POINT('Ctrl Pts',(-19.2274128061745,-30.4011929528604,
124.603980425918)) ;
#46698=CARTESIAN_POINT('Ctrl Pts',(-19.1819439103011,-30.2212038724976,
124.902021223868)) ;
#46699=CARTESIAN_POINT('Ctrl Pts',(-19.4334667110816,-30.4110132843935,
124.617542684811)) ;
#46700=CARTESIAN_POINT('Ctrl Pts',(-19.4395127810917,-30.2310242040306,
124.918975069592)) ;
#46701=CARTESIAN_POINT('Ctrl Pts',(-19.64406951049,-30.4210919456203,124.594736003978)) ;
#46702=CARTESIAN_POINT('Ctrl Pts',(-19.7027659038404,-30.2411028652574,
124.890467615748)) ;
#46703=CARTESIAN_POINT('Ctrl Pts',(-19.8430448442677,-30.4309435409145,
124.537080259069)) ;
#46704=CARTESIAN_POINT('Ctrl Pts',(-19.9514865660436,-30.2509544605516,
124.818398357271)) ;
#46705=CARTESIAN_POINT('Ctrl Pts',(-20.0331712259711,-30.4410166761433,
124.443902678436)) ;
#46706=CARTESIAN_POINT('Ctrl Pts',(-20.1891444820223,-30.2610275957804,
124.701927251076)) ;
#46707=CARTESIAN_POINT('Ctrl Pts',(-20.200339647076,-30.4508591116683,124.32192778539)) ;
#46708=CARTESIAN_POINT('Ctrl Pts',(-20.398106604193,-30.2708700313055,124.549458419366)) ;
#46709=CARTESIAN_POINT('Ctrl Pts',(-20.3462888347876,-30.4608398808017,
124.171191115801)) ;
#46710=CARTESIAN_POINT('Ctrl Pts',(-20.5805436587888,-30.2808508004389,
124.361037704408)) ;
#46711=CARTESIAN_POINT('Ctrl Pts',(-20.4639585613339,-30.4708569820456,
123.996541687798)) ;
#46712=CARTESIAN_POINT('Ctrl Pts',(-20.7276313527105,-30.2908679016827,
124.142726286126)) ;
#46713=CARTESIAN_POINT('Ctrl Pts',(-20.5487810389583,-30.4807454296474,
123.806730562509)) ;
#46714=CARTESIAN_POINT('Ctrl Pts',(-20.8336603363903,-30.3007563492846,
123.905461600815)) ;
#46715=CARTESIAN_POINT('Ctrl Pts',(-20.6002259549947,-30.4908011438283,
123.601702375123)) ;
#46716=CARTESIAN_POINT('Ctrl Pts',(-20.897966874934,-30.3108120634654,123.649176787978)) ;
#46717=CARTESIAN_POINT('Ctrl Pts',(-20.615052892875,-30.5006763502421,123.394610916813)) ;
#46718=CARTESIAN_POINT('Ctrl Pts',(-20.916501105489,-30.3206872698793,123.390311340077)) ;
#46719=CARTESIAN_POINT('Ctrl Pts',(-20.5939426510148,-30.5106714027149,
123.185552599972)) ;
#46720=CARTESIAN_POINT('Ctrl Pts',(-20.8901135577961,-30.330682322352,123.128988240062)) ;
#46721=CARTESIAN_POINT('Ctrl Pts',(-20.536367759922,-30.520693286677,122.982872051517)) ;
#46722=CARTESIAN_POINT('Ctrl Pts',(-20.8181453544106,-30.3407042063141,
122.87563748445)) ;
#46723=CARTESIAN_POINT('Ctrl Pts',(-20.4457706611139,-30.5305972592063,
122.795404854875)) ;
#46724=CARTESIAN_POINT('Ctrl Pts',(-20.7048988527743,-30.3506081788434,
122.641302484579)) ;
#46725=CARTESIAN_POINT('Ctrl Pts',(-20.3232033140456,-30.5405857558672,
122.624895059131)) ;
#46726=CARTESIAN_POINT('Ctrl Pts',(-20.5516896929561,-30.3605966755043,
122.428164932682)) ;
#46727=CARTESIAN_POINT('Ctrl Pts',(-20.1731729387286,-30.5505495531152,
122.478730184432)) ;
#46728=CARTESIAN_POINT('Ctrl Pts',(-20.3641515811051,-30.3705604727523,
122.245458339291)) ;
#46729=CARTESIAN_POINT('Ctrl Pts',(-20.0013435844137,-30.5604535764232,
122.361105057577)) ;
#46730=CARTESIAN_POINT('Ctrl Pts',(-20.1493641423966,-30.3804644960603,
122.098426355358)) ;
#46731=CARTESIAN_POINT('Ctrl Pts',(-19.8086729775666,-30.5705140797448,
122.27392287476)) ;
#46732=CARTESIAN_POINT('Ctrl Pts',(-19.9085262576648,-30.3905249993819,
121.989448658708)) ;
#46733=CARTESIAN_POINT('Ctrl Pts',(-19.6082855481598,-30.5803546148847,
122.222396123201)) ;
#46734=CARTESIAN_POINT('Ctrl Pts',(-19.6580405512922,-30.4003655345218,
121.925039834791)) ;
#46735=CARTESIAN_POINT('Ctrl Pts',(-19.3974190538605,-30.5904168355893,
122.20582075455)) ;
#46736=CARTESIAN_POINT('Ctrl Pts',(-19.3944577950573,-30.4104277552264,
121.904320740095)) ;
#46737=CARTESIAN_POINT('Ctrl Pts',(-19.1903195961826,-30.6003139893655,
122.225997239462)) ;
#46738=CARTESIAN_POINT('Ctrl Pts',(-19.1355824753204,-30.4203249090026,
121.929541442186)) ;
#46739=CARTESIAN_POINT('Ctrl Pts',(-18.9890100939322,-30.610245122751,122.281343791059)) ;
#46740=CARTESIAN_POINT('Ctrl Pts',(-18.8839449757999,-30.4302560423881,
121.998725090014)) ;
#46741=CARTESIAN_POINT('Ctrl Pts',(-18.7983550338524,-30.6202874978967,
122.372017641209)) ;
#46742=CARTESIAN_POINT('Ctrl Pts',(-18.6456264180008,-30.4402984175338,
122.112067478881)) ;
#46743=CARTESIAN_POINT('Ctrl Pts',(-18.6289139729558,-30.6301734356628,
122.492389628347)) ;
#46744=CARTESIAN_POINT('Ctrl Pts',(-18.4338243469554,-30.4501843553,122.26253329312)) ;
#46745=CARTESIAN_POINT('Ctrl Pts',(-18.4811125942436,-30.6401692786477,
122.641749676501)) ;
#46746=CARTESIAN_POINT('Ctrl Pts',(-18.2490727524169,-30.4601801982848,
122.449233759781)) ;
#46747=CARTESIAN_POINT('Ctrl Pts',(-18.3621388083306,-30.6501112565263,
122.813609855738)) ;
#46748=CARTESIAN_POINT('Ctrl Pts',(-18.1003554686225,-30.4701221761634,
122.664059702261)) ;
#46749=CARTESIAN_POINT('Ctrl Pts',(-18.2744107318474,-30.6600706310073,
123.003708981063)) ;
#46750=CARTESIAN_POINT('Ctrl Pts',(-17.9906956060769,-30.4800815506444,
122.901684237793)) ;
#46751=CARTESIAN_POINT('Ctrl Pts',(-18.2207100016037,-30.6700672468411,
123.206915248933)) ;
#46752=CARTESIAN_POINT('Ctrl Pts',(-17.9235701573867,-30.4900781664782,
123.15569235127)) ;
#46753=CARTESIAN_POINT('Ctrl Pts',(-18.2033237827632,-30.6801014654146,
123.4171423923)) ;
#46754=CARTESIAN_POINT('Ctrl Pts',(-17.9018377987369,-30.5001123850517,
123.418476175523)) ;
#46755=CARTESIAN_POINT('Ctrl Pts',(-18.2221037500632,-30.6899545326252,
123.623428518409)) ;
#46756=CARTESIAN_POINT('Ctrl Pts',(-17.9253133851979,-30.5099654522623,
123.676335153502)) ;
#46757=CARTESIAN_POINT('Ctrl Pts',(-18.2764164848045,-30.6999147905028,
123.825650685452)) ;
#46758=CARTESIAN_POINT('Ctrl Pts',(-17.9932051454583,-30.5199257101399,
123.929113114964)) ;
#46759=CARTESIAN_POINT('Ctrl Pts',(-18.3658619188668,-30.7099438172084,
124.016591993771)) ;
#46760=CARTESIAN_POINT('Ctrl Pts',(-18.1050124820995,-30.5299547368455,
124.167789386581)) ;
#46761=CARTESIAN_POINT('Ctrl Pts',(-18.4856036512729,-30.7198540242428,
124.187076921124)) ;
#46762=CARTESIAN_POINT('Ctrl Pts',(-18.2546907015098,-30.5398649438799,
124.380895877564)) ;
#46763=CARTESIAN_POINT('Ctrl Pts',(-18.6331183540979,-30.7297889348904,
124.334947217682)) ;
#46764=CARTESIAN_POINT('Ctrl Pts',(-18.4390851726062,-30.5497998545275,
124.565733591977)) ;
#46765=CARTESIAN_POINT('Ctrl Pts',(-18.805998293057,-30.7398300650696,124.456072455855)) ;
#46766=CARTESIAN_POINT('Ctrl Pts',(-18.6551854058701,-30.5598409847068,
124.71713937099)) ;
#46767=CARTESIAN_POINT('Ctrl Pts',(-18.9943042437929,-30.7497172054396,
124.544111417618)) ;
#46768=CARTESIAN_POINT('Ctrl Pts',(-18.8905691522215,-30.5697281250767,
124.827187732175)) ;
#46769=CARTESIAN_POINT('Ctrl Pts',(-19.1970545158081,-30.7597094829755,
124.599022917554)) ;
#46770=CARTESIAN_POINT('Ctrl Pts',(-19.1440074490238,-30.5797204026127,
124.895826199179)) ;
#46771=CARTESIAN_POINT('Ctrl Pts',(-19.4053746987768,-30.7696580262439,
124.617756988556)) ;
#46772=CARTESIAN_POINT('Ctrl Pts',(-19.4044083048242,-30.589668945881,124.919242868932)) ;
#46773=CARTESIAN_POINT('Ctrl Pts',(-19.6135329763721,-30.7795947010611,
124.60035612135)) ;
#46774=CARTESIAN_POINT('Ctrl Pts',(-19.6646066985077,-30.5996056206982,
124.897490650973)) ;
#46775=CARTESIAN_POINT('Ctrl Pts',(-19.8165585167842,-30.7895781219974,
124.5470606735)) ;
#46776=CARTESIAN_POINT('Ctrl Pts',(-19.9183885696594,-30.6095890416346,
124.830870140857)) ;
#46777=CARTESIAN_POINT('Ctrl Pts',(-20.0081989085124,-30.7996204371867,
124.458507416817)) ;
#46778=CARTESIAN_POINT('Ctrl Pts',(-20.1579384638186,-30.6196313568238,
124.720177686834)) ;
#46779=CARTESIAN_POINT('Ctrl Pts',(-20.1782668651698,-30.8094607546259,
124.340716223305)) ;
#46780=CARTESIAN_POINT('Ctrl Pts',(-20.3705238609549,-30.629471674263,124.572936951925)) ;
#46781=CARTESIAN_POINT('Ctrl Pts',(-20.328476682033,-30.8194904586834,124.192735300873)) ;
#46782=CARTESIAN_POINT('Ctrl Pts',(-20.5582851075911,-30.6395013783205,
124.387959911787)) ;
#46783=CARTESIAN_POINT('Ctrl Pts',(-20.4501392005903,-30.8295114154059,
124.020744611247)) ;
#46784=CARTESIAN_POINT('Ctrl Pts',(-20.7103623023063,-30.649522335043,124.172970910553)) ;
#46785=CARTESIAN_POINT('Ctrl Pts',(-20.5391909200879,-30.8393779577095,
123.833391228608)) ;
#46786=CARTESIAN_POINT('Ctrl Pts',(-20.8216762306296,-30.6593888773466,
123.938777584491)) ;
#46787=CARTESIAN_POINT('Ctrl Pts',(-20.595495855653,-30.8494490576546,123.629308992589)) ;
#46788=CARTESIAN_POINT('Ctrl Pts',(-20.8920560097773,-30.6694599772918,
123.683674797178)) ;
#46789=CARTESIAN_POINT('Ctrl Pts',(-20.6150525003595,-30.8592911318322,
123.423316450362)) ;
#46790=CARTESIAN_POINT('Ctrl Pts',(-20.9165006065021,-30.6793020514693,
123.426182698946)) ;
#46791=CARTESIAN_POINT('Ctrl Pts',(-20.5991170580468,-30.8692519264192,
123.214521188728)) ;
#46792=CARTESIAN_POINT('Ctrl Pts',(-20.8965796706122,-30.6892628460564,
123.165188338066)) ;
#46793=CARTESIAN_POINT('Ctrl Pts',(-20.546363865341,-30.8792897993201,123.010200870518)) ;
#46794=CARTESIAN_POINT('Ctrl Pts',(-20.8306367978976,-30.6993007189572,
122.909788435439)) ;
#46795=CARTESIAN_POINT('Ctrl Pts',(-20.4606968836195,-30.8891640848642,
122.821085418058)) ;
#46796=CARTESIAN_POINT('Ctrl Pts',(-20.7235512011237,-30.7091750045013,
122.673393853135)) ;
#46797=CARTESIAN_POINT('Ctrl Pts',(-20.3411946934181,-30.8992338352781,
122.646376318982)) ;
#46798=CARTESIAN_POINT('Ctrl Pts',(-20.5741723489282,-30.7192447549152,
122.45500866596)) ;
#46799=CARTESIAN_POINT('Ctrl Pts',(-20.19669738145,-30.9090671198127,122.498514065535)) ;
#46800=CARTESIAN_POINT('Ctrl Pts',(-20.3935486500737,-30.7290780394499,
122.270181067719)) ;
#46801=CARTESIAN_POINT('Ctrl Pts',(-20.025723038719,-30.9190974606128,122.375099669013)) ;
#46802=CARTESIAN_POINT('Ctrl Pts',(-20.1798297267143,-30.7391083802499,
122.115914599699)) ;
#46803=CARTESIAN_POINT('Ctrl Pts',(-19.8356036746159,-30.9291293846124,
122.283783083488)) ;
#46804=CARTESIAN_POINT('Ctrl Pts',(-19.9421798972545,-30.7491403042495,
122.001770363478)) ;
#46805=CARTESIAN_POINT('Ctrl Pts',(-19.6367747487569,-30.9389579195483,
122.227591752257)) ;
#46806=CARTESIAN_POINT('Ctrl Pts',(-19.6936420289257,-30.7589688391854,
121.931532551847)) ;
#46807=CARTESIAN_POINT('Ctrl Pts',(-19.4278031799893,-30.948951697313,122.205853025162)) ;
#46808=CARTESIAN_POINT('Ctrl Pts',(-19.4324272173847,-30.7689626169501,
121.904361062443)) ;
#46809=CARTESIAN_POINT('Ctrl Pts',(-19.2175414225101,-30.9589794077985,
122.221194257031)) ;
#46810=CARTESIAN_POINT('Ctrl Pts',(-19.1696001927807,-30.7789903274356,
121.923539411999)) ;
#46811=CARTESIAN_POINT('Ctrl Pts',(-19.0159184250757,-30.9688678186325,
122.271841404524)) ;
#46812=CARTESIAN_POINT('Ctrl Pts',(-18.9175710994844,-30.7888787382696,
121.986850390428)) ;
#46813=CARTESIAN_POINT('Ctrl Pts',(-18.8243211742747,-30.978844669168,122.357145110244)) ;
#46814=CARTESIAN_POINT('Ctrl Pts',(-18.6780751168425,-30.7988555888051,
122.09348195838)) ;
#46815=CARTESIAN_POINT('Ctrl Pts',(-18.6501372622533,-30.9888364657185,
122.474607486696)) ;
#46816=CARTESIAN_POINT('Ctrl Pts',(-18.4603462228554,-30.8088473853556,
122.240311680779)) ;
#46817=CARTESIAN_POINT('Ctrl Pts',(-18.4985386548746,-30.9988724718122,
122.621327863081)) ;
#46818=CARTESIAN_POINT('Ctrl Pts',(-18.2708493730239,-30.8188833914493,
122.42371347671)) ;
#46819=CARTESIAN_POINT('Ctrl Pts',(-18.3767267027261,-31.008723206075,122.788826198165)) ;
#46820=CARTESIAN_POINT('Ctrl Pts',(-18.1185854663055,-30.8287341257121,
122.633088418445)) ;
#46821=CARTESIAN_POINT('Ctrl Pts',(-18.2842463817907,-31.0187144646032,
122.977386152329)) ;
#46822=CARTESIAN_POINT('Ctrl Pts',(-18.0029869058182,-30.8387253842403,
122.868789450594)) ;
#46823=CARTESIAN_POINT('Ctrl Pts',(-18.2262044455862,-31.0286323595064,
123.177677702795)) ;
#46824=CARTESIAN_POINT('Ctrl Pts',(-17.9304364001845,-30.8486432791435,
123.119155041273)) ;
#46825=CARTESIAN_POINT('Ctrl Pts',(-18.2035238002497,-31.0386605011694,
123.387260137324)) ;
#46826=CARTESIAN_POINT('Ctrl Pts',(-17.9020877614499,-30.8586714208065,
123.3811332833)) ;
#46827=CARTESIAN_POINT('Ctrl Pts',(-18.2172919464805,-31.0485456692853,
123.594625950143)) ;
#46828=CARTESIAN_POINT('Ctrl Pts',(-17.9193001864898,-30.8685565889224,
123.640341140622)) ;
#46829=CARTESIAN_POINT('Ctrl Pts',(-18.2668826506638,-31.0585350327913,
123.79869899324)) ;
#46830=CARTESIAN_POINT('Ctrl Pts',(-17.9812908655851,-30.8785459524284,
123.895432047551)) ;
#46831=CARTESIAN_POINT('Ctrl Pts',(-18.3519971283237,-31.0685761678013,
123.991875632271)) ;
#46832=CARTESIAN_POINT('Ctrl Pts',(-18.0876859531419,-30.8885870874385,
124.136901868337)) ;
#46833=CARTESIAN_POINT('Ctrl Pts',(-18.4666381472819,-31.0784088359894,
124.163882158032)) ;
#46834=CARTESIAN_POINT('Ctrl Pts',(-18.2309896742768,-30.8984197556265,
124.35190954771)) ;
#46835=CARTESIAN_POINT('Ctrl Pts',(-18.6113111204173,-31.0884027389439,
124.31623927594)) ;
#46836=CARTESIAN_POINT('Ctrl Pts',(-18.4118327452605,-30.908413658581,124.542354351649)) ;
#46837=CARTESIAN_POINT('Ctrl Pts',(-18.7811066172618,-31.0984320240284,
124.441246279883)) ;
#46838=CARTESIAN_POINT('Ctrl Pts',(-18.6240784848063,-30.9184429436655,
124.698611210536)) ;
#46839=CARTESIAN_POINT('Ctrl Pts',(-18.9669894085724,-31.1083075524703,
124.533744474352)) ;
#46840=CARTESIAN_POINT('Ctrl Pts',(-18.856433654806,-30.9283184721074,124.814232093926)) ;
#46841=CARTESIAN_POINT('Ctrl Pts',(-19.1685234135853,-31.1183078350863,
124.593519235339)) ;
#46842=CARTESIAN_POINT('Ctrl Pts',(-19.1083519713591,-30.9383187547235,
124.888948210804)) ;
#46843=CARTESIAN_POINT('Ctrl Pts',(-19.3755624886653,-31.1282198511434,
124.617355261767)) ;
#46844=CARTESIAN_POINT('Ctrl Pts',(-19.3671515658204,-30.9482307707805,
124.918740815708)) ;
#46845=CARTESIAN_POINT('Ctrl Pts',(-19.5862881147713,-31.1382619264824,
124.604773299215)) ;
#46846=CARTESIAN_POINT('Ctrl Pts',(-19.6305583756846,-30.9582728461195,
124.903010863025)) ;
#46847=CARTESIAN_POINT('Ctrl Pts',(-19.7887432035316,-31.1481617591385,
124.556475850266)) ;
#46848=CARTESIAN_POINT('Ctrl Pts',(-19.8836271403426,-30.9681726787756,
124.842636496997)) ;
#46849=CARTESIAN_POINT('Ctrl Pts',(-19.9816984118981,-31.1581541597165,
124.473418066137)) ;
#46850=CARTESIAN_POINT('Ctrl Pts',(-20.1248202353029,-30.9781650793536,
124.738811837685)) ;
#46851=CARTESIAN_POINT('Ctrl Pts',(-20.1578289058847,-31.1681881814759,
124.357322944161)) ;
#46852=CARTESIAN_POINT('Ctrl Pts',(-20.3449819506173,-30.988199101113,124.593690835872)) ;
#46853=CARTESIAN_POINT('Ctrl Pts',(-20.3087153180884,-31.1780527923171,
124.215054802295)) ;
#46854=CARTESIAN_POINT('Ctrl Pts',(-20.5335886314549,-30.9980637119542,
124.415853378407)) ;
#46855=CARTESIAN_POINT('Ctrl Pts',(-20.4346283251563,-31.1880451917782,
124.046895705598)) ;
#46856=CARTESIAN_POINT('Ctrl Pts',(-20.6909778265813,-31.0080561114154,
124.205652827145)) ;
#46857=CARTESIAN_POINT('Ctrl Pts',(-20.5294345452315,-31.1980771451111,
123.858502766262)) ;
#46858=CARTESIAN_POINT('Ctrl Pts',(-20.8094832862645,-31.0180880647483,
123.970160489407)) ;
#46859=CARTESIAN_POINT('Ctrl Pts',(-20.5893954841832,-31.2079435040528,
123.659927548445)) ;
#46860=CARTESIAN_POINT('Ctrl Pts',(-20.8844320812118,-31.0279544236899,
123.721940205726)) ;
#46861=CARTESIAN_POINT('Ctrl Pts',(-20.6146037556417,-31.2179309795386,
123.451503773627)) ;
#46862=CARTESIAN_POINT('Ctrl Pts',(-20.9159397608911,-31.0379418991757,
123.461410041658)) ;
#46863=CARTESIAN_POINT('Ctrl Pts',(-20.6033971471085,-31.2278758857271,
123.24270000188)) ;
#46864=CARTESIAN_POINT('Ctrl Pts',(-20.9019287886433,-31.0478868053642,
123.200405236579)) ;
#46865=CARTESIAN_POINT('Ctrl Pts',(-20.5555242405054,-31.2379208503873,
123.037041915201)) ;
#46866=CARTESIAN_POINT('Ctrl Pts',(-20.8420850390457,-31.0579317700244,
122.943333258433)) ;
#46867=CARTESIAN_POINT('Ctrl Pts',(-20.4743386324737,-31.2477826572922,
122.846253520561)) ;
#46868=CARTESIAN_POINT('Ctrl Pts',(-20.7406003647243,-31.0677935769293,
122.704848430439)) ;
#46869=CARTESIAN_POINT('Ctrl Pts',(-20.360117950421,-31.2577753295979,122.669966551316)) ;
#46870=CARTESIAN_POINT('Ctrl Pts',(-20.597822144092,-31.0777862492351,122.484491140274)) ;
#46871=CARTESIAN_POINT('Ctrl Pts',(-20.2178975470522,-31.2677040005433,
122.51716583229)) ;
#46872=CARTESIAN_POINT('Ctrl Pts',(-20.4200444703197,-31.0877149201804,
122.293491951008)) ;
#46873=CARTESIAN_POINT('Ctrl Pts',(-20.0511349253016,-31.2776565427686,
122.390821276081)) ;
#46874=CARTESIAN_POINT('Ctrl Pts',(-20.2115893827837,-31.0976674624057,
122.135563380117)) ;
#46875=CARTESIAN_POINT('Ctrl Pts',(-19.8640731557152,-31.2876578987645,
122.294767252677)) ;
#46876=CARTESIAN_POINT('Ctrl Pts',(-19.9777608298293,-31.1076688184016,
122.015498299379)) ;
#46877=CARTESIAN_POINT('Ctrl Pts',(-19.6625721454269,-31.2976865110392,
122.232767913839)) ;
#46878=CARTESIAN_POINT('Ctrl Pts',(-19.7258837090503,-31.1176974306763,
121.93800176093)) ;
#46879=CARTESIAN_POINT('Ctrl Pts',(-19.4568083883109,-31.3075508455887,
122.20682000382)) ;
#46880=CARTESIAN_POINT('Ctrl Pts',(-19.468678402315,-31.1275617652258,121.905569609794)) ;
#46881=CARTESIAN_POINT('Ctrl Pts',(-19.2470034323369,-31.3175431696653,
122.216797567056)) ;
#46882=CARTESIAN_POINT('Ctrl Pts',(-19.2064222623212,-31.1375540893024,
121.918044378445)) ;
#46883=CARTESIAN_POINT('Ctrl Pts',(-19.0433631987087,-31.3274706620311,
122.26264289437)) ;
#46884=CARTESIAN_POINT('Ctrl Pts',(-18.9518724580088,-31.1474815816683,
121.975353810798)) ;
#46885=CARTESIAN_POINT('Ctrl Pts',(-18.8488944828603,-31.337498020582,122.343946304587)) ;
#46886=CARTESIAN_POINT('Ctrl Pts',(-18.7087875925179,-31.1575089402191,
122.076985697164)) ;
#46887=CARTESIAN_POINT('Ctrl Pts',(-18.6738227975292,-31.3473844386331,
122.456025056537)) ;
#46888=CARTESIAN_POINT('Ctrl Pts',(-18.4899494031481,-31.1673953582702,
122.217086576)) ;
#46889=CARTESIAN_POINT('Ctrl Pts',(-18.5185992416469,-31.3574161733685,
122.598745584505)) ;
#46890=CARTESIAN_POINT('Ctrl Pts',(-18.2959218218459,-31.1774270930056,
122.395489361766)) ;
#46891=CARTESIAN_POINT('Ctrl Pts',(-18.3922256515261,-31.3672977546117,
122.76367605931)) ;
#46892=CARTESIAN_POINT('Ctrl Pts',(-18.1379570317836,-31.1873086742489,
122.601654224087)) ;
#46893=CARTESIAN_POINT('Ctrl Pts',(-18.2946472022262,-31.3773597326441,
122.951323265286)) ;
#46894=CARTESIAN_POINT('Ctrl Pts',(-18.0159864387997,-31.1973706522812,
122.836214609579)) ;
#46895=CARTESIAN_POINT('Ctrl Pts',(-18.2323356671991,-31.3872168110058,
123.148990652215)) ;
#46896=CARTESIAN_POINT('Ctrl Pts',(-17.9380997062694,-31.2072277306429,
123.083299705092)) ;
#46897=CARTESIAN_POINT('Ctrl Pts',(-18.2045044604485,-31.3972113841118,
123.357222538529)) ;
#46898=CARTESIAN_POINT('Ctrl Pts',(-17.9033134792368,-31.2172223037489,
123.343589981846)) ;
#46899=CARTESIAN_POINT('Ctrl Pts',(-18.2131184967394,-31.4071371803994,
123.565745265259)) ;
#46900=CARTESIAN_POINT('Ctrl Pts',(-17.9140838363557,-31.2271481000365,
123.604243273479)) ;
#46901=CARTESIAN_POINT('Ctrl Pts',(-18.2581923238068,-31.4171625475691,
123.771616644239)) ;
#46902=CARTESIAN_POINT('Ctrl Pts',(-17.9704288396952,-31.2371734672062,
123.861581949243)) ;
#46903=CARTESIAN_POINT('Ctrl Pts',(-18.3372215849961,-31.427058627223,123.964077719536)) ;
#46904=CARTESIAN_POINT('Ctrl Pts',(-18.0692181290173,-31.2470695468601,
124.102157307068)) ;
#46905=CARTESIAN_POINT('Ctrl Pts',(-18.4492191595014,-31.4370537069285,
124.141874347234)) ;
#46906=CARTESIAN_POINT('Ctrl Pts',(-18.2092168773112,-31.2570646265657,
124.324401074987)) ;
#46907=CARTESIAN_POINT('Ctrl Pts',(-18.5910734083571,-31.4470787947444,
124.297744881585)) ;
#46908=CARTESIAN_POINT('Ctrl Pts',(-18.3865390046239,-31.2670897143815,
124.519239586884)) ;
#46909=CARTESIAN_POINT('Ctrl Pts',(-18.8100884239902,-31.4602626171116,
124.467625344121)) ;
#46910=CARTESIAN_POINT('Ctrl Pts',(-18.6602990640863,-31.2802735367488,
124.731576473087)) ;
#46911=CARTESIAN_POINT('Ctrl Pts',(-19.0709153029651,-31.4735847352576,
124.578138378408)) ;
#46912=CARTESIAN_POINT('Ctrl Pts',(-18.9862948594309,-31.2935956548947,
124.869711357312)) ;
#46913=CARTESIAN_POINT('Ctrl Pts',(-19.3495941389619,-31.4869639448852,
124.6162385658)) ;
#46914=CARTESIAN_POINT('Ctrl Pts',(-19.3347015527575,-31.3069748645223,
124.917347223178)) ;
#46915=CARTESIAN_POINT('Ctrl Pts',(-19.5563094575702,-31.4968021821294,
124.608810856145)) ;
#46916=CARTESIAN_POINT('Ctrl Pts',(-19.5930836021212,-31.3168131017665,
124.908057132309)) ;
#46917=CARTESIAN_POINT('Ctrl Pts',(-19.763395166937,-31.5068751053881,124.564668379505)) ;
#46918=CARTESIAN_POINT('Ctrl Pts',(-19.8519437779237,-31.3268860250252,
124.852876717695)) ;
#46919=CARTESIAN_POINT('Ctrl Pts',(-19.9554908372654,-31.5167317468432,
124.486904342967)) ;
#46920=CARTESIAN_POINT('Ctrl Pts',(-20.0920602272961,-31.3367426664803,
124.755670606679)) ;
#46921=CARTESIAN_POINT('Ctrl Pts',(-20.1337307856986,-31.5267171223493,
124.376027908366)) ;
#46922=CARTESIAN_POINT('Ctrl Pts',(-20.3148623984286,-31.3467280419864,
124.617067390045)) ;
#46923=CARTESIAN_POINT('Ctrl Pts',(-20.3414635779869,-31.5400011538097,
124.189405170033)) ;
#46924=CARTESIAN_POINT('Ctrl Pts',(-20.5745088879433,-31.3600120734468,
124.383813942974)) ;
#46925=CARTESIAN_POINT('Ctrl Pts',(-20.5342357011611,-31.55651994568,123.895695798079)) ;
#46926=CARTESIAN_POINT('Ctrl Pts',(-20.8154916492515,-31.3765308653172,
124.016626072661)) ;
#46927=CARTESIAN_POINT('Ctrl Pts',(-20.615702601322,-31.5733056626867,123.5482462708)) ;
#46928=CARTESIAN_POINT('Ctrl Pts',(-20.9173070492714,-31.3933165823238,
123.582394229583)) ;
#46929=CARTESIAN_POINT('Ctrl Pts',(-20.607065235222,-31.5864188111957,123.272686183113)) ;
#46930=CARTESIAN_POINT('Ctrl Pts',(-20.906515294897,-31.4064297308328,123.237879258058)) ;
#46931=CARTESIAN_POINT('Ctrl Pts',(-20.5647775941507,-31.5964543602758,
123.066008473396)) ;
#46932=CARTESIAN_POINT('Ctrl Pts',(-20.8536524123544,-31.416465279913,122.97954630541)) ;
#46933=CARTESIAN_POINT('Ctrl Pts',(-20.4868139035535,-31.6064704164553,
122.870382663184)) ;
#46934=CARTESIAN_POINT('Ctrl Pts',(-20.7561932613821,-31.4264813360924,
122.73500867879)) ;
#46935=CARTESIAN_POINT('Ctrl Pts',(-20.3416392377526,-31.6196484523213,
122.634448176635)) ;
#46936=CARTESIAN_POINT('Ctrl Pts',(-20.5747356330736,-31.4396593719584,
122.440107128178)) ;
#46937=CARTESIAN_POINT('Ctrl Pts',(-20.0859156395753,-31.6362503295084,
122.3910420022)) ;
#46938=CARTESIAN_POINT('Ctrl Pts',(-20.2550642401252,-31.4562612491455,
122.135837120638)) ;
#46939=CARTESIAN_POINT('Ctrl Pts',(-19.6946086357507,-31.6563134741243,
122.221176683087)) ;
#46940=CARTESIAN_POINT('Ctrl Pts',(-19.7659328719897,-31.4763243937614,
121.923514400748)) ;
#46941=CARTESIAN_POINT('Ctrl Pts',(-19.2743459249407,-31.676114364208,122.195122229128)) ;
#46942=CARTESIAN_POINT('Ctrl Pts',(-19.2406043647874,-31.4961252838451,
121.89094955361)) ;
#46943=CARTESIAN_POINT('Ctrl Pts',(-18.8673343999719,-31.6960574894867,
122.313844662609)) ;
#46944=CARTESIAN_POINT('Ctrl Pts',(-18.731841866447,-31.5160684091238,122.039356586224)) ;
#46945=CARTESIAN_POINT('Ctrl Pts',(-18.5261587627728,-31.7159555346063,
122.564031122159)) ;
#46946=CARTESIAN_POINT('Ctrl Pts',(-18.3053752399663,-31.5359664542434,
122.352092202936)) ;
#46947=CARTESIAN_POINT('Ctrl Pts',(-18.2900690142787,-31.735841294233,122.914876518788)) ;
#46948=CARTESIAN_POINT('Ctrl Pts',(-18.0102664114479,-31.5558522138702,
122.790649876929)) ;
#46949=CARTESIAN_POINT('Ctrl Pts',(-18.1876243917938,-31.7559064694129,
123.328998046209)) ;
#46950=CARTESIAN_POINT('Ctrl Pts',(-17.8822137797069,-31.57591738905,123.30830329177)) ;
#46951=CARTESIAN_POINT('Ctrl Pts',(-18.2322702694616,-31.7757331125157,
123.748268184179)) ;
#46952=CARTESIAN_POINT('Ctrl Pts',(-17.9380242803409,-31.5957440321528,
123.832388879101)) ;
#46953=CARTESIAN_POINT('Ctrl Pts',(-18.4169480013837,-31.7956418219641,
124.129048330367)) ;
#46954=CARTESIAN_POINT('Ctrl Pts',(-18.1688732800194,-31.6156527416012,
124.308361931682)) ;
#46955=CARTESIAN_POINT('Ctrl Pts',(-18.7212311690732,-31.8155936589959,
124.424824302643)) ;
#46956=CARTESIAN_POINT('Ctrl Pts',(-18.5492284834963,-31.635604578633,124.678079899656)) ;
#46957=CARTESIAN_POINT('Ctrl Pts',(-19.109410695338,-31.835602133699,124.59881362796)) ;
#46958=CARTESIAN_POINT('Ctrl Pts',(-19.0344540490019,-31.6556130533361,
124.895564294001)) ;
#46959=CARTESIAN_POINT('Ctrl Pts',(-19.5292929940374,-31.8554035924605,
124.630074904832)) ;
#46960=CARTESIAN_POINT('Ctrl Pts',(-19.5593044714881,-31.6754145120976,
124.934638681105)) ;
#46961=CARTESIAN_POINT('Ctrl Pts',(-19.9381051953959,-31.8753604806964,
124.516346944635)) ;
#46962=CARTESIAN_POINT('Ctrl Pts',(-20.0703188207212,-31.6953714003336,
124.792477849082)) ;
#46963=CARTESIAN_POINT('Ctrl Pts',(-20.2834627517452,-31.8953443181105,
124.268832628097)) ;
#46964=CARTESIAN_POINT('Ctrl Pts',(-20.502014723073,-31.7153552377477,124.483083841928)) ;
#46965=CARTESIAN_POINT('Ctrl Pts',(-20.5222631166498,-31.9151527573315,
123.921823635472)) ;
#46966=CARTESIAN_POINT('Ctrl Pts',(-20.8005129693209,-31.7351636769686,
124.049324638335)) ;
#46967=CARTESIAN_POINT('Ctrl Pts',(-20.6296391609579,-31.9351384667117,
123.510794184968)) ;
#46968=CARTESIAN_POINT('Ctrl Pts',(-20.9347328465596,-31.7551493863488,
123.535538119656)) ;
#46969=CARTESIAN_POINT('Ctrl Pts',(-20.5906472244068,-31.955007989727,123.089943615466)) ;
#46970=CARTESIAN_POINT('Ctrl Pts',(-20.8859933951321,-31.7750189093641,
123.009476827453)) ;
#46971=CARTESIAN_POINT('Ctrl Pts',(-20.4089954990554,-31.9750287288442,
122.705129085206)) ;
#46972=CARTESIAN_POINT('Ctrl Pts',(-20.6589290212962,-31.7950396484813,
122.528458277174)) ;
#46973=CARTESIAN_POINT('Ctrl Pts',(-20.1103555337929,-31.9948327938211,
122.408035535206)) ;
#46974=CARTESIAN_POINT('Ctrl Pts',(-20.2856318116993,-31.8148437134583,
122.157092625036)) ;
#46975=CARTESIAN_POINT('Ctrl Pts',(-19.7236013982933,-32.0148947575519,
122.228362978264)) ;
#46976=CARTESIAN_POINT('Ctrl Pts',(-19.8021889396994,-31.834905677189,121.932500294498)) ;
#46977=CARTESIAN_POINT('Ctrl Pts',(-19.3033421555285,-32.0347279378404,
122.192269701717)) ;
#46978=CARTESIAN_POINT('Ctrl Pts',(-19.2768672597706,-31.8547388574775,
121.88738259078)) ;
#46979=CARTESIAN_POINT('Ctrl Pts',(-18.8940840487304,-32.0546471351664,
122.301037263848)) ;
#46980=CARTESIAN_POINT('Ctrl Pts',(-18.7652950498868,-31.8746580548036,
122.02333953517)) ;
#46981=CARTESIAN_POINT('Ctrl Pts',(-18.5462767706842,-32.0745851602798,
122.543427443625)) ;
#46982=CARTESIAN_POINT('Ctrl Pts',(-18.3305352276764,-31.8945960799169,
122.32632493169)) ;
#46983=CARTESIAN_POINT('Ctrl Pts',(-18.3022836708014,-32.0944632063358,
122.888601365163)) ;
#46984=CARTESIAN_POINT('Ctrl Pts',(-18.0255423060835,-31.914474125973,122.757789608184)) ;
#46985=CARTESIAN_POINT('Ctrl Pts',(-18.1901182041216,-32.1144479406239,
123.298403225457)) ;
#46986=CARTESIAN_POINT('Ctrl Pts',(-17.8853325731395,-31.934458860261,123.270040998411)) ;
#46987=CARTESIAN_POINT('Ctrl Pts',(-18.2243400099676,-32.1343587573024,
123.720498462101)) ;
#46988=CARTESIAN_POINT('Ctrl Pts',(-17.928106557493,-31.9543696769395,123.797659471924)) ;
#46989=CARTESIAN_POINT('Ctrl Pts',(-18.4014838664741,-32.1543577328211,
124.106965037813)) ;
#46990=CARTESIAN_POINT('Ctrl Pts',(-18.1495333782431,-31.9743686524582,
124.280744001209)) ;
#46991=CARTESIAN_POINT('Ctrl Pts',(-18.6967305235978,-32.1741626534663,
124.40735164037)) ;
#46992=CARTESIAN_POINT('Ctrl Pts',(-18.5185878611027,-31.9941735731034,
124.656228575391)) ;
#46993=CARTESIAN_POINT('Ctrl Pts',(-19.0797563575211,-32.1941466137575,
124.59108153163)) ;
#46994=CARTESIAN_POINT('Ctrl Pts',(-18.9973682960231,-32.0141575333947,
124.885894562646)) ;
#46995=CARTESIAN_POINT('Ctrl Pts',(-19.500620909332,-32.2140328174815,124.632705731497)) ;
#46996=CARTESIAN_POINT('Ctrl Pts',(-19.5234477413584,-32.0340437371186,
124.937928873616)) ;
#46997=CARTESIAN_POINT('Ctrl Pts',(-19.91172625123,-32.2339819958047,124.528376651481)) ;
#46998=CARTESIAN_POINT('Ctrl Pts',(-20.0373301585634,-32.0539929154418,
124.807521706156)) ;
#46999=CARTESIAN_POINT('Ctrl Pts',(-20.2616847114276,-32.2538837950442,
124.290492641391)) ;
#47000=CARTESIAN_POINT('Ctrl Pts',(-20.4747803851015,-32.0738947146813,
124.510171457429)) ;
#47001=CARTESIAN_POINT('Ctrl Pts',(-20.5099132977842,-32.2737624000966,
123.948363389314)) ;
#47002=CARTESIAN_POINT('Ctrl Pts',(-20.7850691732621,-32.0937733197337,
124.082510674293)) ;
#47003=CARTESIAN_POINT('Ctrl Pts',(-20.627203071623,-32.2937947598223,123.538857802633)) ;
#47004=CARTESIAN_POINT('Ctrl Pts',(-20.9316880819048,-32.1138056794594,
123.570639458984)) ;
#47005=CARTESIAN_POINT('Ctrl Pts',(-20.6022414190364,-32.3103764857783,
123.187181314506)) ;
#47006=CARTESIAN_POINT('Ctrl Pts',(-20.9004840928426,-32.1303874054155,
123.13101387148)) ;
#47007=CARTESIAN_POINT('Ctrl Pts',(-20.5124528604533,-32.3235706560763,
122.924720422985)) ;
#47008=CARTESIAN_POINT('Ctrl Pts',(-20.7882628387208,-32.1435815757134,
122.802971043195)) ;
#47009=CARTESIAN_POINT('Ctrl Pts',(-20.3776944343899,-32.3368828341695,
122.679500006612)) ;
#47010=CARTESIAN_POINT('Ctrl Pts',(-20.6197762199004,-32.1568937538066,
122.496386987847)) ;
#47011=CARTESIAN_POINT('Ctrl Pts',(-20.1339928139378,-32.3534490137628,
122.425047262597)) ;
#47012=CARTESIAN_POINT('Ctrl Pts',(-20.3152084467147,-32.1734599333999,
122.178383590941)) ;
#47013=CARTESIAN_POINT('Ctrl Pts',(-19.8172190621121,-32.370077208623,122.268225534679)) ;
#47014=CARTESIAN_POINT('Ctrl Pts',(-19.9191951145893,-32.1900881282601,
121.982318684066)) ;
#47015=CARTESIAN_POINT('Ctrl Pts',(-19.5432299461013,-32.3833657903327,
122.213296215293)) ;
#47016=CARTESIAN_POINT('Ctrl Pts',(-19.5767420543761,-32.2033767099699,
121.913670003331)) ;
#47017=CARTESIAN_POINT('Ctrl Pts',(-19.3337508719107,-32.3933340384363,
122.208232309393)) ;
#47018=CARTESIAN_POINT('Ctrl Pts',(-19.3148866166845,-32.2133449580735,
121.907334290486)) ;
#47019=CARTESIAN_POINT('Ctrl Pts',(-19.1276189549108,-32.4032487946925,
122.239193486121)) ;
#47020=CARTESIAN_POINT('Ctrl Pts',(-19.0572238635977,-32.2232597143296,
121.946033185605)) ;
#47021=CARTESIAN_POINT('Ctrl Pts',(-18.9279557063151,-32.4132619453437,
122.305913698926)) ;
#47022=CARTESIAN_POINT('Ctrl Pts',(-18.8076409322538,-32.2332728649808,
122.029433371392)) ;
#47023=CARTESIAN_POINT('Ctrl Pts',(-18.7430842089401,-32.4232746525457,
122.406578399065)) ;
#47024=CARTESIAN_POINT('Ctrl Pts',(-18.5765593857256,-32.2432855721828,
122.155251712162)) ;
#47025=CARTESIAN_POINT('Ctrl Pts',(-18.5254677572598,-32.436493941237,122.579410532713)) ;
#47026=CARTESIAN_POINT('Ctrl Pts',(-18.3044914721772,-32.2565048608741,
122.371339808174)) ;
#47027=CARTESIAN_POINT('Ctrl Pts',(-18.3148360496128,-32.453112622235,122.863088731423)) ;
#47028=CARTESIAN_POINT('Ctrl Pts',(-18.0412520385267,-32.2731235418722,
122.725865756024)) ;
#47029=CARTESIAN_POINT('Ctrl Pts',(-18.2135427727924,-32.4696775300085,
123.200444286709)) ;
#47030=CARTESIAN_POINT('Ctrl Pts',(-17.9146049570504,-32.2896884496456,
123.147620680735)) ;
#47031=CARTESIAN_POINT('Ctrl Pts',(-18.2053428109417,-32.4830760016193,
123.482028619465)) ;
#47032=CARTESIAN_POINT('Ctrl Pts',(-17.904363104532,-32.3030869212564,123.499558748901)) ;
#47033=CARTESIAN_POINT('Ctrl Pts',(-18.2351263930126,-32.4929172571063,
123.686778633759)) ;
#47034=CARTESIAN_POINT('Ctrl Pts',(-17.9415874189062,-32.3129281767434,
123.755505137551)) ;
#47035=CARTESIAN_POINT('Ctrl Pts',(-18.3005104295691,-32.5029035726945,
123.886247272274)) ;
#47036=CARTESIAN_POINT('Ctrl Pts',(-18.0233154440135,-32.3229144923316,
124.004839610842)) ;
#47037=CARTESIAN_POINT('Ctrl Pts',(-18.3989864711992,-32.5128401802809,
124.070517770327)) ;
#47038=CARTESIAN_POINT('Ctrl Pts',(-18.1464078763225,-32.332851099918,124.2351797327)) ;
#47039=CARTESIAN_POINT('Ctrl Pts',(-18.5294794836623,-32.5228900476492,
124.236655331214)) ;
#47040=CARTESIAN_POINT('Ctrl Pts',(-18.3095220075479,-32.3429009672863,
124.44285330986)) ;
#47041=CARTESIAN_POINT('Ctrl Pts',(-18.6836393496476,-32.532740542324,124.374955006091)) ;
#47042=CARTESIAN_POINT('Ctrl Pts',(-18.5022200305885,-32.3527514619611,
124.615730119443)) ;
#47043=CARTESIAN_POINT('Ctrl Pts',(-18.8613101056891,-32.5427123427185,
124.486175930194)) ;
#47044=CARTESIAN_POINT('Ctrl Pts',(-18.7243070867326,-32.3627232623556,
124.754758703636)) ;
#47045=CARTESIAN_POINT('Ctrl Pts',(-19.0561314475104,-32.5527083097443,
124.565050529732)) ;
#47046=CARTESIAN_POINT('Ctrl Pts',(-18.9678327868554,-32.3727192293814,
124.853354582418)) ;
#47047=CARTESIAN_POINT('Ctrl Pts',(-19.2625472172633,-32.5627457691255,
124.608788649609)) ;
#47048=CARTESIAN_POINT('Ctrl Pts',(-19.225851948996,-32.3827566887626,124.90802999486)) ;
#47049=CARTESIAN_POINT('Ctrl Pts',(-19.4693094256783,-32.5725864700262,
124.616272691469)) ;
#47050=CARTESIAN_POINT('Ctrl Pts',(-19.4843048557896,-32.3925973896634,
124.917387851395)) ;
#47051=CARTESIAN_POINT('Ctrl Pts',(-19.6785662287874,-32.5826344912936,
124.587453910695)) ;
#47052=CARTESIAN_POINT('Ctrl Pts',(-19.7458762676805,-32.4026454109307,
124.881367125265)) ;
#47053=CARTESIAN_POINT('Ctrl Pts',(-19.8775350367199,-32.5925818843763,
124.523064897387)) ;
#47054=CARTESIAN_POINT('Ctrl Pts',(-19.9945882738061,-32.4125928040134,
124.800883482138)) ;
#47055=CARTESIAN_POINT('Ctrl Pts',(-20.0619149648412,-32.6024920304227,
124.426032573854)) ;
#47056=CARTESIAN_POINT('Ctrl Pts',(-20.2250646863654,-32.4225029500598,
124.679595400653)) ;
#47057=CARTESIAN_POINT('Ctrl Pts',(-20.2289464125442,-32.6125509442723,
124.296375819046)) ;
#47058=CARTESIAN_POINT('Ctrl Pts',(-20.4338556734805,-32.4325618639094,
124.517526668951)) ;
#47059=CARTESIAN_POINT('Ctrl Pts',(-20.3680971425257,-32.6223917145616,
124.143243416164)) ;
#47060=CARTESIAN_POINT('Ctrl Pts',(-20.6077963923764,-32.4424026341987,
124.326112710777)) ;
#47061=CARTESIAN_POINT('Ctrl Pts',(-20.4812183694655,-32.6324545841402,
123.964505832737)) ;
#47062=CARTESIAN_POINT('Ctrl Pts',(-20.749200205045,-32.4524655037773,124.102692225348)) ;
#47063=CARTESIAN_POINT('Ctrl Pts',(-20.5601018658738,-32.6423489072707,
123.772009901321)) ;
#47064=CARTESIAN_POINT('Ctrl Pts',(-20.8478072363101,-32.4623598269078,
123.862073047581)) ;
#47065=CARTESIAN_POINT('Ctrl Pts',(-20.6051186285884,-32.6522907143652,
123.567933795961)) ;
#47066=CARTESIAN_POINT('Ctrl Pts',(-20.9040808602051,-32.4723016340023,
123.606978235594)) ;
#47067=CARTESIAN_POINT('Ctrl Pts',(-20.6141529517269,-32.6622932253205,
123.357815073032)) ;
#47068=CARTESIAN_POINT('Ctrl Pts',(-20.9153764258059,-32.4823041449576,
123.34432986247)) ;
#47069=CARTESIAN_POINT('Ctrl Pts',(-20.5861553370163,-32.6723279461389,
123.148732523265)) ;
#47070=CARTESIAN_POINT('Ctrl Pts',(-20.8803820948059,-32.492338865776,123.082976331004)) ;
#47071=CARTESIAN_POINT('Ctrl Pts',(-20.5238045844199,-32.6821731236446,
122.95135818224)) ;
#47072=CARTESIAN_POINT('Ctrl Pts',(-20.8024460213099,-32.5021840432817,
122.836257068615)) ;
#47073=CARTESIAN_POINT('Ctrl Pts',(-20.4271596502256,-32.6921578840457,
122.76505202383)) ;
#47074=CARTESIAN_POINT('Ctrl Pts',(-20.6816420858177,-32.5121688036828,
122.603373026614)) ;
#47075=CARTESIAN_POINT('Ctrl Pts',(-20.3002621335287,-32.7020967903621,
122.599012732577)) ;
#47076=CARTESIAN_POINT('Ctrl Pts',(-20.523022050828,-32.5221077099992,122.395822102444)) ;
#47077=CARTESIAN_POINT('Ctrl Pts',(-20.1448530384785,-32.7121390179978,
122.456148065448)) ;
#47078=CARTESIAN_POINT('Ctrl Pts',(-20.3287624729339,-32.5321499376349,
122.217239391601)) ;
#47079=CARTESIAN_POINT('Ctrl Pts',(-19.9698227420243,-32.7220242295822,
122.344065587158)) ;
#47080=CARTESIAN_POINT('Ctrl Pts',(-20.1099755420916,-32.5420351492193,
122.077133850417)) ;
#47081=CARTESIAN_POINT('Ctrl Pts',(-19.7759374579204,-32.7320231597841,
122.262927443023)) ;
#47082=CARTESIAN_POINT('Ctrl Pts',(-19.8676198087422,-32.5520340794212,
121.975708802829)) ;
#47083=CARTESIAN_POINT('Ctrl Pts',(-19.5725517032629,-32.7419405826945,
122.216894103156)) ;
#47084=CARTESIAN_POINT('Ctrl Pts',(-19.6133877400118,-32.5619515023317,
121.918164610241)) ;
#47085=CARTESIAN_POINT('Ctrl Pts',(-19.3615855045364,-32.7519885147733,
122.206786949472)) ;
#47086=CARTESIAN_POINT('Ctrl Pts',(-19.3496802081964,-32.5719994344104,
121.905528177764)) ;
#47087=CARTESIAN_POINT('Ctrl Pts',(-19.1555344402761,-32.7618658905827,
122.232817208028)) ;
#47088=CARTESIAN_POINT('Ctrl Pts',(-19.0921154350541,-32.5818768102198,
121.938063647421)) ;
#47089=CARTESIAN_POINT('Ctrl Pts',(-18.9536242961126,-32.7719197837506,
122.29520263043)) ;
#47090=CARTESIAN_POINT('Ctrl Pts',(-18.8397271603765,-32.5919307033877,
122.016043063102)) ;
#47091=CARTESIAN_POINT('Ctrl Pts',(-18.7684970290784,-32.7818134070039,
122.390109939971)) ;
#47092=CARTESIAN_POINT('Ctrl Pts',(-18.6083164557563,-32.601824326641,122.134675324029)) ;
#47093=CARTESIAN_POINT('Ctrl Pts',(-18.5998696574853,-32.7918760006269,
122.517792698711)) ;
#47094=CARTESIAN_POINT('Ctrl Pts',(-18.3975309341739,-32.611886920264,122.29427674415)) ;
#47095=CARTESIAN_POINT('Ctrl Pts',(-18.4590017312758,-32.8017185746159,
122.669394023076)) ;
#47096=CARTESIAN_POINT('Ctrl Pts',(-18.221443696393,-32.6217294942531,122.483777412127)) ;
#47097=CARTESIAN_POINT('Ctrl Pts',(-18.3445119360111,-32.8117093314989,
122.845452008546)) ;
#47098=CARTESIAN_POINT('Ctrl Pts',(-18.0783294582589,-32.631720251136,122.703848805901)) ;
#47099=CARTESIAN_POINT('Ctrl Pts',(-18.2628657738663,-32.8216373932568,
123.037550195113)) ;
#47100=CARTESIAN_POINT('Ctrl Pts',(-17.9762694762357,-32.6416483128939,
122.943971098664)) ;
#47101=CARTESIAN_POINT('Ctrl Pts',(-18.2151746216112,-32.831625369146,123.242049850644)) ;
#47102=CARTESIAN_POINT('Ctrl Pts',(-17.9166533727178,-32.6516362887831,
123.19959535074)) ;
#47103=CARTESIAN_POINT('Ctrl Pts',(-18.2040142138472,-32.8416610335024,
123.452729593888)) ;
#47104=CARTESIAN_POINT('Ctrl Pts',(-17.9027006002209,-32.6616719531395,
123.462944824449)) ;
#47105=CARTESIAN_POINT('Ctrl Pts',(-18.2288249971323,-32.8515169719221,
123.658452238389)) ;
#47106=CARTESIAN_POINT('Ctrl Pts',(-17.9337120201421,-32.6715278915592,
123.720099296854)) ;
#47107=CARTESIAN_POINT('Ctrl Pts',(-18.2894914318515,-32.861512463319,123.859618101424)) ;
#47108=CARTESIAN_POINT('Ctrl Pts',(-18.0095431011939,-32.6815233829561,
123.971557376319)) ;
#47109=CARTESIAN_POINT('Ctrl Pts',(-18.3833118947942,-32.8714222682724,
124.045643520541)) ;
#47110=CARTESIAN_POINT('Ctrl Pts',(-18.1268171255641,-32.6914331879096,
124.20409067232)) ;
#47111=CARTESIAN_POINT('Ctrl Pts',(-18.509018904418,-32.8814344905392,124.214478322823)) ;
#47112=CARTESIAN_POINT('Ctrl Pts',(-18.2839493311189,-32.7014454101763,
124.41513539528)) ;
#47113=CARTESIAN_POINT('Ctrl Pts',(-18.6626514296269,-32.891462371232,124.358845529882)) ;
#47114=CARTESIAN_POINT('Ctrl Pts',(-18.4759885042275,-32.7114732908691,
124.595595889866)) ;
#47115=CARTESIAN_POINT('Ctrl Pts',(-18.8358044204708,-32.9013187672146,
124.472662632877)) ;
#47116=CARTESIAN_POINT('Ctrl Pts',(-18.6924294796709,-32.7213296868517,
124.737869480862)) ;
#47117=CARTESIAN_POINT('Ctrl Pts',(-19.0291703242302,-32.9113435643946,
124.556493615886)) ;
#47118=CARTESIAN_POINT('Ctrl Pts',(-18.9341360919731,-32.7313544840317,
124.842659911602)) ;
#47119=CARTESIAN_POINT('Ctrl Pts',(-19.2344039020975,-32.9213744943784,
124.605003116564)) ;
#47120=CARTESIAN_POINT('Ctrl Pts',(-19.1906775296738,-32.7413854140155,
124.903298738838)) ;
#47121=CARTESIAN_POINT('Ctrl Pts',(-19.4409936637498,-32.931219096887,124.617286306071)) ;
#47122=CARTESIAN_POINT('Ctrl Pts',(-19.4489157332629,-32.7512300165242,
124.918654695543)) ;
#47123=CARTESIAN_POINT('Ctrl Pts',(-19.6497118954831,-32.9412099481111,
124.593725011282)) ;
#47124=CARTESIAN_POINT('Ctrl Pts',(-19.7098139114528,-32.7612208677483,
124.889204775659)) ;
#47125=CARTESIAN_POINT('Ctrl Pts',(-19.8519756476524,-32.9512477811224,
124.533550068226)) ;
#47126=CARTESIAN_POINT('Ctrl Pts',(-19.962644010255,-32.7712587007595,124.813987935703)) ;
#47127=CARTESIAN_POINT('Ctrl Pts',(-20.0372510161014,-32.9610921695878,
124.441308298038)) ;
#47128=CARTESIAN_POINT('Ctrl Pts',(-20.1942400544308,-32.7811030892249,
124.698686780465)) ;
#47129=CARTESIAN_POINT('Ctrl Pts',(-20.206287933549,-32.9710769739574,124.316898276306)) ;
#47130=CARTESIAN_POINT('Ctrl Pts',(-20.4055373690367,-32.7910878935945,
124.543175419173)) ;
#47131=CARTESIAN_POINT('Ctrl Pts',(-20.3506030576117,-32.9810164934402,
124.165738129342)) ;
#47132=CARTESIAN_POINT('Ctrl Pts',(-20.5859328054878,-32.8010274130773,
124.354225945988)) ;
#47133=CARTESIAN_POINT('Ctrl Pts',(-20.4675814605525,-32.9910562244416,
123.990072866531)) ;
#47134=CARTESIAN_POINT('Ctrl Pts',(-20.7321570744506,-32.8110671440787,
124.134645385839)) ;
#47135=CARTESIAN_POINT('Ctrl Pts',(-20.5511100440207,-33.0009443526879,
123.799699797302)) ;
#47136=CARTESIAN_POINT('Ctrl Pts',(-20.8365696228075,-32.820955272325,123.896678841576)) ;
#47137=CARTESIAN_POINT('Ctrl Pts',(-20.6011952592599,-33.0109340778964,
123.595752254043)) ;
#47138=CARTESIAN_POINT('Ctrl Pts',(-20.8991776003898,-32.8309449975335,
123.641744550588)) ;
#47139=CARTESIAN_POINT('Ctrl Pts',(-20.6149126949009,-33.0208918425979,
123.386861704438)) ;
#47140=CARTESIAN_POINT('Ctrl Pts',(-20.9163259243604,-32.840902762235,123.380631029218)) ;
#47141=CARTESIAN_POINT('Ctrl Pts',(-20.5927628252155,-33.0307941840099,
123.179858179155)) ;
#47142=CARTESIAN_POINT('Ctrl Pts',(-20.8886398161754,-32.850805103647,123.121875613575)) ;
#47143=CARTESIAN_POINT('Ctrl Pts',(-20.5341646522333,-33.0408383797163,
122.977001703688)) ;
#47144=CARTESIAN_POINT('Ctrl Pts',(-20.8153934381563,-32.8608492993534,
122.868304834852)) ;
#47145=CARTESIAN_POINT('Ctrl Pts',(-20.4425109806158,-33.0507457804755,
122.789954482795)) ;
#47146=CARTESIAN_POINT('Ctrl Pts',(-20.7008271858602,-32.8707567001127,
122.634494488512)) ;
#47147=CARTESIAN_POINT('Ctrl Pts',(-20.3187974646894,-33.0607563803499,
122.619697924543)) ;
#47148=CARTESIAN_POINT('Ctrl Pts',(-20.5461862319884,-32.880767299987,122.421673048565)) ;
#47149=CARTESIAN_POINT('Ctrl Pts',(-20.1668178861132,-33.0707866762621,
122.473511957559)) ;
#47150=CARTESIAN_POINT('Ctrl Pts',(-20.356212767659,-32.8907975958992,122.238939688487)) ;
#47151=CARTESIAN_POINT('Ctrl Pts',(-19.9950035419231,-33.0806414559118,
122.357764747843)) ;
#47152=CARTESIAN_POINT('Ctrl Pts',(-20.1414444851523,-32.9006523755489,
122.094253937587)) ;
#47153=CARTESIAN_POINT('Ctrl Pts',(-19.8039737443084,-33.0905987841293,
122.272141541311)) ;
#47154=CARTESIAN_POINT('Ctrl Pts',(-19.9026572208542,-32.9106097037664,
121.987223818498)) ;
#47155=CARTESIAN_POINT('Ctrl Pts',(-19.5992424579009,-33.1006378170362,
122.220935616222)) ;
#47156=CARTESIAN_POINT('Ctrl Pts',(-19.6467435512146,-32.9206487366733,
121.923215339529)) ;
#47157=CARTESIAN_POINT('Ctrl Pts',(-19.3921897280463,-33.1105109289255,
122.205912912299)) ;
#47158=CARTESIAN_POINT('Ctrl Pts',(-19.3879265897767,-32.9305218485626,
121.90443588022)) ;
#47159=CARTESIAN_POINT('Ctrl Pts',(-19.1815696557166,-33.1205842139526,
122.227554268862)) ;
#47160=CARTESIAN_POINT('Ctrl Pts',(-19.1246518188088,-32.9405951335897,
121.93148651026)) ;
#47161=CARTESIAN_POINT('Ctrl Pts',(-18.9828627675349,-33.1304045336893,
122.283747306268)) ;
#47162=CARTESIAN_POINT('Ctrl Pts',(-18.8762664627294,-32.9504154533265,
122.001727342518)) ;
#47163=CARTESIAN_POINT('Ctrl Pts',(-18.7920430269983,-33.1404831990678,
122.37573379343)) ;
#47164=CARTESIAN_POINT('Ctrl Pts',(-18.6377418415184,-32.9604941187049,
122.116709479966)) ;
#47165=CARTESIAN_POINT('Ctrl Pts',(-18.6238449944928,-33.1503347895516,
122.496666905546)) ;
#47166=CARTESIAN_POINT('Ctrl Pts',(-18.4274927507125,-32.9703457091887,
122.267875972372)) ;
#47167=CARTESIAN_POINT('Ctrl Pts',(-18.4758763515475,-33.1604079398705,
122.648110975471)) ;
#47168=CARTESIAN_POINT('Ctrl Pts',(-18.2425317134073,-32.9804188595076,
122.457180219424)) ;
#47169=CARTESIAN_POINT('Ctrl Pts',(-18.3591783280429,-33.1702503198455,
122.8190052862)) ;
#47170=CARTESIAN_POINT('Ctrl Pts',(-18.0966577530102,-32.9902612394826,
122.670798846665)) ;
#47171=CARTESIAN_POINT('Ctrl Pts',(-18.2721117533038,-33.1802312960886,
123.009903540524)) ;
#47172=CARTESIAN_POINT('Ctrl Pts',(-17.987823954365,-33.0002422157257,122.90942173405)) ;
#47173=CARTESIAN_POINT('Ctrl Pts',(-18.2196648188066,-33.1902476244439,
123.213853808958)) ;
#47174=CARTESIAN_POINT('Ctrl Pts',(-17.9222646672302,-33.010258544081,123.164359426917)) ;
#47175=CARTESIAN_POINT('Ctrl Pts',(-18.2033572918697,-33.200145421435,123.421288579882)) ;
#47176=CARTESIAN_POINT('Ctrl Pts',(-17.9018796513175,-33.0201563410721,
123.423653833823)) ;
#47177=CARTESIAN_POINT('Ctrl Pts',(-18.223190034098,-33.2101579781671,123.630863236516)) ;
#47178=CARTESIAN_POINT('Ctrl Pts',(-17.9266701886612,-33.0301688978042,
123.685622214838)) ;
#47179=CARTESIAN_POINT('Ctrl Pts',(-18.2796939241535,-33.2201900130135,
123.834047999503)) ;
#47180=CARTESIAN_POINT('Ctrl Pts',(-17.9972994489001,-33.0402009326507,
123.939603199681)) ;
#47181=CARTESIAN_POINT('Ctrl Pts',(-18.3684191094839,-33.230029413829,124.020926505679)) ;
#47182=CARTESIAN_POINT('Ctrl Pts',(-18.1082062116321,-33.0500403334661,
124.173202825564)) ;
#47183=CARTESIAN_POINT('Ctrl Pts',(-18.4908474188606,-33.2400951994806,
124.193500366468)) ;
#47184=CARTESIAN_POINT('Ctrl Pts',(-18.2612411137015,-33.0601061191177,
124.388920029464)) ;
#47185=CARTESIAN_POINT('Ctrl Pts',(-18.6388594412923,-33.2499856545952,
124.339567692069)) ;
#47186=CARTESIAN_POINT('Ctrl Pts',(-18.4462566311347,-33.0699965742323,
124.571505176903)) ;
#47187=CARTESIAN_POINT('Ctrl Pts',(-18.8114608537052,-33.2599777732309,
124.459283778179)) ;
#47188=CARTESIAN_POINT('Ctrl Pts',(-18.6620084681289,-33.0799886928681,
124.721150558715)) ;
#47189=CARTESIAN_POINT('Ctrl Pts',(-19.0017546265229,-33.269940599994,124.546778303222)) ;
#47190=CARTESIAN_POINT('Ctrl Pts',(-18.8998759883332,-33.0899515196311,
124.830519144683)) ;
#47191=CARTESIAN_POINT('Ctrl Pts',(-19.2030467259017,-33.2798448832669,
124.600106280176)) ;
#47192=CARTESIAN_POINT('Ctrl Pts',(-19.1514920073142,-33.099855802904,124.897179406725)) ;
#47193=CARTESIAN_POINT('Ctrl Pts',(-19.4137849185456,-33.289905317214,124.617764888055)) ;
#47194=CARTESIAN_POINT('Ctrl Pts',(-19.4149143853563,-33.1099162368511,
124.919252762117)) ;
#47195=CARTESIAN_POINT('Ctrl Pts',(-19.6198604520968,-33.2997458698872,
124.599243558957)) ;
#47196=CARTESIAN_POINT('Ctrl Pts',(-19.6725102686655,-33.1197567895243,
124.896100987741)) ;
#47197=CARTESIAN_POINT('Ctrl Pts',(-19.8241111476887,-33.3098080898329,
124.544278855776)) ;
#47198=CARTESIAN_POINT('Ctrl Pts',(-19.9278232585217,-33.12981900947,124.827395120368)) ;
#47199=CARTESIAN_POINT('Ctrl Pts',(-20.0125096552998,-33.3197052291114,
124.455943774085)) ;
#47200=CARTESIAN_POINT('Ctrl Pts',(-20.1633223010035,-33.1397161487486,
124.716975844118)) ;
#47201=CARTESIAN_POINT('Ctrl Pts',(-20.1836814999991,-33.3296364212465,
124.336404331942)) ;
#47202=CARTESIAN_POINT('Ctrl Pts',(-20.377287539303,-33.1496473408836,124.567550900585)) ;
#47203=CARTESIAN_POINT('Ctrl Pts',(-20.3329814659399,-33.3396785758916,
124.187146312258)) ;
#47204=CARTESIAN_POINT('Ctrl Pts',(-20.5639122193513,-33.1596894955287,
124.380978396875)) ;
#47205=CARTESIAN_POINT('Ctrl Pts',(-20.4523759830474,-33.3495653369109,
124.016987842125)) ;
#47206=CARTESIAN_POINT('Ctrl Pts',(-20.7131557897439,-33.169576256548,124.168279265478)) ;
#47207=CARTESIAN_POINT('Ctrl Pts',(-20.5416382969896,-33.3595646386281,
123.826694295305)) ;
#47208=CARTESIAN_POINT('Ctrl Pts',(-20.8247334245669,-33.1795755582652,
123.930412036511)) ;
#47209=CARTESIAN_POINT('Ctrl Pts',(-20.596223942968,-33.3694854367949,123.625368027277)) ;
#47210=CARTESIAN_POINT('Ctrl Pts',(-20.8929652906654,-33.189496356432,123.678753341723)) ;
#47211=CARTESIAN_POINT('Ctrl Pts',(-20.615255722677,-33.3795194903916,123.415304326235)) ;
#47212=CARTESIAN_POINT('Ctrl Pts',(-20.9167545830113,-33.1995304100287,
123.416173818305)) ;
#47213=CARTESIAN_POINT('Ctrl Pts',(-20.5978416091603,-33.389442607958,123.207385396435)) ;
#47214=CARTESIAN_POINT('Ctrl Pts',(-20.894986412613,-33.2094535275951,123.156274431571)) ;
#47215=CARTESIAN_POINT('Ctrl Pts',(-20.5438456870571,-33.3994987314571,
123.003007585044)) ;
#47216=CARTESIAN_POINT('Ctrl Pts',(-20.8274911534907,-33.2195096510942,
122.900802570426)) ;
#47217=CARTESIAN_POINT('Ctrl Pts',(-20.4571105200585,-33.4093441731119,
122.81506612472)) ;
#47218=CARTESIAN_POINT('Ctrl Pts',(-20.7190711618733,-33.2293550927491,
122.665874666496)) ;
#47219=CARTESIAN_POINT('Ctrl Pts',(-20.3382374891591,-33.4193064742361,
122.642647202006)) ;
#47220=CARTESIAN_POINT('Ctrl Pts',(-20.5704789953411,-33.2393173938732,
122.450351068691)) ;
#47221=CARTESIAN_POINT('Ctrl Pts',(-20.1900385777374,-33.4293349535112,
122.492672258745)) ;
#47222=CARTESIAN_POINT('Ctrl Pts',(-20.3852299651721,-33.2493458731483,
122.262882911342)) ;
#47223=CARTESIAN_POINT('Ctrl Pts',(-20.0201373732377,-33.4392453070209,
122.372100343306)) ;
#47224=CARTESIAN_POINT('Ctrl Pts',(-20.172852355375,-33.259256226658,122.112168058019)) ;
#47225=CARTESIAN_POINT('Ctrl Pts',(-19.8316354394708,-33.4491801791981,
122.282138877027)) ;
#47226=CARTESIAN_POINT('Ctrl Pts',(-19.9372239609423,-33.2691910988352,
121.999716737927)) ;
#47227=CARTESIAN_POINT('Ctrl Pts',(-19.628183907834,-33.4592213167838,122.225869096708)) ;
#47228=CARTESIAN_POINT('Ctrl Pts',(-19.6829095119979,-33.2792322364209,
121.92938034057)) ;
#47229=CARTESIAN_POINT('Ctrl Pts',(-19.4212710659109,-33.4691084659983,
122.205941031249)) ;
#47230=CARTESIAN_POINT('Ctrl Pts',(-19.4242673412634,-33.2891193856355,
121.904471017884)) ;
#47231=CARTESIAN_POINT('Ctrl Pts',(-19.2118367929156,-33.4791007007494,
122.222063506245)) ;
#47232=CARTESIAN_POINT('Ctrl Pts',(-19.1624743734912,-33.2991116203865,
121.924625120071)) ;
#47233=CARTESIAN_POINT('Ctrl Pts',(-19.0092605385172,-33.4890494063124,
122.274143933396)) ;
#47234=CARTESIAN_POINT('Ctrl Pts',(-18.9092537722081,-33.3090603259495,
121.989726729914)) ;
#47235=CARTESIAN_POINT('Ctrl Pts',(-18.8189440039273,-33.4989854747361,
122.360209294255)) ;
#47236=CARTESIAN_POINT('Ctrl Pts',(-18.6713579683458,-33.3189963943732,
122.097309682469)) ;
#47237=CARTESIAN_POINT('Ctrl Pts',(-18.6454357357952,-33.5089711589519,
122.478422695815)) ;
#47238=CARTESIAN_POINT('Ctrl Pts',(-18.454473086345,-33.328982078589,122.245077547478)) ;
#47239=CARTESIAN_POINT('Ctrl Pts',(-18.4945213063124,-33.5190115855205,
122.625987981149)) ;
#47240=CARTESIAN_POINT('Ctrl Pts',(-18.2658309062383,-33.3390225051576,
122.429534786724)) ;
#47241=CARTESIAN_POINT('Ctrl Pts',(-18.3736983247787,-33.5288506989843,
122.793886133219)) ;
#47242=CARTESIAN_POINT('Ctrl Pts',(-18.1148023371037,-33.3488616186214,
122.639409270607)) ;
#47243=CARTESIAN_POINT('Ctrl Pts',(-18.28169524401,-33.5388804331601,122.983614959474)) ;
#47244=CARTESIAN_POINT('Ctrl Pts',(-17.9997997485683,-33.3588913527972,
122.876570796198)) ;
#47245=CARTESIAN_POINT('Ctrl Pts',(-18.2246058172832,-33.548902532666,123.186427396069)) ;
#47246=CARTESIAN_POINT('Ctrl Pts',(-17.9284390777351,-33.3689134523031,
123.130086625313)) ;
#47247=CARTESIAN_POINT('Ctrl Pts',(-18.2034007562052,-33.5587709725594,
123.392821859869)) ;
#47248=CARTESIAN_POINT('Ctrl Pts',(-17.9019339658882,-33.3787818921965,
123.388080969439)) ;
#47249=CARTESIAN_POINT('Ctrl Pts',(-18.218661353348,-33.568839837245,123.603931402573)) ;
#47250=CARTESIAN_POINT('Ctrl Pts',(-17.9210110195692,-33.3888507568821,
123.651967424913)) ;
#47251=CARTESIAN_POINT('Ctrl Pts',(-18.2691838785988,-33.5786825103436,
123.804599750498)) ;
#47252=CARTESIAN_POINT('Ctrl Pts',(-17.9841657910811,-33.3986934299808,
123.902803793652)) ;
#47253=CARTESIAN_POINT('Ctrl Pts',(-18.3540908209291,-33.5886431445061,
123.996012857149)) ;
#47254=CARTESIAN_POINT('Ctrl Pts',(-18.0903011027806,-33.4086540641432,
124.142069897794)) ;
#47255=CARTESIAN_POINT('Ctrl Pts',(-18.472193287036,-33.5986810601842,124.170889366581)) ;
#47256=CARTESIAN_POINT('Ctrl Pts',(-18.237930321801,-33.4186919798213,124.360664605472)) ;
#47257=CARTESIAN_POINT('Ctrl Pts',(-18.6162214398664,-33.6085553350436,
124.320419679324)) ;
#47258=CARTESIAN_POINT('Ctrl Pts',(-18.4179673638906,-33.4285662546808,
124.547577121921)) ;
#47259=CARTESIAN_POINT('Ctrl Pts',(-18.787310591261,-33.6186250854188,124.445049310116)) ;
#47260=CARTESIAN_POINT('Ctrl Pts',(-18.6318294560732,-33.4386360050559,
124.703362669157)) ;
#47261=CARTESIAN_POINT('Ctrl Pts',(-18.9729667813463,-33.6284583807933,
124.536013927551)) ;
#47262=CARTESIAN_POINT('Ctrl Pts',(-18.8639015606415,-33.4484693004304,
124.817067545813)) ;
#47263=CARTESIAN_POINT('Ctrl Pts',(-19.1753880863516,-33.6384886782729,
124.595078783209)) ;
#47264=CARTESIAN_POINT('Ctrl Pts',(-19.116928618104,-33.45849959791,124.890896842844)) ;
#47265=CARTESIAN_POINT('Ctrl Pts',(-19.385109828368,-33.6485207647143,124.61748724909)) ;
#47266=CARTESIAN_POINT('Ctrl Pts',(-19.3790808832761,-33.4685316843515,
124.918905806779)) ;
#47267=CARTESIAN_POINT('Ctrl Pts',(-19.5912662914409,-33.6583486932033,
124.603887833734)) ;
#47268=CARTESIAN_POINT('Ctrl Pts',(-19.6367776217658,-33.4783596128404,
124.901904690569)) ;
#47269=CARTESIAN_POINT('Ctrl Pts',(-19.7955034306806,-33.668344734314,124.554404004129)) ;
#47270=CARTESIAN_POINT('Ctrl Pts',(-19.8920737335198,-33.4883556539512,
124.840047977085)) ;
#47271=CARTESIAN_POINT('Ctrl Pts',(-19.9884633521273,-33.6783705464153,
124.469582265232)) ;
#47272=CARTESIAN_POINT('Ctrl Pts',(-20.133272867296,-33.4983814660524,124.734019156174)) ;
#47273=CARTESIAN_POINT('Ctrl Pts',(-20.1614882739156,-33.6882577813101,
124.354388322665)) ;
#47274=CARTESIAN_POINT('Ctrl Pts',(-20.3495536621585,-33.5082687009472,
124.590024685913)) ;
#47275=CARTESIAN_POINT('Ctrl Pts',(-20.3134732484457,-33.6982346475211,
124.209865201567)) ;
#47276=CARTESIAN_POINT('Ctrl Pts',(-20.5395336848334,-33.5182455671582,
124.409369154937)) ;
#47277=CARTESIAN_POINT('Ctrl Pts',(-20.4383121739259,-33.7082275913929,
124.040861571576)) ;
#47278=CARTESIAN_POINT('Ctrl Pts',(-20.6955808166486,-33.52823851103,124.198113299847)) ;
#47279=CARTESIAN_POINT('Ctrl Pts',(-20.5320713712117,-33.7182655140643,
123.851823217952)) ;
#47280=CARTESIAN_POINT('Ctrl Pts',(-20.8127780411408,-33.5382764337014,
123.961814580438)) ;
#47281=CARTESIAN_POINT('Ctrl Pts',(-20.5907682106731,-33.728113978326,123.653255911294)) ;
#47282=CARTESIAN_POINT('Ctrl Pts',(-20.8861474399005,-33.5481248979631,
123.713603887042)) ;
#47283=CARTESIAN_POINT('Ctrl Pts',(-20.6148023086895,-33.73810584507,123.444605714219)) ;
#47284=CARTESIAN_POINT('Ctrl Pts',(-20.9161879631416,-33.5581167647071,
123.452790730188)) ;
#47285=CARTESIAN_POINT('Ctrl Pts',(-20.6024505201895,-33.7480235771112,
123.236442898067)) ;
#47286=CARTESIAN_POINT('Ctrl Pts',(-20.9007460375611,-33.5680344967483,
123.192586764787)) ;
#47287=CARTESIAN_POINT('Ctrl Pts',(-20.5536692961249,-33.7580517620064,
123.031357793843)) ;
#47288=CARTESIAN_POINT('Ctrl Pts',(-20.8397673980302,-33.5780626816436,
122.936230922789)) ;
#47289=CARTESIAN_POINT('Ctrl Pts',(-20.4712833025613,-33.7679369200553,
122.840563071159)) ;
#47290=CARTESIAN_POINT('Ctrl Pts',(-20.7367825952507,-33.5879478396924,
122.697737712798)) ;
#47291=CARTESIAN_POINT('Ctrl Pts',(-20.3562437198245,-33.777926280597,122.664861804041)) ;
#47292=CARTESIAN_POINT('Ctrl Pts',(-20.5929810834346,-33.5979372002341,
122.478112272451)) ;
#47293=CARTESIAN_POINT('Ctrl Pts',(-20.2113763674384,-33.7879674375313,
122.511319512586)) ;
#47294=CARTESIAN_POINT('Ctrl Pts',(-20.4118953447041,-33.6079783571685,
122.28618599598)) ;
#47295=CARTESIAN_POINT('Ctrl Pts',(-20.0457742353741,-33.7978000209865,
122.38760905629)) ;
#47296=CARTESIAN_POINT('Ctrl Pts',(-20.2048905331621,-33.6178109406236,
122.131549195167)) ;
#47297=CARTESIAN_POINT('Ctrl Pts',(-19.8584418259696,-33.8077942409485,
122.29246902554)) ;
#47298=CARTESIAN_POINT('Ctrl Pts',(-19.9707238077735,-33.6278051605856,
122.012626278824)) ;
#47299=CARTESIAN_POINT('Ctrl Pts',(-19.6566211003262,-33.8178223427358,
122.23150371137)) ;
#47300=CARTESIAN_POINT('Ctrl Pts',(-19.718447243707,-33.6378332623729,121.936421881646)) ;
#47301=CARTESIAN_POINT('Ctrl Pts',(-19.4504107987317,-33.8277022873588,
122.206582828826)) ;
#47302=CARTESIAN_POINT('Ctrl Pts',(-19.4606834132683,-33.647713206996,121.905273090565)) ;
#47303=CARTESIAN_POINT('Ctrl Pts',(-19.2406868639278,-33.8376926139159,
122.21764677824)) ;
#47304=CARTESIAN_POINT('Ctrl Pts',(-19.1985284829144,-33.657703533553,121.919105510909)) ;
#47305=CARTESIAN_POINT('Ctrl Pts',(-19.0370644043963,-33.8476335455702,
122.264726339862)) ;
#47306=CARTESIAN_POINT('Ctrl Pts',(-18.9440006247662,-33.6676444652073,
121.977957452937)) ;
#47307=CARTESIAN_POINT('Ctrl Pts',(-18.8436891463967,-33.8576206640731,
122.346553932478)) ;
#47308=CARTESIAN_POINT('Ctrl Pts',(-18.7022824096691,-33.6776315837102,
122.080244334494)) ;
#47309=CARTESIAN_POINT('Ctrl Pts',(-18.6668496652182,-33.8676539969703,
122.461506020677)) ;
#47310=CARTESIAN_POINT('Ctrl Pts',(-18.481234424871,-33.6876649166074,122.223936502288)) ;
#47311=CARTESIAN_POINT('Ctrl Pts',(-18.5149208707951,-33.877520101415,122.602747192623)) ;
#47312=CARTESIAN_POINT('Ctrl Pts',(-18.2913247035046,-33.6975310210521,
122.400490262853)) ;
#47313=CARTESIAN_POINT('Ctrl Pts',(-18.3872775083727,-33.8875862152953,
122.77150901783)) ;
#47314=CARTESIAN_POINT('Ctrl Pts',(-18.1317726324715,-33.7075971349325,
122.611443969021)) ;
#47315=CARTESIAN_POINT('Ctrl Pts',(-18.2928599718456,-33.8974422270637,
122.955967537504)) ;
#47316=CARTESIAN_POINT('Ctrl Pts',(-18.0137527035476,-33.7174531467009,
122.84201884311)) ;
#47317=CARTESIAN_POINT('Ctrl Pts',(-18.2304603251342,-33.9074369306951,
123.156602452202)) ;
#47318=CARTESIAN_POINT('Ctrl Pts',(-17.9357556600526,-33.7274478503322,
123.0928133731)) ;
#47319=CARTESIAN_POINT('Ctrl Pts',(-18.2041945369859,-33.9174682664199,
123.365854471469)) ;
#47320=CARTESIAN_POINT('Ctrl Pts',(-17.9029259941155,-33.7374791860571,
123.354378720209)) ;
#47321=CARTESIAN_POINT('Ctrl Pts',(-18.2141592542206,-33.9273347916236,
123.573047505969)) ;
#47322=CARTESIAN_POINT('Ctrl Pts',(-17.9153845549704,-33.7473457112607,
123.613370405302)) ;
#47323=CARTESIAN_POINT('Ctrl Pts',(-18.2601719129641,-33.9373222196694,
123.777885455416)) ;
#47324=CARTESIAN_POINT('Ctrl Pts',(-17.9729030336068,-33.7573331393065,
123.869417371802)) ;
#47325=CARTESIAN_POINT('Ctrl Pts',(-18.3406253597855,-33.9472671493558,
123.970893068674)) ;
#47326=CARTESIAN_POINT('Ctrl Pts',(-18.0734724275908,-33.767278068993,124.110676065872)) ;
#47327=CARTESIAN_POINT('Ctrl Pts',(-18.4545761365393,-33.9573120674643,
124.148662539094)) ;
#47328=CARTESIAN_POINT('Ctrl Pts',(-18.2159131529908,-33.7773229871015,
124.332886434286)) ;
#47329=CARTESIAN_POINT('Ctrl Pts',(-18.5949446142755,-33.9671740370782,
124.301270643735)) ;
#47330=CARTESIAN_POINT('Ctrl Pts',(-18.3913760380472,-33.7871849567154,
124.523645046325)) ;
#47331=CARTESIAN_POINT('Ctrl Pts',(-18.7615730312214,-33.9771661050995,
124.42915104515)) ;
#47332=CARTESIAN_POINT('Ctrl Pts',(-18.5996633149286,-33.7971770247366,
124.683493416082)) ;
#47333=CARTESIAN_POINT('Ctrl Pts',(-18.946781772386,-33.987097030474,124.525545967815)) ;
#47334=CARTESIAN_POINT('Ctrl Pts',(-18.8311757134717,-33.8071079501112,
124.803984732102)) ;
#47335=CARTESIAN_POINT('Ctrl Pts',(-19.1461772309718,-33.9970476586975,
124.588768735179)) ;
#47336=CARTESIAN_POINT('Ctrl Pts',(-19.0804210325099,-33.8170585783346,
124.883010582507)) ;
#47337=CARTESIAN_POINT('Ctrl Pts',(-19.3545768509614,-34.0070478977566,
124.616672563708)) ;
#47338=CARTESIAN_POINT('Ctrl Pts',(-19.3409209971923,-33.8270588173937,
124.917887617961)) ;
#47339=CARTESIAN_POINT('Ctrl Pts',(-19.5652047456883,-34.0170763531258,
124.607640135001)) ;
#47340=CARTESIAN_POINT('Ctrl Pts',(-19.6042058083092,-33.8370872727629,
124.906594290871)) ;
#47341=CARTESIAN_POINT('Ctrl Pts',(-19.7678153879952,-34.026942387709,124.563211304919)) ;
#47342=CARTESIAN_POINT('Ctrl Pts',(-19.8574687091397,-33.8469533073462,
124.851055548244)) ;
#47343=CARTESIAN_POINT('Ctrl Pts',(-19.9621929863248,-34.0369347094565,
124.483598324612)) ;
#47344=CARTESIAN_POINT('Ctrl Pts',(-20.1004399415462,-33.8569456290936,
124.751536396934)) ;
#47345=CARTESIAN_POINT('Ctrl Pts',(-20.1387770996676,-34.0468669991335,
124.372126827251)) ;
#47346=CARTESIAN_POINT('Ctrl Pts',(-20.3211678423663,-33.8668779187706,
124.612195664073)) ;
#47347=CARTESIAN_POINT('Ctrl Pts',(-20.2945220917022,-34.0568686441042,
124.230877087231)) ;
#47348=CARTESIAN_POINT('Ctrl Pts',(-20.5158504184365,-33.8768795637414,
124.435627299884)) ;
#47349=CARTESIAN_POINT('Ctrl Pts',(-20.4659642035819,-34.0701812775203,
124.009619570015)) ;
#47350=CARTESIAN_POINT('Ctrl Pts',(-20.730134344151,-33.8901921971574,124.159073181011)) ;
#47351=CARTESIAN_POINT('Ctrl Pts',(-20.575254365758,-34.0834130269018,123.750361749611)) ;
#47352=CARTESIAN_POINT('Ctrl Pts',(-20.8667466130496,-33.903423946539,123.835025634149)) ;
#47353=CARTESIAN_POINT('Ctrl Pts',(-20.6136526413231,-34.0967362917189,
123.472950552117)) ;
#47354=CARTESIAN_POINT('Ctrl Pts',(-20.9147529608524,-33.916747211356,123.488209575824)) ;
#47355=CARTESIAN_POINT('Ctrl Pts',(-20.6062950710004,-34.1066119979366,
123.265445897535)) ;
#47356=CARTESIAN_POINT('Ctrl Pts',(-20.9055507233818,-33.9266229175737,
123.228839180932)) ;
#47357=CARTESIAN_POINT('Ctrl Pts',(-20.5627942065194,-34.1166015890366,
123.060012974967)) ;
#47358=CARTESIAN_POINT('Ctrl Pts',(-20.8511725357474,-33.9366125086737,
122.972045792766)) ;
#47359=CARTESIAN_POINT('Ctrl Pts',(-20.4848858375353,-34.126528685492,122.866373888595)) ;
#47360=CARTESIAN_POINT('Ctrl Pts',(-20.7537843023225,-33.9465396051291,
122.72999873487)) ;
#47361=CARTESIAN_POINT('Ctrl Pts',(-20.3734933893588,-34.1365538339966,
122.687478257524)) ;
#47362=CARTESIAN_POINT('Ctrl Pts',(-20.6145413556846,-33.9565647536337,
122.506380398598)) ;
#47363=CARTESIAN_POINT('Ctrl Pts',(-20.2346205228606,-34.1464494881433,
122.532553580072)) ;
#47364=CARTESIAN_POINT('Ctrl Pts',(-20.4409482369391,-33.9664604077804,
122.312726536766)) ;
#47365=CARTESIAN_POINT('Ctrl Pts',(-20.0693873756585,-34.1564530225215,
122.402484078199)) ;
#47366=CARTESIAN_POINT('Ctrl Pts',(-20.234405044289,-33.9764639421586,122.150141791109)) ;
#47367=CARTESIAN_POINT('Ctrl Pts',(-19.8843645713023,-34.1664381609615,
122.303256991677)) ;
#47368=CARTESIAN_POINT('Ctrl Pts',(-20.0031251936759,-33.9864490805987,
122.026110363717)) ;
#47369=CARTESIAN_POINT('Ctrl Pts',(-19.6838837822579,-34.1764740855569,
122.237544345005)) ;
#47370=CARTESIAN_POINT('Ctrl Pts',(-19.7525232072214,-33.996485005194,121.943972168262)) ;
#47371=CARTESIAN_POINT('Ctrl Pts',(-19.4789063239412,-34.1863253609846,
122.207945323593)) ;
#47372=CARTESIAN_POINT('Ctrl Pts',(-19.4963012262117,-34.0063362806217,
121.906976170342)) ;
#47373=CARTESIAN_POINT('Ctrl Pts',(-19.2689143031909,-34.1963176221459,
122.213879430628)) ;
#47374=CARTESIAN_POINT('Ctrl Pts',(-19.2338112579742,-34.0163285417831,
121.914396519971)) ;
#47375=CARTESIAN_POINT('Ctrl Pts',(-19.0622877357805,-34.2063575061635,
122.256906073786)) ;
#47376=CARTESIAN_POINT('Ctrl Pts',(-18.9755284714672,-34.0263684258007,
121.968182550343)) ;
#47377=CARTESIAN_POINT('Ctrl Pts',(-18.8700474354873,-34.216192280666,122.33308360955)) ;
#47378=CARTESIAN_POINT('Ctrl Pts',(-18.7352293588995,-34.0362032003031,
122.063406918151)) ;
#47379=CARTESIAN_POINT('Ctrl Pts',(-18.6896382083871,-34.2262686616863,
122.444048971715)) ;
#47380=CARTESIAN_POINT('Ctrl Pts',(-18.5097194264488,-34.0462795813234,
122.202115742426)) ;
#47381=CARTESIAN_POINT('Ctrl Pts',(-18.5347718576947,-34.2361149348369,
122.581438980249)) ;
#47382=CARTESIAN_POINT('Ctrl Pts',(-18.3161370097982,-34.056125854474,122.37385617066)) ;
#47383=CARTESIAN_POINT('Ctrl Pts',(-18.3597451156534,-34.2494794561221,
122.801234068625)) ;
#47384=CARTESIAN_POINT('Ctrl Pts',(-18.0973641720853,-34.0694903757593,
122.648596301571)) ;
#47385=CARTESIAN_POINT('Ctrl Pts',(-18.2477846712695,-34.2626857005566,
123.058779918869)) ;
#47386=CARTESIAN_POINT('Ctrl Pts',(-17.9574233667404,-34.0826966201937,
122.97048578706)) ;
#47387=CARTESIAN_POINT('Ctrl Pts',(-18.205709003732,-34.2759506552338,123.334400391849)) ;
#47388=CARTESIAN_POINT('Ctrl Pts',(-17.9048166903989,-34.0959615748709,
123.315069758424)) ;
#47389=CARTESIAN_POINT('Ctrl Pts',(-18.2106566690873,-34.2859829357855,
123.545267006591)) ;
#47390=CARTESIAN_POINT('Ctrl Pts',(-17.9110068532374,-34.1059938554226,
123.57864144408)) ;
#47391=CARTESIAN_POINT('Ctrl Pts',(-18.2516149367393,-34.2958916693034,
123.749507046798)) ;
#47392=CARTESIAN_POINT('Ctrl Pts',(-17.9622064695877,-34.1159025889405,
123.833943902984)) ;
#47393=CARTESIAN_POINT('Ctrl Pts',(-18.3271317964583,-34.3058292201709,
123.944308961896)) ;
#47394=CARTESIAN_POINT('Ctrl Pts',(-18.0566040745096,-34.125840139808,124.077443630493)) ;
#47395=CARTESIAN_POINT('Ctrl Pts',(-18.4364641233543,-34.3158590677648,
124.124581975054)) ;
#47396=CARTESIAN_POINT('Ctrl Pts',(-18.1932746081133,-34.1358699874019,
124.302786499422)) ;
#47397=CARTESIAN_POINT('Ctrl Pts',(-18.6196354097619,-34.3290942076852,
124.334139196948)) ;
#47398=CARTESIAN_POINT('Ctrl Pts',(-18.4222258929034,-34.1491051273224,
124.564718290271)) ;
#47399=CARTESIAN_POINT('Ctrl Pts',(-18.9138855860305,-34.3457626720564,
124.531468794228)) ;
#47400=CARTESIAN_POINT('Ctrl Pts',(-18.7900532730984,-34.1657735916935,
124.811391878838)) ;
#47401=CARTESIAN_POINT('Ctrl Pts',(-19.3240781905893,-34.3656336839303,
124.633306467972)) ;
#47402=CARTESIAN_POINT('Ctrl Pts',(-19.3028100031656,-34.1856446035674,
124.938674734945)) ;
#47403=CARTESIAN_POINT('Ctrl Pts',(-19.6773043637108,-34.3823407683133,
124.596000454904)) ;
#47404=CARTESIAN_POINT('Ctrl Pts',(-19.7442781237528,-34.2023516879504,
124.8920557054)) ;
#47405=CARTESIAN_POINT('Ctrl Pts',(-19.9358882444672,-34.3955180496239,
124.496604146033)) ;
#47406=CARTESIAN_POINT('Ctrl Pts',(-20.0675644892654,-34.215528969261,124.767792583565)) ;
#47407=CARTESIAN_POINT('Ctrl Pts',(-20.1754272741693,-34.408785510138,124.353698894968)) ;
#47408=CARTESIAN_POINT('Ctrl Pts',(-20.3669683527793,-34.2287964297751,
124.589169379259)) ;
#47409=CARTESIAN_POINT('Ctrl Pts',(-20.4216795722527,-34.4253994008252,
124.10043464984)) ;
#47410=CARTESIAN_POINT('Ctrl Pts',(-20.6747925423891,-34.2454103204623,
124.272577564532)) ;
#47411=CARTESIAN_POINT('Ctrl Pts',(-20.5958914665089,-34.4453482002526,
123.713647161789)) ;
#47412=CARTESIAN_POINT('Ctrl Pts',(-20.8925501699724,-34.2653591198897,
123.789095141607)) ;
#47413=CARTESIAN_POINT('Ctrl Pts',(-20.6275282466341,-34.4652693117834,
123.291312891227)) ;
#47414=CARTESIAN_POINT('Ctrl Pts',(-20.9320934628038,-34.2852802314206,
123.26117694893)) ;
#47415=CARTESIAN_POINT('Ctrl Pts',(-20.5142733747202,-34.4851357599563,
122.884295294386)) ;
#47416=CARTESIAN_POINT('Ctrl Pts',(-20.7905220573564,-34.3051466795934,
122.752407298956)) ;
#47417=CARTESIAN_POINT('Ctrl Pts',(-20.2668055992271,-34.5051621065734,
122.537830920578)) ;
#47418=CARTESIAN_POINT('Ctrl Pts',(-20.4811847888518,-34.3251730262106,
122.319328242786)) ;
#47419=CARTESIAN_POINT('Ctrl Pts',(-19.9186956223332,-34.525024150963,122.298589670166)) ;
#47420=CARTESIAN_POINT('Ctrl Pts',(-20.0460469289995,-34.3450350706001,
122.020279911706)) ;
#47421=CARTESIAN_POINT('Ctrl Pts',(-19.5084246289227,-34.5449694536441,
122.191442824304)) ;
#47422=CARTESIAN_POINT('Ctrl Pts',(-19.5332082975654,-34.3649803732812,
121.886348768634)) ;
#47423=CARTESIAN_POINT('Ctrl Pts',(-19.0872125174688,-34.564864760703,122.230706330331)) ;
#47424=CARTESIAN_POINT('Ctrl Pts',(-19.0066946739163,-34.3848756803401,
121.93543015809)) ;
#47425=CARTESIAN_POINT('Ctrl Pts',(-18.7043989473763,-34.5847580308706,
122.410642685401)) ;
#47426=CARTESIAN_POINT('Ctrl Pts',(-18.528179666335,-34.4047689505077,122.160351280735)) ;
#47427=CARTESIAN_POINT('Ctrl Pts',(-18.4049696018283,-34.604723623551,122.711540803692)) ;
#47428=CARTESIAN_POINT('Ctrl Pts',(-18.1538942485171,-34.4247345431882,
122.53647446393)) ;
#47429=CARTESIAN_POINT('Ctrl Pts',(-18.2267125295678,-34.6245989472359,
123.094736417654)) ;
#47430=CARTESIAN_POINT('Ctrl Pts',(-17.9310744457826,-34.444609866873,123.015467619857)) ;
#47431=CARTESIAN_POINT('Ctrl Pts',(-18.1893069394518,-34.6445740098108,
123.517829036567)) ;
#47432=CARTESIAN_POINT('Ctrl Pts',(-17.8843177630335,-34.464584929448,123.544333074597)) ;
#47433=CARTESIAN_POINT('Ctrl Pts',(-18.299019392422,-34.6645264194419,123.927638801905)) ;
#47434=CARTESIAN_POINT('Ctrl Pts',(-18.0214586110986,-34.4845373390791,
124.056594429955)) ;
#47435=CARTESIAN_POINT('Ctrl Pts',(-18.5399052285237,-34.684362473678,124.273849716243)) ;
#47436=CARTESIAN_POINT('Ctrl Pts',(-18.3225640751946,-34.5043733933152,
124.489356119812)) ;
#47437=CARTESIAN_POINT('Ctrl Pts',(-18.8866675177332,-34.7043403850956,
124.51920099619)) ;
#47438=CARTESIAN_POINT('Ctrl Pts',(-18.7560161142767,-34.5243513047327,
124.796045846229)) ;
#47439=CARTESIAN_POINT('Ctrl Pts',(-19.2952182234732,-34.7242584345991,
124.630665769838)) ;
#47440=CARTESIAN_POINT('Ctrl Pts',(-19.2667030759239,-34.5442693542362,
124.935377333597)) ;
#47441=CARTESIAN_POINT('Ctrl Pts',(-19.7164297540769,-34.7441265783672,
124.597207733981)) ;
#47442=CARTESIAN_POINT('Ctrl Pts',(-19.7932159078448,-34.5641374980043,
124.893556756045)) ;
#47443=CARTESIAN_POINT('Ctrl Pts',(-20.1040277686893,-34.7641774349545,
124.419895888455)) ;
#47444=CARTESIAN_POINT('Ctrl Pts',(-20.2777146690572,-34.5841883545916,
124.671918199537)) ;
#47445=CARTESIAN_POINT('Ctrl Pts',(-20.404229106633,-34.7839578714104,124.125155942307)) ;
#47446=CARTESIAN_POINT('Ctrl Pts',(-20.6529658815064,-34.6039687910475,
124.303496686845)) ;
#47447=CARTESIAN_POINT('Ctrl Pts',(-20.5886433658768,-34.8039879270882,
123.741366661607)) ;
#47448=CARTESIAN_POINT('Ctrl Pts',(-20.8834863290637,-34.6239988467253,
123.823760909331)) ;
#47449=CARTESIAN_POINT('Ctrl Pts',(-20.630003600706,-34.823869032263,123.320595871531)) ;
#47450=CARTESIAN_POINT('Ctrl Pts',(-20.9351889705778,-34.6438799519001,
123.297798988631)) ;
#47451=CARTESIAN_POINT('Ctrl Pts',(-20.5264818869687,-34.8437494946307,
122.91079906104)) ;
#47452=CARTESIAN_POINT('Ctrl Pts',(-20.805790334357,-34.6637604142679,122.785553366895)) ;
#47453=CARTESIAN_POINT('Ctrl Pts',(-20.2879555038815,-34.8637346417751,
122.55910414027)) ;
#47454=CARTESIAN_POINT('Ctrl Pts',(-20.5076352220214,-34.6837455614122,
122.345932910046)) ;
#47455=CARTESIAN_POINT('Ctrl Pts',(-19.9453039790159,-34.8836252203115,
122.311181550038)) ;
#47456=CARTESIAN_POINT('Ctrl Pts',(-20.0793236955457,-34.7036361399486,
122.036027427117)) ;
#47457=CARTESIAN_POINT('Ctrl Pts',(-19.5387683050646,-34.9035192401859,
122.194334979435)) ;
#47458=CARTESIAN_POINT('Ctrl Pts',(-19.5711560383436,-34.723530159823,121.889965636303)) ;
#47459=CARTESIAN_POINT('Ctrl Pts',(-19.1162346707492,-34.9234406849123,
122.223156044862)) ;
#47460=CARTESIAN_POINT('Ctrl Pts',(-19.0429893283783,-34.7434516045494,
121.925987779891)) ;
#47461=CARTESIAN_POINT('Ctrl Pts',(-18.7288788831415,-34.9433388229677,
122.393621819122)) ;
#47462=CARTESIAN_POINT('Ctrl Pts',(-18.5587933443279,-34.7633497426048,
122.139065599401)) ;
#47463=CARTESIAN_POINT('Ctrl Pts',(-18.4209986101695,-34.9634095781838,
122.68903279055)) ;
#47464=CARTESIAN_POINT('Ctrl Pts',(-18.1739396124289,-34.7834204978209,
122.508326536902)) ;
#47465=CARTESIAN_POINT('Ctrl Pts',(-18.2348330469421,-34.983195128235,123.066398593346)) ;
#47466=CARTESIAN_POINT('Ctrl Pts',(-17.9412291317738,-34.8032060478722,
122.980030562384)) ;
#47467=CARTESIAN_POINT('Ctrl Pts',(-18.1871490528402,-35.0031782031124,
123.488530219856)) ;
#47468=CARTESIAN_POINT('Ctrl Pts',(-17.8816194222905,-34.8231891227495,
123.507694573191)) ;
#47469=CARTESIAN_POINT('Ctrl Pts',(-18.2866725644005,-35.0230872857583,
123.899991070555)) ;
#47470=CARTESIAN_POINT('Ctrl Pts',(-18.0060182323476,-34.8430982053954,
124.022021160858)) ;
#47471=CARTESIAN_POINT('Ctrl Pts',(-18.5190486689243,-35.0429458448811,
124.252608438494)) ;
#47472=CARTESIAN_POINT('Ctrl Pts',(-18.2964865246401,-34.8629567645182,
124.462795926968)) ;
#47473=CARTESIAN_POINT('Ctrl Pts',(-18.8611531383577,-35.0629892887198,
124.506625814478)) ;
#47474=CARTESIAN_POINT('Ctrl Pts',(-18.7241036774144,-34.8830002083569,
124.780319588221)) ;
#47475=CARTESIAN_POINT('Ctrl Pts',(-19.1973105599933,-35.079489353449,124.60730897235)) ;
#47476=CARTESIAN_POINT('Ctrl Pts',(-19.1443314362236,-34.8995002730861,
124.906184977463)) ;
#47477=CARTESIAN_POINT('Ctrl Pts',(-19.4786570547526,-35.0928790932979,
124.615810466112)) ;
#47478=CARTESIAN_POINT('Ctrl Pts',(-19.4959856145689,-34.912890012935,124.916808895163)) ;
#47479=CARTESIAN_POINT('Ctrl Pts',(-19.6837596141147,-35.1027359945063,
124.58607447705)) ;
#47480=CARTESIAN_POINT('Ctrl Pts',(-19.7523697501484,-34.9227469141434,
124.879642738554)) ;
#47481=CARTESIAN_POINT('Ctrl Pts',(-19.8833526181919,-35.1127275203528,
124.520719105362)) ;
#47482=CARTESIAN_POINT('Ctrl Pts',(-20.0018598351797,-34.9327384399899,
124.79795143579)) ;
#47483=CARTESIAN_POINT('Ctrl Pts',(-20.0674176518561,-35.1226522008037,
124.422401605199)) ;
#47484=CARTESIAN_POINT('Ctrl Pts',(-20.2319445660988,-34.9426631204409,
124.675054574799)) ;
#47485=CARTESIAN_POINT('Ctrl Pts',(-20.2330436349176,-35.1326627908481,
124.292596619006)) ;
#47486=CARTESIAN_POINT('Ctrl Pts',(-20.438971803788,-34.9526737104853,124.512809926613)) ;
#47487=CARTESIAN_POINT('Ctrl Pts',(-20.4195165261857,-35.1459220515518,
124.085363429725)) ;
#47488=CARTESIAN_POINT('Ctrl Pts',(-20.6720998991134,-34.9659329711889,
124.253723717875)) ;
#47489=CARTESIAN_POINT('Ctrl Pts',(-20.5482036535186,-35.1592731267021,
123.832398852526)) ;
#47490=CARTESIAN_POINT('Ctrl Pts',(-20.8329350805989,-34.9792840463392,
123.937545082256)) ;
#47491=CARTESIAN_POINT('Ctrl Pts',(-20.6059607274363,-35.1724794359369,
123.560762637728)) ;
#47492=CARTESIAN_POINT('Ctrl Pts',(-20.9051329385635,-34.992490355574,123.598017654249)) ;
#47493=CARTESIAN_POINT('Ctrl Pts',(-20.6137261119894,-35.1824662695272,
123.350990307265)) ;
#47494=CARTESIAN_POINT('Ctrl Pts',(-20.914842890768,-35.0024771891643,123.335798885094)) ;
#47495=CARTESIAN_POINT('Ctrl Pts',(-20.5851416406984,-35.1924189970233,
123.143676946331)) ;
#47496=CARTESIAN_POINT('Ctrl Pts',(-20.8791149640092,-35.0124299166604,
123.076657694403)) ;
#47497=CARTESIAN_POINT('Ctrl Pts',(-20.5202297895318,-35.2024670938648,
122.942679277039)) ;
#47498=CARTESIAN_POINT('Ctrl Pts',(-20.7979778136165,-35.022478013502,122.825409407708)) ;
#47499=CARTESIAN_POINT('Ctrl Pts',(-20.4236321858874,-35.2123085507367,
122.75969231486)) ;
#47500=CARTESIAN_POINT('Ctrl Pts',(-20.6772333062096,-35.0323194703738,
122.596674503416)) ;
#47501=CARTESIAN_POINT('Ctrl Pts',(-20.2952501726806,-35.2222948176502,
122.593621170823)) ;
#47502=CARTESIAN_POINT('Ctrl Pts',(-20.5167579761239,-35.0423057372873,
122.389083764502)) ;
#47503=CARTESIAN_POINT('Ctrl Pts',(-20.1407744583381,-35.2322314185506,
122.45294261696)) ;
#47504=CARTESIAN_POINT('Ctrl Pts',(-20.3236651757576,-35.0522423381877,
122.213233449278)) ;
#47505=CARTESIAN_POINT('Ctrl Pts',(-19.9621957115618,-35.2422813613376,
122.340068651411)) ;
#47506=CARTESIAN_POINT('Ctrl Pts',(-20.1004431975683,-35.0622922809748,
122.072138574706)) ;
#47507=CARTESIAN_POINT('Ctrl Pts',(-19.77064229135,-35.2521315610234,122.261352205955)) ;
#47508=CARTESIAN_POINT('Ctrl Pts',(-19.861002389051,-35.0721424806605,121.973740369883)) ;
#47509=CARTESIAN_POINT('Ctrl Pts',(-19.5659662743928,-35.2621044659555,
122.216007869496)) ;
#47510=CARTESIAN_POINT('Ctrl Pts',(-19.6051578614204,-35.0821153855926,
121.917057183094)) ;
#47511=CARTESIAN_POINT('Ctrl Pts',(-19.3559388586588,-35.2721028404351,
122.20693299255)) ;
#47512=CARTESIAN_POINT('Ctrl Pts',(-19.3426236375317,-35.0921137600722,
121.905710783946)) ;
#47513=CARTESIAN_POINT('Ctrl Pts',(-19.1471235458461,-35.2821230143051,
122.234669898377)) ;
#47514=CARTESIAN_POINT('Ctrl Pts',(-19.0816040718578,-35.1021339339422,
121.940379135869)) ;
#47515=CARTESIAN_POINT('Ctrl Pts',(-18.9486182041443,-35.2920240582471,
122.297318677213)) ;
#47516=CARTESIAN_POINT('Ctrl Pts',(-18.8334713868321,-35.1120349778842,
122.018687487834)) ;
#47517=CARTESIAN_POINT('Ctrl Pts',(-18.7622230203345,-35.3020128619714,
122.394038689284)) ;
#47518=CARTESIAN_POINT('Ctrl Pts',(-18.600476033389,-35.1220237816085,122.139585076272)) ;
#47519=CARTESIAN_POINT('Ctrl Pts',(-18.5959401033665,-35.3119783288032,
122.521468994438)) ;
#47520=CARTESIAN_POINT('Ctrl Pts',(-18.3926205883172,-35.1319892484403,
122.298870811014)) ;
#47521=CARTESIAN_POINT('Ctrl Pts',(-18.4547977142894,-35.3218818910762,
122.674558023421)) ;
#47522=CARTESIAN_POINT('Ctrl Pts',(-18.2161904041538,-35.1418928107133,
122.490230413735)) ;
#47523=CARTESIAN_POINT('Ctrl Pts',(-18.3407694318747,-35.3319425689542,
122.852663128969)) ;
#47524=CARTESIAN_POINT('Ctrl Pts',(-18.0736527312663,-35.1519534885913,
122.712860272288)) ;
#47525=CARTESIAN_POINT('Ctrl Pts',(-18.2609128534862,-35.3417828669036,
123.043535459525)) ;
#47526=CARTESIAN_POINT('Ctrl Pts',(-17.9738293172813,-35.1617937865408,
122.951450001417)) ;
#47527=CARTESIAN_POINT('Ctrl Pts',(-18.2141440011338,-35.3518458618131,
123.24982878148)) ;
#47528=CARTESIAN_POINT('Ctrl Pts',(-17.9153656043643,-35.1718567814502,
123.209316008984)) ;
#47529=CARTESIAN_POINT('Ctrl Pts',(-18.2042462712093,-35.3617401559602,
123.457624789983)) ;
#47530=CARTESIAN_POINT('Ctrl Pts',(-17.9029906881241,-35.1817510755973,
123.469061216247)) ;
#47531=CARTESIAN_POINT('Ctrl Pts',(-18.2301365974252,-35.3716819536571,
123.66499700929)) ;
#47532=CARTESIAN_POINT('Ctrl Pts',(-17.9353509724904,-35.1916928732942,
123.728277083016)) ;
#47533=CARTESIAN_POINT('Ctrl Pts',(-18.2919583226803,-35.3816845311862,
123.866019002124)) ;
#47534=CARTESIAN_POINT('Ctrl Pts',(-18.0126256104855,-35.2016954508233,
123.979555436209)) ;
#47535=CARTESIAN_POINT('Ctrl Pts',(-18.38832214789,-35.3917189951073,124.053667683726)) ;
#47536=CARTESIAN_POINT('Ctrl Pts',(-18.1330779756745,-35.2117299147444,
124.214117512253)) ;
#47537=CARTESIAN_POINT('Ctrl Pts',(-18.5131632869251,-35.4015651336283,
124.218788839764)) ;
#47538=CARTESIAN_POINT('Ctrl Pts',(-18.2891276130123,-35.2215760532655,
124.420521008391)) ;
#47539=CARTESIAN_POINT('Ctrl Pts',(-18.6665221671683,-35.4115463068653,
124.361984621255)) ;
#47540=CARTESIAN_POINT('Ctrl Pts',(-18.4808245709193,-35.2315572265025,
124.59951775017)) ;
#47541=CARTESIAN_POINT('Ctrl Pts',(-18.8419525073359,-35.4214986008226,
124.476017082833)) ;
#47542=CARTESIAN_POINT('Ctrl Pts',(-18.7001113066703,-35.2415095204597,
124.742060651056)) ;
#47543=CARTESIAN_POINT('Ctrl Pts',(-19.0353199148675,-35.4314973959572,
124.558494549662)) ;
#47544=CARTESIAN_POINT('Ctrl Pts',(-18.9418196622479,-35.2515083155943,
124.845159871712)) ;
#47545=CARTESIAN_POINT('Ctrl Pts',(-19.2409602408548,-35.441536504218,124.605934758552)) ;
#47546=CARTESIAN_POINT('Ctrl Pts',(-19.1988694220206,-35.2615474238551,
124.904462676824)) ;
#47547=CARTESIAN_POINT('Ctrl Pts',(-19.4472187958602,-35.4513614456571,
124.617157941758)) ;
#47548=CARTESIAN_POINT('Ctrl Pts',(-19.4566932433114,-35.2713723652943,
124.918494235156)) ;
#47549=CARTESIAN_POINT('Ctrl Pts',(-19.6571046505334,-35.4614161327315,
124.59216665789)) ;
#47550=CARTESIAN_POINT('Ctrl Pts',(-19.7190507496054,-35.2814270523687,
124.887257605285)) ;
#47551=CARTESIAN_POINT('Ctrl Pts',(-19.8571259179256,-35.4713589376717,
124.531443581548)) ;
#47552=CARTESIAN_POINT('Ctrl Pts',(-19.9690783925131,-35.2913698573088,
124.811356103697)) ;
#47553=CARTESIAN_POINT('Ctrl Pts',(-20.0431203480413,-35.4812627236682,
124.437854636446)) ;
#47554=CARTESIAN_POINT('Ctrl Pts',(-20.2015729912878,-35.3012736433053,
124.694371844272)) ;
#47555=CARTESIAN_POINT('Ctrl Pts',(-20.2123551288087,-35.491309540233,124.31150595345)) ;
#47556=CARTESIAN_POINT('Ctrl Pts',(-20.4131178490129,-35.3113204598701,
124.536438012286)) ;
#47557=CARTESIAN_POINT('Ctrl Pts',(-20.355073515676,-35.5012050597117,124.160099178899)) ;
#47558=CARTESIAN_POINT('Ctrl Pts',(-20.5915179796175,-35.3212159793488,
124.347180770753)) ;
#47559=CARTESIAN_POINT('Ctrl Pts',(-20.471223424041,-35.5112671450361,123.983338753384)) ;
#47560=CARTESIAN_POINT('Ctrl Pts',(-20.7367072779153,-35.3312780646732,
124.126231712253)) ;
#47561=CARTESIAN_POINT('Ctrl Pts',(-20.5532221554608,-35.521109855994,123.793329340615)) ;
#47562=CARTESIAN_POINT('Ctrl Pts',(-20.8392082177454,-35.3411207756312,
123.888720096976)) ;
#47563=CARTESIAN_POINT('Ctrl Pts',(-20.6021745079103,-35.5311005733001,
123.589104323875)) ;
#47564=CARTESIAN_POINT('Ctrl Pts',(-20.9004009016988,-35.3511114929372,
123.633439183849)) ;
#47565=CARTESIAN_POINT('Ctrl Pts',(-20.6148094254628,-35.5410286563966,
123.380757851225)) ;
#47566=CARTESIAN_POINT('Ctrl Pts',(-20.9161968438839,-35.3610395760338,
123.373005745111)) ;
#47567=CARTESIAN_POINT('Ctrl Pts',(-20.5912974926631,-35.5510165865084,
123.172091972982)) ;
#47568=CARTESIAN_POINT('Ctrl Pts',(-20.8868090725257,-35.3710275061455,
123.112172972253)) ;
#47569=CARTESIAN_POINT('Ctrl Pts',(-20.5312904374153,-35.5610524126357,
122.969827521401)) ;
#47570=CARTESIAN_POINT('Ctrl Pts',(-20.8118024544747,-35.3810633322728,
122.859341843818)) ;
#47571=CARTESIAN_POINT('Ctrl Pts',(-20.4390581243751,-35.5709077497493,
122.78428606231)) ;
#47572=CARTESIAN_POINT('Ctrl Pts',(-20.6965136129544,-35.3909186693864,
122.627413231324)) ;
#47573=CARTESIAN_POINT('Ctrl Pts',(-20.3145205708958,-35.5809054845995,
122.614998952204)) ;
#47574=CARTESIAN_POINT('Ctrl Pts',(-20.5408432692029,-35.4009164042366,
122.415802979033)) ;
#47575=CARTESIAN_POINT('Ctrl Pts',(-20.1638726572033,-35.5908133885839,
122.471137864884)) ;
#47576=CARTESIAN_POINT('Ctrl Pts',(-20.3525343320192,-35.4108243082211,
122.235974665639)) ;
#47577=CARTESIAN_POINT('Ctrl Pts',(-19.9889273945464,-35.6008244631324,
122.354124867634)) ;
#47578=CARTESIAN_POINT('Ctrl Pts',(-20.1338538119606,-35.4208353827695,
122.089706748638)) ;
#47579=CARTESIAN_POINT('Ctrl Pts',(-19.7958300056756,-35.610852318668,122.269519731036)) ;
#47580=CARTESIAN_POINT('Ctrl Pts',(-19.8924829761476,-35.4308632383051,
121.983948431218)) ;
#47581=CARTESIAN_POINT('Ctrl Pts',(-19.5945466869052,-35.6207099125732,
122.220212795873)) ;
#47582=CARTESIAN_POINT('Ctrl Pts',(-19.6408783355081,-35.4407208322104,
121.922312589415)) ;
#47583=CARTESIAN_POINT('Ctrl Pts',(-19.3842341645356,-35.6307365994113,
122.205941341897)) ;
#47584=CARTESIAN_POINT('Ctrl Pts',(-19.3779878358377,-35.4507475190485,
121.904471410872)) ;
#47585=CARTESIAN_POINT('Ctrl Pts',(-19.1746497432009,-35.6407652685651,
122.228931469731)) ;
#47586=CARTESIAN_POINT('Ctrl Pts',(-19.116007159778,-35.4607761882022,121.933207053321)) ;
#47587=CARTESIAN_POINT('Ctrl Pts',(-18.9758531060999,-35.6506104768465,
122.286508207348)) ;
#47588=CARTESIAN_POINT('Ctrl Pts',(-18.8675097602884,-35.4706213964836,
122.005176454278)) ;
#47589=CARTESIAN_POINT('Ctrl Pts',(-18.78706524933,-35.6606011658096,122.378575193346)) ;
#47590=CARTESIAN_POINT('Ctrl Pts',(-18.6315240046396,-35.4806120854467,
122.120258716243)) ;
#47591=CARTESIAN_POINT('Ctrl Pts',(-18.6166109529874,-35.6706390420919,
122.502982907208)) ;
#47592=CARTESIAN_POINT('Ctrl Pts',(-18.4184551336644,-35.490649961729,122.275766762544)) ;
#47593=CARTESIAN_POINT('Ctrl Pts',(-18.4728999980008,-35.6804834197341,
122.651921164381)) ;
#47594=CARTESIAN_POINT('Ctrl Pts',(-18.2388143581137,-35.5004943393712,
122.461939201288)) ;
#47595=CARTESIAN_POINT('Ctrl Pts',(-18.3552581448824,-35.6904682241255,
122.825736375078)) ;
#47596=CARTESIAN_POINT('Ctrl Pts',(-18.0917605510307,-35.5104791437627,
122.679207506938)) ;
#47597=CARTESIAN_POINT('Ctrl Pts',(-18.2698663052676,-35.7004077543441,
123.016483700906)) ;
#47598=CARTESIAN_POINT('Ctrl Pts',(-17.9850190706446,-35.5204186739812,
122.917641507292)) ;
#47599=CARTESIAN_POINT('Ctrl Pts',(-18.218436347525,-35.710447442381,123.221171010836)) ;
#47600=CARTESIAN_POINT('Ctrl Pts',(-17.9207300902949,-35.5304583620181,
123.173500108613)) ;
#47601=CARTESIAN_POINT('Ctrl Pts',(-18.2034516389984,-35.7203357317493,
123.428524856059)) ;
#47602=CARTESIAN_POINT('Ctrl Pts',(-17.9019975600655,-35.5403466513864,
123.43269321979)) ;
#47603=CARTESIAN_POINT('Ctrl Pts',(-18.2245179381264,-35.7303248554341,
123.637461026191)) ;
#47604=CARTESIAN_POINT('Ctrl Pts',(-17.928329013415,-35.5503357750712,123.693863790479)) ;
#47605=CARTESIAN_POINT('Ctrl Pts',(-18.281534545644,-35.7402848651087,123.838935805631)) ;
#47606=CARTESIAN_POINT('Ctrl Pts',(-17.9995984433313,-35.5602957847458,
123.945708092075)) ;
#47607=CARTESIAN_POINT('Ctrl Pts',(-18.3716800461657,-35.7501852948129,
124.026546743199)) ;
#47608=CARTESIAN_POINT('Ctrl Pts',(-18.1122794989603,-35.57019621445,124.180223126085)) ;
#47609=CARTESIAN_POINT('Ctrl Pts',(-18.4947794817171,-35.7602283762197,
124.198074355247)) ;
#47610=CARTESIAN_POINT('Ctrl Pts',(-18.2661525939819,-35.5802392958568,
124.394633262475)) ;
#47611=CARTESIAN_POINT('Ctrl Pts',(-18.6437627494517,-35.7701357701273,
124.343645611898)) ;
#47612=CARTESIAN_POINT('Ctrl Pts',(-18.4523813317248,-35.5901466897644,
124.576598857662)) ;
#47613=CARTESIAN_POINT('Ctrl Pts',(-18.8173428519059,-35.7801475011165,
124.462690565596)) ;
#47614=CARTESIAN_POINT('Ctrl Pts',(-18.6693558214365,-35.6001584207536,
124.725406064343)) ;
#47615=CARTESIAN_POINT('Ctrl Pts',(-19.0095259153143,-35.7901797188313,
124.549587699707)) ;
#47616=CARTESIAN_POINT('Ctrl Pts',(-18.9095840015776,-35.6101906384684,
124.834028669225)) ;
#47617=CARTESIAN_POINT('Ctrl Pts',(-19.2101294613733,-35.8000322280774,
124.601126477445)) ;
#47618=CARTESIAN_POINT('Ctrl Pts',(-19.1603393482666,-35.6200431477146,
124.898453661677)) ;
#47619=CARTESIAN_POINT('Ctrl Pts',(-19.4188119264436,-35.8099901646204,
124.617871878663)) ;
#47620=CARTESIAN_POINT('Ctrl Pts',(-19.4211928177086,-35.6300010842576,
124.919386454323)) ;
#47621=CARTESIAN_POINT('Ctrl Pts',(-19.6288700822666,-35.8200290346287,
124.59759241421)) ;
#47622=CARTESIAN_POINT('Ctrl Pts',(-19.6837654584528,-35.6400399542659,
124.894038281209)) ;
#47623=CARTESIAN_POINT('Ctrl Pts',(-19.8290080686716,-35.829902189787,124.542441752005)) ;
#47624=CARTESIAN_POINT('Ctrl Pts',(-19.9339392913664,-35.6499131094241,
124.825100619419)) ;
#47625=CARTESIAN_POINT('Ctrl Pts',(-20.0202339068438,-35.8399754646367,
124.45154743179)) ;
#47626=CARTESIAN_POINT('Ctrl Pts',(-20.1729716447795,-35.6599863842738,
124.711483830272)) ;
#47627=CARTESIAN_POINT('Ctrl Pts',(-20.1886685597443,-35.8497957818141,
124.332082596939)) ;
#47628=CARTESIAN_POINT('Ctrl Pts',(-20.3835167615202,-35.6698067014512,
124.562152640001)) ;
#47629=CARTESIAN_POINT('Ctrl Pts',(-20.3376896490082,-35.8598744676076,
124.181528608811)) ;
#47630=CARTESIAN_POINT('Ctrl Pts',(-20.5697933970036,-35.6798853872447,
124.373961088606)) ;
#47631=CARTESIAN_POINT('Ctrl Pts',(-20.455705088691,-35.8697259789907,124.011272096574)) ;
#47632=CARTESIAN_POINT('Ctrl Pts',(-20.7173141230226,-35.6897368986278,
124.161139832778)) ;
#47633=CARTESIAN_POINT('Ctrl Pts',(-20.5444435166218,-35.8797994252973,
123.81902845343)) ;
#47634=CARTESIAN_POINT('Ctrl Pts',(-20.8282376597634,-35.6998103449344,
123.920835993557)) ;
#47635=CARTESIAN_POINT('Ctrl Pts',(-20.5972105460148,-35.889640700422,123.618952464279)) ;
#47636=CARTESIAN_POINT('Ctrl Pts',(-20.8941975462152,-35.7096516200591,
123.670739828049)) ;
#47637=CARTESIAN_POINT('Ctrl Pts',(-20.6153373392273,-35.8996258000788,
123.409838328814)) ;
#47638=CARTESIAN_POINT('Ctrl Pts',(-20.9168565666188,-35.7196367197159,
123.409346913405)) ;
#47639=CARTESIAN_POINT('Ctrl Pts',(-20.5965431076934,-35.9096332762131,
123.200274922463)) ;
#47640=CARTESIAN_POINT('Ctrl Pts',(-20.8933643885283,-35.7296441958502,
123.147392528966)) ;
#47641=CARTESIAN_POINT('Ctrl Pts',(-20.5423042520483,-35.919555863922,122.998856521941)) ;
#47642=CARTESIAN_POINT('Ctrl Pts',(-20.8255661487373,-35.7395667835592,
122.89561863727)) ;
#47643=CARTESIAN_POINT('Ctrl Pts',(-20.453642398187,-35.9295424681954,122.808524797024)) ;
#47644=CARTESIAN_POINT('Ctrl Pts',(-20.7147391058567,-35.7495533878325,
122.657703592569)) ;
#47645=CARTESIAN_POINT('Ctrl Pts',(-20.3323311287311,-35.9395825965295,
122.635813523666)) ;
#47646=CARTESIAN_POINT('Ctrl Pts',(-20.5631005957844,-35.7595935161666,
122.44181432373)) ;
#47647=CARTESIAN_POINT('Ctrl Pts',(-20.1861543358301,-35.9494220310629,
122.48942292078)) ;
#47648=CARTESIAN_POINT('Ctrl Pts',(-20.380378834698,-35.7694329507,122.258824742576)) ;
#47649=CARTESIAN_POINT('Ctrl Pts',(-20.0130523083208,-35.9594860855539,
122.367808286558)) ;
#47650=CARTESIAN_POINT('Ctrl Pts',(-20.1640017994239,-35.779497005191,122.106806406757)) ;
#47651=CARTESIAN_POINT('Ctrl Pts',(-19.8246772259409,-35.969377004791,122.279705165194)) ;
#47652=CARTESIAN_POINT('Ctrl Pts',(-19.9285321533398,-35.7893879244282,
121.996676734452)) ;
#47653=CARTESIAN_POINT('Ctrl Pts',(-19.6219619525249,-35.9793689980971,
122.224671937856)) ;
#47654=CARTESIAN_POINT('Ctrl Pts',(-19.67513790255,-35.7993799177342,121.927884966154)) ;
#47655=CARTESIAN_POINT('Ctrl Pts',(-19.4133577856184,-35.9893318620564,
122.205921690186)) ;
#47656=CARTESIAN_POINT('Ctrl Pts',(-19.4143822634357,-35.8093427816935,
121.904446853395)) ;
#47657=CARTESIAN_POINT('Ctrl Pts',(-19.2058271684787,-35.9992361218741,
122.223048719964)) ;
#47658=CARTESIAN_POINT('Ctrl Pts',(-19.1549680514992,-35.8192470415113,
121.925855666197)) ;
#47659=CARTESIAN_POINT('Ctrl Pts',(-19.0013346182317,-36.0092966124456,
122.276950648324)) ;
#47660=CARTESIAN_POINT('Ctrl Pts',(-18.8993526736226,-35.8293075320827,
121.993232864711)) ;
#47661=CARTESIAN_POINT('Ctrl Pts',(-18.8133472495276,-36.0191369620766,
122.363379425987)) ;
#47662=CARTESIAN_POINT('Ctrl Pts',(-18.6643671184913,-35.8391478817137,
122.101269435871)) ;
#47663=CARTESIAN_POINT('Ctrl Pts',(-18.639274963066,-36.0291999375666,122.483558189516)) ;
#47664=CARTESIAN_POINT('Ctrl Pts',(-18.4467771153745,-35.8492108572037,
122.251492745729)) ;
#47665=CARTESIAN_POINT('Ctrl Pts',(-18.4913225975558,-36.03909425771,122.629802380059)) ;
#47666=CARTESIAN_POINT('Ctrl Pts',(-18.2618359407232,-35.8591051773471,
122.434298711921)) ;
#47667=CARTESIAN_POINT('Ctrl Pts',(-18.3700032350797,-36.0490359708416,
122.799959594122)) ;
#47668=CARTESIAN_POINT('Ctrl Pts',(-18.1101865601334,-35.8690468904787,
122.646995887001)) ;
#47669=CARTESIAN_POINT('Ctrl Pts',(-18.2794097534421,-36.0590388606357,
122.98977331008)) ;
#47670=CARTESIAN_POINT('Ctrl Pts',(-17.9969449047293,-35.8790497802728,
122.884263259516)) ;
#47671=CARTESIAN_POINT('Ctrl Pts',(-18.2233291545152,-36.0690787177962,
123.193235333935)) ;
#47672=CARTESIAN_POINT('Ctrl Pts',(-17.9268443214871,-35.8890896374333,
123.138590645404)) ;
#47673=CARTESIAN_POINT('Ctrl Pts',(-18.2033834024276,-36.0789028986338,
123.39882135021)) ;
#47674=CARTESIAN_POINT('Ctrl Pts',(-17.9019122829128,-35.8989138182709,
123.395574782342)) ;
#47675=CARTESIAN_POINT('Ctrl Pts',(-18.2195239600936,-36.088959872137,123.609616533739)) ;
#47676=CARTESIAN_POINT('Ctrl Pts',(-17.9220883778628,-35.9089707917741,
123.659068393619)) ;
#47677=CARTESIAN_POINT('Ctrl Pts',(-18.271611751821,-36.0988879963241,123.811744957845)) ;
#47678=CARTESIAN_POINT('Ctrl Pts',(-17.9871986049093,-35.9188989159612,
123.911729558089)) ;
#47679=CARTESIAN_POINT('Ctrl Pts',(-18.3577130799816,-36.1088416913975,
124.002470019801)) ;
#47680=CARTESIAN_POINT('Ctrl Pts',(-18.0948259751119,-35.9288526110346,
124.150136156797)) ;
#47681=CARTESIAN_POINT('Ctrl Pts',(-18.4769655018994,-36.1188878849728,
124.176781923495)) ;
#47682=CARTESIAN_POINT('Ctrl Pts',(-18.2438917115577,-35.9388988046099,
124.368025599995)) ;
#47683=CARTESIAN_POINT('Ctrl Pts',(-18.6216180385642,-36.1287359873327,
124.324902759185)) ;
#47684=CARTESIAN_POINT('Ctrl Pts',(-18.4247087145349,-35.9487469069698,
124.553177298368)) ;
#47685=CARTESIAN_POINT('Ctrl Pts',(-18.7913448950173,-36.1386975755603,
124.447570338406)) ;
#47686=CARTESIAN_POINT('Ctrl Pts',(-18.6368680943373,-35.9587084951974,
124.706511430656)) ;
#47687=CARTESIAN_POINT('Ctrl Pts',(-18.9811968842923,-36.1487262457165,
124.539290730649)) ;
#47688=CARTESIAN_POINT('Ctrl Pts',(-18.8741832744797,-35.9687371653537,
124.821161297278)) ;
#47689=CARTESIAN_POINT('Ctrl Pts',(-19.181656131435,-36.1586365485983,124.596034870755)) ;
#47690=CARTESIAN_POINT('Ctrl Pts',(-19.1247583602108,-35.9786474682354,
124.892091064519)) ;
#47691=CARTESIAN_POINT('Ctrl Pts',(-19.3893970231701,-36.1685714324062,
124.617709477038)) ;
#47692=CARTESIAN_POINT('Ctrl Pts',(-19.3844352240823,-35.9885823520433,
124.919183512007)) ;
#47693=CARTESIAN_POINT('Ctrl Pts',(-19.5999475350248,-36.1786125740968,
124.602631344921)) ;
#47694=CARTESIAN_POINT('Ctrl Pts',(-19.6476231191508,-35.9986234937339,
124.900335055066)) ;
#47695=CARTESIAN_POINT('Ctrl Pts',(-19.801594360988,-36.1884996952608,124.552149971975)) ;
#47696=CARTESIAN_POINT('Ctrl Pts',(-19.8996824512963,-36.0085106148979,
124.837232249301)) ;
#47697=CARTESIAN_POINT('Ctrl Pts',(-19.9935521891846,-36.1984920381093,
124.466851568675)) ;
#47698=CARTESIAN_POINT('Ctrl Pts',(-20.1396295182809,-36.0185029577464,
124.730608252142)) ;
#47699=CARTESIAN_POINT('Ctrl Pts',(-20.1670027855748,-36.2084403393333,
124.34997292154)) ;
#47700=CARTESIAN_POINT('Ctrl Pts',(-20.3564426703236,-36.0284512589704,
124.584508836111)) ;
#47701=CARTESIAN_POINT('Ctrl Pts',(-20.317556983034,-36.2183779170154,124.205144373366)) ;
#47702=CARTESIAN_POINT('Ctrl Pts',(-20.5446351269655,-36.0383888366525,
124.403471920414)) ;
#47703=CARTESIAN_POINT('Ctrl Pts',(-20.4414732897196,-36.228364491466,124.035646668692)) ;
#47704=CARTESIAN_POINT('Ctrl Pts',(-20.6995297067376,-36.0483754111031,
124.191598913458)) ;
#47705=CARTESIAN_POINT('Ctrl Pts',(-20.5342434755889,-36.2383933013744,
123.846317983117)) ;
#47706=CARTESIAN_POINT('Ctrl Pts',(-20.8154914356218,-36.0584042210115,
123.954937669147)) ;
#47707=CARTESIAN_POINT('Ctrl Pts',(-20.5920471788539,-36.2482716226812,
123.646853844354)) ;
#47708=CARTESIAN_POINT('Ctrl Pts',(-20.887745257479,-36.0682825423183,123.705606150759)) ;
#47709=CARTESIAN_POINT('Ctrl Pts',(-20.6150868311933,-36.2582632700286,
123.438058171806)) ;
#47710=CARTESIAN_POINT('Ctrl Pts',(-20.9165435264159,-36.0782741896657,
123.444611225449)) ;
#47711=CARTESIAN_POINT('Ctrl Pts',(-20.6010348993728,-36.2682977934664,
123.22757890962)) ;
#47712=CARTESIAN_POINT('Ctrl Pts',(-20.8989774525734,-36.0883087131035,
123.181512331536)) ;
#47713=CARTESIAN_POINT('Ctrl Pts',(-20.5519217356949,-36.278161150345,123.026098209884)) ;
#47714=CARTESIAN_POINT('Ctrl Pts',(-20.8375844347476,-36.0981720699821,
122.929660650926)) ;
#47715=CARTESIAN_POINT('Ctrl Pts',(-20.4668785726101,-36.2882313770253,
122.832246771308)) ;
#47716=CARTESIAN_POINT('Ctrl Pts',(-20.7312794061574,-36.1082422966624,
122.687347241547)) ;
#47717=CARTESIAN_POINT('Ctrl Pts',(-20.3520998438178,-36.2980736851599,
122.660073371831)) ;
#47718=CARTESIAN_POINT('Ctrl Pts',(-20.5878041611143,-36.1180846047971,
122.472130151302)) ;
#47719=CARTESIAN_POINT('Ctrl Pts',(-20.2080189864902,-36.3080344171834,
122.508121261806)) ;
#47720=CARTESIAN_POINT('Ctrl Pts',(-20.4077016432791,-36.1280453368205,
122.282190824122)) ;
#47721=CARTESIAN_POINT('Ctrl Pts',(-20.038192664759,-36.3180723063815,122.382865970972)) ;
#47722=CARTESIAN_POINT('Ctrl Pts',(-20.1954179813049,-36.1380832260186,
122.125622966376)) ;
#47723=CARTESIAN_POINT('Ctrl Pts',(-19.8524204650629,-36.3279465893003,
122.290172252973)) ;
#47724=CARTESIAN_POINT('Ctrl Pts',(-19.9632011127719,-36.1479575089374,
122.009756791366)) ;
#47725=CARTESIAN_POINT('Ctrl Pts',(-19.6494833161937,-36.3380163339178,
122.23000096421)) ;
#47726=CARTESIAN_POINT('Ctrl Pts',(-19.7095295605332,-36.1580272535549,
121.93454430428)) ;
#47727=CARTESIAN_POINT('Ctrl Pts',(-19.4440883718789,-36.3478496442634,
122.206429346095)) ;
#47728=CARTESIAN_POINT('Ctrl Pts',(-19.4527844206973,-36.1678605639005,
121.90508124975)) ;
#47729=CARTESIAN_POINT('Ctrl Pts',(-19.2335726861195,-36.3578798876161,
122.218526616125)) ;
#47730=CARTESIAN_POINT('Ctrl Pts',(-19.1896400044963,-36.1778908072532,
121.920204651437)) ;
#47731=CARTESIAN_POINT('Ctrl Pts',(-19.0284500534322,-36.3679121755945,
122.267618772406)) ;
#47732=CARTESIAN_POINT('Ctrl Pts',(-18.9332371754208,-36.1879230952316,
121.981571396722)) ;
#47733=CARTESIAN_POINT('Ctrl Pts',(-18.838731464373,-36.3777393520626,122.349413172309)) ;
#47734=CARTESIAN_POINT('Ctrl Pts',(-18.6960884547325,-36.1977502716997,
122.083816541885)) ;
#47735=CARTESIAN_POINT('Ctrl Pts',(-18.66275010468,-36.3877447349294,122.464585531392)) ;
#47736=CARTESIAN_POINT('Ctrl Pts',(-18.4761127317123,-36.2077556545666,
122.22778364051)) ;
#47737=CARTESIAN_POINT('Ctrl Pts',(-18.5097875290952,-36.3977273739222,
122.608332945589)) ;
#47738=CARTESIAN_POINT('Ctrl Pts',(-18.2849106465945,-36.2177382935593,
122.407469430057)) ;
#47739=CARTESIAN_POINT('Ctrl Pts',(-18.3835787051131,-36.4077714410588,
122.777596314135)) ;
#47740=CARTESIAN_POINT('Ctrl Pts',(-18.127151161634,-36.2277823606959,122.619049599079)) ;
#47741=CARTESIAN_POINT('Ctrl Pts',(-18.2904495023674,-36.4175926598628,
122.961880766302)) ;
#47742=CARTESIAN_POINT('Ctrl Pts',(-18.0107408057579,-36.2376035794999,
122.849407145954)) ;
#47743=CARTESIAN_POINT('Ctrl Pts',(-18.2289081179151,-36.4276294988008,
123.163709417083)) ;
#47744=CARTESIAN_POINT('Ctrl Pts',(-17.9338160941293,-36.247640418438,123.101693464145)) ;
#47745=CARTESIAN_POINT('Ctrl Pts',(-18.2039726595456,-36.4376539108986,
123.372981004564)) ;
#47746=CARTESIAN_POINT('Ctrl Pts',(-17.902648663204,-36.2576648305357,123.363283148383)) ;
#47747=CARTESIAN_POINT('Ctrl Pts',(-18.215091683057,-36.4475059953039,123.579807254946)) ;
#47748=CARTESIAN_POINT('Ctrl Pts',(-17.9165495303506,-36.267516914941,123.621816862721)) ;
#47749=CARTESIAN_POINT('Ctrl Pts',(-18.2622958006013,-36.457496892047,123.784448454171)) ;
#47750=CARTESIAN_POINT('Ctrl Pts',(-17.9755567901383,-36.2775078116842,
123.877618050233)) ;
#47751=CARTESIAN_POINT('Ctrl Pts',(-18.3436111264905,-36.467414883948,123.976473263927)) ;
#47752=CARTESIAN_POINT('Ctrl Pts',(-18.0772031608818,-36.2874258035851,
124.117648747743)) ;
#47753=CARTESIAN_POINT('Ctrl Pts',(-18.4582275633681,-36.477442999405,124.153397817123)) ;
#47754=CARTESIAN_POINT('Ctrl Pts',(-18.2204755143682,-36.2974539190421,
124.338803226218)) ;
#47755=CARTESIAN_POINT('Ctrl Pts',(-18.5997258463659,-36.4873281753471,
124.305609353233)) ;
#47756=CARTESIAN_POINT('Ctrl Pts',(-18.3973504809565,-36.3073390949842,
124.529066690562)) ;
#47757=CARTESIAN_POINT('Ctrl Pts',(-18.7669421447371,-36.497317533754,124.432667569944)) ;
#47758=CARTESIAN_POINT('Ctrl Pts',(-18.6063723872479,-36.3173284533911,
124.687887703223)) ;
#47759=CARTESIAN_POINT('Ctrl Pts',(-18.9548477278309,-36.5073586813343,
124.528860622711)) ;
#47760=CARTESIAN_POINT('Ctrl Pts',(-18.8412552934419,-36.3273696009714,
124.808127004772)) ;
#47761=CARTESIAN_POINT('Ctrl Pts',(-19.1523079783713,-36.5171913043407,
124.590003139352)) ;
#47762=CARTESIAN_POINT('Ctrl Pts',(-19.088082204701,-36.3372022239778,124.884553235414)) ;
#47763=CARTESIAN_POINT('Ctrl Pts',(-19.3606753506828,-36.5271853754515,
124.616945728491)) ;
#47764=CARTESIAN_POINT('Ctrl Pts',(-19.3485418518654,-36.3471962950886,
124.918229067231)) ;
#47765=CARTESIAN_POINT('Ctrl Pts',(-19.5712789350383,-36.5372140330923,
124.606849592832)) ;
#47766=CARTESIAN_POINT('Ctrl Pts',(-19.6117962054243,-36.3572249527295,
124.905606556835)) ;
#47767=CARTESIAN_POINT('Ctrl Pts',(-19.7740000727098,-36.5470983592851,
124.561235915968)) ;
#47768=CARTESIAN_POINT('Ctrl Pts',(-19.8651977309864,-36.3671092789223,
124.848586979554)) ;
#47769=CARTESIAN_POINT('Ctrl Pts',(-19.9675160561407,-36.5570641027758,
124.48092624152)) ;
#47770=CARTESIAN_POINT('Ctrl Pts',(-20.1070919688669,-36.3770750224129,
124.748197481995)) ;
#47771=CARTESIAN_POINT('Ctrl Pts',(-20.1450804636381,-36.567092481907,124.36727939808)) ;
#47772=CARTESIAN_POINT('Ctrl Pts',(-20.3290461476334,-36.3871034015441,
124.606136879299)) ;
#47773=CARTESIAN_POINT('Ctrl Pts',(-20.2984821281396,-36.5769933281139,
124.226551618622)) ;
#47774=CARTESIAN_POINT('Ctrl Pts',(-20.5207969131445,-36.397004247751,124.430224963369)) ;
#47775=CARTESIAN_POINT('Ctrl Pts',(-20.4270554223315,-36.587051985531,124.058705204649)) ;
#47776=CARTESIAN_POINT('Ctrl Pts',(-20.6815114754316,-36.4070629051681,
124.220415524595)) ;
#47777=CARTESIAN_POINT('Ctrl Pts',(-20.5228088976676,-36.5969095483129,
123.874874545121)) ;
#47778=CARTESIAN_POINT('Ctrl Pts',(-20.8012013743605,-36.41692046795,123.990625446808)) ;
#47779=CARTESIAN_POINT('Ctrl Pts',(-20.5866346710282,-36.6069779508661,
123.673090041248)) ;
#47780=CARTESIAN_POINT('Ctrl Pts',(-20.8809810994181,-36.4269888705032,
123.738394192383)) ;
#47781=CARTESIAN_POINT('Ctrl Pts',(-20.6138518765132,-36.6168333496057,
123.46767623189)) ;
#47782=CARTESIAN_POINT('Ctrl Pts',(-20.9150001537344,-36.4368442692428,
123.481625971228)) ;
#47783=CARTESIAN_POINT('Ctrl Pts',(-20.6054955842666,-36.6268282166796,
123.257725834414)) ;
#47784=CARTESIAN_POINT('Ctrl Pts',(-20.9045521214138,-36.4468391363167,
123.219187981031)) ;
#47785=CARTESIAN_POINT('Ctrl Pts',(-20.5602021180779,-36.636859511663,123.051753465069)) ;
#47786=CARTESIAN_POINT('Ctrl Pts',(-20.8479327596291,-36.4568704313002,
122.961723074886)) ;
#47787=CARTESIAN_POINT('Ctrl Pts',(-20.4814585623447,-36.6467260363896,
122.859848018416)) ;
#47788=CARTESIAN_POINT('Ctrl Pts',(-20.7495006730971,-36.4667369560267,
122.721841789066)) ;
#47789=CARTESIAN_POINT('Ctrl Pts',(-20.3695334272533,-36.6567135070853,
122.682228468216)) ;
#47790=CARTESIAN_POINT('Ctrl Pts',(-20.609591909687,-36.4767244267224,122.499818683266)) ;
#47791=CARTESIAN_POINT('Ctrl Pts',(-20.2291188401914,-36.6666582666492,
122.527284926112)) ;
#47792=CARTESIAN_POINT('Ctrl Pts',(-20.4340715146542,-36.4866691862863,
122.306140896146)) ;
#47793=CARTESIAN_POINT('Ctrl Pts',(-20.0622231051933,-36.676703822598,122.397914061097)) ;
#47794=CARTESIAN_POINT('Ctrl Pts',(-20.2254502142119,-36.4967147422351,
122.144429454285)) ;
#47795=CARTESIAN_POINT('Ctrl Pts',(-19.8789187763763,-36.6865634109731,
122.301092451122)) ;
#47796=CARTESIAN_POINT('Ctrl Pts',(-19.9963181527322,-36.5065743306102,
122.023404639029)) ;
#47797=CARTESIAN_POINT('Ctrl Pts',(-19.6789119610615,-36.6965643661092,
122.23637511333)) ;
#47798=CARTESIAN_POINT('Ctrl Pts',(-19.7463087037596,-36.5165752857463,
121.942510562632)) ;
#47799=CARTESIAN_POINT('Ctrl Pts',(-19.4726764661033,-36.7064685933867,
122.207479051172)) ;
#47800=CARTESIAN_POINT('Ctrl Pts',(-19.4885136890261,-36.5264795130239,
121.906393185174)) ;
#47801=CARTESIAN_POINT('Ctrl Pts',(-19.2617182497028,-36.7165106702819,
122.214872705184)) ;
#47802=CARTESIAN_POINT('Ctrl Pts',(-19.2248160077214,-36.536521589919,121.915638023373)) ;
#47803=CARTESIAN_POINT('Ctrl Pts',(-19.057927154021,-36.726418282968,122.2581086562)) ;
#47804=CARTESIAN_POINT('Ctrl Pts',(-18.9700774883834,-36.5464292026052,
121.969685726458)) ;
#47805=CARTESIAN_POINT('Ctrl Pts',(-18.8619321432003,-36.7364728135838,
122.337188886544)) ;
#47806=CARTESIAN_POINT('Ctrl Pts',(-18.7250847627801,-36.5564837332209,
122.068538595468)) ;
#47807=CARTESIAN_POINT('Ctrl Pts',(-18.6859875564324,-36.7463336001326,
122.446869658722)) ;
#47808=CARTESIAN_POINT('Ctrl Pts',(-18.5051552713082,-36.5663445197698,
122.205642071035)) ;
#47809=CARTESIAN_POINT('Ctrl Pts',(-18.5294655824155,-36.7563273552037,
122.586972488339)) ;
#47810=CARTESIAN_POINT('Ctrl Pts',(-18.309504624998,-36.5763382748409,122.380772756738)) ;
#47811=CARTESIAN_POINT('Ctrl Pts',(-18.4004150751371,-36.7662527154437,
122.750983302961)) ;
#47812=CARTESIAN_POINT('Ctrl Pts',(-18.1481936177485,-36.5862636350808,
122.585788118924)) ;
#47813=CARTESIAN_POINT('Ctrl Pts',(-18.3008055717462,-36.776280644839,122.936753966816)) ;
#47814=CARTESIAN_POINT('Ctrl Pts',(-18.0236841922653,-36.5962915644761,
122.818002834881)) ;
#47815=CARTESIAN_POINT('Ctrl Pts',(-18.2356726374387,-36.7861669116383,
123.134158053417)) ;
#47816=CARTESIAN_POINT('Ctrl Pts',(-17.9422706636189,-36.6061778312754,
123.064758942346)) ;
#47817=CARTESIAN_POINT('Ctrl Pts',(-18.2052669474954,-36.7961986805365,
123.342818627154)) ;
#47818=CARTESIAN_POINT('Ctrl Pts',(-17.9042663342486,-36.6162096001737,
123.325585129761)) ;
#47819=CARTESIAN_POINT('Ctrl Pts',(-18.2112586660847,-36.8060802763801,
123.550511838692)) ;
#47820=CARTESIAN_POINT('Ctrl Pts',(-17.9117588182437,-36.6260911960173,
123.585201643652)) ;
#47821=CARTESIAN_POINT('Ctrl Pts',(-18.2539211094933,-36.8161421618481,
123.757665242363)) ;
#47822=CARTESIAN_POINT('Ctrl Pts',(-17.9650896020763,-36.6361530814852,
123.844142860244)) ;
#47823=CARTESIAN_POINT('Ctrl Pts',(-18.3302768913769,-36.825999595867,123.950348541592)) ;
#47824=CARTESIAN_POINT('Ctrl Pts',(-18.0605371633806,-36.6460105155041,
124.084996144572)) ;
#47825=CARTESIAN_POINT('Ctrl Pts',(-18.4400202960657,-36.8359928389089,
124.129465514795)) ;
#47826=CARTESIAN_POINT('Ctrl Pts',(-18.1977180729179,-36.6560037585461,
124.308890236601)) ;
#47827=CARTESIAN_POINT('Ctrl Pts',(-18.5783392874067,-36.8459235997953,
124.285860530243)) ;
#47828=CARTESIAN_POINT('Ctrl Pts',(-18.3706217888367,-36.6659345194324,
124.504384734692)) ;
#47829=CARTESIAN_POINT('Ctrl Pts',(-18.7977945098984,-36.8592725919925,
124.460845444457)) ;
#47830=CARTESIAN_POINT('Ctrl Pts',(-18.6449288885869,-36.6792835116296,
124.7231001116)) ;
#47831=CARTESIAN_POINT('Ctrl Pts',(-19.0564575910086,-36.8725409648089,
124.573487171901)) ;
#47832=CARTESIAN_POINT('Ctrl Pts',(-18.9682246085567,-36.692551884446,124.863897618014)) ;
#47833=CARTESIAN_POINT('Ctrl Pts',(-19.332518152077,-36.8858239061933,124.615432948066)) ;
#47834=CARTESIAN_POINT('Ctrl Pts',(-19.3133563776516,-36.7058348258304,
124.916340475203)) ;
#47835=CARTESIAN_POINT('Ctrl Pts',(-19.5435804177348,-36.8958666920355,
124.610274690913)) ;
#47836=CARTESIAN_POINT('Ctrl Pts',(-19.5771730601609,-36.7158776116726,
124.9098870958)) ;
#47837=CARTESIAN_POINT('Ctrl Pts',(-19.7466220723449,-36.9057166345876,
124.569566521813)) ;
#47838=CARTESIAN_POINT('Ctrl Pts',(-19.8309776235917,-36.7257275542247,
124.858999538569)) ;
#47839=CARTESIAN_POINT('Ctrl Pts',(-19.9425753325179,-36.9157138675065,
124.493590570334)) ;
#47840=CARTESIAN_POINT('Ctrl Pts',(-20.0759163398289,-36.7357247871437,
124.764028514352)) ;
#47841=CARTESIAN_POINT('Ctrl Pts',(-20.1225212109622,-36.9257287628411,
124.384267908977)) ;
#47842=CARTESIAN_POINT('Ctrl Pts',(-20.3008516831836,-36.7457396824782,
124.627366616209)) ;
#47843=CARTESIAN_POINT('Ctrl Pts',(-20.3318880894533,-36.9389684394793,
124.200821795761)) ;
#47844=CARTESIAN_POINT('Ctrl Pts',(-20.5625371625823,-36.7589793591164,
124.398087289449)) ;
#47845=CARTESIAN_POINT('Ctrl Pts',(-20.528163224449,-36.9555156638846,123.9088995619)) ;
#47846=CARTESIAN_POINT('Ctrl Pts',(-20.8079029753691,-36.7755265835217,
124.033128787356)) ;
#47847=CARTESIAN_POINT('Ctrl Pts',(-20.6137528393046,-36.9721631010157,
123.56536786537)) ;
#47848=CARTESIAN_POINT('Ctrl Pts',(-20.9148689308505,-36.7921740206528,
123.60379676647)) ;
#47849=CARTESIAN_POINT('Ctrl Pts',(-20.6085683059766,-36.9854525984939,
123.286061986322)) ;
#47850=CARTESIAN_POINT('Ctrl Pts',(-20.9083945687103,-36.805463518131,123.254597757722)) ;
#47851=CARTESIAN_POINT('Ctrl Pts',(-20.5693560188396,-36.9953260063163,
123.082217819628)) ;
#47852=CARTESIAN_POINT('Ctrl Pts',(-20.8593749513475,-36.8153369259534,
122.99980702422)) ;
#47853=CARTESIAN_POINT('Ctrl Pts',(-20.4940428412356,-37.005378383909,122.884773388024)) ;
#47854=CARTESIAN_POINT('Ctrl Pts',(-20.7652312032613,-36.8253893035461,
122.752998369539)) ;
#47855=CARTESIAN_POINT('Ctrl Pts',(-20.3871047058436,-37.0152820374499,
122.706108282335)) ;
#47856=CARTESIAN_POINT('Ctrl Pts',(-20.6315577727922,-36.835292957087,122.529670136184)) ;
#47857=CARTESIAN_POINT('Ctrl Pts',(-20.2506236096731,-37.0252263064452,
122.547784485508)) ;
#47858=CARTESIAN_POINT('Ctrl Pts',(-20.4609498467479,-36.8452372260823,
122.331765024518)) ;
#47859=CARTESIAN_POINT('Ctrl Pts',(-20.0335787700198,-37.0385573147779,
122.37035520076)) ;
#47860=CARTESIAN_POINT('Ctrl Pts',(-20.1896663855523,-36.858568234415,122.109990345323)) ;
#47861=CARTESIAN_POINT('Ctrl Pts',(-19.7113303634737,-37.0551788953021,
122.225449965275)) ;
#47862=CARTESIAN_POINT('Ctrl Pts',(-19.7868089891935,-36.8751898149393,
121.928852787723)) ;
#47863=CARTESIAN_POINT('Ctrl Pts',(-19.3605381967804,-37.0717215660005,
122.198625173765)) ;
#47864=CARTESIAN_POINT('Ctrl Pts',(-19.3483970122196,-36.8917324856377,
121.895325330693)) ;
#47865=CARTESIAN_POINT('Ctrl Pts',(-19.084756283337,-37.0850707255635,122.250326858334)) ;
#47866=CARTESIAN_POINT('Ctrl Pts',(-19.0036058959069,-36.9050816452006,
121.959959179237)) ;
#47867=CARTESIAN_POINT('Ctrl Pts',(-18.8243006026364,-37.098298875723,122.34794994263)) ;
#47868=CARTESIAN_POINT('Ctrl Pts',(-18.678061892058,-36.9183097953601,122.081981867065)) ;
#47869=CARTESIAN_POINT('Ctrl Pts',(-18.5364100435384,-37.1149295528605,
122.553165444984)) ;
#47870=CARTESIAN_POINT('Ctrl Pts',(-18.3181836591371,-36.9349404724976,
122.338513488551)) ;
#47871=CARTESIAN_POINT('Ctrl Pts',(-18.2963005996991,-37.1348324921486,
122.901714167161)) ;
#47872=CARTESIAN_POINT('Ctrl Pts',(-18.0180562107992,-36.9548434117857,
122.774198058464)) ;
#47873=CARTESIAN_POINT('Ctrl Pts',(-18.1891582578052,-37.1547353587518,
123.311031502207)) ;
#47874=CARTESIAN_POINT('Ctrl Pts',(-17.884130698863,-36.974746278389,123.285845641894)) ;
#47875=CARTESIAN_POINT('Ctrl Pts',(-18.2275156867731,-37.1746485238567,
123.732793359214)) ;
#47876=CARTESIAN_POINT('Ctrl Pts',(-17.9320811341198,-36.9946594434938,
123.813046654327)) ;
#47877=CARTESIAN_POINT('Ctrl Pts',(-18.409140585469,-37.194684352998,124.118086353196)) ;
#47878=CARTESIAN_POINT('Ctrl Pts',(-18.159115508631,-37.0146952726351,124.294661831118)) ;
#47879=CARTESIAN_POINT('Ctrl Pts',(-18.7080016710259,-37.2145029278761,
124.41531311931)) ;
#47880=CARTESIAN_POINT('Ctrl Pts',(-18.5326928560836,-37.0345138475132,
124.666191700449)) ;
#47881=CARTESIAN_POINT('Ctrl Pts',(-19.0927718739483,-37.2344732289181,
124.594578380774)) ;
#47882=CARTESIAN_POINT('Ctrl Pts',(-19.0136563927245,-37.0544841485552,
124.890270639901)) ;
#47883=CARTESIAN_POINT('Ctrl Pts',(-19.5142339391822,-37.2543647612826,
124.631795562197)) ;
#47884=CARTESIAN_POINT('Ctrl Pts',(-19.5404829664515,-37.0743756809197,
124.936789595179)) ;
#47885=CARTESIAN_POINT('Ctrl Pts',(-19.9254766838517,-37.2743878590991,
124.521993821233)) ;
#47886=CARTESIAN_POINT('Ctrl Pts',(-20.0545360586126,-37.0943987787363,
124.799534983068)) ;
#47887=CARTESIAN_POINT('Ctrl Pts',(-20.2709110278147,-37.2941846120191,
124.281362408259)) ;
#47888=CARTESIAN_POINT('Ctrl Pts',(-20.4863256454403,-37.1141955316562,
124.498745537816)) ;
#47889=CARTESIAN_POINT('Ctrl Pts',(-20.5163858033962,-37.3141457005079,
123.935170853578)) ;
#47890=CARTESIAN_POINT('Ctrl Pts',(-20.7931678599209,-37.134156620145,124.066005974626)) ;
#47891=CARTESIAN_POINT('Ctrl Pts',(-20.6282493094601,-37.33412396944,123.52533621411)) ;
#47892=CARTESIAN_POINT('Ctrl Pts',(-20.9329957734479,-37.1541348890772,
123.553712501942)) ;
#47893=CARTESIAN_POINT('Ctrl Pts',(-20.5944348756213,-37.353943984231,123.105306555051)) ;
#47894=CARTESIAN_POINT('Ctrl Pts',(-20.8907271345775,-37.1739549038682,
123.028678283237)) ;
#47895=CARTESIAN_POINT('Ctrl Pts',(-20.419241626978,-37.3738823934829,122.719230553153)) ;
#47896=CARTESIAN_POINT('Ctrl Pts',(-20.6717362479,-37.19389331312,122.546084069936)) ;
#47897=CARTESIAN_POINT('Ctrl Pts',(-20.1204934119422,-37.3939295108753,
122.415110115247)) ;
#47898=CARTESIAN_POINT('Ctrl Pts',(-20.298300215747,-37.2139404305124,122.165933042875)) ;
#47899=CARTESIAN_POINT('Ctrl Pts',(-19.7397550775313,-37.4137757567091,
122.233254243053)) ;
#47900=CARTESIAN_POINT('Ctrl Pts',(-19.8223796112928,-37.2337866763463,
121.938614397227)) ;
#47901=CARTESIAN_POINT('Ctrl Pts',(-19.3198536517042,-37.4336247252212,
122.19057464082)) ;
#47902=CARTESIAN_POINT('Ctrl Pts',(-19.2975051439848,-37.2536356448583,
121.885263707638)) ;
#47903=CARTESIAN_POINT('Ctrl Pts',(-18.9066386247496,-37.4536750275325,
122.295305344993)) ;
#47904=CARTESIAN_POINT('Ctrl Pts',(-18.7809853427193,-37.2736859471696,
122.01617607887)) ;
#47905=CARTESIAN_POINT('Ctrl Pts',(-18.5576843444494,-37.4735099499637,
122.53234187102)) ;
#47906=CARTESIAN_POINT('Ctrl Pts',(-18.3447935795883,-37.2935208696008,
122.312469305322)) ;
#47907=CARTESIAN_POINT('Ctrl Pts',(-18.3088629623989,-37.4934403511896,
122.87517401801)) ;
#47908=CARTESIAN_POINT('Ctrl Pts',(-18.0337656489116,-37.3134512708267,
122.741007439741)) ;
#47909=CARTESIAN_POINT('Ctrl Pts',(-18.191627159294,-37.5133252965484,123.281572566289)) ;
#47910=CARTESIAN_POINT('Ctrl Pts',(-17.8872187178112,-37.3333362161856,
123.249003693809)) ;
#47911=CARTESIAN_POINT('Ctrl Pts',(-18.2210576117943,-37.5333979046998,
123.707273120117)) ;
#47912=CARTESIAN_POINT('Ctrl Pts',(-17.9240043991043,-37.353408824337,123.781130410511)) ;
#47913=CARTESIAN_POINT('Ctrl Pts',(-18.3915612941918,-37.5531892210279,
124.092070927854)) ;
#47914=CARTESIAN_POINT('Ctrl Pts',(-18.1371306277917,-37.3732001406651,
124.262126611238)) ;
#47915=CARTESIAN_POINT('Ctrl Pts',(-18.6846818237289,-37.5731540107952,
124.399080855856)) ;
#47916=CARTESIAN_POINT('Ctrl Pts',(-18.5035285318798,-37.3931649304323,
124.645891221234)) ;
#47917=CARTESIAN_POINT('Ctrl Pts',(-19.0658286606464,-37.5931369665455,
124.5868719561)) ;
#47918=CARTESIAN_POINT('Ctrl Pts',(-18.979960539183,-37.4131478861826,124.8806328502)) ;
#47919=CARTESIAN_POINT('Ctrl Pts',(-19.4844281526955,-37.6129454885216,
124.633785399383)) ;
#47920=CARTESIAN_POINT('Ctrl Pts',(-19.5032077670167,-37.4329564081588,
124.93927814081)) ;
#47921=CARTESIAN_POINT('Ctrl Pts',(-19.8975569980139,-37.6329310632575,
124.534652953361)) ;
#47922=CARTESIAN_POINT('Ctrl Pts',(-20.0196196742879,-37.4529419828946,
124.815366561225)) ;
#47923=CARTESIAN_POINT('Ctrl Pts',(-20.2503434108889,-37.6528137033259,
124.301519197252)) ;
#47924=CARTESIAN_POINT('Ctrl Pts',(-20.4606042546842,-37.472824622963,124.523953283866)) ;
#47925=CARTESIAN_POINT('Ctrl Pts',(-20.503477443757,-37.6727690154578,123.96110057976)) ;
#47926=CARTESIAN_POINT('Ctrl Pts',(-20.7770251297192,-37.4927799350949,
124.098432867934)) ;
#47927=CARTESIAN_POINT('Ctrl Pts',(-20.6250594607957,-37.6926433720656,
123.556310778876)) ;
#47928=CARTESIAN_POINT('Ctrl Pts',(-20.9290068708027,-37.5126542917027,
123.592447664143)) ;
#47929=CARTESIAN_POINT('Ctrl Pts',(-20.60136228044,-37.7126255789266,123.132144136794)) ;
#47930=CARTESIAN_POINT('Ctrl Pts',(-20.8993899561854,-37.5326364985638,
123.062239130214)) ;
#47931=CARTESIAN_POINT('Ctrl Pts',(-20.4345064783654,-37.7325566568766,
122.742488170039)) ;
#47932=CARTESIAN_POINT('Ctrl Pts',(-20.690825481049,-37.5525675765137,122.575167631245)) ;
#47933=CARTESIAN_POINT('Ctrl Pts',(-20.1449218342173,-37.7524836317316,
122.433312486334)) ;
#47934=CARTESIAN_POINT('Ctrl Pts',(-20.3288457045334,-37.5724945513687,
122.188694790906)) ;
#47935=CARTESIAN_POINT('Ctrl Pts',(-19.769249258697,-37.7723160906805,122.241620195832)) ;
#47936=CARTESIAN_POINT('Ctrl Pts',(-19.8592684233419,-37.5923270103176,
121.94907564169)) ;
#47937=CARTESIAN_POINT('Ctrl Pts',(-19.417912839103,-37.7889737748557,122.197692406398)) ;
#47938=CARTESIAN_POINT('Ctrl Pts',(-19.4200658004663,-37.6089846944928,
121.894159881209)) ;
#47939=CARTESIAN_POINT('Ctrl Pts',(-19.1419000183344,-37.8022229987628,
122.235811998342)) ;
#47940=CARTESIAN_POINT('Ctrl Pts',(-19.0750788995633,-37.6222339183999,
121.941806794377)) ;
#47941=CARTESIAN_POINT('Ctrl Pts',(-18.9408249504578,-37.812272020214,122.300516733024)) ;
#47942=CARTESIAN_POINT('Ctrl Pts',(-18.8237258577179,-37.6322829398511,
122.022687580734)) ;
#47943=CARTESIAN_POINT('Ctrl Pts',(-18.75748940626,-37.8221320284445,122.39727315745)) ;
#47944=CARTESIAN_POINT('Ctrl Pts',(-18.5945663208798,-37.6421429480816,
122.143620577139)) ;
#47945=CARTESIAN_POINT('Ctrl Pts',(-18.5363454819024,-37.8354155416691,
122.567770253279)) ;
#47946=CARTESIAN_POINT('Ctrl Pts',(-18.318087679396,-37.6554264613062,122.356789242169)) ;
#47947=CARTESIAN_POINT('Ctrl Pts',(-18.3218393831635,-37.8520614606699,
122.849331128677)) ;
#47948=CARTESIAN_POINT('Ctrl Pts',(-18.0500066419728,-37.672072380307,122.708670183428)) ;
#47949=CARTESIAN_POINT('Ctrl Pts',(-18.2164325706239,-37.868615438486,123.185138476082)) ;
#47950=CARTESIAN_POINT('Ctrl Pts',(-17.9182173116251,-37.6886263581231,
123.1284860917)) ;
#47951=CARTESIAN_POINT('Ctrl Pts',(-18.2044905733032,-37.8819751674576,
123.465776368873)) ;
#47952=CARTESIAN_POINT('Ctrl Pts',(-17.9032980831102,-37.7019860870947,
123.479244069035)) ;
#47953=CARTESIAN_POINT('Ctrl Pts',(-18.2317111895261,-37.8918682192543,
123.671978883509)) ;
#47954=CARTESIAN_POINT('Ctrl Pts',(-17.9373186787806,-37.7118791388914,
123.737005381468)) ;
#47955=CARTESIAN_POINT('Ctrl Pts',(-18.294652658177,-37.9018581845353,123.87232240774)) ;
#47956=CARTESIAN_POINT('Ctrl Pts',(-18.0159935017335,-37.7218691041725,
123.987433562175)) ;
#47957=CARTESIAN_POINT('Ctrl Pts',(-18.3909713233348,-37.9118100653962,
124.058088930702)) ;
#47958=CARTESIAN_POINT('Ctrl Pts',(-18.1363891804887,-37.7318209850333,
124.219643590471)) ;
#47959=CARTESIAN_POINT('Ctrl Pts',(-18.5194225453027,-37.921858417088,124.225768775159)) ;
#47960=CARTESIAN_POINT('Ctrl Pts',(-18.2969510924967,-37.7418693367251,
124.42924502608)) ;
#47961=CARTESIAN_POINT('Ctrl Pts',(-18.671696215703,-37.9316997011942,124.365864629888)) ;
#47962=CARTESIAN_POINT('Ctrl Pts',(-18.4872912316246,-37.7517106208313,
124.60436691775)) ;
#47963=CARTESIAN_POINT('Ctrl Pts',(-18.8482704727161,-37.9416864043198,
124.479380726251)) ;
#47964=CARTESIAN_POINT('Ctrl Pts',(-18.7080075972399,-37.761697323957,124.746264446467)) ;
#47965=CARTESIAN_POINT('Ctrl Pts',(-19.0408922738897,-37.9516214331373,
124.560242685434)) ;
#47966=CARTESIAN_POINT('Ctrl Pts',(-18.9487838243805,-37.7716323527744,
124.847344520004)) ;
#47967=CARTESIAN_POINT('Ctrl Pts',(-19.2470723983466,-37.9616772280442,
124.606804319472)) ;
#47968=CARTESIAN_POINT('Ctrl Pts',(-19.2065084133453,-37.7816881476813,
124.905549326523)) ;
#47969=CARTESIAN_POINT('Ctrl Pts',(-19.4534751390395,-37.9715055913335,
124.616954335681)) ;
#47970=CARTESIAN_POINT('Ctrl Pts',(-19.4645118314012,-37.7915165109706,
124.918239663582)) ;
#47971=CARTESIAN_POINT('Ctrl Pts',(-19.6633369830596,-37.9815665612314,
124.590805337205)) ;
#47972=CARTESIAN_POINT('Ctrl Pts',(-19.7268395348764,-37.8015774808685,
124.885556198697)) ;
#47973=CARTESIAN_POINT('Ctrl Pts',(-19.8625213753835,-37.9914808401212,
124.529341700821)) ;
#47974=CARTESIAN_POINT('Ctrl Pts',(-19.975820977289,-37.8114917597583,124.808729302256)) ;
#47975=CARTESIAN_POINT('Ctrl Pts',(-20.0499508132267,-38.0014898345894,
124.433695820454)) ;
#47976=CARTESIAN_POINT('Ctrl Pts',(-20.2101091148539,-37.8215007542265,
124.689174409311)) ;
#47977=CARTESIAN_POINT('Ctrl Pts',(-20.2180109913369,-38.0115196691532,
124.306354445413)) ;
#47978=CARTESIAN_POINT('Ctrl Pts',(-20.4201860704738,-37.8315305887903,
124.529999912084)) ;
#47979=CARTESIAN_POINT('Ctrl Pts',(-20.3592543198836,-38.0213778992254,
124.154667140303)) ;
#47980=CARTESIAN_POINT('Ctrl Pts',(-20.596742436033,-37.8413888188625,124.340392518913)) ;
#47981=CARTESIAN_POINT('Ctrl Pts',(-20.4738072405077,-38.0313766049678,
123.978459990424)) ;
#47982=CARTESIAN_POINT('Ctrl Pts',(-20.7399359738029,-37.8513875246049,
124.120135025723)) ;
#47983=CARTESIAN_POINT('Ctrl Pts',(-20.5554252299828,-38.0412712608866,
123.787082603069)) ;
#47984=CARTESIAN_POINT('Ctrl Pts',(-20.8419611023496,-37.8612821805237,
123.880914135963)) ;
#47985=CARTESIAN_POINT('Ctrl Pts',(-20.6032952967785,-38.0513343252705,
123.581049295425)) ;
#47986=CARTESIAN_POINT('Ctrl Pts',(-20.9018013798977,-37.8713452449077,
123.62337316206)) ;
#47987=CARTESIAN_POINT('Ctrl Pts',(-20.6146442268699,-38.0611739835504,
123.374466194036)) ;
#47988=CARTESIAN_POINT('Ctrl Pts',(-20.9159903077687,-37.8811849031876,
123.365144028715)) ;
#47989=CARTESIAN_POINT('Ctrl Pts',(-20.5896648476914,-38.0712371506323,
123.164415788226)) ;
#47990=CARTESIAN_POINT('Ctrl Pts',(-20.8847687942713,-37.8912480702694,
123.102580743054)) ;
#47991=CARTESIAN_POINT('Ctrl Pts',(-20.5294350178213,-38.0811313957594,
122.965294396189)) ;
#47992=CARTESIAN_POINT('Ctrl Pts',(-20.809484036126,-37.9011423153965,122.853677895888)) ;
#47993=CARTESIAN_POINT('Ctrl Pts',(-20.4356240821456,-38.091073217364,122.778550856413)) ;
#47994=CARTESIAN_POINT('Ctrl Pts',(-20.6922226402162,-37.9110841370011,
122.620247034589)) ;
#47995=CARTESIAN_POINT('Ctrl Pts',(-20.3100810134852,-38.1010757482821,
122.609819097008)) ;
#47996=CARTESIAN_POINT('Ctrl Pts',(-20.5352958890887,-37.9210866679192,
122.40933067988)) ;
#47997=CARTESIAN_POINT('Ctrl Pts',(-20.1564607952852,-38.1111103747396,
122.465250449914)) ;
#47998=CARTESIAN_POINT('Ctrl Pts',(-20.3432724835516,-37.9311212943767,
122.228617908719)) ;
#47999=CARTESIAN_POINT('Ctrl Pts',(-19.9835623722376,-38.120955909726,122.351445881566)) ;
#48000=CARTESIAN_POINT('Ctrl Pts',(-20.1271504515569,-37.9409668293631,
122.086359667686)) ;
#48001=CARTESIAN_POINT('Ctrl Pts',(-19.7910718790852,-38.130939334565,122.267833463766)) ;
#48002=CARTESIAN_POINT('Ctrl Pts',(-19.8865382083941,-37.9509502542022,
121.981841696408)) ;
#48003=CARTESIAN_POINT('Ctrl Pts',(-19.5876306579575,-38.1408897249301,
122.219111287809)) ;
#48004=CARTESIAN_POINT('Ctrl Pts',(-19.6322370248592,-37.9609006445672,
121.920936388949)) ;
#48005=CARTESIAN_POINT('Ctrl Pts',(-19.377833549305,-38.1508873652272,122.206109169437)) ;
#48006=CARTESIAN_POINT('Ctrl Pts',(-19.3699906918077,-37.9708982848643,
121.904681189327)) ;
#48007=CARTESIAN_POINT('Ctrl Pts',(-19.1681777198956,-38.1609264457904,
122.230248686122)) ;
#48008=CARTESIAN_POINT('Ctrl Pts',(-19.1079206636273,-37.9809373654275,
121.934852971173)) ;
#48009=CARTESIAN_POINT('Ctrl Pts',(-18.9700348987054,-38.1707525965595,
122.288711476729)) ;
#48010=CARTESIAN_POINT('Ctrl Pts',(-18.860240682653,-37.9907635161966,122.007929238581)) ;
#48011=CARTESIAN_POINT('Ctrl Pts',(-18.7805861370791,-38.1808091714886,
122.382535043644)) ;
#48012=CARTESIAN_POINT('Ctrl Pts',(-18.6234287247367,-38.0008200911257,
122.125206427547)) ;
#48013=CARTESIAN_POINT('Ctrl Pts',(-18.6124721251259,-38.1907497108689,
122.506687338433)) ;
#48014=CARTESIAN_POINT('Ctrl Pts',(-18.4132844279037,-38.010760630506,122.280394942276)) ;
#48015=CARTESIAN_POINT('Ctrl Pts',(-18.4685228176919,-38.2006541038453,
122.657141441856)) ;
#48016=CARTESIAN_POINT('Ctrl Pts',(-18.2333456791287,-38.0206650234824,
122.468461282899)) ;
#48017=CARTESIAN_POINT('Ctrl Pts',(-18.3513466171436,-38.2107007580502,
122.832848241972)) ;
#48018=CARTESIAN_POINT('Ctrl Pts',(-18.0868734496572,-38.0307116776873,
122.68809334047)) ;
#48019=CARTESIAN_POINT('Ctrl Pts',(-18.2675409912502,-38.2205963199886,
123.023293670157)) ;
#48020=CARTESIAN_POINT('Ctrl Pts',(-17.9821139835232,-38.0406072396257,
122.926149688474)) ;
#48021=CARTESIAN_POINT('Ctrl Pts',(-18.2172590198728,-38.2306583978341,
123.228736388666)) ;
#48022=CARTESIAN_POINT('Ctrl Pts',(-17.9192592235961,-38.0506693174713,
123.182952338498)) ;
#48023=CARTESIAN_POINT('Ctrl Pts',(-18.203592355486,-38.2405010962479,123.435232302293)) ;
#48024=CARTESIAN_POINT('Ctrl Pts',(-17.9021734628791,-38.060512015885,123.441072933946)) ;
#48025=CARTESIAN_POINT('Ctrl Pts',(-18.2258256609928,-38.2504918712094,
123.644062640654)) ;
#48026=CARTESIAN_POINT('Ctrl Pts',(-17.9299628607559,-38.0705027908465,
123.702111270586)) ;
#48027=CARTESIAN_POINT('Ctrl Pts',(-18.2836555871143,-38.2604197362285,
123.844617912795)) ;
#48028=CARTESIAN_POINT('Ctrl Pts',(-18.0022482230094,-38.0804306558656,
123.952806457239)) ;
#48029=CARTESIAN_POINT('Ctrl Pts',(-18.3756740561465,-38.2704084809947,
124.033382785649)) ;
#48030=CARTESIAN_POINT('Ctrl Pts',(-18.1172694269985,-38.0904194006318,
124.188763665487)) ;
#48031=CARTESIAN_POINT('Ctrl Pts',(-18.4998651142318,-38.2804412665816,
124.203869104548)) ;
#48032=CARTESIAN_POINT('Ctrl Pts',(-18.2725063779841,-38.1004521862187,
124.401872836885)) ;
#48033=CARTESIAN_POINT('Ctrl Pts',(-18.649102754769,-38.2903079512023,124.347923475099)) ;
#48034=CARTESIAN_POINT('Ctrl Pts',(-18.4590525160662,-38.1103188708394,
124.581942987114)) ;
#48035=CARTESIAN_POINT('Ctrl Pts',(-18.8224168744023,-38.3002698433654,
124.465501995061)) ;
#48036=CARTESIAN_POINT('Ctrl Pts',(-18.6756943059788,-38.1202807630025,
124.728918023254)) ;
#48037=CARTESIAN_POINT('Ctrl Pts',(-19.0150124373623,-38.310303320278,124.551507630539)) ;
#48038=CARTESIAN_POINT('Ctrl Pts',(-18.9164378070942,-38.1303142399151,
124.836426983259)) ;
#48039=CARTESIAN_POINT('Ctrl Pts',(-19.2165276853303,-38.3201876615263,
124.602331746933)) ;
#48040=CARTESIAN_POINT('Ctrl Pts',(-19.1683321359747,-38.1401985811634,
124.899959302381)) ;
#48041=CARTESIAN_POINT('Ctrl Pts',(-19.4274995678866,-38.3302506036474,
124.617665373522)) ;
#48042=CARTESIAN_POINT('Ctrl Pts',(-19.4320465863447,-38.1502615232845,
124.919128358715)) ;
#48043=CARTESIAN_POINT('Ctrl Pts',(-19.6335365424027,-38.340101005267,124.596684953135)) ;
#48044=CARTESIAN_POINT('Ctrl Pts',(-19.6895940464433,-38.1601119249041,
124.892904733968)) ;
#48045=CARTESIAN_POINT('Ctrl Pts',(-19.8364952866382,-38.3501278940566,
124.539756466439)) ;
#48046=CARTESIAN_POINT('Ctrl Pts',(-19.9432929414163,-38.1701388136938,
124.821745925476)) ;
#48047=CARTESIAN_POINT('Ctrl Pts',(-20.0262936192823,-38.3601565090128,
124.447932183891)) ;
#48048=CARTESIAN_POINT('Ctrl Pts',(-20.1805416769707,-38.18016742865,124.706967424635)) ;
#48049=CARTESIAN_POINT('Ctrl Pts',(-20.1943496803359,-38.3700017321329,
124.327134832878)) ;
#48050=CARTESIAN_POINT('Ctrl Pts',(-20.3906137720793,-38.19001265177,124.555971632204)) ;
#48051=CARTESIAN_POINT('Ctrl Pts',(-20.3414292534082,-38.3799924159389,
124.17718516851)) ;
#48052=CARTESIAN_POINT('Ctrl Pts',(-20.574464611682,-38.200003335576,124.368535624673)) ;
#48053=CARTESIAN_POINT('Ctrl Pts',(-20.4604073331127,-38.3900302980113,
124.002897673385)) ;
#48054=CARTESIAN_POINT('Ctrl Pts',(-20.7231886883335,-38.2100412176484,
124.1506774248)) ;
#48055=CARTESIAN_POINT('Ctrl Pts',(-20.5459739903831,-38.3998746576501,
123.814446734929)) ;
#48056=CARTESIAN_POINT('Ctrl Pts',(-20.8301490996899,-38.2198855772873,
123.915113415464)) ;
#48057=CARTESIAN_POINT('Ctrl Pts',(-20.5986469705977,-38.4098595282649,
123.611278948678)) ;
#48058=CARTESIAN_POINT('Ctrl Pts',(-20.8959919668574,-38.229870447902,123.661153850813)) ;
#48059=CARTESIAN_POINT('Ctrl Pts',(-20.6152674854277,-38.4197988115935,
123.402955218507)) ;
#48060=CARTESIAN_POINT('Ctrl Pts',(-20.9167692456538,-38.2398097312307,
123.400748772405)) ;
#48061=CARTESIAN_POINT('Ctrl Pts',(-20.5952009161257,-38.4298394209667,
123.192847662507)) ;
#48062=CARTESIAN_POINT('Ctrl Pts',(-20.8916876625912,-38.2498503406038,
123.138114322854)) ;
#48063=CARTESIAN_POINT('Ctrl Pts',(-20.5399668125986,-38.4397242718799,
122.992486933)) ;
#48064=CARTESIAN_POINT('Ctrl Pts',(-20.8226462971584,-38.259735191517,122.887662089246)) ;
#48065=CARTESIAN_POINT('Ctrl Pts',(-20.4499783459561,-38.4497262280487,
122.802478082637)) ;
#48066=CARTESIAN_POINT('Ctrl Pts',(-20.710161993773,-38.2697371476858,122.650150261944)) ;
#48067=CARTESIAN_POINT('Ctrl Pts',(-20.3294778320045,-38.4596448247692,
122.632260562364)) ;
#48068=CARTESIAN_POINT('Ctrl Pts',(-20.5595370994859,-38.2796557444063,
122.437376954978)) ;
#48069=CARTESIAN_POINT('Ctrl Pts',(-20.1793517400514,-38.469691646845,122.483728376265)) ;
#48070=CARTESIAN_POINT('Ctrl Pts',(-20.3718806509748,-38.2897025664821,
122.251710845181)) ;
#48071=CARTESIAN_POINT('Ctrl Pts',(-20.0087562410276,-38.4795659279577,
122.365386621562)) ;
#48072=CARTESIAN_POINT('Ctrl Pts',(-20.1586361996875,-38.2995768475948,
122.103781930093)) ;
#48073=CARTESIAN_POINT('Ctrl Pts',(-19.8168874460983,-38.4896201280023,
122.27679388918)) ;
#48074=CARTESIAN_POINT('Ctrl Pts',(-19.9188009996355,-38.3096310476394,
121.993039914093)) ;
#48075=CARTESIAN_POINT('Ctrl Pts',(-19.6157267682506,-38.4995155576375,
122.223611335087)) ;
#48076=CARTESIAN_POINT('Ctrl Pts',(-19.6673495935004,-38.3195264772746,
121.926560229075)) ;
#48077=CARTESIAN_POINT('Ctrl Pts',(-19.4049744065646,-38.5095771859549,
122.2058271605)) ;
#48078=CARTESIAN_POINT('Ctrl Pts',(-19.403909575533,-38.329588105592,121.904328761475)) ;
#48079=CARTESIAN_POINT('Ctrl Pts',(-19.198843636696,-38.5194218147848,122.224471407226)) ;
#48080=CARTESIAN_POINT('Ctrl Pts',(-19.1462446840125,-38.3394327344219,
121.927632920062)) ;
#48081=CARTESIAN_POINT('Ctrl Pts',(-18.9965533130945,-38.5293818623904,
122.278528162173)) ;
#48082=CARTESIAN_POINT('Ctrl Pts',(-18.8933810810859,-38.3493927820275,
121.99520301882)) ;
#48083=CARTESIAN_POINT('Ctrl Pts',(-18.8054118271966,-38.5394201685644,
122.367955384898)) ;
#48084=CARTESIAN_POINT('Ctrl Pts',(-18.6544538829586,-38.3594310882016,
122.106985936773)) ;
#48085=CARTESIAN_POINT('Ctrl Pts',(-18.63527681131,-38.5492934679971,122.48691582821)) ;
#48086=CARTESIAN_POINT('Ctrl Pts',(-18.4417836193016,-38.3693043876342,
122.255686315727)) ;
#48087=CARTESIAN_POINT('Ctrl Pts',(-18.4855083632064,-38.5593667295834,
122.636576989724)) ;
#48088=CARTESIAN_POINT('Ctrl Pts',(-18.254572634365,-38.3793776492205,122.442761738888)) ;
#48089=CARTESIAN_POINT('Ctrl Pts',(-18.3667777956026,-38.5691869555401,
122.805528697943)) ;
#48090=CARTESIAN_POINT('Ctrl Pts',(-18.1061577776451,-38.3891978751772,
122.653952116024)) ;
#48091=CARTESIAN_POINT('Ctrl Pts',(-18.2767515118799,-38.5792660194796,
122.997287213327)) ;
#48092=CARTESIAN_POINT('Ctrl Pts',(-17.9936243510384,-38.3992769391167,
122.893649468812)) ;
#48093=CARTESIAN_POINT('Ctrl Pts',(-18.2225229813274,-38.5891161094994,
123.197198324746)) ;
#48094=CARTESIAN_POINT('Ctrl Pts',(-17.9258375544917,-38.4091270291365,
123.143539427592)) ;
#48095=CARTESIAN_POINT('Ctrl Pts',(-18.2032956686347,-38.5991948631132,
123.408157950958)) ;
#48096=CARTESIAN_POINT('Ctrl Pts',(-17.9018026838566,-38.4192057827503,
123.40723841002)) ;
#48097=CARTESIAN_POINT('Ctrl Pts',(-18.2203875577578,-38.6090163303726,
123.613973329019)) ;
#48098=CARTESIAN_POINT('Ctrl Pts',(-17.923166969544,-38.4290272500098,123.664509279081)) ;
#48099=CARTESIAN_POINT('Ctrl Pts',(-18.2739238887591,-38.6190819287303,
123.818650277656)) ;
#48100=CARTESIAN_POINT('Ctrl Pts',(-17.9900867207186,-38.4390928483674,
123.920355248471)) ;
#48101=CARTESIAN_POINT('Ctrl Pts',(-18.3608489444241,-38.628984584505,124.007876019705)) ;
#48102=CARTESIAN_POINT('Ctrl Pts',(-18.0987428644432,-38.4489955041421,
124.156888509072)) ;
#48103=CARTESIAN_POINT('Ctrl Pts',(-18.4809742235416,-38.6390354103346,
124.181656276088)) ;
#48104=CARTESIAN_POINT('Ctrl Pts',(-18.2488988281451,-38.4590463299717,
124.374113939604)) ;
#48105=CARTESIAN_POINT('Ctrl Pts',(-18.6267574232004,-38.6489096146735,
124.329501799845)) ;
#48106=CARTESIAN_POINT('Ctrl Pts',(-18.4311282813033,-38.4689205343106,
124.558922029202)) ;
#48107=CARTESIAN_POINT('Ctrl Pts',(-18.7993133903288,-38.6589820647126,
124.452162400167)) ;
#48108=CARTESIAN_POINT('Ctrl Pts',(-18.6468226000741,-38.4789929843497,
124.712247945028)) ;
#48109=CARTESIAN_POINT('Ctrl Pts',(-18.9859137942603,-38.6688110814861,
124.541017706794)) ;
#48110=CARTESIAN_POINT('Ctrl Pts',(-18.8800743167778,-38.4888220011232,
124.823318123614)) ;
#48111=CARTESIAN_POINT('Ctrl Pts',(-19.1897774494704,-38.6788779274009,
124.597717051206)) ;
#48112=CARTESIAN_POINT('Ctrl Pts',(-19.1349034186575,-38.498888847038,124.894192497804)) ;
#48113=CARTESIAN_POINT('Ctrl Pts',(-19.3967662896624,-38.6887680987027,
124.617671141115)) ;
#48114=CARTESIAN_POINT('Ctrl Pts',(-19.3936404772055,-38.5087790183398,
124.919135574597)) ;
#48115=CARTESIAN_POINT('Ctrl Pts',(-19.6062117856198,-38.6987602923265,
124.601677520649)) ;
#48116=CARTESIAN_POINT('Ctrl Pts',(-19.6554475745632,-38.5187712119636,
124.899143715405)) ;
#48117=CARTESIAN_POINT('Ctrl Pts',(-19.8090578521169,-38.7087231029499,
124.549518835879)) ;
#48118=CARTESIAN_POINT('Ctrl Pts',(-19.9090056650285,-38.5287340225871,
124.833945501294)) ;
#48119=CARTESIAN_POINT('Ctrl Pts',(-19.9988839578665,-38.7186273757934,
124.463912950195)) ;
#48120=CARTESIAN_POINT('Ctrl Pts',(-20.1462891748571,-38.5386382954305,
124.726937805208)) ;
#48121=CARTESIAN_POINT('Ctrl Pts',(-20.1735373576463,-38.728687867598,124.344670095455)) ;
#48122=CARTESIAN_POINT('Ctrl Pts',(-20.3646057034677,-38.5486987872351,
124.577884540204)) ;
#48123=CARTESIAN_POINT('Ctrl Pts',(-20.3217496628908,-38.7385281992703,
124.200302181168)) ;
#48124=CARTESIAN_POINT('Ctrl Pts',(-20.549872151261,-38.5585391189074,124.397423633048)) ;
#48125=CARTESIAN_POINT('Ctrl Pts',(-20.4455536404309,-38.7485912453621,
124.028786981094)) ;
#48126=CARTESIAN_POINT('Ctrl Pts',(-20.7046268368384,-38.5686021649992,
124.183029887266)) ;
#48127=CARTESIAN_POINT('Ctrl Pts',(-20.5360148595755,-38.7584853010572,
123.841460701052)) ;
#48128=CARTESIAN_POINT('Ctrl Pts',(-20.8177037943771,-38.5784962206943,
123.948871113631)) ;
#48129=CARTESIAN_POINT('Ctrl Pts',(-20.5933924658413,-38.7684280013801,
123.640487605806)) ;
#48130=CARTESIAN_POINT('Ctrl Pts',(-20.889425745872,-38.5884389210173,123.697654055537)) ;
#48131=CARTESIAN_POINT('Ctrl Pts',(-20.6151860212168,-38.7784337423077,
123.431245299403)) ;
#48132=CARTESIAN_POINT('Ctrl Pts',(-20.9166674415414,-38.5984446619449,
123.436101061356)) ;
#48133=CARTESIAN_POINT('Ctrl Pts',(-20.6000592508299,-38.7884546528233,
123.221122882198)) ;
#48134=CARTESIAN_POINT('Ctrl Pts',(-20.8977588227754,-38.6084655724604,
123.173448091062)) ;
#48135=CARTESIAN_POINT('Ctrl Pts',(-20.5495758365941,-38.7983453882732,
123.0194036364)) ;
#48136=CARTESIAN_POINT('Ctrl Pts',(-20.8346540510326,-38.6183563079104,
122.921298084122)) ;
#48137=CARTESIAN_POINT('Ctrl Pts',(-20.4642602817029,-38.8083369290021,
122.827465431094)) ;
#48138=CARTESIAN_POINT('Ctrl Pts',(-20.7280091756525,-38.6283478486392,
122.68137528438)) ;
#48139=CARTESIAN_POINT('Ctrl Pts',(-20.3473737278901,-38.8182847894237,
122.654045824063)) ;
#48140=CARTESIAN_POINT('Ctrl Pts',(-20.5819003598894,-38.6382957090609,
122.46460048107)) ;
#48141=CARTESIAN_POINT('Ctrl Pts',(-20.202456742999,-38.8282314586101,122.503277801019)) ;
#48142=CARTESIAN_POINT('Ctrl Pts',(-20.400753356158,-38.6482423782472,122.276140396852)) ;
#48143=CARTESIAN_POINT('Ctrl Pts',(-20.0317199746376,-38.8382795347457,
122.378903058221)) ;
#48144=CARTESIAN_POINT('Ctrl Pts',(-20.1873323482229,-38.6582904543828,
122.12067245961)) ;
#48145=CARTESIAN_POINT('Ctrl Pts',(-19.8458354362141,-38.8481271327513,
122.287756233757)) ;
#48146=CARTESIAN_POINT('Ctrl Pts',(-19.9549752001431,-38.6681380523884,
122.006738756206)) ;
#48147=CARTESIAN_POINT('Ctrl Pts',(-19.6448376579705,-38.8580888558358,
122.228975330459)) ;
#48148=CARTESIAN_POINT('Ctrl Pts',(-19.703727329421,-38.6780997754729,121.933263220706)) ;
#48149=CARTESIAN_POINT('Ctrl Pts',(-19.4352361415482,-38.8681174909188,
122.206096194231)) ;
#48150=CARTESIAN_POINT('Ctrl Pts',(-19.4417254602095,-38.6881284105559,
121.904664952716)) ;
#48151=CARTESIAN_POINT('Ctrl Pts',(-19.2273465752442,-38.8780277992368,
122.219725256983)) ;
#48152=CARTESIAN_POINT('Ctrl Pts',(-19.181862671313,-38.6980387188739,121.921702009282)) ;
#48153=CARTESIAN_POINT('Ctrl Pts',(-19.0243342885466,-38.8879626963727,
122.26883883605)) ;
#48154=CARTESIAN_POINT('Ctrl Pts',(-18.9280968782032,-38.7079736160098,
121.98309499747)) ;
#48155=CARTESIAN_POINT('Ctrl Pts',(-18.8309772013695,-38.8980037793153,
122.353523961238)) ;
#48156=CARTESIAN_POINT('Ctrl Pts',(-18.6864010149185,-38.7180146989524,
122.088952068271)) ;
#48157=CARTESIAN_POINT('Ctrl Pts',(-18.6578590680997,-38.9078911221435,
122.468595150492)) ;
#48158=CARTESIAN_POINT('Ctrl Pts',(-18.4700029594323,-38.7279020417806,
122.232792348805)) ;
#48159=CARTESIAN_POINT('Ctrl Pts',(-18.5055317513843,-38.9178826370828,
122.613211351364)) ;
#48160=CARTESIAN_POINT('Ctrl Pts',(-18.2795943518185,-38.73789355672,122.413563464237)) ;
#48161=CARTESIAN_POINT('Ctrl Pts',(-18.3811911630624,-38.9278340282793,
122.781466926608)) ;
#48162=CARTESIAN_POINT('Ctrl Pts',(-18.1241690742749,-38.7478449479164,
122.623883939098)) ;
#48163=CARTESIAN_POINT('Ctrl Pts',(-18.2878097045155,-38.9377665616119,
122.968234846333)) ;
#48164=CARTESIAN_POINT('Ctrl Pts',(-18.0074429397806,-38.7577774812491,
122.857344924824)) ;
#48165=CARTESIAN_POINT('Ctrl Pts',(-18.2278106534503,-38.9477637195114,
123.1696520482)) ;
#48166=CARTESIAN_POINT('Ctrl Pts',(-17.9324451631841,-38.7677746391485,
123.109116894518)) ;
#48167=CARTESIAN_POINT('Ctrl Pts',(-18.2036416355779,-38.9577487296749,
123.378205341425)) ;
#48168=CARTESIAN_POINT('Ctrl Pts',(-17.9022350151,-38.777759649312,123.369808873099)) ;
#48169=CARTESIAN_POINT('Ctrl Pts',(-18.2164291819651,-38.9677915562447,
123.588920968376)) ;
#48170=CARTESIAN_POINT('Ctrl Pts',(-17.918220476194,-38.7878024758818,123.633203162121)) ;
#48171=CARTESIAN_POINT('Ctrl Pts',(-18.2641206916243,-38.9776217905496,
123.790038485593)) ;
#48172=CARTESIAN_POINT('Ctrl Pts',(-17.9778363800637,-38.7976327101868,
123.884601181613)) ;
#48173=CARTESIAN_POINT('Ctrl Pts',(-18.3479385843405,-38.9876978157843,
123.984532944223)) ;
#48174=CARTESIAN_POINT('Ctrl Pts',(-18.0826097273411,-38.8077087354214,
124.127718361036)) ;
#48175=CARTESIAN_POINT('Ctrl Pts',(-18.4616277736015,-38.9975500522752,
124.157720560445)) ;
#48176=CARTESIAN_POINT('Ctrl Pts',(-18.22472296995,-38.8175609719123,124.344203206639)) ;
#48177=CARTESIAN_POINT('Ctrl Pts',(-18.6066621317061,-39.0076232587093,
124.31198450881)) ;
#48178=CARTESIAN_POINT('Ctrl Pts',(-18.4060166292549,-38.8276341783464,
124.537031920896)) ;
#48179=CARTESIAN_POINT('Ctrl Pts',(-18.7724492303032,-39.0174647682165,
124.435789163625)) ;
#48180=CARTESIAN_POINT('Ctrl Pts',(-18.6132523458117,-38.8374756878536,
124.691787453132)) ;
#48181=CARTESIAN_POINT('Ctrl Pts',(-18.9590824114606,-39.0274257149963,
124.530751648875)) ;
#48182=CARTESIAN_POINT('Ctrl Pts',(-18.8465449135048,-38.8474366346334,
124.810489310294)) ;
#48183=CARTESIAN_POINT('Ctrl Pts',(-19.1610387527157,-39.0374635437963,
124.591933966622)) ;
#48184=CARTESIAN_POINT('Ctrl Pts',(-19.0989906357663,-38.8574744634334,
124.886965770252)) ;
#48185=CARTESIAN_POINT('Ctrl Pts',(-19.3671221533313,-39.0473378535508,
124.617096782991)) ;
#48186=CARTESIAN_POINT('Ctrl Pts',(-19.3565960865171,-38.8673487731879,
124.918417832295)) ;
#48187=CARTESIAN_POINT('Ctrl Pts',(-19.5784931233021,-39.0574075512239,
124.605867995762)) ;
#48188=CARTESIAN_POINT('Ctrl Pts',(-19.620809364879,-38.8774184708611,124.90438027923)) ;
#48189=CARTESIAN_POINT('Ctrl Pts',(-19.7799321898415,-39.0672410225113,
124.55932535313)) ;
#48190=CARTESIAN_POINT('Ctrl Pts',(-19.8726090818737,-38.8872519421485,
124.846200103951)) ;
#48191=CARTESIAN_POINT('Ctrl Pts',(-19.9742453524244,-39.0772706690413,
124.477468158144)) ;
#48192=CARTESIAN_POINT('Ctrl Pts',(-20.1154997478902,-38.8972815886784,
124.743876964785)) ;
#48193=CARTESIAN_POINT('Ctrl Pts',(-20.1511369807371,-39.0873051833686,
124.36251502401)) ;
#48194=CARTESIAN_POINT('Ctrl Pts',(-20.336613329244,-38.9073161030058,124.600184240686)) ;
#48195=CARTESIAN_POINT('Ctrl Pts',(-20.3025021754356,-39.0971304688395,
124.221961302064)) ;
#48196=CARTESIAN_POINT('Ctrl Pts',(-20.525819561072,-38.9171413884767,124.424489904963)) ;
#48197=CARTESIAN_POINT('Ctrl Pts',(-20.4297743163725,-39.1071347103881,
124.05455039433)) ;
#48198=CARTESIAN_POINT('Ctrl Pts',(-20.684908264894,-38.9271456300252,124.215225042705)) ;
#48199=CARTESIAN_POINT('Ctrl Pts',(-20.5257881932866,-39.1171173554672,
123.867889590297)) ;
#48200=CARTESIAN_POINT('Ctrl Pts',(-20.8049240326916,-38.9371282751043,
123.981897983475)) ;
#48201=CARTESIAN_POINT('Ctrl Pts',(-20.588074926157,-39.1271625525587,123.666125982417)) ;
#48202=CARTESIAN_POINT('Ctrl Pts',(-20.8827806719574,-38.9471734721958,
123.729693087427)) ;
#48203=CARTESIAN_POINT('Ctrl Pts',(-20.6141505417572,-39.1369856683188,
123.461258677549)) ;
#48204=CARTESIAN_POINT('Ctrl Pts',(-20.915373446422,-38.9569965879559,123.473607472964)) ;
#48205=CARTESIAN_POINT('Ctrl Pts',(-20.60457754197,-39.1470202801191,123.250519610856)) ;
#48206=CARTESIAN_POINT('Ctrl Pts',(-20.9034051256726,-38.9670311997562,
123.210183840102)) ;
#48207=CARTESIAN_POINT('Ctrl Pts',(-20.5580262468952,-39.1570452888922,
123.044960994217)) ;
#48208=CARTESIAN_POINT('Ctrl Pts',(-20.8452141569218,-38.9770562085294,
122.953236014192)) ;
#48209=CARTESIAN_POINT('Ctrl Pts',(-20.478316885892,-39.1668972137338,122.853791086259)) ;
#48210=CARTESIAN_POINT('Ctrl Pts',(-20.7455751866615,-38.9869081333709,
122.714273478739)) ;
#48211=CARTESIAN_POINT('Ctrl Pts',(-20.3653360181163,-39.1768881520565,
122.676754747224)) ;
#48212=CARTESIAN_POINT('Ctrl Pts',(-20.6043472152323,-38.9968990716936,
122.492979055733)) ;
#48213=CARTESIAN_POINT('Ctrl Pts',(-20.2244345622947,-39.186806137203,122.523026316099)) ;
#48214=CARTESIAN_POINT('Ctrl Pts',(-20.4282184151075,-39.0068170568401,
122.300819554238)) ;
#48215=CARTESIAN_POINT('Ctrl Pts',(-20.0572079878956,-39.1968342380985,
122.394673439318)) ;
#48216=CARTESIAN_POINT('Ctrl Pts',(-20.2191838999621,-39.0168451577356,
122.140380206335)) ;
#48217=CARTESIAN_POINT('Ctrl Pts',(-19.8729210552735,-39.2067194790411,
122.298607224345)) ;
#48218=CARTESIAN_POINT('Ctrl Pts',(-19.988823563365,-39.0267303986782,122.020299045368)) ;
#48219=CARTESIAN_POINT('Ctrl Pts',(-19.6728247514948,-39.2167085920077,
122.234848345753)) ;
#48220=CARTESIAN_POINT('Ctrl Pts',(-19.7387023265392,-39.0367195116448,
121.940602617723)) ;
#48221=CARTESIAN_POINT('Ctrl Pts',(-19.4635439074029,-39.2267506563485,
122.207112896328)) ;
#48222=CARTESIAN_POINT('Ctrl Pts',(-19.477101074724,-39.0467615759856,121.905935512538)) ;
#48223=CARTESIAN_POINT('Ctrl Pts',(-19.2570678726038,-39.236579857753,122.215554269047)) ;
#48224=CARTESIAN_POINT('Ctrl Pts',(-19.2190051557775,-39.0565907773901,
121.91648957557)) ;
#48225=CARTESIAN_POINT('Ctrl Pts',(-19.0514789396674,-39.2465866985112,
122.260060325551)) ;
#48226=CARTESIAN_POINT('Ctrl Pts',(-18.96201942726,-39.0665976181483,121.972124528539)) ;
#48227=CARTESIAN_POINT('Ctrl Pts',(-18.857109213024,-39.2565742227031,122.33957226792)) ;
#48228=CARTESIAN_POINT('Ctrl Pts',(-18.7190580246925,-39.0765851423402,
122.071516726106)) ;
#48229=CARTESIAN_POINT('Ctrl Pts',(-18.6788723961599,-39.2666038685117,
122.452193066981)) ;
#48230=CARTESIAN_POINT('Ctrl Pts',(-18.4962632862226,-39.0866147881488,
122.21229469891)) ;
#48231=CARTESIAN_POINT('Ctrl Pts',(-18.5251202819395,-39.2764778992504,
122.591691852542)) ;
#48232=CARTESIAN_POINT('Ctrl Pts',(-18.3040742602747,-39.0964888188876,
122.386670421096)) ;
#48233=CARTESIAN_POINT('Ctrl Pts',(-18.3961396998256,-39.2864772221145,
122.757647081456)) ;
#48234=CARTESIAN_POINT('Ctrl Pts',(-18.142850412755,-39.1064881417517,122.594116058602)) ;
#48235=CARTESIAN_POINT('Ctrl Pts',(-18.2985886975645,-39.2963880576901,
122.941797700532)) ;
#48236=CARTESIAN_POINT('Ctrl Pts',(-18.0209136491181,-39.1163989773273,
122.824305926561)) ;
#48237=CARTESIAN_POINT('Ctrl Pts',(-18.2336609868071,-39.3064423056642,
123.142915425112)) ;
#48238=CARTESIAN_POINT('Ctrl Pts',(-17.939756418586,-39.1264532253013,123.075703741562)) ;
#48239=CARTESIAN_POINT('Ctrl Pts',(-18.2049530968866,-39.3163010499269,
123.348215710506)) ;
#48240=CARTESIAN_POINT('Ctrl Pts',(-17.9038739773889,-39.136311969564,123.332330097261)) ;
#48241=CARTESIAN_POINT('Ctrl Pts',(-18.2123561541688,-39.3263691359999,
123.559718460866)) ;
#48242=CARTESIAN_POINT('Ctrl Pts',(-17.9131303556298,-39.146380055637,123.596708290308)) ;
#48243=CARTESIAN_POINT('Ctrl Pts',(-18.2554666856692,-39.3362246191794,
123.762394729141)) ;
#48244=CARTESIAN_POINT('Ctrl Pts',(-17.9670211523186,-39.1562355388165,
123.850053708663)) ;
#48245=CARTESIAN_POINT('Ctrl Pts',(-18.333618279946,-39.3462194649736,123.957436253623)) ;
#48246=CARTESIAN_POINT('Ctrl Pts',(-18.0647131560755,-39.1662303846107,
124.093854715308)) ;
#48247=CARTESIAN_POINT('Ctrl Pts',(-18.4452442598356,-39.3562507606361,
124.136365747188)) ;
#48248=CARTESIAN_POINT('Ctrl Pts',(-18.2042478281487,-39.1762616802733,
124.31751521221)) ;
#48249=CARTESIAN_POINT('Ctrl Pts',(-18.5836826690354,-39.366117303926,124.290842760862)) ;
#48250=CARTESIAN_POINT('Ctrl Pts',(-18.3772981542013,-39.1861282235631,
124.510610102635)) ;
#48251=CARTESIAN_POINT('Ctrl Pts',(-18.748604585584,-39.3761046996894,124.420751361441)) ;
#48252=CARTESIAN_POINT('Ctrl Pts',(-18.5834523133935,-39.1961156193265,
124.672993813445)) ;
#48253=CARTESIAN_POINT('Ctrl Pts',(-18.9327894876098,-39.3860497404194,
124.519754705833)) ;
#48254=CARTESIAN_POINT('Ctrl Pts',(-18.8136849281219,-39.2060606600565,
124.796745724654)) ;
#48255=CARTESIAN_POINT('Ctrl Pts',(-19.1333404381493,-39.3960942466361,
124.585800268565)) ;
#48256=CARTESIAN_POINT('Ctrl Pts',(-19.0643744385041,-39.2161051662732,
124.879300115833)) ;
#48257=CARTESIAN_POINT('Ctrl Pts',(-19.3385607919778,-39.4059577527734,
124.615667658985)) ;
#48258=CARTESIAN_POINT('Ctrl Pts',(-19.3209006976939,-39.2259686724105,
124.916631731165)) ;
#48259=CARTESIAN_POINT('Ctrl Pts',(-19.5485278972259,-39.4159506136095,
124.609740631774)) ;
#48260=CARTESIAN_POINT('Ctrl Pts',(-19.5833595972504,-39.2359615332466,
124.909220187151)) ;
#48261=CARTESIAN_POINT('Ctrl Pts',(-19.7529825851974,-39.4258768073284,
124.567812438431)) ;
#48262=CARTESIAN_POINT('Ctrl Pts',(-19.838927622203,-39.2458877269655,124.856807196961)) ;
#48263=CARTESIAN_POINT('Ctrl Pts',(-19.9488284655848,-39.435895733361,124.490360997072)) ;
#48264=CARTESIAN_POINT('Ctrl Pts',(-20.0837340012441,-39.2559066529981,
124.759990302351)) ;
#48265=CARTESIAN_POINT('Ctrl Pts',(-20.126540851108,-39.4458107327286,124.381363000925)) ;
#48266=CARTESIAN_POINT('Ctrl Pts',(-20.3058732169499,-39.2658216523657,
124.623740322462)) ;
#48267=CARTESIAN_POINT('Ctrl Pts',(-20.2847556242028,-39.4558655042859,
124.241221421377)) ;
#48268=CARTESIAN_POINT('Ctrl Pts',(-20.5036398438425,-39.275876423923,124.448561261991)) ;
#48269=CARTESIAN_POINT('Ctrl Pts',(-20.4138101110339,-39.4657244665834,
124.079002697982)) ;
#48270=CARTESIAN_POINT('Ctrl Pts',(-20.6649559413948,-39.2857353862206,
124.245785908657)) ;
#48271=CARTESIAN_POINT('Ctrl Pts',(-20.514413173183,-39.4757187104213,123.894581207319)) ;
#48272=CARTESIAN_POINT('Ctrl Pts',(-20.7907073337683,-39.2957296300584,
124.015257630016)) ;
#48273=CARTESIAN_POINT('Ctrl Pts',(-20.5811176261202,-39.4856439398455,
123.69683639536)) ;
#48274=CARTESIAN_POINT('Ctrl Pts',(-20.8740852786362,-39.3056548594826,
123.76807558954)) ;
#48275=CARTESIAN_POINT('Ctrl Pts',(-20.6127981685667,-39.495671903737,123.488439172828)) ;
#48276=CARTESIAN_POINT('Ctrl Pts',(-20.9136831801555,-39.3156828233741,
123.507578576389)) ;
#48277=CARTESIAN_POINT('Ctrl Pts',(-20.6080961840771,-39.5055581633674,
123.280620724186)) ;
#48278=CARTESIAN_POINT('Ctrl Pts',(-20.9078028794062,-39.3255690830045,
123.247805458002)) ;
#48279=CARTESIAN_POINT('Ctrl Pts',(-20.5669027528603,-39.5155899264452,
123.073819312021)) ;
#48280=CARTESIAN_POINT('Ctrl Pts',(-20.8563083055305,-39.3356008460823,
122.989304179214)) ;
#48281=CARTESIAN_POINT('Ctrl Pts',(-20.4917344516677,-39.5254715527393,
122.880112689592)) ;
#48282=CARTESIAN_POINT('Ctrl Pts',(-20.7623452754649,-39.3454824723765,
122.747171858518)) ;
#48283=CARTESIAN_POINT('Ctrl Pts',(-20.3821947597893,-39.5355333222255,
122.69919029706)) ;
#48284=CARTESIAN_POINT('Ctrl Pts',(-20.6254181998426,-39.3555442418626,
122.521020260046)) ;
#48285=CARTESIAN_POINT('Ctrl Pts',(-20.2457369593962,-39.545391189721,122.543178844289)) ;
#48286=CARTESIAN_POINT('Ctrl Pts',(-20.4548438165245,-39.3654021093581,
122.326007790114)) ;
#48287=CARTESIAN_POINT('Ctrl Pts',(-20.0824035138093,-39.5553828148383,
122.411136991431)) ;
#48288=CARTESIAN_POINT('Ctrl Pts',(-20.2506752048756,-39.3753937344755,
122.160957633342)) ;
#48289=CARTESIAN_POINT('Ctrl Pts',(-19.8995811867269,-39.5653196139466,
122.310034299086)) ;
#48290=CARTESIAN_POINT('Ctrl Pts',(-20.0221459359135,-39.3853305335837,
122.034581725534)) ;
#48291=CARTESIAN_POINT('Ctrl Pts',(-19.7010155069493,-39.5753104435039,
122.241558693215)) ;
#48292=CARTESIAN_POINT('Ctrl Pts',(-19.7739378812529,-39.3953213631411,
121.948989845805)) ;
#48293=CARTESIAN_POINT('Ctrl Pts',(-19.492862253122,-39.5853336792171,122.208735174446)) ;
#48294=CARTESIAN_POINT('Ctrl Pts',(-19.5137457792809,-39.4053445988542,
121.90796320333)) ;
#48295=CARTESIAN_POINT('Ctrl Pts',(-19.2848447608836,-39.5952300272463,
122.212328557573)) ;
#48296=CARTESIAN_POINT('Ctrl Pts',(-19.2537240353539,-39.4152409468834,
121.912457737756)) ;
#48297=CARTESIAN_POINT('Ctrl Pts',(-19.0785873856562,-39.6052195897488,
122.251922424187)) ;
#48298=CARTESIAN_POINT('Ctrl Pts',(-18.9959028450578,-39.4252305093859,
121.961952758598)) ;
#48299=CARTESIAN_POINT('Ctrl Pts',(-18.8815126411,-39.6152598974333,122.327498065648)) ;
#48300=CARTESIAN_POINT('Ctrl Pts',(-18.7495601440801,-39.4352708170704,
122.056425100597)) ;
#48301=CARTESIAN_POINT('Ctrl Pts',(-18.7038945149076,-39.6251022007805,
122.433676485987)) ;
#48302=CARTESIAN_POINT('Ctrl Pts',(-18.5275396488835,-39.4451131204176,
122.189149904879)) ;
#48303=CARTESIAN_POINT('Ctrl Pts',(-18.5443823308829,-39.6351259090596,
122.571330211097)) ;
#48304=CARTESIAN_POINT('Ctrl Pts',(-18.3281491908963,-39.4551368286967,
122.361220908179)) ;
#48305=CARTESIAN_POINT('Ctrl Pts',(-18.3685442000014,-39.6483480865273,
122.786691141863)) ;
#48306=CARTESIAN_POINT('Ctrl Pts',(-18.1083641388758,-39.4683590061644,
122.630415698339)) ;
#48307=CARTESIAN_POINT('Ctrl Pts',(-18.2520900531708,-39.6616406715866,
123.044166683935)) ;
#48308=CARTESIAN_POINT('Ctrl Pts',(-17.9628051141578,-39.4816515912237,
122.952220149241)) ;
#48309=CARTESIAN_POINT('Ctrl Pts',(-18.2067947635487,-39.6749255275082,
123.319772585123)) ;
#48310=CARTESIAN_POINT('Ctrl Pts',(-17.9061735340481,-39.4949364471453,
123.296785705772)) ;
#48311=CARTESIAN_POINT('Ctrl Pts',(-18.2090712913271,-39.684897754681,123.529386284599)) ;
#48312=CARTESIAN_POINT('Ctrl Pts',(-17.9090249687646,-39.5049086743181,
123.558791097656)) ;
#48313=CARTESIAN_POINT('Ctrl Pts',(-18.2471189349561,-39.69480637112,123.734216590928)) ;
#48314=CARTESIAN_POINT('Ctrl Pts',(-17.956586488933,-39.5148172907571,123.814831513861)) ;
#48315=CARTESIAN_POINT('Ctrl Pts',(-18.3212835409877,-39.7048595765037,
123.932106036806)) ;
#48316=CARTESIAN_POINT('Ctrl Pts',(-18.0492936761947,-39.5248704961408,
124.062190998726)) ;
#48317=CARTESIAN_POINT('Ctrl Pts',(-18.4265731448462,-39.714724710264,124.110805164923)) ;
#48318=CARTESIAN_POINT('Ctrl Pts',(-18.1809125138042,-39.5347356299011,
124.285566478985)) ;
#48319=CARTESIAN_POINT('Ctrl Pts',(-18.6083337458461,-39.7280637678903,
124.324363825404)) ;
#48320=CARTESIAN_POINT('Ctrl Pts',(-18.4080910892468,-39.5480746875274,
124.552496993327)) ;
#48321=CARTESIAN_POINT('Ctrl Pts',(-18.8983167375147,-39.7446329552234,
124.524458458027)) ;
#48322=CARTESIAN_POINT('Ctrl Pts',(-18.7706176279161,-39.5646438748606,
124.802631868927)) ;
#48323=CARTESIAN_POINT('Ctrl Pts',(-19.2406669716427,-39.7612780950745,
124.61423815662)) ;
#48324=CARTESIAN_POINT('Ctrl Pts',(-19.1984775012585,-39.5812890147116,
124.914837427631)) ;
#48325=CARTESIAN_POINT('Ctrl Pts',(-19.5196867167119,-39.7745503975479,
124.61271922313)) ;
#48326=CARTESIAN_POINT('Ctrl Pts',(-19.5473160626107,-39.594561317185,124.912945050677)) ;
#48327=CARTESIAN_POINT('Ctrl Pts',(-19.7261653450185,-39.7845313609955,
124.575425604287)) ;
#48328=CARTESIAN_POINT('Ctrl Pts',(-19.8054003621908,-39.6045422806326,
124.866324423649)) ;
#48329=CARTESIAN_POINT('Ctrl Pts',(-19.9223292162796,-39.7944731930648,
124.503237795506)) ;
#48330=CARTESIAN_POINT('Ctrl Pts',(-20.0506098849888,-39.6144841127019,
124.776085831053)) ;
#48331=CARTESIAN_POINT('Ctrl Pts',(-20.1643724086472,-39.8077927622802,
124.362474521717)) ;
#48332=CARTESIAN_POINT('Ctrl Pts',(-20.3531494019142,-39.6278036819174,
124.600140541929)) ;
#48333=CARTESIAN_POINT('Ctrl Pts',(-20.412637735221,-39.824322917213,124.113575614291)) ;
#48334=CARTESIAN_POINT('Ctrl Pts',(-20.6634916788334,-39.6443338368501,
124.289002055755)) ;
#48335=CARTESIAN_POINT('Ctrl Pts',(-20.5921614259415,-39.8443446427051,
123.727677934125)) ;
#48336=CARTESIAN_POINT('Ctrl Pts',(-20.8878880488286,-39.6643555623422,
123.80663214029)) ;
#48337=CARTESIAN_POINT('Ctrl Pts',(-20.62909002806,-39.8641560393119,123.307952932077)) ;
#48338=CARTESIAN_POINT('Ctrl Pts',(-20.9340458411,-39.684166958949,123.281975948021)) ;
#48339=CARTESIAN_POINT('Ctrl Pts',(-20.5203568846511,-39.8841412880207,
122.897261125277)) ;
#48340=CARTESIAN_POINT('Ctrl Pts',(-20.7981256340549,-39.7041522076579,
122.768612564933)) ;
#48341=CARTESIAN_POINT('Ctrl Pts',(-20.2787761694729,-39.9040353506567,
122.549947579521)) ;
#48342=CARTESIAN_POINT('Ctrl Pts',(-20.4961474222789,-39.7240462702938,
122.334473379802)) ;
#48343=CARTESIAN_POINT('Ctrl Pts',(-19.9329494436863,-39.9239670298303,
122.304988298998)) ;
#48344=CARTESIAN_POINT('Ctrl Pts',(-20.0638627446628,-39.7439779494674,
122.028277249774)) ;
#48345=CARTESIAN_POINT('Ctrl Pts',(-19.5235438881534,-39.9439310843023,
122.192828842814)) ;
#48346=CARTESIAN_POINT('Ctrl Pts',(-19.552105313075,-39.7639420039394,121.888081012904)) ;
#48347=CARTESIAN_POINT('Ctrl Pts',(-19.1021579397527,-39.9638119860652,
122.226651373111)) ;
#48348=CARTESIAN_POINT('Ctrl Pts',(-19.0253744540023,-39.7838229057023,
121.930361827111)) ;
#48349=CARTESIAN_POINT('Ctrl Pts',(-18.7163649280739,-39.9837506476736,
122.402373200005)) ;
#48350=CARTESIAN_POINT('Ctrl Pts',(-18.5431348409718,-39.8037615673107,
122.150015941344)) ;
#48351=CARTESIAN_POINT('Ctrl Pts',(-18.4142773535418,-40.0036471729289,
122.698534548937)) ;
#48352=CARTESIAN_POINT('Ctrl Pts',(-18.1655278033416,-39.823658092566,122.520218221338)) ;
#48353=CARTESIAN_POINT('Ctrl Pts',(-18.2307652703842,-40.0235422113832,
123.07969577924)) ;
#48354=CARTESIAN_POINT('Ctrl Pts',(-17.9361396477719,-39.8435531310203,
122.99666905445)) ;
#48355=CARTESIAN_POINT('Ctrl Pts',(-18.1882574040753,-40.0435060346893,
123.502015421763)) ;
#48356=CARTESIAN_POINT('Ctrl Pts',(-17.883006132507,-39.8635169543264,123.524568225147)) ;
#48357=CARTESIAN_POINT('Ctrl Pts',(-18.29165985598,-40.0633801588183,123.911779372075)) ;
#48358=CARTESIAN_POINT('Ctrl Pts',(-18.0122595317287,-39.8833910784555,
124.036771136618)) ;
#48359=CARTESIAN_POINT('Ctrl Pts',(-18.5295568784576,-40.0833552345456,
124.263648018593)) ;
#48360=CARTESIAN_POINT('Ctrl Pts',(-18.3096308451413,-39.9033661541827,
124.476606505038)) ;
#48361=CARTESIAN_POINT('Ctrl Pts',(-18.873213806286,-40.1033088039022,124.512438604021)) ;
#48362=CARTESIAN_POINT('Ctrl Pts',(-18.7392016865621,-39.9233197235393,
124.787593898478)) ;
#48363=CARTESIAN_POINT('Ctrl Pts',(-19.2785655362842,-40.12314671409,124.629117591118)) ;
#48364=CARTESIAN_POINT('Ctrl Pts',(-19.245888696071,-39.9431576337272,124.933442271979)) ;
#48365=CARTESIAN_POINT('Ctrl Pts',(-19.7023551259677,-40.143122542661,124.600718350869)) ;
#48366=CARTESIAN_POINT('Ctrl Pts',(-19.7756254405552,-39.9631334622981,
124.897944226643)) ;
#48367=CARTESIAN_POINT('Ctrl Pts',(-20.0896769698093,-40.1630405873712,
124.429488132005)) ;
#48368=CARTESIAN_POINT('Ctrl Pts',(-20.259776971264,-39.9830515070084,124.68390775287)) ;
#48369=CARTESIAN_POINT('Ctrl Pts',(-20.3954104326446,-40.1829108331589,
124.137764071626)) ;
#48370=CARTESIAN_POINT('Ctrl Pts',(-20.6419438140887,-40.002921752796,124.319255201488)) ;
#48371=CARTESIAN_POINT('Ctrl Pts',(-20.5842765338552,-40.2029598362585,
123.755710496064)) ;
#48372=CARTESIAN_POINT('Ctrl Pts',(-20.8780281936789,-40.0229707558956,
123.841688417852)) ;
#48373=CARTESIAN_POINT('Ctrl Pts',(-20.6312875915322,-40.2227390774993,
123.337660256565)) ;
#48374=CARTESIAN_POINT('Ctrl Pts',(-20.9367938161444,-40.0427499971364,
123.319128562746)) ;
#48375=CARTESIAN_POINT('Ctrl Pts',(-20.532247620092,-40.2427691412082,122.923541794563)) ;
#48376=CARTESIAN_POINT('Ctrl Pts',(-20.8129964068986,-40.0627800608453,
122.801479468829)) ;
#48377=CARTESIAN_POINT('Ctrl Pts',(-20.2989045718909,-40.2626514261102,
122.570943457578)) ;
#48378=CARTESIAN_POINT('Ctrl Pts',(-20.5213204071413,-40.0826623457473,
122.360731282124)) ;
#48379=CARTESIAN_POINT('Ctrl Pts',(-19.9600279754679,-40.2825337270031,
122.318257760773)) ;
#48380=CARTESIAN_POINT('Ctrl Pts',(-20.0977276287473,-40.1025446466403,
122.044872252735)) ;
#48381=CARTESIAN_POINT('Ctrl Pts',(-19.5531288014987,-40.3025168366215,
122.195882017085)) ;
#48382=CARTESIAN_POINT('Ctrl Pts',(-19.5891047472004,-40.1225277562586,
121.891899364651)) ;
#48383=CARTESIAN_POINT('Ctrl Pts',(-19.1308454732642,-40.3224072319994,
122.219647803408)) ;
#48384=CARTESIAN_POINT('Ctrl Pts',(-19.0612514000338,-40.1424181516365,
121.921603035673)) ;
#48385=CARTESIAN_POINT('Ctrl Pts',(-18.7417231158238,-40.3423040220336,
122.38552655651)) ;
#48386=CARTESIAN_POINT('Ctrl Pts',(-18.5748477163413,-40.1623149416708,
122.128947492388)) ;
#48387=CARTESIAN_POINT('Ctrl Pts',(-18.4318742792953,-40.3622210759752,
122.674244241734)) ;
#48388=CARTESIAN_POINT('Ctrl Pts',(-18.1875342172556,-40.1822319956124,
122.489841093225)) ;
#48389=CARTESIAN_POINT('Ctrl Pts',(-18.2384227273083,-40.3822246241788,
123.053097596815)) ;
#48390=CARTESIAN_POINT('Ctrl Pts',(-17.9457158456868,-40.2022355438159,
122.963405930333)) ;
#48391=CARTESIAN_POINT('Ctrl Pts',(-18.1866699600762,-40.4021629178314,
123.473848629645)) ;
#48392=CARTESIAN_POINT('Ctrl Pts',(-17.8810209349113,-40.2221738374685,
123.489343815251)) ;
#48393=CARTESIAN_POINT('Ctrl Pts',(-18.280049631561,-40.4219844052643,123.884838555175)) ;
#48394=CARTESIAN_POINT('Ctrl Pts',(-17.9977400537545,-40.2419953249014,
124.003081008329)) ;
#48395=CARTESIAN_POINT('Ctrl Pts',(-18.5094838644823,-40.4419627982552,
124.242285334387)) ;
#48396=CARTESIAN_POINT('Ctrl Pts',(-18.2845312148424,-40.2619737178923,
124.449892679348)) ;
#48397=CARTESIAN_POINT('Ctrl Pts',(-18.8460247213349,-40.4618611798689,
124.498817471921)) ;
#48398=CARTESIAN_POINT('Ctrl Pts',(-18.7051945465058,-40.281872099506,124.770559205405)) ;
#48399=CARTESIAN_POINT('Ctrl Pts',(-19.1823032913064,-40.4784441105988,
124.604500943763)) ;
#48400=CARTESIAN_POINT('Ctrl Pts',(-19.1255703487818,-40.2984550302359,
124.902674539461)) ;
#48401=CARTESIAN_POINT('Ctrl Pts',(-19.4611720898915,-40.4917183461876,
124.616752614585)) ;
#48402=CARTESIAN_POINT('Ctrl Pts',(-19.4741295857763,-40.3117292658247,
124.917986772684)) ;
#48403=CARTESIAN_POINT('Ctrl Pts',(-19.6705355947193,-40.5017647636438,
124.589137634991)) ;
#48404=CARTESIAN_POINT('Ctrl Pts',(-19.7358425463294,-40.3217756832809,
124.883469686194)) ;
#48405=CARTESIAN_POINT('Ctrl Pts',(-19.8680131387049,-40.5116099888631,
124.527058907304)) ;
#48406=CARTESIAN_POINT('Ctrl Pts',(-19.9826774778135,-40.3316209085002,
124.805881778584)) ;
#48407=CARTESIAN_POINT('Ctrl Pts',(-20.1170123821962,-40.5249449599025,
124.398409715662)) ;
#48408=CARTESIAN_POINT('Ctrl Pts',(-20.293982933582,-40.3449558795396,124.645032731908)) ;
#48409=CARTESIAN_POINT('Ctrl Pts',(-20.3777873292751,-40.5415278166951,
124.160882668887)) ;
#48410=CARTESIAN_POINT('Ctrl Pts',(-20.6198884114383,-40.3615387363322,
124.348182656226)) ;
#48411=CARTESIAN_POINT('Ctrl Pts',(-20.5424028350229,-40.5581708190445,
123.847768971427)) ;
#48412=CARTESIAN_POINT('Ctrl Pts',(-20.8256972515988,-40.3781817386816,
123.956743051151)) ;
#48413=CARTESIAN_POINT('Ctrl Pts',(-20.6040438140094,-40.5714145500762,
123.576158500164)) ;
#48414=CARTESIAN_POINT('Ctrl Pts',(-20.9027340822747,-40.3914254697133,
123.617264907875)) ;
#48415=CARTESIAN_POINT('Ctrl Pts',(-20.6143139077877,-40.5814689447508,
123.36507953087)) ;
#48416=CARTESIAN_POINT('Ctrl Pts',(-20.9155780417739,-40.4014798643879,
123.353409333891)) ;
#48417=CARTESIAN_POINT('Ctrl Pts',(-20.5885990189638,-40.5913100061393,
123.159754071886)) ;
#48418=CARTESIAN_POINT('Ctrl Pts',(-20.8834362366564,-40.4113209257765,
123.096754250363)) ;
#48419=CARTESIAN_POINT('Ctrl Pts',(-20.5264471958815,-40.6013762304958,
122.957500488943)) ;
#48420=CARTESIAN_POINT('Ctrl Pts',(-20.805749324976,-40.421387150133,122.843935791926)) ;
#48421=CARTESIAN_POINT('Ctrl Pts',(-20.4318111963384,-40.6112568434155,
122.772550933144)) ;
#48422=CARTESIAN_POINT('Ctrl Pts',(-20.6874567828035,-40.4312677630526,
122.61274782886)) ;
#48423=CARTESIAN_POINT('Ctrl Pts',(-20.3054294573994,-40.6212501365751,
122.604767036362)) ;
#48424=CARTESIAN_POINT('Ctrl Pts',(-20.5294818312083,-40.4412610562122,
122.403016184153)) ;
#48425=CARTESIAN_POINT('Ctrl Pts',(-20.1524873681173,-40.6312011447987,
122.461975515907)) ;
#48426=CARTESIAN_POINT('Ctrl Pts',(-20.3383061144584,-40.4512120644359,
122.224524733115)) ;
#48427=CARTESIAN_POINT('Ctrl Pts',(-19.9753190448652,-40.6412496591607,
122.346959912909)) ;
#48428=CARTESIAN_POINT('Ctrl Pts',(-20.116847152072,-40.4612605787978,122.080752823443)) ;
#48429=CARTESIAN_POINT('Ctrl Pts',(-19.7849296325353,-40.6510911652234,
122.265920115438)) ;
#48430=CARTESIAN_POINT('Ctrl Pts',(-19.8788615309096,-40.4711020848605,
121.979450513905)) ;
#48431=CARTESIAN_POINT('Ctrl Pts',(-19.5805644894003,-40.6610768178531,
122.218048516374)) ;
#48432=CARTESIAN_POINT('Ctrl Pts',(-19.623405666514,-40.4810877374902,121.919608247054)) ;
#48433=CARTESIAN_POINT('Ctrl Pts',(-19.3719102404823,-40.671015826698,122.206359844049)) ;
#48434=CARTESIAN_POINT('Ctrl Pts',(-19.3625879444289,-40.4910267463351,
121.904994593026)) ;
#48435=CARTESIAN_POINT('Ctrl Pts',(-19.1623259439942,-40.681056751991,122.231380193141)) ;
#48436=CARTESIAN_POINT('Ctrl Pts',(-19.1006071741867,-40.5010676716281,
121.936267236992)) ;
#48437=CARTESIAN_POINT('Ctrl Pts',(-18.9632287027856,-40.6909470737459,
122.291388692216)) ;
#48438=CARTESIAN_POINT('Ctrl Pts',(-18.8517347176778,-40.510957993383,122.011275192603)) ;
#48439=CARTESIAN_POINT('Ctrl Pts',(-18.7754842627344,-40.7009430470793,
122.385762996334)) ;
#48440=CARTESIAN_POINT('Ctrl Pts',(-18.6170528304471,-40.5209539667164,
122.129240595666)) ;
#48441=CARTESIAN_POINT('Ctrl Pts',(-18.6080361030909,-40.7108744466613,
122.51049410798)) ;
#48442=CARTESIAN_POINT('Ctrl Pts',(-18.4077408551288,-40.5308853662985,
122.285152304524)) ;
#48443=CARTESIAN_POINT('Ctrl Pts',(-18.4635012584254,-40.7208799871384,
122.663335115609)) ;
#48444=CARTESIAN_POINT('Ctrl Pts',(-18.2270702114119,-40.5408909067755,
122.476201697503)) ;
#48445=CARTESIAN_POINT('Ctrl Pts',(-18.3477150281808,-40.7309129710697,
122.839629729903)) ;
#48446=CARTESIAN_POINT('Ctrl Pts',(-18.0823350470843,-40.5509238907068,
122.696568451517)) ;
#48447=CARTESIAN_POINT('Ctrl Pts',(-18.2654267208358,-40.7407686018965,
123.029802709535)) ;
#48448=CARTESIAN_POINT('Ctrl Pts',(-17.9794720037659,-40.5607795215337,
122.934283776559)) ;
#48449=CARTESIAN_POINT('Ctrl Pts',(-18.2164553752564,-40.7507680040897,
123.234201010115)) ;
#48450=CARTESIAN_POINT('Ctrl Pts',(-17.9182550889907,-40.5707789237268,
123.189781090327)) ;
#48451=CARTESIAN_POINT('Ctrl Pts',(-18.2036080978333,-40.7606624734508,
123.441855570182)) ;
#48452=CARTESIAN_POINT('Ctrl Pts',(-17.9021932202681,-40.5806733930879,
123.44934937898)) ;
#48453=CARTESIAN_POINT('Ctrl Pts',(-18.2274647702079,-40.770725587615,123.652027977728)) ;
#48454=CARTESIAN_POINT('Ctrl Pts',(-17.932011300945,-40.5907365072521,123.712065167649)) ;
#48455=CARTESIAN_POINT('Ctrl Pts',(-18.2859206509781,-40.7805652333314,
123.85049263691)) ;
#48456=CARTESIAN_POINT('Ctrl Pts',(-18.0050786320666,-40.6005761529685,
123.960147159055)) ;
#48457=CARTESIAN_POINT('Ctrl Pts',(-18.3797695061755,-40.7906284008871,
124.040064614096)) ;
#48458=CARTESIAN_POINT('Ctrl Pts',(-18.122387240134,-40.6106393205242,124.197113300157)) ;
#48459=CARTESIAN_POINT('Ctrl Pts',(-18.5031774126307,-40.800522656682,124.207538533751)) ;
#48460=CARTESIAN_POINT('Ctrl Pts',(-18.2766451104993,-40.6205335763191,
124.406457589584)) ;
#48461=CARTESIAN_POINT('Ctrl Pts',(-18.654084810904,-40.8104644351417,124.352107908462)) ;
#48462=CARTESIAN_POINT('Ctrl Pts',(-18.4652776966857,-40.6304753547788,
124.587171422744)) ;
#48463=CARTESIAN_POINT('Ctrl Pts',(-18.828869034011,-40.8204671279719,124.469083088964)) ;
#48464=CARTESIAN_POINT('Ctrl Pts',(-18.6837565652639,-40.640478047609,124.733392656185)) ;
#48465=CARTESIAN_POINT('Ctrl Pts',(-19.0220064357381,-40.8305011499257,
124.553889575478)) ;
#48466=CARTESIAN_POINT('Ctrl Pts',(-18.9251772147638,-40.6505120695628,
124.839403238279)) ;
#48467=CARTESIAN_POINT('Ctrl Pts',(-19.223072436617,-40.8403489410147,124.603257935098)) ;
#48468=CARTESIAN_POINT('Ctrl Pts',(-19.176509623626,-40.6603598606518,124.901116406676)) ;
#48469=CARTESIAN_POINT('Ctrl Pts',(-19.4324060765276,-40.8503304655638,
124.617611036992)) ;
#48470=CARTESIAN_POINT('Ctrl Pts',(-19.4381766703649,-40.6703413852009,
124.919060383607)) ;
#48471=CARTESIAN_POINT('Ctrl Pts',(-19.6403984022838,-40.8602796890547,
124.595436731621)) ;
#48472=CARTESIAN_POINT('Ctrl Pts',(-19.6981676204706,-40.6802906086918,
124.891345054652)) ;
#48473=CARTESIAN_POINT('Ctrl Pts',(-19.842443083507,-40.8702773452713,124.537454340177)) ;
#48474=CARTESIAN_POINT('Ctrl Pts',(-19.9507242764533,-40.6902882649084,
124.818869487459)) ;
#48475=CARTESIAN_POINT('Ctrl Pts',(-20.0319489132289,-40.8803175583263,
124.444528163005)) ;
#48476=CARTESIAN_POINT('Ctrl Pts',(-20.1876076661773,-40.7003284779634,
124.702714148648)) ;
#48477=CARTESIAN_POINT('Ctrl Pts',(-20.1991246682804,-40.8901456056026,
124.323088911922)) ;
#48478=CARTESIAN_POINT('Ctrl Pts',(-20.39657947432,-40.7101565252397,124.550916691026)) ;
#48479=CARTESIAN_POINT('Ctrl Pts',(-20.346201088897,-40.9001999526349,124.171290921794)) ;
#48480=CARTESIAN_POINT('Ctrl Pts',(-20.5804267072164,-40.7202108722721,
124.361171005036)) ;
#48481=CARTESIAN_POINT('Ctrl Pts',(-20.4630696212735,-40.9101410889635,
123.998019997422)) ;
#48482=CARTESIAN_POINT('Ctrl Pts',(-20.7265146724235,-40.7301520086006,
124.144583500037)) ;
#48483=CARTESIAN_POINT('Ctrl Pts',(-20.5483504789561,-40.9200453220432,
123.808062649806)) ;
#48484=CARTESIAN_POINT('Ctrl Pts',(-20.833118168353,-40.7400562416803,123.907137322024)) ;
#48485=CARTESIAN_POINT('Ctrl Pts',(-20.5999532572044,-40.9300920188868,
123.60326863494)) ;
#48486=CARTESIAN_POINT('Ctrl Pts',(-20.8976239886845,-40.7501029385239,
123.651145500443)) ;
#48487=CARTESIAN_POINT('Ctrl Pts',(-20.6151760608575,-40.9399875701671,
123.395757075014)) ;
#48488=CARTESIAN_POINT('Ctrl Pts',(-20.9166549329738,-40.7599984898042,
123.391755647878)) ;
#48489=CARTESIAN_POINT('Ctrl Pts',(-20.5937893271631,-40.9500496480066,
123.185334655096)) ;
#48490=CARTESIAN_POINT('Ctrl Pts',(-20.8899239295474,-40.7700605676437,
123.128727559493)) ;
#48491=CARTESIAN_POINT('Ctrl Pts',(-20.5375466139094,-40.9598923571026,
122.986176025129)) ;
#48492=CARTESIAN_POINT('Ctrl Pts',(-20.8196225925667,-40.7799032767398,
122.879777795718)) ;
#48493=CARTESIAN_POINT('Ctrl Pts',(-20.4466945331734,-40.9698830893411,
122.796834964654)) ;
#48494=CARTESIAN_POINT('Ctrl Pts',(-20.7060594583057,-40.7898940089782,
122.643100332516)) ;
#48495=CARTESIAN_POINT('Ctrl Pts',(-20.32506530426,-40.9798111145698,122.627205149371)) ;
#48496=CARTESIAN_POINT('Ctrl Pts',(-20.554024482547,-40.799822034207,122.43106134549)) ;
#48497=CARTESIAN_POINT('Ctrl Pts',(-20.1751809243749,-40.9897992612204,
122.480136248305)) ;
#48498=CARTESIAN_POINT('Ctrl Pts',(-20.3666704074435,-40.8098101808575,
122.247223536498)) ;
#48499=CARTESIAN_POINT('Ctrl Pts',(-20.0010440003547,-40.9998342790604,
122.361035774299)) ;
#48500=CARTESIAN_POINT('Ctrl Pts',(-20.1490005900659,-40.8198451986975,
122.098346117619)) ;
#48501=CARTESIAN_POINT('Ctrl Pts',(-19.8122322682539,-41.0096990761655,
122.275263236687)) ;
#48502=CARTESIAN_POINT('Ctrl Pts',(-19.9129860527782,-40.8297099958027,
121.991128079681)) ;
#48503=CARTESIAN_POINT('Ctrl Pts',(-19.6095835568502,-41.0196598085217,
122.222477105135)) ;
#48504=CARTESIAN_POINT('Ctrl Pts',(-19.6596753422036,-40.8396707281588,
121.925143350382)) ;
#48505=CARTESIAN_POINT('Ctrl Pts',(-19.3993089283046,-41.0296932709187,
122.205909546878)) ;
#48506=CARTESIAN_POINT('Ctrl Pts',(-19.3968323127543,-40.8497041905558,
121.904431778563)) ;
#48507=CARTESIAN_POINT('Ctrl Pts',(-19.1923814571992,-41.0395788051301,
122.225463175371)) ;
#48508=CARTESIAN_POINT('Ctrl Pts',(-19.1381719931737,-40.8595897247672,
121.928871855677)) ;
#48509=CARTESIAN_POINT('Ctrl Pts',(-18.9884081997025,-41.0496436458101,
122.281644422525)) ;
#48510=CARTESIAN_POINT('Ctrl Pts',(-18.8832051234913,-40.8696545654472,
121.999096373019)) ;
#48511=CARTESIAN_POINT('Ctrl Pts',(-18.8013257411855,-41.0594917775389,
122.370368828685)) ;
#48512=CARTESIAN_POINT('Ctrl Pts',(-18.6493502439054,-40.8795026971761,
122.110000505807)) ;
#48513=CARTESIAN_POINT('Ctrl Pts',(-18.6291184084903,-41.0695192745291,
122.491953508965)) ;
#48514=CARTESIAN_POINT('Ctrl Pts',(-18.4340900376583,-40.8895301941662,
122.261979815528)) ;
#48515=CARTESIAN_POINT('Ctrl Pts',(-18.4810087173521,-41.0795477265741,
122.642011387807)) ;
#48516=CARTESIAN_POINT('Ctrl Pts',(-18.2489515312442,-40.8995586462113,
122.449550693022)) ;
#48517=CARTESIAN_POINT('Ctrl Pts',(-18.3630810655382,-41.0893929931382,
122.812094313911)) ;
#48518=CARTESIAN_POINT('Ctrl Pts',(-18.1015397641077,-40.9094039127754,
122.662154181766)) ;
#48519=CARTESIAN_POINT('Ctrl Pts',(-18.2746791888148,-41.0993836660792,
123.00262605961)) ;
#48520=CARTESIAN_POINT('Ctrl Pts',(-17.9910357650172,-40.9193945857163,
122.900318312532)) ;
#48521=CARTESIAN_POINT('Ctrl Pts',(-18.2209040134384,-41.1094215481676,
123.206685229747)) ;
#48522=CARTESIAN_POINT('Ctrl Pts',(-17.9238150126673,-40.9294324678048,
123.155391668012)) ;
#48523=CARTESIAN_POINT('Ctrl Pts',(-18.2033541254263,-41.1192659186073,
123.412907134102)) ;
#48524=CARTESIAN_POINT('Ctrl Pts',(-17.9018757959936,-40.9392768382444,
123.413170064838)) ;
#48525=CARTESIAN_POINT('Ctrl Pts',(-18.2217257491831,-41.1292507460027,
123.621985540264)) ;
#48526=CARTESIAN_POINT('Ctrl Pts',(-17.9248387222201,-40.9492616656398,
123.674518463669)) ;
#48527=CARTESIAN_POINT('Ctrl Pts',(-18.2757990112521,-41.139190191408,123.82385763404)) ;
#48528=CARTESIAN_POINT('Ctrl Pts',(-17.9924288980122,-40.9592011110451,
123.926859519996)) ;
#48529=CARTESIAN_POINT('Ctrl Pts',(-18.3650287174585,-41.1492301956939,
124.01511881118)) ;
#48530=CARTESIAN_POINT('Ctrl Pts',(-18.1039644977268,-40.969241115331,124.165936540769)) ;
#48531=CARTESIAN_POINT('Ctrl Pts',(-18.4841771963513,-41.1591173048795,
124.18546666406)) ;
#48532=CARTESIAN_POINT('Ctrl Pts',(-18.2528993475112,-40.9791282245166,
124.378873025714)) ;
#48533=CARTESIAN_POINT('Ctrl Pts',(-18.6325483512414,-41.169117364782,124.334363428523)) ;
#48534=CARTESIAN_POINT('Ctrl Pts',(-18.4383623409919,-40.9891282844191,
124.564995129704)) ;
#48535=CARTESIAN_POINT('Ctrl Pts',(-18.8030499054225,-41.1790347806967,
124.45442108235)) ;
#48536=CARTESIAN_POINT('Ctrl Pts',(-18.6514890497464,-40.9990457003338,
124.715068772833)) ;
#48537=CARTESIAN_POINT('Ctrl Pts',(-18.9942377867766,-41.1890815954375,
124.544124964319)) ;
#48538=CARTESIAN_POINT('Ctrl Pts',(-18.8904730960395,-41.0090925150746,
124.827199842309)) ;
#48539=CARTESIAN_POINT('Ctrl Pts',(-19.194625243992,-41.1989570726341,124.59855210773)) ;
#48540=CARTESIAN_POINT('Ctrl Pts',(-19.1409580665125,-41.0189679922713,
124.895235368087)) ;
#48541=CARTESIAN_POINT('Ctrl Pts',(-19.4051209957553,-41.2090131683554,
124.617812738333)) ;
#48542=CARTESIAN_POINT('Ctrl Pts',(-19.4040773768789,-41.0290240879925,
124.919312459321)) ;
#48543=CARTESIAN_POINT('Ctrl Pts',(-19.612431639119,-41.2189063303704,124.600588284095)) ;
#48544=CARTESIAN_POINT('Ctrl Pts',(-19.6632167072632,-41.0389172500076,
124.897783110469)) ;
#48545=CARTESIAN_POINT('Ctrl Pts',(-19.8169921171162,-41.228968566393,124.546802146257)) ;
#48546=CARTESIAN_POINT('Ctrl Pts',(-19.918917313857,-41.0489794860302,124.830551760871)) ;
#48547=CARTESIAN_POINT('Ctrl Pts',(-20.0049876675589,-41.238813032022,124.460234593198)) ;
#48548=CARTESIAN_POINT('Ctrl Pts',(-20.1539134835327,-41.0588239516591,
124.722342924619)) ;
#48549=CARTESIAN_POINT('Ctrl Pts',(-20.1775149384373,-41.2487731247261,
124.341583226709)) ;
#48550=CARTESIAN_POINT('Ctrl Pts',(-20.3695735130956,-41.0687840443633,
124.574029278927)) ;
#48551=CARTESIAN_POINT('Ctrl Pts',(-20.3276957983037,-41.2588114137072,
124.193333688779)) ;
#48552=CARTESIAN_POINT('Ctrl Pts',(-20.5573002807056,-41.0788223333443,
124.388718288801)) ;
#48553=CARTESIAN_POINT('Ctrl Pts',(-20.4481963084003,-41.2686847368134,
124.024285690543)) ;
#48554=CARTESIAN_POINT('Ctrl Pts',(-20.7079273846869,-41.0886956564505,
124.177407956231)) ;
#48555=CARTESIAN_POINT('Ctrl Pts',(-20.5392295552627,-41.2787579208985,
123.833127087447)) ;
#48556=CARTESIAN_POINT('Ctrl Pts',(-20.8217196875643,-41.0987688405356,
123.938460528923)) ;
#48557=CARTESIAN_POINT('Ctrl Pts',(-20.5945544507421,-41.2885784331864,
123.634173535179)) ;
#48558=CARTESIAN_POINT('Ctrl Pts',(-20.8908771120928,-41.1085893528235,
123.689767340494)) ;
#48559=CARTESIAN_POINT('Ctrl Pts',(-20.6152109322945,-41.2986564293022,
123.4233616068)) ;
#48560=CARTESIAN_POINT('Ctrl Pts',(-20.9166985130199,-41.1186673489393,
123.426252975594)) ;
#48561=CARTESIAN_POINT('Ctrl Pts',(-20.5993528249516,-41.3085105042855,
123.216758416183)) ;
#48562=CARTESIAN_POINT('Ctrl Pts',(-20.8968766070843,-41.1285214239226,
123.167997632845)) ;
#48563=CARTESIAN_POINT('Ctrl Pts',(-20.5470119355056,-41.3185743858692,
123.011801977239)) ;
#48564=CARTESIAN_POINT('Ctrl Pts',(-20.8314512990001,-41.1385853055063,
122.911802236426)) ;
#48565=CARTESIAN_POINT('Ctrl Pts',(-20.4613754347014,-41.3284578118429,
122.822450585418)) ;
#48566=CARTESIAN_POINT('Ctrl Pts',(-20.7244059189189,-41.14846873148,122.675111707094)) ;
#48567=CARTESIAN_POINT('Ctrl Pts',(-20.3430903346169,-41.338458415764,122.648681232655)) ;
#48568=CARTESIAN_POINT('Ctrl Pts',(-20.5765499860383,-41.1584693354011,
122.457899543958)) ;
#48569=CARTESIAN_POINT('Ctrl Pts',(-20.1976579653882,-41.3483782001018,
122.49916106268)) ;
#48570=CARTESIAN_POINT('Ctrl Pts',(-20.3947593959915,-41.168389119739,122.270998373932)) ;
#48571=CARTESIAN_POINT('Ctrl Pts',(-20.0263274877781,-41.3584255504587,
122.375678234952)) ;
#48572=CARTESIAN_POINT('Ctrl Pts',(-20.1805968421938,-41.1784364700958,
122.116644490037)) ;
#48573=CARTESIAN_POINT('Ctrl Pts',(-19.8394159318229,-41.368302892693,122.285119868391)) ;
#48574=CARTESIAN_POINT('Ctrl Pts',(-19.9469565780985,-41.1883138123301,
122.003445575771)) ;
#48575=CARTESIAN_POINT('Ctrl Pts',(-19.6358016808575,-41.3783727737676,
122.227321629888)) ;
#48576=CARTESIAN_POINT('Ctrl Pts',(-19.6924393110652,-41.1983836934047,
121.931197405337)) ;
#48577=CARTESIAN_POINT('Ctrl Pts',(-19.4302105986271,-41.3882024789693,
122.206046078144)) ;
#48578=CARTESIAN_POINT('Ctrl Pts',(-19.4354489668085,-41.2082133986064,
121.904602386854)) ;
#48579=CARTESIAN_POINT('Ctrl Pts',(-19.2191313622272,-41.3982691401357,
122.220859081126)) ;
#48580=CARTESIAN_POINT('Ctrl Pts',(-19.1716002965813,-41.2182800597728,
121.923118301563)) ;
#48581=CARTESIAN_POINT('Ctrl Pts',(-19.0174028500584,-41.408159362003,122.271341345919)) ;
#48582=CARTESIAN_POINT('Ctrl Pts',(-18.9194385507973,-41.2281702816401,
121.986221032481)) ;
#48583=CARTESIAN_POINT('Ctrl Pts',(-18.8253933440022,-41.4181515381132,
122.356520476582)) ;
#48584=CARTESIAN_POINT('Ctrl Pts',(-18.6794263982386,-41.2381624577503,
122.092694865169)) ;
#48585=CARTESIAN_POINT('Ctrl Pts',(-18.6517079385557,-41.4281143682258,
122.473569637497)) ;
#48586=CARTESIAN_POINT('Ctrl Pts',(-18.462319115849,-41.2481252878629,122.239006352315)) ;
#48587=CARTESIAN_POINT('Ctrl Pts',(-18.5014870756419,-41.4380185806261,
122.61777683837)) ;
#48588=CARTESIAN_POINT('Ctrl Pts',(-18.2745423237503,-41.2580295002633,
122.419265967195)) ;
#48589=CARTESIAN_POINT('Ctrl Pts',(-18.3768239906411,-41.448079294714,122.788607618059)) ;
#48590=CARTESIAN_POINT('Ctrl Pts',(-18.1187135739592,-41.2680902143511,
122.632804079682)) ;
#48591=CARTESIAN_POINT('Ctrl Pts',(-18.2854831726733,-41.4579187976968,
122.974241715456)) ;
#48592=CARTESIAN_POINT('Ctrl Pts',(-18.0045368875343,-41.2779297173339,
122.864848022296)) ;
#48593=CARTESIAN_POINT('Ctrl Pts',(-18.2262434983332,-41.4679849362632,
123.177367766874)) ;
#48594=CARTESIAN_POINT('Ctrl Pts',(-17.9304874746578,-41.2879958559003,
123.11875522056)) ;
#48595=CARTESIAN_POINT('Ctrl Pts',(-18.2036641637308,-41.4778674507492,
123.383929826508)) ;
#48596=CARTESIAN_POINT('Ctrl Pts',(-17.902263224335,-41.2978783703863,123.376958924445)) ;
#48597=CARTESIAN_POINT('Ctrl Pts',(-18.217028771755,-41.4878597501047,123.593541694944)) ;
#48598=CARTESIAN_POINT('Ctrl Pts',(-17.9189692034043,-41.3078706697419,
123.638973965491)) ;
#48599=CARTESIAN_POINT('Ctrl Pts',(-18.266354986361,-41.4978128170581,123.796921608966)) ;
#48600=CARTESIAN_POINT('Ctrl Pts',(-17.9806273077311,-41.3178237366953,
123.893199304568)) ;
#48601=CARTESIAN_POINT('Ctrl Pts',(-18.3509953062756,-41.5078475252634,
123.990141633652)) ;
#48602=CARTESIAN_POINT('Ctrl Pts',(-18.0864278200169,-41.3278584449005,
124.134724121174)) ;
#48603=CARTESIAN_POINT('Ctrl Pts',(-18.4660813786671,-41.5177357461675,
124.16327447273)) ;
#48604=CARTESIAN_POINT('Ctrl Pts',(-18.2302862077972,-41.3377466658047,
124.351140926558)) ;
#48605=CARTESIAN_POINT('Ctrl Pts',(-18.6107545882689,-41.527730169198,124.315632016027)) ;
#48606=CARTESIAN_POINT('Ctrl Pts',(-18.411128140004,-41.3477410888351,124.541587743708)) ;
#48607=CARTESIAN_POINT('Ctrl Pts',(-18.7789136987431,-41.5376755086441,
124.439882085286)) ;
#48608=CARTESIAN_POINT('Ctrl Pts',(-18.6213277144287,-41.3576864282813,
124.696900401289)) ;
#48609=CARTESIAN_POINT('Ctrl Pts',(-18.9659468148119,-41.5476228532555,
124.533455179256)) ;
#48610=CARTESIAN_POINT('Ctrl Pts',(-18.8551198560532,-41.3676337728926,
124.813866561764)) ;
#48611=CARTESIAN_POINT('Ctrl Pts',(-19.1684641307119,-41.5576707486665,
124.593501263556)) ;
#48612=CARTESIAN_POINT('Ctrl Pts',(-19.1082663812488,-41.3776816683036,
124.888923688486)) ;
#48613=CARTESIAN_POINT('Ctrl Pts',(-19.3741360186057,-41.5675183941458,
124.617169452633)) ;
#48614=CARTESIAN_POINT('Ctrl Pts',(-19.3653576889217,-41.387529313783,124.918508593892)) ;
#48615=CARTESIAN_POINT('Ctrl Pts',(-19.5832145971549,-41.5774801080598,
124.605278842965)) ;
#48616=CARTESIAN_POINT('Ctrl Pts',(-19.6267063239456,-41.397491027697,124.903644555584)) ;
#48617=CARTESIAN_POINT('Ctrl Pts',(-19.788383314369,-41.5875087323508,124.556678207782)) ;
#48618=CARTESIAN_POINT('Ctrl Pts',(-19.8831669773239,-41.4075196519879,
124.842893155659)) ;
#48619=CARTESIAN_POINT('Ctrl Pts',(-19.979718451431,-41.5974190930075,124.47424697805)) ;
#48620=CARTESIAN_POINT('Ctrl Pts',(-20.1223364379903,-41.4174300126446,
124.739853154527)) ;
#48621=CARTESIAN_POINT('Ctrl Pts',(-20.1545793968166,-41.6073537915808,
124.360016047797)) ;
#48622=CARTESIAN_POINT('Ctrl Pts',(-20.3409126898904,-41.4273647112179,
124.597063389142)) ;
#48623=CARTESIAN_POINT('Ctrl Pts',(-20.3084369890171,-41.617395616435,124.215477929178)) ;
#48624=CARTESIAN_POINT('Ctrl Pts',(-20.5332339905114,-41.4374065360721,
124.416390285309)) ;
#48625=CARTESIAN_POINT('Ctrl Pts',(-20.4330452256544,-41.6272801901794,
124.04915416565)) ;
#48626=CARTESIAN_POINT('Ctrl Pts',(-20.6889942202741,-41.4472911098165,
124.208484214558)) ;
#48627=CARTESIAN_POINT('Ctrl Pts',(-20.5281974762761,-41.6372820395426,
123.861676921121)) ;
#48628=CARTESIAN_POINT('Ctrl Pts',(-20.8079337346372,-41.4572929591797,
123.974137087454)) ;
#48629=CARTESIAN_POINT('Ctrl Pts',(-20.5890105169507,-41.6472013411166,
123.662177464747)) ;
#48630=CARTESIAN_POINT('Ctrl Pts',(-20.8839492756787,-41.4672122607537,
123.724761737193)) ;
#48631=CARTESIAN_POINT('Ctrl Pts',(-20.6145770333962,-41.6572454494619,
123.452589429869)) ;
#48632=CARTESIAN_POINT('Ctrl Pts',(-20.9159063783837,-41.477256369099,123.462776779803)) ;
#48633=CARTESIAN_POINT('Ctrl Pts',(-20.6036034057865,-41.6671298729041,
123.245068543956)) ;
#48634=CARTESIAN_POINT('Ctrl Pts',(-20.9021882404978,-41.4871407925413,
123.203374700093)) ;
#48635=CARTESIAN_POINT('Ctrl Pts',(-20.5565952979151,-41.6771462348136,
123.039799079144)) ;
#48636=CARTESIAN_POINT('Ctrl Pts',(-20.8434269167983,-41.4971571544507,
122.946788139686)) ;
#48637=CARTESIAN_POINT('Ctrl Pts',(-20.4739898693975,-41.687182890319,122.845651147378)) ;
#48638=CARTESIAN_POINT('Ctrl Pts',(-20.740169246239,-41.5071938099561,122.704103736706)) ;
#48639=CARTESIAN_POINT('Ctrl Pts',(-20.3617495143391,-41.6970130205083,
122.672097956593)) ;
#48640=CARTESIAN_POINT('Ctrl Pts',(-20.5998669968465,-41.5170239401454,
122.487161714525)) ;
#48641=CARTESIAN_POINT('Ctrl Pts',(-20.2176578236803,-41.7070890735982,
122.516880089597)) ;
#48642=CARTESIAN_POINT('Ctrl Pts',(-20.4197517580595,-41.5270999932353,
122.293140547087)) ;
#48643=CARTESIAN_POINT('Ctrl Pts',(-20.0525570282774,-41.716941302784,122.391738375316)) ;
#48644=CARTESIAN_POINT('Ctrl Pts',(-20.2133740001492,-41.5369522224211,
122.136713686681)) ;
#48645=CARTESIAN_POINT('Ctrl Pts',(-19.864251762106,-41.7270145105833,122.294921019345)) ;
#48646=CARTESIAN_POINT('Ctrl Pts',(-19.9779921555952,-41.5470254302204,
122.015693380369)) ;
#48647=CARTESIAN_POINT('Ctrl Pts',(-19.666587072999,-41.7368560219347,122.233752490588)) ;
#48648=CARTESIAN_POINT('Ctrl Pts',(-19.7309096530658,-41.5568669415718,
121.939233606283)) ;
#48649=CARTESIAN_POINT('Ctrl Pts',(-19.458933216277,-41.7468169599722,122.206739976442)) ;
#48650=CARTESIAN_POINT('Ctrl Pts',(-19.4713417220652,-41.5668278796093,
121.905469506213)) ;
#48651=CARTESIAN_POINT('Ctrl Pts',(-19.2481470392033,-41.7568548218972,
122.21668888155)) ;
#48652=CARTESIAN_POINT('Ctrl Pts',(-19.2078592032353,-41.5768657415343,
121.917907090772)) ;
#48653=CARTESIAN_POINT('Ctrl Pts',(-19.0455303660746,-41.7667290078943,
122.261958044375)) ;
#48654=CARTESIAN_POINT('Ctrl Pts',(-18.9545877190135,-41.5867399275314,
121.974495320736)) ;
#48655=CARTESIAN_POINT('Ctrl Pts',(-18.8501065214671,-41.7767991674721,
122.343300097971)) ;
#48656=CARTESIAN_POINT('Ctrl Pts',(-18.7103088483806,-41.5968100871093,
122.076174219164)) ;
#48657=CARTESIAN_POINT('Ctrl Pts',(-18.675884913286,-41.786630914898,122.454554501871)) ;
#48658=CARTESIAN_POINT('Ctrl Pts',(-18.4925316287136,-41.6066418345351,
122.215244290512)) ;
#48659=CARTESIAN_POINT('Ctrl Pts',(-18.5201147053539,-41.7966669949693,
122.596849719958)) ;
#48660=CARTESIAN_POINT('Ctrl Pts',(-18.2978201733905,-41.6166779146064,
122.393114575387)) ;
#48661=CARTESIAN_POINT('Ctrl Pts',(-18.3920704361308,-41.8066840418218,
122.764054383414)) ;
#48662=CARTESIAN_POINT('Ctrl Pts',(-18.1377661291796,-41.6266949614589,
122.602121409424)) ;
#48663=CARTESIAN_POINT('Ctrl Pts',(-18.2959657375201,-41.8165662999884,
122.948249336601)) ;
#48664=CARTESIAN_POINT('Ctrl Pts',(-18.0176363964437,-41.6365772196255,
122.832366722384)) ;
#48665=CARTESIAN_POINT('Ctrl Pts',(-18.2324121268901,-41.8265539827847,
123.148349956058)) ;
#48666=CARTESIAN_POINT('Ctrl Pts',(-17.9381960769655,-41.6465649024218,
123.082493245792)) ;
#48667=CARTESIAN_POINT('Ctrl Pts',(-18.2045073332423,-41.8365006395015,
123.355622216733)) ;
#48668=CARTESIAN_POINT('Ctrl Pts',(-17.9033168942799,-41.6565115591386,
123.341584277109)) ;
#48669=CARTESIAN_POINT('Ctrl Pts',(-18.2133253026657,-41.8465576975816,
123.566846105413)) ;
#48670=CARTESIAN_POINT('Ctrl Pts',(-17.9143411683041,-41.6665686172188,
123.605613842751)) ;
#48671=CARTESIAN_POINT('Ctrl Pts',(-18.2573346938639,-41.8563758771311,
123.768519750159)) ;
#48672=CARTESIAN_POINT('Ctrl Pts',(-17.969355045573,-41.6763867967682,123.857706729659)) ;
#48673=CARTESIAN_POINT('Ctrl Pts',(-18.3368951497359,-41.86641181157,123.963925455045)) ;
#48674=CARTESIAN_POINT('Ctrl Pts',(-18.0688075005491,-41.6864227312072,
124.101962973962)) ;
#48675=CARTESIAN_POINT('Ctrl Pts',(-18.449568449613,-41.876436465999,124.142036436665)) ;
#48676=CARTESIAN_POINT('Ctrl Pts',(-18.2096507194806,-41.6964473856362,
124.324600663781)) ;
#48677=CARTESIAN_POINT('Ctrl Pts',(-18.5886702041934,-41.8862884855786,
124.295499146271)) ;
#48678=CARTESIAN_POINT('Ctrl Pts',(-18.3835301012507,-41.7062994052157,
124.51642843277)) ;
#48679=CARTESIAN_POINT('Ctrl Pts',(-18.7543933359487,-41.8962793992935,
124.424504024787)) ;
#48680=CARTESIAN_POINT('Ctrl Pts',(-18.5906854588075,-41.7162903189306,
124.677682956406)) ;
#48681=CARTESIAN_POINT('Ctrl Pts',(-18.9386244083252,-41.9061973881331,
124.522200361594)) ;
#48682=CARTESIAN_POINT('Ctrl Pts',(-18.8209758181354,-41.7262083077702,
124.799801736939)) ;
#48683=CARTESIAN_POINT('Ctrl Pts',(-19.1391682617768,-41.9162254988639,
124.587172771734)) ;
#48684=CARTESIAN_POINT('Ctrl Pts',(-19.0716562721303,-41.736236418501,124.88101516819)) ;
#48685=CARTESIAN_POINT('Ctrl Pts',(-19.3449799514909,-41.9261106967723,
124.616011040742)) ;
#48686=CARTESIAN_POINT('Ctrl Pts',(-19.3289219205496,-41.7461216164094,
124.917060930178)) ;
#48687=CARTESIAN_POINT('Ctrl Pts',(-19.554878431118,-41.9360999720403,124.609111482474)) ;
#48688=CARTESIAN_POINT('Ctrl Pts',(-19.5912951011556,-41.7561108916774,
124.908434150028)) ;
#48689=CARTESIAN_POINT('Ctrl Pts',(-19.7613596240019,-41.9461414302098,
124.565200707997)) ;
#48690=CARTESIAN_POINT('Ctrl Pts',(-19.8493960390687,-41.7661523498469,
124.853543536914)) ;
#48691=CARTESIAN_POINT('Ctrl Pts',(-19.9531398235918,-41.9559728939981,
124.48810716658)) ;
#48692=CARTESIAN_POINT('Ctrl Pts',(-20.089121327571,-41.7759838136352,124.757174104887)) ;
#48693=CARTESIAN_POINT('Ctrl Pts',(-20.1319364909177,-41.965977826302,124.377372382878)) ;
#48694=CARTESIAN_POINT('Ctrl Pts',(-20.3126159520966,-41.7859887459391,
124.618753527264)) ;
#48695=CARTESIAN_POINT('Ctrl Pts',(-20.2884681065489,-41.9759641901967,
124.237408278261)) ;
#48696=CARTESIAN_POINT('Ctrl Pts',(-20.5082790000552,-41.7959751098338,
124.44379651089)) ;
#48697=CARTESIAN_POINT('Ctrl Pts',(-20.4187181316533,-41.9859938190826,
124.071617468983)) ;
#48698=CARTESIAN_POINT('Ctrl Pts',(-20.6710896620277,-41.8060047387197,
124.236556568521)) ;
#48699=CARTESIAN_POINT('Ctrl Pts',(-20.5169261211042,-41.995869041191,123.888684071241)) ;
#48700=CARTESIAN_POINT('Ctrl Pts',(-20.7938478463196,-41.8158799608281,
124.007888084102)) ;
#48701=CARTESIAN_POINT('Ctrl Pts',(-20.5829278692201,-42.0058702535881,
123.689089793923)) ;
#48702=CARTESIAN_POINT('Ctrl Pts',(-20.8763477233689,-41.8258811732252,
123.758394357555)) ;
#48703=CARTESIAN_POINT('Ctrl Pts',(-20.6131956145041,-42.0157788328236,
123.482954015089)) ;
#48704=CARTESIAN_POINT('Ctrl Pts',(-20.9141799974451,-41.8357897524607,
123.500723797923)) ;
#48705=CARTESIAN_POINT('Ctrl Pts',(-20.6070613238518,-42.0258336853796,
123.271692586383)) ;
#48706=CARTESIAN_POINT('Ctrl Pts',(-20.9065096443018,-41.8458446050167,
123.236647196744)) ;
#48707=CARTESIAN_POINT('Ctrl Pts',(-20.5653915462767,-42.0356922676544,
123.068629174948)) ;
#48708=CARTESIAN_POINT('Ctrl Pts',(-20.8544198064542,-41.8557031872915,
122.982817801589)) ;
#48709=CARTESIAN_POINT('Ctrl Pts',(-20.4876191246396,-42.0457603970971,
122.871804464288)) ;
#48710=CARTESIAN_POINT('Ctrl Pts',(-20.7572019522211,-41.8657713167342,
122.736787999825)) ;
#48711=CARTESIAN_POINT('Ctrl Pts',(-20.3791532075603,-42.0556158687862,
122.695250592433)) ;
#48712=CARTESIAN_POINT('Ctrl Pts',(-20.6216170476226,-41.8756267884233,
122.516096462903)) ;
#48713=CARTESIAN_POINT('Ctrl Pts',(-20.2402233414134,-42.0656107171724,
122.53762013048)) ;
#48714=CARTESIAN_POINT('Ctrl Pts',(-20.4479526497867,-41.8856216368096,
122.319060073039)) ;
#48715=CARTESIAN_POINT('Ctrl Pts',(-20.0751431990478,-42.0756420139569,
122.406377183477)) ;
#48716=CARTESIAN_POINT('Ctrl Pts',(-20.2416008599543,-41.895652933594,122.155008415797)) ;
#48717=CARTESIAN_POINT('Ctrl Pts',(-19.8929827389423,-42.085508550167,122.307151426831)) ;
#48718=CARTESIAN_POINT('Ctrl Pts',(-20.0138985646584,-41.9055194698041,
122.030978291943)) ;
#48719=CARTESIAN_POINT('Ctrl Pts',(-19.6940889865307,-42.0954959731278,
122.239940435497)) ;
#48720=CARTESIAN_POINT('Ctrl Pts',(-19.7652803949844,-41.9155068927649,
121.946967065513)) ;
#48721=CARTESIAN_POINT('Ctrl Pts',(-19.4873935007549,-42.1054409121476,
122.208304514953)) ;
#48722=CARTESIAN_POINT('Ctrl Pts',(-19.5069103967345,-41.9254518317847,
121.907424800281)) ;
#48723=CARTESIAN_POINT('Ctrl Pts',(-19.2762891943971,-42.1154857980076,
122.213185852874)) ;
#48724=CARTESIAN_POINT('Ctrl Pts',(-19.2430300937842,-41.9354967176447,
121.913529165086)) ;
#48725=CARTESIAN_POINT('Ctrl Pts',(-19.0728324499465,-42.1253543330938,
122.253813361827)) ;
#48726=CARTESIAN_POINT('Ctrl Pts',(-18.9887092821943,-41.9453652527309,
121.964316287629)) ;
#48727=CARTESIAN_POINT('Ctrl Pts',(-18.877416228865,-42.1353202011005,122.329344157201)) ;
#48728=CARTESIAN_POINT('Ctrl Pts',(-18.7444398718667,-41.9553311207376,
122.058732418128)) ;
#48729=CARTESIAN_POINT('Ctrl Pts',(-18.697163938135,-42.145342848553,122.438490697059)) ;
#48730=CARTESIAN_POINT('Ctrl Pts',(-18.5191258960405,-41.9653537681901,
122.195167959833)) ;
#48731=CARTESIAN_POINT('Ctrl Pts',(-18.5401483686295,-42.1552664875606,
122.575845813976)) ;
#48732=CARTESIAN_POINT('Ctrl Pts',(-18.322858065799,-41.9752774071977,122.366864085304)) ;
#48733=CARTESIAN_POINT('Ctrl Pts',(-18.408710854997,-42.1652092125663,122.738393134439)) ;
#48734=CARTESIAN_POINT('Ctrl Pts',(-18.1585632397569,-41.9852201322034,
122.570050124167)) ;
#48735=CARTESIAN_POINT('Ctrl Pts',(-18.3066794566052,-42.1752548186182,
122.92328748586)) ;
#48736=CARTESIAN_POINT('Ctrl Pts',(-18.0310264117004,-41.9952657382553,
122.80116942064)) ;
#48737=CARTESIAN_POINT('Ctrl Pts',(-18.2393302313391,-42.1851162411393,
123.119379879712)) ;
#48738=CARTESIAN_POINT('Ctrl Pts',(-17.9468424318338,-42.0051271607764,
123.046286075553)) ;
#48739=CARTESIAN_POINT('Ctrl Pts',(-18.2062726029867,-42.1951098095885,
123.32682877589)) ;
#48740=CARTESIAN_POINT('Ctrl Pts',(-17.9055231594074,-42.0151207292256,
123.305597710692)) ;
#48741=CARTESIAN_POINT('Ctrl Pts',(-18.2096058519718,-42.2050352803438,
123.53549760296)) ;
#48742=CARTESIAN_POINT('Ctrl Pts',(-17.9096925519482,-42.0250461999809,
123.56643384868)) ;
#48743=CARTESIAN_POINT('Ctrl Pts',(-18.2495067475796,-42.2150629542996,
123.742474063571)) ;
#48744=CARTESIAN_POINT('Ctrl Pts',(-17.9595713839581,-42.0350738739368,
123.825153894762)) ;
#48745=CARTESIAN_POINT('Ctrl Pts',(-18.3235158516873,-42.2249501323413,
123.936741246355)) ;
#48746=CARTESIAN_POINT('Ctrl Pts',(-18.0520856877186,-42.0449610519785,
124.067987197481)) ;
#48747=CARTESIAN_POINT('Ctrl Pts',(-18.4314996605536,-42.2349785117095,
124.117783872996)) ;
#48748=CARTESIAN_POINT('Ctrl Pts',(-18.187066988808,-42.0549894313466,124.294288291678)) ;
#48749=CARTESIAN_POINT('Ctrl Pts',(-18.5673819663472,-42.244872754431,124.27530549087)) ;
#48750=CARTESIAN_POINT('Ctrl Pts',(-18.3569254897191,-42.0648836740681,
124.491191503969)) ;
#48751=CARTESIAN_POINT('Ctrl Pts',(-18.784709731541,-42.2582256710819,124.452982254129)) ;
#48752=CARTESIAN_POINT('Ctrl Pts',(-18.6285705558117,-42.078236590719,124.71326978042)) ;
#48753=CARTESIAN_POINT('Ctrl Pts',(-19.0405785225545,-42.2714281888286,
124.568605528917)) ;
#48754=CARTESIAN_POINT('Ctrl Pts',(-18.948377526286,-42.0914391084657,124.857795814166)) ;
#48755=CARTESIAN_POINT('Ctrl Pts',(-19.3175485571435,-42.2847840941096,
124.614299554858)) ;
#48756=CARTESIAN_POINT('Ctrl Pts',(-19.2946442505059,-42.1047950137467,
124.914924015773)) ;
#48757=CARTESIAN_POINT('Ctrl Pts',(-19.5256323724528,-42.2946807427474,
124.612199384341)) ;
#48758=CARTESIAN_POINT('Ctrl Pts',(-19.5547381910601,-42.1146916623845,
124.912293117139)) ;
#48759=CARTESIAN_POINT('Ctrl Pts',(-19.7332792605488,-42.3047288807999,
124.573491321626)) ;
#48760=CARTESIAN_POINT('Ctrl Pts',(-19.8142993016192,-42.124739800437,124.86390602345)) ;
#48761=CARTESIAN_POINT('Ctrl Pts',(-19.9279820672216,-42.3146198409776,
124.500461827482)) ;
#48762=CARTESIAN_POINT('Ctrl Pts',(-20.0576759368903,-42.1346307606148,
124.772616402038)) ;
#48763=CARTESIAN_POINT('Ctrl Pts',(-20.1091567639837,-42.3246126768544,
124.394101946924)) ;
#48764=CARTESIAN_POINT('Ctrl Pts',(-20.2841432703349,-42.1446235964915,
124.639664036342)) ;
#48765=CARTESIAN_POINT('Ctrl Pts',(-20.2695244297562,-42.334651771856,124.256910080624)) ;
#48766=CARTESIAN_POINT('Ctrl Pts',(-20.4846006078538,-42.1546626914931,
124.468172605259)) ;
#48767=CARTESIAN_POINT('Ctrl Pts',(-20.4013315978798,-42.3444891277071,
124.097515807606)) ;
#48768=CARTESIAN_POINT('Ctrl Pts',(-20.6493590677972,-42.1645000473443,
124.268925825602)) ;
#48769=CARTESIAN_POINT('Ctrl Pts',(-20.5404892382136,-42.3578820756379,
123.852779647777)) ;
#48770=CARTESIAN_POINT('Ctrl Pts',(-20.8232941424064,-42.177892995275,123.963015567167)) ;
#48771=CARTESIAN_POINT('Ctrl Pts',(-20.6114090444013,-42.3710487520648,
123.581847669317)) ;
#48772=CARTESIAN_POINT('Ctrl Pts',(-20.9119427186459,-42.1910596717019,
123.624389608226)) ;
#48773=CARTESIAN_POINT('Ctrl Pts',(-20.6101088531211,-42.3844335334716,
123.300551825487)) ;
#48774=CARTESIAN_POINT('Ctrl Pts',(-20.9103198254801,-42.2044444531087,
123.272710611957)) ;
#48775=CARTESIAN_POINT('Ctrl Pts',(-20.5732425145346,-42.3942953161154,
123.096486655904)) ;
#48776=CARTESIAN_POINT('Ctrl Pts',(-20.8642332429121,-42.2143062357526,
123.017641919768)) ;
#48777=CARTESIAN_POINT('Ctrl Pts',(-20.5008532734841,-42.4042944640685,
122.899177214063)) ;
#48778=CARTESIAN_POINT('Ctrl Pts',(-20.7737441303443,-42.2243053837056,
122.771002649473)) ;
#48779=CARTESIAN_POINT('Ctrl Pts',(-20.3964434183661,-42.4141972566856,
122.719010769963)) ;
#48780=CARTESIAN_POINT('Ctrl Pts',(-20.6432311626779,-42.2342081763227,
122.545797674276)) ;
#48781=CARTESIAN_POINT('Ctrl Pts',(-20.2603721575889,-42.4242468365765,
122.5574632317)) ;
#48782=CARTESIAN_POINT('Ctrl Pts',(-20.4731343577102,-42.2442577562136,
122.343862138749)) ;
#48783=CARTESIAN_POINT('Ctrl Pts',(-20.0479239998599,-42.437433910386,122.379158143776)) ;
#48784=CARTESIAN_POINT('Ctrl Pts',(-20.2076003346992,-42.2574448300231,
122.12099560958)) ;
#48785=CARTESIAN_POINT('Ctrl Pts',(-19.7251865030468,-42.4541867003572,
122.228834167967)) ;
#48786=CARTESIAN_POINT('Ctrl Pts',(-19.8041265873875,-42.2741976199943,
121.933081385993)) ;
#48787=CARTESIAN_POINT('Ctrl Pts',(-19.3757249735959,-42.4706753524519,
122.198219597745)) ;
#48788=CARTESIAN_POINT('Ctrl Pts',(-19.3673812946828,-42.290686272089,121.894819463525)) ;
#48789=CARTESIAN_POINT('Ctrl Pts',(-19.0992014727295,-42.4840321786353,
122.246369143376)) ;
#48790=CARTESIAN_POINT('Ctrl Pts',(-19.0216618585074,-42.3040430982724,
121.955010874022)) ;
#48791=CARTESIAN_POINT('Ctrl Pts',(-18.9034559148771,-42.4939285635132,
122.317028660144)) ;
#48792=CARTESIAN_POINT('Ctrl Pts',(-18.7769948829387,-42.3139394831503,
122.043336388622)) ;
#48793=CARTESIAN_POINT('Ctrl Pts',(-18.7209921103284,-42.5039350780337,
122.42160568978)) ;
#48794=CARTESIAN_POINT('Ctrl Pts',(-18.5489107993243,-42.3239459976708,
122.174062497428)) ;
#48795=CARTESIAN_POINT('Ctrl Pts',(-18.5074778701341,-42.5171252015501,
122.598716946262)) ;
#48796=CARTESIAN_POINT('Ctrl Pts',(-18.2820313956166,-42.3371361211872,
122.395439854909)) ;
#48797=CARTESIAN_POINT('Ctrl Pts',(-18.3017330813565,-42.5338917626996,
122.889684627251)) ;
#48798=CARTESIAN_POINT('Ctrl Pts',(-18.0248416307128,-42.3539026823368,
122.759167368776)) ;
#48799=CARTESIAN_POINT('Ctrl Pts',(-18.1906918477385,-42.5536762514077,
123.295564658477)) ;
#48800=CARTESIAN_POINT('Ctrl Pts',(-17.886048515107,-42.3736871710448,123.266512292216)) ;
#48801=CARTESIAN_POINT('Ctrl Pts',(-18.2237744744841,-42.5736216990041,
123.718259239701)) ;
#48802=CARTESIAN_POINT('Ctrl Pts',(-17.9274046621304,-42.3936326186413,
123.794881011967)) ;
#48803=CARTESIAN_POINT('Ctrl Pts',(-18.3992319347338,-42.5935333611601,
124.103576998798)) ;
#48804=CARTESIAN_POINT('Ctrl Pts',(-18.1467300052869,-42.4135442807972,
124.276525572974)) ;
#48805=CARTESIAN_POINT('Ctrl Pts',(-18.6947270079494,-42.6134255531789,
124.406289323311)) ;
#48806=CARTESIAN_POINT('Ctrl Pts',(-18.5161004763561,-42.4334364728161,
124.654913018434)) ;
#48807=CARTESIAN_POINT('Ctrl Pts',(-19.078800891227,-42.6334666837336,124.590739441501)) ;
#48808=CARTESIAN_POINT('Ctrl Pts',(-18.9961947812989,-42.4534776033707,
124.885472692553)) ;
#48809=CARTESIAN_POINT('Ctrl Pts',(-19.4981893983463,-42.6532850183492,
124.632822667758)) ;
#48810=CARTESIAN_POINT('Ctrl Pts',(-19.5204288936076,-42.4732959379863,
124.938073341943)) ;
#48811=CARTESIAN_POINT('Ctrl Pts',(-19.9098714360872,-42.6732575835688,
124.529182144137)) ;
#48812=CARTESIAN_POINT('Ctrl Pts',(-20.0350303911064,-42.4932685032059,
124.808520139639)) ;
#48813=CARTESIAN_POINT('Ctrl Pts',(-20.2603190889311,-42.6931467997404,
124.292190471673)) ;
#48814=CARTESIAN_POINT('Ctrl Pts',(-20.473087584271,-42.5131577193775,124.512279231662)) ;
#48815=CARTESIAN_POINT('Ctrl Pts',(-20.5101445680897,-42.7131703740631,
123.947568704461)) ;
#48816=CARTESIAN_POINT('Ctrl Pts',(-20.7853676285003,-42.5331812937002,
124.081500341418)) ;
#48817=CARTESIAN_POINT('Ctrl Pts',(-20.6263908959112,-42.7329675371513,
123.542918161152)) ;
#48818=CARTESIAN_POINT('Ctrl Pts',(-20.9306728526506,-42.5529784567885,
123.575689148436)) ;
#48819=CARTESIAN_POINT('Ctrl Pts',(-20.5983617331869,-42.7529330309751,
123.119413546413)) ;
#48820=CARTESIAN_POINT('Ctrl Pts',(-20.8956352696577,-42.5729439506122,
123.046309019479)) ;
#48821=CARTESIAN_POINT('Ctrl Pts',(-20.4270355343715,-42.7728867387165,
122.731150195956)) ;
#48822=CARTESIAN_POINT('Ctrl Pts',(-20.6814765719901,-42.5928976583536,
122.560980844406)) ;
#48823=CARTESIAN_POINT('Ctrl Pts',(-20.1343395660946,-42.7927941154431,
122.425505425646)) ;
#48824=CARTESIAN_POINT('Ctrl Pts',(-20.3156068294175,-42.6128050350802,
122.178926648595)) ;
#48825=CARTESIAN_POINT('Ctrl Pts',(-19.7563159918193,-42.8126463269917,
122.237523332506)) ;
#48826=CARTESIAN_POINT('Ctrl Pts',(-19.8430795028509,-42.6326572466288,
121.943950043858)) ;
#48827=CARTESIAN_POINT('Ctrl Pts',(-19.3322246512801,-42.8327187139374,
122.189721479614)) ;
#48828=CARTESIAN_POINT('Ctrl Pts',(-19.3129641321421,-42.6527296335745,
121.884197616228)) ;
#48829=CARTESIAN_POINT('Ctrl Pts',(-18.9222367590498,-42.8525565835777,
122.288891061449)) ;
#48830=CARTESIAN_POINT('Ctrl Pts',(-18.8004818960636,-42.6725675032148,
122.008159120081)) ;
#48831=CARTESIAN_POINT('Ctrl Pts',(-18.5694696067115,-42.8724072381308,
122.520633431099)) ;
#48832=CARTESIAN_POINT('Ctrl Pts',(-18.3595239816206,-42.6924181577679,
122.297834685126)) ;
#48833=CARTESIAN_POINT('Ctrl Pts',(-18.314918147968,-42.8924591724712,122.862621733189)) ;
#48834=CARTESIAN_POINT('Ctrl Pts',(-18.0413332378271,-42.7124700921084,
122.725319925752)) ;
#48835=CARTESIAN_POINT('Ctrl Pts',(-18.1937042551041,-42.9122923600373,
123.266633949038)) ;
#48836=CARTESIAN_POINT('Ctrl Pts',(-17.8898151802692,-42.7323032796744,
123.230332622468)) ;
#48837=CARTESIAN_POINT('Ctrl Pts',(-18.2168953535135,-42.932221572268,123.689590915752)) ;
#48838=CARTESIAN_POINT('Ctrl Pts',(-17.9188018275413,-42.7522324919051,
123.759028000003)) ;
#48839=CARTESIAN_POINT('Ctrl Pts',(-18.382321733306,-42.9521065374824,124.078869953119)) ;
#48840=CARTESIAN_POINT('Ctrl Pts',(-18.1255818945999,-42.7721174571195,
124.245626671825)) ;
#48841=CARTESIAN_POINT('Ctrl Pts',(-18.6737062137308,-42.972180278627,124.390635608847)) ;
#48842=CARTESIAN_POINT('Ctrl Pts',(-18.4898112910282,-42.7921911982641,
124.635336040243)) ;
#48843=CARTESIAN_POINT('Ctrl Pts',(-19.0487871348763,-42.9919734604074,
124.581662444527)) ;
#48844=CARTESIAN_POINT('Ctrl Pts',(-18.9586591560268,-42.8119843800445,
124.874120892103)) ;
#48845=CARTESIAN_POINT('Ctrl Pts',(-19.4698565957341,-43.0119361684101,
124.634936091618)) ;
#48846=CARTESIAN_POINT('Ctrl Pts',(-19.4849952307029,-42.8319470880472,
124.940716397595)) ;
#48847=CARTESIAN_POINT('Ctrl Pts',(-19.88406254428,-43.0319191201525,124.540216705959)) ;
#48848=CARTESIAN_POINT('Ctrl Pts',(-20.0027532085215,-42.8519300397896,
124.822320272742)) ;
#48849=CARTESIAN_POINT('Ctrl Pts',(-20.2384793849242,-43.0517297399247,
124.312505833384)) ;
#48850=CARTESIAN_POINT('Ctrl Pts',(-20.4457748038711,-42.8717406595618,
124.537685736192)) ;
#48851=CARTESIAN_POINT('Ctrl Pts',(-20.4964670998854,-43.0717134559576,
123.975002267441)) ;
#48852=CARTESIAN_POINT('Ctrl Pts',(-20.7682626054881,-42.8917243755947,
124.115808826861)) ;
#48853=CARTESIAN_POINT('Ctrl Pts',(-20.6231390461281,-43.0915949198549,
123.571582193787)) ;
#48854=CARTESIAN_POINT('Ctrl Pts',(-20.9266062652679,-42.911605839492,123.611535793601)) ;
#48855=CARTESIAN_POINT('Ctrl Pts',(-20.6047789342682,-43.1115502496993,
123.147760811554)) ;
#48856=CARTESIAN_POINT('Ctrl Pts',(-20.9036603572419,-42.9315611693364,
123.081759157368)) ;
#48857=CARTESIAN_POINT('Ctrl Pts',(-20.4437676887391,-43.1314257105047,
122.756956257546)) ;
#48858=CARTESIAN_POINT('Ctrl Pts',(-20.7024014511106,-42.9514366301419,
122.593252469761)) ;
#48859=CARTESIAN_POINT('Ctrl Pts',(-20.1577658156796,-43.1514100305563,
122.442758918448)) ;
#48860=CARTESIAN_POINT('Ctrl Pts',(-20.3449003201343,-42.9714209501934,
122.200502446689)) ;
#48861=CARTESIAN_POINT('Ctrl Pts',(-19.7825309062967,-43.1713380633459,
122.245718411537)) ;
#48862=CARTESIAN_POINT('Ctrl Pts',(-19.8758679528504,-42.991348982983,121.954198379585)) ;
#48863=CARTESIAN_POINT('Ctrl Pts',(-19.4327161765644,-43.1879468252857,
122.19803250865)) ;
#48864=CARTESIAN_POINT('Ctrl Pts',(-19.438573167792,-43.0079577449228,121.894584975642)) ;
#48865=CARTESIAN_POINT('Ctrl Pts',(-19.1575751517247,-43.2011344639758,
122.232458878335)) ;
#48866=CARTESIAN_POINT('Ctrl Pts',(-19.0946716817039,-43.0211453836129,
121.937615803098)) ;
#48867=CARTESIAN_POINT('Ctrl Pts',(-18.9568164762122,-43.2111208983359,
122.29383159449)) ;
#48868=CARTESIAN_POINT('Ctrl Pts',(-18.8437153066299,-43.031131817973,122.014331380066)) ;
#48869=CARTESIAN_POINT('Ctrl Pts',(-18.7693989059073,-43.2211302722953,
122.389560213479)) ;
#48870=CARTESIAN_POINT('Ctrl Pts',(-18.6094527009105,-43.0411411919324,
122.133980200505)) ;
#48871=CARTESIAN_POINT('Ctrl Pts',(-18.5463444276645,-43.2344203058605,
122.557741103274)) ;
#48872=CARTESIAN_POINT('Ctrl Pts',(-18.3305857336724,-43.0544312254977,
122.344252306569)) ;
#48873=CARTESIAN_POINT('Ctrl Pts',(-18.3288675857434,-43.251014293523,122.835683924907)) ;
#48874=CARTESIAN_POINT('Ctrl Pts',(-18.0587919012148,-43.0710252131601,
122.691613440136)) ;
#48875=CARTESIAN_POINT('Ctrl Pts',(-18.2190954075611,-43.2676465487985,
123.171796668551)) ;
#48876=CARTESIAN_POINT('Ctrl Pts',(-17.9215463024505,-43.0876574684357,
123.111805424013)) ;
#48877=CARTESIAN_POINT('Ctrl Pts',(-18.2039836097742,-43.2808889324664,
123.449819348037)) ;
#48878=CARTESIAN_POINT('Ctrl Pts',(-17.9026645543824,-43.1008998521035,
123.459298795023)) ;
#48879=CARTESIAN_POINT('Ctrl Pts',(-18.2283482509571,-43.2908031406938,
123.656820558235)) ;
#48880=CARTESIAN_POINT('Ctrl Pts',(-17.9331154384697,-43.1108140603309,
123.718057560274)) ;
#48881=CARTESIAN_POINT('Ctrl Pts',(-18.289369033941,-43.3008597799655,123.85923089601)) ;
#48882=CARTESIAN_POINT('Ctrl Pts',(-18.0093888248284,-43.1208706996026,
123.971069080689)) ;
#48883=CARTESIAN_POINT('Ctrl Pts',(-18.382402147398,-43.3107055863856,124.044152684337)) ;
#48884=CARTESIAN_POINT('Ctrl Pts',(-18.1256799001394,-43.1307165060227,
124.202224696424)) ;
#48885=CARTESIAN_POINT('Ctrl Pts',(-18.5083351564249,-43.3207505860188,
124.213670912525)) ;
#48886=CARTESIAN_POINT('Ctrl Pts',(-18.2830849970775,-43.1407615056559,
124.414117164475)) ;
#48887=CARTESIAN_POINT('Ctrl Pts',(-18.7114677451612,-43.3340316083915,
124.405150502509)) ;
#48888=CARTESIAN_POINT('Ctrl Pts',(-18.537043251934,-43.1540425280286,124.65350405423)) ;
#48889=CARTESIAN_POINT('Ctrl Pts',(-18.9580635205512,-43.3472290549162,
124.539134994554)) ;
#48890=CARTESIAN_POINT('Ctrl Pts',(-18.8452649773422,-43.1672399745533,
124.820961905211)) ;
#48891=CARTESIAN_POINT('Ctrl Pts',(-19.232360254932,-43.3606433527231,124.60475396977)) ;
#48892=CARTESIAN_POINT('Ctrl Pts',(-19.1881152200042,-43.1806542723603,
124.902985565981)) ;
#48893=CARTESIAN_POINT('Ctrl Pts',(-19.4388332017117,-43.3704824181259,
124.617341847239)) ;
#48894=CARTESIAN_POINT('Ctrl Pts',(-19.4462101896744,-43.190493337763,124.918723959337)) ;
#48895=CARTESIAN_POINT('Ctrl Pts',(-19.6473989067929,-43.3804656244036,
124.594097451494)) ;
#48896=CARTESIAN_POINT('Ctrl Pts',(-19.7069166424415,-43.2004765440407,
124.889671060815)) ;
#48897=CARTESIAN_POINT('Ctrl Pts',(-19.8481271767385,-43.3904168593164,
124.535103924099)) ;
#48898=CARTESIAN_POINT('Ctrl Pts',(-19.9578281238234,-43.2104277789535,
124.815931888651)) ;
#48899=CARTESIAN_POINT('Ctrl Pts',(-20.0366117400743,-43.400417859018,124.441917217521)) ;
#48900=CARTESIAN_POINT('Ctrl Pts',(-20.1934350689946,-43.2204287786551,
124.699450981921)) ;
#48901=CARTESIAN_POINT('Ctrl Pts',(-20.2063611151425,-43.4104492048053,
124.316781602561)) ;
#48902=CARTESIAN_POINT('Ctrl Pts',(-20.4056235278496,-43.2304601244425,
124.543033701341)) ;
#48903=CARTESIAN_POINT('Ctrl Pts',(-20.3494415293354,-43.4203029695104,
124.166967548006)) ;
#48904=CARTESIAN_POINT('Ctrl Pts',(-20.5844761556059,-43.2403138891475,
124.355767995576)) ;
#48905=CARTESIAN_POINT('Ctrl Pts',(-20.4660990695742,-43.4302736231787,
123.992841247419)) ;
#48906=CARTESIAN_POINT('Ctrl Pts',(-20.7303004788071,-43.2502845428158,
124.138111587072)) ;
#48907=CARTESIAN_POINT('Ctrl Pts',(-20.550990914283,-43.4402708668359,123.800540309338)) ;
#48908=CARTESIAN_POINT('Ctrl Pts',(-20.836417878929,-43.260281786473,123.897736472941)) ;
#48909=CARTESIAN_POINT('Ctrl Pts',(-20.6011102529221,-43.4503043227801,
123.595664099876)) ;
#48910=CARTESIAN_POINT('Ctrl Pts',(-20.8990697974022,-43.2703152424172,
123.641641842364)) ;
#48911=CARTESIAN_POINT('Ctrl Pts',(-20.614988288072,-43.4601598270805,123.388915446738)) ;
#48912=CARTESIAN_POINT('Ctrl Pts',(-20.9164201484356,-43.2801707467176,
123.383205983392)) ;
#48913=CARTESIAN_POINT('Ctrl Pts',(-20.5927177301591,-43.4701592633666,
123.179916340754)) ;
#48914=CARTESIAN_POINT('Ctrl Pts',(-20.8885847142338,-43.2901701830037,
123.121956715712)) ;
#48915=CARTESIAN_POINT('Ctrl Pts',(-20.5353148533199,-43.4800537228825,
122.979940150803)) ;
#48916=CARTESIAN_POINT('Ctrl Pts',(-20.8168337005953,-43.3000646425196,
122.871985466953)) ;
#48917=CARTESIAN_POINT('Ctrl Pts',(-20.4424830563002,-43.4901168423341,
122.789877503651)) ;
#48918=CARTESIAN_POINT('Ctrl Pts',(-20.7007964614407,-43.3101277619712,
122.634405971093)) ;
#48919=CARTESIAN_POINT('Ctrl Pts',(-20.3209670354075,-43.4999564767461,
122.622428572666)) ;
#48920=CARTESIAN_POINT('Ctrl Pts',(-20.5489034190072,-43.3199673963832,
122.425092863815)) ;
#48921=CARTESIAN_POINT('Ctrl Pts',(-20.1690754221766,-43.5100196842319,
122.475206765639)) ;
#48922=CARTESIAN_POINT('Ctrl Pts',(-20.3590408300149,-43.330030603869,122.2410636791)) ;
#48923=CARTESIAN_POINT('Ctrl Pts',(-19.9967306491501,-43.5199137916111,
122.358701622462)) ;
#48924=CARTESIAN_POINT('Ctrl Pts',(-20.1436111274021,-43.3399247112482,
122.095429795694)) ;
#48925=CARTESIAN_POINT('Ctrl Pts',(-19.8061253691053,-43.5298561238035,
122.272988374327)) ;
#48926=CARTESIAN_POINT('Ctrl Pts',(-19.9053553865041,-43.3498670434406,
121.988285686092)) ;
#48927=CARTESIAN_POINT('Ctrl Pts',(-19.6023104751595,-43.5398567501185,
122.221256111772)) ;
#48928=CARTESIAN_POINT('Ctrl Pts',(-19.6505873376339,-43.3598676697556,
121.923617759925)) ;
#48929=CARTESIAN_POINT('Ctrl Pts',(-19.3917705372051,-43.5498984844004,
122.206031467105)) ;
#48930=CARTESIAN_POINT('Ctrl Pts',(-19.3874126433953,-43.3699094040375,
121.904584247529)) ;
#48931=CARTESIAN_POINT('Ctrl Pts',(-19.1862281430007,-43.5597239103495,
122.226676883472)) ;
#48932=CARTESIAN_POINT('Ctrl Pts',(-19.1304837624484,-43.3797348299866,
121.930388446646)) ;
#48933=CARTESIAN_POINT('Ctrl Pts',(-18.9826551708029,-43.5697807368771,
122.283706162221)) ;
#48934=CARTESIAN_POINT('Ctrl Pts',(-18.876016923458,-43.3897916565143,122.001672516022)) ;
#48935=CARTESIAN_POINT('Ctrl Pts',(-18.7946320656292,-43.5797081699987,
122.374314662117)) ;
#48936=CARTESIAN_POINT('Ctrl Pts',(-18.6409865992809,-43.3997190896358,
122.114930897131)) ;
#48937=CARTESIAN_POINT('Ctrl Pts',(-18.6244661109234,-43.5896581624049,
122.495982615423)) ;
#48938=CARTESIAN_POINT('Ctrl Pts',(-18.428277440835,-43.4096690820421,122.267013929381)) ;
#48939=CARTESIAN_POINT('Ctrl Pts',(-18.4767445700098,-43.5997133634789,
122.647173613548)) ;
#48940=CARTESIAN_POINT('Ctrl Pts',(-18.2436237169547,-43.4197242831161,
122.456000772691)) ;
#48941=CARTESIAN_POINT('Ctrl Pts',(-18.3599557995264,-43.6095356375312,
122.817488686517)) ;
#48942=CARTESIAN_POINT('Ctrl Pts',(-18.0976352137637,-43.4295465571684,
122.668893815947)) ;
#48943=CARTESIAN_POINT('Ctrl Pts',(-18.2721502560574,-43.6195915314905,
123.009781982913)) ;
#48944=CARTESIAN_POINT('Ctrl Pts',(-17.987876075402,-43.4396024511276,122.909259308021)) ;
#48945=CARTESIAN_POINT('Ctrl Pts',(-18.2200294874752,-43.6295322533356,
123.212171534823)) ;
#48946=CARTESIAN_POINT('Ctrl Pts',(-17.9227225617815,-43.4495431729727,
123.162245934171)) ;
#48947=CARTESIAN_POINT('Ctrl Pts',(-18.2032511636616,-43.6394365974222,
123.419718607872)) ;
#48948=CARTESIAN_POINT('Ctrl Pts',(-17.9017472036595,-43.4594475170593,
123.421680109374)) ;
#48949=CARTESIAN_POINT('Ctrl Pts',(-18.2231767398449,-43.6494832647217,
123.629971456285)) ;
#48950=CARTESIAN_POINT('Ctrl Pts',(-17.926651728431,-43.4694941843588,123.684496298927)) ;
#48951=CARTESIAN_POINT('Ctrl Pts',(-18.2782926714603,-43.6593788231716,
123.830608023793)) ;
#48952=CARTESIAN_POINT('Ctrl Pts',(-17.9955444787495,-43.4793897428087,
123.935293204385)) ;
#48953=CARTESIAN_POINT('Ctrl Pts',(-18.368880857869,-43.6694409018763,124.021733140042)) ;
#48954=CARTESIAN_POINT('Ctrl Pts',(-18.1087774586024,-43.4894518215134,
124.174200467457)) ;
#48955=CARTESIAN_POINT('Ctrl Pts',(-18.4885436290757,-43.6792836003421,
124.19057641474)) ;
#48956=CARTESIAN_POINT('Ctrl Pts',(-18.258354480537,-43.4992945199792,124.38525663974)) ;
#48957=CARTESIAN_POINT('Ctrl Pts',(-18.637534073092,-43.6892743742365,124.338585277532)) ;
#48958=CARTESIAN_POINT('Ctrl Pts',(-18.4445910638163,-43.5092852938737,
124.570269448432)) ;
#48959=CARTESIAN_POINT('Ctrl Pts',(-18.8089243606345,-43.6992022434715,
124.457711598807)) ;
#48960=CARTESIAN_POINT('Ctrl Pts',(-18.6588280253988,-43.5192131631086,
124.719179491474)) ;
#48961=CARTESIAN_POINT('Ctrl Pts',(-18.9994025238417,-43.7091909724413,
124.546144010481)) ;
#48962=CARTESIAN_POINT('Ctrl Pts',(-18.8969249830435,-43.5292018920784,
124.829722059016)) ;
#48963=CARTESIAN_POINT('Ctrl Pts',(-19.2034513375471,-43.7192303744251,
124.600051021114)) ;
#48964=CARTESIAN_POINT('Ctrl Pts',(-19.1519853155007,-43.5392412940622,
124.897107996918)) ;
#48965=CARTESIAN_POINT('Ctrl Pts',(-19.4095740593302,-43.7290705421618,
124.617767680818)) ;
#48966=CARTESIAN_POINT('Ctrl Pts',(-19.4096395220042,-43.549081461799,124.91925607013)) ;
#48967=CARTESIAN_POINT('Ctrl Pts',(-19.6200056310843,-43.7391187525363,
124.599348020896)) ;
#48968=CARTESIAN_POINT('Ctrl Pts',(-19.6726790143965,-43.5591296721735,
124.896233588286)) ;
#48969=CARTESIAN_POINT('Ctrl Pts',(-19.8219167217474,-43.7490659228241,
124.544896993531)) ;
#48970=CARTESIAN_POINT('Ctrl Pts',(-19.9250688422305,-43.5690768424612,
124.828171804027)) ;
#48971=CARTESIAN_POINT('Ctrl Pts',(-20.0108816230602,-43.7589767710792,
124.457103125973)) ;
#48972=CARTESIAN_POINT('Ctrl Pts',(-20.1612764162791,-43.5789876907163,
124.718431010593)) ;
#48973=CARTESIAN_POINT('Ctrl Pts',(-20.1841105037693,-43.7690330987569,
124.335929383685)) ;
#48974=CARTESIAN_POINT('Ctrl Pts',(-20.3778135163567,-43.5890440183941,
124.566965650242)) ;
#48975=CARTESIAN_POINT('Ctrl Pts',(-20.3307480730598,-43.7788835115255,
124.189689219311)) ;
#48976=CARTESIAN_POINT('Ctrl Pts',(-20.561112631005,-43.5988944311626,124.384166137477)) ;
#48977=CARTESIAN_POINT('Ctrl Pts',(-20.4523107242859,-43.7889103973592,
124.017478146335)) ;
#48978=CARTESIAN_POINT('Ctrl Pts',(-20.7130674436225,-43.6089213169963,
124.168903399289)) ;
#48979=CARTESIAN_POINT('Ctrl Pts',(-20.5416506384017,-43.79893901299,123.826498737951)) ;
#48980=CARTESIAN_POINT('Ctrl Pts',(-20.8247441401648,-43.6189499326271,
123.930180059024)) ;
#48981=CARTESIAN_POINT('Ctrl Pts',(-20.5958423754753,-43.8087842363675,
123.626753384018)) ;
#48982=CARTESIAN_POINT('Ctrl Pts',(-20.8924859435401,-43.6287951560046,
123.680497788512)) ;
#48983=CARTESIAN_POINT('Ctrl Pts',(-20.6153678869501,-43.8187749184691,
123.417621815396)) ;
#48984=CARTESIAN_POINT('Ctrl Pts',(-20.9168945752152,-43.6387858381062,
123.419083293922)) ;
#48985=CARTESIAN_POINT('Ctrl Pts',(-20.5977356287722,-43.8288128071015,
123.207333737344)) ;
#48986=CARTESIAN_POINT('Ctrl Pts',(-20.8948561360059,-43.6488237267386,
123.156223171646)) ;
#48987=CARTESIAN_POINT('Ctrl Pts',(-20.5452446975445,-43.8386571422047,
123.007134061094)) ;
#48988=CARTESIAN_POINT('Ctrl Pts',(-20.8292438813552,-43.6586680618418,
122.905971997117)) ;
#48989=CARTESIAN_POINT('Ctrl Pts',(-20.4579454357753,-43.8486421044022,
122.816264363838)) ;
#48990=CARTESIAN_POINT('Ctrl Pts',(-20.7201211840109,-43.6686530240393,
122.667383970185)) ;
#48991=CARTESIAN_POINT('Ctrl Pts',(-20.3394267685731,-43.8585810459356,
122.644144630097)) ;
#48992=CARTESIAN_POINT('Ctrl Pts',(-20.5719738572654,-43.6785919655727,
122.452232949088)) ;
#48993=CARTESIAN_POINT('Ctrl Pts',(-20.1912921885784,-43.868622930907,122.493758530072)) ;
#48994=CARTESIAN_POINT('Ctrl Pts',(-20.3868068904669,-43.6886338505441,
122.264249292356)) ;
#48995=CARTESIAN_POINT('Ctrl Pts',(-20.0220013238299,-43.8785094788153,
122.373139062939)) ;
#48996=CARTESIAN_POINT('Ctrl Pts',(-20.1751934660884,-43.6985203984524,
122.113473137318)) ;
#48997=CARTESIAN_POINT('Ctrl Pts',(-19.8324762444945,-43.8885034043153,
122.282516116147)) ;
#48998=CARTESIAN_POINT('Ctrl Pts',(-19.9382875919748,-43.7085143239524,
122.000193047115)) ;
#48999=CARTESIAN_POINT('Ctrl Pts',(-19.6312362520306,-43.8984394954417,
122.226393147008)) ;
#49000=CARTESIAN_POINT('Ctrl Pts',(-19.6867374287566,-43.7184504150789,
121.930037797555)) ;
#49001=CARTESIAN_POINT('Ctrl Pts',(-19.4214139020312,-43.9084687644217,
122.205920422731)) ;
#49002=CARTESIAN_POINT('Ctrl Pts',(-19.4244597082895,-43.7284796840588,
121.904445450491)) ;
#49003=CARTESIAN_POINT('Ctrl Pts',(-19.2142240963958,-43.918351146981,122.221693374748)) ;
#49004=CARTESIAN_POINT('Ctrl Pts',(-19.1654713412245,-43.7383620666181,
121.924160359803)) ;
#49005=CARTESIAN_POINT('Ctrl Pts',(-19.009498669417,-43.9284036640689,122.274004896839)) ;
#49006=CARTESIAN_POINT('Ctrl Pts',(-18.909564469388,-43.748414583706,121.989548406113)) ;
#49007=CARTESIAN_POINT('Ctrl Pts',(-18.819892626088,-43.9382977848928,122.359628820028)) ;
#49008=CARTESIAN_POINT('Ctrl Pts',(-18.672555542748,-43.7583087045299,122.096577505371)) ;
#49009=CARTESIAN_POINT('Ctrl Pts',(-18.6451418431221,-43.9483597643132,
122.478785235648)) ;
#49010=CARTESIAN_POINT('Ctrl Pts',(-18.4541166120411,-43.7683706839503,
122.245521781435)) ;
#49011=CARTESIAN_POINT('Ctrl Pts',(-18.4969665742692,-43.9582042975421,
122.623287056138)) ;
#49012=CARTESIAN_POINT('Ctrl Pts',(-18.2688956918944,-43.7782152171792,
122.426149066543)) ;
#49013=CARTESIAN_POINT('Ctrl Pts',(-18.3741086579576,-43.9681643764484,
122.792844278905)) ;
#49014=CARTESIAN_POINT('Ctrl Pts',(-18.1153222214896,-43.7881752960855,
122.63809537997)) ;
#49015=CARTESIAN_POINT('Ctrl Pts',(-18.2822146957173,-43.978202653021,122.982811873734)) ;
#49016=CARTESIAN_POINT('Ctrl Pts',(-18.0004538039104,-43.7982135726581,
122.875554226971)) ;
#49017=CARTESIAN_POINT('Ctrl Pts',(-18.2252522008148,-43.9880760395588,
123.182444364765)) ;
#49018=CARTESIAN_POINT('Ctrl Pts',(-17.9292494152414,-43.8080869591959,
123.125095646778)) ;
#49019=CARTESIAN_POINT('Ctrl Pts',(-18.2034535742499,-43.9981489823259,
123.393043925117)) ;
#49020=CARTESIAN_POINT('Ctrl Pts',(-17.902000155212,-43.818159901963,123.388344568531)) ;
#49021=CARTESIAN_POINT('Ctrl Pts',(-18.2179298683599,-44.0079703964542,
123.599052536948)) ;
#49022=CARTESIAN_POINT('Ctrl Pts',(-17.9200947062017,-43.8279813160913,
123.645856942376)) ;
#49023=CARTESIAN_POINT('Ctrl Pts',(-18.2689797272042,-44.0180450265265,
123.804569296683)) ;
#49024=CARTESIAN_POINT('Ctrl Pts',(-17.9839061111706,-43.8380559461636,
123.902752660032)) ;
#49025=CARTESIAN_POINT('Ctrl Pts',(-18.3532690236661,-44.0279116638434,
123.994127168066)) ;
#49026=CARTESIAN_POINT('Ctrl Pts',(-18.0892674357171,-43.8479225834805,
124.139701464723)) ;
#49027=CARTESIAN_POINT('Ctrl Pts',(-18.4705660574724,-44.0379352092152,
124.169178578053)) ;
#49028=CARTESIAN_POINT('Ctrl Pts',(-18.2358881550822,-43.8579461288523,
124.358516056916)) ;
#49029=CARTESIAN_POINT('Ctrl Pts',(-18.6168901850746,-44.0479609607324,
124.320901604425)) ;
#49030=CARTESIAN_POINT('Ctrl Pts',(-18.4187926357899,-43.8679718803695,
124.54817037461)) ;
#49031=CARTESIAN_POINT('Ctrl Pts',(-18.7841854234927,-44.0578145477417,
124.443049390508)) ;
#49032=CARTESIAN_POINT('Ctrl Pts',(-18.6279123309116,-43.8778254673789,
124.700856473428)) ;
#49033=CARTESIAN_POINT('Ctrl Pts',(-18.9722447032616,-44.0677915079697,
124.535943542531)) ;
#49034=CARTESIAN_POINT('Ctrl Pts',(-18.8629865023443,-43.8878024276068,
124.816974766263)) ;
#49035=CARTESIAN_POINT('Ctrl Pts',(-19.1745538584046,-44.0778126509981,
124.594687633836)) ;
#49036=CARTESIAN_POINT('Ctrl Pts',(-19.1158727506149,-43.8978235706353,
124.890405499117)) ;
#49037=CARTESIAN_POINT('Ctrl Pts',(-19.3810867415163,-44.0876952570181,
124.617517604128)) ;
#49038=CARTESIAN_POINT('Ctrl Pts',(-19.3740398930884,-43.9077061766552,
124.918943559724)) ;
#49039=CARTESIAN_POINT('Ctrl Pts',(-19.5922777528914,-44.0977637276508,
124.603809178215)) ;
#49040=CARTESIAN_POINT('Ctrl Pts',(-19.6380282810842,-43.9177746472879,
124.901808568913)) ;
#49041=CARTESIAN_POINT('Ctrl Pts',(-19.7931371162424,-44.1075938108345,
124.555043900469)) ;
#49042=CARTESIAN_POINT('Ctrl Pts',(-19.889104080618,-43.9276047304716,124.840852015822)) ;
#49043=CARTESIAN_POINT('Ctrl Pts',(-19.9870797834277,-44.1176603705148,
124.470429298828)) ;
#49044=CARTESIAN_POINT('Ctrl Pts',(-20.1315321754818,-43.937671290152,124.735084209406)) ;
#49045=CARTESIAN_POINT('Ctrl Pts',(-20.1602737104804,-44.1275506203441,
124.355334521144)) ;
#49046=CARTESIAN_POINT('Ctrl Pts',(-20.3480256593167,-43.9475615399812,
124.591215461382)) ;
#49047=CARTESIAN_POINT('Ctrl Pts',(-20.3126945664649,-44.1375427860929,
124.210797364723)) ;
#49048=CARTESIAN_POINT('Ctrl Pts',(-20.5385520107773,-43.95755370573,124.41054400151)) ;
#49049=CARTESIAN_POINT('Ctrl Pts',(-20.4371805511039,-44.147505629689,124.042362117162)) ;
#49050=CARTESIAN_POINT('Ctrl Pts',(-20.6941599747678,-43.9675165493261,
124.199999732193)) ;
#49051=CARTESIAN_POINT('Ctrl Pts',(-20.5304651406943,-44.1574097985167,
123.856190907026)) ;
#49052=CARTESIAN_POINT('Ctrl Pts',(-20.8107661786076,-43.9774207181539,
123.967284902334)) ;
#49053=CARTESIAN_POINT('Ctrl Pts',(-20.5907535668492,-44.1674706734111,
123.653482764697)) ;
#49054=CARTESIAN_POINT('Ctrl Pts',(-20.8861267321908,-43.9874815930482,
123.713900101275)) ;
#49055=CARTESIAN_POINT('Ctrl Pts',(-20.6146904777119,-44.1773095767404,
123.447994903833)) ;
#49056=CARTESIAN_POINT('Ctrl Pts',(-20.9160480543138,-43.9973204963776,
123.457038808334)) ;
#49057=CARTESIAN_POINT('Ctrl Pts',(-20.6025093175598,-44.1873779531143,
123.236711105022)) ;
#49058=CARTESIAN_POINT('Ctrl Pts',(-20.9008215569112,-44.0073888727515,
123.192934464757)) ;
#49059=CARTESIAN_POINT('Ctrl Pts',(-20.5546520539257,-44.197258569747,123.034546463508)) ;
#49060=CARTESIAN_POINT('Ctrl Pts',(-20.8409996767229,-44.0172694893841,
122.940227571329)) ;
#49061=CARTESIAN_POINT('Ctrl Pts',(-20.4719127587511,-44.207249729976,122.841516718461)) ;
#49062=CARTESIAN_POINT('Ctrl Pts',(-20.7375752826336,-44.0272606496131,
122.698940269794)) ;
#49063=CARTESIAN_POINT('Ctrl Pts',(-20.3573466961592,-44.2172028034081,
122.666384942682)) ;
#49064=CARTESIAN_POINT('Ctrl Pts',(-20.5943672382838,-44.0372137230452,
122.480025241818)) ;
#49065=CARTESIAN_POINT('Ctrl Pts',(-20.2129041498641,-44.2272386390207,
122.512619796291)) ;
#49066=CARTESIAN_POINT('Ctrl Pts',(-20.413814021043,-44.0472495586578,122.28781904818)) ;
#49067=CARTESIAN_POINT('Ctrl Pts',(-20.0464710387891,-44.2371287657509,
122.387973352536)) ;
#49068=CARTESIAN_POINT('Ctrl Pts',(-20.2057716275745,-44.057139685388,122.132010547474)) ;
#49069=CARTESIAN_POINT('Ctrl Pts',(-19.8591825427843,-44.2471209475202,
122.292859773078)) ;
#49070=CARTESIAN_POINT('Ctrl Pts',(-19.9716606492844,-44.0671318671573,
122.013118819397)) ;
#49071=CARTESIAN_POINT('Ctrl Pts',(-19.6591233355574,-44.2570668874946,
122.232057906524)) ;
#49072=CARTESIAN_POINT('Ctrl Pts',(-19.721585969689,-44.0770778071318,121.93711664901)) ;
#49073=CARTESIAN_POINT('Ctrl Pts',(-19.4515603480813,-44.2670140712541,
122.206490694919)) ;
#49074=CARTESIAN_POINT('Ctrl Pts',(-19.4621316011703,-44.0870249908912,
121.905158079447)) ;
#49075=CARTESIAN_POINT('Ctrl Pts',(-19.2406254966303,-44.2770620095444,
122.217696911722)) ;
#49076=CARTESIAN_POINT('Ctrl Pts',(-19.1984633098486,-44.0970729291816,
121.91916626143)) ;
#49077=CARTESIAN_POINT('Ctrl Pts',(-19.0388958129296,-44.286909644358,122.264239155619)) ;
#49078=CARTESIAN_POINT('Ctrl Pts',(-18.9462999517132,-44.1069205639951,
121.977344862777)) ;
#49079=CARTESIAN_POINT('Ctrl Pts',(-18.8458583821311,-44.296871358056,122.345428988857)) ;
#49080=CARTESIAN_POINT('Ctrl Pts',(-18.7050030349617,-44.1168822776931,
122.078833023626)) ;
#49081=CARTESIAN_POINT('Ctrl Pts',(-18.6687933154075,-44.3068999938771,
122.459902791905)) ;
#49082=CARTESIAN_POINT('Ctrl Pts',(-18.4836721334991,-44.1269109135143,
122.221925767037)) ;
#49083=CARTESIAN_POINT('Ctrl Pts',(-18.5160880962946,-44.3168103086289,
122.601623849684)) ;
#49084=CARTESIAN_POINT('Ctrl Pts',(-18.2927904240574,-44.136821228266,122.39907817817)) ;
#49085=CARTESIAN_POINT('Ctrl Pts',(-18.3895506603922,-44.3267451792916,
122.767800295044)) ;
#49086=CARTESIAN_POINT('Ctrl Pts',(-18.1346189321038,-44.1467560989287,
122.60679979726)) ;
#49087=CARTESIAN_POINT('Ctrl Pts',(-18.2929514113174,-44.3367863616933,
122.955488189601)) ;
#49088=CARTESIAN_POINT('Ctrl Pts',(-18.0138706731733,-44.1567972813305,
122.841409864127)) ;
#49089=CARTESIAN_POINT('Ctrl Pts',(-18.2312003577601,-44.3466733331581,
123.153977478668)) ;
#49090=CARTESIAN_POINT('Ctrl Pts',(-17.9366823755265,-44.1666842527952,
123.089522740013)) ;
#49091=CARTESIAN_POINT('Ctrl Pts',(-18.2042924362549,-44.3566727654207,
123.362440492209)) ;
#49092=CARTESIAN_POINT('Ctrl Pts',(-17.903048419426,-44.1766836850578,123.350101781409)) ;
#49093=CARTESIAN_POINT('Ctrl Pts',(-18.2137740339436,-44.3665928306773,
123.5708007757)) ;
#49094=CARTESIAN_POINT('Ctrl Pts',(-17.9149014701427,-44.1866037503144,
123.610552838708)) ;
#49095=CARTESIAN_POINT('Ctrl Pts',(-18.2597764971867,-44.3766296832615,
123.776719598034)) ;
#49096=CARTESIAN_POINT('Ctrl Pts',(-17.9724055290717,-44.1966406028986,
123.867950986159)) ;
#49097=CARTESIAN_POINT('Ctrl Pts',(-18.3398426561002,-44.3865423426014,
123.969124187214)) ;
#49098=CARTESIAN_POINT('Ctrl Pts',(-18.072489495965,-44.2065532622386,124.10845708331)) ;
#49099=CARTESIAN_POINT('Ctrl Pts',(-18.4526095787518,-44.3965335545164,
124.146348677994)) ;
#49100=CARTESIAN_POINT('Ctrl Pts',(-18.2134492761814,-44.2165444741535,
124.329987229818)) ;
#49101=CARTESIAN_POINT('Ctrl Pts',(-18.5954817229628,-44.4065751959195,
124.301740665686)) ;
#49102=CARTESIAN_POINT('Ctrl Pts',(-18.3920400927921,-44.2265861155566,
124.524226386298)) ;
#49103=CARTESIAN_POINT('Ctrl Pts',(-18.7593291885529,-44.4164039901265,
124.427686436395)) ;
#49104=CARTESIAN_POINT('Ctrl Pts',(-18.5968513118657,-44.2364149097636,
124.681658511536)) ;
#49105=CARTESIAN_POINT('Ctrl Pts',(-18.9470682784548,-44.4264804012478,
124.525725017682)) ;
#49106=CARTESIAN_POINT('Ctrl Pts',(-18.8315253713429,-44.2464913208849,
124.804205426187)) ;
#49107=CARTESIAN_POINT('Ctrl Pts',(-19.1445330347221,-44.4363325342902,
124.588381426749)) ;
#49108=CARTESIAN_POINT('Ctrl Pts',(-19.0783578845555,-44.2563434539274,
124.882525081973)) ;
#49109=CARTESIAN_POINT('Ctrl Pts',(-19.3543837050247,-44.4464057686315,
124.616582421442)) ;
#49110=CARTESIAN_POINT('Ctrl Pts',(-19.3406710042076,-44.2664166882687,
124.917774928891)) ;
#49111=CARTESIAN_POINT('Ctrl Pts',(-19.561120757118,-44.4562472699582,124.608057607434)) ;
#49112=CARTESIAN_POINT('Ctrl Pts',(-19.5990935689742,-44.2762581895953,
124.907117526406)) ;
#49113=CARTESIAN_POINT('Ctrl Pts',(-19.7658378555304,-44.466208221553,124.564003318983)) ;
#49114=CARTESIAN_POINT('Ctrl Pts',(-19.8549900005199,-44.2862191411901,
124.852048007979)) ;
#49115=CARTESIAN_POINT('Ctrl Pts',(-19.9611338445933,-44.4762460392736,
124.484072288273)) ;
#49116=CARTESIAN_POINT('Ctrl Pts',(-20.0991093096047,-44.2962569589108,
124.752132918042)) ;
#49117=CARTESIAN_POINT('Ctrl Pts',(-20.1369108495217,-44.4861203885307,
124.373589262142)) ;
#49118=CARTESIAN_POINT('Ctrl Pts',(-20.3188305768388,-44.3061313081678,
124.61402724624)) ;
#49119=CARTESIAN_POINT('Ctrl Pts',(-20.2938275249447,-44.4961899392729,
124.231536291723)) ;
#49120=CARTESIAN_POINT('Ctrl Pts',(-20.5149750943613,-44.31620085891,124.436460091646)) ;
#49121=CARTESIAN_POINT('Ctrl Pts',(-20.4207811078669,-44.5060239587815,
124.068339987398)) ;
#49122=CARTESIAN_POINT('Ctrl Pts',(-20.6736665782886,-44.3260348784186,
124.232462693714)) ;
#49123=CARTESIAN_POINT('Ctrl Pts',(-20.5199150721139,-44.516058113361,123.882148162082)) ;
#49124=CARTESIAN_POINT('Ctrl Pts',(-20.7975823820433,-44.3360690329981,
123.999722159393)) ;
#49125=CARTESIAN_POINT('Ctrl Pts',(-20.5846066652837,-44.5260740391835,
123.68175257298)) ;
#49126=CARTESIAN_POINT('Ctrl Pts',(-20.8784453196383,-44.3460849588206,
123.749227159064)) ;
#49127=CARTESIAN_POINT('Ctrl Pts',(-20.6135027473333,-44.5359562943777,
123.476012739199)) ;
#49128=CARTESIAN_POINT('Ctrl Pts',(-20.914563804666,-44.3559672140149,123.492051220715)) ;
#49129=CARTESIAN_POINT('Ctrl Pts',(-20.6064192234333,-44.5459451008887,
123.266159254011)) ;
#49130=CARTESIAN_POINT('Ctrl Pts',(-20.9057075528016,-44.3659560205258,
123.229734225039)) ;
#49131=CARTESIAN_POINT('Ctrl Pts',(-20.5633248096925,-44.5558936681514,
123.061463359673)) ;
#49132=CARTESIAN_POINT('Ctrl Pts',(-20.8518375941005,-44.3759045877885,
122.973864298052)) ;
#49133=CARTESIAN_POINT('Ctrl Pts',(-20.4843220668197,-44.5659484734534,
122.865422401674)) ;
#49134=CARTESIAN_POINT('Ctrl Pts',(-20.7530825570645,-44.3859593930905,
122.728813985344)) ;
#49135=CARTESIAN_POINT('Ctrl Pts',(-20.3753421768984,-44.575767256717,122.69010150794)) ;
#49136=CARTESIAN_POINT('Ctrl Pts',(-20.616855401469,-44.3957781763541,122.509662800884)) ;
#49137=CARTESIAN_POINT('Ctrl Pts',(-20.2349634944572,-44.5858030290775,
122.532602841201)) ;
#49138=CARTESIAN_POINT('Ctrl Pts',(-20.4413805689007,-44.4058139487147,
122.312790934125)) ;
#49139=CARTESIAN_POINT('Ctrl Pts',(-20.0691703030276,-44.5958277281062,
122.402480939027)) ;
#49140=CARTESIAN_POINT('Ctrl Pts',(-20.2341379246685,-44.4158386477433,
122.150140067367)) ;
#49141=CARTESIAN_POINT('Ctrl Pts',(-19.8867241174746,-44.6056797313652,
122.304432926397)) ;
#49142=CARTESIAN_POINT('Ctrl Pts',(-20.0060783372853,-44.4256906510024,
122.027581366541)) ;
#49143=CARTESIAN_POINT('Ctrl Pts',(-19.6873786654677,-44.6156706657625,
122.238342902669)) ;
#49144=CARTESIAN_POINT('Ctrl Pts',(-19.7568956897588,-44.4356815853996,
121.944970803461)) ;
#49145=CARTESIAN_POINT('Ctrl Pts',(-19.481074169139,-44.6255885881936,122.207949395056)) ;
#49146=CARTESIAN_POINT('Ctrl Pts',(-19.4990141869541,-44.4455995078307,
121.906980973465)) ;
#49147=CARTESIAN_POINT('Ctrl Pts',(-19.2703469798628,-44.6356169438759,
122.213857027712)) ;
#49148=CARTESIAN_POINT('Ctrl Pts',(-19.2356052976764,-44.455627863513,121.914367687928)) ;
#49149=CARTESIAN_POINT('Ctrl Pts',(-19.0667685393293,-44.6455012283865,
122.255560649441)) ;
#49150=CARTESIAN_POINT('Ctrl Pts',(-18.9811319610234,-44.4655121480236,
121.966499520298)) ;
#49151=CARTESIAN_POINT('Ctrl Pts',(-18.8712365177251,-44.6554939122944,
122.332371985697)) ;
#49152=CARTESIAN_POINT('Ctrl Pts',(-18.7367176525546,-44.4755048319315,
122.06251590164)) ;
#49153=CARTESIAN_POINT('Ctrl Pts',(-18.6915565635913,-44.6655226493021,
122.442678617086)) ;
#49154=CARTESIAN_POINT('Ctrl Pts',(-18.5121188960608,-44.4855335689392,
122.20040107881)) ;
#49155=CARTESIAN_POINT('Ctrl Pts',(-18.5358279806812,-44.675408045931,122.580307301666)) ;
#49156=CARTESIAN_POINT('Ctrl Pts',(-18.3174591681186,-44.4954189655681,
122.372439116343)) ;
#49157=CARTESIAN_POINT('Ctrl Pts',(-18.4048030817091,-44.6853959313449,
122.74436173368)) ;
#49158=CARTESIAN_POINT('Ctrl Pts',(-18.1536797930773,-44.505406850982,122.577508760622)) ;
#49159=CARTESIAN_POINT('Ctrl Pts',(-18.3045194431609,-44.6953466340055,
122.927987236834)) ;
#49160=CARTESIAN_POINT('Ctrl Pts',(-18.0283271818904,-44.5153575536426,
122.807042074314)) ;
#49161=CARTESIAN_POINT('Ctrl Pts',(-18.2371653977238,-44.7053869521029,
123.128009185341)) ;
#49162=CARTESIAN_POINT('Ctrl Pts',(-17.9441368874462,-44.52539787174,123.057070192369)) ;
#49163=CARTESIAN_POINT('Ctrl Pts',(-18.2058765293099,-44.7152615174361,
123.333255667552)) ;
#49164=CARTESIAN_POINT('Ctrl Pts',(-17.9050280766287,-44.5352724370732,
123.313629339727)) ;
#49165=CARTESIAN_POINT('Ctrl Pts',(-18.2104928246588,-44.7252611774972,
123.543394996734)) ;
#49166=CARTESIAN_POINT('Ctrl Pts',(-17.9108009163294,-44.5452720971343,
123.576303554644)) ;
#49167=CARTESIAN_POINT('Ctrl Pts',(-18.2509713151308,-44.7351701726649,
123.747780176754)) ;
#49168=CARTESIAN_POINT('Ctrl Pts',(-17.9614015776546,-44.555181092302,123.831785012484)) ;
#49169=CARTESIAN_POINT('Ctrl Pts',(-18.3274676749511,-44.7452249138281,
123.944798878115)) ;
#49170=CARTESIAN_POINT('Ctrl Pts',(-18.0570243118767,-44.5652358334653,
124.078057381489)) ;
#49171=CARTESIAN_POINT('Ctrl Pts',(-18.4347054519244,-44.7550835257419,
124.122200708846)) ;
#49172=CARTESIAN_POINT('Ctrl Pts',(-18.1910740418543,-44.5750944453791,
124.299808917657)) ;
#49173=CARTESIAN_POINT('Ctrl Pts',(-18.5738749657264,-44.7651516480213,
124.281638187706)) ;
#49174=CARTESIAN_POINT('Ctrl Pts',(-18.3650377633451,-44.5851625676584,
124.499103963352)) ;
#49175=CARTESIAN_POINT('Ctrl Pts',(-18.7351819980848,-44.7750071187245,
124.411700343814)) ;
#49176=CARTESIAN_POINT('Ctrl Pts',(-18.5666736485935,-44.5950180383616,
124.661680062319)) ;
#49177=CARTESIAN_POINT('Ctrl Pts',(-18.9188616429352,-44.7850019782178,
124.513733292732)) ;
#49178=CARTESIAN_POINT('Ctrl Pts',(-18.7962745857909,-44.605012897855,124.789218966965)) ;
#49179=CARTESIAN_POINT('Ctrl Pts',(-19.1183492113281,-44.7950332315598,
124.58214803004)) ;
#49180=CARTESIAN_POINT('Ctrl Pts',(-19.0456348868395,-44.6150441511969,
124.874734939455)) ;
#49181=CARTESIAN_POINT('Ctrl Pts',(-19.323218690417,-44.8048999304329,124.61467366931)) ;
#49182=CARTESIAN_POINT('Ctrl Pts',(-19.3017226630708,-44.62491085007,124.915389460278)) ;
#49183=CARTESIAN_POINT('Ctrl Pts',(-19.5331246188192,-44.8148867461841,
124.61143594484)) ;
#49184=CARTESIAN_POINT('Ctrl Pts',(-19.5641051552104,-44.6348976658212,
124.911339609303)) ;
#49185=CARTESIAN_POINT('Ctrl Pts',(-19.7385308241501,-44.8248339513795,
124.572042427275)) ;
#49186=CARTESIAN_POINT('Ctrl Pts',(-19.8208626335505,-44.6448448710167,
124.862095013778)) ;
#49187=CARTESIAN_POINT('Ctrl Pts',(-19.9357852330403,-44.8348769395058,
124.496793289442)) ;
#49188=CARTESIAN_POINT('Ctrl Pts',(-20.0674296681808,-44.6548878591429,
124.76803108169)) ;
#49189=CARTESIAN_POINT('Ctrl Pts',(-20.1138908734245,-44.8447442941273,
124.39042646345)) ;
#49190=CARTESIAN_POINT('Ctrl Pts',(-20.2900606909374,-44.6647552137644,
124.635070010698)) ;
#49191=CARTESIAN_POINT('Ctrl Pts',(-20.2727462782933,-44.8547101874254,
124.25383373658)) ;
#49192=CARTESIAN_POINT('Ctrl Pts',(-20.4886282483647,-44.6747211070625,
124.464326907893)) ;
#49193=CARTESIAN_POINT('Ctrl Pts',(-20.4060875110616,-44.8647339648015,
124.090636353554)) ;
#49194=CARTESIAN_POINT('Ctrl Pts',(-20.6553026894128,-44.6847448844386,
124.260328412907)) ;
#49195=CARTESIAN_POINT('Ctrl Pts',(-20.5080877736395,-44.8746595127332,
123.908610854612)) ;
#49196=CARTESIAN_POINT('Ctrl Pts',(-20.7828007334005,-44.6946704323703,
124.032794984382)) ;
#49197=CARTESIAN_POINT('Ctrl Pts',(-20.5775102693516,-44.8845999891542,
123.711485460031)) ;
#49198=CARTESIAN_POINT('Ctrl Pts',(-20.8695762747895,-44.7046109087913,
123.786387153745)) ;
#49199=CARTESIAN_POINT('Ctrl Pts',(-20.6117719571326,-44.8946461988171,
123.503092758623)) ;
#49200=CARTESIAN_POINT('Ctrl Pts',(-20.912400649323,-44.7146571184542,123.525895807852)) ;
#49201=CARTESIAN_POINT('Ctrl Pts',(-20.6095960962421,-44.9045074554789,
123.295771336016)) ;
#49202=CARTESIAN_POINT('Ctrl Pts',(-20.9096780311405,-44.724518375116,123.26674378884)) ;
#49203=CARTESIAN_POINT('Ctrl Pts',(-20.5713071076348,-44.9145010837542,
123.08922311595)) ;
#49204=CARTESIAN_POINT('Ctrl Pts',(-20.8618140135343,-44.7345120033913,
123.008558951118)) ;
#49205=CARTESIAN_POINT('Ctrl Pts',(-20.4983191373996,-44.9244264810644,
122.893708018613)) ;
#49206=CARTESIAN_POINT('Ctrl Pts',(-20.7705763697433,-44.7444374007015,
122.764165937578)) ;
#49207=CARTESIAN_POINT('Ctrl Pts',(-20.391433863342,-44.9344543889746,122.712025942917)) ;
#49208=CARTESIAN_POINT('Ctrl Pts',(-20.6369673169243,-44.7544653086117,
122.537064718162)) ;
#49209=CARTESIAN_POINT('Ctrl Pts',(-20.2566836205498,-44.9443407046438,
122.55374389634)) ;
#49210=CARTESIAN_POINT('Ctrl Pts',(-20.4685272889073,-44.7643516242809,
122.33921389434)) ;
#49211=CARTESIAN_POINT('Ctrl Pts',(-20.0942650307571,-44.9543722995476,
122.419270807689)) ;
#49212=CARTESIAN_POINT('Ctrl Pts',(-20.2655021977993,-44.7743832191847,
122.171124667766)) ;
#49213=CARTESIAN_POINT('Ctrl Pts',(-19.9137299172441,-44.9642545424993,
122.316394133528)) ;
#49214=CARTESIAN_POINT('Ctrl Pts',(-20.0398318506451,-44.7842654621364,
122.042531241798)) ;
#49215=CARTESIAN_POINT('Ctrl Pts',(-19.7146500331995,-44.9743140135291,
122.24510774136)) ;
#49216=CARTESIAN_POINT('Ctrl Pts',(-19.790980965489,-44.7943249331663,121.953425884434)) ;
#49217=CARTESIAN_POINT('Ctrl Pts',(-19.5101771870513,-44.9841804581923,
122.210176444507)) ;
#49218=CARTESIAN_POINT('Ctrl Pts',(-19.5353894138272,-44.8041913778294,
121.909764540214)) ;
#49219=CARTESIAN_POINT('Ctrl Pts',(-19.3006636334398,-44.994146582641,122.210628861832)) ;
#49220=CARTESIAN_POINT('Ctrl Pts',(-19.2734974473692,-44.8141575022781,
121.910332881293)) ;
#49221=CARTESIAN_POINT('Ctrl Pts',(-19.0931406754314,-45.0041768260321,
122.248023638702)) ;
#49222=CARTESIAN_POINT('Ctrl Pts',(-19.0140941942044,-44.8241877456692,
121.957079096099)) ;
#49223=CARTESIAN_POINT('Ctrl Pts',(-18.8978469326455,-45.0140698609852,
122.319615465346)) ;
#49224=CARTESIAN_POINT('Ctrl Pts',(-18.7699778546539,-44.8340807806223,
122.04657166839)) ;
#49225=CARTESIAN_POINT('Ctrl Pts',(-18.7150830259635,-45.024120775222,122.425627543441)) ;
#49226=CARTESIAN_POINT('Ctrl Pts',(-18.5415249218624,-44.8441316948591,
122.179088598224)) ;
#49227=CARTESIAN_POINT('Ctrl Pts',(-18.5560590605076,-45.0340106014466,
122.559577916951)) ;
#49228=CARTESIAN_POINT('Ctrl Pts',(-18.3427444001931,-44.8540215210837,
122.346531093265)) ;
#49229=CARTESIAN_POINT('Ctrl Pts',(-18.3758084791143,-45.0473454164935,
122.774344433157)) ;
#49230=CARTESIAN_POINT('Ctrl Pts',(-18.1174461021876,-44.8673563361306,
122.614979487024)) ;
#49231=CARTESIAN_POINT('Ctrl Pts',(-18.2567530669862,-45.060622507665,123.03030649385)) ;
#49232=CARTESIAN_POINT('Ctrl Pts',(-17.9686335760902,-44.8806334273021,
122.934896659141)) ;
#49233=CARTESIAN_POINT('Ctrl Pts',(-18.2079946984886,-45.0738707962633,
123.304511382558)) ;
#49234=CARTESIAN_POINT('Ctrl Pts',(-17.9076731562678,-44.8938817159004,
123.277709414345)) ;
#49235=CARTESIAN_POINT('Ctrl Pts',(-18.2078213156215,-45.0839256377574,
123.515872423413)) ;
#49236=CARTESIAN_POINT('Ctrl Pts',(-17.9074623164892,-44.9039365573945,
123.541899571283)) ;
#49237=CARTESIAN_POINT('Ctrl Pts',(-18.2432033461838,-45.0937566270649,
123.719534287493)) ;
#49238=CARTESIAN_POINT('Ctrl Pts',(-17.9516919899064,-44.913767546702,123.796479325853)) ;
#49239=CARTESIAN_POINT('Ctrl Pts',(-18.3149935437228,-45.1038331913881,
123.918803697903)) ;
#49240=CARTESIAN_POINT('Ctrl Pts',(-18.0414310833544,-44.9238441110252,
124.045563596302)) ;
#49241=CARTESIAN_POINT('Ctrl Pts',(-18.4179463690853,-45.1136825165221,
124.098479005577)) ;
#49242=CARTESIAN_POINT('Ctrl Pts',(-18.1701298255741,-44.9336934361592,
124.270160085588)) ;
#49243=CARTESIAN_POINT('Ctrl Pts',(-18.5971230912793,-45.1270305161593,
124.314496308919)) ;
#49244=CARTESIAN_POINT('Ctrl Pts',(-18.3940753258795,-44.9470414357965,
124.540160290177)) ;
#49245=CARTESIAN_POINT('Ctrl Pts',(-18.8849989168967,-45.1436152756959,
124.518050402463)) ;
#49246=CARTESIAN_POINT('Ctrl Pts',(-18.7539725180923,-44.963626195333,124.794623795617)) ;
#49247=CARTESIAN_POINT('Ctrl Pts',(-19.224601952066,-45.160183827044,124.611932790248)) ;
#49248=CARTESIAN_POINT('Ctrl Pts',(-19.1783954643001,-44.9801947466811,
124.911954796591)) ;
#49249=CARTESIAN_POINT('Ctrl Pts',(-19.5054327742707,-45.173543651863,124.613960046694)) ;
#49250=CARTESIAN_POINT('Ctrl Pts',(-19.5295000394639,-44.9935545715001,
124.914496420765)) ;
#49251=CARTESIAN_POINT('Ctrl Pts',(-19.7108114161679,-45.1834490606937,
124.579447586727)) ;
#49252=CARTESIAN_POINT('Ctrl Pts',(-19.7862085515421,-45.0034599803308,
124.87135192276)) ;
#49253=CARTESIAN_POINT('Ctrl Pts',(-19.9082218453753,-45.1934090872777,
124.509714834404)) ;
#49254=CARTESIAN_POINT('Ctrl Pts',(-20.0329770475992,-45.0134200069148,
124.784181635824)) ;
#49255=CARTESIAN_POINT('Ctrl Pts',(-20.1511287525541,-45.206666671463,124.372952742759)) ;
#49256=CARTESIAN_POINT('Ctrl Pts',(-20.3365929403509,-45.0266775911001,
124.613239797289)) ;
#49257=CARTESIAN_POINT('Ctrl Pts',(-20.4042739888879,-45.2233178829577,
124.12545280733)) ;
#49258=CARTESIAN_POINT('Ctrl Pts',(-20.6530388478672,-45.0433288025948,
124.303846929761)) ;
#49259=CARTESIAN_POINT('Ctrl Pts',(-20.5876289534092,-45.243236097068,123.743705041852)) ;
#49260=CARTESIAN_POINT('Ctrl Pts',(-20.8822225928719,-45.0632470167051,
123.826665489803)) ;
#49261=CARTESIAN_POINT('Ctrl Pts',(-20.630530145128,-45.2631138602888,123.323172796485)) ;
#49262=CARTESIAN_POINT('Ctrl Pts',(-20.9358462100671,-45.0831247799259,
123.300999284693)) ;
#49263=CARTESIAN_POINT('Ctrl Pts',(-20.5263138562725,-45.283126528076,122.910688719133)) ;
#49264=CARTESIAN_POINT('Ctrl Pts',(-20.8055712371326,-45.1031374477131,
122.785395465323)) ;
#49265=CARTESIAN_POINT('Ctrl Pts',(-20.2902208181443,-45.3029390507426,
122.561698389052)) ;
#49266=CARTESIAN_POINT('Ctrl Pts',(-20.5104525719544,-45.1229499703797,
122.349160972193)) ;
#49267=CARTESIAN_POINT('Ctrl Pts',(-19.9467946863038,-45.3229223507425,
122.31164395972)) ;
#49268=CARTESIAN_POINT('Ctrl Pts',(-20.081167872577,-45.1429332703796,122.036595982268)) ;
#49269=CARTESIAN_POINT('Ctrl Pts',(-19.5402451083145,-45.3428166278438,
122.194572866398)) ;
#49270=CARTESIAN_POINT('Ctrl Pts',(-19.5729808270998,-45.1628275474809,
121.890260817414)) ;
#49271=CARTESIAN_POINT('Ctrl Pts',(-19.1173631256665,-45.3627493896015,
122.222652545081)) ;
#49272=CARTESIAN_POINT('Ctrl Pts',(-19.0443792388159,-45.1827603092387,
121.925363493254)) ;
#49273=CARTESIAN_POINT('Ctrl Pts',(-18.7289083515365,-45.3827153953663,
122.393915397857)) ;
#49274=CARTESIAN_POINT('Ctrl Pts',(-18.5588123388653,-45.2027263150034,
122.139444767471)) ;
#49275=CARTESIAN_POINT('Ctrl Pts',(-18.4233281728612,-45.4025939275311,
122.685968903404)) ;
#49276=CARTESIAN_POINT('Ctrl Pts',(-18.1768400075753,-45.2226048471683,
122.504512707876)) ;
#49277=CARTESIAN_POINT('Ctrl Pts',(-18.2348448265652,-45.4225335941915,
123.065690568163)) ;
#49278=CARTESIAN_POINT('Ctrl Pts',(-17.9412382746725,-45.2425445138286,
122.979165174917)) ;
#49279=CARTESIAN_POINT('Ctrl Pts',(-18.1872285477888,-45.4424284688368,
123.486065831409)) ;
#49280=CARTESIAN_POINT('Ctrl Pts',(-17.8817201357155,-45.262439388474,123.504633155352)) ;
#49281=CARTESIAN_POINT('Ctrl Pts',(-18.2855438839301,-45.4623356081302,
123.897669851793)) ;
#49282=CARTESIAN_POINT('Ctrl Pts',(-18.0046155637013,-45.2823465277673,
124.019136501102)) ;
#49283=CARTESIAN_POINT('Ctrl Pts',(-18.5179787925655,-45.4822461562087,
124.251671884329)) ;
#49284=CARTESIAN_POINT('Ctrl Pts',(-18.2951592685282,-45.3022570758458,
124.461637555377)) ;
#49285=CARTESIAN_POINT('Ctrl Pts',(-18.8603532025877,-45.5023147415659,
124.506196821107)) ;
#49286=CARTESIAN_POINT('Ctrl Pts',(-18.7231289192442,-45.322325661203,124.779793280886)) ;
#49287=CARTESIAN_POINT('Ctrl Pts',(-19.2632916538043,-45.5220965388806,
124.627332831793)) ;
#49288=CARTESIAN_POINT('Ctrl Pts',(-19.2267990765381,-45.3421074585177,
124.931211593154)) ;
#49289=CARTESIAN_POINT('Ctrl Pts',(-19.6879024854321,-45.5421040858251,
124.604065554752)) ;
#49290=CARTESIAN_POINT('Ctrl Pts',(-19.7575625515052,-45.3621150054623,
124.902127405188)) ;
#49291=CARTESIAN_POINT('Ctrl Pts',(-20.0757175915424,-45.561925824128,124.438753736194)) ;
#49292=CARTESIAN_POINT('Ctrl Pts',(-20.2423289587424,-45.3819367437651,
124.695488931146)) ;
#49293=CARTESIAN_POINT('Ctrl Pts',(-20.3866991980944,-45.5819058440321,
124.149413523319)) ;
#49294=CARTESIAN_POINT('Ctrl Pts',(-20.6310564599377,-45.4019167636693,
124.333814619466)) ;
#49295=CARTESIAN_POINT('Ctrl Pts',(-20.579213898747,-45.6018232952944,123.772183038511)) ;
#49296=CARTESIAN_POINT('Ctrl Pts',(-20.8717000555941,-45.4218342149315,
123.862278018821)) ;
#49297=CARTESIAN_POINT('Ctrl Pts',(-20.6323140250136,-45.6216982164671,
123.35290988801)) ;
#49298=CARTESIAN_POINT('Ctrl Pts',(-20.9380767680918,-45.4417091361042,
123.338188475184)) ;
#49299=CARTESIAN_POINT('Ctrl Pts',(-20.5381944095279,-45.6417225850179,
122.937699622663)) ;
#49300=CARTESIAN_POINT('Ctrl Pts',(-20.8204289201312,-45.461733504655,122.819174893006)) ;
#49301=CARTESIAN_POINT('Ctrl Pts',(-20.3096913478822,-45.6615892693914,
122.582336964708)) ;
#49302=CARTESIAN_POINT('Ctrl Pts',(-20.5348026192168,-45.4816001890285,
122.374971928378)) ;
#49303=CARTESIAN_POINT('Ctrl Pts',(-19.9728378596493,-45.6815330912376,
122.324818392206)) ;
#49304=CARTESIAN_POINT('Ctrl Pts',(-20.113737828752,-45.5015440108747,122.053072103722)) ;
#49305=CARTESIAN_POINT('Ctrl Pts',(-19.5689770807575,-45.7014404604891,
122.198058930962)) ;
#49306=CARTESIAN_POINT('Ctrl Pts',(-19.6089136734289,-45.5214513801262,
121.894620584429)) ;
#49307=CARTESIAN_POINT('Ctrl Pts',(-19.1467685091688,-45.7213151582358,
122.215906390113)) ;
#49308=CARTESIAN_POINT('Ctrl Pts',(-19.0811541092211,-45.5413260778729,
121.916926618997)) ;
#49309=CARTESIAN_POINT('Ctrl Pts',(-18.7538192203983,-45.7412971007575,
122.377543259028)) ;
#49310=CARTESIAN_POINT('Ctrl Pts',(-18.5899663032709,-45.5613080203947,
122.11896949238)) ;
#49311=CARTESIAN_POINT('Ctrl Pts',(-18.4411535486972,-45.7611997676684,
122.662651717635)) ;
#49312=CARTESIAN_POINT('Ctrl Pts',(-18.1991325996576,-45.5812106873055,
122.475351878754)) ;
#49313=CARTESIAN_POINT('Ctrl Pts',(-18.2438603449424,-45.7810551252071,
123.035964325074)) ;
#49314=CARTESIAN_POINT('Ctrl Pts',(-17.9525130136247,-45.6010660448442,
122.94198968938)) ;
#49315=CARTESIAN_POINT('Ctrl Pts',(-18.1856815046609,-45.8011191639231,
123.458527247341)) ;
#49316=CARTESIAN_POINT('Ctrl Pts',(-17.8797853306708,-45.6211300835602,
123.470193368152)) ;
#49317=CARTESIAN_POINT('Ctrl Pts',(-18.2744755391468,-45.8209743436481,
123.871419259032)) ;
#49318=CARTESIAN_POINT('Ctrl Pts',(-17.9907738386166,-45.6409852632853,
123.986308188026)) ;
#49319=CARTESIAN_POINT('Ctrl Pts',(-18.4997930018078,-45.8409544483126,
124.231383616986)) ;
#49320=CARTESIAN_POINT('Ctrl Pts',(-18.2724161799833,-45.6609653679497,
124.436265927067)) ;
#49321=CARTESIAN_POINT('Ctrl Pts',(-18.8314673108359,-45.8607635534824,
124.49118909027)) ;
#49322=CARTESIAN_POINT('Ctrl Pts',(-18.6870078952182,-45.6807744731195,
124.761025281335)) ;
#49323=CARTESIAN_POINT('Ctrl Pts',(-19.2352299421936,-45.8807561738231,
124.623756846675)) ;
#49324=CARTESIAN_POINT('Ctrl Pts',(-19.1916999501427,-45.7007670934602,
124.926741074859)) ;
#49325=CARTESIAN_POINT('Ctrl Pts',(-19.586815630739,-45.8972956563272,124.612921446625)) ;
#49326=CARTESIAN_POINT('Ctrl Pts',(-19.6312118173371,-45.7173065759643,
124.913196409966)) ;
#49327=CARTESIAN_POINT('Ctrl Pts',(-19.8558718361537,-45.9106599743914,
124.532044526927)) ;
#49328=CARTESIAN_POINT('Ctrl Pts',(-19.9674993568783,-45.7306708940285,
124.812112387644)) ;
#49329=CARTESIAN_POINT('Ctrl Pts',(-20.1042094269978,-45.9238775768929,
124.407362624785)) ;
#49330=CARTESIAN_POINT('Ctrl Pts',(-20.2779790594621,-45.74388849653,124.656227492421)) ;
#49331=CARTESIAN_POINT('Ctrl Pts',(-20.368961477355,-45.9405351711707,124.172135837994)) ;
#49332=CARTESIAN_POINT('Ctrl Pts',(-20.6088613725694,-45.7605460908078,
124.362235325753)) ;
#49333=CARTESIAN_POINT('Ctrl Pts',(-20.5701552804557,-45.9604008732124,
123.800652640584)) ;
#49334=CARTESIAN_POINT('Ctrl Pts',(-20.8603771681575,-45.7804117928495,
123.897882285973)) ;
#49335=CARTESIAN_POINT('Ctrl Pts',(-20.6228240088762,-45.9770305999024,
123.451100482239)) ;
#49336=CARTESIAN_POINT('Ctrl Pts',(-20.9262145451772,-45.7970415195396,
123.460911151536)) ;
#49337=CARTESIAN_POINT('Ctrl Pts',(-20.5914361189551,-45.9903197150403,
123.173415800151)) ;
#49338=CARTESIAN_POINT('Ctrl Pts',(-20.8869828199733,-45.8103306346774,
123.113835882224)) ;
#49339=CARTESIAN_POINT('Ctrl Pts',(-20.5323594467668,-46.0002840620174,
122.972457040269)) ;
#49340=CARTESIAN_POINT('Ctrl Pts',(-20.813137221631,-45.8202949816545,122.862628158048)) ;
#49341=CARTESIAN_POINT('Ctrl Pts',(-20.4397374973719,-46.0102124300189,
122.785404683368)) ;
#49342=CARTESIAN_POINT('Ctrl Pts',(-20.6973720958994,-45.830223349656,122.628822672111)) ;
#49343=CARTESIAN_POINT('Ctrl Pts',(-20.2747057487913,-46.0234958631076,
122.560148912213)) ;
#49344=CARTESIAN_POINT('Ctrl Pts',(-20.491036246019,-45.8435067827447,122.347203200446)) ;
#49345=CARTESIAN_POINT('Ctrl Pts',(-19.9984819879349,-46.0401479408479,
122.338567938627)) ;
#49346=CARTESIAN_POINT('Ctrl Pts',(-20.145826084982,-45.8601588604851,122.070280119537)) ;
#49347=CARTESIAN_POINT('Ctrl Pts',(-19.6654083029669,-46.0566993101488,
122.225111293764)) ;
#49348=CARTESIAN_POINT('Ctrl Pts',(-19.7294257177558,-45.8767102297859,
121.928426697341)) ;
#49349=CARTESIAN_POINT('Ctrl Pts',(-19.3866709636188,-46.0699867382977,
122.205956450198)) ;
#49350=CARTESIAN_POINT('Ctrl Pts',(-19.3810452958569,-45.8899976579349,
121.904492705596)) ;
#49351=CARTESIAN_POINT('Ctrl Pts',(-19.1767289526485,-46.0800312779978,
122.228493274204)) ;
#49352=CARTESIAN_POINT('Ctrl Pts',(-19.1186091401649,-45.900042197635,121.932658291026)) ;
#49353=CARTESIAN_POINT('Ctrl Pts',(-18.9778591393557,-46.0898741198217,
122.285724273761)) ;
#49354=CARTESIAN_POINT('Ctrl Pts',(-18.8700233535146,-45.9098850394588,
122.00419504513)) ;
#49355=CARTESIAN_POINT('Ctrl Pts',(-18.7890949169887,-46.0998584040686,
122.37747258679)) ;
#49356=CARTESIAN_POINT('Ctrl Pts',(-18.6340661750229,-45.9198693237057,
122.118877741184)) ;
#49357=CARTESIAN_POINT('Ctrl Pts',(-18.6197187705816,-46.1098080494678,
122.500228764062)) ;
#49358=CARTESIAN_POINT('Ctrl Pts',(-18.4223444457942,-45.9298189691049,
122.272320772615)) ;
#49359=CARTESIAN_POINT('Ctrl Pts',(-18.4733104190095,-46.1198078111562,
122.651108437036)) ;
#49360=CARTESIAN_POINT('Ctrl Pts',(-18.2393318883207,-45.9398187307933,
122.460918444187)) ;
#49361=CARTESIAN_POINT('Ctrl Pts',(-18.3552472327061,-46.1298391571151,
122.825850445849)) ;
#49362=CARTESIAN_POINT('Ctrl Pts',(-18.0917505487203,-45.9498500767522,
122.679344429148)) ;
#49363=CARTESIAN_POINT('Ctrl Pts',(-18.2705494607926,-46.1396941115922,
123.014933391385)) ;
#49364=CARTESIAN_POINT('Ctrl Pts',(-17.9858757132729,-45.9597050312293,
122.915697062005)) ;
#49365=CARTESIAN_POINT('Ctrl Pts',(-18.2188977661992,-46.1496666495927,
123.218103084829)) ;
#49366=CARTESIAN_POINT('Ctrl Pts',(-17.9213083460971,-45.9696775692299,
123.1696585988)) ;
#49367=CARTESIAN_POINT('Ctrl Pts',(-18.2032838337834,-46.1596616433277,
123.427680803576)) ;
#49368=CARTESIAN_POINT('Ctrl Pts',(-17.9017881316978,-45.9796725629648,
123.43163061832)) ;
#49369=CARTESIAN_POINT('Ctrl Pts',(-18.2246312081846,-46.1696957021218,
123.637527281541)) ;
#49370=CARTESIAN_POINT('Ctrl Pts',(-17.9284695515831,-45.9897066217589,
123.693939039804)) ;
#49371=CARTESIAN_POINT('Ctrl Pts',(-18.2807599390842,-46.1795510449448,
123.836991427032)) ;
#49372=CARTESIAN_POINT('Ctrl Pts',(-17.9986278342862,-45.9995619645819,
123.943270201395)) ;
#49373=CARTESIAN_POINT('Ctrl Pts',(-18.3717042160913,-46.1895505242904,
124.026480311802)) ;
#49374=CARTESIAN_POINT('Ctrl Pts',(-18.1123057056934,-46.0095614439275,
124.180132595263)) ;
#49375=CARTESIAN_POINT('Ctrl Pts',(-18.4927341945723,-46.1994449730457,
124.195705746537)) ;
#49376=CARTESIAN_POINT('Ctrl Pts',(-18.2635910838762,-46.0194558926828,
124.391666206078)) ;
#49377=CARTESIAN_POINT('Ctrl Pts',(-18.6438307854289,-46.2095080924802,
124.343730651591)) ;
#49378=CARTESIAN_POINT('Ctrl Pts',(-18.4524598572534,-46.0295190121173,
124.576699295059)) ;
#49379=CARTESIAN_POINT('Ctrl Pts',(-18.8143876956358,-46.2193477377214,
124.460844662452)) ;
#49380=CARTESIAN_POINT('Ctrl Pts',(-18.6656547763294,-46.0393586573585,
124.723094304069)) ;
#49381=CARTESIAN_POINT('Ctrl Pts',(-19.0067961425218,-46.2294109019075,
124.548731031768)) ;
#49382=CARTESIAN_POINT('Ctrl Pts',(-18.9061641632514,-46.0494218215446,
124.832954725746)) ;
#49383=CARTESIAN_POINT('Ctrl Pts',(-19.2082002254343,-46.2393051716563,
124.60082520619)) ;
#49384=CARTESIAN_POINT('Ctrl Pts',(-19.1579188977088,-46.0593160912934,
124.898075179652)) ;
#49385=CARTESIAN_POINT('Ctrl Pts',(-19.4164887508991,-46.2492468976701,
124.617795648775)) ;
#49386=CARTESIAN_POINT('Ctrl Pts',(-19.4182795982721,-46.0692578173072,
124.919290922679)) ;
#49387=CARTESIAN_POINT('Ctrl Pts',(-19.625908760725,-46.2592497863295,124.598307790084)) ;
#49388=CARTESIAN_POINT('Ctrl Pts',(-19.6800549445947,-46.0792607059666,
124.894933738321)) ;
#49389=CARTESIAN_POINT('Ctrl Pts',(-19.8293605211461,-46.2692896351235,
124.542189850238)) ;
#49390=CARTESIAN_POINT('Ctrl Pts',(-19.9343703358343,-46.0893005547606,
124.824788939864)) ;
#49391=CARTESIAN_POINT('Ctrl Pts',(-20.0161177451334,-46.2791138505843,
124.453953136808)) ;
#49392=CARTESIAN_POINT('Ctrl Pts',(-20.1678185633982,-46.0991247702215,
124.714495173511)) ;
#49393=CARTESIAN_POINT('Ctrl Pts',(-20.1888529807882,-46.2891706940779,
124.332063949481)) ;
#49394=CARTESIAN_POINT('Ctrl Pts',(-20.3837390423242,-46.109181613715,124.562135863679)) ;
#49395=CARTESIAN_POINT('Ctrl Pts',(-20.3357237419567,-46.2990993034739,
124.183735609964)) ;
#49396=CARTESIAN_POINT('Ctrl Pts',(-20.5673296043918,-46.119110223111,124.376727071012)) ;
#49397=CARTESIAN_POINT('Ctrl Pts',(-20.4553698807106,-46.3090511875118,
124.012092768846)) ;
#49398=CARTESIAN_POINT('Ctrl Pts',(-20.7168895335636,-46.1290621071489,
124.162174744986)) ;
#49399=CARTESIAN_POINT('Ctrl Pts',(-20.5439344328811,-46.3191041403194,
123.820215375579)) ;
#49400=CARTESIAN_POINT('Ctrl Pts',(-20.8275975547341,-46.1391150599565,
123.922329195858)) ;
#49401=CARTESIAN_POINT('Ctrl Pts',(-20.5969834126444,-46.3289270167856,
123.620621819729)) ;
#49402=CARTESIAN_POINT('Ctrl Pts',(-20.8939114402365,-46.1489379364227,
123.672837152796)) ;
#49403=CARTESIAN_POINT('Ctrl Pts',(-20.6153551246027,-46.3389827493557,
123.41003275426)) ;
#49404=CARTESIAN_POINT('Ctrl Pts',(-20.9168785394599,-46.1589936689928,
123.409601144836)) ;
#49405=CARTESIAN_POINT('Ctrl Pts',(-20.5967235165246,-46.3489235143433,
123.201871132053)) ;
#49406=CARTESIAN_POINT('Ctrl Pts',(-20.893591540016,-46.1689344339805,123.149398558187)) ;
#49407=CARTESIAN_POINT('Ctrl Pts',(-20.5430611916777,-46.358827847249,123.000680696278)) ;
#49408=CARTESIAN_POINT('Ctrl Pts',(-20.8265158340173,-46.1788387668861,
122.89790937762)) ;
#49409=CARTESIAN_POINT('Ctrl Pts',(-20.4539067996073,-46.3688745161297,
122.809226303737)) ;
#49410=CARTESIAN_POINT('Ctrl Pts',(-20.7150751051334,-46.1888854357668,
122.658590446776)) ;
#49411=CARTESIAN_POINT('Ctrl Pts',(-20.3348107304018,-46.3787700794355,
122.638612779929)) ;
#49412=CARTESIAN_POINT('Ctrl Pts',(-20.5662066575866,-46.1987809990726,
122.445321690522)) ;
#49413=CARTESIAN_POINT('Ctrl Pts',(-20.1854730789962,-46.3888321371358,
122.48883600952)) ;
#49414=CARTESIAN_POINT('Ctrl Pts',(-20.379536426161,-46.2088430567729,122.258099155572)) ;
#49415=CARTESIAN_POINT('Ctrl Pts',(-20.0161942508695,-46.3986749147633,
122.369786755293)) ;
#49416=CARTESIAN_POINT('Ctrl Pts',(-20.1679385535702,-46.2186858344004,
122.109285146216)) ;
#49417=CARTESIAN_POINT('Ctrl Pts',(-19.8262618796166,-46.4086653930151,
122.28019126902)) ;
#49418=CARTESIAN_POINT('Ctrl Pts',(-19.9305238988353,-46.2286763126523,
121.997288664891)) ;
#49419=CARTESIAN_POINT('Ctrl Pts',(-19.6248584878059,-46.4185943656587,
122.225294019457)) ;
#49420=CARTESIAN_POINT('Ctrl Pts',(-19.6787697821799,-46.2386052852958,
121.928664786175)) ;
#49421=CARTESIAN_POINT('Ctrl Pts',(-19.4157226032529,-46.4285855025382,
122.205756739938)) ;
#49422=CARTESIAN_POINT('Ctrl Pts',(-19.4173499655239,-46.2485964221754,
121.904240994676)) ;
#49423=CARTESIAN_POINT('Ctrl Pts',(-19.2057405057304,-46.4386076200272,
122.223135749663)) ;
#49424=CARTESIAN_POINT('Ctrl Pts',(-19.1548721753511,-46.2586185396643,
121.92596250925)) ;
#49425=CARTESIAN_POINT('Ctrl Pts',(-19.0043894905299,-46.4485081304294,
122.275869896389)) ;
#49426=CARTESIAN_POINT('Ctrl Pts',(-18.9031822162054,-46.2685190500665,
121.991878228814)) ;
#49427=CARTESIAN_POINT('Ctrl Pts',(-18.813429020907,-46.4584971231755,122.363241063598)) ;
#49428=CARTESIAN_POINT('Ctrl Pts',(-18.6644805817943,-46.2785080428126,
122.101090338779)) ;
#49429=CARTESIAN_POINT('Ctrl Pts',(-18.6410397094411,-46.4684623672261,
122.482274292673)) ;
#49430=CARTESIAN_POINT('Ctrl Pts',(-18.4489924497402,-46.2884732868632,
122.249880282488)) ;
#49431=CARTESIAN_POINT('Ctrl Pts',(-18.4924874516743,-46.4783666317393,
122.62819862701)) ;
#49432=CARTESIAN_POINT('Ctrl Pts',(-18.2633002251361,-46.2983775513764,
122.43228474134)) ;
#49433=CARTESIAN_POINT('Ctrl Pts',(-18.3697789016585,-46.4884247234375,
122.800382922365)) ;
#49434=CARTESIAN_POINT('Ctrl Pts',(-18.1099129937586,-46.3084356430746,
122.64751373004)) ;
#49435=CARTESIAN_POINT('Ctrl Pts',(-18.2805605389299,-46.4982746638659,
122.987267125253)) ;
#49436=CARTESIAN_POINT('Ctrl Pts',(-17.9983877780156,-46.318285583503,122.881119052211)) ;
#49437=CARTESIAN_POINT('Ctrl Pts',(-18.2236525306218,-46.5083016750394,
123.190235923869)) ;
#49438=CARTESIAN_POINT('Ctrl Pts',(-17.9272509867176,-46.3283125946766,
123.13482951254)) ;
#49439=CARTESIAN_POINT('Ctrl Pts',(-18.2033939632025,-46.5183302616515,
123.400103024954)) ;
#49440=CARTESIAN_POINT('Ctrl Pts',(-17.901925769436,-46.3383411812886,123.397163125626)) ;
#49441=CARTESIAN_POINT('Ctrl Pts',(-18.2191889497681,-46.5281754757642,
123.606465447685)) ;
#49442=CARTESIAN_POINT('Ctrl Pts',(-17.9216676872438,-46.3481863954013,
123.655117412453)) ;
#49443=CARTESIAN_POINT('Ctrl Pts',(-18.2707942324504,-46.5381662239437,
123.810069040328)) ;
#49444=CARTESIAN_POINT('Ctrl Pts',(-17.9861726596863,-46.3581771435809,
123.909622518266)) ;
#49445=CARTESIAN_POINT('Ctrl Pts',(-18.357794261464,-46.5482038575292,124.002323055344)) ;
#49446=CARTESIAN_POINT('Ctrl Pts',(-18.0949209308514,-46.3682147771664,
124.149940691054)) ;
#49447=CARTESIAN_POINT('Ctrl Pts',(-18.4742897524447,-46.5580491467421,
124.173407953581)) ;
#49448=CARTESIAN_POINT('Ctrl Pts',(-18.2405394895734,-46.3780600663792,
124.363798772761)) ;
#49449=CARTESIAN_POINT('Ctrl Pts',(-18.620370895161,-46.568030547548,124.324028601828)) ;
#49450=CARTESIAN_POINT('Ctrl Pts',(-18.4231399414147,-46.3880414671851,
124.552075901713)) ;
#49451=CARTESIAN_POINT('Ctrl Pts',(-18.7899363735675,-46.5779827805379,
124.44660926478)) ;
#49452=CARTESIAN_POINT('Ctrl Pts',(-18.6350962163679,-46.397993700175,124.705303329863)) ;
#49453=CARTESIAN_POINT('Ctrl Pts',(-18.9789812034734,-46.5879815919945,
124.538563788364)) ;
#49454=CARTESIAN_POINT('Ctrl Pts',(-18.8714017008727,-46.4079925116317,
124.820247929086)) ;
#49455=CARTESIAN_POINT('Ctrl Pts',(-19.1820191632644,-46.5980206959252,
124.596131546056)) ;
#49456=CARTESIAN_POINT('Ctrl Pts',(-19.1251985398827,-46.4180316155623,
124.892209201477)) ;
#49457=CARTESIAN_POINT('Ctrl Pts',(-19.3874680290362,-46.6078456383445,
124.617557565118)) ;
#49458=CARTESIAN_POINT('Ctrl Pts',(-19.3820108279109,-46.4278565579816,
124.918993385592)) ;
#49459=CARTESIAN_POINT('Ctrl Pts',(-19.5983341246022,-46.6179003258204,
124.602993200605)) ;
#49460=CARTESIAN_POINT('Ctrl Pts',(-19.64559328927,-46.4379112454576,124.900789356719)) ;
#49461=CARTESIAN_POINT('Ctrl Pts',(-19.8011174374927,-46.6278431281773,
124.552252454525)) ;
#49462=CARTESIAN_POINT('Ctrl Pts',(-19.8990733415374,-46.4478540478144,
124.837364781521)) ;
#49463=CARTESIAN_POINT('Ctrl Pts',(-19.9915187465345,-46.637746924117,124.467991218211)) ;
#49464=CARTESIAN_POINT('Ctrl Pts',(-20.1370762828401,-46.4577578437542,
124.732039090923)) ;
#49465=CARTESIAN_POINT('Ctrl Pts',(-20.166805154378,-46.6477937034921,124.350181343917)) ;
#49466=CARTESIAN_POINT('Ctrl Pts',(-20.3561848751386,-46.4678046231292,
124.584777991393)) ;
#49467=CARTESIAN_POINT('Ctrl Pts',(-20.3168442450622,-46.6576893617867,
124.20602634747)) ;
#49468=CARTESIAN_POINT('Ctrl Pts',(-20.5437352889847,-46.4777002814238,
124.40458454613)) ;
#49469=CARTESIAN_POINT('Ctrl Pts',(-20.4416202810829,-46.6677509290373,
124.035249876144)) ;
#49470=CARTESIAN_POINT('Ctrl Pts',(-20.6997061794261,-46.4877618486744,
124.191114977027)) ;
#49471=CARTESIAN_POINT('Ctrl Pts',(-20.5328807367812,-46.6775955734746,
123.849484643393)) ;
#49472=CARTESIAN_POINT('Ctrl Pts',(-20.8137834732747,-46.4976064931117,
123.958907813317)) ;
#49473=CARTESIAN_POINT('Ctrl Pts',(-20.5918946295246,-46.6875556197173,
123.64858424823)) ;
#49474=CARTESIAN_POINT('Ctrl Pts',(-20.8875519244176,-46.5075665393544,
123.707782162122)) ;
#49475=CARTESIAN_POINT('Ctrl Pts',(-20.6148993357899,-46.6975939157357,
123.43881520395)) ;
#49476=CARTESIAN_POINT('Ctrl Pts',(-20.9163089327259,-46.5176048353728,
123.445571143073)) ;
#49477=CARTESIAN_POINT('Ctrl Pts',(-20.6017530846061,-46.707467257154,123.231632331)) ;
#49478=CARTESIAN_POINT('Ctrl Pts',(-20.8998770457403,-46.5274781767911,
123.186591367245)) ;
#49479=CARTESIAN_POINT('Ctrl Pts',(-20.5517975292825,-46.7175403609533,
123.025882379625)) ;
#49480=CARTESIAN_POINT('Ctrl Pts',(-20.8374336990215,-46.5375512805904,
122.92940409922)) ;
#49481=CARTESIAN_POINT('Ctrl Pts',(-20.4692073505912,-46.7273611760722,
122.836612568494)) ;
#49482=CARTESIAN_POINT('Ctrl Pts',(-20.7341962066025,-46.5473720957093,
122.692815045796)) ;
#49483=CARTESIAN_POINT('Ctrl Pts',(-20.3522770027166,-46.7374380411502,
122.660005076197)) ;
#49484=CARTESIAN_POINT('Ctrl Pts',(-20.5880342149854,-46.5574489607873,
122.472055591262)) ;
#49485=CARTESIAN_POINT('Ctrl Pts',(-20.2094265317654,-46.7473027808054,
122.509626266143)) ;
#49486=CARTESIAN_POINT('Ctrl Pts',(-20.4094709146945,-46.5673137004426,
122.28408059887)) ;
#49487=CARTESIAN_POINT('Ctrl Pts',(-20.0403249054971,-46.7573251840468,
122.383941295046)) ;
#49488=CARTESIAN_POINT('Ctrl Pts',(-20.1980943113753,-46.5773361036839,
122.126973882739)) ;
#49489=CARTESIAN_POINT('Ctrl Pts',(-19.8516517065092,-46.7673509083353,
122.28995820191)) ;
#49490=CARTESIAN_POINT('Ctrl Pts',(-19.962253273062,-46.5873618279724,122.009494285123)) ;
#49491=CARTESIAN_POINT('Ctrl Pts',(-19.6531005041751,-46.7772056913566,
122.23083936213)) ;
#49492=CARTESIAN_POINT('Ctrl Pts',(-19.7140632034375,-46.5972166109937,
121.935594664619)) ;
#49493=CARTESIAN_POINT('Ctrl Pts',(-19.4447550366577,-46.7871845350798,
122.206249292003)) ;
#49494=CARTESIAN_POINT('Ctrl Pts',(-19.453631099447,-46.607195454717,121.904856532763)) ;
#49495=CARTESIAN_POINT('Ctrl Pts',(-19.2345000747721,-46.7972034273165,
122.218618665142)) ;
#49496=CARTESIAN_POINT('Ctrl Pts',(-19.1908123744642,-46.6172143469536,
121.920317600805)) ;
#49497=CARTESIAN_POINT('Ctrl Pts',(-19.0322268033516,-46.8070866363575,
122.266237363921)) ;
#49498=CARTESIAN_POINT('Ctrl Pts',(-18.9379696064049,-46.6270975559946,
121.979840758629)) ;
#49499=CARTESIAN_POINT('Ctrl Pts',(-18.8378107169686,-46.8171549456977,
122.349847749281)) ;
#49500=CARTESIAN_POINT('Ctrl Pts',(-18.6949496716682,-46.6371658653348,
122.084353104064)) ;
#49501=CARTESIAN_POINT('Ctrl Pts',(-18.6648606133521,-46.8269850710304,
122.463033827998)) ;
#49502=CARTESIAN_POINT('Ctrl Pts',(-18.4787605240765,-46.6469959906675,
122.225836194928)) ;
#49503=CARTESIAN_POINT('Ctrl Pts',(-18.5104293304733,-46.8370516234074,
122.607686193805)) ;
#49504=CARTESIAN_POINT('Ctrl Pts',(-18.2857214966169,-46.6570625430445,
122.406651152196)) ;
#49505=CARTESIAN_POINT('Ctrl Pts',(-18.3857520045829,-46.8469418603011,
122.774114785356)) ;
#49506=CARTESIAN_POINT('Ctrl Pts',(-18.1298739186722,-46.6669527799382,
122.614687511568)) ;
#49507=CARTESIAN_POINT('Ctrl Pts',(-18.2905056904675,-46.8569340850951,
122.961335246674)) ;
#49508=CARTESIAN_POINT('Ctrl Pts',(-18.0108157653476,-46.6769450047322,
122.848713195629)) ;
#49509=CARTESIAN_POINT('Ctrl Pts',(-18.2295789136963,-46.866896705446,123.161719579238)) ;
#49510=CARTESIAN_POINT('Ctrl Pts',(-17.9346569102099,-46.6869076250832,
123.099193972045)) ;
#49511=CARTESIAN_POINT('Ctrl Pts',(-18.2040027326687,-46.8768017082092,
123.368391035254)) ;
#49512=CARTESIAN_POINT('Ctrl Pts',(-17.9026865142012,-46.6968126278463,
123.35753421386)) ;
#49513=CARTESIAN_POINT('Ctrl Pts',(-18.2150087934461,-46.8868594706073,
123.579531972586)) ;
#49514=CARTESIAN_POINT('Ctrl Pts',(-17.9164439568202,-46.7068703902444,
123.621460054285)) ;
#49515=CARTESIAN_POINT('Ctrl Pts',(-18.261371220002,-46.8967099899861,123.781380377064)) ;
#49516=CARTESIAN_POINT('Ctrl Pts',(-17.9743972615009,-46.7167209096232,
123.873771940566)) ;
#49517=CARTESIAN_POINT('Ctrl Pts',(-18.3431220571985,-46.9067415669843,
123.975771653837)) ;
#49518=CARTESIAN_POINT('Ctrl Pts',(-18.076585890768,-46.7267524866214,124.116760874155)) ;
#49519=CARTESIAN_POINT('Ctrl Pts',(-18.4574955443547,-46.9167513020892,
124.152440425366)) ;
#49520=CARTESIAN_POINT('Ctrl Pts',(-18.2195527491891,-46.7367622217263,
124.337596888945)) ;
#49521=CARTESIAN_POINT('Ctrl Pts',(-18.5992104285265,-46.9266608787155,
124.305119300968)) ;
#49522=CARTESIAN_POINT('Ctrl Pts',(-18.3966970018907,-46.7466717983526,
124.528446109055)) ;
#49523=CARTESIAN_POINT('Ctrl Pts',(-18.765279645767,-46.9365882645721,124.431541302977)) ;
#49524=CARTESIAN_POINT('Ctrl Pts',(-18.6042842738298,-46.7565991842093,
124.686473857333)) ;
#49525=CARTESIAN_POINT('Ctrl Pts',(-18.9530362774689,-46.9466331990624,
124.528179929632)) ;
#49526=CARTESIAN_POINT('Ctrl Pts',(-18.8389799600762,-46.7666441186995,
124.807271873775)) ;
#49527=CARTESIAN_POINT('Ctrl Pts',(-19.151511474355,-46.9565191312504,124.589883618221)) ;
#49528=CARTESIAN_POINT('Ctrl Pts',(-19.0870750670697,-46.7765300508875,
124.884401576548)) ;
#49529=CARTESIAN_POINT('Ctrl Pts',(-19.3598549427328,-46.9665124372034,
124.616830207834)) ;
#49530=CARTESIAN_POINT('Ctrl Pts',(-19.3475046537344,-46.7865233568405,
124.918084459445)) ;
#49531=CARTESIAN_POINT('Ctrl Pts',(-19.5687199932944,-46.9764580749853,
124.607155449397)) ;
#49532=CARTESIAN_POINT('Ctrl Pts',(-19.6085865453895,-46.7964689946224,
124.905990634094)) ;
#49533=CARTESIAN_POINT('Ctrl Pts',(-19.7728690713917,-46.9864053433312,
124.561770557663)) ;
#49534=CARTESIAN_POINT('Ctrl Pts',(-19.8637733413823,-46.8064162629683,
124.84925888775)) ;
#49535=CARTESIAN_POINT('Ctrl Pts',(-19.9678843674529,-46.9964532454683,
124.480604259967)) ;
#49536=CARTESIAN_POINT('Ctrl Pts',(-20.1075420667063,-46.8164641651054,
124.747800719658)) ;
#49537=CARTESIAN_POINT('Ctrl Pts',(-20.1423977281203,-47.0063009403085,
124.369220465197)) ;
#49538=CARTESIAN_POINT('Ctrl Pts',(-20.3256846821778,-46.8263118599456,
124.608569806517)) ;
#49539=CARTESIAN_POINT('Ctrl Pts',(-20.2971232610949,-47.0162624500529,
124.228102585513)) ;
#49540=CARTESIAN_POINT('Ctrl Pts',(-20.5190914280319,-46.83627336969,124.432171593144)) ;
#49541=CARTESIAN_POINT('Ctrl Pts',(-20.4256537019022,-47.0262918416617,
124.060947461949)) ;
#49542=CARTESIAN_POINT('Ctrl Pts',(-20.6797539090321,-46.8463027612989,
124.223227378211)) ;
#49543=CARTESIAN_POINT('Ctrl Pts',(-20.5221200134929,-47.0361993372165,
123.876344757324)) ;
#49544=CARTESIAN_POINT('Ctrl Pts',(-20.8003366055072,-46.8562102568536,
123.992472885729)) ;
#49545=CARTESIAN_POINT('Ctrl Pts',(-20.585700963853,-47.0461447288795,123.677180951145)) ;
#49546=CARTESIAN_POINT('Ctrl Pts',(-20.8798121649612,-46.8661556485166,
123.743517315993)) ;
#49547=CARTESIAN_POINT('Ctrl Pts',(-20.6140236281274,-47.0561466464769,
123.468796635054)) ;
#49548=CARTESIAN_POINT('Ctrl Pts',(-20.915214625767,-46.876157566114,123.48303667498)) ;
#49549=CARTESIAN_POINT('Ctrl Pts',(-20.6053144754768,-47.0661867140291,
123.257921725322)) ;
#49550=CARTESIAN_POINT('Ctrl Pts',(-20.9043274469187,-46.8861976336662,
123.219443241607)) ;
#49551=CARTESIAN_POINT('Ctrl Pts',(-20.5615451992037,-47.0760110254689,
123.056057517403)) ;
#49552=CARTESIAN_POINT('Ctrl Pts',(-20.8496146260734,-46.896021945106,122.967111685229)) ;
#49553=CARTESIAN_POINT('Ctrl Pts',(-20.48182941958,-47.086067266625,122.860270767228)) ;
#49554=CARTESIAN_POINT('Ctrl Pts',(-20.7499690603553,-46.9060781862621,
122.722378928017)) ;
#49555=CARTESIAN_POINT('Ctrl Pts',(-20.3705003700426,-47.0959981883606,
122.683623151021)) ;
#49556=CARTESIAN_POINT('Ctrl Pts',(-20.6108065948018,-46.9160091079977,
122.501569334543)) ;
#49557=CARTESIAN_POINT('Ctrl Pts',(-20.2303667268952,-47.1059414244368,
122.528548074826)) ;
#49558=CARTESIAN_POINT('Ctrl Pts',(-20.4356383205666,-46.925952344074,122.307725777461)) ;
#49559=CARTESIAN_POINT('Ctrl Pts',(-20.0648823735269,-47.1159227084493,
122.399473602791)) ;
#49560=CARTESIAN_POINT('Ctrl Pts',(-20.2287819479061,-46.9359336280864,
122.146383450111)) ;
#49561=CARTESIAN_POINT('Ctrl Pts',(-19.878210560702,-47.125967010075,122.300821311272)) ;
#49562=CARTESIAN_POINT('Ctrl Pts',(-19.9954418662365,-46.9459779297121,
122.023069093696)) ;
#49563=CARTESIAN_POINT('Ctrl Pts',(-19.6816640223288,-47.1357950912944,
122.236998796321)) ;
#49564=CARTESIAN_POINT('Ctrl Pts',(-19.7497569427276,-46.9558060109315,
121.943291660823)) ;
#49565=CARTESIAN_POINT('Ctrl Pts',(-19.4719363919362,-47.1458716941436,
122.207454533547)) ;
#49566=CARTESIAN_POINT('Ctrl Pts',(-19.4875976586509,-46.9658826137807,
121.90636263565)) ;
#49567=CARTESIAN_POINT('Ctrl Pts',(-19.2648901369236,-47.1557237732621,
122.214511172754)) ;
#49568=CARTESIAN_POINT('Ctrl Pts',(-19.228788648694,-46.9757346928992,121.915184765414)) ;
#49569=CARTESIAN_POINT('Ctrl Pts',(-19.0577050674081,-47.165797031571,122.258180662651)) ;
#49570=CARTESIAN_POINT('Ctrl Pts',(-18.9698079849325,-46.9858079512082,
121.969772870616)) ;
#49571=CARTESIAN_POINT('Ctrl Pts',(-18.8657477434276,-47.1756384909513,
122.335414466867)) ;
#49572=CARTESIAN_POINT('Ctrl Pts',(-18.7298606158885,-46.9956494105884,
122.066316849577)) ;
#49573=CARTESIAN_POINT('Ctrl Pts',(-18.6875856486329,-47.1855995863637,
122.445455661587)) ;
#49574=CARTESIAN_POINT('Ctrl Pts',(-18.507158497528,-47.0056105060008,122.203869923558)) ;
#49575=CARTESIAN_POINT('Ctrl Pts',(-18.5303140250955,-47.1956368707604,
122.586136597021)) ;
#49576=CARTESIAN_POINT('Ctrl Pts',(-18.3105700406655,-47.0156477903975,
122.379722097263)) ;
#49577=CARTESIAN_POINT('Ctrl Pts',(-18.4016481952308,-47.2055132094957,
122.749125228209)) ;
#49578=CARTESIAN_POINT('Ctrl Pts',(-18.1497383800558,-47.0255241291328,
122.583459652795)) ;
#49579=CARTESIAN_POINT('Ctrl Pts',(-18.3013741603539,-47.2155753356489,
122.935356273905)) ;
#49580=CARTESIAN_POINT('Ctrl Pts',(-18.0243973839348,-47.0355862552861,
122.816248967698)) ;
#49581=CARTESIAN_POINT('Ctrl Pts',(-18.2361754948208,-47.2254435096255,
123.132331116174)) ;
#49582=CARTESIAN_POINT('Ctrl Pts',(-17.942900261197,-47.0454544292626,123.062469015826)) ;
#49583=CARTESIAN_POINT('Ctrl Pts',(-18.205338043931,-47.2354490581293,123.340378376433)) ;
#49584=CARTESIAN_POINT('Ctrl Pts',(-17.9043551712799,-47.0554599777664,
123.322528432364)) ;
#49585=CARTESIAN_POINT('Ctrl Pts',(-18.2111535129992,-47.2454316900249,
123.550202526117)) ;
#49586=CARTESIAN_POINT('Ctrl Pts',(-17.911626244223,-47.065442609662,123.58480879542)) ;
#49587=CARTESIAN_POINT('Ctrl Pts',(-18.2537758997071,-47.2554756324466,
123.756993471745)) ;
#49588=CARTESIAN_POINT('Ctrl Pts',(-17.964905818864,-47.0754865520838,123.843296984547)) ;
#49589=CARTESIAN_POINT('Ctrl Pts',(-18.3297319147639,-47.2653037804738,
123.94914374406)) ;
#49590=CARTESIAN_POINT('Ctrl Pts',(-18.0598529385593,-47.0853147001109,
124.083485382796)) ;
#49591=CARTESIAN_POINT('Ctrl Pts',(-18.4391033103602,-47.2752936478482,
124.128436677712)) ;
#49592=CARTESIAN_POINT('Ctrl Pts',(-18.1965689479448,-47.0953045674853,
124.307600675723)) ;
#49593=CARTESIAN_POINT('Ctrl Pts',(-18.5791042370888,-47.2853373868037,
124.286501486607)) ;
#49594=CARTESIAN_POINT('Ctrl Pts',(-18.3715713484641,-47.1053483064408,
124.505180389695)) ;
#49595=CARTESIAN_POINT('Ctrl Pts',(-18.7405005083197,-47.2951591353416,
124.415289290748)) ;
#49596=CARTESIAN_POINT('Ctrl Pts',(-18.5733188648744,-47.1151700549788,
124.666164420579)) ;
#49597=CARTESIAN_POINT('Ctrl Pts',(-18.9254963348016,-47.3051941129514,
124.516697212118)) ;
#49598=CARTESIAN_POINT('Ctrl Pts',(-18.8045645528301,-47.1252050325885,
124.792922450378)) ;
#49599=CARTESIAN_POINT('Ctrl Pts',(-19.1252827024843,-47.3152190257091,
124.583820831396)) ;
#49600=CARTESIAN_POINT('Ctrl Pts',(-19.0542980945525,-47.1352299453462,
124.876825162639)) ;
#49601=CARTESIAN_POINT('Ctrl Pts',(-19.3300236054208,-47.3250709688029,
124.615141144271)) ;
#49602=CARTESIAN_POINT('Ctrl Pts',(-19.3102255315884,-47.14508188844,124.915973693937)) ;
#49603=CARTESIAN_POINT('Ctrl Pts',(-19.5399921824132,-47.335061930132,124.61069150491)) ;
#49604=CARTESIAN_POINT('Ctrl Pts',(-19.5726863790115,-47.1550728497691,
124.910409512825)) ;
#49605=CARTESIAN_POINT('Ctrl Pts',(-19.7445687503477,-47.3449798050004,
124.570275657887)) ;
#49606=CARTESIAN_POINT('Ctrl Pts',(-19.8284072327233,-47.1649907246376,
124.859887472714)) ;
#49607=CARTESIAN_POINT('Ctrl Pts',(-19.9411645038063,-47.3550083240017,
124.494169080804)) ;
#49608=CARTESIAN_POINT('Ctrl Pts',(-20.074151105226,-47.1750192436388,124.764752235649)) ;
#49609=CARTESIAN_POINT('Ctrl Pts',(-20.1190316044298,-47.3648920027995,
124.386736912704)) ;
#49610=CARTESIAN_POINT('Ctrl Pts',(-20.2964844789698,-47.1849029224366,
124.630459757665)) ;
#49611=CARTESIAN_POINT('Ctrl Pts',(-20.2776029483936,-47.3748869462393,
124.248868784575)) ;
#49612=CARTESIAN_POINT('Ctrl Pts',(-20.4946972413566,-47.1948978658764,
124.458122754185)) ;
#49613=CARTESIAN_POINT('Ctrl Pts',(-20.4099687757007,-47.3849138000617,
124.084811617486)) ;
#49614=CARTESIAN_POINT('Ctrl Pts',(-20.6601527760735,-47.2049247196988,
124.253049913782)) ;
#49615=CARTESIAN_POINT('Ctrl Pts',(-20.510642437193,-47.3947979644006,123.90302150782)) ;
#49616=CARTESIAN_POINT('Ctrl Pts',(-20.7859931800233,-47.2148088840377,
124.025810555363)) ;
#49617=CARTESIAN_POINT('Ctrl Pts',(-20.5791870198789,-47.404786062443,123.704564661141)) ;
#49618=CARTESIAN_POINT('Ctrl Pts',(-20.8716717234267,-47.2247969820801,
123.777738571855)) ;
#49619=CARTESIAN_POINT('Ctrl Pts',(-20.6122318337484,-47.4147371689001,
123.497960882242)) ;
#49620=CARTESIAN_POINT('Ctrl Pts',(-20.912975435298,-47.2347480885372,123.519483140428)) ;
#49621=CARTESIAN_POINT('Ctrl Pts',(-20.6087528151844,-47.4247822200682,
123.286823087064)) ;
#49622=CARTESIAN_POINT('Ctrl Pts',(-20.908624300372,-47.2447931397053,123.255561025828)) ;
#49623=CARTESIAN_POINT('Ctrl Pts',(-20.5695080656403,-47.4346439804265,
123.083245164977)) ;
#49624=CARTESIAN_POINT('Ctrl Pts',(-20.8595658745191,-47.2546549000636,
123.001088343712)) ;
#49625=CARTESIAN_POINT('Ctrl Pts',(-20.495357370561,-47.4446067972569,122.88735923458)) ;
#49626=CARTESIAN_POINT('Ctrl Pts',(-20.7668750532524,-47.264617716894,122.756231591829)) ;
#49627=CARTESIAN_POINT('Ctrl Pts',(-20.3872427945494,-47.4546414785377,
122.706219208448)) ;
#49628=CARTESIAN_POINT('Ctrl Pts',(-20.6317297453688,-47.2746523981748,
122.529807845383)) ;
#49629=CARTESIAN_POINT('Ctrl Pts',(-20.2516200642963,-47.4645265083184,
122.548722650758)) ;
#49630=CARTESIAN_POINT('Ctrl Pts',(-20.4621990513068,-47.2845374279556,
122.332938364002)) ;
#49631=CARTESIAN_POINT('Ctrl Pts',(-20.0877899814674,-47.4745921017164,
122.414841028809)) ;
#49632=CARTESIAN_POINT('Ctrl Pts',(-20.2574099722437,-47.2946030213536,
122.16558837992)) ;
#49633=CARTESIAN_POINT('Ctrl Pts',(-19.9073992267312,-47.4844312700779,
122.313551418133)) ;
#49634=CARTESIAN_POINT('Ctrl Pts',(-20.0319196599626,-47.3044421897151,
122.038978242884)) ;
#49635=CARTESIAN_POINT('Ctrl Pts',(-19.7078787306478,-47.4944938678194,
122.243312824082)) ;
#49636=CARTESIAN_POINT('Ctrl Pts',(-19.7825183008089,-47.3145047874566,
121.95118250225)) ;
#49637=CARTESIAN_POINT('Ctrl Pts',(-19.5025547915718,-47.5043908802264,
122.209566875106)) ;
#49638=CARTESIAN_POINT('Ctrl Pts',(-19.5258624977633,-47.3244017998635,
121.909002521009)) ;
#49639=CARTESIAN_POINT('Ctrl Pts',(-19.2937789957374,-47.514322202052,122.211297493397)) ;
#49640=CARTESIAN_POINT('Ctrl Pts',(-19.2648924723534,-47.3343331216891,
121.911168475374)) ;
#49641=CARTESIAN_POINT('Ctrl Pts',(-19.0862316655902,-47.5243639648065,
122.249899659143)) ;
#49642=CARTESIAN_POINT('Ctrl Pts',(-19.0054588236434,-47.3443748844436,
121.959423773206)) ;
#49643=CARTESIAN_POINT('Ctrl Pts',(-18.8914968548924,-47.5342521636972,
122.322686181889)) ;
#49644=CARTESIAN_POINT('Ctrl Pts',(-18.7620408415515,-47.3542630833343,
122.050409572673)) ;
#49645=CARTESIAN_POINT('Ctrl Pts',(-18.7102985265331,-47.544246102297,122.429005812639)) ;
#49646=CARTESIAN_POINT('Ctrl Pts',(-18.5355442147587,-47.3642570219342,
122.18331150089)) ;
#49647=CARTESIAN_POINT('Ctrl Pts',(-18.5511494828585,-47.5541869233339,
122.564478677246)) ;
#49648=CARTESIAN_POINT('Ctrl Pts',(-18.3366094811848,-47.374197842971,122.352654796007)) ;
#49649=CARTESIAN_POINT('Ctrl Pts',(-18.4175024086679,-47.5641463056221,
122.725638878256)) ;
#49650=CARTESIAN_POINT('Ctrl Pts',(-18.1695526330089,-47.3841572252593,
122.554106932035)) ;
#49651=CARTESIAN_POINT('Ctrl Pts',(-18.3133427089413,-47.5741440652745,
122.90822294444)) ;
#49652=CARTESIAN_POINT('Ctrl Pts',(-18.0393553532008,-47.3941549849116,
122.782338451518)) ;
#49653=CARTESIAN_POINT('Ctrl Pts',(-18.2424783139921,-47.5841802014768,
123.106952131826)) ;
#49654=CARTESIAN_POINT('Ctrl Pts',(-17.9507774145601,-47.4041911211139,
123.03075086766)) ;
#49655=CARTESIAN_POINT('Ctrl Pts',(-18.2076066802903,-47.5940309989677,
123.311088085714)) ;
#49656=CARTESIAN_POINT('Ctrl Pts',(-17.9071905133116,-47.4140419186048,
123.285921661673)) ;
#49657=CARTESIAN_POINT('Ctrl Pts',(-18.2080983621174,-47.603991864044,123.520488926134)) ;
#49658=CARTESIAN_POINT('Ctrl Pts',(-17.9078079177087,-47.4240027836811,
123.547672833049)) ;
#49659=CARTESIAN_POINT('Ctrl Pts',(-18.2454476002955,-47.6140207316744,
123.728004942344)) ;
#49660=CARTESIAN_POINT('Ctrl Pts',(-17.9544972057267,-47.4340316513115,
123.807067402969)) ;
#49661=CARTESIAN_POINT('Ctrl Pts',(-18.3173323666115,-47.6239309678108,
123.92354610878)) ;
#49662=CARTESIAN_POINT('Ctrl Pts',(-18.0443558522348,-47.4439418874479,
124.051493099895)) ;
#49663=CARTESIAN_POINT('Ctrl Pts',(-18.4218727530156,-47.6338659211253,
124.10437188864)) ;
#49664=CARTESIAN_POINT('Ctrl Pts',(-18.1750338402729,-47.4538768407624,
124.27752403088)) ;
#49665=CARTESIAN_POINT('Ctrl Pts',(-18.5577961313791,-47.6439068515349,
124.265872819916)) ;
#49666=CARTESIAN_POINT('Ctrl Pts',(-18.3449402389459,-47.463917771172,124.479398422713)) ;
#49667=CARTESIAN_POINT('Ctrl Pts',(-18.7171539318421,-47.6537947483165,
124.399365872321)) ;
#49668=CARTESIAN_POINT('Ctrl Pts',(-18.5441394208993,-47.4738056679536,
124.646262687843)) ;
#49669=CARTESIAN_POINT('Ctrl Pts',(-18.8989130954372,-47.6637841999752,
124.504559353168)) ;
#49670=CARTESIAN_POINT('Ctrl Pts',(-18.7713398491585,-47.4837951196123,
124.777752129253)) ;
#49671=CARTESIAN_POINT('Ctrl Pts',(-19.0956328686204,-47.6737432903405,
124.57621883154)) ;
#49672=CARTESIAN_POINT('Ctrl Pts',(-19.0172406224052,-47.4937542099777,
124.867323859579)) ;
#49673=CARTESIAN_POINT('Ctrl Pts',(-19.3004544560536,-47.6836406026468,
124.612933945687)) ;
#49674=CARTESIAN_POINT('Ctrl Pts',(-19.2732681589925,-47.503651522284,124.913214982479)) ;
#49675=CARTESIAN_POINT('Ctrl Pts',(-19.5118542835427,-47.6936970285471,
124.613436471454)) ;
#49676=CARTESIAN_POINT('Ctrl Pts',(-19.5375180334294,-47.5137079481842,
124.913840318976)) ;
#49677=CARTESIAN_POINT('Ctrl Pts',(-19.7163232652421,-47.7035670311368,
124.577994785846)) ;
#49678=CARTESIAN_POINT('Ctrl Pts',(-19.7931038035126,-47.523577950774,124.86953541503)) ;
#49679=CARTESIAN_POINT('Ctrl Pts',(-19.9142840722972,-47.7135709643141,
124.507042269719)) ;
#49680=CARTESIAN_POINT('Ctrl Pts',(-20.0405538778607,-47.5335818839512,
124.780842159389)) ;
#49681=CARTESIAN_POINT('Ctrl Pts',(-20.0966064940378,-47.723558224778,124.402844984413)) ;
#49682=CARTESIAN_POINT('Ctrl Pts',(-20.2684557085201,-47.5435691444151,
124.650592871632)) ;
#49683=CARTESIAN_POINT('Ctrl Pts',(-20.2585947292332,-47.7335852763637,
124.267974135904)) ;
#49684=CARTESIAN_POINT('Ctrl Pts',(-20.470938720581,-47.5535961960008,124.482002870623)) ;
#49685=CARTESIAN_POINT('Ctrl Pts',(-20.393034986563,-47.7434763661898,124.109317573844)) ;
#49686=CARTESIAN_POINT('Ctrl Pts',(-20.6389889194383,-47.5634872858269,
124.283677447582)) ;
#49687=CARTESIAN_POINT('Ctrl Pts',(-20.5342723905065,-47.7567741209708,
123.868088225556)) ;
#49688=CARTESIAN_POINT('Ctrl Pts',(-20.8155222736475,-47.576785040608,123.982153459967)) ;
#49689=CARTESIAN_POINT('Ctrl Pts',(-20.6091851589647,-47.769972180579,123.597577696433)) ;
#49690=CARTESIAN_POINT('Ctrl Pts',(-20.9091627271371,-47.5899831002161,
123.644050843664)) ;
#49691=CARTESIAN_POINT('Ctrl Pts',(-20.6114219199646,-47.7833689211482,
123.316008276815)) ;
#49692=CARTESIAN_POINT('Ctrl Pts',(-20.911961468793,-47.6033798407853,123.29203099922)) ;
#49693=CARTESIAN_POINT('Ctrl Pts',(-20.5772346324987,-47.7932398332216,
123.111276079564)) ;
#49694=CARTESIAN_POINT('Ctrl Pts',(-20.8692234169841,-47.6132507528587,
123.036128094905)) ;
#49695=CARTESIAN_POINT('Ctrl Pts',(-20.506620197884,-47.8033133949897,122.911669655053)) ;
#49696=CARTESIAN_POINT('Ctrl Pts',(-20.7809529679,-47.6233243146269,122.78661751852)) ;
#49697=CARTESIAN_POINT('Ctrl Pts',(-20.4051985250744,-47.8131348075781,
122.731761328968)) ;
#49698=CARTESIAN_POINT('Ctrl Pts',(-20.6541739490141,-47.6331457272152,
122.561735103917)) ;
#49699=CARTESIAN_POINT('Ctrl Pts',(-20.2709276734717,-47.8232088248091,
122.568046641826)) ;
#49700=CARTESIAN_POINT('Ctrl Pts',(-20.4863320285724,-47.6432197444462,
122.357091382162)) ;
#49701=CARTESIAN_POINT('Ctrl Pts',(-20.0611060975047,-47.8363676117737,
122.387657282842)) ;
#49702=CARTESIAN_POINT('Ctrl Pts',(-20.2240587467137,-47.6563785314108,
122.131615915309)) ;
#49703=CARTESIAN_POINT('Ctrl Pts',(-19.805342502725,-47.8497337148678,122.263873713802)) ;
#49704=CARTESIAN_POINT('Ctrl Pts',(-19.904396611808,-47.669744634505,121.976897634996)) ;
#49705=CARTESIAN_POINT('Ctrl Pts',(-19.5302562535324,-47.8630476497569,
122.211981763288)) ;
#49706=CARTESIAN_POINT('Ctrl Pts',(-19.5604802159987,-47.683058569394,121.912018372431)) ;
#49707=CARTESIAN_POINT('Ctrl Pts',(-19.3221676696211,-47.8729476892044,
122.209028722341)) ;
#49708=CARTESIAN_POINT('Ctrl Pts',(-19.3003815270742,-47.6929586088415,
121.908333183184)) ;
#49709=CARTESIAN_POINT('Ctrl Pts',(-19.115305104631,-47.8829120923389,122.242126287116)) ;
#49710=CARTESIAN_POINT('Ctrl Pts',(-19.0418005240808,-47.702923011976,121.949706846036)) ;
#49711=CARTESIAN_POINT('Ctrl Pts',(-18.9160968655024,-47.89294205946,122.311266661747)) ;
#49712=CARTESIAN_POINT('Ctrl Pts',(-18.7927924422109,-47.7129529790972,
122.036134213176)) ;
#49713=CARTESIAN_POINT('Ctrl Pts',(-18.7342345587612,-47.9028443360691,
122.412551802451)) ;
#49714=CARTESIAN_POINT('Ctrl Pts',(-18.5654632174081,-47.7228552557062,
122.162745640329)) ;
#49715=CARTESIAN_POINT('Ctrl Pts',(-18.5173604794192,-47.9161102652382,
122.58797464885)) ;
#49716=CARTESIAN_POINT('Ctrl Pts',(-18.2943866086344,-47.7361211848754,
122.382011147429)) ;
#49717=CARTESIAN_POINT('Ctrl Pts',(-18.309565842614,-47.9327317963447,122.873754193906)) ;
#49718=CARTESIAN_POINT('Ctrl Pts',(-18.0346303797176,-47.7527427159818,
122.739250673809)) ;
#49719=CARTESIAN_POINT('Ctrl Pts',(-18.1920101676508,-47.9526066249893,
123.279717316389)) ;
#49720=CARTESIAN_POINT('Ctrl Pts',(-17.8876997701404,-47.7726175446265,
123.246720784385)) ;
#49721=CARTESIAN_POINT('Ctrl Pts',(-18.2154597866439,-47.9692798330912,
123.633471891769)) ;
#49722=CARTESIAN_POINT('Ctrl Pts',(-17.917000592734,-47.7892907527283,123.68884871812)) ;
#49723=CARTESIAN_POINT('Ctrl Pts',(-18.3053614681726,-47.9825309580725,
123.897116716914)) ;
#49724=CARTESIAN_POINT('Ctrl Pts',(-18.0293936752082,-47.8025418777096,
124.018462677686)) ;
#49725=CARTESIAN_POINT('Ctrl Pts',(-18.4387378594094,-47.9957732768933,
124.141560057195)) ;
#49726=CARTESIAN_POINT('Ctrl Pts',(-18.1961054880451,-47.8157841965304,
124.323995100748)) ;
#49727=CARTESIAN_POINT('Ctrl Pts',(-18.6845127413368,-48.0125065172328,
124.39871352638)) ;
#49728=CARTESIAN_POINT('Ctrl Pts',(-18.5033373266895,-47.8325174368699,
124.645448284564)) ;
#49729=CARTESIAN_POINT('Ctrl Pts',(-19.0624327367419,-48.0323356654207,
124.585830606366)) ;
#49730=CARTESIAN_POINT('Ctrl Pts',(-18.9757346113331,-47.8523465850579,
124.879336049279)) ;
#49731=CARTESIAN_POINT('Ctrl Pts',(-19.4832475920745,-48.0522603605214,
124.633977070229)) ;
#49732=CARTESIAN_POINT('Ctrl Pts',(-19.5017537468954,-47.8722712801585,
124.939516678205)) ;
#49733=CARTESIAN_POINT('Ctrl Pts',(-19.8953466515693,-48.0721835891048,
124.53556105767)) ;
#49734=CARTESIAN_POINT('Ctrl Pts',(-20.016875861944,-47.8921945087419,124.816493222092)) ;
#49735=CARTESIAN_POINT('Ctrl Pts',(-20.2491680892978,-48.0921107282309,
124.302550900816)) ;
#49736=CARTESIAN_POINT('Ctrl Pts',(-20.4591503180632,-47.912121647868,124.525228376918)) ;
#49737=CARTESIAN_POINT('Ctrl Pts',(-20.5020771655509,-48.1119871908466,
123.963916176458)) ;
#49738=CARTESIAN_POINT('Ctrl Pts',(-20.7752836476955,-47.9319981104837,
124.101934449769)) ;
#49739=CARTESIAN_POINT('Ctrl Pts',(-20.6250718690425,-48.1319644194519,
123.557348462164)) ;
#49740=CARTESIAN_POINT('Ctrl Pts',(-20.9290246638759,-47.951975339089,123.593724361099)) ;
#49741=CARTESIAN_POINT('Ctrl Pts',(-20.6016537275589,-48.1518992774256,
123.134089906052)) ;
#49742=CARTESIAN_POINT('Ctrl Pts',(-20.899749641412,-47.9719101970627,123.064652071563)) ;
#49743=CARTESIAN_POINT('Ctrl Pts',(-20.4359503230159,-48.1717957263564,
122.744874511836)) ;
#49744=CARTESIAN_POINT('Ctrl Pts',(-20.6926191392148,-47.9918066459935,
122.578134849579)) ;
#49745=CARTESIAN_POINT('Ctrl Pts',(-20.1473267208655,-48.191717010423,122.434822386439)) ;
#49746=CARTESIAN_POINT('Ctrl Pts',(-20.3318393279067,-48.0117279300601,
122.190571444876)) ;
#49747=CARTESIAN_POINT('Ctrl Pts',(-19.7694900246731,-48.2116736600939,
122.241648838417)) ;
#49748=CARTESIAN_POINT('Ctrl Pts',(-19.859543379667,-48.0316845797311,121.949105900427)) ;
#49749=CARTESIAN_POINT('Ctrl Pts',(-19.3501801167776,-48.2315509532055,
122.189092571805)) ;
#49750=CARTESIAN_POINT('Ctrl Pts',(-19.3354077539481,-48.0515618728427,
121.883411775971)) ;
#49751=CARTESIAN_POINT('Ctrl Pts',(-18.9375691670233,-48.251437425434,122.281750555441)) ;
#49752=CARTESIAN_POINT('Ctrl Pts',(-18.8196458602332,-48.0714483450711,
121.999233714919)) ;
#49753=CARTESIAN_POINT('Ctrl Pts',(-18.5785832798502,-48.271498991358,122.512179757162)) ;
#49754=CARTESIAN_POINT('Ctrl Pts',(-18.3709126385938,-48.0915099109951,
122.287270877205)) ;
#49755=CARTESIAN_POINT('Ctrl Pts',(-18.3229725036018,-48.2913393988987,
122.847760478558)) ;
#49756=CARTESIAN_POINT('Ctrl Pts',(-18.0514008754144,-48.1113503185359,
122.706744756814)) ;
#49757=CARTESIAN_POINT('Ctrl Pts',(-18.1954566816947,-48.3111907228717,
123.250147542051)) ;
#49758=CARTESIAN_POINT('Ctrl Pts',(-17.8920053839532,-48.1312016425088,
123.209726070964)) ;
#49759=CARTESIAN_POINT('Ctrl Pts',(-18.2137292660296,-48.3312439928231,
123.676086435332)) ;
#49760=CARTESIAN_POINT('Ctrl Pts',(-17.9148449517258,-48.1512549124602,
123.742150506195)) ;
#49761=CARTESIAN_POINT('Ctrl Pts',(-18.3743522701606,-48.3510646502064,
124.065843827562)) ;
#49762=CARTESIAN_POINT('Ctrl Pts',(-18.1156214422887,-48.1710755698436,
124.229345578872)) ;
#49763=CARTESIAN_POINT('Ctrl Pts',(-18.6598163322656,-48.3710360715369,
124.380035479297)) ;
#49764=CARTESIAN_POINT('Ctrl Pts',(-18.4724496628158,-48.1910469911741,
124.622086302263)) ;
#49765=CARTESIAN_POINT('Ctrl Pts',(-19.0341051163834,-48.3909295639006,
124.577408934611)) ;
#49766=CARTESIAN_POINT('Ctrl Pts',(-18.9403084788893,-48.2109404835378,
124.86880464151)) ;
#49767=CARTESIAN_POINT('Ctrl Pts',(-19.4558297886332,-48.4109536501417,
124.635272002044)) ;
#49768=CARTESIAN_POINT('Ctrl Pts',(-19.4674642242549,-48.2309645697788,
124.941135895711)) ;
#49769=CARTESIAN_POINT('Ctrl Pts',(-19.8676091497869,-48.4307585292546,
124.54692460703)) ;
#49770=CARTESIAN_POINT('Ctrl Pts',(-19.982186864098,-48.2507694488917,124.830704772301)) ;
#49771=CARTESIAN_POINT('Ctrl Pts',(-20.2278594836264,-48.4507175449524,
124.322628489146)) ;
#49772=CARTESIAN_POINT('Ctrl Pts',(-20.4325013285474,-48.2707284645896,
124.550337764469)) ;
#49773=CARTESIAN_POINT('Ctrl Pts',(-20.4895249553124,-48.4707035685815,
123.987793204805)) ;
#49774=CARTESIAN_POINT('Ctrl Pts',(-20.7595855617661,-48.2907144882186,
124.131795730191)) ;
#49775=CARTESIAN_POINT('Ctrl Pts',(-20.620851700236,-48.490512064342,123.587567929602)) ;
#49776=CARTESIAN_POINT('Ctrl Pts',(-20.9237469669242,-48.3105229839791,
123.631516939085)) ;
#49777=CARTESIAN_POINT('Ctrl Pts',(-20.6081359744809,-48.5104947034476,
123.162963885691)) ;
#49778=CARTESIAN_POINT('Ctrl Pts',(-20.9078563777569,-48.3305056230847,
123.100761863428)) ;
#49779=CARTESIAN_POINT('Ctrl Pts',(-20.4519095426807,-48.5303761512416,
122.770042814153)) ;
#49780=CARTESIAN_POINT('Ctrl Pts',(-20.7125774921877,-48.3503870708787,
122.609609792286)) ;
#49781=CARTESIAN_POINT('Ctrl Pts',(-20.1703007545969,-48.5503326179791,
122.452751245619)) ;
#49782=CARTESIAN_POINT('Ctrl Pts',(-20.3605699834758,-48.3703435376163,
122.212992650453)) ;
#49783=CARTESIAN_POINT('Ctrl Pts',(-19.7987956805758,-48.5702100149347,
122.251075325285)) ;
#49784=CARTESIAN_POINT('Ctrl Pts',(-19.8961915070511,-48.3902209345718,
121.960894036844)) ;
#49785=CARTESIAN_POINT('Ctrl Pts',(-19.3787174367408,-48.59019196111,122.187732374788)) ;
#49786=CARTESIAN_POINT('Ctrl Pts',(-19.3710944052881,-48.4102028807471,
121.881710834972)) ;
#49787=CARTESIAN_POINT('Ctrl Pts',(-18.9632548947561,-48.6101210601467,
122.271556210172)) ;
#49788=CARTESIAN_POINT('Ctrl Pts',(-18.8517658005324,-48.4301319797839,
121.986485155074)) ;
#49789=CARTESIAN_POINT('Ctrl Pts',(-18.6014532782387,-48.6300496833594,
122.491970120177)) ;
#49790=CARTESIAN_POINT('Ctrl Pts',(-18.3995108077568,-48.4500606029965,
122.262000851826)) ;
#49791=CARTESIAN_POINT('Ctrl Pts',(-18.3371474305036,-48.6498840074658,
122.820662580448)) ;
#49792=CARTESIAN_POINT('Ctrl Pts',(-18.0691275875861,-48.4698949271029,
122.672852581631)) ;
#49793=CARTESIAN_POINT('Ctrl Pts',(-18.2224259879656,-48.6665362948492,
123.155533978461)) ;
#49794=CARTESIAN_POINT('Ctrl Pts',(-17.9257131670204,-48.4865472144863,
123.091471777967)) ;
#49795=CARTESIAN_POINT('Ctrl Pts',(-18.2035092636524,-48.6797967958714,
123.433741752069)) ;
#49796=CARTESIAN_POINT('Ctrl Pts',(-17.9020712050957,-48.4998077155085,
123.439203218313)) ;
#49797=CARTESIAN_POINT('Ctrl Pts',(-18.2254971301078,-48.6897982730727,
123.64284321915)) ;
#49798=CARTESIAN_POINT('Ctrl Pts',(-17.9295520562288,-48.5098091927098,
123.700586123899)) ;
#49799=CARTESIAN_POINT('Ctrl Pts',(-18.2839780007626,-48.6998302939322,
123.845485351349)) ;
#49800=CARTESIAN_POINT('Ctrl Pts',(-18.002650404669,-48.5198412135693,123.953887639431)) ;
#49801=CARTESIAN_POINT('Ctrl Pts',(-18.3749627895114,-48.7096938376577,
124.03181215673)) ;
#49802=CARTESIAN_POINT('Ctrl Pts',(-18.116381192127,-48.5297047572949,124.186799307421)) ;
#49803=CARTESIAN_POINT('Ctrl Pts',(-18.4977838557843,-48.7196625513279,
124.201640045108)) ;
#49804=CARTESIAN_POINT('Ctrl Pts',(-18.2698960730485,-48.539673470965,124.399078392856)) ;
#49805=CARTESIAN_POINT('Ctrl Pts',(-18.6994061492759,-48.7330082987316,
124.396656788491)) ;
#49806=CARTESIAN_POINT('Ctrl Pts',(-18.5219675225796,-48.5530192183687,
124.642888173834)) ;
#49807=CARTESIAN_POINT('Ctrl Pts',(-18.9435543299916,-48.7461588538042,
124.533062447628)) ;
#49808=CARTESIAN_POINT('Ctrl Pts',(-18.8271260677206,-48.5661697734414,
124.813370160914)) ;
#49809=CARTESIAN_POINT('Ctrl Pts',(-19.2163009315313,-48.7595442343541,
124.602291897744)) ;
#49810=CARTESIAN_POINT('Ctrl Pts',(-19.1680417733709,-48.5795551539912,
124.899907926004)) ;
#49811=CARTESIAN_POINT('Ctrl Pts',(-19.4236287954365,-48.7694321703469,
124.617669125966)) ;
#49812=CARTESIAN_POINT('Ctrl Pts',(-19.4272046606678,-48.5894430899841,
124.919132760716)) ;
#49813=CARTESIAN_POINT('Ctrl Pts',(-19.6326234694383,-48.7794233601596,
124.59695356156)) ;
#49814=CARTESIAN_POINT('Ctrl Pts',(-19.6884474342547,-48.5994342797967,
124.893240945766)) ;
#49815=CARTESIAN_POINT('Ctrl Pts',(-19.8341362224527,-48.7893754586979,
124.54055689342)) ;
#49816=CARTESIAN_POINT('Ctrl Pts',(-19.9403393905158,-48.609386378335,124.822747843543)) ;
#49817=CARTESIAN_POINT('Ctrl Pts',(-20.0244791000905,-48.7994217151483,
124.449067132527)) ;
#49818=CARTESIAN_POINT('Ctrl Pts',(-20.1782692262088,-48.6194326347855,
124.708388111913)) ;
#49819=CARTESIAN_POINT('Ctrl Pts',(-20.1927872751713,-48.8092711625425,
124.328441823876)) ;
#49820=CARTESIAN_POINT('Ctrl Pts',(-20.3886560573569,-48.6292820821796,
124.557608789877)) ;
#49821=CARTESIAN_POINT('Ctrl Pts',(-20.3397216534064,-48.8192338150376,
124.179192839321)) ;
#49822=CARTESIAN_POINT('Ctrl Pts',(-20.572326095922,-48.6392447346748,124.371049479693)) ;
#49823=CARTESIAN_POINT('Ctrl Pts',(-20.4590010872859,-48.8292569006798,
124.005486486065)) ;
#49824=CARTESIAN_POINT('Ctrl Pts',(-20.7214277473186,-48.6492678203169,
124.153918077393)) ;
#49825=CARTESIAN_POINT('Ctrl Pts',(-20.5456810010499,-48.8391820164367,
123.815659921871)) ;
#49826=CARTESIAN_POINT('Ctrl Pts',(-20.8297802315917,-48.6591929360738,
123.916635975645)) ;
#49827=CARTESIAN_POINT('Ctrl Pts',(-20.5986636057936,-48.8492344948365,
123.611094978186)) ;
#49828=CARTESIAN_POINT('Ctrl Pts',(-20.8960112318138,-48.6692454144736,
123.660930444406)) ;
#49829=CARTESIAN_POINT('Ctrl Pts',(-20.6151308206564,-48.8590859935392,
123.4046256451)) ;
#49830=CARTESIAN_POINT('Ctrl Pts',(-20.9165980681484,-48.6790969131764,
123.402843889694)) ;
#49831=CARTESIAN_POINT('Ctrl Pts',(-20.5958067267319,-48.8690577327418,
123.19590749213)) ;
#49832=CARTESIAN_POINT('Ctrl Pts',(-20.8924457354999,-48.6890686523789,
123.141945824781)) ;
#49833=CARTESIAN_POINT('Ctrl Pts',(-20.5403646088462,-48.8790529405074,
122.993187529069)) ;
#49834=CARTESIAN_POINT('Ctrl Pts',(-20.8231457686488,-48.6990638601446,
122.888545055584)) ;
#49835=CARTESIAN_POINT('Ctrl Pts',(-20.4500071936649,-48.8890869419765,
122.802593518848)) ;
#49836=CARTESIAN_POINT('Ctrl Pts',(-20.71020152793,-48.7090978616136,122.650301300846)) ;
#49837=CARTESIAN_POINT('Ctrl Pts',(-20.3303491214858,-48.8989423000689,
122.633423450339)) ;
#49838=CARTESIAN_POINT('Ctrl Pts',(-20.5606310889083,-48.718953219706,122.438836911348)) ;
#49839=CARTESIAN_POINT('Ctrl Pts',(-20.1812231910538,-48.9089417756622,
122.485307584382)) ;
#49840=CARTESIAN_POINT('Ctrl Pts',(-20.3742255768515,-48.7289526952993,
122.253690036881)) ;
#49841=CARTESIAN_POINT('Ctrl Pts',(-20.0105298951127,-48.9188362241573,
122.366356746529)) ;
#49842=CARTESIAN_POINT('Ctrl Pts',(-20.1608603226581,-48.7388471437944,
122.104999075767)) ;
#49843=CARTESIAN_POINT('Ctrl Pts',(-19.8186007680799,-48.928899348385,122.277447738823)) ;
#49844=CARTESIAN_POINT('Ctrl Pts',(-19.9209501103882,-48.7489102680221,
121.993860313604)) ;
#49845=CARTESIAN_POINT('Ctrl Pts',(-19.6186814141664,-48.9387389747136,
122.224180471466)) ;
#49846=CARTESIAN_POINT('Ctrl Pts',(-19.6710512311322,-48.7587498943507,
121.927273469944)) ;
#49847=CARTESIAN_POINT('Ctrl Pts',(-19.4079521083204,-48.9488022097566,
122.205769170469)) ;
#49848=CARTESIAN_POINT('Ctrl Pts',(-19.4076398792598,-48.7688131293937,
121.904256633562)) ;
#49849=CARTESIAN_POINT('Ctrl Pts',(-19.2007357621224,-48.9586962149906,
122.224096611744)) ;
#49850=CARTESIAN_POINT('Ctrl Pts',(-19.1486188793919,-48.7787071346277,
121.927163232832)) ;
#49851=CARTESIAN_POINT('Ctrl Pts',(-18.9987560013201,-48.9686389282064,
122.277825494424)) ;
#49852=CARTESIAN_POINT('Ctrl Pts',(-18.8961432339119,-48.7886498478435,
121.99432181877)) ;
#49853=CARTESIAN_POINT('Ctrl Pts',(-18.8079128243991,-48.9786446680046,
122.36634819626)) ;
#49854=CARTESIAN_POINT('Ctrl Pts',(-18.6575880747036,-48.7986555876417,
122.104972809918)) ;
#49855=CARTESIAN_POINT('Ctrl Pts',(-18.6352354087058,-48.988665570151,122.48702462515)) ;
#49856=CARTESIAN_POINT('Ctrl Pts',(-18.4417397385889,-48.8086764897881,
122.255816146101)) ;
#49857=CARTESIAN_POINT('Ctrl Pts',(-18.4878939976367,-48.9985563401998,
122.633756235366)) ;
#49858=CARTESIAN_POINT('Ctrl Pts',(-18.2575608011542,-48.818567259837,122.439229061463)) ;
#49859=CARTESIAN_POINT('Ctrl Pts',(-18.366802071252,-49.0085477509796,122.805381393975)) ;
#49860=CARTESIAN_POINT('Ctrl Pts',(-18.106193675921,-48.8285586706167,122.653759103654)) ;
#49861=CARTESIAN_POINT('Ctrl Pts',(-18.2777961208184,-49.0184960966441,
122.994637884771)) ;
#49862=CARTESIAN_POINT('Ctrl Pts',(-17.9949337392161,-48.8385070162812,
122.890328842219)) ;
#49863=CARTESIAN_POINT('Ctrl Pts',(-18.2225909158697,-49.0284409547052,
123.196309162691)) ;
#49864=CARTESIAN_POINT('Ctrl Pts',(-17.9259246879504,-48.8484518743424,
123.142417551886)) ;
#49865=CARTESIAN_POINT('Ctrl Pts',(-18.2033401476526,-49.0384957900982,
123.40679518885)) ;
#49866=CARTESIAN_POINT('Ctrl Pts',(-17.9018586345267,-48.8585067097353,
123.405524737978)) ;
#49867=CARTESIAN_POINT('Ctrl Pts',(-18.2201677805228,-49.0483181621996,
123.612623482533)) ;
#49868=CARTESIAN_POINT('Ctrl Pts',(-17.9228907005279,-48.8683290818368,
123.662811089171)) ;
#49869=CARTESIAN_POINT('Ctrl Pts',(-18.2733451038834,-49.0583740296434,
123.817216281984)) ;
#49870=CARTESIAN_POINT('Ctrl Pts',(-17.9893599290882,-48.8783849492805,
123.918552606262)) ;
#49871=CARTESIAN_POINT('Ctrl Pts',(-18.3605807016632,-49.0683147595013,
124.007132559612)) ;
#49872=CARTESIAN_POINT('Ctrl Pts',(-18.0984022475195,-48.8883256791384,
124.155949320405)) ;
#49873=CARTESIAN_POINT('Ctrl Pts',(-18.478492080276,-49.0782190980524,124.178754700712)) ;
#49874=CARTESIAN_POINT('Ctrl Pts',(-18.2457897778608,-48.8982300176895,
124.370478803514)) ;
#49875=CARTESIAN_POINT('Ctrl Pts',(-18.6265896771452,-49.0882657794809,
124.329321820747)) ;
#49876=CARTESIAN_POINT('Ctrl Pts',(-18.4309099578703,-48.908276699118,124.558689346407)) ;
#49877=CARTESIAN_POINT('Ctrl Pts',(-18.7959241485075,-49.0981612869501,
124.450228240295)) ;
#49878=CARTESIAN_POINT('Ctrl Pts',(-18.6425771224679,-48.9181722065873,
124.709824664085)) ;
#49879=CARTESIAN_POINT('Ctrl Pts',(-18.9867862815912,-49.1082235554488,
124.541375926304)) ;
#49880=CARTESIAN_POINT('Ctrl Pts',(-18.8811535876977,-48.9282344750859,
124.823761366572)) ;
#49881=CARTESIAN_POINT('Ctrl Pts',(-19.1861338900622,-49.1180655457194,
124.596897992535)) ;
#49882=CARTESIAN_POINT('Ctrl Pts',(-19.1303382919628,-48.9380764653565,
124.893166471091)) ;
#49883=CARTESIAN_POINT('Ctrl Pts',(-19.3951586958825,-49.1280589626003,
124.617736026602)) ;
#49884=CARTESIAN_POINT('Ctrl Pts',(-19.3916192445913,-48.9480698822375,
124.919216288475)) ;
#49885=CARTESIAN_POINT('Ctrl Pts',(-19.6032371853687,-49.1379834504525,
124.602087040925)) ;
#49886=CARTESIAN_POINT('Ctrl Pts',(-19.6517180268275,-48.9579943700896,
124.899657271309)) ;
#49887=CARTESIAN_POINT('Ctrl Pts',(-19.8069854701028,-49.147983084361,124.550380447897)) ;
#49888=CARTESIAN_POINT('Ctrl Pts',(-19.9064040385048,-48.9679940039981,
124.835026142014)) ;
#49889=CARTESIAN_POINT('Ctrl Pts',(-19.9984490408071,-49.1579691946177,
124.464185024781)) ;
#49890=CARTESIAN_POINT('Ctrl Pts',(-20.145734566015,-48.9779801142549,124.72728379971)) ;
#49891=CARTESIAN_POINT('Ctrl Pts',(-20.1727370286862,-49.1680051458049,
124.345311201538)) ;
#49892=CARTESIAN_POINT('Ctrl Pts',(-20.363595758635,-48.988016065442,124.578693439179)) ;
#49893=CARTESIAN_POINT('Ctrl Pts',(-20.3212855419175,-49.1778617841397,
124.200809116619)) ;
#49894=CARTESIAN_POINT('Ctrl Pts',(-20.5492835774246,-48.9978727037768,
124.398066759077)) ;
#49895=CARTESIAN_POINT('Ctrl Pts',(-20.4444358570333,-49.1878607442177,
124.030495135267)) ;
#49896=CARTESIAN_POINT('Ctrl Pts',(-20.7032232576622,-49.0078716638548,
124.185175408038)) ;
#49897=CARTESIAN_POINT('Ctrl Pts',(-20.5354258116152,-49.1977559745315,
123.843382253148)) ;
#49898=CARTESIAN_POINT('Ctrl Pts',(-20.8169628556699,-49.0177668941686,
123.951284538968)) ;
#49899=CARTESIAN_POINT('Ctrl Pts',(-20.5934596272314,-49.2078164870001,
123.640024401084)) ;
#49900=CARTESIAN_POINT('Ctrl Pts',(-20.8895070310717,-49.0278274066372,
123.697088016909)) ;
#49901=CARTESIAN_POINT('Ctrl Pts',(-20.614964621342,-49.2176657785463,123.434065207261)) ;
#49902=CARTESIAN_POINT('Ctrl Pts',(-20.9163903855367,-49.0376766981834,
123.439638200355)) ;
#49903=CARTESIAN_POINT('Ctrl Pts',(-20.6006524939482,-49.2276929644785,
123.223753772235)) ;
#49904=CARTESIAN_POINT('Ctrl Pts',(-20.8985020837487,-49.0477038841156,
123.176748817994)) ;
#49905=CARTESIAN_POINT('Ctrl Pts',(-20.5494925233518,-49.2377215009378,
123.019212625671)) ;
#49906=CARTESIAN_POINT('Ctrl Pts',(-20.8345541010092,-49.0577324205749,
122.921071960557)) ;
#49907=CARTESIAN_POINT('Ctrl Pts',(-20.4655325528851,-49.2475667409028,
122.830041408162)) ;
#49908=CARTESIAN_POINT('Ctrl Pts',(-20.7296054273253,-49.0675776605399,
122.68460614522)) ;
#49909=CARTESIAN_POINT('Ctrl Pts',(-20.3487525475356,-49.257557435826,122.655457201128)) ;
#49910=CARTESIAN_POINT('Ctrl Pts',(-20.5836317515741,-49.0775683554631,
122.466374760989)) ;
#49911=CARTESIAN_POINT('Ctrl Pts',(-20.2024139642059,-49.2675952565846,
122.503414527449)) ;
#49912=CARTESIAN_POINT('Ctrl Pts',(-20.4007099669352,-49.0876061762217,
122.276320211683)) ;
#49913=CARTESIAN_POINT('Ctrl Pts',(-20.0353851635832,-49.2774398503615,
122.381196686235)) ;
#49914=CARTESIAN_POINT('Ctrl Pts',(-20.1919240683842,-49.0974507699987,
122.123545795109)) ;
#49915=CARTESIAN_POINT('Ctrl Pts',(-19.8472610421014,-49.2874238457376,
122.288151641728)) ;
#49916=CARTESIAN_POINT('Ctrl Pts',(-19.9567693977097,-49.1074347653747,
122.00723791885)) ;
#49917=CARTESIAN_POINT('Ctrl Pts',(-19.6465098945046,-49.297372894299,122.229404619294)) ;
#49918=CARTESIAN_POINT('Ctrl Pts',(-19.705830459049,-49.1173838139361,121.933802445044)) ;
#49919=CARTESIAN_POINT('Ctrl Pts',(-19.4375191683223,-49.3073753332735,
122.206058321571)) ;
#49920=CARTESIAN_POINT('Ctrl Pts',(-19.4445921214419,-49.1273862529106,
121.904618015651)) ;
#49921=CARTESIAN_POINT('Ctrl Pts',(-19.2272793153479,-49.3173965745699,
122.219664475617)) ;
#49922=CARTESIAN_POINT('Ctrl Pts',(-19.1817922313132,-49.137407494207,121.921624060379)) ;
#49923=CARTESIAN_POINT('Ctrl Pts',(-19.0251633000382,-49.3272892530094,
122.268684611015)) ;
#49924=CARTESIAN_POINT('Ctrl Pts',(-18.9291459751133,-49.1473001726465,
121.982897915693)) ;
#49925=CARTESIAN_POINT('Ctrl Pts',(-18.8326207757844,-49.337279306957,122.352565184891)) ;
#49926=CARTESIAN_POINT('Ctrl Pts',(-18.6884670363836,-49.1572902265941,
122.087747388181)) ;
#49927=CARTESIAN_POINT('Ctrl Pts',(-18.65820968593,-49.3472376681055,122.468356623585)) ;
#49928=CARTESIAN_POINT('Ctrl Pts',(-18.4704519830292,-49.1672485877426,
122.232485671817)) ;
#49929=CARTESIAN_POINT('Ctrl Pts',(-18.5070800115735,-49.3571372949903,
122.611463780261)) ;
#49930=CARTESIAN_POINT('Ctrl Pts',(-18.2815383415692,-49.1771482146274,
122.411369259889)) ;
#49931=CARTESIAN_POINT('Ctrl Pts',(-18.3813177298446,-49.3671851917937,
122.781158712775)) ;
#49932=CARTESIAN_POINT('Ctrl Pts',(-18.1243345330828,-49.1871961114308,
122.623486945981)) ;
#49933=CARTESIAN_POINT('Ctrl Pts',(-18.2881930918701,-49.3770805494297,
122.96721883373)) ;
#49934=CARTESIAN_POINT('Ctrl Pts',(-18.0079271717103,-49.1970914690668,
122.856062333984)) ;
#49935=CARTESIAN_POINT('Ctrl Pts',(-18.2277777790016,-49.3871422018863,
123.169910866014)) ;
#49936=CARTESIAN_POINT('Ctrl Pts',(-17.9324068931307,-49.2071531215235,
123.109426695893)) ;
#49937=CARTESIAN_POINT('Ctrl Pts',(-18.2039634409259,-49.3969868061583,
123.375507420365)) ;
#49938=CARTESIAN_POINT('Ctrl Pts',(-17.9026375541845,-49.2169977257954,
123.366423552934)) ;
#49939=CARTESIAN_POINT('Ctrl Pts',(-18.21560282813,-49.4069469278563,123.584573029196)) ;
#49940=CARTESIAN_POINT('Ctrl Pts',(-17.9171858178237,-49.2269578474934,
123.62775607521)) ;
#49941=CARTESIAN_POINT('Ctrl Pts',(-18.2641366558949,-49.4169849622188,
123.789939361942)) ;
#49942=CARTESIAN_POINT('Ctrl Pts',(-17.9778519477484,-49.2369958818559,
123.884464098742)) ;
#49943=CARTESIAN_POINT('Ctrl Pts',(-18.3458936811806,-49.4268592748053,
123.980778500139)) ;
#49944=CARTESIAN_POINT('Ctrl Pts',(-18.0800477463435,-49.2468701944424,
124.123014445666)) ;
#49945=CARTESIAN_POINT('Ctrl Pts',(-18.4617697259283,-49.436928755588,124.1579063665)) ;
#49946=CARTESIAN_POINT('Ctrl Pts',(-18.2248917333607,-49.2569396752251,
124.344424493672)) ;
#49947=CARTESIAN_POINT('Ctrl Pts',(-18.6032069971224,-49.4467630916051,
124.308729317286)) ;
#49948=CARTESIAN_POINT('Ctrl Pts',(-18.4016886197062,-49.2667740112422,
124.532954912051)) ;
#49949=CARTESIAN_POINT('Ctrl Pts',(-18.7716598122527,-49.4567960493333,
124.435654755595)) ;
#49950=CARTESIAN_POINT('Ctrl Pts',(-18.612254092902,-49.2768069689704,124.691612235755)) ;
#49951=CARTESIAN_POINT('Ctrl Pts',(-18.9596285266735,-49.4668164479085,
124.530768810622)) ;
#49952=CARTESIAN_POINT('Ctrl Pts',(-18.8472145112584,-49.2868273675456,
124.810505656813)) ;
#49953=CARTESIAN_POINT('Ctrl Pts',(-19.1580012266402,-49.4766820216797,
124.591362825177)) ;
#49954=CARTESIAN_POINT('Ctrl Pts',(-19.0951813191321,-49.2966929413168,
124.886249263445)) ;
#49955=CARTESIAN_POINT('Ctrl Pts',(-19.3680870984409,-49.4867508963358,
124.617111323159)) ;
#49956=CARTESIAN_POINT('Ctrl Pts',(-19.3577881565911,-49.3067618159729,
124.918435602837)) ;
#49957=CARTESIAN_POINT('Ctrl Pts',(-19.5747954024805,-49.4965963272413,
124.606267618942)) ;
#49958=CARTESIAN_POINT('Ctrl Pts',(-19.6161749842658,-49.3166072468784,
124.904881658473)) ;
#49959=CARTESIAN_POINT('Ctrl Pts',(-19.7793647307938,-49.506575952112,124.559725510975)) ;
#49960=CARTESIAN_POINT('Ctrl Pts',(-19.8718870581051,-49.3265868717491,
124.846704436863)) ;
#49961=CARTESIAN_POINT('Ctrl Pts',(-19.9733472943274,-49.5165946350261,
124.477683630801)) ;
#49962=CARTESIAN_POINT('Ctrl Pts',(-20.1143655069739,-49.3366055546632,
124.74415269252)) ;
#49963=CARTESIAN_POINT('Ctrl Pts',(-20.1480134440682,-49.5264779002099,
124.365106465105)) ;
#49964=CARTESIAN_POINT('Ctrl Pts',(-20.3326993754849,-49.346488819847,124.603431043373)) ;
#49965=CARTESIAN_POINT('Ctrl Pts',(-20.3032270535751,-49.5365461943013,
124.221241519737)) ;
#49966=CARTESIAN_POINT('Ctrl Pts',(-20.5267164375359,-49.3565571139384,
124.423600519391)) ;
#49967=CARTESIAN_POINT('Ctrl Pts',(-20.4283133218922,-49.5463763244866,
124.056692970203)) ;
#49968=CARTESIAN_POINT('Ctrl Pts',(-20.6830755384687,-49.3663872441237,
124.217913860219)) ;
#49969=CARTESIAN_POINT('Ctrl Pts',(-20.5254162570907,-49.5564428727018,
123.868692053615)) ;
#49970=CARTESIAN_POINT('Ctrl Pts',(-20.8044543031149,-49.3764537923389,
123.982913211132)) ;
#49971=CARTESIAN_POINT('Ctrl Pts',(-20.5871922984484,-49.5663331213904,
123.67013049004)) ;
#49972=CARTESIAN_POINT('Ctrl Pts',(-20.881675014768,-49.3863440410275,123.734710364339)) ;
#49973=CARTESIAN_POINT('Ctrl Pts',(-20.6142760100577,-49.5763253031664,
123.461828924434)) ;
#49974=CARTESIAN_POINT('Ctrl Pts',(-20.9155298639726,-49.3963362228035,
123.474333218862)) ;
#49975=CARTESIAN_POINT('Ctrl Pts',(-20.6046113032203,-49.5862880837942,
123.252607087574)) ;
#49976=CARTESIAN_POINT('Ctrl Pts',(-20.9034492216854,-49.4062990034313,
123.212805454271)) ;
#49977=CARTESIAN_POINT('Ctrl Pts',(-20.5595393091731,-49.5961924884679,
123.049307305498)) ;
#49978=CARTESIAN_POINT('Ctrl Pts',(-20.847109080545,-49.4162034081051,122.958679801309)) ;
#49979=CARTESIAN_POINT('Ctrl Pts',(-20.478467374034,-49.606252482947,122.853990633004)) ;
#49980=CARTESIAN_POINT('Ctrl Pts',(-20.7457693980106,-49.4262634025841,
122.714534227944)) ;
#49981=CARTESIAN_POINT('Ctrl Pts',(-20.3672356635817,-49.6161011049168,
122.679339657836)) ;
#49982=CARTESIAN_POINT('Ctrl Pts',(-20.6067290420419,-49.4361120245539,
122.496219298933)) ;
#49983=CARTESIAN_POINT('Ctrl Pts',(-20.2251544951592,-49.6261315443286,
122.523536505665)) ;
#49984=CARTESIAN_POINT('Ctrl Pts',(-20.4291275579387,-49.4461424639657,
122.301465539573)) ;
#49985=CARTESIAN_POINT('Ctrl Pts',(-20.0582370192232,-49.6361412599634,
122.395350931652)) ;
#49986=CARTESIAN_POINT('Ctrl Pts',(-20.2204806965298,-49.4561521796005,
122.141233524308)) ;
#49987=CARTESIAN_POINT('Ctrl Pts',(-19.8735746846781,-49.646052012656,122.298896339654)) ;
#49988=CARTESIAN_POINT('Ctrl Pts',(-19.9896519589518,-49.4660629322931,
122.020664911616)) ;
#49989=CARTESIAN_POINT('Ctrl Pts',(-19.6747293616063,-49.6559812856024,
122.23534414131)) ;
#49990=CARTESIAN_POINT('Ctrl Pts',(-19.7410945155268,-49.4759922052395,
121.941224683221)) ;
#49991=CARTESIAN_POINT('Ctrl Pts',(-19.4655008779412,-49.666023976995,122.207142648671)) ;
#49992=CARTESIAN_POINT('Ctrl Pts',(-19.4795590978915,-49.4860348966322,
121.90597303431)) ;
#49993=CARTESIAN_POINT('Ctrl Pts',(-19.2578087514022,-49.6759105102126,
122.215430584698)) ;
#49994=CARTESIAN_POINT('Ctrl Pts',(-19.219942862055,-49.4959214298497,121.916333239462)) ;
#49995=CARTESIAN_POINT('Ctrl Pts',(-19.0524672632715,-49.6859036551446,
122.259778671092)) ;
#49996=CARTESIAN_POINT('Ctrl Pts',(-18.9632658837388,-49.5059145747817,
121.971768765229)) ;
#49997=CARTESIAN_POINT('Ctrl Pts',(-18.8588885046853,-49.6958493359811,
122.3388088344)) ;
#49998=CARTESIAN_POINT('Ctrl Pts',(-18.7212920167133,-49.5158602556182,
122.070557018529)) ;
#49999=CARTESIAN_POINT('Ctrl Pts',(-18.6817080873745,-49.7057965931296,
122.449910909112)) ;
#50000=CARTESIAN_POINT('Ctrl Pts',(-18.499816284014,-49.5258075127667,122.209435357243)) ;
#50001=CARTESIAN_POINT('Ctrl Pts',(-18.5251114478869,-49.7158444970016,
122.591672777569)) ;
#50002=CARTESIAN_POINT('Ctrl Pts',(-18.3040709556974,-49.5358554166387,
122.386637839566)) ;
#50003=CARTESIAN_POINT('Ctrl Pts',(-18.3979488536748,-49.7256921960996,
122.755046538999)) ;
#50004=CARTESIAN_POINT('Ctrl Pts',(-18.1451172426182,-49.5457031157367,
122.590856449756)) ;
#50005=CARTESIAN_POINT('Ctrl Pts',(-18.2993856740285,-49.7356536870782,
122.939814886333)) ;
#50006=CARTESIAN_POINT('Ctrl Pts',(-18.0219137176075,-49.5556646067154,
122.821817640682)) ;
#50007=CARTESIAN_POINT('Ctrl Pts',(-18.2342214042971,-49.7456831494922,
123.140352456418)) ;
#50008=CARTESIAN_POINT('Ctrl Pts',(-17.940459021946,-49.5656940691293,123.072489705636)) ;
#50009=CARTESIAN_POINT('Ctrl Pts',(-18.2051140091869,-49.7555903805921,
123.346589615801)) ;
#50010=CARTESIAN_POINT('Ctrl Pts',(-17.9040753303837,-49.5756013002292,
123.330287135663)) ;
#50011=CARTESIAN_POINT('Ctrl Pts',(-18.211860951267,-49.7655367592695,123.555572269236)) ;
#50012=CARTESIAN_POINT('Ctrl Pts',(-17.9125098782815,-49.5855476789066,
123.591516015328)) ;
#50013=CARTESIAN_POINT('Ctrl Pts',(-18.2549768342654,-49.7755415280784,
123.761455951672)) ;
#50014=CARTESIAN_POINT('Ctrl Pts',(-17.9664056109614,-49.5955524477155,
123.848870528812)) ;
#50015=CARTESIAN_POINT('Ctrl Pts',(-18.3335291933488,-49.7855626490986,
123.956934913202)) ;
#50016=CARTESIAN_POINT('Ctrl Pts',(-18.0645967713653,-49.6055735687357,
124.09321890463)) ;
#50017=CARTESIAN_POINT('Ctrl Pts',(-18.4431860931502,-49.7954535149512,
124.133615577516)) ;
#50018=CARTESIAN_POINT('Ctrl Pts',(-18.201669169235,-49.6154644345883,124.314070124033)) ;
#50019=CARTESIAN_POINT('Ctrl Pts',(-18.5830122161219,-49.8054443237105,
124.290330824793)) ;
#50020=CARTESIAN_POINT('Ctrl Pts',(-18.3764527037186,-49.6254552433476,
124.509963682935)) ;
#50021=CARTESIAN_POINT('Ctrl Pts',(-18.747304518671,-49.8153949818908,124.419846948591)) ;
#50022=CARTESIAN_POINT('Ctrl Pts',(-18.5818191091062,-49.6354059015279,
124.671858407225)) ;
#50023=CARTESIAN_POINT('Ctrl Pts',(-18.9311656323854,-49.8253311915329,
124.518959631838)) ;
#50024=CARTESIAN_POINT('Ctrl Pts',(-18.8116465771157,-49.64534211117,124.795748611683)) ;
#50025=CARTESIAN_POINT('Ctrl Pts',(-19.1303351595038,-49.8353143582578,
124.585224682126)) ;
#50026=CARTESIAN_POINT('Ctrl Pts',(-19.0606091019556,-49.6553252778949,
124.878578886078)) ;
#50027=CARTESIAN_POINT('Ctrl Pts',(-19.3392535954594,-49.8453581554681,
124.615693199531)) ;
#50028=CARTESIAN_POINT('Ctrl Pts',(-19.3217571085356,-49.6653690751052,
124.916663479526)) ;
#50029=CARTESIAN_POINT('Ctrl Pts',(-19.5458273359172,-49.8551863716364,
124.610045735336)) ;
#50030=CARTESIAN_POINT('Ctrl Pts',(-19.5799756953038,-49.6751972912734,
124.909602892924)) ;
#50031=CARTESIAN_POINT('Ctrl Pts',(-19.7533454043374,-49.8652629391056,
124.567682590718)) ;
#50032=CARTESIAN_POINT('Ctrl Pts',(-19.8393726054235,-49.6852738587427,
124.85664781919)) ;
#50033=CARTESIAN_POINT('Ctrl Pts',(-19.9460859117418,-49.875115024795,124.491728264813)) ;
#50034=CARTESIAN_POINT('Ctrl Pts',(-20.0802989166778,-49.6951259444321,
124.761703259049)) ;
#50035=CARTESIAN_POINT('Ctrl Pts',(-20.126701616753,-49.8851882922004,124.381226191815)) ;
#50036=CARTESIAN_POINT('Ctrl Pts',(-20.3060674976311,-49.7051992118375,
124.623574721995)) ;
#50037=CARTESIAN_POINT('Ctrl Pts',(-20.2817328321541,-49.895029708624,124.244194431429)) ;
#50038=CARTESIAN_POINT('Ctrl Pts',(-20.4998566127892,-49.7150406282611,
124.452283158232)) ;
#50039=CARTESIAN_POINT('Ctrl Pts',(-20.4127836030217,-49.9049909667667,
124.080861209861)) ;
#50040=CARTESIAN_POINT('Ctrl Pts',(-20.6636690759953,-49.7250018864038,
124.248115309277)) ;
#50041=CARTESIAN_POINT('Ctrl Pts',(-20.5138903858792,-49.9150276431986,
123.895664527938)) ;
#50042=CARTESIAN_POINT('Ctrl Pts',(-20.7900512077694,-49.7350385628358,
124.016618869433)) ;
#50043=CARTESIAN_POINT('Ctrl Pts',(-20.5805838627807,-49.9249062510625,
123.698962304801)) ;
#50044=CARTESIAN_POINT('Ctrl Pts',(-20.8734168716423,-49.7449171706996,
123.770739635616)) ;
#50045=CARTESIAN_POINT('Ctrl Pts',(-20.6127292545574,-49.9349664797013,
123.489949368876)) ;
#50046=CARTESIAN_POINT('Ctrl Pts',(-20.9135969834897,-49.7549773993384,
123.509473505377)) ;
#50047=CARTESIAN_POINT('Ctrl Pts',(-20.6082434967595,-49.9448334638621,
123.282536648227)) ;
#50048=CARTESIAN_POINT('Ctrl Pts',(-20.9079881465136,-49.7648443834992,
123.250206599961)) ;
#50049=CARTESIAN_POINT('Ctrl Pts',(-20.5676533220387,-49.9548390301148,
123.076169983753)) ;
#50050=CARTESIAN_POINT('Ctrl Pts',(-20.8572486896229,-49.7748499497519,
122.992248525013)) ;
#50051=CARTESIAN_POINT('Ctrl Pts',(-20.4919395617635,-49.9648228185294,
122.880371545976)) ;
#50052=CARTESIAN_POINT('Ctrl Pts',(-20.762604793769,-49.7848337381665,122.747500893272)) ;
#50053=CARTESIAN_POINT('Ctrl Pts',(-20.3825347856944,-49.974868675332,122.699741996269)) ;
#50054=CARTESIAN_POINT('Ctrl Pts',(-20.6258474889343,-49.7948795949691,
122.521714953431)) ;
#50055=CARTESIAN_POINT('Ctrl Pts',(-20.246666531369,-49.984694552548,122.544142027715)) ;
#50056=CARTESIAN_POINT('Ctrl Pts',(-20.4560100049214,-49.8047054721851,
122.327215170071)) ;
#50057=CARTESIAN_POINT('Ctrl Pts',(-20.0835826601991,-49.9946850283893,
122.411791016735)) ;
#50058=CARTESIAN_POINT('Ctrl Pts',(-20.2521537953988,-49.8146959480264,
122.161777820883)) ;
#50059=CARTESIAN_POINT('Ctrl Pts',(-19.8987503711464,-50.0047286042881,
122.309710132215)) ;
#50060=CARTESIAN_POINT('Ctrl Pts',(-20.0211126978458,-49.8247395239252,
122.03417835331)) ;
#50061=CARTESIAN_POINT('Ctrl Pts',(-19.7035546402409,-50.0145503965861,
122.242375343609)) ;
#50062=CARTESIAN_POINT('Ctrl Pts',(-19.7771162248852,-49.8345613162232,
121.950011278901)) ;
#50063=CARTESIAN_POINT('Ctrl Pts',(-19.495286249998,-50.024585362212,122.208741496858)) ;
#50064=CARTESIAN_POINT('Ctrl Pts',(-19.5167805110166,-49.8445962818491,
121.907971037279)) ;
#50065=CARTESIAN_POINT('Ctrl Pts',(-19.2845564519754,-50.034610279145,122.21236484356)) ;
#50066=CARTESIAN_POINT('Ctrl Pts',(-19.25336832143,-49.8546211987822,121.912502122807)) ;
#50067=CARTESIAN_POINT('Ctrl Pts',(-19.0811423574655,-50.0444622175212,
122.251384498715)) ;
#50068=CARTESIAN_POINT('Ctrl Pts',(-18.9991000929311,-49.8644731371583,
121.961278882292)) ;
#50069=CARTESIAN_POINT('Ctrl Pts',(-18.8847759421629,-50.0544531935459,
122.325861032936)) ;
#50070=CARTESIAN_POINT('Ctrl Pts',(-18.7536426685323,-49.8744641131831,
122.054376600934)) ;
#50071=CARTESIAN_POINT('Ctrl Pts',(-18.7055278261908,-50.0643710143496,
122.432422183055)) ;
#50072=CARTESIAN_POINT('Ctrl Pts',(-18.5295831349131,-49.8843819339867,
122.187580190448)) ;
#50073=CARTESIAN_POINT('Ctrl Pts',(-18.5457533128135,-50.0743997349142,
122.569951039098)) ;
#50074=CARTESIAN_POINT('Ctrl Pts',(-18.3298664401693,-49.8944106545513,
122.359492881508)) ;
#50075=CARTESIAN_POINT('Ctrl Pts',(-18.4140890328722,-50.0842826615234,
122.730702151589)) ;
#50076=CARTESIAN_POINT('Ctrl Pts',(-18.1652873217021,-49.9042935811605,
122.56043375668)) ;
#50077=CARTESIAN_POINT('Ctrl Pts',(-18.3108162869546,-50.0942869466428,
122.913895712092)) ;
#50078=CARTESIAN_POINT('Ctrl Pts',(-18.0361983461571,-49.91429786628,122.789426912467)) ;
#50079=CARTESIAN_POINT('Ctrl Pts',(-18.2410673724431,-50.1042706278507,
123.111893587272)) ;
#50080=CARTESIAN_POINT('Ctrl Pts',(-17.949014297203,-49.9242815474878,123.036925185848)) ;
#50081=CARTESIAN_POINT('Ctrl Pts',(-18.20680742649,-50.1143116265806,123.320172550146)) ;
#50082=CARTESIAN_POINT('Ctrl Pts',(-17.9061915789435,-49.9343225462177,
123.297274155865)) ;
#50083=CARTESIAN_POINT('Ctrl Pts',(-18.2088904962245,-50.1241440714477,
123.52687311072)) ;
#50084=CARTESIAN_POINT('Ctrl Pts',(-17.9087977233851,-49.9441549910849,
123.555650792521)) ;
#50085=CARTESIAN_POINT('Ctrl Pts',(-18.2468487955305,-50.1341390698781,
123.733536628154)) ;
#50086=CARTESIAN_POINT('Ctrl Pts',(-17.9562480238635,-49.9541499895152,
123.81397987155)) ;
#50087=CARTESIAN_POINT('Ctrl Pts',(-18.3208110885934,-50.1441706186277,
123.931048389592)) ;
#50088=CARTESIAN_POINT('Ctrl Pts',(-18.0487030674048,-49.9641815382648,
124.060868717992)) ;
#50089=CARTESIAN_POINT('Ctrl Pts',(-18.4259334331203,-50.1540359969332,
124.109821606205)) ;
#50090=CARTESIAN_POINT('Ctrl Pts',(-18.1801084382992,-49.9740469165703,
124.284334653721)) ;
#50091=CARTESIAN_POINT('Ctrl Pts',(-18.5613765662075,-50.1639978443934,
124.26956672375)) ;
#50092=CARTESIAN_POINT('Ctrl Pts',(-18.3494144439518,-49.9840087640306,
124.484014610873)) ;
#50093=CARTESIAN_POINT('Ctrl Pts',(-18.7238875342035,-50.1740327852077,
124.404073431431)) ;
#50094=CARTESIAN_POINT('Ctrl Pts',(-18.5525546909306,-49.9940437048448,
124.652146083478)) ;
#50095=CARTESIAN_POINT('Ctrl Pts',(-18.9044058295045,-50.1839177462248,
124.507085840432)) ;
#50096=CARTESIAN_POINT('Ctrl Pts',(-18.7782043027359,-50.003928665862,124.780909685819)) ;
#50097=CARTESIAN_POINT('Ctrl Pts',(-19.103599497382,-50.1939833551437,124.578405574943)) ;
#50098=CARTESIAN_POINT('Ctrl Pts',(-19.0271970940224,-50.0139942747808,
124.870056934491)) ;
#50099=CARTESIAN_POINT('Ctrl Pts',(-19.3074891707686,-50.2038225301854,
124.613469337633)) ;
#50100=CARTESIAN_POINT('Ctrl Pts',(-19.2820603187455,-50.0238334498225,
124.913884244235)) ;
#50101=CARTESIAN_POINT('Ctrl Pts',(-19.5190104294486,-50.2138850856853,
124.612870871899)) ;
#50102=CARTESIAN_POINT('Ctrl Pts',(-19.5464617510403,-50.0338960053224,
124.913133557086)) ;
#50103=CARTESIAN_POINT('Ctrl Pts',(-19.7237883029565,-50.2237822603782,
124.575939416995)) ;
#50104=CARTESIAN_POINT('Ctrl Pts',(-19.8024340996347,-50.0437931800154,
124.866966630769)) ;
#50105=CARTESIAN_POINT('Ctrl Pts',(-19.9199318195631,-50.2337129753016,
124.504433105692)) ;
#50106=CARTESIAN_POINT('Ctrl Pts',(-20.0476128622874,-50.0537238949387,
124.777581121014)) ;
#50107=CARTESIAN_POINT('Ctrl Pts',(-20.1026202548277,-50.2437570033792,
124.398553787405)) ;
#50108=CARTESIAN_POINT('Ctrl Pts',(-20.2759720546877,-50.0637679230163,
124.645229703549)) ;
#50109=CARTESIAN_POINT('Ctrl Pts',(-20.2617301651388,-50.2536432052325,
124.264811495273)) ;
#50110=CARTESIAN_POINT('Ctrl Pts',(-20.4748580560086,-50.0736541248696,
124.478049522978)) ;
#50111=CARTESIAN_POINT('Ctrl Pts',(-20.3968653014659,-50.2636363716993,
124.103982279919)) ;
#50112=CARTESIAN_POINT('Ctrl Pts',(-20.6437749690615,-50.0836472913365,
124.277011182732)) ;
#50113=CARTESIAN_POINT('Ctrl Pts',(-20.5015352977048,-50.2735758426865,
123.923098316065)) ;
#50114=CARTESIAN_POINT('Ctrl Pts',(-20.7746102355523,-50.0935867623236,
124.050904663364)) ;
#50115=CARTESIAN_POINT('Ctrl Pts',(-20.5737859343558,-50.2835923570407,
123.725325502378)) ;
#50116=CARTESIAN_POINT('Ctrl Pts',(-20.8649209945911,-50.1036032766778,
123.803687664981)) ;
#50117=CARTESIAN_POINT('Ctrl Pts',(-20.6104642438826,-50.2935223835175,
123.519782917965)) ;
#50118=CARTESIAN_POINT('Ctrl Pts',(-20.9107662307901,-50.1135333031546,
123.546758707773)) ;
#50119=CARTESIAN_POINT('Ctrl Pts',(-20.6108086522076,-50.303574919027,123.308465111307)) ;
#50120=CARTESIAN_POINT('Ctrl Pts',(-20.9111940114087,-50.1235858386641,
123.282611468914)) ;
#50121=CARTESIAN_POINT('Ctrl Pts',(-20.5753140283502,-50.3134213222466,
123.104521388382)) ;
#50122=CARTESIAN_POINT('Ctrl Pts',(-20.8668229607071,-50.1334322418838,
123.02768188537)) ;
#50123=CARTESIAN_POINT('Ctrl Pts',(-20.5047639569835,-50.3233833651007,
122.907340910753)) ;
#50124=CARTESIAN_POINT('Ctrl Pts',(-20.7786326898469,-50.1433942847378,
122.781207115451)) ;
#50125=CARTESIAN_POINT('Ctrl Pts',(-20.4001053609626,-50.3334119158914,
122.724304136021)) ;
#50126=CARTESIAN_POINT('Ctrl Pts',(-20.6478070135381,-50.1534228355285,
122.552412487854)) ;
#50127=CARTESIAN_POINT('Ctrl Pts',(-20.2669138933572,-50.343322241609,122.564103535408)) ;
#50128=CARTESIAN_POINT('Ctrl Pts',(-20.4813154002532,-50.1633331612461,
122.352163354463)) ;
#50129=CARTESIAN_POINT('Ctrl Pts',(-20.1078761445415,-50.3532571534386,
122.428702223204)) ;
#50130=CARTESIAN_POINT('Ctrl Pts',(-20.2825162867384,-50.1732680730757,
122.182913771946)) ;
#50131=CARTESIAN_POINT('Ctrl Pts',(-19.9257330097845,-50.3632981602067,
122.32201626754)) ;
#50132=CARTESIAN_POINT('Ctrl Pts',(-20.0548359115821,-50.1833090798438,
122.049558725394)) ;
#50133=CARTESIAN_POINT('Ctrl Pts',(-19.7308882493759,-50.3731857930389,
122.249563232581)) ;
#50134=CARTESIAN_POINT('Ctrl Pts',(-19.8112788264307,-50.193196712676,121.958995011386)) ;
#50135=CARTESIAN_POINT('Ctrl Pts',(-19.5243853029293,-50.3831762241369,
122.211289416377)) ;
#50136=CARTESIAN_POINT('Ctrl Pts',(-19.5531495649687,-50.203187143774,121.911155500967)) ;
#50137=CARTESIAN_POINT('Ctrl Pts',(-19.3150912519442,-50.3931316606941,
122.209571649096)) ;
#50138=CARTESIAN_POINT('Ctrl Pts',(-19.2915318676096,-50.2131425803313,
121.909011127631)) ;
#50139=CARTESIAN_POINT('Ctrl Pts',(-19.1095552736864,-50.4030426087935,
122.243685794913)) ;
#50140=CARTESIAN_POINT('Ctrl Pts',(-19.0346123538421,-50.2230535284306,
121.951656547324)) ;
#50141=CARTESIAN_POINT('Ctrl Pts',(-18.9109486179919,-50.4130546848912,
122.313456614259)) ;
#50142=CARTESIAN_POINT('Ctrl Pts',(-18.7863546985664,-50.2330656045283,
122.038872975967)) ;
#50143=CARTESIAN_POINT('Ctrl Pts',(-18.727435602444,-50.4230820069661,122.417161220471)) ;
#50144=CARTESIAN_POINT('Ctrl Pts',(-18.5569655230889,-50.2430929266033,
122.168505406507)) ;
#50145=CARTESIAN_POINT('Ctrl Pts',(-18.5670779315736,-50.4329407819203,
122.548532884562)) ;
#50146=CARTESIAN_POINT('Ctrl Pts',(-18.3565173091822,-50.2529517015574,
122.332725267675)) ;
#50147=CARTESIAN_POINT('Ctrl Pts',(-18.3833334191599,-50.4463669747327,
122.762717425023)) ;
#50148=CARTESIAN_POINT('Ctrl Pts',(-18.126853897068,-50.2663778943698,122.600443072369)) ;
#50149=CARTESIAN_POINT('Ctrl Pts',(-18.2623681721055,-50.4594509905141,
123.013391436687)) ;
#50150=CARTESIAN_POINT('Ctrl Pts',(-17.975652168747,-50.2794619101513,122.913754436189)) ;
#50151=CARTESIAN_POINT('Ctrl Pts',(-18.2092179613212,-50.4729244392694,
123.29151187479)) ;
#50152=CARTESIAN_POINT('Ctrl Pts',(-17.909201931477,-50.2929353589065,123.261460162963)) ;
#50153=CARTESIAN_POINT('Ctrl Pts',(-18.2065405992436,-50.4827573970752,
123.498250206426)) ;
#50154=CARTESIAN_POINT('Ctrl Pts',(-17.9058612706939,-50.3027683167123,
123.519872041659)) ;
#50155=CARTESIAN_POINT('Ctrl Pts',(-18.2393587707171,-50.4927206705259,
123.705106522157)) ;
#50156=CARTESIAN_POINT('Ctrl Pts',(-17.9468858271895,-50.312731590163,123.778444889116)) ;
#50157=CARTESIAN_POINT('Ctrl Pts',(-18.3085355723821,-50.5027577443438,
123.904453594488)) ;
#50158=CARTESIAN_POINT('Ctrl Pts',(-18.0333597051189,-50.322768663981,124.027627149675)) ;
#50159=CARTESIAN_POINT('Ctrl Pts',(-18.409286084184,-50.5126327473555,124.085999426355)) ;
#50160=CARTESIAN_POINT('Ctrl Pts',(-18.1593001786209,-50.3326436669926,
124.254558222492)) ;
#50161=CARTESIAN_POINT('Ctrl Pts',(-18.5425517962584,-50.5227004269817,
124.250393752023)) ;
#50162=CARTESIAN_POINT('Ctrl Pts',(-18.3258841681713,-50.3427113466188,
124.460049111905)) ;
#50163=CARTESIAN_POINT('Ctrl Pts',(-18.6986982462725,-50.5325412771994,
124.386149557232)) ;
#50164=CARTESIAN_POINT('Ctrl Pts',(-18.5210703743217,-50.3525521968365,
124.629743114865)) ;
#50165=CARTESIAN_POINT('Ctrl Pts',(-18.9386955742681,-50.5458774756753,
124.531065619422)) ;
#50166=CARTESIAN_POINT('Ctrl Pts',(-18.8210606852671,-50.3658883953125,
124.810877501075)) ;
#50167=CARTESIAN_POINT('Ctrl Pts',(-19.2087059356425,-50.5590949994898,
124.609228100724)) ;
#50168=CARTESIAN_POINT('Ctrl Pts',(-19.1585310682997,-50.3791059191269,
124.908576997203)) ;
#50169=CARTESIAN_POINT('Ctrl Pts',(-19.488920896454,-50.572429925981,124.615199991677)) ;
#50170=CARTESIAN_POINT('Ctrl Pts',(-19.5088595130066,-50.3924408456182,
124.916046147867)) ;
#50171=CARTESIAN_POINT('Ctrl Pts',(-19.6963926036681,-50.5824130265756,
124.583239687426)) ;
#50172=CARTESIAN_POINT('Ctrl Pts',(-19.7681867122454,-50.4024239462128,
124.876091752188)) ;
#50173=CARTESIAN_POINT('Ctrl Pts',(-19.8962274127877,-50.5924578024753,
124.515046658216)) ;
#50174=CARTESIAN_POINT('Ctrl Pts',(-20.0179829922131,-50.4124687221124,
124.790847910221)) ;
#50175=CARTESIAN_POINT('Ctrl Pts',(-20.0772393222898,-50.6022757256612,
124.415835187125)) ;
#50176=CARTESIAN_POINT('Ctrl Pts',(-20.2442444733831,-50.4222866452983,
124.666833014598)) ;
#50177=CARTESIAN_POINT('Ctrl Pts',(-20.2423226616433,-50.6123250396165,
124.284011355845)) ;
#50178=CARTESIAN_POINT('Ctrl Pts',(-20.4505999318951,-50.4323359592536,
124.502045800867)) ;
#50179=CARTESIAN_POINT('Ctrl Pts',(-20.4268261999454,-50.6256287802391,
124.073810716125)) ;
#50180=CARTESIAN_POINT('Ctrl Pts',(-20.6812147142531,-50.4456396998762,
124.239319481561)) ;
#50181=CARTESIAN_POINT('Ctrl Pts',(-20.5831565120962,-50.6421189757157,
123.759929328214)) ;
#50182=CARTESIAN_POINT('Ctrl Pts',(-20.8766371020504,-50.4621298953529,
123.846918741757)) ;
#50183=CARTESIAN_POINT('Ctrl Pts',(-20.6233943821416,-50.6588381406404,
123.40675844073)) ;
#50184=CARTESIAN_POINT('Ctrl Pts',(-20.9269267933237,-50.4788490602775,
123.405534034858)) ;
#50185=CARTESIAN_POINT('Ctrl Pts',(-20.5824794471599,-50.6719991343105,
123.133106842893)) ;
#50186=CARTESIAN_POINT('Ctrl Pts',(-20.8757804021482,-50.4920100539476,
123.063406602128)) ;
#50187=CARTESIAN_POINT('Ctrl Pts',(-20.516519250953,-50.6819953564158,122.933581400906)) ;
#50188=CARTESIAN_POINT('Ctrl Pts',(-20.7933286314175,-50.5020062760529,
122.814013822185)) ;
#50189=CARTESIAN_POINT('Ctrl Pts',(-20.4162173833348,-50.6920191959495,
122.748251975362)) ;
#50190=CARTESIAN_POINT('Ctrl Pts',(-20.66794702487,-50.5120301155866,122.58234791319)) ;
#50191=CARTESIAN_POINT('Ctrl Pts',(-20.2443086428061,-50.7052125179428,
122.530542353315)) ;
#50192=CARTESIAN_POINT('Ctrl Pts',(-20.4530703195707,-50.5252234375799,
122.310222407941)) ;
#50193=CARTESIAN_POINT('Ctrl Pts',(-19.9606322188696,-50.7218716897201,
122.318490004045)) ;
#50194=CARTESIAN_POINT('Ctrl Pts',(-20.0984605249334,-50.5418826093572,
122.04515035663)) ;
#50195=CARTESIAN_POINT('Ctrl Pts',(-19.5552783088555,-50.7417818652058,
122.196329453374)) ;
#50196=CARTESIAN_POINT('Ctrl Pts',(-19.5917715291836,-50.5617927848429,
121.89245685484)) ;
#50197=CARTESIAN_POINT('Ctrl Pts',(-19.1329219062142,-50.7616718530502,
122.218924903769)) ;
#50198=CARTESIAN_POINT('Ctrl Pts',(-19.0638261203489,-50.5816827726873,
121.920703930916)) ;
#50199=CARTESIAN_POINT('Ctrl Pts',(-18.7416302883475,-50.781677301065,122.385558421519)) ;
#50200=CARTESIAN_POINT('Ctrl Pts',(-18.5747132438789,-50.6016882207021,
122.12899945876)) ;
#50201=CARTESIAN_POINT('Ctrl Pts',(-18.4328824089552,-50.8015136950923,
122.673074672253)) ;
#50202=CARTESIAN_POINT('Ctrl Pts',(-18.1887817456848,-50.6215246147294,
122.488396023025)) ;
#50203=CARTESIAN_POINT('Ctrl Pts',(-18.2390777335758,-50.821521488989,123.051656272595)) ;
#50204=CARTESIAN_POINT('Ctrl Pts',(-17.9465286197536,-50.6415324086261,
122.961624501261)) ;
#50205=CARTESIAN_POINT('Ctrl Pts',(-18.1864063154851,-50.8413481252829,
123.469998542685)) ;
#50206=CARTESIAN_POINT('Ctrl Pts',(-17.880692353325,-50.66135904492,123.484550765059)) ;
#50207=CARTESIAN_POINT('Ctrl Pts',(-18.279598430072,-50.8613270682368,123.884440335655)) ;
#50208=CARTESIAN_POINT('Ctrl Pts',(-17.9971845806245,-50.6813379878739,
124.002602226816)) ;
#50209=CARTESIAN_POINT('Ctrl Pts',(-18.5086965529277,-50.8812588701058,
124.240917370752)) ;
#50210=CARTESIAN_POINT('Ctrl Pts',(-18.2835587250181,-50.701269789743,124.448196582327)) ;
#50211=CARTESIAN_POINT('Ctrl Pts',(-18.8431584214289,-50.9010831706034,
124.497674618011)) ;
#50212=CARTESIAN_POINT('Ctrl Pts',(-18.7016353948024,-50.7210940902405,
124.769140330186)) ;
#50213=CARTESIAN_POINT('Ctrl Pts',(-19.2506039421692,-50.9211791719433,
124.62581638792)) ;
#50214=CARTESIAN_POINT('Ctrl Pts',(-19.2109425558882,-50.7411900915803,
124.929317666213)) ;
#50215=CARTESIAN_POINT('Ctrl Pts',(-19.6705888408136,-50.9409375880472,
124.607973358778)) ;
#50216=CARTESIAN_POINT('Ctrl Pts',(-19.7359254653028,-50.7609485076843,
124.90700825648)) ;
#50217=CARTESIAN_POINT('Ctrl Pts',(-20.0654721859542,-50.9610312809313,
124.445475299511)) ;
#50218=CARTESIAN_POINT('Ctrl Pts',(-20.2295077365795,-50.7810422005684,
124.703903011743)) ;
#50219=CARTESIAN_POINT('Ctrl Pts',(-20.2716279154534,-50.9741422468379,
124.257625275152)) ;
#50220=CARTESIAN_POINT('Ctrl Pts',(-20.4872438678407,-50.7941531664751,
124.469055541275)) ;
#50221=CARTESIAN_POINT('Ctrl Pts',(-20.357892637621,-50.9808556216258,124.146615798218)) ;
#50222=CARTESIAN_POINT('Ctrl Pts',(-20.5950497967257,-50.8008665412629,
124.330315451401)) ;
#50223=CARTESIAN_POINT('',(-20.8451118641281,-12.0000000003486,123.237406291927)) ;
#50224=CARTESIAN_POINT('Ctrl Pts',(-20.6521254138848,-12.1170415160268,
123.278341315447)) ;
#50225=CARTESIAN_POINT('Ctrl Pts',(-20.6736893170551,-12.104042490247,123.276781066563)) ;
#50226=CARTESIAN_POINT('Ctrl Pts',(-20.6956426458393,-12.0907896304746,
123.274049785805)) ;
#50227=CARTESIAN_POINT('Ctrl Pts',(-20.7176046968127,-12.0775058642284,
123.270287525093)) ;
#50228=CARTESIAN_POINT('Ctrl Pts',(-20.7393375909741,-12.0643607036855,
123.266564520626)) ;
#50229=CARTESIAN_POINT('Ctrl Pts',(-20.7610782944406,-12.0511852792471,
123.261830892347)) ;
#50230=CARTESIAN_POINT('Ctrl Pts',(-20.782453340365,-12.0381956240751,123.256276579118)) ;
#50231=CARTESIAN_POINT('Ctrl Pts',(-20.8022914638292,-12.0261399595413,
123.251121635732)) ;
#50232=CARTESIAN_POINT('Ctrl Pts',(-20.8218141748009,-12.0142443106129,
123.245260029577)) ;
#50233=CARTESIAN_POINT('Ctrl Pts',(-20.8407272069771,-12.0026813802067,
123.238894624384)) ;
#50234=CARTESIAN_POINT('Ctrl Pts',(-20.8421924596759,-12.0017855632469,
123.238401476217)) ;
#50235=CARTESIAN_POINT('Ctrl Pts',(-20.8436540570881,-12.0008917432925,
123.237905329914)) ;
#50236=CARTESIAN_POINT('Ctrl Pts',(-20.8451118646125,-12.0000000006492,
123.237406292805)) ;
#50237=CARTESIAN_POINT('Ctrl Pts',(-20.8451118656667,-12.0000000000044,
123.237406292444)) ;
#50238=CARTESIAN_POINT('Ctrl Pts',(-20.847700442803,-12.0000000000052,123.284550346716)) ;
#50239=CARTESIAN_POINT('Ctrl Pts',(-20.8479707594182,-12.,123.331561909933)) ;
#50240=CARTESIAN_POINT('Ctrl Pts',(-20.8459837280419,-12.,123.37822134492)) ;
#50241=CARTESIAN_POINT('Ctrl Pts',(-20.8424452760623,-12.,123.461311210567)) ;
#50242=CARTESIAN_POINT('Ctrl Pts',(-20.8317433199247,-12.,123.543372575294)) ;
#50243=CARTESIAN_POINT('Ctrl Pts',(-20.8138854213481,-12.,123.624030867736)) ;
#50244=CARTESIAN_POINT('Ctrl Pts',(-20.8018655450891,-12.,123.678320721061)) ;
#50245=CARTESIAN_POINT('Ctrl Pts',(-20.7866123388131,-11.9999999780286,
123.73193986445)) ;
#50246=CARTESIAN_POINT('Ctrl Pts',(-20.7684896206078,-11.9999999870879,
123.784085115621)) ;
#50247=CARTESIAN_POINT('Ctrl Pts',(-20.759636032663,-11.9999999915136,123.809559912609)) ;
#50248=CARTESIAN_POINT('Ctrl Pts',(-20.7500973712125,-12.,123.834683706848)) ;
#50249=CARTESIAN_POINT('Ctrl Pts',(-20.7399146692478,-12.,123.859367148951)) ;
#50250=CARTESIAN_POINT('Ctrl Pts',(-20.7147385522311,-12.,123.92039547217)) ;
#50251=CARTESIAN_POINT('Ctrl Pts',(-20.6856174547214,-12.0000000184731,
123.97875125416)) ;
#50252=CARTESIAN_POINT('Ctrl Pts',(-20.6525030990685,-12.0000000058446,
124.034758195809)) ;
#50253=CARTESIAN_POINT('Ctrl Pts',(-20.644710021447,-12.0000000028726,124.047938776708)) ;
#50254=CARTESIAN_POINT('Ctrl Pts',(-20.6366958712216,-12.,124.060989060861)) ;
#50255=CARTESIAN_POINT('Ctrl Pts',(-20.6284602057521,-12.,124.073912891062)) ;
#50256=CARTESIAN_POINT('Ctrl Pts',(-20.5990742768858,-12.,124.120026803335)) ;
#50257=CARTESIAN_POINT('Ctrl Pts',(-20.5668676415575,-11.9999999840944,
124.164531604601)) ;
#50258=CARTESIAN_POINT('Ctrl Pts',(-20.5324147688095,-11.9999999908829,
124.206739731105)) ;
#50259=CARTESIAN_POINT('Ctrl Pts',(-20.5160790288264,-11.9999999941016,
124.226752604482)) ;
#50260=CARTESIAN_POINT('Ctrl Pts',(-20.4992378958615,-12.,124.246249796365)) ;
#50261=CARTESIAN_POINT('Ctrl Pts',(-20.4819503101481,-12.,124.26516140249)) ;
#50262=CARTESIAN_POINT('Ctrl Pts',(-20.4318371386434,-12.,124.319982276665)) ;
#50263=CARTESIAN_POINT('Ctrl Pts',(-20.3779831633315,-12.0000000080437,
124.369871658523)) ;
#50264=CARTESIAN_POINT('Ctrl Pts',(-20.3205125767886,-12.000000000871,124.415059804215)) ;
#50265=CARTESIAN_POINT('Ctrl Pts',(-20.3162101513788,-12.0000000003341,
124.418442728211)) ;
#50266=CARTESIAN_POINT('Ctrl Pts',(-20.3118874716527,-12.,124.421799285237)) ;
#50267=CARTESIAN_POINT('Ctrl Pts',(-20.3075445973449,-12.,124.425129563068)) ;
#50268=CARTESIAN_POINT('Ctrl Pts',(-20.260709657936,-12.,124.461044339641)) ;
#50269=CARTESIAN_POINT('Ctrl Pts',(-20.2115143902064,-11.9999999923458,
124.493911559955)) ;
#50270=CARTESIAN_POINT('Ctrl Pts',(-20.1607019561465,-11.9999999967179,
124.523266658752)) ;
#50271=CARTESIAN_POINT('Ctrl Pts',(-20.1437230877502,-11.9999999981788,
124.53307560352)) ;
#50272=CARTESIAN_POINT('Ctrl Pts',(-20.1265633242237,-12.,124.542492681273)) ;
#50273=CARTESIAN_POINT('Ctrl Pts',(-20.1092493826613,-12.,124.551501370856)) ;
#50274=CARTESIAN_POINT('Ctrl Pts',(-20.0504925213261,-12.,124.582073399919)) ;
#50275=CARTESIAN_POINT('Ctrl Pts',(-19.9900187394448,-11.9999999984792,
124.607913308289)) ;
#50276=CARTESIAN_POINT('Ctrl Pts',(-19.9286682933254,-11.9999999996238,
124.62902433523)) ;
#50277=CARTESIAN_POINT('Ctrl Pts',(-19.9176392817622,-11.9999999998296,
124.632819478949)) ;
#50278=CARTESIAN_POINT('Ctrl Pts',(-19.9065818042026,-12.,124.636461817088)) ;
#50279=CARTESIAN_POINT('Ctrl Pts',(-19.8955005664695,-12.,124.639951394143)) ;
#50280=CARTESIAN_POINT('Ctrl Pts',(-19.8225767572884,-12.,124.66291572876)) ;
#50281=CARTESIAN_POINT('Ctrl Pts',(-19.7485397875236,-12.,124.679290222045)) ;
#50282=CARTESIAN_POINT('Ctrl Pts',(-19.6735413567767,-12.,124.68913473109)) ;
#50283=CARTESIAN_POINT('Ctrl Pts',(-19.6163274050979,-12.,124.696644798423)) ;
#50284=CARTESIAN_POINT('Ctrl Pts',(-19.5585508018213,-11.9999999945779,
124.70035487014)) ;
#50285=CARTESIAN_POINT('Ctrl Pts',(-19.501082391029,-11.9999999978038,124.700220064632)) ;
#50286=CARTESIAN_POINT('Ctrl Pts',(-19.4831056672055,-11.9999999988129,
124.70017789605)) ;
#50287=CARTESIAN_POINT('Ctrl Pts',(-19.4651587236123,-12.,124.699759581626)) ;
#50288=CARTESIAN_POINT('Ctrl Pts',(-19.4472671863275,-12.,124.698963935301)) ;
#50289=CARTESIAN_POINT('Ctrl Pts',(-19.3889308676436,-12.,124.696369687707)) ;
#50290=CARTESIAN_POINT('Ctrl Pts',(-19.3312538085245,-11.9999999905181,
124.689768246184)) ;
#50291=CARTESIAN_POINT('Ctrl Pts',(-19.2749239756733,-11.9999999963922,
124.679509940194)) ;
#50292=CARTESIAN_POINT('Ctrl Pts',(-19.2585509511539,-11.9999999980996,
124.676528225409)) ;
#50293=CARTESIAN_POINT('Ctrl Pts',(-19.2422914255352,-12.,124.673237459633)) ;
#50294=CARTESIAN_POINT('Ctrl Pts',(-19.226161509904,-12.,124.669645992527)) ;
#50295=CARTESIAN_POINT('Ctrl Pts',(-19.1608299156492,-12.,124.655099340383)) ;
#50296=CARTESIAN_POINT('Ctrl Pts',(-19.0975570030699,-12.0000000087182,
124.63560435259)) ;
#50297=CARTESIAN_POINT('Ctrl Pts',(-19.0361906764906,-12.0000000012434,
124.611239898637)) ;
#50298=CARTESIAN_POINT('Ctrl Pts',(-19.0300689734446,-12.0000000004977,
124.608809380789)) ;
#50299=CARTESIAN_POINT('Ctrl Pts',(-19.0239662846671,-12.,124.606330417063)) ;
#50300=CARTESIAN_POINT('Ctrl Pts',(-19.0178824861837,-12.,124.603803095076)) ;
#50301=CARTESIAN_POINT('Ctrl Pts',(-18.9993535486714,-12.,124.596105833028)) ;
#50302=CARTESIAN_POINT('Ctrl Pts',(-18.9809968021315,-11.9999999988781,
124.58795874914)) ;
#50303=CARTESIAN_POINT('Ctrl Pts',(-18.9628485324419,-11.9999999980959,
124.579378422602)) ;
#50304=CARTESIAN_POINT('Ctrl Pts',(-18.2740109056134,-10.1799890803629,
123.800437437226)) ;
#50305=CARTESIAN_POINT('Ctrl Pts',(-17.9901976315307,-9.9999999998824,123.897592500224)) ;
#50306=CARTESIAN_POINT('Ctrl Pts',(-18.3189528014318,-10.186615931181,123.93177221557)) ;
#50307=CARTESIAN_POINT('Ctrl Pts',(-18.0463587733103,-10.0066268507005,
124.061733136893)) ;
#50308=CARTESIAN_POINT('Ctrl Pts',(-18.4544999825326,-10.199846557662,124.178242251159)) ;
#50309=CARTESIAN_POINT('Ctrl Pts',(-18.2158202081591,-10.0198574771815,
124.369865791322)) ;
#50310=CARTESIAN_POINT('Ctrl Pts',(-18.7737258963307,-10.2198221789206,
124.458448669119)) ;
#50311=CARTESIAN_POINT('Ctrl Pts',(-18.6148367044047,-10.0398330984402,
124.720100586921)) ;
#50312=CARTESIAN_POINT('Ctrl Pts',(-19.1683517049307,-10.2397395138226,
124.612076715426)) ;
#50313=CARTESIAN_POINT('Ctrl Pts',(-19.1081207669815,-10.0597504333421,
124.91214190006)) ;
#50314=CARTESIAN_POINT('Ctrl Pts',(-19.5908221387894,-10.2596127905386,
124.622761896565)) ;
#50315=CARTESIAN_POINT('Ctrl Pts',(-19.6362061149637,-10.0796237100581,
124.925498515678)) ;
#50316=CARTESIAN_POINT('Ctrl Pts',(-19.9944586595383,-10.2796372807025,
124.487357143018)) ;
#50317=CARTESIAN_POINT('Ctrl Pts',(-20.1407529321144,-10.0996482002221,
124.756244590511)) ;
#50318=CARTESIAN_POINT('Ctrl Pts',(-20.3250726893908,-10.2995051218533,
124.224284503461)) ;
#50319=CARTESIAN_POINT('Ctrl Pts',(-20.5540202997451,-10.1195160413728,
124.427406225565)) ;
#50320=CARTESIAN_POINT('Ctrl Pts',(-20.5474404603406,-10.3194507727328,
123.863209826147)) ;
#50321=CARTESIAN_POINT('Ctrl Pts',(-20.8319818409441,-10.1394616922523,
123.976064807505)) ;
#50322=CARTESIAN_POINT('Ctrl Pts',(-20.6329204930996,-10.3393561733498,
123.448689022605)) ;
#50323=CARTESIAN_POINT('Ctrl Pts',(-20.9388342402948,-10.1593670928693,
123.457915382841)) ;
#50324=CARTESIAN_POINT('Ctrl Pts',(-20.5727382583942,-10.3592304011661,
123.030414178423)) ;
#50325=CARTESIAN_POINT('Ctrl Pts',(-20.8636098404201,-10.1792413206857,
122.935072644665)) ;
#50326=CARTESIAN_POINT('Ctrl Pts',(-20.3723372035374,-10.3792161920437,
122.655670923463)) ;
#50327=CARTESIAN_POINT('Ctrl Pts',(-20.6131115835654,-10.1992271115633,
122.466642059104)) ;
#50328=CARTESIAN_POINT('Ctrl Pts',(-20.0574028124706,-10.3991104347035,
122.373313004285)) ;
#50329=CARTESIAN_POINT('Ctrl Pts',(-20.2194466572948,-10.219121354223,122.11369274918)) ;
#50330=CARTESIAN_POINT('Ctrl Pts',(-19.6656681691958,-10.4189891507756,
122.214436559376)) ;
#50331=CARTESIAN_POINT('Ctrl Pts',(-19.7297807740349,-10.2390000702951,
121.915093775182)) ;
#50332=CARTESIAN_POINT('Ctrl Pts',(-19.2398981074651,-10.4390286006202,
122.199163423108)) ;
#50333=CARTESIAN_POINT('Ctrl Pts',(-19.1975679684493,-10.2590395201397,
121.895998337618)) ;
#50334=CARTESIAN_POINT('Ctrl Pts',(-18.8378689724914,-10.458891762158,122.328984896592)) ;
#50335=CARTESIAN_POINT('Ctrl Pts',(-18.6950312338989,-10.2789026816776,
122.058270950061)) ;
#50336=CARTESIAN_POINT('Ctrl Pts',(-18.5023795521869,-10.4788711301723,
122.589370841986)) ;
#50337=CARTESIAN_POINT('Ctrl Pts',(-18.2756669290296,-10.2988820496918,
122.383749835429)) ;
#50338=CARTESIAN_POINT('Ctrl Pts',(-18.2772917542457,-10.4986817106951,
122.945518138246)) ;
#50339=CARTESIAN_POINT('Ctrl Pts',(-17.9943038603936,-10.3186926302146,
122.828930487485)) ;
#50340=CARTESIAN_POINT('Ctrl Pts',(-18.1858955375249,-10.5186626389807,
123.360335745372)) ;
#50341=CARTESIAN_POINT('Ctrl Pts',(-17.88005400599,-10.3386735585002,123.347451469635)) ;
#50342=CARTESIAN_POINT('Ctrl Pts',(-18.2415877544767,-10.5385553108501,
123.779674054783)) ;
#50343=CARTESIAN_POINT('Ctrl Pts',(-17.9496636134843,-10.3585662303696,
123.871624239583)) ;
#50344=CARTESIAN_POINT('Ctrl Pts',(-18.4366892236376,-10.5584816411372,
124.155765874511)) ;
#50345=CARTESIAN_POINT('Ctrl Pts',(-18.1935384903263,-10.3784925606567,
124.341742095362)) ;
#50346=CARTESIAN_POINT('Ctrl Pts',(-18.7493758900079,-10.5784521952295,
124.443056780365)) ;
#50347=CARTESIAN_POINT('Ctrl Pts',(-18.5843830564956,-10.398463114749,124.700856014448)) ;
#50348=CARTESIAN_POINT('Ctrl Pts',(-19.0736750036282,-10.5949840343171,
124.578605622473)) ;
#50349=CARTESIAN_POINT('Ctrl Pts',(-18.9897866675444,-10.4149949538366,
124.87030674853)) ;
#50350=CARTESIAN_POINT('Ctrl Pts',(-19.3515822133367,-10.6083237731447,
124.616534422033)) ;
#50351=CARTESIAN_POINT('Ctrl Pts',(-19.3371420473512,-10.4283346926642,
124.917711789974)) ;
#50352=CARTESIAN_POINT('Ctrl Pts',(-19.5623087353055,-10.6183560153633,
124.608012512987)) ;
#50353=CARTESIAN_POINT('Ctrl Pts',(-19.6005562667581,-10.4383669348828,
124.907063768978)) ;
#50354=CARTESIAN_POINT('Ctrl Pts',(-19.7648570829155,-10.6282137160067,
124.564122231623)) ;
#50355=CARTESIAN_POINT('Ctrl Pts',(-19.8537397871316,-10.4482246355263,
124.852203726934)) ;
#50356=CARTESIAN_POINT('Ctrl Pts',(-19.9594412369529,-10.638205580646,124.485025335786)) ;
#50357=CARTESIAN_POINT('Ctrl Pts',(-20.0969735540684,-10.4582165001655,
124.753332920259)) ;
#50358=CARTESIAN_POINT('Ctrl Pts',(-20.1360906792147,-10.6481281304061,
124.374071893985)) ;
#50359=CARTESIAN_POINT('Ctrl Pts',(-20.3177787347582,-10.4681390499256,
124.614652183523)) ;
#50360=CARTESIAN_POINT('Ctrl Pts',(-20.3435921685771,-10.6614059038996,
124.187345412144)) ;
#50361=CARTESIAN_POINT('Ctrl Pts',(-20.5771970982889,-10.4814168234191,
124.381203459018)) ;
#50362=CARTESIAN_POINT('Ctrl Pts',(-20.4979359412099,-10.6747532428402,
123.949230531229)) ;
#50363=CARTESIAN_POINT('Ctrl Pts',(-20.7701003709952,-10.4947641623597,
124.083584310545)) ;
#50364=CARTESIAN_POINT('Ctrl Pts',(-20.5838202221108,-10.6879604746334,
123.685128933396)) ;
#50365=CARTESIAN_POINT('Ctrl Pts',(-20.8774553695642,-10.5079713941529,
123.753475217099)) ;
#50366=CARTESIAN_POINT('Ctrl Pts',(-20.6134756841563,-10.6979475907231,
123.477310674119)) ;
#50367=CARTESIAN_POINT('Ctrl Pts',(-20.9145282393183,-10.5179585102426,
123.493699384286)) ;
#50368=CARTESIAN_POINT('Ctrl Pts',(-20.6067552821165,-10.7078984963028,
123.26817900999)) ;
#50369=CARTESIAN_POINT('Ctrl Pts',(-20.9061303771679,-10.5279094158224,
123.232285620244)) ;
#50370=CARTESIAN_POINT('Ctrl Pts',(-20.5631517199141,-10.7179535983103,
123.061365279476)) ;
#50371=CARTESIAN_POINT('Ctrl Pts',(-20.8516285274051,-10.5379645178298,
122.97376743029)) ;
#50372=CARTESIAN_POINT('Ctrl Pts',(-20.4864480135789,-10.7277752716314,
122.869632358223)) ;
#50373=CARTESIAN_POINT('Ctrl Pts',(-20.7557521456489,-10.5477861911509,
122.734100762243)) ;
#50374=CARTESIAN_POINT('Ctrl Pts',(-20.3753148949047,-10.7378337427063,
122.689756073264)) ;
#50375=CARTESIAN_POINT('Ctrl Pts',(-20.6168357132107,-10.5578446622258,
122.509252277596)) ;
#50376=CARTESIAN_POINT('Ctrl Pts',(-20.2362698429268,-10.7477583538828,
122.534165638144)) ;
#50377=CARTESIAN_POINT('Ctrl Pts',(-20.4430403515289,-10.5677692734023,
122.314768071312)) ;
#50378=CARTESIAN_POINT('Ctrl Pts',(-20.0174236370264,-10.7610356927832,
122.360928612314)) ;
#50379=CARTESIAN_POINT('Ctrl Pts',(-20.1694406713987,-10.5810466123027,
122.098190251733)) ;
#50380=CARTESIAN_POINT('Ctrl Pts',(-19.7578453903065,-10.7743345720208,
122.248851511266)) ;
#50381=CARTESIAN_POINT('Ctrl Pts',(-19.8449850135388,-10.5943454915403,
121.958111265145)) ;
#50382=CARTESIAN_POINT('Ctrl Pts',(-19.4824813143237,-10.7875734441915,
122.208088439905)) ;
#50383=CARTESIAN_POINT('Ctrl Pts',(-19.5008057716461,-10.607584363711,121.907157355451)) ;
#50384=CARTESIAN_POINT('Ctrl Pts',(-19.2721785775522,-10.7975800623281,
122.213521358078)) ;
#50385=CARTESIAN_POINT('Ctrl Pts',(-19.2379220825648,-10.6175909818476,
121.913944971208)) ;
#50386=CARTESIAN_POINT('Ctrl Pts',(-19.0656000898289,-10.8076110073896,
122.255887753777)) ;
#50387=CARTESIAN_POINT('Ctrl Pts',(-18.9796997396923,-10.6276219269091,
121.966900411235)) ;
#50388=CARTESIAN_POINT('Ctrl Pts',(-18.8727746571245,-10.8174671807414,
122.33177975615)) ;
#50389=CARTESIAN_POINT('Ctrl Pts',(-18.7386663422547,-10.6374781002609,
122.061762842425)) ;
#50390=CARTESIAN_POINT('Ctrl Pts',(-18.6933942950045,-10.8274664517043,
122.441317819794)) ;
#50391=CARTESIAN_POINT('Ctrl Pts',(-18.5144394577593,-10.6474773712238,
122.198683103259)) ;
#50392=CARTESIAN_POINT('Ctrl Pts',(-18.5371942685893,-10.8373609034616,
122.578747643145)) ;
#50393=CARTESIAN_POINT('Ctrl Pts',(-18.3191873795342,-10.6573718229811,
122.370468477296)) ;
#50394=CARTESIAN_POINT('Ctrl Pts',(-18.4051122896899,-10.847424219271,122.743966469464)) ;
#50395=CARTESIAN_POINT('Ctrl Pts',(-18.1540827675879,-10.6674351387905,
122.576990252157)) ;
#50396=CARTESIAN_POINT('Ctrl Pts',(-18.3057391169289,-10.8572630760106,
122.925417587621)) ;
#50397=CARTESIAN_POINT('Ctrl Pts',(-18.0298636945232,-10.6772739955301,
122.80380319054)) ;
#50398=CARTESIAN_POINT('Ctrl Pts',(-18.2376490708675,-10.8673291978282,
123.125750203822)) ;
#50399=CARTESIAN_POINT('Ctrl Pts',(-17.9447485716292,-10.6873401173477,
123.054218033055)) ;
#50400=CARTESIAN_POINT('Ctrl Pts',(-18.2060503452321,-10.8772124255524,
123.331137906529)) ;
#50401=CARTESIAN_POINT('Ctrl Pts',(-17.9052474069522,-10.697223345072,123.310952604454)) ;
#50402=CARTESIAN_POINT('Ctrl Pts',(-18.2101816179164,-10.8872018868312,
123.541086163132)) ;
#50403=CARTESIAN_POINT('Ctrl Pts',(-17.9104088181944,-10.7072128063507,
123.573388107833)) ;
#50404=CARTESIAN_POINT('Ctrl Pts',(-18.2506800550467,-10.8971655972577,
123.746612755988)) ;
#50405=CARTESIAN_POINT('Ctrl Pts',(-17.9610292608973,-10.7171765167772,
123.830297050036)) ;
#50406=CARTESIAN_POINT('Ctrl Pts',(-18.3262823417106,-10.9071605999886,
123.942684202324)) ;
#50407=CARTESIAN_POINT('Ctrl Pts',(-18.0555296750301,-10.7271715195081,
124.075387412866)) ;
#50408=CARTESIAN_POINT('Ctrl Pts',(-18.4354992661144,-10.9171969309989,
124.123200848044)) ;
#50409=CARTESIAN_POINT('Ctrl Pts',(-18.1920485021804,-10.7372078505184,
124.301034604056)) ;
#50410=CARTESIAN_POINT('Ctrl Pts',(-18.5715282260324,-10.9270431603412,
124.279245467908)) ;
#50411=CARTESIAN_POINT('Ctrl Pts',(-18.3620830672947,-10.7470540798607,
124.496092551368)) ;
#50412=CARTESIAN_POINT('Ctrl Pts',(-18.734581283145,-10.9370286586164,124.411415680481)) ;
#50413=CARTESIAN_POINT('Ctrl Pts',(-18.5658978744819,-10.7570395781359,
124.661307440099)) ;
#50414=CARTESIAN_POINT('Ctrl Pts',(-18.9171658090595,-10.9469635615994,
124.512917995207)) ;
#50415=CARTESIAN_POINT('Ctrl Pts',(-18.7941275673887,-10.7669744811189,
124.788187738408)) ;
#50416=CARTESIAN_POINT('Ctrl Pts',(-19.1170341754858,-10.9570210646946,
124.581816159323)) ;
#50417=CARTESIAN_POINT('Ctrl Pts',(-19.0439620659481,-10.7770319842141,
124.87431287259)) ;
#50418=CARTESIAN_POINT('Ctrl Pts',(-19.3209344460454,-10.9668427210651,
124.614507954261)) ;
#50419=CARTESIAN_POINT('Ctrl Pts',(-19.2988377714655,-10.7868536405847,
124.915180256384)) ;
#50420=CARTESIAN_POINT('Ctrl Pts',(-19.5323077477126,-10.9768987837303,
124.611618015789)) ;
#50421=CARTESIAN_POINT('Ctrl Pts',(-19.5630543230825,-10.7969097032498,
124.911570311967)) ;
#50422=CARTESIAN_POINT('Ctrl Pts',(-19.7375399994228,-10.9868394484335,
124.572149859508)) ;
#50423=CARTESIAN_POINT('Ctrl Pts',(-19.8195954463956,-10.806850367953,124.862237558484)) ;
#50424=CARTESIAN_POINT('Ctrl Pts',(-19.932315810984,-10.996743852382,124.498530010297)) ;
#50425=CARTESIAN_POINT('Ctrl Pts',(-20.0630665621227,-10.8167547719015,
124.770214821818)) ;
#50426=CARTESIAN_POINT('Ctrl Pts',(-20.1138352643569,-11.0067903373756,
124.39058103883)) ;
#50427=CARTESIAN_POINT('Ctrl Pts',(-20.2899670416995,-10.8268012568951,
124.635280761928)) ;
#50428=CARTESIAN_POINT('Ctrl Pts',(-20.271611629066,-11.0166865651873,124.254920335698)) ;
#50429=CARTESIAN_POINT('Ctrl Pts',(-20.4871895042753,-10.8366974847068,
124.465706330345)) ;
#50430=CARTESIAN_POINT('Ctrl Pts',(-20.4056065237285,-11.0267461487508,
124.09133118011)) ;
#50431=CARTESIAN_POINT('Ctrl Pts',(-20.6546848717609,-10.8467570682703,
124.261221540637)) ;
#50432=CARTESIAN_POINT('Ctrl Pts',(-20.5070605056192,-11.0365981584196,
123.910749358251)) ;
#50433=CARTESIAN_POINT('Ctrl Pts',(-20.7815048416838,-10.8566090779391,
124.035494716895)) ;
#50434=CARTESIAN_POINT('Ctrl Pts',(-20.5770451368418,-11.0465606898592,
123.713354618847)) ;
#50435=CARTESIAN_POINT('Ctrl Pts',(-20.8689878384845,-10.8665716093787,
123.788751735745)) ;
#50436=CARTESIAN_POINT('Ctrl Pts',(-20.6116136924991,-11.0565922380985,
123.505305288482)) ;
#50437=CARTESIAN_POINT('Ctrl Pts',(-20.9122007991014,-10.8766031576181,
123.528690516746)) ;
#50438=CARTESIAN_POINT('Ctrl Pts',(-20.6097611314172,-11.0664836493116,
123.297365165469)) ;
#50439=CARTESIAN_POINT('Ctrl Pts',(-20.9098873497408,-10.8864945688311,
123.268764662023)) ;
#50440=CARTESIAN_POINT('Ctrl Pts',(-20.5717257520097,-11.0764999030196,
123.090247708174)) ;
#50441=CARTESIAN_POINT('Ctrl Pts',(-20.862345248179,-10.8965108225391,123.009867420348)) ;
#50442=CARTESIAN_POINT('Ctrl Pts',(-20.4977797269794,-11.0865300058643,
122.892777790247)) ;
#50443=CARTESIAN_POINT('Ctrl Pts',(-20.7699148715379,-10.9065409253838,
122.763029266248)) ;
#50444=CARTESIAN_POINT('Ctrl Pts',(-20.3928580773295,-11.096386454818,122.714076335493)) ;
#50445=CARTESIAN_POINT('Ctrl Pts',(-20.6387642263058,-10.9163973743375,
122.53965056498)) ;
#50446=CARTESIAN_POINT('Ctrl Pts',(-20.2567901765193,-11.1063854655903,
122.553889016232)) ;
#50447=CARTESIAN_POINT('Ctrl Pts',(-20.4686808695235,-10.9263963851098,
122.339414946257)) ;
#50448=CARTESIAN_POINT('Ctrl Pts',(-20.0967506938251,-11.1162806825083,
122.420933108959)) ;
#50449=CARTESIAN_POINT('Ctrl Pts',(-20.2686322563454,-10.9362916020278,
122.173218025888)) ;
#50450=CARTESIAN_POINT('Ctrl Pts',(-19.9130792390864,-11.1263411978656,
122.316112855486)) ;
#50451=CARTESIAN_POINT('Ctrl Pts',(-20.0390441622467,-10.9463521173851,
122.042191046808)) ;
#50452=CARTESIAN_POINT('Ctrl Pts',(-19.7181773873714,-11.1361904912527,
122.246149401792)) ;
#50453=CARTESIAN_POINT('Ctrl Pts',(-19.7954165502643,-10.9562014107722,
121.954734482314)) ;
#50454=CARTESIAN_POINT('Ctrl Pts',(-19.5105138121636,-11.1462176669327,
122.209933979005)) ;
#50455=CARTESIAN_POINT('Ctrl Pts',(-19.5358374377871,-10.9662285864522,
121.9094633788)) ;
#50456=CARTESIAN_POINT('Ctrl Pts',(-19.2996733625681,-11.1562462425598,
122.210880868471)) ;
#50457=CARTESIAN_POINT('Ctrl Pts',(-19.2722869357614,-10.9762571620794,
121.910644965915)) ;
#50458=CARTESIAN_POINT('Ctrl Pts',(-19.0959460919219,-11.1660913361057,
122.247342057068)) ;
#50459=CARTESIAN_POINT('Ctrl Pts',(-19.017626412583,-10.9861022556252,121.956219772702)) ;
#50460=CARTESIAN_POINT('Ctrl Pts',(-18.8985578247058,-11.1760825775375,
122.319166361709)) ;
#50461=CARTESIAN_POINT('Ctrl Pts',(-18.7708903037758,-10.996093497057,122.045998590294)) ;
#50462=CARTESIAN_POINT('Ctrl Pts',(-18.7160448813455,-11.1861183586808,
122.425022343304)) ;
#50463=CARTESIAN_POINT('Ctrl Pts',(-18.5427482921645,-11.0061292782003,
122.178316885851)) ;
#50464=CARTESIAN_POINT('Ctrl Pts',(-18.5574679836989,-11.1959705644105,
122.558254372856)) ;
#50465=CARTESIAN_POINT('Ctrl Pts',(-18.344525155852,-11.01598148393,122.344856285485)) ;
#50466=CARTESIAN_POINT('Ctrl Pts',(-18.4224794756724,-11.2059326585275,
122.718377576205)) ;
#50467=CARTESIAN_POINT('Ctrl Pts',(-18.1757880511084,-11.025943578047,122.545009574719)) ;
#50468=CARTESIAN_POINT('Ctrl Pts',(-18.3169268323872,-11.2159552193546,
122.900738727932)) ;
#50469=CARTESIAN_POINT('Ctrl Pts',(-18.0438458204898,-11.0359661388741,
122.772960142216)) ;
#50470=CARTESIAN_POINT('Ctrl Pts',(-18.2451248266948,-11.2258829910061,
123.096732722796)) ;
#50471=CARTESIAN_POINT('Ctrl Pts',(-17.9540915964206,-11.0458939105257,
123.017952668875)) ;
#50472=CARTESIAN_POINT('Ctrl Pts',(-18.2080492813558,-11.235925375131,123.304558510364)) ;
#50473=CARTESIAN_POINT('Ctrl Pts',(-17.9077456058753,-11.0559362946505,
123.277734456011)) ;
#50474=CARTESIAN_POINT('Ctrl Pts',(-18.2075431826477,-11.2458145992016,
123.512472427979)) ;
#50475=CARTESIAN_POINT('Ctrl Pts',(-17.9071113954451,-11.0658255187211,
123.537627775353)) ;
#50476=CARTESIAN_POINT('Ctrl Pts',(-18.2431137932323,-11.2558038473689,
123.719436413788)) ;
#50477=CARTESIAN_POINT('Ctrl Pts',(-17.9515732676146,-11.0758147668884,
123.796333212602)) ;
#50478=CARTESIAN_POINT('Ctrl Pts',(-18.3140127800185,-11.2657624244109,
123.916420734498)) ;
#50479=CARTESIAN_POINT('Ctrl Pts',(-18.0401957305614,-11.0857733439304,
124.042564530928)) ;
#50480=CARTESIAN_POINT('Ctrl Pts',(-18.4169840173117,-11.2756619935022,
124.097296523522)) ;
#50481=CARTESIAN_POINT('Ctrl Pts',(-18.1689090610639,-11.0956729130217,
124.268660685229)) ;
#50482=CARTESIAN_POINT('Ctrl Pts',(-18.5518230953768,-11.2857099055862,
124.259873078024)) ;
#50483=CARTESIAN_POINT('Ctrl Pts',(-18.3374567293609,-11.1057208251057,
124.471882073921)) ;
#50484=CARTESIAN_POINT('Ctrl Pts',(-18.7103328750192,-11.2956052598934,
124.394651304533)) ;
#50485=CARTESIAN_POINT('Ctrl Pts',(-18.53559381129,-11.1156161794129,124.640356432315)) ;
#50486=CARTESIAN_POINT('Ctrl Pts',(-18.8927897807584,-11.3056669103846,
124.50162581541)) ;
#50487=CARTESIAN_POINT('Ctrl Pts',(-18.7636640135305,-11.1256778299041,
124.774075514003)) ;
#50488=CARTESIAN_POINT('Ctrl Pts',(-19.0867894285585,-11.315511525847,124.573745609378)) ;
#50489=CARTESIAN_POINT('Ctrl Pts',(-19.0061643663833,-11.1355224453666,
124.864226909417)) ;
#50490=CARTESIAN_POINT('Ctrl Pts',(-19.2926054693123,-11.3254716047484,
124.612260164776)) ;
#50491=CARTESIAN_POINT('Ctrl Pts',(-19.263434682634,-11.145482524268,124.912371167907)) ;
#50492=CARTESIAN_POINT('Ctrl Pts',(-19.5036241030656,-11.3355097991068,
124.6140594671)) ;
#50493=CARTESIAN_POINT('Ctrl Pts',(-19.5272078042134,-11.1555207186263,
124.914621442972)) ;
#50494=CARTESIAN_POINT('Ctrl Pts',(-19.7084368116268,-11.3453835145064,
124.580138707835)) ;
#50495=CARTESIAN_POINT('Ctrl Pts',(-19.7832249579071,-11.1653944340259,
124.872221302339)) ;
#50496=CARTESIAN_POINT('Ctrl Pts',(-19.9081154986966,-11.3554552240407,
124.509785415039)) ;
#50497=CARTESIAN_POINT('Ctrl Pts',(-20.0328232712861,-11.1754661435602,
124.784280775746)) ;
#50498=CARTESIAN_POINT('Ctrl Pts',(-20.0882613339957,-11.3652876644932,
124.408381333972)) ;
#50499=CARTESIAN_POINT('Ctrl Pts',(-20.2580073161576,-11.1852985840127,
124.657525797751)) ;
#50500=CARTESIAN_POINT('Ctrl Pts',(-20.251660229155,-11.3753194854186,124.275048143701)) ;
#50501=CARTESIAN_POINT('Ctrl Pts',(-20.4622563155218,-11.1953304049381,
124.490859965189)) ;
#50502=CARTESIAN_POINT('Ctrl Pts',(-20.388818370831,-11.3853398553042,124.115153399644)) ;
#50503=CARTESIAN_POINT('Ctrl Pts',(-20.6337047074071,-11.2053507748237,
124.290992198971)) ;
#50504=CARTESIAN_POINT('Ctrl Pts',(-20.4949578126602,-11.3952066264379,
123.936918605361)) ;
#50505=CARTESIAN_POINT('Ctrl Pts',(-20.7663802890228,-11.2152175459574,
124.068198059802)) ;
#50506=CARTESIAN_POINT('Ctrl Pts',(-20.5700397801666,-11.4052773976273,
123.738981962488)) ;
#50507=CARTESIAN_POINT('Ctrl Pts',(-20.8602333251997,-11.2252883171468,
123.820777914761)) ;
#50508=CARTESIAN_POINT('Ctrl Pts',(-20.608748085118,-11.4151205581489,123.535688979496)) ;
#50509=CARTESIAN_POINT('Ctrl Pts',(-20.9086197173424,-11.2351314776684,
123.566660443412)) ;
#50510=CARTESIAN_POINT('Ctrl Pts',(-20.6122979783934,-11.4251007913353,
123.32590993056)) ;
#50511=CARTESIAN_POINT('Ctrl Pts',(-20.9130575839416,-11.2451117108548,
123.304436329193)) ;
#50512=CARTESIAN_POINT('Ctrl Pts',(-20.5788422571338,-11.4351193113705,
123.117968685033)) ;
#50513=CARTESIAN_POINT('Ctrl Pts',(-20.8712385790231,-11.25513023089,123.044509679207)) ;
#50514=CARTESIAN_POINT('Ctrl Pts',(-20.5111294875309,-11.4450026197542,
122.921507091262)) ;
#50515=CARTESIAN_POINT('Ctrl Pts',(-20.7865977120134,-11.2650135392737,
122.798931493899)) ;
#50516=CARTESIAN_POINT('Ctrl Pts',(-20.4083944122188,-11.455070903925,122.736483235784)) ;
#50517=CARTESIAN_POINT('Ctrl Pts',(-20.6581795185986,-11.2750818234445,
122.567651782526)) ;
#50518=CARTESIAN_POINT('Ctrl Pts',(-20.278392781555,-11.4649010305926,122.575789839308)) ;
#50519=CARTESIAN_POINT('Ctrl Pts',(-20.4956768375376,-11.2849119501121,
122.366783576156)) ;
#50520=CARTESIAN_POINT('Ctrl Pts',(-20.1189455476198,-11.4749676027992,
122.43668549405)) ;
#50521=CARTESIAN_POINT('Ctrl Pts',(-20.2963683003265,-11.2949785223187,
122.19290316997)) ;
#50522=CARTESIAN_POINT('Ctrl Pts',(-19.9408261904973,-11.4848577590399,
122.329373206102)) ;
#50523=CARTESIAN_POINT('Ctrl Pts',(-20.07371839416,-11.3048686785594,122.058761956605)) ;
#50524=CARTESIAN_POINT('Ctrl Pts',(-19.7449718071379,-11.4948502866163,
122.253435565076)) ;
#50525=CARTESIAN_POINT('Ctrl Pts',(-19.8289002832583,-11.3148612061358,
121.963839656132)) ;
#50526=CARTESIAN_POINT('Ctrl Pts',(-19.5394995838217,-11.5048117764906,
122.212958774971)) ;
#50527=CARTESIAN_POINT('Ctrl Pts',(-19.572059601315,-11.3248226960101,121.913243324839)) ;
#50528=CARTESIAN_POINT('Ctrl Pts',(-19.3312195995513,-11.5147209983778,
122.208316709471)) ;
#50529=CARTESIAN_POINT('Ctrl Pts',(-19.3117087063637,-11.3347319178973,
121.907440658184)) ;
#50530=CARTESIAN_POINT('Ctrl Pts',(-19.1224333832175,-11.5247695781881,
122.240425699493)) ;
#50531=CARTESIAN_POINT('Ctrl Pts',(-19.0507261790371,-11.3447804977076,
121.947576761734)) ;
#50532=CARTESIAN_POINT('Ctrl Pts',(-18.9256450998965,-11.5346525526582,
122.307117491957)) ;
#50533=CARTESIAN_POINT('Ctrl Pts',(-18.8047397505395,-11.3546634721777,
122.030941792002)) ;
#50534=CARTESIAN_POINT('Ctrl Pts',(-18.7411595782649,-11.5446474638009,
122.407688727702)) ;
#50535=CARTESIAN_POINT('Ctrl Pts',(-18.5741327463721,-11.3646583833204,
122.156656021912)) ;
#50536=CARTESIAN_POINT('Ctrl Pts',(-18.5766849466755,-11.5546678503745,
122.539338975724)) ;
#50537=CARTESIAN_POINT('Ctrl Pts',(-18.3685394794627,-11.374678769894,122.321218804719)) ;
#50538=CARTESIAN_POINT('Ctrl Pts',(-18.4390281447,-11.5645779542315,122.69570721258)) ;
#50539=CARTESIAN_POINT('Ctrl Pts',(-18.1964679001567,-11.3845888737511,
122.51667981643)) ;
#50540=CARTESIAN_POINT('Ctrl Pts',(-18.3299418694843,-11.5745056664414,
122.873650877876)) ;
#50541=CARTESIAN_POINT('Ctrl Pts',(-18.0601098922916,-11.394516585961,122.739110167139)) ;
#50542=CARTESIAN_POINT('Ctrl Pts',(-18.2526908814426,-11.5845487762087,
123.070140221989)) ;
#50543=CARTESIAN_POINT('Ctrl Pts',(-17.9635464109793,-11.4045596957282,
122.984721718086)) ;
#50544=CARTESIAN_POINT('Ctrl Pts',(-18.2112504293198,-11.5944351966642,
123.273822369061)) ;
#50545=CARTESIAN_POINT('Ctrl Pts',(-17.9117458663191,-11.4144461161838,
123.239325516345)) ;
#50546=CARTESIAN_POINT('Ctrl Pts',(-18.2053899399513,-11.6044283742699,
123.48381708741)) ;
#50547=CARTESIAN_POINT('Ctrl Pts',(-17.9044206320669,-11.4244392937894,
123.501819128661)) ;
#50548=CARTESIAN_POINT('Ctrl Pts',(-18.2360155974427,-11.6143740371738,
123.690651541286)) ;
#50549=CARTESIAN_POINT('Ctrl Pts',(-17.9427031376008,-11.4343849566933,
123.760362733626)) ;
#50550=CARTESIAN_POINT('Ctrl Pts',(-18.3016977196334,-11.624321333379,123.889202740392)) ;
#50551=CARTESIAN_POINT('Ctrl Pts',(-18.0248064635829,-11.4443322528985,
124.00855211509)) ;
#50552=CARTESIAN_POINT('Ctrl Pts',(-18.4020577550734,-11.6343690989569,
124.075068550386)) ;
#50553=CARTESIAN_POINT('Ctrl Pts',(-18.1502567638643,-11.4543800184764,
124.240883955251)) ;
#50554=CARTESIAN_POINT('Ctrl Pts',(-18.53043452236,-11.6442173121745,124.237499635771)) ;
#50555=CARTESIAN_POINT('Ctrl Pts',(-18.3107289742964,-11.464228231694,124.443923603848)) ;
#50556=CARTESIAN_POINT('Ctrl Pts',(-18.6863539195395,-11.6541768849686,
124.377247513015)) ;
#50557=CARTESIAN_POINT('Ctrl Pts',(-18.50562907952,-11.4741878044881,124.618608196157)) ;
#50558=CARTESIAN_POINT('Ctrl Pts',(-18.8657358234262,-11.6642135060011,
124.488337618152)) ;
#50559=CARTESIAN_POINT('Ctrl Pts',(-18.7298566495651,-11.4842244255206,
124.757470221492)) ;
#50560=CARTESIAN_POINT('Ctrl Pts',(-19.0585401018813,-11.6740940208114,
124.565687771704)) ;
#50561=CARTESIAN_POINT('Ctrl Pts',(-18.9708633136044,-11.494104940331,124.85415763862)) ;
#50562=CARTESIAN_POINT('Ctrl Pts',(-19.2653207495063,-11.6841466721185,
124.609197173488)) ;
#50563=CARTESIAN_POINT('Ctrl Pts',(-19.2293390121218,-11.504157591638,124.908543575185)) ;
#50564=CARTESIAN_POINT('Ctrl Pts',(-19.4732739400485,-11.6940420703985,
124.616120019601)) ;
#50565=CARTESIAN_POINT('Ctrl Pts',(-19.4892814881059,-11.514052989918,124.917196362711)) ;
#50566=CARTESIAN_POINT('Ctrl Pts',(-19.6824421140478,-11.7040921921046,
124.586475455409)) ;
#50567=CARTESIAN_POINT('Ctrl Pts',(-19.7507413265629,-11.5241031116241,
124.88013986058)) ;
#50568=CARTESIAN_POINT('Ctrl Pts',(-19.8800272774462,-11.7139764716465,
124.522061203542)) ;
#50569=CARTESIAN_POINT('Ctrl Pts',(-19.9977235239475,-11.533987391166,124.799620909496)) ;
#50570=CARTESIAN_POINT('Ctrl Pts',(-20.0656260604384,-11.7239712529384,
124.423592328542)) ;
#50571=CARTESIAN_POINT('Ctrl Pts',(-20.2297217102498,-11.5439821724579,
124.6765338389)) ;
#50572=CARTESIAN_POINT('Ctrl Pts',(-20.2305069833902,-11.7339190981252,
124.294916040327)) ;
#50573=CARTESIAN_POINT('Ctrl Pts',(-20.4358226951657,-11.5539300176447,
124.515687379196)) ;
#50574=CARTESIAN_POINT('Ctrl Pts',(-20.3705912261117,-11.7438560615126,
124.139963124901)) ;
#50575=CARTESIAN_POINT('Ctrl Pts',(-20.6109276228693,-11.5638669810321,
124.321995035013)) ;
#50576=CARTESIAN_POINT('Ctrl Pts',(-20.482403685854,-11.7538390262498,123.962322659801)) ;
#50577=CARTESIAN_POINT('Ctrl Pts',(-20.7506923361084,-11.5738499457693,
124.099943608009)) ;
#50578=CARTESIAN_POINT('Ctrl Pts',(-20.5617787036582,-11.7638828776654,
123.766682247549)) ;
#50579=CARTESIAN_POINT('Ctrl Pts',(-20.8499100761848,-11.583893797185,123.855392878915)) ;
#50580=CARTESIAN_POINT('Ctrl Pts',(-20.6055180822358,-11.7737110790002,
123.564713422646)) ;
#50581=CARTESIAN_POINT('Ctrl Pts',(-20.9045834155349,-11.5937219985197,
123.602930177834)) ;
#50582=CARTESIAN_POINT('Ctrl Pts',(-20.6138247387092,-11.7837876515982,
123.353078389392)) ;
#50583=CARTESIAN_POINT('Ctrl Pts',(-20.9149654651719,-11.6037985711178,
123.338386769827)) ;
#50584=CARTESIAN_POINT('Ctrl Pts',(-20.5859865681062,-11.7936397316058,
123.147790724545)) ;
#50585=CARTESIAN_POINT('Ctrl Pts',(-20.880166307973,-11.6136506511253,123.081776137389)) ;
#50586=CARTESIAN_POINT('Ctrl Pts',(-20.5217060175956,-11.8037130166099,
122.94604661898)) ;
#50587=CARTESIAN_POINT('Ctrl Pts',(-20.7998144514066,-11.6237239361294,
122.82959680013)) ;
#50588=CARTESIAN_POINT('Ctrl Pts',(-20.4255657745516,-11.8135543683204,
122.7628267317)) ;
#50589=CARTESIAN_POINT('Ctrl Pts',(-20.6796373592565,-11.6335652878399,
122.600571403664)) ;
#50590=CARTESIAN_POINT('Ctrl Pts',(-20.2981587765571,-11.8235158677169,
122.596634860964)) ;
#50591=CARTESIAN_POINT('Ctrl Pts',(-20.5203770953298,-11.6435267872364,
122.392832222476)) ;
#50592=CARTESIAN_POINT('Ctrl Pts',(-20.1424149976007,-11.8335516438469,
122.454293214028)) ;
#50593=CARTESIAN_POINT('Ctrl Pts',(-20.3256964582165,-11.6535625633664,
122.214906329133)) ;
#50594=CARTESIAN_POINT('Ctrl Pts',(-19.9670619376452,-11.8434400704844,
122.342638696447)) ;
#50595=CARTESIAN_POINT('Ctrl Pts',(-20.1065035193812,-11.663450990004,122.075338994146)) ;
#50596=CARTESIAN_POINT('Ctrl Pts',(-19.7726633460982,-11.8534553925594,
122.261733680716)) ;
#50597=CARTESIAN_POINT('Ctrl Pts',(-19.8635046296482,-11.6734663120789,
121.974209274792)) ;
#50598=CARTESIAN_POINT('Ctrl Pts',(-19.5667618955136,-11.8634857414596,
122.216223716099)) ;
#50599=CARTESIAN_POINT('Ctrl Pts',(-19.6061275734969,-11.6834966609791,
121.917323321404)) ;
#50600=CARTESIAN_POINT('Ctrl Pts',(-19.3600373542584,-11.8733291170662,
122.206909440911)) ;
#50601=CARTESIAN_POINT('Ctrl Pts',(-19.347720607516,-11.6933400365858,121.905682077626)) ;
#50602=CARTESIAN_POINT('Ctrl Pts',(-19.150888532225,-11.8833585539634,122.233670381781)) ;
#50603=CARTESIAN_POINT('Ctrl Pts',(-19.0862848802304,-11.7033694734829,
121.93913503971)) ;
#50604=CARTESIAN_POINT('Ctrl Pts',(-18.9496827788183,-11.8933904318963,
122.296907578933)) ;
#50605=CARTESIAN_POINT('Ctrl Pts',(-18.8347782583479,-11.7134013514158,
122.018183058997)) ;
#50606=CARTESIAN_POINT('Ctrl Pts',(-18.7661111079611,-11.9032200550018,
122.391777133203)) ;
#50607=CARTESIAN_POINT('Ctrl Pts',(-18.6053133474058,-11.7232309745213,
122.13677215079)) ;
#50608=CARTESIAN_POINT('Ctrl Pts',(-18.5987322084384,-11.9132095261549,
122.518627177409)) ;
#50609=CARTESIAN_POINT('Ctrl Pts',(-18.3960907643913,-11.7332204456744,
122.295336373426)) ;
#50610=CARTESIAN_POINT('Ctrl Pts',(-18.4555426602971,-11.9232533749173,
122.673809920536)) ;
#50611=CARTESIAN_POINT('Ctrl Pts',(-18.2171052461789,-11.7432642944368,
122.489315907923)) ;
#50612=CARTESIAN_POINT('Ctrl Pts',(-18.3436356389824,-11.933075080449,122.847337567212)) ;
#50613=CARTESIAN_POINT('Ctrl Pts',(-18.0772224087066,-11.7530859999685,
122.70622755982)) ;
#50614=CARTESIAN_POINT('Ctrl Pts',(-18.2613427697256,-11.9431101202768,
123.041592805838)) ;
#50615=CARTESIAN_POINT('Ctrl Pts',(-17.9743582754355,-11.7631210397963,
122.949047319972)) ;
#50616=CARTESIAN_POINT('Ctrl Pts',(-18.2146441937951,-11.9531348271682,
123.247112574505)) ;
#50617=CARTESIAN_POINT('Ctrl Pts',(-17.9159869174325,-11.7731457466878,
123.205947428696)) ;
#50618=CARTESIAN_POINT('Ctrl Pts',(-18.2040790572873,-11.962987531509,123.453976992299)) ;
#50619=CARTESIAN_POINT('Ctrl Pts',(-17.9027824758796,-11.7829984510285,
123.464529062491)) ;
#50620=CARTESIAN_POINT('Ctrl Pts',(-18.2295779813126,-11.9729756537167,
123.662389605254)) ;
#50621=CARTESIAN_POINT('Ctrl Pts',(-17.9346582753254,-11.7929865732362,
123.725044751931)) ;
#50622=CARTESIAN_POINT('Ctrl Pts',(-18.2905062794645,-11.982904123824,123.862032052655)) ;
#50623=CARTESIAN_POINT('Ctrl Pts',(-18.0108208428839,-11.8029150433435,
123.974597685058)) ;
#50624=CARTESIAN_POINT('Ctrl Pts',(-18.3854419619658,-11.9928931009912,
124.049358952293)) ;
#50625=CARTESIAN_POINT('Ctrl Pts',(-18.1294925170237,-11.8129040205107,
124.208755459254)) ;
#50626=CARTESIAN_POINT('Ctrl Pts',(-18.51235689706,-12.0029309082709,124.217948281748)) ;
#50627=CARTESIAN_POINT('Ctrl Pts',(-18.288137840982,-11.8229418277904,124.419490767738)) ;
#50628=CARTESIAN_POINT('Ctrl Pts',(-18.6634476701596,-12.0127772091342,
124.359445076949)) ;
#50629=CARTESIAN_POINT('Ctrl Pts',(-18.4770035095754,-11.8327881286537,
124.596360779369)) ;
#50630=CARTESIAN_POINT('Ctrl Pts',(-18.8397147754035,-12.0228029525135,
124.475014140463)) ;
#50631=CARTESIAN_POINT('Ctrl Pts',(-18.6973386410408,-11.842813872033,124.740820127215)) ;
#50632=CARTESIAN_POINT('Ctrl Pts',(-19.03368933323,-12.0328338189525,124.557760416671)) ;
#50633=CARTESIAN_POINT('Ctrl Pts',(-18.9398076656581,-11.852844738472,124.844250930718)) ;
#50634=CARTESIAN_POINT('Ctrl Pts',(-19.2350138531615,-12.0426711777513,
124.605047798355)) ;
#50635=CARTESIAN_POINT('Ctrl Pts',(-19.191464763686,-11.8626820972708,124.903358127503)) ;
#50636=CARTESIAN_POINT('Ctrl Pts',(-19.4447121805973,-12.052663138685,124.61740552715)) ;
#50637=CARTESIAN_POINT('Ctrl Pts',(-19.4535879451902,-11.8726740582045,
124.918802860039)) ;
#50638=CARTESIAN_POINT('Ctrl Pts',(-19.654174209039,-12.0626955012416,124.59264506007)) ;
#50639=CARTESIAN_POINT('Ctrl Pts',(-19.7154151681685,-11.8827064207611,
124.887849956872)) ;
#50640=CARTESIAN_POINT('Ctrl Pts',(-19.8528431822894,-12.072560661816,124.53314903407)) ;
#50641=CARTESIAN_POINT('Ctrl Pts',(-19.9637513982511,-11.8925715813355,
124.813477415279)) ;
#50642=CARTESIAN_POINT('Ctrl Pts',(-20.0402625333132,-12.0825225663937,
124.439673578487)) ;
#50643=CARTESIAN_POINT('Ctrl Pts',(-20.1980246865614,-11.9025334859132,
124.696630723516)) ;
#50644=CARTESIAN_POINT('Ctrl Pts',(-20.2096190237234,-12.0925574964694,
124.313895264945)) ;
#50645=CARTESIAN_POINT('Ctrl Pts',(-20.4097188089495,-11.9125684159889,
124.539405883278)) ;
#50646=CARTESIAN_POINT('Ctrl Pts',(-20.3526800116948,-12.102442443323,124.163124144137)) ;
#50647=CARTESIAN_POINT('Ctrl Pts',(-20.5885436052506,-11.9224533628425,
124.350939834847)) ;
#50648=CARTESIAN_POINT('Ctrl Pts',(-20.4694104296519,-12.1125081196345,
123.986661950019)) ;
#50649=CARTESIAN_POINT('Ctrl Pts',(-20.7344544463685,-11.932519039154,124.13036082969)) ;
#50650=CARTESIAN_POINT('Ctrl Pts',(-20.5520515995571,-12.1223470392694,
123.797005493285)) ;
#50651=CARTESIAN_POINT('Ctrl Pts',(-20.8377538537587,-11.9423579587889,
123.893288587483)) ;
#50652=CARTESIAN_POINT('Ctrl Pts',(-20.6018640316816,-12.1324105490038,
123.591417354039)) ;
#50653=CARTESIAN_POINT('Ctrl Pts',(-20.9000168315464,-11.9524214685233,
123.636302931618)) ;
#50654=CARTESIAN_POINT('Ctrl Pts',(-20.6148291614051,-12.1423041621656,
123.383802604213)) ;
#50655=CARTESIAN_POINT('Ctrl Pts',(-20.9162207083321,-11.9623150816851,
123.376783859031)) ;
#50656=CARTESIAN_POINT('Ctrl Pts',(-20.5919863900176,-12.152248168979,123.176028489943)) ;
#50657=CARTESIAN_POINT('Ctrl Pts',(-20.8876645645134,-11.9722590884985,
123.117066234062)) ;
#50658=CARTESIAN_POINT('Ctrl Pts',(-20.5331562624697,-12.1622491233333,
122.974141880329)) ;
#50659=CARTESIAN_POINT('Ctrl Pts',(-20.8141243157822,-11.9822600428528,
122.864708641729)) ;
#50660=CARTESIAN_POINT('Ctrl Pts',(-20.4394990832698,-12.1722878810256,
122.785036123018)) ;
#50661=CARTESIAN_POINT('Ctrl Pts',(-20.6970504998674,-11.9922988005451,
122.628327620901)) ;
#50662=CARTESIAN_POINT('Ctrl Pts',(-20.3174467550257,-12.1821120651956,
122.618401426981)) ;
#50663=CARTESIAN_POINT('Ctrl Pts',(-20.5444825753375,-12.0021229847151,
122.420035360874)) ;
#50664=CARTESIAN_POINT('Ctrl Pts',(-20.1650056351834,-12.192170130795,122.471888778406)) ;
#50665=CARTESIAN_POINT('Ctrl Pts',(-20.353929339677,-12.0121810503145,122.236896566172)) ;
#50666=CARTESIAN_POINT('Ctrl Pts',(-19.9914963261328,-12.2021001775697,
122.355781356402)) ;
#50667=CARTESIAN_POINT('Ctrl Pts',(-20.1370409748098,-12.0221110970892,
122.09176436784)) ;
#50668=CARTESIAN_POINT('Ctrl Pts',(-19.8002835579305,-12.2120516199068,
122.270882760811)) ;
#50669=CARTESIAN_POINT('Ctrl Pts',(-19.8980237232306,-12.0320625394263,
121.985643564512)) ;
#50670=CARTESIAN_POINT('Ctrl Pts',(-19.5952237413981,-12.2220984170861,
122.220273264171)) ;
#50671=CARTESIAN_POINT('Ctrl Pts',(-19.641698308601,-12.0421093366056,121.922384338782)) ;
#50672=CARTESIAN_POINT('Ctrl Pts',(-19.388673024252,-12.2319463577662,122.206126303153)) ;
#50673=CARTESIAN_POINT('Ctrl Pts',(-19.3835093232641,-12.0519572772857,
121.904703348146)) ;
#50674=CARTESIAN_POINT('Ctrl Pts',(-19.180367514707,-12.2419079891088,122.227663750523)) ;
#50675=CARTESIAN_POINT('Ctrl Pts',(-19.1231275996939,-12.0619189086283,
121.931627958094)) ;
#50676=CARTESIAN_POINT('Ctrl Pts',(-18.9776624918692,-12.2519366484847,
122.285690175812)) ;
#50677=CARTESIAN_POINT('Ctrl Pts',(-18.869747044192,-12.0719475680042,122.004163670663)) ;
#50678=CARTESIAN_POINT('Ctrl Pts',(-18.7903389023048,-12.2618469513729,
122.376871314838)) ;
#50679=CARTESIAN_POINT('Ctrl Pts',(-18.6355935849324,-12.0818578708924,
122.118142692973)) ;
#50680=CARTESIAN_POINT('Ctrl Pts',(-18.6209407245683,-12.2717818459351,
122.499062432989)) ;
#50681=CARTESIAN_POINT('Ctrl Pts',(-18.4238474018539,-12.0917927654546,
122.270883952905)) ;
#50682=CARTESIAN_POINT('Ctrl Pts',(-18.4739251947791,-12.281822944602,122.650538595866)) ;
#50683=CARTESIAN_POINT('Ctrl Pts',(-18.2400799716367,-12.1018338641215,
122.460231143075)) ;
#50684=CARTESIAN_POINT('Ctrl Pts',(-18.3571294374524,-12.2917102271064,
122.822498446866)) ;
#50685=CARTESIAN_POINT('Ctrl Pts',(-18.094087509158,-12.1117211466259,122.67518267211)) ;
#50686=CARTESIAN_POINT('Ctrl Pts',(-18.270751539422,-12.3017019676169,123.013960222828)) ;
#50687=CARTESIAN_POINT('Ctrl Pts',(-17.9861176821352,-12.1217128871364,
122.914511116754)) ;
#50688=CARTESIAN_POINT('Ctrl Pts',(-18.2192070084759,-12.3116525168523,
123.216713043698)) ;
#50689=CARTESIAN_POINT('Ctrl Pts',(-17.9216897294066,-12.1316634363718,
123.167952928698)) ;
#50690=CARTESIAN_POINT('Ctrl Pts',(-18.203364387181,-12.3215881944871,123.424977839185)) ;
#50691=CARTESIAN_POINT('Ctrl Pts',(-17.9018892646537,-12.1415991140066,
123.42828420322)) ;
#50692=CARTESIAN_POINT('Ctrl Pts',(-18.2238062767761,-12.3315736122799,
123.63392140019)) ;
#50693=CARTESIAN_POINT('Ctrl Pts',(-17.9274444396139,-12.1515845317994,
123.689463440915)) ;
#50694=CARTESIAN_POINT('Ctrl Pts',(-18.2807096673845,-12.3416024051504,
123.83693264531)) ;
#50695=CARTESIAN_POINT('Ctrl Pts',(-17.9985764203864,-12.1616133246699,
123.943226816806)) ;
#50696=CARTESIAN_POINT('Ctrl Pts',(-18.3704393887249,-12.3514819163783,
124.024245376824)) ;
#50697=CARTESIAN_POINT('Ctrl Pts',(-18.1107411248912,-12.1714928358979,
124.177366527478)) ;
#50698=CARTESIAN_POINT('Ctrl Pts',(-18.4923386110279,-12.3614754530513,
124.195371559684)) ;
#50699=CARTESIAN_POINT('Ctrl Pts',(-18.2631174663862,-12.1814863725708,
124.391272663602)) ;
#50700=CARTESIAN_POINT('Ctrl Pts',(-18.6429752247149,-12.3715077213151,
124.342978657029)) ;
#50701=CARTESIAN_POINT('Ctrl Pts',(-18.4514152852325,-12.1915186408346,
124.575779592157)) ;
#50702=CARTESIAN_POINT('Ctrl Pts',(-18.8138083567616,-12.381371683321,124.460571682728)) ;
#50703=CARTESIAN_POINT('Ctrl Pts',(-18.6649582254015,-12.2013826028405,
124.722768521465)) ;
#50704=CARTESIAN_POINT('Ctrl Pts',(-19.0063512318433,-12.3914417446659,
124.548529857693)) ;
#50705=CARTESIAN_POINT('Ctrl Pts',(-18.905638121289,-12.2114526641854,124.832713751757)) ;
#50706=CARTESIAN_POINT('Ctrl Pts',(-19.2066412567903,-12.4012841090146,
124.600516981642)) ;
#50707=CARTESIAN_POINT('Ctrl Pts',(-19.1560012005411,-12.2212950285341,
124.897694900769)) ;
#50708=CARTESIAN_POINT('Ctrl Pts',(-19.4153191948693,-12.4112447815171,
124.61790415066)) ;
#50709=CARTESIAN_POINT('Ctrl Pts',(-19.4168488001027,-12.2312557010366,
124.919426126901)) ;
#50710=CARTESIAN_POINT('Ctrl Pts',(-19.6254227673264,-12.4212828525849,
124.598226325567)) ;
#50711=CARTESIAN_POINT('Ctrl Pts',(-19.6794781670687,-12.2412937721044,
124.894826056609)) ;
#50712=CARTESIAN_POINT('Ctrl Pts',(-19.8257277780076,-12.4311564675453,
124.54365478677)) ;
#50713=CARTESIAN_POINT('Ctrl Pts',(-19.9298584470985,-12.2511673870648,
124.826609084916)) ;
#50714=CARTESIAN_POINT('Ctrl Pts',(-20.0172039066253,-12.4412287021266,
124.453332611574)) ;
#50715=CARTESIAN_POINT('Ctrl Pts',(-20.1692027686534,-12.2612396216461,
124.713703675033)) ;
#50716=CARTESIAN_POINT('Ctrl Pts',(-20.1860304534501,-12.4510527205754,
124.334292333234)) ;
#50717=CARTESIAN_POINT('Ctrl Pts',(-20.3802336085828,-12.2710636400949,
124.56490174171)) ;
#50718=CARTESIAN_POINT('Ctrl Pts',(-20.3353241205461,-12.4611176415514,
124.184411186943)) ;
#50719=CARTESIAN_POINT('Ctrl Pts',(-20.5668505340547,-12.2811285610709,
124.377546847526)) ;
#50720=CARTESIAN_POINT('Ctrl Pts',(-20.4942292788694,-12.4743279398461,
123.956554640027)) ;
#50721=CARTESIAN_POINT('Ctrl Pts',(-20.7654710390159,-12.2943388593657,
124.092731380787)) ;
#50722=CARTESIAN_POINT('Ctrl Pts',(-20.5910323234022,-12.4876433865781,
123.690569761034)) ;
#50723=CARTESIAN_POINT('Ctrl Pts',(-20.8864681736876,-12.3076543060976,
123.760293059377)) ;
#50724=CARTESIAN_POINT('Ctrl Pts',(-20.6153241142933,-12.5009336318454,
123.412181900129)) ;
#50725=CARTESIAN_POINT('Ctrl Pts',(-20.9168412404455,-12.3209445513649,
123.412248798329)) ;
#50726=CARTESIAN_POINT('Ctrl Pts',(-20.5967460044986,-12.5109843814525,
123.20173674764)) ;
#50727=CARTESIAN_POINT('Ctrl Pts',(-20.8936136566243,-12.330995300972,123.149204261549)) ;
#50728=CARTESIAN_POINT('Ctrl Pts',(-20.5435845802291,-12.5207969884347,
123.002381741764)) ;
#50729=CARTESIAN_POINT('Ctrl Pts',(-20.8271599102325,-12.3408079079542,
122.900008574039)) ;
#50730=CARTESIAN_POINT('Ctrl Pts',(-20.4546049045706,-12.530868086429,122.81028950204)) ;
#50731=CARTESIAN_POINT('Ctrl Pts',(-20.71593398742,-12.3508790059485,122.659895486336)) ;
#50732=CARTESIAN_POINT('Ctrl Pts',(-20.3356089336191,-12.5407576592038,
122.639785901111)) ;
#50733=CARTESIAN_POINT('Ctrl Pts',(-20.5671825472654,-12.3607685787234,
122.446765213206)) ;
#50734=CARTESIAN_POINT('Ctrl Pts',(-20.1392326312349,-12.5540277660071,
122.441591528531)) ;
#50735=CARTESIAN_POINT('Ctrl Pts',(-20.3217335959038,-12.3740386855267,
122.199036770017)) ;
#50736=CARTESIAN_POINT('Ctrl Pts',(-19.8341063016993,-12.5706444529296,
122.263562945351)) ;
#50737=CARTESIAN_POINT('Ctrl Pts',(-19.9402799223981,-12.3906553724492,
121.976489962995)) ;
#50738=CARTESIAN_POINT('Ctrl Pts',(-19.4873858216236,-12.5872184962459,
122.20023473755)) ;
#50739=CARTESIAN_POINT('Ctrl Pts',(-19.5069560654211,-12.4072294157654,
121.897341845689)) ;
#50740=CARTESIAN_POINT('Ctrl Pts',(-19.208770852032,-12.6005150636777,122.222555120843)) ;
#50741=CARTESIAN_POINT('Ctrl Pts',(-19.1586250795814,-12.4205259831972,
121.925240968507)) ;
#50742=CARTESIAN_POINT('Ctrl Pts',(-19.004699994285,-12.6105451272551,122.27569208682)) ;
#50743=CARTESIAN_POINT('Ctrl Pts',(-18.9035497914933,-12.4305560467746,
121.99166480072)) ;
#50744=CARTESIAN_POINT('Ctrl Pts',(-18.8155802354143,-12.6204390191043,
122.362230085653)) ;
#50745=CARTESIAN_POINT('Ctrl Pts',(-18.6671468528082,-12.4404499386238,
122.099840645801)) ;
#50746=CARTESIAN_POINT('Ctrl Pts',(-18.5855888789982,-12.6336917748899,
122.519603205496)) ;
#50747=CARTESIAN_POINT('Ctrl Pts',(-18.3796682059846,-12.4537026944094,
122.29654963732)) ;
#50748=CARTESIAN_POINT('Ctrl Pts',(-18.354522049861,-12.6504198798823,122.789922613237)) ;
#50749=CARTESIAN_POINT('Ctrl Pts',(-18.0908280311932,-12.4704307994018,
122.634462100616)) ;
#50750=CARTESIAN_POINT('Ctrl Pts',(-18.2063394457701,-12.6702507163608,
123.184767083892)) ;
#50751=CARTESIAN_POINT('Ctrl Pts',(-17.9056069775823,-12.4902616358803,
123.128014485486)) ;
#50752=CARTESIAN_POINT('Ctrl Pts',(-18.2007363155492,-12.690176108251,123.608303510177)) ;
#50753=CARTESIAN_POINT('Ctrl Pts',(-17.8986058472055,-12.5101870277705,
123.657435239702)) ;
#50754=CARTESIAN_POINT('Ctrl Pts',(-18.3400998829644,-12.710101321603,124.008460954811)) ;
#50755=CARTESIAN_POINT('Ctrl Pts',(-18.072813481075,-12.5301122411225,124.157630024527)) ;
#50756=CARTESIAN_POINT('Ctrl Pts',(-18.6074924622381,-12.7300263350881,
124.337014382701)) ;
#50757=CARTESIAN_POINT('Ctrl Pts',(-18.4070561282593,-12.5500372546076,
124.568319257499)) ;
#50758=CARTESIAN_POINT('Ctrl Pts',(-18.9698313696597,-12.7499028067881,
124.554607895198)) ;
#50759=CARTESIAN_POINT('Ctrl Pts',(-18.8599799730538,-12.5699137263076,
124.840308097152)) ;
#50760=CARTESIAN_POINT('Ctrl Pts',(-19.3867523160162,-12.7698821246969,
124.636089846791)) ;
#50761=CARTESIAN_POINT('Ctrl Pts',(-19.3811313633257,-12.5898930442165,
124.942158139895)) ;
#50762=CARTESIAN_POINT('Ctrl Pts',(-19.8054691433214,-12.7898151282729,
124.570240660478)) ;
#50763=CARTESIAN_POINT('Ctrl Pts',(-19.904526260389,-12.6098260477925,124.859844414658)) ;
#50764=CARTESIAN_POINT('Ctrl Pts',(-20.1760444374323,-12.8097103983006,
124.366269150013)) ;
#50765=CARTESIAN_POINT('Ctrl Pts',(-20.3677432425444,-12.6297213178202,
124.604878989456)) ;
#50766=CARTESIAN_POINT('Ctrl Pts',(-20.4554911510886,-12.8296317362065,
124.047921898696)) ;
#50767=CARTESIAN_POINT('Ctrl Pts',(-20.7170498597673,-12.649642655726,124.206944794391)) ;
#50768=CARTESIAN_POINT('Ctrl Pts',(-20.6097246596929,-12.8495893594727,
123.652566976865)) ;
#50769=CARTESIAN_POINT('Ctrl Pts',(-20.9098403567553,-12.6696002789922,
123.712751204381)) ;
#50770=CARTESIAN_POINT('Ctrl Pts',(-20.6198419912611,-12.8694691914299,
123.23005419397)) ;
#50771=CARTESIAN_POINT('Ctrl Pts',(-20.9224859852008,-12.6894801109494,
123.18461209714)) ;
#50772=CARTESIAN_POINT('Ctrl Pts',(-20.4862162340303,-12.8893510427268,
122.828900869269)) ;
#50773=CARTESIAN_POINT('Ctrl Pts',(-20.755454544681,-12.7093619622463,122.683172172741)) ;
#50774=CARTESIAN_POINT('Ctrl Pts',(-20.2206736454974,-12.9094220598306,
122.494883082429)) ;
#50775=CARTESIAN_POINT('Ctrl Pts',(-20.4235254245616,-12.7294329793501,
122.265649140896)) ;
#50776=CARTESIAN_POINT('Ctrl Pts',(-19.8617901510047,-12.9292292835837,
122.274337723655)) ;
#50777=CARTESIAN_POINT('Ctrl Pts',(-19.974923765594,-12.7492402031032,121.989968961296)) ;
#50778=CARTESIAN_POINT('Ctrl Pts',(-19.4458827143192,-12.9492104191524,
122.187802603992)) ;
#50779=CARTESIAN_POINT('Ctrl Pts',(-19.4550399386843,-12.769221338672,121.881799009353)) ;
#50780=CARTESIAN_POINT('Ctrl Pts',(-19.0266575984833,-12.9691379124917,
122.249044591949)) ;
#50781=CARTESIAN_POINT('Ctrl Pts',(-18.9310095255051,-12.7891488320112,
121.958350587115)) ;
#50782=CARTESIAN_POINT('Ctrl Pts',(-18.6546793341104,-12.9889585738495,
122.447395484881)) ;
#50783=CARTESIAN_POINT('Ctrl Pts',(-18.466037843445,-12.808969493369,122.206286369056)) ;
#50784=CARTESIAN_POINT('Ctrl Pts',(-18.3694697209431,-13.0090557630713,
122.765395487489)) ;
#50785=CARTESIAN_POINT('Ctrl Pts',(-18.109523705677,-12.8290666825908,122.6037861273)) ;
#50786=CARTESIAN_POINT('Ctrl Pts',(-18.2121462510153,-13.0288194420796,
123.155285689063)) ;
#50787=CARTESIAN_POINT('Ctrl Pts',(-17.912868524015,-12.8488303615991,123.091145395835)) ;
#50788=CARTESIAN_POINT('Ctrl Pts',(-18.1966161351743,-13.0488767207527,
123.581287391373)) ;
#50789=CARTESIAN_POINT('Ctrl Pts',(-17.8934532248138,-12.8688876402722,
123.623648070262)) ;
#50790=CARTESIAN_POINT('Ctrl Pts',(-18.3260055582142,-13.0686721445001,
123.981930815811)) ;
#50791=CARTESIAN_POINT('Ctrl Pts',(-18.0551868056977,-12.8886830640196,
124.124451004314)) ;
#50792=CARTESIAN_POINT('Ctrl Pts',(-18.585401546907,-13.0886357892277,124.317872249246)) ;
#50793=CARTESIAN_POINT('Ctrl Pts',(-18.3794288062783,-12.9086467087472,
124.544379679974)) ;
#50794=CARTESIAN_POINT('Ctrl Pts',(-18.9448204747835,-13.1086192805018,
124.544510743668)) ;
#50795=CARTESIAN_POINT('Ctrl Pts',(-18.8287006510793,-12.9286302000213,
124.82768037988)) ;
#50796=CARTESIAN_POINT('Ctrl Pts',(-19.3561968961379,-13.1284267756511,
124.634949141891)) ;
#50797=CARTESIAN_POINT('Ctrl Pts',(-19.3429186866214,-12.9484376951706,
124.94073162018)) ;
#50798=CARTESIAN_POINT('Ctrl Pts',(-19.7773691623945,-13.1484093663712,
124.579587344744)) ;
#50799=CARTESIAN_POINT('Ctrl Pts',(-19.8693844497786,-12.9684202858907,
124.871533418585)) ;
#50800=CARTESIAN_POINT('Ctrl Pts',(-20.1526165065807,-13.1682920203624,
124.384654627234)) ;
#50801=CARTESIAN_POINT('Ctrl Pts',(-20.3384447755885,-12.988302939882,124.627871581508)) ;
#50802=CARTESIAN_POINT('Ctrl Pts',(-20.4400164199857,-13.1882502652255,
124.072540016501)) ;
#50803=CARTESIAN_POINT('Ctrl Pts',(-20.6976976849805,-13.008261184745,124.237731507752)) ;
#50804=CARTESIAN_POINT('Ctrl Pts',(-20.6032765964651,-13.2081258522671,
123.682670644288)) ;
#50805=CARTESIAN_POINT('Ctrl Pts',(-20.9017768871207,-13.0281367717866,
123.750397269488)) ;
#50806=CARTESIAN_POINT('Ctrl Pts',(-20.6240984710499,-13.2281067404023,
123.258361807286)) ;
#50807=CARTESIAN_POINT('Ctrl Pts',(-20.9278087945966,-13.0481176599219,
123.220011471901)) ;
#50808=CARTESIAN_POINT('Ctrl Pts',(-20.498818644834,-13.2480418815133,122.853364041742)) ;
#50809=CARTESIAN_POINT('Ctrl Pts',(-20.7712144055599,-13.0680528010329,
122.713763278136)) ;
#50810=CARTESIAN_POINT('Ctrl Pts',(-20.2434545299471,-13.2679538995244,
122.515712779495)) ;
#50811=CARTESIAN_POINT('Ctrl Pts',(-20.4520106817377,-13.0879648190439,
122.291696114126)) ;
#50812=CARTESIAN_POINT('Ctrl Pts',(-19.8888180187742,-13.287842117768,122.285335601894)) ;
#50813=CARTESIAN_POINT('Ctrl Pts',(-20.00872858781,-13.1078530372875,122.003722192525)) ;
#50814=CARTESIAN_POINT('Ctrl Pts',(-19.5451472567373,-13.3044404216149,
122.205327702706)) ;
#50815=CARTESIAN_POINT('Ctrl Pts',(-19.5791090604786,-13.1244513411344,
121.903703056024)) ;
#50816=CARTESIAN_POINT('Ctrl Pts',(-19.2662111497509,-13.3177130115177,
122.214345970221)) ;
#50817=CARTESIAN_POINT('Ctrl Pts',(-19.2304680801221,-13.1377239310372,
121.914976366428)) ;
#50818=CARTESIAN_POINT('Ctrl Pts',(-19.0602727562378,-13.3277204264686,
122.257344197933)) ;
#50819=CARTESIAN_POINT('Ctrl Pts',(-18.9730360738755,-13.1477313459881,
121.968723010214)) ;
#50820=CARTESIAN_POINT('Ctrl Pts',(-18.8649743558658,-13.3377277732012,
122.335630979356)) ;
#50821=CARTESIAN_POINT('Ctrl Pts',(-18.7289237746943,-13.1577386927207,
122.066570256141)) ;
#50822=CARTESIAN_POINT('Ctrl Pts',(-18.6279877995192,-13.3509941330028,
122.482594738179)) ;
#50823=CARTESIAN_POINT('Ctrl Pts',(-18.4326373530418,-13.1710050525223,
122.25031691369)) ;
#50824=CARTESIAN_POINT('Ctrl Pts',(-18.38714068302,-13.3675087906257,122.738147005354)) ;
#50825=CARTESIAN_POINT('Ctrl Pts',(-18.1316373286166,-13.1875197101453,
122.569692622174)) ;
#50826=CARTESIAN_POINT('Ctrl Pts',(-18.2465546320846,-13.3841062238684,
123.06176278507)) ;
#50827=CARTESIAN_POINT('Ctrl Pts',(-17.9558681005146,-13.2041171433879,
122.974265631434)) ;
#50828=CARTESIAN_POINT('Ctrl Pts',(-18.2054801703779,-13.3974542210134,
123.339422999475)) ;
#50829=CARTESIAN_POINT('Ctrl Pts',(-17.9045373894855,-13.2174651405329,
123.321302564881)) ;
#50830=CARTESIAN_POINT('Ctrl Pts',(-18.2109540995371,-13.407349975365,123.547385217031)) ;
#50831=CARTESIAN_POINT('Ctrl Pts',(-17.9113737955999,-13.2273608948845,
123.581262925404)) ;
#50832=CARTESIAN_POINT('Ctrl Pts',(-18.2525836667426,-13.4173379292963,
123.753181102987)) ;
#50833=CARTESIAN_POINT('Ctrl Pts',(-17.9634088819123,-13.2373488488159,
123.838506352594)) ;
#50834=CARTESIAN_POINT('Ctrl Pts',(-18.3290068072186,-13.4272951530011,
123.948090648861)) ;
#50835=CARTESIAN_POINT('Ctrl Pts',(-18.058934973792,-13.2473060725206,124.082144873738)) ;
#50836=CARTESIAN_POINT('Ctrl Pts',(-18.4390335780382,-13.4373306995577,
124.128090732076)) ;
#50837=CARTESIAN_POINT('Ctrl Pts',(-18.1964661584521,-13.2573416190773,
124.307146372582)) ;
#50838=CARTESIAN_POINT('Ctrl Pts',(-18.576478403772,-13.4472178108339,124.284038519252)) ;
#50839=CARTESIAN_POINT('Ctrl Pts',(-18.3682700532266,-13.2672287303534,
124.502082982848)) ;
#50840=CARTESIAN_POINT('Ctrl Pts',(-18.7403986017361,-13.4572092159347,
124.415367414347)) ;
#50841=CARTESIAN_POINT('Ctrl Pts',(-18.5731685999717,-13.2772201354542,
124.666246335996)) ;
#50842=CARTESIAN_POINT('Ctrl Pts',(-18.9238269690954,-13.4671548371495,
124.515725679001)) ;
#50843=CARTESIAN_POINT('Ctrl Pts',(-18.8024527486131,-13.287165756669,124.791696662309)) ;
#50844=CARTESIAN_POINT('Ctrl Pts',(-19.1218420695638,-13.4771040854178,
124.583140773883)) ;
#50845=CARTESIAN_POINT('Ctrl Pts',(-19.0499707908993,-13.2971150049373,
124.875968223362)) ;
#50846=CARTESIAN_POINT('Ctrl Pts',(-19.3305917291493,-13.4871505805864,
124.615215322897)) ;
#50847=CARTESIAN_POINT('Ctrl Pts',(-19.3109074952256,-13.3071615001059,
124.916064204666)) ;
#50848=CARTESIAN_POINT('Ctrl Pts',(-19.5376622730773,-13.4970019233779,
124.610852955936)) ;
#50849=CARTESIAN_POINT('Ctrl Pts',(-19.5697458477462,-13.3170128428975,
124.910614060324)) ;
#50850=CARTESIAN_POINT('Ctrl Pts',(-19.7433819757979,-13.5069737035053,
124.570637442649)) ;
#50851=CARTESIAN_POINT('Ctrl Pts',(-19.826896127891,-13.3269846230248,124.860347401869)) ;
#50852=CARTESIAN_POINT('Ctrl Pts',(-19.9394995576033,-13.516968903483,124.495094530682)) ;
#50853=CARTESIAN_POINT('Ctrl Pts',(-20.0720441859589,-13.3369798230025,
124.765921346822)) ;
#50854=CARTESIAN_POINT('Ctrl Pts',(-20.1200428835865,-13.527002895179,124.386031569206)) ;
#50855=CARTESIAN_POINT('Ctrl Pts',(-20.2977248333267,-13.3470138146985,
124.629595035507)) ;
#50856=CARTESIAN_POINT('Ctrl Pts',(-20.2763242405218,-13.5368583001515,
124.249969630593)) ;
#50857=CARTESIAN_POINT('Ctrl Pts',(-20.493078540568,-13.356869219671,124.459519571261)) ;
#50858=CARTESIAN_POINT('Ctrl Pts',(-20.4086965221813,-13.5468575979973,
124.086710547082)) ;
#50859=CARTESIAN_POINT('Ctrl Pts',(-20.6585461153618,-13.3668685175168,
124.255447402453)) ;
#50860=CARTESIAN_POINT('Ctrl Pts',(-20.5098783796781,-13.5567527106025,
123.904908826794)) ;
#50861=CARTESIAN_POINT('Ctrl Pts',(-20.7850259765466,-13.376763630122,124.028196369772)) ;
#50862=CARTESIAN_POINT('Ctrl Pts',(-20.5790528982995,-13.5668133561375,
123.705062953625)) ;
#50863=CARTESIAN_POINT('Ctrl Pts',(-20.8714967334466,-13.386824275657,123.778389961167)) ;
#50864=CARTESIAN_POINT('Ctrl Pts',(-20.6118978850877,-13.5766622331267,
123.500614031643)) ;
#50865=CARTESIAN_POINT('Ctrl Pts',(-20.9125557496579,-13.3966731526462,
123.522828864956)) ;
#50866=CARTESIAN_POINT('Ctrl Pts',(-20.6092193159514,-13.5866909442203,
123.289798847138)) ;
#50867=CARTESIAN_POINT('Ctrl Pts',(-20.9092102413502,-13.4067018637398,
123.259309807944)) ;
#50868=CARTESIAN_POINT('Ctrl Pts',(-20.5694097322058,-13.5967203454764,
123.082737299415)) ;
#50869=CARTESIAN_POINT('Ctrl Pts',(-20.8594509752274,-13.4167312649959,
123.000482346226)) ;
#50870=CARTESIAN_POINT('Ctrl Pts',(-20.4961008853216,-13.6065605372724,
122.889286624956)) ;
#50871=CARTESIAN_POINT('Ctrl Pts',(-20.7678172837384,-13.4265714567919,
122.758667592089)) ;
#50872=CARTESIAN_POINT('Ctrl Pts',(-20.3889086577013,-13.6165639664654,
122.708376154055)) ;
#50873=CARTESIAN_POINT('Ctrl Pts',(-20.6338292438647,-13.4365748859849,
122.532528062918)) ;
#50874=CARTESIAN_POINT('Ctrl Pts',(-20.2520895253684,-13.6265494789316,
122.549112630056)) ;
#50875=CARTESIAN_POINT('Ctrl Pts',(-20.4628072719018,-13.4465603984511,
122.333446821007)) ;
#50876=CARTESIAN_POINT('Ctrl Pts',(-20.0887000777735,-13.6365905753156,
122.415484766701)) ;
#50877=CARTESIAN_POINT('Ctrl Pts',(-20.258572195346,-13.4566014948351,122.166409914417)) ;
#50878=CARTESIAN_POINT('Ctrl Pts',(-19.9083265613386,-13.6464337712666,
122.314020661915)) ;
#50879=CARTESIAN_POINT('Ctrl Pts',(-20.0331061121941,-13.4664446907861,
122.03957718777)) ;
#50880=CARTESIAN_POINT('Ctrl Pts',(-19.7104267761794,-13.656420082321,122.244041727144)) ;
#50881=CARTESIAN_POINT('Ctrl Pts',(-19.7857320971964,-13.4764310018405,
121.952101012254)) ;
#50882=CARTESIAN_POINT('Ctrl Pts',(-19.5044018483537,-13.6663547675787,
122.209514866081)) ;
#50883=CARTESIAN_POINT('Ctrl Pts',(-19.5282010412024,-13.4863656870982,
121.90893984682)) ;
#50884=CARTESIAN_POINT('Ctrl Pts',(-19.2929999960134,-13.6764123287957,
122.211492627575)) ;
#50885=CARTESIAN_POINT('Ctrl Pts',(-19.2639488168424,-13.4964232483152,
121.91140943863)) ;
#50886=CARTESIAN_POINT('Ctrl Pts',(-19.0899192604328,-13.6862339704043,
122.248938878938)) ;
#50887=CARTESIAN_POINT('Ctrl Pts',(-19.0100966675006,-13.5062448899238,
121.958214887959)) ;
#50888=CARTESIAN_POINT('Ctrl Pts',(-18.8917066678072,-13.6962900339953,
122.32241535315)) ;
#50889=CARTESIAN_POINT('Ctrl Pts',(-18.7623301681439,-13.5163009535148,
122.050058119778)) ;
#50890=CARTESIAN_POINT('Ctrl Pts',(-18.711524790799,-13.7062307097571,122.428304767284)) ;
#50891=CARTESIAN_POINT('Ctrl Pts',(-18.5371012424823,-13.5262416292766,
122.182417857127)) ;
#50892=CARTESIAN_POINT('Ctrl Pts',(-18.5526279674509,-13.7161350685454,
122.562874462865)) ;
#50893=CARTESIAN_POINT('Ctrl Pts',(-18.338478245471,-13.5361459880649,122.350628473773)) ;
#50894=CARTESIAN_POINT('Ctrl Pts',(-18.4177132106572,-13.7261817231212,
122.725360080974)) ;
#50895=CARTESIAN_POINT('Ctrl Pts',(-18.1698329824766,-13.5461926426408,
122.553733855453)) ;
#50896=CARTESIAN_POINT('Ctrl Pts',(-18.3144502475993,-13.7360773177641,
122.905994660676)) ;
#50897=CARTESIAN_POINT('Ctrl Pts',(-18.0407519034869,-13.5560882372836,
122.779526388093)) ;
#50898=CARTESIAN_POINT('Ctrl Pts',(-18.2429366007976,-13.7461392644209,
123.105048153552)) ;
#50899=CARTESIAN_POINT('Ctrl Pts',(-17.9513576419596,-13.5661501839405,
123.028342279805)) ;
#50900=CARTESIAN_POINT('Ctrl Pts',(-18.2077846553653,-13.7559888883531,
123.309123594396)) ;
#50901=CARTESIAN_POINT('Ctrl Pts',(-17.9074152111613,-13.5759998078726,
123.283436990154)) ;
#50902=CARTESIAN_POINT('Ctrl Pts',(-18.2079178316408,-13.7659521273829,
123.518569880535)) ;
#50903=CARTESIAN_POINT('Ctrl Pts',(-17.9075794488089,-13.5859630469025,
123.545245160135)) ;
#50904=CARTESIAN_POINT('Ctrl Pts',(-18.2449311630796,-13.7759767021588,
123.726054826624)) ;
#50905=CARTESIAN_POINT('Ctrl Pts',(-17.9538438450152,-13.5959876216783,
123.804601716905)) ;
#50906=CARTESIAN_POINT('Ctrl Pts',(-18.3165097926261,-13.7858952648465,
123.921897886242)) ;
#50907=CARTESIAN_POINT('Ctrl Pts',(-18.0433151852417,-13.605906184366,124.049406829383)) ;
#50908=CARTESIAN_POINT('Ctrl Pts',(-18.4214705157971,-13.7958874515705,
124.103877790771)) ;
#50909=CARTESIAN_POINT('Ctrl Pts',(-18.1745142881597,-13.61589837109,124.276882942917)) ;
#50910=CARTESIAN_POINT('Ctrl Pts',(-18.5572880042135,-13.8059222501547,
124.265295046581)) ;
#50911=CARTESIAN_POINT('Ctrl Pts',(-18.3442843562415,-13.6259331696742,
124.478655912856)) ;
#50912=CARTESIAN_POINT('Ctrl Pts',(-18.7159640539968,-13.8157774408283,
124.398542881549)) ;
#50913=CARTESIAN_POINT('Ctrl Pts',(-18.5426287177336,-13.6357883603479,
124.645217964171)) ;
#50914=CARTESIAN_POINT('Ctrl Pts',(-18.8978051688274,-13.8257767889813,
124.503949795873)) ;
#50915=CARTESIAN_POINT('Ctrl Pts',(-18.7699291705139,-13.6457877085009,
124.776978498032)) ;
#50916=CARTESIAN_POINT('Ctrl Pts',(-19.0931163675303,-13.8356719146565,
124.575663890585)) ;
#50917=CARTESIAN_POINT('Ctrl Pts',(-19.0140681533063,-13.655682834176,124.86662328365)) ;
#50918=CARTESIAN_POINT('Ctrl Pts',(-19.3012793398308,-13.8457324576046,
124.612957137398)) ;
#50919=CARTESIAN_POINT('Ctrl Pts',(-19.2742712713046,-13.6657433771241,
124.913241818178)) ;
#50920=CARTESIAN_POINT('Ctrl Pts',(-19.5083568286429,-13.8555817318715,
124.613644904383)) ;
#50921=CARTESIAN_POINT('Ctrl Pts',(-19.533119164813,-13.675592651391,124.914103545098)) ;
#50922=CARTESIAN_POINT('Ctrl Pts',(-19.7161637957389,-13.8656089564414,
124.578258675114)) ;
#50923=CARTESIAN_POINT('Ctrl Pts',(-19.7928781485442,-13.6856198759609,
124.869872597829)) ;
#50924=CARTESIAN_POINT('Ctrl Pts',(-19.9145234172926,-13.8756373556292,
124.506794850628)) ;
#50925=CARTESIAN_POINT('Ctrl Pts',(-20.0408282969519,-13.6956482751487,
124.780544744332)) ;
#50926=CARTESIAN_POINT('Ctrl Pts',(-20.0942981409798,-13.8854831060427,
124.404230045374)) ;
#50927=CARTESIAN_POINT('Ctrl Pts',(-20.2655486147779,-13.7054940255622,
124.652339842869)) ;
#50928=CARTESIAN_POINT('Ctrl Pts',(-20.2562410694359,-13.8954718964434,
124.27052516634)) ;
#50929=CARTESIAN_POINT('Ctrl Pts',(-20.4679785319862,-13.715482815963,124.485209945461)) ;
#50930=CARTESIAN_POINT('Ctrl Pts',(-20.3928548044161,-13.9055168248431,
124.109502618488)) ;
#50931=CARTESIAN_POINT('Ctrl Pts',(-20.6387470356566,-13.7255277443626,
124.283933112368)) ;
#50932=CARTESIAN_POINT('Ctrl Pts',(-20.4975212772136,-13.9153413096321,
123.931431530893)) ;
#50933=CARTESIAN_POINT('Ctrl Pts',(-20.7695822852688,-13.7353522291516,
124.061344007663)) ;
#50934=CARTESIAN_POINT('Ctrl Pts',(-20.5716663162285,-13.9253987071733,
123.733438159543)) ;
#50935=CARTESIAN_POINT('Ctrl Pts',(-20.8622650303472,-13.7454096266928,
123.813853115612)) ;
#50936=CARTESIAN_POINT('Ctrl Pts',(-20.6095387245746,-13.9353247987595,
123.528210702811)) ;
#50937=CARTESIAN_POINT('Ctrl Pts',(-20.9096073546648,-13.755335718279,123.557318498523)) ;
#50938=CARTESIAN_POINT('Ctrl Pts',(-20.6117482503137,-13.945279583904,123.318943735867)) ;
#50939=CARTESIAN_POINT('Ctrl Pts',(-20.9123708212694,-13.7652905034236,
123.295734355708)) ;
#50940=CARTESIAN_POINT('Ctrl Pts',(-20.5770731565774,-13.9553169535617,
123.110795951615)) ;
#50941=CARTESIAN_POINT('Ctrl Pts',(-20.8690285858304,-13.7753278730812,
123.035549479052)) ;
#50942=CARTESIAN_POINT('Ctrl Pts',(-20.5079730266207,-13.9652057636833,
122.914716225052)) ;
#50943=CARTESIAN_POINT('Ctrl Pts',(-20.7826546063666,-13.7852166832028,
122.790448432854)) ;
#50944=CARTESIAN_POINT('Ctrl Pts',(-20.4051720006662,-13.9751951227343,
122.731595284921)) ;
#50945=CARTESIAN_POINT('Ctrl Pts',(-20.6541544834532,-13.7952060422539,
122.561546360004)) ;
#50946=CARTESIAN_POINT('Ctrl Pts',(-20.2724273246368,-13.9851536701904,
122.569707167163)) ;
#50947=CARTESIAN_POINT('Ctrl Pts',(-20.4882245282922,-13.80516458971,122.35918492389)) ;
#50948=CARTESIAN_POINT('Ctrl Pts',(-20.1148509111908,-13.9950532467415,
122.433733040983)) ;
#50949=CARTESIAN_POINT('Ctrl Pts',(-20.2912542117038,-13.815064166261,122.189215690004)) ;
#50950=CARTESIAN_POINT('Ctrl Pts',(-19.9333707547642,-14.0051011585722,
122.32566998488)) ;
#50951=CARTESIAN_POINT('Ctrl Pts',(-20.0644048945837,-13.8251120780917,
122.054135819747)) ;
#50952=CARTESIAN_POINT('Ctrl Pts',(-19.738890370448,-14.0149965064327,122.251724804565)) ;
#50953=CARTESIAN_POINT('Ctrl Pts',(-19.8213040212828,-13.8350074259523,
121.961702812235)) ;
#50954=CARTESIAN_POINT('Ctrl Pts',(-19.5311506381738,-14.0250581829639,
122.211995828632)) ;
#50955=CARTESIAN_POINT('Ctrl Pts',(-19.5616299166127,-13.8450691024834,
121.912040392263)) ;
#50956=CARTESIAN_POINT('Ctrl Pts',(-19.3242027583877,-14.0349027007131,
122.208972747124)) ;
#50957=CARTESIAN_POINT('Ctrl Pts',(-19.3029437659801,-13.8549136202326,
121.908260248604)) ;
#50958=CARTESIAN_POINT('Ctrl Pts',(-19.1173623183453,-14.0448631444279,
122.241578718461)) ;
#50959=CARTESIAN_POINT('Ctrl Pts',(-19.0443926106295,-13.8648740639474,
121.949016797417)) ;
#50960=CARTESIAN_POINT('Ctrl Pts',(-18.917933653831,-14.0548999772461,122.310497086348)) ;
#50961=CARTESIAN_POINT('Ctrl Pts',(-18.7951065532493,-13.8749108967656,
122.035163624094)) ;
#50962=CARTESIAN_POINT('Ctrl Pts',(-18.7362181804366,-14.0647787739929,
122.41109597588)) ;
#50963=CARTESIAN_POINT('Ctrl Pts',(-18.5679607591708,-13.8847896935124,
122.160911880305)) ;
#50964=CARTESIAN_POINT('Ctrl Pts',(-18.5717693082948,-14.0748380901212,
122.544026993693)) ;
#50965=CARTESIAN_POINT('Ctrl Pts',(-18.3623992979497,-13.8948490096408,
122.327074678563)) ;
#50966=CARTESIAN_POINT('Ctrl Pts',(-18.4354824503582,-14.0847085368744,
122.700520863806)) ;
#50967=CARTESIAN_POINT('Ctrl Pts',(-18.1920392189904,-13.904719456394,122.522692233356)) ;
#50968=CARTESIAN_POINT('Ctrl Pts',(-18.3266320599271,-14.0947011751325,
122.880198948747)) ;
#50969=CARTESIAN_POINT('Ctrl Pts',(-18.0559754685677,-13.914712094652,122.747289602209)) ;
#50970=CARTESIAN_POINT('Ctrl Pts',(-18.2507605415013,-14.1047331906804,
123.076976227112)) ;
#50971=CARTESIAN_POINT('Ctrl Pts',(-17.9611352241743,-13.9247441101999,
122.993260746161)) ;
#50972=CARTESIAN_POINT('Ctrl Pts',(-18.2104322023642,-14.114599046987,123.280449832988)) ;
#50973=CARTESIAN_POINT('Ctrl Pts',(-17.9107237976247,-13.9346099665065,
123.247603809007)) ;
#50974=CARTESIAN_POINT('Ctrl Pts',(-18.2059368718994,-14.1246683364561,
123.492066961254)) ;
#50975=CARTESIAN_POINT('Ctrl Pts',(-17.9051038743598,-13.9446792559756,
123.512124786781)) ;
#50976=CARTESIAN_POINT('Ctrl Pts',(-18.2375102294898,-14.1345118940074,
123.696598560914)) ;
#50977=CARTESIAN_POINT('Ctrl Pts',(-17.9445700336421,-13.9545228135269,
123.767790797039)) ;
#50978=CARTESIAN_POINT('Ctrl Pts',(-18.3043848267997,-14.1444920207952,
123.895462028567)) ;
#50979=CARTESIAN_POINT('Ctrl Pts',(-18.0281629108298,-13.9645029403147,
124.016370584177)) ;
#50980=CARTESIAN_POINT('Ctrl Pts',(-18.4055151657071,-14.1545105693952,
124.080209802711)) ;
#50981=CARTESIAN_POINT('Ctrl Pts',(-18.1545752561932,-13.9745214889147,
124.247305606121)) ;
#50982=CARTESIAN_POINT('Ctrl Pts',(-18.5350837698109,-14.1643938699184,
124.242672415459)) ;
#50983=CARTESIAN_POINT('Ctrl Pts',(-18.3165363212011,-13.9844047894379,
124.450385028089)) ;
#50984=CARTESIAN_POINT('Ctrl Pts',(-18.6938257864244,-14.1744621569665,
124.382634186157)) ;
#50985=CARTESIAN_POINT('Ctrl Pts',(-18.5149631926093,-13.994473076486,124.625337357564)) ;
#50986=CARTESIAN_POINT('Ctrl Pts',(-18.8701172743958,-14.1842922799851,
124.490542166158)) ;
#50987=CARTESIAN_POINT('Ctrl Pts',(-18.735328647287,-14.0043031995047,124.760223493844)) ;
#50988=CARTESIAN_POINT('Ctrl Pts',(-19.0669291678649,-14.1943588639105,
124.568249490539)) ;
#50989=CARTESIAN_POINT('Ctrl Pts',(-18.9813430292244,-14.01436978343,124.857357794822)) ;
#50990=CARTESIAN_POINT('Ctrl Pts',(-19.2706943838824,-14.2042489769249,
124.609750952324)) ;
#50991=CARTESIAN_POINT('Ctrl Pts',(-19.236050504993,-14.0242598964445,124.909235187497)) ;
#50992=CARTESIAN_POINT('Ctrl Pts',(-19.4806689201278,-14.2142416656876,
124.615742309981)) ;
#50993=CARTESIAN_POINT('Ctrl Pts',(-19.4985188781258,-14.0342525852071,
124.916724579679)) ;
#50994=CARTESIAN_POINT('Ctrl Pts',(-19.6878386126546,-14.2242025540433,
124.585132160337)) ;
#50995=CARTESIAN_POINT('Ctrl Pts',(-19.7574815058879,-14.0442134735629,
124.878462065285)) ;
#50996=CARTESIAN_POINT('Ctrl Pts',(-19.8857808498602,-14.2341204989233,
124.519648220953)) ;
#50997=CARTESIAN_POINT('Ctrl Pts',(-20.0049101278269,-14.0541314184429,
124.796606975694)) ;
#50998=CARTESIAN_POINT('Ctrl Pts',(-20.0711543280967,-14.2441282520195,
124.42009338198)) ;
#50999=CARTESIAN_POINT('Ctrl Pts',(-20.2366270329595,-14.0641391715391,
124.672163407257)) ;
#51000=CARTESIAN_POINT('Ctrl Pts',(-20.2365214427845,-14.2541593459786,
124.289244206464)) ;
#51001=CARTESIAN_POINT('Ctrl Pts',(-20.4433359396728,-14.0741702654981,
124.50860215391)) ;
#51002=CARTESIAN_POINT('Ctrl Pts',(-20.3744629268658,-14.2640073140066,
124.134836918703)) ;
#51003=CARTESIAN_POINT('Ctrl Pts',(-20.615763730972,-14.0840182335261,124.315591986996)) ;
#51004=CARTESIAN_POINT('Ctrl Pts',(-20.4860083257482,-14.2740692701324,
123.95512196643)) ;
#51005=CARTESIAN_POINT('Ctrl Pts',(-20.7551952258906,-14.094080189652,124.090948557051)) ;
#51006=CARTESIAN_POINT('Ctrl Pts',(-20.5631955250995,-14.2839664817336,
123.761889219392)) ;
#51007=CARTESIAN_POINT('Ctrl Pts',(-20.8516795938104,-14.1039774012531,
123.849406694929)) ;
#51008=CARTESIAN_POINT('Ctrl Pts',(-20.6064757403202,-14.2938976483982,
123.557644080804)) ;
#51009=CARTESIAN_POINT('Ctrl Pts',(-20.9057797424506,-14.1139085679177,
123.594099508441)) ;
#51010=CARTESIAN_POINT('Ctrl Pts',(-20.6134856977865,-14.3039398326024,
123.346645043293)) ;
#51011=CARTESIAN_POINT('Ctrl Pts',(-20.9145419980729,-14.1239507521219,
123.330350913857)) ;
#51012=CARTESIAN_POINT('Ctrl Pts',(-20.5843602960543,-14.3138265008555,
123.140837465138)) ;
#51013=CARTESIAN_POINT('Ctrl Pts',(-20.8781348523199,-14.1338374203751,
123.073090399062)) ;
#51014=CARTESIAN_POINT('Ctrl Pts',(-20.5195898101172,-14.3238196128338,
122.940995926319)) ;
#51015=CARTESIAN_POINT('Ctrl Pts',(-20.7971713177884,-14.1438305323533,
122.823288399559)) ;
#51016=CARTESIAN_POINT('Ctrl Pts',(-20.4214970858592,-14.3337652904496,
122.756344163075)) ;
#51017=CARTESIAN_POINT('Ctrl Pts',(-20.6745548237651,-14.1537762099691,
122.592473334144)) ;
#51018=CARTESIAN_POINT('Ctrl Pts',(-20.2931422169085,-14.3437125934346,
122.591232662632)) ;
#51019=CARTESIAN_POINT('Ctrl Pts',(-20.5141104751308,-14.1637235129541,
122.386083823413)) ;
#51020=CARTESIAN_POINT('Ctrl Pts',(-20.1363573288779,-14.3537603171813,
122.449682535313)) ;
#51021=CARTESIAN_POINT('Ctrl Pts',(-20.3181292652433,-14.1737712367009,
122.20914664792)) ;
#51022=CARTESIAN_POINT('Ctrl Pts',(-19.9610119228354,-14.3636086909439,
122.339593196702)) ;
#51023=CARTESIAN_POINT('Ctrl Pts',(-20.0989460634751,-14.1836196104634,
122.071534647339)) ;
#51024=CARTESIAN_POINT('Ctrl Pts',(-19.7673215762674,-14.3735676633896,
122.260098624231)) ;
#51025=CARTESIAN_POINT('Ctrl Pts',(-19.8568324062144,-14.1935785829091,
121.972166958739)) ;
#51026=CARTESIAN_POINT('Ctrl Pts',(-19.5610549600458,-14.3836065252707,
122.215459746428)) ;
#51027=CARTESIAN_POINT('Ctrl Pts',(-19.5989991593869,-14.2036174447902,
121.916368996424)) ;
#51028=CARTESIAN_POINT('Ctrl Pts',(-19.3535221005735,-14.3934851294425,
122.207111470236)) ;
#51029=CARTESIAN_POINT('Ctrl Pts',(-19.3395819370179,-14.2134960489621,
121.905934350524)) ;
#51030=CARTESIAN_POINT('Ctrl Pts',(-19.1441263617507,-14.4035366706458,
122.235315239726)) ;
#51031=CARTESIAN_POINT('Ctrl Pts',(-19.0778376414323,-14.2235475901654,
121.941189793679)) ;
#51032=CARTESIAN_POINT('Ctrl Pts',(-18.9458547057129,-14.4134320686262,
122.298408849419)) ;
#51033=CARTESIAN_POINT('Ctrl Pts',(-18.8299973983688,-14.2334429881457,
122.02005786211)) ;
#51034=CARTESIAN_POINT('Ctrl Pts',(-18.7586516298394,-14.4234833011715,
122.396359934609)) ;
#51035=CARTESIAN_POINT('Ctrl Pts',(-18.5959941771249,-14.243494220691,122.142497342869)) ;
#51036=CARTESIAN_POINT('Ctrl Pts',(-18.5939939088903,-14.4333694917958,
122.523221653132)) ;
#51037=CARTESIAN_POINT('Ctrl Pts',(-18.3901717061082,-14.2533804113153,
122.301075810648)) ;
#51038=CARTESIAN_POINT('Ctrl Pts',(-18.4520997591911,-14.4433620311115,
122.678107054398)) ;
#51039=CARTESIAN_POINT('Ctrl Pts',(-18.2128046215638,-14.2633729506311,
122.494683384561)) ;
#51040=CARTESIAN_POINT('Ctrl Pts',(-18.3397922812975,-14.4533104770063,
122.854559106031)) ;
#51041=CARTESIAN_POINT('Ctrl Pts',(-18.0724208012427,-14.2733213965258,
122.715249428695)) ;
#51042=CARTESIAN_POINT('Ctrl Pts',(-18.2596593833855,-14.4632472795382,
123.047461897236)) ;
#51043=CARTESIAN_POINT('Ctrl Pts',(-17.9722554345249,-14.2832581990577,
122.956378922606)) ;
#51044=CARTESIAN_POINT('Ctrl Pts',(-18.2137581958001,-14.4732302869895,
123.252282638572)) ;
#51045=CARTESIAN_POINT('Ctrl Pts',(-17.9148800448479,-14.293241206509,123.212405357777)) ;
#51046=CARTESIAN_POINT('Ctrl Pts',(-18.2044493527583,-14.4832741284043,
123.463206431544)) ;
#51047=CARTESIAN_POINT('Ctrl Pts',(-17.9032450352358,-14.3032850479238,
123.476059954935)) ;
#51048=CARTESIAN_POINT('Ctrl Pts',(-18.2308383801991,-14.4931023270282,
123.668165335843)) ;
#51049=CARTESIAN_POINT('Ctrl Pts',(-17.9362327114259,-14.3131132465477,
123.73225986307)) ;
#51050=CARTESIAN_POINT('Ctrl Pts',(-18.2938523410951,-14.5031789204704,
123.870372485691)) ;
#51051=CARTESIAN_POINT('Ctrl Pts',(-18.0150012317243,-14.3231898399899,
123.985018013504)) ;
#51052=CARTESIAN_POINT('Ctrl Pts',(-18.3887993193818,-14.513030919812,124.0544990199)) ;
#51053=CARTESIAN_POINT('Ctrl Pts',(-18.1336866674195,-14.3330418393315,
124.215176688704)) ;
#51054=CARTESIAN_POINT('Ctrl Pts',(-18.516907971024,-14.5231045066358,124.223090197898)) ;
#51055=CARTESIAN_POINT('Ctrl Pts',(-18.2938233160263,-14.3431154261554,
124.425914521078)) ;
#51056=CARTESIAN_POINT('Ctrl Pts',(-18.6688091775145,-14.5329447317333,
124.363553032254)) ;
#51057=CARTESIAN_POINT('Ctrl Pts',(-18.4837016927803,-14.3529556512529,
124.601492972364)) ;
#51058=CARTESIAN_POINT('Ctrl Pts',(-18.8445804362272,-14.542910435762,124.477535027406)) ;
#51059=CARTESIAN_POINT('Ctrl Pts',(-18.7034169617488,-14.3629213552815,
124.743969337186)) ;
#51060=CARTESIAN_POINT('Ctrl Pts',(-19.0387987115393,-14.5529370690686,
124.559495745125)) ;
#51061=CARTESIAN_POINT('Ctrl Pts',(-18.9461903268235,-14.3729479885881,
124.846418837784)) ;
#51062=CARTESIAN_POINT('Ctrl Pts',(-19.2419467311579,-14.5628513647804,
124.606096057943)) ;
#51063=CARTESIAN_POINT('Ctrl Pts',(-19.2001264119576,-14.3828622842999,
124.904667897302)) ;
#51064=CARTESIAN_POINT('Ctrl Pts',(-19.4516521953088,-14.5728396534728,
124.61717510903)) ;
#51065=CARTESIAN_POINT('Ctrl Pts',(-19.4622585244037,-14.3928505729924,
124.918515058981)) ;
#51066=CARTESIAN_POINT('Ctrl Pts',(-19.6610834565671,-14.5828783866312,
124.591166378612)) ;
#51067=CARTESIAN_POINT('Ctrl Pts',(-19.7240472766413,-14.4028893061507,
124.886002641623)) ;
#51068=CARTESIAN_POINT('Ctrl Pts',(-19.858998903738,-14.5927217184587,124.530728055798)) ;
#51069=CARTESIAN_POINT('Ctrl Pts',(-19.9714422785436,-14.4127326379783,
124.810452800166)) ;
#51070=CARTESIAN_POINT('Ctrl Pts',(-20.0470907094626,-14.6027494443383,
124.43551748704)) ;
#51071=CARTESIAN_POINT('Ctrl Pts',(-20.2065561511846,-14.4227603638579,
124.691438006676)) ;
#51072=CARTESIAN_POINT('Ctrl Pts',(-20.215531250739,-14.6127817807269,124.308574127084)) ;
#51073=CARTESIAN_POINT('Ctrl Pts',(-20.4171057820378,-14.4327927002464,
124.532757562509)) ;
#51074=CARTESIAN_POINT('Ctrl Pts',(-20.3567549827595,-14.6226112810275,
124.157731091938)) ;
#51075=CARTESIAN_POINT('Ctrl Pts',(-20.5936350312441,-14.442622200547,124.344201635672)) ;
#51076=CARTESIAN_POINT('Ctrl Pts',(-20.4720182760222,-14.6326007849443,
123.982171250015)) ;
#51077=CARTESIAN_POINT('Ctrl Pts',(-20.737712608456,-14.4526117044638,124.124750610664)) ;
#51078=CARTESIAN_POINT('Ctrl Pts',(-20.5550029183584,-14.6426446254567,
123.788010434387)) ;
#51079=CARTESIAN_POINT('Ctrl Pts',(-20.8414417060553,-14.4626555449762,
123.882049023621)) ;
#51080=CARTESIAN_POINT('Ctrl Pts',(-20.6023692510491,-14.6524663312247,
123.587034176731)) ;
#51081=CARTESIAN_POINT('Ctrl Pts',(-20.9006480361569,-14.4724772507443,
123.630827043139)) ;
#51082=CARTESIAN_POINT('Ctrl Pts',(-20.614891393778,-14.6625013783571,123.376438673923)) ;
#51083=CARTESIAN_POINT('Ctrl Pts',(-20.9162986356404,-14.4825122978766,
123.367582647653)) ;
#51084=CARTESIAN_POINT('Ctrl Pts',(-20.5901024671484,-14.672526055794,123.167143676446)) ;
#51085=CARTESIAN_POINT('Ctrl Pts',(-20.8853105897408,-14.4925369753135,
123.105964149127)) ;
#51086=CARTESIAN_POINT('Ctrl Pts',(-20.5308125782497,-14.6823788706484,
122.968674050456)) ;
#51087=CARTESIAN_POINT('Ctrl Pts',(-20.8111959913455,-14.502389790168,122.857876731608)) ;
#51088=CARTESIAN_POINT('Ctrl Pts',(-20.4370276643577,-14.692366580256,122.780826892626)) ;
#51089=CARTESIAN_POINT('Ctrl Pts',(-20.6939628550224,-14.5123774997755,
122.623068574683)) ;
#51090=CARTESIAN_POINT('Ctrl Pts',(-20.3127672555841,-14.7022965902501,
122.613067626526)) ;
#51091=CARTESIAN_POINT('Ctrl Pts',(-20.5386353140637,-14.5223075097696,
122.413370344733)) ;
#51092=CARTESIAN_POINT('Ctrl Pts',(-20.1605796757999,-14.7122863454692,
122.468335495329)) ;
#51093=CARTESIAN_POINT('Ctrl Pts',(-20.3483991861106,-14.5322972649888,
122.232456679477)) ;
#51094=CARTESIAN_POINT('Ctrl Pts',(-19.9847778139171,-14.7223129541521,
122.352025348161)) ;
#51095=CARTESIAN_POINT('Ctrl Pts',(-20.1286457022629,-14.5423238736717,
122.08707080773)) ;
#51096=CARTESIAN_POINT('Ctrl Pts',(-19.7942886748206,-14.732196894174,122.269022419418)) ;
#51097=CARTESIAN_POINT('Ctrl Pts',(-19.8905327192874,-14.5522078136935,
121.983318872729)) ;
#51098=CARTESIAN_POINT('Ctrl Pts',(-19.5902331312652,-14.7421861217125,
122.219359207184)) ;
#51099=CARTESIAN_POINT('Ctrl Pts',(-19.6354625878385,-14.562197041232,121.92124208015)) ;
#51100=CARTESIAN_POINT('Ctrl Pts',(-19.3795093368715,-14.7522289922362,
122.206246194729)) ;
#51101=CARTESIAN_POINT('Ctrl Pts',(-19.3720577988247,-14.5722399117557,
121.904853032833)) ;
#51102=CARTESIAN_POINT('Ctrl Pts',(-19.1740714005142,-14.7620613789916,
122.229097308269)) ;
#51103=CARTESIAN_POINT('Ctrl Pts',(-19.1152596799946,-14.5820722985111,
121.933419317654)) ;
#51104=CARTESIAN_POINT('Ctrl Pts',(-18.9723061416938,-14.7720546721632,
122.287639558838)) ;
#51105=CARTESIAN_POINT('Ctrl Pts',(-18.8630536664399,-14.5920655916827,
122.006599511698)) ;
#51106=CARTESIAN_POINT('Ctrl Pts',(-18.7832226625352,-14.7820866778116,
122.381086795298)) ;
#51107=CARTESIAN_POINT('Ctrl Pts',(-18.6267003874203,-14.6020975973311,
122.123410637807)) ;
#51108=CARTESIAN_POINT('Ctrl Pts',(-18.6159274829548,-14.7919519337806,
122.503651125695)) ;
#51109=CARTESIAN_POINT('Ctrl Pts',(-18.4175822403367,-14.6119628533001,
122.276618419778)) ;
#51110=CARTESIAN_POINT('Ctrl Pts',(-18.4706094581403,-14.8019138136881,
122.654469653778)) ;
#51111=CARTESIAN_POINT('Ctrl Pts',(-18.2359363518528,-14.6219247332076,
122.465143513875)) ;
#51112=CARTESIAN_POINT('Ctrl Pts',(-18.3531243947538,-14.81194874705,122.829681165894)) ;
#51113=CARTESIAN_POINT('Ctrl Pts',(-18.0890820794357,-14.6319596665695,
122.684159240986)) ;
#51114=CARTESIAN_POINT('Ctrl Pts',(-18.2687841779479,-14.8218337054293,
123.019642132794)) ;
#51115=CARTESIAN_POINT('Ctrl Pts',(-17.983658882904,-14.6418446249488,122.921611991584)) ;
#51116=CARTESIAN_POINT('Ctrl Pts',(-18.2178545293784,-14.8318993323519,
123.224997323136)) ;
#51117=CARTESIAN_POINT('Ctrl Pts',(-17.9199993002954,-14.6519102518714,
123.178306439045)) ;
#51118=CARTESIAN_POINT('Ctrl Pts',(-18.2034666313483,-14.8417384380163,
123.431379104992)) ;
#51119=CARTESIAN_POINT('Ctrl Pts',(-17.9020169236197,-14.6617493575358,
123.436284553323)) ;
#51120=CARTESIAN_POINT('Ctrl Pts',(-18.2253374188485,-14.8518012530216,
123.641768968564)) ;
#51121=CARTESIAN_POINT('Ctrl Pts',(-17.9293579838891,-14.6718121725412,
123.699271479275)) ;
#51122=CARTESIAN_POINT('Ctrl Pts',(-18.2826422959049,-14.8616974590703,
123.841793280128)) ;
#51123=CARTESIAN_POINT('Ctrl Pts',(-18.0009916817392,-14.6817083785898,
123.949301618053)) ;
#51124=CARTESIAN_POINT('Ctrl Pts',(-18.3736753162085,-14.8716382820956,
124.029885460281)) ;
#51125=CARTESIAN_POINT('Ctrl Pts',(-18.1147854786849,-14.6916492016151,
124.184415931346)) ;
#51126=CARTESIAN_POINT('Ctrl Pts',(-18.4967554476146,-14.8816428650742,
124.200469969171)) ;
#51127=CARTESIAN_POINT('Ctrl Pts',(-18.2686378472388,-14.7016537845938,
124.39764506361)) ;
#51128=CARTESIAN_POINT('Ctrl Pts',(-18.6479893488011,-14.891663759519,124.347127592409)) ;
#51129=CARTESIAN_POINT('Ctrl Pts',(-18.4576820791071,-14.7116746790385,
124.580965224335)) ;
#51130=CARTESIAN_POINT('Ctrl Pts',(-18.8200089658471,-14.9015556801084,
124.463997418573)) ;
#51131=CARTESIAN_POINT('Ctrl Pts',(-18.6727084409181,-14.7215665996279,
124.727050531161)) ;
#51132=CARTESIAN_POINT('Ctrl Pts',(-19.0115199934511,-14.9115491124538,
124.550366690489)) ;
#51133=CARTESIAN_POINT('Ctrl Pts',(-18.9120984380812,-14.7315600319733,
124.835009694432)) ;
#51134=CARTESIAN_POINT('Ctrl Pts',(-19.2141671143431,-14.9214947173536,
124.601860043974)) ;
#51135=CARTESIAN_POINT('Ctrl Pts',(-19.1654082296755,-14.7415056368732,
124.899373825416)) ;
#51136=CARTESIAN_POINT('Ctrl Pts',(-19.422692143887,-14.9314419908352,124.617812488144)) ;
#51137=CARTESIAN_POINT('Ctrl Pts',(-19.4260649276648,-14.7514529103547,
124.919311654215)) ;
#51138=CARTESIAN_POINT('Ctrl Pts',(-19.6328836255055,-14.9414899053115,
124.596874131456)) ;
#51139=CARTESIAN_POINT('Ctrl Pts',(-19.6888039980711,-14.7615008248311,
124.89313599866)) ;
#51140=CARTESIAN_POINT('Ctrl Pts',(-19.8322491561593,-14.9513375456589,
124.541062785767)) ;
#51141=CARTESIAN_POINT('Ctrl Pts',(-19.9380105597996,-14.7713484651784,
124.823369065598)) ;
#51142=CARTESIAN_POINT('Ctrl Pts',(-20.0213303949895,-14.9612992610355,
124.451042034006)) ;
#51143=CARTESIAN_POINT('Ctrl Pts',(-20.1743610166879,-14.781310180555,124.710840541292)) ;
#51144=CARTESIAN_POINT('Ctrl Pts',(-20.1929184638276,-14.9713278846083,
124.328511186806)) ;
#51145=CARTESIAN_POINT('Ctrl Pts',(-20.3888445240509,-14.7913388041278,
124.557674698041)) ;
#51146=CARTESIAN_POINT('Ctrl Pts',(-20.3389145430226,-14.9812382466747,
124.179885799862)) ;
#51147=CARTESIAN_POINT('Ctrl Pts',(-20.571337784828,-14.8012491661942,124.371890859746)) ;
#51148=CARTESIAN_POINT('Ctrl Pts',(-20.4576406506801,-14.9911729403271,
124.008044457199)) ;
#51149=CARTESIAN_POINT('Ctrl Pts',(-20.7197431783026,-14.8111838598466,
124.157087470562)) ;
#51150=CARTESIAN_POINT('Ctrl Pts',(-20.5454669216902,-15.001214783455,123.816080842499)) ;
#51151=CARTESIAN_POINT('Ctrl Pts',(-20.8295234846959,-14.8212257029745,
123.917131743908)) ;
#51152=CARTESIAN_POINT('Ctrl Pts',(-20.5979816592684,-15.0110992890254,
123.615000802519)) ;
#51153=CARTESIAN_POINT('Ctrl Pts',(-20.8951642261479,-14.8311102085449,
123.66578082451)) ;
#51154=CARTESIAN_POINT('Ctrl Pts',(-20.6152250273524,-15.0211013928106,
123.405463995573)) ;
#51155=CARTESIAN_POINT('Ctrl Pts',(-20.9167156316037,-14.8411123123301,
123.403859517349)) ;
#51156=CARTESIAN_POINT('Ctrl Pts',(-20.5961521969141,-15.0310197442256,
123.197788238171)) ;
#51157=CARTESIAN_POINT('Ctrl Pts',(-20.8928717592807,-14.8510306637451,
123.144264974563)) ;
#51158=CARTESIAN_POINT('Ctrl Pts',(-20.5405596861251,-15.0410674002465,
122.994035665252)) ;
#51159=CARTESIAN_POINT('Ctrl Pts',(-20.8233784418533,-14.861078319766,122.889574983687)) ;
#51160=CARTESIAN_POINT('Ctrl Pts',(-20.4521948522776,-15.0509385932747,
122.806217337189)) ;
#51161=CARTESIAN_POINT('Ctrl Pts',(-20.7129195793855,-14.8709495127942,
122.654803032881)) ;
#51162=CARTESIAN_POINT('Ctrl Pts',(-20.330284242075,-15.0610043064182,122.633308943981)) ;
#51163=CARTESIAN_POINT('Ctrl Pts',(-20.5605298605741,-14.8810152259377,
122.438669790485)) ;
#51164=CARTESIAN_POINT('Ctrl Pts',(-20.1834794070481,-15.0708567669908,
122.487109307967)) ;
#51165=CARTESIAN_POINT('Ctrl Pts',(-20.3770184512462,-14.8908676865104,
122.255919658866)) ;
#51166=CARTESIAN_POINT('Ctrl Pts',(-19.9518872310143,-15.0842852297134,
122.325790591143)) ;
#51167=CARTESIAN_POINT('Ctrl Pts',(-20.0875427688117,-14.9042961492329,
122.054287113997)) ;
#51168=CARTESIAN_POINT('Ctrl Pts',(-19.6903665057396,-15.0973661772305,
122.230682396376)) ;
#51169=CARTESIAN_POINT('Ctrl Pts',(-19.7606733442006,-14.91737709675,121.935403530336)) ;
#51170=CARTESIAN_POINT('Ctrl Pts',(-19.4082962992305,-15.110840675465,122.205756665579)) ;
#51171=CARTESIAN_POINT('Ctrl Pts',(-19.4080294143567,-14.9308515949846,
121.904239537887)) ;
#51172=CARTESIAN_POINT('Ctrl Pts',(-19.2023473006596,-15.1206727790745,
122.223870629062)) ;
#51173=CARTESIAN_POINT('Ctrl Pts',(-19.1506048229786,-14.940683698594,121.926886772447)) ;
#51174=CARTESIAN_POINT('Ctrl Pts',(-18.9998068488561,-15.1306386822012,
122.277363273524)) ;
#51175=CARTESIAN_POINT('Ctrl Pts',(-18.8974267386482,-14.9506496017207,
121.993755117813)) ;
#51176=CARTESIAN_POINT('Ctrl Pts',(-18.8085430621808,-15.1406660915114,
122.366073015869)) ;
#51177=CARTESIAN_POINT('Ctrl Pts',(-18.6583498544115,-14.9606770110309,
122.104643278196)) ;
#51178=CARTESIAN_POINT('Ctrl Pts',(-18.6376088448104,-15.150577122878,122.48516450023)) ;
#51179=CARTESIAN_POINT('Ctrl Pts',(-18.4446798400263,-14.9705880423975,
122.253516252839)) ;
#51180=CARTESIAN_POINT('Ctrl Pts',(-18.4395743724625,-15.163821430499,122.681015377369)) ;
#51181=CARTESIAN_POINT('Ctrl Pts',(-18.1971580266742,-14.9838323500186,
122.498300087625)) ;
#51182=CARTESIAN_POINT('Ctrl Pts',(-18.2607335132502,-15.1805219131702,
122.987645959784)) ;
#51183=CARTESIAN_POINT('Ctrl Pts',(-17.9735883958197,-15.0005328326897,
122.881645823186)) ;
#51184=CARTESIAN_POINT('Ctrl Pts',(-18.1977869763505,-15.197028742326,123.333061812602)) ;
#51185=CARTESIAN_POINT('Ctrl Pts',(-17.8949212633086,-15.0170396618455,
123.3133312933)) ;
#51186=CARTESIAN_POINT('Ctrl Pts',(-18.2199642495241,-15.2103393705636,
123.611928517238)) ;
#51187=CARTESIAN_POINT('Ctrl Pts',(-17.9226408361223,-15.0303502900831,
123.661981974287)) ;
#51188=CARTESIAN_POINT('Ctrl Pts',(-18.2726848636332,-15.2203319341037,
123.815325721179)) ;
#51189=CARTESIAN_POINT('Ctrl Pts',(-17.9885443790157,-15.0403428536232,
123.916213406542)) ;
#51190=CARTESIAN_POINT('Ctrl Pts',(-18.3604503080189,-15.2303620171052,
124.007021668416)) ;
#51191=CARTESIAN_POINT('Ctrl Pts',(-18.0982567043705,-15.0503729366247,
124.155839488653)) ;
#51192=CARTESIAN_POINT('Ctrl Pts',(-18.5172815670806,-15.243535621103,124.235376320227)) ;
#51193=CARTESIAN_POINT('Ctrl Pts',(-18.2942816286453,-15.0635465406225,
124.441261778011)) ;
#51194=CARTESIAN_POINT('Ctrl Pts',(-18.785763220475,-15.2601733263344,124.465502936072)) ;
#51195=CARTESIAN_POINT('Ctrl Pts',(-18.629900480376,-15.0801842458539,124.728937538322)) ;
#51196=CARTESIAN_POINT('Ctrl Pts',(-19.1813810887829,-15.2800550889018,
124.614910728195)) ;
#51197=CARTESIAN_POINT('Ctrl Pts',(-19.1244402676743,-15.1000660084213,
124.91568323805)) ;
#51198=CARTESIAN_POINT('Ctrl Pts',(-19.536304822624,-15.2967514411183,124.619219755491)) ;
#51199=CARTESIAN_POINT('Ctrl Pts',(-19.5680268437064,-15.1167623606378,
124.921075711026)) ;
#51200=CARTESIAN_POINT('Ctrl Pts',(-19.8044165799873,-15.3099084689074,
124.551173766666)) ;
#51201=CARTESIAN_POINT('Ctrl Pts',(-19.9032277012803,-15.1299193884269,
124.836006277141)) ;
#51202=CARTESIAN_POINT('Ctrl Pts',(-20.0610790101127,-15.3232858235509,
124.436222758126)) ;
#51203=CARTESIAN_POINT('Ctrl Pts',(-20.2240299228811,-15.1432967430705,
124.692326184218)) ;
#51204=CARTESIAN_POINT('Ctrl Pts',(-20.3337494420324,-15.3398166578097,
124.214377221525)) ;
#51205=CARTESIAN_POINT('Ctrl Pts',(-20.5648835409731,-15.1598275773293,
124.415004995592)) ;
#51206=CARTESIAN_POINT('Ctrl Pts',(-20.552438862062,-15.3597813475528,123.850580679781)) ;
#51207=CARTESIAN_POINT('Ctrl Pts',(-20.8382356612196,-15.1797922670724,
123.960261264847)) ;
#51208=CARTESIAN_POINT('Ctrl Pts',(-20.6332747084739,-15.3796978409765,
123.434880640488)) ;
#51209=CARTESIAN_POINT('Ctrl Pts',(-20.9392779041822,-15.199708760496,123.440635012871)) ;
#51210=CARTESIAN_POINT('Ctrl Pts',(-20.5683199143235,-15.399587560326,123.016946237213)) ;
#51211=CARTESIAN_POINT('Ctrl Pts',(-20.858080531106,-15.2195984798456,122.918218801379)) ;
#51212=CARTESIAN_POINT('Ctrl Pts',(-20.3631949850862,-15.4195942899739,
122.644342249502)) ;
#51213=CARTESIAN_POINT('Ctrl Pts',(-20.6016712397754,-15.2396052094934,
122.452465436855)) ;
#51214=CARTESIAN_POINT('Ctrl Pts',(-20.0460283351885,-15.4394323436208,
122.366126910109)) ;
#51215=CARTESIAN_POINT('Ctrl Pts',(-20.2052118911002,-15.2594432631403,
122.104699831963)) ;
#51216=CARTESIAN_POINT('Ctrl Pts',(-19.6501954328286,-15.4594256818344,
122.211302972032)) ;
#51217=CARTESIAN_POINT('Ctrl Pts',(-19.7104197648899,-15.2794366013539,
121.911172705937)) ;
#51218=CARTESIAN_POINT('Ctrl Pts',(-19.22747548443,-15.479308481241,122.20116645109)) ;
#51219=CARTESIAN_POINT('Ctrl Pts',(-19.1820210308517,-15.2993194007605,
121.898505003943)) ;
#51220=CARTESIAN_POINT('Ctrl Pts',(-18.8264426794319,-15.4992006621597,
122.335208188009)) ;
#51221=CARTESIAN_POINT('Ctrl Pts',(-18.6807320924974,-15.3192115816792,
122.066058969295)) ;
#51222=CARTESIAN_POINT('Ctrl Pts',(-18.4944215574731,-15.5191028406548,
122.597782843408)) ;
#51223=CARTESIAN_POINT('Ctrl Pts',(-18.2657076845191,-15.3391137601743,
122.394277865511)) ;
#51224=CARTESIAN_POINT('Ctrl Pts',(-18.2711780684696,-15.5391401518585,
122.960525542868)) ;
#51225=CARTESIAN_POINT('Ctrl Pts',(-17.9866547279515,-15.359151071378,122.847707709297)) ;
#51226=CARTESIAN_POINT('Ctrl Pts',(-18.1854465994955,-15.5589525933994,
123.373166514348)) ;
#51227=CARTESIAN_POINT('Ctrl Pts',(-17.879492215553,-15.3789635129189,123.363506708318)) ;
#51228=CARTESIAN_POINT('Ctrl Pts',(-18.2465194115136,-15.5790178341343,
123.795207249882)) ;
#51229=CARTESIAN_POINT('Ctrl Pts',(-17.9558345968631,-15.3990287536538,
123.891058298206)) ;
#51230=CARTESIAN_POINT('Ctrl Pts',(-18.4447532133238,-15.5987750389901,
124.16581727744)) ;
#51231=CARTESIAN_POINT('Ctrl Pts',(-18.2036257716139,-15.4187859585096,
124.354317293493)) ;
#51232=CARTESIAN_POINT('Ctrl Pts',(-18.7611937431446,-15.6188083116358,
124.450642539288)) ;
#51233=CARTESIAN_POINT('Ctrl Pts',(-18.5991767272437,-15.4388192311553,
124.710349085209)) ;
#51234=CARTESIAN_POINT('Ctrl Pts',(-19.1518899017671,-15.6386212200896,
124.608729629548)) ;
#51235=CARTESIAN_POINT('Ctrl Pts',(-19.0875441523598,-15.4586321396092,
124.907957059647)) ;
#51236=CARTESIAN_POINT('Ctrl Pts',(-19.5765723952849,-15.6586173662171,
124.624694592537)) ;
#51237=CARTESIAN_POINT('Ctrl Pts',(-19.6183970906581,-15.4786282857366,
124.927914166643)) ;
#51238=CARTESIAN_POINT('Ctrl Pts',(-19.9789149548444,-15.6784791194396,
124.495740343834)) ;
#51239=CARTESIAN_POINT('Ctrl Pts',(-20.1213238856596,-15.4984900389591,
124.766723103384)) ;
#51240=CARTESIAN_POINT('Ctrl Pts',(-20.3161903072829,-15.6985476365677,
124.234500907358)) ;
#51241=CARTESIAN_POINT('Ctrl Pts',(-20.5429196527663,-15.5185585560872,
124.440174246545)) ;
#51242=CARTESIAN_POINT('Ctrl Pts',(-20.5412403283249,-15.7183785095645,
123.877812094549)) ;
#51243=CARTESIAN_POINT('Ctrl Pts',(-20.8242320697883,-15.538389429084,123.994315885988)) ;
#51244=CARTESIAN_POINT('Ctrl Pts',(-20.6325525181329,-15.7383004203812,
123.464277815718)) ;
#51245=CARTESIAN_POINT('Ctrl Pts',(-20.938374323766,-15.5583113399007,123.477399544052)) ;
#51246=CARTESIAN_POINT('Ctrl Pts',(-20.5770999387733,-15.7582298638165,
123.044097906908)) ;
#51247=CARTESIAN_POINT('Ctrl Pts',(-20.8690610709312,-15.578240783336,122.952175131957)) ;
#51248=CARTESIAN_POINT('Ctrl Pts',(-20.3819841700265,-15.7781395339329,
122.668482285981)) ;
#51249=CARTESIAN_POINT('Ctrl Pts',(-20.6251692264673,-15.5981504534524,
122.482655310818)) ;
#51250=CARTESIAN_POINT('Ctrl Pts',(-20.071398669403,-15.7980128911957,122.381885903197)) ;
#51251=CARTESIAN_POINT('Ctrl Pts',(-20.2369405025118,-15.6180238107153,
122.124408326918)) ;
#51252=CARTESIAN_POINT('Ctrl Pts',(-19.6794075493568,-15.8180044258137,
122.217622884656)) ;
#51253=CARTESIAN_POINT('Ctrl Pts',(-19.7469529682798,-15.6380153453332,
121.919076471675)) ;
#51254=CARTESIAN_POINT('Ctrl Pts',(-19.2574526738448,-15.8378700432244,
122.196935178988)) ;
#51255=CARTESIAN_POINT('Ctrl Pts',(-19.2195107524635,-15.6578809627439,
121.893213319118)) ;
#51256=CARTESIAN_POINT('Ctrl Pts',(-18.8513755370978,-15.8578509730526,
122.321775663419)) ;
#51257=CARTESIAN_POINT('Ctrl Pts',(-18.7119132759403,-15.6778618925722,
122.049260143465)) ;
#51258=CARTESIAN_POINT('Ctrl Pts',(-18.5132612033128,-15.8777894351358,
122.577542069427)) ;
#51259=CARTESIAN_POINT('Ctrl Pts',(-18.289268421837,-15.6978003546553,122.368964780119)) ;
#51260=CARTESIAN_POINT('Ctrl Pts',(-18.2826819587382,-15.8976816283575,
122.932185153396)) ;
#51261=CARTESIAN_POINT('Ctrl Pts',(-18.0010412601392,-15.717692547877,122.812265657322)) ;
#51262=CARTESIAN_POINT('Ctrl Pts',(-18.1868169762122,-15.9176523433929,
123.34575803658)) ;
#51263=CARTESIAN_POINT('Ctrl Pts',(-17.8812058281196,-15.7376632629124,
123.329230583623)) ;
#51264=CARTESIAN_POINT('Ctrl Pts',(-18.2367313458389,-15.937462015059,123.764098817235)) ;
#51265=CARTESIAN_POINT('Ctrl Pts',(-17.9435942350171,-15.7574729345785,
123.852155946831)) ;
#51266=CARTESIAN_POINT('Ctrl Pts',(-18.4277666040295,-15.9574552317502,
124.143691492752)) ;
#51267=CARTESIAN_POINT('Ctrl Pts',(-18.1823832686069,-15.7774661512697,
124.326648974628)) ;
#51268=CARTESIAN_POINT('Ctrl Pts',(-18.7346680099378,-15.9773061439465,
124.433713845188)) ;
#51269=CARTESIAN_POINT('Ctrl Pts',(-18.5660086877581,-15.797317063466,124.689180060819)) ;
#51270=CARTESIAN_POINT('Ctrl Pts',(-19.1263185071962,-15.9973807502655,
124.603150136167)) ;
#51271=CARTESIAN_POINT('Ctrl Pts',(-19.0555605459573,-15.8173916697851,
124.900980308438)) ;
#51272=CARTESIAN_POINT('Ctrl Pts',(-19.4769940370043,-16.0138973821489,
124.624006616587)) ;
#51273=CARTESIAN_POINT('Ctrl Pts',(-19.493934124644,-15.8339083016684,124.927054797122)) ;
#51274=CARTESIAN_POINT('Ctrl Pts',(-19.7517414985942,-16.027236089843,124.568093364996)) ;
#51275=CARTESIAN_POINT('Ctrl Pts',(-19.8373421473109,-15.8472470093625,
124.857167360089)) ;
#51276=CARTESIAN_POINT('Ctrl Pts',(-19.9444057679308,-16.0370784641513,
124.492551498524)) ;
#51277=CARTESIAN_POINT('Ctrl Pts',(-20.0781804979996,-15.8570893836708,
124.762739876029)) ;
#51278=CARTESIAN_POINT('Ctrl Pts',(-20.1249049321985,-16.047133484134,124.382567620846)) ;
#51279=CARTESIAN_POINT('Ctrl Pts',(-20.3037960539398,-15.8671444036535,
124.625272793391)) ;
#51280=CARTESIAN_POINT('Ctrl Pts',(-20.3337092884455,-16.0603656407916,
124.198785774196)) ;
#51281=CARTESIAN_POINT('Ctrl Pts',(-20.5648469002763,-15.8803765603111,
124.395495442231)) ;
#51282=CARTESIAN_POINT('Ctrl Pts',(-20.5299755382867,-16.0769806081367,
123.904990129354)) ;
#51283=CARTESIAN_POINT('Ctrl Pts',(-20.8101326081078,-15.8969915276562,
124.02832371337)) ;
#51284=CARTESIAN_POINT('Ctrl Pts',(-20.6139164154991,-16.0935751951479,
123.562338411869)) ;
#51285=CARTESIAN_POINT('Ctrl Pts',(-20.9150857053266,-15.9135861146674,
123.599951810543)) ;
#51286=CARTESIAN_POINT('Ctrl Pts',(-20.6085033819079,-16.1068087635033,
123.284128846805)) ;
#51287=CARTESIAN_POINT('Ctrl Pts',(-20.9083137995466,-15.9268196830228,
123.252228775175)) ;
#51288=CARTESIAN_POINT('Ctrl Pts',(-20.5678420997152,-16.1168523813119,
123.076956614971)) ;
#51289=CARTESIAN_POINT('Ctrl Pts',(-20.8574915955287,-15.9368633008315,
122.993254896118)) ;
#51290=CARTESIAN_POINT('Ctrl Pts',(-20.4930658285917,-16.1267393055468,
122.882997750619)) ;
#51291=CARTESIAN_POINT('Ctrl Pts',(-20.7640240612381,-15.9467502250663,
122.750807958824)) ;
#51292=CARTESIAN_POINT('Ctrl Pts',(-20.3849611897659,-16.1367299599936,
122.702938885806)) ;
#51293=CARTESIAN_POINT('Ctrl Pts',(-20.6288932483085,-15.9567408795131,
122.525730668272)) ;
#51294=CARTESIAN_POINT('Ctrl Pts',(-20.2475814117215,-16.1466917184475,
122.544854107054)) ;
#51295=CARTESIAN_POINT('Ctrl Pts',(-20.4571800170958,-15.9667026379671,
122.328129169663)) ;
#51296=CARTESIAN_POINT('Ctrl Pts',(-20.0298504240982,-16.1600315835148,
122.368082548189)) ;
#51297=CARTESIAN_POINT('Ctrl Pts',(-20.1849716449942,-15.9800425030343,
122.107130949227)) ;
#51298=CARTESIAN_POINT('Ctrl Pts',(-19.7713257253914,-16.1733403664281,
122.253045017901)) ;
#51299=CARTESIAN_POINT('Ctrl Pts',(-19.8618390549998,-15.9933512859476,
121.963354375823)) ;
#51300=CARTESIAN_POINT('Ctrl Pts',(-19.4973854044494,-16.1865361238721,
122.209149372698)) ;
#51301=CARTESIAN_POINT('Ctrl Pts',(-19.519435246012,-16.0065470433916,121.908483591754)) ;
#51302=CARTESIAN_POINT('Ctrl Pts',(-19.2879723974171,-16.1964980075486,
122.211840246962)) ;
#51303=CARTESIAN_POINT('Ctrl Pts',(-19.257664641132,-16.0165089270682,121.911843867943)) ;
#51304=CARTESIAN_POINT('Ctrl Pts',(-19.0805966754575,-16.2065411170633,
122.251508529244)) ;
#51305=CARTESIAN_POINT('Ctrl Pts',(-18.9984455353408,-16.0265520365828,
121.961426597221)) ;
#51306=CARTESIAN_POINT('Ctrl Pts',(-18.8869132560321,-16.2163933670625,
122.324927691343)) ;
#51307=CARTESIAN_POINT('Ctrl Pts',(-18.756339852645,-16.036404286582,122.053197919674)) ;
#51308=CARTESIAN_POINT('Ctrl Pts',(-18.7065271330224,-16.226364904013,122.431685493257)) ;
#51309=CARTESIAN_POINT('Ctrl Pts',(-18.5308557512395,-16.0463758235325,
122.186642824369)) ;
#51310=CARTESIAN_POINT('Ctrl Pts',(-18.5470082080786,-16.2363601694905,
122.56851706965)) ;
#51311=CARTESIAN_POINT('Ctrl Pts',(-18.3314551895401,-16.05637108901,122.357680218266)) ;
#51312=CARTESIAN_POINT('Ctrl Pts',(-18.413387011108,-16.2463941423641,122.731722217809)) ;
#51313=CARTESIAN_POINT('Ctrl Pts',(-18.1644264950383,-16.0664050618836,
122.561684900237)) ;
#51314=CARTESIAN_POINT('Ctrl Pts',(-18.3116651483155,-16.2562495571265,
122.91224766768)) ;
#51315=CARTESIAN_POINT('Ctrl Pts',(-18.0372716141847,-16.076260476646,122.787340539563)) ;
#51316=CARTESIAN_POINT('Ctrl Pts',(-18.2415770596379,-16.2662488346353,
123.110397616458)) ;
#51317=CARTESIAN_POINT('Ctrl Pts',(-17.9496588450067,-16.0862597541548,
123.035027131205)) ;
#51318=CARTESIAN_POINT('Ctrl Pts',(-18.2070866766184,-16.2761440187983,
123.315582482187)) ;
#51319=CARTESIAN_POINT('Ctrl Pts',(-17.9065430992982,-16.0961549383178,
123.291508010325)) ;
#51320=CARTESIAN_POINT('Ctrl Pts',(-18.2087980539472,-16.2862043984391,
123.527047846686)) ;
#51321=CARTESIAN_POINT('Ctrl Pts',(-17.9086795501049,-16.1062153179586,
123.555839709405)) ;
#51322=CARTESIAN_POINT('Ctrl Pts',(-18.2462808343881,-16.2960542674472,
123.730723195858)) ;
#51323=CARTESIAN_POINT('Ctrl Pts',(-17.9555303864305,-16.1160651869667,
123.810434776904)) ;
#51324=CARTESIAN_POINT('Ctrl Pts',(-18.3194286022039,-16.3060858286551,
123.928512270352)) ;
#51325=CARTESIAN_POINT('Ctrl Pts',(-18.0469625661562,-16.1260967481746,
124.057672087781)) ;
#51326=CARTESIAN_POINT('Ctrl Pts',(-18.425966779491,-16.3160962775374,124.110026603965)) ;
#51327=CARTESIAN_POINT('Ctrl Pts',(-18.1801329407007,-16.1361071970569,
124.284566442548)) ;
#51328=CARTESIAN_POINT('Ctrl Pts',(-18.560797825782,-16.3260030169544,124.268754201217)) ;
#51329=CARTESIAN_POINT('Ctrl Pts',(-18.3486698657087,-16.1460139364739,
124.482977937669)) ;
#51330=CARTESIAN_POINT('Ctrl Pts',(-18.7213836715412,-16.3359410330228,
124.402388892912)) ;
#51331=CARTESIAN_POINT('Ctrl Pts',(-18.549400664377,-16.1559519525423,124.650023534822)) ;
#51332=CARTESIAN_POINT('Ctrl Pts',(-18.9039216281586,-16.3459462794739,
124.506949932254)) ;
#51333=CARTESIAN_POINT('Ctrl Pts',(-18.7775718600517,-16.1659571989935,
124.780727182853)) ;
#51334=CARTESIAN_POINT('Ctrl Pts',(-19.1025026858816,-16.3559803405302,
124.578083634945)) ;
#51335=CARTESIAN_POINT('Ctrl Pts',(-19.025797253829,-16.1759912600497,124.869646857172)) ;
#51336=CARTESIAN_POINT('Ctrl Pts',(-19.3064644872942,-16.3658254215884,
124.613343041828)) ;
#51337=CARTESIAN_POINT('Ctrl Pts',(-19.2807496064473,-16.1858363411079,
124.913723831407)) ;
#51338=CARTESIAN_POINT('Ctrl Pts',(-19.5163642119704,-16.3758112275419,
124.61303502221)) ;
#51339=CARTESIAN_POINT('Ctrl Pts',(-19.5431244270231,-16.1958221470614,
124.91334140973)) ;
#51340=CARTESIAN_POINT('Ctrl Pts',(-19.7220636700193,-16.3857460480961,
124.576608850265)) ;
#51341=CARTESIAN_POINT('Ctrl Pts',(-19.8002495182627,-16.2057569676156,
124.86781116913)) ;
#51342=CARTESIAN_POINT('Ctrl Pts',(-19.9206078791978,-16.3958035732283,
124.503981755754)) ;
#51343=CARTESIAN_POINT('Ctrl Pts',(-20.0484305676392,-16.2158144927478,
124.777029791005)) ;
#51344=CARTESIAN_POINT('Ctrl Pts',(-20.0994392626122,-16.4056252238796,
124.400718208666)) ;
#51345=CARTESIAN_POINT('Ctrl Pts',(-20.2719717474174,-16.2256361433992,
124.647952173923)) ;
#51346=CARTESIAN_POINT('Ctrl Pts',(-20.2616227730663,-16.4156812873844,
124.265132165577)) ;
#51347=CARTESIAN_POINT('Ctrl Pts',(-20.4747026405701,-16.2356922069039,
124.478471590854)) ;
#51348=CARTESIAN_POINT('Ctrl Pts',(-20.3959657201901,-16.4256219544483,
124.105038813883)) ;
#51349=CARTESIAN_POINT('Ctrl Pts',(-20.6426334924399,-16.2456328739678,
124.278356285914)) ;
#51350=CARTESIAN_POINT('Ctrl Pts',(-20.5006527032414,-16.4355263481143,
123.925043149726)) ;
#51351=CARTESIAN_POINT('Ctrl Pts',(-20.7734945783761,-16.2555372676338,
124.053362462571)) ;
#51352=CARTESIAN_POINT('Ctrl Pts',(-20.5733913233739,-16.4455728718773,
123.726774248668)) ;
#51353=CARTESIAN_POINT('Ctrl Pts',(-20.8644201158758,-16.2655837913968,
123.805527276541)) ;
#51354=CARTESIAN_POINT('Ctrl Pts',(-20.6102491313444,-16.4554689548937,
123.521980484657)) ;
#51355=CARTESIAN_POINT('Ctrl Pts',(-20.9104948423804,-16.2754798744132,
123.549534920319)) ;
#51356=CARTESIAN_POINT('Ctrl Pts',(-20.6109490500216,-16.4655356541237,
123.310385747446)) ;
#51357=CARTESIAN_POINT('Ctrl Pts',(-20.9113721564966,-16.2855465736432,
123.28504171042)) ;
#51358=CARTESIAN_POINT('Ctrl Pts',(-20.5759933517223,-16.4753592645248,
123.106810422099)) ;
#51359=CARTESIAN_POINT('Ctrl Pts',(-20.8676796984875,-16.2953701840443,
123.030571216628)) ;
#51360=CARTESIAN_POINT('Ctrl Pts',(-20.504941661928,-16.4854151247023,122.907730675288)) ;
#51361=CARTESIAN_POINT('Ctrl Pts',(-20.7788672824088,-16.3054260442218,
122.781720920148)) ;
#51362=CARTESIAN_POINT('Ctrl Pts',(-20.4014184334642,-16.4953482710072,
122.726342025547)) ;
#51363=CARTESIAN_POINT('Ctrl Pts',(-20.6494650622992,-16.3153591905267,
122.554983567569)) ;
#51364=CARTESIAN_POINT('Ctrl Pts',(-20.2681709832991,-16.5052935267778,
122.565253208005)) ;
#51365=CARTESIAN_POINT('Ctrl Pts',(-20.4829072058743,-16.3253044462973,
122.353620794786)) ;
#51366=CARTESIAN_POINT('Ctrl Pts',(-20.1084390136851,-16.5152768252163,
122.429067661281)) ;
#51367=CARTESIAN_POINT('Ctrl Pts',(-20.2832435138796,-16.3352877447358,
122.183387066426)) ;
#51368=CARTESIAN_POINT('Ctrl Pts',(-19.9264011878482,-16.5253140053629,
122.322380814143)) ;
#51369=CARTESIAN_POINT('Ctrl Pts',(-20.0556974558092,-16.3453249248824,
122.050026596241)) ;
#51370=CARTESIAN_POINT('Ctrl Pts',(-19.7322826676452,-16.5351685580724,
122.24994521566)) ;
#51371=CARTESIAN_POINT('Ctrl Pts',(-19.8130492091403,-16.3551794775919,
121.959479734029)) ;
#51372=CARTESIAN_POINT('Ctrl Pts',(-19.5256465946988,-16.5451680765197,
122.211483731313)) ;
#51373=CARTESIAN_POINT('Ctrl Pts',(-19.5547543717607,-16.3651789960392,
121.911400782408)) ;
#51374=CARTESIAN_POINT('Ctrl Pts',(-19.3175976842918,-16.5550631589818,
122.209284349518)) ;
#51375=CARTESIAN_POINT('Ctrl Pts',(-19.2946925229252,-16.3750740785013,
121.908649507568)) ;
#51376=CARTESIAN_POINT('Ctrl Pts',(-19.1089595995031,-16.5651237044879,
122.243820775951)) ;
#51377=CARTESIAN_POINT('Ctrl Pts',(-19.0338948184378,-16.3851346240074,
121.951817978714)) ;
#51378=CARTESIAN_POINT('Ctrl Pts',(-18.9135973762475,-16.5749730117359,
122.312488918254)) ;
#51379=CARTESIAN_POINT('Ctrl Pts',(-18.7896903908939,-16.3949839312554,
122.037651600256)) ;
#51380=CARTESIAN_POINT('Ctrl Pts',(-18.7296234980827,-16.5850001018232,
122.415390660692)) ;
#51381=CARTESIAN_POINT('Ctrl Pts',(-18.5597221684491,-16.4050110213428,
122.166277137721)) ;
#51382=CARTESIAN_POINT('Ctrl Pts',(-18.5666258182799,-16.5950290059602,
122.549139612565)) ;
#51383=CARTESIAN_POINT('Ctrl Pts',(-18.3559738382257,-16.4150399254797,
122.333461717316)) ;
#51384=CARTESIAN_POINT('Ctrl Pts',(-18.4315607292266,-16.6048728710595,
122.705925530433)) ;
#51385=CARTESIAN_POINT('Ctrl Pts',(-18.1871403033564,-16.424883790579,122.529443722396)) ;
#51386=CARTESIAN_POINT('Ctrl Pts',(-18.3236876247588,-16.6148686977679,
122.886268946656)) ;
#51387=CARTESIAN_POINT('Ctrl Pts',(-18.0522973394285,-16.4348796172874,
122.754872248822)) ;
#51388=CARTESIAN_POINT('Ctrl Pts',(-18.2489074259559,-16.6248939144169,
123.083322704059)) ;
#51389=CARTESIAN_POINT('Ctrl Pts',(-17.9588203684048,-16.4449048339364,
123.001188739164)) ;
#51390=CARTESIAN_POINT('Ctrl Pts',(-18.2097358480084,-16.6347837465745,
123.287518104386)) ;
#51391=CARTESIAN_POINT('Ctrl Pts',(-17.9098539907051,-16.454794666094,123.256433493442)) ;
#51392=CARTESIAN_POINT('Ctrl Pts',(-18.2062951743029,-16.6447746026592,
123.497522176624)) ;
#51393=CARTESIAN_POINT('Ctrl Pts',(-17.905551463918,-16.4647855221787,123.518938743189)) ;
#51394=CARTESIAN_POINT('Ctrl Pts',(-18.2392588330395,-16.6547196972521,
123.70398395006)) ;
#51395=CARTESIAN_POINT('Ctrl Pts',(-17.946754439527,-16.4747306167716,123.777016725502)) ;
#51396=CARTESIAN_POINT('Ctrl Pts',(-18.3072491133093,-16.6646716010202,
123.901857207325)) ;
#51397=CARTESIAN_POINT('Ctrl Pts',(-18.0317409620989,-16.4846825205397,
124.0243592607)) ;
#51398=CARTESIAN_POINT('Ctrl Pts',(-18.4095792800101,-16.6747080004896,
124.086372613872)) ;
#51399=CARTESIAN_POINT('Ctrl Pts',(-18.1596521830573,-16.4947189200091,
124.255004194096)) ;
#51400=CARTESIAN_POINT('Ctrl Pts',(-18.5403323023959,-16.6845970705783,
124.24801603038)) ;
#51401=CARTESIAN_POINT('Ctrl Pts',(-18.323092810584,-16.5046079900978,124.457060171017)) ;
#51402=CARTESIAN_POINT('Ctrl Pts',(-18.6984981846878,-16.6945863599492,
124.386161267394)) ;
#51403=CARTESIAN_POINT('Ctrl Pts',(-18.5207993713785,-16.5145972794687,
124.629742950679)) ;
#51404=CARTESIAN_POINT('Ctrl Pts',(-18.8777747357484,-16.7045449261589,
124.494277089496)) ;
#51405=CARTESIAN_POINT('Ctrl Pts',(-18.7448946530804,-16.5245558456784,
124.764889240913)) ;
#51406=CARTESIAN_POINT('Ctrl Pts',(-19.071775886629,-16.7144444973757,124.569661405429)) ;
#51407=CARTESIAN_POINT('Ctrl Pts',(-18.9873964306121,-16.5344554168952,
124.859121188033)) ;
#51408=CARTESIAN_POINT('Ctrl Pts',(-19.2789592287976,-16.7244924117899,
124.6107434715)) ;
#51409=CARTESIAN_POINT('Ctrl Pts',(-19.2463751320816,-16.5445033313095,
124.910475054248)) ;
#51410=CARTESIAN_POINT('Ctrl Pts',(-19.4869725711741,-16.7343877546505,
124.615324364318)) ;
#51411=CARTESIAN_POINT('Ctrl Pts',(-19.5063926931803,-16.55439867417,124.916202482364)) ;
#51412=CARTESIAN_POINT('Ctrl Pts',(-19.6960268210127,-16.7444494485979,
124.583223874358)) ;
#51413=CARTESIAN_POINT('Ctrl Pts',(-19.7677103787035,-16.5644603681175,
124.876078188876)) ;
#51414=CARTESIAN_POINT('Ctrl Pts',(-19.8920494172545,-16.7542939016821,
124.51680250823)) ;
#51415=CARTESIAN_POINT('Ctrl Pts',(-20.01274028279,-16.5743048212016,124.793052261306)) ;
#51416=CARTESIAN_POINT('Ctrl Pts',(-20.0760402865908,-16.7642545866405,
124.416833948505)) ;
#51417=CARTESIAN_POINT('Ctrl Pts',(-20.2427297442584,-16.5842655061601,
124.668092227986)) ;
#51418=CARTESIAN_POINT('Ctrl Pts',(-20.2409080973794,-16.7742905191491,
124.285163854322)) ;
#51419=CARTESIAN_POINT('Ctrl Pts',(-20.4488151081097,-16.5943014386686,
124.50350557831)) ;
#51420=CARTESIAN_POINT('Ctrl Pts',(-20.3785099430271,-16.7841791348371,
124.129336922064)) ;
#51421=CARTESIAN_POINT('Ctrl Pts',(-20.620818876143,-16.6041900543566,124.308721851052)) ;
#51422=CARTESIAN_POINT('Ctrl Pts',(-20.4887120097041,-16.7941935439796,
123.949931511366)) ;
#51423=CARTESIAN_POINT('Ctrl Pts',(-20.7585722336861,-16.6142044634991,
124.08446554872)) ;
#51424=CARTESIAN_POINT('Ctrl Pts',(-20.5657191627696,-16.8042273529374,
123.753561423584)) ;
#51425=CARTESIAN_POINT('Ctrl Pts',(-20.8548321534226,-16.6242382724569,
123.839003471693)) ;
#51426=CARTESIAN_POINT('Ctrl Pts',(-20.6071867597122,-16.8140578071936,
123.551072730248)) ;
#51427=CARTESIAN_POINT('Ctrl Pts',(-20.906667816104,-16.6340687267131,123.585891332069)) ;
#51428=CARTESIAN_POINT('Ctrl Pts',(-20.6130753200358,-16.8241354747718,
123.339330931498)) ;
#51429=CARTESIAN_POINT('Ctrl Pts',(-20.9140293674957,-16.6441463942913,
123.321214560571)) ;
#51430=CARTESIAN_POINT('Ctrl Pts',(-20.582897122482,-16.833987342894,123.134379068764)) ;
#51431=CARTESIAN_POINT('Ctrl Pts',(-20.8763072382661,-16.6539982624135,
123.06502331283)) ;
#51432=CARTESIAN_POINT('Ctrl Pts',(-20.5163171737132,-16.8440603804594,
122.933388787276)) ;
#51433=CARTESIAN_POINT('Ctrl Pts',(-20.7930831563984,-16.6640712999789,
122.813785637992)) ;
#51434=CARTESIAN_POINT('Ctrl Pts',(-20.4180968317784,-16.8539029338102,
122.751244860052)) ;
#51435=CARTESIAN_POINT('Ctrl Pts',(-20.6703077318771,-16.6739138533298,
122.58610411904)) ;
#51436=CARTESIAN_POINT('Ctrl Pts',(-20.2885154375274,-16.8638833293037,
122.586232749684)) ;
#51437=CARTESIAN_POINT('Ctrl Pts',(-20.5083311852049,-16.6838942488232,
122.379838432665)) ;
#51438=CARTESIAN_POINT('Ctrl Pts',(-20.1313776052616,-16.8739018072815,
122.445995465439)) ;
#51439=CARTESIAN_POINT('Ctrl Pts',(-20.3119093380775,-16.693912726801,122.204541346618)) ;
#51440=CARTESIAN_POINT('Ctrl Pts',(-19.9549021525347,-16.8837851215876,
122.336275047287)) ;
#51441=CARTESIAN_POINT('Ctrl Pts',(-20.0913143431546,-16.7037960411071,
122.067389838445)) ;
#51442=CARTESIAN_POINT('Ctrl Pts',(-19.7584673745493,-16.8938534241263,
122.257523549518)) ;
#51443=CARTESIAN_POINT('Ctrl Pts',(-19.8457714437735,-16.7138643436458,
121.968950139383)) ;
#51444=CARTESIAN_POINT('Ctrl Pts',(-19.5562266361521,-16.9036834713997,
122.214849851963)) ;
#51445=CARTESIAN_POINT('Ctrl Pts',(-19.5929691002895,-16.7236943909192,
121.915607289787)) ;
#51446=CARTESIAN_POINT('Ctrl Pts',(-19.3447520721929,-16.9137503428152,
122.207507802747)) ;
#51447=CARTESIAN_POINT('Ctrl Pts',(-19.3286263043278,-16.7337612623347,
121.906429428128)) ;
#51448=CARTESIAN_POINT('Ctrl Pts',(-19.1388680110044,-16.9236393816143,
122.236594479174)) ;
#51449=CARTESIAN_POINT('Ctrl Pts',(-19.0712701351057,-16.7436503011338,
121.942787563432)) ;
#51450=CARTESIAN_POINT('Ctrl Pts',(-18.9389316545158,-16.9336360797484,
122.301281101622)) ;
#51451=CARTESIAN_POINT('Ctrl Pts',(-18.8213494437003,-16.7536469992679,
122.023645715545)) ;
#51452=CARTESIAN_POINT('Ctrl Pts',(-18.7540959744669,-16.9435885054603,
122.39935968639)) ;
#51453=CARTESIAN_POINT('Ctrl Pts',(-18.5903042631905,-16.7635994249799,
122.146243992507)) ;
#51454=CARTESIAN_POINT('Ctrl Pts',(-18.5891273339633,-16.9535298076933,
122.527650967993)) ;
#51455=CARTESIAN_POINT('Ctrl Pts',(-18.3840928902973,-16.7735407272128,
122.306608387276)) ;
#51456=CARTESIAN_POINT('Ctrl Pts',(-18.4481547796409,-16.9635130467772,
122.683169969797)) ;
#51457=CARTESIAN_POINT('Ctrl Pts',(-18.2078769997332,-16.7835239662967,
122.501007316653)) ;
#51458=CARTESIAN_POINT('Ctrl Pts',(-18.3360050079193,-16.9735518483458,
122.861931794176)) ;
#51459=CARTESIAN_POINT('Ctrl Pts',(-18.067689740393,-16.7935627678653,122.724459360808)) ;
#51460=CARTESIAN_POINT('Ctrl Pts',(-18.2577181334253,-16.9833999544674,
123.053617948428)) ;
#51461=CARTESIAN_POINT('Ctrl Pts',(-17.9698306081202,-16.803410873987,122.964068373344)) ;
#51462=CARTESIAN_POINT('Ctrl Pts',(-18.2127741605597,-16.9934601500428,
123.260266613058)) ;
#51463=CARTESIAN_POINT('Ctrl Pts',(-17.9136507969245,-16.8134710695623,
123.2223788709)) ;
#51464=CARTESIAN_POINT('Ctrl Pts',(-18.2047179854304,-17.0033578333542,
123.468199338141)) ;
#51465=CARTESIAN_POINT('Ctrl Pts',(-17.9035805404894,-16.8233687528737,
123.48229577624)) ;
#51466=CARTESIAN_POINT('Ctrl Pts',(-18.232302562789,-17.0132888737282,123.675146887286)) ;
#51467=CARTESIAN_POINT('Ctrl Pts',(-17.9380616313287,-16.8332997932477,
123.740980891387)) ;
#51468=CARTESIAN_POINT('Ctrl Pts',(-18.2963248753717,-17.0233310913848,
123.876321281435)) ;
#51469=CARTESIAN_POINT('Ctrl Pts',(-18.0180896344632,-16.8433420109043,
123.992448629491)) ;
#51470=CARTESIAN_POINT('Ctrl Pts',(-18.3926605695863,-17.0332177521188,
124.06050712681)) ;
#51471=CARTESIAN_POINT('Ctrl Pts',(-18.1385099719493,-16.8532286716383,
124.222681786436)) ;
#51472=CARTESIAN_POINT('Ctrl Pts',(-18.5205878645769,-17.0432108607212,
124.227139826993)) ;
#51473=CARTESIAN_POINT('Ctrl Pts',(-18.2984195186076,-16.8632217802408,
124.43097259029)) ;
#51474=CARTESIAN_POINT('Ctrl Pts',(-18.674831224359,-17.0531565593595,124.368304779055)) ;
#51475=CARTESIAN_POINT('Ctrl Pts',(-18.4912243939608,-16.873167478879,124.607428923853)) ;
#51476=CARTESIAN_POINT('Ctrl Pts',(-18.8510481817693,-17.0631037816305,
124.480927513138)) ;
#51477=CARTESIAN_POINT('Ctrl Pts',(-18.7114963547142,-16.8831147011501,
124.74820721351)) ;
#51478=CARTESIAN_POINT('Ctrl Pts',(-19.0461761282001,-17.0731518072107,
124.561829669415)) ;
#51479=CARTESIAN_POINT('Ctrl Pts',(-18.9554062189033,-16.8931627267302,
124.849334420093)) ;
#51480=CARTESIAN_POINT('Ctrl Pts',(-19.2482340808857,-17.0829990543536,
124.606880354677)) ;
#51481=CARTESIAN_POINT('Ctrl Pts',(-19.2079801341209,-16.9030099738731,
124.905647600131)) ;
#51482=CARTESIAN_POINT('Ctrl Pts',(-19.4574454956206,-17.0929622314443,
124.616933495659)) ;
#51483=CARTESIAN_POINT('Ctrl Pts',(-19.4694948938914,-16.9129731509638,
124.918213293197)) ;
#51484=CARTESIAN_POINT('Ctrl Pts',(-19.6665745901204,-17.1029919524777,
124.590015336654)) ;
#51485=CARTESIAN_POINT('Ctrl Pts',(-19.7309060814968,-16.9230028719973,
124.88456498197)) ;
#51486=CARTESIAN_POINT('Ctrl Pts',(-19.8654350785867,-17.1128964200106,
124.528216237133)) ;
#51487=CARTESIAN_POINT('Ctrl Pts',(-19.979482337591,-16.9329073395301,124.807315147101)) ;
#51488=CARTESIAN_POINT('Ctrl Pts',(-20.0527821290814,-17.1229209058404,
124.431754757046)) ;
#51489=CARTESIAN_POINT('Ctrl Pts',(-20.2136657522635,-16.9429318253599,
124.686737651533)) ;
#51490=CARTESIAN_POINT('Ctrl Pts',(-20.2186621175981,-17.1328247409643,
124.305869214479)) ;
#51491=CARTESIAN_POINT('Ctrl Pts',(-20.4210159640352,-16.9528356604838,
124.529379524933)) ;
#51492=CARTESIAN_POINT('Ctrl Pts',(-20.362268269371,-17.1428759316743,124.150890987089)) ;
#51493=CARTESIAN_POINT('Ctrl Pts',(-20.60052287167,-16.9628868511938,124.335656355053)) ;
#51494=CARTESIAN_POINT('Ctrl Pts',(-20.4749404633162,-17.1527603743326,
123.976262382427)) ;
#51495=CARTESIAN_POINT('Ctrl Pts',(-20.7413629700132,-16.9727712938521,
124.117369250374)) ;
#51496=CARTESIAN_POINT('Ctrl Pts',(-20.5568101272468,-17.1627533821844,
123.782806970068)) ;
#51497=CARTESIAN_POINT('Ctrl Pts',(-20.8436992078529,-16.982764301704,123.875549411277)) ;
#51498=CARTESIAN_POINT('Ctrl Pts',(-20.6035732599445,-17.1727017019007,
123.578943176126)) ;
#51499=CARTESIAN_POINT('Ctrl Pts',(-20.9021522989073,-16.9927126214203,
123.620718922307)) ;
#51500=CARTESIAN_POINT('Ctrl Pts',(-20.6145132332225,-17.1826385406102,
123.370344649638)) ;
#51501=CARTESIAN_POINT('Ctrl Pts',(-20.9158262171433,-17.0026494601297,
123.35997007018)) ;
#51502=CARTESIAN_POINT('Ctrl Pts',(-20.589206594443,-17.1926215295298,123.16197490794)) ;
#51503=CARTESIAN_POINT('Ctrl Pts',(-20.8841917167147,-17.0126324490493,
123.099507780355)) ;
#51504=CARTESIAN_POINT('Ctrl Pts',(-20.5273748243571,-17.2026654088939,
122.960102497268)) ;
#51505=CARTESIAN_POINT('Ctrl Pts',(-20.8069010686547,-17.0226763284134,
122.847167752317)) ;
#51506=CARTESIAN_POINT('Ctrl Pts',(-20.4339045567548,-17.2124934742523,
122.775800529378)) ;
#51507=CARTESIAN_POINT('Ctrl Pts',(-20.6900614938181,-17.0325043937718,
122.616789554191)) ;
#51508=CARTESIAN_POINT('Ctrl Pts',(-20.3068302236449,-17.2225705628072,
122.606349678098)) ;
#51509=CARTESIAN_POINT('Ctrl Pts',(-20.5312178371621,-17.0425814823267,
122.404977089916)) ;
#51510=CARTESIAN_POINT('Ctrl Pts',(-20.1557656867094,-17.2324207149635,
122.464630719431)) ;
#51511=CARTESIAN_POINT('Ctrl Pts',(-20.3423853677775,-17.052431634483,122.227828485067)) ;
#51512=CARTESIAN_POINT('Ctrl Pts',(-19.9784714409174,-17.2425011954158,
122.348631483285)) ;
#51513=CARTESIAN_POINT('Ctrl Pts',(-20.1207672097145,-17.0625121149354,
122.082830799731)) ;
#51514=CARTESIAN_POINT('Ctrl Pts',(-19.7888488448021,-17.2523156931847,
122.267175683269)) ;
#51515=CARTESIAN_POINT('Ctrl Pts',(-19.883737034809,-17.0723266127042,121.98101173803)) ;
#51516=CARTESIAN_POINT('Ctrl Pts',(-19.582938898268,-17.2623839892048,122.218356656156)) ;
#51517=CARTESIAN_POINT('Ctrl Pts',(-19.6263495978875,-17.0823949087243,
121.919989507208)) ;
#51518=CARTESIAN_POINT('Ctrl Pts',(-19.3751318674818,-17.2722828216876,
122.206291542029)) ;
#51519=CARTESIAN_POINT('Ctrl Pts',(-19.3665898868727,-17.0922937412071,
121.904909547214)) ;
#51520=CARTESIAN_POINT('Ctrl Pts',(-19.1652559904925,-17.2823357017021,
122.230785552897)) ;
#51521=CARTESIAN_POINT('Ctrl Pts',(-19.1042454568957,-17.1023466212216,
121.93552853605)) ;
#51522=CARTESIAN_POINT('Ctrl Pts',(-18.9663707089697,-17.2922055171983,
122.29008319877)) ;
#51523=CARTESIAN_POINT('Ctrl Pts',(-18.8556383074436,-17.1122164367178,
122.009652399114)) ;
#51524=CARTESIAN_POINT('Ctrl Pts',(-18.7770326931717,-17.3022781982811,
122.384835344758)) ;
#51525=CARTESIAN_POINT('Ctrl Pts',(-18.6189668204918,-17.1222891178006,
122.128093849574)) ;
#51526=CARTESIAN_POINT('Ctrl Pts',(-18.6109839358936,-17.312110676852,122.507981598294)) ;
#51527=CARTESIAN_POINT('Ctrl Pts',(-18.4114058095582,-17.1321215963716,
122.28202873535)) ;
#51528=CARTESIAN_POINT('Ctrl Pts',(-18.4655538333765,-17.3221413108381,
122.660674634817)) ;
#51529=CARTESIAN_POINT('Ctrl Pts',(-18.2296195607227,-17.1421522303577,
122.472896223297)) ;
#51530=CARTESIAN_POINT('Ctrl Pts',(-18.349337760532,-17.3321728680573,122.83667359108)) ;
#51531=CARTESIAN_POINT('Ctrl Pts',(-18.0843508672524,-17.1521837875768,
122.692895741802)) ;
#51532=CARTESIAN_POINT('Ctrl Pts',(-18.2667484940145,-17.342002576929,123.026088129245)) ;
#51533=CARTESIAN_POINT('Ctrl Pts',(-17.9811153910442,-17.1620134964485,
122.929665784977)) ;
#51534=CARTESIAN_POINT('Ctrl Pts',(-18.2169009601804,-17.3519920257311,
123.230102550982)) ;
#51535=CARTESIAN_POINT('Ctrl Pts',(-17.9188078332525,-17.1720029452506,
123.184684449005)) ;
#51536=CARTESIAN_POINT('Ctrl Pts',(-18.20369487068,-17.3620358781311,123.440840534949)) ;
#51537=CARTESIAN_POINT('Ctrl Pts',(-17.9023020183694,-17.1820467976506,
123.448106892895)) ;
#51538=CARTESIAN_POINT('Ctrl Pts',(-18.2263343781215,-17.3718575914632,
123.646078297448)) ;
#51539=CARTESIAN_POINT('Ctrl Pts',(-17.9306034520585,-17.1918685109827,
123.70465512796)) ;
#51540=CARTESIAN_POINT('Ctrl Pts',(-18.2850268408009,-17.3818925964519,
123.848716320605)) ;
#51541=CARTESIAN_POINT('Ctrl Pts',(-18.0039709950905,-17.2019035159714,
123.957951977025)) ;
#51542=CARTESIAN_POINT('Ctrl Pts',(-18.3784463059481,-17.3919174348995,
124.037642069545)) ;
#51543=CARTESIAN_POINT('Ctrl Pts',(-18.1207470221514,-17.211928354419,124.194108297335)) ;
#51544=CARTESIAN_POINT('Ctrl Pts',(-18.5007395484921,-17.4017696478547,
124.204809326343)) ;
#51545=CARTESIAN_POINT('Ctrl Pts',(-18.2736158123272,-17.2217805673742,
124.40306698236)) ;
#51546=CARTESIAN_POINT('Ctrl Pts',(-18.6520320192726,-17.4117596040485,
124.350454005425)) ;
#51547=CARTESIAN_POINT('Ctrl Pts',(-18.4627330155444,-17.231770523568,124.58512141866)) ;
#51548=CARTESIAN_POINT('Ctrl Pts',(-18.8252452575916,-17.4216877143317,
124.466918774105)) ;
#51549=CARTESIAN_POINT('Ctrl Pts',(-18.6792511906033,-17.2416986338513,
124.730700896827)) ;
#51550=CARTESIAN_POINT('Ctrl Pts',(-19.0170751012007,-17.4316763144113,
124.552359737803)) ;
#51551=CARTESIAN_POINT('Ctrl Pts',(-18.9190395512915,-17.2516872339308,
124.837500136019)) ;
#51552=CARTESIAN_POINT('Ctrl Pts',(-19.2216700740144,-17.4417029063388,
124.603105177326)) ;
#51553=CARTESIAN_POINT('Ctrl Pts',(-19.1747837504834,-17.2617138258583,
124.90092984062)) ;
#51554=CARTESIAN_POINT('Ctrl Pts',(-19.4289770875473,-17.451588034403,124.617568828443)) ;
#51555=CARTESIAN_POINT('Ctrl Pts',(-19.4339184087877,-17.2715989539225,
124.91900725603)) ;
#51556=CARTESIAN_POINT('Ctrl Pts',(-19.6379253432582,-17.4615791518765,
124.596058505797)) ;
#51557=CARTESIAN_POINT('Ctrl Pts',(-19.6951036460035,-17.281590071396,124.89211702281)) ;
#51558=CARTESIAN_POINT('Ctrl Pts',(-19.8408352338707,-17.4716197677283,
124.537884142129)) ;
#51559=CARTESIAN_POINT('Ctrl Pts',(-19.948740310109,-17.2916306872478,124.819396963056)) ;
#51560=CARTESIAN_POINT('Ctrl Pts',(-20.0267858411353,-17.481452758582,124.447583261545)) ;
#51561=CARTESIAN_POINT('Ctrl Pts',(-20.1811784263094,-17.3014636781015,
124.706518373557)) ;
#51562=CARTESIAN_POINT('Ctrl Pts',(-20.1973125975978,-17.4914458900323,
124.324881213278)) ;
#51563=CARTESIAN_POINT('Ctrl Pts',(-20.3943355472786,-17.3114568095518,
124.55313875721)) ;
#51564=CARTESIAN_POINT('Ctrl Pts',(-20.3442096502401,-17.5014779384677,
124.173532276575)) ;
#51565=CARTESIAN_POINT('Ctrl Pts',(-20.5779551584514,-17.3214888579872,
124.363950983944)) ;
#51566=CARTESIAN_POINT('Ctrl Pts',(-20.460827682046,-17.5113431850101,124.002039230905)) ;
#51567=CARTESIAN_POINT('Ctrl Pts',(-20.7237261255781,-17.3313541045296,
124.1495827215)) ;
#51568=CARTESIAN_POINT('Ctrl Pts',(-20.5472792275311,-17.5213050598369,
123.811278450178)) ;
#51569=CARTESIAN_POINT('Ctrl Pts',(-20.8317883622719,-17.3413159793564,
123.911130472961)) ;
#51570=CARTESIAN_POINT('Ctrl Pts',(-20.5993376398069,-17.5313400229482,
123.606847846578)) ;
#51571=CARTESIAN_POINT('Ctrl Pts',(-20.8968589919692,-17.3513509424677,
123.655591647141)) ;
#51572=CARTESIAN_POINT('Ctrl Pts',(-20.615228249655,-17.5412248674106,123.399615410114)) ;
#51573=CARTESIAN_POINT('Ctrl Pts',(-20.9167197831636,-17.3612357869301,
123.396550342784)) ;
#51574=CARTESIAN_POINT('Ctrl Pts',(-20.5944747720619,-17.5512909202513,
123.189052375223)) ;
#51575=CARTESIAN_POINT('Ctrl Pts',(-20.8907754478071,-17.3713018397708,
123.133346946197)) ;
#51576=CARTESIAN_POINT('Ctrl Pts',(-20.5389734302153,-17.5611284361603,
122.989783502597)) ;
#51577=CARTESIAN_POINT('Ctrl Pts',(-20.8213961194626,-17.3811393556798,
122.884260853011)) ;
#51578=CARTESIAN_POINT('Ctrl Pts',(-20.4478531306755,-17.5711971842692,
122.798763312751)) ;
#51579=CARTESIAN_POINT('Ctrl Pts',(-20.7074934612371,-17.3912081037887,
122.645486865845)) ;
#51580=CARTESIAN_POINT('Ctrl Pts',(-20.3271452161414,-17.5810777013002,
122.629676892913)) ;
#51581=CARTESIAN_POINT('Ctrl Pts',(-20.556606167494,-17.4010886208197,122.434129920155)) ;
#51582=CARTESIAN_POINT('Ctrl Pts',(-20.1775948897127,-17.5910688882346,
122.482227937037)) ;
#51583=CARTESIAN_POINT('Ctrl Pts',(-20.3696663137793,-17.4110798077542,
122.2498205318)) ;
#51584=CARTESIAN_POINT('Ctrl Pts',(-20.0053412492469,-17.6010219545096,
122.363377773261)) ;
#51585=CARTESIAN_POINT('Ctrl Pts',(-20.1543475644743,-17.4210328740291,
122.101259878652)) ;
#51586=CARTESIAN_POINT('Ctrl Pts',(-19.8135014291807,-17.6110577920422,
122.275600289609)) ;
#51587=CARTESIAN_POINT('Ctrl Pts',(-19.9145466996496,-17.4310687115617,
121.991540433596)) ;
#51588=CARTESIAN_POINT('Ctrl Pts',(-19.6123051874755,-17.6209479182536,
122.223092310276)) ;
#51589=CARTESIAN_POINT('Ctrl Pts',(-19.6630503154373,-17.4409588377731,
121.925907930471)) ;
#51590=CARTESIAN_POINT('Ctrl Pts',(-19.4029610311012,-17.6309401001616,
122.205808818066)) ;
#51591=CARTESIAN_POINT('Ctrl Pts',(-19.4013697921705,-17.4509510196811,
121.904306259189)) ;
#51592=CARTESIAN_POINT('Ctrl Pts',(-19.1947594778902,-17.6408860401002,
122.225118763395)) ;
#51593=CARTESIAN_POINT('Ctrl Pts',(-19.1411178680451,-17.4608969596197,
121.928446401683)) ;
#51594=CARTESIAN_POINT('Ctrl Pts',(-18.9929258923836,-17.6508332238642,
122.279886430677)) ;
#51595=CARTESIAN_POINT('Ctrl Pts',(-18.888826411622,-17.4708441433838,121.99690869262)) ;
#51596=CARTESIAN_POINT('Ctrl Pts',(-18.8018677982958,-17.6608811621717,
122.369974731862)) ;
#51597=CARTESIAN_POINT('Ctrl Pts',(-18.6500049663537,-17.4808920816912,
122.109521528189)) ;
#51598=CARTESIAN_POINT('Ctrl Pts',(-18.6326849760237,-17.670728796912,122.489300515306)) ;
#51599=CARTESIAN_POINT('Ctrl Pts',(-18.4385276906649,-17.4907397164315,
122.258681232071)) ;
#51600=CARTESIAN_POINT('Ctrl Pts',(-18.48464394166,-17.6806905108858,122.637419729703)) ;
#51601=CARTESIAN_POINT('Ctrl Pts',(-18.2534782915333,-17.5007014304053,
122.443832320165)) ;
#51602=CARTESIAN_POINT('Ctrl Pts',(-18.3639692527773,-17.6907191456766,
122.810318421013)) ;
#51603=CARTESIAN_POINT('Ctrl Pts',(-18.1026371826534,-17.5107300651962,
122.659957308343)) ;
#51604=CARTESIAN_POINT('Ctrl Pts',(-18.2761446006497,-17.7006294642738,
122.999238769557)) ;
#51605=CARTESIAN_POINT('Ctrl Pts',(-17.9928588041681,-17.5206403837933,
122.896109111931)) ;
#51606=CARTESIAN_POINT('Ctrl Pts',(-18.2217890454544,-17.7105643205853,
123.200911892758)) ;
#51607=CARTESIAN_POINT('Ctrl Pts',(-17.9249170446057,-17.5305752401048,
123.148201377883)) ;
#51608=CARTESIAN_POINT('Ctrl Pts',(-18.2032822313656,-17.720605556546,123.411187682898)) ;
#51609=CARTESIAN_POINT('Ctrl Pts',(-17.9017863179622,-17.5406164760655,
123.411046406639)) ;
#51610=CARTESIAN_POINT('Ctrl Pts',(-18.2211170108079,-17.730492328126,123.618292553974)) ;
#51611=CARTESIAN_POINT('Ctrl Pts',(-17.9240826083119,-17.5505032476455,
123.66992741687)) ;
#51612=CARTESIAN_POINT('Ctrl Pts',(-18.2749965572381,-17.7404925068322,
123.821474487423)) ;
#51613=CARTESIAN_POINT('Ctrl Pts',(-17.9914347891507,-17.5605034263517,
123.923904178052)) ;
#51614=CARTESIAN_POINT('Ctrl Pts',(-18.36246816189,-17.7504097850418,124.010768806246)) ;
#51615=CARTESIAN_POINT('Ctrl Pts',(-18.1007768931829,-17.5704207045613,
124.16052097631)) ;
#51616=CARTESIAN_POINT('Ctrl Pts',(-18.48305480673,-17.7604570314554,124.184154003306)) ;
#51617=CARTESIAN_POINT('Ctrl Pts',(-18.2515125584344,-17.580467950975,124.377250917439)) ;
#51618=CARTESIAN_POINT('Ctrl Pts',(-18.629232331941,-17.7703309204367,124.331582621373)) ;
#51619=CARTESIAN_POINT('Ctrl Pts',(-18.4342365121,-17.5903418399563,124.561534748493)) ;
#51620=CARTESIAN_POINT('Ctrl Pts',(-18.8019032378778,-17.7803929380173,
124.453733894309)) ;
#51621=CARTESIAN_POINT('Ctrl Pts',(-18.650076844081,-17.6004038575368,124.714221581174)) ;
#51622=CARTESIAN_POINT('Ctrl Pts',(-18.9895800757917,-17.7902639997516,
124.542325237439)) ;
#51623=CARTESIAN_POINT('Ctrl Pts',(-18.8846741124634,-17.6102749192711,
124.824958215824)) ;
#51624=CARTESIAN_POINT('Ctrl Pts',(-19.1921134940513,-17.8002580631119,
124.598226493753)) ;
#51625=CARTESIAN_POINT('Ctrl Pts',(-19.1378416764375,-17.6202689826314,
124.894832090757)) ;
#51626=CARTESIAN_POINT('Ctrl Pts',(-19.4021121856622,-17.8102902211453,
124.617721341239)) ;
#51627=CARTESIAN_POINT('Ctrl Pts',(-19.4003404043866,-17.6303011406648,
124.919197850925)) ;
#51628=CARTESIAN_POINT('Ctrl Pts',(-19.608844588004,-17.8201540973854,124.601197546684)) ;
#51629=CARTESIAN_POINT('Ctrl Pts',(-19.6587556166783,-17.640165016905,124.898540309073)) ;
#51630=CARTESIAN_POINT('Ctrl Pts',(-19.8137331839509,-17.8302246120237,
124.54797156307)) ;
#51631=CARTESIAN_POINT('Ctrl Pts',(-19.9148657636733,-17.6502355315432,
124.832005118478)) ;
#51632=CARTESIAN_POINT('Ctrl Pts',(-20.0019178911935,-17.8400652489647,
124.461988692631)) ;
#51633=CARTESIAN_POINT('Ctrl Pts',(-20.1500954777308,-17.6600761684842,
124.72452389297)) ;
#51634=CARTESIAN_POINT('Ctrl Pts',(-20.1748685848524,-17.8500323778049,
124.343718173055)) ;
#51635=CARTESIAN_POINT('Ctrl Pts',(-20.3662817218057,-17.6700432973244,
124.576684082019)) ;
#51636=CARTESIAN_POINT('Ctrl Pts',(-20.3252263227975,-17.8600463509294,
124.196347627969)) ;
#51637=CARTESIAN_POINT('Ctrl Pts',(-20.5542290544657,-17.6800572704489,
124.392466662775)) ;
#51638=CARTESIAN_POINT('Ctrl Pts',(-20.4877929513438,-17.8733310847927,
123.96921781494)) ;
#51639=CARTESIAN_POINT('Ctrl Pts',(-20.7574242466932,-17.6933420043122,
124.108563216924)) ;
#51640=CARTESIAN_POINT('Ctrl Pts',(-20.5871211093539,-17.8865563495074,
123.706157520284)) ;
#51641=CARTESIAN_POINT('Ctrl Pts',(-20.8815792329842,-17.706567269027,123.779776387275)) ;
#51642=CARTESIAN_POINT('Ctrl Pts',(-20.6152234023706,-17.8998668720623,
123.427758973367)) ;
#51643=CARTESIAN_POINT('Ctrl Pts',(-20.9167156269414,-17.7198777915818,
123.431719811705)) ;
#51644=CARTESIAN_POINT('Ctrl Pts',(-20.5994871791015,-17.9098955169645,
123.217511431126)) ;
#51645=CARTESIAN_POINT('Ctrl Pts',(-20.8970403047877,-17.729906436484,123.168922156201)) ;
#51646=CARTESIAN_POINT('Ctrl Pts',(-20.5484258087731,-17.9197765493184,
123.01615172322)) ;
#51647=CARTESIAN_POINT('Ctrl Pts',(-20.8332113376201,-17.7397874688379,
122.917220164126)) ;
#51648=CARTESIAN_POINT('Ctrl Pts',(-20.462715022261,-17.9297575219985,122.82462433537)) ;
#51649=CARTESIAN_POINT('Ctrl Pts',(-20.7260717928648,-17.749768441518,122.677813694305)) ;
#51650=CARTESIAN_POINT('Ctrl Pts',(-20.3449102482183,-17.9397386495845,
122.650999042694)) ;
#51651=CARTESIAN_POINT('Ctrl Pts',(-20.5788081878734,-17.759749569104,122.460780264954)) ;
#51652=CARTESIAN_POINT('Ctrl Pts',(-20.1513290480844,-17.9529818398459,
122.450788742147)) ;
#51653=CARTESIAN_POINT('Ctrl Pts',(-20.3368568948601,-17.7729927593654,
122.210535455664)) ;
#51654=CARTESIAN_POINT('Ctrl Pts',(-19.8474795977767,-17.9696498352067,
122.268601957147)) ;
#51655=CARTESIAN_POINT('Ctrl Pts',(-19.9569936986042,-17.7896607547262,
121.982786748318)) ;
#51656=CARTESIAN_POINT('Ctrl Pts',(-19.5025885485555,-17.9861703352187,
122.201337269194)) ;
#51657=CARTESIAN_POINT('Ctrl Pts',(-19.5259606159794,-17.8061812547382,
121.898720901943)) ;
#51658=CARTESIAN_POINT('Ctrl Pts',(-19.2234322226272,-17.9994833515347,
122.220261932405)) ;
#51659=CARTESIAN_POINT('Ctrl Pts',(-19.1769501917379,-17.8194942710542,
121.922374301717)) ;
#51660=CARTESIAN_POINT('Ctrl Pts',(-19.0209334833378,-18.0093999097677,
122.270017422137)) ;
#51661=CARTESIAN_POINT('Ctrl Pts',(-18.9238414463317,-17.8294108292872,
121.98457134201)) ;
#51662=CARTESIAN_POINT('Ctrl Pts',(-18.8281337131634,-18.0194275780706,
122.355152407899)) ;
#51663=CARTESIAN_POINT('Ctrl Pts',(-18.682836795022,-17.8394384975901,122.090994480556)) ;
#51664=CARTESIAN_POINT('Ctrl Pts',(-18.5974653025486,-18.0326081678152,
122.508905891752)) ;
#51665=CARTESIAN_POINT('Ctrl Pts',(-18.3945158970904,-17.8526190873348,
122.283176068274)) ;
#51666=CARTESIAN_POINT('Ctrl Pts',(-18.3626740824795,-18.0493563069346,
122.776403364024)) ;
#51667=CARTESIAN_POINT('Ctrl Pts',(-18.1010163557202,-17.8693672264541,
122.617564692442)) ;
#51668=CARTESIAN_POINT('Ctrl Pts',(-18.2093429381581,-18.0691510494452,
123.168585983566)) ;
#51669=CARTESIAN_POINT('Ctrl Pts',(-17.909361184376,-17.8891619689647,123.107788785538)) ;
#51670=CARTESIAN_POINT('Ctrl Pts',(-18.1984950373618,-18.089195442254,123.594497284543)) ;
#51671=CARTESIAN_POINT('Ctrl Pts',(-17.8958042829193,-17.9092063617735,
123.640179567838)) ;
#51672=CARTESIAN_POINT('Ctrl Pts',(-18.3326878160101,-18.1090346245527,
123.994538645704)) ;
#51673=CARTESIAN_POINT('Ctrl Pts',(-18.0635490481216,-17.9290455440722,
124.140228438926)) ;
#51674=CARTESIAN_POINT('Ctrl Pts',(-18.595526380158,-18.1289599482456,124.326686433183)) ;
#51675=CARTESIAN_POINT('Ctrl Pts',(-18.3920994918679,-17.9489708677651,
124.555410464807)) ;
#51676=CARTESIAN_POINT('Ctrl Pts',(-18.9560767803861,-18.1488835862971,
124.549228315396)) ;
#51677=CARTESIAN_POINT('Ctrl Pts',(-18.842788696295,-17.9688945058166,124.833584548361)) ;
#51678=CARTESIAN_POINT('Ctrl Pts',(-19.3708100254435,-18.1688084597626,
124.63548572576)) ;
#51679=CARTESIAN_POINT('Ctrl Pts',(-19.361205130707,-17.9888193792821,124.941403037366)) ;
#51680=CARTESIAN_POINT('Ctrl Pts',(-19.7892611661208,-18.1886870668415,
124.575714298968)) ;
#51681=CARTESIAN_POINT('Ctrl Pts',(-19.8842672961857,-18.008697986361,124.866686275216)) ;
#51682=CARTESIAN_POINT('Ctrl Pts',(-20.1641187112948,-18.2086645096735,
124.375945013966)) ;
#51683=CARTESIAN_POINT('Ctrl Pts',(-20.3528378764047,-18.028675429193,124.616972672933)) ;
#51684=CARTESIAN_POINT('Ctrl Pts',(-20.4474662277744,-18.2285963577582,
124.06073373373)) ;
#51685=CARTESIAN_POINT('Ctrl Pts',(-20.7070199753462,-18.0486072772777,
124.222957551493)) ;
#51686=CARTESIAN_POINT('Ctrl Pts',(-20.6063082660546,-18.2484916261008,
123.668688283209)) ;
#51687=CARTESIAN_POINT('Ctrl Pts',(-20.905570212033,-18.0685025456203,123.7329012805)) ;
#51688=CARTESIAN_POINT('Ctrl Pts',(-20.6223259515978,-18.2684141245129,
123.245374252905)) ;
#51689=CARTESIAN_POINT('Ctrl Pts',(-20.9255908590547,-18.0884250440324,
123.203759760779)) ;
#51690=CARTESIAN_POINT('Ctrl Pts',(-20.4925770960382,-18.2883736063889,
122.841276292266)) ;
#51691=CARTESIAN_POINT('Ctrl Pts',(-20.7634037512627,-18.1083845259084,
122.698638234427)) ;
#51692=CARTESIAN_POINT('Ctrl Pts',(-20.2338987435689,-18.3082513588482,
122.507109401429)) ;
#51693=CARTESIAN_POINT('Ctrl Pts',(-20.4400561874545,-18.1282622783678,
122.280931726581)) ;
#51694=CARTESIAN_POINT('Ctrl Pts',(-19.8771610118705,-18.3281331495828,
122.280132547987)) ;
#51695=CARTESIAN_POINT('Ctrl Pts',(-19.9941357018043,-18.1481440691023,
121.997211525519)) ;
#51696=CARTESIAN_POINT('Ctrl Pts',(-19.4603627437856,-18.3482064884338,
122.188495687106)) ;
#51697=CARTESIAN_POINT('Ctrl Pts',(-19.4731366764473,-18.1682174079533,
121.882665391042)) ;
#51698=CARTESIAN_POINT('Ctrl Pts',(-19.0428183765593,-18.3680109556696,
122.243747752997)) ;
#51699=CARTESIAN_POINT('Ctrl Pts',(-18.9512092801426,-18.1880218751891,
121.951729931177)) ;
#51700=CARTESIAN_POINT('Ctrl Pts',(-18.6655136826897,-18.3879942960774,
122.439019897287)) ;
#51701=CARTESIAN_POINT('Ctrl Pts',(-18.4795781027084,-18.2080052155969,
122.195819043092)) ;
#51702=CARTESIAN_POINT('Ctrl Pts',(-18.3789384655421,-18.4079092606754,
122.750760297529)) ;
#51703=CARTESIAN_POINT('Ctrl Pts',(-18.1213593077318,-18.2279201801949,
122.585493056673)) ;
#51704=CARTESIAN_POINT('Ctrl Pts',(-18.2152038691917,-18.4277777953917,
123.140286780608)) ;
#51705=CARTESIAN_POINT('Ctrl Pts',(-17.9166900269877,-18.2477887149113,
123.072398846917)) ;
#51706=CARTESIAN_POINT('Ctrl Pts',(-18.1947300807791,-18.4478301796035,
123.566037893384)) ;
#51707=CARTESIAN_POINT('Ctrl Pts',(-17.8910961294277,-18.267841099123,123.60458827601)) ;
#51708=CARTESIAN_POINT('Ctrl Pts',(-18.3185671471098,-18.4676041433927,
123.96801283456)) ;
#51709=CARTESIAN_POINT('Ctrl Pts',(-18.0458895720213,-18.2876150629122,
124.10705494621)) ;
#51710=CARTESIAN_POINT('Ctrl Pts',(-18.5752678737993,-18.487658522414,124.308284568343)) ;
#51711=CARTESIAN_POINT('Ctrl Pts',(-18.3667637787216,-18.3076694419336,
124.532396665767)) ;
#51712=CARTESIAN_POINT('Ctrl Pts',(-18.9284212326359,-18.5074552599873,
124.537569903936)) ;
#51713=CARTESIAN_POINT('Ctrl Pts',(-18.8082021317787,-18.3274661795068,
124.819004328928)) ;
#51714=CARTESIAN_POINT('Ctrl Pts',(-19.3416803678244,-18.5274230723387,
124.634498823647)) ;
#51715=CARTESIAN_POINT('Ctrl Pts',(-19.3247749684636,-18.3474339918583,
124.940168786696)) ;
#51716=CARTESIAN_POINT('Ctrl Pts',(-19.7631205986786,-18.5473820484038,
124.583927911147)) ;
#51717=CARTESIAN_POINT('Ctrl Pts',(-19.8515753100361,-18.3673929679233,
124.876958419638)) ;
#51718=CARTESIAN_POINT('Ctrl Pts',(-20.1408243512989,-18.5672769666812,
124.393475715096)) ;
#51719=CARTESIAN_POINT('Ctrl Pts',(-20.3237057376105,-18.3872878862007,
124.638896796487)) ;
#51720=CARTESIAN_POINT('Ctrl Pts',(-20.4312496937618,-18.5871732791315,
124.085918903188)) ;
#51721=CARTESIAN_POINT('Ctrl Pts',(-20.6867396806704,-18.407184198651,124.254454113061)) ;
#51722=CARTESIAN_POINT('Ctrl Pts',(-20.5998462621265,-18.6070812125056,
123.69761409053)) ;
#51723=CARTESIAN_POINT('Ctrl Pts',(-20.8974889911539,-18.4270921320251,
123.769075405474)) ;
#51724=CARTESIAN_POINT('Ctrl Pts',(-20.6258188714983,-18.6270311027941,
123.274258003805)) ;
#51725=CARTESIAN_POINT('Ctrl Pts',(-20.9299591276609,-18.4470420223136,
123.239880881314)) ;
#51726=CARTESIAN_POINT('Ctrl Pts',(-20.5065921902261,-18.6469083332954,
122.868736889825)) ;
#51727=CARTESIAN_POINT('Ctrl Pts',(-20.7809301920066,-18.4669192528149,
122.732978965298)) ;
#51728=CARTESIAN_POINT('Ctrl Pts',(-20.2550219026943,-18.6668910021664,
122.526359546569)) ;
#51729=CARTESIAN_POINT('Ctrl Pts',(-20.4664719536268,-18.4869019216859,
122.305004321763)) ;
#51730=CARTESIAN_POINT('Ctrl Pts',(-19.9023778798508,-18.6868238887468,
122.291166846904)) ;
#51731=CARTESIAN_POINT('Ctrl Pts',(-20.0256670326926,-18.5068348082663,
122.011010323903)) ;
#51732=CARTESIAN_POINT('Ctrl Pts',(-19.4912013862512,-18.7067366347647,
122.190280264544)) ;
#51733=CARTESIAN_POINT('Ctrl Pts',(-19.5117084694542,-18.5267475542842,
121.884894904074)) ;
#51734=CARTESIAN_POINT('Ctrl Pts',(-19.1409101901299,-18.7233063561065,
122.227714641459)) ;
#51735=CARTESIAN_POINT('Ctrl Pts',(-19.0738118335659,-18.543317275626,121.931691304887)) ;
#51736=CARTESIAN_POINT('Ctrl Pts',(-18.8799531775115,-18.7366063674115,
122.328226065219)) ;
#51737=CARTESIAN_POINT('Ctrl Pts',(-18.7476501459494,-18.556617286931,122.057314468729)) ;
#51738=CARTESIAN_POINT('Ctrl Pts',(-18.6408115625997,-18.7498765551614,
122.471815662188)) ;
#51739=CARTESIAN_POINT('Ctrl Pts',(-18.448665698478,-18.5698874746809,122.236842368626)) ;
#51740=CARTESIAN_POINT('Ctrl Pts',(-18.3949285657691,-18.7665039375268,
122.725952569314)) ;
#51741=CARTESIAN_POINT('Ctrl Pts',(-18.141372227169,-18.5865148570463,122.554451894984)) ;
#51742=CARTESIAN_POINT('Ctrl Pts',(-18.2507607995782,-18.783126227272,123.048601698657)) ;
#51743=CARTESIAN_POINT('Ctrl Pts',(-17.9611265354326,-18.6031371467915,
122.957810899803)) ;
#51744=CARTESIAN_POINT('Ctrl Pts',(-18.2066124842382,-18.7963714416665,
123.323560231487)) ;
#51745=CARTESIAN_POINT('Ctrl Pts',(-17.9059528959397,-18.616382361186,123.301475150394)) ;
#51746=CARTESIAN_POINT('Ctrl Pts',(-18.2091963113951,-18.8062834066272,
123.531933666297)) ;
#51747=CARTESIAN_POINT('Ctrl Pts',(-17.9091768532067,-18.6262943261467,
123.561948497641)) ;
#51748=CARTESIAN_POINT('Ctrl Pts',(-18.2487269856474,-18.8163420297916,
123.739647393853)) ;
#51749=CARTESIAN_POINT('Ctrl Pts',(-17.9585883653442,-18.6363529493112,
123.821589557163)) ;
#51750=CARTESIAN_POINT('Ctrl Pts',(-18.3218273859011,-18.8261821439075,
123.933204366604)) ;
#51751=CARTESIAN_POINT('Ctrl Pts',(-18.0499609715988,-18.646193063427,124.063536985095)) ;
#51752=CARTESIAN_POINT('Ctrl Pts',(-18.4296324438484,-18.8362479288651,
124.115263613763)) ;
#51753=CARTESIAN_POINT('Ctrl Pts',(-18.1847150491307,-18.6562588483846,
124.291112489709)) ;
#51754=CARTESIAN_POINT('Ctrl Pts',(-18.5650197569021,-18.846131246653,124.27291340767)) ;
#51755=CARTESIAN_POINT('Ctrl Pts',(-18.3539469881779,-18.6661421661725,
124.488176476417)) ;
#51756=CARTESIAN_POINT('Ctrl Pts',(-18.7271216090986,-18.8561206845115,
124.40639870705)) ;
#51757=CARTESIAN_POINT('Ctrl Pts',(-18.5565725703095,-18.6761316040311,
124.65503529775)) ;
#51758=CARTESIAN_POINT('Ctrl Pts',(-18.9095316281554,-18.8660843985643,
124.509393822221)) ;
#51759=CARTESIAN_POINT('Ctrl Pts',(-18.7845837389449,-18.6860953180838,
124.783781642448)) ;
#51760=CARTESIAN_POINT('Ctrl Pts',(-19.1076061689565,-18.8760794102235,
124.579581320828)) ;
#51761=CARTESIAN_POINT('Ctrl Pts',(-19.0321760408192,-18.696090329743,124.871518685456)) ;
#51762=CARTESIAN_POINT('Ctrl Pts',(-19.3157436958266,-18.8861157019177,
124.61412399333)) ;
#51763=CARTESIAN_POINT('Ctrl Pts',(-19.2923475774005,-18.7061266214373,
124.91469979869)) ;
#51764=CARTESIAN_POINT('Ctrl Pts',(-19.5227505678203,-18.8959620796112,
124.612380202904)) ;
#51765=CARTESIAN_POINT('Ctrl Pts',(-19.5511061455556,-18.7159729991307,
124.912522869944)) ;
#51766=CARTESIAN_POINT('Ctrl Pts',(-19.7292055330348,-18.9059470237619,
124.57459229136)) ;
#51767=CARTESIAN_POINT('Ctrl Pts',(-19.8091754394727,-18.7259579432814,
124.865290742925)) ;
#51768=CARTESIAN_POINT('Ctrl Pts',(-19.9251198106704,-18.9158839948918,
124.501974601842)) ;
#51769=CARTESIAN_POINT('Ctrl Pts',(-20.0540693303344,-18.7358949144114,
124.774521245491)) ;
#51770=CARTESIAN_POINT('Ctrl Pts',(-20.1073932158431,-18.9259337795236,
124.395175327921)) ;
#51771=CARTESIAN_POINT('Ctrl Pts',(-20.2819125650072,-18.7459446990431,
124.64102455538)) ;
#51772=CARTESIAN_POINT('Ctrl Pts',(-20.2652907922645,-18.9357842416011,
124.261160532584)) ;
#51773=CARTESIAN_POINT('Ctrl Pts',(-20.4792864443041,-18.7557951611206,
124.473508135984)) ;
#51774=CARTESIAN_POINT('Ctrl Pts',(-20.3995458132042,-18.9457562551215,
124.100179995345)) ;
#51775=CARTESIAN_POINT('Ctrl Pts',(-20.6471074505212,-18.765767174641,124.272284173965)) ;
#51776=CARTESIAN_POINT('Ctrl Pts',(-20.5040579564351,-18.9557514022409,
123.91784560784)) ;
#51777=CARTESIAN_POINT('Ctrl Pts',(-20.7777500988216,-18.7757623217604,
124.044367513439)) ;
#51778=CARTESIAN_POINT('Ctrl Pts',(-20.5753422248365,-18.965785371977,123.71932854599)) ;
#51779=CARTESIAN_POINT('Ctrl Pts',(-20.8668580983504,-18.7857962914965,
123.796222100984)) ;
#51780=CARTESIAN_POINT('Ctrl Pts',(-20.6107665468007,-18.9756409176476,
123.515165091888)) ;
#51781=CARTESIAN_POINT('Ctrl Pts',(-20.9111412972564,-18.7956518371671,
123.541018035031)) ;
#51782=CARTESIAN_POINT('Ctrl Pts',(-20.6104909571507,-18.9856396746608,
123.304993816628)) ;
#51783=CARTESIAN_POINT('Ctrl Pts',(-20.9107995973893,-18.8056505941803,
123.278303845402)) ;
#51784=CARTESIAN_POINT('Ctrl Pts',(-20.5742854817518,-18.995536809898,123.100067497722)) ;
#51785=CARTESIAN_POINT('Ctrl Pts',(-20.8655454313835,-18.8155477294175,
123.022145216634)) ;
#51786=CARTESIAN_POINT('Ctrl Pts',(-20.5019793355474,-19.0055899057376,
122.901496245715)) ;
#51787=CARTESIAN_POINT('Ctrl Pts',(-20.7751653504057,-18.8256008252571,
122.773930212784)) ;
#51788=CARTESIAN_POINT('Ctrl Pts',(-20.3980758274042,-19.0154734144682,
122.721542018855)) ;
#51789=CARTESIAN_POINT('Ctrl Pts',(-20.6452882014999,-18.8354843339877,
122.548985779827)) ;
#51790=CARTESIAN_POINT('Ctrl Pts',(-20.2633899531571,-19.0254682871143,
122.560268873648)) ;
#51791=CARTESIAN_POINT('Ctrl Pts',(-20.4769328740491,-18.8454792066338,
122.347392525838)) ;
#51792=CARTESIAN_POINT('Ctrl Pts',(-20.1021192146536,-19.03548824875,122.424730589061)) ;
#51793=CARTESIAN_POINT('Ctrl Pts',(-20.2753461931857,-18.8554991682695,
122.177967546713)) ;
#51794=CARTESIAN_POINT('Ctrl Pts',(-19.9219503779301,-19.0453936125498,
122.320315131971)) ;
#51795=CARTESIAN_POINT('Ctrl Pts',(-20.0501362496351,-18.8654045320694,
122.047445707067)) ;
#51796=CARTESIAN_POINT('Ctrl Pts',(-19.725850127901,-19.0553342001574,122.248117440437)) ;
#51797=CARTESIAN_POINT('Ctrl Pts',(-19.8050116122728,-18.8753451196769,
121.957195984655)) ;
#51798=CARTESIAN_POINT('Ctrl Pts',(-19.5188889597631,-19.065337018258,122.21070880174)) ;
#51799=CARTESIAN_POINT('Ctrl Pts',(-19.5463105434704,-18.8853479377776,
121.910432554747)) ;
#51800=CARTESIAN_POINT('Ctrl Pts',(-19.3079401318783,-19.0753717299822,
122.210144775601)) ;
#51801=CARTESIAN_POINT('Ctrl Pts',(-19.2826245313251,-18.8953826495017,
121.909724812158)) ;
#51802=CARTESIAN_POINT('Ctrl Pts',(-19.1039450954541,-19.0852166367195,
122.245193265837)) ;
#51803=CARTESIAN_POINT('Ctrl Pts',(-19.0276297317247,-18.905227556239,121.953532899753)) ;
#51804=CARTESIAN_POINT('Ctrl Pts',(-18.9062559735361,-19.0952024892885,
122.315743265558)) ;
#51805=CARTESIAN_POINT('Ctrl Pts',(-18.7805173028512,-18.915213408808,122.041718001844)) ;
#51806=CARTESIAN_POINT('Ctrl Pts',(-18.7246158514163,-19.1051372977015,
122.418922406294)) ;
#51807=CARTESIAN_POINT('Ctrl Pts',(-18.5534655976268,-18.9251482172211,
122.170689853472)) ;
#51808=CARTESIAN_POINT('Ctrl Pts',(-18.5618355249981,-19.1151948247826,
122.553818901335)) ;
#51809=CARTESIAN_POINT('Ctrl Pts',(-18.3499886136617,-18.9352057443021,
122.339308389629)) ;
#51810=CARTESIAN_POINT('Ctrl Pts',(-18.4278858922511,-19.1250164797797,
122.710986226802)) ;
#51811=CARTESIAN_POINT('Ctrl Pts',(-18.1825491266174,-18.9450273992992,
122.535766487413)) ;
#51812=CARTESIAN_POINT('Ctrl Pts',(-18.3204432885905,-19.1350725239527,
122.893038269463)) ;
#51813=CARTESIAN_POINT('Ctrl Pts',(-18.048243794037,-18.9550834434722,122.763330187335)) ;
#51814=CARTESIAN_POINT('Ctrl Pts',(-18.2474379776068,-19.1450132639979,
123.088867079134)) ;
#51815=CARTESIAN_POINT('Ctrl Pts',(-17.9569846491174,-18.9650241835174,
123.008115620685)) ;
#51816=CARTESIAN_POINT('Ctrl Pts',(-18.2090421542517,-19.1549173850707,
123.293514642458)) ;
#51817=CARTESIAN_POINT('Ctrl Pts',(-17.9089873946553,-18.9749283045903,
123.26392514925)) ;
#51818=CARTESIAN_POINT('Ctrl Pts',(-18.2068596104492,-19.164964926225,123.504719529866)) ;
#51819=CARTESIAN_POINT('Ctrl Pts',(-17.9062567712307,-18.9849758457445,
123.527931134962)) ;
#51820=CARTESIAN_POINT('Ctrl Pts',(-18.2407268057589,-19.1748636778254,
123.710075861997)) ;
#51821=CARTESIAN_POINT('Ctrl Pts',(-17.9485884794036,-18.9948745973449,
123.784627499361)) ;
#51822=CARTESIAN_POINT('Ctrl Pts',(-18.3106763440572,-19.1849121567912,
123.909385049677)) ;
#51823=CARTESIAN_POINT('Ctrl Pts',(-18.0360231029504,-19.0049230763107,
124.033764662997)) ;
#51824=CARTESIAN_POINT('Ctrl Pts',(-18.4125198148673,-19.1947996538749,
124.09061780245)) ;
#51825=CARTESIAN_POINT('Ctrl Pts',(-18.1633256706012,-19.0148105733944,
124.26030732657)) ;
#51826=CARTESIAN_POINT('Ctrl Pts',(-18.5453641416013,-19.204792744173,124.253347261805)) ;
#51827=CARTESIAN_POINT('Ctrl Pts',(-18.3293793930391,-19.0248036636925,
124.463720725845)) ;
#51828=CARTESIAN_POINT('Ctrl Pts',(-18.70386501416,-19.2147449142333,124.389942305651)) ;
#51829=CARTESIAN_POINT('Ctrl Pts',(-18.527504240545,-19.0347558337528,124.634466520031)) ;
#51830=CARTESIAN_POINT('Ctrl Pts',(-18.8832573055452,-19.2246833341478,
124.497026002691)) ;
#51831=CARTESIAN_POINT('Ctrl Pts',(-18.7517438316603,-19.0446942536673,
124.768323297008)) ;
#51832=CARTESIAN_POINT('Ctrl Pts',(-19.0793846745513,-19.2346684642334,
124.571917646202)) ;
#51833=CARTESIAN_POINT('Ctrl Pts',(-18.996902443479,-19.0546793837529,124.861939963005)) ;
#51834=CARTESIAN_POINT('Ctrl Pts',(-19.2866263766652,-19.2447051536475,
124.611508315712)) ;
#51835=CARTESIAN_POINT('Ctrl Pts',(-19.2559540582178,-19.064716073167,124.911430512006)) ;
#51836=CARTESIAN_POINT('Ctrl Pts',(-19.4937950988768,-19.25455983764,124.614789826941)) ;
#51837=CARTESIAN_POINT('Ctrl Pts',(-19.5149158429262,-19.0745707571595,
124.915534596148)) ;
#51838=CARTESIAN_POINT('Ctrl Pts',(-19.7013848668796,-19.2645593216878,
124.581864338488)) ;
#51839=CARTESIAN_POINT('Ctrl Pts',(-19.7744035154957,-19.0845702412073,
124.874379795897)) ;
#51840=CARTESIAN_POINT('Ctrl Pts',(-19.8981684622734,-19.2744544104647,
124.514296465217)) ;
#51841=CARTESIAN_POINT('Ctrl Pts',(-20.0203843649361,-19.0944653299842,
124.789921645823)) ;
#51842=CARTESIAN_POINT('Ctrl Pts',(-20.0832105036019,-19.2845149651109,
124.411914232186)) ;
#51843=CARTESIAN_POINT('Ctrl Pts',(-20.2516876996053,-19.1045258846304,
124.661945764523)) ;
#51844=CARTESIAN_POINT('Ctrl Pts',(-20.2443173608154,-19.2943642294838,
124.281814272574)) ;
#51845=CARTESIAN_POINT('Ctrl Pts',(-20.453073345448,-19.1143751490033,124.499321729765)) ;
#51846=CARTESIAN_POINT('Ctrl Pts',(-20.383234603429,-19.3043914819316,124.123263298254)) ;
#51847=CARTESIAN_POINT('Ctrl Pts',(-20.6267212721774,-19.1244024014511,
124.301134265008)) ;
#51848=CARTESIAN_POINT('Ctrl Pts',(-20.4920569293237,-19.3144197795018,
123.942681895053)) ;
#51849=CARTESIAN_POINT('Ctrl Pts',(-20.7627508779272,-19.1344306990213,
124.07540861647)) ;
#51850=CARTESIAN_POINT('Ctrl Pts',(-20.5668588209695,-19.3242659085078,
123.749683017547)) ;
#51851=CARTESIAN_POINT('Ctrl Pts',(-20.856255422354,-19.1442768280273,123.83415966172)) ;
#51852=CARTESIAN_POINT('Ctrl Pts',(-20.608133965986,-19.3342598138698,123.543674588756)) ;
#51853=CARTESIAN_POINT('Ctrl Pts',(-20.9078510942606,-19.1542707333894,
123.576649296559)) ;
#51854=CARTESIAN_POINT('Ctrl Pts',(-20.6126495317417,-19.3442839115529,
123.332979210101)) ;
#51855=CARTESIAN_POINT('Ctrl Pts',(-20.913497410932,-19.1642948310724,123.313280162648)) ;
#51856=CARTESIAN_POINT('Ctrl Pts',(-20.5812020044249,-19.3541737394069,
123.127452597675)) ;
#51857=CARTESIAN_POINT('Ctrl Pts',(-20.8741896284399,-19.1741846589264,
123.056370784459)) ;
#51858=CARTESIAN_POINT('Ctrl Pts',(-20.5141513741435,-19.3641657208373,
122.928386984327)) ;
#51859=CARTESIAN_POINT('Ctrl Pts',(-20.7903778748862,-19.1841766403569,
122.807538053426)) ;
#51860=CARTESIAN_POINT('Ctrl Pts',(-20.4139600151984,-19.3741127256032,
122.744833669231)) ;
#51861=CARTESIAN_POINT('Ctrl Pts',(-20.6651399258501,-19.1941236451227,
122.578095153179)) ;
#51862=CARTESIAN_POINT('Ctrl Pts',(-20.2836802509689,-19.384062376993,122.581175213375)) ;
#51863=CARTESIAN_POINT('Ctrl Pts',(-20.5022911488961,-19.2040732965125,
122.373520731154)) ;
#51864=CARTESIAN_POINT('Ctrl Pts',(-20.1254838491908,-19.3940993799704,
122.441545872889)) ;
#51865=CARTESIAN_POINT('Ctrl Pts',(-20.3045468223484,-19.2141102994899,
122.198982921327)) ;
#51866=CARTESIAN_POINT('Ctrl Pts',(-19.9481679622584,-19.4039882884054,
122.332997305238)) ;
#51867=CARTESIAN_POINT('Ctrl Pts',(-20.0829020054468,-19.2239992079249,
122.063295386197)) ;
#51868=CARTESIAN_POINT('Ctrl Pts',(-19.7528840797197,-19.4139776208829,
122.255763547514)) ;
#51869=CARTESIAN_POINT('Ctrl Pts',(-19.8387974858014,-19.2339885404024,
121.966751761662)) ;
#51870=CARTESIAN_POINT('Ctrl Pts',(-19.5477596783419,-19.42393617632,122.213894358969)) ;
#51871=CARTESIAN_POINT('Ctrl Pts',(-19.5823918613981,-19.2439470958395,
121.914413714354)) ;
#51872=CARTESIAN_POINT('Ctrl Pts',(-19.339716261487,-19.4338357475205,122.20779695739)) ;
#51873=CARTESIAN_POINT('Ctrl Pts',(-19.3223367513791,-19.25384666704,121.90679061317)) ;
#51874=CARTESIAN_POINT('Ctrl Pts',(-19.1307330189891,-19.4438836727725,
122.238435863334)) ;
#51875=CARTESIAN_POINT('Ctrl Pts',(-19.0611077173533,-19.263894592292,121.945087876607)) ;
#51876=CARTESIAN_POINT('Ctrl Pts',(-18.9331863686477,-19.4537789722985,
122.303747134582)) ;
#51877=CARTESIAN_POINT('Ctrl Pts',(-18.8141731330482,-19.273789891818,122.026726024878)) ;
#51878=CARTESIAN_POINT('Ctrl Pts',(-18.7469349813943,-19.4638408287464,
122.403975883156)) ;
#51879=CARTESIAN_POINT('Ctrl Pts',(-18.5813585769284,-19.283851748266,122.152010675275)) ;
#51880=CARTESIAN_POINT('Ctrl Pts',(-18.5844603918164,-19.4736846751631,
122.532169779838)) ;
#51881=CARTESIAN_POINT('Ctrl Pts',(-18.3782635157995,-19.2936955946826,
122.31225286632)) ;
#51882=CARTESIAN_POINT('Ctrl Pts',(-18.444520656928,-19.4836476242911,122.687999610544)) ;
#51883=CARTESIAN_POINT('Ctrl Pts',(-18.2033377995914,-19.3036585438106,
122.507039819506)) ;
#51884=CARTESIAN_POINT('Ctrl Pts',(-18.3332595420171,-19.4936816607191,
122.867226494345)) ;
#51885=CARTESIAN_POINT('Ctrl Pts',(-18.0642605164211,-19.3136925802387,
122.731072712996)) ;
#51886=CARTESIAN_POINT('Ctrl Pts',(-18.2557552508508,-19.5035690876772,
123.060098414967)) ;
#51887=CARTESIAN_POINT('Ctrl Pts',(-17.9673787964987,-19.3235800071967,
122.972163161399)) ;
#51888=CARTESIAN_POINT('Ctrl Pts',(-18.2119716822401,-19.5135835220135,
123.266045020976)) ;
#51889=CARTESIAN_POINT('Ctrl Pts',(-17.91264845191,-19.3335944415331,123.229596243472)) ;
#51890=CARTESIAN_POINT('Ctrl Pts',(-18.2051271781336,-19.5236184666485,
123.476886047581)) ;
#51891=CARTESIAN_POINT('Ctrl Pts',(-17.9040917214434,-19.343629386168,123.493147352369)) ;
#51892=CARTESIAN_POINT('Ctrl Pts',(-18.2338373099495,-19.5334508166795,
123.681614438135)) ;
#51893=CARTESIAN_POINT('Ctrl Pts',(-17.9399787129284,-19.353461736199,123.749059430718)) ;
#51894=CARTESIAN_POINT('Ctrl Pts',(-18.2991584830252,-19.5435262557967,
123.883066110455)) ;
#51895=CARTESIAN_POINT('Ctrl Pts',(-18.0216292178934,-19.3635371753162,
124.00087385622)) ;
#51896=CARTESIAN_POINT('Ctrl Pts',(-18.3962015107462,-19.5533787210313,
124.066105872207)) ;
#51897=CARTESIAN_POINT('Ctrl Pts',(-18.1429328955144,-19.3733896405508,
124.229675102713)) ;
#51898=CARTESIAN_POINT('Ctrl Pts',(-18.5262180602235,-19.5634515986082,
124.233211940351)) ;
#51899=CARTESIAN_POINT('Ctrl Pts',(-18.3054527182946,-19.3834625181277,
124.43855780695)) ;
#51900=CARTESIAN_POINT('Ctrl Pts',(-18.6797419077355,-19.5732941948007,
124.371972025685)) ;
#51901=CARTESIAN_POINT('Ctrl Pts',(-18.4973580638429,-19.3933051143202,
124.612009431647)) ;
#51902=CARTESIAN_POINT('Ctrl Pts',(-18.8570829768545,-19.583274578916,124.484089894838)) ;
#51903=CARTESIAN_POINT('Ctrl Pts',(-18.7190343989905,-19.4032854984355,
124.752157350515)) ;
#51904=CARTESIAN_POINT('Ctrl Pts',(-19.0520979345884,-19.5932930595648,
124.563638386236)) ;
#51905=CARTESIAN_POINT('Ctrl Pts',(-18.9628028394282,-19.4133039790843,
124.851593566146)) ;
#51906=CARTESIAN_POINT('Ctrl Pts',(-19.2551201360957,-19.6031763745651,
124.60795747562)) ;
#51907=CARTESIAN_POINT('Ctrl Pts',(-19.2165815610686,-19.4231872940847,
124.906993129146)) ;
#51908=CARTESIAN_POINT('Ctrl Pts',(-19.4665835366487,-19.6132446716556,
124.616412950505)) ;
#51909=CARTESIAN_POINT('Ctrl Pts',(-19.4809103809794,-19.4332555911751,
124.917562972864)) ;
#51910=CARTESIAN_POINT('Ctrl Pts',(-19.6714432989599,-19.6230747400279,
124.588929074882)) ;
#51911=CARTESIAN_POINT('Ctrl Pts',(-19.7369866665315,-19.4430856595474,
124.883208337484)) ;
#51912=CARTESIAN_POINT('Ctrl Pts',(-19.8731711829206,-19.6331415324963,
124.525058281319)) ;
#51913=CARTESIAN_POINT('Ctrl Pts',(-19.9891462344997,-19.4531524520158,
124.803370269155)) ;
#51914=CARTESIAN_POINT('Ctrl Pts',(-20.0574611220455,-19.6430308659848,
124.428741148867)) ;
#51915=CARTESIAN_POINT('Ctrl Pts',(-20.2195097661445,-19.4630417855043,
124.682973671371)) ;
#51916=CARTESIAN_POINT('Ctrl Pts',(-20.2242497094466,-19.6530329974009,
124.300749095355)) ;
#51917=CARTESIAN_POINT('Ctrl Pts',(-20.4279957457152,-19.4730439169204,
124.522983695242)) ;
#51918=CARTESIAN_POINT('Ctrl Pts',(-20.3653190292274,-19.6629568670219,
124.146990412121)) ;
#51919=CARTESIAN_POINT('Ctrl Pts',(-20.6043330329384,-19.4829677865414,
124.330784900666)) ;
#51920=CARTESIAN_POINT('Ctrl Pts',(-20.4788115638029,-19.6730003825391,
123.968976465865)) ;
#51921=CARTESIAN_POINT('Ctrl Pts',(-20.746198747271,-19.4930113020586,124.108267757333)) ;
#51922=CARTESIAN_POINT('Ctrl Pts',(-20.5586220167799,-19.6828825954274,
123.777121275203)) ;
#51923=CARTESIAN_POINT('Ctrl Pts',(-20.8459623355023,-19.5028935149469,
123.868447779249)) ;
#51924=CARTESIAN_POINT('Ctrl Pts',(-20.6047386809469,-19.6929506726468,
123.570583320886)) ;
#51925=CARTESIAN_POINT('Ctrl Pts',(-20.9036081811708,-19.5129615921663,
123.61027574671)) ;
#51926=CARTESIAN_POINT('Ctrl Pts',(-20.6142646304395,-19.702789177381,123.36393271165)) ;
#51927=CARTESIAN_POINT('Ctrl Pts',(-20.9155157126523,-19.5228000969005,
123.35196100677)) ;
#51928=CARTESIAN_POINT('Ctrl Pts',(-20.5874658464836,-19.7128519458104,
123.154111705371)) ;
#51929=CARTESIAN_POINT('Ctrl Pts',(-20.8820171907135,-19.5328628653299,
123.089685129333)) ;
#51930=CARTESIAN_POINT('Ctrl Pts',(-20.5254497535726,-19.7227489390931,
122.955490377615)) ;
#51931=CARTESIAN_POINT('Ctrl Pts',(-20.8044967775685,-19.5427598586126,
122.841407511821)) ;
#51932=CARTESIAN_POINT('Ctrl Pts',(-20.4301860161421,-19.7326801667279,
122.769710863237)) ;
#51933=CARTESIAN_POINT('Ctrl Pts',(-20.6854165302219,-19.5526910862474,
122.609182603885)) ;
#51934=CARTESIAN_POINT('Ctrl Pts',(-20.3025172159415,-19.74272232537,122.601572700884)) ;
#51935=CARTESIAN_POINT('Ctrl Pts',(-20.5258305093351,-19.5627332448896,
122.39901017822)) ;
#51936=CARTESIAN_POINT('Ctrl Pts',(-20.1500853642892,-19.7526090349011,
122.460258580595)) ;
#51937=CARTESIAN_POINT('Ctrl Pts',(-20.3352897322211,-19.5726199544206,
122.22236696754)) ;
#51938=CARTESIAN_POINT('Ctrl Pts',(-19.973762981087,-19.7626020073297,122.346058634074)) ;
#51939=CARTESIAN_POINT('Ctrl Pts',(-20.1148863728096,-19.5826129268492,
122.079617245332)) ;
#51940=CARTESIAN_POINT('Ctrl Pts',(-19.7811555655468,-19.7725482018663,
122.26467134964)) ;
#51941=CARTESIAN_POINT('Ctrl Pts',(-19.8741264227168,-19.5925591213858,
121.977883228999)) ;
#51942=CARTESIAN_POINT('Ctrl Pts',(-19.577440733495,-19.7824935767178,122.217515204757)) ;
#51943=CARTESIAN_POINT('Ctrl Pts',(-19.6194821905745,-19.6025044962373,
121.918938430687)) ;
#51944=CARTESIAN_POINT('Ctrl Pts',(-19.3663571883107,-19.7925484960777,
122.206654014904)) ;
#51945=CARTESIAN_POINT('Ctrl Pts',(-19.3556280435111,-19.6125594155972,
121.905362356651)) ;
#51946=CARTESIAN_POINT('Ctrl Pts',(-19.1613655130489,-19.8023700155212,
122.231619206292)) ;
#51947=CARTESIAN_POINT('Ctrl Pts',(-19.0993869104664,-19.6223809350407,
121.936569596231)) ;
#51948=CARTESIAN_POINT('Ctrl Pts',(-18.9588961884829,-19.8124357842881,
122.293030078192)) ;
#51949=CARTESIAN_POINT('Ctrl Pts',(-18.8463008166021,-19.6324467038076,
122.013333704134)) ;
#51950=CARTESIAN_POINT('Ctrl Pts',(-18.7732037589491,-19.8223377059431,
122.387203432726)) ;
#51951=CARTESIAN_POINT('Ctrl Pts',(-18.6141847412785,-19.6423486254627,
122.131051370965)) ;
#51952=CARTESIAN_POINT('Ctrl Pts',(-18.6042436666865,-19.8323807647642,
122.513786536381)) ;
#51953=CARTESIAN_POINT('Ctrl Pts',(-18.4029852172294,-19.6523916842837,
122.289280682482)) ;
#51954=CARTESIAN_POINT('Ctrl Pts',(-18.4618641617122,-19.8422867588069,
122.665775366195)) ;
#51955=CARTESIAN_POINT('Ctrl Pts',(-18.2250106930519,-19.6622976783264,
122.479267826183)) ;
#51956=CARTESIAN_POINT('Ctrl Pts',(-18.347162029579,-19.8522245318887,122.840394738477)) ;
#51957=CARTESIAN_POINT('Ctrl Pts',(-18.0816334126947,-19.6722354514082,
122.69754307757)) ;
#51958=CARTESIAN_POINT('Ctrl Pts',(-18.2638779267283,-19.862264895621,123.034345828099)) ;
#51959=CARTESIAN_POINT('Ctrl Pts',(-17.9775290974317,-19.6822758151405,
122.939982086256)) ;
#51960=CARTESIAN_POINT('Ctrl Pts',(-18.2161158206728,-19.8721522393445,
123.236657619917)) ;
#51961=CARTESIAN_POINT('Ctrl Pts',(-17.9178270662773,-19.692163158864,123.192873036768)) ;
#51962=CARTESIAN_POINT('Ctrl Pts',(-18.2037362405876,-19.8821444699132,
123.446346397897)) ;
#51963=CARTESIAN_POINT('Ctrl Pts',(-17.9023535728988,-19.7021553894327,
123.454984271164)) ;
#51964=CARTESIAN_POINT('Ctrl Pts',(-18.2279073020014,-19.8920929976968,
123.65410610834)) ;
#51965=CARTESIAN_POINT('Ctrl Pts',(-17.9325684278091,-19.7121039172163,
123.714684335737)) ;
#51966=CARTESIAN_POINT('Ctrl Pts',(-18.2874238407614,-19.9020297814201,
123.854332451644)) ;
#51967=CARTESIAN_POINT('Ctrl Pts',(-18.0069653211823,-19.7220407009396,
123.964967568161)) ;
#51968=CARTESIAN_POINT('Ctrl Pts',(-18.3810183276697,-19.912012782217,124.042211329903)) ;
#51969=CARTESIAN_POINT('Ctrl Pts',(-18.1239596002325,-19.7320237017366,
124.199815869791)) ;
#51970=CARTESIAN_POINT('Ctrl Pts',(-18.5068566623067,-19.9220566690578,
124.211741307508)) ;
#51971=CARTESIAN_POINT('Ctrl Pts',(-18.2812582375545,-19.7420675885773,
124.411727571379)) ;
#51972=CARTESIAN_POINT('Ctrl Pts',(-18.656625770795,-19.9318846926323,124.354124004755)) ;
#51973=CARTESIAN_POINT('Ctrl Pts',(-18.4684715102243,-19.7518956121519,
124.58970605607)) ;
#51974=CARTESIAN_POINT('Ctrl Pts',(-18.8330935902759,-19.941961940846,124.47126421145)) ;
#51975=CARTESIAN_POINT('Ctrl Pts',(-18.6890566140146,-19.7619728603655,
124.736130030248)) ;
#51976=CARTESIAN_POINT('Ctrl Pts',(-19.0228690100662,-19.9518114961513,
124.55424093318)) ;
#51977=CARTESIAN_POINT('Ctrl Pts',(-18.9262775518615,-19.7718224156708,
124.839850242476)) ;
#51978=CARTESIAN_POINT('Ctrl Pts',(-19.2288113073246,-19.961894204349,124.604205688793)) ;
#51979=CARTESIAN_POINT('Ctrl Pts',(-19.1837052991387,-19.7819051238685,
124.902304787866)) ;
#51980=CARTESIAN_POINT('Ctrl Pts',(-19.434720498365,-19.9717067972754,124.617486778315)) ;
#51981=CARTESIAN_POINT('Ctrl Pts',(-19.4410933758835,-19.791717716795,124.918904855453)) ;
#51982=CARTESIAN_POINT('Ctrl Pts',(-19.645072882955,-19.9817739895334,124.594577329218)) ;
#51983=CARTESIAN_POINT('Ctrl Pts',(-19.704033340018,-19.8017849090529,124.890266579547)) ;
#51984=CARTESIAN_POINT('Ctrl Pts',(-19.8449282407417,-19.991672818996,124.536378177571)) ;
#51985=CARTESIAN_POINT('Ctrl Pts',(-19.9538529269763,-19.8116837385155,
124.81751598121)) ;
#51986=CARTESIAN_POINT('Ctrl Pts',(-20.0345223013733,-20.0017268101862,
124.443044256288)) ;
#51987=CARTESIAN_POINT('Ctrl Pts',(-20.1908446169872,-19.8217377297057,
124.700847328497)) ;
#51988=CARTESIAN_POINT('Ctrl Pts',(-20.2021184222333,-20.0115985349694,
124.320569621367)) ;
#51989=CARTESIAN_POINT('Ctrl Pts',(-20.4003396794263,-19.8316094544889,
124.547752149723)) ;
#51990=CARTESIAN_POINT('Ctrl Pts',(-20.3487795362929,-20.0216689770996,
124.167933913824)) ;
#51991=CARTESIAN_POINT('Ctrl Pts',(-20.583664674412,-19.8416798966191,124.35695666658)) ;
#51992=CARTESIAN_POINT('Ctrl Pts',(-20.4640387398854,-20.0315020555299,
123.996302242053)) ;
#51993=CARTESIAN_POINT('Ctrl Pts',(-20.7277380469989,-19.8515129750494,
124.142415105711)) ;
#51994=CARTESIAN_POINT('Ctrl Pts',(-20.5499655152487,-20.0415325290313,
123.803739463889)) ;
#51995=CARTESIAN_POINT('Ctrl Pts',(-20.835144817367,-19.8615434485508,123.901710971222)) ;
#51996=CARTESIAN_POINT('Ctrl Pts',(-20.6005657766499,-20.0515641283299,
123.59899153)) ;
#51997=CARTESIAN_POINT('Ctrl Pts',(-20.8983935516064,-19.8715750478495,
123.645775745979)) ;
#51998=CARTESIAN_POINT('Ctrl Pts',(-20.6149874000634,-20.0613938293681,
123.392858537114)) ;
#51999=CARTESIAN_POINT('Ctrl Pts',(-20.9164189117006,-19.8814047488876,
123.388108112835)) ;
#52000=CARTESIAN_POINT('Ctrl Pts',(-20.593669608918,-20.0713832674246,123.183927476953)) ;
#52001=CARTESIAN_POINT('Ctrl Pts',(-20.8897697073004,-19.8913941869441,
123.126944309938)) ;
#52002=CARTESIAN_POINT('Ctrl Pts',(-20.5355721040913,-20.0814271706407,
122.980925519128)) ;
#52003=CARTESIAN_POINT('Ctrl Pts',(-20.817146145232,-19.9014380901602,122.873192498194)) ;
#52004=CARTESIAN_POINT('Ctrl Pts',(-20.445542899385,-20.0912486914542,122.795106271871)) ;
#52005=CARTESIAN_POINT('Ctrl Pts',(-20.7046073619337,-19.9112596109737,
122.640918152562)) ;
#52006=CARTESIAN_POINT('Ctrl Pts',(-20.3223921732371,-20.1012844157013,
122.623800659788)) ;
#52007=CARTESIAN_POINT('Ctrl Pts',(-20.5506673335657,-19.9212953352208,
122.426787436303)) ;
#52008=CARTESIAN_POINT('Ctrl Pts',(-20.1711768869751,-20.1113065696338,
122.477056253106)) ;
#52009=CARTESIAN_POINT('Ctrl Pts',(-20.3616469062413,-19.9313174891533,
122.243358309421)) ;
#52010=CARTESIAN_POINT('Ctrl Pts',(-19.9997783644996,-20.1211688013911,
122.360421499363)) ;
#52011=CARTESIAN_POINT('Ctrl Pts',(-20.1473968173766,-19.9411797209106,
122.097565987301)) ;
#52012=CARTESIAN_POINT('Ctrl Pts',(-19.8090973942944,-20.131127871849,122.273937081549)) ;
#52013=CARTESIAN_POINT('Ctrl Pts',(-19.9090443946481,-19.9511387913685,
121.989462309613)) ;
#52014=CARTESIAN_POINT('Ctrl Pts',(-19.6046796800119,-20.1411630442251,
122.221797594559)) ;
#52015=CARTESIAN_POINT('Ctrl Pts',(-19.6535218175709,-19.9611739637447,
121.9242899919)) ;
#52016=CARTESIAN_POINT('Ctrl Pts',(-19.3975520285983,-20.1510434293834,
122.205875090006)) ;
#52017=CARTESIAN_POINT('Ctrl Pts',(-19.3946113132456,-19.9710543489029,
121.904388967312)) ;
#52018=CARTESIAN_POINT('Ctrl Pts',(-19.1871508596279,-20.1611001439773,
122.226434671735)) ;
#52019=CARTESIAN_POINT('Ctrl Pts',(-19.1316102592034,-19.9811110634969,
121.930090607087)) ;
#52020=CARTESIAN_POINT('Ctrl Pts',(-18.9870826370418,-20.1709794125494,
122.28223552978)) ;
#52021=CARTESIAN_POINT('Ctrl Pts',(-18.8815248169901,-19.9909903320689,
121.999843995858)) ;
#52022=CARTESIAN_POINT('Ctrl Pts',(-18.7973905879869,-20.1809703700351,
122.372426720586)) ;
#52023=CARTESIAN_POINT('Ctrl Pts',(-18.6444106248268,-20.0009812895546,
122.112585153675)) ;
#52024=CARTESIAN_POINT('Ctrl Pts',(-18.6256580137942,-20.1910110286703,
122.495170942343)) ;
#52025=CARTESIAN_POINT('Ctrl Pts',(-18.4297462674752,-20.0110219481898,
122.266017180196)) ;
#52026=CARTESIAN_POINT('Ctrl Pts',(-18.4806610276397,-20.2008440083783,
122.642504839744)) ;
#52027=CARTESIAN_POINT('Ctrl Pts',(-18.2485010033221,-20.0208549278978,
122.450186849421)) ;
#52028=CARTESIAN_POINT('Ctrl Pts',(-18.3610435893545,-20.210837141628,122.81520973265)) ;
#52029=CARTESIAN_POINT('Ctrl Pts',(-18.0989811416555,-20.0308480611475,
122.666069459548)) ;
#52030=CARTESIAN_POINT('Ctrl Pts',(-18.2732819316886,-20.2208691940113,
123.00699894088)) ;
#52031=CARTESIAN_POINT('Ctrl Pts',(-17.9892812122869,-20.0408801135309,
122.905806909193)) ;
#52032=CARTESIAN_POINT('Ctrl Pts',(-18.2207950634058,-20.2307344229627,
123.207634736704)) ;
#52033=CARTESIAN_POINT('Ctrl Pts',(-17.9236747633923,-20.0507453424822,
123.156602970146)) ;
#52034=CARTESIAN_POINT('Ctrl Pts',(-18.2031854904533,-20.2406963642059,
123.416330007382)) ;
#52035=CARTESIAN_POINT('Ctrl Pts',(-17.9016652915636,-20.0607072837254,
123.417472522823)) ;
#52036=CARTESIAN_POINT('Ctrl Pts',(-18.2225552242185,-20.2507310792426,
123.626390528993)) ;
#52037=CARTESIAN_POINT('Ctrl Pts',(-17.9258798986461,-20.0707419987622,
123.680047915011)) ;
#52038=CARTESIAN_POINT('Ctrl Pts',(-18.2769648586683,-20.2606168495867,
123.826997944236)) ;
#52039=CARTESIAN_POINT('Ctrl Pts',(-17.9938945219827,-20.0806277691062,
123.930807070549)) ;
#52040=CARTESIAN_POINT('Ctrl Pts',(-18.3669425663381,-20.2706794469754,
124.018428595502)) ;
#52041=CARTESIAN_POINT('Ctrl Pts',(-18.1063688769933,-20.090690366495,124.170094182649)) ;
#52042=CARTESIAN_POINT('Ctrl Pts',(-18.4861705032572,-20.2805298588107,
124.187769337836)) ;
#52043=CARTESIAN_POINT('Ctrl Pts',(-18.2554062653276,-20.1005407783302,
124.381769206499)) ;
#52044=CARTESIAN_POINT('Ctrl Pts',(-18.6352264586599,-20.2905570280966,
124.336825287887)) ;
#52045=CARTESIAN_POINT('Ctrl Pts',(-18.4417280627902,-20.1105679476161,
124.568087271063)) ;
#52046=CARTESIAN_POINT('Ctrl Pts',(-18.8082335054071,-20.3005845088108,
124.457297088272)) ;
#52047=CARTESIAN_POINT('Ctrl Pts',(-18.6579883239994,-20.1205954283303,
124.718674943261)) ;
#52048=CARTESIAN_POINT('Ctrl Pts',(-18.9958279314293,-20.3104275613901,
124.544623627874)) ;
#52049=CARTESIAN_POINT('Ctrl Pts',(-18.8924830332573,-20.1304384809096,
124.827831022369)) ;
#52050=CARTESIAN_POINT('Ctrl Pts',(-19.19866746115,-20.3204214648287,124.599389527813)) ;
#52051=CARTESIAN_POINT('Ctrl Pts',(-19.1460332395822,-20.1404323843482,
124.896285826052)) ;
#52052=CARTESIAN_POINT('Ctrl Pts',(-19.4086704937467,-20.3304485876051,
124.617780480722)) ;
#52053=CARTESIAN_POINT('Ctrl Pts',(-19.4085372828639,-20.1504595071246,
124.919271899914)) ;
#52054=CARTESIAN_POINT('Ctrl Pts',(-19.6158404873169,-20.3403392924971,
124.599938377875)) ;
#52055=CARTESIAN_POINT('Ctrl Pts',(-19.6674999586841,-20.1603502120167,
124.896966576289)) ;
#52056=CARTESIAN_POINT('Ctrl Pts',(-19.8188925643533,-20.3503313193475,
124.546143797245)) ;
#52057=CARTESIAN_POINT('Ctrl Pts',(-19.9213144644297,-20.170342238867,124.829720703372)) ;
#52058=CARTESIAN_POINT('Ctrl Pts',(-20.0086203150577,-20.360277300836,124.458257930678)) ;
#52059=CARTESIAN_POINT('Ctrl Pts',(-20.1584732284019,-20.1802882203555,
124.719860821216)) ;
#52060=CARTESIAN_POINT('Ctrl Pts',(-20.1804782509526,-20.3702244734579,
124.339088999519)) ;
#52061=CARTESIAN_POINT('Ctrl Pts',(-20.3732942472186,-20.1902353929774,
124.570897282549)) ;
#52062=CARTESIAN_POINT('Ctrl Pts',(-20.3303594599015,-20.3802724147841,
124.190244480905)) ;
#52063=CARTESIAN_POINT('Ctrl Pts',(-20.560643830539,-20.2002833343036,124.384839709469)) ;
#52064=CARTESIAN_POINT('Ctrl Pts',(-20.4498405364493,-20.3901200485918,
124.021171300404)) ;
#52065=CARTESIAN_POINT('Ctrl Pts',(-20.7099931678964,-20.2101309681114,
124.173496321079)) ;
#52066=CARTESIAN_POINT('Ctrl Pts',(-20.5397614536319,-20.4000817632769,
123.832042454196)) ;
#52067=CARTESIAN_POINT('Ctrl Pts',(-20.8223918372433,-20.2200926827964,
123.937083946843)) ;
#52068=CARTESIAN_POINT('Ctrl Pts',(-20.5955998308358,-20.4101103961554,
123.628724338267)) ;
#52069=CARTESIAN_POINT('Ctrl Pts',(-20.8921871414343,-20.2301213156749,
123.682935524413)) ;
#52070=CARTESIAN_POINT('Ctrl Pts',(-20.6151216491279,-20.4200207216905,
123.421303306592)) ;
#52071=CARTESIAN_POINT('Ctrl Pts',(-20.9165866655154,-20.2400316412101,
123.423658765386)) ;
#52072=CARTESIAN_POINT('Ctrl Pts',(-20.5988309906371,-20.4299555521623,
123.213073747542)) ;
#52073=CARTESIAN_POINT('Ctrl Pts',(-20.8962205048612,-20.2499664716818,
123.163371888236)) ;
#52074=CARTESIAN_POINT('Ctrl Pts',(-20.5458999153234,-20.4399968845442,
123.008717300108)) ;
#52075=CARTESIAN_POINT('Ctrl Pts',(-20.830054005879,-20.2600078040638,122.907927043648)) ;
#52076=CARTESIAN_POINT('Ctrl Pts',(-20.4596544020495,-20.4498897579831,
122.819465298956)) ;
#52077=CARTESIAN_POINT('Ctrl Pts',(-20.7222442143101,-20.2699006775026,
122.671362855036)) ;
#52078=CARTESIAN_POINT('Ctrl Pts',(-20.3413828244053,-20.459858923801,122.646430648159)) ;
#52079=CARTESIAN_POINT('Ctrl Pts',(-20.5744033926892,-20.2798698433205,
122.455071839325)) ;
#52080=CARTESIAN_POINT('Ctrl Pts',(-20.1937587502541,-20.4698876575175,
122.49593053107)) ;
#52081=CARTESIAN_POINT('Ctrl Pts',(-20.3898674158491,-20.289898577037,122.266945763513)) ;
#52082=CARTESIAN_POINT('Ctrl Pts',(-19.9684033928012,-20.4830801762886,
122.334134273859)) ;
#52083=CARTESIAN_POINT('Ctrl Pts',(-20.1081899356053,-20.3030910958082,
122.064717611177)) ;
#52084=CARTESIAN_POINT('Ctrl Pts',(-19.7027899632007,-20.4964400443313,
122.233638145416)) ;
#52085=CARTESIAN_POINT('Ctrl Pts',(-19.7762004294729,-20.3164509638508,
121.939098029861)) ;
#52086=CARTESIAN_POINT('Ctrl Pts',(-19.4261080021341,-20.5096653814802,
122.206033322011)) ;
#52087=CARTESIAN_POINT('Ctrl Pts',(-19.4302944299203,-20.3296763009997,
121.904585070662)) ;
#52088=CARTESIAN_POINT('Ctrl Pts',(-19.2168158322053,-20.5196466073208,
122.221163224534)) ;
#52089=CARTESIAN_POINT('Ctrl Pts',(-19.1686900557135,-20.3396575268403,
121.923502397254)) ;
#52090=CARTESIAN_POINT('Ctrl Pts',(-19.0123335437991,-20.5296821743037,
122.273082359298)) ;
#52091=CARTESIAN_POINT('Ctrl Pts',(-18.9130849261336,-20.3496930938232,
121.988403504141)) ;
#52092=CARTESIAN_POINT('Ctrl Pts',(-18.8230767712462,-20.5395452522658,
122.357856292057)) ;
#52093=CARTESIAN_POINT('Ctrl Pts',(-18.6765159439737,-20.3595561717853,
122.094373600116)) ;
#52094=CARTESIAN_POINT('Ctrl Pts',(-18.6478204664462,-20.5496155510669,
122.476584772983)) ;
#52095=CARTESIAN_POINT('Ctrl Pts',(-18.4574468060373,-20.3696264705864,
122.242786566347)) ;
#52096=CARTESIAN_POINT('Ctrl Pts',(-18.4992676427898,-20.5594578496347,
122.620634851231)) ;
#52097=CARTESIAN_POINT('Ctrl Pts',(-18.2717579004152,-20.3794687691542,
122.42285107559)) ;
#52098=CARTESIAN_POINT('Ctrl Pts',(-18.3759064700005,-20.5694185478045,
122.789841274378)) ;
#52099=CARTESIAN_POINT('Ctrl Pts',(-18.1175586645594,-20.389429467324,122.634360677971)) ;
#52100=CARTESIAN_POINT('Ctrl Pts',(-18.283462315847,-20.579456581984,122.979538516165)) ;
#52101=CARTESIAN_POINT('Ctrl Pts',(-18.0020059070318,-20.3994675015035,
122.871483585711)) ;
#52102=CARTESIAN_POINT('Ctrl Pts',(-18.2259264092377,-20.5893303188304,
123.179010973159)) ;
#52103=CARTESIAN_POINT('Ctrl Pts',(-17.9300887191848,-20.40934123835,123.120824683872)) ;
#52104=CARTESIAN_POINT('Ctrl Pts',(-18.203489149074,-20.5994021027557,123.389529384903)) ;
#52105=CARTESIAN_POINT('Ctrl Pts',(-17.9020448472088,-20.4194130222752,
123.383973224122)) ;
#52106=CARTESIAN_POINT('Ctrl Pts',(-18.217479141793,-20.6092342239569,123.595777992507)) ;
#52107=CARTESIAN_POINT('Ctrl Pts',(-17.9195350317834,-20.4292451434764,
123.641783391218)) ;
#52108=CARTESIAN_POINT('Ctrl Pts',(-18.2675235725742,-20.6192672479823,
123.800670607276)) ;
#52109=CARTESIAN_POINT('Ctrl Pts',(-17.9820931574861,-20.4392781675018,
123.897898640848)) ;
#52110=CARTESIAN_POINT('Ctrl Pts',(-18.3527418081313,-20.629283128179,123.993235721321)) ;
#52111=CARTESIAN_POINT('Ctrl Pts',(-18.0886185612783,-20.4492940476985,
124.138604141941)) ;
#52112=CARTESIAN_POINT('Ctrl Pts',(-18.4682220622006,-20.6391666472732,
124.165972783851)) ;
#52113=CARTESIAN_POINT('Ctrl Pts',(-18.2329706507137,-20.4591775667927,
124.354523332002)) ;
#52114=CARTESIAN_POINT('Ctrl Pts',(-18.6132891948029,-20.6491570596368,
124.317833664429)) ;
#52115=CARTESIAN_POINT('Ctrl Pts',(-18.4143074090082,-20.4691679791564,
124.544348991668)) ;
#52116=CARTESIAN_POINT('Ctrl Pts',(-18.8379391592786,-20.6624202228403,
124.483045377824)) ;
#52117=CARTESIAN_POINT('Ctrl Pts',(-18.6951170309133,-20.4824311423598,
124.750853866939)) ;
#52118=CARTESIAN_POINT('Ctrl Pts',(-19.1007465541756,-20.6756977930915,
124.586193595685)) ;
#52119=CARTESIAN_POINT('Ctrl Pts',(-19.0235816254098,-20.495708712611,124.879780338638)) ;
#52120=CARTESIAN_POINT('Ctrl Pts',(-19.3792304841943,-20.6890280955981,
124.617392370144)) ;
#52121=CARTESIAN_POINT('Ctrl Pts',(-19.3717460245729,-20.5090390151176,
124.918788838466)) ;
#52122=CARTESIAN_POINT('Ctrl Pts',(-19.5869463660609,-20.6989267774145,
124.604614305006)) ;
#52123=CARTESIAN_POINT('Ctrl Pts',(-19.631378352173,-20.518937696934,124.90281115376)) ;
#52124=CARTESIAN_POINT('Ctrl Pts',(-19.7911870424571,-20.708916292462,124.555761796128)) ;
#52125=CARTESIAN_POINT('Ctrl Pts',(-19.8866819314184,-20.5289272119815,
124.841743662689)) ;
#52126=CARTESIAN_POINT('Ctrl Pts',(-19.9830582667155,-20.718864344237,124.472519591824)) ;
#52127=CARTESIAN_POINT('Ctrl Pts',(-20.1265183760902,-20.5388752637566,
124.737689396251)) ;
#52128=CARTESIAN_POINT('Ctrl Pts',(-20.1575675432332,-20.7288057475155,
124.357539674552)) ;
#52129=CARTESIAN_POINT('Ctrl Pts',(-20.3446556458458,-20.5488166670351,
124.593959706132)) ;
#52130=CARTESIAN_POINT('Ctrl Pts',(-20.3608485699155,-20.7420924122965,
124.165903707027)) ;
#52131=CARTESIAN_POINT('Ctrl Pts',(-20.5987445477632,-20.562103331816,124.354427858085)) ;
#52132=CARTESIAN_POINT('Ctrl Pts',(-20.5464483543658,-20.7587028339513,
123.865472903908)) ;
#52133=CARTESIAN_POINT('Ctrl Pts',(-20.830752172196,-20.5787137534708,123.978870507254)) ;
#52134=CARTESIAN_POINT('Ctrl Pts',(-20.6330141955444,-20.7786140962021,
123.451029395144)) ;
#52135=CARTESIAN_POINT('Ctrl Pts',(-20.9389514262488,-20.5986250157216,
123.460821316343)) ;
#52136=CARTESIAN_POINT('Ctrl Pts',(-20.5730157601791,-20.7985582253669,
123.03120703151)) ;
#52137=CARTESIAN_POINT('Ctrl Pts',(-20.8639502683867,-20.6185691448865,
122.936042849548)) ;
#52138=CARTESIAN_POINT('Ctrl Pts',(-20.3735473898492,-20.8184813879721,
122.657531564048)) ;
#52139=CARTESIAN_POINT('Ctrl Pts',(-20.6146112120165,-20.6384923074917,
122.468951374425)) ;
#52140=CARTESIAN_POINT('Ctrl Pts',(-20.0594536899428,-20.8383715103787,
122.374229560323)) ;
#52141=CARTESIAN_POINT('Ctrl Pts',(-20.2219924332169,-20.6583824298982,
122.114827126758)) ;
#52142=CARTESIAN_POINT('Ctrl Pts',(-19.6652757918242,-20.8583764639788,
122.21454943932)) ;
#52143=CARTESIAN_POINT('Ctrl Pts',(-19.7292685933043,-20.6783873834983,
121.915230361373)) ;
#52144=CARTESIAN_POINT('Ctrl Pts',(-19.2436756516205,-20.8782147209944,
122.198755207655)) ;
#52145=CARTESIAN_POINT('Ctrl Pts',(-19.2022698837424,-20.6982256405139,
121.895490958005)) ;
#52146=CARTESIAN_POINT('Ctrl Pts',(-18.8388276678669,-20.8982090217809,
122.328339296805)) ;
#52147=CARTESIAN_POINT('Ctrl Pts',(-18.6962108823091,-20.7182199413004,
122.05747386277)) ;
#52148=CARTESIAN_POINT('Ctrl Pts',(-18.5045195812377,-20.9180942638254,
122.587219380678)) ;
#52149=CARTESIAN_POINT('Ctrl Pts',(-18.2783285951133,-20.7381051833449,
122.381075560739)) ;
#52150=CARTESIAN_POINT('Ctrl Pts',(-18.2777383338491,-20.9379692103013,
122.943809989293)) ;
#52151=CARTESIAN_POINT('Ctrl Pts',(-17.9948546691342,-20.7579801298208,
122.826813664057)) ;
#52152=CARTESIAN_POINT('Ctrl Pts',(-18.1858465710656,-20.9580022802424,
123.359778806522)) ;
#52153=CARTESIAN_POINT('Ctrl Pts',(-17.8799919146204,-20.7780131997619,
123.34677562979)) ;
#52154=CARTESIAN_POINT('Ctrl Pts',(-18.2415322925881,-20.9778907871428,
123.778943620506)) ;
#52155=CARTESIAN_POINT('Ctrl Pts',(-17.9496011376497,-20.7979017066623,
123.870729922747)) ;
#52156=CARTESIAN_POINT('Ctrl Pts',(-18.4353283530407,-20.9977456469241,
124.154075261847)) ;
#52157=CARTESIAN_POINT('Ctrl Pts',(-18.1918462217504,-20.8177565664436,
124.339642131921)) ;
#52158=CARTESIAN_POINT('Ctrl Pts',(-18.7489158886705,-21.0177964807118,
124.442758777326)) ;
#52159=CARTESIAN_POINT('Ctrl Pts',(-18.5838321067188,-20.8378074002313,
124.700496054301)) ;
#52160=CARTESIAN_POINT('Ctrl Pts',(-19.136624015985,-21.037562422601,124.605282240514)) ;
#52161=CARTESIAN_POINT('Ctrl Pts',(-19.0684642767864,-20.8575733421206,
124.903648312077)) ;
#52162=CARTESIAN_POINT('Ctrl Pts',(-19.5614777516072,-21.0575751540604,
124.626836375853)) ;
#52163=CARTESIAN_POINT('Ctrl Pts',(-19.5995315082897,-20.8775860735799,
124.930591112367)) ;
#52164=CARTESIAN_POINT('Ctrl Pts',(-19.9658070655714,-21.0774679890039,
124.50224819763)) ;
#52165=CARTESIAN_POINT('Ctrl Pts',(-20.1049415620224,-20.8974789085235,
124.77485635548)) ;
#52166=CARTESIAN_POINT('Ctrl Pts',(-20.3038411949213,-21.0973750123435,
124.247672615778)) ;
#52167=CARTESIAN_POINT('Ctrl Pts',(-20.5274834957616,-20.917385931863,124.45663837145)) ;
#52168=CARTESIAN_POINT('Ctrl Pts',(-20.5353184672274,-21.1172902772442,
123.892968169314)) ;
#52169=CARTESIAN_POINT('Ctrl Pts',(-20.8168305786149,-20.9373011967637,
124.013259477154)) ;
#52170=CARTESIAN_POINT('Ctrl Pts',(-20.6318648780347,-21.1373219694039,
123.478162570319)) ;
#52171=CARTESIAN_POINT('Ctrl Pts',(-20.9375148306312,-20.9573328889234,
123.494752291658)) ;
#52172=CARTESIAN_POINT('Ctrl Pts',(-20.5815599947794,-21.1571650159769,
123.059210144883)) ;
#52173=CARTESIAN_POINT('Ctrl Pts',(-20.874635385849,-20.9771759354964,122.971063764394)) ;
#52174=CARTESIAN_POINT('Ctrl Pts',(-20.3915208487305,-21.1770815638767,
122.680835228278)) ;
#52175=CARTESIAN_POINT('Ctrl Pts',(-20.6370889548768,-20.9970924833962,
122.498095047605)) ;
#52176=CARTESIAN_POINT('Ctrl Pts',(-20.083403861949,-21.197013806868,122.389779528303)) ;
#52177=CARTESIAN_POINT('Ctrl Pts',(-20.2519449230364,-21.0170247263875,
122.134274226548)) ;
#52178=CARTESIAN_POINT('Ctrl Pts',(-19.69516019848,-21.2169176416773,122.221394595349)) ;
#52179=CARTESIAN_POINT('Ctrl Pts',(-19.7666424549111,-21.0369285611968,
121.923791009996)) ;
#52180=CARTESIAN_POINT('Ctrl Pts',(-19.2728466795046,-21.2368180418648,
122.195076901029)) ;
#52181=CARTESIAN_POINT('Ctrl Pts',(-19.2387517746074,-21.0568289613843,
121.890890792198)) ;
#52182=CARTESIAN_POINT('Ctrl Pts',(-18.8658292690085,-21.2567677182441,
122.314583734304)) ;
#52183=CARTESIAN_POINT('Ctrl Pts',(-18.7299794805959,-21.0767786377636,
122.040270945646)) ;
#52184=CARTESIAN_POINT('Ctrl Pts',(-18.5243803368553,-21.2767002424645,
122.565662246867)) ;
#52185=CARTESIAN_POINT('Ctrl Pts',(-18.3031667101425,-21.096711161984,122.354115893551)) ;
#52186=CARTESIAN_POINT('Ctrl Pts',(-18.288939857507,-21.2966202514507,122.917786612455)) ;
#52187=CARTESIAN_POINT('Ctrl Pts',(-18.0088633207704,-21.1166311709702,
122.794268679454)) ;
#52188=CARTESIAN_POINT('Ctrl Pts',(-18.1876872131217,-21.3165771576268,
123.329823315717)) ;
#52189=CARTESIAN_POINT('Ctrl Pts',(-17.8822937306169,-21.1365880771464,
123.309313272752)) ;
#52190=CARTESIAN_POINT('Ctrl Pts',(-18.2325869540117,-21.3364629971283,
123.750340197414)) ;
#52191=CARTESIAN_POINT('Ctrl Pts',(-17.9384143244842,-21.1564739166479,
123.834958994866)) ;
#52192=CARTESIAN_POINT('Ctrl Pts',(-18.4190587415346,-21.3564341692642,
124.131743478507)) ;
#52193=CARTESIAN_POINT('Ctrl Pts',(-18.1714993858125,-21.1764450887837,
124.311714842778)) ;
#52194=CARTESIAN_POINT('Ctrl Pts',(-18.721795903564,-21.3762483662486,124.42483382689)) ;
#52195=CARTESIAN_POINT('Ctrl Pts',(-18.5499193846094,-21.1962592857681,
124.678080172102)) ;
#52196=CARTESIAN_POINT('Ctrl Pts',(-19.109257994725,-21.3962295522168,124.59893775336)) ;
#52197=CARTESIAN_POINT('Ctrl Pts',(-19.0342352621433,-21.2162404717363,
124.895714964124)) ;
#52198=CARTESIAN_POINT('Ctrl Pts',(-19.460775786385,-21.4128050576061,124.624819419925)) ;
#52199=CARTESIAN_POINT('Ctrl Pts',(-19.4736619237856,-21.2328159771256,
124.928069751386)) ;
#52200=CARTESIAN_POINT('Ctrl Pts',(-19.7357438512233,-21.4261145054697,
124.572846707991)) ;
#52201=CARTESIAN_POINT('Ctrl Pts',(-19.8173383619621,-21.2461254249892,
124.863112509831)) ;
#52202=CARTESIAN_POINT('Ctrl Pts',(-19.9985231275647,-21.4394822032463,
124.473349278481)) ;
#52203=CARTESIAN_POINT('Ctrl Pts',(-20.1458733463898,-21.2594931227658,
124.73871434383)) ;
#52204=CARTESIAN_POINT('Ctrl Pts',(-20.2833722213967,-21.4559727749122,
124.268798347122)) ;
#52205=CARTESIAN_POINT('Ctrl Pts',(-20.5018728443593,-21.2759836944317,
124.483060829802)) ;
#52206=CARTESIAN_POINT('Ctrl Pts',(-20.5233223205152,-21.475893047245,123.919846821527)) ;
#52207=CARTESIAN_POINT('Ctrl Pts',(-20.8018337603635,-21.2959039667645,
124.046874735423)) ;
#52208=CARTESIAN_POINT('Ctrl Pts',(-20.6120012444767,-21.492510082966,123.577832825468)) ;
#52209=CARTESIAN_POINT('Ctrl Pts',(-20.9126872839273,-21.3125210024855,
123.619326861739)) ;
#52210=CARTESIAN_POINT('Ctrl Pts',(-20.6099160380865,-21.5058009332471,
123.298380195676)) ;
#52211=CARTESIAN_POINT('Ctrl Pts',(-20.9100801366087,-21.3258118527666,
123.27004113055)) ;
#52212=CARTESIAN_POINT('Ctrl Pts',(-20.5720819647299,-21.5157699784016,
123.092270132128)) ;
#52213=CARTESIAN_POINT('Ctrl Pts',(-20.8627908878946,-21.3357808979211,
123.012396956888)) ;
#52214=CARTESIAN_POINT('Ctrl Pts',(-20.499885467458,-21.5256733690351,122.8969600671)) ;
#52215=CARTESIAN_POINT('Ctrl Pts',(-20.7725483588989,-21.3456842885546,
122.768260657527)) ;
#52216=CARTESIAN_POINT('Ctrl Pts',(-20.3931639686196,-21.5357311551478,
122.714452129114)) ;
#52217=CARTESIAN_POINT('Ctrl Pts',(-20.6391462594904,-21.3557420746674,
122.540122041308)) ;
#52218=CARTESIAN_POINT('Ctrl Pts',(-20.2592745444822,-21.5455831917976,
122.556386418772)) ;
#52219=CARTESIAN_POINT('Ctrl Pts',(-20.4717962814078,-21.3655941113171,
122.342544854286)) ;
#52220=CARTESIAN_POINT('Ctrl Pts',(-20.0435430288408,-21.5589483159408,
122.376446565359)) ;
#52221=CARTESIAN_POINT('Ctrl Pts',(-20.2020865685586,-21.3789592354603,
122.117585029482)) ;
#52222=CARTESIAN_POINT('Ctrl Pts',(-19.7882330766326,-21.5721743789038,
122.25842779773)) ;
#52223=CARTESIAN_POINT('Ctrl Pts',(-19.8829746643488,-21.3921852984233,
121.970083355878)) ;
#52224=CARTESIAN_POINT('Ctrl Pts',(-19.512730849252,-21.5854780271861,122.210256078633)) ;
#52225=CARTESIAN_POINT('Ctrl Pts',(-19.5386166648438,-21.4054889467056,
121.909867161661)) ;
#52226=CARTESIAN_POINT('Ctrl Pts',(-19.3026540676817,-21.5954695583491,
122.210450686566)) ;
#52227=CARTESIAN_POINT('Ctrl Pts',(-19.2760167649021,-21.4154804778686,
121.910107183446)) ;
#52228=CARTESIAN_POINT('Ctrl Pts',(-19.0948968921359,-21.6055090061484,
122.247567522211)) ;
#52229=CARTESIAN_POINT('Ctrl Pts',(-19.0163207495948,-21.4255199256679,
121.956500605288)) ;
#52230=CARTESIAN_POINT('Ctrl Pts',(-18.9004687004283,-21.6153527816622,
122.318496927726)) ;
#52231=CARTESIAN_POINT('Ctrl Pts',(-18.7732843138488,-21.4353637011818,
122.04515967745)) ;
#52232=CARTESIAN_POINT('Ctrl Pts',(-18.7185579083454,-21.6253384230499,
122.423213533386)) ;
#52233=CARTESIAN_POINT('Ctrl Pts',(-18.5458944196074,-21.4453493425694,
122.17605303618)) ;
#52234=CARTESIAN_POINT('Ctrl Pts',(-18.5582565476501,-21.6352752074117,
122.557220506057)) ;
#52235=CARTESIAN_POINT('Ctrl Pts',(-18.3455158401512,-21.4552861269312,
122.343559635606)) ;
#52236=CARTESIAN_POINT('Ctrl Pts',(-18.4222459587121,-21.645325041879,122.718871713832)) ;
#52237=CARTESIAN_POINT('Ctrl Pts',(-18.1755004122376,-21.4653359613986,
122.545621876998)) ;
#52238=CARTESIAN_POINT('Ctrl Pts',(-18.3183162605906,-21.6551754913822,
122.898008987532)) ;
#52239=CARTESIAN_POINT('Ctrl Pts',(-18.0455857950081,-21.4751864109017,
122.769542152805)) ;
#52240=CARTESIAN_POINT('Ctrl Pts',(-18.2456911500029,-21.6651475053643,
123.09464249712)) ;
#52241=CARTESIAN_POINT('Ctrl Pts',(-17.9548017335226,-21.4851584248838,
123.015333175384)) ;
#52242=CARTESIAN_POINT('Ctrl Pts',(-18.2082412582699,-21.6751426632114,
123.301442369805)) ;
#52243=CARTESIAN_POINT('Ctrl Pts',(-17.9079865987969,-21.4951535827309,
123.273832595286)) ;
#52244=CARTESIAN_POINT('Ctrl Pts',(-18.2075185297832,-21.6851765895751,
123.512368066183)) ;
#52245=CARTESIAN_POINT('Ctrl Pts',(-17.9070803716444,-21.5051875090946,
123.537489745404)) ;
#52246=CARTESIAN_POINT('Ctrl Pts',(-18.2424799085402,-21.6950322980075,
123.716614333339)) ;
#52247=CARTESIAN_POINT('Ctrl Pts',(-17.9507793756721,-21.515043217527,123.792798278283)) ;
#52248=CARTESIAN_POINT('Ctrl Pts',(-18.3130824839469,-21.7050304473461,
123.914559389374)) ;
#52249=CARTESIAN_POINT('Ctrl Pts',(-18.0390300006346,-21.5250413668657,
124.040230621224)) ;
#52250=CARTESIAN_POINT('Ctrl Pts',(-18.4158251214299,-21.7149298505197,
124.095582065844)) ;
#52251=CARTESIAN_POINT('Ctrl Pts',(-18.1674560176647,-21.5349407700392,
124.266510551727)) ;
#52252=CARTESIAN_POINT('Ctrl Pts',(-18.5504028728454,-21.7249810474082,
124.258463624392)) ;
#52253=CARTESIAN_POINT('Ctrl Pts',(-18.3356760698946,-21.5449919669277,
124.470114255126)) ;
#52254=CARTESIAN_POINT('Ctrl Pts',(-18.7085246366495,-21.734863371221,124.393249383885)) ;
#52255=CARTESIAN_POINT('Ctrl Pts',(-18.5333267196021,-21.5548742907406,
124.638598757011)) ;
#52256=CARTESIAN_POINT('Ctrl Pts',(-18.8894290935753,-21.7448582668776,
124.500128199222)) ;
#52257=CARTESIAN_POINT('Ctrl Pts',(-18.7594560017684,-21.5648691863972,
124.772199668162)) ;
#52258=CARTESIAN_POINT('Ctrl Pts',(-19.0867831919036,-21.7548793662602,
124.573882631177)) ;
#52259=CARTESIAN_POINT('Ctrl Pts',(-19.0061476935039,-21.5748902857797,
124.864395292446)) ;
#52260=CARTESIAN_POINT('Ctrl Pts',(-19.2915499840716,-21.7647866341222,
124.611973404616)) ;
#52261=CARTESIAN_POINT('Ctrl Pts',(-19.2621059878413,-21.5847975536418,
124.912011501778)) ;
#52262=CARTESIAN_POINT('Ctrl Pts',(-19.5004581738309,-21.7747249779475,
124.614356734753)) ;
#52263=CARTESIAN_POINT('Ctrl Pts',(-19.5232414618439,-21.594735897467,124.914993347379)) ;
#52264=CARTESIAN_POINT('Ctrl Pts',(-19.7080148034449,-21.784728397248,124.580333186118)) ;
#52265=CARTESIAN_POINT('Ctrl Pts',(-19.782687760914,-21.6047393167675,124.872466522489)) ;
#52266=CARTESIAN_POINT('Ctrl Pts',(-19.9069801683133,-21.7947629479551,
124.510252770105)) ;
#52267=CARTESIAN_POINT('Ctrl Pts',(-20.0313953526975,-21.6147738674746,
124.784868563619)) ;
#52268=CARTESIAN_POINT('Ctrl Pts',(-20.0874764819987,-21.8046078975607,
124.408942640164)) ;
#52269=CARTESIAN_POINT('Ctrl Pts',(-20.2570175362163,-21.6246188170802,
124.658232944639)) ;
#52270=CARTESIAN_POINT('Ctrl Pts',(-20.2501460126216,-21.8145937396736,
124.276289518342)) ;
#52271=CARTESIAN_POINT('Ctrl Pts',(-20.4603562192985,-21.6346046591931,
124.492418458019)) ;
#52272=CARTESIAN_POINT('Ctrl Pts',(-20.3867706955757,-21.8245285470427,
124.118261781283)) ;
#52273=CARTESIAN_POINT('Ctrl Pts',(-20.6311392303299,-21.6445394665622,
124.294885221629)) ;
#52274=CARTESIAN_POINT('Ctrl Pts',(-20.4950064678875,-21.834586088756,123.936658959793)) ;
#52275=CARTESIAN_POINT('Ctrl Pts',(-20.766436127896,-21.6545970082755,124.067883129763)) ;
#52276=CARTESIAN_POINT('Ctrl Pts',(-20.568620634059,-21.8444076862681,123.743721916865)) ;
#52277=CARTESIAN_POINT('Ctrl Pts',(-20.8584564950463,-21.6644186057876,
123.826712005231)) ;
#52278=CARTESIAN_POINT('Ctrl Pts',(-20.6089246273583,-21.8544639457486,
123.53620346997)) ;
#52279=CARTESIAN_POINT('Ctrl Pts',(-20.9088388980703,-21.6744748652681,
123.567314526505)) ;
#52280=CARTESIAN_POINT('Ctrl Pts',(-20.6121758192455,-21.864403882049,123.327248711453)) ;
#52281=CARTESIAN_POINT('Ctrl Pts',(-20.9129054423695,-21.6844148015685,
123.306120784304)) ;
#52282=CARTESIAN_POINT('Ctrl Pts',(-20.5798268668381,-21.8743110027934,
123.121499920529)) ;
#52283=CARTESIAN_POINT('Ctrl Pts',(-20.8724715627851,-21.6943219223129,
123.048933898869)) ;
#52284=CARTESIAN_POINT('Ctrl Pts',(-20.5112454372603,-21.8843539087187,
122.921820528397)) ;
#52285=CARTESIAN_POINT('Ctrl Pts',(-20.7867471088795,-21.7043648282382,
122.799333949638)) ;
#52286=CARTESIAN_POINT('Ctrl Pts',(-20.4104399306398,-21.8942616898179,
122.739536472857)) ;
#52287=CARTESIAN_POINT('Ctrl Pts',(-20.6607421012304,-21.7142726093374,
122.571477249499)) ;
#52288=CARTESIAN_POINT('Ctrl Pts',(-20.2784482766661,-21.9042720588203,
122.57561542797)) ;
#52289=CARTESIAN_POINT('Ctrl Pts',(-20.4957543257105,-21.7242829783398,
122.366574426196)) ;
#52290=CARTESIAN_POINT('Ctrl Pts',(-20.1193995034889,-21.9143028973891,
122.437148355259)) ;
#52291=CARTESIAN_POINT('Ctrl Pts',(-20.2969450013414,-21.7343138169086,
122.19348877068)) ;
#52292=CARTESIAN_POINT('Ctrl Pts',(-19.9421174960905,-21.9241557370288,
122.33000905002)) ;
#52293=CARTESIAN_POINT('Ctrl Pts',(-20.0753430041324,-21.7441666565483,
122.059562188737)) ;
#52294=CARTESIAN_POINT('Ctrl Pts',(-19.7464337621037,-21.9341437381937,
122.253902994198)) ;
#52295=CARTESIAN_POINT('Ctrl Pts',(-19.8307389892566,-21.7541546577133,
121.964427436232)) ;
#52296=CARTESIAN_POINT('Ctrl Pts',(-19.5417073868984,-21.9440725571729,
122.213164409012)) ;
#52297=CARTESIAN_POINT('Ctrl Pts',(-19.574830987795,-21.7640834766924,121.913501885693)) ;
#52298=CARTESIAN_POINT('Ctrl Pts',(-19.3317819851724,-21.9540602598952,
122.208211065697)) ;
#52299=CARTESIAN_POINT('Ctrl Pts',(-19.3124241042316,-21.7740711794147,
121.907308023859)) ;
#52300=CARTESIAN_POINT('Ctrl Pts',(-19.1232546991255,-21.9640962596979,
122.240283219505)) ;
#52301=CARTESIAN_POINT('Ctrl Pts',(-19.0517647366953,-21.7841071792174,
121.94739595785)) ;
#52302=CARTESIAN_POINT('Ctrl Pts',(-18.9269352967466,-21.9739511294993,
122.306534700964)) ;
#52303=CARTESIAN_POINT('Ctrl Pts',(-18.8063639186395,-21.7939620490188,
122.030208536967)) ;
#52304=CARTESIAN_POINT('Ctrl Pts',(-18.7423427052336,-21.9839505599228,
122.407048270959)) ;
#52305=CARTESIAN_POINT('Ctrl Pts',(-18.5756220535138,-21.8039614794424,
122.155848712689)) ;
#52306=CARTESIAN_POINT('Ctrl Pts',(-18.5795278154634,-21.9938456773881,
122.536588268655)) ;
#52307=CARTESIAN_POINT('Ctrl Pts',(-18.3721015981138,-21.8138565969077,
122.31777256952)) ;
#52308=CARTESIAN_POINT('Ctrl Pts',(-18.4394307306069,-22.0039061709051,
122.695002768727)) ;
#52309=CARTESIAN_POINT('Ctrl Pts',(-18.1969788649172,-21.8239170904246,
122.515789156967)) ;
#52310=CARTESIAN_POINT('Ctrl Pts',(-18.3311666833367,-22.0137556511063,
122.871529628342)) ;
#52311=CARTESIAN_POINT('Ctrl Pts',(-18.0616465447384,-21.8337665706258,
122.736447563555)) ;
#52312=CARTESIAN_POINT('Ctrl Pts',(-18.253333217475,-22.0237821013701,123.067418185129)) ;
#52313=CARTESIAN_POINT('Ctrl Pts',(-17.9643529995753,-21.8437930208896,
122.981307539506)) ;
#52314=CARTESIAN_POINT('Ctrl Pts',(-18.2112421000978,-22.0338133918482,
123.274069161545)) ;
#52315=CARTESIAN_POINT('Ctrl Pts',(-17.9117371291873,-21.8538243113677,
123.239620782799)) ;
#52316=CARTESIAN_POINT('Ctrl Pts',(-18.2053271335064,-22.0436547795,123.480882845049)) ;
#52317=CARTESIAN_POINT('Ctrl Pts',(-17.9043414973988,-21.8636656990195,
123.498138969847)) ;
#52318=CARTESIAN_POINT('Ctrl Pts',(-18.235499498762,-22.0536581803912,123.688988918486)) ;
#52319=CARTESIAN_POINT('Ctrl Pts',(-17.9420552178321,-21.8736690999107,
123.758271923752)) ;
#52320=CARTESIAN_POINT('Ctrl Pts',(-18.3013232908441,-22.0636425631824,
123.88834285791)) ;
#52321=CARTESIAN_POINT('Ctrl Pts',(-18.0243333210938,-21.8836534827019,
124.007465107923)) ;
#52322=CARTESIAN_POINT('Ctrl Pts',(-18.4014559554124,-22.0736816531958,
124.074106712805)) ;
#52323=CARTESIAN_POINT('Ctrl Pts',(-18.1494974493961,-21.8936925727153,
124.239670692976)) ;
#52324=CARTESIAN_POINT('Ctrl Pts',(-18.5295972273494,-22.0835274621049,
124.236682169581)) ;
#52325=CARTESIAN_POINT('Ctrl Pts',(-18.3096733741346,-21.9035383816245,
124.442892027309)) ;
#52326=CARTESIAN_POINT('Ctrl Pts',(-18.6858761362846,-22.0935118849239,
124.376767470781)) ;
#52327=CARTESIAN_POINT('Ctrl Pts',(-18.5050211084145,-21.9135228044435,
124.6180000343)) ;
#52328=CARTESIAN_POINT('Ctrl Pts',(-18.8633080302938,-22.1034515101651,
124.487199990123)) ;
#52329=CARTESIAN_POINT('Ctrl Pts',(-18.7268105925925,-21.9234624296847,
124.756042327827)) ;
#52330=CARTESIAN_POINT('Ctrl Pts',(-19.0591476044493,-22.1134911996838,
124.565868443362)) ;
#52331=CARTESIAN_POINT('Ctrl Pts',(-18.97160932169,-21.9335021192033,124.854379340784)) ;
#52332=CARTESIAN_POINT('Ctrl Pts',(-19.2625612087232,-22.1233793881024,
124.608789289149)) ;
#52333=CARTESIAN_POINT('Ctrl Pts',(-19.2258769015398,-21.9433903076219,
124.908032136519)) ;
#52334=CARTESIAN_POINT('Ctrl Pts',(-19.4724346347167,-22.1333689141044,
124.616203338408)) ;
#52335=CARTESIAN_POINT('Ctrl Pts',(-19.4882188467866,-21.953379833624,124.91730115363)) ;
#52336=CARTESIAN_POINT('Ctrl Pts',(-19.6797404481245,-22.1433274154596,
124.586994703036)) ;
#52337=CARTESIAN_POINT('Ctrl Pts',(-19.7473517520764,-21.9633383349792,
124.880791790202)) ;
#52338=CARTESIAN_POINT('Ctrl Pts',(-19.8778238010788,-22.1532270094633,
124.523101680733)) ;
#52339=CARTESIAN_POINT('Ctrl Pts',(-19.9949571853938,-21.9732379289828,
124.800926502776)) ;
#52340=CARTESIAN_POINT('Ctrl Pts',(-20.0644952954339,-22.1632748975846,
124.424277452298)) ;
#52341=CARTESIAN_POINT('Ctrl Pts',(-20.2282969936015,-21.9832858171041,
124.677397513745)) ;
#52342=CARTESIAN_POINT('Ctrl Pts',(-20.2287857483374,-22.1731703228301,
124.296606248266)) ;
#52343=CARTESIAN_POINT('Ctrl Pts',(-20.4336615726803,-21.9931812423496,
124.517808969355)) ;
#52344=CARTESIAN_POINT('Ctrl Pts',(-20.3707381562611,-22.1832317135307,
124.139823950091)) ;
#52345=CARTESIAN_POINT('Ctrl Pts',(-20.6111028162825,-22.0032426330502,
124.3218322011)) ;
#52346=CARTESIAN_POINT('Ctrl Pts',(-20.4809482851262,-22.1930772972174,
123.964606584726)) ;
#52347=CARTESIAN_POINT('Ctrl Pts',(-20.7488672565389,-22.0130882167369,
124.102810049163)) ;
#52348=CARTESIAN_POINT('Ctrl Pts',(-20.5606363459277,-22.2030402705266,
123.770920839856)) ;
#52349=CARTESIAN_POINT('Ctrl Pts',(-20.8484784323989,-22.0230511900461,
123.860702848423)) ;
#52350=CARTESIAN_POINT('Ctrl Pts',(-20.605498138732,-22.2130659373523,123.564965764745)) ;
#52351=CARTESIAN_POINT('Ctrl Pts',(-20.9045567469638,-22.0330768568719,
123.603259320329)) ;
#52352=CARTESIAN_POINT('Ctrl Pts',(-20.6139362962588,-22.2229804152186,
123.356710312389)) ;
#52353=CARTESIAN_POINT('Ctrl Pts',(-20.9151055480402,-22.0429913347382,
123.342939247578)) ;
#52354=CARTESIAN_POINT('Ctrl Pts',(-20.5862899774463,-22.2329689298936,
123.148530954525)) ;
#52355=CARTESIAN_POINT('Ctrl Pts',(-20.8805485315078,-22.0529798494131,
123.082714706899)) ;
#52356=CARTESIAN_POINT('Ctrl Pts',(-20.5221446354155,-22.2430130408091,
122.947370956092)) ;
#52357=CARTESIAN_POINT('Ctrl Pts',(-20.8003679519831,-22.0630239603286,
122.831264561791)) ;
#52358=CARTESIAN_POINT('Ctrl Pts',(-20.4265781092213,-22.2528411784036,
122.764149083107)) ;
#52359=CARTESIAN_POINT('Ctrl Pts',(-20.6809098954698,-22.0728520979232,
122.602235481541)) ;
#52360=CARTESIAN_POINT('Ctrl Pts',(-20.2975883675018,-22.2629177464626,
122.596160440805)) ;
#52361=CARTESIAN_POINT('Ctrl Pts',(-20.5196736796909,-22.0829286659821,
122.392249516322)) ;
#52362=CARTESIAN_POINT('Ctrl Pts',(-20.1448753794696,-22.2727699083667,
122.456169185964)) ;
#52363=CARTESIAN_POINT('Ctrl Pts',(-20.3287820285072,-22.0927808278863,
122.217258955641)) ;
#52364=CARTESIAN_POINT('Ctrl Pts',(-19.9664229552607,-22.2828428703236,
122.342221971823)) ;
#52365=CARTESIAN_POINT('Ctrl Pts',(-20.1057172726509,-22.1028537898431,
122.074824536813)) ;
#52366=CARTESIAN_POINT('Ctrl Pts',(-19.7753081970072,-22.2926854323265,
122.26285604015)) ;
#52367=CARTESIAN_POINT('Ctrl Pts',(-19.8668228113996,-22.112696351846,121.975615871241)) ;
#52368=CARTESIAN_POINT('Ctrl Pts',(-19.5706672880173,-22.3026658688203,
122.216568225967)) ;
#52369=CARTESIAN_POINT('Ctrl Pts',(-19.6110214816396,-22.1226767883398,
121.91775555396)) ;
#52370=CARTESIAN_POINT('Ctrl Pts',(-19.3602768856682,-22.3126841741447,
122.206883478724)) ;
#52371=CARTESIAN_POINT('Ctrl Pts',(-19.3480335183731,-22.1326950936642,
121.90564896849)) ;
#52372=CARTESIAN_POINT('Ctrl Pts',(-19.1541230507367,-22.3225681380641,
122.233089766057)) ;
#52373=CARTESIAN_POINT('Ctrl Pts',(-19.0903400796923,-22.1425790575837,
121.938406486908)) ;
#52374=CARTESIAN_POINT('Ctrl Pts',(-18.9520588230378,-22.3326340148027,
122.295865398734)) ;
#52375=CARTESIAN_POINT('Ctrl Pts',(-18.8377600204012,-22.1526449343222,
122.016875429247)) ;
#52376=CARTESIAN_POINT('Ctrl Pts',(-18.7681011669116,-22.3424731156636,
122.390486931831)) ;
#52377=CARTESIAN_POINT('Ctrl Pts',(-18.6078114381129,-22.1624840351831,
122.135152615045)) ;
#52378=CARTESIAN_POINT('Ctrl Pts',(-18.5998200970519,-22.3525061985293,
122.517638100478)) ;
#52379=CARTESIAN_POINT('Ctrl Pts',(-18.3974600456383,-22.1725171180488,
122.29409131668)) ;
#52380=CARTESIAN_POINT('Ctrl Pts',(-18.4567024912476,-22.3625278838048,
122.672277268552)) ;
#52381=CARTESIAN_POINT('Ctrl Pts',(-18.2185627412109,-22.1825388033243,
122.487389938012)) ;
#52382=CARTESIAN_POINT('Ctrl Pts',(-18.3441099722616,-22.3723945789033,
122.846470293017)) ;
#52383=CARTESIAN_POINT('Ctrl Pts',(-18.0778211452312,-22.1924054984228,
122.705132096587)) ;
#52384=CARTESIAN_POINT('Ctrl Pts',(-18.2621912773549,-22.3823544686378,
123.039178686657)) ;
#52385=CARTESIAN_POINT('Ctrl Pts',(-17.97542250724,-22.2023653881573,122.946017980709)) ;
#52386=CARTESIAN_POINT('Ctrl Pts',(-18.214942034536,-22.3923894564633,123.2447729843)) ;
#52387=CARTESIAN_POINT('Ctrl Pts',(-17.9163607640091,-22.2124003759828,
123.203010659007)) ;
#52388=CARTESIAN_POINT('Ctrl Pts',(-18.2039207070877,-22.4022761605376,
123.452359252462)) ;
#52389=CARTESIAN_POINT('Ctrl Pts',(-17.9025839572868,-22.2222870800571,
123.462494584702)) ;
#52390=CARTESIAN_POINT('Ctrl Pts',(-18.2296104639163,-22.4123413047705,
123.662360780197)) ;
#52391=CARTESIAN_POINT('Ctrl Pts',(-17.9346959978912,-22.23235222429,123.724996117195)) ;
#52392=CARTESIAN_POINT('Ctrl Pts',(-18.2898035554938,-22.422180595499,123.860294782693)) ;
#52393=CARTESIAN_POINT('Ctrl Pts',(-18.009937769009,-22.2421915150186,123.972415043935)) ;
#52394=CARTESIAN_POINT('Ctrl Pts',(-18.3852909858274,-22.4322431529375,
124.049037318576)) ;
#52395=CARTESIAN_POINT('Ctrl Pts',(-18.1292969689133,-22.252254072457,124.208342841575)) ;
#52396=CARTESIAN_POINT('Ctrl Pts',(-18.5102142780944,-22.4421402041896,
124.215443211625)) ;
#52397=CARTESIAN_POINT('Ctrl Pts',(-18.2854516847869,-22.2621511237091,
124.416351010957)) ;
#52398=CARTESIAN_POINT('Ctrl Pts',(-18.6621688535695,-22.4520714109378,
124.358617696287)) ;
#52399=CARTESIAN_POINT('Ctrl Pts',(-18.4753956188901,-22.2720823304574,
124.595319409378)) ;
#52400=CARTESIAN_POINT('Ctrl Pts',(-18.8387544421233,-22.4621135951567,
124.474321570263)) ;
#52401=CARTESIAN_POINT('Ctrl Pts',(-18.6961275310475,-22.2821245146762,
124.739948983759)) ;
#52402=CARTESIAN_POINT('Ctrl Pts',(-19.0296939400006,-22.4720002232676,
124.556460841573)) ;
#52403=CARTESIAN_POINT('Ctrl Pts',(-18.9348029986145,-22.2920111427871,
124.842623278303)) ;
#52404=CARTESIAN_POINT('Ctrl Pts',(-19.234076559489,-22.4819934958,124.605048925011)) ;
#52405=CARTESIAN_POINT('Ctrl Pts',(-19.1902815584304,-22.3020044153195,
124.903358057962)) ;
#52406=CARTESIAN_POINT('Ctrl Pts',(-19.4427962027987,-22.4919385713414,
124.617281907534)) ;
#52407=CARTESIAN_POINT('Ctrl Pts',(-19.4511817330651,-22.311949490861,124.918648968721)) ;
#52408=CARTESIAN_POINT('Ctrl Pts',(-19.6506180805942,-22.5018881220697,
124.593481317551)) ;
#52409=CARTESIAN_POINT('Ctrl Pts',(-19.7109595709045,-22.3218990415892,
124.888897659365)) ;
#52410=CARTESIAN_POINT('Ctrl Pts',(-19.8528843773795,-22.5119274569177,
124.5332335477)) ;
#52411=CARTESIAN_POINT('Ctrl Pts',(-19.9637921602865,-22.3319383764372,
124.813587576332)) ;
#52412=CARTESIAN_POINT('Ctrl Pts',(-20.0388462005348,-22.5218135958616,
124.440381350932)) ;
#52413=CARTESIAN_POINT('Ctrl Pts',(-20.1962451731678,-22.3418245153811,
124.697521392997)) ;
#52414=CARTESIAN_POINT('Ctrl Pts',(-20.2078788172091,-22.5318117088353,
124.315489125279)) ;
#52415=CARTESIAN_POINT('Ctrl Pts',(-20.407535706162,-22.3518226283548,124.541405526316)) ;
#52416=CARTESIAN_POINT('Ctrl Pts',(-20.3516487618174,-22.5417314711877,
124.164389810808)) ;
#52417=CARTESIAN_POINT('Ctrl Pts',(-20.5872481936241,-22.3617423907073,
124.352530361896)) ;
#52418=CARTESIAN_POINT('Ctrl Pts',(-20.4684258196986,-22.5517708668004,
123.98859191938)) ;
#52419=CARTESIAN_POINT('Ctrl Pts',(-20.7332188477992,-22.3717817863199,
124.13278276774)) ;
#52420=CARTESIAN_POINT('Ctrl Pts',(-20.5517552452748,-22.5616800525887,
123.797660250607)) ;
#52421=CARTESIAN_POINT('Ctrl Pts',(-20.8373803850382,-22.3816909721082,
123.894117096707)) ;
#52422=CARTESIAN_POINT('Ctrl Pts',(-20.6013649615286,-22.5716152367462,
123.594766848094)) ;
#52423=CARTESIAN_POINT('Ctrl Pts',(-20.8993918234264,-22.3916261562657,
123.640499494851)) ;
#52424=CARTESIAN_POINT('Ctrl Pts',(-20.6149297753148,-22.5816562941321,
123.384113634597)) ;
#52425=CARTESIAN_POINT('Ctrl Pts',(-20.9163470245203,-22.4016672136516,
123.377183112354)) ;
#52426=CARTESIAN_POINT('Ctrl Pts',(-20.5922146510685,-22.5915434521654,
123.177488411578)) ;
#52427=CARTESIAN_POINT('Ctrl Pts',(-20.8879521473968,-22.4115543716849,
123.118900643908)) ;
#52428=CARTESIAN_POINT('Ctrl Pts',(-20.5336910768669,-22.6015357318413,
122.975751109046)) ;
#52429=CARTESIAN_POINT('Ctrl Pts',(-20.8147966668249,-22.4215466513608,
122.866729097571)) ;
#52430=CARTESIAN_POINT('Ctrl Pts',(-20.4413703874593,-22.6114842488863,
122.788067427756)) ;
#52431=CARTESIAN_POINT('Ctrl Pts',(-20.6993946934881,-22.4314951684059,
122.632124438187)) ;
#52432=CARTESIAN_POINT('Ctrl Pts',(-20.3182652486574,-22.6214210264567,
122.619313417233)) ;
#52433=CARTESIAN_POINT('Ctrl Pts',(-20.5455120188652,-22.4414319459763,
122.4211820476)) ;
#52434=CARTESIAN_POINT('Ctrl Pts',(-20.1671801256002,-22.6314040626037,
122.473601909739)) ;
#52435=CARTESIAN_POINT('Ctrl Pts',(-20.3566546114606,-22.4514149821232,
122.239043334053)) ;
#52436=CARTESIAN_POINT('Ctrl Pts',(-19.991856607727,-22.6414478141974,122.355972854816)) ;
#52437=CARTESIAN_POINT('Ctrl Pts',(-20.137499793827,-22.4614587337169,122.092007982287)) ;
#52438=CARTESIAN_POINT('Ctrl Pts',(-19.8030570092897,-22.65127634341,122.271939115384)) ;
#52439=CARTESIAN_POINT('Ctrl Pts',(-19.9014984820513,-22.4712872629295,
121.986966332183)) ;
#52440=CARTESIAN_POINT('Ctrl Pts',(-19.5975962709593,-22.6613517043187,
122.220614922131)) ;
#52441=CARTESIAN_POINT('Ctrl Pts',(-19.6446726698257,-22.4813626238382,
121.922812414235)) ;
#52442=CARTESIAN_POINT('Ctrl Pts',(-19.3908522666017,-22.6712083032059,
122.205989042453)) ;
#52443=CARTESIAN_POINT('Ctrl Pts',(-19.3862413607588,-22.4912192227254,
121.904531259396)) ;
#52444=CARTESIAN_POINT('Ctrl Pts',(-19.1804545485629,-22.6812712972238,
122.227705733918)) ;
#52445=CARTESIAN_POINT('Ctrl Pts',(-19.1232446772798,-22.5012822167433,
121.931678446453)) ;
#52446=CARTESIAN_POINT('Ctrl Pts',(-18.9806951570671,-22.6911492315132,
122.284594628893)) ;
#52447=CARTESIAN_POINT('Ctrl Pts',(-18.8735448281078,-22.5111601510327,
122.002791143705)) ;
#52448=CARTESIAN_POINT('Ctrl Pts',(-18.7914526517928,-22.7011498790713,
122.376106438856)) ;
#52449=CARTESIAN_POINT('Ctrl Pts',(-18.6369922198873,-22.5211607985908,
122.117182285902)) ;
#52450=CARTESIAN_POINT('Ctrl Pts',(-18.6222332954635,-22.7110677255094,
122.497984639726)) ;
#52451=CARTESIAN_POINT('Ctrl Pts',(-18.425468334263,-22.5310786450289,122.269531684328)) ;
#52452=CARTESIAN_POINT('Ctrl Pts',(-18.474883672655,-22.721118842515,122.649391564558)) ;
#52453=CARTESIAN_POINT('Ctrl Pts',(-18.2412825267933,-22.5411297620345,
122.458791235445)) ;
#52454=CARTESIAN_POINT('Ctrl Pts',(-18.3579599908217,-22.7309895778256,
122.820875939281)) ;
#52455=CARTESIAN_POINT('Ctrl Pts',(-18.0951286475045,-22.5510004973451,
122.673148447016)) ;
#52456=CARTESIAN_POINT('Ctrl Pts',(-18.270849081835,-22.7410602850686,123.013805427642)) ;
#52457=CARTESIAN_POINT('Ctrl Pts',(-17.98624161006,-22.5610712045881,122.914310640353)) ;
#52458=CARTESIAN_POINT('Ctrl Pts',(-18.2196899669182,-22.7508932925205,
123.214115396645)) ;
#52459=CARTESIAN_POINT('Ctrl Pts',(-17.9222939722818,-22.57090421204,123.16469974728)) ;
#52460=CARTESIAN_POINT('Ctrl Pts',(-18.203176745519,-22.7609237848228,123.42433279345)) ;
#52461=CARTESIAN_POINT('Ctrl Pts',(-17.9016542677263,-22.5809347043423,
123.427471548308)) ;
#52462=CARTESIAN_POINT('Ctrl Pts',(-18.2240311555207,-22.7709553798962,
123.634206914964)) ;
#52463=CARTESIAN_POINT('Ctrl Pts',(-17.9277238839754,-22.5909662994157,
123.689813957238)) ;
#52464=CARTESIAN_POINT('Ctrl Pts',(-18.2794406669794,-22.7807850790344,
123.83327619676)) ;
#52465=CARTESIAN_POINT('Ctrl Pts',(-17.9969878121301,-22.6007959985539,
123.938651312499)) ;
#52466=CARTESIAN_POINT('Ctrl Pts',(-18.3694648397809,-22.790774528916,124.023019043572)) ;
#52467=CARTESIAN_POINT('Ctrl Pts',(-18.1095198727546,-22.6107854484355,
124.175829192089)) ;
#52468=CARTESIAN_POINT('Ctrl Pts',(-18.4921611930021,-22.8008183867317,
124.194863216364)) ;
#52469=CARTESIAN_POINT('Ctrl Pts',(-18.2628916856146,-22.6208293062512,
124.39063324651)) ;
#52470=CARTESIAN_POINT('Ctrl Pts',(-18.6391999982746,-22.8106400773219,
124.339828342554)) ;
#52471=CARTESIAN_POINT('Ctrl Pts',(-18.4466924341392,-22.6306509968414,
124.571839161944)) ;
#52472=CARTESIAN_POINT('Ctrl Pts',(-18.8125751270944,-22.8206751678623,
124.460026469785)) ;
#52473=CARTESIAN_POINT('Ctrl Pts',(-18.6634124376899,-22.6406860873818,
124.722085054606)) ;
#52474=CARTESIAN_POINT('Ctrl Pts',(-19.0042354854205,-22.830699686845,124.547700241937)) ;
#52475=CARTESIAN_POINT('Ctrl Pts',(-18.9029886661836,-22.6507106063645,
124.831675526202)) ;
#52476=CARTESIAN_POINT('Ctrl Pts',(-19.2047392934395,-22.8405595322552,
124.600226995631)) ;
#52477=CARTESIAN_POINT('Ctrl Pts',(-19.153619877724,-22.6605704517747,124.897332264316)) ;
#52478=CARTESIAN_POINT('Ctrl Pts',(-19.4133825738018,-22.8505193085708,
124.617890170241)) ;
#52479=CARTESIAN_POINT('Ctrl Pts',(-19.4144244913009,-22.6705302280904,
124.919409093164)) ;
#52480=CARTESIAN_POINT('Ctrl Pts',(-19.6233229031397,-22.8605475058855,
124.598638239538)) ;
#52481=CARTESIAN_POINT('Ctrl Pts',(-19.6768496651642,-22.680558425405,124.895342097839)) ;
#52482=CARTESIAN_POINT('Ctrl Pts',(-19.8243679055007,-22.8704550481758,
124.544126078897)) ;
#52483=CARTESIAN_POINT('Ctrl Pts',(-19.9281559636795,-22.6904659676953,
124.827199647168)) ;
#52484=CARTESIAN_POINT('Ctrl Pts',(-20.0152757096399,-22.8804876987396,
124.454494142613)) ;
#52485=CARTESIAN_POINT('Ctrl Pts',(-20.1667897462987,-22.7004986182592,
124.715157775253)) ;
#52486=CARTESIAN_POINT('Ctrl Pts',(-20.1852178949266,-22.8903716551663,
124.33491330894)) ;
#52487=CARTESIAN_POINT('Ctrl Pts',(-20.379216821132,-22.7103825746858,124.565679509401)) ;
#52488=CARTESIAN_POINT('Ctrl Pts',(-20.3337523313298,-22.9003613565281,
124.186436934306)) ;
#52489=CARTESIAN_POINT('Ctrl Pts',(-20.5648833311247,-22.7203722760477,
124.380082284195)) ;
#52490=CARTESIAN_POINT('Ctrl Pts',(-20.4544985548872,-22.9104023518042,
124.013286908638)) ;
#52491=CARTESIAN_POINT('Ctrl Pts',(-20.7158142405199,-22.7304132713237,
124.163643560049)) ;
#52492=CARTESIAN_POINT('Ctrl Pts',(-20.5418120177757,-22.9202352410725,
123.825917664307)) ;
#52493=CARTESIAN_POINT('Ctrl Pts',(-20.8249543881168,-22.7402461605921,
123.929430163631)) ;
#52494=CARTESIAN_POINT('Ctrl Pts',(-20.5967197719903,-22.93022839944,123.623135595412)) ;
#52495=CARTESIAN_POINT('Ctrl Pts',(-20.8935867561145,-22.7502393189595,
123.675951817877)) ;
#52496=CARTESIAN_POINT('Ctrl Pts',(-20.6152207366922,-22.9402604417921,
123.413033506782)) ;
#52497=CARTESIAN_POINT('Ctrl Pts',(-20.9167106284998,-22.7602713613116,
123.413324039136)) ;
#52498=CARTESIAN_POINT('Ctrl Pts',(-20.5975204253957,-22.9501256857505,
123.2064025244)) ;
#52499=CARTESIAN_POINT('Ctrl Pts',(-20.8945827855904,-22.77013660527,123.155034786058)) ;
#52500=CARTESIAN_POINT('Ctrl Pts',(-20.5442580745083,-22.9600875769965,
123.003852214581)) ;
#52501=CARTESIAN_POINT('Ctrl Pts',(-20.8280023410754,-22.780098496516,122.901847296174)) ;
#52502=CARTESIAN_POINT('Ctrl Pts',(-20.4556884997879,-22.970122477015,122.812391064617)) ;
#52503=CARTESIAN_POINT('Ctrl Pts',(-20.717288160566,-22.7901333965345,122.662521920289)) ;
#52504=CARTESIAN_POINT('Ctrl Pts',(-20.3372800803288,-22.9800075574296,
122.641575983214)) ;
#52505=CARTESIAN_POINT('Ctrl Pts',(-20.5692752426324,-22.8000184769491,
122.449004039096)) ;
#52506=CARTESIAN_POINT('Ctrl Pts',(-20.1883694042385,-22.9900727295544,
122.491279319789)) ;
#52507=CARTESIAN_POINT('Ctrl Pts',(-20.3831352082,-22.8100836490739,122.261135086105)) ;
#52508=CARTESIAN_POINT('Ctrl Pts',(-20.0193951599007,-22.9999199642779,
122.37164075247)) ;
#52509=CARTESIAN_POINT('Ctrl Pts',(-20.1719153766987,-22.8199308837974,
122.111588554318)) ;
#52510=CARTESIAN_POINT('Ctrl Pts',(-19.8289685430891,-23.0099507755956,
122.281076764927)) ;
#52511=CARTESIAN_POINT('Ctrl Pts',(-19.9338810020407,-22.8299616951152,
121.998385955038)) ;
#52512=CARTESIAN_POINT('Ctrl Pts',(-19.6259877305142,-23.0199603915091,
122.225477205925)) ;
#52513=CARTESIAN_POINT('Ctrl Pts',(-19.6801542546596,-22.8399713110287,
121.928888950518)) ;
#52514=CARTESIAN_POINT('Ctrl Pts',(-19.4185677638405,-23.0298711709128,
122.205958909889)) ;
#52515=CARTESIAN_POINT('Ctrl Pts',(-19.4208786354212,-22.8498820904324,
121.904493618235)) ;
#52516=CARTESIAN_POINT('Ctrl Pts',(-19.2104507212989,-23.0398004367019,
122.222263809827)) ;
#52517=CARTESIAN_POINT('Ctrl Pts',(-19.1607322268029,-22.8598113562214,
121.924877430704)) ;
#52518=CARTESIAN_POINT('Ctrl Pts',(-19.0060800631454,-23.0498431300145,
122.275221685096)) ;
#52519=CARTESIAN_POINT('Ctrl Pts',(-18.9052696005558,-22.869854049534,121.991077325466)) ;
#52520=CARTESIAN_POINT('Ctrl Pts',(-18.816920652705,-23.0597296627092,122.361382751279)) ;
#52521=CARTESIAN_POINT('Ctrl Pts',(-18.6688210507499,-22.8797405822288,
122.098781259374)) ;
#52522=CARTESIAN_POINT('Ctrl Pts',(-18.6435653180198,-23.0697228078125,
122.480041622256)) ;
#52523=CARTESIAN_POINT('Ctrl Pts',(-18.4521283291421,-22.889733727332,122.247107144834)) ;
#52524=CARTESIAN_POINT('Ctrl Pts',(-18.4942067621472,-23.0796684884866,
122.626365687683)) ;
#52525=CARTESIAN_POINT('Ctrl Pts',(-18.2654318574781,-22.8996794080061,
122.430014319101)) ;
#52526=CARTESIAN_POINT('Ctrl Pts',(-18.3721507507593,-23.0896157461133,
122.796186530113)) ;
#52527=CARTESIAN_POINT('Ctrl Pts',(-18.1128639586572,-22.9096266656328,
122.642292140885)) ;
#52528=CARTESIAN_POINT('Ctrl Pts',(-18.280738860759,-23.0996636482348,122.986614485634)) ;
#52529=CARTESIAN_POINT('Ctrl Pts',(-17.9986015570663,-22.9196745677543,
122.880328253764)) ;
#52530=CARTESIAN_POINT('Ctrl Pts',(-18.2247452921894,-23.1095113538565,
123.185929489645)) ;
#52531=CARTESIAN_POINT('Ctrl Pts',(-17.9286121289633,-22.929522273376,123.129473138882)) ;
#52532=CARTESIAN_POINT('Ctrl Pts',(-18.203315371917,-23.1194728204906,123.394243964455)) ;
#52533=CARTESIAN_POINT('Ctrl Pts',(-17.9018275040741,-22.9394837400101,
123.389866643999)) ;
#52534=CARTESIAN_POINT('Ctrl Pts',(-18.2187690231212,-23.1295023737588,
123.604537566451)) ;
#52535=CARTESIAN_POINT('Ctrl Pts',(-17.9211473397104,-22.9495132932783,
123.652733485407)) ;
#52536=CARTESIAN_POINT('Ctrl Pts',(-18.2697520445231,-23.1394092657862,
123.806478018759)) ;
#52537=CARTESIAN_POINT('Ctrl Pts',(-17.9848788715612,-22.9594201853057,
123.905158576466)) ;
#52538=CARTESIAN_POINT('Ctrl Pts',(-18.3549970966278,-23.1493569098992,
123.997428173794)) ;
#52539=CARTESIAN_POINT('Ctrl Pts',(-18.0914378076412,-22.9693678294187,
124.143845240132)) ;
#52540=CARTESIAN_POINT('Ctrl Pts',(-18.4726356234465,-23.1593569529281,
124.171699257656)) ;
#52541=CARTESIAN_POINT('Ctrl Pts',(-18.2384883380865,-22.9793678724476,
124.361682579546)) ;
#52542=CARTESIAN_POINT('Ctrl Pts',(-18.6195515746322,-23.1693957189221,
124.323190189224)) ;
#52543=CARTESIAN_POINT('Ctrl Pts',(-18.4221353270186,-22.9894066384416,
124.551044334256)) ;
#52544=CARTESIAN_POINT('Ctrl Pts',(-18.7866669271075,-23.1792207809443,
124.444609990743)) ;
#52545=CARTESIAN_POINT('Ctrl Pts',(-18.6310313254401,-22.9992317004638,
124.702816918919)) ;
#52546=CARTESIAN_POINT('Ctrl Pts',(-18.9764845901678,-23.1892753282707,
124.537586105056)) ;
#52547=CARTESIAN_POINT('Ctrl Pts',(-18.868304680293,-23.0092862477902,124.819034540594)) ;
#52548=CARTESIAN_POINT('Ctrl Pts',(-19.1774335204479,-23.1992185717199,
124.595200515695)) ;
#52549=CARTESIAN_POINT('Ctrl Pts',(-19.1194917232944,-23.0192294912394,
124.891049871391)) ;
#52550=CARTESIAN_POINT('Ctrl Pts',(-19.3844025852747,-23.2091207433278,
124.617601381638)) ;
#52551=CARTESIAN_POINT('Ctrl Pts',(-19.3782034066437,-23.0291316628473,
124.919048155935)) ;
#52552=CARTESIAN_POINT('Ctrl Pts',(-19.5952575378545,-23.219173578938,124.603384824931)) ;
#52553=CARTESIAN_POINT('Ctrl Pts',(-19.6417720055843,-23.0391844984575,
124.901274622995)) ;
#52554=CARTESIAN_POINT('Ctrl Pts',(-19.796808082773,-23.2290466366235,124.553754633832)) ;
#52555=CARTESIAN_POINT('Ctrl Pts',(-19.8937094830556,-23.049057556143,124.839234191646)) ;
#52556=CARTESIAN_POINT('Ctrl Pts',(-19.9892291256445,-23.2390418981492,
124.469324547835)) ;
#52557=CARTESIAN_POINT('Ctrl Pts',(-20.1342348699008,-23.0590528176687,
124.733693798557)) ;
#52558=CARTESIAN_POINT('Ctrl Pts',(-20.1643902735447,-23.2490672675697,
124.352097383469)) ;
#52559=CARTESIAN_POINT('Ctrl Pts',(-20.3531841876872,-23.0690781870892,
124.587158170286)) ;
#52560=CARTESIAN_POINT('Ctrl Pts',(-20.3146713289308,-23.2589571000963,
124.208405044587)) ;
#52561=CARTESIAN_POINT('Ctrl Pts',(-20.5410358789933,-23.0789680196158,
124.407538040095)) ;
#52562=CARTESIAN_POINT('Ctrl Pts',(-20.4803738058375,-23.2722550709057,
123.98326749613)) ;
#52563=CARTESIAN_POINT('Ctrl Pts',(-20.7481493172849,-23.0922659904252,
124.126127329856)) ;
#52564=CARTESIAN_POINT('Ctrl Pts',(-20.5831671550575,-23.2854534660148,
123.722071678799)) ;
#52565=CARTESIAN_POINT('Ctrl Pts',(-20.8766367897417,-23.1054643855344,
123.799667857784)) ;
#52566=CARTESIAN_POINT('Ctrl Pts',(-20.6148571245368,-23.2988489082943,
123.442305301246)) ;
#52567=CARTESIAN_POINT('Ctrl Pts',(-20.9162580763179,-23.1188598278138,
123.449902418927)) ;
#52568=CARTESIAN_POINT('Ctrl Pts',(-20.6022321518531,-23.3087247465333,
123.235027259948)) ;
#52569=CARTESIAN_POINT('Ctrl Pts',(-20.9004717405058,-23.1287356660528,
123.190816756839)) ;
#52570=CARTESIAN_POINT('Ctrl Pts',(-20.5530100746428,-23.318786149131,123.029348117295)) ;
#52571=CARTESIAN_POINT('Ctrl Pts',(-20.8389416668189,-23.1387970686505,
122.933714938976)) ;
#52572=CARTESIAN_POINT('Ctrl Pts',(-20.470495204662,-23.3286512060661,122.839039896976)) ;
#52573=CARTESIAN_POINT('Ctrl Pts',(-20.7357971608877,-23.1486621255857,
122.695832837286)) ;
#52574=CARTESIAN_POINT('Ctrl Pts',(-20.3548367842642,-23.3386633020149,
122.663215896037)) ;
#52575=CARTESIAN_POINT('Ctrl Pts',(-20.5912157871722,-23.1586742215345,
122.476050346765)) ;
#52576=CARTESIAN_POINT('Ctrl Pts',(-20.1631967914319,-23.3519406111604,
122.460187922931)) ;
#52577=CARTESIAN_POINT('Ctrl Pts',(-20.3516936595275,-23.1719515306799,
122.222286259261)) ;
#52578=CARTESIAN_POINT('Ctrl Pts',(-19.8630377268875,-23.3685396366677,
122.274632914981)) ;
#52579=CARTESIAN_POINT('Ctrl Pts',(-19.9764398068349,-23.1885505561872,
121.990323874469)) ;
#52580=CARTESIAN_POINT('Ctrl Pts',(-19.517487437228,-23.3851386847007,122.202591928007)) ;
#52581=CARTESIAN_POINT('Ctrl Pts',(-19.5445846288438,-23.2051496042202,
121.900290049093)) ;
#52582=CARTESIAN_POINT('Ctrl Pts',(-19.23951312528,-23.3983820967316,122.217815968059)) ;
#52583=CARTESIAN_POINT('Ctrl Pts',(-19.1970504323452,-23.2183930162512,
121.919316506711)) ;
#52584=CARTESIAN_POINT('Ctrl Pts',(-19.0339916765018,-23.4084195244201,
122.265667627133)) ;
#52585=CARTESIAN_POINT('Ctrl Pts',(-18.9401631490547,-23.2284304439396,
121.979134289516)) ;
#52586=CARTESIAN_POINT('Ctrl Pts',(-18.8424913044911,-23.4183238263757,
122.347410808801)) ;
#52587=CARTESIAN_POINT('Ctrl Pts',(-18.7007825061689,-23.2383347458952,
122.081317818087)) ;
#52588=CARTESIAN_POINT('Ctrl Pts',(-18.6084602838952,-23.4315906663508,
122.499189778994)) ;
#52589=CARTESIAN_POINT('Ctrl Pts',(-18.408261872732,-23.2516015858704,122.271030307372)) ;
#52590=CARTESIAN_POINT('Ctrl Pts',(-18.3717345959788,-23.4482168644408,
122.761707590166)) ;
#52591=CARTESIAN_POINT('Ctrl Pts',(-18.1123399886004,-23.2682277839603,
122.599191193648)) ;
#52592=CARTESIAN_POINT('Ctrl Pts',(-18.2123565640676,-23.4681359798242,
123.154114455554)) ;
#52593=CARTESIAN_POINT('Ctrl Pts',(-17.9131297579677,-23.2881468993437,
123.089717711746)) ;
#52594=CARTESIAN_POINT('Ctrl Pts',(-18.1988208253406,-23.4847424029584,
123.506996953541)) ;
#52595=CARTESIAN_POINT('Ctrl Pts',(-17.8962057485835,-23.3047533224779,
123.530754190481)) ;
#52596=CARTESIAN_POINT('Ctrl Pts',(-18.2607588524776,-23.4980386234541,
123.779530753442)) ;
#52597=CARTESIAN_POINT('Ctrl Pts',(-17.9736383078827,-23.3180495429737,
123.871481315145)) ;
#52598=CARTESIAN_POINT('Ctrl Pts',(-18.3683238744161,-23.5113074557956,
124.036997547401)) ;
#52599=CARTESIAN_POINT('Ctrl Pts',(-18.1080876893351,-23.3313183753151,
124.193291225541)) ;
#52600=CARTESIAN_POINT('Ctrl Pts',(-18.585515956159,-23.5279987038287,124.31755527357)) ;
#52601=CARTESIAN_POINT('Ctrl Pts',(-18.3795904844463,-23.3480096233482,
124.544002089777)) ;
#52602=CARTESIAN_POINT('Ctrl Pts',(-18.9413317824027,-23.5478084355015,
124.543077586913)) ;
#52603=CARTESIAN_POINT('Ctrl Pts',(-18.824358003802,-23.367819355021,124.825895671739)) ;
#52604=CARTESIAN_POINT('Ctrl Pts',(-19.3559796542478,-23.56778604283,124.635208528437)) ;
#52605=CARTESIAN_POINT('Ctrl Pts',(-19.3426692477334,-23.3877969623496,
124.941057197869)) ;
#52606=CARTESIAN_POINT('Ctrl Pts',(-19.7759608022422,-23.5877123518879,
124.579685890579)) ;
#52607=CARTESIAN_POINT('Ctrl Pts',(-19.8676443127225,-23.4077232714074,
124.871649885416)) ;
#52608=CARTESIAN_POINT('Ctrl Pts',(-20.1505472402133,-23.6075292120526,
124.386491448277)) ;
#52609=CARTESIAN_POINT('Ctrl Pts',(-20.3358743902777,-23.4275401315721,
124.630155280744)) ;
#52610=CARTESIAN_POINT('Ctrl Pts',(-20.4401428515061,-23.6276290276466,
124.072390207339)) ;
#52611=CARTESIAN_POINT('Ctrl Pts',(-20.6978674017851,-23.4476399471661,
124.237525821871)) ;
#52612=CARTESIAN_POINT('Ctrl Pts',(-20.6026657871358,-23.6473859915291,
123.684825873049)) ;
#52613=CARTESIAN_POINT('Ctrl Pts',(-20.9010174943812,-23.4673969110487,
123.753071870161)) ;
#52614=CARTESIAN_POINT('Ctrl Pts',(-20.6242876059637,-23.6674229175986,
123.259481688023)) ;
#52615=CARTESIAN_POINT('Ctrl Pts',(-20.9280426937593,-23.4874338371181,
123.221391133689)) ;
#52616=CARTESIAN_POINT('Ctrl Pts',(-20.4997957023964,-23.6872924999801,
122.855645078802)) ;
#52617=CARTESIAN_POINT('Ctrl Pts',(-20.7724260969431,-23.5073034194996,
122.716597558687)) ;
#52618=CARTESIAN_POINT('Ctrl Pts',(-20.2454865673464,-23.7071970717333,
122.517448321673)) ;
#52619=CARTESIAN_POINT('Ctrl Pts',(-20.4545393934971,-23.5272079912528,
122.293853596945)) ;
#52620=CARTESIAN_POINT('Ctrl Pts',(-19.8900271158853,-23.7271496739318,
122.285727883188)) ;
#52621=CARTESIAN_POINT('Ctrl Pts',(-20.0102149505342,-23.5471605934513,
122.004204373787)) ;
#52622=CARTESIAN_POINT('Ctrl Pts',(-19.4778464728188,-23.747059164902,122.189596892363)) ;
#52623=CARTESIAN_POINT('Ctrl Pts',(-19.4949902617054,-23.5670700844216,
121.884042017014)) ;
#52624=CARTESIAN_POINT('Ctrl Pts',(-19.0585021845433,-23.7669105336015,
122.238587168872)) ;
#52625=CARTESIAN_POINT('Ctrl Pts',(-18.9708122647086,-23.586921453121,121.945279500449)) ;
#52626=CARTESIAN_POINT('Ctrl Pts',(-18.6771515985997,-23.7869907297375,
122.43039174872)) ;
#52627=CARTESIAN_POINT('Ctrl Pts',(-18.4941229339348,-23.607001649257,122.185035924184)) ;
#52628=CARTESIAN_POINT('Ctrl Pts',(-18.3880786328134,-23.8067916733129,
122.736642917923)) ;
#52629=CARTESIAN_POINT('Ctrl Pts',(-18.1327837983887,-23.6268025928324,
122.567847534477)) ;
#52630=CARTESIAN_POINT('Ctrl Pts',(-18.2185138748618,-23.8267756498224,
123.126183556028)) ;
#52631=CARTESIAN_POINT('Ctrl Pts',(-17.920826926211,-23.6467865693419,123.054772698321)) ;
#52632=CARTESIAN_POINT('Ctrl Pts',(-18.1928000702527,-23.846691612798,123.54886807584)) ;
#52633=CARTESIAN_POINT('Ctrl Pts',(-17.8886839108745,-23.6667025323175,
123.583127051789)) ;
#52634=CARTESIAN_POINT('Ctrl Pts',(-18.3114981929088,-23.8665620476199,
123.954437415859)) ;
#52635=CARTESIAN_POINT('Ctrl Pts',(-18.0370543004863,-23.6865729671394,
124.090087584611)) ;
#52636=CARTESIAN_POINT('Ctrl Pts',(-18.5641851710754,-23.886612332853,124.297650548748)) ;
#52637=CARTESIAN_POINT('Ctrl Pts',(-18.352912073492,-23.7066232523725,124.519105466917)) ;
#52638=CARTESIAN_POINT('Ctrl Pts',(-18.9138459519034,-23.9063863016123,
124.531438448419)) ;
#52639=CARTESIAN_POINT('Ctrl Pts',(-18.789984541193,-23.7263972211318,124.811340608037)) ;
#52640=CARTESIAN_POINT('Ctrl Pts',(-19.327728107229,-23.9264427597318,124.633511754983)) ;
#52641=CARTESIAN_POINT('Ctrl Pts',(-19.3073372095481,-23.7464536792514,
124.938934907489)) ;
#52642=CARTESIAN_POINT('Ctrl Pts',(-19.7463440551213,-23.9462376427228,
124.588636490226)) ;
#52643=CARTESIAN_POINT('Ctrl Pts',(-19.8306051755594,-23.7662485622424,
124.882843707718)) ;
#52644=CARTESIAN_POINT('Ctrl Pts',(-20.128134455108,-23.9662042980252,124.403168082798)) ;
#52645=CARTESIAN_POINT('Ctrl Pts',(-20.3078444226172,-23.7862152175447,
124.651011447884)) ;
#52646=CARTESIAN_POINT('Ctrl Pts',(-20.4232185491835,-23.9861632681017,
124.098054033906)) ;
#52647=CARTESIAN_POINT('Ctrl Pts',(-20.6767016463538,-23.8061741876212,
124.269621393474)) ;
#52648=CARTESIAN_POINT('Ctrl Pts',(-20.5961622014183,-24.0060593556918,
123.711998667547)) ;
#52649=CARTESIAN_POINT('Ctrl Pts',(-20.8928840689229,-23.8260702752113,
123.787054530361)) ;
#52650=CARTESIAN_POINT('Ctrl Pts',(-20.6274889819743,-24.0259575256034,
123.290106766545)) ;
#52651=CARTESIAN_POINT('Ctrl Pts',(-20.9320464016076,-23.8459684451229,
123.2596908132)) ;
#52652=CARTESIAN_POINT('Ctrl Pts',(-20.513337763902,-24.0458633609705,122.882506566483)) ;
#52653=CARTESIAN_POINT('Ctrl Pts',(-20.7893616370779,-23.86587428049,122.75019007212)) ;
#52654=CARTESIAN_POINT('Ctrl Pts',(-20.266431677999,-24.0658132859084,122.537627079781)) ;
#52655=CARTESIAN_POINT('Ctrl Pts',(-20.4807327589992,-23.8858242054279,
122.319088447541)) ;
#52656=CARTESIAN_POINT('Ctrl Pts',(-19.9180548383199,-24.0856924758188,
122.298181469176)) ;
#52657=CARTESIAN_POINT('Ctrl Pts',(-20.0452649317032,-23.9057033953383,
122.019778092057)) ;
#52658=CARTESIAN_POINT('Ctrl Pts',(-19.5069122512383,-24.1056738000994,
122.191249797151)) ;
#52659=CARTESIAN_POINT('Ctrl Pts',(-19.5313379425127,-23.9256847196189,
121.886108845858)) ;
#52660=CARTESIAN_POINT('Ctrl Pts',(-19.0849454561733,-24.1256035843077,
122.231166566416)) ;
#52661=CARTESIAN_POINT('Ctrl Pts',(-19.0038793189648,-23.9456145038272,
121.936000230664)) ;
#52662=CARTESIAN_POINT('Ctrl Pts',(-18.7022509031181,-24.1455235736985,
122.412432300618)) ;
#52663=CARTESIAN_POINT('Ctrl Pts',(-18.5255093849516,-23.965534493218,122.162577000511)) ;
#52664=CARTESIAN_POINT('Ctrl Pts',(-18.4045331289834,-24.1653787690525,
122.711900017558)) ;
#52665=CARTESIAN_POINT('Ctrl Pts',(-18.1533588422071,-23.985389688572,122.536910497454)) ;
#52666=CARTESIAN_POINT('Ctrl Pts',(-18.2256300026401,-24.1854247707119,
123.098661615411)) ;
#52667=CARTESIAN_POINT('Ctrl Pts',(-17.9297252153932,-24.0054356902314,
123.020349675048)) ;
#52668=CARTESIAN_POINT('Ctrl Pts',(-18.1956840876194,-24.2019245179217,
123.448290706154)) ;
#52669=CARTESIAN_POINT('Ctrl Pts',(-17.8922881635453,-24.0219354374412,
123.457418896118)) ;
#52670=CARTESIAN_POINT('Ctrl Pts',(-18.244751099481,-24.2153131223698,123.725437756677)) ;
#52671=CARTESIAN_POINT('Ctrl Pts',(-17.9536182367235,-24.0353240418893,
123.803823185487)) ;
#52672=CARTESIAN_POINT('Ctrl Pts',(-18.3158010212771,-24.2251749507047,
123.92021291796)) ;
#52673=CARTESIAN_POINT('Ctrl Pts',(-18.0424306540763,-24.0451858702242,
124.047300970939)) ;
#52674=CARTESIAN_POINT('Ctrl Pts',(-18.4201246805275,-24.2351410934622,
124.101932284297)) ;
#52675=CARTESIAN_POINT('Ctrl Pts',(-18.1728224346428,-24.0551520129818,
124.274441107822)) ;
#52676=CARTESIAN_POINT('Ctrl Pts',(-18.600479700421,-24.2485028395872,124.317163919076)) ;
#52677=CARTESIAN_POINT('Ctrl Pts',(-18.3983154768799,-24.0685137591067,
124.543527593529)) ;
#52678=CARTESIAN_POINT('Ctrl Pts',(-18.8864879871126,-24.2649571685423,
124.518993893139)) ;
#52679=CARTESIAN_POINT('Ctrl Pts',(-18.7557534013296,-24.0849680880618,
124.795766078485)) ;
#52680=CARTESIAN_POINT('Ctrl Pts',(-19.2302450355489,-24.2817244135906,
124.612794594497)) ;
#52681=CARTESIAN_POINT('Ctrl Pts',(-19.1855079887439,-24.1017353331101,
124.913045707211)) ;
#52682=CARTESIAN_POINT('Ctrl Pts',(-19.5076006939437,-24.2949109788646,
124.613694249436)) ;
#52683=CARTESIAN_POINT('Ctrl Pts',(-19.5321625872062,-24.1149218983841,
124.914163508311)) ;
#52684=CARTESIAN_POINT('Ctrl Pts',(-19.714585996907,-24.3049004376092,124.57853472076)) ;
#52685=CARTESIAN_POINT('Ctrl Pts',(-19.7909027433766,-24.1249113571287,
124.870218955484)) ;
#52686=CARTESIAN_POINT('Ctrl Pts',(-19.9117282679633,-24.3148542100903,
124.508226632481)) ;
#52687=CARTESIAN_POINT('Ctrl Pts',(-20.0373293988633,-24.1348651296098,
124.782335916297)) ;
#52688=CARTESIAN_POINT('Ctrl Pts',(-20.0952429868065,-24.324902026623,124.40366816945)) ;
#52689=CARTESIAN_POINT('Ctrl Pts',(-20.2667248445847,-24.1449129461425,
124.651640371413)) ;
#52690=CARTESIAN_POINT('Ctrl Pts',(-20.2546683283464,-24.3347435597455,
124.271759801232)) ;
#52691=CARTESIAN_POINT('Ctrl Pts',(-20.4660081193213,-24.154754479265,124.486757064612)) ;
#52692=CARTESIAN_POINT('Ctrl Pts',(-20.3910452829839,-24.3447298019652,
124.112189741865)) ;
#52693=CARTESIAN_POINT('Ctrl Pts',(-20.6364815532312,-24.1647407214847,
124.287296273957)) ;
#52694=CARTESIAN_POINT('Ctrl Pts',(-20.4972397987561,-24.3546664253901,
123.932255968931)) ;
#52695=CARTESIAN_POINT('Ctrl Pts',(-20.7692271458693,-24.1746773449096,
124.062380425014)) ;
#52696=CARTESIAN_POINT('Ctrl Pts',(-20.5712954604918,-24.3647163027731,
123.73440257886)) ;
#52697=CARTESIAN_POINT('Ctrl Pts',(-20.8617993884923,-24.1847272222926,
123.815064619635)) ;
#52698=CARTESIAN_POINT('Ctrl Pts',(-20.6092665986412,-24.3745667415506,
123.530810616257)) ;
#52699=CARTESIAN_POINT('Ctrl Pts',(-20.9092661002677,-24.1945776610702,
123.560575071878)) ;
#52700=CARTESIAN_POINT('Ctrl Pts',(-20.6118828892727,-24.3845387555194,
123.321210192378)) ;
#52701=CARTESIAN_POINT('Ctrl Pts',(-20.9125392725062,-24.2045496750389,
123.298574461704)) ;
#52702=CARTESIAN_POINT('Ctrl Pts',(-20.5779494879227,-24.3945339241455,
123.113804511949)) ;
#52703=CARTESIAN_POINT('Ctrl Pts',(-20.8701252719288,-24.214544843665,123.03931683066)) ;
#52704=CARTESIAN_POINT('Ctrl Pts',(-20.5080285322928,-24.4045678074067,
122.914803419106)) ;
#52705=CARTESIAN_POINT('Ctrl Pts',(-20.7827267212142,-24.2245787269262,
122.790564493733)) ;
#52706=CARTESIAN_POINT('Ctrl Pts',(-20.4067104297543,-24.41442367747,122.734046050817)) ;
#52707=CARTESIAN_POINT('Ctrl Pts',(-20.6560814229748,-24.2344345969895,
122.564616215034)) ;
#52708=CARTESIAN_POINT('Ctrl Pts',(-20.2739437816179,-24.4244212233872,
122.571137981273)) ;
#52709=CARTESIAN_POINT('Ctrl Pts',(-20.4901252099915,-24.2444321429067,
122.360979293762)) ;
#52710=CARTESIAN_POINT('Ctrl Pts',(-20.1163503321144,-24.4343293502864,
122.434915065284)) ;
#52711=CARTESIAN_POINT('Ctrl Pts',(-20.2931350358495,-24.254340269806,122.190698398369)) ;
#52712=CARTESIAN_POINT('Ctrl Pts',(-19.9358381554827,-24.4443397218086,
122.326707961461)) ;
#52713=CARTESIAN_POINT('Ctrl Pts',(-20.0674961655237,-24.2643506413281,
122.055437128018)) ;
#52714=CARTESIAN_POINT('Ctrl Pts',(-19.7387342050816,-24.454370164556,122.251783176735)) ;
#52715=CARTESIAN_POINT('Ctrl Pts',(-19.8211172047794,-24.2743810840756,
121.961778537546)) ;
#52716=CARTESIAN_POINT('Ctrl Pts',(-19.5354521664302,-24.4642181171093,
122.212461214448)) ;
#52717=CARTESIAN_POINT('Ctrl Pts',(-19.5670147879019,-24.2842290366288,
121.91262331826)) ;
#52718=CARTESIAN_POINT('Ctrl Pts',(-19.3239551652899,-24.4742807861303,
122.208794045191)) ;
#52719=CARTESIAN_POINT('Ctrl Pts',(-19.3026436245649,-24.2942917056498,
121.908036630812)) ;
#52720=CARTESIAN_POINT('Ctrl Pts',(-19.1185123192759,-24.4841751615942,
122.241504281932)) ;
#52721=CARTESIAN_POINT('Ctrl Pts',(-19.045839313324,-24.3041860811137,121.948921771681)) ;
#52722=CARTESIAN_POINT('Ctrl Pts',(-18.9207873898694,-24.4941169599123,
122.309170126325)) ;
#52723=CARTESIAN_POINT('Ctrl Pts',(-18.7986820357959,-24.3141278794319,
122.033501629662)) ;
#52724=CARTESIAN_POINT('Ctrl Pts',(-18.7366115575641,-24.5041194536396,
122.410711220208)) ;
#52725=CARTESIAN_POINT('Ctrl Pts',(-18.5684608874913,-24.3241303731592,
122.160425707756)) ;
#52726=CARTESIAN_POINT('Ctrl Pts',(-18.5725769314898,-24.5141542521466,
122.543347790697)) ;
#52727=CARTESIAN_POINT('Ctrl Pts',(-18.3634159133862,-24.3341651716661,
122.326219304036)) ;
#52728=CARTESIAN_POINT('Ctrl Pts',(-18.4364059179355,-24.5239991361259,
122.699231885075)) ;
#52729=CARTESIAN_POINT('Ctrl Pts',(-18.1931997742607,-24.3440100556455,
122.521073096057)) ;
#52730=CARTESIAN_POINT('Ctrl Pts',(-18.3275230682562,-24.533984992944,122.878683232876)) ;
#52731=CARTESIAN_POINT('Ctrl Pts',(-18.057093903249,-24.3539959124635,122.745386068075)) ;
#52732=CARTESIAN_POINT('Ctrl Pts',(-18.2516769257629,-24.5439198071187,
123.073327761756)) ;
#52733=CARTESIAN_POINT('Ctrl Pts',(-17.9622837119148,-24.3639307266383,
122.988691099146)) ;
#52734=CARTESIAN_POINT('Ctrl Pts',(-18.2104726947077,-24.5539773069041,
123.280683690247)) ;
#52735=CARTESIAN_POINT('Ctrl Pts',(-17.9107758864736,-24.3739882264236,
123.247885387982)) ;
#52736=CARTESIAN_POINT('Ctrl Pts',(-18.2056888743538,-24.5637990653224,
123.487134857633)) ;
#52737=CARTESIAN_POINT('Ctrl Pts',(-17.9047935450164,-24.3838099848419,
123.505950068642)) ;
#52738=CARTESIAN_POINT('Ctrl Pts',(-18.2371668828863,-24.5738547231064,
123.696162130977)) ;
#52739=CARTESIAN_POINT('Ctrl Pts',(-17.9441385893979,-24.3938656426259,
123.767234420961)) ;
#52740=CARTESIAN_POINT('Ctrl Pts',(-18.3040695591823,-24.5837969052864,
123.894192986261)) ;
#52741=CARTESIAN_POINT('Ctrl Pts',(-18.0277646256718,-24.4038078248059,
124.014774122558)) ;
#52742=CARTESIAN_POINT('Ctrl Pts',(-18.4034039808886,-24.5937021139811,
124.07720850749)) ;
#52743=CARTESIAN_POINT('Ctrl Pts',(-18.1519307757942,-24.4137130335006,
124.243545142441)) ;
#52744=CARTESIAN_POINT('Ctrl Pts',(-18.5348467278453,-24.6037439049435,
124.242401635363)) ;
#52745=CARTESIAN_POINT('Ctrl Pts',(-18.316232248357,-24.4237548244631,124.450038001012)) ;
#52746=CARTESIAN_POINT('Ctrl Pts',(-18.6908591823526,-24.6136516794158,
124.380420797567)) ;
#52747=CARTESIAN_POINT('Ctrl Pts',(-18.5112465950193,-24.4336625989353,
124.622564118321)) ;
#52748=CARTESIAN_POINT('Ctrl Pts',(-18.8701202015806,-24.6236631796434,
124.490724089556)) ;
#52749=CARTESIAN_POINT('Ctrl Pts',(-18.7353216881692,-24.4436740991629,
124.760445263061)) ;
#52750=CARTESIAN_POINT('Ctrl Pts',(-19.0663816760572,-24.6336959400361,
124.567979438688)) ;
#52751=CARTESIAN_POINT('Ctrl Pts',(-18.9806475911172,-24.4537068595556,
124.8570167095)) ;
#52752=CARTESIAN_POINT('Ctrl Pts',(-19.2692552137906,-24.643546509171,124.609578863151)) ;
#52753=CARTESIAN_POINT('Ctrl Pts',(-19.2342398512218,-24.4635574286905,
124.909018470008)) ;
#52754=CARTESIAN_POINT('Ctrl Pts',(-19.4791376987757,-24.6535351187009,
124.615797717259)) ;
#52755=CARTESIAN_POINT('Ctrl Pts',(-19.4965930730634,-24.4735460382204,
124.916794313041)) ;
#52756=CARTESIAN_POINT('Ctrl Pts',(-19.6856874087961,-24.663463774725,124.585656540183)) ;
#52757=CARTESIAN_POINT('Ctrl Pts',(-19.7547810174489,-24.4834746942445,
124.879120016073)) ;
#52758=CARTESIAN_POINT('Ctrl Pts',(-19.8851618333618,-24.6734515209028,
124.520055763717)) ;
#52759=CARTESIAN_POINT('Ctrl Pts',(-20.0041249025935,-24.4934624404223,
124.797121058293)) ;
#52760=CARTESIAN_POINT('Ctrl Pts',(-20.0709240901513,-24.6834875098385,
124.420032910437)) ;
#52761=CARTESIAN_POINT('Ctrl Pts',(-20.2363287244765,-24.503498429358,124.672094532665)) ;
#52762=CARTESIAN_POINT('Ctrl Pts',(-20.2337420876468,-24.6933423796521,
124.291888982276)) ;
#52763=CARTESIAN_POINT('Ctrl Pts',(-20.4398532895244,-24.5133532991716,
124.511915769027)) ;
#52764=CARTESIAN_POINT('Ctrl Pts',(-20.3740410207416,-24.7033418208939,
124.135384425764)) ;
#52765=CARTESIAN_POINT('Ctrl Pts',(-20.6152286147795,-24.5233527404134,
124.316286380267)) ;
#52766=CARTESIAN_POINT('Ctrl Pts',(-20.4841026431737,-24.713236895074,123.958818728685)) ;
#52767=CARTESIAN_POINT('Ctrl Pts',(-20.7528077613622,-24.5332478145935,
124.095579716456)) ;
#52768=CARTESIAN_POINT('Ctrl Pts',(-20.5630911584333,-24.7232975509137,
123.762644267269)) ;
#52769=CARTESIAN_POINT('Ctrl Pts',(-20.851545217851,-24.5433084704332,123.850362627653)) ;
#52770=CARTESIAN_POINT('Ctrl Pts',(-20.6060224074376,-24.7331464251093,
123.560073880987)) ;
#52771=CARTESIAN_POINT('Ctrl Pts',(-20.9052114658555,-24.5531573446288,
123.59714904621)) ;
#52772=CARTESIAN_POINT('Ctrl Pts',(-20.6137892692649,-24.7431751370725,
123.349384846586)) ;
#52773=CARTESIAN_POINT('Ctrl Pts',(-20.9149218986309,-24.5631860565921,
123.333787858273)) ;
#52774=CARTESIAN_POINT('Ctrl Pts',(-20.5842846845228,-24.7532045376556,
123.140605694628)) ;
#52775=CARTESIAN_POINT('Ctrl Pts',(-20.8780431869163,-24.5732154571752,
123.072813707574)) ;
#52776=CARTESIAN_POINT('Ctrl Pts',(-20.5206480631986,-24.7630447312725,
122.943761957022)) ;
#52777=CARTESIAN_POINT('Ctrl Pts',(-20.7984988602342,-24.583055650792,122.826757371382)) ;
#52778=CARTESIAN_POINT('Ctrl Pts',(-20.4225485419105,-24.7730481538477,
122.757764156564)) ;
#52779=CARTESIAN_POINT('Ctrl Pts',(-20.6758759733845,-24.5930590733672,
122.594259198526)) ;
#52780=CARTESIAN_POINT('Ctrl Pts',(-20.2937856669965,-24.7830336909408,
122.591919417926)) ;
#52781=CARTESIAN_POINT('Ctrl Pts',(-20.5149236680147,-24.6030446104603,
122.386952011193)) ;
#52782=CARTESIAN_POINT('Ctrl Pts',(-20.1372175607481,-24.7930746954276,
122.450362162771)) ;
#52783=CARTESIAN_POINT('Ctrl Pts',(-20.3192148830929,-24.6130856149471,
122.210004149915)) ;
#52784=CARTESIAN_POINT('Ctrl Pts',(-19.9620847517272,-24.8029182343688,
122.340090117792)) ;
#52785=CARTESIAN_POINT('Ctrl Pts',(-20.1002988243913,-24.6229291538883,
122.07216197411)) ;
#52786=CARTESIAN_POINT('Ctrl Pts',(-19.7679204826026,-24.8129032653596,
122.260388804538)) ;
#52787=CARTESIAN_POINT('Ctrl Pts',(-19.8575938758335,-24.6329141848791,
121.972533729718)) ;
#52788=CARTESIAN_POINT('Ctrl Pts',(-19.5637613025099,-24.8228427278816,
122.215721170497)) ;
#52789=CARTESIAN_POINT('Ctrl Pts',(-19.6023947115002,-24.6428536474011,
121.916697509379)) ;
#52790=CARTESIAN_POINT('Ctrl Pts',(-19.3528855208101,-24.8328824601054,
122.207143938468)) ;
#52791=CARTESIAN_POINT('Ctrl Pts',(-19.3388001962124,-24.6528933796249,
121.905974359141)) ;
#52792=CARTESIAN_POINT('Ctrl Pts',(-19.1468393604488,-24.8427706404226,
122.234788301827)) ;
#52793=CARTESIAN_POINT('Ctrl Pts',(-19.0812413724602,-24.6627815599421,
121.940528367414)) ;
#52794=CARTESIAN_POINT('Ctrl Pts',(-18.9465910465543,-24.8527601561251,
122.298052941285)) ;
#52795=CARTESIAN_POINT('Ctrl Pts',(-18.8309303395174,-24.6727710756446,
122.019607849722)) ;
#52796=CARTESIAN_POINT('Ctrl Pts',(-18.7610210692701,-24.8627187067798,
122.394969542259)) ;
#52797=CARTESIAN_POINT('Ctrl Pts',(-18.5989667872647,-24.6827296262993,
122.140752466129)) ;
#52798=CARTESIAN_POINT('Ctrl Pts',(-18.5957514950734,-24.8726181138848,
122.521477714569)) ;
#52799=CARTESIAN_POINT('Ctrl Pts',(-18.3923783175925,-24.6926290334043,
122.298887165085)) ;
#52800=CARTESIAN_POINT('Ctrl Pts',(-18.4529280511965,-24.8826667003011,
122.677100505805)) ;
#52801=CARTESIAN_POINT('Ctrl Pts',(-18.2138481635963,-24.7026776198206,
122.493414575647)) ;
#52802=CARTESIAN_POINT('Ctrl Pts',(-18.3408505972411,-24.8925595192655,
122.85234593428)) ;
#52803=CARTESIAN_POINT('Ctrl Pts',(-18.0737497674036,-24.7125704387851,
122.712471449021)) ;
#52804=CARTESIAN_POINT('Ctrl Pts',(-18.2595668677293,-24.9026306367953,
123.047801925644)) ;
#52805=CARTESIAN_POINT('Ctrl Pts',(-17.9721440402677,-24.7226415563149,
122.9567905855)) ;
#52806=CARTESIAN_POINT('Ctrl Pts',(-18.2143360447103,-24.9124463307614,
123.249180345051)) ;
#52807=CARTESIAN_POINT('Ctrl Pts',(-17.9156039985749,-24.7324572502809,
123.208514840496)) ;
#52808=CARTESIAN_POINT('Ctrl Pts',(-18.2042126503118,-24.9225127082587,
123.460520176297)) ;
#52809=CARTESIAN_POINT('Ctrl Pts',(-17.9029486723776,-24.7425236277782,
123.472689210437)) ;
#52810=CARTESIAN_POINT('Ctrl Pts',(-18.2305681873623,-24.9324116943406,
123.667004534321)) ;
#52811=CARTESIAN_POINT('Ctrl Pts',(-17.9358920953055,-24.7524226138601,
123.730795685759)) ;
#52812=CARTESIAN_POINT('Ctrl Pts',(-18.2932377700678,-24.9424658743341,
123.868822725467)) ;
#52813=CARTESIAN_POINT('Ctrl Pts',(-18.0142279452828,-24.7624767938536,
123.983068491453)) ;
#52814=CARTESIAN_POINT('Ctrl Pts',(-18.3880943306794,-24.9523366872668,
124.053444339054)) ;
#52815=CARTESIAN_POINT('Ctrl Pts',(-18.1327982651776,-24.7723476067863,
124.21384699712)) ;
#52816=CARTESIAN_POINT('Ctrl Pts',(-18.5160928318226,-24.9624105881206,
124.222110708763)) ;
#52817=CARTESIAN_POINT('Ctrl Pts',(-18.2927953164419,-24.7824215076401,
124.424680232179)) ;
#52818=CARTESIAN_POINT('Ctrl Pts',(-18.6674180149936,-24.9722307435072,
124.362618007818)) ;
#52819=CARTESIAN_POINT('Ctrl Pts',(-18.4819523061609,-24.7922416630268,
124.600316091069)) ;
#52820=CARTESIAN_POINT('Ctrl Pts',(-18.8452136411496,-24.9823094504595,
124.477780776126)) ;
#52821=CARTESIAN_POINT('Ctrl Pts',(-18.7041959808431,-24.802320369979,124.74427000949)) ;
#52822=CARTESIAN_POINT('Ctrl Pts',(-19.0359724593799,-24.9921610389983,
124.558567319872)) ;
#52823=CARTESIAN_POINT('Ctrl Pts',(-18.9426453969579,-24.8121719585178,
124.845254460415)) ;
#52824=CARTESIAN_POINT('Ctrl Pts',(-19.2422734738344,-25.0022341555233,
124.606210580914)) ;
#52825=CARTESIAN_POINT('Ctrl Pts',(-19.2005210691097,-24.8222450750428,
124.904809172746)) ;
#52826=CARTESIAN_POINT('Ctrl Pts',(-19.4489294427733,-25.0120766726191,
124.617025230768)) ;
#52827=CARTESIAN_POINT('Ctrl Pts',(-19.4588424041229,-24.8320875921386,
124.918328324967)) ;
#52828=CARTESIAN_POINT('Ctrl Pts',(-19.6572595399181,-25.022057134173,124.592142989449)) ;
#52829=CARTESIAN_POINT('Ctrl Pts',(-19.7192553918332,-24.8420680536926,
124.887225976324)) ;
#52830=CARTESIAN_POINT('Ctrl Pts',(-19.858754508053,-25.0320753841638,124.530845580541)) ;
#52831=CARTESIAN_POINT('Ctrl Pts',(-19.9711242826763,-24.8520863036833,
124.810604842255)) ;
#52832=CARTESIAN_POINT('Ctrl Pts',(-20.0442458404208,-25.0419595443576,
124.437141256552)) ;
#52833=CARTESIAN_POINT('Ctrl Pts',(-20.2029896411673,-24.8619704638771,
124.693474375356)) ;
#52834=CARTESIAN_POINT('Ctrl Pts',(-20.2136336533158,-25.0520246913326,
124.310362839137)) ;
#52835=CARTESIAN_POINT('Ctrl Pts',(-20.4147243952556,-24.8720356108521,
124.53500199197)) ;
#52836=CARTESIAN_POINT('Ctrl Pts',(-20.3553327642867,-25.0618665149734,
124.159573795063)) ;
#52837=CARTESIAN_POINT('Ctrl Pts',(-20.5918496188217,-24.8818774344929,
124.34651493067)) ;
#52838=CARTESIAN_POINT('Ctrl Pts',(-20.4713227735349,-25.0718959874342,
123.98349792825)) ;
#52839=CARTESIAN_POINT('Ctrl Pts',(-20.7368372686807,-24.8919069069537,
124.126420308734)) ;
#52840=CARTESIAN_POINT('Ctrl Pts',(-20.5544183696664,-25.0819228426962,
123.789765828092)) ;
#52841=CARTESIAN_POINT('Ctrl Pts',(-20.8407071586523,-24.9019337622158,
123.884255456055)) ;
#52842=CARTESIAN_POINT('Ctrl Pts',(-20.6022129333517,-25.0917660928068,
123.58842207058)) ;
#52843=CARTESIAN_POINT('Ctrl Pts',(-20.9004509564866,-24.9117770123263,
123.632574419176)) ;
#52844=CARTESIAN_POINT('Ctrl Pts',(-20.6148605428865,-25.1018145323899,
123.377557024283)) ;
#52845=CARTESIAN_POINT('Ctrl Pts',(-20.9162606114389,-24.9218254519095,
123.368993380638)) ;
#52846=CARTESIAN_POINT('Ctrl Pts',(-20.590610957124,-25.1117640266378,123.16979691793)) ;
#52847=CARTESIAN_POINT('Ctrl Pts',(-20.8859488525621,-24.9317749461574,
123.109292637729)) ;
#52848=CARTESIAN_POINT('Ctrl Pts',(-20.5315027514083,-25.1216718823638,
122.970053451003)) ;
#52849=CARTESIAN_POINT('Ctrl Pts',(-20.8120633746983,-24.9416828018834,
122.859612422468)) ;
#52850=CARTESIAN_POINT('Ctrl Pts',(-20.4370028959412,-25.1317313590138,
122.780884060618)) ;
#52851=CARTESIAN_POINT('Ctrl Pts',(-20.6939388266364,-24.9517422785333,
122.623150935538)) ;
#52852=CARTESIAN_POINT('Ctrl Pts',(-20.3140267459724,-25.1415721684225,
122.614484936629)) ;
#52853=CARTESIAN_POINT('Ctrl Pts',(-20.5402177798436,-24.961583087942,122.415150839197)) ;
#52854=CARTESIAN_POINT('Ctrl Pts',(-20.1608696779371,-25.1516343187233,
122.46860151475)) ;
#52855=CARTESIAN_POINT('Ctrl Pts',(-20.348771652223,-24.9716452382428,122.232796879371)) ;
#52856=CARTESIAN_POINT('Ctrl Pts',(-19.9874513742878,-25.1615314798458,
122.353608540262)) ;
#52857=CARTESIAN_POINT('Ctrl Pts',(-20.1319979379793,-24.9815423993653,
122.089055106544)) ;
#52858=CARTESIAN_POINT('Ctrl Pts',(-19.7963375421497,-25.1714626542499,
122.269557911198)) ;
#52859=CARTESIAN_POINT('Ctrl Pts',(-19.8931048763315,-24.9914735737694,
121.983991783482)) ;
#52860=CARTESIAN_POINT('Ctrl Pts',(-19.5912085972719,-25.1815048579749,
122.219637399699)) ;
#52861=CARTESIAN_POINT('Ctrl Pts',(-19.6366938542674,-25.0015157774944,
121.921591372191)) ;
#52862=CARTESIAN_POINT('Ctrl Pts',(-19.3837898601191,-25.1913914404053,
122.206149497569)) ;
#52863=CARTESIAN_POINT('Ctrl Pts',(-19.3774193320278,-25.0114023599249,
121.904731667555)) ;
#52864=CARTESIAN_POINT('Ctrl Pts',(-19.174930617181,-25.2013848761537,122.228779671047)) ;
#52865=CARTESIAN_POINT('Ctrl Pts',(-19.1163451180377,-25.0213957956732,
121.933019785875)) ;
#52866=CARTESIAN_POINT('Ctrl Pts',(-18.9741668937736,-25.2113293445118,
122.287109961351)) ;
#52867=CARTESIAN_POINT('Ctrl Pts',(-18.8653899853022,-25.0313402640314,
122.005933155517)) ;
#52868=CARTESIAN_POINT('Ctrl Pts',(-18.7862616744613,-25.2212811607574,
122.379130251146)) ;
#52869=CARTESIAN_POINT('Ctrl Pts',(-18.6305081903496,-25.0412920802769,
122.120959220952)) ;
#52870=CARTESIAN_POINT('Ctrl Pts',(-18.6158633692364,-25.2313185968719,
122.503584025425)) ;
#52871=CARTESIAN_POINT('Ctrl Pts',(-18.4175106983079,-25.0513295163914,
122.276526693717)) ;
#52872=CARTESIAN_POINT('Ctrl Pts',(-18.4717187038832,-25.2412035560482,
122.653303494758)) ;
#52873=CARTESIAN_POINT('Ctrl Pts',(-18.2373294885558,-25.0612144755677,
122.463677159448)) ;
#52874=CARTESIAN_POINT('Ctrl Pts',(-18.3542495988289,-25.2512016742602,
122.827576694392)) ;
#52875=CARTESIAN_POINT('Ctrl Pts',(-18.0904935271512,-25.0712125937797,
122.681519130247)) ;
#52876=CARTESIAN_POINT('Ctrl Pts',(-18.2693324752695,-25.2611226067721,
123.018101116052)) ;
#52877=CARTESIAN_POINT('Ctrl Pts',(-17.984347411207,-25.0811335262917,122.91967563865)) ;
#52878=CARTESIAN_POINT('Ctrl Pts',(-18.2181276836119,-25.2711639069942,
123.2228864421)) ;
#52879=CARTESIAN_POINT('Ctrl Pts',(-17.9203421283148,-25.0911748265137,
123.175657289264)) ;
#52880=CARTESIAN_POINT('Ctrl Pts',(-18.203527625728,-25.2810708253842,123.430650481538)) ;
#52881=CARTESIAN_POINT('Ctrl Pts',(-17.9020926496286,-25.1010817449037,
123.435363279088)) ;
#52882=CARTESIAN_POINT('Ctrl Pts',(-18.2246915361504,-25.2910066170932,
123.638458055856)) ;
#52883=CARTESIAN_POINT('Ctrl Pts',(-17.9285484879378,-25.1110175366128,
123.695123310117)) ;
#52884=CARTESIAN_POINT('Ctrl Pts',(-18.2824223938012,-25.3010475116711,
123.841496647617)) ;
#52885=CARTESIAN_POINT('Ctrl Pts',(-18.0007127840701,-25.1210584311907,
123.948921150005)) ;
#52886=CARTESIAN_POINT('Ctrl Pts',(-18.3729909834067,-25.310934713385,124.028599784085)) ;
#52887=CARTESIAN_POINT('Ctrl Pts',(-18.1139247513715,-25.1309456329045,
124.182800630761)) ;
#52888=CARTESIAN_POINT('Ctrl Pts',(-18.4956664931269,-25.3209269811466,
124.19910961797)) ;
#52889=CARTESIAN_POINT('Ctrl Pts',(-18.2672700655301,-25.1409379006661,
124.395937506981)) ;
#52890=CARTESIAN_POINT('Ctrl Pts',(-18.6454852083747,-25.3308755021684,
124.345063822644)) ;
#52891=CARTESIAN_POINT('Ctrl Pts',(-18.45454452636,-25.1508864216879,124.578379945201)) ;
#52892=CARTESIAN_POINT('Ctrl Pts',(-18.8179761803924,-25.3408122757461,
124.462875898515)) ;
#52893=CARTESIAN_POINT('Ctrl Pts',(-18.6701593793859,-25.1608231952656,
124.725644505682)) ;
#52894=CARTESIAN_POINT('Ctrl Pts',(-19.0091199998643,-25.3507953238871,
124.549608305468)) ;
#52895=CARTESIAN_POINT('Ctrl Pts',(-18.9090898745599,-25.1708062434066,
124.834059046588)) ;
#52896=CARTESIAN_POINT('Ctrl Pts',(-19.2137039022557,-25.3608390314972,
124.601767255972)) ;
#52897=CARTESIAN_POINT('Ctrl Pts',(-19.164819826109,-25.1808499510167,124.899256681918)) ;
#52898=CARTESIAN_POINT('Ctrl Pts',(-19.4197410435178,-25.3706677246505,
124.617749119944)) ;
#52899=CARTESIAN_POINT('Ctrl Pts',(-19.422367781993,-25.19067864417,124.91923291457)) ;
#52900=CARTESIAN_POINT('Ctrl Pts',(-19.6305293861476,-25.3807424737799,
124.597364532467)) ;
#52901=CARTESIAN_POINT('Ctrl Pts',(-19.6858526790908,-25.2007533932995,
124.89375095602)) ;
#52902=CARTESIAN_POINT('Ctrl Pts',(-19.8303729849827,-25.3906077995755,
124.541808861825)) ;
#52903=CARTESIAN_POINT('Ctrl Pts',(-19.9356579462846,-25.210618719095,124.824304856749)) ;
#52904=CARTESIAN_POINT('Ctrl Pts',(-20.0207155288672,-25.4006299739324,
124.451476082817)) ;
#52905=CARTESIAN_POINT('Ctrl Pts',(-20.1735854694028,-25.2206408934519,
124.711387601756)) ;
#52906=CARTESIAN_POINT('Ctrl Pts',(-20.1922659082655,-25.4106560271393,
124.328983469291)) ;
#52907=CARTESIAN_POINT('Ctrl Pts',(-20.3880226562012,-25.2306669466589,
124.558270853534)) ;
#52908=CARTESIAN_POINT('Ctrl Pts',(-20.3376209909237,-25.4205097239856,
124.181407992117)) ;
#52909=CARTESIAN_POINT('Ctrl Pts',(-20.5697163880298,-25.2405206435051,
124.373799671804)) ;
#52910=CARTESIAN_POINT('Ctrl Pts',(-20.4569372871272,-25.4304691287386,
124.009344969333)) ;
#52911=CARTESIAN_POINT('Ctrl Pts',(-20.718860691556,-25.2504800482581,124.158719634618)) ;
#52912=CARTESIAN_POINT('Ctrl Pts',(-20.5449097818086,-25.4405073744435,
123.817532980503)) ;
#52913=CARTESIAN_POINT('Ctrl Pts',(-20.8288249196996,-25.260518293963,123.918954163227)) ;
#52914=CARTESIAN_POINT('Ctrl Pts',(-20.5977398559491,-25.4503815586055,
123.616753729714)) ;
#52915=CARTESIAN_POINT('Ctrl Pts',(-20.894861231508,-25.270392478125,123.667978712709)) ;
#52916=CARTESIAN_POINT('Ctrl Pts',(-20.6152318947396,-25.4604513417434,
123.405808054371)) ;
#52917=CARTESIAN_POINT('Ctrl Pts',(-20.9167246663165,-25.2804622612629,
123.404296836378)) ;
#52918=CARTESIAN_POINT('Ctrl Pts',(-20.5963934662247,-25.4702845967642,
123.199925169976)) ;
#52919=CARTESIAN_POINT('Ctrl Pts',(-20.8931748952391,-25.2902955162837,
123.146942101497)) ;
#52920=CARTESIAN_POINT('Ctrl Pts',(-20.5415866211297,-25.4803150228959,
122.99630793319)) ;
#52921=CARTESIAN_POINT('Ctrl Pts',(-20.824664603681,-25.3003259424154,122.892421113354)) ;
#52922=CARTESIAN_POINT('Ctrl Pts',(-20.4516839654255,-25.4903466350829,
122.805521136802)) ;
#52923=CARTESIAN_POINT('Ctrl Pts',(-20.7122848540759,-25.3103575546024,
122.653938383704)) ;
#52924=CARTESIAN_POINT('Ctrl Pts',(-20.3328358727724,-25.5001763319375,
122.636482789407)) ;
#52925=CARTESIAN_POINT('Ctrl Pts',(-20.5637225649554,-25.320187251457,122.442640422349)) ;
#52926=CARTESIAN_POINT('Ctrl Pts',(-20.1844921702679,-25.51016577384,122.487819824173)) ;
#52927=CARTESIAN_POINT('Ctrl Pts',(-20.3782914260521,-25.3301766933595,
122.256812972949)) ;
#52928=CARTESIAN_POINT('Ctrl Pts',(-20.0113511337868,-25.5202096658556,
122.366957918595)) ;
#52929=CARTESIAN_POINT('Ctrl Pts',(-20.1618642263382,-25.3402205853752,
122.105737144848)) ;
#52930=CARTESIAN_POINT('Ctrl Pts',(-19.8242733803076,-25.5300312276249,
122.279578448375)) ;
#52931=CARTESIAN_POINT('Ctrl Pts',(-19.9280150892942,-25.3500421471444,
121.996514020371)) ;
#52932=CARTESIAN_POINT('Ctrl Pts',(-19.6206530982633,-25.5400667992491,
122.2243313612)) ;
#52933=CARTESIAN_POINT('Ctrl Pts',(-19.6734892887198,-25.3600777187686,
121.927457195512)) ;
#52934=CARTESIAN_POINT('Ctrl Pts',(-19.4106109576734,-25.5500960735309,
122.205921274925)) ;
#52935=CARTESIAN_POINT('Ctrl Pts',(-19.4109364974857,-25.3701069930504,
121.904446478551)) ;
#52936=CARTESIAN_POINT('Ctrl Pts',(-19.2046030647571,-25.5599299106495,
122.22335172287)) ;
#52937=CARTESIAN_POINT('Ctrl Pts',(-19.1534256982825,-25.3799408301691,
121.926236678516)) ;
#52938=CARTESIAN_POINT('Ctrl Pts',(-19.000259823004,-25.5699823067377,122.277212320983)) ;
#52939=CARTESIAN_POINT('Ctrl Pts',(-18.8979973838233,-25.3899932262572,
121.993564432234)) ;
#52940=CARTESIAN_POINT('Ctrl Pts',(-18.8106744902198,-25.5799190736882,
122.364971233025)) ;
#52941=CARTESIAN_POINT('Ctrl Pts',(-18.6610161339955,-25.3999299932077,
122.103265136426)) ;
#52942=CARTESIAN_POINT('Ctrl Pts',(-18.6389522732557,-25.5898533086675,
122.483834336028)) ;
#52943=CARTESIAN_POINT('Ctrl Pts',(-18.4463642083147,-25.409864228187,122.251846102257)) ;
#52944=CARTESIAN_POINT('Ctrl Pts',(-18.4892297183612,-25.5998770719943,
122.632124416292)) ;
#52945=CARTESIAN_POINT('Ctrl Pts',(-18.2592125480049,-25.4198879915138,
122.437210228585)) ;
#52946=CARTESIAN_POINT('Ctrl Pts',(-18.3690729527359,-25.6097634133789,
122.801712077461)) ;
#52947=CARTESIAN_POINT('Ctrl Pts',(-18.1090179639727,-25.4297743328985,
122.649196677297)) ;
#52948=CARTESIAN_POINT('Ctrl Pts',(-18.2788188736161,-25.6197524621459,
122.991336888981)) ;
#52949=CARTESIAN_POINT('Ctrl Pts',(-17.9962023975018,-25.4397633816654,
122.886228834254)) ;
#52950=CARTESIAN_POINT('Ctrl Pts',(-18.2229938244163,-25.6297936828433,
123.194918820965)) ;
#52951=CARTESIAN_POINT('Ctrl Pts',(-17.9264232478463,-25.4498046023628,
123.140706746034)) ;
#52952=CARTESIAN_POINT('Ctrl Pts',(-18.2034358522084,-25.6396263230212,
123.400700722428)) ;
#52953=CARTESIAN_POINT('Ctrl Pts',(-17.9019779828745,-25.4596372425407,
123.397935296116)) ;
#52954=CARTESIAN_POINT('Ctrl Pts',(-18.2195753607672,-25.6496202523291,
123.610182629394)) ;
#52955=CARTESIAN_POINT('Ctrl Pts',(-17.9221548128454,-25.4696311718487,
123.659787613436)) ;
#52956=CARTESIAN_POINT('Ctrl Pts',(-18.2724604743426,-25.6596494600097,
123.814289690547)) ;
#52957=CARTESIAN_POINT('Ctrl Pts',(-17.988263462569,-25.4796603795292,123.914920832019)) ;
#52958=CARTESIAN_POINT('Ctrl Pts',(-18.358339643957,-25.6695252717138,124.003328990778)) ;
#52959=CARTESIAN_POINT('Ctrl Pts',(-18.0956149026414,-25.4895361912333,
124.151219574902)) ;
#52960=CARTESIAN_POINT('Ctrl Pts',(-18.4769919261622,-25.6795244986852,
124.176823257226)) ;
#52961=CARTESIAN_POINT('Ctrl Pts',(-18.2439323542707,-25.4995354182047,
124.368086107319)) ;
#52962=CARTESIAN_POINT('Ctrl Pts',(-18.6225453670208,-25.6894339798409,
124.325912667589)) ;
#52963=CARTESIAN_POINT('Ctrl Pts',(-18.4258762773874,-25.5094448993604,
124.554446462921)) ;
#52964=CARTESIAN_POINT('Ctrl Pts',(-18.7942023877807,-25.6994872101418,
124.449174674582)) ;
#52965=CARTESIAN_POINT('Ctrl Pts',(-18.6404489286503,-25.5194981296613,
124.708521880127)) ;
#52966=CARTESIAN_POINT('Ctrl Pts',(-18.9811834854639,-25.7093578266928,
124.539201485248)) ;
#52967=CARTESIAN_POINT('Ctrl Pts',(-18.8741769468847,-25.5293687462124,
124.821053391439)) ;
#52968=CARTESIAN_POINT('Ctrl Pts',(-19.1838697790237,-25.7193794884249,
124.596699644364)) ;
#52969=CARTESIAN_POINT('Ctrl Pts',(-19.1275355267002,-25.5393904079444,
124.892923586862)) ;
#52970=CARTESIAN_POINT('Ctrl Pts',(-19.3935471693339,-25.729402301606,124.617654797258)) ;
#52971=CARTESIAN_POINT('Ctrl Pts',(-19.3896325300255,-25.5494132211255,
124.919115026399)) ;
#52972=CARTESIAN_POINT('Ctrl Pts',(-19.6004203943415,-25.7392694660659,
124.60247790701)) ;
#52973=CARTESIAN_POINT('Ctrl Pts',(-19.6482244565418,-25.5592803855855,
124.900141299554)) ;
#52974=CARTESIAN_POINT('Ctrl Pts',(-19.804222528808,-25.7492629082859,124.551424075459)) ;
#52975=CARTESIAN_POINT('Ctrl Pts',(-19.9029765856325,-25.5692738278054,
124.836321404756)) ;
#52976=CARTESIAN_POINT('Ctrl Pts',(-19.9966241110481,-25.7592945818862,
124.465058729289)) ;
#52977=CARTESIAN_POINT('Ctrl Pts',(-20.1434775003674,-25.5793055014057,
124.728362358445)) ;
#52978=CARTESIAN_POINT('Ctrl Pts',(-20.1684200868147,-25.7691610169992,
124.348807750651)) ;
#52979=CARTESIAN_POINT('Ctrl Pts',(-20.3582214203252,-25.5891719365187,
124.583046155799)) ;
#52980=CARTESIAN_POINT('Ctrl Pts',(-20.3194620562051,-25.7791484675323,
124.202992595232)) ;
#52981=CARTESIAN_POINT('Ctrl Pts',(-20.5470220994703,-25.5991593870518,
124.400775187966)) ;
#52982=CARTESIAN_POINT('Ctrl Pts',(-20.4424893830337,-25.7890933973602,
124.033909844264)) ;
#52983=CARTESIAN_POINT('Ctrl Pts',(-20.7008042111351,-25.6091043168797,
124.189419968522)) ;
#52984=CARTESIAN_POINT('Ctrl Pts',(-20.5350834451132,-25.7991382924153,
123.844138661879)) ;
#52985=CARTESIAN_POINT('Ctrl Pts',(-20.816544361093,-25.6191492119349,123.952204828917)) ;
#52986=CARTESIAN_POINT('Ctrl Pts',(-20.5924455699357,-25.8090003541012,
123.64488433114)) ;
#52987=CARTESIAN_POINT('Ctrl Pts',(-20.888244530367,-25.6290112736207,123.703135751178)) ;
#52988=CARTESIAN_POINT('Ctrl Pts',(-20.6150418051958,-25.818992076888,123.436062409259)) ;
#52989=CARTESIAN_POINT('Ctrl Pts',(-20.9164870896894,-25.6390029964076,
123.442107956855)) ;
#52990=CARTESIAN_POINT('Ctrl Pts',(-20.6010425706833,-25.828924291128,123.22772327375)) ;
#52991=CARTESIAN_POINT('Ctrl Pts',(-20.898985287242,-25.6489352106475,123.181683998665)) ;
#52992=CARTESIAN_POINT('Ctrl Pts',(-20.5515128182878,-25.8388636096937,
123.024716518231)) ;
#52993=CARTESIAN_POINT('Ctrl Pts',(-20.8370703425302,-25.6588745292133,
122.927926047606)) ;
#52994=CARTESIAN_POINT('Ctrl Pts',(-20.4664264572267,-25.8489077844696,
122.831461041933)) ;
#52995=CARTESIAN_POINT('Ctrl Pts',(-20.7307098428418,-25.6689187039891,
122.686357803528)) ;
#52996=CARTESIAN_POINT('Ctrl Pts',(-20.3511977884892,-25.8587783385346,
122.658884676041)) ;
#52997=CARTESIAN_POINT('Ctrl Pts',(-20.5866715411754,-25.6787892580541,
122.470638672497)) ;
#52998=CARTESIAN_POINT('Ctrl Pts',(-20.2068205658345,-25.8687433208888,
122.507083215677)) ;
#52999=CARTESIAN_POINT('Ctrl Pts',(-20.406197903006,-25.6887542404083,122.280888722029)) ;
#53000=CARTESIAN_POINT('Ctrl Pts',(-20.0369803709032,-25.8787740237786,
122.382099598688)) ;
#53001=CARTESIAN_POINT('Ctrl Pts',(-20.1938959520374,-25.6987849432981,
122.124661424507)) ;
#53002=CARTESIAN_POINT('Ctrl Pts',(-19.8507320191725,-25.8886663638038,
122.289510710408)) ;
#53003=CARTESIAN_POINT('Ctrl Pts',(-19.9610841221135,-25.7086772833233,
122.008927766371)) ;
#53004=CARTESIAN_POINT('Ctrl Pts',(-19.6480507991876,-25.8987195969637,
122.229703855428)) ;
#53005=CARTESIAN_POINT('Ctrl Pts',(-19.7077317559677,-25.7187305164833,
121.934171888426)) ;
#53006=CARTESIAN_POINT('Ctrl Pts',(-19.4416056541742,-25.9086008414405,
122.206269923725)) ;
#53007=CARTESIAN_POINT('Ctrl Pts',(-19.4496748815484,-25.72861176096,121.904882259166)) ;
#53008=CARTESIAN_POINT('Ctrl Pts',(-19.2311053037005,-25.9186339623115,
122.219073769285)) ;
#53009=CARTESIAN_POINT('Ctrl Pts',(-19.186549549454,-25.738644881831,121.920889891472)) ;
#53010=CARTESIAN_POINT('Ctrl Pts',(-19.0290124695695,-25.9285151725866,
122.267326061068)) ;
#53011=CARTESIAN_POINT('Ctrl Pts',(-18.9339340957259,-25.7485260921061,
121.981208014828)) ;
#53012=CARTESIAN_POINT('Ctrl Pts',(-18.8349223161673,-25.9385772483559,
122.351365482574)) ;
#53013=CARTESIAN_POINT('Ctrl Pts',(-18.6913224501782,-25.7585881678754,
122.086259918591)) ;
#53014=CARTESIAN_POINT('Ctrl Pts',(-18.6618773393018,-25.9484343067377,
122.465428901543)) ;
#53015=CARTESIAN_POINT('Ctrl Pts',(-18.4750177695224,-25.7684452262572,
122.228841554535)) ;
#53016=CARTESIAN_POINT('Ctrl Pts',(-18.508920686306,-25.9584288620267,122.609440179343)) ;
#53017=CARTESIAN_POINT('Ctrl Pts',(-18.2838238475802,-25.7784397815462,
122.408857735578)) ;
#53018=CARTESIAN_POINT('Ctrl Pts',(-18.3840592104564,-25.9683547495622,
122.776670958682)) ;
#53019=CARTESIAN_POINT('Ctrl Pts',(-18.1277492564418,-25.7883656690817,
122.617897877515)) ;
#53020=CARTESIAN_POINT('Ctrl Pts',(-18.2891587151755,-25.9783797695574,
122.964835760839)) ;
#53021=CARTESIAN_POINT('Ctrl Pts',(-18.0091260992142,-25.798390689077,122.853105228262)) ;
#53022=CARTESIAN_POINT('Ctrl Pts',(-18.2290682932492,-25.9882771466611,
123.164050381415)) ;
#53023=CARTESIAN_POINT('Ctrl Pts',(-17.934015776066,-25.8082880661806,123.102124235141)) ;
#53024=CARTESIAN_POINT('Ctrl Pts',(-18.2037946806714,-25.998267383742,123.3725562714)) ;
#53025=CARTESIAN_POINT('Ctrl Pts',(-17.9024264990664,-25.8182783032615,
123.362756958179)) ;
#53026=CARTESIAN_POINT('Ctrl Pts',(-18.2155658880432,-26.0083039965508,
123.583225928318)) ;
#53027=CARTESIAN_POINT('Ctrl Pts',(-17.9171433200862,-25.8283149160703,
123.626094022958)) ;
#53028=CARTESIAN_POINT('Ctrl Pts',(-18.2625157876823,-26.0181538799688,
123.784916905059)) ;
#53029=CARTESIAN_POINT('Ctrl Pts',(-17.9758333007663,-25.8381647994883,
123.878206838419)) ;
#53030=CARTESIAN_POINT('Ctrl Pts',(-18.3446404620089,-26.0281574968712,
123.978504100519)) ;
#53031=CARTESIAN_POINT('Ctrl Pts',(-18.0784917993927,-25.8481684163907,
124.120189945172)) ;
#53032=CARTESIAN_POINT('Ctrl Pts',(-18.4590946254507,-26.0381469086364,
124.154624318019)) ;
#53033=CARTESIAN_POINT('Ctrl Pts',(-18.2215613396099,-25.8581578281559,
124.340338257024)) ;
#53034=CARTESIAN_POINT('Ctrl Pts',(-18.6028685076964,-26.0481656699812,
124.308517074879)) ;
#53035=CARTESIAN_POINT('Ctrl Pts',(-18.4012825633872,-25.8681765895007,
124.53270427943)) ;
#53036=CARTESIAN_POINT('Ctrl Pts',(-18.8247544491437,-26.0613843453623,
124.475917456974)) ;
#53037=CARTESIAN_POINT('Ctrl Pts',(-18.6786331145576,-25.8813952648818,
124.741942400174)) ;
#53038=CARTESIAN_POINT('Ctrl Pts',(-19.0869231326057,-26.074694652607,124.582399606467)) ;
#53039=CARTESIAN_POINT('Ctrl Pts',(-19.0063037436097,-25.8947055721265,
124.87503799084)) ;
#53040=CARTESIAN_POINT('Ctrl Pts',(-19.363072798974,-26.087932318833,124.616808325891)) ;
#53041=CARTESIAN_POINT('Ctrl Pts',(-19.3515492792957,-25.9079432383525,
124.91805906262)) ;
#53042=CARTESIAN_POINT('Ctrl Pts',(-19.5713918157783,-26.0978520142437,
124.606935546831)) ;
#53043=CARTESIAN_POINT('Ctrl Pts',(-19.6119358669811,-25.9178629337632,
124.905712873674)) ;
#53044=CARTESIAN_POINT('Ctrl Pts',(-19.7774861802108,-26.1079048812422,
124.560193148227)) ;
#53045=CARTESIAN_POINT('Ctrl Pts',(-19.8695568707557,-25.9279158007617,
124.847282647042)) ;
#53046=CARTESIAN_POINT('Ctrl Pts',(-19.9686281474796,-26.1177602895715,
124.480186051397)) ;
#53047=CARTESIAN_POINT('Ctrl Pts',(-20.1084811471548,-25.937771209091,124.747272818746)) ;
#53048=CARTESIAN_POINT('Ctrl Pts',(-20.14637377885,-26.1277989212481,124.366438520996)) ;
#53049=CARTESIAN_POINT('Ctrl Pts',(-20.3306652048825,-25.9478098407676,
124.605081165826)) ;
#53050=CARTESIAN_POINT('Ctrl Pts',(-20.3519626171017,-26.1411011035151,
124.176812384291)) ;
#53051=CARTESIAN_POINT('Ctrl Pts',(-20.5876341490242,-25.9611120230346,
124.368071353143)) ;
#53052=CARTESIAN_POINT('Ctrl Pts',(-20.5406207798638,-26.157646116598,123.879908726874)) ;
#53053=CARTESIAN_POINT('Ctrl Pts',(-20.8234715240876,-25.9776570361175,
123.996893725458)) ;
#53054=CARTESIAN_POINT('Ctrl Pts',(-20.6172088047157,-26.1742981326742,
123.534214772238)) ;
#53055=CARTESIAN_POINT('Ctrl Pts',(-20.919190598142,-25.9943090521937,123.56485434145)) ;
#53056=CARTESIAN_POINT('Ctrl Pts',(-20.6051217054238,-26.1875212235794,
123.256506578879)) ;
#53057=CARTESIAN_POINT('Ctrl Pts',(-20.9040855808188,-26.007532143099,123.21765581557)) ;
#53058=CARTESIAN_POINT('Ctrl Pts',(-20.5603924279369,-26.1974821831388,
123.05192147308)) ;
#53059=CARTESIAN_POINT('Ctrl Pts',(-20.8481710290793,-26.0174931026583,
122.961938491769)) ;
#53060=CARTESIAN_POINT('Ctrl Pts',(-20.4800725687243,-26.2075069798899,
122.857083849691)) ;
#53061=CARTESIAN_POINT('Ctrl Pts',(-20.747767274539,-26.0275178994094,122.718386742788)) ;
#53062=CARTESIAN_POINT('Ctrl Pts',(-20.3313987181556,-26.2207314272857,
122.62210740137)) ;
#53063=CARTESIAN_POINT('Ctrl Pts',(-20.5619333819627,-26.0407423468052,
122.424679164623)) ;
#53064=CARTESIAN_POINT('Ctrl Pts',(-20.0717140768469,-26.2373652119848,
122.382085717408)) ;
#53065=CARTESIAN_POINT('Ctrl Pts',(-20.2373134507681,-26.0573761315043,
122.124643357243)) ;
#53066=CARTESIAN_POINT('Ctrl Pts',(-19.6815099293272,-26.2572678787097,
122.218198924247)) ;
#53067=CARTESIAN_POINT('Ctrl Pts',(-19.7495611854334,-26.0772787982292,
121.919792632076)) ;
#53068=CARTESIAN_POINT('Ctrl Pts',(-19.2589510713564,-26.2771681064916,
122.196756051272)) ;
#53069=CARTESIAN_POINT('Ctrl Pts',(-19.2213622812154,-26.0971790260111,
121.892991857086)) ;
#53070=CARTESIAN_POINT('Ctrl Pts',(-18.8539777559444,-26.2970855940231,
122.320631928225)) ;
#53071=CARTESIAN_POINT('Ctrl Pts',(-18.7151476740853,-26.1170965135426,
122.047840068717)) ;
#53072=CARTESIAN_POINT('Ctrl Pts',(-18.5152044782925,-26.31701511984,122.575227475119)) ;
#53073=CARTESIAN_POINT('Ctrl Pts',(-18.2916834897623,-26.1370260393595,
122.366086543186)) ;
#53074=CARTESIAN_POINT('Ctrl Pts',(-18.2833320361407,-26.3369773877262,
122.930774152276)) ;
#53075=CARTESIAN_POINT('Ctrl Pts',(-18.0018457089775,-26.1569883072458,
122.810521280933)) ;
#53076=CARTESIAN_POINT('Ctrl Pts',(-18.187043146482,-26.3568675826784,123.342528444568)) ;
#53077=CARTESIAN_POINT('Ctrl Pts',(-17.8814876926625,-26.176878502198,123.32521358711)) ;
#53078=CARTESIAN_POINT('Ctrl Pts',(-18.2360005587426,-26.3767578274247,
123.762699469235)) ;
#53079=CARTESIAN_POINT('Ctrl Pts',(-17.9426863606114,-26.1967687469442,
123.850425839093)) ;
#53080=CARTESIAN_POINT('Ctrl Pts',(-18.4278756911333,-26.3968321999872,
124.143912754518)) ;
#53081=CARTESIAN_POINT('Ctrl Pts',(-18.1825328724787,-26.2168431195067,
124.326942241205)) ;
#53082=CARTESIAN_POINT('Ctrl Pts',(-18.7338400806782,-26.4166175773475,
124.432727082962)) ;
#53083=CARTESIAN_POINT('Ctrl Pts',(-18.5649877789369,-26.236628496867,124.68795667233)) ;
#53084=CARTESIAN_POINT('Ctrl Pts',(-19.1228257813227,-26.4365794514146,
124.602461953777)) ;
#53085=CARTESIAN_POINT('Ctrl Pts',(-19.0512197802809,-26.2565903709341,
124.900124064348)) ;
#53086=CARTESIAN_POINT('Ctrl Pts',(-19.5468805261724,-26.4565594269051,
124.628280549384)) ;
#53087=CARTESIAN_POINT('Ctrl Pts',(-19.5812880978611,-26.2765703464246,
124.932395779943)) ;
#53088=CARTESIAN_POINT('Ctrl Pts',(-19.9511224656437,-26.476371856783,124.509636259826)) ;
#53089=CARTESIAN_POINT('Ctrl Pts',(-20.0865875255273,-26.2963827763026,
124.784090581465)) ;
#53090=CARTESIAN_POINT('Ctrl Pts',(-20.2937255390238,-26.4963519648733,
124.258562719939)) ;
#53091=CARTESIAN_POINT('Ctrl Pts',(-20.5148410358532,-26.3163628843929,
124.470248873586)) ;
#53092=CARTESIAN_POINT('Ctrl Pts',(-20.5290130856317,-26.5162463484706,
123.906914863893)) ;
#53093=CARTESIAN_POINT('Ctrl Pts',(-20.8089496482753,-26.3362572679901,
124.030690459126)) ;
#53094=CARTESIAN_POINT('Ctrl Pts',(-20.6306703899268,-26.5361732764478,
123.495687774504)) ;
#53095=CARTESIAN_POINT('Ctrl Pts',(-20.9360216457934,-26.3561841959673,
123.516657893166)) ;
#53096=CARTESIAN_POINT('Ctrl Pts',(-20.58650883794,-26.556068133749,123.074882964739)) ;
#53097=CARTESIAN_POINT('Ctrl Pts',(-20.8808211230265,-26.3760790532686,
122.99065319296)) ;
#53098=CARTESIAN_POINT('Ctrl Pts',(-20.3997314232741,-26.5761073273527,
122.691961278104)) ;
#53099=CARTESIAN_POINT('Ctrl Pts',(-20.6473502028228,-26.3961182468722,
122.512000068487)) ;
#53100=CARTESIAN_POINT('Ctrl Pts',(-20.0964143874877,-26.5959472952634,
122.39871350997)) ;
#53101=CARTESIAN_POINT('Ctrl Pts',(-20.2682064550597,-26.415958214783,122.14544089517)) ;
#53102=CARTESIAN_POINT('Ctrl Pts',(-19.7103017728837,-26.6158621122275,
122.224956806707)) ;
#53103=CARTESIAN_POINT('Ctrl Pts',(-19.7855675978862,-26.435873031747,121.928243360059)) ;
#53104=CARTESIAN_POINT('Ctrl Pts',(-19.2874660199691,-26.6358043576238,
122.193640512695)) ;
#53105=CARTESIAN_POINT('Ctrl Pts',(-19.257023805954,-26.4558152771433,121.889095738547)) ;
#53106=CARTESIAN_POINT('Ctrl Pts',(-18.8804463278445,-26.6556764057383,
122.30743483587)) ;
#53107=CARTESIAN_POINT('Ctrl Pts',(-18.7482497387927,-26.4756873252578,
122.031335489751)) ;
#53108=CARTESIAN_POINT('Ctrl Pts',(-18.534656096257,-26.6756874706924,122.555130633679)) ;
#53109=CARTESIAN_POINT('Ctrl Pts',(-18.3160101802198,-26.4956983902119,
122.340952921464)) ;
#53110=CARTESIAN_POINT('Ctrl Pts',(-18.2958118938891,-26.695498994996,122.902353695436)) ;
#53111=CARTESIAN_POINT('Ctrl Pts',(-18.0174531567046,-26.5155099145155,
122.774978345783)) ;
#53112=CARTESIAN_POINT('Ctrl Pts',(-18.1886180442207,-26.7155942069594,
123.315793755655)) ;
#53113=CARTESIAN_POINT('Ctrl Pts',(-17.8834572828486,-26.5356051264789,
123.291778439974)) ;
#53114=CARTESIAN_POINT('Ctrl Pts',(-18.2284182206714,-26.7353749308792,
123.734667026007)) ;
#53115=CARTESIAN_POINT('Ctrl Pts',(-17.9332038024577,-26.5553858503987,
123.815368387787)) ;
#53116=CARTESIAN_POINT('Ctrl Pts',(-18.4096610154177,-26.755366006522,124.118979626269)) ;
#53117=CARTESIAN_POINT('Ctrl Pts',(-18.1597535328344,-26.5753769260415,
124.295760857053)) ;
#53118=CARTESIAN_POINT('Ctrl Pts',(-18.7099242034501,-26.775247945565,124.416730191879)) ;
#53119=CARTESIAN_POINT('Ctrl Pts',(-18.5350790244108,-26.5952588650845,
124.667951356178)) ;
#53120=CARTESIAN_POINT('Ctrl Pts',(-19.0947640893078,-26.7952005500682,
124.595125233846)) ;
#53121=CARTESIAN_POINT('Ctrl Pts',(-19.0161267181659,-26.6152114695878,
124.890949085933)) ;
#53122=CARTESIAN_POINT('Ctrl Pts',(-19.5163545803771,-26.8150994187989,
124.631394180349)) ;
#53123=CARTESIAN_POINT('Ctrl Pts',(-19.543113858081,-26.6351103383184,124.936289536642)) ;
#53124=CARTESIAN_POINT('Ctrl Pts',(-19.9249223900067,-26.8349928186085,
124.522185577163)) ;
#53125=CARTESIAN_POINT('Ctrl Pts',(-20.0538241490257,-26.655003738128,124.799784245875)) ;
#53126=CARTESIAN_POINT('Ctrl Pts',(-20.2724780813472,-26.8549019494485,
124.28036241543)) ;
#53127=CARTESIAN_POINT('Ctrl Pts',(-20.4882718451227,-26.674912868968,124.49750710335)) ;
#53128=CARTESIAN_POINT('Ctrl Pts',(-20.5176077328645,-26.8749340492121,
123.93208451665)) ;
#53129=CARTESIAN_POINT('Ctrl Pts',(-20.7946862218573,-26.6949449687316,
124.062171882856)) ;
#53130=CARTESIAN_POINT('Ctrl Pts',(-20.6098098899142,-26.8914661223815,
123.592826429201)) ;
#53131=CARTESIAN_POINT('Ctrl Pts',(-20.9099487233214,-26.711477041901,123.638071483034)) ;
#53132=CARTESIAN_POINT('Ctrl Pts',(-20.6110911401444,-26.9048014629875,
123.312495899499)) ;
#53133=CARTESIAN_POINT('Ctrl Pts',(-20.9115489479595,-26.724812382507,123.287684923659)) ;
#53134=CARTESIAN_POINT('Ctrl Pts',(-20.5764556782728,-26.9146440215272,
123.108474267684)) ;
#53135=CARTESIAN_POINT('Ctrl Pts',(-20.8682561093862,-26.7346549410467,
123.032650001393)) ;
#53136=CARTESIAN_POINT('Ctrl Pts',(-20.505658826445,-26.9246959283771,122.909381601415)) ;
#53137=CARTESIAN_POINT('Ctrl Pts',(-20.7797708304391,-26.7447068478966,
122.783795004268)) ;
#53138=CARTESIAN_POINT('Ctrl Pts',(-20.3681524800132,-26.937944442768,122.66718118586)) ;
#53139=CARTESIAN_POINT('Ctrl Pts',(-20.6078481494887,-26.7579553622875,
122.480989791496)) ;
#53140=CARTESIAN_POINT('Ctrl Pts',(-20.1207621070725,-26.9545436177157,
122.415419343604)) ;
#53141=CARTESIAN_POINT('Ctrl Pts',(-20.2986718810643,-26.7745545372353,
122.166348506496)) ;
#53142=CARTESIAN_POINT('Ctrl Pts',(-19.8026232747545,-26.9711324035108,
122.26320952748)) ;
#53143=CARTESIAN_POINT('Ctrl Pts',(-19.9009478345659,-26.7911433230303,
121.97604809687)) ;
#53144=CARTESIAN_POINT('Ctrl Pts',(-19.5282752383854,-26.9844082198528,
122.211739570841)) ;
#53145=CARTESIAN_POINT('Ctrl Pts',(-19.558049630064,-26.8044191393723,121.911724128013)) ;
#53146=CARTESIAN_POINT('Ctrl Pts',(-19.318603845964,-26.9943820706466,122.209154533502)) ;
#53147=CARTESIAN_POINT('Ctrl Pts',(-19.2959531359057,-26.8143929901661,
121.908486612894)) ;
#53148=CARTESIAN_POINT('Ctrl Pts',(-19.1105694524777,-27.004411102739,122.243420895193)) ;
#53149=CARTESIAN_POINT('Ctrl Pts',(-19.0359115385964,-26.8244220222585,
121.951317774941)) ;
#53150=CARTESIAN_POINT('Ctrl Pts',(-18.9143115037935,-27.0143012282409,
122.3121202507)) ;
#53151=CARTESIAN_POINT('Ctrl Pts',(-18.7905877642444,-26.8343121477604,
122.037189061852)) ;
#53152=CARTESIAN_POINT('Ctrl Pts',(-18.730980558228,-27.0242937065124,122.414640859144)) ;
#53153=CARTESIAN_POINT('Ctrl Pts',(-18.5614228029118,-26.8443046260319,
122.165337469909)) ;
#53154=CARTESIAN_POINT('Ctrl Pts',(-18.5687919015397,-27.0342449216098,
122.546836923164)) ;
#53155=CARTESIAN_POINT('Ctrl Pts',(-18.3586851594981,-26.8542558411293,
122.330580371029)) ;
#53156=CARTESIAN_POINT('Ctrl Pts',(-18.4308500276103,-27.0442934233648,
122.706804310669)) ;
#53157=CARTESIAN_POINT('Ctrl Pts',(-18.1862556412038,-26.8643043428843,
122.53053785768)) ;
#53158=CARTESIAN_POINT('Ctrl Pts',(-18.324778682574,-27.0541347729816,122.884464775646)) ;
#53159=CARTESIAN_POINT('Ctrl Pts',(-18.0536640722972,-26.8741456925011,
122.75261195662)) ;
#53160=CARTESIAN_POINT('Ctrl Pts',(-18.2496811215229,-27.0641210640018,
123.080480376407)) ;
#53161=CARTESIAN_POINT('Ctrl Pts',(-17.9597894557877,-26.8841319835213,
122.997630523659)) ;
#53162=CARTESIAN_POINT('Ctrl Pts',(-18.2098424384287,-27.0740576757304,
123.285580848838)) ;
#53163=CARTESIAN_POINT('Ctrl Pts',(-17.9099883259853,-26.8940685952499,
123.254005646112)) ;
#53164=CARTESIAN_POINT('Ctrl Pts',(-18.206286456587,-27.084107551098,123.496809557806)) ;
#53165=CARTESIAN_POINT('Ctrl Pts',(-17.9055405280551,-26.9041184706175,
123.518041545868)) ;
#53166=CARTESIAN_POINT('Ctrl Pts',(-18.2386548673565,-27.0939580096334,
123.701367310787)) ;
#53167=CARTESIAN_POINT('Ctrl Pts',(-17.9459982767413,-26.9139689291529,
123.773739288648)) ;
#53168=CARTESIAN_POINT('Ctrl Pts',(-18.3063479731576,-27.1039299465862,
123.899751686817)) ;
#53169=CARTESIAN_POINT('Ctrl Pts',(-18.0306120392557,-26.9239408661057,
124.021720774611)) ;
#53170=CARTESIAN_POINT('Ctrl Pts',(-18.4077546179831,-27.1139254035183,
124.083836779179)) ;
#53171=CARTESIAN_POINT('Ctrl Pts',(-18.1573679301595,-26.9339363230378,
124.251828560832)) ;
#53172=CARTESIAN_POINT('Ctrl Pts',(-18.5402337139463,-27.1239582105714,
124.247943977524)) ;
#53173=CARTESIAN_POINT('Ctrl Pts',(-18.3229646346915,-26.9439691300909,
124.456964358689)) ;
#53174=CARTESIAN_POINT('Ctrl Pts',(-18.696288367492,-27.1338180971613,124.384394875918)) ;
#53175=CARTESIAN_POINT('Ctrl Pts',(-18.5180312777449,-26.9538290166809,
124.627530239121)) ;
#53176=CARTESIAN_POINT('Ctrl Pts',(-18.8757602839204,-27.1438071777266,
124.493403942456)) ;
#53177=CARTESIAN_POINT('Ctrl Pts',(-18.7423698225916,-26.9638180972461,
124.763794005634)) ;
#53178=CARTESIAN_POINT('Ctrl Pts',(-19.0703285555277,-27.1537386569357,
124.569162296289)) ;
#53179=CARTESIAN_POINT('Ctrl Pts',(-18.9855793301058,-26.9737495764553,
124.858494604094)) ;
#53180=CARTESIAN_POINT('Ctrl Pts',(-19.2761569854026,-27.1637245163817,
124.610551053502)) ;
#53181=CARTESIAN_POINT('Ctrl Pts',(-19.2428644372017,-26.9837354359012,
124.91023326765)) ;
#53182=CARTESIAN_POINT('Ctrl Pts',(-19.4871247300181,-27.1737626670289,
124.61522608717)) ;
#53183=CARTESIAN_POINT('Ctrl Pts',(-19.5065740592413,-26.9937735865484,
124.916079842873)) ;
#53184=CARTESIAN_POINT('Ctrl Pts',(-19.6918470853474,-27.1836107575333,
124.584217748348)) ;
#53185=CARTESIAN_POINT('Ctrl Pts',(-19.762477808703,-27.0036216770528,124.877322071589)) ;
#53186=CARTESIAN_POINT('Ctrl Pts',(-19.8923339922519,-27.1936716660512,
124.516888561277)) ;
#53187=CARTESIAN_POINT('Ctrl Pts',(-20.0130872707817,-27.0136825855708,
124.793163185026)) ;
#53188=CARTESIAN_POINT('Ctrl Pts',(-20.0749863200746,-27.2035665132092,
124.417294329767)) ;
#53189=CARTESIAN_POINT('Ctrl Pts',(-20.2414042797993,-27.0235774327288,
124.668672645465)) ;
#53190=CARTESIAN_POINT('Ctrl Pts',(-20.2386525978464,-27.2135081852543,
124.287347778684)) ;
#53191=CARTESIAN_POINT('Ctrl Pts',(-20.4459889976083,-27.0335191047738,
124.506241389388)) ;
#53192=CARTESIAN_POINT('Ctrl Pts',(-20.3782156387396,-27.2235107123797,
124.130014539962)) ;
#53193=CARTESIAN_POINT('Ctrl Pts',(-20.62044484462,-27.0435216318993,124.309576543661)) ;
#53194=CARTESIAN_POINT('Ctrl Pts',(-20.4883897656227,-27.2335455035672,
123.950121732222)) ;
#53195=CARTESIAN_POINT('Ctrl Pts',(-20.7581648057283,-27.0535564230867,
124.084711962501)) ;
#53196=CARTESIAN_POINT('Ctrl Pts',(-20.5645263195821,-27.2433903834263,
123.757649358259)) ;
#53197=CARTESIAN_POINT('Ctrl Pts',(-20.8533381773429,-27.0634013029458,
123.844121950457)) ;
#53198=CARTESIAN_POINT('Ctrl Pts',(-20.6070596189447,-27.2533762640448,
123.552103054265)) ;
#53199=CARTESIAN_POINT('Ctrl Pts',(-20.9065073832557,-27.0733871835643,
123.587189440401)) ;
#53200=CARTESIAN_POINT('Ctrl Pts',(-20.6133781384881,-27.263310987138,123.343300034861)) ;
#53201=CARTESIAN_POINT('Ctrl Pts',(-20.9144081116271,-27.0833219066575,
123.326185418471)) ;
#53202=CARTESIAN_POINT('Ctrl Pts',(-20.5827915728053,-27.2733688274492,
123.134108713238)) ;
#53203=CARTESIAN_POINT('Ctrl Pts',(-20.8761775036442,-27.0933797469687,
123.064696003657)) ;
#53204=CARTESIAN_POINT('Ctrl Pts',(-20.5182131701365,-27.2831893148457,
122.937983170637)) ;
#53205=CARTESIAN_POINT('Ctrl Pts',(-20.7954566742065,-27.1032002343652,
122.819537535194)) ;
#53206=CARTESIAN_POINT('Ctrl Pts',(-20.4185100813219,-27.2932497161908,
122.751485493187)) ;
#53207=CARTESIAN_POINT('Ctrl Pts',(-20.6708300596876,-27.1132606357103,
122.586414372741)) ;
#53208=CARTESIAN_POINT('Ctrl Pts',(-20.2893670926231,-27.3031806817437,
122.587408843276)) ;
#53209=CARTESIAN_POINT('Ctrl Pts',(-20.5094030854592,-27.1231916012632,
122.381316698496)) ;
#53210=CARTESIAN_POINT('Ctrl Pts',(-20.1339171194866,-27.3131195440802,
122.447821260435)) ;
#53211=CARTESIAN_POINT('Ctrl Pts',(-20.3150919760581,-27.1331304635997,
122.206830149551)) ;
#53212=CARTESIAN_POINT('Ctrl Pts',(-19.9557909141703,-27.3231052750064,
122.336681000777)) ;
#53213=CARTESIAN_POINT('Ctrl Pts',(-20.0924353594494,-27.1431161945259,
122.067902692348)) ;
#53214=CARTESIAN_POINT('Ctrl Pts',(-19.7602720484493,-27.3331296604338,
122.258075382976)) ;
#53215=CARTESIAN_POINT('Ctrl Pts',(-19.8480377025749,-27.1531405799533,
121.969643384991)) ;
#53216=CARTESIAN_POINT('Ctrl Pts',(-19.5565899889511,-27.3430329447871,
122.214817299832)) ;
#53217=CARTESIAN_POINT('Ctrl Pts',(-19.5934350819641,-27.1630438643066,
121.915568323224)) ;
#53218=CARTESIAN_POINT('Ctrl Pts',(-19.3452475882926,-27.3530929493651,
122.207539583544)) ;
#53219=CARTESIAN_POINT('Ctrl Pts',(-19.3292573389798,-27.1731038688846,
121.906468774083)) ;
#53220=CARTESIAN_POINT('Ctrl Pts',(-19.1402979082901,-27.3629362184342,
122.236294727092)) ;
#53221=CARTESIAN_POINT('Ctrl Pts',(-19.0730690560102,-27.1829471379537,
121.942410468897)) ;
#53222=CARTESIAN_POINT('Ctrl Pts',(-18.9404022090521,-27.3729267840419,
122.300676483571)) ;
#53223=CARTESIAN_POINT('Ctrl Pts',(-18.8231985705939,-27.1929377035614,
122.022885561969)) ;
#53224=CARTESIAN_POINT('Ctrl Pts',(-18.7558672982378,-27.3828549158207,
122.398221029593)) ;
#53225=CARTESIAN_POINT('Ctrl Pts',(-18.5925284414569,-27.2028658353402,
122.144814464852)) ;
#53226=CARTESIAN_POINT('Ctrl Pts',(-18.5898557423788,-27.3928428029016,
122.526807079815)) ;
#53227=CARTESIAN_POINT('Ctrl Pts',(-18.3850125183994,-27.2128537224211,
122.305545417157)) ;
#53228=CARTESIAN_POINT('Ctrl Pts',(-18.4482910581977,-27.4028787524703,
122.68324070113)) ;
#53229=CARTESIAN_POINT('Ctrl Pts',(-18.2080550366544,-27.2228896719898,
122.501085855534)) ;
#53230=CARTESIAN_POINT('Ctrl Pts',(-18.3377591304148,-27.4127336388491,
122.858492901612)) ;
#53231=CARTESIAN_POINT('Ctrl Pts',(-18.0698877943292,-27.2327445583686,
122.720150718042)) ;
#53232=CARTESIAN_POINT('Ctrl Pts',(-18.2579406650141,-27.422733053197,123.052931220241)) ;
#53233=CARTESIAN_POINT('Ctrl Pts',(-17.9701127118475,-27.2427439727165,
122.963197940017)) ;
#53234=CARTESIAN_POINT('Ctrl Pts',(-18.2133303124607,-27.4326282183875,
123.256154680513)) ;
#53235=CARTESIAN_POINT('Ctrl Pts',(-17.9143476219476,-27.252639137907,123.217227543727)) ;
#53236=CARTESIAN_POINT('Ctrl Pts',(-18.204564058286,-27.4426885370794,123.467444615832)) ;
#53237=CARTESIAN_POINT('Ctrl Pts',(-17.9033877646461,-27.262699456599,123.481339637192)) ;
#53238=CARTESIAN_POINT('Ctrl Pts',(-18.2319167259409,-27.4525386688555,
123.672729223044)) ;
#53239=CARTESIAN_POINT('Ctrl Pts',(-17.9375767427707,-27.272549588375,123.737946697401)) ;
#53240=CARTESIAN_POINT('Ctrl Pts',(-18.2951613085268,-27.4625692393058,
123.87388597203)) ;
#53241=CARTESIAN_POINT('Ctrl Pts',(-18.0166306720555,-27.2825801588253,
123.989393136794)) ;
#53242=CARTESIAN_POINT('Ctrl Pts',(-18.392639370384,-27.4725833899786,124.060501742582)) ;
#53243=CARTESIAN_POINT('Ctrl Pts',(-18.1384764759036,-27.2925943094981,
124.222663794601)) ;
#53244=CARTESIAN_POINT('Ctrl Pts',(-18.5192133454885,-27.482476323524,124.225536129967)) ;
#53245=CARTESIAN_POINT('Ctrl Pts',(-18.2966929163298,-27.3024872430435,
124.428958569374)) ;
#53246=CARTESIAN_POINT('Ctrl Pts',(-18.6738373848897,-27.4924658375142,
124.367619074625)) ;
#53247=CARTESIAN_POINT('Ctrl Pts',(-18.4899718702957,-27.3124767570338,
124.606563738886)) ;
#53248=CARTESIAN_POINT('Ctrl Pts',(-18.8501175734663,-27.5024196081667,
124.480434768082)) ;
#53249=CARTESIAN_POINT('Ctrl Pts',(-18.7103215044996,-27.3224305276862,
124.747585098985)) ;
#53250=CARTESIAN_POINT('Ctrl Pts',(-19.0451588516024,-27.5124673768272,
124.561494657488)) ;
#53251=CARTESIAN_POINT('Ctrl Pts',(-18.9541222140301,-27.3324782963468,
124.84891159702)) ;
#53252=CARTESIAN_POINT('Ctrl Pts',(-19.2470679046849,-27.522309103267,124.606762346263)) ;
#53253=CARTESIAN_POINT('Ctrl Pts',(-19.20650929812,-27.3423200227866,124.905498198181)) ;
#53254=CARTESIAN_POINT('Ctrl Pts',(-19.4567187804264,-27.5322946200898,
124.616878516761)) ;
#53255=CARTESIAN_POINT('Ctrl Pts',(-19.468573060207,-27.3523055396093,124.918145049147)) ;
#53256=CARTESIAN_POINT('Ctrl Pts',(-19.6640500637913,-27.5422339517853,
124.590629381917)) ;
#53257=CARTESIAN_POINT('Ctrl Pts',(-19.7277379052966,-27.3622448713049,
124.885335148881)) ;
#53258=CARTESIAN_POINT('Ctrl Pts',(-19.8656328349993,-27.5522737214829,
124.52812532427)) ;
#53259=CARTESIAN_POINT('Ctrl Pts',(-19.9797167084176,-27.3722846410024,
124.807206664891)) ;
#53260=CARTESIAN_POINT('Ctrl Pts',(-20.050539305733,-27.5621618827317,124.433105551511)) ;
#53261=CARTESIAN_POINT('Ctrl Pts',(-20.2108513393927,-27.3821728022512,
124.688432935448)) ;
#53262=CARTESIAN_POINT('Ctrl Pts',(-20.2180592426687,-27.5721514372341,
124.306460221141)) ;
#53263=CARTESIAN_POINT('Ctrl Pts',(-20.4202523050526,-27.3921623567536,
124.530127299279)) ;
#53264=CARTESIAN_POINT('Ctrl Pts',(-20.3604835812191,-27.5821098517577,
124.153021019065)) ;
#53265=CARTESIAN_POINT('Ctrl Pts',(-20.5982841262608,-27.4021207712772,
124.338329003616)) ;
#53266=CARTESIAN_POINT('Ctrl Pts',(-20.473871725562,-27.5920097645871,123.978479224777)) ;
#53267=CARTESIAN_POINT('Ctrl Pts',(-20.7400208954016,-27.4120206841066,
124.120151747233)) ;
#53268=CARTESIAN_POINT('Ctrl Pts',(-20.5563690525815,-27.602056464237,123.784065248068)) ;
#53269=CARTESIAN_POINT('Ctrl Pts',(-20.8431437132464,-27.4220673837565,
123.877134998745)) ;
#53270=CARTESIAN_POINT('Ctrl Pts',(-20.6033030576586,-27.6119563245426,
123.581267591945)) ;
#53271=CARTESIAN_POINT('Ctrl Pts',(-20.9018126857167,-27.4319672440621,
123.623637353375)) ;
#53272=CARTESIAN_POINT('Ctrl Pts',(-20.6145464495285,-27.622007728748,123.370284273142)) ;
#53273=CARTESIAN_POINT('Ctrl Pts',(-20.9158681863817,-27.4420186482676,
123.359908517839)) ;
#53274=CARTESIAN_POINT('Ctrl Pts',(-20.5894865428159,-27.6318887656692,
123.164040601756)) ;
#53275=CARTESIAN_POINT('Ctrl Pts',(-20.8845444217385,-27.4518996851887,
123.102102763074)) ;
#53276=CARTESIAN_POINT('Ctrl Pts',(-20.5285619224102,-27.6418885978467,
122.96287053044)) ;
#53277=CARTESIAN_POINT('Ctrl Pts',(-20.8083897019526,-27.4618995173662,
122.850639705346)) ;
#53278=CARTESIAN_POINT('Ctrl Pts',(-20.4345314205031,-27.6518066008316,
122.776728506564)) ;
#53279=CARTESIAN_POINT('Ctrl Pts',(-20.6908521997633,-27.4718175203511,
122.617961007216)) ;
#53280=CARTESIAN_POINT('Ctrl Pts',(-20.307917816095,-27.6618579067061,122.607595735028)) ;
#53281=CARTESIAN_POINT('Ctrl Pts',(-20.5325862277936,-27.4818688262257,
122.406544566008)) ;
#53282=CARTESIAN_POINT('Ctrl Pts',(-20.1567577654715,-27.6717277300977,
122.465387827078)) ;
#53283=CARTESIAN_POINT('Ctrl Pts',(-20.3436360269097,-27.4917386496172,
122.228783160542)) ;
#53284=CARTESIAN_POINT('Ctrl Pts',(-19.979678811247,-27.681801896148,122.349293202809)) ;
#53285=CARTESIAN_POINT('Ctrl Pts',(-20.1222882554318,-27.5018128156675,
122.083664260518)) ;
#53286=CARTESIAN_POINT('Ctrl Pts',(-19.7900524651862,-27.6916219802896,
122.267545505754)) ;
#53287=CARTESIAN_POINT('Ctrl Pts',(-19.8852542609095,-27.5116328998091,
121.981478175887)) ;
#53288=CARTESIAN_POINT('Ctrl Pts',(-19.5839641602467,-27.7017007070255,
122.218539726718)) ;
#53289=CARTESIAN_POINT('Ctrl Pts',(-19.6276445349011,-27.521711626545,121.92022023308)) ;
#53290=CARTESIAN_POINT('Ctrl Pts',(-19.3771678744328,-27.711552287675,122.206266541028)) ;
#53291=CARTESIAN_POINT('Ctrl Pts',(-19.3691479103132,-27.5315632071945,
121.904877852162)) ;
#53292=CARTESIAN_POINT('Ctrl Pts',(-19.1668198410956,-27.7216254159734,
122.230427368706)) ;
#53293=CARTESIAN_POINT('Ctrl Pts',(-19.1062132173185,-27.5416363354929,
121.93507808783)) ;
#53294=CARTESIAN_POINT('Ctrl Pts',(-18.9684654062851,-27.7314678938648,
122.289410143151)) ;
#53295=CARTESIAN_POINT('Ctrl Pts',(-18.8582685979339,-27.5514788133843,
122.008806224701)) ;
#53296=CARTESIAN_POINT('Ctrl Pts',(-18.7804810737789,-27.7414485004629,
122.382594626151)) ;
#53297=CARTESIAN_POINT('Ctrl Pts',(-18.6232876860456,-27.5614594199824,
122.125286522703)) ;
#53298=CARTESIAN_POINT('Ctrl Pts',(-18.6111314469125,-27.7514662094817,
122.50779197817)) ;
#53299=CARTESIAN_POINT('Ctrl Pts',(-18.4116002703336,-27.5714771290012,
122.281782687831)) ;
#53300=CARTESIAN_POINT('Ctrl Pts',(-18.46769289707,-27.7613523885191,122.65822099697)) ;
#53301=CARTESIAN_POINT('Ctrl Pts',(-18.2323009869276,-27.5813633080386,
122.469819398419)) ;
#53302=CARTESIAN_POINT('Ctrl Pts',(-18.3505632690495,-27.7714100010914,
122.834235024386)) ;
#53303=CARTESIAN_POINT('Ctrl Pts',(-18.0858887220002,-27.591420920611,122.689836403978)) ;
#53304=CARTESIAN_POINT('Ctrl Pts',(-18.2672711578626,-27.7812863944636,
123.024442583232)) ;
#53305=CARTESIAN_POINT('Ctrl Pts',(-17.9817726805274,-27.6012973139831,
122.927596725617)) ;
#53306=CARTESIAN_POINT('Ctrl Pts',(-18.2171766731924,-27.791281422614,123.228504736778)) ;
#53307=CARTESIAN_POINT('Ctrl Pts',(-17.9191542663906,-27.6112923421335,
123.182674524713)) ;
#53308=CARTESIAN_POINT('Ctrl Pts',(-18.2035981744951,-27.80130216946,123.438743704045)) ;
#53309=CARTESIAN_POINT('Ctrl Pts',(-17.9021807328002,-27.6213130889795,
123.445473162296)) ;
#53310=CARTESIAN_POINT('Ctrl Pts',(-18.2262128560997,-27.8112042381264,
123.645681904527)) ;
#53311=CARTESIAN_POINT('Ctrl Pts',(-17.9304488695077,-27.6312151576459,
123.704146901877)) ;
#53312=CARTESIAN_POINT('Ctrl Pts',(-18.284639933744,-27.8211949779461,123.847429809037)) ;
#53313=CARTESIAN_POINT('Ctrl Pts',(-18.0034825910525,-27.6412058974656,
123.9563320642)) ;
#53314=CARTESIAN_POINT('Ctrl Pts',(-18.3770881160731,-27.8311581741564,
124.035370273374)) ;
#53315=CARTESIAN_POINT('Ctrl Pts',(-18.1190427860943,-27.6511690936759,
124.19125816354)) ;
#53316=CARTESIAN_POINT('Ctrl Pts',(-18.4996327245681,-27.8410623584565,
124.203730145458)) ;
#53317=CARTESIAN_POINT('Ctrl Pts',(-18.2722240569279,-27.661073277976,124.401708795507)) ;
#53318=CARTESIAN_POINT('Ctrl Pts',(-18.652006072211,-27.8511228188474,124.350375168077)) ;
#53319=CARTESIAN_POINT('Ctrl Pts',(-18.4626903999136,-27.6711337383669,
124.585014918637)) ;
#53320=CARTESIAN_POINT('Ctrl Pts',(-18.8235862046144,-27.8609633647182,
124.466005825925)) ;
#53321=CARTESIAN_POINT('Ctrl Pts',(-18.6771667744732,-27.6809742842377,
124.729554078446)) ;
#53322=CARTESIAN_POINT('Ctrl Pts',(-19.0167402747536,-27.8710255854299,
124.552208647531)) ;
#53323=CARTESIAN_POINT('Ctrl Pts',(-18.9186090602696,-27.6910365049495,
124.837307374996)) ;
#53324=CARTESIAN_POINT('Ctrl Pts',(-19.2186463887635,-27.8809227284465,
124.602519019844)) ;
#53325=CARTESIAN_POINT('Ctrl Pts',(-19.1709926750218,-27.700933647966,124.900195583921)) ;
#53326=CARTESIAN_POINT('Ctrl Pts',(-19.4268700305496,-27.8908539048637,
124.617749388412)) ;
#53327=CARTESIAN_POINT('Ctrl Pts',(-19.4312729665514,-27.7108648243832,
124.919233320845)) ;
#53328=CARTESIAN_POINT('Ctrl Pts',(-19.6368755079311,-27.9008961186423,
124.596126506695)) ;
#53329=CARTESIAN_POINT('Ctrl Pts',(-19.6937795869261,-27.7209070381618,
124.892204557448)) ;
#53330=CARTESIAN_POINT('Ctrl Pts',(-19.8368447731837,-27.910782658845,124.539408291931)) ;
#53331=CARTESIAN_POINT('Ctrl Pts',(-19.9437421484284,-27.7307935783645,
124.821306255873)) ;
#53332=CARTESIAN_POINT('Ctrl Pts',(-20.026076968928,-27.9207762534504,124.448165743483)) ;
#53333=CARTESIAN_POINT('Ctrl Pts',(-20.1802824077118,-27.74078717297,124.707252644304)) ;
#53334=CARTESIAN_POINT('Ctrl Pts',(-20.1957478692997,-27.930720128608,124.326020666064)) ;
#53335=CARTESIAN_POINT('Ctrl Pts',(-20.3923713221862,-27.7507310481275,
124.554570637575)) ;
#53336=CARTESIAN_POINT('Ctrl Pts',(-20.3420563337105,-27.9406806647228,
124.176229596615)) ;
#53337=CARTESIAN_POINT('Ctrl Pts',(-20.5752568935258,-27.7606915842423,
124.367331130145)) ;
#53338=CARTESIAN_POINT('Ctrl Pts',(-20.4606861174511,-27.9506772680455,
124.002726210929)) ;
#53339=CARTESIAN_POINT('Ctrl Pts',(-20.7235437792058,-27.7706881875651,
124.150451479983)) ;
#53340=CARTESIAN_POINT('Ctrl Pts',(-20.5474206151358,-27.960710351,123.810462365008)) ;
#53341=CARTESIAN_POINT('Ctrl Pts',(-20.8319614752254,-27.7807212705196,
123.910121632777)) ;
#53342=CARTESIAN_POINT('Ctrl Pts',(-20.5987649896307,-27.9705615197016,
123.609829364369)) ;
#53343=CARTESIAN_POINT('Ctrl Pts',(-20.8961417942239,-27.7905724392211,
123.659328927923)) ;
#53344=CARTESIAN_POINT('Ctrl Pts',(-20.6152871156439,-27.9805240104005,
123.401046818215)) ;
#53345=CARTESIAN_POINT('Ctrl Pts',(-20.9167937430027,-27.80053492992,123.398350225032)) ;
#53346=CARTESIAN_POINT('Ctrl Pts',(-20.5949125271602,-27.9905524388182,
123.191192264674)) ;
#53347=CARTESIAN_POINT('Ctrl Pts',(-20.8913248729586,-27.8105633583378,
123.136032193831)) ;
#53348=CARTESIAN_POINT('Ctrl Pts',(-20.53914584983,-28.0004628061828,122.990457378277)) ;
#53349=CARTESIAN_POINT('Ctrl Pts',(-20.821615644239,-27.8204737257023,122.885112920353)) ;
#53350=CARTESIAN_POINT('Ctrl Pts',(-20.4496374418431,-28.0103976737979,
122.801740219199)) ;
#53351=CARTESIAN_POINT('Ctrl Pts',(-20.7097290523873,-27.8304085933174,
122.649216253035)) ;
#53352=CARTESIAN_POINT('Ctrl Pts',(-20.3272748886815,-28.0204388157769,
122.629733634215)) ;
#53353=CARTESIAN_POINT('Ctrl Pts',(-20.5567753119051,-27.8404497352964,
122.434208642508)) ;
#53354=CARTESIAN_POINT('Ctrl Pts',(-20.1793010965195,-28.0303259519801,
122.483741362788)) ;
#53355=CARTESIAN_POINT('Ctrl Pts',(-20.3718067250228,-27.8503368714996,
122.251718186762)) ;
#53356=CARTESIAN_POINT('Ctrl Pts',(-20.0066274113567,-28.0403182343835,
122.364130675041)) ;
#53357=CARTESIAN_POINT('Ctrl Pts',(-20.1559638842904,-27.860329153903,122.102205529622)) ;
#53358=CARTESIAN_POINT('Ctrl Pts',(-19.8165954509597,-28.0502667623487,
122.276745364225)) ;
#53359=CARTESIAN_POINT('Ctrl Pts',(-19.9184230348921,-27.8702776818682,
121.992974547454)) ;
#53360=CARTESIAN_POINT('Ctrl Pts',(-19.6146202820985,-28.0602034935108,
122.223467272798)) ;
#53361=CARTESIAN_POINT('Ctrl Pts',(-19.6659531803205,-27.8802144130303,
121.926377817634)) ;
#53362=CARTESIAN_POINT('Ctrl Pts',(-19.4054676734705,-28.0701867043708,
122.205721541684)) ;
#53363=CARTESIAN_POINT('Ctrl Pts',(-19.4045120642442,-27.8901976238903,
121.904196806999)) ;
#53364=CARTESIAN_POINT('Ctrl Pts',(-19.1952379005433,-28.0802298035207,
122.225046803646)) ;
#53365=CARTESIAN_POINT('Ctrl Pts',(-19.1417251311324,-27.9002407230402,
121.928354401077)) ;
#53366=CARTESIAN_POINT('Ctrl Pts',(-18.9956932343111,-28.0900607677956,
122.278974247708)) ;
#53367=CARTESIAN_POINT('Ctrl Pts',(-18.8922932247184,-27.9100716873151,
121.995765252323)) ;
#53368=CARTESIAN_POINT('Ctrl Pts',(-18.8039248705908,-28.1001336201815,
122.368723820022)) ;
#53369=CARTESIAN_POINT('Ctrl Pts',(-18.6525836804044,-27.920144539701,122.107953193198)) ;
#53370=CARTESIAN_POINT('Ctrl Pts',(-18.6342195703199,-28.1099977478933,
122.487946903188)) ;
#53371=CARTESIAN_POINT('Ctrl Pts',(-18.4404518361072,-27.9300086674128,
122.25698372832)) ;
#53372=CARTESIAN_POINT('Ctrl Pts',(-18.4851003678343,-28.1200199500282,
122.636789063921)) ;
#53373=CARTESIAN_POINT('Ctrl Pts',(-18.2540538809201,-27.9400308695477,
122.443037416563)) ;
#53374=CARTESIAN_POINT('Ctrl Pts',(-18.3644270649533,-28.1300471429966,
122.809651509413)) ;
#53375=CARTESIAN_POINT('Ctrl Pts',(-18.1032133228676,-27.9500580625161,
122.659116134809)) ;
#53376=CARTESIAN_POINT('Ctrl Pts',(-18.2768385867952,-28.1399027369636,
122.997405819395)) ;
#53377=CARTESIAN_POINT('Ctrl Pts',(-17.9937284541553,-27.9599136564831,
122.893810711227)) ;
#53378=CARTESIAN_POINT('Ctrl Pts',(-18.2220200004676,-28.1498599088289,
123.199439317662)) ;
#53379=CARTESIAN_POINT('Ctrl Pts',(-17.9252066475916,-27.9698708283484,
123.146353412734)) ;
#53380=CARTESIAN_POINT('Ctrl Pts',(-18.2033226183059,-28.1598987528273,
123.409644983658)) ;
#53381=CARTESIAN_POINT('Ctrl Pts',(-17.9018363924116,-27.9799096723468,
123.409110487333)) ;
#53382=CARTESIAN_POINT('Ctrl Pts',(-18.2207487622362,-28.1697727767028,
123.616522805315)) ;
#53383=CARTESIAN_POINT('Ctrl Pts',(-17.9236207435737,-27.9897836962224,
123.667708642649)) ;
#53384=CARTESIAN_POINT('Ctrl Pts',(-18.2748756328717,-28.1798426026932,
123.821155710981)) ;
#53385=CARTESIAN_POINT('Ctrl Pts',(-17.9912807795422,-27.9998535222128,
123.923499029308)) ;
#53386=CARTESIAN_POINT('Ctrl Pts',(-18.3615430076775,-28.1896758465905,
124.008855877301)) ;
#53387=CARTESIAN_POINT('Ctrl Pts',(-18.0996170114153,-28.00968676611,124.158124720537)) ;
#53388=CARTESIAN_POINT('Ctrl Pts',(-18.4813453459947,-28.1997062743635,
124.18238158238)) ;
#53389=CARTESIAN_POINT('Ctrl Pts',(-18.2493713826694,-28.0197171938831,
124.37503074541)) ;
#53390=CARTESIAN_POINT('Ctrl Pts',(-18.6299243812976,-28.2097378911087,
124.332069289836)) ;
#53391=CARTESIAN_POINT('Ctrl Pts',(-18.4350962679651,-28.0297488106282,
124.562139179393)) ;
#53392=CARTESIAN_POINT('Ctrl Pts',(-18.7984985629321,-28.2195675680894,
124.451573981328)) ;
#53393=CARTESIAN_POINT('Ctrl Pts',(-18.6458160518969,-28.0395784876089,
124.711519341909)) ;
#53394=CARTESIAN_POINT('Ctrl Pts',(-18.9880488787878,-28.2295570849293,
124.542006375535)) ;
#53395=CARTESIAN_POINT('Ctrl Pts',(-18.8827549499808,-28.0495680044489,
124.824558144054)) ;
#53396=CARTESIAN_POINT('Ctrl Pts',(-19.1916515256229,-28.2396006970691,
124.597937925507)) ;
#53397=CARTESIAN_POINT('Ctrl Pts',(-19.1372585886768,-28.0596116165886,
124.894470815725)) ;
#53398=CARTESIAN_POINT('Ctrl Pts',(-19.3972114936263,-28.2494233034044,
124.617664945189)) ;
#53399=CARTESIAN_POINT('Ctrl Pts',(-19.3942099817859,-28.0694342229239,
124.919127791887)) ;
#53400=CARTESIAN_POINT('Ctrl Pts',(-19.6076212256826,-28.2594615333036,
124.601522484725)) ;
#53401=CARTESIAN_POINT('Ctrl Pts',(-19.6572218646358,-28.0794724528232,
124.898947663215)) ;
#53402=CARTESIAN_POINT('Ctrl Pts',(-19.8113776911949,-28.2694725680956,
124.548753711217)) ;
#53403=CARTESIAN_POINT('Ctrl Pts',(-19.9119170105172,-28.0894834876151,
124.832984826556)) ;
#53404=CARTESIAN_POINT('Ctrl Pts',(-20.0008298539462,-28.2793702990627,
124.462706665286)) ;
#53405=CARTESIAN_POINT('Ctrl Pts',(-20.1487320478173,-28.0993812185822,
124.725423875452)) ;
#53406=CARTESIAN_POINT('Ctrl Pts',(-20.1742139857442,-28.2893599269132,
124.344205140818)) ;
#53407=CARTESIAN_POINT('Ctrl Pts',(-20.3654611749712,-28.1093708464327,
124.577295140952)) ;
#53408=CARTESIAN_POINT('Ctrl Pts',(-20.3238283363393,-28.2993157173592,
124.19784376409)) ;
#53409=CARTESIAN_POINT('Ctrl Pts',(-20.5524779417521,-28.1193266368787,
124.394341663562)) ;
#53410=CARTESIAN_POINT('Ctrl Pts',(-20.4457396566452,-28.3092431159212,
124.028437006786)) ;
#53411=CARTESIAN_POINT('Ctrl Pts',(-20.704865620646,-28.1292540354408,124.182581520384)) ;
#53412=CARTESIAN_POINT('Ctrl Pts',(-20.5372193180134,-28.3192687110311,
123.838562812821)) ;
#53413=CARTESIAN_POINT('Ctrl Pts',(-20.8192132353029,-28.1392796305506,
123.945237856662)) ;
#53414=CARTESIAN_POINT('Ctrl Pts',(-20.5936698159923,-28.3291545617007,
123.638543561245)) ;
#53415=CARTESIAN_POINT('Ctrl Pts',(-20.8897744389928,-28.1491654812202,
123.695212486605)) ;
#53416=CARTESIAN_POINT('Ctrl Pts',(-20.6152462524492,-28.3391437415449,
123.429645094941)) ;
#53417=CARTESIAN_POINT('Ctrl Pts',(-20.9167426864684,-28.1591546610644,
123.434089007645)) ;
#53418=CARTESIAN_POINT('Ctrl Pts',(-20.5997049484337,-28.3491849286484,
123.219121094953)) ;
#53419=CARTESIAN_POINT('Ctrl Pts',(-20.8973138531456,-28.169195848168,123.170934263091)) ;
#53420=CARTESIAN_POINT('Ctrl Pts',(-20.5492532199071,-28.3590175721244,
123.018663279547)) ;
#53421=CARTESIAN_POINT('Ctrl Pts',(-20.834246726357,-28.1790284916439,122.920361624785)) ;
#53422=CARTESIAN_POINT('Ctrl Pts',(-20.4639239618416,-28.3690115218339,
122.826668029978)) ;
#53423=CARTESIAN_POINT('Ctrl Pts',(-20.7275828727774,-28.1890224413534,
122.680368443555)) ;
#53424=CARTESIAN_POINT('Ctrl Pts',(-20.3457702484628,-28.3790406446104,
122.652037807507)) ;
#53425=CARTESIAN_POINT('Ctrl Pts',(-20.579888806851,-28.1990515641299,122.46208199399)) ;
#53426=CARTESIAN_POINT('Ctrl Pts',(-20.2015610995993,-28.3889167755291,
122.502648999928)) ;
#53427=CARTESIAN_POINT('Ctrl Pts',(-20.3996251642612,-28.2089276950486,
122.275347174398)) ;
#53428=CARTESIAN_POINT('Ctrl Pts',(-20.0317039479304,-28.3989148105461,
122.37888357769)) ;
#53429=CARTESIAN_POINT('Ctrl Pts',(-20.1873021800458,-28.2189257300656,
122.120642324578)) ;
#53430=CARTESIAN_POINT('Ctrl Pts',(-19.8445504166726,-28.4088287403048,
122.287101606991)) ;
#53431=CARTESIAN_POINT('Ctrl Pts',(-19.9533587456366,-28.2288396598243,
122.00591689841)) ;
#53432=CARTESIAN_POINT('Ctrl Pts',(-19.6417453548372,-28.4188719280426,
122.228424618647)) ;
#53433=CARTESIAN_POINT('Ctrl Pts',(-19.6998517914313,-28.2388828475621,
121.932573093112)) ;
#53434=CARTESIAN_POINT('Ctrl Pts',(-19.4348032819945,-28.428771770183,122.206158950053)) ;
#53435=CARTESIAN_POINT('Ctrl Pts',(-19.441173435824,-28.2487826897025,121.904743447041)) ;
#53436=CARTESIAN_POINT('Ctrl Pts',(-19.225199951328,-28.438763036991,122.219845479332)) ;
#53437=CARTESIAN_POINT('Ctrl Pts',(-19.1791693222261,-28.2587739565105,
121.921854203863)) ;
#53438=CARTESIAN_POINT('Ctrl Pts',(-19.0204087974407,-28.4487951391229,
122.270276783567)) ;
#53439=CARTESIAN_POINT('Ctrl Pts',(-18.9231809982585,-28.2688060586425,
121.984895781266)) ;
#53440=CARTESIAN_POINT('Ctrl Pts',(-18.8305583447142,-28.4586620200777,
122.353843034253)) ;
#53441=CARTESIAN_POINT('Ctrl Pts',(-18.6858684266711,-28.2786729395972,
122.089356190467)) ;
#53442=CARTESIAN_POINT('Ctrl Pts',(-18.6556330787561,-28.4686538113658,
122.470151417965)) ;
#53443=CARTESIAN_POINT('Ctrl Pts',(-18.4672132263357,-28.2886647308854,
122.234743944221)) ;
#53444=CARTESIAN_POINT('Ctrl Pts',(-18.5032314430184,-28.4786859272774,
122.61594277691)) ;
#53445=CARTESIAN_POINT('Ctrl Pts',(-18.276712974009,-28.2986968467969,122.416985014453)) ;
#53446=CARTESIAN_POINT('Ctrl Pts',(-18.380260915545,-28.4885522440774,122.782991829368)) ;
#53447=CARTESIAN_POINT('Ctrl Pts',(-18.1230016339298,-28.3085631635969,
122.625798314926)) ;
#53448=CARTESIAN_POINT('Ctrl Pts',(-18.286740408124,-28.498539725551,122.970954331532)) ;
#53449=CARTESIAN_POINT('Ctrl Pts',(-18.0061033567244,-28.3185506450705,
122.860752752778)) ;
#53450=CARTESIAN_POINT('Ctrl Pts',(-18.2274077058308,-28.5084846499299,
123.171464369965)) ;
#53451=CARTESIAN_POINT('Ctrl Pts',(-17.931940003729,-28.3284955694494,123.111391293671)) ;
#53452=CARTESIAN_POINT('Ctrl Pts',(-18.2036772806348,-28.5185295358406,
123.381282408305)) ;
#53453=CARTESIAN_POINT('Ctrl Pts',(-17.9022796486701,-28.3385404553601,
123.373664123606)) ;
#53454=CARTESIAN_POINT('Ctrl Pts',(-18.2163217636226,-28.5283916395532,
123.588243745579)) ;
#53455=CARTESIAN_POINT('Ctrl Pts',(-17.9180879854139,-28.3484025590727,
123.632366059938)) ;
#53456=CARTESIAN_POINT('Ctrl Pts',(-18.2649253863527,-28.5383832033776,
123.792581695052)) ;
#53457=CARTESIAN_POINT('Ctrl Pts',(-17.9788452221271,-28.3583941228972,
123.887787950783)) ;
#53458=CARTESIAN_POINT('Ctrl Pts',(-18.3478659471332,-28.5483160114405,
123.984221813374)) ;
#53459=CARTESIAN_POINT('Ctrl Pts',(-18.0825235358457,-28.3683269309601,
124.127337211431)) ;
#53460=CARTESIAN_POINT('Ctrl Pts',(-18.4624497179601,-28.5582531136769,
124.158918671784)) ;
#53461=CARTESIAN_POINT('Ctrl Pts',(-18.2257556809892,-28.3782640331964,
124.345706898359)) ;
#53462=CARTESIAN_POINT('Ctrl Pts',(-18.6074717807451,-28.5683055599473,
124.312619227432)) ;
#53463=CARTESIAN_POINT('Ctrl Pts',(-18.4070352869244,-28.3883164794668,
124.537830699445)) ;
#53464=CARTESIAN_POINT('Ctrl Pts',(-18.7733489453358,-28.5781516755289,
124.436472624767)) ;
#53465=CARTESIAN_POINT('Ctrl Pts',(-18.6143836430854,-28.3981625950484,
124.692645379623)) ;
#53466=CARTESIAN_POINT('Ctrl Pts',(-18.9618249797804,-28.5881996952438,
124.531831590146)) ;
#53467=CARTESIAN_POINT('Ctrl Pts',(-18.8499799672981,-28.4082106147633,
124.811841582675)) ;
#53468=CARTESIAN_POINT('Ctrl Pts',(-19.1619711895627,-28.5981416468727,
124.592099396301)) ;
#53469=CARTESIAN_POINT('Ctrl Pts',(-19.1001636768918,-28.4181525663922,
124.887173703538)) ;
#53470=CARTESIAN_POINT('Ctrl Pts',(-19.36940458292,-28.6080804278718,124.617204452178)) ;
#53471=CARTESIAN_POINT('Ctrl Pts',(-19.3594558684191,-28.4280913473913,
124.918552242727)) ;
#53472=CARTESIAN_POINT('Ctrl Pts',(-19.5798534901081,-28.6181064765979,
124.605652962537)) ;
#53473=CARTESIAN_POINT('Ctrl Pts',(-19.6225169288704,-28.4381173961174,
124.904110048559)) ;
#53474=CARTESIAN_POINT('Ctrl Pts',(-19.7823487906233,-28.6279933370061,
124.558649540917)) ;
#53475=CARTESIAN_POINT('Ctrl Pts',(-19.8756354818893,-28.4480042565256,
124.845353062541)) ;
#53476=CARTESIAN_POINT('Ctrl Pts',(-19.9763812601013,-28.6380246121379,
124.476122124052)) ;
#53477=CARTESIAN_POINT('Ctrl Pts',(-20.1181752201208,-28.4580355316574,
124.742190925263)) ;
#53478=CARTESIAN_POINT('Ctrl Pts',(-20.1507052106711,-28.6479075894383,
124.362992233123)) ;
#53479=CARTESIAN_POINT('Ctrl Pts',(-20.3360779498188,-28.4679185089578,
124.600777052441)) ;
#53480=CARTESIAN_POINT('Ctrl Pts',(-20.3053443200726,-28.6579644428455,
124.218890410107)) ;
#53481=CARTESIAN_POINT('Ctrl Pts',(-20.5293776950201,-28.477975362365,124.420644315049)) ;
#53482=CARTESIAN_POINT('Ctrl Pts',(-20.4724604666755,-28.6711326839214,
123.998058155589)) ;
#53483=CARTESIAN_POINT('Ctrl Pts',(-20.738256336222,-28.4911436034409,124.144618304064)) ;
#53484=CARTESIAN_POINT('Ctrl Pts',(-20.5799131365806,-28.6845337131479,
123.73425819107)) ;
#53485=CARTESIAN_POINT('Ctrl Pts',(-20.8725696185319,-28.5045446326674,
123.814898573048)) ;
#53486=CARTESIAN_POINT('Ctrl Pts',(-20.6142236375671,-28.6977466298788,
123.458567013862)) ;
#53487=CARTESIAN_POINT('Ctrl Pts',(-20.9154664866282,-28.5177575493983,
123.470229804434)) ;
#53488=CARTESIAN_POINT('Ctrl Pts',(-20.604352967794,-28.707675024332,123.250109379369)) ;
#53489=CARTESIAN_POINT('Ctrl Pts',(-20.9031228606174,-28.5276859438515,
123.209668872552)) ;
#53490=CARTESIAN_POINT('Ctrl Pts',(-20.5583282587321,-28.7176565244601,
123.045346923892)) ;
#53491=CARTESIAN_POINT('Ctrl Pts',(-20.8455899285438,-28.5376674439796,
122.953713451743)) ;
#53492=CARTESIAN_POINT('Ctrl Pts',(-20.4767166915395,-28.7276970677302,
122.850689815527)) ;
#53493=CARTESIAN_POINT('Ctrl Pts',(-20.7435726951601,-28.5477079872497,
122.710393832247)) ;
#53494=CARTESIAN_POINT('Ctrl Pts',(-20.3649428036905,-28.7375463995133,
122.676381992891)) ;
#53495=CARTESIAN_POINT('Ctrl Pts',(-20.6038530331542,-28.5575573190328,
122.492510433852)) ;
#53496=CARTESIAN_POINT('Ctrl Pts',(-20.2229203006753,-28.747541803985,122.521509294334)) ;
#53497=CARTESIAN_POINT('Ctrl Pts',(-20.4263234255606,-28.5675527235045,
122.298921849141)) ;
#53498=CARTESIAN_POINT('Ctrl Pts',(-20.0555849748291,-28.7575581314336,
122.393679057562)) ;
#53499=CARTESIAN_POINT('Ctrl Pts',(-20.2171504398344,-28.5775690509531,
122.139134607409)) ;
#53500=CARTESIAN_POINT('Ctrl Pts',(-19.8088912325934,-28.7707817886001,
122.265428926498)) ;
#53501=CARTESIAN_POINT('Ctrl Pts',(-19.9087920778577,-28.5907927081196,
121.978832990084)) ;
#53502=CARTESIAN_POINT('Ctrl Pts',(-19.5330216381452,-28.7840760799895,
122.203967929054)) ;
#53503=CARTESIAN_POINT('Ctrl Pts',(-19.5639959876234,-28.604086999509,121.902007063373)) ;
#53504=CARTESIAN_POINT('Ctrl Pts',(-19.2539859157199,-28.797360430921,122.215868648645)) ;
#53505=CARTESIAN_POINT('Ctrl Pts',(-19.2151418343441,-28.6173713504405,
121.916882629458)) ;
#53506=CARTESIAN_POINT('Ctrl Pts',(-19.0492445151565,-28.8073328119828,
122.260874137876)) ;
#53507=CARTESIAN_POINT('Ctrl Pts',(-18.9592277476723,-28.6273437315023,
121.973142750564)) ;
#53508=CARTESIAN_POINT('Ctrl Pts',(-18.8564919194603,-28.8172411916084,
122.339917001314)) ;
#53509=CARTESIAN_POINT('Ctrl Pts',(-18.7182849242685,-28.6372521111279,
122.071948770138)) ;
#53510=CARTESIAN_POINT('Ctrl Pts',(-18.6778931742279,-28.8272951903564,
122.452918665696)) ;
#53511=CARTESIAN_POINT('Ctrl Pts',(-18.4950390576537,-28.647306109876,122.213201779879)) ;
#53512=CARTESIAN_POINT('Ctrl Pts',(-18.524471696003,-28.8371573874727,122.592405825859)) ;
#53513=CARTESIAN_POINT('Ctrl Pts',(-18.3032620687074,-28.6571683069923,
122.387567726256)) ;
#53514=CARTESIAN_POINT('Ctrl Pts',(-18.3524307607685,-28.8505045138469,
122.814082154856)) ;
#53515=CARTESIAN_POINT('Ctrl Pts',(-18.0882237965495,-28.6705154333664,
122.664637872048)) ;
#53516=CARTESIAN_POINT('Ctrl Pts',(-18.2159876348167,-28.8670414794883,
123.138150036716)) ;
#53517=CARTESIAN_POINT('Ctrl Pts',(-17.9176634710199,-28.6870523990078,
123.069772556829)) ;
#53518=CARTESIAN_POINT('Ctrl Pts',(-18.1976653162901,-28.8836760836622,
123.491362438096)) ;
#53519=CARTESIAN_POINT('Ctrl Pts',(-17.8947632867105,-28.7036870031818,
123.511208297094)) ;
#53520=CARTESIAN_POINT('Ctrl Pts',(-18.2560525173173,-28.8969658769049,
123.764590199396)) ;
#53521=CARTESIAN_POINT('Ctrl Pts',(-17.9677541224921,-28.7169767964244,
123.852806493827)) ;
#53522=CARTESIAN_POINT('Ctrl Pts',(-18.3343741631932,-28.9069185081643,
123.958600107731)) ;
#53523=CARTESIAN_POINT('Ctrl Pts',(-18.0656567607898,-28.7269294276838,
124.095304375522)) ;
#53524=CARTESIAN_POINT('Ctrl Pts',(-18.4449965967694,-28.916870475469,124.136207394979)) ;
#53525=CARTESIAN_POINT('Ctrl Pts',(-18.2039394801543,-28.7368813949885,
124.317317362376)) ;
#53526=CARTESIAN_POINT('Ctrl Pts',(-18.6328431511708,-28.9302377339328,
124.345197379133)) ;
#53527=CARTESIAN_POINT('Ctrl Pts',(-18.4387363199644,-28.7502486534523,
124.578542730308)) ;
#53528=CARTESIAN_POINT('Ctrl Pts',(-18.9269841780433,-28.9467545458819,
124.537227554656)) ;
#53529=CARTESIAN_POINT('Ctrl Pts',(-18.8064292375309,-28.7667654654015,
124.818587726068)) ;
#53530=CARTESIAN_POINT('Ctrl Pts',(-19.3414615997305,-28.9667804408883,
124.634301072555)) ;
#53531=CARTESIAN_POINT('Ctrl Pts',(-19.3245222155823,-28.7867913604078,
124.939922033255)) ;
#53532=CARTESIAN_POINT('Ctrl Pts',(-19.759850235118,-28.9865911710184,124.584749330712)) ;
#53533=CARTESIAN_POINT('Ctrl Pts',(-19.8475073461012,-28.806602090538,124.877979440318)) ;
#53534=CARTESIAN_POINT('Ctrl Pts',(-20.1396804889429,-29.0065683871483,
124.394678367115)) ;
#53535=CARTESIAN_POINT('Ctrl Pts',(-20.322293027408,-28.8265793066678,124.640387404806)) ;
#53536=CARTESIAN_POINT('Ctrl Pts',(-20.4305598017003,-29.0264952625436,
124.086638339135)) ;
#53537=CARTESIAN_POINT('Ctrl Pts',(-20.6858890815036,-28.8465061820631,
124.255335344435)) ;
#53538=CARTESIAN_POINT('Ctrl Pts',(-20.5992504484349,-29.0463167240198,
123.700349376274)) ;
#53539=CARTESIAN_POINT('Ctrl Pts',(-20.8967489378324,-28.8663276435394,
123.772474684078)) ;
#53540=CARTESIAN_POINT('Ctrl Pts',(-20.626046085885,-29.0663910418292,123.274422117827)) ;
#53541=CARTESIAN_POINT('Ctrl Pts',(-20.9302406515358,-28.8864019613487,
123.24006458239)) ;
#53542=CARTESIAN_POINT('Ctrl Pts',(-20.506795066352,-29.0862390108371,122.869477985307)) ;
#53543=CARTESIAN_POINT('Ctrl Pts',(-20.7811745277581,-28.9062499303566,
122.73388681703)) ;
#53544=CARTESIAN_POINT('Ctrl Pts',(-20.2560944539261,-29.1061860449003,
122.527490551716)) ;
#53545=CARTESIAN_POINT('Ctrl Pts',(-20.467797326148,-28.9261969644198,122.306404432427)) ;
#53546=CARTESIAN_POINT('Ctrl Pts',(-19.9044790885967,-29.1260819958724,
122.292205363375)) ;
#53547=CARTESIAN_POINT('Ctrl Pts',(-20.028278033369,-28.946092915392,122.012300463349)) ;
#53548=CARTESIAN_POINT('Ctrl Pts',(-19.493912747964,-29.1459774754907,122.190368785616)) ;
#53549=CARTESIAN_POINT('Ctrl Pts',(-19.5150711784691,-28.9659883950102,
121.885006524989)) ;
#53550=CARTESIAN_POINT('Ctrl Pts',(-19.0718902420119,-29.1659335864555,
122.234795537404)) ;
#53551=CARTESIAN_POINT('Ctrl Pts',(-18.9875437561079,-28.985944505975,121.940541079164)) ;
#53552=CARTESIAN_POINT('Ctrl Pts',(-18.6914823643913,-29.1858381344955,
122.420160422829)) ;
#53553=CARTESIAN_POINT('Ctrl Pts',(-18.5120357099676,-29.005849054015,122.172247469313)) ;
#53554=CARTESIAN_POINT('Ctrl Pts',(-18.3967545767849,-29.2057122588146,
122.723103992137)) ;
#53555=CARTESIAN_POINT('Ctrl Pts',(-18.1436273508337,-29.0257231783341,
122.550925494711)) ;
#53556=CARTESIAN_POINT('Ctrl Pts',(-18.2221384336728,-29.2257667888136,
123.11205184558)) ;
#53557=CARTESIAN_POINT('Ctrl Pts',(-17.9253569899085,-29.0457777083331,
123.037111210443)) ;
#53558=CARTESIAN_POINT('Ctrl Pts',(-18.190981362348,-29.2455743025736,123.532149795036)) ;
#53559=CARTESIAN_POINT('Ctrl Pts',(-17.8864107134353,-29.0655852220931,
123.562230606224)) ;
#53560=CARTESIAN_POINT('Ctrl Pts',(-18.3051612613185,-29.2655576583413,
123.941359506721)) ;
#53561=CARTESIAN_POINT('Ctrl Pts',(-18.0291344863836,-29.0855685778608,
124.073742812839)) ;
#53562=CARTESIAN_POINT('Ctrl Pts',(-18.5518768276411,-29.2854759609252,
124.285589142629)) ;
#53563=CARTESIAN_POINT('Ctrl Pts',(-18.337527532579,-29.1054868804448,124.504029337641)) ;
#53564=CARTESIAN_POINT('Ctrl Pts',(-18.8998033234493,-29.305344176371,124.525350894694)) ;
#53565=CARTESIAN_POINT('Ctrl Pts',(-18.7724331767163,-29.1253550958905,
124.803732067833)) ;
#53566=CARTESIAN_POINT('Ctrl Pts',(-19.3123749934706,-29.3253944931673,
124.632263603809)) ;
#53567=CARTESIAN_POINT('Ctrl Pts',(-19.2881479518997,-29.1454054126868,
124.937374691363)) ;
#53568=CARTESIAN_POINT('Ctrl Pts',(-19.7312061051285,-29.3451705550497,
124.593056434788)) ;
#53569=CARTESIAN_POINT('Ctrl Pts',(-19.8116842877083,-29.1651814745693,
124.888368150248)) ;
#53570=CARTESIAN_POINT('Ctrl Pts',(-20.1166949902579,-29.3652251607422,
124.411179447447)) ;
#53571=CARTESIAN_POINT('Ctrl Pts',(-20.2935470560524,-29.1852360802617,
124.661024000832)) ;
#53572=CARTESIAN_POINT('Ctrl Pts',(-20.413193850282,-29.3850188498981,124.112306030586)) ;
#53573=CARTESIAN_POINT('Ctrl Pts',(-20.6641709205852,-29.2050297694176,
124.28743570741)) ;
#53574=CARTESIAN_POINT('Ctrl Pts',(-20.5924104104792,-29.4049855414925,
123.727541429383)) ;
#53575=CARTESIAN_POINT('Ctrl Pts',(-20.888194638405,-29.224996461012,123.806481690376)) ;
#53576=CARTESIAN_POINT('Ctrl Pts',(-20.6289121024175,-29.4249455872434,
123.304630992729)) ;
#53577=CARTESIAN_POINT('Ctrl Pts',(-20.9338249695065,-29.244956506763,123.277844260725)) ;
#53578=CARTESIAN_POINT('Ctrl Pts',(-20.5195428798539,-29.4448438473937,
122.895946670909)) ;
#53579=CARTESIAN_POINT('Ctrl Pts',(-20.7971171358388,-29.2648547669132,
122.766988876723)) ;
#53580=CARTESIAN_POINT('Ctrl Pts',(-20.2777340208433,-29.4647387629429,
122.548875500711)) ;
#53581=CARTESIAN_POINT('Ctrl Pts',(-20.4948597931304,-29.2847496824624,
122.333148374869)) ;
#53582=CARTESIAN_POINT('Ctrl Pts',(-19.9319526108886,-29.4846489433565,
122.30463596634)) ;
#53583=CARTESIAN_POINT('Ctrl Pts',(-20.0626359965801,-29.304659862876,122.027845909541)) ;
#53584=CARTESIAN_POINT('Ctrl Pts',(-19.5230900240382,-29.5045847424707,
122.192721165908)) ;
#53585=CARTESIAN_POINT('Ctrl Pts',(-19.5515593327358,-29.3245956619903,
121.887948224183)) ;
#53586=CARTESIAN_POINT('Ctrl Pts',(-19.1005503152697,-29.5245226041249,
122.227022561574)) ;
#53587=CARTESIAN_POINT('Ctrl Pts',(-19.023384693824,-29.3445335236444,121.930820616893)) ;
#53588=CARTESIAN_POINT('Ctrl Pts',(-18.7153085805982,-29.5444416507625,
122.403062773862)) ;
#53589=CARTESIAN_POINT('Ctrl Pts',(-18.5418309888662,-29.3644525702821,
122.150865733139)) ;
#53590=CARTESIAN_POINT('Ctrl Pts',(-18.4127914875677,-29.5643905488167,
122.700380117268)) ;
#53591=CARTESIAN_POINT('Ctrl Pts',(-18.1636813292534,-29.3844014683362,
122.52251140325)) ;
#53592=CARTESIAN_POINT('Ctrl Pts',(-18.2301756318706,-29.5842963762597,
123.082237752554)) ;
#53593=CARTESIAN_POINT('Ctrl Pts',(-17.9354075382581,-29.4043072957793,
122.99982127121)) ;
#53594=CARTESIAN_POINT('Ctrl Pts',(-18.1953684956847,-29.600879071625,123.433028159498)) ;
#53595=CARTESIAN_POINT('Ctrl Pts',(-17.8918934977912,-29.4208899911446,
123.438338526595)) ;
#53596=CARTESIAN_POINT('Ctrl Pts',(-18.24027601235,-29.6141532853487,123.708522208439)) ;
#53597=CARTESIAN_POINT('Ctrl Pts',(-17.9480247350242,-29.4341642048682,
123.78267941021)) ;
#53598=CARTESIAN_POINT('Ctrl Pts',(-18.3100397706379,-29.624200004548,123.907851703837)) ;
#53599=CARTESIAN_POINT('Ctrl Pts',(-18.0352295819817,-29.4442109240675,
124.031850013709)) ;
#53600=CARTESIAN_POINT('Ctrl Pts',(-18.4110966673818,-29.6340440391937,
124.088481382499)) ;
#53601=CARTESIAN_POINT('Ctrl Pts',(-18.1615379685972,-29.4540549587132,
124.257627504453)) ;
#53602=CARTESIAN_POINT('Ctrl Pts',(-18.5878370635189,-29.6473784240982,
124.305998065082)) ;
#53603=CARTESIAN_POINT('Ctrl Pts',(-18.3825117399585,-29.4673893436177,
124.529570908678)) ;
#53604=CARTESIAN_POINT('Ctrl Pts',(-18.8736671997377,-29.663965641398,124.512799362027)) ;
#53605=CARTESIAN_POINT('Ctrl Pts',(-18.7397290348442,-29.4839765609175,
124.788022651668)) ;
#53606=CARTESIAN_POINT('Ctrl Pts',(-19.2135861785788,-29.6805988534359,
124.610126724355)) ;
#53607=CARTESIAN_POINT('Ctrl Pts',(-19.1646822605497,-29.5006097729554,
124.909710774765)) ;
#53608=CARTESIAN_POINT('Ctrl Pts',(-19.4928463617671,-29.6938812957081,
124.61484124617)) ;
#53609=CARTESIAN_POINT('Ctrl Pts',(-19.5137203885411,-29.5138922152276,
124.915596996321)) ;
#53610=CARTESIAN_POINT('Ctrl Pts',(-19.6985621110543,-29.7037871836223,
124.582563757789)) ;
#53611=CARTESIAN_POINT('Ctrl Pts',(-19.7708729287918,-29.5237981031418,
124.875254844547)) ;
#53612=CARTESIAN_POINT('Ctrl Pts',(-19.8973061665422,-29.7137756017274,
124.514736011145)) ;
#53613=CARTESIAN_POINT('Ctrl Pts',(-20.0193014855349,-29.5337865212469,
124.790472867402)) ;
#53614=CARTESIAN_POINT('Ctrl Pts',(-20.0817838352029,-29.7237990289661,
124.412880710944)) ;
#53615=CARTESIAN_POINT('Ctrl Pts',(-20.2499022752962,-29.5438099484857,
124.663153811416)) ;
#53616=CARTESIAN_POINT('Ctrl Pts',(-20.2438922250525,-29.7337034600831,
124.282207760991)) ;
#53617=CARTESIAN_POINT('Ctrl Pts',(-20.4525327561427,-29.5537143796027,
124.499823981735)) ;
#53618=CARTESIAN_POINT('Ctrl Pts',(-20.4278473297483,-29.7469666126936,
124.072677307792)) ;
#53619=CARTESIAN_POINT('Ctrl Pts',(-20.682512025619,-29.5669775322131,124.237867726939)) ;
#53620=CARTESIAN_POINT('Ctrl Pts',(-20.5532267657517,-29.7602915105975,
123.81863575924)) ;
#53621=CARTESIAN_POINT('Ctrl Pts',(-20.8392151518599,-29.580302430117,123.920338199566)) ;
#53622=CARTESIAN_POINT('Ctrl Pts',(-20.607805933461,-29.7735472542131,123.545295424663)) ;
#53623=CARTESIAN_POINT('Ctrl Pts',(-20.9074394906536,-29.5935581737326,
123.578684401669)) ;
#53624=CARTESIAN_POINT('Ctrl Pts',(-20.6128379852353,-29.7835066276604,
123.336009205538)) ;
#53625=CARTESIAN_POINT('Ctrl Pts',(-20.9137330390343,-29.6035175471799,
123.317072430931)) ;
#53626=CARTESIAN_POINT('Ctrl Pts',(-20.5817572009049,-29.7934504515873,
123.129255120168)) ;
#53627=CARTESIAN_POINT('Ctrl Pts',(-20.8748846543688,-29.6134613711069,
123.058630457407)) ;
#53628=CARTESIAN_POINT('Ctrl Pts',(-20.5143943920179,-29.8034983957346,
122.929061237664)) ;
#53629=CARTESIAN_POINT('Ctrl Pts',(-20.7906838439836,-29.6235093152542,
122.808386846906)) ;
#53630=CARTESIAN_POINT('Ctrl Pts',(-20.4154235821622,-29.8133493669528,
122.747128077914)) ;
#53631=CARTESIAN_POINT('Ctrl Pts',(-20.6669727396954,-29.6333602864723,
122.580969032537)) ;
#53632=CARTESIAN_POINT('Ctrl Pts',(-20.2852290763675,-29.8233211843949,
122.582848316609)) ;
#53633=CARTESIAN_POINT('Ctrl Pts',(-20.504231739186,-29.6433321039144,122.375617475075)) ;
#53634=CARTESIAN_POINT('Ctrl Pts',(-20.128053971246,-29.833316606687,122.443331037292)) ;
#53635=CARTESIAN_POINT('Ctrl Pts',(-20.3077646579128,-29.6533275262065,
122.201218734591)) ;
#53636=CARTESIAN_POINT('Ctrl Pts',(-19.9482825221474,-29.8433496718107,
122.333015974272)) ;
#53637=CARTESIAN_POINT('Ctrl Pts',(-20.0830517817784,-29.6633605913302,
122.063322482912)) ;
#53638=CARTESIAN_POINT('Ctrl Pts',(-19.7554396738521,-29.8532150044759,
122.25669701737)) ;
#53639=CARTESIAN_POINT('Ctrl Pts',(-19.8419990548365,-29.6732259239954,
121.967921099517)) ;
#53640=CARTESIAN_POINT('Ctrl Pts',(-19.5504291193949,-29.8631755470735,
122.214013364722)) ;
#53641=CARTESIAN_POINT('Ctrl Pts',(-19.5857362753766,-29.683186466593,121.914563791376)) ;
#53642=CARTESIAN_POINT('Ctrl Pts',(-19.3395885460387,-29.8732092325752,
122.207884141582)) ;
#53643=CARTESIAN_POINT('Ctrl Pts',(-19.3221856204141,-29.6932201520947,
121.90689947155)) ;
#53644=CARTESIAN_POINT('Ctrl Pts',(-19.1338922316553,-29.8830940645654,
122.237651972592)) ;
#53645=CARTESIAN_POINT('Ctrl Pts',(-19.0650645565471,-29.703104984085,121.944106565147)) ;
#53646=CARTESIAN_POINT('Ctrl Pts',(-18.93291875455,-29.8931614913253,122.303910124113)) ;
#53647=CARTESIAN_POINT('Ctrl Pts',(-18.8138468784148,-29.7131724108448,
122.026926609258)) ;
#53648=CARTESIAN_POINT('Ctrl Pts',(-18.7505843551157,-29.9029999804841,
122.40163291113)) ;
#53649=CARTESIAN_POINT('Ctrl Pts',(-18.5859272207128,-29.7230109000037,
122.149077864622)) ;
#53650=CARTESIAN_POINT('Ctrl Pts',(-18.5841468216196,-29.9130634616742,
122.532193860216)) ;
#53651=CARTESIAN_POINT('Ctrl Pts',(-18.3778786569488,-29.7330743811938,
122.312276880498)) ;
#53652=CARTESIAN_POINT('Ctrl Pts',(-18.445382712112,-29.9229576194894,122.687180679488)) ;
#53653=CARTESIAN_POINT('Ctrl Pts',(-18.2044212591461,-29.7429685390089,
122.506008819954)) ;
#53654=CARTESIAN_POINT('Ctrl Pts',(-18.3346512088788,-29.9328994762337,
122.864415832755)) ;
#53655=CARTESIAN_POINT('Ctrl Pts',(-18.0660044706819,-29.7529103957532,
122.727551566379)) ;
#53656=CARTESIAN_POINT('Ctrl Pts',(-18.2558045501675,-29.9429019539051,
123.059389134583)) ;
#53657=CARTESIAN_POINT('Ctrl Pts',(-17.9674436494209,-29.7629128734246,
122.971267274044)) ;
#53658=CARTESIAN_POINT('Ctrl Pts',(-18.2122015809126,-29.9529367582094,
123.265783338575)) ;
#53659=CARTESIAN_POINT('Ctrl Pts',(-17.9129372900069,-29.7729476777289,
123.22925945364)) ;
#53660=CARTESIAN_POINT('Ctrl Pts',(-18.204883750954,-29.962781635055,123.472638058067)) ;
#53661=CARTESIAN_POINT('Ctrl Pts',(-17.9037873255447,-29.7827925545746,
123.487828320686)) ;
#53662=CARTESIAN_POINT('Ctrl Pts',(-18.2336070809338,-29.9727675146106,
123.680563989553)) ;
#53663=CARTESIAN_POINT('Ctrl Pts',(-17.9396889312473,-29.7927784341301,
123.747736250566)) ;
#53664=CARTESIAN_POINT('Ctrl Pts',(-18.2975455094374,-29.9827022449691,
123.879438238451)) ;
#53665=CARTESIAN_POINT('Ctrl Pts',(-18.019609620223,-29.8027131644886,123.99633015856)) ;
#53666=CARTESIAN_POINT('Ctrl Pts',(-18.3963927749203,-29.992760057282,124.066318685816)) ;
#53667=CARTESIAN_POINT('Ctrl Pts',(-18.1431663385628,-29.8127709768015,
124.229931834542)) ;
#53668=CARTESIAN_POINT('Ctrl Pts',(-18.5228873624992,-30.0025806494063,
124.229532798022)) ;
#53669=CARTESIAN_POINT('Ctrl Pts',(-18.3012830486464,-29.8225915689259,
124.433951657035)) ;
#53670=CARTESIAN_POINT('Ctrl Pts',(-18.6793976240298,-30.0126472350161,
124.371920994788)) ;
#53671=CARTESIAN_POINT('Ctrl Pts',(-18.4969190822941,-29.8326581545357,
124.611938648336)) ;
#53672=CARTESIAN_POINT('Ctrl Pts',(-18.8553834505121,-30.0225468155979,
124.483111642296)) ;
#53673=CARTESIAN_POINT('Ctrl Pts',(-18.7169004532694,-29.8425577351175,
124.75092934053)) ;
#53674=CARTESIAN_POINT('Ctrl Pts',(-19.0508479412311,-30.0325984152762,
124.563308795256)) ;
#53675=CARTESIAN_POINT('Ctrl Pts',(-18.9612300161591,-29.8526093347957,
124.851178041724)) ;
#53676=CARTESIAN_POINT('Ctrl Pts',(-19.2536676439756,-30.0424726016932,
124.607724013289)) ;
#53677=CARTESIAN_POINT('Ctrl Pts',(-19.2147547487628,-29.8624835212127,
124.906699600906)) ;
#53678=CARTESIAN_POINT('Ctrl Pts',(-19.4648637458808,-30.0525290775741,
124.616538418553)) ;
#53679=CARTESIAN_POINT('Ctrl Pts',(-19.4787496446914,-29.8725399970936,
124.91772003209)) ;
#53680=CARTESIAN_POINT('Ctrl Pts',(-19.6710664677573,-30.0624220088767,
124.589069886953)) ;
#53681=CARTESIAN_POINT('Ctrl Pts',(-19.7365039466891,-29.8824329283962,
124.883386678024)) ;
#53682=CARTESIAN_POINT('Ctrl Pts',(-19.8727094603673,-30.0724847875893,
124.525198764561)) ;
#53683=CARTESIAN_POINT('Ctrl Pts',(-19.9885582401686,-29.8924957071088,
124.803550123814)) ;
#53684=CARTESIAN_POINT('Ctrl Pts',(-20.0561959945725,-30.0823273131705,
124.429495466673)) ;
#53685=CARTESIAN_POINT('Ctrl Pts',(-20.217918273044,-29.90233823269,124.683922711897)) ;
#53686=CARTESIAN_POINT('Ctrl Pts',(-20.2230137933602,-30.0923180785953,
124.301917210482)) ;
#53687=CARTESIAN_POINT('Ctrl Pts',(-20.4264420363515,-29.9123289981149,
124.524451584386)) ;
#53688=CARTESIAN_POINT('Ctrl Pts',(-20.364251196426,-30.1022461545934,124.148229737283)) ;
#53689=CARTESIAN_POINT('Ctrl Pts',(-20.6029907906799,-29.9222570741129,
124.332343420945)) ;
#53690=CARTESIAN_POINT('Ctrl Pts',(-20.4776444590878,-30.1122340649804,
123.971491927839)) ;
#53691=CARTESIAN_POINT('Ctrl Pts',(-20.7447343010342,-29.9322449844999,
124.111422181951)) ;
#53692=CARTESIAN_POINT('Ctrl Pts',(-20.5586797306925,-30.1222699771053,
123.776696813867)) ;
#53693=CARTESIAN_POINT('Ctrl Pts',(-20.8460304547474,-29.9422808966249,
123.867929241438)) ;
#53694=CARTESIAN_POINT('Ctrl Pts',(-20.6041716223551,-30.132124989953,123.57455346389)) ;
#53695=CARTESIAN_POINT('Ctrl Pts',(-20.902897647784,-29.9521359094725,123.615249639807)) ;
#53696=CARTESIAN_POINT('Ctrl Pts',(-20.6143059846248,-30.1421239358693,
123.364622415793)) ;
#53697=CARTESIAN_POINT('Ctrl Pts',(-20.9155677103917,-29.9621348553888,
123.352835793809)) ;
#53698=CARTESIAN_POINT('Ctrl Pts',(-20.5882986886202,-30.1520208483173,
123.158157718472)) ;
#53699=CARTESIAN_POINT('Ctrl Pts',(-20.8830605296324,-29.9720317678368,
123.094753953374)) ;
#53700=CARTESIAN_POINT('Ctrl Pts',(-20.5259041849406,-30.1620746464108,
122.956241447257)) ;
#53701=CARTESIAN_POINT('Ctrl Pts',(-20.8050694041104,-29.9820855659303,
122.842358190255)) ;
#53702=CARTESIAN_POINT('Ctrl Pts',(-20.4310894011429,-30.1719555672375,
122.771388410386)) ;
#53703=CARTESIAN_POINT('Ctrl Pts',(-20.6865523393541,-29.991966486757,122.611290225727)) ;
#53704=CARTESIAN_POINT('Ctrl Pts',(-20.3043799559765,-30.1819600932352,
122.603543945781)) ;
#53705=CARTESIAN_POINT('Ctrl Pts',(-20.5281670017028,-30.0019710127547,
122.401483413238)) ;
#53706=CARTESIAN_POINT('Ctrl Pts',(-20.1506815547945,-30.1919440568527,
122.460549966187)) ;
#53707=CARTESIAN_POINT('Ctrl Pts',(-20.3360451641608,-30.0119549763722,
122.222739387046)) ;
#53708=CARTESIAN_POINT('Ctrl Pts',(-19.9734411230241,-30.201983697404,122.345973899521)) ;
#53709=CARTESIAN_POINT('Ctrl Pts',(-20.1144958156502,-30.0219946169235,
122.079517699013)) ;
#53710=CARTESIAN_POINT('Ctrl Pts',(-19.782871813628,-30.2118277230187,122.26527172513)) ;
#53711=CARTESIAN_POINT('Ctrl Pts',(-19.8762838855184,-30.0318386425382,
121.978637774514)) ;
#53712=CARTESIAN_POINT('Ctrl Pts',(-19.5783094050863,-30.221818728836,122.217602614152)) ;
#53713=CARTESIAN_POINT('Ctrl Pts',(-19.6205810796765,-30.0418296483556,
121.919049659153)) ;
#53714=CARTESIAN_POINT('Ctrl Pts',(-19.3675704704491,-30.2318565203682,
122.206603916104)) ;
#53715=CARTESIAN_POINT('Ctrl Pts',(-19.3571576412079,-30.0518674398877,
121.905299415955)) ;
#53716=CARTESIAN_POINT('Ctrl Pts',(-19.1621069099491,-30.2417009201566,
122.231506538147)) ;
#53717=CARTESIAN_POINT('Ctrl Pts',(-19.10032681686,-30.0617118396761,121.93642608354)) ;
#53718=CARTESIAN_POINT('Ctrl Pts',(-18.9611771135097,-30.2516857207133,
122.292157840187)) ;
#53719=CARTESIAN_POINT('Ctrl Pts',(-18.8491638610565,-30.0716966402329,
122.012238721506)) ;
#53720=CARTESIAN_POINT('Ctrl Pts',(-18.7745889266096,-30.2616252441245,
122.386291238736)) ;
#53721=CARTESIAN_POINT('Ctrl Pts',(-18.6159274222133,-30.081636163644,122.129904287597)) ;
#53722=CARTESIAN_POINT('Ctrl Pts',(-18.6055578608464,-30.2716649632255,
122.512666339246)) ;
#53723=CARTESIAN_POINT('Ctrl Pts',(-18.4046377385621,-30.091675882745,122.2878717801)) ;
#53724=CARTESIAN_POINT('Ctrl Pts',(-18.4631237680064,-30.2815531351448,
122.664098676228)) ;
#53725=CARTESIAN_POINT('Ctrl Pts',(-18.2265933388627,-30.1015640546643,
122.477161788212)) ;
#53726=CARTESIAN_POINT('Ctrl Pts',(-18.3476602750316,-30.2915426975618,
122.839512639782)) ;
#53727=CARTESIAN_POINT('Ctrl Pts',(-18.0822626444727,-30.1115536170813,
122.696428624347)) ;
#53728=CARTESIAN_POINT('Ctrl Pts',(-18.264811021222,-30.3015010697565,123.031774138297)) ;
#53729=CARTESIAN_POINT('Ctrl Pts',(-17.9786995240026,-30.121511989276,122.936755300646)) ;
#53730=CARTESIAN_POINT('Ctrl Pts',(-18.2163954880168,-30.3114011439872,
123.234202863219)) ;
#53731=CARTESIAN_POINT('Ctrl Pts',(-17.9181786120005,-30.1314120635067,
123.189791746327)) ;
#53732=CARTESIAN_POINT('Ctrl Pts',(-18.2037078203567,-30.3214472403608,
123.445012427325)) ;
#53733=CARTESIAN_POINT('Ctrl Pts',(-17.9023177044386,-30.1414581598803,
123.45330342739)) ;
#53734=CARTESIAN_POINT('Ctrl Pts',(-18.2274762171961,-30.3313558243579,
123.651971116123)) ;
#53735=CARTESIAN_POINT('Ctrl Pts',(-17.9320269695146,-30.1513667438774,
123.712002752109)) ;
#53736=CARTESIAN_POINT('Ctrl Pts',(-18.2870541787712,-30.3413664029488,
123.853819127414)) ;
#53737=CARTESIAN_POINT('Ctrl Pts',(-18.0064982863463,-30.1613773224683,
123.964313150679)) ;
#53738=CARTESIAN_POINT('Ctrl Pts',(-18.3813325232713,-30.3513955610616,
124.042419862782)) ;
#53739=CARTESIAN_POINT('Ctrl Pts',(-18.1243449646427,-30.1714064805811,
124.200064581448)) ;
#53740=CARTESIAN_POINT('Ctrl Pts',(-18.5044666604839,-30.3612484428997,
124.20896945013)) ;
#53741=CARTESIAN_POINT('Ctrl Pts',(-18.2782623862379,-30.1812593624192,
124.408253321778)) ;
#53742=CARTESIAN_POINT('Ctrl Pts',(-18.6558439163059,-30.3712080040507,
124.353634907533)) ;
#53743=CARTESIAN_POINT('Ctrl Pts',(-18.4674836003833,-30.1912189235702,
124.589086196553)) ;
#53744=CARTESIAN_POINT('Ctrl Pts',(-18.8316171646393,-30.3812464386398,
124.470406891884)) ;
#53745=CARTESIAN_POINT('Ctrl Pts',(-18.6871993887316,-30.2012573581593,
124.735052040907)) ;
#53746=CARTESIAN_POINT('Ctrl Pts',(-19.0216991726386,-30.3911197108669,
124.553872844899)) ;
#53747=CARTESIAN_POINT('Ctrl Pts',(-18.9248025260445,-30.2111306303864,
124.83938585053)) ;
#53748=CARTESIAN_POINT('Ctrl Pts',(-19.2274128061745,-30.4011929528604,
124.603980425918)) ;
#53749=CARTESIAN_POINT('Ctrl Pts',(-19.1819439102714,-30.22120387238,124.902021224063)) ;
#53750=CARTESIAN_POINT('Ctrl Pts',(-19.4334667110816,-30.4110132843935,
124.617542684811)) ;
#53751=CARTESIAN_POINT('Ctrl Pts',(-19.4395127810957,-30.231024203913,124.918975069789)) ;
#53752=CARTESIAN_POINT('Ctrl Pts',(-19.64406951049,-30.4210919456203,124.594736003978)) ;
#53753=CARTESIAN_POINT('Ctrl Pts',(-19.7027659038787,-30.2411028651398,
124.890467615941)) ;
#53754=CARTESIAN_POINT('Ctrl Pts',(-19.8430448442677,-30.4309435409145,
124.537080259069)) ;
#53755=CARTESIAN_POINT('Ctrl Pts',(-19.9514865661145,-30.250954460434,124.818398357454)) ;
#53756=CARTESIAN_POINT('Ctrl Pts',(-20.0331712259711,-30.4410166761433,
124.443902678436)) ;
#53757=CARTESIAN_POINT('Ctrl Pts',(-20.1891444821242,-30.2610275956628,
124.701927251244)) ;
#53758=CARTESIAN_POINT('Ctrl Pts',(-20.200339647076,-30.4508591116683,124.32192778539)) ;
#53759=CARTESIAN_POINT('Ctrl Pts',(-20.3981066043222,-30.2708700311879,
124.549458419515)) ;
#53760=CARTESIAN_POINT('Ctrl Pts',(-20.3462888347876,-30.4608398808017,
124.171191115801)) ;
#53761=CARTESIAN_POINT('Ctrl Pts',(-20.5805436589418,-30.2808508003213,
124.361037704532)) ;
#53762=CARTESIAN_POINT('Ctrl Pts',(-20.4639585613339,-30.4708569820456,
123.996541687798)) ;
#53763=CARTESIAN_POINT('Ctrl Pts',(-20.7276313528828,-30.2908679015651,
124.142726286221)) ;
#53764=CARTESIAN_POINT('Ctrl Pts',(-20.5487810389583,-30.4807454296474,
123.806730562509)) ;
#53765=CARTESIAN_POINT('Ctrl Pts',(-20.8336603365764,-30.300756349167,123.905461600879)) ;
#53766=CARTESIAN_POINT('Ctrl Pts',(-20.6002259549947,-30.4908011438283,
123.601702375123)) ;
#53767=CARTESIAN_POINT('Ctrl Pts',(-20.8979668751286,-30.3108120633478,
123.649176788009)) ;
#53768=CARTESIAN_POINT('Ctrl Pts',(-20.615052892875,-30.5006763502421,123.394610916813)) ;
#53769=CARTESIAN_POINT('Ctrl Pts',(-20.916501105686,-30.3206872697617,123.390311340074)) ;
#53770=CARTESIAN_POINT('Ctrl Pts',(-20.5939426510148,-30.5106714027149,
123.185552599972)) ;
#53771=CARTESIAN_POINT('Ctrl Pts',(-20.8901135579896,-30.3306823222344,
123.128988240025)) ;
#53772=CARTESIAN_POINT('Ctrl Pts',(-20.536367759922,-30.520693286677,122.982872051517)) ;
#53773=CARTESIAN_POINT('Ctrl Pts',(-20.8181453545947,-30.3407042061965,
122.87563748438)) ;
#53774=CARTESIAN_POINT('Ctrl Pts',(-20.4457706611139,-30.5305972592063,
122.795404854875)) ;
#53775=CARTESIAN_POINT('Ctrl Pts',(-20.7048988529436,-30.3506081787258,
122.641302484479)) ;
#53776=CARTESIAN_POINT('Ctrl Pts',(-20.3232033140456,-30.5405857558672,
122.624895059131)) ;
#53777=CARTESIAN_POINT('Ctrl Pts',(-20.5516896931054,-30.3605966753867,
122.428164932553)) ;
#53778=CARTESIAN_POINT('Ctrl Pts',(-20.1731729387286,-30.5505495531152,
122.478730184432)) ;
#53779=CARTESIAN_POINT('Ctrl Pts',(-20.3641515812298,-30.3705604726347,
122.245458339138)) ;
#53780=CARTESIAN_POINT('Ctrl Pts',(-20.0013435844137,-30.5604535764232,
122.361105057577)) ;
#53781=CARTESIAN_POINT('Ctrl Pts',(-20.1493641424933,-30.3804644959427,
122.098426355187)) ;
#53782=CARTESIAN_POINT('Ctrl Pts',(-19.8086729775666,-30.5705140797448,
122.27392287476)) ;
#53783=CARTESIAN_POINT('Ctrl Pts',(-19.90852625773,-30.3905249992643,121.989448658522)) ;
#53784=CARTESIAN_POINT('Ctrl Pts',(-19.6082855481598,-30.5803546148847,
122.222396123201)) ;
#53785=CARTESIAN_POINT('Ctrl Pts',(-19.6580405513247,-30.4003655344042,
121.925039834597)) ;
#53786=CARTESIAN_POINT('Ctrl Pts',(-19.3974190538605,-30.5904168355893,
122.20582075455)) ;
#53787=CARTESIAN_POINT('Ctrl Pts',(-19.3944577950554,-30.4104277551088,
121.904320739898)) ;
#53788=CARTESIAN_POINT('Ctrl Pts',(-19.1903195961826,-30.6003139893655,
122.225997239462)) ;
#53789=CARTESIAN_POINT('Ctrl Pts',(-19.1355824752847,-30.420324908885,121.929541441992)) ;
#53790=CARTESIAN_POINT('Ctrl Pts',(-18.9890100939322,-30.610245122751,122.281343791059)) ;
#53791=CARTESIAN_POINT('Ctrl Pts',(-18.8839449757313,-30.4302560422705,
121.998725089829)) ;
#53792=CARTESIAN_POINT('Ctrl Pts',(-18.7983550338524,-30.6202874978967,
122.372017641209)) ;
#53793=CARTESIAN_POINT('Ctrl Pts',(-18.645626417901,-30.4402984174162,122.112067478711)) ;
#53794=CARTESIAN_POINT('Ctrl Pts',(-18.6289139729558,-30.6301734356628,
122.492389628347)) ;
#53795=CARTESIAN_POINT('Ctrl Pts',(-18.4338243468279,-30.4501843551824,
122.26253329297)) ;
#53796=CARTESIAN_POINT('Ctrl Pts',(-18.4811125942436,-30.6401692786477,
122.641749676501)) ;
#53797=CARTESIAN_POINT('Ctrl Pts',(-18.2490727522653,-30.4601801981672,
122.449233759655)) ;
#53798=CARTESIAN_POINT('Ctrl Pts',(-18.3621388083306,-30.6501112565263,
122.813609855738)) ;
#53799=CARTESIAN_POINT('Ctrl Pts',(-18.1003554684514,-30.4701221760458,
122.664059702163)) ;
#53800=CARTESIAN_POINT('Ctrl Pts',(-18.2744107318474,-30.6600706310073,
123.003708981063)) ;
#53801=CARTESIAN_POINT('Ctrl Pts',(-17.9906956058916,-30.4800815505268,
122.901684237727)) ;
#53802=CARTESIAN_POINT('Ctrl Pts',(-18.2207100016037,-30.6700672468411,
123.206915248933)) ;
#53803=CARTESIAN_POINT('Ctrl Pts',(-17.9235701571925,-30.4900781663606,
123.155692351236)) ;
#53804=CARTESIAN_POINT('Ctrl Pts',(-18.2033237827632,-30.6801014654146,
123.4171423923)) ;
#53805=CARTESIAN_POINT('Ctrl Pts',(-17.9018377985399,-30.5001123849341,
123.418476175523)) ;
#53806=CARTESIAN_POINT('Ctrl Pts',(-18.2221037500632,-30.6899545326252,
123.623428518409)) ;
#53807=CARTESIAN_POINT('Ctrl Pts',(-17.9253133850039,-30.5099654521447,
123.676335153536)) ;
#53808=CARTESIAN_POINT('Ctrl Pts',(-18.2764164848045,-30.6999147905028,
123.825650685452)) ;
#53809=CARTESIAN_POINT('Ctrl Pts',(-17.9932051452733,-30.5199257100223,
123.929113115031)) ;
#53810=CARTESIAN_POINT('Ctrl Pts',(-18.3658619188668,-30.7099438172084,
124.016591993771)) ;
#53811=CARTESIAN_POINT('Ctrl Pts',(-18.1050124819291,-30.5299547367279,
124.167789386679)) ;
#53812=CARTESIAN_POINT('Ctrl Pts',(-18.4856036512729,-30.7198540242428,
124.187076921124)) ;
#53813=CARTESIAN_POINT('Ctrl Pts',(-18.2546907013589,-30.5398649437623,
124.38089587769)) ;
#53814=CARTESIAN_POINT('Ctrl Pts',(-18.6331183540979,-30.7297889348904,
124.334947217682)) ;
#53815=CARTESIAN_POINT('Ctrl Pts',(-18.4390851724794,-30.5497998544099,
124.565733592128)) ;
#53816=CARTESIAN_POINT('Ctrl Pts',(-18.805998293057,-30.7398300650696,124.456072455855)) ;
#53817=CARTESIAN_POINT('Ctrl Pts',(-18.6551854057715,-30.5598409845892,
124.71713937116)) ;
#53818=CARTESIAN_POINT('Ctrl Pts',(-18.9943042437929,-30.7497172054396,
124.544111417618)) ;
#53819=CARTESIAN_POINT('Ctrl Pts',(-18.8905691521537,-30.5697281249591,
124.82718773236)) ;
#53820=CARTESIAN_POINT('Ctrl Pts',(-19.1970545158081,-30.7597094829755,
124.599022917554)) ;
#53821=CARTESIAN_POINT('Ctrl Pts',(-19.1440074489892,-30.5797204024951,
124.895826199373)) ;
#53822=CARTESIAN_POINT('Ctrl Pts',(-19.4053746987768,-30.7696580262439,
124.617756988556)) ;
#53823=CARTESIAN_POINT('Ctrl Pts',(-19.4044083048236,-30.5896689457634,
124.919242869129)) ;
#53824=CARTESIAN_POINT('Ctrl Pts',(-19.6135329763721,-30.7795947010611,
124.60035612135)) ;
#53825=CARTESIAN_POINT('Ctrl Pts',(-19.6646066985411,-30.5996056205806,
124.897490651167)) ;
#53826=CARTESIAN_POINT('Ctrl Pts',(-19.8165585167842,-30.7895781219974,
124.5470606735)) ;
#53827=CARTESIAN_POINT('Ctrl Pts',(-19.9183885697259,-30.609589041517,124.830870141042)) ;
#53828=CARTESIAN_POINT('Ctrl Pts',(-20.0081989085124,-30.7996204371867,
124.458507416817)) ;
#53829=CARTESIAN_POINT('Ctrl Pts',(-20.1579384639164,-30.6196313567062,
124.720177687005)) ;
#53830=CARTESIAN_POINT('Ctrl Pts',(-20.1782668651698,-30.8094607546259,
124.340716223305)) ;
#53831=CARTESIAN_POINT('Ctrl Pts',(-20.3705238610805,-30.6294716741454,
124.572936952077)) ;
#53832=CARTESIAN_POINT('Ctrl Pts',(-20.328476682033,-30.8194904586834,124.192735300873)) ;
#53833=CARTESIAN_POINT('Ctrl Pts',(-20.5582851077413,-30.6395013782029,
124.387959911914)) ;
#53834=CARTESIAN_POINT('Ctrl Pts',(-20.4501392005903,-30.8295114154059,
124.020744611247)) ;
#53835=CARTESIAN_POINT('Ctrl Pts',(-20.7103623024763,-30.6495223349254,
124.172970910652)) ;
#53836=CARTESIAN_POINT('Ctrl Pts',(-20.5391909200879,-30.8393779577095,
123.833391228608)) ;
#53837=CARTESIAN_POINT('Ctrl Pts',(-20.8216762308141,-30.659388877229,123.93877758456)) ;
#53838=CARTESIAN_POINT('Ctrl Pts',(-20.595495855653,-30.8494490576546,123.629308992589)) ;
#53839=CARTESIAN_POINT('Ctrl Pts',(-20.892056009971,-30.6694599771742,123.683674797214)) ;
#53840=CARTESIAN_POINT('Ctrl Pts',(-20.6150525003595,-30.8592911318322,
123.423316450362)) ;
#53841=CARTESIAN_POINT('Ctrl Pts',(-20.9165006066991,-30.6793020513517,
123.426182698948)) ;
#53842=CARTESIAN_POINT('Ctrl Pts',(-20.5991170580468,-30.8692519264192,
123.214521188728)) ;
#53843=CARTESIAN_POINT('Ctrl Pts',(-20.8965796708066,-30.6892628459388,
123.165188338034)) ;
#53844=CARTESIAN_POINT('Ctrl Pts',(-20.546363865341,-30.8792897993201,123.010200870518)) ;
#53845=CARTESIAN_POINT('Ctrl Pts',(-20.8306367980833,-30.6993007188396,
122.909788435374)) ;
#53846=CARTESIAN_POINT('Ctrl Pts',(-20.4606968836195,-30.8891640848642,
122.821085418058)) ;
#53847=CARTESIAN_POINT('Ctrl Pts',(-20.7235512012954,-30.7091750043837,
122.673393853038)) ;
#53848=CARTESIAN_POINT('Ctrl Pts',(-20.3411946934181,-30.8992338352781,
122.646376318982)) ;
#53849=CARTESIAN_POINT('Ctrl Pts',(-20.5741723490804,-30.7192447547976,
122.455008665835)) ;
#53850=CARTESIAN_POINT('Ctrl Pts',(-20.19669738145,-30.9090671198127,122.498514065535)) ;
#53851=CARTESIAN_POINT('Ctrl Pts',(-20.3935486502023,-30.7290780393323,
122.27018106757)) ;
#53852=CARTESIAN_POINT('Ctrl Pts',(-20.025723038719,-30.9190974606128,122.375099669013)) ;
#53853=CARTESIAN_POINT('Ctrl Pts',(-20.179829726815,-30.7391083801323,122.11591459953)) ;
#53854=CARTESIAN_POINT('Ctrl Pts',(-19.8356036746159,-30.9291293846124,
122.283783083488)) ;
#53855=CARTESIAN_POINT('Ctrl Pts',(-19.9421798973241,-30.7491403041319,
122.001770363294)) ;
#53856=CARTESIAN_POINT('Ctrl Pts',(-19.6367747487569,-30.9389579195483,
122.227591752257)) ;
#53857=CARTESIAN_POINT('Ctrl Pts',(-19.6936420289628,-30.7589688390678,
121.931532551654)) ;
#53858=CARTESIAN_POINT('Ctrl Pts',(-19.4278031799893,-30.948951697313,122.205853025162)) ;
#53859=CARTESIAN_POINT('Ctrl Pts',(-19.4324272173877,-30.7689626168325,
121.904361062246)) ;
#53860=CARTESIAN_POINT('Ctrl Pts',(-19.2175414225101,-30.9589794077985,
122.221194257031)) ;
#53861=CARTESIAN_POINT('Ctrl Pts',(-19.1696001927494,-30.778990327318,121.923539411805)) ;
#53862=CARTESIAN_POINT('Ctrl Pts',(-19.0159184250757,-30.9688678186325,
122.271841404524)) ;
#53863=CARTESIAN_POINT('Ctrl Pts',(-18.9175710994201,-30.788878738152,121.986850390242)) ;
#53864=CARTESIAN_POINT('Ctrl Pts',(-18.8243211742747,-30.978844669168,122.357145110244)) ;
#53865=CARTESIAN_POINT('Ctrl Pts',(-18.678075116747,-30.7988555886875,122.093481958208)) ;
#53866=CARTESIAN_POINT('Ctrl Pts',(-18.6501372622533,-30.9888364657185,
122.474607486696)) ;
#53867=CARTESIAN_POINT('Ctrl Pts',(-18.4603462227314,-30.808847385238,122.240311680626)) ;
#53868=CARTESIAN_POINT('Ctrl Pts',(-18.4985386548746,-30.9988724718122,
122.621327863081)) ;
#53869=CARTESIAN_POINT('Ctrl Pts',(-18.2708493728752,-30.8188833913317,
122.423713476581)) ;
#53870=CARTESIAN_POINT('Ctrl Pts',(-18.3767267027261,-31.008723206075,122.788826198165)) ;
#53871=CARTESIAN_POINT('Ctrl Pts',(-18.1185854661369,-30.8287341255945,
122.633088418343)) ;
#53872=CARTESIAN_POINT('Ctrl Pts',(-18.2842463817907,-31.0187144646032,
122.977386152329)) ;
#53873=CARTESIAN_POINT('Ctrl Pts',(-18.0029869056345,-30.8387253841227,
122.868789450523)) ;
#53874=CARTESIAN_POINT('Ctrl Pts',(-18.2262044455862,-31.0286323595064,
123.177677702795)) ;
#53875=CARTESIAN_POINT('Ctrl Pts',(-17.9304363999913,-30.8486432790259,
123.119155041234)) ;
#53876=CARTESIAN_POINT('Ctrl Pts',(-18.2035238002497,-31.0386605011694,
123.387260137324)) ;
#53877=CARTESIAN_POINT('Ctrl Pts',(-17.9020877612529,-30.8586714206889,
123.381133283296)) ;
#53878=CARTESIAN_POINT('Ctrl Pts',(-18.2172919464805,-31.0485456692853,
123.594625950143)) ;
#53879=CARTESIAN_POINT('Ctrl Pts',(-17.9193001862951,-30.8685565888048,
123.640341140652)) ;
#53880=CARTESIAN_POINT('Ctrl Pts',(-18.2668826506638,-31.0585350327913,
123.79869899324)) ;
#53881=CARTESIAN_POINT('Ctrl Pts',(-17.9812908653985,-30.8785459523108,
123.895432047614)) ;
#53882=CARTESIAN_POINT('Ctrl Pts',(-18.3519971283237,-31.0685761678013,
123.991875632271)) ;
#53883=CARTESIAN_POINT('Ctrl Pts',(-18.0876859529692,-30.8885870873209,
124.136901868432)) ;
#53884=CARTESIAN_POINT('Ctrl Pts',(-18.4666381472819,-31.0784088359894,
124.163882158032)) ;
#53885=CARTESIAN_POINT('Ctrl Pts',(-18.2309896741229,-30.8984197555089,
124.351909547832)) ;
#53886=CARTESIAN_POINT('Ctrl Pts',(-18.6113111204173,-31.0884027389439,
124.31623927594)) ;
#53887=CARTESIAN_POINT('Ctrl Pts',(-18.4118327451302,-30.9084136584634,
124.542354351797)) ;
#53888=CARTESIAN_POINT('Ctrl Pts',(-18.7811066172618,-31.0984320240284,
124.441246279883)) ;
#53889=CARTESIAN_POINT('Ctrl Pts',(-18.6240784847037,-30.9184429435479,
124.698611210705)) ;
#53890=CARTESIAN_POINT('Ctrl Pts',(-18.9669894085724,-31.1083075524703,
124.533744474352)) ;
#53891=CARTESIAN_POINT('Ctrl Pts',(-18.8564336547338,-30.9283184719898,
124.814232094109)) ;
#53892=CARTESIAN_POINT('Ctrl Pts',(-19.1685234135853,-31.1183078350863,
124.593519235339)) ;
#53893=CARTESIAN_POINT('Ctrl Pts',(-19.1083519713198,-30.9383187546059,
124.888948210997)) ;
#53894=CARTESIAN_POINT('Ctrl Pts',(-19.3755624886653,-31.1282198511434,
124.617355261767)) ;
#53895=CARTESIAN_POINT('Ctrl Pts',(-19.3671515658149,-30.9482307706629,
124.918740815905)) ;
#53896=CARTESIAN_POINT('Ctrl Pts',(-19.5862881147713,-31.1382619264824,
124.604773299215)) ;
#53897=CARTESIAN_POINT('Ctrl Pts',(-19.6305583757135,-30.9582728460019,
124.903010863219)) ;
#53898=CARTESIAN_POINT('Ctrl Pts',(-19.7887432035316,-31.1481617591385,
124.556475850266)) ;
#53899=CARTESIAN_POINT('Ctrl Pts',(-19.8836271404046,-30.968172678658,124.842636497184)) ;
#53900=CARTESIAN_POINT('Ctrl Pts',(-19.9816984118981,-31.1581541597165,
124.473418066137)) ;
#53901=CARTESIAN_POINT('Ctrl Pts',(-20.1248202353964,-30.978165079236,124.738811837859)) ;
#53902=CARTESIAN_POINT('Ctrl Pts',(-20.1578289058847,-31.1681881814759,
124.357322944161)) ;
#53903=CARTESIAN_POINT('Ctrl Pts',(-20.3449819507396,-30.9881991009954,
124.593690836026)) ;
#53904=CARTESIAN_POINT('Ctrl Pts',(-20.3087153180884,-31.1780527923171,
124.215054802295)) ;
#53905=CARTESIAN_POINT('Ctrl Pts',(-20.5335886316018,-30.9980637118366,
124.415853378538)) ;
#53906=CARTESIAN_POINT('Ctrl Pts',(-20.4346283251563,-31.1880451917782,
124.046895705598)) ;
#53907=CARTESIAN_POINT('Ctrl Pts',(-20.6909778267488,-31.0080561112978,
124.205652827249)) ;
#53908=CARTESIAN_POINT('Ctrl Pts',(-20.5294345452315,-31.1980771451111,
123.858502766262)) ;
#53909=CARTESIAN_POINT('Ctrl Pts',(-20.8094832864475,-31.0180880646307,
123.97016048948)) ;
#53910=CARTESIAN_POINT('Ctrl Pts',(-20.5893954841832,-31.2079435040528,
123.659927548445)) ;
#53911=CARTESIAN_POINT('Ctrl Pts',(-20.8844320814046,-31.0279544235723,
123.721940205766)) ;
#53912=CARTESIAN_POINT('Ctrl Pts',(-20.6146037556417,-31.2179309795386,
123.451503773627)) ;
#53913=CARTESIAN_POINT('Ctrl Pts',(-20.915939761088,-31.0379418990581,123.461410041665)) ;
#53914=CARTESIAN_POINT('Ctrl Pts',(-20.6033971471085,-31.2278758857271,
123.24270000188)) ;
#53915=CARTESIAN_POINT('Ctrl Pts',(-20.9019287888384,-31.0478868052466,
123.200405236552)) ;
#53916=CARTESIAN_POINT('Ctrl Pts',(-20.5555242405054,-31.2379208503873,
123.037041915201)) ;
#53917=CARTESIAN_POINT('Ctrl Pts',(-20.842085039233,-31.0579317699068,122.943333258372)) ;
#53918=CARTESIAN_POINT('Ctrl Pts',(-20.4743386324737,-31.2477826572922,
122.846253520561)) ;
#53919=CARTESIAN_POINT('Ctrl Pts',(-20.7406003648983,-31.0677935768117,
122.704848430347)) ;
#53920=CARTESIAN_POINT('Ctrl Pts',(-20.360117950421,-31.2577753295979,122.669966551316)) ;
#53921=CARTESIAN_POINT('Ctrl Pts',(-20.5978221442473,-31.0777862491175,
122.484491140152)) ;
#53922=CARTESIAN_POINT('Ctrl Pts',(-20.2178975470522,-31.2677040005433,
122.51716583229)) ;
#53923=CARTESIAN_POINT('Ctrl Pts',(-20.4200444704518,-31.0877149200628,
122.293491950862)) ;
#53924=CARTESIAN_POINT('Ctrl Pts',(-20.0511349253016,-31.2776565427686,
122.390821276081)) ;
#53925=CARTESIAN_POINT('Ctrl Pts',(-20.2115893828886,-31.0976674622881,
122.13556337995)) ;
#53926=CARTESIAN_POINT('Ctrl Pts',(-19.8640731557152,-31.2876578987645,
122.294767252677)) ;
#53927=CARTESIAN_POINT('Ctrl Pts',(-19.9777608299036,-31.107668818284,122.015498299197)) ;
#53928=CARTESIAN_POINT('Ctrl Pts',(-19.6625721454269,-31.2976865110392,
122.232767913839)) ;
#53929=CARTESIAN_POINT('Ctrl Pts',(-19.7258837090917,-31.1176974305587,
121.938001760738)) ;
#53930=CARTESIAN_POINT('Ctrl Pts',(-19.4568083883109,-31.3075508455887,
122.20682000382)) ;
#53931=CARTESIAN_POINT('Ctrl Pts',(-19.4686784023227,-31.1275617651082,
121.905569609597)) ;
#53932=CARTESIAN_POINT('Ctrl Pts',(-19.2470034323369,-31.3175431696653,
122.216797567056)) ;
#53933=CARTESIAN_POINT('Ctrl Pts',(-19.2064222622947,-31.1375540891848,
121.918044378249)) ;
#53934=CARTESIAN_POINT('Ctrl Pts',(-19.0433631987087,-31.3274706620311,
122.26264289437)) ;
#53935=CARTESIAN_POINT('Ctrl Pts',(-18.951872457949,-31.1474815815507,121.97535381061)) ;
#53936=CARTESIAN_POINT('Ctrl Pts',(-18.8488944828603,-31.337498020582,122.343946304587)) ;
#53937=CARTESIAN_POINT('Ctrl Pts',(-18.7087875924264,-31.1575089401015,
122.07698569699)) ;
#53938=CARTESIAN_POINT('Ctrl Pts',(-18.6738227975292,-31.3473844386331,
122.456025056537)) ;
#53939=CARTESIAN_POINT('Ctrl Pts',(-18.489949403028,-31.1673953581526,122.217086575843)) ;
#53940=CARTESIAN_POINT('Ctrl Pts',(-18.5185992416469,-31.3574161733685,
122.598745584505)) ;
#53941=CARTESIAN_POINT('Ctrl Pts',(-18.2959218217005,-31.177427092888,122.395489361633)) ;
#53942=CARTESIAN_POINT('Ctrl Pts',(-18.3922256515261,-31.3672977546117,
122.76367605931)) ;
#53943=CARTESIAN_POINT('Ctrl Pts',(-18.1379570316175,-31.1873086741313,
122.601654223981)) ;
#53944=CARTESIAN_POINT('Ctrl Pts',(-18.2946472022262,-31.3773597326441,
122.951323265286)) ;
#53945=CARTESIAN_POINT('Ctrl Pts',(-18.0159864386177,-31.1973706521636,
122.836214609503)) ;
#53946=CARTESIAN_POINT('Ctrl Pts',(-18.2323356671991,-31.3872168110058,
123.148990652215)) ;
#53947=CARTESIAN_POINT('Ctrl Pts',(-17.9380997060772,-31.2072277305253,
123.083299705049)) ;
#53948=CARTESIAN_POINT('Ctrl Pts',(-18.2045044604485,-31.3972113841118,
123.357222538529)) ;
#53949=CARTESIAN_POINT('Ctrl Pts',(-17.90331347904,-31.2172223036313,123.343589981837)) ;
#53950=CARTESIAN_POINT('Ctrl Pts',(-18.2131184967394,-31.4071371803994,
123.565745265259)) ;
#53951=CARTESIAN_POINT('Ctrl Pts',(-17.9140838361603,-31.2271480999189,
123.604243273505)) ;
#53952=CARTESIAN_POINT('Ctrl Pts',(-18.2581923238068,-31.4171625475691,
123.771616644239)) ;
#53953=CARTESIAN_POINT('Ctrl Pts',(-17.9704288395072,-31.2371734670886,
123.861581949302)) ;
#53954=CARTESIAN_POINT('Ctrl Pts',(-18.3372215849961,-31.427058627223,123.964077719536)) ;
#53955=CARTESIAN_POINT('Ctrl Pts',(-18.0692181288422,-31.2470695467425,
124.102157307158)) ;
#53956=CARTESIAN_POINT('Ctrl Pts',(-18.4492191595014,-31.4370537069285,
124.141874347234)) ;
#53957=CARTESIAN_POINT('Ctrl Pts',(-18.2092168771544,-31.2570646264481,
124.324401075106)) ;
#53958=CARTESIAN_POINT('Ctrl Pts',(-18.5910734083571,-31.4470787947444,
124.297744881585)) ;
#53959=CARTESIAN_POINT('Ctrl Pts',(-18.3865390044903,-31.2670897142639,
124.519239587028)) ;
#53960=CARTESIAN_POINT('Ctrl Pts',(-18.8100884239902,-31.4602626171116,
124.467625344121)) ;
#53961=CARTESIAN_POINT('Ctrl Pts',(-18.6602990639884,-31.2802735366311,
124.73157647326)) ;
#53962=CARTESIAN_POINT('Ctrl Pts',(-19.0709153029651,-31.4735847352576,
124.578138378408)) ;
#53963=CARTESIAN_POINT('Ctrl Pts',(-18.9862948593756,-31.2935956547771,
124.869711357503)) ;
#53964=CARTESIAN_POINT('Ctrl Pts',(-19.3495941389619,-31.4869639448852,
124.6162385658)) ;
#53965=CARTESIAN_POINT('Ctrl Pts',(-19.3347015527478,-31.3069748644047,
124.917347223375)) ;
#53966=CARTESIAN_POINT('Ctrl Pts',(-19.5563094575702,-31.4968021821294,
124.608810856145)) ;
#53967=CARTESIAN_POINT('Ctrl Pts',(-19.5930836021452,-31.3168131016489,
124.908057132505)) ;
#53968=CARTESIAN_POINT('Ctrl Pts',(-19.763395166937,-31.5068751053881,124.564668379505)) ;
#53969=CARTESIAN_POINT('Ctrl Pts',(-19.8519437779816,-31.3268860249076,
124.852876717883)) ;
#53970=CARTESIAN_POINT('Ctrl Pts',(-19.9554908372654,-31.5167317468432,
124.486904342967)) ;
#53971=CARTESIAN_POINT('Ctrl Pts',(-20.0920602273854,-31.3367426663627,
124.755670606854)) ;
#53972=CARTESIAN_POINT('Ctrl Pts',(-20.1337307856986,-31.5267171223493,
124.376027908366)) ;
#53973=CARTESIAN_POINT('Ctrl Pts',(-20.3148623985469,-31.3467280418688,
124.617067390202)) ;
#53974=CARTESIAN_POINT('Ctrl Pts',(-20.3414635779869,-31.5400011538097,
124.189405170033)) ;
#53975=CARTESIAN_POINT('Ctrl Pts',(-20.5745088880955,-31.3600120733292,
124.383813943101)) ;
#53976=CARTESIAN_POINT('Ctrl Pts',(-20.5342357011611,-31.55651994568,123.895695798079)) ;
#53977=CARTESIAN_POINT('Ctrl Pts',(-20.8154916494353,-31.3765308651996,
124.01662607274)) ;
#53978=CARTESIAN_POINT('Ctrl Pts',(-20.615702601322,-31.5733056626867,123.5482462708)) ;
#53979=CARTESIAN_POINT('Ctrl Pts',(-20.9173070494684,-31.3933165822062,
123.582394229606)) ;
#53980=CARTESIAN_POINT('Ctrl Pts',(-20.607065235222,-31.5864188111957,123.272686183113)) ;
#53981=CARTESIAN_POINT('Ctrl Pts',(-20.9065152950927,-31.4064297307152,
123.237879258035)) ;
#53982=CARTESIAN_POINT('Ctrl Pts',(-20.5647775941507,-31.5964543602758,
123.066008473396)) ;
#53983=CARTESIAN_POINT('Ctrl Pts',(-20.8536524125432,-31.4164652797954,
122.979546305353)) ;
#53984=CARTESIAN_POINT('Ctrl Pts',(-20.4868139035535,-31.6064704164553,
122.870382663184)) ;
#53985=CARTESIAN_POINT('Ctrl Pts',(-20.7561932615581,-31.4264813359748,
122.735008678701)) ;
#53986=CARTESIAN_POINT('Ctrl Pts',(-20.3416392377526,-31.6196484523213,
122.634448176635)) ;
#53987=CARTESIAN_POINT('Ctrl Pts',(-20.5747356332259,-31.4396593718408,
122.440107128051)) ;
#53988=CARTESIAN_POINT('Ctrl Pts',(-20.0859156395753,-31.6362503295084,
122.3910420022)) ;
#53989=CARTESIAN_POINT('Ctrl Pts',(-20.2550642402357,-31.4562612490279,
122.135837120471)) ;
#53990=CARTESIAN_POINT('Ctrl Pts',(-19.6946086357507,-31.6563134741243,
122.221176683087)) ;
#53991=CARTESIAN_POINT('Ctrl Pts',(-19.7659328720363,-31.4763243936438,
121.923514400553)) ;
#53992=CARTESIAN_POINT('Ctrl Pts',(-19.2743459249407,-31.676114364208,122.195122229128)) ;
#53993=CARTESIAN_POINT('Ctrl Pts',(-19.2406043647654,-31.4961252837275,
121.890949553411)) ;
#53994=CARTESIAN_POINT('Ctrl Pts',(-18.8673343999719,-31.6960574894867,
122.313844662609)) ;
#53995=CARTESIAN_POINT('Ctrl Pts',(-18.7318418663585,-31.5160684090062,
122.039356586045)) ;
#53996=CARTESIAN_POINT('Ctrl Pts',(-18.5261587627728,-31.7159555346063,
122.564031122159)) ;
#53997=CARTESIAN_POINT('Ctrl Pts',(-18.305375239822,-31.5359664541258,122.352092202797)) ;
#53998=CARTESIAN_POINT('Ctrl Pts',(-18.2900690142787,-31.735841294233,122.914876518788)) ;
#53999=CARTESIAN_POINT('Ctrl Pts',(-18.0102664112651,-31.5558522137526,
122.790649876847)) ;
#54000=CARTESIAN_POINT('Ctrl Pts',(-18.1876243917938,-31.7559064694129,
123.328998046209)) ;
#54001=CARTESIAN_POINT('Ctrl Pts',(-17.8822137795074,-31.5759173889324,
123.308303291757)) ;
#54002=CARTESIAN_POINT('Ctrl Pts',(-18.2322702694616,-31.7757331125157,
123.748268184179)) ;
#54003=CARTESIAN_POINT('Ctrl Pts',(-17.9380242801486,-31.5957440320352,
123.832388879156)) ;
#54004=CARTESIAN_POINT('Ctrl Pts',(-18.4169480013837,-31.7956418219641,
124.129048330367)) ;
#54005=CARTESIAN_POINT('Ctrl Pts',(-18.1688732798574,-31.6156527414836,
124.308361931799)) ;
#54006=CARTESIAN_POINT('Ctrl Pts',(-18.7212311690732,-31.8155936589959,
124.424824302643)) ;
#54007=CARTESIAN_POINT('Ctrl Pts',(-18.5492284833839,-31.6356045785154,
124.678079899821)) ;
#54008=CARTESIAN_POINT('Ctrl Pts',(-19.109410695338,-31.835602133699,124.59881362796)) ;
#54009=CARTESIAN_POINT('Ctrl Pts',(-19.034454048953,-31.6556130532185,124.895564294194)) ;
#54010=CARTESIAN_POINT('Ctrl Pts',(-19.5292929940374,-31.8554035924605,
124.630074904832)) ;
#54011=CARTESIAN_POINT('Ctrl Pts',(-19.5593044715077,-31.67541451198,124.934638681304)) ;
#54012=CARTESIAN_POINT('Ctrl Pts',(-19.9381051953959,-31.8753604806964,
124.516346944635)) ;
#54013=CARTESIAN_POINT('Ctrl Pts',(-20.0703188208076,-31.695371400216,124.792477849263)) ;
#54014=CARTESIAN_POINT('Ctrl Pts',(-20.2834627517452,-31.8953443181105,
124.268832628097)) ;
#54015=CARTESIAN_POINT('Ctrl Pts',(-20.5020147232158,-31.7153552376301,
124.483083842068)) ;
#54016=CARTESIAN_POINT('Ctrl Pts',(-20.5222631166498,-31.9151527573315,
123.921823635472)) ;
#54017=CARTESIAN_POINT('Ctrl Pts',(-20.8005129695027,-31.735163676851,124.049324638418)) ;
#54018=CARTESIAN_POINT('Ctrl Pts',(-20.6296391609579,-31.9351384667117,
123.510794184968)) ;
#54019=CARTESIAN_POINT('Ctrl Pts',(-20.934732846759,-31.7551493862312,123.535538119672)) ;
#54020=CARTESIAN_POINT('Ctrl Pts',(-20.5906472244068,-31.955007989727,123.089943615466)) ;
#54021=CARTESIAN_POINT('Ctrl Pts',(-20.885993395325,-31.7750189092465,123.0094768274)) ;
#54022=CARTESIAN_POINT('Ctrl Pts',(-20.4089954990554,-31.9750287288442,
122.705129085206)) ;
#54023=CARTESIAN_POINT('Ctrl Pts',(-20.6589290214595,-31.7950396483637,
122.528458277059)) ;
#54024=CARTESIAN_POINT('Ctrl Pts',(-20.1103555337929,-31.9948327938211,
122.408035535206)) ;
#54025=CARTESIAN_POINT('Ctrl Pts',(-20.2856318118138,-31.8148437133407,
122.157092624872)) ;
#54026=CARTESIAN_POINT('Ctrl Pts',(-19.7236013982933,-32.0148947575519,
122.228362978264)) ;
#54027=CARTESIAN_POINT('Ctrl Pts',(-19.8021889397508,-31.8349056770714,
121.932500294305)) ;
#54028=CARTESIAN_POINT('Ctrl Pts',(-19.3033421555285,-32.0347279378404,
122.192269701717)) ;
#54029=CARTESIAN_POINT('Ctrl Pts',(-19.2768672597533,-31.8547388573599,
121.887382590581)) ;
#54030=CARTESIAN_POINT('Ctrl Pts',(-18.8940840487304,-32.0546471351664,
122.301037263848)) ;
#54031=CARTESIAN_POINT('Ctrl Pts',(-18.7652950498026,-31.874658054686,122.023339534989)) ;
#54032=CARTESIAN_POINT('Ctrl Pts',(-18.5462767706842,-32.0745851602798,
122.543427443625)) ;
#54033=CARTESIAN_POINT('Ctrl Pts',(-18.3305352275354,-31.8945960797993,
122.326324931548)) ;
#54034=CARTESIAN_POINT('Ctrl Pts',(-18.3022836708014,-32.0944632063358,
122.888601365163)) ;
#54035=CARTESIAN_POINT('Ctrl Pts',(-18.0255423059027,-31.9144741258554,
122.757789608099)) ;
#54036=CARTESIAN_POINT('Ctrl Pts',(-18.1901182041216,-32.1144479406239,
123.298403225457)) ;
#54037=CARTESIAN_POINT('Ctrl Pts',(-17.8853325729404,-31.9344588601434,
123.270040998392)) ;
#54038=CARTESIAN_POINT('Ctrl Pts',(-18.2243400099676,-32.1343587573024,
123.720498462101)) ;
#54039=CARTESIAN_POINT('Ctrl Pts',(-17.9281065572994,-31.9543696768219,
123.797659471974)) ;
#54040=CARTESIAN_POINT('Ctrl Pts',(-18.4014838664741,-32.1543577328211,
124.106965037813)) ;
#54041=CARTESIAN_POINT('Ctrl Pts',(-18.1495333780784,-31.9743686523406,
124.280744001322)) ;
#54042=CARTESIAN_POINT('Ctrl Pts',(-18.6967305235978,-32.1741626534663,
124.40735164037)) ;
#54043=CARTESIAN_POINT('Ctrl Pts',(-18.5185878609863,-31.9941735729858,
124.656228575554)) ;
#54044=CARTESIAN_POINT('Ctrl Pts',(-19.0797563575211,-32.1941466137575,
124.59108153163)) ;
#54045=CARTESIAN_POINT('Ctrl Pts',(-18.9973682959692,-32.0141575332771,
124.885894562839)) ;
#54046=CARTESIAN_POINT('Ctrl Pts',(-19.500620909332,-32.2140328174815,124.632705731497)) ;
#54047=CARTESIAN_POINT('Ctrl Pts',(-19.5234477413733,-32.034043737001,124.937928873815)) ;
#54048=CARTESIAN_POINT('Ctrl Pts',(-19.91172625123,-32.2339819958047,124.528376651481)) ;
#54049=CARTESIAN_POINT('Ctrl Pts',(-20.0373301586455,-32.0539929153242,
124.807521706338)) ;
#54050=CARTESIAN_POINT('Ctrl Pts',(-20.2616847114276,-32.2538837950442,
124.290492641391)) ;
#54051=CARTESIAN_POINT('Ctrl Pts',(-20.4747803852408,-32.0738947145637,
124.510171457573)) ;
#54052=CARTESIAN_POINT('Ctrl Pts',(-20.5099132977842,-32.2737624000966,
123.948363389314)) ;
#54053=CARTESIAN_POINT('Ctrl Pts',(-20.7850691734418,-32.0937733196161,
124.082510674381)) ;
#54054=CARTESIAN_POINT('Ctrl Pts',(-20.627203071623,-32.2937947598223,123.538857802633)) ;
#54055=CARTESIAN_POINT('Ctrl Pts',(-20.9316880821038,-32.1138056793418,
123.570639459005)) ;
#54056=CARTESIAN_POINT('Ctrl Pts',(-20.6022414190364,-32.3103764857783,
123.187181314506)) ;
#54057=CARTESIAN_POINT('Ctrl Pts',(-20.9004840930374,-32.1303874052979,
123.131013871443)) ;
#54058=CARTESIAN_POINT('Ctrl Pts',(-20.5124528604533,-32.3235706560763,
122.924720422985)) ;
#54059=CARTESIAN_POINT('Ctrl Pts',(-20.788262838901,-32.1435815755958,122.802971043115)) ;
#54060=CARTESIAN_POINT('Ctrl Pts',(-20.3776944343899,-32.3368828341695,
122.679500006612)) ;
#54061=CARTESIAN_POINT('Ctrl Pts',(-20.6197762200585,-32.156893753689,122.496386987727)) ;
#54062=CARTESIAN_POINT('Ctrl Pts',(-20.1339928139378,-32.3534490137628,
122.425047262597)) ;
#54063=CARTESIAN_POINT('Ctrl Pts',(-20.3152084468331,-32.1734599332823,
122.178383590779)) ;
#54064=CARTESIAN_POINT('Ctrl Pts',(-19.8172190621121,-32.370077208623,122.268225534679)) ;
#54065=CARTESIAN_POINT('Ctrl Pts',(-19.9191951146559,-32.1900881281425,
121.98231868388)) ;
#54066=CARTESIAN_POINT('Ctrl Pts',(-19.5432299461013,-32.3833657903327,
122.213296215293)) ;
#54067=CARTESIAN_POINT('Ctrl Pts',(-19.576742054398,-32.2033767098523,121.913670003135)) ;
#54068=CARTESIAN_POINT('Ctrl Pts',(-19.3337508719107,-32.3933340384363,
122.208232309393)) ;
#54069=CARTESIAN_POINT('Ctrl Pts',(-19.3148866166722,-32.2133449579559,
121.90733429029)) ;
#54070=CARTESIAN_POINT('Ctrl Pts',(-19.1276189549108,-32.4032487946925,
122.239193486121)) ;
#54071=CARTESIAN_POINT('Ctrl Pts',(-19.0572238635517,-32.223259714212,121.946033185413)) ;
#54072=CARTESIAN_POINT('Ctrl Pts',(-18.9279557063151,-32.4132619453437,
122.305913698926)) ;
#54073=CARTESIAN_POINT('Ctrl Pts',(-18.8076409321752,-32.2332728648632,
122.029433371211)) ;
#54074=CARTESIAN_POINT('Ctrl Pts',(-18.7430842089401,-32.4232746525457,
122.406578399065)) ;
#54075=CARTESIAN_POINT('Ctrl Pts',(-18.5765593856167,-32.2432855720652,
122.155251711997)) ;
#54076=CARTESIAN_POINT('Ctrl Pts',(-18.5254677572598,-32.436493941237,122.579410532713)) ;
#54077=CARTESIAN_POINT('Ctrl Pts',(-18.3044914720328,-32.2565048607565,
122.371339808038)) ;
#54078=CARTESIAN_POINT('Ctrl Pts',(-18.3148360496128,-32.453112622235,122.863088731423)) ;
#54079=CARTESIAN_POINT('Ctrl Pts',(-18.041252038348,-32.2731235417546,122.725865755934)) ;
#54080=CARTESIAN_POINT('Ctrl Pts',(-18.2135427727924,-32.4696775300085,
123.200444286709)) ;
#54081=CARTESIAN_POINT('Ctrl Pts',(-17.9146049568551,-32.289688449528,123.147620680701)) ;
#54082=CARTESIAN_POINT('Ctrl Pts',(-18.2053428109417,-32.4830760016193,
123.482028619465)) ;
#54083=CARTESIAN_POINT('Ctrl Pts',(-17.9043631043354,-32.3030869211388,
123.499558748913)) ;
#54084=CARTESIAN_POINT('Ctrl Pts',(-18.2351263930126,-32.4929172571063,
123.686778633759)) ;
#54085=CARTESIAN_POINT('Ctrl Pts',(-17.9415874187144,-32.3129281766258,
123.755505137596)) ;
#54086=CARTESIAN_POINT('Ctrl Pts',(-18.3005104295691,-32.5029035726945,
123.886247272274)) ;
#54087=CARTESIAN_POINT('Ctrl Pts',(-18.0233154438323,-32.322914492214,124.00483961092)) ;
#54088=CARTESIAN_POINT('Ctrl Pts',(-18.3989864711992,-32.5128401802809,
124.070517770327)) ;
#54089=CARTESIAN_POINT('Ctrl Pts',(-18.1464078761575,-32.3328510998004,
124.235179732808)) ;
#54090=CARTESIAN_POINT('Ctrl Pts',(-18.5294794836623,-32.5228900476492,
124.236655331214)) ;
#54091=CARTESIAN_POINT('Ctrl Pts',(-18.3095220074042,-32.3429009671687,
124.442853309995)) ;
#54092=CARTESIAN_POINT('Ctrl Pts',(-18.6836393496476,-32.532740542324,124.374955006091)) ;
#54093=CARTESIAN_POINT('Ctrl Pts',(-18.50222003047,-32.3527514618435,124.615730119601)) ;
#54094=CARTESIAN_POINT('Ctrl Pts',(-18.8613101056891,-32.5427123427185,
124.486175930194)) ;
#54095=CARTESIAN_POINT('Ctrl Pts',(-18.7243070866431,-32.362723262238,124.754758703811)) ;
#54096=CARTESIAN_POINT('Ctrl Pts',(-19.0561314475104,-32.5527083097443,
124.565050529732)) ;
#54097=CARTESIAN_POINT('Ctrl Pts',(-18.9678327867977,-32.3727192292638,
124.853354582607)) ;
#54098=CARTESIAN_POINT('Ctrl Pts',(-19.2625472172633,-32.5627457691255,
124.608788649609)) ;
#54099=CARTESIAN_POINT('Ctrl Pts',(-19.225851948972,-32.382756688645,124.908029995055)) ;
#54100=CARTESIAN_POINT('Ctrl Pts',(-19.4693094256783,-32.5725864700262,
124.616272691469)) ;
#54101=CARTESIAN_POINT('Ctrl Pts',(-19.4843048557994,-32.3925973895458,
124.917387851591)) ;
#54102=CARTESIAN_POINT('Ctrl Pts',(-19.6785662287874,-32.5826344912936,
124.587453910695)) ;
#54103=CARTESIAN_POINT('Ctrl Pts',(-19.7458762677244,-32.4026454108131,
124.881367125457)) ;
#54104=CARTESIAN_POINT('Ctrl Pts',(-19.8775350367199,-32.5925818843763,
124.523064897387)) ;
#54105=CARTESIAN_POINT('Ctrl Pts',(-19.9945882738826,-32.4125928038958,
124.80088348232)) ;
#54106=CARTESIAN_POINT('Ctrl Pts',(-20.0619149648412,-32.6024920304227,
124.426032573854)) ;
#54107=CARTESIAN_POINT('Ctrl Pts',(-20.225064686472,-32.4225029499422,124.679595400819)) ;
#54108=CARTESIAN_POINT('Ctrl Pts',(-20.2289464125442,-32.6125509442723,
124.296375819046)) ;
#54109=CARTESIAN_POINT('Ctrl Pts',(-20.4338556736144,-32.4325618637918,
124.517526669095)) ;
#54110=CARTESIAN_POINT('Ctrl Pts',(-20.3680971425257,-32.6223917145616,
124.143243416164)) ;
#54111=CARTESIAN_POINT('Ctrl Pts',(-20.607796392533,-32.4424026340811,124.326112710897)) ;
#54112=CARTESIAN_POINT('Ctrl Pts',(-20.4812183694655,-32.6324545841402,
123.964505832737)) ;
#54113=CARTESIAN_POINT('Ctrl Pts',(-20.7492002052201,-32.4524655036597,
124.102692225439)) ;
#54114=CARTESIAN_POINT('Ctrl Pts',(-20.5601018658738,-32.6423489072707,
123.772009901321)) ;
#54115=CARTESIAN_POINT('Ctrl Pts',(-20.8478072364981,-32.4623598267902,
123.86207304764)) ;
#54116=CARTESIAN_POINT('Ctrl Pts',(-20.6051186285884,-32.6522907143652,
123.567933795961)) ;
#54117=CARTESIAN_POINT('Ctrl Pts',(-20.9040808604004,-32.4723016338847,
123.606978235619)) ;
#54118=CARTESIAN_POINT('Ctrl Pts',(-20.6141529517269,-32.6622932253205,
123.357815073032)) ;
#54119=CARTESIAN_POINT('Ctrl Pts',(-20.9153764260027,-32.48230414484,123.344329862461)) ;
#54120=CARTESIAN_POINT('Ctrl Pts',(-20.5861553370163,-32.6723279461389,
123.148732523265)) ;
#54121=CARTESIAN_POINT('Ctrl Pts',(-20.8803820949981,-32.4923388656584,
123.082976330961)) ;
#54122=CARTESIAN_POINT('Ctrl Pts',(-20.5238045844199,-32.6821731236446,
122.95135818224)) ;
#54123=CARTESIAN_POINT('Ctrl Pts',(-20.8024460214919,-32.5021840431641,
122.83625706854)) ;
#54124=CARTESIAN_POINT('Ctrl Pts',(-20.4271596502256,-32.6921578840457,
122.76505202383)) ;
#54125=CARTESIAN_POINT('Ctrl Pts',(-20.6816420859839,-32.5121688035652,
122.603373026508)) ;
#54126=CARTESIAN_POINT('Ctrl Pts',(-20.3002621335287,-32.7020967903621,
122.599012732577)) ;
#54127=CARTESIAN_POINT('Ctrl Pts',(-20.5230220509735,-32.5221077098816,
122.395822102311)) ;
#54128=CARTESIAN_POINT('Ctrl Pts',(-20.1448530384785,-32.7121390179978,
122.456148065448)) ;
#54129=CARTESIAN_POINT('Ctrl Pts',(-20.328762473054,-32.5321499375173,122.217239391445)) ;
#54130=CARTESIAN_POINT('Ctrl Pts',(-19.9698227420243,-32.7220242295822,
122.344065587158)) ;
#54131=CARTESIAN_POINT('Ctrl Pts',(-20.1099755421832,-32.5420351491017,
122.077133850243)) ;
#54132=CARTESIAN_POINT('Ctrl Pts',(-19.7759374579204,-32.7320231597841,
122.262927443023)) ;
#54133=CARTESIAN_POINT('Ctrl Pts',(-19.8676198088022,-32.5520340793036,
121.975708802641)) ;
#54134=CARTESIAN_POINT('Ctrl Pts',(-19.5725517032629,-32.7419405826945,
122.216894103156)) ;
#54135=CARTESIAN_POINT('Ctrl Pts',(-19.6133877400385,-32.5619515022141,
121.918164610046)) ;
#54136=CARTESIAN_POINT('Ctrl Pts',(-19.3615855045364,-32.7519885147733,
122.206786949472)) ;
#54137=CARTESIAN_POINT('Ctrl Pts',(-19.3496802081886,-32.5719994342928,
121.905528177567)) ;
#54138=CARTESIAN_POINT('Ctrl Pts',(-19.1555344402761,-32.7618658905827,
122.232817208028)) ;
#54139=CARTESIAN_POINT('Ctrl Pts',(-19.0921154350127,-32.5818768101022,
121.938063647228)) ;
#54140=CARTESIAN_POINT('Ctrl Pts',(-18.9536242961126,-32.7719197837506,
122.29520263043)) ;
#54141=CARTESIAN_POINT('Ctrl Pts',(-18.839727160302,-32.5919307032701,122.01604306292)) ;
#54142=CARTESIAN_POINT('Ctrl Pts',(-18.7684970290784,-32.7818134070039,
122.390109939971)) ;
#54143=CARTESIAN_POINT('Ctrl Pts',(-18.6083164556516,-32.6018243265234,
122.134675323862)) ;
#54144=CARTESIAN_POINT('Ctrl Pts',(-18.5998696574853,-32.7918760006269,
122.517792698711)) ;
#54145=CARTESIAN_POINT('Ctrl Pts',(-18.3975309340417,-32.6118869201464,
122.294276744004)) ;
#54146=CARTESIAN_POINT('Ctrl Pts',(-18.4590017312758,-32.8017185746159,
122.669394023076)) ;
#54147=CARTESIAN_POINT('Ctrl Pts',(-18.2214436962378,-32.6217294941355,
122.483777412006)) ;
#54148=CARTESIAN_POINT('Ctrl Pts',(-18.3445119360111,-32.8117093314989,
122.845452008546)) ;
#54149=CARTESIAN_POINT('Ctrl Pts',(-18.078329458085,-32.6317202510184,122.703848805808)) ;
#54150=CARTESIAN_POINT('Ctrl Pts',(-18.2628657738663,-32.8216373932568,
123.037550195113)) ;
#54151=CARTESIAN_POINT('Ctrl Pts',(-17.9762694760485,-32.6416483127763,
122.943971098603)) ;
#54152=CARTESIAN_POINT('Ctrl Pts',(-18.2151746216112,-32.831625369146,123.242049850644)) ;
#54153=CARTESIAN_POINT('Ctrl Pts',(-17.9166533725228,-32.6516362886655,
123.199595350713)) ;
#54154=CARTESIAN_POINT('Ctrl Pts',(-18.2040142138472,-32.8416610335024,
123.452729593888)) ;
#54155=CARTESIAN_POINT('Ctrl Pts',(-17.902700600024,-32.6616719530219,123.462944824455)) ;
#54156=CARTESIAN_POINT('Ctrl Pts',(-18.2288249971323,-32.8515169719221,
123.658452238389)) ;
#54157=CARTESIAN_POINT('Ctrl Pts',(-17.9337120199493,-32.6715278914416,
123.720099296894)) ;
#54158=CARTESIAN_POINT('Ctrl Pts',(-18.2894914318515,-32.861512463319,123.859618101424)) ;
#54159=CARTESIAN_POINT('Ctrl Pts',(-18.009543101011,-32.6815233828385,123.971557376393)) ;
#54160=CARTESIAN_POINT('Ctrl Pts',(-18.3833118947942,-32.8714222682724,
124.045643520541)) ;
#54161=CARTESIAN_POINT('Ctrl Pts',(-18.1268171253965,-32.691433187792,124.204090672423)) ;
#54162=CARTESIAN_POINT('Ctrl Pts',(-18.509018904418,-32.8814344905392,124.214478322823)) ;
#54163=CARTESIAN_POINT('Ctrl Pts',(-18.2839493309718,-32.7014454100587,
124.415135395411)) ;
#54164=CARTESIAN_POINT('Ctrl Pts',(-18.6626514296269,-32.891462371232,124.358845529882)) ;
#54165=CARTESIAN_POINT('Ctrl Pts',(-18.4759885041055,-32.7114732907515,
124.59559589002)) ;
#54166=CARTESIAN_POINT('Ctrl Pts',(-18.8358044204708,-32.9013187672146,
124.472662632877)) ;
#54167=CARTESIAN_POINT('Ctrl Pts',(-18.6924294795772,-32.7213296867342,
124.737869481036)) ;
#54168=CARTESIAN_POINT('Ctrl Pts',(-19.0291703242302,-32.9113435643946,
124.556493615886)) ;
#54169=CARTESIAN_POINT('Ctrl Pts',(-18.934136091911,-32.7313544839141,124.842659911789)) ;
#54170=CARTESIAN_POINT('Ctrl Pts',(-19.2344039020975,-32.9213744943784,
124.605003116564)) ;
#54171=CARTESIAN_POINT('Ctrl Pts',(-19.1906775296452,-32.7413854138979,
124.903298739033)) ;
#54172=CARTESIAN_POINT('Ctrl Pts',(-19.4409936637498,-32.931219096887,124.617286306071)) ;
#54173=CARTESIAN_POINT('Ctrl Pts',(-19.4489157332681,-32.7512300164066,
124.91865469574)) ;
#54174=CARTESIAN_POINT('Ctrl Pts',(-19.6497118954831,-32.9412099481111,
124.593725011282)) ;
#54175=CARTESIAN_POINT('Ctrl Pts',(-19.7098139114921,-32.7612208676307,
124.889204775852)) ;
#54176=CARTESIAN_POINT('Ctrl Pts',(-19.8519756476524,-32.9512477811224,
124.533550068226)) ;
#54177=CARTESIAN_POINT('Ctrl Pts',(-19.9626440103273,-32.7712587006419,
124.813987935886)) ;
#54178=CARTESIAN_POINT('Ctrl Pts',(-20.0372510161014,-32.9610921695878,
124.441308298038)) ;
#54179=CARTESIAN_POINT('Ctrl Pts',(-20.1942400545334,-32.7811030891073,
124.698686780633)) ;
#54180=CARTESIAN_POINT('Ctrl Pts',(-20.206287933549,-32.9710769739574,124.316898276306)) ;
#54181=CARTESIAN_POINT('Ctrl Pts',(-20.4055373691669,-32.7910878934769,
124.543175419321)) ;
#54182=CARTESIAN_POINT('Ctrl Pts',(-20.3506030576117,-32.9810164934402,
124.165738129342)) ;
#54183=CARTESIAN_POINT('Ctrl Pts',(-20.5859328056416,-32.8010274129597,
124.354225946112)) ;
#54184=CARTESIAN_POINT('Ctrl Pts',(-20.4675814605525,-32.9910562244416,
123.990072866531)) ;
#54185=CARTESIAN_POINT('Ctrl Pts',(-20.7321570746235,-32.8110671439611,
124.134645385933)) ;
#54186=CARTESIAN_POINT('Ctrl Pts',(-20.5511100440207,-33.0009443526879,
123.799699797302)) ;
#54187=CARTESIAN_POINT('Ctrl Pts',(-20.836569622994,-32.8209552722074,123.896678841639)) ;
#54188=CARTESIAN_POINT('Ctrl Pts',(-20.6011952592599,-33.0109340778964,
123.595752254043)) ;
#54189=CARTESIAN_POINT('Ctrl Pts',(-20.8991776005845,-32.8309449974159,
123.641744550618)) ;
#54190=CARTESIAN_POINT('Ctrl Pts',(-20.6149126949009,-33.0208918425979,
123.386861704438)) ;
#54191=CARTESIAN_POINT('Ctrl Pts',(-20.9163259245573,-32.8409027621174,
123.380631029214)) ;
#54192=CARTESIAN_POINT('Ctrl Pts',(-20.5927628252155,-33.0307941840099,
123.179858179155)) ;
#54193=CARTESIAN_POINT('Ctrl Pts',(-20.8886398163687,-32.8508051035294,
123.121875613537)) ;
#54194=CARTESIAN_POINT('Ctrl Pts',(-20.5341646522333,-33.0408383797163,
122.977001703688)) ;
#54195=CARTESIAN_POINT('Ctrl Pts',(-20.81539343834,-32.8608492992358,122.868304834781)) ;
#54196=CARTESIAN_POINT('Ctrl Pts',(-20.4425109806158,-33.0507457804755,
122.789954482795)) ;
#54197=CARTESIAN_POINT('Ctrl Pts',(-20.700827186029,-32.870756699995,122.63449448841)) ;
#54198=CARTESIAN_POINT('Ctrl Pts',(-20.3187974646894,-33.0607563803499,
122.619697924543)) ;
#54199=CARTESIAN_POINT('Ctrl Pts',(-20.546186232137,-32.8807672998694,122.421673048436)) ;
#54200=CARTESIAN_POINT('Ctrl Pts',(-20.1668178861132,-33.0707866762621,
122.473511957559)) ;
#54201=CARTESIAN_POINT('Ctrl Pts',(-20.3562127677828,-32.8907975957816,
122.238939688334)) ;
#54202=CARTESIAN_POINT('Ctrl Pts',(-19.9950035419231,-33.0806414559118,
122.357764747843)) ;
#54203=CARTESIAN_POINT('Ctrl Pts',(-20.1414444852479,-32.9006523754313,
122.094253937415)) ;
#54204=CARTESIAN_POINT('Ctrl Pts',(-19.8039737443084,-33.0905987841293,
122.272141541311)) ;
#54205=CARTESIAN_POINT('Ctrl Pts',(-19.9026572209187,-32.9106097036488,
121.987223818312)) ;
#54206=CARTESIAN_POINT('Ctrl Pts',(-19.5992424579009,-33.1006378170362,
122.220935616222)) ;
#54207=CARTESIAN_POINT('Ctrl Pts',(-19.6467435512456,-32.9206487365557,
121.923215339334)) ;
#54208=CARTESIAN_POINT('Ctrl Pts',(-19.3921897280463,-33.1105109289255,
122.205912912299)) ;
#54209=CARTESIAN_POINT('Ctrl Pts',(-19.3879265897739,-32.930521848445,121.904435880023)) ;
#54210=CARTESIAN_POINT('Ctrl Pts',(-19.1815696557166,-33.1205842139526,
122.227554268862)) ;
#54211=CARTESIAN_POINT('Ctrl Pts',(-19.1246518187716,-32.9405951334721,
121.931486510067)) ;
#54212=CARTESIAN_POINT('Ctrl Pts',(-18.9828627675349,-33.1304045336893,
122.283747306268)) ;
#54213=CARTESIAN_POINT('Ctrl Pts',(-18.8762664626598,-32.9504154532089,
122.001727342334)) ;
#54214=CARTESIAN_POINT('Ctrl Pts',(-18.7920430269983,-33.1404831990678,
122.37573379343)) ;
#54215=CARTESIAN_POINT('Ctrl Pts',(-18.6377418414176,-32.9604941185873,
122.116709479796)) ;
#54216=CARTESIAN_POINT('Ctrl Pts',(-18.6238449944928,-33.1503347895516,
122.496666905546)) ;
#54217=CARTESIAN_POINT('Ctrl Pts',(-18.4274927505842,-32.9703457090711,
122.267875972223)) ;
#54218=CARTESIAN_POINT('Ctrl Pts',(-18.4758763515475,-33.1604079398705,
122.648110975471)) ;
#54219=CARTESIAN_POINT('Ctrl Pts',(-18.2425317132548,-32.98041885939,122.457180219299)) ;
#54220=CARTESIAN_POINT('Ctrl Pts',(-18.3591783280429,-33.1702503198455,
122.8190052862)) ;
#54221=CARTESIAN_POINT('Ctrl Pts',(-18.0966577528387,-32.9902612393651,
122.670798846568)) ;
#54222=CARTESIAN_POINT('Ctrl Pts',(-18.2721117533038,-33.1802312960886,
123.009903540524)) ;
#54223=CARTESIAN_POINT('Ctrl Pts',(-17.9878239541792,-33.0002422156081,
122.909421733985)) ;
#54224=CARTESIAN_POINT('Ctrl Pts',(-18.2196648188066,-33.1902476244439,
123.213853808958)) ;
#54225=CARTESIAN_POINT('Ctrl Pts',(-17.9222646670359,-33.0102585439634,
123.164359426885)) ;
#54226=CARTESIAN_POINT('Ctrl Pts',(-18.2033572918697,-33.200145421435,123.421288579882)) ;
#54227=CARTESIAN_POINT('Ctrl Pts',(-17.9018796511205,-33.0201563409545,
123.423653833824)) ;
#54228=CARTESIAN_POINT('Ctrl Pts',(-18.223190034098,-33.2101579781671,123.630863236516)) ;
#54229=CARTESIAN_POINT('Ctrl Pts',(-17.9266701884675,-33.0301688976866,
123.685622214874)) ;
#54230=CARTESIAN_POINT('Ctrl Pts',(-18.2796939241535,-33.2201900130135,
123.834047999503)) ;
#54231=CARTESIAN_POINT('Ctrl Pts',(-17.9972994487156,-33.0402009325331,
123.93960319975)) ;
#54232=CARTESIAN_POINT('Ctrl Pts',(-18.3684191094839,-33.230029413829,124.020926505679)) ;
#54233=CARTESIAN_POINT('Ctrl Pts',(-18.1082062114621,-33.0500403333485,
124.173202825663)) ;
#54234=CARTESIAN_POINT('Ctrl Pts',(-18.4908474188606,-33.2400951994806,
124.193500366468)) ;
#54235=CARTESIAN_POINT('Ctrl Pts',(-18.2612411135515,-33.0601061190001,
124.388920029592)) ;
#54236=CARTESIAN_POINT('Ctrl Pts',(-18.6388594412923,-33.2499856545952,
124.339567692069)) ;
#54237=CARTESIAN_POINT('Ctrl Pts',(-18.4462566310089,-33.0699965741147,
124.571505177055)) ;
#54238=CARTESIAN_POINT('Ctrl Pts',(-18.8114608537052,-33.2599777732309,
124.459283778179)) ;
#54239=CARTESIAN_POINT('Ctrl Pts',(-18.6620084680312,-33.0799886927505,
124.721150558887)) ;
#54240=CARTESIAN_POINT('Ctrl Pts',(-19.0017546265229,-33.269940599994,124.546778303222)) ;
#54241=CARTESIAN_POINT('Ctrl Pts',(-18.8998759882666,-33.0899515195135,
124.830519144868)) ;
#54242=CARTESIAN_POINT('Ctrl Pts',(-19.2030467259017,-33.2798448832669,
124.600106280176)) ;
#54243=CARTESIAN_POINT('Ctrl Pts',(-19.1514920072806,-33.0998558027864,
124.897179406919)) ;
#54244=CARTESIAN_POINT('Ctrl Pts',(-19.4137849185456,-33.289905317214,124.617764888055)) ;
#54245=CARTESIAN_POINT('Ctrl Pts',(-19.414914385357,-33.1099162367335,124.919252762314)) ;
#54246=CARTESIAN_POINT('Ctrl Pts',(-19.6198604520968,-33.2997458698872,
124.599243558957)) ;
#54247=CARTESIAN_POINT('Ctrl Pts',(-19.6725102686999,-33.1197567894067,
124.896100987935)) ;
#54248=CARTESIAN_POINT('Ctrl Pts',(-19.8241111476887,-33.3098080898329,
124.544278855776)) ;
#54249=CARTESIAN_POINT('Ctrl Pts',(-19.9278232585895,-33.1298190093524,
124.827395120553)) ;
#54250=CARTESIAN_POINT('Ctrl Pts',(-20.0125096552998,-33.3197052291114,
124.455943774085)) ;
#54251=CARTESIAN_POINT('Ctrl Pts',(-20.163322301102,-33.139716148631,124.716975844288)) ;
#54252=CARTESIAN_POINT('Ctrl Pts',(-20.1836814999991,-33.3296364212465,
124.336404331942)) ;
#54253=CARTESIAN_POINT('Ctrl Pts',(-20.3772875394294,-33.149647340766,124.567550900736)) ;
#54254=CARTESIAN_POINT('Ctrl Pts',(-20.3329814659399,-33.3396785758916,
124.187146312258)) ;
#54255=CARTESIAN_POINT('Ctrl Pts',(-20.5639122195022,-33.1596894954111,
124.380978397001)) ;
#54256=CARTESIAN_POINT('Ctrl Pts',(-20.4523759830474,-33.3495653369109,
124.016987842125)) ;
#54257=CARTESIAN_POINT('Ctrl Pts',(-20.7131557899143,-33.1695762564304,
124.168279265577)) ;
#54258=CARTESIAN_POINT('Ctrl Pts',(-20.5416382969896,-33.3595646386281,
123.826694295305)) ;
#54259=CARTESIAN_POINT('Ctrl Pts',(-20.8247334247518,-33.1795755581476,
123.930412036579)) ;
#54260=CARTESIAN_POINT('Ctrl Pts',(-20.596223942968,-33.3694854367949,123.625368027277)) ;
#54261=CARTESIAN_POINT('Ctrl Pts',(-20.8929652908593,-33.1894963563144,
123.678753341758)) ;
#54262=CARTESIAN_POINT('Ctrl Pts',(-20.615255722677,-33.3795194903916,123.415304326235)) ;
#54263=CARTESIAN_POINT('Ctrl Pts',(-20.9167545832082,-33.1995304099111,
123.416173818306)) ;
#54264=CARTESIAN_POINT('Ctrl Pts',(-20.5978416091603,-33.389442607958,123.207385396435)) ;
#54265=CARTESIAN_POINT('Ctrl Pts',(-20.8949864128072,-33.2094535274775,
123.156274431538)) ;
#54266=CARTESIAN_POINT('Ctrl Pts',(-20.5438456870571,-33.3994987314571,
123.003007585044)) ;
#54267=CARTESIAN_POINT('Ctrl Pts',(-20.827491153676,-33.2195096509766,122.90080257036)) ;
#54268=CARTESIAN_POINT('Ctrl Pts',(-20.4571105200585,-33.4093441731119,
122.81506612472)) ;
#54269=CARTESIAN_POINT('Ctrl Pts',(-20.7190711620445,-33.2293550926315,
122.665874666399)) ;
#54270=CARTESIAN_POINT('Ctrl Pts',(-20.3382374891591,-33.4193064742361,
122.642647202006)) ;
#54271=CARTESIAN_POINT('Ctrl Pts',(-20.5704789954929,-33.2393173937556,
122.450351068565)) ;
#54272=CARTESIAN_POINT('Ctrl Pts',(-20.1900385777374,-33.4293349535112,
122.492672258745)) ;
#54273=CARTESIAN_POINT('Ctrl Pts',(-20.3852299652996,-33.2493458730307,
122.262882911192)) ;
#54274=CARTESIAN_POINT('Ctrl Pts',(-20.0201373732377,-33.4392453070209,
122.372100343306)) ;
#54275=CARTESIAN_POINT('Ctrl Pts',(-20.1728523554748,-33.2592562265404,
122.11216805785)) ;
#54276=CARTESIAN_POINT('Ctrl Pts',(-19.8316354394708,-33.4491801791981,
122.282138877027)) ;
#54277=CARTESIAN_POINT('Ctrl Pts',(-19.9372239610113,-33.2691910987176,
121.999716737743)) ;
#54278=CARTESIAN_POINT('Ctrl Pts',(-19.628183907834,-33.4592213167838,122.225869096708)) ;
#54279=CARTESIAN_POINT('Ctrl Pts',(-19.6829095120336,-33.2792322363033,
121.929380340376)) ;
#54280=CARTESIAN_POINT('Ctrl Pts',(-19.4212710659109,-33.4691084659983,
122.205941031249)) ;
#54281=CARTESIAN_POINT('Ctrl Pts',(-19.4242673412654,-33.2891193855178,
121.904471017687)) ;
#54282=CARTESIAN_POINT('Ctrl Pts',(-19.2118367929156,-33.4791007007494,
122.222063506245)) ;
#54283=CARTESIAN_POINT('Ctrl Pts',(-19.162474373459,-33.2991116202689,121.924625119876)) ;
#54284=CARTESIAN_POINT('Ctrl Pts',(-19.0092605385172,-33.4890494063124,
122.274143933396)) ;
#54285=CARTESIAN_POINT('Ctrl Pts',(-18.9092537721428,-33.3090603258319,
121.989726729729)) ;
#54286=CARTESIAN_POINT('Ctrl Pts',(-18.8189440039273,-33.4989854747361,
122.360209294255)) ;
#54287=CARTESIAN_POINT('Ctrl Pts',(-18.6713579682493,-33.3189963942556,
122.097309682297)) ;
#54288=CARTESIAN_POINT('Ctrl Pts',(-18.6454357357952,-33.5089711589519,
122.478422695815)) ;
#54289=CARTESIAN_POINT('Ctrl Pts',(-18.4544730862203,-33.3289820784714,
122.245077547326)) ;
#54290=CARTESIAN_POINT('Ctrl Pts',(-18.4945213063124,-33.5190115855205,
122.625987981149)) ;
#54291=CARTESIAN_POINT('Ctrl Pts',(-18.2658309060889,-33.33902250504,122.429534786595)) ;
#54292=CARTESIAN_POINT('Ctrl Pts',(-18.3736983247787,-33.5288506989843,
122.793886133219)) ;
#54293=CARTESIAN_POINT('Ctrl Pts',(-18.1148023369346,-33.3488616185038,
122.639409270506)) ;
#54294=CARTESIAN_POINT('Ctrl Pts',(-18.28169524401,-33.5388804331601,122.983614959474)) ;
#54295=CARTESIAN_POINT('Ctrl Pts',(-17.9997997483841,-33.3588913526796,
122.876570796128)) ;
#54296=CARTESIAN_POINT('Ctrl Pts',(-18.2246058172832,-33.548902532666,123.186427396069)) ;
#54297=CARTESIAN_POINT('Ctrl Pts',(-17.9284390775416,-33.3689134521855,
123.130086625276)) ;
#54298=CARTESIAN_POINT('Ctrl Pts',(-18.2034007562052,-33.5587709725594,
123.392821859869)) ;
#54299=CARTESIAN_POINT('Ctrl Pts',(-17.9019339656912,-33.3787818920789,
123.388080969436)) ;
#54300=CARTESIAN_POINT('Ctrl Pts',(-18.218661353348,-33.568839837245,123.603931402573)) ;
#54301=CARTESIAN_POINT('Ctrl Pts',(-17.9210110193747,-33.3888507567645,
123.651967424945)) ;
#54302=CARTESIAN_POINT('Ctrl Pts',(-18.2691838785988,-33.5786825103436,
123.804599750498)) ;
#54303=CARTESIAN_POINT('Ctrl Pts',(-17.9841657908949,-33.3986934298632,
123.902803793716)) ;
#54304=CARTESIAN_POINT('Ctrl Pts',(-18.3540908209291,-33.5886431445061,
123.996012857149)) ;
#54305=CARTESIAN_POINT('Ctrl Pts',(-18.0903011026082,-33.4086540640256,
124.142069897889)) ;
#54306=CARTESIAN_POINT('Ctrl Pts',(-18.472193287036,-33.5986810601842,124.170889366581)) ;
#54307=CARTESIAN_POINT('Ctrl Pts',(-18.2379303216479,-33.4186919797037,
124.360664605596)) ;
#54308=CARTESIAN_POINT('Ctrl Pts',(-18.6162214398664,-33.6085553350436,
124.320419679324)) ;
#54309=CARTESIAN_POINT('Ctrl Pts',(-18.4179673637611,-33.4285662545632,
124.54757712207)) ;
#54310=CARTESIAN_POINT('Ctrl Pts',(-18.787310591261,-33.6186250854188,124.445049310116)) ;
#54311=CARTESIAN_POINT('Ctrl Pts',(-18.6318294559716,-33.4386360049383,
124.703362669326)) ;
#54312=CARTESIAN_POINT('Ctrl Pts',(-18.9729667813463,-33.6284583807933,
124.536013927551)) ;
#54313=CARTESIAN_POINT('Ctrl Pts',(-18.8639015605702,-33.4484693003128,
124.817067545996)) ;
#54314=CARTESIAN_POINT('Ctrl Pts',(-19.1753880863516,-33.6384886782729,
124.595078783209)) ;
#54315=CARTESIAN_POINT('Ctrl Pts',(-19.1169286180659,-33.4584995977924,
124.890896843037)) ;
#54316=CARTESIAN_POINT('Ctrl Pts',(-19.385109828368,-33.6485207647143,124.61748724909)) ;
#54317=CARTESIAN_POINT('Ctrl Pts',(-19.3790808832722,-33.4685316842339,
124.918905806976)) ;
#54318=CARTESIAN_POINT('Ctrl Pts',(-19.5912662914409,-33.6583486932033,
124.603887833734)) ;
#54319=CARTESIAN_POINT('Ctrl Pts',(-19.6367776217956,-33.4783596127228,
124.901904690763)) ;
#54320=CARTESIAN_POINT('Ctrl Pts',(-19.7955034306806,-33.668344734314,124.554404004129)) ;
#54321=CARTESIAN_POINT('Ctrl Pts',(-19.8920737335829,-33.4883556538336,
124.840047977271)) ;
#54322=CARTESIAN_POINT('Ctrl Pts',(-19.9884633521273,-33.6783705464153,
124.469582265232)) ;
#54323=CARTESIAN_POINT('Ctrl Pts',(-20.1332728673906,-33.4983814659348,
124.734019156347)) ;
#54324=CARTESIAN_POINT('Ctrl Pts',(-20.1614882739156,-33.6882577813101,
124.354388322665)) ;
#54325=CARTESIAN_POINT('Ctrl Pts',(-20.3495536622814,-33.5082687008296,
124.590024686067)) ;
#54326=CARTESIAN_POINT('Ctrl Pts',(-20.3134732484457,-33.6982346475211,
124.209865201567)) ;
#54327=CARTESIAN_POINT('Ctrl Pts',(-20.5395336849811,-33.5182455670407,
124.409369155067)) ;
#54328=CARTESIAN_POINT('Ctrl Pts',(-20.4383121739259,-33.7082275913929,
124.040861571576)) ;
#54329=CARTESIAN_POINT('Ctrl Pts',(-20.6955808168167,-33.5282385109124,
124.198113299949)) ;
#54330=CARTESIAN_POINT('Ctrl Pts',(-20.5320713712117,-33.7182655140643,
123.851823217952)) ;
#54331=CARTESIAN_POINT('Ctrl Pts',(-20.8127780413242,-33.5382764335838,
123.961814580509)) ;
#54332=CARTESIAN_POINT('Ctrl Pts',(-20.5907682106731,-33.728113978326,123.653255911294)) ;
#54333=CARTESIAN_POINT('Ctrl Pts',(-20.8861474400935,-33.5481248978455,
123.713603887081)) ;
#54334=CARTESIAN_POINT('Ctrl Pts',(-20.6148023086895,-33.73810584507,123.444605714219)) ;
#54335=CARTESIAN_POINT('Ctrl Pts',(-20.9161879633385,-33.5581167645895,
123.452790730193)) ;
#54336=CARTESIAN_POINT('Ctrl Pts',(-20.6024505201895,-33.7480235771112,
123.236442898067)) ;
#54337=CARTESIAN_POINT('Ctrl Pts',(-20.900746037756,-33.5680344966307,123.192586764759)) ;
#54338=CARTESIAN_POINT('Ctrl Pts',(-20.5536692961249,-33.7580517620064,
123.031357793843)) ;
#54339=CARTESIAN_POINT('Ctrl Pts',(-20.8397673982171,-33.578062681526,122.936230922727)) ;
#54340=CARTESIAN_POINT('Ctrl Pts',(-20.4712833025613,-33.7679369200553,
122.840563071159)) ;
#54341=CARTESIAN_POINT('Ctrl Pts',(-20.7367825954241,-33.5879478395748,
122.697737712705)) ;
#54342=CARTESIAN_POINT('Ctrl Pts',(-20.3562437198245,-33.777926280597,122.664861804041)) ;
#54343=CARTESIAN_POINT('Ctrl Pts',(-20.5929810835893,-33.5979372001165,
122.478112272329)) ;
#54344=CARTESIAN_POINT('Ctrl Pts',(-20.2113763674384,-33.7879674375313,
122.511319512586)) ;
#54345=CARTESIAN_POINT('Ctrl Pts',(-20.4118953448351,-33.6079783570509,
122.286185995833)) ;
#54346=CARTESIAN_POINT('Ctrl Pts',(-20.0457742353741,-33.7978000209865,
122.38760905629)) ;
#54347=CARTESIAN_POINT('Ctrl Pts',(-20.2048905332661,-33.617810940506,122.131549195)) ;
#54348=CARTESIAN_POINT('Ctrl Pts',(-19.8584418259696,-33.8077942409485,
122.29246902554)) ;
#54349=CARTESIAN_POINT('Ctrl Pts',(-19.9707238078469,-33.627805160468,122.012626278641)) ;
#54350=CARTESIAN_POINT('Ctrl Pts',(-19.6566211003262,-33.8178223427358,
122.23150371137)) ;
#54351=CARTESIAN_POINT('Ctrl Pts',(-19.7184472437474,-33.6378332622553,
121.936421881453)) ;
#54352=CARTESIAN_POINT('Ctrl Pts',(-19.4504107987317,-33.8277022873588,
122.206582828826)) ;
#54353=CARTESIAN_POINT('Ctrl Pts',(-19.460683413275,-33.6477132068784,121.905273090368)) ;
#54354=CARTESIAN_POINT('Ctrl Pts',(-19.2406868639278,-33.8376926139159,
122.21764677824)) ;
#54355=CARTESIAN_POINT('Ctrl Pts',(-19.1985284828869,-33.6577035334354,
121.919105510714)) ;
#54356=CARTESIAN_POINT('Ctrl Pts',(-19.0370644043963,-33.8476335455702,
122.264726339862)) ;
#54357=CARTESIAN_POINT('Ctrl Pts',(-18.9440006247054,-33.6676444650897,
121.97795745275)) ;
#54358=CARTESIAN_POINT('Ctrl Pts',(-18.8436891463967,-33.8576206640731,
122.346553932478)) ;
#54359=CARTESIAN_POINT('Ctrl Pts',(-18.7022824095767,-33.6776315835926,
122.08024433432)) ;
#54360=CARTESIAN_POINT('Ctrl Pts',(-18.6668496652182,-33.8676539969703,
122.461506020677)) ;
#54361=CARTESIAN_POINT('Ctrl Pts',(-18.4812344247497,-33.6876649164898,
122.223936502133)) ;
#54362=CARTESIAN_POINT('Ctrl Pts',(-18.5149208707951,-33.877520101415,122.602747192623)) ;
#54363=CARTESIAN_POINT('Ctrl Pts',(-18.2913247033585,-33.6975310209345,
122.400490262721)) ;
#54364=CARTESIAN_POINT('Ctrl Pts',(-18.3872775083727,-33.8875862152953,
122.77150901783)) ;
#54365=CARTESIAN_POINT('Ctrl Pts',(-18.1317726323046,-33.7075971348149,
122.611443968916)) ;
#54366=CARTESIAN_POINT('Ctrl Pts',(-18.2928599718456,-33.8974422270637,
122.955967537504)) ;
#54367=CARTESIAN_POINT('Ctrl Pts',(-18.0137527033652,-33.7174531465833,
122.842018843036)) ;
#54368=CARTESIAN_POINT('Ctrl Pts',(-18.2304603251342,-33.9074369306951,
123.156602452202)) ;
#54369=CARTESIAN_POINT('Ctrl Pts',(-17.9357556598601,-33.7274478502146,
123.092813373059)) ;
#54370=CARTESIAN_POINT('Ctrl Pts',(-18.2041945369859,-33.9174682664199,
123.365854471469)) ;
#54371=CARTESIAN_POINT('Ctrl Pts',(-17.9029259939187,-33.7374791859395,
123.354378720202)) ;
#54372=CARTESIAN_POINT('Ctrl Pts',(-18.2141592542206,-33.9273347916236,
123.573047505969)) ;
#54373=CARTESIAN_POINT('Ctrl Pts',(-17.9153845547752,-33.7473457111431,
123.613370405328)) ;
#54374=CARTESIAN_POINT('Ctrl Pts',(-18.2601719129641,-33.9373222196694,
123.777885455416)) ;
#54375=CARTESIAN_POINT('Ctrl Pts',(-17.9729030334191,-33.7573331391889,
123.869417371862)) ;
#54376=CARTESIAN_POINT('Ctrl Pts',(-18.3406253597855,-33.9472671493558,
123.970893068674)) ;
#54377=CARTESIAN_POINT('Ctrl Pts',(-18.0734724274163,-33.7672780688754,
124.110676065963)) ;
#54378=CARTESIAN_POINT('Ctrl Pts',(-18.4545761365393,-33.9573120674643,
124.148662539094)) ;
#54379=CARTESIAN_POINT('Ctrl Pts',(-18.2159131528349,-33.7773229869839,
124.332886434406)) ;
#54380=CARTESIAN_POINT('Ctrl Pts',(-18.5949446142755,-33.9671740370782,
124.301270643735)) ;
#54381=CARTESIAN_POINT('Ctrl Pts',(-18.3913760379142,-33.7871849565978,
124.52364504647)) ;
#54382=CARTESIAN_POINT('Ctrl Pts',(-18.7615730312214,-33.9771661050995,
124.42915104515)) ;
#54383=CARTESIAN_POINT('Ctrl Pts',(-18.5996633148228,-33.797177024619,124.683493416248)) ;
#54384=CARTESIAN_POINT('Ctrl Pts',(-18.946781772386,-33.987097030474,124.525545967815)) ;
#54385=CARTESIAN_POINT('Ctrl Pts',(-18.8311757133962,-33.8071079499936,
124.803984732283)) ;
#54386=CARTESIAN_POINT('Ctrl Pts',(-19.1461772309718,-33.9970476586975,
124.588768735179)) ;
#54387=CARTESIAN_POINT('Ctrl Pts',(-19.080421032467,-33.817058578217,124.883010582699)) ;
#54388=CARTESIAN_POINT('Ctrl Pts',(-19.3545768509614,-34.0070478977566,
124.616672563708)) ;
#54389=CARTESIAN_POINT('Ctrl Pts',(-19.3409209971834,-33.8270588172761,
124.917887618158)) ;
#54390=CARTESIAN_POINT('Ctrl Pts',(-19.5652047456883,-34.0170763531258,
124.607640135001)) ;
#54391=CARTESIAN_POINT('Ctrl Pts',(-19.6042058083347,-33.8370872726453,
124.906594291066)) ;
#54392=CARTESIAN_POINT('Ctrl Pts',(-19.7678153879952,-34.026942387709,124.563211304919)) ;
#54393=CARTESIAN_POINT('Ctrl Pts',(-19.8574687091983,-33.8469533072286,
124.851055548432)) ;
#54394=CARTESIAN_POINT('Ctrl Pts',(-19.9621929863248,-34.0369347094565,
124.483598324612)) ;
#54395=CARTESIAN_POINT('Ctrl Pts',(-20.1004399416366,-33.856945628976,124.751536397109)) ;
#54396=CARTESIAN_POINT('Ctrl Pts',(-20.1387770996676,-34.0468669991335,
124.372126827251)) ;
#54397=CARTESIAN_POINT('Ctrl Pts',(-20.3211678424855,-33.866877918653,124.61219566423)) ;
#54398=CARTESIAN_POINT('Ctrl Pts',(-20.2945220917022,-34.0568686441042,
124.230877087231)) ;
#54399=CARTESIAN_POINT('Ctrl Pts',(-20.5158504185811,-33.8768795636238,
124.435627300018)) ;
#54400=CARTESIAN_POINT('Ctrl Pts',(-20.4659642035819,-34.0701812775203,
124.009619570015)) ;
#54401=CARTESIAN_POINT('Ctrl Pts',(-20.7301343443236,-33.8901921970398,
124.159073181108)) ;
#54402=CARTESIAN_POINT('Ctrl Pts',(-20.575254365758,-34.0834130269018,123.750361749611)) ;
#54403=CARTESIAN_POINT('Ctrl Pts',(-20.8667466132401,-33.9034239464214,
123.835025634204)) ;
#54404=CARTESIAN_POINT('Ctrl Pts',(-20.6136526413231,-34.0967362917189,
123.472950552117)) ;
#54405=CARTESIAN_POINT('Ctrl Pts',(-20.9147529610491,-33.9167472112384,
123.488209575834)) ;
#54406=CARTESIAN_POINT('Ctrl Pts',(-20.6062950710004,-34.1066119979366,
123.265445897535)) ;
#54407=CARTESIAN_POINT('Ctrl Pts',(-20.9055507235774,-33.9266229174561,
123.228839180909)) ;
#54408=CARTESIAN_POINT('Ctrl Pts',(-20.5627942065194,-34.1166015890366,
123.060012974967)) ;
#54409=CARTESIAN_POINT('Ctrl Pts',(-20.8511725359358,-33.9366125085561,
122.972045792708)) ;
#54410=CARTESIAN_POINT('Ctrl Pts',(-20.4848858375353,-34.126528685492,122.866373888595)) ;
#54411=CARTESIAN_POINT('Ctrl Pts',(-20.7537843024981,-33.9465396050116,
122.72999873478)) ;
#54412=CARTESIAN_POINT('Ctrl Pts',(-20.3734933893588,-34.1365538339966,
122.687478257524)) ;
#54413=CARTESIAN_POINT('Ctrl Pts',(-20.6145413558421,-33.9565647535161,
122.506380398479)) ;
#54414=CARTESIAN_POINT('Ctrl Pts',(-20.2346205228606,-34.1464494881433,
122.532553580072)) ;
#54415=CARTESIAN_POINT('Ctrl Pts',(-20.4409482370739,-33.9664604076628,
122.312726536622)) ;
#54416=CARTESIAN_POINT('Ctrl Pts',(-20.0693873756585,-34.1564530225215,
122.402484078199)) ;
#54417=CARTESIAN_POINT('Ctrl Pts',(-20.2344050443968,-33.976463942041,122.150141790944)) ;
#54418=CARTESIAN_POINT('Ctrl Pts',(-19.8843645713023,-34.1664381609615,
122.303256991677)) ;
#54419=CARTESIAN_POINT('Ctrl Pts',(-20.0031251937535,-33.9864490804811,
122.026110363536)) ;
#54420=CARTESIAN_POINT('Ctrl Pts',(-19.6838837822579,-34.1764740855569,
122.237544345005)) ;
#54421=CARTESIAN_POINT('Ctrl Pts',(-19.7525232072663,-33.9964850050764,
121.94397216807)) ;
#54422=CARTESIAN_POINT('Ctrl Pts',(-19.4789063239412,-34.1863253609846,
122.207945323593)) ;
#54423=CARTESIAN_POINT('Ctrl Pts',(-19.4963012262231,-34.0063362805041,
121.906976170145)) ;
#54424=CARTESIAN_POINT('Ctrl Pts',(-19.2689143031909,-34.1963176221459,
122.213879430628)) ;
#54425=CARTESIAN_POINT('Ctrl Pts',(-19.2338112579513,-34.0163285416655,
121.914396519775)) ;
#54426=CARTESIAN_POINT('Ctrl Pts',(-19.0622877357805,-34.2063575061635,
122.256906073786)) ;
#54427=CARTESIAN_POINT('Ctrl Pts',(-18.9755284714105,-34.0263684256831,
121.968182550154)) ;
#54428=CARTESIAN_POINT('Ctrl Pts',(-18.8700474354873,-34.216192280666,122.33308360955)) ;
#54429=CARTESIAN_POINT('Ctrl Pts',(-18.7352293588114,-34.0362032001855,
122.063406917974)) ;
#54430=CARTESIAN_POINT('Ctrl Pts',(-18.6896382083871,-34.2262686616863,
122.444048971715)) ;
#54431=CARTESIAN_POINT('Ctrl Pts',(-18.5097194263312,-34.0462795812058,
122.202115742268)) ;
#54432=CARTESIAN_POINT('Ctrl Pts',(-18.5347718576947,-34.2361149348369,
122.581438980249)) ;
#54433=CARTESIAN_POINT('Ctrl Pts',(-18.3161370096554,-34.0561258543564,
122.373856170524)) ;
#54434=CARTESIAN_POINT('Ctrl Pts',(-18.3597451156534,-34.2494794561221,
122.801234068625)) ;
#54435=CARTESIAN_POINT('Ctrl Pts',(-18.0973641719139,-34.0694903756417,
122.648596301471)) ;
#54436=CARTESIAN_POINT('Ctrl Pts',(-18.2477846712695,-34.2626857005566,
123.058779918869)) ;
#54437=CARTESIAN_POINT('Ctrl Pts',(-17.9574233665507,-34.0826966200761,
122.970485787003)) ;
#54438=CARTESIAN_POINT('Ctrl Pts',(-18.205709003732,-34.2759506552338,123.334400391849)) ;
#54439=CARTESIAN_POINT('Ctrl Pts',(-17.9048166902023,-34.0959615747533,
123.315069758411)) ;
#54440=CARTESIAN_POINT('Ctrl Pts',(-18.2106566690873,-34.2859829357855,
123.545267006591)) ;
#54441=CARTESIAN_POINT('Ctrl Pts',(-17.9110068530417,-34.105993855305,123.578641444101)) ;
#54442=CARTESIAN_POINT('Ctrl Pts',(-18.2516149367393,-34.2958916693034,
123.749507046798)) ;
#54443=CARTESIAN_POINT('Ctrl Pts',(-17.9622064693986,-34.1159025888229,
123.833943903039)) ;
#54444=CARTESIAN_POINT('Ctrl Pts',(-18.3271317964583,-34.3058292201709,
123.944308961896)) ;
#54445=CARTESIAN_POINT('Ctrl Pts',(-18.0566040743328,-34.1258401396904,
124.07744363058)) ;
#54446=CARTESIAN_POINT('Ctrl Pts',(-18.4364641233543,-34.3158590677648,
124.124581975054)) ;
#54447=CARTESIAN_POINT('Ctrl Pts',(-18.1932746079544,-34.1358699872843,
124.302786499538)) ;
#54448=CARTESIAN_POINT('Ctrl Pts',(-18.6196354097619,-34.3290942076852,
124.334139196948)) ;
#54449=CARTESIAN_POINT('Ctrl Pts',(-18.4222258927744,-34.1491051272048,
124.564718290422)) ;
#54450=CARTESIAN_POINT('Ctrl Pts',(-18.9138855860305,-34.3457626720564,
124.531468794228)) ;
#54451=CARTESIAN_POINT('Ctrl Pts',(-18.7900532730175,-34.1657735915759,
124.811391879021)) ;
#54452=CARTESIAN_POINT('Ctrl Pts',(-19.3240781905893,-34.3656336839303,
124.633306467972)) ;
#54453=CARTESIAN_POINT('Ctrl Pts',(-19.3028100031517,-34.1856446034498,
124.938674735145)) ;
#54454=CARTESIAN_POINT('Ctrl Pts',(-19.6773043637108,-34.3823407683133,
124.596000454904)) ;
#54455=CARTESIAN_POINT('Ctrl Pts',(-19.7442781237966,-34.2023516878328,
124.892055705593)) ;
#54456=CARTESIAN_POINT('Ctrl Pts',(-19.9358882444672,-34.3955180496239,
124.496604146033)) ;
#54457=CARTESIAN_POINT('Ctrl Pts',(-20.0675644893515,-34.2155289691434,
124.767792583742)) ;
#54458=CARTESIAN_POINT('Ctrl Pts',(-20.1754272741693,-34.408785510138,124.353698894968)) ;
#54459=CARTESIAN_POINT('Ctrl Pts',(-20.3669683529045,-34.2287964296575,
124.589169379413)) ;
#54460=CARTESIAN_POINT('Ctrl Pts',(-20.4216795722527,-34.4253994008252,
124.10043464984)) ;
#54461=CARTESIAN_POINT('Ctrl Pts',(-20.6747925425545,-34.2454103203447,
124.272577564644)) ;
#54462=CARTESIAN_POINT('Ctrl Pts',(-20.5958914665089,-34.4453482002526,
123.713647161789)) ;
#54463=CARTESIAN_POINT('Ctrl Pts',(-20.8925501701662,-34.2653591197721,
123.789095141657)) ;
#54464=CARTESIAN_POINT('Ctrl Pts',(-20.6275282466341,-34.4652693117834,
123.291312891227)) ;
#54465=CARTESIAN_POINT('Ctrl Pts',(-20.9320934630028,-34.285280231303,123.26117694891)) ;
#54466=CARTESIAN_POINT('Ctrl Pts',(-20.5142733747202,-34.4851357599563,
122.884295294386)) ;
#54467=CARTESIAN_POINT('Ctrl Pts',(-20.7905220575369,-34.3051466794758,
122.75240729887)) ;
#54468=CARTESIAN_POINT('Ctrl Pts',(-20.2668055992271,-34.5051621065734,
122.537830920578)) ;
#54469=CARTESIAN_POINT('Ctrl Pts',(-20.4811847889919,-34.325173026093,122.319328242643)) ;
#54470=CARTESIAN_POINT('Ctrl Pts',(-19.9186956223332,-34.525024150963,122.298589670166)) ;
#54471=CARTESIAN_POINT('Ctrl Pts',(-20.0460469290827,-34.3450350704825,
122.020279911525)) ;
#54472=CARTESIAN_POINT('Ctrl Pts',(-19.5084246289227,-34.5449694536441,
122.191442824304)) ;
#54473=CARTESIAN_POINT('Ctrl Pts',(-19.5332082975816,-34.3649803731636,
121.886348768435)) ;
#54474=CARTESIAN_POINT('Ctrl Pts',(-19.0872125174688,-34.564864760703,122.230706330331)) ;
#54475=CARTESIAN_POINT('Ctrl Pts',(-19.0066946738637,-34.3848756802225,
121.935430157897)) ;
#54476=CARTESIAN_POINT('Ctrl Pts',(-18.7043989473763,-34.5847580308706,
122.410642685401)) ;
#54477=CARTESIAN_POINT('Ctrl Pts',(-18.5281796662199,-34.4047689503901,
122.160351280571)) ;
#54478=CARTESIAN_POINT('Ctrl Pts',(-18.4049696018283,-34.604723623551,122.711540803692)) ;
#54479=CARTESIAN_POINT('Ctrl Pts',(-18.1538942483531,-34.4247345430706,
122.536474463816)) ;
#54480=CARTESIAN_POINT('Ctrl Pts',(-18.2267125295678,-34.6245989472359,
123.094736417654)) ;
#54481=CARTESIAN_POINT('Ctrl Pts',(-17.9310744455895,-34.4446098667554,
123.015467619805)) ;
#54482=CARTESIAN_POINT('Ctrl Pts',(-18.1893069394518,-34.6445740098108,
123.517829036567)) ;
#54483=CARTESIAN_POINT('Ctrl Pts',(-17.8843177628342,-34.4645849293304,
123.544333074614)) ;
#54484=CARTESIAN_POINT('Ctrl Pts',(-18.299019392422,-34.6645264194419,123.927638801905)) ;
#54485=CARTESIAN_POINT('Ctrl Pts',(-18.0214586109173,-34.4845373389615,
124.05659443004)) ;
#54486=CARTESIAN_POINT('Ctrl Pts',(-18.5399052285237,-34.684362473678,124.273849716243)) ;
#54487=CARTESIAN_POINT('Ctrl Pts',(-18.3225640750526,-34.5043733931976,
124.489356119952)) ;
#54488=CARTESIAN_POINT('Ctrl Pts',(-18.8866675177332,-34.7043403850956,
124.51920099619)) ;
#54489=CARTESIAN_POINT('Ctrl Pts',(-18.7560161141913,-34.5243513046151,
124.79604584641)) ;
#54490=CARTESIAN_POINT('Ctrl Pts',(-19.2952182234732,-34.7242584345991,
124.630665769838)) ;
#54491=CARTESIAN_POINT('Ctrl Pts',(-19.2667030759053,-34.5442693541186,
124.935377333796)) ;
#54492=CARTESIAN_POINT('Ctrl Pts',(-19.7164297540769,-34.7441265783672,
124.597207733981)) ;
#54493=CARTESIAN_POINT('Ctrl Pts',(-19.793215907895,-34.5641374978867,124.893556756238)) ;
#54494=CARTESIAN_POINT('Ctrl Pts',(-20.1040277686893,-34.7641774349545,
124.419895888455)) ;
#54495=CARTESIAN_POINT('Ctrl Pts',(-20.2777146691707,-34.584188354474,124.671918199702)) ;
#54496=CARTESIAN_POINT('Ctrl Pts',(-20.404229106633,-34.7839578714104,124.125155942307)) ;
#54497=CARTESIAN_POINT('Ctrl Pts',(-20.652965881669,-34.6039687909299,124.303496686961)) ;
#54498=CARTESIAN_POINT('Ctrl Pts',(-20.5886433658768,-34.8039879270882,
123.741366661607)) ;
#54499=CARTESIAN_POINT('Ctrl Pts',(-20.8834863292564,-34.6239988466077,
123.823760909385)) ;
#54500=CARTESIAN_POINT('Ctrl Pts',(-20.630003600706,-34.823869032263,123.320595871531)) ;
#54501=CARTESIAN_POINT('Ctrl Pts',(-20.9351889707772,-34.6438799517825,
123.297798988616)) ;
#54502=CARTESIAN_POINT('Ctrl Pts',(-20.5264818869687,-34.8437494946307,
122.91079906104)) ;
#54503=CARTESIAN_POINT('Ctrl Pts',(-20.8057903345395,-34.6637604141503,
122.785553366813)) ;
#54504=CARTESIAN_POINT('Ctrl Pts',(-20.2879555038815,-34.8637346417751,
122.55910414027)) ;
#54505=CARTESIAN_POINT('Ctrl Pts',(-20.5076352221649,-34.6837455612946,
122.345932909906)) ;
#54506=CARTESIAN_POINT('Ctrl Pts',(-19.9453039790159,-34.8836252203115,
122.311181550038)) ;
#54507=CARTESIAN_POINT('Ctrl Pts',(-20.0793236956332,-34.703636139831,122.036027426937)) ;
#54508=CARTESIAN_POINT('Ctrl Pts',(-19.5387683050646,-34.9035192401859,
122.194334979435)) ;
#54509=CARTESIAN_POINT('Ctrl Pts',(-19.5711560383647,-34.7235301597054,
121.889965636104)) ;
#54510=CARTESIAN_POINT('Ctrl Pts',(-19.1162346707492,-34.9234406849123,
122.223156044862)) ;
#54511=CARTESIAN_POINT('Ctrl Pts',(-19.0429893283305,-34.7434516044318,
121.925987779697)) ;
#54512=CARTESIAN_POINT('Ctrl Pts',(-18.7288788831415,-34.9433388229677,
122.393621819122)) ;
#54513=CARTESIAN_POINT('Ctrl Pts',(-18.5587933442167,-34.7633497424872,
122.139065599235)) ;
#54514=CARTESIAN_POINT('Ctrl Pts',(-18.4209986101695,-34.9634095781838,
122.68903279055)) ;
#54515=CARTESIAN_POINT('Ctrl Pts',(-18.1739396122675,-34.7834204977033,
122.508326536784)) ;
#54516=CARTESIAN_POINT('Ctrl Pts',(-18.2348330469421,-34.983195128235,123.066398593346)) ;
#54517=CARTESIAN_POINT('Ctrl Pts',(-17.941229131582,-34.8032060477545,122.980030562327)) ;
#54518=CARTESIAN_POINT('Ctrl Pts',(-18.1871490528402,-35.0031782031124,
123.488530219856)) ;
#54519=CARTESIAN_POINT('Ctrl Pts',(-17.8816194220909,-34.8231891226319,
123.507694573203)) ;
#54520=CARTESIAN_POINT('Ctrl Pts',(-18.2866725644005,-35.0230872857583,
123.899991070555)) ;
#54521=CARTESIAN_POINT('Ctrl Pts',(-18.0060182321643,-34.8430982052778,
124.022021160938)) ;
#54522=CARTESIAN_POINT('Ctrl Pts',(-18.5190486689243,-35.0429458448811,
124.252608438494)) ;
#54523=CARTESIAN_POINT('Ctrl Pts',(-18.2964865244947,-34.8629567644006,
124.462795927105)) ;
#54524=CARTESIAN_POINT('Ctrl Pts',(-18.8611531383577,-35.0629892887198,
124.506625814478)) ;
#54525=CARTESIAN_POINT('Ctrl Pts',(-18.7241036773249,-34.8830002082393,
124.7803195884)) ;
#54526=CARTESIAN_POINT('Ctrl Pts',(-19.1973105599933,-35.079489353449,124.60730897235)) ;
#54527=CARTESIAN_POINT('Ctrl Pts',(-19.144331436189,-34.8995002729685,124.906184977658)) ;
#54528=CARTESIAN_POINT('Ctrl Pts',(-19.4786570547526,-35.0928790932979,
124.615810466112)) ;
#54529=CARTESIAN_POINT('Ctrl Pts',(-19.4959856145802,-34.9128900128174,
124.916808895359)) ;
#54530=CARTESIAN_POINT('Ctrl Pts',(-19.6837596141147,-35.1027359945063,
124.58607447705)) ;
#54531=CARTESIAN_POINT('Ctrl Pts',(-19.7523697501932,-34.9227469140258,
124.879642738746)) ;
#54532=CARTESIAN_POINT('Ctrl Pts',(-19.8833526181919,-35.1127275203528,
124.520719105362)) ;
#54533=CARTESIAN_POINT('Ctrl Pts',(-20.0018598352572,-34.9327384398723,
124.797951435971)) ;
#54534=CARTESIAN_POINT('Ctrl Pts',(-20.0674176518561,-35.1226522008037,
124.422401605199)) ;
#54535=CARTESIAN_POINT('Ctrl Pts',(-20.2319445662063,-34.9426631203233,
124.675054574964)) ;
#54536=CARTESIAN_POINT('Ctrl Pts',(-20.2330436349176,-35.1326627908481,
124.292596619006)) ;
#54537=CARTESIAN_POINT('Ctrl Pts',(-20.4389718039225,-34.9526737103677,
124.512809926757)) ;
#54538=CARTESIAN_POINT('Ctrl Pts',(-20.4195165261857,-35.1459220515518,
124.085363429725)) ;
#54539=CARTESIAN_POINT('Ctrl Pts',(-20.6720998992785,-34.9659329710713,
124.253723717985)) ;
#54540=CARTESIAN_POINT('Ctrl Pts',(-20.5482036535186,-35.1592731267021,
123.832398852526)) ;
#54541=CARTESIAN_POINT('Ctrl Pts',(-20.8329350807849,-34.9792840462216,
123.937545082325)) ;
#54542=CARTESIAN_POINT('Ctrl Pts',(-20.6059607274363,-35.1724794359369,
123.560762637728)) ;
#54543=CARTESIAN_POINT('Ctrl Pts',(-20.905132938759,-34.9924903554564,123.598017654273)) ;
#54544=CARTESIAN_POINT('Ctrl Pts',(-20.6137261119894,-35.1824662695272,
123.350990307265)) ;
#54545=CARTESIAN_POINT('Ctrl Pts',(-20.9148428909647,-35.0024771890467,
123.335798885084)) ;
#54546=CARTESIAN_POINT('Ctrl Pts',(-20.5851416406984,-35.1924189970233,
123.143676946331)) ;
#54547=CARTESIAN_POINT('Ctrl Pts',(-20.8791149642013,-35.0124299165428,
123.07665769436)) ;
#54548=CARTESIAN_POINT('Ctrl Pts',(-20.5202297895318,-35.2024670938648,
122.942679277039)) ;
#54549=CARTESIAN_POINT('Ctrl Pts',(-20.7979778137979,-35.0224780133844,
122.825409407631)) ;
#54550=CARTESIAN_POINT('Ctrl Pts',(-20.4236321858874,-35.2123085507367,
122.75969231486)) ;
#54551=CARTESIAN_POINT('Ctrl Pts',(-20.6772333063753,-35.0323194702562,
122.596674503309)) ;
#54552=CARTESIAN_POINT('Ctrl Pts',(-20.2952501726806,-35.2222948176502,
122.593621170823)) ;
#54553=CARTESIAN_POINT('Ctrl Pts',(-20.5167579762687,-35.0423057371697,
122.389083764368)) ;
#54554=CARTESIAN_POINT('Ctrl Pts',(-20.1407744583381,-35.2322314185506,
122.45294261696)) ;
#54555=CARTESIAN_POINT('Ctrl Pts',(-20.3236651758771,-35.0522423380701,
122.213233449122)) ;
#54556=CARTESIAN_POINT('Ctrl Pts',(-19.9621957115618,-35.2422813613376,
122.340068651411)) ;
#54557=CARTESIAN_POINT('Ctrl Pts',(-20.1004431976586,-35.0622922808572,
122.072138574531)) ;
#54558=CARTESIAN_POINT('Ctrl Pts',(-19.77064229135,-35.2521315610234,122.261352205955)) ;
#54559=CARTESIAN_POINT('Ctrl Pts',(-19.86100238911,-35.0721424805429,121.973740369695)) ;
#54560=CARTESIAN_POINT('Ctrl Pts',(-19.5659662743928,-35.2621044659555,
122.216007869496)) ;
#54561=CARTESIAN_POINT('Ctrl Pts',(-19.605157861446,-35.082115385475,121.917057182898)) ;
#54562=CARTESIAN_POINT('Ctrl Pts',(-19.3559388586588,-35.2721028404351,
122.20693299255)) ;
#54563=CARTESIAN_POINT('Ctrl Pts',(-19.342623637523,-35.0921137599546,121.90571078375)) ;
#54564=CARTESIAN_POINT('Ctrl Pts',(-19.1471235458461,-35.2821230143051,
122.234669898377)) ;
#54565=CARTESIAN_POINT('Ctrl Pts',(-19.081604071815,-35.1021339338246,121.940379135676)) ;
#54566=CARTESIAN_POINT('Ctrl Pts',(-18.9486182041443,-35.2920240582471,
122.297318677213)) ;
#54567=CARTESIAN_POINT('Ctrl Pts',(-18.8334713867569,-35.1120349777666,
122.018687487652)) ;
#54568=CARTESIAN_POINT('Ctrl Pts',(-18.7622230203345,-35.3020128619714,
122.394038689284)) ;
#54569=CARTESIAN_POINT('Ctrl Pts',(-18.6004760332833,-35.1220237814909,
122.139585076105)) ;
#54570=CARTESIAN_POINT('Ctrl Pts',(-18.5959401033665,-35.3119783288032,
122.521468994438)) ;
#54571=CARTESIAN_POINT('Ctrl Pts',(-18.3926205881844,-35.1319892483227,
122.298870810869)) ;
#54572=CARTESIAN_POINT('Ctrl Pts',(-18.4547977142894,-35.3218818910762,
122.674558023421)) ;
#54573=CARTESIAN_POINT('Ctrl Pts',(-18.2161904039979,-35.1418928105957,
122.490230413614)) ;
#54574=CARTESIAN_POINT('Ctrl Pts',(-18.3407694318747,-35.3319425689542,
122.852663128969)) ;
#54575=CARTESIAN_POINT('Ctrl Pts',(-18.0736527310918,-35.1519534884737,
122.712860272197)) ;
#54576=CARTESIAN_POINT('Ctrl Pts',(-18.2609128534862,-35.3417828669036,
123.043535459525)) ;
#54577=CARTESIAN_POINT('Ctrl Pts',(-17.9738293170937,-35.1617937864232,
122.951450001356)) ;
#54578=CARTESIAN_POINT('Ctrl Pts',(-18.2141440011338,-35.3518458618131,
123.24982878148)) ;
#54579=CARTESIAN_POINT('Ctrl Pts',(-17.9153656041691,-35.1718567813326,
123.209316008957)) ;
#54580=CARTESIAN_POINT('Ctrl Pts',(-18.2042462712093,-35.3617401559602,
123.457624789983)) ;
#54581=CARTESIAN_POINT('Ctrl Pts',(-17.9029906879273,-35.1817510754797,
123.469061216254)) ;
#54582=CARTESIAN_POINT('Ctrl Pts',(-18.2301365974252,-35.3716819536571,
123.66499700929)) ;
#54583=CARTESIAN_POINT('Ctrl Pts',(-17.9353509722978,-35.1916928731766,
123.728277083057)) ;
#54584=CARTESIAN_POINT('Ctrl Pts',(-18.2919583226803,-35.3816845311862,
123.866019002124)) ;
#54585=CARTESIAN_POINT('Ctrl Pts',(-18.012625610303,-35.2016954507057,123.979555436283)) ;
#54586=CARTESIAN_POINT('Ctrl Pts',(-18.38832214789,-35.3917189951073,124.053667683726)) ;
#54587=CARTESIAN_POINT('Ctrl Pts',(-18.1330779755077,-35.2117299146268,
124.214117512358)) ;
#54588=CARTESIAN_POINT('Ctrl Pts',(-18.5131632869251,-35.4015651336283,
124.218788839764)) ;
#54589=CARTESIAN_POINT('Ctrl Pts',(-18.2891276128659,-35.2215760531479,
124.420521008523)) ;
#54590=CARTESIAN_POINT('Ctrl Pts',(-18.6665221671683,-35.4115463068653,
124.361984621255)) ;
#54591=CARTESIAN_POINT('Ctrl Pts',(-18.480824570798,-35.2315572263849,124.599517750325)) ;
#54592=CARTESIAN_POINT('Ctrl Pts',(-18.8419525073359,-35.4214986008226,
124.476017082833)) ;
#54593=CARTESIAN_POINT('Ctrl Pts',(-18.7001113065776,-35.2415095203421,
124.74206065123)) ;
#54594=CARTESIAN_POINT('Ctrl Pts',(-19.0353199148675,-35.4314973959572,
124.558494549662)) ;
#54595=CARTESIAN_POINT('Ctrl Pts',(-18.9418196621868,-35.2515083154767,
124.845159871899)) ;
#54596=CARTESIAN_POINT('Ctrl Pts',(-19.2409602408548,-35.441536504218,124.605934758552)) ;
#54597=CARTESIAN_POINT('Ctrl Pts',(-19.1988694219931,-35.2615474237375,
124.904462677019)) ;
#54598=CARTESIAN_POINT('Ctrl Pts',(-19.4472187958602,-35.4513614456571,
124.617157941758)) ;
#54599=CARTESIAN_POINT('Ctrl Pts',(-19.4566932433176,-35.2713723651767,
124.918494235353)) ;
#54600=CARTESIAN_POINT('Ctrl Pts',(-19.6571046505334,-35.4614161327315,
124.59216665789)) ;
#54601=CARTESIAN_POINT('Ctrl Pts',(-19.7190507496458,-35.2814270522511,
124.887257605478)) ;
#54602=CARTESIAN_POINT('Ctrl Pts',(-19.8571259179256,-35.4713589376717,
124.531443581548)) ;
#54603=CARTESIAN_POINT('Ctrl Pts',(-19.9690783925862,-35.2913698571912,
124.81135610388)) ;
#54604=CARTESIAN_POINT('Ctrl Pts',(-20.0431203480413,-35.4812627236682,
124.437854636446)) ;
#54605=CARTESIAN_POINT('Ctrl Pts',(-20.2015729913914,-35.3012736431877,
124.69437184444)) ;
#54606=CARTESIAN_POINT('Ctrl Pts',(-20.2123551288087,-35.491309540233,124.31150595345)) ;
#54607=CARTESIAN_POINT('Ctrl Pts',(-20.4131178491441,-35.3113204597525,
124.536438012433)) ;
#54608=CARTESIAN_POINT('Ctrl Pts',(-20.355073515676,-35.5012050597117,124.160099178899)) ;
#54609=CARTESIAN_POINT('Ctrl Pts',(-20.591517979772,-35.3212159792312,124.347180770875)) ;
#54610=CARTESIAN_POINT('Ctrl Pts',(-20.471223424041,-35.5112671450361,123.983338753384)) ;
#54611=CARTESIAN_POINT('Ctrl Pts',(-20.7367072780887,-35.3312780645556,
124.126231712347)) ;
#54612=CARTESIAN_POINT('Ctrl Pts',(-20.5532221554608,-35.521109855994,123.793329340615)) ;
#54613=CARTESIAN_POINT('Ctrl Pts',(-20.8392082179323,-35.3411207755136,
123.888720097038)) ;
#54614=CARTESIAN_POINT('Ctrl Pts',(-20.6021745079103,-35.5311005733001,
123.589104323875)) ;
#54615=CARTESIAN_POINT('Ctrl Pts',(-20.9004009018937,-35.3511114928196,
123.633439183878)) ;
#54616=CARTESIAN_POINT('Ctrl Pts',(-20.6148094254628,-35.5410286563966,
123.380757851225)) ;
#54617=CARTESIAN_POINT('Ctrl Pts',(-20.9161968440808,-35.3610395759162,
123.373005745106)) ;
#54618=CARTESIAN_POINT('Ctrl Pts',(-20.5912974926631,-35.5510165865084,
123.172091972982)) ;
#54619=CARTESIAN_POINT('Ctrl Pts',(-20.8868090727188,-35.3710275060279,
123.112172972214)) ;
#54620=CARTESIAN_POINT('Ctrl Pts',(-20.5312904374153,-35.5610524126357,
122.969827521401)) ;
#54621=CARTESIAN_POINT('Ctrl Pts',(-20.811802454658,-35.3810633321552,122.859341843746)) ;
#54622=CARTESIAN_POINT('Ctrl Pts',(-20.4390581243751,-35.5709077497493,
122.78428606231)) ;
#54623=CARTESIAN_POINT('Ctrl Pts',(-20.6965136131226,-35.3909186692688,
122.627413231222)) ;
#54624=CARTESIAN_POINT('Ctrl Pts',(-20.3145205708958,-35.5809054845995,
122.614998952204)) ;
#54625=CARTESIAN_POINT('Ctrl Pts',(-20.5408432693508,-35.400916404119,122.415802978902)) ;
#54626=CARTESIAN_POINT('Ctrl Pts',(-20.1638726572033,-35.5908133885839,
122.471137864884)) ;
#54627=CARTESIAN_POINT('Ctrl Pts',(-20.3525343321425,-35.4108243081035,
122.235974665486)) ;
#54628=CARTESIAN_POINT('Ctrl Pts',(-19.9889273945464,-35.6008244631324,
122.354124867634)) ;
#54629=CARTESIAN_POINT('Ctrl Pts',(-20.1338538120552,-35.4208353826519,
122.089706748465)) ;
#54630=CARTESIAN_POINT('Ctrl Pts',(-19.7958300056756,-35.610852318668,122.269519731036)) ;
#54631=CARTESIAN_POINT('Ctrl Pts',(-19.8924829762107,-35.4308632381875,
121.983948431032)) ;
#54632=CARTESIAN_POINT('Ctrl Pts',(-19.5945466869052,-35.6207099125732,
122.220212795873)) ;
#54633=CARTESIAN_POINT('Ctrl Pts',(-19.6408783355384,-35.4407208320928,
121.922312589221)) ;
#54634=CARTESIAN_POINT('Ctrl Pts',(-19.3842341645356,-35.6307365994113,
122.205941341897)) ;
#54635=CARTESIAN_POINT('Ctrl Pts',(-19.3779878358336,-35.4507475189309,
121.904471410675)) ;
#54636=CARTESIAN_POINT('Ctrl Pts',(-19.1746497432009,-35.6407652685651,
122.228931469731)) ;
#54637=CARTESIAN_POINT('Ctrl Pts',(-19.1160071597397,-35.4607761880846,
121.933207053127)) ;
#54638=CARTESIAN_POINT('Ctrl Pts',(-18.9758531060999,-35.6506104768465,
122.286508207348)) ;
#54639=CARTESIAN_POINT('Ctrl Pts',(-18.8675097602176,-35.470621396366,122.005176454094)) ;
#54640=CARTESIAN_POINT('Ctrl Pts',(-18.78706524933,-35.6606011658096,122.378575193346)) ;
#54641=CARTESIAN_POINT('Ctrl Pts',(-18.6315240045379,-35.4806120853291,
122.120258716074)) ;
#54642=CARTESIAN_POINT('Ctrl Pts',(-18.6166109529874,-35.6706390420919,
122.502982907208)) ;
#54643=CARTESIAN_POINT('Ctrl Pts',(-18.4184551335349,-35.4906499616114,
122.275766762395)) ;
#54644=CARTESIAN_POINT('Ctrl Pts',(-18.4728999980008,-35.6804834197341,
122.651921164381)) ;
#54645=CARTESIAN_POINT('Ctrl Pts',(-18.2388143579608,-35.5004943392536,
122.461939201164)) ;
#54646=CARTESIAN_POINT('Ctrl Pts',(-18.3552581448824,-35.6904682241255,
122.825736375078)) ;
#54647=CARTESIAN_POINT('Ctrl Pts',(-18.0917605508585,-35.5104791436451,
122.679207506843)) ;
#54648=CARTESIAN_POINT('Ctrl Pts',(-18.2698663052676,-35.7004077543441,
123.016483700906)) ;
#54649=CARTESIAN_POINT('Ctrl Pts',(-17.9850190704585,-35.5204186738636,
122.917641507228)) ;
#54650=CARTESIAN_POINT('Ctrl Pts',(-18.218436347525,-35.710447442381,123.221171010836)) ;
#54651=CARTESIAN_POINT('Ctrl Pts',(-17.9207300901003,-35.5304583619005,
123.173500108582)) ;
#54652=CARTESIAN_POINT('Ctrl Pts',(-18.2034516389984,-35.7203357317493,
123.428524856059)) ;
#54653=CARTESIAN_POINT('Ctrl Pts',(-17.9019975598686,-35.5403466512688,
123.432693219793)) ;
#54654=CARTESIAN_POINT('Ctrl Pts',(-18.2245179381264,-35.7303248554341,
123.637461026191)) ;
#54655=CARTESIAN_POINT('Ctrl Pts',(-17.9283290132215,-35.5503357749536,
123.693863790516)) ;
#54656=CARTESIAN_POINT('Ctrl Pts',(-18.281534545644,-35.7402848651087,123.838935805631)) ;
#54657=CARTESIAN_POINT('Ctrl Pts',(-17.9995984431471,-35.5602957846282,
123.945708092145)) ;
#54658=CARTESIAN_POINT('Ctrl Pts',(-18.3716800461657,-35.7501852948129,
124.026546743199)) ;
#54659=CARTESIAN_POINT('Ctrl Pts',(-18.1122794987908,-35.5701962143325,
124.180223126185)) ;
#54660=CARTESIAN_POINT('Ctrl Pts',(-18.4947794817171,-35.7602283762197,
124.198074355247)) ;
#54661=CARTESIAN_POINT('Ctrl Pts',(-18.2661525938325,-35.5802392957392,
124.394633262603)) ;
#54662=CARTESIAN_POINT('Ctrl Pts',(-18.6437627494517,-35.7701357701273,
124.343645611898)) ;
#54663=CARTESIAN_POINT('Ctrl Pts',(-18.4523813315997,-35.5901466896469,
124.576598857815)) ;
#54664=CARTESIAN_POINT('Ctrl Pts',(-18.8173428519059,-35.7801475011165,
124.462690565596)) ;
#54665=CARTESIAN_POINT('Ctrl Pts',(-18.6693558213399,-35.600158420636,124.725406064514)) ;
#54666=CARTESIAN_POINT('Ctrl Pts',(-19.0095259153143,-35.7901797188313,
124.549587699707)) ;
#54667=CARTESIAN_POINT('Ctrl Pts',(-18.9095840015123,-35.6101906383508,
124.834028669411)) ;
#54668=CARTESIAN_POINT('Ctrl Pts',(-19.2101294613733,-35.8000322280774,
124.601126477445)) ;
#54669=CARTESIAN_POINT('Ctrl Pts',(-19.1603393482341,-35.620043147597,124.898453661871)) ;
#54670=CARTESIAN_POINT('Ctrl Pts',(-19.4188119264436,-35.8099901646204,
124.617871878663)) ;
#54671=CARTESIAN_POINT('Ctrl Pts',(-19.4211928177101,-35.63000108414,124.91938645452)) ;
#54672=CARTESIAN_POINT('Ctrl Pts',(-19.6288700822666,-35.8200290346287,
124.59759241421)) ;
#54673=CARTESIAN_POINT('Ctrl Pts',(-19.6837654584886,-35.6400399541482,
124.894038281402)) ;
#54674=CARTESIAN_POINT('Ctrl Pts',(-19.8290080686716,-35.829902189787,124.542441752005)) ;
#54675=CARTESIAN_POINT('Ctrl Pts',(-19.933939291435,-35.6499131093065,124.825100619604)) ;
#54676=CARTESIAN_POINT('Ctrl Pts',(-20.0202339068438,-35.8399754646367,
124.45154743179)) ;
#54677=CARTESIAN_POINT('Ctrl Pts',(-20.1729716448793,-35.6599863841562,
124.711483830442)) ;
#54678=CARTESIAN_POINT('Ctrl Pts',(-20.1886685597443,-35.8497957818141,
124.332082596939)) ;
#54679=CARTESIAN_POINT('Ctrl Pts',(-20.3835167616475,-35.6698067013336,
124.562152640152)) ;
#54680=CARTESIAN_POINT('Ctrl Pts',(-20.3376896490082,-35.8598744676076,
124.181528608811)) ;
#54681=CARTESIAN_POINT('Ctrl Pts',(-20.5697933971552,-35.6798853871271,
124.373961088732)) ;
#54682=CARTESIAN_POINT('Ctrl Pts',(-20.455705088691,-35.8697259789907,124.011272096574)) ;
#54683=CARTESIAN_POINT('Ctrl Pts',(-20.7173141231935,-35.6897368985102,
124.161139832875)) ;
#54684=CARTESIAN_POINT('Ctrl Pts',(-20.5444435166218,-35.8797994252973,
123.81902845343)) ;
#54685=CARTESIAN_POINT('Ctrl Pts',(-20.8282376599489,-35.6998103448168,
123.920835993623)) ;
#54686=CARTESIAN_POINT('Ctrl Pts',(-20.5972105460148,-35.889640700422,123.618952464279)) ;
#54687=CARTESIAN_POINT('Ctrl Pts',(-20.8941975464092,-35.7096516199415,
123.670739828083)) ;
#54688=CARTESIAN_POINT('Ctrl Pts',(-20.6153373392273,-35.8996258000788,
123.409838328814)) ;
#54689=CARTESIAN_POINT('Ctrl Pts',(-20.9168565668158,-35.7196367195983,
123.409346913404)) ;
#54690=CARTESIAN_POINT('Ctrl Pts',(-20.5965431076934,-35.9096332762131,
123.200274922463)) ;
#54691=CARTESIAN_POINT('Ctrl Pts',(-20.8933643887222,-35.7296441957326,
123.147392528931)) ;
#54692=CARTESIAN_POINT('Ctrl Pts',(-20.5423042520483,-35.919555863922,122.998856521941)) ;
#54693=CARTESIAN_POINT('Ctrl Pts',(-20.8255661489224,-35.7395667834416,
122.895618637202)) ;
#54694=CARTESIAN_POINT('Ctrl Pts',(-20.453642398187,-35.9295424681954,122.808524797024)) ;
#54695=CARTESIAN_POINT('Ctrl Pts',(-20.7147391060273,-35.7495533877149,
122.657703592471)) ;
#54696=CARTESIAN_POINT('Ctrl Pts',(-20.3323311287311,-35.9395825965295,
122.635813523666)) ;
#54697=CARTESIAN_POINT('Ctrl Pts',(-20.5631005959352,-35.759593516049,122.441814323604)) ;
#54698=CARTESIAN_POINT('Ctrl Pts',(-20.1861543358301,-35.9494220310629,
122.48942292078)) ;
#54699=CARTESIAN_POINT('Ctrl Pts',(-20.3803788348249,-35.7694329505824,
122.258824742426)) ;
#54700=CARTESIAN_POINT('Ctrl Pts',(-20.0130523083208,-35.9594860855539,
122.367808286558)) ;
#54701=CARTESIAN_POINT('Ctrl Pts',(-20.1640017995225,-35.7794970050734,
122.106806406587)) ;
#54702=CARTESIAN_POINT('Ctrl Pts',(-19.8246772259409,-35.969377004791,122.279705165194)) ;
#54703=CARTESIAN_POINT('Ctrl Pts',(-19.9285321534077,-35.7893879243106,
121.996676734267)) ;
#54704=CARTESIAN_POINT('Ctrl Pts',(-19.6219619525249,-35.9793689980971,
122.224671937856)) ;
#54705=CARTESIAN_POINT('Ctrl Pts',(-19.6751379025847,-35.7993799176166,
121.92788496596)) ;
#54706=CARTESIAN_POINT('Ctrl Pts',(-19.4133577856184,-35.9893318620564,
122.205921690186)) ;
#54707=CARTESIAN_POINT('Ctrl Pts',(-19.4143822634364,-35.8093427815759,
121.904446853198)) ;
#54708=CARTESIAN_POINT('Ctrl Pts',(-19.2058271684787,-35.9992361218741,
122.223048719964)) ;
#54709=CARTESIAN_POINT('Ctrl Pts',(-19.1549680514659,-35.8192470413937,
121.925855666003)) ;
#54710=CARTESIAN_POINT('Ctrl Pts',(-19.0013346182317,-36.0092966124456,
122.276950648324)) ;
#54711=CARTESIAN_POINT('Ctrl Pts',(-18.899352673556,-35.8293075319651,121.993232864525)) ;
#54712=CARTESIAN_POINT('Ctrl Pts',(-18.8133472495276,-36.0191369620766,
122.363379425987)) ;
#54713=CARTESIAN_POINT('Ctrl Pts',(-18.664367118394,-35.8391478815961,122.101269435699)) ;
#54714=CARTESIAN_POINT('Ctrl Pts',(-18.639274963066,-36.0291999375666,122.483558189516)) ;
#54715=CARTESIAN_POINT('Ctrl Pts',(-18.4467771152488,-35.8492108570861,
122.251492745577)) ;
#54716=CARTESIAN_POINT('Ctrl Pts',(-18.4913225975558,-36.03909425771,122.629802380059)) ;
#54717=CARTESIAN_POINT('Ctrl Pts',(-18.2618359405732,-35.8591051772295,
122.434298711793)) ;
#54718=CARTESIAN_POINT('Ctrl Pts',(-18.3700032350797,-36.0490359708416,
122.799959594122)) ;
#54719=CARTESIAN_POINT('Ctrl Pts',(-18.1101865599637,-35.8690468903611,
122.646995886901)) ;
#54720=CARTESIAN_POINT('Ctrl Pts',(-18.2794097534421,-36.0590388606357,
122.98977331008)) ;
#54721=CARTESIAN_POINT('Ctrl Pts',(-17.9969449045447,-35.8790497801552,
122.884263259447)) ;
#54722=CARTESIAN_POINT('Ctrl Pts',(-18.2233291545152,-36.0690787177962,
123.193235333935)) ;
#54723=CARTESIAN_POINT('Ctrl Pts',(-17.9268443212934,-35.8890896373157,
123.138590645368)) ;
#54724=CARTESIAN_POINT('Ctrl Pts',(-18.2033834024276,-36.0789028986338,
123.39882135021)) ;
#54725=CARTESIAN_POINT('Ctrl Pts',(-17.9019122827158,-35.8989138181533,
123.39557478234)) ;
#54726=CARTESIAN_POINT('Ctrl Pts',(-18.2195239600936,-36.088959872137,123.609616533739)) ;
#54727=CARTESIAN_POINT('Ctrl Pts',(-17.9220883776684,-35.9089707916565,
123.659068393651)) ;
#54728=CARTESIAN_POINT('Ctrl Pts',(-18.271611751821,-36.0988879963241,123.811744957845)) ;
#54729=CARTESIAN_POINT('Ctrl Pts',(-17.9871986047235,-35.9188989158436,
123.911729558155)) ;
#54730=CARTESIAN_POINT('Ctrl Pts',(-18.3577130799816,-36.1088416913975,
124.002470019801)) ;
#54731=CARTESIAN_POINT('Ctrl Pts',(-18.0948259749401,-35.928852610917,124.150136156894)) ;
#54732=CARTESIAN_POINT('Ctrl Pts',(-18.4769655018994,-36.1188878849728,
124.176781923495)) ;
#54733=CARTESIAN_POINT('Ctrl Pts',(-18.2438917114054,-35.9388988044923,
124.36802560012)) ;
#54734=CARTESIAN_POINT('Ctrl Pts',(-18.6216180385642,-36.1287359873327,
124.324902759185)) ;
#54735=CARTESIAN_POINT('Ctrl Pts',(-18.4247087144062,-35.9487469068522,
124.553177298517)) ;
#54736=CARTESIAN_POINT('Ctrl Pts',(-18.7913448950173,-36.1386975755603,
124.447570338406)) ;
#54737=CARTESIAN_POINT('Ctrl Pts',(-18.6368680942363,-35.9587084950798,
124.706511430825)) ;
#54738=CARTESIAN_POINT('Ctrl Pts',(-18.9811968842923,-36.1487262457165,
124.539290730649)) ;
#54739=CARTESIAN_POINT('Ctrl Pts',(-18.8741832744098,-35.9687371652361,
124.821161297462)) ;
#54740=CARTESIAN_POINT('Ctrl Pts',(-19.181656131435,-36.1586365485983,124.596034870755)) ;
#54741=CARTESIAN_POINT('Ctrl Pts',(-19.1247583601736,-35.9786474681178,
124.892091064712)) ;
#54742=CARTESIAN_POINT('Ctrl Pts',(-19.3893970231701,-36.1685714324062,
124.617709477038)) ;
#54743=CARTESIAN_POINT('Ctrl Pts',(-19.3844352240791,-35.9885823519257,
124.919183512204)) ;
#54744=CARTESIAN_POINT('Ctrl Pts',(-19.5999475350248,-36.1786125740968,
124.602631344921)) ;
#54745=CARTESIAN_POINT('Ctrl Pts',(-19.6476231191819,-35.9986234936163,
124.90033505526)) ;
#54746=CARTESIAN_POINT('Ctrl Pts',(-19.801594360988,-36.1884996952608,124.552149971975)) ;
#54747=CARTESIAN_POINT('Ctrl Pts',(-19.8996824513604,-36.0085106147803,
124.837232249488)) ;
#54748=CARTESIAN_POINT('Ctrl Pts',(-19.9935521891846,-36.1984920381093,
124.466851568675)) ;
#54749=CARTESIAN_POINT('Ctrl Pts',(-20.1396295183763,-36.0185029576288,
124.730608252314)) ;
#54750=CARTESIAN_POINT('Ctrl Pts',(-20.1670027855748,-36.2084403393333,
124.34997292154)) ;
#54751=CARTESIAN_POINT('Ctrl Pts',(-20.3564426704474,-36.0284512588528,
124.584508836264)) ;
#54752=CARTESIAN_POINT('Ctrl Pts',(-20.317556983034,-36.2183779170154,124.205144373366)) ;
#54753=CARTESIAN_POINT('Ctrl Pts',(-20.5446351271139,-36.0383888365349,
124.403471920544)) ;
#54754=CARTESIAN_POINT('Ctrl Pts',(-20.4414732897196,-36.228364491466,124.035646668692)) ;
#54755=CARTESIAN_POINT('Ctrl Pts',(-20.6995297069063,-36.0483754109855,
124.19159891356)) ;
#54756=CARTESIAN_POINT('Ctrl Pts',(-20.5342434755889,-36.2383933013744,
123.846317983117)) ;
#54757=CARTESIAN_POINT('Ctrl Pts',(-20.8154914358056,-36.0584042208939,
123.954937669218)) ;
#54758=CARTESIAN_POINT('Ctrl Pts',(-20.5920471788539,-36.2482716226812,
123.646853844354)) ;
#54759=CARTESIAN_POINT('Ctrl Pts',(-20.8877452576722,-36.0682825422007,
123.705606150798)) ;
#54760=CARTESIAN_POINT('Ctrl Pts',(-20.6150868311933,-36.2582632700286,
123.438058171806)) ;
#54761=CARTESIAN_POINT('Ctrl Pts',(-20.9165435266129,-36.0782741895481,
123.444611225453)) ;
#54762=CARTESIAN_POINT('Ctrl Pts',(-20.6010348993728,-36.2682977934664,
123.22757890962)) ;
#54763=CARTESIAN_POINT('Ctrl Pts',(-20.8989774527681,-36.0883087129859,
123.181512331506)) ;
#54764=CARTESIAN_POINT('Ctrl Pts',(-20.5519217356949,-36.278161150345,123.026098209884)) ;
#54765=CARTESIAN_POINT('Ctrl Pts',(-20.8375844349343,-36.0981720698645,
122.929660650863)) ;
#54766=CARTESIAN_POINT('Ctrl Pts',(-20.4668785726101,-36.2882313770253,
122.832246771308)) ;
#54767=CARTESIAN_POINT('Ctrl Pts',(-20.7312794063302,-36.1082422965448,
122.687347241453)) ;
#54768=CARTESIAN_POINT('Ctrl Pts',(-20.3520998438178,-36.2980736851599,
122.660073371831)) ;
#54769=CARTESIAN_POINT('Ctrl Pts',(-20.5878041612683,-36.1180846046795,
122.472130151179)) ;
#54770=CARTESIAN_POINT('Ctrl Pts',(-20.2080189864902,-36.3080344171834,
122.508121261806)) ;
#54771=CARTESIAN_POINT('Ctrl Pts',(-20.4077016434096,-36.1280453367029,
122.282190823974)) ;
#54772=CARTESIAN_POINT('Ctrl Pts',(-20.038192664759,-36.3180723063815,122.382865970972)) ;
#54773=CARTESIAN_POINT('Ctrl Pts',(-20.1954179814077,-36.138083225901,122.125622966208)) ;
#54774=CARTESIAN_POINT('Ctrl Pts',(-19.8524204650629,-36.3279465893003,
122.290172252973)) ;
#54775=CARTESIAN_POINT('Ctrl Pts',(-19.9632011128443,-36.1479575088198,
122.009756791183)) ;
#54776=CARTESIAN_POINT('Ctrl Pts',(-19.6494833161937,-36.3380163339178,
122.23000096421)) ;
#54777=CARTESIAN_POINT('Ctrl Pts',(-19.7095295605724,-36.1580272534373,
121.934544304087)) ;
#54778=CARTESIAN_POINT('Ctrl Pts',(-19.4440883718789,-36.3478496442634,
122.206429346095)) ;
#54779=CARTESIAN_POINT('Ctrl Pts',(-19.4527844207029,-36.1678605637829,
121.905081249553)) ;
#54780=CARTESIAN_POINT('Ctrl Pts',(-19.2335726861195,-36.3578798876161,
122.218526616125)) ;
#54781=CARTESIAN_POINT('Ctrl Pts',(-19.1896400044676,-36.1778908071356,
121.920204651242)) ;
#54782=CARTESIAN_POINT('Ctrl Pts',(-19.0284500534322,-36.3679121755945,
122.267618772406)) ;
#54783=CARTESIAN_POINT('Ctrl Pts',(-18.9332371753586,-36.187923095114,121.981571396535)) ;
#54784=CARTESIAN_POINT('Ctrl Pts',(-18.838731464373,-36.3777393520626,122.349413172309)) ;
#54785=CARTESIAN_POINT('Ctrl Pts',(-18.6960884546393,-36.1977502715821,
122.083816541711)) ;
#54786=CARTESIAN_POINT('Ctrl Pts',(-18.66275010468,-36.3877447349294,122.464585531392)) ;
#54787=CARTESIAN_POINT('Ctrl Pts',(-18.4761127315903,-36.207755654449,122.227783640355)) ;
#54788=CARTESIAN_POINT('Ctrl Pts',(-18.5097875290952,-36.3977273739222,
122.608332945589)) ;
#54789=CARTESIAN_POINT('Ctrl Pts',(-18.2849106464476,-36.2177382934417,
122.407469429926)) ;
#54790=CARTESIAN_POINT('Ctrl Pts',(-18.3835787051131,-36.4077714410588,
122.777596314135)) ;
#54791=CARTESIAN_POINT('Ctrl Pts',(-18.1271511614665,-36.2277823605783,
122.619049598976)) ;
#54792=CARTESIAN_POINT('Ctrl Pts',(-18.2904495023674,-36.4175926598628,
122.961880766302)) ;
#54793=CARTESIAN_POINT('Ctrl Pts',(-18.0107408055752,-36.2376035793823,
122.849407145881)) ;
#54794=CARTESIAN_POINT('Ctrl Pts',(-18.2289081179151,-36.4276294988008,
123.163709417083)) ;
#54795=CARTESIAN_POINT('Ctrl Pts',(-17.9338160939365,-36.2476404183204,
123.101693464105)) ;
#54796=CARTESIAN_POINT('Ctrl Pts',(-18.2039726595456,-36.4376539108986,
123.372981004564)) ;
#54797=CARTESIAN_POINT('Ctrl Pts',(-17.9026486630072,-36.2576648304181,
123.363283148377)) ;
#54798=CARTESIAN_POINT('Ctrl Pts',(-18.215091683057,-36.4475059953039,123.579807254946)) ;
#54799=CARTESIAN_POINT('Ctrl Pts',(-17.9165495301555,-36.2675169148234,
123.621816862749)) ;
#54800=CARTESIAN_POINT('Ctrl Pts',(-18.2622958006013,-36.457496892047,123.784448454171)) ;
#54801=CARTESIAN_POINT('Ctrl Pts',(-17.975556789951,-36.2775078115666,123.877618050294)) ;
#54802=CARTESIAN_POINT('Ctrl Pts',(-18.3436111264905,-36.467414883948,123.976473263927)) ;
#54803=CARTESIAN_POINT('Ctrl Pts',(-18.0772031607077,-36.2874258034675,
124.117648747835)) ;
#54804=CARTESIAN_POINT('Ctrl Pts',(-18.4582275633681,-36.477442999405,124.153397817123)) ;
#54805=CARTESIAN_POINT('Ctrl Pts',(-18.2204755142129,-36.2974539189245,
124.338803226339)) ;
#54806=CARTESIAN_POINT('Ctrl Pts',(-18.5997258463659,-36.4873281753471,
124.305609353233)) ;
#54807=CARTESIAN_POINT('Ctrl Pts',(-18.3973504808242,-36.3073390948666,
124.529066690708)) ;
#54808=CARTESIAN_POINT('Ctrl Pts',(-18.7669421447371,-36.497317533754,124.432667569944)) ;
#54809=CARTESIAN_POINT('Ctrl Pts',(-18.606372387143,-36.3173284532735,124.68788770339)) ;
#54810=CARTESIAN_POINT('Ctrl Pts',(-18.9548477278309,-36.5073586813343,
124.528860622711)) ;
#54811=CARTESIAN_POINT('Ctrl Pts',(-18.8412552933677,-36.3273696008538,
124.808127004954)) ;
#54812=CARTESIAN_POINT('Ctrl Pts',(-19.1523079783713,-36.5171913043407,
124.590003139352)) ;
#54813=CARTESIAN_POINT('Ctrl Pts',(-19.088082204659,-36.3372022238602,124.884553235607)) ;
#54814=CARTESIAN_POINT('Ctrl Pts',(-19.3606753506828,-36.5271853754515,
124.616945728491)) ;
#54815=CARTESIAN_POINT('Ctrl Pts',(-19.3485418518574,-36.347196294971,124.918229067427)) ;
#54816=CARTESIAN_POINT('Ctrl Pts',(-19.5712789350383,-36.5372140330923,
124.606849592832)) ;
#54817=CARTESIAN_POINT('Ctrl Pts',(-19.6117962054508,-36.3572249526119,
124.90560655703)) ;
#54818=CARTESIAN_POINT('Ctrl Pts',(-19.7740000727098,-36.5470983592851,
124.561235915968)) ;
#54819=CARTESIAN_POINT('Ctrl Pts',(-19.865197731046,-36.3671092788047,124.848586979742)) ;
#54820=CARTESIAN_POINT('Ctrl Pts',(-19.9675160561407,-36.5570641027758,
124.48092624152)) ;
#54821=CARTESIAN_POINT('Ctrl Pts',(-20.1070919689581,-36.3770750222953,
124.748197482169)) ;
#54822=CARTESIAN_POINT('Ctrl Pts',(-20.1450804636381,-36.567092481907,124.36727939808)) ;
#54823=CARTESIAN_POINT('Ctrl Pts',(-20.3290461477536,-36.3871034014265,
124.606136879455)) ;
#54824=CARTESIAN_POINT('Ctrl Pts',(-20.2984821281396,-36.5769933281139,
124.226551618622)) ;
#54825=CARTESIAN_POINT('Ctrl Pts',(-20.5207969132898,-36.3970042476334,
124.430224963502)) ;
#54826=CARTESIAN_POINT('Ctrl Pts',(-20.4270554223315,-36.587051985531,124.058705204649)) ;
#54827=CARTESIAN_POINT('Ctrl Pts',(-20.6815114755978,-36.4070629050505,
124.220415524701)) ;
#54828=CARTESIAN_POINT('Ctrl Pts',(-20.5228088976676,-36.5969095483129,
123.874874545121)) ;
#54829=CARTESIAN_POINT('Ctrl Pts',(-20.8012013745424,-36.4169204678324,
123.990625446884)) ;
#54830=CARTESIAN_POINT('Ctrl Pts',(-20.5866346710282,-36.6069779508661,
123.673090041248)) ;
#54831=CARTESIAN_POINT('Ctrl Pts',(-20.8809810996104,-36.4269888703856,
123.738394192425)) ;
#54832=CARTESIAN_POINT('Ctrl Pts',(-20.6138518765132,-36.6168333496057,
123.46767623189)) ;
#54833=CARTESIAN_POINT('Ctrl Pts',(-20.9150001539312,-36.4368442691252,
123.481625971237)) ;
#54834=CARTESIAN_POINT('Ctrl Pts',(-20.6054955842666,-36.6268282166796,
123.257725834414)) ;
#54835=CARTESIAN_POINT('Ctrl Pts',(-20.9045521216092,-36.4468391361991,
123.219187981006)) ;
#54836=CARTESIAN_POINT('Ctrl Pts',(-20.5602021180779,-36.636859511663,123.051753465069)) ;
#54837=CARTESIAN_POINT('Ctrl Pts',(-20.8479327598171,-36.4568704311826,
122.961723074827)) ;
#54838=CARTESIAN_POINT('Ctrl Pts',(-20.4814585623447,-36.6467260363896,
122.859848018416)) ;
#54839=CARTESIAN_POINT('Ctrl Pts',(-20.7495006732723,-36.4667369559091,
122.721841788976)) ;
#54840=CARTESIAN_POINT('Ctrl Pts',(-20.3695334272533,-36.6567135070853,
122.682228468216)) ;
#54841=CARTESIAN_POINT('Ctrl Pts',(-20.6095919098438,-36.4767244266048,
122.499818683147)) ;
#54842=CARTESIAN_POINT('Ctrl Pts',(-20.2291188401914,-36.6666582666492,
122.527284926112)) ;
#54843=CARTESIAN_POINT('Ctrl Pts',(-20.4340715147881,-36.4866691861687,
122.306140896001)) ;
#54844=CARTESIAN_POINT('Ctrl Pts',(-20.0622231051933,-36.676703822598,122.397914061097)) ;
#54845=CARTESIAN_POINT('Ctrl Pts',(-20.2254502143185,-36.4967147421175,
122.14442945412)) ;
#54846=CARTESIAN_POINT('Ctrl Pts',(-19.8789187763763,-36.6865634109731,
122.301092451122)) ;
#54847=CARTESIAN_POINT('Ctrl Pts',(-19.9963181528089,-36.5065743304926,
122.023404638847)) ;
#54848=CARTESIAN_POINT('Ctrl Pts',(-19.6789119610615,-36.6965643661092,
122.23637511333)) ;
#54849=CARTESIAN_POINT('Ctrl Pts',(-19.7463087038037,-36.5165752856287,
121.94251056244)) ;
#54850=CARTESIAN_POINT('Ctrl Pts',(-19.4726764661033,-36.7064685933867,
122.207479051172)) ;
#54851=CARTESIAN_POINT('Ctrl Pts',(-19.4885136890364,-36.5264795129063,
121.906393184978)) ;
#54852=CARTESIAN_POINT('Ctrl Pts',(-19.2617182497028,-36.7165106702819,
122.214872705184)) ;
#54853=CARTESIAN_POINT('Ctrl Pts',(-19.2248160076973,-36.5365215898014,
121.915638023178)) ;
#54854=CARTESIAN_POINT('Ctrl Pts',(-19.057927154021,-36.726418282968,122.2581086562)) ;
#54855=CARTESIAN_POINT('Ctrl Pts',(-18.970077488326,-36.5464292024876,121.96968572627)) ;
#54856=CARTESIAN_POINT('Ctrl Pts',(-18.8619321432003,-36.7364728135838,
122.337188886544)) ;
#54857=CARTESIAN_POINT('Ctrl Pts',(-18.7250847626907,-36.5564837331033,
122.068538595293)) ;
#54858=CARTESIAN_POINT('Ctrl Pts',(-18.6859875564324,-36.7463336001326,
122.446869658722)) ;
#54859=CARTESIAN_POINT('Ctrl Pts',(-18.5051552711901,-36.5663445196522,
122.205642070878)) ;
#54860=CARTESIAN_POINT('Ctrl Pts',(-18.5294655824155,-36.7563273552037,
122.586972488339)) ;
#54861=CARTESIAN_POINT('Ctrl Pts',(-18.3095046248543,-36.5763382747232,
122.380772756603)) ;
#54862=CARTESIAN_POINT('Ctrl Pts',(-18.4004150751371,-36.7662527154437,
122.750983302961)) ;
#54863=CARTESIAN_POINT('Ctrl Pts',(-18.1481936175837,-36.5862636349632,
122.585788118816)) ;
#54864=CARTESIAN_POINT('Ctrl Pts',(-18.3008055717462,-36.776280644839,122.936753966816)) ;
#54865=CARTESIAN_POINT('Ctrl Pts',(-18.0236841920842,-36.5962915643585,
122.818002834803)) ;
#54866=CARTESIAN_POINT('Ctrl Pts',(-18.2356726374387,-36.7861669116383,
123.134158053417)) ;
#54867=CARTESIAN_POINT('Ctrl Pts',(-17.9422706634272,-36.6061778311578,
123.0647589423)) ;
#54868=CARTESIAN_POINT('Ctrl Pts',(-18.2052669474954,-36.7961986805365,
123.342818627154)) ;
#54869=CARTESIAN_POINT('Ctrl Pts',(-17.904266334052,-36.6162096000561,123.32558512975)) ;
#54870=CARTESIAN_POINT('Ctrl Pts',(-18.2112586660847,-36.8060802763801,
123.550511838692)) ;
#54871=CARTESIAN_POINT('Ctrl Pts',(-17.911758818048,-36.6260911958997,123.585201643674)) ;
#54872=CARTESIAN_POINT('Ctrl Pts',(-18.2539211094933,-36.8161421618481,
123.757665242363)) ;
#54873=CARTESIAN_POINT('Ctrl Pts',(-17.9650896018875,-36.6361530813676,
123.844142860301)) ;
#54874=CARTESIAN_POINT('Ctrl Pts',(-18.3302768913769,-36.825999595867,123.950348541592)) ;
#54875=CARTESIAN_POINT('Ctrl Pts',(-18.0605371632043,-36.6460105153865,
124.08499614466)) ;
#54876=CARTESIAN_POINT('Ctrl Pts',(-18.4400202960657,-36.8359928389089,
124.129465514795)) ;
#54877=CARTESIAN_POINT('Ctrl Pts',(-18.1977180727596,-36.6560037584285,
124.308890236718)) ;
#54878=CARTESIAN_POINT('Ctrl Pts',(-18.5783392874067,-36.8459235997953,
124.285860530243)) ;
#54879=CARTESIAN_POINT('Ctrl Pts',(-18.370621788701,-36.6659345193148,124.504384734835)) ;
#54880=CARTESIAN_POINT('Ctrl Pts',(-18.7977945098984,-36.8592725919925,
124.460845444457)) ;
#54881=CARTESIAN_POINT('Ctrl Pts',(-18.644928888487,-36.679283511512,124.723100111771)) ;
#54882=CARTESIAN_POINT('Ctrl Pts',(-19.0564575910086,-36.8725409648089,
124.573487171901)) ;
#54883=CARTESIAN_POINT('Ctrl Pts',(-18.968224608499,-36.6925518843284,124.863897618204)) ;
#54884=CARTESIAN_POINT('Ctrl Pts',(-19.332518152077,-36.8858239061933,124.615432948066)) ;
#54885=CARTESIAN_POINT('Ctrl Pts',(-19.3133563776391,-36.7058348257128,
124.9163404754)) ;
#54886=CARTESIAN_POINT('Ctrl Pts',(-19.5435804177348,-36.8958666920355,
124.610274690913)) ;
#54887=CARTESIAN_POINT('Ctrl Pts',(-19.5771730601829,-36.715877611555,124.909887095996)) ;
#54888=CARTESIAN_POINT('Ctrl Pts',(-19.7466220723449,-36.9057166345876,
124.569566521813)) ;
#54889=CARTESIAN_POINT('Ctrl Pts',(-19.8309776236468,-36.7257275541071,
124.858999538759)) ;
#54890=CARTESIAN_POINT('Ctrl Pts',(-19.9425753325179,-36.9157138675065,
124.493590570334)) ;
#54891=CARTESIAN_POINT('Ctrl Pts',(-20.075916339916,-36.7357247870261,124.764028514529)) ;
#54892=CARTESIAN_POINT('Ctrl Pts',(-20.1225212109622,-36.9257287628411,
124.384267908977)) ;
#54893=CARTESIAN_POINT('Ctrl Pts',(-20.3008516833001,-36.7457396823606,
124.627366616368)) ;
#54894=CARTESIAN_POINT('Ctrl Pts',(-20.3318880894533,-36.9389684394793,
124.200821795761)) ;
#54895=CARTESIAN_POINT('Ctrl Pts',(-20.562537162733,-36.7589793589988,124.398087289578)) ;
#54896=CARTESIAN_POINT('Ctrl Pts',(-20.528163224449,-36.9555156638846,123.9088995619)) ;
#54897=CARTESIAN_POINT('Ctrl Pts',(-20.8079029755518,-36.7755265834041,
124.033128787437)) ;
#54898=CARTESIAN_POINT('Ctrl Pts',(-20.6137528393046,-36.9721631010157,
123.56536786537)) ;
#54899=CARTESIAN_POINT('Ctrl Pts',(-20.9148689310472,-36.7921740205352,
123.603796766495)) ;
#54900=CARTESIAN_POINT('Ctrl Pts',(-20.6085683059766,-36.9854525984939,
123.286061986322)) ;
#54901=CARTESIAN_POINT('Ctrl Pts',(-20.9083945689062,-36.8054635180134,
123.254597757702)) ;
#54902=CARTESIAN_POINT('Ctrl Pts',(-20.5693560188396,-36.9953260063163,
123.082217819628)) ;
#54903=CARTESIAN_POINT('Ctrl Pts',(-20.859374951537,-36.8153369258358,122.999807024166)) ;
#54904=CARTESIAN_POINT('Ctrl Pts',(-20.4940428412356,-37.005378383909,122.884773388024)) ;
#54905=CARTESIAN_POINT('Ctrl Pts',(-20.7652312034385,-36.8253893034285,
122.752998369453)) ;
#54906=CARTESIAN_POINT('Ctrl Pts',(-20.3871047058436,-37.0152820374499,
122.706108282335)) ;
#54907=CARTESIAN_POINT('Ctrl Pts',(-20.631557772952,-36.8352929569694,122.529670136068)) ;
#54908=CARTESIAN_POINT('Ctrl Pts',(-20.2506236096731,-37.0252263064452,
122.547784485508)) ;
#54909=CARTESIAN_POINT('Ctrl Pts',(-20.4609498468853,-36.8452372259647,
122.331765024377)) ;
#54910=CARTESIAN_POINT('Ctrl Pts',(-20.0335787700198,-37.0385573147779,
122.37035520076)) ;
#54911=CARTESIAN_POINT('Ctrl Pts',(-20.1896663856543,-36.8585682342974,
122.109990345153)) ;
#54912=CARTESIAN_POINT('Ctrl Pts',(-19.7113303634737,-37.0551788953021,
122.225449965275)) ;
#54913=CARTESIAN_POINT('Ctrl Pts',(-19.7868089892428,-36.8751898148217,
121.928852787529)) ;
#54914=CARTESIAN_POINT('Ctrl Pts',(-19.3605381967804,-37.0717215660005,
122.198625173765)) ;
#54915=CARTESIAN_POINT('Ctrl Pts',(-19.3483970122116,-36.8917324855201,
121.895325330495)) ;
#54916=CARTESIAN_POINT('Ctrl Pts',(-19.084756283337,-37.0850707255635,122.250326858334)) ;
#54917=CARTESIAN_POINT('Ctrl Pts',(-19.0036058958539,-36.905081645083,121.959959179047)) ;
#54918=CARTESIAN_POINT('Ctrl Pts',(-18.8243006026364,-37.098298875723,122.34794994263)) ;
#54919=CARTESIAN_POINT('Ctrl Pts',(-18.6780618919625,-36.9183097952425,
122.081981866891)) ;
#54920=CARTESIAN_POINT('Ctrl Pts',(-18.5364100435384,-37.1149295528605,
122.553165444984)) ;
#54921=CARTESIAN_POINT('Ctrl Pts',(-18.3181836589945,-36.93494047238,122.338513488411)) ;
#54922=CARTESIAN_POINT('Ctrl Pts',(-18.2963005996991,-37.1348324921486,
122.901714167161)) ;
#54923=CARTESIAN_POINT('Ctrl Pts',(-18.0180562106174,-36.9548434116681,
122.774198058381)) ;
#54924=CARTESIAN_POINT('Ctrl Pts',(-18.1891582578052,-37.1547353587518,
123.311031502207)) ;
#54925=CARTESIAN_POINT('Ctrl Pts',(-17.8841306986637,-36.9747462782714,
123.285845641878)) ;
#54926=CARTESIAN_POINT('Ctrl Pts',(-18.2275156867731,-37.1746485238567,
123.732793359214)) ;
#54927=CARTESIAN_POINT('Ctrl Pts',(-17.9320811339268,-36.9946594433762,
123.813046654379)) ;
#54928=CARTESIAN_POINT('Ctrl Pts',(-18.409140585469,-37.194684352998,124.118086353196)) ;
#54929=CARTESIAN_POINT('Ctrl Pts',(-18.1591155084676,-37.0146952725175,
124.294661831233)) ;
#54930=CARTESIAN_POINT('Ctrl Pts',(-18.7080016710259,-37.2145029278761,
124.41531311931)) ;
#54931=CARTESIAN_POINT('Ctrl Pts',(-18.5326928559691,-37.0345138473956,
124.666191700612)) ;
#54932=CARTESIAN_POINT('Ctrl Pts',(-19.0927718739483,-37.2344732289181,
124.594578380774)) ;
#54933=CARTESIAN_POINT('Ctrl Pts',(-19.0136563926728,-37.0544841484376,
124.890270640094)) ;
#54934=CARTESIAN_POINT('Ctrl Pts',(-19.5142339391822,-37.2543647612826,
124.631795562197)) ;
#54935=CARTESIAN_POINT('Ctrl Pts',(-19.5404829664687,-37.0743756808021,
124.936789595379)) ;
#54936=CARTESIAN_POINT('Ctrl Pts',(-19.9254766838517,-37.2743878590991,
124.521993821233)) ;
#54937=CARTESIAN_POINT('Ctrl Pts',(-20.0545360586969,-37.0943987786187,
124.799534983249)) ;
#54938=CARTESIAN_POINT('Ctrl Pts',(-20.2709110278147,-37.2941846120191,
124.281362408259)) ;
#54939=CARTESIAN_POINT('Ctrl Pts',(-20.486325645581,-37.1141955315386,124.498745537958)) ;
#54940=CARTESIAN_POINT('Ctrl Pts',(-20.5163858033962,-37.3141457005079,
123.935170853578)) ;
#54941=CARTESIAN_POINT('Ctrl Pts',(-20.7931678601018,-37.1341566200274,
124.066005974711)) ;
#54942=CARTESIAN_POINT('Ctrl Pts',(-20.6282493094601,-37.33412396944,123.52533621411)) ;
#54943=CARTESIAN_POINT('Ctrl Pts',(-20.9329957736471,-37.1541348889596,
123.55371250196)) ;
#54944=CARTESIAN_POINT('Ctrl Pts',(-20.5944348756213,-37.353943984231,123.105306555051)) ;
#54945=CARTESIAN_POINT('Ctrl Pts',(-20.8907271347711,-37.1739549037506,
123.028678283187)) ;
#54946=CARTESIAN_POINT('Ctrl Pts',(-20.419241626978,-37.3738823934829,122.719230553153)) ;
#54947=CARTESIAN_POINT('Ctrl Pts',(-20.671736248065,-37.1938933130024,122.546084069823)) ;
#54948=CARTESIAN_POINT('Ctrl Pts',(-20.1204934119422,-37.3939295108753,
122.415110115247)) ;
#54949=CARTESIAN_POINT('Ctrl Pts',(-20.2983002158632,-37.2139404303948,
122.165933042712)) ;
#54950=CARTESIAN_POINT('Ctrl Pts',(-19.7397550775313,-37.4137757567091,
122.233254243053)) ;
#54951=CARTESIAN_POINT('Ctrl Pts',(-19.8223796113468,-37.2337866762287,
121.938614397034)) ;
#54952=CARTESIAN_POINT('Ctrl Pts',(-19.3198536517042,-37.4336247252212,
122.19057464082)) ;
#54953=CARTESIAN_POINT('Ctrl Pts',(-19.2975051439702,-37.2536356447407,
121.885263707439)) ;
#54954=CARTESIAN_POINT('Ctrl Pts',(-18.9066386247496,-37.4536750275325,
122.295305344993)) ;
#54955=CARTESIAN_POINT('Ctrl Pts',(-18.7809853426372,-37.273685947052,122.016176078688)) ;
#54956=CARTESIAN_POINT('Ctrl Pts',(-18.5576843444494,-37.4735099499637,
122.53234187102)) ;
#54957=CARTESIAN_POINT('Ctrl Pts',(-18.3447935794492,-37.2935208694832,
122.312469305178)) ;
#54958=CARTESIAN_POINT('Ctrl Pts',(-18.3088629623989,-37.4934403511896,
122.87517401801)) ;
#54959=CARTESIAN_POINT('Ctrl Pts',(-18.0337656487318,-37.3134512707091,
122.741007439653)) ;
#54960=CARTESIAN_POINT('Ctrl Pts',(-18.191627159294,-37.5133252965484,123.281572566289)) ;
#54961=CARTESIAN_POINT('Ctrl Pts',(-17.8872187176123,-37.333336216068,123.249003693787)) ;
#54962=CARTESIAN_POINT('Ctrl Pts',(-18.2210576117943,-37.5333979046998,
123.707273120117)) ;
#54963=CARTESIAN_POINT('Ctrl Pts',(-17.9240043989102,-37.3534088242194,
123.781130410559)) ;
#54964=CARTESIAN_POINT('Ctrl Pts',(-18.3915612941918,-37.5531892210279,
124.092070927854)) ;
#54965=CARTESIAN_POINT('Ctrl Pts',(-18.1371306276255,-37.3732001405475,
124.26212661135)) ;
#54966=CARTESIAN_POINT('Ctrl Pts',(-18.6846818237289,-37.5731540107952,
124.399080855856)) ;
#54967=CARTESIAN_POINT('Ctrl Pts',(-18.5035285317614,-37.3931649303147,
124.645891221395)) ;
#54968=CARTESIAN_POINT('Ctrl Pts',(-19.0658286606464,-37.5931369665455,
124.5868719561)) ;
#54969=CARTESIAN_POINT('Ctrl Pts',(-18.9799605391269,-37.413147886065,124.880632850392)) ;
#54970=CARTESIAN_POINT('Ctrl Pts',(-19.4844281526955,-37.6129454885216,
124.633785399383)) ;
#54971=CARTESIAN_POINT('Ctrl Pts',(-19.5032077670289,-37.4329564080412,
124.93927814101)) ;
#54972=CARTESIAN_POINT('Ctrl Pts',(-19.8975569980139,-37.6329310632575,
124.534652953361)) ;
#54973=CARTESIAN_POINT('Ctrl Pts',(-20.0196196743676,-37.452941982777,124.815366561409)) ;
#54974=CARTESIAN_POINT('Ctrl Pts',(-20.2503434108889,-37.6528137033259,
124.301519197252)) ;
#54975=CARTESIAN_POINT('Ctrl Pts',(-20.4606042548216,-37.4728246228454,
124.523953284012)) ;
#54976=CARTESIAN_POINT('Ctrl Pts',(-20.503477443757,-37.6727690154578,123.96110057976)) ;
#54977=CARTESIAN_POINT('Ctrl Pts',(-20.7770251298979,-37.4927799349773,
124.098432868024)) ;
#54978=CARTESIAN_POINT('Ctrl Pts',(-20.6250594607957,-37.6926433720656,
123.556310778876)) ;
#54979=CARTESIAN_POINT('Ctrl Pts',(-20.9290068710013,-37.5126542915851,
123.592447664167)) ;
#54980=CARTESIAN_POINT('Ctrl Pts',(-20.60136228044,-37.7126255789266,123.132144136794)) ;
#54981=CARTESIAN_POINT('Ctrl Pts',(-20.8993899563802,-37.5326364984462,
123.062239130168)) ;
#54982=CARTESIAN_POINT('Ctrl Pts',(-20.4345064783654,-37.7325566568766,
122.742488170039)) ;
#54983=CARTESIAN_POINT('Ctrl Pts',(-20.6908254812165,-37.5525675763961,
122.575167631135)) ;
#54984=CARTESIAN_POINT('Ctrl Pts',(-20.1449218342173,-37.7524836317316,
122.433312486334)) ;
#54985=CARTESIAN_POINT('Ctrl Pts',(-20.3288457046536,-37.5724945512511,
122.188694790746)) ;
#54986=CARTESIAN_POINT('Ctrl Pts',(-19.769249258697,-37.7723160906805,122.241620195832)) ;
#54987=CARTESIAN_POINT('Ctrl Pts',(-19.8592684234008,-37.5923270102,121.949075641498)) ;
#54988=CARTESIAN_POINT('Ctrl Pts',(-19.417912839103,-37.7889737748557,122.197692406398)) ;
#54989=CARTESIAN_POINT('Ctrl Pts',(-19.4200658004677,-37.6089846943752,
121.894159881011)) ;
#54990=CARTESIAN_POINT('Ctrl Pts',(-19.1419000183344,-37.8022229987628,
122.235811998342)) ;
#54991=CARTESIAN_POINT('Ctrl Pts',(-19.0750788995196,-37.6222339182823,
121.941806794184)) ;
#54992=CARTESIAN_POINT('Ctrl Pts',(-18.9408249504578,-37.812272020214,122.300516733024)) ;
#54993=CARTESIAN_POINT('Ctrl Pts',(-18.8237258576414,-37.6322829397335,
122.022687580553)) ;
#54994=CARTESIAN_POINT('Ctrl Pts',(-18.75748940626,-37.8221320284445,122.39727315745)) ;
#54995=CARTESIAN_POINT('Ctrl Pts',(-18.5945663207733,-37.642142947964,122.143620576973)) ;
#54996=CARTESIAN_POINT('Ctrl Pts',(-18.5363454819024,-37.8354155416691,
122.567770253279)) ;
#54997=CARTESIAN_POINT('Ctrl Pts',(-18.3180876792533,-37.6554264611886,
122.356789242031)) ;
#54998=CARTESIAN_POINT('Ctrl Pts',(-18.3218393831635,-37.8520614606699,
122.849331128677)) ;
#54999=CARTESIAN_POINT('Ctrl Pts',(-18.0500066417951,-37.6720723801894,
122.708670183336)) ;
#55000=CARTESIAN_POINT('Ctrl Pts',(-18.2164325706239,-37.868615438486,123.185138476082)) ;
#55001=CARTESIAN_POINT('Ctrl Pts',(-17.9182173114303,-37.6886263580055,
123.128486091663)) ;
#55002=CARTESIAN_POINT('Ctrl Pts',(-18.2044905733032,-37.8819751674576,
123.465776368873)) ;
#55003=CARTESIAN_POINT('Ctrl Pts',(-17.9032980829134,-37.7019860869771,
123.479244069044)) ;
#55004=CARTESIAN_POINT('Ctrl Pts',(-18.2317111895261,-37.8918682192543,
123.671978883509)) ;
#55005=CARTESIAN_POINT('Ctrl Pts',(-17.9373186785882,-37.7118791387738,
123.73700538151)) ;
#55006=CARTESIAN_POINT('Ctrl Pts',(-18.294652658177,-37.9018581845353,123.87232240774)) ;
#55007=CARTESIAN_POINT('Ctrl Pts',(-18.0159935015514,-37.7218691040548,
123.98743356225)) ;
#55008=CARTESIAN_POINT('Ctrl Pts',(-18.3909713233348,-37.9118100653962,
124.058088930702)) ;
#55009=CARTESIAN_POINT('Ctrl Pts',(-18.1363891803224,-37.7318209849157,
124.219643590577)) ;
#55010=CARTESIAN_POINT('Ctrl Pts',(-18.5194225453027,-37.921858417088,124.225768775159)) ;
#55011=CARTESIAN_POINT('Ctrl Pts',(-18.2969510923513,-37.7418693366075,
124.429245026213)) ;
#55012=CARTESIAN_POINT('Ctrl Pts',(-18.671696215703,-37.9316997011942,124.365864629888)) ;
#55013=CARTESIAN_POINT('Ctrl Pts',(-18.4872912315041,-37.7517106207137,
124.604366917906)) ;
#55014=CARTESIAN_POINT('Ctrl Pts',(-18.8482704727161,-37.9416864043198,
124.479380726251)) ;
#55015=CARTESIAN_POINT('Ctrl Pts',(-18.7080075971483,-37.7616973238393,
124.746264446641)) ;
#55016=CARTESIAN_POINT('Ctrl Pts',(-19.0408922738897,-37.9516214331373,
124.560242685434)) ;
#55017=CARTESIAN_POINT('Ctrl Pts',(-18.9487838243204,-37.7716323526568,
124.847344520191)) ;
#55018=CARTESIAN_POINT('Ctrl Pts',(-19.2470723983466,-37.9616772280442,
124.606804319472)) ;
#55019=CARTESIAN_POINT('Ctrl Pts',(-19.2065084133188,-37.7816881475637,
124.905549326719)) ;
#55020=CARTESIAN_POINT('Ctrl Pts',(-19.4534751390395,-37.9715055913335,
124.616954335681)) ;
#55021=CARTESIAN_POINT('Ctrl Pts',(-19.4645118314084,-37.791516510853,124.918239663779)) ;
#55022=CARTESIAN_POINT('Ctrl Pts',(-19.6633369830596,-37.9815665612314,
124.590805337205)) ;
#55023=CARTESIAN_POINT('Ctrl Pts',(-19.7268395349179,-37.8015774807509,
124.88555619889)) ;
#55024=CARTESIAN_POINT('Ctrl Pts',(-19.8625213753835,-37.9914808401212,
124.529341700821)) ;
#55025=CARTESIAN_POINT('Ctrl Pts',(-19.9758209773631,-37.8114917596407,
124.808729302438)) ;
#55026=CARTESIAN_POINT('Ctrl Pts',(-20.0499508132267,-38.0014898345894,
124.433695820454)) ;
#55027=CARTESIAN_POINT('Ctrl Pts',(-20.2101091149585,-37.821500754109,124.689174409478)) ;
#55028=CARTESIAN_POINT('Ctrl Pts',(-20.2180109913369,-38.0115196691532,
124.306354445413)) ;
#55029=CARTESIAN_POINT('Ctrl Pts',(-20.4201860706059,-37.8315305886727,
124.52999991223)) ;
#55030=CARTESIAN_POINT('Ctrl Pts',(-20.3592543198836,-38.0213778992254,
124.154667140303)) ;
#55031=CARTESIAN_POINT('Ctrl Pts',(-20.5967424361881,-37.8413888187449,
124.340392519034)) ;
#55032=CARTESIAN_POINT('Ctrl Pts',(-20.4738072405077,-38.0313766049678,
123.978459990424)) ;
#55033=CARTESIAN_POINT('Ctrl Pts',(-20.7399359739768,-37.8513875244874,
124.120135025815)) ;
#55034=CARTESIAN_POINT('Ctrl Pts',(-20.5554252299828,-38.0412712608866,
123.787082603069)) ;
#55035=CARTESIAN_POINT('Ctrl Pts',(-20.8419611025368,-37.8612821804061,
123.880914136025)) ;
#55036=CARTESIAN_POINT('Ctrl Pts',(-20.6032952967785,-38.0513343252705,
123.581049295425)) ;
#55037=CARTESIAN_POINT('Ctrl Pts',(-20.9018013800927,-37.8713452447901,
123.623373162088)) ;
#55038=CARTESIAN_POINT('Ctrl Pts',(-20.6146442268699,-38.0611739835504,
123.374466194036)) ;
#55039=CARTESIAN_POINT('Ctrl Pts',(-20.9159903079656,-37.88118490307,123.365144028709)) ;
#55040=CARTESIAN_POINT('Ctrl Pts',(-20.5896648476914,-38.0712371506323,
123.164415788226)) ;
#55041=CARTESIAN_POINT('Ctrl Pts',(-20.8847687944641,-37.8912480701518,
123.102580743013)) ;
#55042=CARTESIAN_POINT('Ctrl Pts',(-20.5294350178213,-38.0811313957594,
122.965294396189)) ;
#55043=CARTESIAN_POINT('Ctrl Pts',(-20.809484036309,-37.9011423152789,122.853677895815)) ;
#55044=CARTESIAN_POINT('Ctrl Pts',(-20.4356240821456,-38.091073217364,122.778550856413)) ;
#55045=CARTESIAN_POINT('Ctrl Pts',(-20.6922226403838,-37.9110841368836,
122.620247034485)) ;
#55046=CARTESIAN_POINT('Ctrl Pts',(-20.3100810134852,-38.1010757482821,
122.609819097008)) ;
#55047=CARTESIAN_POINT('Ctrl Pts',(-20.5352958892359,-37.9210866678016,
122.409330679749)) ;
#55048=CARTESIAN_POINT('Ctrl Pts',(-20.1564607952852,-38.1111103747396,
122.465250449914)) ;
#55049=CARTESIAN_POINT('Ctrl Pts',(-20.3432724836737,-37.9311212942591,
122.228617908564)) ;
#55050=CARTESIAN_POINT('Ctrl Pts',(-19.9835623722376,-38.120955909726,122.351445881566)) ;
#55051=CARTESIAN_POINT('Ctrl Pts',(-20.1271504516508,-37.9409668292455,
122.086359667513)) ;
#55052=CARTESIAN_POINT('Ctrl Pts',(-19.7910718790852,-38.130939334565,122.267833463766)) ;
#55053=CARTESIAN_POINT('Ctrl Pts',(-19.8865382084565,-37.9509502540846,
121.981841696221)) ;
#55054=CARTESIAN_POINT('Ctrl Pts',(-19.5876306579575,-38.1408897249301,
122.219111287809)) ;
#55055=CARTESIAN_POINT('Ctrl Pts',(-19.6322370248883,-37.9609006444496,
121.920936388754)) ;
#55056=CARTESIAN_POINT('Ctrl Pts',(-19.377833549305,-38.1508873652272,122.206109169437)) ;
#55057=CARTESIAN_POINT('Ctrl Pts',(-19.3699906918026,-37.9708982847467,
121.90468118913)) ;
#55058=CARTESIAN_POINT('Ctrl Pts',(-19.1681777198956,-38.1609264457904,
122.230248686122)) ;
#55059=CARTESIAN_POINT('Ctrl Pts',(-19.1079206635879,-37.9809373653099,
121.93485297098)) ;
#55060=CARTESIAN_POINT('Ctrl Pts',(-18.9700348987054,-38.1707525965595,
122.288711476729)) ;
#55061=CARTESIAN_POINT('Ctrl Pts',(-18.8602406825813,-37.990763516079,122.007929238397)) ;
#55062=CARTESIAN_POINT('Ctrl Pts',(-18.7805861370791,-38.1808091714886,
122.382535043644)) ;
#55063=CARTESIAN_POINT('Ctrl Pts',(-18.623428724634,-38.0008200910081,122.125206427379)) ;
#55064=CARTESIAN_POINT('Ctrl Pts',(-18.6124721251259,-38.1907497108689,
122.506687338433)) ;
#55065=CARTESIAN_POINT('Ctrl Pts',(-18.4132844277735,-38.0107606303884,
122.280394942129)) ;
#55066=CARTESIAN_POINT('Ctrl Pts',(-18.4685228176919,-38.2006541038453,
122.657141441856)) ;
#55067=CARTESIAN_POINT('Ctrl Pts',(-18.2333456789751,-38.0206650233648,
122.468461282775)) ;
#55068=CARTESIAN_POINT('Ctrl Pts',(-18.3513466171436,-38.2107007580502,
122.832848241972)) ;
#55069=CARTESIAN_POINT('Ctrl Pts',(-18.0868734494844,-38.0307116775697,
122.688093340376)) ;
#55070=CARTESIAN_POINT('Ctrl Pts',(-18.2675409912502,-38.2205963199886,
123.023293670157)) ;
#55071=CARTESIAN_POINT('Ctrl Pts',(-17.9821139833367,-38.0406072395081,
122.92614968841)) ;
#55072=CARTESIAN_POINT('Ctrl Pts',(-18.2172590198728,-38.2306583978341,
123.228736388666)) ;
#55073=CARTESIAN_POINT('Ctrl Pts',(-17.9192592234014,-38.0506693173537,
123.182952338468)) ;
#55074=CARTESIAN_POINT('Ctrl Pts',(-18.203592355486,-38.2405010962479,123.435232302293)) ;
#55075=CARTESIAN_POINT('Ctrl Pts',(-17.9021734626821,-38.0605120157674,
123.44107293395)) ;
#55076=CARTESIAN_POINT('Ctrl Pts',(-18.2258256609928,-38.2504918712094,
123.644062640654)) ;
#55077=CARTESIAN_POINT('Ctrl Pts',(-17.9299628605626,-38.0705027907289,
123.702111270624)) ;
#55078=CARTESIAN_POINT('Ctrl Pts',(-18.2836555871143,-38.2604197362285,
123.844617912795)) ;
#55079=CARTESIAN_POINT('Ctrl Pts',(-18.0022482228255,-38.080430655748,123.95280645731)) ;
#55080=CARTESIAN_POINT('Ctrl Pts',(-18.3756740561465,-38.2704084809947,
124.033382785649)) ;
#55081=CARTESIAN_POINT('Ctrl Pts',(-18.1172694268296,-38.0904194005142,
124.188763665589)) ;
#55082=CARTESIAN_POINT('Ctrl Pts',(-18.4998651142318,-38.2804412665816,
124.203869104548)) ;
#55083=CARTESIAN_POINT('Ctrl Pts',(-18.2725063778356,-38.1004521861012,
124.401872837014)) ;
#55084=CARTESIAN_POINT('Ctrl Pts',(-18.649102754769,-38.2903079512023,124.347923475099)) ;
#55085=CARTESIAN_POINT('Ctrl Pts',(-18.459052515942,-38.1103188707218,124.581942987267)) ;
#55086=CARTESIAN_POINT('Ctrl Pts',(-18.8224168744023,-38.3002698433654,
124.465501995061)) ;
#55087=CARTESIAN_POINT('Ctrl Pts',(-18.675694305883,-38.1202807628849,124.728918023426)) ;
#55088=CARTESIAN_POINT('Ctrl Pts',(-19.0150124373623,-38.310303320278,124.551507630539)) ;
#55089=CARTESIAN_POINT('Ctrl Pts',(-18.9164378070298,-38.1303142397975,
124.836426983445)) ;
#55090=CARTESIAN_POINT('Ctrl Pts',(-19.2165276853303,-38.3201876615263,
124.602331746933)) ;
#55091=CARTESIAN_POINT('Ctrl Pts',(-19.1683321359432,-38.1401985810458,
124.899959302576)) ;
#55092=CARTESIAN_POINT('Ctrl Pts',(-19.4274995678866,-38.3302506036474,
124.617665373522)) ;
#55093=CARTESIAN_POINT('Ctrl Pts',(-19.4320465863477,-38.1502615231669,
124.919128358912)) ;
#55094=CARTESIAN_POINT('Ctrl Pts',(-19.6335365424027,-38.340101005267,124.596684953135)) ;
#55095=CARTESIAN_POINT('Ctrl Pts',(-19.68959404648,-38.1601119247865,124.892904734161)) ;
#55096=CARTESIAN_POINT('Ctrl Pts',(-19.8364952866382,-38.3501278940566,
124.539756466439)) ;
#55097=CARTESIAN_POINT('Ctrl Pts',(-19.9432929414861,-38.1701388135762,
124.82174592566)) ;
#55098=CARTESIAN_POINT('Ctrl Pts',(-20.0262936192823,-38.3601565090128,
124.447932183891)) ;
#55099=CARTESIAN_POINT('Ctrl Pts',(-20.1805416770714,-38.1801674285324,
124.706967424804)) ;
#55100=CARTESIAN_POINT('Ctrl Pts',(-20.1943496803359,-38.3700017321329,
124.327134832878)) ;
#55101=CARTESIAN_POINT('Ctrl Pts',(-20.3906137722075,-38.1900126516524,
124.555971632354)) ;
#55102=CARTESIAN_POINT('Ctrl Pts',(-20.3414292534082,-38.3799924159389,
124.17718516851)) ;
#55103=CARTESIAN_POINT('Ctrl Pts',(-20.5744646118342,-38.2000033354584,
124.368535624798)) ;
#55104=CARTESIAN_POINT('Ctrl Pts',(-20.4604073331127,-38.3900302980113,
124.002897673385)) ;
#55105=CARTESIAN_POINT('Ctrl Pts',(-20.7231886885052,-38.2100412175308,
124.150677424897)) ;
#55106=CARTESIAN_POINT('Ctrl Pts',(-20.5459739903831,-38.3998746576501,
123.814446734929)) ;
#55107=CARTESIAN_POINT('Ctrl Pts',(-20.8301490998756,-38.2198855771697,
123.915113415529)) ;
#55108=CARTESIAN_POINT('Ctrl Pts',(-20.5986469705977,-38.4098595282649,
123.611278948678)) ;
#55109=CARTESIAN_POINT('Ctrl Pts',(-20.8959919670517,-38.2298704477844,
123.661153850846)) ;
#55110=CARTESIAN_POINT('Ctrl Pts',(-20.6152674854277,-38.4197988115935,
123.402955218507)) ;
#55111=CARTESIAN_POINT('Ctrl Pts',(-20.9167692458508,-38.2398097311131,
123.400748772404)) ;
#55112=CARTESIAN_POINT('Ctrl Pts',(-20.5952009161257,-38.4298394209667,
123.192847662507)) ;
#55113=CARTESIAN_POINT('Ctrl Pts',(-20.8916876627849,-38.2498503404862,
123.138114322818)) ;
#55114=CARTESIAN_POINT('Ctrl Pts',(-20.5399668125986,-38.4397242718799,
122.992486933)) ;
#55115=CARTESIAN_POINT('Ctrl Pts',(-20.8226462973431,-38.2597351913994,
122.887662089178)) ;
#55116=CARTESIAN_POINT('Ctrl Pts',(-20.4499783459561,-38.4497262280487,
122.802478082637)) ;
#55117=CARTESIAN_POINT('Ctrl Pts',(-20.710161993943,-38.2697371475682,122.650150261845)) ;
#55118=CARTESIAN_POINT('Ctrl Pts',(-20.3294778320045,-38.4596448247692,
122.632260562364)) ;
#55119=CARTESIAN_POINT('Ctrl Pts',(-20.5595370996362,-38.2796557442887,
122.437376954851)) ;
#55120=CARTESIAN_POINT('Ctrl Pts',(-20.1793517400514,-38.469691646845,122.483728376265)) ;
#55121=CARTESIAN_POINT('Ctrl Pts',(-20.3718806511006,-38.2897025663645,
122.25171084503)) ;
#55122=CARTESIAN_POINT('Ctrl Pts',(-20.0087562410276,-38.4795659279577,
122.365386621562)) ;
#55123=CARTESIAN_POINT('Ctrl Pts',(-20.1586361997854,-38.2995768474772,
122.103781929922)) ;
#55124=CARTESIAN_POINT('Ctrl Pts',(-19.8168874460983,-38.4896201280023,
122.27679388918)) ;
#55125=CARTESIAN_POINT('Ctrl Pts',(-19.9188009997021,-38.3096310475218,
121.993039913908)) ;
#55126=CARTESIAN_POINT('Ctrl Pts',(-19.6157267682506,-38.4995155576375,
122.223611335087)) ;
#55127=CARTESIAN_POINT('Ctrl Pts',(-19.6673495935341,-38.319526477157,121.926560228881)) ;
#55128=CARTESIAN_POINT('Ctrl Pts',(-19.4049744065646,-38.5095771859549,
122.2058271605)) ;
#55129=CARTESIAN_POINT('Ctrl Pts',(-19.4039095755323,-38.3295881054744,
121.904328761278)) ;
#55130=CARTESIAN_POINT('Ctrl Pts',(-19.198843636696,-38.5194218147848,122.224471407226)) ;
#55131=CARTESIAN_POINT('Ctrl Pts',(-19.1462446839781,-38.3394327343043,
121.927632919868)) ;
#55132=CARTESIAN_POINT('Ctrl Pts',(-18.9965533130945,-38.5293818623904,
122.278528162173)) ;
#55133=CARTESIAN_POINT('Ctrl Pts',(-18.8933810810185,-38.3493927819099,
121.995203018635)) ;
#55134=CARTESIAN_POINT('Ctrl Pts',(-18.8054118271966,-38.5394201685644,
122.367955384898)) ;
#55135=CARTESIAN_POINT('Ctrl Pts',(-18.6544538828599,-38.359431088084,122.106985936602)) ;
#55136=CARTESIAN_POINT('Ctrl Pts',(-18.63527681131,-38.5492934679971,122.48691582821)) ;
#55137=CARTESIAN_POINT('Ctrl Pts',(-18.4417836191752,-38.3693043875166,
122.255686315576)) ;
#55138=CARTESIAN_POINT('Ctrl Pts',(-18.4855083632064,-38.5593667295834,
122.636576989724)) ;
#55139=CARTESIAN_POINT('Ctrl Pts',(-18.2545726342141,-38.3793776491029,
122.442761738762)) ;
#55140=CARTESIAN_POINT('Ctrl Pts',(-18.3667777956026,-38.5691869555401,
122.805528697943)) ;
#55141=CARTESIAN_POINT('Ctrl Pts',(-18.1061577774749,-38.3891978750596,
122.653952115925)) ;
#55142=CARTESIAN_POINT('Ctrl Pts',(-18.2767515118799,-38.5792660194796,
122.997287213327)) ;
#55143=CARTESIAN_POINT('Ctrl Pts',(-17.9936243508535,-38.3992769389991,
122.893649468744)) ;
#55144=CARTESIAN_POINT('Ctrl Pts',(-18.2225229813274,-38.5891161094994,
123.197198324746)) ;
#55145=CARTESIAN_POINT('Ctrl Pts',(-17.9258375542978,-38.4091270290189,
123.143539427557)) ;
#55146=CARTESIAN_POINT('Ctrl Pts',(-18.2032956686347,-38.5991948631132,
123.408157950958)) ;
#55147=CARTESIAN_POINT('Ctrl Pts',(-17.9018026836596,-38.4192057826327,
123.407238410019)) ;
#55148=CARTESIAN_POINT('Ctrl Pts',(-18.2203875577578,-38.6090163303726,
123.613973329019)) ;
#55149=CARTESIAN_POINT('Ctrl Pts',(-17.9231669693498,-38.4290272498922,
123.664509279114)) ;
#55150=CARTESIAN_POINT('Ctrl Pts',(-18.2739238887591,-38.6190819287303,
123.818650277656)) ;
#55151=CARTESIAN_POINT('Ctrl Pts',(-17.9900867205332,-38.4390928482498,
123.920355248538)) ;
#55152=CARTESIAN_POINT('Ctrl Pts',(-18.3608489444241,-38.628984584505,124.007876019705)) ;
#55153=CARTESIAN_POINT('Ctrl Pts',(-18.098742864272,-38.4489955040245,124.156888509169)) ;
#55154=CARTESIAN_POINT('Ctrl Pts',(-18.4809742235416,-38.6390354103346,
124.181656276088)) ;
#55155=CARTESIAN_POINT('Ctrl Pts',(-18.2488988279935,-38.4590463298541,
124.37411393973)) ;
#55156=CARTESIAN_POINT('Ctrl Pts',(-18.6267574232004,-38.6489096146735,
124.329501799845)) ;
#55157=CARTESIAN_POINT('Ctrl Pts',(-18.4311282811755,-38.468920534193,124.558922029352)) ;
#55158=CARTESIAN_POINT('Ctrl Pts',(-18.7993133903288,-38.6589820647126,
124.452162400167)) ;
#55159=CARTESIAN_POINT('Ctrl Pts',(-18.6468225999744,-38.4789929842321,
124.712247945198)) ;
#55160=CARTESIAN_POINT('Ctrl Pts',(-18.9859137942603,-38.6688110814861,
124.541017706794)) ;
#55161=CARTESIAN_POINT('Ctrl Pts',(-18.8800743167086,-38.4888220010056,
124.823318123798)) ;
#55162=CARTESIAN_POINT('Ctrl Pts',(-19.1897774494704,-38.6788779274009,
124.597717051206)) ;
#55163=CARTESIAN_POINT('Ctrl Pts',(-19.1349034186217,-38.4988888469204,
124.894192497998)) ;
#55164=CARTESIAN_POINT('Ctrl Pts',(-19.3967662896624,-38.6887680987027,
124.617671141115)) ;
#55165=CARTESIAN_POINT('Ctrl Pts',(-19.3936404772035,-38.5087790182222,
124.919135574794)) ;
#55166=CARTESIAN_POINT('Ctrl Pts',(-19.6062117856198,-38.6987602923265,
124.601677520649)) ;
#55167=CARTESIAN_POINT('Ctrl Pts',(-19.6554475745954,-38.518771211846,124.899143715599)) ;
#55168=CARTESIAN_POINT('Ctrl Pts',(-19.8090578521169,-38.7087231029499,
124.549518835879)) ;
#55169=CARTESIAN_POINT('Ctrl Pts',(-19.9090056650938,-38.5287340224695,
124.83394550148)) ;
#55170=CARTESIAN_POINT('Ctrl Pts',(-19.9988839578665,-38.7186273757934,
124.463912950195)) ;
#55171=CARTESIAN_POINT('Ctrl Pts',(-20.1462891749534,-38.5386382953129,
124.726937805379)) ;
#55172=CARTESIAN_POINT('Ctrl Pts',(-20.1735373576463,-38.728687867598,124.344670095455)) ;
#55173=CARTESIAN_POINT('Ctrl Pts',(-20.3646057035926,-38.5486987871175,
124.577884540357)) ;
#55174=CARTESIAN_POINT('Ctrl Pts',(-20.3217496628908,-38.7385281992703,
124.200302181168)) ;
#55175=CARTESIAN_POINT('Ctrl Pts',(-20.54987215141,-38.5585391187898,124.397423633177)) ;
#55176=CARTESIAN_POINT('Ctrl Pts',(-20.4455536404309,-38.7485912453621,
124.028786981094)) ;
#55177=CARTESIAN_POINT('Ctrl Pts',(-20.7046268370077,-38.5686021648816,
124.183029887367)) ;
#55178=CARTESIAN_POINT('Ctrl Pts',(-20.5360148595755,-38.7584853010572,
123.841460701052)) ;
#55179=CARTESIAN_POINT('Ctrl Pts',(-20.8177037945612,-38.5784962205767,
123.948871113701)) ;
#55180=CARTESIAN_POINT('Ctrl Pts',(-20.5933924658413,-38.7684280013801,
123.640487605806)) ;
#55181=CARTESIAN_POINT('Ctrl Pts',(-20.8894257460655,-38.5884389208997,
123.697654055574)) ;
#55182=CARTESIAN_POINT('Ctrl Pts',(-20.6151860212168,-38.7784337423077,
123.431245299403)) ;
#55183=CARTESIAN_POINT('Ctrl Pts',(-20.9166674417384,-38.5984446618273,
123.436101061359)) ;
#55184=CARTESIAN_POINT('Ctrl Pts',(-20.6000592508299,-38.7884546528233,
123.221122882198)) ;
#55185=CARTESIAN_POINT('Ctrl Pts',(-20.8977588229699,-38.6084655723428,
123.173448091031)) ;
#55186=CARTESIAN_POINT('Ctrl Pts',(-20.5495758365941,-38.7983453882732,
123.0194036364)) ;
#55187=CARTESIAN_POINT('Ctrl Pts',(-20.8346540512189,-38.6183563077928,
122.921298084057)) ;
#55188=CARTESIAN_POINT('Ctrl Pts',(-20.4642602817029,-38.8083369290021,
122.827465431094)) ;
#55189=CARTESIAN_POINT('Ctrl Pts',(-20.7280091758248,-38.6283478485216,
122.681375284284)) ;
#55190=CARTESIAN_POINT('Ctrl Pts',(-20.3473737278901,-38.8182847894237,
122.654045824063)) ;
#55191=CARTESIAN_POINT('Ctrl Pts',(-20.5819003600427,-38.6382957089433,
122.464600480947)) ;
#55192=CARTESIAN_POINT('Ctrl Pts',(-20.202456742999,-38.8282314586101,122.503277801019)) ;
#55193=CARTESIAN_POINT('Ctrl Pts',(-20.4007533562876,-38.6482423781296,
122.276140396703)) ;
#55194=CARTESIAN_POINT('Ctrl Pts',(-20.0317199746376,-38.8382795347457,
122.378903058221)) ;
#55195=CARTESIAN_POINT('Ctrl Pts',(-20.1873323483246,-38.6582904542652,
122.120672459441)) ;
#55196=CARTESIAN_POINT('Ctrl Pts',(-19.8458354362141,-38.8481271327513,
122.287756233757)) ;
#55197=CARTESIAN_POINT('Ctrl Pts',(-19.9549752002144,-38.6681380522708,
122.006738756022)) ;
#55198=CARTESIAN_POINT('Ctrl Pts',(-19.6448376579705,-38.8580888558358,
122.228975330459)) ;
#55199=CARTESIAN_POINT('Ctrl Pts',(-19.7037273294594,-38.6780997753553,
121.933263220513)) ;
#55200=CARTESIAN_POINT('Ctrl Pts',(-19.4352361415482,-38.8681174909188,
122.206096194231)) ;
#55201=CARTESIAN_POINT('Ctrl Pts',(-19.4417254602137,-38.6881284104383,
121.904664952519)) ;
#55202=CARTESIAN_POINT('Ctrl Pts',(-19.2273465752442,-38.8780277992368,
122.219725256983)) ;
#55203=CARTESIAN_POINT('Ctrl Pts',(-19.1818626712833,-38.6980387187563,
121.921702009087)) ;
#55204=CARTESIAN_POINT('Ctrl Pts',(-19.0243342885466,-38.8879626963727,
122.26883883605)) ;
#55205=CARTESIAN_POINT('Ctrl Pts',(-18.9280968781403,-38.7079736158922,
121.983094997283)) ;
#55206=CARTESIAN_POINT('Ctrl Pts',(-18.8309772013695,-38.8980037793153,
122.353523961238)) ;
#55207=CARTESIAN_POINT('Ctrl Pts',(-18.686401014824,-38.7180146988348,122.088952068099)) ;
#55208=CARTESIAN_POINT('Ctrl Pts',(-18.6578590680997,-38.9078911221435,
122.468595150492)) ;
#55209=CARTESIAN_POINT('Ctrl Pts',(-18.4700029593095,-38.727902041663,122.232792348651)) ;
#55210=CARTESIAN_POINT('Ctrl Pts',(-18.5055317513843,-38.9178826370828,
122.613211351364)) ;
#55211=CARTESIAN_POINT('Ctrl Pts',(-18.2795943516708,-38.7378935566024,
122.413563464107)) ;
#55212=CARTESIAN_POINT('Ctrl Pts',(-18.3811911630624,-38.9278340282793,
122.781466926608)) ;
#55213=CARTESIAN_POINT('Ctrl Pts',(-18.124169074107,-38.7478449477989,122.623883938995)) ;
#55214=CARTESIAN_POINT('Ctrl Pts',(-18.2878097045155,-38.9377665616119,
122.968234846333)) ;
#55215=CARTESIAN_POINT('Ctrl Pts',(-18.0074429395974,-38.7577774811314,
122.857344924751)) ;
#55216=CARTESIAN_POINT('Ctrl Pts',(-18.2278106534503,-38.9477637195114,
123.1696520482)) ;
#55217=CARTESIAN_POINT('Ctrl Pts',(-17.9324451629911,-38.7677746390309,
123.109116894478)) ;
#55218=CARTESIAN_POINT('Ctrl Pts',(-18.2036416355779,-38.9577487296749,
123.378205341425)) ;
#55219=CARTESIAN_POINT('Ctrl Pts',(-17.902235014903,-38.7777596491944,123.369808873094)) ;
#55220=CARTESIAN_POINT('Ctrl Pts',(-18.2164291819651,-38.9677915562447,
123.588920968376)) ;
#55221=CARTESIAN_POINT('Ctrl Pts',(-17.9182204759992,-38.7878024757642,
123.63320316215)) ;
#55222=CARTESIAN_POINT('Ctrl Pts',(-18.2641206916243,-38.9776217905496,
123.790038485593)) ;
#55223=CARTESIAN_POINT('Ctrl Pts',(-17.9778363798766,-38.7976327100692,
123.884601181675)) ;
#55224=CARTESIAN_POINT('Ctrl Pts',(-18.3479385843405,-38.9876978157843,
123.984532944223)) ;
#55225=CARTESIAN_POINT('Ctrl Pts',(-18.0826097271677,-38.8077087353038,
124.12771836113)) ;
#55226=CARTESIAN_POINT('Ctrl Pts',(-18.4616277736015,-38.9975500522752,
124.157720560445)) ;
#55227=CARTESIAN_POINT('Ctrl Pts',(-18.2247229697952,-38.8175609717947,
124.344203206761)) ;
#55228=CARTESIAN_POINT('Ctrl Pts',(-18.6066621317061,-39.0076232587093,
124.31198450881)) ;
#55229=CARTESIAN_POINT('Ctrl Pts',(-18.4060166291239,-38.8276341782288,
124.537031921043)) ;
#55230=CARTESIAN_POINT('Ctrl Pts',(-18.7724492303032,-39.0174647682165,
124.435789163625)) ;
#55231=CARTESIAN_POINT('Ctrl Pts',(-18.6132523457077,-38.837475687736,124.691787453299)) ;
#55232=CARTESIAN_POINT('Ctrl Pts',(-18.9590824114606,-39.0274257149963,
124.530751648875)) ;
#55233=CARTESIAN_POINT('Ctrl Pts',(-18.8465449134313,-38.8474366345158,
124.810489310477)) ;
#55234=CARTESIAN_POINT('Ctrl Pts',(-19.1610387527157,-39.0374635437963,
124.591933966622)) ;
#55235=CARTESIAN_POINT('Ctrl Pts',(-19.0989906357257,-38.8574744633158,
124.886965770445)) ;
#55236=CARTESIAN_POINT('Ctrl Pts',(-19.3671221533313,-39.0473378535508,
124.617096782991)) ;
#55237=CARTESIAN_POINT('Ctrl Pts',(-19.3565960865102,-38.8673487730703,
124.918417832492)) ;
#55238=CARTESIAN_POINT('Ctrl Pts',(-19.5784931233021,-39.0574075512239,
124.605867995762)) ;
#55239=CARTESIAN_POINT('Ctrl Pts',(-19.6208093649066,-38.8774184707435,
124.904380279425)) ;
#55240=CARTESIAN_POINT('Ctrl Pts',(-19.7799321898415,-39.0672410225113,
124.55932535313)) ;
#55241=CARTESIAN_POINT('Ctrl Pts',(-19.8726090819343,-38.8872519420309,
124.846200104138)) ;
#55242=CARTESIAN_POINT('Ctrl Pts',(-19.9742453524244,-39.0772706690413,
124.477468158144)) ;
#55243=CARTESIAN_POINT('Ctrl Pts',(-20.1154997479825,-38.8972815885608,
124.74387696496)) ;
#55244=CARTESIAN_POINT('Ctrl Pts',(-20.1511369807371,-39.0873051833686,
124.36251502401)) ;
#55245=CARTESIAN_POINT('Ctrl Pts',(-20.3366133293652,-38.9073161028882,
124.600184240841)) ;
#55246=CARTESIAN_POINT('Ctrl Pts',(-20.3025021754356,-39.0971304688395,
124.221961302064)) ;
#55247=CARTESIAN_POINT('Ctrl Pts',(-20.5258195612179,-38.9171413883591,
124.424489905095)) ;
#55248=CARTESIAN_POINT('Ctrl Pts',(-20.4297743163725,-39.1071347103881,
124.05455039433)) ;
#55249=CARTESIAN_POINT('Ctrl Pts',(-20.6849082650607,-38.9271456299076,
124.21522504281)) ;
#55250=CARTESIAN_POINT('Ctrl Pts',(-20.5257881932866,-39.1171173554672,
123.867889590297)) ;
#55251=CARTESIAN_POINT('Ctrl Pts',(-20.8049240328739,-38.9371282749867,
123.98189798355)) ;
#55252=CARTESIAN_POINT('Ctrl Pts',(-20.588074926157,-39.1271625525587,123.666125982417)) ;
#55253=CARTESIAN_POINT('Ctrl Pts',(-20.8827806721499,-38.9471734720782,
123.729693087469)) ;
#55254=CARTESIAN_POINT('Ctrl Pts',(-20.6141505417572,-39.1369856683188,
123.461258677549)) ;
#55255=CARTESIAN_POINT('Ctrl Pts',(-20.9153734466188,-38.9569965878383,
123.473607472972)) ;
#55256=CARTESIAN_POINT('Ctrl Pts',(-20.60457754197,-39.1470202801191,123.250519610856)) ;
#55257=CARTESIAN_POINT('Ctrl Pts',(-20.9034051258679,-38.9670311996386,
123.210183840075)) ;
#55258=CARTESIAN_POINT('Ctrl Pts',(-20.5580262468952,-39.1570452888922,
123.044960994217)) ;
#55259=CARTESIAN_POINT('Ctrl Pts',(-20.8452141571095,-38.9770562084118,
122.953236014132)) ;
#55260=CARTESIAN_POINT('Ctrl Pts',(-20.478316885892,-39.1668972137338,122.853791086259)) ;
#55261=CARTESIAN_POINT('Ctrl Pts',(-20.7455751868361,-38.9869081332533,
122.714273478648)) ;
#55262=CARTESIAN_POINT('Ctrl Pts',(-20.3653360181163,-39.1768881520565,
122.676754747224)) ;
#55263=CARTESIAN_POINT('Ctrl Pts',(-20.6043472153885,-38.996899071576,122.492979055613)) ;
#55264=CARTESIAN_POINT('Ctrl Pts',(-20.2244345622947,-39.186806137203,122.523026316099)) ;
#55265=CARTESIAN_POINT('Ctrl Pts',(-20.4282184152407,-39.0068170567225,
122.300819554093)) ;
#55266=CARTESIAN_POINT('Ctrl Pts',(-20.0572079878956,-39.1968342380985,
122.394673439318)) ;
#55267=CARTESIAN_POINT('Ctrl Pts',(-20.2191839000679,-39.016845157618,122.140380206169)) ;
#55268=CARTESIAN_POINT('Ctrl Pts',(-19.8729210552735,-39.2067194790411,
122.298607224345)) ;
#55269=CARTESIAN_POINT('Ctrl Pts',(-19.9888235634407,-39.0267303985606,
122.020299045186)) ;
#55270=CARTESIAN_POINT('Ctrl Pts',(-19.6728247514948,-39.2167085920077,
122.234848345753)) ;
#55271=CARTESIAN_POINT('Ctrl Pts',(-19.7387023265823,-39.0367195115272,
121.940602617531)) ;
#55272=CARTESIAN_POINT('Ctrl Pts',(-19.4635439074029,-39.2267506563485,
122.207112896328)) ;
#55273=CARTESIAN_POINT('Ctrl Pts',(-19.4771010747328,-39.046761575868,121.905935512341)) ;
#55274=CARTESIAN_POINT('Ctrl Pts',(-19.2570678726038,-39.236579857753,122.215554269047)) ;
#55275=CARTESIAN_POINT('Ctrl Pts',(-19.2190051557527,-39.0565907772725,
121.916489575375)) ;
#55276=CARTESIAN_POINT('Ctrl Pts',(-19.0514789396674,-39.2465866985112,
122.260060325551)) ;
#55277=CARTESIAN_POINT('Ctrl Pts',(-18.9620194272015,-39.0665976180307,
121.972124528351)) ;
#55278=CARTESIAN_POINT('Ctrl Pts',(-18.857109213024,-39.2565742227031,122.33957226792)) ;
#55279=CARTESIAN_POINT('Ctrl Pts',(-18.7190580246023,-39.0765851422226,
122.071516725931)) ;
#55280=CARTESIAN_POINT('Ctrl Pts',(-18.6788723961599,-39.2666038685117,
122.452193066981)) ;
#55281=CARTESIAN_POINT('Ctrl Pts',(-18.4962632861033,-39.0866147880312,
122.212294698753)) ;
#55282=CARTESIAN_POINT('Ctrl Pts',(-18.5251202819395,-39.2764778992504,
122.591691852542)) ;
#55283=CARTESIAN_POINT('Ctrl Pts',(-18.3040742601302,-39.09648881877,122.386670420962)) ;
#55284=CARTESIAN_POINT('Ctrl Pts',(-18.3961396998256,-39.2864772221145,
122.757647081456)) ;
#55285=CARTESIAN_POINT('Ctrl Pts',(-18.1428504125895,-39.1064881416341,
122.594116058495)) ;
#55286=CARTESIAN_POINT('Ctrl Pts',(-18.2985886975645,-39.2963880576901,
122.941797700532)) ;
#55287=CARTESIAN_POINT('Ctrl Pts',(-18.0209136489367,-39.1163989772096,
122.824305926484)) ;
#55288=CARTESIAN_POINT('Ctrl Pts',(-18.2336609868071,-39.3064423056642,
123.142915425112)) ;
#55289=CARTESIAN_POINT('Ctrl Pts',(-17.939756418394,-39.1264532251837,123.075703741518)) ;
#55290=CARTESIAN_POINT('Ctrl Pts',(-18.2049530968866,-39.3163010499269,
123.348215710506)) ;
#55291=CARTESIAN_POINT('Ctrl Pts',(-17.9038739771922,-39.1363119694464,
123.332330097251)) ;
#55292=CARTESIAN_POINT('Ctrl Pts',(-18.2123561541688,-39.3263691359999,
123.559718460866)) ;
#55293=CARTESIAN_POINT('Ctrl Pts',(-17.9131303554343,-39.1463800555194,
123.596708290332)) ;
#55294=CARTESIAN_POINT('Ctrl Pts',(-18.2554666856692,-39.3362246191794,
123.762394729141)) ;
#55295=CARTESIAN_POINT('Ctrl Pts',(-17.9670211521301,-39.1562355386989,
123.850053708721)) ;
#55296=CARTESIAN_POINT('Ctrl Pts',(-18.333618279946,-39.3462194649736,123.957436253623)) ;
#55297=CARTESIAN_POINT('Ctrl Pts',(-18.0647131558998,-39.1662303844931,
124.093854715397)) ;
#55298=CARTESIAN_POINT('Ctrl Pts',(-18.4452442598356,-39.3562507606361,
124.136365747188)) ;
#55299=CARTESIAN_POINT('Ctrl Pts',(-18.2042478279912,-39.1762616801557,
124.317515212328)) ;
#55300=CARTESIAN_POINT('Ctrl Pts',(-18.5836826690354,-39.366117303926,124.290842760862)) ;
#55301=CARTESIAN_POINT('Ctrl Pts',(-18.3772981540665,-39.1861282234455,
124.510610102778)) ;
#55302=CARTESIAN_POINT('Ctrl Pts',(-18.748604585584,-39.3761046996894,124.420751361441)) ;
#55303=CARTESIAN_POINT('Ctrl Pts',(-18.5834523132856,-39.1961156192089,
124.67299381361)) ;
#55304=CARTESIAN_POINT('Ctrl Pts',(-18.9327894876098,-39.3860497404194,
124.519754705833)) ;
#55305=CARTESIAN_POINT('Ctrl Pts',(-18.8136849280441,-39.2060606599389,
124.796745724835)) ;
#55306=CARTESIAN_POINT('Ctrl Pts',(-19.1333404381493,-39.3960942466361,
124.585800268565)) ;
#55307=CARTESIAN_POINT('Ctrl Pts',(-19.0643744384591,-39.2161051661556,
124.879300116025)) ;
#55308=CARTESIAN_POINT('Ctrl Pts',(-19.3385607919778,-39.4059577527734,
124.615667658985)) ;
#55309=CARTESIAN_POINT('Ctrl Pts',(-19.3209006976824,-39.2259686722929,
124.916631731361)) ;
#55310=CARTESIAN_POINT('Ctrl Pts',(-19.5485278972259,-39.4159506136095,
124.609740631774)) ;
#55311=CARTESIAN_POINT('Ctrl Pts',(-19.5833595972731,-39.235961533129,124.909220187346)) ;
#55312=CARTESIAN_POINT('Ctrl Pts',(-19.7529825851974,-39.4258768073284,
124.567812438431)) ;
#55313=CARTESIAN_POINT('Ctrl Pts',(-19.8389276222592,-39.2458877268479,
124.85680719715)) ;
#55314=CARTESIAN_POINT('Ctrl Pts',(-19.9488284655848,-39.435895733361,124.490360997072)) ;
#55315=CARTESIAN_POINT('Ctrl Pts',(-20.0837340013322,-39.2559066528805,
124.759990302527)) ;
#55316=CARTESIAN_POINT('Ctrl Pts',(-20.126540851108,-39.4458107327286,124.381363000925)) ;
#55317=CARTESIAN_POINT('Ctrl Pts',(-20.3058732170671,-39.2658216522481,
124.62374032262)) ;
#55318=CARTESIAN_POINT('Ctrl Pts',(-20.2847556242028,-39.4558655042859,
124.241221421377)) ;
#55319=CARTESIAN_POINT('Ctrl Pts',(-20.5036398439855,-39.2758764238054,
124.448561262126)) ;
#55320=CARTESIAN_POINT('Ctrl Pts',(-20.4138101110339,-39.4657244665834,
124.079002697982)) ;
#55321=CARTESIAN_POINT('Ctrl Pts',(-20.6649559415589,-39.285735386103,124.245785908766)) ;
#55322=CARTESIAN_POINT('Ctrl Pts',(-20.514413173183,-39.4757187104213,123.894581207319)) ;
#55323=CARTESIAN_POINT('Ctrl Pts',(-20.7907073339488,-39.2957296299408,
124.015257630094)) ;
#55324=CARTESIAN_POINT('Ctrl Pts',(-20.5811176261202,-39.4856439398455,
123.69683639536)) ;
#55325=CARTESIAN_POINT('Ctrl Pts',(-20.8740852788276,-39.305654859365,123.768075589586)) ;
#55326=CARTESIAN_POINT('Ctrl Pts',(-20.6127981685667,-39.495671903737,123.488439172828)) ;
#55327=CARTESIAN_POINT('Ctrl Pts',(-20.9136831803521,-39.3156828232565,
123.507578576401)) ;
#55328=CARTESIAN_POINT('Ctrl Pts',(-20.6080961840771,-39.5055581633674,
123.280620724186)) ;
#55329=CARTESIAN_POINT('Ctrl Pts',(-20.9078028796021,-39.3255690828869,
123.24780545798)) ;
#55330=CARTESIAN_POINT('Ctrl Pts',(-20.5669027528603,-39.5155899264452,
123.073819312021)) ;
#55331=CARTESIAN_POINT('Ctrl Pts',(-20.8563083057196,-39.3356008459647,
122.989304179159)) ;
#55332=CARTESIAN_POINT('Ctrl Pts',(-20.4917344516677,-39.5254715527393,
122.880112689592)) ;
#55333=CARTESIAN_POINT('Ctrl Pts',(-20.7623452756417,-39.3454824722589,
122.747171858432)) ;
#55334=CARTESIAN_POINT('Ctrl Pts',(-20.3821947597893,-39.5355333222255,
122.69919029706)) ;
#55335=CARTESIAN_POINT('Ctrl Pts',(-20.6254182000016,-39.355544241745,122.521020259929)) ;
#55336=CARTESIAN_POINT('Ctrl Pts',(-20.2457369593962,-39.545391189721,122.543178844289)) ;
#55337=CARTESIAN_POINT('Ctrl Pts',(-20.4548438166612,-39.3654021092405,
122.326007789972)) ;
#55338=CARTESIAN_POINT('Ctrl Pts',(-20.0824035138093,-39.5553828148383,
122.411136991431)) ;
#55339=CARTESIAN_POINT('Ctrl Pts',(-20.2506752049855,-39.3753937343579,
122.160957633179)) ;
#55340=CARTESIAN_POINT('Ctrl Pts',(-19.8995811867269,-39.5653196139466,
122.310034299086)) ;
#55341=CARTESIAN_POINT('Ctrl Pts',(-20.0221459359936,-39.3853305334661,
122.034581725354)) ;
#55342=CARTESIAN_POINT('Ctrl Pts',(-19.7010155069493,-39.5753104435039,
122.241558693215)) ;
#55343=CARTESIAN_POINT('Ctrl Pts',(-19.7739378813006,-39.3953213630234,
121.948989845614)) ;
#55344=CARTESIAN_POINT('Ctrl Pts',(-19.492862253122,-39.5853336792171,122.208735174446)) ;
#55345=CARTESIAN_POINT('Ctrl Pts',(-19.5137457792946,-39.4053445987366,
121.907963203133)) ;
#55346=CARTESIAN_POINT('Ctrl Pts',(-19.2848447608836,-39.5952300272463,
122.212328557573)) ;
#55347=CARTESIAN_POINT('Ctrl Pts',(-19.2537240353336,-39.4152409467658,
121.91245773756)) ;
#55348=CARTESIAN_POINT('Ctrl Pts',(-19.0785873856562,-39.6052195897488,
122.251922424187)) ;
#55349=CARTESIAN_POINT('Ctrl Pts',(-18.9959028450038,-39.4252305092683,
121.961952758409)) ;
#55350=CARTESIAN_POINT('Ctrl Pts',(-18.8815126411,-39.6152598974333,122.327498065648)) ;
#55351=CARTESIAN_POINT('Ctrl Pts',(-18.7495601439939,-39.4352708169529,
122.05642510042)) ;
#55352=CARTESIAN_POINT('Ctrl Pts',(-18.7038945149076,-39.6251022007805,
122.433676485987)) ;
#55353=CARTESIAN_POINT('Ctrl Pts',(-18.5275396487683,-39.4451131203,122.189149904719)) ;
#55354=CARTESIAN_POINT('Ctrl Pts',(-18.5443823308829,-39.6351259090596,
122.571330211097)) ;
#55355=CARTESIAN_POINT('Ctrl Pts',(-18.328149190755,-39.4551368285791,122.361220908042)) ;
#55356=CARTESIAN_POINT('Ctrl Pts',(-18.3685442000014,-39.6483480865273,
122.786691141863)) ;
#55357=CARTESIAN_POINT('Ctrl Pts',(-18.1083641387058,-39.4683590060468,
122.630415698237)) ;
#55358=CARTESIAN_POINT('Ctrl Pts',(-18.2520900531708,-39.6616406715866,
123.044166683935)) ;
#55359=CARTESIAN_POINT('Ctrl Pts',(-17.9628051139688,-39.4816515911061,
122.952220149181)) ;
#55360=CARTESIAN_POINT('Ctrl Pts',(-18.2067947635487,-39.6749255275082,
123.319772585123)) ;
#55361=CARTESIAN_POINT('Ctrl Pts',(-17.9061735338517,-39.4949364470277,
123.296785705757)) ;
#55362=CARTESIAN_POINT('Ctrl Pts',(-18.2090712913271,-39.684897754681,123.529386284599)) ;
#55363=CARTESIAN_POINT('Ctrl Pts',(-17.9090249685685,-39.5049086742005,
123.558791097675)) ;
#55364=CARTESIAN_POINT('Ctrl Pts',(-18.2471189349561,-39.69480637112,123.734216590928)) ;
#55365=CARTESIAN_POINT('Ctrl Pts',(-17.9565864887432,-39.5148172906395,
123.814831513913)) ;
#55366=CARTESIAN_POINT('Ctrl Pts',(-18.3212835409877,-39.7048595765037,
123.932106036806)) ;
#55367=CARTESIAN_POINT('Ctrl Pts',(-18.049293676017,-39.5248704960232,124.06219099881)) ;
#55368=CARTESIAN_POINT('Ctrl Pts',(-18.4265731448462,-39.714724710264,124.110805164923)) ;
#55369=CARTESIAN_POINT('Ctrl Pts',(-18.1809125136437,-39.5347356297835,
124.285566479099)) ;
#55370=CARTESIAN_POINT('Ctrl Pts',(-18.6083337458461,-39.7280637678903,
124.324363825404)) ;
#55371=CARTESIAN_POINT('Ctrl Pts',(-18.408091089116,-39.5480746874098,124.552496993476)) ;
#55372=CARTESIAN_POINT('Ctrl Pts',(-18.8983167375147,-39.7446329552234,
124.524458458027)) ;
#55373=CARTESIAN_POINT('Ctrl Pts',(-18.7706176278326,-39.564643874743,124.802631869108)) ;
#55374=CARTESIAN_POINT('Ctrl Pts',(-19.2406669716427,-39.7612780950745,
124.61423815662)) ;
#55375=CARTESIAN_POINT('Ctrl Pts',(-19.1984775012309,-39.581289014594,124.914837427828)) ;
#55376=CARTESIAN_POINT('Ctrl Pts',(-19.5196867167119,-39.7745503975479,
124.61271922313)) ;
#55377=CARTESIAN_POINT('Ctrl Pts',(-19.5473160626287,-39.5945613170674,
124.912945050873)) ;
#55378=CARTESIAN_POINT('Ctrl Pts',(-19.7261653450185,-39.7845313609955,
124.575425604287)) ;
#55379=CARTESIAN_POINT('Ctrl Pts',(-19.8054003622426,-39.604542280515,124.866324423839)) ;
#55380=CARTESIAN_POINT('Ctrl Pts',(-19.9223292162796,-39.7944731930648,
124.503237795506)) ;
#55381=CARTESIAN_POINT('Ctrl Pts',(-20.0506098850726,-39.6144841125843,
124.776085831231)) ;
#55382=CARTESIAN_POINT('Ctrl Pts',(-20.1643724086472,-39.8077927622802,
124.362474521717)) ;
#55383=CARTESIAN_POINT('Ctrl Pts',(-20.3531494020375,-39.6278036817997,
124.600140542085)) ;
#55384=CARTESIAN_POINT('Ctrl Pts',(-20.412637735221,-39.824322917213,124.113575614291)) ;
#55385=CARTESIAN_POINT('Ctrl Pts',(-20.6634916789973,-39.6443338367325,
124.28900205587)) ;
#55386=CARTESIAN_POINT('Ctrl Pts',(-20.5921614259415,-39.8443446427051,
123.727677934125)) ;
#55387=CARTESIAN_POINT('Ctrl Pts',(-20.8878880490218,-39.6643555622246,
123.806632140342)) ;
#55388=CARTESIAN_POINT('Ctrl Pts',(-20.62909002806,-39.8641560393119,123.307952932077)) ;
#55389=CARTESIAN_POINT('Ctrl Pts',(-20.9340458412992,-39.6841669588314,
123.281975948005)) ;
#55390=CARTESIAN_POINT('Ctrl Pts',(-20.5203568846511,-39.8841412880207,
122.897261125277)) ;
#55391=CARTESIAN_POINT('Ctrl Pts',(-20.7981256342363,-39.7041522075403,
122.768612564849)) ;
#55392=CARTESIAN_POINT('Ctrl Pts',(-20.2787761694729,-39.9040353506567,
122.549947579521)) ;
#55393=CARTESIAN_POINT('Ctrl Pts',(-20.4961474224209,-39.7240462701762,
122.334473379661)) ;
#55394=CARTESIAN_POINT('Ctrl Pts',(-19.9329494436863,-39.9239670298303,
122.304988298998)) ;
#55395=CARTESIAN_POINT('Ctrl Pts',(-20.0638627447484,-39.7439779493498,
122.028277249593)) ;
#55396=CARTESIAN_POINT('Ctrl Pts',(-19.5235438881534,-39.9439310843023,
122.192828842814)) ;
#55397=CARTESIAN_POINT('Ctrl Pts',(-19.5521053130937,-39.7639420038218,
121.888081012705)) ;
#55398=CARTESIAN_POINT('Ctrl Pts',(-19.1021579397527,-39.9638119860652,
122.226651373111)) ;
#55399=CARTESIAN_POINT('Ctrl Pts',(-19.0253744539521,-39.7838229055847,
121.930361826918)) ;
#55400=CARTESIAN_POINT('Ctrl Pts',(-18.7163649280739,-39.9837506476736,
122.402373200005)) ;
#55401=CARTESIAN_POINT('Ctrl Pts',(-18.5431348408587,-39.8037615671931,
122.150015941179)) ;
#55402=CARTESIAN_POINT('Ctrl Pts',(-18.4142773535418,-40.0036471729289,
122.698534548937)) ;
#55403=CARTESIAN_POINT('Ctrl Pts',(-18.1655278031791,-39.8236580924484,
122.520218221222)) ;
#55404=CARTESIAN_POINT('Ctrl Pts',(-18.2307652703842,-40.0235422113832,
123.07969577924)) ;
#55405=CARTESIAN_POINT('Ctrl Pts',(-17.9361396475794,-39.8435531309027,
122.996669054395)) ;
#55406=CARTESIAN_POINT('Ctrl Pts',(-18.1882574040753,-40.0435060346893,
123.502015421763)) ;
#55407=CARTESIAN_POINT('Ctrl Pts',(-17.8830061323076,-39.8635169542088,
123.524568225162)) ;
#55408=CARTESIAN_POINT('Ctrl Pts',(-18.29165985598,-40.0633801588183,123.911779372075)) ;
#55409=CARTESIAN_POINT('Ctrl Pts',(-18.0122595315461,-39.8833910783379,
124.036771136699)) ;
#55410=CARTESIAN_POINT('Ctrl Pts',(-18.5295568784576,-40.0833552345456,
124.263648018593)) ;
#55411=CARTESIAN_POINT('Ctrl Pts',(-18.3096308449976,-39.9033661540651,
124.476606505177)) ;
#55412=CARTESIAN_POINT('Ctrl Pts',(-18.873213806286,-40.1033088039022,124.512438604021)) ;
#55413=CARTESIAN_POINT('Ctrl Pts',(-18.7392016864746,-39.9233197234217,
124.787593898658)) ;
#55414=CARTESIAN_POINT('Ctrl Pts',(-19.2785655362842,-40.12314671409,124.629117591118)) ;
#55415=CARTESIAN_POINT('Ctrl Pts',(-19.2458886960496,-39.9431576336096,
124.933442272178)) ;
#55416=CARTESIAN_POINT('Ctrl Pts',(-19.7023551259677,-40.143122542661,124.600718350869)) ;
#55417=CARTESIAN_POINT('Ctrl Pts',(-19.775625440603,-39.9631334621805,124.897944226838)) ;
#55418=CARTESIAN_POINT('Ctrl Pts',(-20.0896769698093,-40.1630405873712,
124.429488132005)) ;
#55419=CARTESIAN_POINT('Ctrl Pts',(-20.2597769713751,-39.9830515068908,
124.683907753037)) ;
#55420=CARTESIAN_POINT('Ctrl Pts',(-20.3954104326446,-40.1829108331589,
124.137764071626)) ;
#55421=CARTESIAN_POINT('Ctrl Pts',(-20.6419438142498,-40.0029217526784,
124.319255201606)) ;
#55422=CARTESIAN_POINT('Ctrl Pts',(-20.5842765338552,-40.2029598362585,
123.755710496064)) ;
#55423=CARTESIAN_POINT('Ctrl Pts',(-20.8780281938708,-40.022970755778,123.841688417909)) ;
#55424=CARTESIAN_POINT('Ctrl Pts',(-20.6312875915322,-40.2227390774993,
123.337660256565)) ;
#55425=CARTESIAN_POINT('Ctrl Pts',(-20.936793816344,-40.0427499970188,123.319128562733)) ;
#55426=CARTESIAN_POINT('Ctrl Pts',(-20.532247620092,-40.2427691412082,122.923541794563)) ;
#55427=CARTESIAN_POINT('Ctrl Pts',(-20.812996407082,-40.0627800607277,122.801479468749)) ;
#55428=CARTESIAN_POINT('Ctrl Pts',(-20.2989045718909,-40.2626514261102,
122.570943457578)) ;
#55429=CARTESIAN_POINT('Ctrl Pts',(-20.5213204072867,-40.0826623456297,
122.360731281986)) ;
#55430=CARTESIAN_POINT('Ctrl Pts',(-19.9600279754679,-40.2825337270031,
122.318257760773)) ;
#55431=CARTESIAN_POINT('Ctrl Pts',(-20.0977276288373,-40.1025446465226,
122.044872252557)) ;
#55432=CARTESIAN_POINT('Ctrl Pts',(-19.5531288014987,-40.3025168366215,
122.195882017085)) ;
#55433=CARTESIAN_POINT('Ctrl Pts',(-19.5891047472239,-40.122527756141,121.891899364453)) ;
#55434=CARTESIAN_POINT('Ctrl Pts',(-19.1308454732642,-40.3224072319994,
122.219647803408)) ;
#55435=CARTESIAN_POINT('Ctrl Pts',(-19.0612513999883,-40.1424181515189,
121.921603035478)) ;
#55436=CARTESIAN_POINT('Ctrl Pts',(-18.7417231158238,-40.3423040220336,
122.38552655651)) ;
#55437=CARTESIAN_POINT('Ctrl Pts',(-18.5748477162323,-40.1623149415532,
122.128947492221)) ;
#55438=CARTESIAN_POINT('Ctrl Pts',(-18.4318742792953,-40.3622210759752,
122.674244241734)) ;
#55439=CARTESIAN_POINT('Ctrl Pts',(-18.187534217096,-40.1822319954948,122.489841093105)) ;
#55440=CARTESIAN_POINT('Ctrl Pts',(-18.2384227273083,-40.3822246241788,
123.053097596815)) ;
#55441=CARTESIAN_POINT('Ctrl Pts',(-17.9457158454956,-40.2022355436983,
122.963405930275)) ;
#55442=CARTESIAN_POINT('Ctrl Pts',(-18.1866699600762,-40.4021629178314,
123.473848629645)) ;
#55443=CARTESIAN_POINT('Ctrl Pts',(-17.8810209347116,-40.2221738373509,
123.489343815261)) ;
#55444=CARTESIAN_POINT('Ctrl Pts',(-18.280049631561,-40.4219844052643,123.884838555175)) ;
#55445=CARTESIAN_POINT('Ctrl Pts',(-17.99774005357,-40.2419953247838,124.003081008406)) ;
#55446=CARTESIAN_POINT('Ctrl Pts',(-18.5094838644823,-40.4419627982552,
124.242285334387)) ;
#55447=CARTESIAN_POINT('Ctrl Pts',(-18.2845312146954,-40.2619737177747,
124.449892679484)) ;
#55448=CARTESIAN_POINT('Ctrl Pts',(-18.8460247213349,-40.4618611798689,
124.498817471921)) ;
#55449=CARTESIAN_POINT('Ctrl Pts',(-18.7051945464138,-40.2818720993884,
124.770559205583)) ;
#55450=CARTESIAN_POINT('Ctrl Pts',(-19.1823032913064,-40.4784441105988,
124.604500943763)) ;
#55451=CARTESIAN_POINT('Ctrl Pts',(-19.1255703487447,-40.2984550301183,
124.902674539656)) ;
#55452=CARTESIAN_POINT('Ctrl Pts',(-19.4611720898915,-40.4917183461876,
124.616752614585)) ;
#55453=CARTESIAN_POINT('Ctrl Pts',(-19.4741295857848,-40.3117292657071,
124.917986772881)) ;
#55454=CARTESIAN_POINT('Ctrl Pts',(-19.6705355947193,-40.5017647636438,
124.589137634991)) ;
#55455=CARTESIAN_POINT('Ctrl Pts',(-19.735842546372,-40.3217756831633,124.883469686386)) ;
#55456=CARTESIAN_POINT('Ctrl Pts',(-19.8680131387049,-40.5116099888631,
124.527058907304)) ;
#55457=CARTESIAN_POINT('Ctrl Pts',(-19.9826774778884,-40.3316209083826,
124.805881778766)) ;
#55458=CARTESIAN_POINT('Ctrl Pts',(-20.1170123821962,-40.5249449599025,
124.398409715662)) ;
#55459=CARTESIAN_POINT('Ctrl Pts',(-20.2939829336976,-40.344955879422,124.645032732069)) ;
#55460=CARTESIAN_POINT('Ctrl Pts',(-20.3777873292751,-40.5415278166951,
124.160882668887)) ;
#55461=CARTESIAN_POINT('Ctrl Pts',(-20.6198884115965,-40.3615387362146,
124.348182656348)) ;
#55462=CARTESIAN_POINT('Ctrl Pts',(-20.5424028350229,-40.5581708190445,
123.847768971427)) ;
#55463=CARTESIAN_POINT('Ctrl Pts',(-20.8256972517839,-40.378181738564,123.956743051222)) ;
#55464=CARTESIAN_POINT('Ctrl Pts',(-20.6040438140094,-40.5714145500762,
123.576158500164)) ;
#55465=CARTESIAN_POINT('Ctrl Pts',(-20.9027340824699,-40.3914254695957,
123.617264907902)) ;
#55466=CARTESIAN_POINT('Ctrl Pts',(-20.6143139077877,-40.5814689447508,
123.36507953087)) ;
#55467=CARTESIAN_POINT('Ctrl Pts',(-20.9155780419708,-40.4014798642703,
123.353409333883)) ;
#55468=CARTESIAN_POINT('Ctrl Pts',(-20.5885990189638,-40.5913100061393,
123.159754071886)) ;
#55469=CARTESIAN_POINT('Ctrl Pts',(-20.8834362368491,-40.4113209256588,
123.096754250321)) ;
#55470=CARTESIAN_POINT('Ctrl Pts',(-20.5264471958815,-40.6013762304958,
122.957500488943)) ;
#55471=CARTESIAN_POINT('Ctrl Pts',(-20.8057493251585,-40.4213871500153,
122.843935791852)) ;
#55472=CARTESIAN_POINT('Ctrl Pts',(-20.4318111963384,-40.6112568434155,
122.772550933144)) ;
#55473=CARTESIAN_POINT('Ctrl Pts',(-20.6874567829705,-40.431267762935,122.612747828755)) ;
#55474=CARTESIAN_POINT('Ctrl Pts',(-20.3054294573994,-40.6212501365751,
122.604767036362)) ;
#55475=CARTESIAN_POINT('Ctrl Pts',(-20.5294818313547,-40.4412610560946,
122.403016184021)) ;
#55476=CARTESIAN_POINT('Ctrl Pts',(-20.1524873681173,-40.6312011447987,
122.461975515907)) ;
#55477=CARTESIAN_POINT('Ctrl Pts',(-20.3383061145798,-40.4512120643182,
122.22452473296)) ;
#55478=CARTESIAN_POINT('Ctrl Pts',(-19.9753190448652,-40.6412496591607,
122.346959912909)) ;
#55479=CARTESIAN_POINT('Ctrl Pts',(-20.1168471521644,-40.4612605786802,
122.080752823269)) ;
#55480=CARTESIAN_POINT('Ctrl Pts',(-19.7849296325353,-40.6510911652234,
122.265920115438)) ;
#55481=CARTESIAN_POINT('Ctrl Pts',(-19.878861530971,-40.4711020847429,121.979450513718)) ;
#55482=CARTESIAN_POINT('Ctrl Pts',(-19.5805644894003,-40.6610768178531,
122.218048516374)) ;
#55483=CARTESIAN_POINT('Ctrl Pts',(-19.623405666542,-40.4810877373726,121.919608246859)) ;
#55484=CARTESIAN_POINT('Ctrl Pts',(-19.3719102404823,-40.671015826698,122.206359844049)) ;
#55485=CARTESIAN_POINT('Ctrl Pts',(-19.3625879444229,-40.4910267462175,
121.904994592829)) ;
#55486=CARTESIAN_POINT('Ctrl Pts',(-19.1623259439942,-40.681056751991,122.231380193141)) ;
#55487=CARTESIAN_POINT('Ctrl Pts',(-19.1006071741464,-40.5010676715105,
121.936267236799)) ;
#55488=CARTESIAN_POINT('Ctrl Pts',(-18.9632287027856,-40.6909470737459,
122.291388692216)) ;
#55489=CARTESIAN_POINT('Ctrl Pts',(-18.851734717605,-40.5109579932654,122.01127519242)) ;
#55490=CARTESIAN_POINT('Ctrl Pts',(-18.7754842627344,-40.7009430470793,
122.385762996334)) ;
#55491=CARTESIAN_POINT('Ctrl Pts',(-18.6170528303436,-40.5209539665988,
122.129240595498)) ;
#55492=CARTESIAN_POINT('Ctrl Pts',(-18.6080361030909,-40.7108744466613,
122.51049410798)) ;
#55493=CARTESIAN_POINT('Ctrl Pts',(-18.4077408549979,-40.5308853661809,
122.285152304377)) ;
#55494=CARTESIAN_POINT('Ctrl Pts',(-18.4635012584254,-40.7208799871384,
122.663335115609)) ;
#55495=CARTESIAN_POINT('Ctrl Pts',(-18.2270702112574,-40.5408909066579,
122.47620169738)) ;
#55496=CARTESIAN_POINT('Ctrl Pts',(-18.3477150281808,-40.7309129710697,
122.839629729903)) ;
#55497=CARTESIAN_POINT('Ctrl Pts',(-18.0823350469109,-40.5509238905892,
122.696568451424)) ;
#55498=CARTESIAN_POINT('Ctrl Pts',(-18.2654267208358,-40.7407686018965,
123.029802709535)) ;
#55499=CARTESIAN_POINT('Ctrl Pts',(-17.9794720035791,-40.5607795214161,
122.934283776496)) ;
#55500=CARTESIAN_POINT('Ctrl Pts',(-18.2164553752564,-40.7507680040897,
123.234201010115)) ;
#55501=CARTESIAN_POINT('Ctrl Pts',(-17.9182550887959,-40.5707789236092,
123.189781090298)) ;
#55502=CARTESIAN_POINT('Ctrl Pts',(-18.2036080978333,-40.7606624734508,
123.441855570182)) ;
#55503=CARTESIAN_POINT('Ctrl Pts',(-17.9021932200711,-40.5806733929703,
123.449349378985)) ;
#55504=CARTESIAN_POINT('Ctrl Pts',(-18.2274647702079,-40.770725587615,123.652027977728)) ;
#55505=CARTESIAN_POINT('Ctrl Pts',(-17.932011300752,-40.5907365071345,123.712065167688)) ;
#55506=CARTESIAN_POINT('Ctrl Pts',(-18.2859206509781,-40.7805652333314,
123.85049263691)) ;
#55507=CARTESIAN_POINT('Ctrl Pts',(-18.0050786318831,-40.6005761528509,
123.960147159126)) ;
#55508=CARTESIAN_POINT('Ctrl Pts',(-18.3797695061755,-40.7906284008871,
124.040064614096)) ;
#55509=CARTESIAN_POINT('Ctrl Pts',(-18.1223872399659,-40.6106393204066,
124.19711330026)) ;
#55510=CARTESIAN_POINT('Ctrl Pts',(-18.5031774126307,-40.800522656682,124.207538533751)) ;
#55511=CARTESIAN_POINT('Ctrl Pts',(-18.2766451103513,-40.6205335762015,
124.406457589714)) ;
#55512=CARTESIAN_POINT('Ctrl Pts',(-18.654084810904,-40.8104644351417,124.352107908462)) ;
#55513=CARTESIAN_POINT('Ctrl Pts',(-18.4652776965624,-40.6304753546612,
124.587171422897)) ;
#55514=CARTESIAN_POINT('Ctrl Pts',(-18.828869034011,-40.8204671279719,124.469083088964)) ;
#55515=CARTESIAN_POINT('Ctrl Pts',(-18.6837565651691,-40.6404780474914,
124.733392656357)) ;
#55516=CARTESIAN_POINT('Ctrl Pts',(-19.0220064357381,-40.8305011499257,
124.553889575478)) ;
#55517=CARTESIAN_POINT('Ctrl Pts',(-18.9251772147006,-40.6505120694452,
124.839403238466)) ;
#55518=CARTESIAN_POINT('Ctrl Pts',(-19.223072436617,-40.8403489410147,124.603257935098)) ;
#55519=CARTESIAN_POINT('Ctrl Pts',(-19.1765096235955,-40.6603598605342,
124.90111640687)) ;
#55520=CARTESIAN_POINT('Ctrl Pts',(-19.4324060765276,-40.8503304655638,
124.617611036992)) ;
#55521=CARTESIAN_POINT('Ctrl Pts',(-19.4381766703686,-40.6703413850833,
124.919060383803)) ;
#55522=CARTESIAN_POINT('Ctrl Pts',(-19.6403984022838,-40.8602796890547,
124.595436731621)) ;
#55523=CARTESIAN_POINT('Ctrl Pts',(-19.6981676205083,-40.6802906085742,
124.891345054845)) ;
#55524=CARTESIAN_POINT('Ctrl Pts',(-19.842443083507,-40.8702773452713,124.537454340177)) ;
#55525=CARTESIAN_POINT('Ctrl Pts',(-19.9507242765241,-40.6902882647908,
124.818869487643)) ;
#55526=CARTESIAN_POINT('Ctrl Pts',(-20.0319489132289,-40.8803175583263,
124.444528163005)) ;
#55527=CARTESIAN_POINT('Ctrl Pts',(-20.187607666279,-40.7003284778458,124.702714148817)) ;
#55528=CARTESIAN_POINT('Ctrl Pts',(-20.1991246682804,-40.8901456056026,
124.323088911922)) ;
#55529=CARTESIAN_POINT('Ctrl Pts',(-20.396579474449,-40.7101565251221,124.550916691175)) ;
#55530=CARTESIAN_POINT('Ctrl Pts',(-20.346201088897,-40.9001999526349,124.171290921794)) ;
#55531=CARTESIAN_POINT('Ctrl Pts',(-20.5804267073695,-40.7202108721545,
124.36117100516)) ;
#55532=CARTESIAN_POINT('Ctrl Pts',(-20.4630696212735,-40.9101410889635,
123.998019997422)) ;
#55533=CARTESIAN_POINT('Ctrl Pts',(-20.7265146725956,-40.730152008483,124.144583500133)) ;
#55534=CARTESIAN_POINT('Ctrl Pts',(-20.5483504789561,-40.9200453220432,
123.808062649806)) ;
#55535=CARTESIAN_POINT('Ctrl Pts',(-20.833118168539,-40.7400562415627,123.907137322088)) ;
#55536=CARTESIAN_POINT('Ctrl Pts',(-20.5999532572044,-40.9300920188868,
123.60326863494)) ;
#55537=CARTESIAN_POINT('Ctrl Pts',(-20.8976239888789,-40.7501029384063,
123.651145500474)) ;
#55538=CARTESIAN_POINT('Ctrl Pts',(-20.6151760608575,-40.9399875701671,
123.395757075014)) ;
#55539=CARTESIAN_POINT('Ctrl Pts',(-20.9166549331708,-40.7599984896866,
123.391755647876)) ;
#55540=CARTESIAN_POINT('Ctrl Pts',(-20.5937893271631,-40.9500496480066,
123.185334655096)) ;
#55541=CARTESIAN_POINT('Ctrl Pts',(-20.8899239297409,-40.7700605675261,
123.128727559456)) ;
#55542=CARTESIAN_POINT('Ctrl Pts',(-20.5375466139094,-40.9598923571026,
122.986176025129)) ;
#55543=CARTESIAN_POINT('Ctrl Pts',(-20.819622592751,-40.7799032766222,122.879777795648)) ;
#55544=CARTESIAN_POINT('Ctrl Pts',(-20.4466945331734,-40.9698830893411,
122.796834964654)) ;
#55545=CARTESIAN_POINT('Ctrl Pts',(-20.7060594584752,-40.7898940088606,
122.643100332415)) ;
#55546=CARTESIAN_POINT('Ctrl Pts',(-20.32506530426,-40.9798111145698,122.627205149371)) ;
#55547=CARTESIAN_POINT('Ctrl Pts',(-20.5540244826966,-40.7998220340894,
122.431061345362)) ;
#55548=CARTESIAN_POINT('Ctrl Pts',(-20.1751809243749,-40.9897992612204,
122.480136248305)) ;
#55549=CARTESIAN_POINT('Ctrl Pts',(-20.3666704075686,-40.8098101807399,
122.247223536346)) ;
#55550=CARTESIAN_POINT('Ctrl Pts',(-20.0010440003547,-40.9998342790604,
122.361035774299)) ;
#55551=CARTESIAN_POINT('Ctrl Pts',(-20.1490005901625,-40.8198451985799,
122.098346117447)) ;
#55552=CARTESIAN_POINT('Ctrl Pts',(-19.8122322682539,-41.0096990761655,
122.275263236687)) ;
#55553=CARTESIAN_POINT('Ctrl Pts',(-19.912986052844,-40.8297099956851,121.991128079495)) ;
#55554=CARTESIAN_POINT('Ctrl Pts',(-19.6095835568502,-41.0196598085217,
122.222477105135)) ;
#55555=CARTESIAN_POINT('Ctrl Pts',(-19.6596753422363,-40.8396707280412,
121.925143350188)) ;
#55556=CARTESIAN_POINT('Ctrl Pts',(-19.3993089283046,-41.0296932709187,
122.205909546878)) ;
#55557=CARTESIAN_POINT('Ctrl Pts',(-19.3968323127526,-40.8497041904382,
121.904431778366)) ;
#55558=CARTESIAN_POINT('Ctrl Pts',(-19.1923814571992,-41.0395788051301,
122.225463175371)) ;
#55559=CARTESIAN_POINT('Ctrl Pts',(-19.1381719931382,-40.8595897246496,
121.928871855483)) ;
#55560=CARTESIAN_POINT('Ctrl Pts',(-18.9884081997025,-41.0496436458101,
122.281644422525)) ;
#55561=CARTESIAN_POINT('Ctrl Pts',(-18.8832051234226,-40.8696545653296,
121.999096372835)) ;
#55562=CARTESIAN_POINT('Ctrl Pts',(-18.8013257411855,-41.0594917775389,
122.370368828685)) ;
#55563=CARTESIAN_POINT('Ctrl Pts',(-18.6493502438061,-40.8795026970585,
122.110000505637)) ;
#55564=CARTESIAN_POINT('Ctrl Pts',(-18.6291184084903,-41.0695192745291,
122.491953508965)) ;
#55565=CARTESIAN_POINT('Ctrl Pts',(-18.4340900375309,-40.8895301940486,
122.261979815377)) ;
#55566=CARTESIAN_POINT('Ctrl Pts',(-18.4810087173521,-41.0795477265741,
122.642011387807)) ;
#55567=CARTESIAN_POINT('Ctrl Pts',(-18.2489515310926,-40.8995586460937,
122.449550692896)) ;
#55568=CARTESIAN_POINT('Ctrl Pts',(-18.3630810655382,-41.0893929931382,
122.812094313911)) ;
#55569=CARTESIAN_POINT('Ctrl Pts',(-18.1015397639368,-40.9094039126578,
122.662154181668)) ;
#55570=CARTESIAN_POINT('Ctrl Pts',(-18.2746791888148,-41.0993836660792,
123.00262605961)) ;
#55571=CARTESIAN_POINT('Ctrl Pts',(-17.9910357648319,-40.9193945855987,
122.900318312465)) ;
#55572=CARTESIAN_POINT('Ctrl Pts',(-18.2209040134384,-41.1094215481676,
123.206685229747)) ;
#55573=CARTESIAN_POINT('Ctrl Pts',(-17.9238150124732,-40.9294324676872,
123.155391667979)) ;
#55574=CARTESIAN_POINT('Ctrl Pts',(-18.2033541254263,-41.1192659186073,
123.412907134102)) ;
#55575=CARTESIAN_POINT('Ctrl Pts',(-17.9018757957966,-40.9392768381268,
123.413170064838)) ;
#55576=CARTESIAN_POINT('Ctrl Pts',(-18.2217257491831,-41.1292507460027,
123.621985540264)) ;
#55577=CARTESIAN_POINT('Ctrl Pts',(-17.9248387220261,-40.9492616655222,
123.674518463703)) ;
#55578=CARTESIAN_POINT('Ctrl Pts',(-18.2757990112521,-41.139190191408,123.82385763404)) ;
#55579=CARTESIAN_POINT('Ctrl Pts',(-17.9924288978271,-40.9592011109275,
123.926859520064)) ;
#55580=CARTESIAN_POINT('Ctrl Pts',(-18.3650287174585,-41.1492301956939,
124.01511881118)) ;
#55581=CARTESIAN_POINT('Ctrl Pts',(-18.1039644975563,-40.9692411152134,
124.165936540867)) ;
#55582=CARTESIAN_POINT('Ctrl Pts',(-18.4841771963513,-41.1591173048795,
124.18546666406)) ;
#55583=CARTESIAN_POINT('Ctrl Pts',(-18.2528993473601,-40.979128224399,124.378873025841)) ;
#55584=CARTESIAN_POINT('Ctrl Pts',(-18.6325483512414,-41.169117364782,124.334363428523)) ;
#55585=CARTESIAN_POINT('Ctrl Pts',(-18.438362340865,-40.9891282843015,124.564995129855)) ;
#55586=CARTESIAN_POINT('Ctrl Pts',(-18.8030499054225,-41.1790347806967,
124.45442108235)) ;
#55587=CARTESIAN_POINT('Ctrl Pts',(-18.6514890496474,-40.9990457002162,
124.715068773003)) ;
#55588=CARTESIAN_POINT('Ctrl Pts',(-18.9942377867766,-41.1890815954375,
124.544124964319)) ;
#55589=CARTESIAN_POINT('Ctrl Pts',(-18.8904730959717,-41.009092514957,124.827199842494)) ;
#55590=CARTESIAN_POINT('Ctrl Pts',(-19.194625243992,-41.1989570726341,124.59855210773)) ;
#55591=CARTESIAN_POINT('Ctrl Pts',(-19.1409580664775,-41.0189679921537,
124.895235368281)) ;
#55592=CARTESIAN_POINT('Ctrl Pts',(-19.4051209957553,-41.2090131683554,
124.617812738333)) ;
#55593=CARTESIAN_POINT('Ctrl Pts',(-19.4040773768782,-41.0290240878749,
124.919312459518)) ;
#55594=CARTESIAN_POINT('Ctrl Pts',(-19.612431639119,-41.2189063303704,124.600588284095)) ;
#55595=CARTESIAN_POINT('Ctrl Pts',(-19.6632167072964,-41.03891724989,124.897783110664)) ;
#55596=CARTESIAN_POINT('Ctrl Pts',(-19.8169921171162,-41.228968566393,124.546802146257)) ;
#55597=CARTESIAN_POINT('Ctrl Pts',(-19.9189173139236,-41.0489794859126,
124.830551761056)) ;
#55598=CARTESIAN_POINT('Ctrl Pts',(-20.0049876675589,-41.238813032022,124.460234593198)) ;
#55599=CARTESIAN_POINT('Ctrl Pts',(-20.15391348363,-41.0588239515415,124.72234292479)) ;
#55600=CARTESIAN_POINT('Ctrl Pts',(-20.1775149384373,-41.2487731247261,
124.341583226709)) ;
#55601=CARTESIAN_POINT('Ctrl Pts',(-20.3695735132211,-41.0687840442456,
124.574029279079)) ;
#55602=CARTESIAN_POINT('Ctrl Pts',(-20.3276957983037,-41.2588114137072,
124.193333688779)) ;
#55603=CARTESIAN_POINT('Ctrl Pts',(-20.5573002808556,-41.0788223332267,
124.388718288929)) ;
#55604=CARTESIAN_POINT('Ctrl Pts',(-20.4481963084003,-41.2686847368134,
124.024285690543)) ;
#55605=CARTESIAN_POINT('Ctrl Pts',(-20.7079273848566,-41.0886956563329,
124.177407956331)) ;
#55606=CARTESIAN_POINT('Ctrl Pts',(-20.5392295552627,-41.2787579208985,
123.833127087447)) ;
#55607=CARTESIAN_POINT('Ctrl Pts',(-20.8217196877489,-41.098768840418,123.938460528992)) ;
#55608=CARTESIAN_POINT('Ctrl Pts',(-20.5945544507421,-41.2885784331864,
123.634173535179)) ;
#55609=CARTESIAN_POINT('Ctrl Pts',(-20.8908771122864,-41.1085893527059,
123.68976734053)) ;
#55610=CARTESIAN_POINT('Ctrl Pts',(-20.6152109322945,-41.2986564293022,
123.4233616068)) ;
#55611=CARTESIAN_POINT('Ctrl Pts',(-20.9166985132169,-41.1186673488217,
123.426252975596)) ;
#55612=CARTESIAN_POINT('Ctrl Pts',(-20.5993528249516,-41.3085105042855,
123.216758416183)) ;
#55613=CARTESIAN_POINT('Ctrl Pts',(-20.8968766072787,-41.128521423805,123.167997632814)) ;
#55614=CARTESIAN_POINT('Ctrl Pts',(-20.5470119355056,-41.3185743858692,
123.011801977239)) ;
#55615=CARTESIAN_POINT('Ctrl Pts',(-20.831451299186,-41.1385853053887,122.911802236361)) ;
#55616=CARTESIAN_POINT('Ctrl Pts',(-20.4613754347014,-41.3284578118429,
122.822450585418)) ;
#55617=CARTESIAN_POINT('Ctrl Pts',(-20.7244059190907,-41.1484687313624,
122.675111706998)) ;
#55618=CARTESIAN_POINT('Ctrl Pts',(-20.3430903346169,-41.338458415764,122.648681232655)) ;
#55619=CARTESIAN_POINT('Ctrl Pts',(-20.5765499861908,-41.1584693352835,
122.457899543833)) ;
#55620=CARTESIAN_POINT('Ctrl Pts',(-20.1976579653882,-41.3483782001018,
122.49916106268)) ;
#55621=CARTESIAN_POINT('Ctrl Pts',(-20.3947593961203,-41.1683891196214,
122.270998373783)) ;
#55622=CARTESIAN_POINT('Ctrl Pts',(-20.0263274877781,-41.3584255504587,
122.375678234952)) ;
#55623=CARTESIAN_POINT('Ctrl Pts',(-20.1805968422946,-41.1784364699782,
122.116644489868)) ;
#55624=CARTESIAN_POINT('Ctrl Pts',(-19.8394159318229,-41.368302892693,122.285119868391)) ;
#55625=CARTESIAN_POINT('Ctrl Pts',(-19.9469565781688,-41.1883138122125,
122.003445575587)) ;
#55626=CARTESIAN_POINT('Ctrl Pts',(-19.6358016808575,-41.3783727737676,
122.227321629888)) ;
#55627=CARTESIAN_POINT('Ctrl Pts',(-19.6924393111022,-41.1983836932871,
121.931197405143)) ;
#55628=CARTESIAN_POINT('Ctrl Pts',(-19.4302105986271,-41.3882024789693,
122.206046078144)) ;
#55629=CARTESIAN_POINT('Ctrl Pts',(-19.435448966812,-41.2082133984888,121.904602386657)) ;
#55630=CARTESIAN_POINT('Ctrl Pts',(-19.2191313622272,-41.3982691401357,
122.220859081126)) ;
#55631=CARTESIAN_POINT('Ctrl Pts',(-19.1716002965502,-41.2182800596552,
121.923118301368)) ;
#55632=CARTESIAN_POINT('Ctrl Pts',(-19.0174028500584,-41.408159362003,122.271341345919)) ;
#55633=CARTESIAN_POINT('Ctrl Pts',(-18.9194385507333,-41.2281702815225,
121.986221032295)) ;
#55634=CARTESIAN_POINT('Ctrl Pts',(-18.8253933440022,-41.4181515381132,
122.356520476582)) ;
#55635=CARTESIAN_POINT('Ctrl Pts',(-18.6794263981433,-41.2381624576327,
122.092694864997)) ;
#55636=CARTESIAN_POINT('Ctrl Pts',(-18.6517079385557,-41.4281143682258,
122.473569637497)) ;
#55637=CARTESIAN_POINT('Ctrl Pts',(-18.4623191157253,-41.2481252877453,
122.239006352162)) ;
#55638=CARTESIAN_POINT('Ctrl Pts',(-18.5014870756419,-41.4380185806261,
122.61777683837)) ;
#55639=CARTESIAN_POINT('Ctrl Pts',(-18.274542323602,-41.2580295001457,122.419265967065)) ;
#55640=CARTESIAN_POINT('Ctrl Pts',(-18.3768239906411,-41.448079294714,122.788607618059)) ;
#55641=CARTESIAN_POINT('Ctrl Pts',(-18.1187135737905,-41.2680902142335,
122.63280407958)) ;
#55642=CARTESIAN_POINT('Ctrl Pts',(-18.2854831726733,-41.4579187976968,
122.974241715456)) ;
#55643=CARTESIAN_POINT('Ctrl Pts',(-18.0045368873507,-41.2779297172163,
122.864848022224)) ;
#55644=CARTESIAN_POINT('Ctrl Pts',(-18.2262434983332,-41.4679849362632,
123.177367766874)) ;
#55645=CARTESIAN_POINT('Ctrl Pts',(-17.9304874744645,-41.2879958557827,
123.118755220522)) ;
#55646=CARTESIAN_POINT('Ctrl Pts',(-18.2036641637308,-41.4778674507492,
123.383929826508)) ;
#55647=CARTESIAN_POINT('Ctrl Pts',(-17.902263224138,-41.2978783702687,123.37695892444)) ;
#55648=CARTESIAN_POINT('Ctrl Pts',(-18.217028771755,-41.4878597501047,123.593541694944)) ;
#55649=CARTESIAN_POINT('Ctrl Pts',(-17.9189692032096,-41.3078706696243,
123.638973965521)) ;
#55650=CARTESIAN_POINT('Ctrl Pts',(-18.266354986361,-41.4978128170581,123.796921608966)) ;
#55651=CARTESIAN_POINT('Ctrl Pts',(-17.9806273075444,-41.3178237365777,
123.893199304631)) ;
#55652=CARTESIAN_POINT('Ctrl Pts',(-18.3509953062756,-41.5078475252634,
123.990141633652)) ;
#55653=CARTESIAN_POINT('Ctrl Pts',(-18.0864278198441,-41.3278584447829,
124.134724121269)) ;
#55654=CARTESIAN_POINT('Ctrl Pts',(-18.4660813786671,-41.5177357461675,
124.16327447273)) ;
#55655=CARTESIAN_POINT('Ctrl Pts',(-18.2302862076432,-41.3377466656871,
124.351140926681)) ;
#55656=CARTESIAN_POINT('Ctrl Pts',(-18.6107545882689,-41.527730169198,124.315632016027)) ;
#55657=CARTESIAN_POINT('Ctrl Pts',(-18.4111281398735,-41.3477410887175,
124.541587743856)) ;
#55658=CARTESIAN_POINT('Ctrl Pts',(-18.7789136987431,-41.5376755086441,
124.439882085286)) ;
#55659=CARTESIAN_POINT('Ctrl Pts',(-18.6213277143257,-41.3576864281637,
124.696900401457)) ;
#55660=CARTESIAN_POINT('Ctrl Pts',(-18.9659468148119,-41.5476228532555,
124.533455179256)) ;
#55661=CARTESIAN_POINT('Ctrl Pts',(-18.8551198559808,-41.367633772775,124.813866561947)) ;
#55662=CARTESIAN_POINT('Ctrl Pts',(-19.1684641307119,-41.5576707486665,
124.593501263556)) ;
#55663=CARTESIAN_POINT('Ctrl Pts',(-19.1082663812095,-41.377681668186,124.888923688679)) ;
#55664=CARTESIAN_POINT('Ctrl Pts',(-19.3741360186057,-41.5675183941458,
124.617169452633)) ;
#55665=CARTESIAN_POINT('Ctrl Pts',(-19.365357688916,-41.3875293136654,124.918508594089)) ;
#55666=CARTESIAN_POINT('Ctrl Pts',(-19.5832145971549,-41.5774801080598,
124.605278842965)) ;
#55667=CARTESIAN_POINT('Ctrl Pts',(-19.626706323974,-41.3974910275794,124.903644555779)) ;
#55668=CARTESIAN_POINT('Ctrl Pts',(-19.788383314369,-41.5875087323508,124.556678207782)) ;
#55669=CARTESIAN_POINT('Ctrl Pts',(-19.8831669773859,-41.4075196518703,
124.842893155846)) ;
#55670=CARTESIAN_POINT('Ctrl Pts',(-19.979718451431,-41.5974190930075,124.47424697805)) ;
#55671=CARTESIAN_POINT('Ctrl Pts',(-20.1223364380835,-41.417430012527,124.7398531547)) ;
#55672=CARTESIAN_POINT('Ctrl Pts',(-20.1545793968166,-41.6073537915808,
124.360016047797)) ;
#55673=CARTESIAN_POINT('Ctrl Pts',(-20.3409126900121,-41.4273647111003,
124.597063389296)) ;
#55674=CARTESIAN_POINT('Ctrl Pts',(-20.3084369890171,-41.617395616435,124.215477929178)) ;
#55675=CARTESIAN_POINT('Ctrl Pts',(-20.5332339906583,-41.4374065359545,
124.416390285441)) ;
#55676=CARTESIAN_POINT('Ctrl Pts',(-20.4330452256544,-41.6272801901794,
124.04915416565)) ;
#55677=CARTESIAN_POINT('Ctrl Pts',(-20.6889942204414,-41.4472911096989,
124.208484214662)) ;
#55678=CARTESIAN_POINT('Ctrl Pts',(-20.5281974762761,-41.6372820395426,
123.861676921121)) ;
#55679=CARTESIAN_POINT('Ctrl Pts',(-20.80793373482,-41.4572929590621,123.974137087528)) ;
#55680=CARTESIAN_POINT('Ctrl Pts',(-20.5890105169507,-41.6472013411166,
123.662177464747)) ;
#55681=CARTESIAN_POINT('Ctrl Pts',(-20.8839492758714,-41.4672122606361,
123.724761737234)) ;
#55682=CARTESIAN_POINT('Ctrl Pts',(-20.6145770333962,-41.6572454494619,
123.452589429869)) ;
#55683=CARTESIAN_POINT('Ctrl Pts',(-20.9159063785806,-41.4772563689814,
123.46277677981)) ;
#55684=CARTESIAN_POINT('Ctrl Pts',(-20.6036034057865,-41.6671298729041,
123.245068543956)) ;
#55685=CARTESIAN_POINT('Ctrl Pts',(-20.9021882406929,-41.4871407924237,
123.203374700065)) ;
#55686=CARTESIAN_POINT('Ctrl Pts',(-20.5565952979151,-41.6771462348136,
123.039799079144)) ;
#55687=CARTESIAN_POINT('Ctrl Pts',(-20.8434269169857,-41.4971571543331,
122.946788139625)) ;
#55688=CARTESIAN_POINT('Ctrl Pts',(-20.4739898693975,-41.687182890319,122.845651147378)) ;
#55689=CARTESIAN_POINT('Ctrl Pts',(-20.7401692464129,-41.5071938098385,
122.704103736614)) ;
#55690=CARTESIAN_POINT('Ctrl Pts',(-20.3617495143391,-41.6970130205083,
122.672097956593)) ;
#55691=CARTESIAN_POINT('Ctrl Pts',(-20.599866997002,-41.5170239400278,122.487161714405)) ;
#55692=CARTESIAN_POINT('Ctrl Pts',(-20.2176578236803,-41.7070890735982,
122.516880089597)) ;
#55693=CARTESIAN_POINT('Ctrl Pts',(-20.4197517581915,-41.5270999931177,
122.293140546941)) ;
#55694=CARTESIAN_POINT('Ctrl Pts',(-20.0525570282774,-41.716941302784,122.391738375316)) ;
#55695=CARTESIAN_POINT('Ctrl Pts',(-20.2133740002542,-41.5369522223035,
122.136713686514)) ;
#55696=CARTESIAN_POINT('Ctrl Pts',(-19.864251762106,-41.7270145105833,122.294921019345)) ;
#55697=CARTESIAN_POINT('Ctrl Pts',(-19.9779921556695,-41.5470254301028,
122.015693380186)) ;
#55698=CARTESIAN_POINT('Ctrl Pts',(-19.666587072999,-41.7368560219347,122.233752490588)) ;
#55699=CARTESIAN_POINT('Ctrl Pts',(-19.7309096531078,-41.5568669414542,
121.93923360609)) ;
#55700=CARTESIAN_POINT('Ctrl Pts',(-19.458933216277,-41.7468169599722,122.206739976442)) ;
#55701=CARTESIAN_POINT('Ctrl Pts',(-19.4713417220733,-41.5668278794917,
121.905469506016)) ;
#55702=CARTESIAN_POINT('Ctrl Pts',(-19.2481470392033,-41.7568548218972,
122.21668888155)) ;
#55703=CARTESIAN_POINT('Ctrl Pts',(-19.207859203209,-41.5768657414167,121.917907090577)) ;
#55704=CARTESIAN_POINT('Ctrl Pts',(-19.0455303660746,-41.7667290078943,
122.261958044375)) ;
#55705=CARTESIAN_POINT('Ctrl Pts',(-18.9545877189541,-41.5867399274138,
121.974495320548)) ;
#55706=CARTESIAN_POINT('Ctrl Pts',(-18.8501065214671,-41.7767991674721,
122.343300097971)) ;
#55707=CARTESIAN_POINT('Ctrl Pts',(-18.7103088482893,-41.5968100869917,
122.07617421899)) ;
#55708=CARTESIAN_POINT('Ctrl Pts',(-18.675884913286,-41.786630914898,122.454554501871)) ;
#55709=CARTESIAN_POINT('Ctrl Pts',(-18.4925316285938,-41.6066418344175,
122.215244290356)) ;
#55710=CARTESIAN_POINT('Ctrl Pts',(-18.5201147053539,-41.7966669949693,
122.596849719958)) ;
#55711=CARTESIAN_POINT('Ctrl Pts',(-18.2978201732453,-41.6166779144888,
122.393114575254)) ;
#55712=CARTESIAN_POINT('Ctrl Pts',(-18.3920704361308,-41.8066840418218,
122.764054383414)) ;
#55713=CARTESIAN_POINT('Ctrl Pts',(-18.1377661290135,-41.6266949613413,
122.602121409318)) ;
#55714=CARTESIAN_POINT('Ctrl Pts',(-18.2959657375201,-41.8165662999884,
122.948249336601)) ;
#55715=CARTESIAN_POINT('Ctrl Pts',(-18.0176363962618,-41.6365772195079,
122.832366722308)) ;
#55716=CARTESIAN_POINT('Ctrl Pts',(-18.2324121268901,-41.8265539827847,
123.148349956058)) ;
#55717=CARTESIAN_POINT('Ctrl Pts',(-17.9381960767732,-41.6465649023042,
123.082493245749)) ;
#55718=CARTESIAN_POINT('Ctrl Pts',(-18.2045073332423,-41.8365006395015,
123.355622216733)) ;
#55719=CARTESIAN_POINT('Ctrl Pts',(-17.9033168940831,-41.656511559021,123.341584277099)) ;
#55720=CARTESIAN_POINT('Ctrl Pts',(-18.2133253026657,-41.8465576975816,
123.566846105413)) ;
#55721=CARTESIAN_POINT('Ctrl Pts',(-17.9143411681088,-41.6665686171012,
123.605613842776)) ;
#55722=CARTESIAN_POINT('Ctrl Pts',(-18.2573346938639,-41.8563758771311,
123.768519750159)) ;
#55723=CARTESIAN_POINT('Ctrl Pts',(-17.9693550453848,-41.6763867966506,
123.857706729718)) ;
#55724=CARTESIAN_POINT('Ctrl Pts',(-18.3368951497359,-41.86641181157,123.963925455045)) ;
#55725=CARTESIAN_POINT('Ctrl Pts',(-18.068807500374,-41.6864227310896,124.101962974052)) ;
#55726=CARTESIAN_POINT('Ctrl Pts',(-18.449568449613,-41.876436465999,124.142036436665)) ;
#55727=CARTESIAN_POINT('Ctrl Pts',(-18.2096507193238,-41.6964473855186,
124.3246006639)) ;
#55728=CARTESIAN_POINT('Ctrl Pts',(-18.5886702041934,-41.8862884855786,
124.295499146271)) ;
#55729=CARTESIAN_POINT('Ctrl Pts',(-18.3835301011167,-41.7062994050981,
124.516428432914)) ;
#55730=CARTESIAN_POINT('Ctrl Pts',(-18.7543933359487,-41.8962793992935,
124.424504024787)) ;
#55731=CARTESIAN_POINT('Ctrl Pts',(-18.5906854587006,-41.716290318813,124.677682956572)) ;
#55732=CARTESIAN_POINT('Ctrl Pts',(-18.9386244083252,-41.9061973881331,
124.522200361594)) ;
#55733=CARTESIAN_POINT('Ctrl Pts',(-18.8209758180586,-41.7262083076526,
124.79980173712)) ;
#55734=CARTESIAN_POINT('Ctrl Pts',(-19.1391682617768,-41.9162254988639,
124.587172771734)) ;
#55735=CARTESIAN_POINT('Ctrl Pts',(-19.0716562720862,-41.7362364183834,
124.881015168382)) ;
#55736=CARTESIAN_POINT('Ctrl Pts',(-19.3449799514909,-41.9261106967723,
124.616011040742)) ;
#55737=CARTESIAN_POINT('Ctrl Pts',(-19.3289219205391,-41.7461216162918,
124.917060930375)) ;
#55738=CARTESIAN_POINT('Ctrl Pts',(-19.554878431118,-41.9360999720403,124.609111482474)) ;
#55739=CARTESIAN_POINT('Ctrl Pts',(-19.5912951011794,-41.7561108915598,
124.908434150223)) ;
#55740=CARTESIAN_POINT('Ctrl Pts',(-19.7613596240019,-41.9461414302098,
124.565200707997)) ;
#55741=CARTESIAN_POINT('Ctrl Pts',(-19.8493960391262,-41.7661523497293,
124.853543537103)) ;
#55742=CARTESIAN_POINT('Ctrl Pts',(-19.9531398235918,-41.9559728939981,
124.48810716658)) ;
#55743=CARTESIAN_POINT('Ctrl Pts',(-20.0891213276599,-41.7759838135176,
124.757174105062)) ;
#55744=CARTESIAN_POINT('Ctrl Pts',(-20.1319364909177,-41.965977826302,124.377372382878)) ;
#55745=CARTESIAN_POINT('Ctrl Pts',(-20.3126159522147,-41.7859887458215,
124.618753527422)) ;
#55746=CARTESIAN_POINT('Ctrl Pts',(-20.2884681065489,-41.9759641901967,
124.237408278261)) ;
#55747=CARTESIAN_POINT('Ctrl Pts',(-20.5082790001988,-41.7959751097162,
124.443796511025)) ;
#55748=CARTESIAN_POINT('Ctrl Pts',(-20.4187181316533,-41.9859938190826,
124.071617468983)) ;
#55749=CARTESIAN_POINT('Ctrl Pts',(-20.6710896621926,-41.8060047386021,
124.236556568629)) ;
#55750=CARTESIAN_POINT('Ctrl Pts',(-20.5169261211042,-41.995869041191,123.888684071241)) ;
#55751=CARTESIAN_POINT('Ctrl Pts',(-20.7938478465005,-41.8158799607105,
124.00788808418)) ;
#55752=CARTESIAN_POINT('Ctrl Pts',(-20.5829278692201,-42.0058702535881,
123.689089793923)) ;
#55753=CARTESIAN_POINT('Ctrl Pts',(-20.8763477235606,-41.8258811731076,
123.7583943576)) ;
#55754=CARTESIAN_POINT('Ctrl Pts',(-20.6131956145041,-42.0157788328236,
123.482954015089)) ;
#55755=CARTESIAN_POINT('Ctrl Pts',(-20.9141799976417,-41.8357897523431,
123.500723797935)) ;
#55756=CARTESIAN_POINT('Ctrl Pts',(-20.6070613238518,-42.0258336853796,
123.271692586383)) ;
#55757=CARTESIAN_POINT('Ctrl Pts',(-20.9065096444975,-41.8458446048991,
123.236647196721)) ;
#55758=CARTESIAN_POINT('Ctrl Pts',(-20.5653915462767,-42.0356922676544,
123.068629174948)) ;
#55759=CARTESIAN_POINT('Ctrl Pts',(-20.8544198066431,-41.8557031871739,
122.982817801533)) ;
#55760=CARTESIAN_POINT('Ctrl Pts',(-20.4876191246396,-42.0457603970971,
122.871804464288)) ;
#55761=CARTESIAN_POINT('Ctrl Pts',(-20.7572019523973,-41.8657713166166,
122.736787999736)) ;
#55762=CARTESIAN_POINT('Ctrl Pts',(-20.3791532075603,-42.0556158687862,
122.695250592433)) ;
#55763=CARTESIAN_POINT('Ctrl Pts',(-20.621617047781,-41.8756267883057,122.516096462786)) ;
#55764=CARTESIAN_POINT('Ctrl Pts',(-20.2402233414134,-42.0656107171724,
122.53762013048)) ;
#55765=CARTESIAN_POINT('Ctrl Pts',(-20.4479526499224,-41.885621636692,122.319060072896)) ;
#55766=CARTESIAN_POINT('Ctrl Pts',(-20.0751431990478,-42.0756420139569,
122.406377183477)) ;
#55767=CARTESIAN_POINT('Ctrl Pts',(-20.241600860063,-41.8956529334764,122.155008415633)) ;
#55768=CARTESIAN_POINT('Ctrl Pts',(-19.8929827389423,-42.085508550167,122.307151426831)) ;
#55769=CARTESIAN_POINT('Ctrl Pts',(-20.0138985647374,-41.9055194696865,
122.030978291762)) ;
#55770=CARTESIAN_POINT('Ctrl Pts',(-19.6940889865307,-42.0954959731278,
122.239940435497)) ;
#55771=CARTESIAN_POINT('Ctrl Pts',(-19.7652803950309,-41.9155068926473,
121.946967065322)) ;
#55772=CARTESIAN_POINT('Ctrl Pts',(-19.4873935007549,-42.1054409121476,
122.208304514953)) ;
#55773=CARTESIAN_POINT('Ctrl Pts',(-19.5069103967473,-41.9254518316671,
121.907424800085)) ;
#55774=CARTESIAN_POINT('Ctrl Pts',(-19.2762891943971,-42.1154857980076,
122.213185852874)) ;
#55775=CARTESIAN_POINT('Ctrl Pts',(-19.2430300937624,-41.9354967175271,
121.91352916489)) ;
#55776=CARTESIAN_POINT('Ctrl Pts',(-19.0728324499465,-42.1253543330938,
122.253813361827)) ;
#55777=CARTESIAN_POINT('Ctrl Pts',(-18.9887092821394,-41.9453652526133,
121.96431628744)) ;
#55778=CARTESIAN_POINT('Ctrl Pts',(-18.877416228865,-42.1353202011005,122.329344157201)) ;
#55779=CARTESIAN_POINT('Ctrl Pts',(-18.7444398717798,-41.95533112062,122.058732417951)) ;
#55780=CARTESIAN_POINT('Ctrl Pts',(-18.697163938135,-42.145342848553,122.438490697059)) ;
#55781=CARTESIAN_POINT('Ctrl Pts',(-18.5191258959242,-41.9653537680725,
122.195167959674)) ;
#55782=CARTESIAN_POINT('Ctrl Pts',(-18.5401483686295,-42.1552664875606,
122.575845813976)) ;
#55783=CARTESIAN_POINT('Ctrl Pts',(-18.322858065657,-41.9752774070801,122.366864085167)) ;
#55784=CARTESIAN_POINT('Ctrl Pts',(-18.408710854997,-42.1652092125663,122.738393134439)) ;
#55785=CARTESIAN_POINT('Ctrl Pts',(-18.1585632395934,-41.9852201320858,
122.570050124057)) ;
#55786=CARTESIAN_POINT('Ctrl Pts',(-18.3066794566052,-42.1752548186182,
122.92328748586)) ;
#55787=CARTESIAN_POINT('Ctrl Pts',(-18.0310264115202,-41.9952657381377,
122.80116942056)) ;
#55788=CARTESIAN_POINT('Ctrl Pts',(-18.2393302313391,-42.1851162411393,
123.119379879712)) ;
#55789=CARTESIAN_POINT('Ctrl Pts',(-17.9468424316427,-42.0051271606588,
123.046286075505)) ;
#55790=CARTESIAN_POINT('Ctrl Pts',(-18.2062726029867,-42.1951098095885,
123.32682877589)) ;
#55791=CARTESIAN_POINT('Ctrl Pts',(-17.9055231592109,-42.015120729108,123.305597710678)) ;
#55792=CARTESIAN_POINT('Ctrl Pts',(-18.2096058519718,-42.2050352803438,
123.53549760296)) ;
#55793=CARTESIAN_POINT('Ctrl Pts',(-17.9096925517523,-42.0250461998633,
123.5664338487)) ;
#55794=CARTESIAN_POINT('Ctrl Pts',(-18.2495067475796,-42.2150629542996,
123.742474063571)) ;
#55795=CARTESIAN_POINT('Ctrl Pts',(-17.9595713837686,-42.0350738738192,
123.825153894816)) ;
#55796=CARTESIAN_POINT('Ctrl Pts',(-18.3235158516873,-42.2249501323413,
123.936741246355)) ;
#55797=CARTESIAN_POINT('Ctrl Pts',(-18.0520856875413,-42.0449610518609,
124.067987197566)) ;
#55798=CARTESIAN_POINT('Ctrl Pts',(-18.4314996605536,-42.2349785117095,
124.117783872996)) ;
#55799=CARTESIAN_POINT('Ctrl Pts',(-18.1870669886483,-42.054989431229,124.294288291793)) ;
#55800=CARTESIAN_POINT('Ctrl Pts',(-18.5673819663472,-42.244872754431,124.27530549087)) ;
#55801=CARTESIAN_POINT('Ctrl Pts',(-18.3569254895816,-42.0648836739505,
124.49119150411)) ;
#55802=CARTESIAN_POINT('Ctrl Pts',(-18.784709731541,-42.2582256710819,124.452982254129)) ;
#55803=CARTESIAN_POINT('Ctrl Pts',(-18.6285705557097,-42.0782365906014,
124.71326978059)) ;
#55804=CARTESIAN_POINT('Ctrl Pts',(-19.0405785225545,-42.2714281888286,
124.568605528917)) ;
#55805=CARTESIAN_POINT('Ctrl Pts',(-18.9483775262258,-42.0914391083481,
124.857795814355)) ;
#55806=CARTESIAN_POINT('Ctrl Pts',(-19.3175485571435,-42.2847840941096,
124.614299554858)) ;
#55807=CARTESIAN_POINT('Ctrl Pts',(-19.294644250491,-42.1047950136291,124.91492401597)) ;
#55808=CARTESIAN_POINT('Ctrl Pts',(-19.5256323724528,-42.2946807427474,
124.612199384341)) ;
#55809=CARTESIAN_POINT('Ctrl Pts',(-19.5547381910791,-42.1146916622669,
124.912293117335)) ;
#55810=CARTESIAN_POINT('Ctrl Pts',(-19.7332792605488,-42.3047288807999,
124.573491321626)) ;
#55811=CARTESIAN_POINT('Ctrl Pts',(-19.8142993016721,-42.1247398003194,
124.86390602364)) ;
#55812=CARTESIAN_POINT('Ctrl Pts',(-19.9279820672216,-42.3146198409776,
124.500461827482)) ;
#55813=CARTESIAN_POINT('Ctrl Pts',(-20.057675936975,-42.1346307604971,124.772616402216)) ;
#55814=CARTESIAN_POINT('Ctrl Pts',(-20.1091567639837,-42.3246126768544,
124.394101946924)) ;
#55815=CARTESIAN_POINT('Ctrl Pts',(-20.2841432704492,-42.1446235963739,
124.639664036503)) ;
#55816=CARTESIAN_POINT('Ctrl Pts',(-20.2695244297562,-42.334651771856,124.256910080624)) ;
#55817=CARTESIAN_POINT('Ctrl Pts',(-20.4846006079943,-42.1546626913755,
124.468172605397)) ;
#55818=CARTESIAN_POINT('Ctrl Pts',(-20.4013315978798,-42.3444891277071,
124.097515807606)) ;
#55819=CARTESIAN_POINT('Ctrl Pts',(-20.6493590679593,-42.1645000472267,
124.268925825714)) ;
#55820=CARTESIAN_POINT('Ctrl Pts',(-20.5404892382136,-42.3578820756379,
123.852779647777)) ;
#55821=CARTESIAN_POINT('Ctrl Pts',(-20.8232941425912,-42.1778929951574,
123.963015567239)) ;
#55822=CARTESIAN_POINT('Ctrl Pts',(-20.6114090444013,-42.3710487520648,
123.581847669317)) ;
#55823=CARTESIAN_POINT('Ctrl Pts',(-20.9119427188423,-42.1910596715843,
123.624389608254)) ;
#55824=CARTESIAN_POINT('Ctrl Pts',(-20.6101088531211,-42.3844335334716,
123.300551825487)) ;
#55825=CARTESIAN_POINT('Ctrl Pts',(-20.9103198256763,-42.2044444529911,
123.272710611939)) ;
#55826=CARTESIAN_POINT('Ctrl Pts',(-20.5732425145346,-42.3942953161154,
123.096486655904)) ;
#55827=CARTESIAN_POINT('Ctrl Pts',(-20.8642332431022,-42.214306235635,123.017641919717)) ;
#55828=CARTESIAN_POINT('Ctrl Pts',(-20.5008532734841,-42.4042944640685,
122.899177214063)) ;
#55829=CARTESIAN_POINT('Ctrl Pts',(-20.7737441305226,-42.224305383588,122.77100264939)) ;
#55830=CARTESIAN_POINT('Ctrl Pts',(-20.3964434183661,-42.4141972566856,
122.719010769963)) ;
#55831=CARTESIAN_POINT('Ctrl Pts',(-20.6432311628392,-42.2342081762051,
122.545797674163)) ;
#55832=CARTESIAN_POINT('Ctrl Pts',(-20.2603721575889,-42.4242468365765,
122.5574632317)) ;
#55833=CARTESIAN_POINT('Ctrl Pts',(-20.4731343578492,-42.244257756096,122.343862138609)) ;
#55834=CARTESIAN_POINT('Ctrl Pts',(-20.0479239998599,-42.437433910386,122.379158143776)) ;
#55835=CARTESIAN_POINT('Ctrl Pts',(-20.2076003348036,-42.2574448299055,
122.120995609412)) ;
#55836=CARTESIAN_POINT('Ctrl Pts',(-19.7251865030468,-42.4541867003572,
122.228834167967)) ;
#55837=CARTESIAN_POINT('Ctrl Pts',(-19.804126587439,-42.2741976198767,121.9330813858)) ;
#55838=CARTESIAN_POINT('Ctrl Pts',(-19.3757249735959,-42.4706753524519,
122.198219597745)) ;
#55839=CARTESIAN_POINT('Ctrl Pts',(-19.3673812946773,-42.2906862719714,
121.894819463327)) ;
#55840=CARTESIAN_POINT('Ctrl Pts',(-19.0992014727295,-42.4840321786353,
122.246369143376)) ;
#55841=CARTESIAN_POINT('Ctrl Pts',(-19.0216618584567,-42.3040430981548,
121.955010873832)) ;
#55842=CARTESIAN_POINT('Ctrl Pts',(-18.9034559148771,-42.4939285635132,
122.317028660144)) ;
#55843=CARTESIAN_POINT('Ctrl Pts',(-18.7769948828561,-42.3139394830327,
122.043336388444)) ;
#55844=CARTESIAN_POINT('Ctrl Pts',(-18.7209921103284,-42.5039350780337,
122.42160568978)) ;
#55845=CARTESIAN_POINT('Ctrl Pts',(-18.5489107992119,-42.3239459975532,
122.174062497267)) ;
#55846=CARTESIAN_POINT('Ctrl Pts',(-18.5074778701341,-42.5171252015501,
122.598716946262)) ;
#55847=CARTESIAN_POINT('Ctrl Pts',(-18.2820313954693,-42.3371361210696,
122.395439854776)) ;
#55848=CARTESIAN_POINT('Ctrl Pts',(-18.3017330813565,-42.5338917626996,
122.889684627251)) ;
#55849=CARTESIAN_POINT('Ctrl Pts',(-18.0248416305318,-42.3539026822191,
122.759167368691)) ;
#55850=CARTESIAN_POINT('Ctrl Pts',(-18.1906918477385,-42.5536762514077,
123.295564658477)) ;
#55851=CARTESIAN_POINT('Ctrl Pts',(-17.886048514908,-42.3736871709272,123.266512292197)) ;
#55852=CARTESIAN_POINT('Ctrl Pts',(-18.2237744744841,-42.5736216990041,
123.718259239701)) ;
#55853=CARTESIAN_POINT('Ctrl Pts',(-17.9274046619368,-42.3936326185237,
123.794881012017)) ;
#55854=CARTESIAN_POINT('Ctrl Pts',(-18.3992319347338,-42.5935333611601,
124.103576998798)) ;
#55855=CARTESIAN_POINT('Ctrl Pts',(-18.1467300051219,-42.4135442806796,
124.276525573087)) ;
#55856=CARTESIAN_POINT('Ctrl Pts',(-18.6947270079494,-42.6134255531789,
124.406289323311)) ;
#55857=CARTESIAN_POINT('Ctrl Pts',(-18.5161004762394,-42.4334364726985,
124.654913018596)) ;
#55858=CARTESIAN_POINT('Ctrl Pts',(-19.078800891227,-42.6334666837336,124.590739441501)) ;
#55859=CARTESIAN_POINT('Ctrl Pts',(-18.996194781245,-42.4534776032531,124.885472692746)) ;
#55860=CARTESIAN_POINT('Ctrl Pts',(-19.4981893983463,-42.6532850183492,
124.632822667758)) ;
#55861=CARTESIAN_POINT('Ctrl Pts',(-19.5204288936221,-42.4732959378687,
124.938073342143)) ;
#55862=CARTESIAN_POINT('Ctrl Pts',(-19.9098714360872,-42.6732575835688,
124.529182144137)) ;
#55863=CARTESIAN_POINT('Ctrl Pts',(-20.0350303911881,-42.4932685030883,
124.808520139821)) ;
#55864=CARTESIAN_POINT('Ctrl Pts',(-20.2603190889311,-42.6931467997404,
124.292190471673)) ;
#55865=CARTESIAN_POINT('Ctrl Pts',(-20.4730875844101,-42.5131577192599,
124.512279231806)) ;
#55866=CARTESIAN_POINT('Ctrl Pts',(-20.5101445680897,-42.7131703740631,
123.947568704461)) ;
#55867=CARTESIAN_POINT('Ctrl Pts',(-20.7853676286801,-42.5331812935826,
124.081500341505)) ;
#55868=CARTESIAN_POINT('Ctrl Pts',(-20.6263908959112,-42.7329675371513,
123.542918161152)) ;
#55869=CARTESIAN_POINT('Ctrl Pts',(-20.9306728528494,-42.5529784566708,
123.575689148458)) ;
#55870=CARTESIAN_POINT('Ctrl Pts',(-20.5983617331869,-42.7529330309751,
123.119413546413)) ;
#55871=CARTESIAN_POINT('Ctrl Pts',(-20.8956352698519,-42.5729439504946,
123.046309019431)) ;
#55872=CARTESIAN_POINT('Ctrl Pts',(-20.4270355343715,-42.7728867387165,
122.731150195956)) ;
#55873=CARTESIAN_POINT('Ctrl Pts',(-20.6814765721563,-42.592897658236,122.560980844295)) ;
#55874=CARTESIAN_POINT('Ctrl Pts',(-20.1343395660946,-42.7927941154431,
122.425505425646)) ;
#55875=CARTESIAN_POINT('Ctrl Pts',(-20.3156068295359,-42.6128050349627,
122.178926648433)) ;
#55876=CARTESIAN_POINT('Ctrl Pts',(-19.7563159918193,-42.8126463269917,
122.237523332506)) ;
#55877=CARTESIAN_POINT('Ctrl Pts',(-19.8430795029076,-42.6326572465112,
121.943950043666)) ;
#55878=CARTESIAN_POINT('Ctrl Pts',(-19.3322246512801,-42.8327187139374,
122.189721479614)) ;
#55879=CARTESIAN_POINT('Ctrl Pts',(-19.3129641321296,-42.6527296334569,
121.884197616029)) ;
#55880=CARTESIAN_POINT('Ctrl Pts',(-18.9222367590498,-42.8525565835777,
122.288891061449)) ;
#55881=CARTESIAN_POINT('Ctrl Pts',(-18.800481895984,-42.6725675030972,122.008159119898)) ;
#55882=CARTESIAN_POINT('Ctrl Pts',(-18.5694696067115,-42.8724072381308,
122.520633431099)) ;
#55883=CARTESIAN_POINT('Ctrl Pts',(-18.3595239814835,-42.6924181576503,
122.297834684981)) ;
#55884=CARTESIAN_POINT('Ctrl Pts',(-18.314918147968,-42.8924591724712,122.862621733189)) ;
#55885=CARTESIAN_POINT('Ctrl Pts',(-18.0413332376484,-42.7124700919908,
122.725319925663)) ;
#55886=CARTESIAN_POINT('Ctrl Pts',(-18.1937042551041,-42.9122923600373,
123.266633949038)) ;
#55887=CARTESIAN_POINT('Ctrl Pts',(-17.8898151800707,-42.7323032795568,
123.230332622444)) ;
#55888=CARTESIAN_POINT('Ctrl Pts',(-18.2168953535135,-42.932221572268,123.689590915752)) ;
#55889=CARTESIAN_POINT('Ctrl Pts',(-17.9188018273465,-42.7522324917875,
123.759028000048)) ;
#55890=CARTESIAN_POINT('Ctrl Pts',(-18.382321733306,-42.9521065374824,124.078869953119)) ;
#55891=CARTESIAN_POINT('Ctrl Pts',(-18.1255818944321,-42.7721174570019,
124.245626671934)) ;
#55892=CARTESIAN_POINT('Ctrl Pts',(-18.6737062137308,-42.972180278627,124.390635608847)) ;
#55893=CARTESIAN_POINT('Ctrl Pts',(-18.489811290908,-42.7921911981465,124.635336040402)) ;
#55894=CARTESIAN_POINT('Ctrl Pts',(-19.0487871348763,-42.9919734604074,
124.581662444527)) ;
#55895=CARTESIAN_POINT('Ctrl Pts',(-18.958659155968,-42.8119843799269,124.874120892294)) ;
#55896=CARTESIAN_POINT('Ctrl Pts',(-19.4698565957341,-43.0119361684101,
124.634936091618)) ;
#55897=CARTESIAN_POINT('Ctrl Pts',(-19.4849952307128,-42.8319470879296,
124.940716397795)) ;
#55898=CARTESIAN_POINT('Ctrl Pts',(-19.88406254428,-43.0319191201525,124.540216705959)) ;
#55899=CARTESIAN_POINT('Ctrl Pts',(-20.0027532085991,-42.851930039672,124.822320272926)) ;
#55900=CARTESIAN_POINT('Ctrl Pts',(-20.2384793849242,-43.0517297399247,
124.312505833384)) ;
#55901=CARTESIAN_POINT('Ctrl Pts',(-20.4457748040066,-42.8717406594442,
124.537685736339)) ;
#55902=CARTESIAN_POINT('Ctrl Pts',(-20.4964670998854,-43.0717134559576,
123.975002267441)) ;
#55903=CARTESIAN_POINT('Ctrl Pts',(-20.7682626056657,-42.8917243754771,
124.115808826953)) ;
#55904=CARTESIAN_POINT('Ctrl Pts',(-20.6231390461281,-43.0915949198549,
123.571582193787)) ;
#55905=CARTESIAN_POINT('Ctrl Pts',(-20.9266062654661,-42.9116058393744,
123.611535793627)) ;
#55906=CARTESIAN_POINT('Ctrl Pts',(-20.6047789342682,-43.1115502496993,
123.147760811554)) ;
#55907=CARTESIAN_POINT('Ctrl Pts',(-20.9036603574372,-42.9315611692188,
123.081759157325)) ;
#55908=CARTESIAN_POINT('Ctrl Pts',(-20.4437676887391,-43.1314257105047,
122.756956257546)) ;
#55909=CARTESIAN_POINT('Ctrl Pts',(-20.7024014512796,-42.9514366300243,
122.593252469654)) ;
#55910=CARTESIAN_POINT('Ctrl Pts',(-20.1577658156796,-43.1514100305563,
122.442758918448)) ;
#55911=CARTESIAN_POINT('Ctrl Pts',(-20.3449003202566,-42.9714209500758,
122.200502446531)) ;
#55912=CARTESIAN_POINT('Ctrl Pts',(-19.7825309062967,-43.1713380633459,
122.245718411537)) ;
#55913=CARTESIAN_POINT('Ctrl Pts',(-19.8758679529114,-42.9913489828654,
121.954198379395)) ;
#55914=CARTESIAN_POINT('Ctrl Pts',(-19.4327161765644,-43.1879468252857,
122.19803250865)) ;
#55915=CARTESIAN_POINT('Ctrl Pts',(-19.4385731677958,-43.0079577448052,
121.894584975443)) ;
#55916=CARTESIAN_POINT('Ctrl Pts',(-19.1575751517247,-43.2011344639758,
122.232458878335)) ;
#55917=CARTESIAN_POINT('Ctrl Pts',(-19.0946716816628,-43.0211453834953,
121.937615802905)) ;
#55918=CARTESIAN_POINT('Ctrl Pts',(-18.9568164762122,-43.2111208983359,
122.29383159449)) ;
#55919=CARTESIAN_POINT('Ctrl Pts',(-18.843715306556,-43.0311318178554,122.014331379883)) ;
#55920=CARTESIAN_POINT('Ctrl Pts',(-18.7693989059073,-43.2211302722953,
122.389560213479)) ;
#55921=CARTESIAN_POINT('Ctrl Pts',(-18.609452700806,-43.0411411918148,122.133980200338)) ;
#55922=CARTESIAN_POINT('Ctrl Pts',(-18.5463444276645,-43.2344203058605,
122.557741103274)) ;
#55923=CARTESIAN_POINT('Ctrl Pts',(-18.3305857335314,-43.05443122538,122.34425230643)) ;
#55924=CARTESIAN_POINT('Ctrl Pts',(-18.3288675857434,-43.251014293523,122.835683924907)) ;
#55925=CARTESIAN_POINT('Ctrl Pts',(-18.0587919010383,-43.0710252130425,
122.691613440042)) ;
#55926=CARTESIAN_POINT('Ctrl Pts',(-18.2190954075611,-43.2676465487985,
123.171796668551)) ;
#55927=CARTESIAN_POINT('Ctrl Pts',(-17.9215463022561,-43.087657468318,123.111805423973)) ;
#55928=CARTESIAN_POINT('Ctrl Pts',(-18.2039836097742,-43.2808889324664,
123.449819348037)) ;
#55929=CARTESIAN_POINT('Ctrl Pts',(-17.9026645541855,-43.1008998519859,
123.459298795029)) ;
#55930=CARTESIAN_POINT('Ctrl Pts',(-18.2283482509571,-43.2908031406938,
123.656820558235)) ;
#55931=CARTESIAN_POINT('Ctrl Pts',(-17.9331154382768,-43.1108140602133,
123.718057560314)) ;
#55932=CARTESIAN_POINT('Ctrl Pts',(-18.289369033941,-43.3008597799655,123.85923089601)) ;
#55933=CARTESIAN_POINT('Ctrl Pts',(-18.0093888246454,-43.120870699485,123.971069080762)) ;
#55934=CARTESIAN_POINT('Ctrl Pts',(-18.382402147398,-43.3107055863856,124.044152684337)) ;
#55935=CARTESIAN_POINT('Ctrl Pts',(-18.1256798999717,-43.1307165059051,
124.202224696527)) ;
#55936=CARTESIAN_POINT('Ctrl Pts',(-18.5083351564249,-43.3207505860188,
124.213670912525)) ;
#55937=CARTESIAN_POINT('Ctrl Pts',(-18.2830849969303,-43.1407615055383,
124.414117164606)) ;
#55938=CARTESIAN_POINT('Ctrl Pts',(-18.7114677451612,-43.3340316083915,
124.405150502509)) ;
#55939=CARTESIAN_POINT('Ctrl Pts',(-18.53704325182,-43.1540425279111,124.653504054392)) ;
#55940=CARTESIAN_POINT('Ctrl Pts',(-18.9580635205512,-43.3472290549162,
124.539134994554)) ;
#55941=CARTESIAN_POINT('Ctrl Pts',(-18.8452649772685,-43.1672399744357,
124.820961905395)) ;
#55942=CARTESIAN_POINT('Ctrl Pts',(-19.232360254932,-43.3606433527231,124.60475396977)) ;
#55943=CARTESIAN_POINT('Ctrl Pts',(-19.1881152199753,-43.1806542722426,
124.902985566176)) ;
#55944=CARTESIAN_POINT('Ctrl Pts',(-19.4388332017117,-43.3704824181259,
124.617341847239)) ;
#55945=CARTESIAN_POINT('Ctrl Pts',(-19.4462101896793,-43.1904933376454,
124.918723959534)) ;
#55946=CARTESIAN_POINT('Ctrl Pts',(-19.6473989067929,-43.3804656244036,
124.594097451494)) ;
#55947=CARTESIAN_POINT('Ctrl Pts',(-19.7069166424804,-43.2004765439231,
124.889671061008)) ;
#55948=CARTESIAN_POINT('Ctrl Pts',(-19.8481271767385,-43.3904168593164,
124.535103924099)) ;
#55949=CARTESIAN_POINT('Ctrl Pts',(-19.9578281238951,-43.2104277788359,
124.815931888834)) ;
#55950=CARTESIAN_POINT('Ctrl Pts',(-20.0366117400743,-43.400417859018,124.441917217521)) ;
#55951=CARTESIAN_POINT('Ctrl Pts',(-20.1934350690971,-43.2204287785375,
124.699450982089)) ;
#55952=CARTESIAN_POINT('Ctrl Pts',(-20.2063611151425,-43.4104492048053,
124.316781602561)) ;
#55953=CARTESIAN_POINT('Ctrl Pts',(-20.4056235279798,-43.2304601243249,
124.543033701489)) ;
#55954=CARTESIAN_POINT('Ctrl Pts',(-20.3494415293354,-43.4203029695104,
124.166967548006)) ;
#55955=CARTESIAN_POINT('Ctrl Pts',(-20.5844761557595,-43.2403138890299,
124.3557679957)) ;
#55956=CARTESIAN_POINT('Ctrl Pts',(-20.4660990695742,-43.4302736231787,
123.992841247419)) ;
#55957=CARTESIAN_POINT('Ctrl Pts',(-20.7303004789797,-43.2502845426982,
124.138111587167)) ;
#55958=CARTESIAN_POINT('Ctrl Pts',(-20.550990914283,-43.4402708668359,123.800540309338)) ;
#55959=CARTESIAN_POINT('Ctrl Pts',(-20.8364178791155,-43.2602817863554,
123.897736473004)) ;
#55960=CARTESIAN_POINT('Ctrl Pts',(-20.6011102529221,-43.4503043227801,
123.595664099876)) ;
#55961=CARTESIAN_POINT('Ctrl Pts',(-20.8990697975969,-43.2703152422996,
123.641641842394)) ;
#55962=CARTESIAN_POINT('Ctrl Pts',(-20.614988288072,-43.4601598270805,123.388915446738)) ;
#55963=CARTESIAN_POINT('Ctrl Pts',(-20.9164201486326,-43.2801707466,123.383205983388)) ;
#55964=CARTESIAN_POINT('Ctrl Pts',(-20.5927177301591,-43.4701592633666,
123.179916340754)) ;
#55965=CARTESIAN_POINT('Ctrl Pts',(-20.8885847144271,-43.2901701828861,
123.121956715674)) ;
#55966=CARTESIAN_POINT('Ctrl Pts',(-20.5353148533199,-43.4800537228825,
122.979940150803)) ;
#55967=CARTESIAN_POINT('Ctrl Pts',(-20.8168337007792,-43.300064642402,122.871985466882)) ;
#55968=CARTESIAN_POINT('Ctrl Pts',(-20.4424830563002,-43.4901168423341,
122.789877503651)) ;
#55969=CARTESIAN_POINT('Ctrl Pts',(-20.7007964616095,-43.3101277618536,
122.634405970991)) ;
#55970=CARTESIAN_POINT('Ctrl Pts',(-20.3209670354075,-43.4999564767461,
122.622428572666)) ;
#55971=CARTESIAN_POINT('Ctrl Pts',(-20.5489034191562,-43.3199673962656,
122.425092863686)) ;
#55972=CARTESIAN_POINT('Ctrl Pts',(-20.1690754221766,-43.5100196842319,
122.475206765639)) ;
#55973=CARTESIAN_POINT('Ctrl Pts',(-20.359040830139,-43.3300306037514,122.241063678947)) ;
#55974=CARTESIAN_POINT('Ctrl Pts',(-19.9967306491501,-43.5199137916111,
122.358701622462)) ;
#55975=CARTESIAN_POINT('Ctrl Pts',(-20.1436111274981,-43.3399247111306,
122.095429795522)) ;
#55976=CARTESIAN_POINT('Ctrl Pts',(-19.8061253691053,-43.5298561238035,
122.272988374327)) ;
#55977=CARTESIAN_POINT('Ctrl Pts',(-19.9053553865689,-43.349867043323,121.988285685906)) ;
#55978=CARTESIAN_POINT('Ctrl Pts',(-19.6023104751595,-43.5398567501185,
122.221256111772)) ;
#55979=CARTESIAN_POINT('Ctrl Pts',(-19.6505873376654,-43.359867669638,121.92361775973)) ;
#55980=CARTESIAN_POINT('Ctrl Pts',(-19.3917705372051,-43.5498984844004,
122.206031467105)) ;
#55981=CARTESIAN_POINT('Ctrl Pts',(-19.3874126433925,-43.3699094039199,
121.904584247332)) ;
#55982=CARTESIAN_POINT('Ctrl Pts',(-19.1862281430007,-43.5597239103495,
122.226676883472)) ;
#55983=CARTESIAN_POINT('Ctrl Pts',(-19.1304837624119,-43.379734829869,121.930388446453)) ;
#55984=CARTESIAN_POINT('Ctrl Pts',(-18.9826551708029,-43.5697807368771,
122.283706162221)) ;
#55985=CARTESIAN_POINT('Ctrl Pts',(-18.8760169233883,-43.3897916563967,
122.001672515838)) ;
#55986=CARTESIAN_POINT('Ctrl Pts',(-18.7946320656292,-43.5797081699987,
122.374314662117)) ;
#55987=CARTESIAN_POINT('Ctrl Pts',(-18.6409865991805,-43.3997190895182,
122.114930896961)) ;
#55988=CARTESIAN_POINT('Ctrl Pts',(-18.6244661109234,-43.5896581624049,
122.495982615423)) ;
#55989=CARTESIAN_POINT('Ctrl Pts',(-18.4282774407069,-43.4096690819245,
122.267013929231)) ;
#55990=CARTESIAN_POINT('Ctrl Pts',(-18.4767445700098,-43.5997133634789,
122.647173613548)) ;
#55991=CARTESIAN_POINT('Ctrl Pts',(-18.2436237168024,-43.4197242829985,
122.456000772566)) ;
#55992=CARTESIAN_POINT('Ctrl Pts',(-18.3599557995264,-43.6095356375312,
122.817488686517)) ;
#55993=CARTESIAN_POINT('Ctrl Pts',(-18.0976352135923,-43.4295465570507,
122.66889381585)) ;
#55994=CARTESIAN_POINT('Ctrl Pts',(-18.2721502560574,-43.6195915314905,
123.009781982913)) ;
#55995=CARTESIAN_POINT('Ctrl Pts',(-17.9878760752162,-43.43960245101,122.909259307955)) ;
#55996=CARTESIAN_POINT('Ctrl Pts',(-18.2200294874752,-43.6295322533356,
123.212171534823)) ;
#55997=CARTESIAN_POINT('Ctrl Pts',(-17.9227225615872,-43.4495431728551,
123.162245934138)) ;
#55998=CARTESIAN_POINT('Ctrl Pts',(-18.2032511636616,-43.6394365974222,
123.419718607872)) ;
#55999=CARTESIAN_POINT('Ctrl Pts',(-17.9017472034625,-43.4594475169417,
123.421680109375)) ;
#56000=CARTESIAN_POINT('Ctrl Pts',(-18.2231767398449,-43.6494832647217,
123.629971456285)) ;
#56001=CARTESIAN_POINT('Ctrl Pts',(-17.9266517282372,-43.4694941842412,
123.684496298962)) ;
#56002=CARTESIAN_POINT('Ctrl Pts',(-18.2782926714603,-43.6593788231716,
123.830608023793)) ;
#56003=CARTESIAN_POINT('Ctrl Pts',(-17.9955444785647,-43.4793897426911,
123.935293204453)) ;
#56004=CARTESIAN_POINT('Ctrl Pts',(-18.368880857869,-43.6694409018763,124.021733140042)) ;
#56005=CARTESIAN_POINT('Ctrl Pts',(-18.1087774584325,-43.4894518213958,
124.174200467556)) ;
#56006=CARTESIAN_POINT('Ctrl Pts',(-18.4885436290757,-43.6792836003421,
124.19057641474)) ;
#56007=CARTESIAN_POINT('Ctrl Pts',(-18.2583544803866,-43.4992945198616,
124.385256639868)) ;
#56008=CARTESIAN_POINT('Ctrl Pts',(-18.637534073092,-43.6892743742365,124.338585277532)) ;
#56009=CARTESIAN_POINT('Ctrl Pts',(-18.4445910636902,-43.5092852937561,
124.570269448584)) ;
#56010=CARTESIAN_POINT('Ctrl Pts',(-18.8089243606345,-43.6992022434715,
124.457711598807)) ;
#56011=CARTESIAN_POINT('Ctrl Pts',(-18.6588280253007,-43.519213162991,124.719179491645)) ;
#56012=CARTESIAN_POINT('Ctrl Pts',(-18.9994025238417,-43.7091909724413,
124.546144010481)) ;
#56013=CARTESIAN_POINT('Ctrl Pts',(-18.8969249829765,-43.5292018919608,
124.829722059201)) ;
#56014=CARTESIAN_POINT('Ctrl Pts',(-19.2034513375471,-43.7192303744251,
124.600051021114)) ;
#56015=CARTESIAN_POINT('Ctrl Pts',(-19.1519853154671,-43.5392412939446,
124.897107997112)) ;
#56016=CARTESIAN_POINT('Ctrl Pts',(-19.4095740593302,-43.7290705421618,
124.617767680818)) ;
#56017=CARTESIAN_POINT('Ctrl Pts',(-19.4096395220042,-43.5490814616814,
124.919256070327)) ;
#56018=CARTESIAN_POINT('Ctrl Pts',(-19.6200056310843,-43.7391187525363,
124.599348020896)) ;
#56019=CARTESIAN_POINT('Ctrl Pts',(-19.6726790144309,-43.5591296720559,
124.89623358848)) ;
#56020=CARTESIAN_POINT('Ctrl Pts',(-19.8219167217474,-43.7490659228241,
124.544896993531)) ;
#56021=CARTESIAN_POINT('Ctrl Pts',(-19.9250688422979,-43.5690768423436,
124.828171804212)) ;
#56022=CARTESIAN_POINT('Ctrl Pts',(-20.0108816230602,-43.7589767710792,
124.457103125973)) ;
#56023=CARTESIAN_POINT('Ctrl Pts',(-20.1612764163773,-43.5789876905987,
124.718431010764)) ;
#56024=CARTESIAN_POINT('Ctrl Pts',(-20.1841105037693,-43.7690330987569,
124.335929383685)) ;
#56025=CARTESIAN_POINT('Ctrl Pts',(-20.3778135164832,-43.5890440182765,
124.566965650393)) ;
#56026=CARTESIAN_POINT('Ctrl Pts',(-20.3307480730598,-43.7788835115255,
124.189689219311)) ;
#56027=CARTESIAN_POINT('Ctrl Pts',(-20.5611126311556,-43.598894431045,124.384166137604)) ;
#56028=CARTESIAN_POINT('Ctrl Pts',(-20.4523107242859,-43.7889103973592,
124.017478146335)) ;
#56029=CARTESIAN_POINT('Ctrl Pts',(-20.7130674437929,-43.6089213168787,
124.168903399387)) ;
#56030=CARTESIAN_POINT('Ctrl Pts',(-20.5416506384017,-43.79893901299,123.826498737951)) ;
#56031=CARTESIAN_POINT('Ctrl Pts',(-20.8247441403498,-43.6189499325095,
123.930180059091)) ;
#56032=CARTESIAN_POINT('Ctrl Pts',(-20.5958423754753,-43.8087842363675,
123.626753384018)) ;
#56033=CARTESIAN_POINT('Ctrl Pts',(-20.892485943734,-43.628795155887,123.680497788547)) ;
#56034=CARTESIAN_POINT('Ctrl Pts',(-20.6153678869501,-43.8187749184691,
123.417621815396)) ;
#56035=CARTESIAN_POINT('Ctrl Pts',(-20.9168945754122,-43.6387858379886,
123.419083293923)) ;
#56036=CARTESIAN_POINT('Ctrl Pts',(-20.5977356287722,-43.8288128071015,
123.207333737344)) ;
#56037=CARTESIAN_POINT('Ctrl Pts',(-20.8948561362001,-43.648823726621,123.156223171612)) ;
#56038=CARTESIAN_POINT('Ctrl Pts',(-20.5452446975445,-43.8386571422047,
123.007134061094)) ;
#56039=CARTESIAN_POINT('Ctrl Pts',(-20.8292438815407,-43.6586680617242,
122.905971997051)) ;
#56040=CARTESIAN_POINT('Ctrl Pts',(-20.4579454357753,-43.8486421044022,
122.816264363838)) ;
#56041=CARTESIAN_POINT('Ctrl Pts',(-20.7201211841822,-43.6686530239217,
122.667383970088)) ;
#56042=CARTESIAN_POINT('Ctrl Pts',(-20.3394267685731,-43.8585810459356,
122.644144630097)) ;
#56043=CARTESIAN_POINT('Ctrl Pts',(-20.5719738574173,-43.6785919654551,
122.452232948962)) ;
#56044=CARTESIAN_POINT('Ctrl Pts',(-20.1912921885784,-43.868622930907,122.493758530072)) ;
#56045=CARTESIAN_POINT('Ctrl Pts',(-20.3868068905947,-43.6886338504265,
122.264249292206)) ;
#56046=CARTESIAN_POINT('Ctrl Pts',(-20.0220013238299,-43.8785094788153,
122.373139062939)) ;
#56047=CARTESIAN_POINT('Ctrl Pts',(-20.1751934661885,-43.6985203983348,
122.113473137148)) ;
#56048=CARTESIAN_POINT('Ctrl Pts',(-19.8324762444945,-43.8885034043153,
122.282516116147)) ;
#56049=CARTESIAN_POINT('Ctrl Pts',(-19.9382875920439,-43.7085143238348,
122.00019304693)) ;
#56050=CARTESIAN_POINT('Ctrl Pts',(-19.6312362520306,-43.8984394954417,
122.226393147008)) ;
#56051=CARTESIAN_POINT('Ctrl Pts',(-19.6867374287928,-43.7184504149613,
121.930037797362)) ;
#56052=CARTESIAN_POINT('Ctrl Pts',(-19.4214139020312,-43.9084687644217,
122.205920422731)) ;
#56053=CARTESIAN_POINT('Ctrl Pts',(-19.4244597082915,-43.7284796839412,
121.904445450295)) ;
#56054=CARTESIAN_POINT('Ctrl Pts',(-19.2142240963958,-43.918351146981,122.221693374748)) ;
#56055=CARTESIAN_POINT('Ctrl Pts',(-19.1654713411927,-43.7383620665005,
121.924160359609)) ;
#56056=CARTESIAN_POINT('Ctrl Pts',(-19.009498669417,-43.9284036640689,122.274004896839)) ;
#56057=CARTESIAN_POINT('Ctrl Pts',(-18.9095644693227,-43.7484145835884,
121.989548405927)) ;
#56058=CARTESIAN_POINT('Ctrl Pts',(-18.819892626088,-43.9382977848928,122.359628820028)) ;
#56059=CARTESIAN_POINT('Ctrl Pts',(-18.6725555426517,-43.7583087044123,
122.096577505199)) ;
#56060=CARTESIAN_POINT('Ctrl Pts',(-18.6451418431221,-43.9483597643132,
122.478785235648)) ;
#56061=CARTESIAN_POINT('Ctrl Pts',(-18.4541166119163,-43.7683706838327,
122.245521781282)) ;
#56062=CARTESIAN_POINT('Ctrl Pts',(-18.4969665742692,-43.9582042975421,
122.623287056138)) ;
#56063=CARTESIAN_POINT('Ctrl Pts',(-18.2688956917454,-43.7782152170616,
122.426149066414)) ;
#56064=CARTESIAN_POINT('Ctrl Pts',(-18.3741086579576,-43.9681643764484,
122.792844278905)) ;
#56065=CARTESIAN_POINT('Ctrl Pts',(-18.1153222213205,-43.7881752959679,
122.638095379869)) ;
#56066=CARTESIAN_POINT('Ctrl Pts',(-18.2822146957173,-43.978202653021,122.982811873734)) ;
#56067=CARTESIAN_POINT('Ctrl Pts',(-18.0004538037263,-43.7982135725405,
122.875554226901)) ;
#56068=CARTESIAN_POINT('Ctrl Pts',(-18.2252522008148,-43.9880760395588,
123.182444364765)) ;
#56069=CARTESIAN_POINT('Ctrl Pts',(-17.929249415048,-43.8080869590783,123.125095646741)) ;
#56070=CARTESIAN_POINT('Ctrl Pts',(-18.2034535742499,-43.9981489823259,
123.393043925117)) ;
#56071=CARTESIAN_POINT('Ctrl Pts',(-17.902000155015,-43.8181599018454,123.388344568527)) ;
#56072=CARTESIAN_POINT('Ctrl Pts',(-18.2179298683599,-44.0079703964542,
123.599052536948)) ;
#56073=CARTESIAN_POINT('Ctrl Pts',(-17.9200947060071,-43.8279813159737,
123.645856942406)) ;
#56074=CARTESIAN_POINT('Ctrl Pts',(-18.2689797272042,-44.0180450265265,
123.804569296683)) ;
#56075=CARTESIAN_POINT('Ctrl Pts',(-17.9839061109843,-43.8380559460461,
123.902752660096)) ;
#56076=CARTESIAN_POINT('Ctrl Pts',(-18.3532690236661,-44.0279116638434,
123.994127168066)) ;
#56077=CARTESIAN_POINT('Ctrl Pts',(-18.0892674355446,-43.8479225833629,
124.139701464818)) ;
#56078=CARTESIAN_POINT('Ctrl Pts',(-18.4705660574724,-44.0379352092152,
124.169178578053)) ;
#56079=CARTESIAN_POINT('Ctrl Pts',(-18.2358881549288,-43.8579461287347,
124.35851605704)) ;
#56080=CARTESIAN_POINT('Ctrl Pts',(-18.6168901850746,-44.0479609607324,
124.320901604425)) ;
#56081=CARTESIAN_POINT('Ctrl Pts',(-18.4187926356605,-43.8679718802519,
124.548170374758)) ;
#56082=CARTESIAN_POINT('Ctrl Pts',(-18.7841854234927,-44.0578145477417,
124.443049390508)) ;
#56083=CARTESIAN_POINT('Ctrl Pts',(-18.6279123308095,-43.8778254672613,
124.700856473596)) ;
#56084=CARTESIAN_POINT('Ctrl Pts',(-18.9722447032616,-44.0677915079697,
124.535943542531)) ;
#56085=CARTESIAN_POINT('Ctrl Pts',(-18.8629865022729,-43.8878024274892,
124.816974766447)) ;
#56086=CARTESIAN_POINT('Ctrl Pts',(-19.1745538584046,-44.0778126509981,
124.594687633836)) ;
#56087=CARTESIAN_POINT('Ctrl Pts',(-19.1158727505766,-43.8978235705177,
124.890405499311)) ;
#56088=CARTESIAN_POINT('Ctrl Pts',(-19.3810867415163,-44.0876952570181,
124.617517604128)) ;
#56089=CARTESIAN_POINT('Ctrl Pts',(-19.3740398930838,-43.9077061765376,
124.918943559921)) ;
#56090=CARTESIAN_POINT('Ctrl Pts',(-19.5922777528914,-44.0977637276508,
124.603809178215)) ;
#56091=CARTESIAN_POINT('Ctrl Pts',(-19.638028281114,-43.9177746471703,124.901808569108)) ;
#56092=CARTESIAN_POINT('Ctrl Pts',(-19.7931371162424,-44.1075938108345,
124.555043900469)) ;
#56093=CARTESIAN_POINT('Ctrl Pts',(-19.8891040806807,-43.927604730354,124.840852016009)) ;
#56094=CARTESIAN_POINT('Ctrl Pts',(-19.9870797834277,-44.1176603705148,
124.470429298828)) ;
#56095=CARTESIAN_POINT('Ctrl Pts',(-20.1315321755762,-43.9376712900344,
124.735084209579)) ;
#56096=CARTESIAN_POINT('Ctrl Pts',(-20.1602737104804,-44.1275506203441,
124.355334521144)) ;
#56097=CARTESIAN_POINT('Ctrl Pts',(-20.3480256594393,-43.9475615398636,
124.591215461536)) ;
#56098=CARTESIAN_POINT('Ctrl Pts',(-20.3126945664649,-44.1375427860929,
124.210797364723)) ;
#56099=CARTESIAN_POINT('Ctrl Pts',(-20.5385520109249,-43.9575537056124,
124.410544001641)) ;
#56100=CARTESIAN_POINT('Ctrl Pts',(-20.4371805511039,-44.147505629689,124.042362117162)) ;
#56101=CARTESIAN_POINT('Ctrl Pts',(-20.6941599749357,-43.9675165492085,
124.199999732296)) ;
#56102=CARTESIAN_POINT('Ctrl Pts',(-20.5304651406943,-44.1574097985167,
123.856190907026)) ;
#56103=CARTESIAN_POINT('Ctrl Pts',(-20.8107661787907,-43.9774207180363,
123.967284902407)) ;
#56104=CARTESIAN_POINT('Ctrl Pts',(-20.5907535668492,-44.1674706734111,
123.653482764697)) ;
#56105=CARTESIAN_POINT('Ctrl Pts',(-20.8861267323837,-43.9874815929306,
123.713900101314)) ;
#56106=CARTESIAN_POINT('Ctrl Pts',(-20.6146904777119,-44.1773095767404,
123.447994903833)) ;
#56107=CARTESIAN_POINT('Ctrl Pts',(-20.9160480545107,-43.99732049626,123.45703880834)) ;
#56108=CARTESIAN_POINT('Ctrl Pts',(-20.6025093175598,-44.1873779531143,
123.236711105022)) ;
#56109=CARTESIAN_POINT('Ctrl Pts',(-20.9008215571062,-44.0073888726339,
123.192934464728)) ;
#56110=CARTESIAN_POINT('Ctrl Pts',(-20.5546520539257,-44.197258569747,123.034546463508)) ;
#56111=CARTESIAN_POINT('Ctrl Pts',(-20.84099967691,-44.0172694892665,122.940227571267)) ;
#56112=CARTESIAN_POINT('Ctrl Pts',(-20.4719127587511,-44.207249729976,122.841516718461)) ;
#56113=CARTESIAN_POINT('Ctrl Pts',(-20.7375752828072,-44.0272606494955,
122.6989402697)) ;
#56114=CARTESIAN_POINT('Ctrl Pts',(-20.3573466961592,-44.2172028034081,
122.666384942682)) ;
#56115=CARTESIAN_POINT('Ctrl Pts',(-20.5943672384386,-44.0372137229276,
122.480025241696)) ;
#56116=CARTESIAN_POINT('Ctrl Pts',(-20.2129041498641,-44.2272386390207,
122.512619796291)) ;
#56117=CARTESIAN_POINT('Ctrl Pts',(-20.4138140211742,-44.0472495585402,
122.287819048033)) ;
#56118=CARTESIAN_POINT('Ctrl Pts',(-20.0464710387891,-44.2371287657509,
122.387973352536)) ;
#56119=CARTESIAN_POINT('Ctrl Pts',(-20.2057716276786,-44.0571396852704,
122.132010547307)) ;
#56120=CARTESIAN_POINT('Ctrl Pts',(-19.8591825427843,-44.2471209475202,
122.292859773078)) ;
#56121=CARTESIAN_POINT('Ctrl Pts',(-19.9716606493578,-44.0671318670397,
122.013118819214)) ;
#56122=CARTESIAN_POINT('Ctrl Pts',(-19.6591233355574,-44.2570668874946,
122.232057906524)) ;
#56123=CARTESIAN_POINT('Ctrl Pts',(-19.7215859697298,-44.0770778070142,
121.937116648818)) ;
#56124=CARTESIAN_POINT('Ctrl Pts',(-19.4515603480813,-44.2670140712541,
122.206490694919)) ;
#56125=CARTESIAN_POINT('Ctrl Pts',(-19.4621316011772,-44.0870249907736,
121.90515807925)) ;
#56126=CARTESIAN_POINT('Ctrl Pts',(-19.2406254966303,-44.2770620095444,
122.217696911722)) ;
#56127=CARTESIAN_POINT('Ctrl Pts',(-19.1984633098211,-44.097072929064,121.919166261235)) ;
#56128=CARTESIAN_POINT('Ctrl Pts',(-19.0388958129296,-44.286909644358,122.264239155619)) ;
#56129=CARTESIAN_POINT('Ctrl Pts',(-18.9462999516527,-44.1069205638775,
121.977344862589)) ;
#56130=CARTESIAN_POINT('Ctrl Pts',(-18.8458583821311,-44.296871358056,122.345428988857)) ;
#56131=CARTESIAN_POINT('Ctrl Pts',(-18.7050030348697,-44.1168822775755,
122.078833023452)) ;
#56132=CARTESIAN_POINT('Ctrl Pts',(-18.6687933154075,-44.3068999938771,
122.459902791905)) ;
#56133=CARTESIAN_POINT('Ctrl Pts',(-18.4836721333782,-44.1269109133967,
122.221925766882)) ;
#56134=CARTESIAN_POINT('Ctrl Pts',(-18.5160880962946,-44.3168103086289,
122.601623849684)) ;
#56135=CARTESIAN_POINT('Ctrl Pts',(-18.2927904239115,-44.1368212281484,
122.399078178037)) ;
#56136=CARTESIAN_POINT('Ctrl Pts',(-18.3895506603922,-44.3267451792916,
122.767800295044)) ;
#56137=CARTESIAN_POINT('Ctrl Pts',(-18.1346189319372,-44.1467560988111,
122.606799797155)) ;
#56138=CARTESIAN_POINT('Ctrl Pts',(-18.2929514113174,-44.3367863616933,
122.955488189601)) ;
#56139=CARTESIAN_POINT('Ctrl Pts',(-18.0138706729909,-44.1567972812129,
122.841409864053)) ;
#56140=CARTESIAN_POINT('Ctrl Pts',(-18.2312003577601,-44.3466733331581,
123.153977478668)) ;
#56141=CARTESIAN_POINT('Ctrl Pts',(-17.9366823753341,-44.1666842526776,
123.089522739971)) ;
#56142=CARTESIAN_POINT('Ctrl Pts',(-18.2042924362549,-44.3566727654207,
123.362440492209)) ;
#56143=CARTESIAN_POINT('Ctrl Pts',(-17.9030484192292,-44.1766836849402,
123.350101781401)) ;
#56144=CARTESIAN_POINT('Ctrl Pts',(-18.2137740339436,-44.3665928306773,
123.5708007757)) ;
#56145=CARTESIAN_POINT('Ctrl Pts',(-17.9149014699475,-44.1866037501968,
123.610552838734)) ;
#56146=CARTESIAN_POINT('Ctrl Pts',(-18.2597764971867,-44.3766296832615,
123.776719598034)) ;
#56147=CARTESIAN_POINT('Ctrl Pts',(-17.9724055288839,-44.196640602781,123.867950986219)) ;
#56148=CARTESIAN_POINT('Ctrl Pts',(-18.3398426561002,-44.3865423426014,
123.969124187214)) ;
#56149=CARTESIAN_POINT('Ctrl Pts',(-18.0724894957903,-44.206553262121,124.108457083401)) ;
#56150=CARTESIAN_POINT('Ctrl Pts',(-18.4526095787518,-44.3965335545164,
124.146348677994)) ;
#56151=CARTESIAN_POINT('Ctrl Pts',(-18.2134492760252,-44.2165444740359,
124.329987229938)) ;
#56152=CARTESIAN_POINT('Ctrl Pts',(-18.5954817229628,-44.4065751959195,
124.301740665686)) ;
#56153=CARTESIAN_POINT('Ctrl Pts',(-18.3920400926591,-44.226586115439,124.524226386443)) ;
#56154=CARTESIAN_POINT('Ctrl Pts',(-18.7593291885529,-44.4164039901265,
124.427686436395)) ;
#56155=CARTESIAN_POINT('Ctrl Pts',(-18.5968513117596,-44.236414909646,124.681658511702)) ;
#56156=CARTESIAN_POINT('Ctrl Pts',(-18.9470682784548,-44.4264804012478,
124.525725017682)) ;
#56157=CARTESIAN_POINT('Ctrl Pts',(-18.8315253712674,-44.2464913207673,
124.804205426369)) ;
#56158=CARTESIAN_POINT('Ctrl Pts',(-19.1445330347221,-44.4363325342902,
124.588381426749)) ;
#56159=CARTESIAN_POINT('Ctrl Pts',(-19.0783578845123,-44.2563434538097,
124.882525082165)) ;
#56160=CARTESIAN_POINT('Ctrl Pts',(-19.3543837050247,-44.4464057686315,
124.616582421442)) ;
#56161=CARTESIAN_POINT('Ctrl Pts',(-19.3406710041986,-44.2664166881511,
124.917774929088)) ;
#56162=CARTESIAN_POINT('Ctrl Pts',(-19.561120757118,-44.4562472699582,124.608057607434)) ;
#56163=CARTESIAN_POINT('Ctrl Pts',(-19.599093568999,-44.2762581894777,124.907117526601)) ;
#56164=CARTESIAN_POINT('Ctrl Pts',(-19.7658378555304,-44.466208221553,124.564003318983)) ;
#56165=CARTESIAN_POINT('Ctrl Pts',(-19.8549900005781,-44.2862191410725,
124.852048008168)) ;
#56166=CARTESIAN_POINT('Ctrl Pts',(-19.9611338445933,-44.4762460392736,
124.484072288273)) ;
#56167=CARTESIAN_POINT('Ctrl Pts',(-20.0991093096949,-44.2962569587932,
124.752132918217)) ;
#56168=CARTESIAN_POINT('Ctrl Pts',(-20.1369108495217,-44.4861203885307,
124.373589262142)) ;
#56169=CARTESIAN_POINT('Ctrl Pts',(-20.3188305769576,-44.3061313080502,
124.614027246397)) ;
#56170=CARTESIAN_POINT('Ctrl Pts',(-20.2938275249447,-44.4961899392729,
124.231536291723)) ;
#56171=CARTESIAN_POINT('Ctrl Pts',(-20.5149750945058,-44.3162008587924,
124.43646009178)) ;
#56172=CARTESIAN_POINT('Ctrl Pts',(-20.4207811078669,-44.5060239587815,
124.068339987398)) ;
#56173=CARTESIAN_POINT('Ctrl Pts',(-20.6736665784538,-44.326034878301,124.232462693822)) ;
#56174=CARTESIAN_POINT('Ctrl Pts',(-20.5199150721139,-44.516058113361,123.882148162082)) ;
#56175=CARTESIAN_POINT('Ctrl Pts',(-20.7975823822247,-44.3360690328805,
123.99972215947)) ;
#56176=CARTESIAN_POINT('Ctrl Pts',(-20.5846066652837,-44.5260740391835,
123.68175257298)) ;
#56177=CARTESIAN_POINT('Ctrl Pts',(-20.8784453198303,-44.346084958703,123.749227159108)) ;
#56178=CARTESIAN_POINT('Ctrl Pts',(-20.6135027473333,-44.5359562943777,
123.476012739199)) ;
#56179=CARTESIAN_POINT('Ctrl Pts',(-20.9145638048627,-44.3559672138973,
123.492051220725)) ;
#56180=CARTESIAN_POINT('Ctrl Pts',(-20.6064192234333,-44.5459451008887,
123.266159254011)) ;
#56181=CARTESIAN_POINT('Ctrl Pts',(-20.9057075529971,-44.3659560204082,
123.229734225015)) ;
#56182=CARTESIAN_POINT('Ctrl Pts',(-20.5633248096925,-44.5558936681514,
123.061463359673)) ;
#56183=CARTESIAN_POINT('Ctrl Pts',(-20.851837594289,-44.3759045876709,122.973864297995)) ;
#56184=CARTESIAN_POINT('Ctrl Pts',(-20.4843220668197,-44.5659484734534,
122.865422401674)) ;
#56185=CARTESIAN_POINT('Ctrl Pts',(-20.7530825572401,-44.3859593929729,
122.728813985254)) ;
#56186=CARTESIAN_POINT('Ctrl Pts',(-20.3753421768984,-44.575767256717,122.69010150794)) ;
#56187=CARTESIAN_POINT('Ctrl Pts',(-20.6168554016268,-44.3957781762364,
122.509662800766)) ;
#56188=CARTESIAN_POINT('Ctrl Pts',(-20.2349634944572,-44.5858030290775,
122.532602841201)) ;
#56189=CARTESIAN_POINT('Ctrl Pts',(-20.4413805690355,-44.4058139485971,
122.312790933982)) ;
#56190=CARTESIAN_POINT('Ctrl Pts',(-20.0691703030276,-44.5958277281062,
122.402480939027)) ;
#56191=CARTESIAN_POINT('Ctrl Pts',(-20.2341379247763,-44.4158386476257,
122.150140067202)) ;
#56192=CARTESIAN_POINT('Ctrl Pts',(-19.8867241174746,-44.6056797313652,
122.304432926397)) ;
#56193=CARTESIAN_POINT('Ctrl Pts',(-20.0060783373633,-44.4256906508848,
122.02758136636)) ;
#56194=CARTESIAN_POINT('Ctrl Pts',(-19.6873786654677,-44.6156706657625,
122.238342902669)) ;
#56195=CARTESIAN_POINT('Ctrl Pts',(-19.7568956898042,-44.435681585282,121.94497080327)) ;
#56196=CARTESIAN_POINT('Ctrl Pts',(-19.481074169139,-44.6255885881936,122.207949395056)) ;
#56197=CARTESIAN_POINT('Ctrl Pts',(-19.4990141869659,-44.4455995077131,
121.906980973268)) ;
#56198=CARTESIAN_POINT('Ctrl Pts',(-19.2703469798628,-44.6356169438759,
122.213857027712)) ;
#56199=CARTESIAN_POINT('Ctrl Pts',(-19.2356052976537,-44.4556278633954,
121.914367687732)) ;
#56200=CARTESIAN_POINT('Ctrl Pts',(-19.0667685393293,-44.6455012283865,
122.255560649441)) ;
#56201=CARTESIAN_POINT('Ctrl Pts',(-18.9811319609674,-44.465512147906,121.96649952011)) ;
#56202=CARTESIAN_POINT('Ctrl Pts',(-18.8712365177251,-44.6554939122944,
122.332371985697)) ;
#56203=CARTESIAN_POINT('Ctrl Pts',(-18.7367176524667,-44.4755048318139,
122.062515901464)) ;
#56204=CARTESIAN_POINT('Ctrl Pts',(-18.6915565635913,-44.6655226493021,
122.442678617086)) ;
#56205=CARTESIAN_POINT('Ctrl Pts',(-18.5121188959435,-44.4855335688216,
122.200401078651)) ;
#56206=CARTESIAN_POINT('Ctrl Pts',(-18.5358279806812,-44.675408045931,122.580307301666)) ;
#56207=CARTESIAN_POINT('Ctrl Pts',(-18.3174591679759,-44.4954189654505,
122.372439116207)) ;
#56208=CARTESIAN_POINT('Ctrl Pts',(-18.4048030817091,-44.6853959313449,
122.74436173368)) ;
#56209=CARTESIAN_POINT('Ctrl Pts',(-18.1536797929132,-44.5054068508644,
122.577508760513)) ;
#56210=CARTESIAN_POINT('Ctrl Pts',(-18.3045194431609,-44.6953466340055,
122.927987236834)) ;
#56211=CARTESIAN_POINT('Ctrl Pts',(-18.0283271817099,-44.515357553525,122.807042074235)) ;
#56212=CARTESIAN_POINT('Ctrl Pts',(-18.2371653977238,-44.7053869521029,
123.128009185341)) ;
#56213=CARTESIAN_POINT('Ctrl Pts',(-17.9441368872548,-44.5253978716224,
123.057070192323)) ;
#56214=CARTESIAN_POINT('Ctrl Pts',(-18.2058765293099,-44.7152615174361,
123.333255667552)) ;
#56215=CARTESIAN_POINT('Ctrl Pts',(-17.9050280764321,-44.5352724369556,
123.313629339714)) ;
#56216=CARTESIAN_POINT('Ctrl Pts',(-18.2104928246588,-44.7252611774972,
123.543394996734)) ;
#56217=CARTESIAN_POINT('Ctrl Pts',(-17.9108009161335,-44.5452720970167,
123.576303554665)) ;
#56218=CARTESIAN_POINT('Ctrl Pts',(-18.2509713151308,-44.7351701726649,
123.747780176754)) ;
#56219=CARTESIAN_POINT('Ctrl Pts',(-17.9614015774654,-44.5551810921844,
123.831785012539)) ;
#56220=CARTESIAN_POINT('Ctrl Pts',(-18.3274676749511,-44.7452249138281,
123.944798878115)) ;
#56221=CARTESIAN_POINT('Ctrl Pts',(-18.0570243117,-44.5652358333477,124.078057381576)) ;
#56222=CARTESIAN_POINT('Ctrl Pts',(-18.4347054519244,-44.7550835257419,
124.122200708846)) ;
#56223=CARTESIAN_POINT('Ctrl Pts',(-18.1910740416951,-44.5750944452614,
124.299808917773)) ;
#56224=CARTESIAN_POINT('Ctrl Pts',(-18.5738749657264,-44.7651516480213,
124.281638187706)) ;
#56225=CARTESIAN_POINT('Ctrl Pts',(-18.3650377632087,-44.5851625675408,
124.499103963494)) ;
#56226=CARTESIAN_POINT('Ctrl Pts',(-18.7351819980848,-44.7750071187245,
124.411700343814)) ;
#56227=CARTESIAN_POINT('Ctrl Pts',(-18.5666736484834,-44.595018038244,124.661680062482)) ;
#56228=CARTESIAN_POINT('Ctrl Pts',(-18.9188616429352,-44.7850019782178,
124.513733292732)) ;
#56229=CARTESIAN_POINT('Ctrl Pts',(-18.7962745857108,-44.6050128977374,
124.789218967145)) ;
#56230=CARTESIAN_POINT('Ctrl Pts',(-19.1183492113281,-44.7950332315598,
124.58214803004)) ;
#56231=CARTESIAN_POINT('Ctrl Pts',(-19.045634886792,-44.6150441510793,124.874734939647)) ;
#56232=CARTESIAN_POINT('Ctrl Pts',(-19.323218690417,-44.8048999304329,124.61467366931)) ;
#56233=CARTESIAN_POINT('Ctrl Pts',(-19.3017226630567,-44.6249108499524,
124.915389460474)) ;
#56234=CARTESIAN_POINT('Ctrl Pts',(-19.5331246188192,-44.8148867461841,
124.61143594484)) ;
#56235=CARTESIAN_POINT('Ctrl Pts',(-19.5641051552307,-44.6348976657036,
124.911339609499)) ;
#56236=CARTESIAN_POINT('Ctrl Pts',(-19.7385308241501,-44.8248339513795,
124.572042427275)) ;
#56237=CARTESIAN_POINT('Ctrl Pts',(-19.8208626336043,-44.644844870899,124.862095013967)) ;
#56238=CARTESIAN_POINT('Ctrl Pts',(-19.9357852330403,-44.8348769395058,
124.496793289442)) ;
#56239=CARTESIAN_POINT('Ctrl Pts',(-20.0674296682668,-44.6548878590253,
124.768031081867)) ;
#56240=CARTESIAN_POINT('Ctrl Pts',(-20.1138908734245,-44.8447442941273,
124.39042646345)) ;
#56241=CARTESIAN_POINT('Ctrl Pts',(-20.2900606910525,-44.6647552136468,
124.635070010857)) ;
#56242=CARTESIAN_POINT('Ctrl Pts',(-20.2727462782933,-44.8547101874254,
124.25383373658)) ;
#56243=CARTESIAN_POINT('Ctrl Pts',(-20.4886282485058,-44.6747211069449,
124.464326908031)) ;
#56244=CARTESIAN_POINT('Ctrl Pts',(-20.4060875110616,-44.8647339648015,
124.090636353554)) ;
#56245=CARTESIAN_POINT('Ctrl Pts',(-20.6553026895756,-44.684744884321,124.260328413018)) ;
#56246=CARTESIAN_POINT('Ctrl Pts',(-20.5080877736395,-44.8746595127332,
123.908610854612)) ;
#56247=CARTESIAN_POINT('Ctrl Pts',(-20.78280073358,-44.6946704322527,124.032794984463)) ;
#56248=CARTESIAN_POINT('Ctrl Pts',(-20.5775102693516,-44.8845999891542,
123.711485460031)) ;
#56249=CARTESIAN_POINT('Ctrl Pts',(-20.8695762749803,-44.7046109086737,
123.786387153794)) ;
#56250=CARTESIAN_POINT('Ctrl Pts',(-20.6117719571326,-44.8946461988171,
123.503092758623)) ;
#56251=CARTESIAN_POINT('Ctrl Pts',(-20.9124006495194,-44.7146571183366,
123.525895807867)) ;
#56252=CARTESIAN_POINT('Ctrl Pts',(-20.6095960962421,-44.9045074554789,
123.295771336016)) ;
#56253=CARTESIAN_POINT('Ctrl Pts',(-20.9096780313366,-44.7245183749984,
123.266743788821)) ;
#56254=CARTESIAN_POINT('Ctrl Pts',(-20.5713071076348,-44.9145010837542,
123.08922311595)) ;
#56255=CARTESIAN_POINT('Ctrl Pts',(-20.8618140137241,-44.7345120032737,
123.008558951065)) ;
#56256=CARTESIAN_POINT('Ctrl Pts',(-20.4983191373996,-44.9244264810644,
122.893708018613)) ;
#56257=CARTESIAN_POINT('Ctrl Pts',(-20.7705763699212,-44.7444374005839,
122.764165937493)) ;
#56258=CARTESIAN_POINT('Ctrl Pts',(-20.391433863342,-44.9344543889746,122.712025942917)) ;
#56259=CARTESIAN_POINT('Ctrl Pts',(-20.6369673170847,-44.7544653084941,
122.537064718047)) ;
#56260=CARTESIAN_POINT('Ctrl Pts',(-20.2566836205498,-44.9443407046438,
122.55374389634)) ;
#56261=CARTESIAN_POINT('Ctrl Pts',(-20.4685272890457,-44.7643516241633,
122.339213894199)) ;
#56262=CARTESIAN_POINT('Ctrl Pts',(-20.0942650307571,-44.9543722995476,
122.419270807689)) ;
#56263=CARTESIAN_POINT('Ctrl Pts',(-20.2655021979111,-44.7743832190671,
122.171124667604)) ;
#56264=CARTESIAN_POINT('Ctrl Pts',(-19.9137299172441,-44.9642545424993,
122.316394133528)) ;
#56265=CARTESIAN_POINT('Ctrl Pts',(-20.0398318507275,-44.7842654620188,
122.042531241619)) ;
#56266=CARTESIAN_POINT('Ctrl Pts',(-19.7146500331995,-44.9743140135291,
122.24510774136)) ;
#56267=CARTESIAN_POINT('Ctrl Pts',(-19.7909809655389,-44.7943249330486,
121.953425884244)) ;
#56268=CARTESIAN_POINT('Ctrl Pts',(-19.5101771870513,-44.9841804581923,
122.210176444507)) ;
#56269=CARTESIAN_POINT('Ctrl Pts',(-19.5353894138437,-44.8041913777118,
121.909764540017)) ;
#56270=CARTESIAN_POINT('Ctrl Pts',(-19.3006636334398,-44.994146582641,122.210628861832)) ;
#56271=CARTESIAN_POINT('Ctrl Pts',(-19.2734974473515,-44.8141575021605,
121.910332881096)) ;
#56272=CARTESIAN_POINT('Ctrl Pts',(-19.0931406754314,-45.0041768260321,
122.248023638702)) ;
#56273=CARTESIAN_POINT('Ctrl Pts',(-19.0140941941528,-44.8241877455516,
121.957079095909)) ;
#56274=CARTESIAN_POINT('Ctrl Pts',(-18.8978469326455,-45.0140698609852,
122.319615465346)) ;
#56275=CARTESIAN_POINT('Ctrl Pts',(-18.7699778545703,-44.8340807805047,
122.046571668212)) ;
#56276=CARTESIAN_POINT('Ctrl Pts',(-18.7150830259635,-45.024120775222,122.425627543441)) ;
#56277=CARTESIAN_POINT('Ctrl Pts',(-18.541524921749,-44.8441316947415,122.179088598063)) ;
#56278=CARTESIAN_POINT('Ctrl Pts',(-18.5560590605076,-45.0340106014466,
122.559577916951)) ;
#56279=CARTESIAN_POINT('Ctrl Pts',(-18.3427444000537,-44.8540215209661,
122.346531093126)) ;
#56280=CARTESIAN_POINT('Ctrl Pts',(-18.3758084791143,-45.0473454164935,
122.774344433157)) ;
#56281=CARTESIAN_POINT('Ctrl Pts',(-18.1174461020188,-44.867356336013,122.614979486919)) ;
#56282=CARTESIAN_POINT('Ctrl Pts',(-18.2567530669862,-45.060622507665,123.03030649385)) ;
#56283=CARTESIAN_POINT('Ctrl Pts',(-17.9686335759019,-44.8806334271845,
122.934896659079)) ;
#56284=CARTESIAN_POINT('Ctrl Pts',(-18.2079946984886,-45.0738707962633,
123.304511382558)) ;
#56285=CARTESIAN_POINT('Ctrl Pts',(-17.9076731560715,-44.8938817157828,
123.277709414328)) ;
#56286=CARTESIAN_POINT('Ctrl Pts',(-18.2078213156215,-45.0839256377574,
123.515872423413)) ;
#56287=CARTESIAN_POINT('Ctrl Pts',(-17.9074623162929,-44.9039365572769,
123.5418995713)) ;
#56288=CARTESIAN_POINT('Ctrl Pts',(-18.2432033461838,-45.0937566270649,
123.719534287493)) ;
#56289=CARTESIAN_POINT('Ctrl Pts',(-17.951691989716,-44.9137675465844,123.796479325904)) ;
#56290=CARTESIAN_POINT('Ctrl Pts',(-18.3149935437228,-45.1038331913881,
123.918803697903)) ;
#56291=CARTESIAN_POINT('Ctrl Pts',(-18.0414310831757,-44.9238441109076,
124.045563596384)) ;
#56292=CARTESIAN_POINT('Ctrl Pts',(-18.4179463690853,-45.1136825165221,
124.098479005577)) ;
#56293=CARTESIAN_POINT('Ctrl Pts',(-18.1701298254122,-44.9336934360416,
124.2701600857)) ;
#56294=CARTESIAN_POINT('Ctrl Pts',(-18.5971230912793,-45.1270305161593,
124.314496308919)) ;
#56295=CARTESIAN_POINT('Ctrl Pts',(-18.3940753257468,-44.9470414356789,
124.540160290324)) ;
#56296=CARTESIAN_POINT('Ctrl Pts',(-18.8849989168967,-45.1436152756959,
124.518050402463)) ;
#56297=CARTESIAN_POINT('Ctrl Pts',(-18.7539725180067,-44.9636261952154,
124.794623795797)) ;
#56298=CARTESIAN_POINT('Ctrl Pts',(-19.224601952066,-45.160183827044,124.611932790248)) ;
#56299=CARTESIAN_POINT('Ctrl Pts',(-19.1783954642699,-44.9801947465635,
124.911954796787)) ;
#56300=CARTESIAN_POINT('Ctrl Pts',(-19.5054327742707,-45.173543651863,124.613960046694)) ;
#56301=CARTESIAN_POINT('Ctrl Pts',(-19.5295000394796,-44.9935545713825,
124.914496420961)) ;
#56302=CARTESIAN_POINT('Ctrl Pts',(-19.7108114161679,-45.1834490606937,
124.579447586727)) ;
#56303=CARTESIAN_POINT('Ctrl Pts',(-19.7862085515913,-45.0034599802132,
124.871351922951)) ;
#56304=CARTESIAN_POINT('Ctrl Pts',(-19.9082218453753,-45.1934090872777,
124.509714834404)) ;
#56305=CARTESIAN_POINT('Ctrl Pts',(-20.0329770476807,-45.0134200067972,
124.784181636003)) ;
#56306=CARTESIAN_POINT('Ctrl Pts',(-20.1511287525541,-45.206666671463,124.372952742759)) ;
#56307=CARTESIAN_POINT('Ctrl Pts',(-20.3365929404721,-45.0266775909825,
124.613239797446)) ;
#56308=CARTESIAN_POINT('Ctrl Pts',(-20.4042739888879,-45.2233178829577,
124.12545280733)) ;
#56309=CARTESIAN_POINT('Ctrl Pts',(-20.6530388480297,-45.0433288024772,
124.303846929878)) ;
#56310=CARTESIAN_POINT('Ctrl Pts',(-20.5876289534092,-45.243236097068,123.743705041852)) ;
#56311=CARTESIAN_POINT('Ctrl Pts',(-20.8822225930643,-45.0632470165875,
123.826665489857)) ;
#56312=CARTESIAN_POINT('Ctrl Pts',(-20.630530145128,-45.2631138602888,123.323172796485)) ;
#56313=CARTESIAN_POINT('Ctrl Pts',(-20.9358462102665,-45.0831247798083,
123.300999284678)) ;
#56314=CARTESIAN_POINT('Ctrl Pts',(-20.5263138562725,-45.283126528076,122.910688719133)) ;
#56315=CARTESIAN_POINT('Ctrl Pts',(-20.8055712373151,-45.1031374475955,
122.785395465241)) ;
#56316=CARTESIAN_POINT('Ctrl Pts',(-20.2902208181443,-45.3029390507426,
122.561698389052)) ;
#56317=CARTESIAN_POINT('Ctrl Pts',(-20.5104525720983,-45.1229499702621,
122.349160972054)) ;
#56318=CARTESIAN_POINT('Ctrl Pts',(-19.9467946863038,-45.3229223507425,
122.31164395972)) ;
#56319=CARTESIAN_POINT('Ctrl Pts',(-20.0811678726648,-45.142933270262,122.036595982088)) ;
#56320=CARTESIAN_POINT('Ctrl Pts',(-19.5402451083145,-45.3428166278438,
122.194572866398)) ;
#56321=CARTESIAN_POINT('Ctrl Pts',(-19.5729808271212,-45.1628275473633,
121.890260817215)) ;
#56322=CARTESIAN_POINT('Ctrl Pts',(-19.1173631256665,-45.3627493896015,
122.222652545081)) ;
#56323=CARTESIAN_POINT('Ctrl Pts',(-19.0443792387682,-45.1827603091211,
121.925363493059)) ;
#56324=CARTESIAN_POINT('Ctrl Pts',(-18.7289083515365,-45.3827153953663,
122.393915397857)) ;
#56325=CARTESIAN_POINT('Ctrl Pts',(-18.5588123387542,-45.2027263148858,
122.139444767304)) ;
#56326=CARTESIAN_POINT('Ctrl Pts',(-18.4233281728612,-45.4025939275311,
122.685968903404)) ;
#56327=CARTESIAN_POINT('Ctrl Pts',(-18.1768400074142,-45.2226048470507,
122.504512707757)) ;
#56328=CARTESIAN_POINT('Ctrl Pts',(-18.2348448265652,-45.4225335941915,
123.065690568163)) ;
#56329=CARTESIAN_POINT('Ctrl Pts',(-17.9412382744807,-45.242544513711,122.97916517486)) ;
#56330=CARTESIAN_POINT('Ctrl Pts',(-18.1872285477888,-45.4424284688368,
123.486065831409)) ;
#56331=CARTESIAN_POINT('Ctrl Pts',(-17.8817201355159,-45.2624393883564,
123.504633155364)) ;
#56332=CARTESIAN_POINT('Ctrl Pts',(-18.2855438839301,-45.4623356081302,
123.897669851793)) ;
#56333=CARTESIAN_POINT('Ctrl Pts',(-18.0046155635177,-45.2823465276497,
124.019136501182)) ;
#56334=CARTESIAN_POINT('Ctrl Pts',(-18.5179787925655,-45.4822461562087,
124.251671884329)) ;
#56335=CARTESIAN_POINT('Ctrl Pts',(-18.2951592683826,-45.3022570757282,
124.461637555515)) ;
#56336=CARTESIAN_POINT('Ctrl Pts',(-18.8603532025877,-45.5023147415659,
124.506196821107)) ;
#56337=CARTESIAN_POINT('Ctrl Pts',(-18.7231289191546,-45.3223256610853,
124.779793281065)) ;
#56338=CARTESIAN_POINT('Ctrl Pts',(-19.2632916538043,-45.5220965388806,
124.627332831793)) ;
#56339=CARTESIAN_POINT('Ctrl Pts',(-19.2267990765142,-45.3421074584001,
124.931211593352)) ;
#56340=CARTESIAN_POINT('Ctrl Pts',(-19.6879024854321,-45.5421040858251,
124.604065554752)) ;
#56341=CARTESIAN_POINT('Ctrl Pts',(-19.7575625515508,-45.3621150053447,
124.902127405383)) ;
#56342=CARTESIAN_POINT('Ctrl Pts',(-20.0757175915424,-45.561925824128,124.438753736194)) ;
#56343=CARTESIAN_POINT('Ctrl Pts',(-20.2423289588513,-45.3819367436475,
124.695488931314)) ;
#56344=CARTESIAN_POINT('Ctrl Pts',(-20.3866991980944,-45.5819058440321,
124.149413523319)) ;
#56345=CARTESIAN_POINT('Ctrl Pts',(-20.6310564600973,-45.4019167635517,
124.333814619586)) ;
#56346=CARTESIAN_POINT('Ctrl Pts',(-20.579213898747,-45.6018232952944,123.772183038511)) ;
#56347=CARTESIAN_POINT('Ctrl Pts',(-20.8717000557852,-45.4218342148139,
123.86227801888)) ;
#56348=CARTESIAN_POINT('Ctrl Pts',(-20.6323140250136,-45.6216982164671,
123.35290988801)) ;
#56349=CARTESIAN_POINT('Ctrl Pts',(-20.9380767682915,-45.4417091359866,
123.338188475174)) ;
#56350=CARTESIAN_POINT('Ctrl Pts',(-20.5381944095279,-45.6417225850179,
122.937699622663)) ;
#56351=CARTESIAN_POINT('Ctrl Pts',(-20.8204289203156,-45.4617335045374,
122.819174892928)) ;
#56352=CARTESIAN_POINT('Ctrl Pts',(-20.3096913478822,-45.6615892693914,
122.582336964708)) ;
#56353=CARTESIAN_POINT('Ctrl Pts',(-20.5348026193638,-45.4816001889109,
122.374971928243)) ;
#56354=CARTESIAN_POINT('Ctrl Pts',(-19.9728378596493,-45.6815330912376,
122.324818392206)) ;
#56355=CARTESIAN_POINT('Ctrl Pts',(-20.1137378288441,-45.5015440107571,
122.053072103545)) ;
#56356=CARTESIAN_POINT('Ctrl Pts',(-19.5689770807575,-45.7014404604891,
122.198058930962)) ;
#56357=CARTESIAN_POINT('Ctrl Pts',(-19.608913673455,-45.5214513800086,121.89462058423)) ;
#56358=CARTESIAN_POINT('Ctrl Pts',(-19.1467685091688,-45.7213151582358,
122.215906390113)) ;
#56359=CARTESIAN_POINT('Ctrl Pts',(-19.0811541091783,-45.5413260777553,
121.916926618802)) ;
#56360=CARTESIAN_POINT('Ctrl Pts',(-18.7538192203983,-45.7412971007575,
122.377543259028)) ;
#56361=CARTESIAN_POINT('Ctrl Pts',(-18.5899663031638,-45.5613080202771,
122.118969492211)) ;
#56362=CARTESIAN_POINT('Ctrl Pts',(-18.4411535486972,-45.7611997676684,
122.662651717635)) ;
#56363=CARTESIAN_POINT('Ctrl Pts',(-18.1991325994995,-45.5812106871879,
122.475351878632)) ;
#56364=CARTESIAN_POINT('Ctrl Pts',(-18.2438603449424,-45.7810551252071,
123.035964325074)) ;
#56365=CARTESIAN_POINT('Ctrl Pts',(-17.9525130134343,-45.6010660447266,
122.941989689319)) ;
#56366=CARTESIAN_POINT('Ctrl Pts',(-18.1856815046609,-45.8011191639231,
123.458527247341)) ;
#56367=CARTESIAN_POINT('Ctrl Pts',(-17.879785330471,-45.6211300834426,123.47019336816)) ;
#56368=CARTESIAN_POINT('Ctrl Pts',(-18.2744755391468,-45.8209743436481,
123.871419259032)) ;
#56369=CARTESIAN_POINT('Ctrl Pts',(-17.9907738384312,-45.6409852631677,
123.986308188101)) ;
#56370=CARTESIAN_POINT('Ctrl Pts',(-18.4997930018078,-45.8409544483126,
124.231383616986)) ;
#56371=CARTESIAN_POINT('Ctrl Pts',(-18.2724161798347,-45.6609653678321,
124.4362659272)) ;
#56372=CARTESIAN_POINT('Ctrl Pts',(-18.8314673108359,-45.8607635534824,
124.49118909027)) ;
#56373=CARTESIAN_POINT('Ctrl Pts',(-18.6870078951238,-45.6807744730019,
124.761025281512)) ;
#56374=CARTESIAN_POINT('Ctrl Pts',(-19.2352299421936,-45.8807561738231,
124.623756846675)) ;
#56375=CARTESIAN_POINT('Ctrl Pts',(-19.1916999501142,-45.7007670933426,
124.926741075057)) ;
#56376=CARTESIAN_POINT('Ctrl Pts',(-19.586815630739,-45.8972956563272,124.612921446625)) ;
#56377=CARTESIAN_POINT('Ctrl Pts',(-19.6312118173661,-45.7173065758467,
124.913196410162)) ;
#56378=CARTESIAN_POINT('Ctrl Pts',(-19.8558718361537,-45.9106599743914,
124.532044526927)) ;
#56379=CARTESIAN_POINT('Ctrl Pts',(-19.9674993569513,-45.7306708939109,
124.812112387827)) ;
#56380=CARTESIAN_POINT('Ctrl Pts',(-20.1042094269978,-45.9238775768929,
124.407362624785)) ;
#56381=CARTESIAN_POINT('Ctrl Pts',(-20.2779790595756,-45.7438884964124,
124.656227492583)) ;
#56382=CARTESIAN_POINT('Ctrl Pts',(-20.368961477355,-45.9405351711707,124.172135837994)) ;
#56383=CARTESIAN_POINT('Ctrl Pts',(-20.6088613727262,-45.7605460906902,
124.362235325877)) ;
#56384=CARTESIAN_POINT('Ctrl Pts',(-20.5701552804557,-45.9604008732124,
123.800652640584)) ;
#56385=CARTESIAN_POINT('Ctrl Pts',(-20.8603771683471,-45.7804117927319,
123.897882286037)) ;
#56386=CARTESIAN_POINT('Ctrl Pts',(-20.6228240088762,-45.9770305999024,
123.451100482239)) ;
#56387=CARTESIAN_POINT('Ctrl Pts',(-20.9262145453754,-45.797041519422,123.460911151543)) ;
#56388=CARTESIAN_POINT('Ctrl Pts',(-20.5914361189551,-45.9903197150403,
123.173415800151)) ;
#56389=CARTESIAN_POINT('Ctrl Pts',(-20.8869828201664,-45.8103306345598,
123.113835882185)) ;
#56390=CARTESIAN_POINT('Ctrl Pts',(-20.5323594467668,-46.0002840620174,
122.972457040269)) ;
#56391=CARTESIAN_POINT('Ctrl Pts',(-20.8131372218145,-45.8202949815369,
122.862628157977)) ;
#56392=CARTESIAN_POINT('Ctrl Pts',(-20.4397374973719,-46.0102124300189,
122.785404683368)) ;
#56393=CARTESIAN_POINT('Ctrl Pts',(-20.6973720960677,-45.8302233495384,
122.628822672009)) ;
#56394=CARTESIAN_POINT('Ctrl Pts',(-20.2747057487913,-46.0234958631076,
122.560148912213)) ;
#56395=CARTESIAN_POINT('Ctrl Pts',(-20.4910362461603,-45.8435067826271,
122.347203200307)) ;
#56396=CARTESIAN_POINT('Ctrl Pts',(-19.9984819879349,-46.0401479408479,
122.338567938627)) ;
#56397=CARTESIAN_POINT('Ctrl Pts',(-20.1458260850782,-45.8601588603674,
122.070280119361)) ;
#56398=CARTESIAN_POINT('Ctrl Pts',(-19.6654083029669,-46.0566993101488,
122.225111293764)) ;
#56399=CARTESIAN_POINT('Ctrl Pts',(-19.7294257177977,-45.8767102296683,
121.928426697148)) ;
#56400=CARTESIAN_POINT('Ctrl Pts',(-19.3866709636188,-46.0699867382977,
122.205956450198)) ;
#56401=CARTESIAN_POINT('Ctrl Pts',(-19.3810452958533,-45.8899976578173,
121.904492705399)) ;
#56402=CARTESIAN_POINT('Ctrl Pts',(-19.1767289526485,-46.0800312779978,
122.228493274204)) ;
#56403=CARTESIAN_POINT('Ctrl Pts',(-19.1186091401269,-45.9000421975174,
121.932658290832)) ;
#56404=CARTESIAN_POINT('Ctrl Pts',(-18.9778591393557,-46.0898741198217,
122.285724273761)) ;
#56405=CARTESIAN_POINT('Ctrl Pts',(-18.8700233534441,-45.9098850393412,
122.004195044946)) ;
#56406=CARTESIAN_POINT('Ctrl Pts',(-18.7890949169887,-46.0998584040686,
122.37747258679)) ;
#56407=CARTESIAN_POINT('Ctrl Pts',(-18.6340661749216,-45.9198693235881,
122.118877741015)) ;
#56408=CARTESIAN_POINT('Ctrl Pts',(-18.6197187705816,-46.1098080494678,
122.500228764062)) ;
#56409=CARTESIAN_POINT('Ctrl Pts',(-18.4223444456652,-45.9298189689873,
122.272320772466)) ;
#56410=CARTESIAN_POINT('Ctrl Pts',(-18.4733104190095,-46.1198078111562,
122.651108437036)) ;
#56411=CARTESIAN_POINT('Ctrl Pts',(-18.2393318881678,-45.9398187306757,
122.460918444063)) ;
#56412=CARTESIAN_POINT('Ctrl Pts',(-18.3552472327061,-46.1298391571151,
122.825850445849)) ;
#56413=CARTESIAN_POINT('Ctrl Pts',(-18.0917505485482,-45.9498500766346,
122.679344429052)) ;
#56414=CARTESIAN_POINT('Ctrl Pts',(-18.2705494607926,-46.1396941115922,
123.014933391385)) ;
#56415=CARTESIAN_POINT('Ctrl Pts',(-17.9858757130869,-45.9597050311117,
122.91569706194)) ;
#56416=CARTESIAN_POINT('Ctrl Pts',(-18.2188977661992,-46.1496666495927,
123.218103084829)) ;
#56417=CARTESIAN_POINT('Ctrl Pts',(-17.9213083459026,-45.9696775691122,
123.169658598768)) ;
#56418=CARTESIAN_POINT('Ctrl Pts',(-18.2032838337834,-46.1596616433277,
123.427680803576)) ;
#56419=CARTESIAN_POINT('Ctrl Pts',(-17.9017881315009,-45.9796725628472,
123.431630618323)) ;
#56420=CARTESIAN_POINT('Ctrl Pts',(-18.2246312081846,-46.1696957021218,
123.637527281541)) ;
#56421=CARTESIAN_POINT('Ctrl Pts',(-17.9284695513896,-45.9897066216413,
123.693939039841)) ;
#56422=CARTESIAN_POINT('Ctrl Pts',(-18.2807599390842,-46.1795510449448,
123.836991427032)) ;
#56423=CARTESIAN_POINT('Ctrl Pts',(-17.9986278341019,-45.9995619644643,
123.943270201465)) ;
#56424=CARTESIAN_POINT('Ctrl Pts',(-18.3717042160913,-46.1895505242904,
124.026480311802)) ;
#56425=CARTESIAN_POINT('Ctrl Pts',(-18.1123057055239,-46.0095614438099,
124.180132595363)) ;
#56426=CARTESIAN_POINT('Ctrl Pts',(-18.4927341945723,-46.1994449730457,
124.195705746537)) ;
#56427=CARTESIAN_POINT('Ctrl Pts',(-18.2635910837265,-46.0194558925652,
124.391666206206)) ;
#56428=CARTESIAN_POINT('Ctrl Pts',(-18.6438307854289,-46.2095080924802,
124.343730651591)) ;
#56429=CARTESIAN_POINT('Ctrl Pts',(-18.4524598571284,-46.0295190119997,
124.576699295211)) ;
#56430=CARTESIAN_POINT('Ctrl Pts',(-18.8143876956358,-46.2193477377214,
124.460844662452)) ;
#56431=CARTESIAN_POINT('Ctrl Pts',(-18.6656547762322,-46.0393586572409,
124.72309430424)) ;
#56432=CARTESIAN_POINT('Ctrl Pts',(-19.0067961425218,-46.2294109019075,
124.548731031768)) ;
#56433=CARTESIAN_POINT('Ctrl Pts',(-18.9061641631857,-46.049421821427,124.832954725932)) ;
#56434=CARTESIAN_POINT('Ctrl Pts',(-19.2082002254343,-46.2393051716563,
124.60082520619)) ;
#56435=CARTESIAN_POINT('Ctrl Pts',(-19.157918897676,-46.0593160911758,124.898075179846)) ;
#56436=CARTESIAN_POINT('Ctrl Pts',(-19.4164887508991,-46.2492468976701,
124.617795648775)) ;
#56437=CARTESIAN_POINT('Ctrl Pts',(-19.4182795982732,-46.0692578171896,
124.919290922876)) ;
#56438=CARTESIAN_POINT('Ctrl Pts',(-19.625908760725,-46.2592497863295,124.598307790084)) ;
#56439=CARTESIAN_POINT('Ctrl Pts',(-19.6800549446301,-46.079260705849,124.894933738514)) ;
#56440=CARTESIAN_POINT('Ctrl Pts',(-19.8293605211461,-46.2692896351235,
124.542189850238)) ;
#56441=CARTESIAN_POINT('Ctrl Pts',(-19.934370335903,-46.089300554643,124.824788940048)) ;
#56442=CARTESIAN_POINT('Ctrl Pts',(-20.0161177451334,-46.2791138505843,
124.453953136808)) ;
#56443=CARTESIAN_POINT('Ctrl Pts',(-20.1678185634973,-46.0991247701039,
124.714495173681)) ;
#56444=CARTESIAN_POINT('Ctrl Pts',(-20.1888529807882,-46.2891706940779,
124.332063949481)) ;
#56445=CARTESIAN_POINT('Ctrl Pts',(-20.3837390424516,-46.1091816135974,
124.562135863829)) ;
#56446=CARTESIAN_POINT('Ctrl Pts',(-20.3357237419567,-46.2990993034739,
124.183735609964)) ;
#56447=CARTESIAN_POINT('Ctrl Pts',(-20.5673296045431,-46.1191102229934,
124.376727071138)) ;
#56448=CARTESIAN_POINT('Ctrl Pts',(-20.4553698807106,-46.3090511875118,
124.012092768846)) ;
#56449=CARTESIAN_POINT('Ctrl Pts',(-20.7168895337345,-46.1290621070313,
124.162174745084)) ;
#56450=CARTESIAN_POINT('Ctrl Pts',(-20.5439344328811,-46.3191041403194,
123.820215375579)) ;
#56451=CARTESIAN_POINT('Ctrl Pts',(-20.8275975549194,-46.1391150598389,
123.922329195925)) ;
#56452=CARTESIAN_POINT('Ctrl Pts',(-20.5969834126444,-46.3289270167856,
123.620621819729)) ;
#56453=CARTESIAN_POINT('Ctrl Pts',(-20.8939114404305,-46.1489379363051,
123.67283715283)) ;
#56454=CARTESIAN_POINT('Ctrl Pts',(-20.6153551246027,-46.3389827493557,
123.41003275426)) ;
#56455=CARTESIAN_POINT('Ctrl Pts',(-20.9168785396569,-46.1589936688752,
123.409601144835)) ;
#56456=CARTESIAN_POINT('Ctrl Pts',(-20.5967235165246,-46.3489235143433,
123.201871132053)) ;
#56457=CARTESIAN_POINT('Ctrl Pts',(-20.8935915402099,-46.1689344338629,
123.149398558152)) ;
#56458=CARTESIAN_POINT('Ctrl Pts',(-20.5430611916777,-46.358827847249,123.000680696278)) ;
#56459=CARTESIAN_POINT('Ctrl Pts',(-20.8265158342025,-46.1788387667685,
122.897909377553)) ;
#56460=CARTESIAN_POINT('Ctrl Pts',(-20.4539067996073,-46.3688745161297,
122.809226303737)) ;
#56461=CARTESIAN_POINT('Ctrl Pts',(-20.715075105304,-46.1888854356492,122.658590446678)) ;
#56462=CARTESIAN_POINT('Ctrl Pts',(-20.3348107304018,-46.3787700794355,
122.638612779929)) ;
#56463=CARTESIAN_POINT('Ctrl Pts',(-20.5662066577378,-46.198780998955,122.445321690395)) ;
#56464=CARTESIAN_POINT('Ctrl Pts',(-20.1854730789962,-46.3888321371358,
122.48883600952)) ;
#56465=CARTESIAN_POINT('Ctrl Pts',(-20.3795364262878,-46.2088430566553,
122.258099155421)) ;
#56466=CARTESIAN_POINT('Ctrl Pts',(-20.0161942508695,-46.3986749147633,
122.369786755293)) ;
#56467=CARTESIAN_POINT('Ctrl Pts',(-20.1679385536693,-46.2186858342828,
122.109285146046)) ;
#56468=CARTESIAN_POINT('Ctrl Pts',(-19.8262618796166,-46.4086653930151,
122.28019126902)) ;
#56469=CARTESIAN_POINT('Ctrl Pts',(-19.9305238989034,-46.2286763125346,
121.997288664706)) ;
#56470=CARTESIAN_POINT('Ctrl Pts',(-19.6248584878059,-46.4185943656587,
122.225294019457)) ;
#56471=CARTESIAN_POINT('Ctrl Pts',(-19.6787697822152,-46.2386052851782,
121.928664785981)) ;
#56472=CARTESIAN_POINT('Ctrl Pts',(-19.4157226032529,-46.4285855025382,
122.205756739938)) ;
#56473=CARTESIAN_POINT('Ctrl Pts',(-19.417349965525,-46.2485964220577,121.904240994479)) ;
#56474=CARTESIAN_POINT('Ctrl Pts',(-19.2057405057304,-46.4386076200272,
122.223135749663)) ;
#56475=CARTESIAN_POINT('Ctrl Pts',(-19.1548721753179,-46.2586185395467,
121.925962509056)) ;
#56476=CARTESIAN_POINT('Ctrl Pts',(-19.0043894905299,-46.4485081304294,
122.275869896389)) ;
#56477=CARTESIAN_POINT('Ctrl Pts',(-18.9031822161393,-46.2685190499489,
121.991878228629)) ;
#56478=CARTESIAN_POINT('Ctrl Pts',(-18.813429020907,-46.4584971231755,122.363241063598)) ;
#56479=CARTESIAN_POINT('Ctrl Pts',(-18.664480581697,-46.278508042695,122.101090338607)) ;
#56480=CARTESIAN_POINT('Ctrl Pts',(-18.6410397094411,-46.4684623672261,
122.482274292673)) ;
#56481=CARTESIAN_POINT('Ctrl Pts',(-18.4489924496147,-46.2884732867456,
122.249880282336)) ;
#56482=CARTESIAN_POINT('Ctrl Pts',(-18.4924874516743,-46.4783666317393,
122.62819862701)) ;
#56483=CARTESIAN_POINT('Ctrl Pts',(-18.2633002249864,-46.2983775512588,
122.432284741212)) ;
#56484=CARTESIAN_POINT('Ctrl Pts',(-18.3697789016585,-46.4884247234375,
122.800382922365)) ;
#56485=CARTESIAN_POINT('Ctrl Pts',(-18.1099129935888,-46.308435642957,122.64751372994)) ;
#56486=CARTESIAN_POINT('Ctrl Pts',(-18.2805605389299,-46.4982746638659,
122.987267125253)) ;
#56487=CARTESIAN_POINT('Ctrl Pts',(-17.9983877778313,-46.3182855833854,
122.881119052142)) ;
#56488=CARTESIAN_POINT('Ctrl Pts',(-18.2236525306218,-46.5083016750394,
123.190235923869)) ;
#56489=CARTESIAN_POINT('Ctrl Pts',(-17.9272509865239,-46.328312594559,123.134829512504)) ;
#56490=CARTESIAN_POINT('Ctrl Pts',(-18.2033939632025,-46.5183302616515,
123.400103024954)) ;
#56491=CARTESIAN_POINT('Ctrl Pts',(-17.901925769239,-46.338341181171,123.397163125624)) ;
#56492=CARTESIAN_POINT('Ctrl Pts',(-18.2191889497681,-46.5281754757642,
123.606465447685)) ;
#56493=CARTESIAN_POINT('Ctrl Pts',(-17.9216676870494,-46.3481863952837,
123.655117412485)) ;
#56494=CARTESIAN_POINT('Ctrl Pts',(-18.2707942324504,-46.5381662239437,
123.810069040328)) ;
#56495=CARTESIAN_POINT('Ctrl Pts',(-17.9861726595003,-46.3581771434633,
123.909622518331)) ;
#56496=CARTESIAN_POINT('Ctrl Pts',(-18.357794261464,-46.5482038575292,124.002323055344)) ;
#56497=CARTESIAN_POINT('Ctrl Pts',(-18.0949209306796,-46.3682147770488,
124.14994069115)) ;
#56498=CARTESIAN_POINT('Ctrl Pts',(-18.4742897524447,-46.5580491467421,
124.173407953581)) ;
#56499=CARTESIAN_POINT('Ctrl Pts',(-18.2405394894206,-46.3780600662616,
124.363798772885)) ;
#56500=CARTESIAN_POINT('Ctrl Pts',(-18.620370895161,-46.568030547548,124.324028601828)) ;
#56501=CARTESIAN_POINT('Ctrl Pts',(-18.4231399412858,-46.3880414670675,
124.552075901862)) ;
#56502=CARTESIAN_POINT('Ctrl Pts',(-18.7899363735675,-46.5779827805379,
124.44660926478)) ;
#56503=CARTESIAN_POINT('Ctrl Pts',(-18.6350962162667,-46.3979937000574,
124.705303330032)) ;
#56504=CARTESIAN_POINT('Ctrl Pts',(-18.9789812034734,-46.5879815919945,
124.538563788364)) ;
#56505=CARTESIAN_POINT('Ctrl Pts',(-18.8714017008024,-46.4079925115141,
124.82024792927)) ;
#56506=CARTESIAN_POINT('Ctrl Pts',(-19.1820191632644,-46.5980206959252,
124.596131546056)) ;
#56507=CARTESIAN_POINT('Ctrl Pts',(-19.1251985398455,-46.4180316154447,
124.89220920167)) ;
#56508=CARTESIAN_POINT('Ctrl Pts',(-19.3874680290362,-46.6078456383445,
124.617557565118)) ;
#56509=CARTESIAN_POINT('Ctrl Pts',(-19.3820108279074,-46.427856557864,124.918993385789)) ;
#56510=CARTESIAN_POINT('Ctrl Pts',(-19.5983341246022,-46.6179003258204,
124.602993200605)) ;
#56511=CARTESIAN_POINT('Ctrl Pts',(-19.6455932893009,-46.43791124534,124.900789356914)) ;
#56512=CARTESIAN_POINT('Ctrl Pts',(-19.8011174374927,-46.6278431281773,
124.552252454525)) ;
#56513=CARTESIAN_POINT('Ctrl Pts',(-19.8990733416014,-46.4478540476968,
124.837364781707)) ;
#56514=CARTESIAN_POINT('Ctrl Pts',(-19.9915187465345,-46.637746924117,124.467991218211)) ;
#56515=CARTESIAN_POINT('Ctrl Pts',(-20.1370762829352,-46.4577578436366,
124.732039091095)) ;
#56516=CARTESIAN_POINT('Ctrl Pts',(-20.166805154378,-46.6477937034921,124.350181343917)) ;
#56517=CARTESIAN_POINT('Ctrl Pts',(-20.3561848752623,-46.4678046230116,
124.584777991546)) ;
#56518=CARTESIAN_POINT('Ctrl Pts',(-20.3168442450622,-46.6576893617867,
124.20602634747)) ;
#56519=CARTESIAN_POINT('Ctrl Pts',(-20.543735289133,-46.4777002813062,124.40458454626)) ;
#56520=CARTESIAN_POINT('Ctrl Pts',(-20.4416202810829,-46.6677509290373,
124.035249876144)) ;
#56521=CARTESIAN_POINT('Ctrl Pts',(-20.6997061795947,-46.4877618485568,
124.191114977129)) ;
#56522=CARTESIAN_POINT('Ctrl Pts',(-20.5328807367812,-46.6775955734746,
123.849484643393)) ;
#56523=CARTESIAN_POINT('Ctrl Pts',(-20.8137834734582,-46.4976064929941,
123.958907813388)) ;
#56524=CARTESIAN_POINT('Ctrl Pts',(-20.5918946295246,-46.6875556197173,
123.64858424823)) ;
#56525=CARTESIAN_POINT('Ctrl Pts',(-20.8875519246108,-46.5075665392368,
123.707782162161)) ;
#56526=CARTESIAN_POINT('Ctrl Pts',(-20.6148993357899,-46.6975939157357,
123.43881520395)) ;
#56527=CARTESIAN_POINT('Ctrl Pts',(-20.9163089329228,-46.5176048352552,
123.445571143077)) ;
#56528=CARTESIAN_POINT('Ctrl Pts',(-20.6017530846061,-46.707467257154,123.231632331)) ;
#56529=CARTESIAN_POINT('Ctrl Pts',(-20.899877045935,-46.5274781766735,123.186591367216)) ;
#56530=CARTESIAN_POINT('Ctrl Pts',(-20.5517975292825,-46.7175403609533,
123.025882379625)) ;
#56531=CARTESIAN_POINT('Ctrl Pts',(-20.8374336992081,-46.5375512804728,
122.929404099157)) ;
#56532=CARTESIAN_POINT('Ctrl Pts',(-20.4692073505912,-46.7273611760722,
122.836612568494)) ;
#56533=CARTESIAN_POINT('Ctrl Pts',(-20.7341962067756,-46.5473720955917,
122.692815045702)) ;
#56534=CARTESIAN_POINT('Ctrl Pts',(-20.3522770027166,-46.7374380411502,
122.660005076197)) ;
#56535=CARTESIAN_POINT('Ctrl Pts',(-20.5880342151394,-46.5574489606697,
122.472055591139)) ;
#56536=CARTESIAN_POINT('Ctrl Pts',(-20.2094265317654,-46.7473027808054,
122.509626266143)) ;
#56537=CARTESIAN_POINT('Ctrl Pts',(-20.4094709148252,-46.567313700325,122.284080598722)) ;
#56538=CARTESIAN_POINT('Ctrl Pts',(-20.0403249054971,-46.7573251840468,
122.383941295046)) ;
#56539=CARTESIAN_POINT('Ctrl Pts',(-20.1980943114784,-46.5773361035663,
122.126973882571)) ;
#56540=CARTESIAN_POINT('Ctrl Pts',(-19.8516517065092,-46.7673509083353,
122.28995820191)) ;
#56541=CARTESIAN_POINT('Ctrl Pts',(-19.9622532731343,-46.5873618278548,
122.009494284939)) ;
#56542=CARTESIAN_POINT('Ctrl Pts',(-19.6531005041751,-46.7772056913566,
122.23083936213)) ;
#56543=CARTESIAN_POINT('Ctrl Pts',(-19.7140632034774,-46.5972166108761,
121.935594664426)) ;
#56544=CARTESIAN_POINT('Ctrl Pts',(-19.4447550366577,-46.7871845350798,
122.206249292003)) ;
#56545=CARTESIAN_POINT('Ctrl Pts',(-19.4536310994528,-46.6071954545993,
121.904856532566)) ;
#56546=CARTESIAN_POINT('Ctrl Pts',(-19.2345000747721,-46.7972034273165,
122.218618665142)) ;
#56547=CARTESIAN_POINT('Ctrl Pts',(-19.1908123744356,-46.617214346836,121.92031760061)) ;
#56548=CARTESIAN_POINT('Ctrl Pts',(-19.0322268033516,-46.8070866363575,
122.266237363921)) ;
#56549=CARTESIAN_POINT('Ctrl Pts',(-18.9379696063433,-46.627097555877,121.979840758441)) ;
#56550=CARTESIAN_POINT('Ctrl Pts',(-18.8378107169686,-46.8171549456977,
122.349847749281)) ;
#56551=CARTESIAN_POINT('Ctrl Pts',(-18.6949496715749,-46.6371658652172,
122.084353103891)) ;
#56552=CARTESIAN_POINT('Ctrl Pts',(-18.6648606133521,-46.8269850710304,
122.463033827998)) ;
#56553=CARTESIAN_POINT('Ctrl Pts',(-18.4787605239549,-46.6469959905499,
122.225836194773)) ;
#56554=CARTESIAN_POINT('Ctrl Pts',(-18.5104293304733,-46.8370516234074,
122.607686193805)) ;
#56555=CARTESIAN_POINT('Ctrl Pts',(-18.2857214964701,-46.6570625429269,
122.406651152064)) ;
#56556=CARTESIAN_POINT('Ctrl Pts',(-18.3857520045829,-46.8469418603011,
122.774114785356)) ;
#56557=CARTESIAN_POINT('Ctrl Pts',(-18.1298739185051,-46.6669527798206,
122.614687511464)) ;
#56558=CARTESIAN_POINT('Ctrl Pts',(-18.2905056904675,-46.8569340850951,
122.961335246674)) ;
#56559=CARTESIAN_POINT('Ctrl Pts',(-18.0108157651648,-46.6769450046146,
122.848713195555)) ;
#56560=CARTESIAN_POINT('Ctrl Pts',(-18.2295789136963,-46.866896705446,123.161719579238)) ;
#56561=CARTESIAN_POINT('Ctrl Pts',(-17.9346569100172,-46.6869076249655,
123.099193972004)) ;
#56562=CARTESIAN_POINT('Ctrl Pts',(-18.2040027326687,-46.8768017082092,
123.368391035254)) ;
#56563=CARTESIAN_POINT('Ctrl Pts',(-17.9026865140043,-46.6968126277287,
123.357534213853)) ;
#56564=CARTESIAN_POINT('Ctrl Pts',(-18.2150087934461,-46.8868594706073,
123.579531972586)) ;
#56565=CARTESIAN_POINT('Ctrl Pts',(-17.9164439566252,-46.7068703901268,
123.621460054312)) ;
#56566=CARTESIAN_POINT('Ctrl Pts',(-18.261371220002,-46.8967099899861,123.781380377064)) ;
#56567=CARTESIAN_POINT('Ctrl Pts',(-17.9743972613134,-46.7167209095056,
123.873771940626)) ;
#56568=CARTESIAN_POINT('Ctrl Pts',(-18.3431220571985,-46.9067415669843,
123.975771653837)) ;
#56569=CARTESIAN_POINT('Ctrl Pts',(-18.0765858905938,-46.7267524865038,
124.116760874247)) ;
#56570=CARTESIAN_POINT('Ctrl Pts',(-18.4574955443547,-46.9167513020892,
124.152440425366)) ;
#56571=CARTESIAN_POINT('Ctrl Pts',(-18.2195527490337,-46.7367622216087,
124.337596889066)) ;
#56572=CARTESIAN_POINT('Ctrl Pts',(-18.5992104285265,-46.9266608787155,
124.305119300968)) ;
#56573=CARTESIAN_POINT('Ctrl Pts',(-18.3966970017583,-46.746671798235,124.528446109201)) ;
#56574=CARTESIAN_POINT('Ctrl Pts',(-18.765279645767,-46.9365882645721,124.431541302977)) ;
#56575=CARTESIAN_POINT('Ctrl Pts',(-18.6042842737246,-46.7565991840916,
124.6864738575)) ;
#56576=CARTESIAN_POINT('Ctrl Pts',(-18.9530362774689,-46.9466331990624,
124.528179929632)) ;
#56577=CARTESIAN_POINT('Ctrl Pts',(-18.8389799600017,-46.7666441185819,
124.807271873958)) ;
#56578=CARTESIAN_POINT('Ctrl Pts',(-19.151511474355,-46.9565191312504,124.589883618221)) ;
#56579=CARTESIAN_POINT('Ctrl Pts',(-19.0870750670276,-46.7765300507699,
124.88440157674)) ;
#56580=CARTESIAN_POINT('Ctrl Pts',(-19.3598549427328,-46.9665124372034,
124.616830207834)) ;
#56581=CARTESIAN_POINT('Ctrl Pts',(-19.3475046537263,-46.7865233567229,
124.918084459642)) ;
#56582=CARTESIAN_POINT('Ctrl Pts',(-19.5687199932944,-46.9764580749853,
124.607155449397)) ;
#56583=CARTESIAN_POINT('Ctrl Pts',(-19.6085865454155,-46.7964689945048,
124.90599063429)) ;
#56584=CARTESIAN_POINT('Ctrl Pts',(-19.7728690713917,-46.9864053433312,
124.561770557663)) ;
#56585=CARTESIAN_POINT('Ctrl Pts',(-19.8637733414417,-46.8064162628507,
124.849258887938)) ;
#56586=CARTESIAN_POINT('Ctrl Pts',(-19.9678843674529,-46.9964532454683,
124.480604259967)) ;
#56587=CARTESIAN_POINT('Ctrl Pts',(-20.1075420667976,-46.8164641649878,
124.747800719833)) ;
#56588=CARTESIAN_POINT('Ctrl Pts',(-20.1423977281203,-47.0063009403085,
124.369220465197)) ;
#56589=CARTESIAN_POINT('Ctrl Pts',(-20.3256846822976,-46.826311859828,124.608569806674)) ;
#56590=CARTESIAN_POINT('Ctrl Pts',(-20.2971232610949,-47.0162624500529,
124.228102585513)) ;
#56591=CARTESIAN_POINT('Ctrl Pts',(-20.519091428177,-46.8362733695724,124.432171593278)) ;
#56592=CARTESIAN_POINT('Ctrl Pts',(-20.4256537019022,-47.0262918416617,
124.060947461949)) ;
#56593=CARTESIAN_POINT('Ctrl Pts',(-20.6797539091981,-46.8463027611812,
124.223227378317)) ;
#56594=CARTESIAN_POINT('Ctrl Pts',(-20.5221200134929,-47.0361993372165,
123.876344757324)) ;
#56595=CARTESIAN_POINT('Ctrl Pts',(-20.800336605689,-46.856210256736,123.992472885805)) ;
#56596=CARTESIAN_POINT('Ctrl Pts',(-20.585700963853,-47.0461447288795,123.677180951145)) ;
#56597=CARTESIAN_POINT('Ctrl Pts',(-20.8798121651534,-46.866155648399,123.743517316037)) ;
#56598=CARTESIAN_POINT('Ctrl Pts',(-20.6140236281274,-47.0561466464769,
123.468796635054)) ;
#56599=CARTESIAN_POINT('Ctrl Pts',(-20.9152146259637,-46.8761575659964,
123.483036674989)) ;
#56600=CARTESIAN_POINT('Ctrl Pts',(-20.6053144754768,-47.0661867140291,
123.257921725322)) ;
#56601=CARTESIAN_POINT('Ctrl Pts',(-20.9043274471141,-46.8861976335486,
123.219443241582)) ;
#56602=CARTESIAN_POINT('Ctrl Pts',(-20.5615451992037,-47.0760110254689,
123.056057517403)) ;
#56603=CARTESIAN_POINT('Ctrl Pts',(-20.8496146262616,-46.8960219449884,
122.967111685171)) ;
#56604=CARTESIAN_POINT('Ctrl Pts',(-20.48182941958,-47.086067266625,122.860270767228)) ;
#56605=CARTESIAN_POINT('Ctrl Pts',(-20.7499690605305,-46.9060781861445,
122.722378927927)) ;
#56606=CARTESIAN_POINT('Ctrl Pts',(-20.3705003700426,-47.0959981883606,
122.683623151021)) ;
#56607=CARTESIAN_POINT('Ctrl Pts',(-20.6108065949588,-46.9160091078801,
122.501569334424)) ;
#56608=CARTESIAN_POINT('Ctrl Pts',(-20.2303667268952,-47.1059414244368,
122.528548074826)) ;
#56609=CARTESIAN_POINT('Ctrl Pts',(-20.4356383207007,-46.9259523439564,
122.307725777316)) ;
#56610=CARTESIAN_POINT('Ctrl Pts',(-20.0648823735269,-47.1159227084493,
122.399473602791)) ;
#56611=CARTESIAN_POINT('Ctrl Pts',(-20.2287819480132,-46.9359336279688,
122.146383449946)) ;
#56612=CARTESIAN_POINT('Ctrl Pts',(-19.878210560702,-47.125967010075,122.300821311272)) ;
#56613=CARTESIAN_POINT('Ctrl Pts',(-19.9954418663131,-46.9459779295945,
122.023069093514)) ;
#56614=CARTESIAN_POINT('Ctrl Pts',(-19.6816640223288,-47.1357950912944,
122.236998796321)) ;
#56615=CARTESIAN_POINT('Ctrl Pts',(-19.7497569427721,-46.9558060108139,
121.943291660631)) ;
#56616=CARTESIAN_POINT('Ctrl Pts',(-19.4719363919362,-47.1458716941436,
122.207454533547)) ;
#56617=CARTESIAN_POINT('Ctrl Pts',(-19.4875976586612,-46.9658826136631,
121.906362635453)) ;
#56618=CARTESIAN_POINT('Ctrl Pts',(-19.2648901369236,-47.1557237732621,
122.214511172754)) ;
#56619=CARTESIAN_POINT('Ctrl Pts',(-19.2287886486704,-46.9757346927816,
121.915184765219)) ;
#56620=CARTESIAN_POINT('Ctrl Pts',(-19.0577050674081,-47.165797031571,122.258180662651)) ;
#56621=CARTESIAN_POINT('Ctrl Pts',(-18.9698079848751,-46.9858079510905,
121.969772870427)) ;
#56622=CARTESIAN_POINT('Ctrl Pts',(-18.8657477434276,-47.1756384909513,
122.335414466867)) ;
#56623=CARTESIAN_POINT('Ctrl Pts',(-18.7298606157997,-46.9956494104708,
122.066316849402)) ;
#56624=CARTESIAN_POINT('Ctrl Pts',(-18.6875856486329,-47.1855995863637,
122.445455661587)) ;
#56625=CARTESIAN_POINT('Ctrl Pts',(-18.5071584974101,-47.0056105058832,
122.2038699234)) ;
#56626=CARTESIAN_POINT('Ctrl Pts',(-18.5303140250955,-47.1956368707604,
122.586136597021)) ;
#56627=CARTESIAN_POINT('Ctrl Pts',(-18.3105700405219,-47.0156477902799,
122.379722097128)) ;
#56628=CARTESIAN_POINT('Ctrl Pts',(-18.4016481952308,-47.2055132094957,
122.749125228209)) ;
#56629=CARTESIAN_POINT('Ctrl Pts',(-18.1497383798912,-47.0255241290152,
122.583459652687)) ;
#56630=CARTESIAN_POINT('Ctrl Pts',(-18.3013741603539,-47.2155753356489,
122.935356273905)) ;
#56631=CARTESIAN_POINT('Ctrl Pts',(-18.0243973837538,-47.0355862551685,
122.816248967621)) ;
#56632=CARTESIAN_POINT('Ctrl Pts',(-18.2361754948208,-47.2254435096255,
123.132331116174)) ;
#56633=CARTESIAN_POINT('Ctrl Pts',(-17.9429002610054,-47.045454429145,123.06246901578)) ;
#56634=CARTESIAN_POINT('Ctrl Pts',(-18.205338043931,-47.2354490581293,123.340378376433)) ;
#56635=CARTESIAN_POINT('Ctrl Pts',(-17.9043551710832,-47.0554599776488,
123.322528432353)) ;
#56636=CARTESIAN_POINT('Ctrl Pts',(-18.2111535129992,-47.2454316900249,
123.550202526117)) ;
#56637=CARTESIAN_POINT('Ctrl Pts',(-17.9116262440273,-47.0654426095444,
123.584808795442)) ;
#56638=CARTESIAN_POINT('Ctrl Pts',(-18.2537758997071,-47.2554756324466,
123.756993471745)) ;
#56639=CARTESIAN_POINT('Ctrl Pts',(-17.9649058186753,-47.0754865519662,
123.843296984603)) ;
#56640=CARTESIAN_POINT('Ctrl Pts',(-18.3297319147639,-47.2653037804738,
123.94914374406)) ;
#56641=CARTESIAN_POINT('Ctrl Pts',(-18.059852938383,-47.0853146999933,124.083485382884)) ;
#56642=CARTESIAN_POINT('Ctrl Pts',(-18.4391033103602,-47.2752936478482,
124.128436677712)) ;
#56643=CARTESIAN_POINT('Ctrl Pts',(-18.1965689477864,-47.0953045673677,
124.30760067584)) ;
#56644=CARTESIAN_POINT('Ctrl Pts',(-18.5791042370888,-47.2853373868037,
124.286501486607)) ;
#56645=CARTESIAN_POINT('Ctrl Pts',(-18.3715713483285,-47.1053483063232,
124.505180389838)) ;
#56646=CARTESIAN_POINT('Ctrl Pts',(-18.7405005083197,-47.2951591353416,
124.415289290748)) ;
#56647=CARTESIAN_POINT('Ctrl Pts',(-18.5733188647652,-47.1151700548612,
124.666164420743)) ;
#56648=CARTESIAN_POINT('Ctrl Pts',(-18.9254963348016,-47.3051941129514,
124.516697212118)) ;
#56649=CARTESIAN_POINT('Ctrl Pts',(-18.804564552751,-47.1252050324709,124.792922450559)) ;
#56650=CARTESIAN_POINT('Ctrl Pts',(-19.1252827024843,-47.3152190257091,
124.583820831396)) ;
#56651=CARTESIAN_POINT('Ctrl Pts',(-19.0542980945061,-47.1352299452286,
124.87682516283)) ;
#56652=CARTESIAN_POINT('Ctrl Pts',(-19.3300236054208,-47.3250709688029,
124.615141144271)) ;
#56653=CARTESIAN_POINT('Ctrl Pts',(-19.3102255315755,-47.1450818883224,
124.915973694134)) ;
#56654=CARTESIAN_POINT('Ctrl Pts',(-19.5399921824132,-47.335061930132,124.61069150491)) ;
#56655=CARTESIAN_POINT('Ctrl Pts',(-19.5726863790328,-47.1550728496515,
124.910409513021)) ;
#56656=CARTESIAN_POINT('Ctrl Pts',(-19.7445687503477,-47.3449798050004,
124.570275657887)) ;
#56657=CARTESIAN_POINT('Ctrl Pts',(-19.8284072327781,-47.16499072452,124.859887472904)) ;
#56658=CARTESIAN_POINT('Ctrl Pts',(-19.9411645038063,-47.3550083240017,
124.494169080804)) ;
#56659=CARTESIAN_POINT('Ctrl Pts',(-20.0741511053129,-47.1750192435212,
124.764752235826)) ;
#56660=CARTESIAN_POINT('Ctrl Pts',(-20.1190316044298,-47.3648920027995,
124.386736912704)) ;
#56661=CARTESIAN_POINT('Ctrl Pts',(-20.2964844790858,-47.184902922319,124.630459757824)) ;
#56662=CARTESIAN_POINT('Ctrl Pts',(-20.2776029483936,-47.3748869462393,
124.248868784575)) ;
#56663=CARTESIAN_POINT('Ctrl Pts',(-20.4946972414984,-47.1948978657588,
124.458122754322)) ;
#56664=CARTESIAN_POINT('Ctrl Pts',(-20.4099687757007,-47.3849138000617,
124.084811617486)) ;
#56665=CARTESIAN_POINT('Ctrl Pts',(-20.660152776237,-47.2049247195812,124.253049913892)) ;
#56666=CARTESIAN_POINT('Ctrl Pts',(-20.510642437193,-47.3947979644006,123.90302150782)) ;
#56667=CARTESIAN_POINT('Ctrl Pts',(-20.7859931802032,-47.2148088839201,
124.025810555443)) ;
#56668=CARTESIAN_POINT('Ctrl Pts',(-20.5791870198789,-47.404786062443,123.704564661141)) ;
#56669=CARTESIAN_POINT('Ctrl Pts',(-20.8716717236178,-47.2247969819625,
123.777738571902)) ;
#56670=CARTESIAN_POINT('Ctrl Pts',(-20.6122318337484,-47.4147371689001,
123.497960882242)) ;
#56671=CARTESIAN_POINT('Ctrl Pts',(-20.9129754354945,-47.2347480884196,
123.519483140442)) ;
#56672=CARTESIAN_POINT('Ctrl Pts',(-20.6087528151844,-47.4247822200682,
123.286823087064)) ;
#56673=CARTESIAN_POINT('Ctrl Pts',(-20.908624300568,-47.2447931395877,123.255561025808)) ;
#56674=CARTESIAN_POINT('Ctrl Pts',(-20.5695080656403,-47.4346439804265,
123.083245164977)) ;
#56675=CARTESIAN_POINT('Ctrl Pts',(-20.8595658747086,-47.254654899946,123.001088343658)) ;
#56676=CARTESIAN_POINT('Ctrl Pts',(-20.495357370561,-47.4446067972569,122.88735923458)) ;
#56677=CARTESIAN_POINT('Ctrl Pts',(-20.7668750534298,-47.2646177167764,
122.756231591743)) ;
#56678=CARTESIAN_POINT('Ctrl Pts',(-20.3872427945494,-47.4546414785377,
122.706219208448)) ;
#56679=CARTESIAN_POINT('Ctrl Pts',(-20.6317297455285,-47.2746523980572,
122.529807845268)) ;
#56680=CARTESIAN_POINT('Ctrl Pts',(-20.2516200642963,-47.4645265083184,
122.548722650758)) ;
#56681=CARTESIAN_POINT('Ctrl Pts',(-20.4621990514444,-47.284537427838,122.332938363861)) ;
#56682=CARTESIAN_POINT('Ctrl Pts',(-20.0877899814674,-47.4745921017164,
122.414841028809)) ;
#56683=CARTESIAN_POINT('Ctrl Pts',(-20.2574099723545,-47.294603021236,122.165588379758)) ;
#56684=CARTESIAN_POINT('Ctrl Pts',(-19.9073992267312,-47.4844312700779,
122.313551418133)) ;
#56685=CARTESIAN_POINT('Ctrl Pts',(-20.031919660044,-47.3044421895975,122.038978242705)) ;
#56686=CARTESIAN_POINT('Ctrl Pts',(-19.7078787306478,-47.4944938678194,
122.243312824082)) ;
#56687=CARTESIAN_POINT('Ctrl Pts',(-19.7825183008576,-47.3145047873389,
121.951182502059)) ;
#56688=CARTESIAN_POINT('Ctrl Pts',(-19.5025547915718,-47.5043908802264,
122.209566875106)) ;
#56689=CARTESIAN_POINT('Ctrl Pts',(-19.5258624977785,-47.3244017997459,
121.909002520812)) ;
#56690=CARTESIAN_POINT('Ctrl Pts',(-19.2937789957374,-47.514322202052,122.211297493397)) ;
#56691=CARTESIAN_POINT('Ctrl Pts',(-19.2648924723345,-47.3343331215715,
121.911168475178)) ;
#56692=CARTESIAN_POINT('Ctrl Pts',(-19.0862316655902,-47.5243639648065,
122.249899659143)) ;
#56693=CARTESIAN_POINT('Ctrl Pts',(-19.0054588235907,-47.344374884326,121.959423773016)) ;
#56694=CARTESIAN_POINT('Ctrl Pts',(-18.8914968548924,-47.5342521636972,
122.322686181889)) ;
#56695=CARTESIAN_POINT('Ctrl Pts',(-18.7620408414669,-47.3542630832167,
122.050409572496)) ;
#56696=CARTESIAN_POINT('Ctrl Pts',(-18.7102985265331,-47.544246102297,122.429005812639)) ;
#56697=CARTESIAN_POINT('Ctrl Pts',(-18.5355442146445,-47.3642570218165,
122.183311500729)) ;
#56698=CARTESIAN_POINT('Ctrl Pts',(-18.5511494828585,-47.5541869233339,
122.564478677246)) ;
#56699=CARTESIAN_POINT('Ctrl Pts',(-18.3366094810446,-47.3741978428534,
122.352654795869)) ;
#56700=CARTESIAN_POINT('Ctrl Pts',(-18.4175024086679,-47.5641463056221,
122.725638878256)) ;
#56701=CARTESIAN_POINT('Ctrl Pts',(-18.1695526328469,-47.3841572251416,
122.554106931922)) ;
#56702=CARTESIAN_POINT('Ctrl Pts',(-18.3133427089413,-47.5741440652745,
122.90822294444)) ;
#56703=CARTESIAN_POINT('Ctrl Pts',(-18.0393553530217,-47.394154984794,122.782338451435)) ;
#56704=CARTESIAN_POINT('Ctrl Pts',(-18.2424783139921,-47.5841802014768,
123.106952131826)) ;
#56705=CARTESIAN_POINT('Ctrl Pts',(-17.9507774143695,-47.4041911209963,
123.030750867611)) ;
#56706=CARTESIAN_POINT('Ctrl Pts',(-18.2076066802903,-47.5940309989677,
123.311088085714)) ;
#56707=CARTESIAN_POINT('Ctrl Pts',(-17.9071905131153,-47.4140419184872,
123.285921661657)) ;
#56708=CARTESIAN_POINT('Ctrl Pts',(-18.2080983621174,-47.603991864044,123.520488926134)) ;
#56709=CARTESIAN_POINT('Ctrl Pts',(-17.9078079175125,-47.4240027835635,
123.547672833067)) ;
#56710=CARTESIAN_POINT('Ctrl Pts',(-18.2454476002955,-47.6140207316744,
123.728004942344)) ;
#56711=CARTESIAN_POINT('Ctrl Pts',(-17.9544972055366,-47.4340316511939,
123.80706740302)) ;
#56712=CARTESIAN_POINT('Ctrl Pts',(-18.3173323666115,-47.6239309678108,
123.92354610878)) ;
#56713=CARTESIAN_POINT('Ctrl Pts',(-18.0443558520564,-47.4439418873303,
124.051493099978)) ;
#56714=CARTESIAN_POINT('Ctrl Pts',(-18.4218727530156,-47.6338659211253,
124.10437188864)) ;
#56715=CARTESIAN_POINT('Ctrl Pts',(-18.1750338401117,-47.4538768406448,
124.277524030993)) ;
#56716=CARTESIAN_POINT('Ctrl Pts',(-18.5577961313791,-47.6439068515349,
124.265872819916)) ;
#56717=CARTESIAN_POINT('Ctrl Pts',(-18.3449402388069,-47.4639177710544,
124.479398422852)) ;
#56718=CARTESIAN_POINT('Ctrl Pts',(-18.7171539318421,-47.6537947483165,
124.399365872321)) ;
#56719=CARTESIAN_POINT('Ctrl Pts',(-18.5441394207863,-47.473805667836,124.646262688005)) ;
#56720=CARTESIAN_POINT('Ctrl Pts',(-18.8989130954372,-47.6637841999752,
124.504559353168)) ;
#56721=CARTESIAN_POINT('Ctrl Pts',(-18.7713398490752,-47.4837951194947,
124.777752129431)) ;
#56722=CARTESIAN_POINT('Ctrl Pts',(-19.0956328686204,-47.6737432903405,
124.57621883154)) ;
#56723=CARTESIAN_POINT('Ctrl Pts',(-19.017240622354,-47.4937542098601,124.867323859769)) ;
#56724=CARTESIAN_POINT('Ctrl Pts',(-19.3004544560536,-47.6836406026468,
124.612933945687)) ;
#56725=CARTESIAN_POINT('Ctrl Pts',(-19.2732681589748,-47.5036515221664,
124.913214982675)) ;
#56726=CARTESIAN_POINT('Ctrl Pts',(-19.5118542835427,-47.6936970285471,
124.613436471454)) ;
#56727=CARTESIAN_POINT('Ctrl Pts',(-19.5375180334462,-47.5137079480666,
124.913840319172)) ;
#56728=CARTESIAN_POINT('Ctrl Pts',(-19.7163232652421,-47.7035670311368,
124.577994785846)) ;
#56729=CARTESIAN_POINT('Ctrl Pts',(-19.7931038035627,-47.5235779506564,
124.86953541522)) ;
#56730=CARTESIAN_POINT('Ctrl Pts',(-19.9142840722972,-47.7135709643141,
124.507042269719)) ;
#56731=CARTESIAN_POINT('Ctrl Pts',(-20.0405538779432,-47.5335818838336,
124.780842159568)) ;
#56732=CARTESIAN_POINT('Ctrl Pts',(-20.0966064940378,-47.723558224778,124.402844984413)) ;
#56733=CARTESIAN_POINT('Ctrl Pts',(-20.2684557086324,-47.5435691442975,
124.650592871794)) ;
#56734=CARTESIAN_POINT('Ctrl Pts',(-20.2585947292332,-47.7335852763637,
124.267974135904)) ;
#56735=CARTESIAN_POINT('Ctrl Pts',(-20.4709387207198,-47.5535961958832,
124.482002870763)) ;
#56736=CARTESIAN_POINT('Ctrl Pts',(-20.393034986563,-47.7434763661898,124.109317573844)) ;
#56737=CARTESIAN_POINT('Ctrl Pts',(-20.638988919599,-47.5634872857093,124.283677447696)) ;
#56738=CARTESIAN_POINT('Ctrl Pts',(-20.5342723905065,-47.7567741209708,
123.868088225556)) ;
#56739=CARTESIAN_POINT('Ctrl Pts',(-20.8155222738313,-47.5767850404904,
123.982153460042)) ;
#56740=CARTESIAN_POINT('Ctrl Pts',(-20.6091851589647,-47.769972180579,123.597577696433)) ;
#56741=CARTESIAN_POINT('Ctrl Pts',(-20.9091627273331,-47.5899831000985,
123.644050843694)) ;
#56742=CARTESIAN_POINT('Ctrl Pts',(-20.6114219199646,-47.7833689211482,
123.316008276815)) ;
#56743=CARTESIAN_POINT('Ctrl Pts',(-20.9119614689893,-47.6033798406677,
123.292030999204)) ;
#56744=CARTESIAN_POINT('Ctrl Pts',(-20.5772346324987,-47.7932398332216,
123.111276079564)) ;
#56745=CARTESIAN_POINT('Ctrl Pts',(-20.8692234171749,-47.6132507527411,
123.036128094856)) ;
#56746=CARTESIAN_POINT('Ctrl Pts',(-20.506620197884,-47.8033133949897,122.911669655053)) ;
#56747=CARTESIAN_POINT('Ctrl Pts',(-20.7809529680792,-47.6233243145093,
122.786617518438)) ;
#56748=CARTESIAN_POINT('Ctrl Pts',(-20.4051985250744,-47.8131348075781,
122.731761328968)) ;
#56749=CARTESIAN_POINT('Ctrl Pts',(-20.6541739491768,-47.6331457270976,
122.561735103806)) ;
#56750=CARTESIAN_POINT('Ctrl Pts',(-20.2709276734717,-47.8232088248091,
122.568046641826)) ;
#56751=CARTESIAN_POINT('Ctrl Pts',(-20.4863320287132,-47.6432197443286,
122.357091382024)) ;
#56752=CARTESIAN_POINT('Ctrl Pts',(-20.0611060975047,-47.8363676117737,
122.387657282842)) ;
#56753=CARTESIAN_POINT('Ctrl Pts',(-20.2240587468201,-47.6563785312932,
122.131615915142)) ;
#56754=CARTESIAN_POINT('Ctrl Pts',(-19.805342502725,-47.8497337148678,122.263873713802)) ;
#56755=CARTESIAN_POINT('Ctrl Pts',(-19.9043966118727,-47.6697446343874,
121.976897634809)) ;
#56756=CARTESIAN_POINT('Ctrl Pts',(-19.5302562535324,-47.8630476497569,
122.211981763288)) ;
#56757=CARTESIAN_POINT('Ctrl Pts',(-19.5604802160185,-47.6830585692764,
121.912018372235)) ;
#56758=CARTESIAN_POINT('Ctrl Pts',(-19.3221676696211,-47.8729476892044,
122.209028722341)) ;
#56759=CARTESIAN_POINT('Ctrl Pts',(-19.3003815270599,-47.6929586087239,
121.908333182987)) ;
#56760=CARTESIAN_POINT('Ctrl Pts',(-19.115305104631,-47.8829120923389,122.242126287116)) ;
#56761=CARTESIAN_POINT('Ctrl Pts',(-19.0418005240328,-47.7029230118584,
121.949706845845)) ;
#56762=CARTESIAN_POINT('Ctrl Pts',(-18.9160968655024,-47.89294205946,122.311266661747)) ;
#56763=CARTESIAN_POINT('Ctrl Pts',(-18.7927924421303,-47.7129529789796,
122.036134212996)) ;
#56764=CARTESIAN_POINT('Ctrl Pts',(-18.7342345587612,-47.9028443360691,
122.412551802451)) ;
#56765=CARTESIAN_POINT('Ctrl Pts',(-18.5654632172978,-47.7228552555886,
122.162745640166)) ;
#56766=CARTESIAN_POINT('Ctrl Pts',(-18.5173604794192,-47.9161102652382,
122.58797464885)) ;
#56767=CARTESIAN_POINT('Ctrl Pts',(-18.2943866084887,-47.7361211847578,
122.382011147295)) ;
#56768=CARTESIAN_POINT('Ctrl Pts',(-18.309565842614,-47.9327317963447,122.873754193906)) ;
#56769=CARTESIAN_POINT('Ctrl Pts',(-18.0346303795379,-47.7527427158642,
122.739250673721)) ;
#56770=CARTESIAN_POINT('Ctrl Pts',(-18.1920101676508,-47.9526066249893,
123.279717316389)) ;
#56771=CARTESIAN_POINT('Ctrl Pts',(-17.8876997699416,-47.7726175445089,
123.246720784364)) ;
#56772=CARTESIAN_POINT('Ctrl Pts',(-18.2154597866439,-47.9692798330912,
123.633471891769)) ;
#56773=CARTESIAN_POINT('Ctrl Pts',(-17.917000592539,-47.7892907526107,123.688848718156)) ;
#56774=CARTESIAN_POINT('Ctrl Pts',(-18.3053614681726,-47.9825309580725,
123.897116716914)) ;
#56775=CARTESIAN_POINT('Ctrl Pts',(-18.0293936750279,-47.802541877592,124.018462677766)) ;
#56776=CARTESIAN_POINT('Ctrl Pts',(-18.4387378594094,-47.9957732768933,
124.141560057195)) ;
#56777=CARTESIAN_POINT('Ctrl Pts',(-18.1961054878866,-47.8157841964128,
124.323995100867)) ;
#56778=CARTESIAN_POINT('Ctrl Pts',(-18.6845127413368,-48.0125065172328,
124.39871352638)) ;
#56779=CARTESIAN_POINT('Ctrl Pts',(-18.5033373265711,-47.8325174367523,
124.645448284726)) ;
#56780=CARTESIAN_POINT('Ctrl Pts',(-19.0624327367419,-48.0323356654207,
124.585830606366)) ;
#56781=CARTESIAN_POINT('Ctrl Pts',(-18.9757346112765,-47.8523465849403,
124.879336049471)) ;
#56782=CARTESIAN_POINT('Ctrl Pts',(-19.4832475920745,-48.0522603605214,
124.633977070229)) ;
#56783=CARTESIAN_POINT('Ctrl Pts',(-19.5017537469075,-47.8722712800409,
124.939516678405)) ;
#56784=CARTESIAN_POINT('Ctrl Pts',(-19.8953466515693,-48.0721835891048,
124.53556105767)) ;
#56785=CARTESIAN_POINT('Ctrl Pts',(-20.0168758620234,-47.8921945086243,
124.816493222276)) ;
#56786=CARTESIAN_POINT('Ctrl Pts',(-20.2491680892978,-48.0921107282309,
124.302550900816)) ;
#56787=CARTESIAN_POINT('Ctrl Pts',(-20.4591503182004,-47.9121216477504,
124.525228377064)) ;
#56788=CARTESIAN_POINT('Ctrl Pts',(-20.5020771655509,-48.1119871908466,
123.963916176458)) ;
#56789=CARTESIAN_POINT('Ctrl Pts',(-20.775283647874,-47.9319981103661,124.101934449859)) ;
#56790=CARTESIAN_POINT('Ctrl Pts',(-20.6250718690425,-48.1319644194519,
123.557348462164)) ;
#56791=CARTESIAN_POINT('Ctrl Pts',(-20.9290246640745,-47.9519753389714,
123.593724361123)) ;
#56792=CARTESIAN_POINT('Ctrl Pts',(-20.6016537275589,-48.1518992774256,
123.134089906052)) ;
#56793=CARTESIAN_POINT('Ctrl Pts',(-20.8997496416068,-47.9719101969451,
123.064652071518)) ;
#56794=CARTESIAN_POINT('Ctrl Pts',(-20.4359503230159,-48.1717957263564,
122.744874511836)) ;
#56795=CARTESIAN_POINT('Ctrl Pts',(-20.6926191393825,-47.9918066458759,
122.57813484947)) ;
#56796=CARTESIAN_POINT('Ctrl Pts',(-20.1473267208655,-48.191717010423,122.434822386439)) ;
#56797=CARTESIAN_POINT('Ctrl Pts',(-20.3318393280273,-48.0117279299425,
122.190571444716)) ;
#56798=CARTESIAN_POINT('Ctrl Pts',(-19.7694900246731,-48.2116736600939,
122.241648838417)) ;
#56799=CARTESIAN_POINT('Ctrl Pts',(-19.8595433797258,-48.0316845796135,
121.949105900236)) ;
#56800=CARTESIAN_POINT('Ctrl Pts',(-19.3501801167776,-48.2315509532055,
122.189092571805)) ;
#56801=CARTESIAN_POINT('Ctrl Pts',(-19.3354077539385,-48.0515618727251,
121.883411775771)) ;
#56802=CARTESIAN_POINT('Ctrl Pts',(-18.9375691670233,-48.251437425434,122.281750555441)) ;
#56803=CARTESIAN_POINT('Ctrl Pts',(-18.8196458601561,-48.0714483449535,
121.999233714734)) ;
#56804=CARTESIAN_POINT('Ctrl Pts',(-18.5785832798502,-48.271498991358,122.512179757162)) ;
#56805=CARTESIAN_POINT('Ctrl Pts',(-18.3709126384581,-48.0915099108775,
122.287270877058)) ;
#56806=CARTESIAN_POINT('Ctrl Pts',(-18.3229725036018,-48.2913393988987,
122.847760478558)) ;
#56807=CARTESIAN_POINT('Ctrl Pts',(-18.051400875237,-48.1113503184183,122.706744756722)) ;
#56808=CARTESIAN_POINT('Ctrl Pts',(-18.1954566816947,-48.3111907228717,
123.250147542051)) ;
#56809=CARTESIAN_POINT('Ctrl Pts',(-17.8920053837549,-48.1312016423912,
123.209726070938)) ;
#56810=CARTESIAN_POINT('Ctrl Pts',(-18.2137292660296,-48.3312439928231,
123.676086435332)) ;
#56811=CARTESIAN_POINT('Ctrl Pts',(-17.9148449515305,-48.1512549123426,
123.742150506238)) ;
#56812=CARTESIAN_POINT('Ctrl Pts',(-18.3743522701606,-48.3510646502064,
124.065843827562)) ;
#56813=CARTESIAN_POINT('Ctrl Pts',(-18.1156214421197,-48.171075569726,124.229345578979)) ;
#56814=CARTESIAN_POINT('Ctrl Pts',(-18.6598163322656,-48.3710360715369,
124.380035479297)) ;
#56815=CARTESIAN_POINT('Ctrl Pts',(-18.4724496626934,-48.1910469910565,
124.622086302421)) ;
#56816=CARTESIAN_POINT('Ctrl Pts',(-19.0341051163834,-48.3909295639006,
124.577408934611)) ;
#56817=CARTESIAN_POINT('Ctrl Pts',(-18.9403084788281,-48.2109404834202,
124.868804641701)) ;
#56818=CARTESIAN_POINT('Ctrl Pts',(-19.4558297886332,-48.4109536501417,
124.635272002044)) ;
#56819=CARTESIAN_POINT('Ctrl Pts',(-19.4674642242625,-48.2309645696612,
124.941135895911)) ;
#56820=CARTESIAN_POINT('Ctrl Pts',(-19.8676091497869,-48.4307585292546,
124.54692460703)) ;
#56821=CARTESIAN_POINT('Ctrl Pts',(-19.9821868641728,-48.2507694487741,
124.830704772486)) ;
#56822=CARTESIAN_POINT('Ctrl Pts',(-20.2278594836264,-48.4507175449524,
124.322628489146)) ;
#56823=CARTESIAN_POINT('Ctrl Pts',(-20.4325013286811,-48.270728464472,124.550337764618)) ;
#56824=CARTESIAN_POINT('Ctrl Pts',(-20.4895249553124,-48.4707035685815,
123.987793204805)) ;
#56825=CARTESIAN_POINT('Ctrl Pts',(-20.7595855619426,-48.290714488101,124.131795730285)) ;
#56826=CARTESIAN_POINT('Ctrl Pts',(-20.620851700236,-48.490512064342,123.587567929602)) ;
#56827=CARTESIAN_POINT('Ctrl Pts',(-20.9237469671221,-48.3105229838615,
123.631516939114)) ;
#56828=CARTESIAN_POINT('Ctrl Pts',(-20.6081359744809,-48.5104947034476,
123.162963885691)) ;
#56829=CARTESIAN_POINT('Ctrl Pts',(-20.9078563779527,-48.3305056229671,
123.100761863387)) ;
#56830=CARTESIAN_POINT('Ctrl Pts',(-20.4519095426807,-48.5303761512416,
122.770042814153)) ;
#56831=CARTESIAN_POINT('Ctrl Pts',(-20.712577492358,-48.3503870707611,122.609609792181)) ;
#56832=CARTESIAN_POINT('Ctrl Pts',(-20.1703007545969,-48.5503326179791,
122.452751245619)) ;
#56833=CARTESIAN_POINT('Ctrl Pts',(-20.3605699836002,-48.3703435374986,
122.212992650296)) ;
#56834=CARTESIAN_POINT('Ctrl Pts',(-19.7987956805758,-48.5702100149347,
122.251075325285)) ;
#56835=CARTESIAN_POINT('Ctrl Pts',(-19.8961915071148,-48.3902209344542,
121.960894036655)) ;
#56836=CARTESIAN_POINT('Ctrl Pts',(-19.3787174367408,-48.59019196111,122.187732374788)) ;
#56837=CARTESIAN_POINT('Ctrl Pts',(-19.3710944052831,-48.4102028806295,
121.881710834772)) ;
#56838=CARTESIAN_POINT('Ctrl Pts',(-18.9632548947561,-48.6101210601467,
122.271556210172)) ;
#56839=CARTESIAN_POINT('Ctrl Pts',(-18.8517658004596,-48.4301319796663,
121.986485154888)) ;
#56840=CARTESIAN_POINT('Ctrl Pts',(-18.6014532782387,-48.6300496833594,
122.491970120177)) ;
#56841=CARTESIAN_POINT('Ctrl Pts',(-18.3995108076249,-48.4500606028789,
122.262000851676)) ;
#56842=CARTESIAN_POINT('Ctrl Pts',(-18.3371474305036,-48.6498840074658,
122.820662580448)) ;
#56843=CARTESIAN_POINT('Ctrl Pts',(-18.0691275874109,-48.4698949269853,
122.672852581534)) ;
#56844=CARTESIAN_POINT('Ctrl Pts',(-18.2224259879656,-48.6665362948492,
123.155533978461)) ;
#56845=CARTESIAN_POINT('Ctrl Pts',(-17.9257131668265,-48.4865472143687,
123.091471777925)) ;
#56846=CARTESIAN_POINT('Ctrl Pts',(-18.2035092636524,-48.6797967958714,
123.433741752069)) ;
#56847=CARTESIAN_POINT('Ctrl Pts',(-17.9020712048987,-48.4998077153909,
123.439203218317)) ;
#56848=CARTESIAN_POINT('Ctrl Pts',(-18.2254971301078,-48.6897982730727,
123.64284321915)) ;
#56849=CARTESIAN_POINT('Ctrl Pts',(-17.9295520560355,-48.5098091925922,
123.700586123937)) ;
#56850=CARTESIAN_POINT('Ctrl Pts',(-18.2839780007626,-48.6998302939322,
123.845485351349)) ;
#56851=CARTESIAN_POINT('Ctrl Pts',(-18.0026504044852,-48.5198412134517,
123.953887639501)) ;
#56852=CARTESIAN_POINT('Ctrl Pts',(-18.3749627895114,-48.7096938376577,
124.03181215673)) ;
#56853=CARTESIAN_POINT('Ctrl Pts',(-18.1163811919581,-48.5297047571772,
124.186799307523)) ;
#56854=CARTESIAN_POINT('Ctrl Pts',(-18.4977838557843,-48.7196625513279,
124.201640045108)) ;
#56855=CARTESIAN_POINT('Ctrl Pts',(-18.2698960728996,-48.5396734708474,
124.399078392985)) ;
#56856=CARTESIAN_POINT('Ctrl Pts',(-18.6994061492759,-48.7330082987316,
124.396656788491)) ;
#56857=CARTESIAN_POINT('Ctrl Pts',(-18.5219675224637,-48.5530192182511,
124.642888173995)) ;
#56858=CARTESIAN_POINT('Ctrl Pts',(-18.9435543299916,-48.7461588538042,
124.533062447628)) ;
#56859=CARTESIAN_POINT('Ctrl Pts',(-18.8271260676445,-48.5661697733238,
124.813370161097)) ;
#56860=CARTESIAN_POINT('Ctrl Pts',(-19.2163009315313,-48.7595442343541,
124.602291897744)) ;
#56861=CARTESIAN_POINT('Ctrl Pts',(-19.1680417733394,-48.5795551538736,
124.899907926198)) ;
#56862=CARTESIAN_POINT('Ctrl Pts',(-19.4236287954365,-48.7694321703469,
124.617669125966)) ;
#56863=CARTESIAN_POINT('Ctrl Pts',(-19.4272046606702,-48.5894430898665,
124.919132760913)) ;
#56864=CARTESIAN_POINT('Ctrl Pts',(-19.6326234694383,-48.7794233601596,
124.59695356156)) ;
#56865=CARTESIAN_POINT('Ctrl Pts',(-19.6884474342912,-48.5994342796791,
124.89324094596)) ;
#56866=CARTESIAN_POINT('Ctrl Pts',(-19.8341362224527,-48.7893754586979,
124.54055689342)) ;
#56867=CARTESIAN_POINT('Ctrl Pts',(-19.9403393905852,-48.6093863782174,
124.822747843727)) ;
#56868=CARTESIAN_POINT('Ctrl Pts',(-20.0244791000905,-48.7994217151483,
124.449067132527)) ;
#56869=CARTESIAN_POINT('Ctrl Pts',(-20.1782692263093,-48.6194326346679,
124.708388112083)) ;
#56870=CARTESIAN_POINT('Ctrl Pts',(-20.1927872751713,-48.8092711625425,
124.328441823876)) ;
#56871=CARTESIAN_POINT('Ctrl Pts',(-20.3886560574849,-48.629282082062,124.557608790027)) ;
#56872=CARTESIAN_POINT('Ctrl Pts',(-20.3397216534064,-48.8192338150376,
124.179192839321)) ;
#56873=CARTESIAN_POINT('Ctrl Pts',(-20.572326096074,-48.6392447345572,124.371049479818)) ;
#56874=CARTESIAN_POINT('Ctrl Pts',(-20.4590010872859,-48.8292569006798,
124.005486486065)) ;
#56875=CARTESIAN_POINT('Ctrl Pts',(-20.7214277474901,-48.6492678201993,
124.15391807749)) ;
#56876=CARTESIAN_POINT('Ctrl Pts',(-20.5456810010499,-48.8391820164367,
123.815659921871)) ;
#56877=CARTESIAN_POINT('Ctrl Pts',(-20.8297802317773,-48.6591929359562,
123.916635975711)) ;
#56878=CARTESIAN_POINT('Ctrl Pts',(-20.5986636057936,-48.8492344948365,
123.611094978186)) ;
#56879=CARTESIAN_POINT('Ctrl Pts',(-20.8960112320081,-48.669245414356,123.660930444439)) ;
#56880=CARTESIAN_POINT('Ctrl Pts',(-20.6151308206564,-48.8590859935392,
123.4046256451)) ;
#56881=CARTESIAN_POINT('Ctrl Pts',(-20.9165980683453,-48.6790969130588,
123.402843889693)) ;
#56882=CARTESIAN_POINT('Ctrl Pts',(-20.5958067267319,-48.8690577327418,
123.19590749213)) ;
#56883=CARTESIAN_POINT('Ctrl Pts',(-20.8924457356937,-48.6890686522613,
123.141945824746)) ;
#56884=CARTESIAN_POINT('Ctrl Pts',(-20.5403646088462,-48.8790529405074,
122.993187529069)) ;
#56885=CARTESIAN_POINT('Ctrl Pts',(-20.8231457688336,-48.699063860027,122.888545055515)) ;
#56886=CARTESIAN_POINT('Ctrl Pts',(-20.4500071936649,-48.8890869419765,
122.802593518848)) ;
#56887=CARTESIAN_POINT('Ctrl Pts',(-20.7102015281,-48.709097861496,122.650301300747)) ;
#56888=CARTESIAN_POINT('Ctrl Pts',(-20.3303491214858,-48.8989423000689,
122.633423450339)) ;
#56889=CARTESIAN_POINT('Ctrl Pts',(-20.5606310890588,-48.7189532195884,
122.438836911221)) ;
#56890=CARTESIAN_POINT('Ctrl Pts',(-20.1812231910538,-48.9089417756622,
122.485307584382)) ;
#56891=CARTESIAN_POINT('Ctrl Pts',(-20.3742255769776,-48.7289526951817,
122.253690036729)) ;
#56892=CARTESIAN_POINT('Ctrl Pts',(-20.0105298951127,-48.9188362241573,
122.366356746529)) ;
#56893=CARTESIAN_POINT('Ctrl Pts',(-20.1608603227563,-48.7388471436768,
122.104999075597)) ;
#56894=CARTESIAN_POINT('Ctrl Pts',(-19.8186007680799,-48.928899348385,122.277447738823)) ;
#56895=CARTESIAN_POINT('Ctrl Pts',(-19.920950110455,-48.7489102679045,121.993860313418)) ;
#56896=CARTESIAN_POINT('Ctrl Pts',(-19.6186814141664,-48.9387389747136,
122.224180471466)) ;
#56897=CARTESIAN_POINT('Ctrl Pts',(-19.6710512311664,-48.7587498942331,
121.92727346975)) ;
#56898=CARTESIAN_POINT('Ctrl Pts',(-19.4079521083204,-48.9488022097566,
122.205769170469)) ;
#56899=CARTESIAN_POINT('Ctrl Pts',(-19.4076398792596,-48.7688131292761,
121.904256633365)) ;
#56900=CARTESIAN_POINT('Ctrl Pts',(-19.2007357621224,-48.9586962149906,
122.224096611744)) ;
#56901=CARTESIAN_POINT('Ctrl Pts',(-19.1486188793578,-48.7787071345101,
121.927163232638)) ;
#56902=CARTESIAN_POINT('Ctrl Pts',(-18.9987560013201,-48.9686389282064,
122.277825494424)) ;
#56903=CARTESIAN_POINT('Ctrl Pts',(-18.8961432338449,-48.7886498477259,
121.994321818585)) ;
#56904=CARTESIAN_POINT('Ctrl Pts',(-18.8079128243991,-48.9786446680046,
122.36634819626)) ;
#56905=CARTESIAN_POINT('Ctrl Pts',(-18.6575880746054,-48.7986555875241,
122.104972809747)) ;
#56906=CARTESIAN_POINT('Ctrl Pts',(-18.6352354087058,-48.988665570151,122.48702462515)) ;
#56907=CARTESIAN_POINT('Ctrl Pts',(-18.4417397384624,-48.8086764896705,
122.25581614595)) ;
#56908=CARTESIAN_POINT('Ctrl Pts',(-18.4878939976367,-48.9985563401998,
122.633756235366)) ;
#56909=CARTESIAN_POINT('Ctrl Pts',(-18.2575608010037,-48.8185672597194,
122.439229061336)) ;
#56910=CARTESIAN_POINT('Ctrl Pts',(-18.366802071252,-49.0085477509796,122.805381393975)) ;
#56911=CARTESIAN_POINT('Ctrl Pts',(-18.1061936757507,-48.8285586704991,
122.653759103555)) ;
#56912=CARTESIAN_POINT('Ctrl Pts',(-18.2777961208184,-49.0184960966441,
122.994637884771)) ;
#56913=CARTESIAN_POINT('Ctrl Pts',(-17.9949337390312,-48.8385070161635,
122.890328842151)) ;
#56914=CARTESIAN_POINT('Ctrl Pts',(-18.2225909158697,-49.0284409547052,
123.196309162691)) ;
#56915=CARTESIAN_POINT('Ctrl Pts',(-17.9259246877566,-48.8484518742248,
123.142417551851)) ;
#56916=CARTESIAN_POINT('Ctrl Pts',(-18.2033401476526,-49.0384957900982,
123.40679518885)) ;
#56917=CARTESIAN_POINT('Ctrl Pts',(-17.9018586343297,-48.8585067096177,
123.405524737977)) ;
#56918=CARTESIAN_POINT('Ctrl Pts',(-18.2201677805228,-49.0483181621996,
123.612623482533)) ;
#56919=CARTESIAN_POINT('Ctrl Pts',(-17.9228907003336,-48.8683290817192,
123.662811089204)) ;
#56920=CARTESIAN_POINT('Ctrl Pts',(-18.2733451038834,-49.0583740296434,
123.817216281984)) ;
#56921=CARTESIAN_POINT('Ctrl Pts',(-17.9893599289027,-48.8783849491629,
123.918552606328)) ;
#56922=CARTESIAN_POINT('Ctrl Pts',(-18.3605807016632,-49.0683147595013,
124.007132559612)) ;
#56923=CARTESIAN_POINT('Ctrl Pts',(-18.0984022473482,-48.8883256790208,
124.155949320502)) ;
#56924=CARTESIAN_POINT('Ctrl Pts',(-18.478492080276,-49.0782190980524,124.178754700712)) ;
#56925=CARTESIAN_POINT('Ctrl Pts',(-18.2457897777088,-48.8982300175719,
124.370478803639)) ;
#56926=CARTESIAN_POINT('Ctrl Pts',(-18.6265896771452,-49.0882657794809,
124.329321820747)) ;
#56927=CARTESIAN_POINT('Ctrl Pts',(-18.4309099577425,-48.9082766990004,
124.558689346557)) ;
#56928=CARTESIAN_POINT('Ctrl Pts',(-18.7959241485075,-49.0981612869501,
124.450228240295)) ;
#56929=CARTESIAN_POINT('Ctrl Pts',(-18.6425771223677,-48.9181722064697,
124.709824664254)) ;
#56930=CARTESIAN_POINT('Ctrl Pts',(-18.9867862815912,-49.1082235554488,
124.541375926304)) ;
#56931=CARTESIAN_POINT('Ctrl Pts',(-18.8811535876287,-48.9282344749683,
124.823761366756)) ;
#56932=CARTESIAN_POINT('Ctrl Pts',(-19.1861338900622,-49.1180655457194,
124.596897992535)) ;
#56933=CARTESIAN_POINT('Ctrl Pts',(-19.1303382919264,-48.9380764652389,
124.893166471284)) ;
#56934=CARTESIAN_POINT('Ctrl Pts',(-19.3951586958825,-49.1280589626003,
124.617736026602)) ;
#56935=CARTESIAN_POINT('Ctrl Pts',(-19.391619244589,-48.9480698821199,124.919216288672)) ;
#56936=CARTESIAN_POINT('Ctrl Pts',(-19.6032371853687,-49.1379834504525,
124.602087040925)) ;
#56937=CARTESIAN_POINT('Ctrl Pts',(-19.6517180268592,-48.957994369972,124.899657271503)) ;
#56938=CARTESIAN_POINT('Ctrl Pts',(-19.8069854701028,-49.147983084361,124.550380447897)) ;
#56939=CARTESIAN_POINT('Ctrl Pts',(-19.9064040385698,-48.9679940038805,
124.835026142199)) ;
#56940=CARTESIAN_POINT('Ctrl Pts',(-19.9984490408071,-49.1579691946177,
124.464185024781)) ;
#56941=CARTESIAN_POINT('Ctrl Pts',(-20.1457345661112,-48.9779801141373,
124.727283799882)) ;
#56942=CARTESIAN_POINT('Ctrl Pts',(-20.1727370286862,-49.1680051458049,
124.345311201538)) ;
#56943=CARTESIAN_POINT('Ctrl Pts',(-20.3635957587597,-48.9880160653244,
124.578693439331)) ;
#56944=CARTESIAN_POINT('Ctrl Pts',(-20.3212855419175,-49.1778617841397,
124.200809116619)) ;
#56945=CARTESIAN_POINT('Ctrl Pts',(-20.5492835775736,-48.9978727036592,
124.398066759206)) ;
#56946=CARTESIAN_POINT('Ctrl Pts',(-20.4444358570333,-49.1878607442177,
124.030495135267)) ;
#56947=CARTESIAN_POINT('Ctrl Pts',(-20.7032232578313,-49.0078716637372,
124.185175408139)) ;
#56948=CARTESIAN_POINT('Ctrl Pts',(-20.5354258116152,-49.1977559745315,
123.843382253148)) ;
#56949=CARTESIAN_POINT('Ctrl Pts',(-20.8169628558538,-49.017766894051,123.951284539038)) ;
#56950=CARTESIAN_POINT('Ctrl Pts',(-20.5934596272314,-49.2078164870001,
123.640024401084)) ;
#56951=CARTESIAN_POINT('Ctrl Pts',(-20.8895070312652,-49.0278274065196,
123.697088016947)) ;
#56952=CARTESIAN_POINT('Ctrl Pts',(-20.614964621342,-49.2176657785463,123.434065207261)) ;
#56953=CARTESIAN_POINT('Ctrl Pts',(-20.9163903857337,-49.0376766980658,
123.439638200358)) ;
#56954=CARTESIAN_POINT('Ctrl Pts',(-20.6006524939482,-49.2276929644785,
123.223753772235)) ;
#56955=CARTESIAN_POINT('Ctrl Pts',(-20.8985020839433,-49.047703883998,123.176748817964)) ;
#56956=CARTESIAN_POINT('Ctrl Pts',(-20.5494925233518,-49.2377215009378,
123.019212625671)) ;
#56957=CARTESIAN_POINT('Ctrl Pts',(-20.8345541011954,-49.0577324204573,
122.921071960493)) ;
#56958=CARTESIAN_POINT('Ctrl Pts',(-20.4655325528851,-49.2475667409028,
122.830041408162)) ;
#56959=CARTESIAN_POINT('Ctrl Pts',(-20.7296054274978,-49.0675776604223,
122.684606145125)) ;
#56960=CARTESIAN_POINT('Ctrl Pts',(-20.3487525475356,-49.257557435826,122.655457201128)) ;
#56961=CARTESIAN_POINT('Ctrl Pts',(-20.5836317517276,-49.0775683553455,
122.466374760866)) ;
#56962=CARTESIAN_POINT('Ctrl Pts',(-20.2024139642059,-49.2675952565846,
122.503414527449)) ;
#56963=CARTESIAN_POINT('Ctrl Pts',(-20.4007099670647,-49.0876061761041,
122.276320211535)) ;
#56964=CARTESIAN_POINT('Ctrl Pts',(-20.0353851635832,-49.2774398503615,
122.381196686235)) ;
#56965=CARTESIAN_POINT('Ctrl Pts',(-20.1919240684865,-49.097450769881,122.123545794941)) ;
#56966=CARTESIAN_POINT('Ctrl Pts',(-19.8472610421014,-49.2874238457376,
122.288151641728)) ;
#56967=CARTESIAN_POINT('Ctrl Pts',(-19.9567693977813,-49.1074347652571,
122.007237918667)) ;
#56968=CARTESIAN_POINT('Ctrl Pts',(-19.6465098945046,-49.297372894299,122.229404619294)) ;
#56969=CARTESIAN_POINT('Ctrl Pts',(-19.7058304590878,-49.1173838138185,
121.933802444851)) ;
#56970=CARTESIAN_POINT('Ctrl Pts',(-19.4375191683223,-49.3073753332735,
122.206058321571)) ;
#56971=CARTESIAN_POINT('Ctrl Pts',(-19.4445921214465,-49.127386252793,121.904618015454)) ;
#56972=CARTESIAN_POINT('Ctrl Pts',(-19.2272793153479,-49.3173965745699,
122.219664475617)) ;
#56973=CARTESIAN_POINT('Ctrl Pts',(-19.1817922312834,-49.1374074940894,
121.921624060184)) ;
#56974=CARTESIAN_POINT('Ctrl Pts',(-19.0251633000382,-49.3272892530094,
122.268684611015)) ;
#56975=CARTESIAN_POINT('Ctrl Pts',(-18.9291459750505,-49.1473001725289,
121.982897915506)) ;
#56976=CARTESIAN_POINT('Ctrl Pts',(-18.8326207757844,-49.337279306957,122.352565184891)) ;
#56977=CARTESIAN_POINT('Ctrl Pts',(-18.6884670362895,-49.1572902264765,
122.087747388008)) ;
#56978=CARTESIAN_POINT('Ctrl Pts',(-18.65820968593,-49.3472376681055,122.468356623585)) ;
#56979=CARTESIAN_POINT('Ctrl Pts',(-18.4704519829065,-49.167248587625,122.232485671663)) ;
#56980=CARTESIAN_POINT('Ctrl Pts',(-18.5070800115735,-49.3571372949903,
122.611463780261)) ;
#56981=CARTESIAN_POINT('Ctrl Pts',(-18.2815383414218,-49.1771482145098,
122.411369259759)) ;
#56982=CARTESIAN_POINT('Ctrl Pts',(-18.3813177298446,-49.3671851917937,
122.781158712775)) ;
#56983=CARTESIAN_POINT('Ctrl Pts',(-18.1243345329149,-49.1871961113132,
122.623486945878)) ;
#56984=CARTESIAN_POINT('Ctrl Pts',(-18.2881930918701,-49.3770805494297,
122.96721883373)) ;
#56985=CARTESIAN_POINT('Ctrl Pts',(-18.0079271715272,-49.1970914689492,
122.856062333911)) ;
#56986=CARTESIAN_POINT('Ctrl Pts',(-18.2277777790016,-49.3871422018863,
123.169910866014)) ;
#56987=CARTESIAN_POINT('Ctrl Pts',(-17.9324068929377,-49.2071531214059,
123.109426695854)) ;
#56988=CARTESIAN_POINT('Ctrl Pts',(-18.2039634409259,-49.3969868061583,
123.375507420365)) ;
#56989=CARTESIAN_POINT('Ctrl Pts',(-17.9026375539876,-49.2169977256778,
123.366423552928)) ;
#56990=CARTESIAN_POINT('Ctrl Pts',(-18.21560282813,-49.4069469278563,123.584573029196)) ;
#56991=CARTESIAN_POINT('Ctrl Pts',(-17.9171858176287,-49.2269578473758,
123.627756075238)) ;
#56992=CARTESIAN_POINT('Ctrl Pts',(-18.2641366558949,-49.4169849622188,
123.789939361942)) ;
#56993=CARTESIAN_POINT('Ctrl Pts',(-17.9778519475614,-49.2369958817383,
123.884464098804)) ;
#56994=CARTESIAN_POINT('Ctrl Pts',(-18.3458936811806,-49.4268592748053,
123.980778500139)) ;
#56995=CARTESIAN_POINT('Ctrl Pts',(-18.0800477461698,-49.2468701943248,
124.123014445759)) ;
#56996=CARTESIAN_POINT('Ctrl Pts',(-18.4617697259283,-49.436928755588,124.1579063665)) ;
#56997=CARTESIAN_POINT('Ctrl Pts',(-18.2248917332059,-49.2569396751075,
124.344424493794)) ;
#56998=CARTESIAN_POINT('Ctrl Pts',(-18.6032069971224,-49.4467630916051,
124.308729317286)) ;
#56999=CARTESIAN_POINT('Ctrl Pts',(-18.4016886195746,-49.2667740111246,
124.532954912197)) ;
#57000=CARTESIAN_POINT('Ctrl Pts',(-18.7716598122527,-49.4567960493333,
124.435654755595)) ;
#57001=CARTESIAN_POINT('Ctrl Pts',(-18.6122540927978,-49.2768069688528,
124.691612235922)) ;
#57002=CARTESIAN_POINT('Ctrl Pts',(-18.9596285266735,-49.4668164479085,
124.530768810622)) ;
#57003=CARTESIAN_POINT('Ctrl Pts',(-18.8472145111849,-49.286827367428,124.810505656996)) ;
#57004=CARTESIAN_POINT('Ctrl Pts',(-19.1580012266402,-49.4766820216797,
124.591362825177)) ;
#57005=CARTESIAN_POINT('Ctrl Pts',(-19.0951813190911,-49.2966929411992,
124.886249263638)) ;
#57006=CARTESIAN_POINT('Ctrl Pts',(-19.3680870984409,-49.4867508963358,
124.617111323159)) ;
#57007=CARTESIAN_POINT('Ctrl Pts',(-19.3577881565843,-49.3067618158553,
124.918435603033)) ;
#57008=CARTESIAN_POINT('Ctrl Pts',(-19.5747954024805,-49.4965963272413,
124.606267618942)) ;
#57009=CARTESIAN_POINT('Ctrl Pts',(-19.6161749842929,-49.3166072467608,
124.904881658668)) ;
#57010=CARTESIAN_POINT('Ctrl Pts',(-19.7793647307938,-49.506575952112,124.559725510975)) ;
#57011=CARTESIAN_POINT('Ctrl Pts',(-19.8718870581655,-49.3265868716315,
124.846704437051)) ;
#57012=CARTESIAN_POINT('Ctrl Pts',(-19.9733472943274,-49.5165946350261,
124.477683630801)) ;
#57013=CARTESIAN_POINT('Ctrl Pts',(-20.1143655070661,-49.3366055545456,
124.744152692694)) ;
#57014=CARTESIAN_POINT('Ctrl Pts',(-20.1480134440682,-49.5264779002099,
124.365106465105)) ;
#57015=CARTESIAN_POINT('Ctrl Pts',(-20.3326993756055,-49.3464888197294,
124.603431043529)) ;
#57016=CARTESIAN_POINT('Ctrl Pts',(-20.3032270535751,-49.5365461943013,
124.221241519737)) ;
#57017=CARTESIAN_POINT('Ctrl Pts',(-20.5267164376819,-49.3565571138208,
124.423600519523)) ;
#57018=CARTESIAN_POINT('Ctrl Pts',(-20.4283133218922,-49.5463763244866,
124.056692970203)) ;
#57019=CARTESIAN_POINT('Ctrl Pts',(-20.6830755386352,-49.3663872440061,
124.217913860324)) ;
#57020=CARTESIAN_POINT('Ctrl Pts',(-20.5254162570907,-49.5564428727018,
123.868692053615)) ;
#57021=CARTESIAN_POINT('Ctrl Pts',(-20.8044543032973,-49.3764537922212,
123.982913211206)) ;
#57022=CARTESIAN_POINT('Ctrl Pts',(-20.5871922984484,-49.5663331213904,
123.67013049004)) ;
#57023=CARTESIAN_POINT('Ctrl Pts',(-20.8816750149605,-49.3863440409099,
123.734710364382)) ;
#57024=CARTESIAN_POINT('Ctrl Pts',(-20.6142760100577,-49.5763253031664,
123.461828924434)) ;
#57025=CARTESIAN_POINT('Ctrl Pts',(-20.9155298641694,-49.3963362226859,
123.47433321887)) ;
#57026=CARTESIAN_POINT('Ctrl Pts',(-20.6046113032203,-49.5862880837942,
123.252607087574)) ;
#57027=CARTESIAN_POINT('Ctrl Pts',(-20.9034492218807,-49.4062990033137,
123.212805454245)) ;
#57028=CARTESIAN_POINT('Ctrl Pts',(-20.5595393091731,-49.5961924884679,
123.049307305498)) ;
#57029=CARTESIAN_POINT('Ctrl Pts',(-20.8471090807329,-49.4162034079875,
122.95867980125)) ;
#57030=CARTESIAN_POINT('Ctrl Pts',(-20.478467374034,-49.606252482947,122.853990633004)) ;
#57031=CARTESIAN_POINT('Ctrl Pts',(-20.7457693981853,-49.4262634024665,
122.714534227853)) ;
#57032=CARTESIAN_POINT('Ctrl Pts',(-20.3672356635817,-49.6161011049168,
122.679339657836)) ;
#57033=CARTESIAN_POINT('Ctrl Pts',(-20.6067290421984,-49.4361120244363,
122.496219298813)) ;
#57034=CARTESIAN_POINT('Ctrl Pts',(-20.2251544951592,-49.6261315443286,
122.523536505665)) ;
#57035=CARTESIAN_POINT('Ctrl Pts',(-20.429127558072,-49.4461424638481,122.301465539428)) ;
#57036=CARTESIAN_POINT('Ctrl Pts',(-20.0582370192232,-49.6361412599634,
122.395350931652)) ;
#57037=CARTESIAN_POINT('Ctrl Pts',(-20.2204806966358,-49.4561521794829,
122.141233524141)) ;
#57038=CARTESIAN_POINT('Ctrl Pts',(-19.8735746846781,-49.646052012656,122.298896339654)) ;
#57039=CARTESIAN_POINT('Ctrl Pts',(-19.9896519590277,-49.4660629321755,
122.020664911434)) ;
#57040=CARTESIAN_POINT('Ctrl Pts',(-19.6747293616063,-49.6559812856024,
122.23534414131)) ;
#57041=CARTESIAN_POINT('Ctrl Pts',(-19.7410945155702,-49.4759922051219,
121.941224683029)) ;
#57042=CARTESIAN_POINT('Ctrl Pts',(-19.4655008779412,-49.666023976995,122.207142648671)) ;
#57043=CARTESIAN_POINT('Ctrl Pts',(-19.4795590979007,-49.4860348965146,
121.905973034113)) ;
#57044=CARTESIAN_POINT('Ctrl Pts',(-19.2578087514022,-49.6759105102126,
122.215430584698)) ;
#57045=CARTESIAN_POINT('Ctrl Pts',(-19.2199428620303,-49.4959214297321,
121.916333239267)) ;
#57046=CARTESIAN_POINT('Ctrl Pts',(-19.0524672632715,-49.6859036551446,
122.259778671092)) ;
#57047=CARTESIAN_POINT('Ctrl Pts',(-18.9632658836805,-49.5059145746641,
121.971768765041)) ;
#57048=CARTESIAN_POINT('Ctrl Pts',(-18.8588885046853,-49.6958493359811,
122.3388088344)) ;
#57049=CARTESIAN_POINT('Ctrl Pts',(-18.7212920166234,-49.5158602555006,
122.070557018354)) ;
#57050=CARTESIAN_POINT('Ctrl Pts',(-18.6817080873745,-49.7057965931296,
122.449910909112)) ;
#57051=CARTESIAN_POINT('Ctrl Pts',(-18.4998162838952,-49.5258075126491,
122.209435357085)) ;
#57052=CARTESIAN_POINT('Ctrl Pts',(-18.5251114478869,-49.7158444970016,
122.591672777569)) ;
#57053=CARTESIAN_POINT('Ctrl Pts',(-18.304070955553,-49.5358554165211,122.386637839432)) ;
#57054=CARTESIAN_POINT('Ctrl Pts',(-18.3979488536748,-49.7256921960996,
122.755046538999)) ;
#57055=CARTESIAN_POINT('Ctrl Pts',(-18.145117242453,-49.5457031156191,122.590856449649)) ;
#57056=CARTESIAN_POINT('Ctrl Pts',(-18.2993856740285,-49.7356536870782,
122.939814886333)) ;
#57057=CARTESIAN_POINT('Ctrl Pts',(-18.0219137174262,-49.5556646065978,
122.821817640605)) ;
#57058=CARTESIAN_POINT('Ctrl Pts',(-18.2342214042971,-49.7456831494922,
123.140352456418)) ;
#57059=CARTESIAN_POINT('Ctrl Pts',(-17.9404590217541,-49.5656940690117,
123.072489705592)) ;
#57060=CARTESIAN_POINT('Ctrl Pts',(-18.2051140091869,-49.7555903805921,
123.346589615801)) ;
#57061=CARTESIAN_POINT('Ctrl Pts',(-17.904075330187,-49.5756013001116,123.330287135653)) ;
#57062=CARTESIAN_POINT('Ctrl Pts',(-18.211860951267,-49.7655367592695,123.555572269236)) ;
#57063=CARTESIAN_POINT('Ctrl Pts',(-17.912509878086,-49.585547678789,123.591516015352)) ;
#57064=CARTESIAN_POINT('Ctrl Pts',(-18.2549768342654,-49.7755415280784,
123.761455951672)) ;
#57065=CARTESIAN_POINT('Ctrl Pts',(-17.9664056107729,-49.5955524475979,
123.848870528869)) ;
#57066=CARTESIAN_POINT('Ctrl Pts',(-18.3335291933488,-49.7855626490986,
123.956934913202)) ;
#57067=CARTESIAN_POINT('Ctrl Pts',(-18.0645967711896,-49.6055735686181,
124.093218904719)) ;
#57068=CARTESIAN_POINT('Ctrl Pts',(-18.4431860931502,-49.7954535149512,
124.133615577516)) ;
#57069=CARTESIAN_POINT('Ctrl Pts',(-18.2016691690772,-49.6154644344707,
124.314070124151)) ;
#57070=CARTESIAN_POINT('Ctrl Pts',(-18.5830122161219,-49.8054443237105,
124.290330824793)) ;
#57071=CARTESIAN_POINT('Ctrl Pts',(-18.3764527035837,-49.62545524323,124.509963683078)) ;
#57072=CARTESIAN_POINT('Ctrl Pts',(-18.747304518671,-49.8153949818908,124.419846948591)) ;
#57073=CARTESIAN_POINT('Ctrl Pts',(-18.5818191089981,-49.6354059014103,
124.671858407389)) ;
#57074=CARTESIAN_POINT('Ctrl Pts',(-18.9311656323854,-49.8253311915329,
124.518959631838)) ;
#57075=CARTESIAN_POINT('Ctrl Pts',(-18.8116465770376,-49.6453421110524,
124.795748611864)) ;
#57076=CARTESIAN_POINT('Ctrl Pts',(-19.1303351595038,-49.8353143582578,
124.585224682126)) ;
#57077=CARTESIAN_POINT('Ctrl Pts',(-19.0606091019101,-49.6553252777773,
124.87857888627)) ;
#57078=CARTESIAN_POINT('Ctrl Pts',(-19.3392535954594,-49.8453581554681,
124.615693199531)) ;
#57079=CARTESIAN_POINT('Ctrl Pts',(-19.3217571085241,-49.6653690749876,
124.916663479723)) ;
#57080=CARTESIAN_POINT('Ctrl Pts',(-19.5458273359172,-49.8551863716364,
124.610045735336)) ;
#57081=CARTESIAN_POINT('Ctrl Pts',(-19.5799756953261,-49.6751972911558,
124.90960289312)) ;
#57082=CARTESIAN_POINT('Ctrl Pts',(-19.7533454043374,-49.8652629391056,
124.567682590718)) ;
#57083=CARTESIAN_POINT('Ctrl Pts',(-19.8393726054797,-49.6852738586251,
124.856647819379)) ;
#57084=CARTESIAN_POINT('Ctrl Pts',(-19.9460859117418,-49.875115024795,124.491728264813)) ;
#57085=CARTESIAN_POINT('Ctrl Pts',(-20.0802989167655,-49.6951259443145,
124.761703259226)) ;
#57086=CARTESIAN_POINT('Ctrl Pts',(-20.126701616753,-49.8851882922004,124.381226191815)) ;
#57087=CARTESIAN_POINT('Ctrl Pts',(-20.3060674977483,-49.7051992117199,
124.623574722153)) ;
#57088=CARTESIAN_POINT('Ctrl Pts',(-20.2817328321541,-49.895029708624,124.244194431429)) ;
#57089=CARTESIAN_POINT('Ctrl Pts',(-20.4998566129317,-49.7150406281435,
124.452283158368)) ;
#57090=CARTESIAN_POINT('Ctrl Pts',(-20.4127836030217,-49.9049909667667,
124.080861209861)) ;
#57091=CARTESIAN_POINT('Ctrl Pts',(-20.6636690761592,-49.7250018862862,
124.248115309387)) ;
#57092=CARTESIAN_POINT('Ctrl Pts',(-20.5138903858792,-49.9150276431986,
123.895664527938)) ;
#57093=CARTESIAN_POINT('Ctrl Pts',(-20.7900512079499,-49.7350385627182,
124.016618869512)) ;
#57094=CARTESIAN_POINT('Ctrl Pts',(-20.5805838627807,-49.9249062510625,
123.698962304801)) ;
#57095=CARTESIAN_POINT('Ctrl Pts',(-20.8734168718336,-49.744917170582,123.770739635663)) ;
#57096=CARTESIAN_POINT('Ctrl Pts',(-20.6127292545574,-49.9349664797013,
123.489949368876)) ;
#57097=CARTESIAN_POINT('Ctrl Pts',(-20.9135969836862,-49.7549773992208,
123.50947350539)) ;
#57098=CARTESIAN_POINT('Ctrl Pts',(-20.6082434967595,-49.9448334638621,
123.282536648227)) ;
#57099=CARTESIAN_POINT('Ctrl Pts',(-20.9079881467094,-49.7648443833816,
123.250206599939)) ;
#57100=CARTESIAN_POINT('Ctrl Pts',(-20.5676533220387,-49.9548390301148,
123.076169983753)) ;
#57101=CARTESIAN_POINT('Ctrl Pts',(-20.8572486898122,-49.7748499496343,
122.992248524958)) ;
#57102=CARTESIAN_POINT('Ctrl Pts',(-20.4919395617635,-49.9648228185294,
122.880371545976)) ;
#57103=CARTESIAN_POINT('Ctrl Pts',(-20.7626047939458,-49.7848337380489,
122.747500893185)) ;
#57104=CARTESIAN_POINT('Ctrl Pts',(-20.3825347856944,-49.974868675332,122.699741996269)) ;
#57105=CARTESIAN_POINT('Ctrl Pts',(-20.6258474890933,-49.7948795948515,
122.521714953315)) ;
#57106=CARTESIAN_POINT('Ctrl Pts',(-20.246666531369,-49.984694552548,122.544142027715)) ;
#57107=CARTESIAN_POINT('Ctrl Pts',(-20.4560100050582,-49.8047054720675,
122.327215169929)) ;
#57108=CARTESIAN_POINT('Ctrl Pts',(-20.0835826601991,-49.9946850283893,
122.411791016735)) ;
#57109=CARTESIAN_POINT('Ctrl Pts',(-20.252153795509,-49.8146959479088,122.16177782072)) ;
#57110=CARTESIAN_POINT('Ctrl Pts',(-19.8987503711464,-50.0047286042881,
122.309710132215)) ;
#57111=CARTESIAN_POINT('Ctrl Pts',(-20.0211126979257,-49.8247395238076,
122.03417835313)) ;
#57112=CARTESIAN_POINT('Ctrl Pts',(-19.7035546402409,-50.0145503965861,
122.242375343609)) ;
#57113=CARTESIAN_POINT('Ctrl Pts',(-19.7771162249332,-49.8345613161056,
121.95001127871)) ;
#57114=CARTESIAN_POINT('Ctrl Pts',(-19.495286249998,-50.024585362212,122.208741496858)) ;
#57115=CARTESIAN_POINT('Ctrl Pts',(-19.5167805110306,-49.8445962817315,
121.907971037083)) ;
#57116=CARTESIAN_POINT('Ctrl Pts',(-19.2845564519754,-50.034610279145,122.21236484356)) ;
#57117=CARTESIAN_POINT('Ctrl Pts',(-19.2533683214096,-49.8546211986646,
121.912502122611)) ;
#57118=CARTESIAN_POINT('Ctrl Pts',(-19.0811423574655,-50.0444622175212,
122.251384498715)) ;
#57119=CARTESIAN_POINT('Ctrl Pts',(-18.9991000928775,-49.8644731370407,
121.961278882103)) ;
#57120=CARTESIAN_POINT('Ctrl Pts',(-18.8847759421629,-50.0544531935459,
122.325861032936)) ;
#57121=CARTESIAN_POINT('Ctrl Pts',(-18.7536426684467,-49.8744641130654,
122.054376600757)) ;
#57122=CARTESIAN_POINT('Ctrl Pts',(-18.7055278261908,-50.0643710143496,
122.432422183055)) ;
#57123=CARTESIAN_POINT('Ctrl Pts',(-18.5295831347982,-49.8843819338691,
122.187580190288)) ;
#57124=CARTESIAN_POINT('Ctrl Pts',(-18.5457533128135,-50.0743997349142,
122.569951039098)) ;
#57125=CARTESIAN_POINT('Ctrl Pts',(-18.3298664400282,-49.8944106544337,
122.35949288137)) ;
#57126=CARTESIAN_POINT('Ctrl Pts',(-18.4140890328722,-50.0842826615234,
122.730702151589)) ;
#57127=CARTESIAN_POINT('Ctrl Pts',(-18.1652873215396,-49.9042935810429,
122.560433756569)) ;
#57128=CARTESIAN_POINT('Ctrl Pts',(-18.3108162869546,-50.0942869466428,
122.913895712092)) ;
#57129=CARTESIAN_POINT('Ctrl Pts',(-18.0361983459777,-49.9142978661624,
122.789426912386)) ;
#57130=CARTESIAN_POINT('Ctrl Pts',(-18.2410673724431,-50.1042706278507,
123.111893587272)) ;
#57131=CARTESIAN_POINT('Ctrl Pts',(-17.9490142970122,-49.9242815473702,
123.036925185799)) ;
#57132=CARTESIAN_POINT('Ctrl Pts',(-18.20680742649,-50.1143116265806,123.320172550146)) ;
#57133=CARTESIAN_POINT('Ctrl Pts',(-17.9061915787471,-49.9343225461001,
123.29727415585)) ;
#57134=CARTESIAN_POINT('Ctrl Pts',(-18.2088904962245,-50.1241440714477,
123.52687311072)) ;
#57135=CARTESIAN_POINT('Ctrl Pts',(-17.908797723189,-49.9441549909672,123.555650792539)) ;
#57136=CARTESIAN_POINT('Ctrl Pts',(-18.2468487955305,-50.1341390698781,
123.733536628154)) ;
#57137=CARTESIAN_POINT('Ctrl Pts',(-17.9562480236737,-49.9541499893976,
123.813979871603)) ;
#57138=CARTESIAN_POINT('Ctrl Pts',(-18.3208110885934,-50.1441706186277,
123.931048389592)) ;
#57139=CARTESIAN_POINT('Ctrl Pts',(-18.048703067227,-49.9641815381472,124.060868718077)) ;
#57140=CARTESIAN_POINT('Ctrl Pts',(-18.4259334331203,-50.1540359969332,
124.109821606205)) ;
#57141=CARTESIAN_POINT('Ctrl Pts',(-18.1801084381385,-49.9740469164527,
124.284334653835)) ;
#57142=CARTESIAN_POINT('Ctrl Pts',(-18.5613765662075,-50.1639978443934,
124.26956672375)) ;
#57143=CARTESIAN_POINT('Ctrl Pts',(-18.3494144438133,-49.984008763913,124.484014611013)) ;
#57144=CARTESIAN_POINT('Ctrl Pts',(-18.7238875342035,-50.1740327852077,
124.404073431431)) ;
#57145=CARTESIAN_POINT('Ctrl Pts',(-18.5525546908186,-49.9940437047272,
124.65214608364)) ;
#57146=CARTESIAN_POINT('Ctrl Pts',(-18.9044058295045,-50.1839177462248,
124.507085840432)) ;
#57147=CARTESIAN_POINT('Ctrl Pts',(-18.7782043026535,-50.0039286657444,
124.780909685997)) ;
#57148=CARTESIAN_POINT('Ctrl Pts',(-19.103599497382,-50.1939833551437,124.578405574943)) ;
#57149=CARTESIAN_POINT('Ctrl Pts',(-19.0271970939725,-50.0139942746632,
124.870056934682)) ;
#57150=CARTESIAN_POINT('Ctrl Pts',(-19.3074891707686,-50.2038225301854,
124.613469337633)) ;
#57151=CARTESIAN_POINT('Ctrl Pts',(-19.2820603187289,-50.0238334497049,
124.913884244431)) ;
#57152=CARTESIAN_POINT('Ctrl Pts',(-19.5190104294486,-50.2138850856853,
124.612870871899)) ;
#57153=CARTESIAN_POINT('Ctrl Pts',(-19.5464617510583,-50.0338960052048,
124.913133557283)) ;
#57154=CARTESIAN_POINT('Ctrl Pts',(-19.7237883029565,-50.2237822603782,
124.575939416995)) ;
#57155=CARTESIAN_POINT('Ctrl Pts',(-19.8024340996861,-50.0437931798978,
124.86696663096)) ;
#57156=CARTESIAN_POINT('Ctrl Pts',(-19.9199318195631,-50.2337129753016,
124.504433105692)) ;
#57157=CARTESIAN_POINT('Ctrl Pts',(-20.0476128623709,-50.0537238948211,
124.777581121193)) ;
#57158=CARTESIAN_POINT('Ctrl Pts',(-20.1026202548277,-50.2437570033792,
124.398553787405)) ;
#57159=CARTESIAN_POINT('Ctrl Pts',(-20.2759720548009,-50.0637679228987,
124.64522970371)) ;
#57160=CARTESIAN_POINT('Ctrl Pts',(-20.2617301651388,-50.2536432052325,
124.264811495273)) ;
#57161=CARTESIAN_POINT('Ctrl Pts',(-20.4748580561478,-50.073654124752,124.478049523118)) ;
#57162=CARTESIAN_POINT('Ctrl Pts',(-20.3968653014659,-50.2636363716993,
124.103982279919)) ;
#57163=CARTESIAN_POINT('Ctrl Pts',(-20.6437749692228,-50.0836472912189,
124.277011182846)) ;
#57164=CARTESIAN_POINT('Ctrl Pts',(-20.5015352977048,-50.2735758426865,
123.923098316065)) ;
#57165=CARTESIAN_POINT('Ctrl Pts',(-20.7746102357307,-50.093586762206,124.050904663447)) ;
#57166=CARTESIAN_POINT('Ctrl Pts',(-20.5737859343558,-50.2835923570407,
123.725325502378)) ;
#57167=CARTESIAN_POINT('Ctrl Pts',(-20.8649209947813,-50.1036032765602,
123.803687665032)) ;
#57168=CARTESIAN_POINT('Ctrl Pts',(-20.6104642438826,-50.2935223835175,
123.519782917965)) ;
#57169=CARTESIAN_POINT('Ctrl Pts',(-20.9107662309863,-50.113533303037,123.546758707791)) ;
#57170=CARTESIAN_POINT('Ctrl Pts',(-20.6108086522076,-50.303574919027,123.308465111307)) ;
#57171=CARTESIAN_POINT('Ctrl Pts',(-20.911194011605,-50.1235858385465,123.282611468897)) ;
#57172=CARTESIAN_POINT('Ctrl Pts',(-20.5753140283502,-50.3134213222466,
123.104521388382)) ;
#57173=CARTESIAN_POINT('Ctrl Pts',(-20.8668229608976,-50.1334322417662,
123.02768188532)) ;
#57174=CARTESIAN_POINT('Ctrl Pts',(-20.5047639569835,-50.3233833651007,
122.907340910753)) ;
#57175=CARTESIAN_POINT('Ctrl Pts',(-20.7786326900258,-50.1433942846202,
122.781207115368)) ;
#57176=CARTESIAN_POINT('Ctrl Pts',(-20.4001053609626,-50.3334119158914,
122.724304136021)) ;
#57177=CARTESIAN_POINT('Ctrl Pts',(-20.6478070137,-50.1534228354109,122.552412487742)) ;
#57178=CARTESIAN_POINT('Ctrl Pts',(-20.2669138933572,-50.343322241609,122.564103535408)) ;
#57179=CARTESIAN_POINT('Ctrl Pts',(-20.4813154003933,-50.1633331611285,
122.352163354325)) ;
#57180=CARTESIAN_POINT('Ctrl Pts',(-20.1078761445415,-50.3532571534386,
122.428702223204)) ;
#57181=CARTESIAN_POINT('Ctrl Pts',(-20.2825162868525,-50.1732680729581,
122.182913771785)) ;
#57182=CARTESIAN_POINT('Ctrl Pts',(-19.9257330097845,-50.3632981602067,
122.32201626754)) ;
#57183=CARTESIAN_POINT('Ctrl Pts',(-20.0548359116665,-50.1833090797262,
122.049558725216)) ;
#57184=CARTESIAN_POINT('Ctrl Pts',(-19.7308882493759,-50.3731857930389,
122.249563232581)) ;
#57185=CARTESIAN_POINT('Ctrl Pts',(-19.8112788264832,-50.1931967125584,
121.958995011196)) ;
#57186=CARTESIAN_POINT('Ctrl Pts',(-19.5243853029293,-50.3831762241369,
122.211289416377)) ;
#57187=CARTESIAN_POINT('Ctrl Pts',(-19.5531495649875,-50.2031871436564,
121.911155500771)) ;
#57188=CARTESIAN_POINT('Ctrl Pts',(-19.3150912519442,-50.3931316606941,
122.209571649096)) ;
#57189=CARTESIAN_POINT('Ctrl Pts',(-19.2915318675942,-50.2131425802137,
121.909011127435)) ;
#57190=CARTESIAN_POINT('Ctrl Pts',(-19.1095552736864,-50.4030426087935,
122.243685794913)) ;
#57191=CARTESIAN_POINT('Ctrl Pts',(-19.0346123537931,-50.223053528313,121.951656547133)) ;
#57192=CARTESIAN_POINT('Ctrl Pts',(-18.9109486179919,-50.4130546848912,
122.313456614259)) ;
#57193=CARTESIAN_POINT('Ctrl Pts',(-18.786354698485,-50.2330656044107,122.038872975787)) ;
#57194=CARTESIAN_POINT('Ctrl Pts',(-18.727435602444,-50.4230820069661,122.417161220471)) ;
#57195=CARTESIAN_POINT('Ctrl Pts',(-18.5569655229776,-50.2430929264857,
122.168505406345)) ;
#57196=CARTESIAN_POINT('Ctrl Pts',(-18.5670779315736,-50.4329407819203,
122.548532884562)) ;
#57197=CARTESIAN_POINT('Ctrl Pts',(-18.3565173090446,-50.2529517014398,
122.332725267534)) ;
#57198=CARTESIAN_POINT('Ctrl Pts',(-18.3833334191599,-50.4463669747327,
122.762717425023)) ;
#57199=CARTESIAN_POINT('Ctrl Pts',(-18.1268538969004,-50.2663778942522,
122.600443072263)) ;
#57200=CARTESIAN_POINT('Ctrl Pts',(-18.2623681721055,-50.4594509905141,
123.013391436687)) ;
#57201=CARTESIAN_POINT('Ctrl Pts',(-17.9756521685596,-50.2794619100337,
122.913754436123)) ;
#57202=CARTESIAN_POINT('Ctrl Pts',(-18.2092179613212,-50.4729244392694,
123.29151187479)) ;
#57203=CARTESIAN_POINT('Ctrl Pts',(-17.9092019312809,-50.2929353587889,
123.261460162943)) ;
#57204=CARTESIAN_POINT('Ctrl Pts',(-18.2065405992436,-50.4827573970752,
123.498250206426)) ;
#57205=CARTESIAN_POINT('Ctrl Pts',(-17.9058612704974,-50.3027683165947,
123.519872041673)) ;
#57206=CARTESIAN_POINT('Ctrl Pts',(-18.2393587707171,-50.4927206705259,
123.705106522157)) ;
#57207=CARTESIAN_POINT('Ctrl Pts',(-17.9468858269984,-50.3127315900454,
123.778444889164)) ;
#57208=CARTESIAN_POINT('Ctrl Pts',(-18.3085355723821,-50.5027577443438,
123.904453594488)) ;
#57209=CARTESIAN_POINT('Ctrl Pts',(-18.0333597049391,-50.3227686638634,
124.027627149756)) ;
#57210=CARTESIAN_POINT('Ctrl Pts',(-18.409286084184,-50.5126327473555,124.085999426355)) ;
#57211=CARTESIAN_POINT('Ctrl Pts',(-18.1593001784576,-50.332643666875,124.254558222602)) ;
#57212=CARTESIAN_POINT('Ctrl Pts',(-18.5425517962584,-50.5227004269817,
124.250393752023)) ;
#57213=CARTESIAN_POINT('Ctrl Pts',(-18.3258841680297,-50.3427113465012,
124.460049112042)) ;
#57214=CARTESIAN_POINT('Ctrl Pts',(-18.6986982462725,-50.5325412771994,
124.386149557232)) ;
#57215=CARTESIAN_POINT('Ctrl Pts',(-18.5210703742057,-50.3525521967189,
124.629743115024)) ;
#57216=CARTESIAN_POINT('Ctrl Pts',(-18.9386955742681,-50.5458774756753,
124.531065619422)) ;
#57217=CARTESIAN_POINT('Ctrl Pts',(-18.8210606851902,-50.3658883951949,
124.810877501258)) ;
#57218=CARTESIAN_POINT('Ctrl Pts',(-19.2087059356425,-50.5590949994898,
124.609228100724)) ;
#57219=CARTESIAN_POINT('Ctrl Pts',(-19.1585310682669,-50.3791059190093,
124.908576997398)) ;
#57220=CARTESIAN_POINT('Ctrl Pts',(-19.488920896454,-50.572429925981,124.615199991677)) ;
#57221=CARTESIAN_POINT('Ctrl Pts',(-19.5088595130197,-50.3924408455006,
124.916046148063)) ;
#57222=CARTESIAN_POINT('Ctrl Pts',(-19.6963926036681,-50.5824130265756,
124.583239687426)) ;
#57223=CARTESIAN_POINT('Ctrl Pts',(-19.7681867122923,-50.4024239460952,
124.876091752379)) ;
#57224=CARTESIAN_POINT('Ctrl Pts',(-19.8962274127877,-50.5924578024753,
124.515046658216)) ;
#57225=CARTESIAN_POINT('Ctrl Pts',(-20.0179829922926,-50.4124687219948,
124.790847910401)) ;
#57226=CARTESIAN_POINT('Ctrl Pts',(-20.0772393222898,-50.6022757256612,
124.415835187125)) ;
#57227=CARTESIAN_POINT('Ctrl Pts',(-20.2442444734922,-50.4222866451807,
124.666833014762)) ;
#57228=CARTESIAN_POINT('Ctrl Pts',(-20.2423226616433,-50.6123250396165,
124.284011355845)) ;
#57229=CARTESIAN_POINT('Ctrl Pts',(-20.4505999320312,-50.432335959136,124.502045801009)) ;
#57230=CARTESIAN_POINT('Ctrl Pts',(-20.4268261999454,-50.6256287802391,
124.073810716125)) ;
#57231=CARTESIAN_POINT('Ctrl Pts',(-20.6812147144193,-50.4456396997586,
124.239319481669)) ;
#57232=CARTESIAN_POINT('Ctrl Pts',(-20.5831565120962,-50.6421189757157,
123.759929328214)) ;
#57233=CARTESIAN_POINT('Ctrl Pts',(-20.8766371022421,-50.4621298952353,
123.846918741814)) ;
#57234=CARTESIAN_POINT('Ctrl Pts',(-20.6233943821416,-50.6588381406404,
123.40675844073)) ;
#57235=CARTESIAN_POINT('Ctrl Pts',(-20.926926793522,-50.4788490601599,123.405534034858)) ;
#57236=CARTESIAN_POINT('Ctrl Pts',(-20.5824794471599,-50.6719991343105,
123.133106842893)) ;
#57237=CARTESIAN_POINT('Ctrl Pts',(-20.8757804023398,-50.49201005383,123.063406602083)) ;
#57238=CARTESIAN_POINT('Ctrl Pts',(-20.516519250953,-50.6819953564158,122.933581400906)) ;
#57239=CARTESIAN_POINT('Ctrl Pts',(-20.7933286315983,-50.5020062759353,
122.814013822107)) ;
#57240=CARTESIAN_POINT('Ctrl Pts',(-20.4162173833348,-50.6920191959495,
122.748251975362)) ;
#57241=CARTESIAN_POINT('Ctrl Pts',(-20.6679470250345,-50.512030115469,122.582347913081)) ;
#57242=CARTESIAN_POINT('Ctrl Pts',(-20.2443086428061,-50.7052125179428,
122.530542353315)) ;
#57243=CARTESIAN_POINT('Ctrl Pts',(-20.4530703197071,-50.5252234374623,
122.310222407797)) ;
#57244=CARTESIAN_POINT('Ctrl Pts',(-19.9606322188696,-50.7218716897201,
122.318490004045)) ;
#57245=CARTESIAN_POINT('Ctrl Pts',(-20.0984605250235,-50.5418826092396,
122.045150356451)) ;
#57246=CARTESIAN_POINT('Ctrl Pts',(-19.5552783088555,-50.7417818652058,
122.196329453374)) ;
#57247=CARTESIAN_POINT('Ctrl Pts',(-19.5917715292075,-50.5617927847253,
121.892456854642)) ;
#57248=CARTESIAN_POINT('Ctrl Pts',(-19.1329219062142,-50.7616718530502,
122.218924903769)) ;
#57249=CARTESIAN_POINT('Ctrl Pts',(-19.0638261203038,-50.5816827725697,
121.920703930721)) ;
#57250=CARTESIAN_POINT('Ctrl Pts',(-18.7416302883475,-50.781677301065,122.385558421519)) ;
#57251=CARTESIAN_POINT('Ctrl Pts',(-18.5747132437699,-50.6016882205845,
122.128999458592)) ;
#57252=CARTESIAN_POINT('Ctrl Pts',(-18.4328824089552,-50.8015136950923,
122.673074672253)) ;
#57253=CARTESIAN_POINT('Ctrl Pts',(-18.1887817455253,-50.6215246146118,
122.488396022904)) ;
#57254=CARTESIAN_POINT('Ctrl Pts',(-18.2390777335758,-50.821521488989,123.051656272595)) ;
#57255=CARTESIAN_POINT('Ctrl Pts',(-17.9465286195624,-50.6415324085085,
122.961624501202)) ;
#57256=CARTESIAN_POINT('Ctrl Pts',(-18.1864063154851,-50.8413481252829,
123.469998542685)) ;
#57257=CARTESIAN_POINT('Ctrl Pts',(-17.8806923531252,-50.6613590448024,
123.484550765069)) ;
#57258=CARTESIAN_POINT('Ctrl Pts',(-18.279598430072,-50.8613270682368,123.884440335655)) ;
#57259=CARTESIAN_POINT('Ctrl Pts',(-17.99718458044,-50.6813379877563,124.002602226893)) ;
#57260=CARTESIAN_POINT('Ctrl Pts',(-18.5086965529277,-50.8812588701058,
124.240917370752)) ;
#57261=CARTESIAN_POINT('Ctrl Pts',(-18.283558724871,-50.7012697896254,124.448196582463)) ;
#57262=CARTESIAN_POINT('Ctrl Pts',(-18.8431584214289,-50.9010831706034,
124.497674618011)) ;
#57263=CARTESIAN_POINT('Ctrl Pts',(-18.7016353947099,-50.7210940901229,
124.769140330364)) ;
#57264=CARTESIAN_POINT('Ctrl Pts',(-19.2506039421692,-50.9211791719433,
124.62581638792)) ;
#57265=CARTESIAN_POINT('Ctrl Pts',(-19.2109425558623,-50.7411900914627,
124.929317666411)) ;
#57266=CARTESIAN_POINT('Ctrl Pts',(-19.6705888408136,-50.9409375880472,
124.607973358778)) ;
#57267=CARTESIAN_POINT('Ctrl Pts',(-19.7359254653455,-50.7609485075667,
124.907008256675)) ;
#57268=CARTESIAN_POINT('Ctrl Pts',(-20.0654721859542,-50.9610312809313,
124.445475299511)) ;
#57269=CARTESIAN_POINT('Ctrl Pts',(-20.2295077366867,-50.7810422004508,
124.703903011912)) ;
#57270=CARTESIAN_POINT('Ctrl Pts',(-20.2716279154534,-50.9741422468379,
124.257625275152)) ;
#57271=CARTESIAN_POINT('Ctrl Pts',(-20.4872438679816,-50.7941531663575,
124.469055541413)) ;
#57272=CARTESIAN_POINT('Ctrl Pts',(-20.357892637621,-50.9808556216258,124.146615798218)) ;
#57273=CARTESIAN_POINT('Ctrl Pts',(-20.5950497968806,-50.8008665411453,
124.330315451521)) ;
#57274=CARTESIAN_POINT('',(-18.0898543520415,-12.1693713464509,124.125218065099)) ;
#57275=CARTESIAN_POINT('',(-17.9274924084134,-12.1498929727495,123.644402320537)) ;
#57276=CARTESIAN_POINT('Ctrl Pts',(-18.0898543518917,-12.1693713463351,
124.125218065234)) ;
#57277=CARTESIAN_POINT('Ctrl Pts',(-18.1107251988235,-12.1855021497363,
124.106411345451)) ;
#57278=CARTESIAN_POINT('Ctrl Pts',(-18.1304694810459,-12.2014740553584,
124.085663653832)) ;
#57279=CARTESIAN_POINT('Ctrl Pts',(-18.1672576147845,-12.2331466325994,
124.038148222986)) ;
#57280=CARTESIAN_POINT('Ctrl Pts',(-18.1843150887597,-12.2490832455646,
124.010368233214)) ;
#57281=CARTESIAN_POINT('Ctrl Pts',(-18.2056877954049,-12.2722339064756,
123.958712601024)) ;
#57282=CARTESIAN_POINT('Ctrl Pts',(-18.2123701677247,-12.2807335431958,
123.935854209123)) ;
#57283=CARTESIAN_POINT('Ctrl Pts',(-18.2181185876305,-12.291774580405,123.895191373631)) ;
#57284=CARTESIAN_POINT('Ctrl Pts',(-18.21884719455,-12.2953090478409,123.878001998223)) ;
#57285=CARTESIAN_POINT('Ctrl Pts',(-18.2166942034222,-12.2989586422489,
123.849069156915)) ;
#57286=CARTESIAN_POINT('Ctrl Pts',(-18.2149368250641,-12.2998030471561,
123.837528420933)) ;
#57287=CARTESIAN_POINT('Ctrl Pts',(-18.2110620214478,-12.3000404731419,
123.821269100306)) ;
#57288=CARTESIAN_POINT('Ctrl Pts',(-18.2097329849641,-12.2999877851218,
123.816451295881)) ;
#57289=CARTESIAN_POINT('Ctrl Pts',(-18.207972662911,-12.2997790216126,123.810859304896)) ;
#57290=CARTESIAN_POINT('Ctrl Pts',(-18.2077076065518,-12.2997444373638,
123.810035197199)) ;
#57291=CARTESIAN_POINT('Ctrl Pts',(-18.2074255071376,-12.299704400868,123.809176454917)) ;
#57292=CARTESIAN_POINT('Ctrl Pts',(-18.2074135269255,-12.2997026946395,
123.809140019673)) ;
#57293=CARTESIAN_POINT('Ctrl Pts',(-18.2073953439793,-12.2997000959883,
123.809084771462)) ;
#57294=CARTESIAN_POINT('Ctrl Pts',(-18.207389148473,-12.2996992089591,123.809065955664)) ;
#57295=CARTESIAN_POINT('Ctrl Pts',(-18.2073762490693,-12.2996973588126,
123.809026798846)) ;
#57296=CARTESIAN_POINT('Ctrl Pts',(-18.2073695447124,-12.2996963953616,
123.809006457953)) ;
#57297=CARTESIAN_POINT('Ctrl Pts',(-18.2073595638262,-12.2996949583005,
123.808976191801)) ;
#57298=CARTESIAN_POINT('Ctrl Pts',(-18.2073562896495,-12.2996944864394,
123.808966265658)) ;
#57299=CARTESIAN_POINT('Ctrl Pts',(-18.207350487964,-12.299693649543,123.808948681443)) ;
#57300=CARTESIAN_POINT('Ctrl Pts',(-18.2073479607712,-12.2996932847316,
123.808941023316)) ;
#57301=CARTESIAN_POINT('Ctrl Pts',(-18.2073426945459,-12.2996925239825,
123.808925068233)) ;
#57302=CARTESIAN_POINT('Ctrl Pts',(-18.2073399554604,-12.2996921279915,
123.808916771376)) ;
#57303=CARTESIAN_POINT('Ctrl Pts',(-18.2073328524603,-12.299691100309,123.808895260494)) ;
#57304=CARTESIAN_POINT('Ctrl Pts',(-18.2073284877422,-12.2996904680284,
123.808882046723)) ;
#57305=CARTESIAN_POINT('Ctrl Pts',(-18.2073102435383,-12.2996878218805,
123.808826832669)) ;
#57306=CARTESIAN_POINT('Ctrl Pts',(-18.2072963521413,-12.299685799183,123.808784836724)) ;
#57307=CARTESIAN_POINT('Ctrl Pts',(-18.2067002687993,-12.2995986671134,
123.806984700008)) ;
#57308=CARTESIAN_POINT('Ctrl Pts',(-18.2060950417741,-12.2994964054139,
123.805235382609)) ;
#57309=CARTESIAN_POINT('Ctrl Pts',(-18.2029100719787,-12.2988910495203,
123.796412826518)) ;
#57310=CARTESIAN_POINT('Ctrl Pts',(-18.1999823466222,-12.2981229845307,
123.789508567045)) ;
#57311=CARTESIAN_POINT('Ctrl Pts',(-18.1907776852835,-12.2952052971042,
123.770713859956)) ;
#57312=CARTESIAN_POINT('Ctrl Pts',(-18.1837783560155,-12.2924682785729,
123.759423255741)) ;
#57313=CARTESIAN_POINT('Ctrl Pts',(-18.1647286466641,-12.2841136491298,
123.734251409911)) ;
#57314=CARTESIAN_POINT('Ctrl Pts',(-18.1519831900975,-12.27787160617,123.721427746504)) ;
#57315=CARTESIAN_POINT('Ctrl Pts',(-18.1183690064087,-12.2604608869746,
123.694387616855)) ;
#57316=CARTESIAN_POINT('Ctrl Pts',(-18.0964700298874,-12.2483832091272,
123.682080321854)) ;
#57317=CARTESIAN_POINT('Ctrl Pts',(-18.031885753796,-12.2118235042901,123.655137433837)) ;
#57318=CARTESIAN_POINT('Ctrl Pts',(-17.9824298926407,-12.1827151160779,
123.645606479208)) ;
#57319=CARTESIAN_POINT('Ctrl Pts',(-17.9274924082143,-12.1498929726306,
123.644402320532)) ;
#57320=CARTESIAN_POINT('',(-20.5746457983858,-12.,122.467488525849)) ;
#57321=CARTESIAN_POINT('Ctrl Pts',(-20.5746457983858,-12.,122.467488525849)) ;
#57322=CARTESIAN_POINT('Ctrl Pts',(-20.5627382419342,-12.0007217907825,
122.452815451161)) ;
#57323=CARTESIAN_POINT('Ctrl Pts',(-20.4947798807797,-12.0047464667125,
122.372266602231)) ;
#57324=CARTESIAN_POINT('Ctrl Pts',(-20.3539293395536,-12.0121810504321,
122.236896566325)) ;
#57325=CARTESIAN_POINT('Ctrl Pts',(-20.1370409747147,-12.0221110972068,
122.091764368012)) ;
#57326=CARTESIAN_POINT('Ctrl Pts',(-19.8980237231667,-12.0320625395439,
121.985643564698)) ;
#57327=CARTESIAN_POINT('Ctrl Pts',(-19.6416983085707,-12.0421093367232,
121.922384338977)) ;
#57328=CARTESIAN_POINT('Ctrl Pts',(-19.3835093232675,-12.0519572774033,
121.904703348343)) ;
#57329=CARTESIAN_POINT('Ctrl Pts',(-19.1231275997313,-12.0619189087459,
121.931627958287)) ;
#57330=CARTESIAN_POINT('Ctrl Pts',(-18.8697470442625,-12.0719475681218,
122.004163670847)) ;
#57331=CARTESIAN_POINT('Ctrl Pts',(-18.6355935850335,-12.08185787101,122.118142693142)) ;
#57332=CARTESIAN_POINT('Ctrl Pts',(-18.4238474019827,-12.0917927655722,
122.270883953054)) ;
#57333=CARTESIAN_POINT('Ctrl Pts',(-18.2400799717895,-12.1018338642391,
122.460231143199)) ;
#57334=CARTESIAN_POINT('Ctrl Pts',(-18.0940875093298,-12.1117211467435,
122.675182672206)) ;
#57335=CARTESIAN_POINT('Ctrl Pts',(-17.9861176823212,-12.121712887254,122.914511116819)) ;
#57336=CARTESIAN_POINT('Ctrl Pts',(-17.921689729601,-12.1316634364894,123.16795292873)) ;
#57337=CARTESIAN_POINT('Ctrl Pts',(-17.9030108427875,-12.1410363173938,
123.413537993095)) ;
#57338=CARTESIAN_POINT('Ctrl Pts',(-17.9162454187765,-12.1471236046148,
123.57278095633)) ;
#57339=CARTESIAN_POINT('Ctrl Pts',(-17.9274924084134,-12.1498929727495,
123.644402320537)) ;
#57340=CARTESIAN_POINT('',(-20.6888487350626,-11.9999999997025,122.656717008064)) ;
#57341=CARTESIAN_POINT('Ctrl Pts',(-20.5746457983858,-12.,122.467488525849)) ;
#57342=CARTESIAN_POINT('Ctrl Pts',(-20.5960286970766,-12.,122.497557942705)) ;
#57343=CARTESIAN_POINT('Ctrl Pts',(-20.6162418843401,-12.0000000000049,
122.528364603676)) ;
#57344=CARTESIAN_POINT('Ctrl Pts',(-20.6543685264773,-12.0000000000049,
122.591550197525)) ;
#57345=CARTESIAN_POINT('Ctrl Pts',(-20.6722191984465,-12.,122.62383024764)) ;
#57346=CARTESIAN_POINT('Ctrl Pts',(-20.6888487341057,-12.,122.656717008548)) ;
#57347=CARTESIAN_POINT('Ctrl Pts',(-20.6888487348625,-11.9999999994367,
122.656717007968)) ;
#57348=CARTESIAN_POINT('Ctrl Pts',(-20.6504013293531,-12.0242010028557,
122.669878337729)) ;
#57349=CARTESIAN_POINT('Ctrl Pts',(-20.6126735676598,-12.0487776575878,
122.685887455227)) ;
#57350=CARTESIAN_POINT('Ctrl Pts',(-20.5429100063498,-12.0961255449868,
122.722350893296)) ;
#57351=CARTESIAN_POINT('Ctrl Pts',(-20.5100459148922,-12.1193501392808,
122.742829239747)) ;
#57352=CARTESIAN_POINT('Ctrl Pts',(-20.4795958757324,-12.1420202642929,
122.766130796517)) ;
#57353=CARTESIAN_POINT('Ctrl Pts',(-18.0898543520415,-12.1693713464509,
124.125218065099)) ;
#57354=CARTESIAN_POINT('Ctrl Pts',(-18.0987410756712,-12.1700845612802,
124.141640469505)) ;
#57355=CARTESIAN_POINT('Ctrl Pts',(-18.1505706173883,-12.174105036101,124.233279228286)) ;
#57356=CARTESIAN_POINT('Ctrl Pts',(-18.263117466536,-12.1814863726884,124.391272663474)) ;
#57357=CARTESIAN_POINT('Ctrl Pts',(-18.4514152853576,-12.1915186409522,
124.575779592005)) ;
#57358=CARTESIAN_POINT('Ctrl Pts',(-18.6649582254988,-12.2013826029581,
124.722768521293)) ;
#57359=CARTESIAN_POINT('Ctrl Pts',(-18.9056381213548,-12.211452664303,124.832713751572)) ;
#57360=CARTESIAN_POINT('Ctrl Pts',(-19.1560012005742,-12.2212950286517,
124.897694900574)) ;
#57361=CARTESIAN_POINT('Ctrl Pts',(-19.4168488001017,-12.2312557011542,
124.919426126704)) ;
#57362=CARTESIAN_POINT('Ctrl Pts',(-19.6794781670334,-12.241293772222,124.894826056415)) ;
#57363=CARTESIAN_POINT('Ctrl Pts',(-19.9298584470305,-12.2511673871824,
124.826609084731)) ;
#57364=CARTESIAN_POINT('Ctrl Pts',(-20.1692027685541,-12.2612396217637,
124.713703674863)) ;
#57365=CARTESIAN_POINT('Ctrl Pts',(-20.3802336084559,-12.2710636402125,
124.56490174156)) ;
#57366=CARTESIAN_POINT('Ctrl Pts',(-20.5668505339034,-12.2811285611885,
124.3775468474)) ;
#57367=CARTESIAN_POINT('Ctrl Pts',(-20.7654710388387,-12.2943388594833,
124.092731380698)) ;
#57368=CARTESIAN_POINT('Ctrl Pts',(-20.8864681734945,-12.3076543062152,
123.760293059331)) ;
#57369=CARTESIAN_POINT('Ctrl Pts',(-20.9168412402485,-12.3209445514825,
123.412248798329)) ;
#57370=CARTESIAN_POINT('Ctrl Pts',(-20.8936136564304,-12.3309953010896,
123.149204261583)) ;
#57371=CARTESIAN_POINT('Ctrl Pts',(-20.8271599100472,-12.3408079080718,
122.900008574106)) ;
#57372=CARTESIAN_POINT('Ctrl Pts',(-20.7159339872492,-12.3508790060661,
122.659895486434)) ;
#57373=CARTESIAN_POINT('Ctrl Pts',(-20.5671825471141,-12.360768578841,122.446765213332)) ;
#57374=CARTESIAN_POINT('Ctrl Pts',(-20.3217335957846,-12.3740386856443,
122.199036770175)) ;
#57375=CARTESIAN_POINT('Ctrl Pts',(-19.9402799223287,-12.3906553725668,
121.976489963183)) ;
#57376=CARTESIAN_POINT('Ctrl Pts',(-19.5069560654083,-12.407229415883,121.897341845887)) ;
#57377=CARTESIAN_POINT('Ctrl Pts',(-19.1586250796142,-12.4205259833148,
121.925240968701)) ;
#57378=CARTESIAN_POINT('Ctrl Pts',(-18.9035497915594,-12.4305560468922,
121.991664800906)) ;
#57379=CARTESIAN_POINT('Ctrl Pts',(-18.6671468529052,-12.4404499387415,
122.099840645972)) ;
#57380=CARTESIAN_POINT('Ctrl Pts',(-18.3796682061191,-12.453702694527,122.296549637466)) ;
#57381=CARTESIAN_POINT('Ctrl Pts',(-18.0908280313655,-12.4704307995195,
122.634462100718)) ;
#57382=CARTESIAN_POINT('Ctrl Pts',(-17.9056069777788,-12.4902616359979,
123.128014485523)) ;
#57383=CARTESIAN_POINT('Ctrl Pts',(-17.8986058474029,-12.5101870278881,
123.65743523967)) ;
#57384=CARTESIAN_POINT('Ctrl Pts',(-18.0728134812496,-12.5301122412401,
124.157630024429)) ;
#57385=CARTESIAN_POINT('Ctrl Pts',(-18.4070561283902,-12.5500372547252,
124.568319257347)) ;
#57386=CARTESIAN_POINT('Ctrl Pts',(-18.8599799731256,-12.5699137264252,
124.840308096966)) ;
#57387=CARTESIAN_POINT('Ctrl Pts',(-19.3811313633293,-12.5898930443341,
124.942158139695)) ;
#57388=CARTESIAN_POINT('Ctrl Pts',(-19.9045262603243,-12.6098260479101,
124.859844414469)) ;
#57389=CARTESIAN_POINT('Ctrl Pts',(-20.3677432424192,-12.6297213179378,
124.6048789893)) ;
#57390=CARTESIAN_POINT('Ctrl Pts',(-20.7170498595964,-12.6496426558436,
124.206944794287)) ;
#57391=CARTESIAN_POINT('Ctrl Pts',(-20.9098403565593,-12.6696002791098,
123.712751204342)) ;
#57392=CARTESIAN_POINT('Ctrl Pts',(-20.922485985003,-12.689480111067,123.18461209717)) ;
#57393=CARTESIAN_POINT('Ctrl Pts',(-20.7554545445051,-12.7093619623639,
122.683172172836)) ;
#57394=CARTESIAN_POINT('Ctrl Pts',(-20.4235254244291,-12.7294329794677,
122.265649141046)) ;
#57395=CARTESIAN_POINT('Ctrl Pts',(-19.9749237655201,-12.7492402032208,
121.989968961482)) ;
#57396=CARTESIAN_POINT('Ctrl Pts',(-19.4550399386783,-12.7692213387896,
121.881799009553)) ;
#57397=CARTESIAN_POINT('Ctrl Pts',(-18.9310095255677,-12.7891488321288,
121.958350587305)) ;
#57398=CARTESIAN_POINT('Ctrl Pts',(-18.4660378435683,-12.8089694934866,
122.206286369213)) ;
#57399=CARTESIAN_POINT('Ctrl Pts',(-18.1095237058469,-12.8290666827084,
122.603786127405)) ;
#57400=CARTESIAN_POINT('Ctrl Pts',(-17.9128685242105,-12.8488303617167,
123.091145395877)) ;
#57401=CARTESIAN_POINT('Ctrl Pts',(-17.8934532250119,-12.8688876403898,
123.623648070234)) ;
#57402=CARTESIAN_POINT('Ctrl Pts',(-18.0551868058747,-12.8886830641372,
124.124451004221)) ;
#57403=CARTESIAN_POINT('Ctrl Pts',(-18.3794288064129,-12.9086467088648,
124.544379679826)) ;
#57404=CARTESIAN_POINT('Ctrl Pts',(-18.8287006511552,-12.9286302001389,
124.827680379695)) ;
#57405=CARTESIAN_POINT('Ctrl Pts',(-19.3429186866301,-12.9484376952882,
124.94073161998)) ;
#57406=CARTESIAN_POINT('Ctrl Pts',(-19.8693844497185,-12.9684202860083,
124.871533418394)) ;
#57407=CARTESIAN_POINT('Ctrl Pts',(-20.3384447754671,-12.9883029399996,
124.627871581349)) ;
#57408=CARTESIAN_POINT('Ctrl Pts',(-20.6976976848122,-13.0082611848626,
124.237731507644)) ;
#57409=CARTESIAN_POINT('Ctrl Pts',(-20.9017768869257,-13.0281367719042,
123.750397269444)) ;
#57410=CARTESIAN_POINT('Ctrl Pts',(-20.9278087943981,-13.0481176600395,
123.220011471926)) ;
#57411=CARTESIAN_POINT('Ctrl Pts',(-20.7712144053819,-13.0680528011505,
122.713763278227)) ;
#57412=CARTESIAN_POINT('Ctrl Pts',(-20.4520106816014,-13.0879648191615,
122.291696114272)) ;
#57413=CARTESIAN_POINT('Ctrl Pts',(-20.0087285877316,-13.1078530374051,
122.003722192709)) ;
#57414=CARTESIAN_POINT('Ctrl Pts',(-19.5791090604564,-13.124451341252,121.903703056221)) ;
#57415=CARTESIAN_POINT('Ctrl Pts',(-19.2304680801455,-13.1377239311549,
121.914976366624)) ;
#57416=CARTESIAN_POINT('Ctrl Pts',(-18.9730360739326,-13.1477313461057,
121.968723010403)) ;
#57417=CARTESIAN_POINT('Ctrl Pts',(-18.7289237747832,-13.1577386928383,
122.066570256317)) ;
#57418=CARTESIAN_POINT('Ctrl Pts',(-18.4326373531694,-13.1710050526399,
122.250316913842)) ;
#57419=CARTESIAN_POINT('Ctrl Pts',(-18.1316373287835,-13.1875197102629,
122.569692622284)) ;
#57420=CARTESIAN_POINT('Ctrl Pts',(-17.9558681007045,-13.2041171435055,
122.974265631492)) ;
#57421=CARTESIAN_POINT('Ctrl Pts',(-17.9045373896821,-13.2174651406505,
123.321302564893)) ;
#57422=CARTESIAN_POINT('Ctrl Pts',(-17.9113737957956,-13.2273608950021,
123.581262925382)) ;
#57423=CARTESIAN_POINT('Ctrl Pts',(-17.9634088821012,-13.2373488489335,
123.838506352538)) ;
#57424=CARTESIAN_POINT('Ctrl Pts',(-18.0589349739685,-13.2473060726382,
124.082144873651)) ;
#57425=CARTESIAN_POINT('Ctrl Pts',(-18.1964661586106,-13.2573416191949,
124.307146372465)) ;
#57426=CARTESIAN_POINT('Ctrl Pts',(-18.3682700533626,-13.267228730471,124.502082982706)) ;
#57427=CARTESIAN_POINT('Ctrl Pts',(-18.573168600081,-13.2772201355718,124.666246335832)) ;
#57428=CARTESIAN_POINT('Ctrl Pts',(-18.8024527486924,-13.2871657567866,
124.791696662128)) ;
#57429=CARTESIAN_POINT('Ctrl Pts',(-19.0499707909463,-13.2971150050549,
124.87596822317)) ;
#57430=CARTESIAN_POINT('Ctrl Pts',(-19.3109074952385,-13.3071615002235,
124.91606420447)) ;
#57431=CARTESIAN_POINT('Ctrl Pts',(-19.5697458477253,-13.3170128430151,
124.910614060128)) ;
#57432=CARTESIAN_POINT('Ctrl Pts',(-19.8268961278364,-13.3269846231424,
124.86034740168)) ;
#57433=CARTESIAN_POINT('Ctrl Pts',(-20.0720441858723,-13.3369798231201,
124.765921346646)) ;
#57434=CARTESIAN_POINT('Ctrl Pts',(-20.2977248332106,-13.3470138148161,
124.629595035348)) ;
#57435=CARTESIAN_POINT('Ctrl Pts',(-20.4930785404264,-13.3568692197887,
124.459519571124)) ;
#57436=CARTESIAN_POINT('Ctrl Pts',(-20.6585461151986,-13.3668685176344,
124.255447402342)) ;
#57437=CARTESIAN_POINT('Ctrl Pts',(-20.7850259763668,-13.3767636302396,
124.028196369691)) ;
#57438=CARTESIAN_POINT('Ctrl Pts',(-20.8714967332555,-13.3868242757746,
123.778389961119)) ;
#57439=CARTESIAN_POINT('Ctrl Pts',(-20.9125557494614,-13.3966731527638,
123.522828864941)) ;
#57440=CARTESIAN_POINT('Ctrl Pts',(-20.9092102411542,-13.4067018638574,
123.259309807964)) ;
#57441=CARTESIAN_POINT('Ctrl Pts',(-20.8594509750379,-13.4167312651135,
123.00048234628)) ;
#57442=CARTESIAN_POINT('Ctrl Pts',(-20.7678172835609,-13.4265714569095,
122.758667592175)) ;
#57443=CARTESIAN_POINT('Ctrl Pts',(-20.6338292437046,-13.4365748861025,
122.532528063033)) ;
#57444=CARTESIAN_POINT('Ctrl Pts',(-20.4628072717642,-13.4465603985687,
122.333446821148)) ;
#57445=CARTESIAN_POINT('Ctrl Pts',(-20.258572195235,-13.4566014949527,122.16640991458)) ;
#57446=CARTESIAN_POINT('Ctrl Pts',(-20.0331061121126,-13.4664446909037,
122.03957718795)) ;
#57447=CARTESIAN_POINT('Ctrl Pts',(-19.7857320971473,-13.4764310019581,
121.952101012445)) ;
#57448=CARTESIAN_POINT('Ctrl Pts',(-19.5282010411868,-13.4863656872158,
121.908939847016)) ;
#57449=CARTESIAN_POINT('Ctrl Pts',(-19.2639488168614,-13.4964232484328,
121.911409438826)) ;
#57450=CARTESIAN_POINT('Ctrl Pts',(-19.0100966675528,-13.5062448900415,
121.958214888149)) ;
#57451=CARTESIAN_POINT('Ctrl Pts',(-18.7623301682284,-13.5163009536324,
122.050058119956)) ;
#57452=CARTESIAN_POINT('Ctrl Pts',(-18.5371012425962,-13.5262416293942,
122.182417857288)) ;
#57453=CARTESIAN_POINT('Ctrl Pts',(-18.338478245611,-13.5361459881825,122.350628473911)) ;
#57454=CARTESIAN_POINT('Ctrl Pts',(-18.1698329826385,-13.5461926427584,
122.553733855565)) ;
#57455=CARTESIAN_POINT('Ctrl Pts',(-18.0407519036657,-13.5560882374012,
122.779526388176)) ;
#57456=CARTESIAN_POINT('Ctrl Pts',(-17.9513576421501,-13.5661501840581,
123.028342279855)) ;
#57457=CARTESIAN_POINT('Ctrl Pts',(-17.9074152113575,-13.5759998079902,
123.283436990171)) ;
#57458=CARTESIAN_POINT('Ctrl Pts',(-17.9075794490051,-13.5859630470201,
123.545245160118)) ;
#57459=CARTESIAN_POINT('Ctrl Pts',(-17.9538438452054,-13.5959876217959,
123.804601716854)) ;
#57460=CARTESIAN_POINT('Ctrl Pts',(-18.0433151854202,-13.6059061844836,
124.0494068293)) ;
#57461=CARTESIAN_POINT('Ctrl Pts',(-18.1745142883211,-13.6158983712076,
124.276882942804)) ;
#57462=CARTESIAN_POINT('Ctrl Pts',(-18.3442843563806,-13.6259331697918,
124.478655912716)) ;
#57463=CARTESIAN_POINT('Ctrl Pts',(-18.5426287178469,-13.6357883604655,
124.645217964009)) ;
#57464=CARTESIAN_POINT('Ctrl Pts',(-18.7699291705974,-13.6457877086185,
124.776978497853)) ;
#57465=CARTESIAN_POINT('Ctrl Pts',(-19.0140681533579,-13.6556828342936,
124.86662328346)) ;
#57466=CARTESIAN_POINT('Ctrl Pts',(-19.2742712713222,-13.6657433772417,
124.913241817981)) ;
#57467=CARTESIAN_POINT('Ctrl Pts',(-19.5331191647968,-13.6755926515086,
124.914103544901)) ;
#57468=CARTESIAN_POINT('Ctrl Pts',(-19.792878148494,-13.6856198760785,124.869872597639)) ;
#57469=CARTESIAN_POINT('Ctrl Pts',(-20.0408282968694,-13.6956482752663,
124.780544744153)) ;
#57470=CARTESIAN_POINT('Ctrl Pts',(-20.2655486146661,-13.7054940256798,
124.652339842706)) ;
#57471=CARTESIAN_POINT('Ctrl Pts',(-20.4679785318478,-13.7154828160805,
124.485209945321)) ;
#57472=CARTESIAN_POINT('Ctrl Pts',(-20.638747035496,-13.7255277444802,124.283933112254)) ;
#57473=CARTESIAN_POINT('Ctrl Pts',(-20.7695822850911,-13.7353522292692,
124.061344007578)) ;
#57474=CARTESIAN_POINT('Ctrl Pts',(-20.8622650301573,-13.7454096268104,
123.813853115559)) ;
#57475=CARTESIAN_POINT('Ctrl Pts',(-20.9096073544687,-13.7553357183966,
123.557318498504)) ;
#57476=CARTESIAN_POINT('Ctrl Pts',(-20.9123708210729,-13.7652905035412,
123.295734355723)) ;
#57477=CARTESIAN_POINT('Ctrl Pts',(-20.8690285856397,-13.7753278731988,
123.035549479101)) ;
#57478=CARTESIAN_POINT('Ctrl Pts',(-20.7826546061871,-13.7852166833204,
122.790448432935)) ;
#57479=CARTESIAN_POINT('Ctrl Pts',(-20.6541544832906,-13.7952060423715,
122.561546360115)) ;
#57480=CARTESIAN_POINT('Ctrl Pts',(-20.4882245281512,-13.8051645898276,
122.359184924028)) ;
#57481=CARTESIAN_POINT('Ctrl Pts',(-20.2912542115885,-13.8150641663786,
122.189215690163)) ;
#57482=CARTESIAN_POINT('Ctrl Pts',(-20.0644048944981,-13.8251120782093,
122.054135819925)) ;
#57483=CARTESIAN_POINT('Ctrl Pts',(-19.8213040212289,-13.8350074260699,
121.961702812424)) ;
#57484=CARTESIAN_POINT('Ctrl Pts',(-19.5616299165928,-13.8450691026011,
121.912040392459)) ;
#57485=CARTESIAN_POINT('Ctrl Pts',(-19.302943765994,-13.8549136203502,121.908260248801)) ;
#57486=CARTESIAN_POINT('Ctrl Pts',(-19.0443926106772,-13.864874064065,121.949016797608)) ;
#57487=CARTESIAN_POINT('Ctrl Pts',(-18.7951065533296,-13.8749108968832,
122.035163624274)) ;
#57488=CARTESIAN_POINT('Ctrl Pts',(-18.5679607592808,-13.88478969363,122.160911880469)) ;
#57489=CARTESIAN_POINT('Ctrl Pts',(-18.3623992980865,-13.8948490097584,
122.327074678705)) ;
#57490=CARTESIAN_POINT('Ctrl Pts',(-18.1920392191495,-13.9047194565116,
122.522692233472)) ;
#57491=CARTESIAN_POINT('Ctrl Pts',(-18.0559754687445,-13.9147120947696,
122.747289602296)) ;
#57492=CARTESIAN_POINT('Ctrl Pts',(-17.9611352243635,-13.9247441103175,
122.993260746216)) ;
#57493=CARTESIAN_POINT('Ctrl Pts',(-17.9107237978205,-13.9346099666241,
123.247603809028)) ;
#57494=CARTESIAN_POINT('Ctrl Pts',(-17.9051038745564,-13.9446792560932,
123.512124786768)) ;
#57495=CARTESIAN_POINT('Ctrl Pts',(-17.9445700338335,-13.9545228136446,
123.767790796992)) ;
#57496=CARTESIAN_POINT('Ctrl Pts',(-18.0281629110103,-13.9645029404324,
124.016370584098)) ;
#57497=CARTESIAN_POINT('Ctrl Pts',(-18.1545752563571,-13.9745214890323,
124.247305606012)) ;
#57498=CARTESIAN_POINT('Ctrl Pts',(-18.3165363213439,-13.9844047895555,
124.450385027953)) ;
#57499=CARTESIAN_POINT('Ctrl Pts',(-18.4859844039085,-13.9930026771457,
124.599786853217)) ;
#57500=CARTESIAN_POINT('Ctrl Pts',(-18.5982098542005,-13.9981476377442,
124.674581361741)) ;
#57501=CARTESIAN_POINT('Ctrl Pts',(-18.6398461652381,-13.9999999999504,
124.699448408814)) ;
#57502=CARTESIAN_POINT('Ctrl Pts',(-17.9901976317162,-10.,123.897592500161)) ;
#57503=CARTESIAN_POINT('Ctrl Pts',(-18.2740109056134,-9.82001091963712,
123.800437437226)) ;
#57504=CARTESIAN_POINT('Ctrl Pts',(-18.0463587734884,-10.0066268508181,
124.061733136808)) ;
#57505=CARTESIAN_POINT('Ctrl Pts',(-18.318952820002,-9.82663777045524,123.931772257896)) ;
#57506=CARTESIAN_POINT('Ctrl Pts',(-18.2158202083151,-10.0198574772991,
124.369865791197)) ;
#57507=CARTESIAN_POINT('Ctrl Pts',(-18.4544999964107,-9.83986839693625,
124.178242269465)) ;
#57508=CARTESIAN_POINT('Ctrl Pts',(-18.6148367045085,-10.0398330985578,
124.72010058675)) ;
#57509=CARTESIAN_POINT('Ctrl Pts',(-18.7737259547846,-9.85984401819488,
124.458448709452)) ;
#57510=CARTESIAN_POINT('Ctrl Pts',(-19.1081207670208,-10.0597504334597,
124.912141899864)) ;
#57511=CARTESIAN_POINT('Ctrl Pts',(-19.1683517739458,-9.87976135309682,
124.612076728176)) ;
#57512=CARTESIAN_POINT('Ctrl Pts',(-19.636206114934,-10.0796237101757,124.92549851548)) ;
#57513=CARTESIAN_POINT('Ctrl Pts',(-19.5908222086086,-9.89963462981282,
124.622761886445)) ;
#57514=CARTESIAN_POINT('Ctrl Pts',(-20.1407529320189,-10.0996482003397,
124.756244590335)) ;
#57515=CARTESIAN_POINT('Ctrl Pts',(-19.994458721673,-9.91965911997678,124.487357109044)) ;
#57516=CARTESIAN_POINT('Ctrl Pts',(-20.5540202995955,-10.1195160414904,
124.427406225433)) ;
#57517=CARTESIAN_POINT('Ctrl Pts',(-20.3250727353524,-9.9395269611275,124.224284451464)) ;
#57518=CARTESIAN_POINT('Ctrl Pts',(-20.8319818407582,-10.1394616923699,
123.976064807431)) ;
#57519=CARTESIAN_POINT('Ctrl Pts',(-20.547440485577,-9.95947261200706,123.863209762279)) ;
#57520=CARTESIAN_POINT('Ctrl Pts',(-20.9388342400949,-10.1593670929869,
123.457915382835)) ;
#57521=CARTESIAN_POINT('Ctrl Pts',(-20.6329204948871,-9.97937801262402,
123.448688955287)) ;
#57522=CARTESIAN_POINT('Ctrl Pts',(-20.8636098402301,-10.1792413208033,
122.935072644727)) ;
#57523=CARTESIAN_POINT('Ctrl Pts',(-20.5727382379585,-9.99925224044038,
123.03041411648)) ;
#57524=CARTESIAN_POINT('Ctrl Pts',(-20.6131115834081,-10.1992271116809,
122.466642059227)) ;
#57525=CARTESIAN_POINT('Ctrl Pts',(-20.3723371633396,-10.019238031318,122.655670872381)) ;
#57526=CARTESIAN_POINT('Ctrl Pts',(-20.219446657189,-10.2191213543406,122.11369274935)) ;
#57527=CARTESIAN_POINT('Ctrl Pts',(-20.0574027588299,-10.0391322739778,
122.373312971228)) ;
#57528=CARTESIAN_POINT('Ctrl Pts',(-19.729780773993,-10.2390000704127,121.915093775378)) ;
#57529=CARTESIAN_POINT('Ctrl Pts',(-19.6656681100072,-10.0590109900498,
122.21443654672)) ;
#57530=CARTESIAN_POINT('Ctrl Pts',(-19.1975679684769,-10.2590395202573,
121.895998337816)) ;
#57531=CARTESIAN_POINT('Ctrl Pts',(-19.2398980466007,-10.0790504398944,
122.199163431724)) ;
#57532=CARTESIAN_POINT('Ctrl Pts',(-18.6950312339923,-10.2789026817952,
122.058270950238)) ;
#57533=CARTESIAN_POINT('Ctrl Pts',(-18.837868920824,-10.0989136014323,122.328984924085)) ;
#57534=CARTESIAN_POINT('Ctrl Pts',(-18.2756669291778,-10.2988820498094,
122.383749835563)) ;
#57535=CARTESIAN_POINT('Ctrl Pts',(-18.5023795133954,-10.1188929694465,
122.589370885141)) ;
#57536=CARTESIAN_POINT('Ctrl Pts',(-17.9943038605785,-10.3186926303322,
122.828930487561)) ;
#57537=CARTESIAN_POINT('Ctrl Pts',(-18.2772917344201,-10.1387035499693,
122.945518187819)) ;
#57538=CARTESIAN_POINT('Ctrl Pts',(-17.8800540061898,-10.3386735586178,
123.347451469643)) ;
#57539=CARTESIAN_POINT('Ctrl Pts',(-18.1858955346146,-10.1586844782549,
123.360335798021)) ;
#57540=CARTESIAN_POINT('Ctrl Pts',(-17.949663613675,-10.3585662304872,123.871624239523)) ;
#57541=CARTESIAN_POINT('Ctrl Pts',(-18.2415877728661,-10.1785771501243,
123.779674103343)) ;
#57542=CARTESIAN_POINT('Ctrl Pts',(-18.1935384904851,-10.3784925607743,
124.34174209524)) ;
#57543=CARTESIAN_POINT('Ctrl Pts',(-18.4366892418074,-10.1985034804115,
124.155765909524)) ;
#57544=CARTESIAN_POINT('Ctrl Pts',(-18.5843830566034,-10.3984631148666,
124.700856014279)) ;
#57545=CARTESIAN_POINT('Ctrl Pts',(-18.7493759717748,-10.2184740345037,
124.44305681766)) ;
#57546=CARTESIAN_POINT('Ctrl Pts',(-18.9897866675992,-10.4149949539542,
124.870306748339)) ;
#57547=CARTESIAN_POINT('Ctrl Pts',(-19.0736749228579,-10.2350058735914,
124.578605598989)) ;
#57548=CARTESIAN_POINT('Ctrl Pts',(-19.3371420473607,-10.4283346927818,
124.917711789777)) ;
#57549=CARTESIAN_POINT('Ctrl Pts',(-19.3515822796175,-10.2483456124189,
124.6165344309)) ;
#57550=CARTESIAN_POINT('Ctrl Pts',(-19.6005562667331,-10.4383669350004,
124.907063768782)) ;
#57551=CARTESIAN_POINT('Ctrl Pts',(-19.5623087731277,-10.2583778546375,
124.608012505296)) ;
#57552=CARTESIAN_POINT('Ctrl Pts',(-19.8537397870735,-10.4482246356439,
124.852203726746)) ;
#57553=CARTESIAN_POINT('Ctrl Pts',(-19.7648571225557,-10.268235555281,124.564122220758)) ;
#57554=CARTESIAN_POINT('Ctrl Pts',(-20.0969735539785,-10.4582165002831,
124.753332920083)) ;
#57555=CARTESIAN_POINT('Ctrl Pts',(-19.9594412734619,-10.2782274199202,
124.485025314983)) ;
#57556=CARTESIAN_POINT('Ctrl Pts',(-20.3177787346395,-10.4681390500432,
124.614652183365)) ;
#57557=CARTESIAN_POINT('Ctrl Pts',(-20.1360907041886,-10.2881499696804,
124.374071880139)) ;
#57558=CARTESIAN_POINT('Ctrl Pts',(-20.5771970981362,-10.4814168235367,
124.381203458891)) ;
#57559=CARTESIAN_POINT('Ctrl Pts',(-20.3435922192053,-10.3014277431738,
124.18734533642)) ;
#57560=CARTESIAN_POINT('Ctrl Pts',(-20.7701003708174,-10.4947641624773,
124.083584310457)) ;
#57561=CARTESIAN_POINT('Ctrl Pts',(-20.4979358992389,-10.3147750821144,
123.949230612993)) ;
#57562=CARTESIAN_POINT('Ctrl Pts',(-20.8774553693723,-10.5079713942705,
123.753475217054)) ;
#57563=CARTESIAN_POINT('Ctrl Pts',(-20.5838202404129,-10.3279823139076,
123.685128879657)) ;
#57564=CARTESIAN_POINT('Ctrl Pts',(-20.9145282391216,-10.5179585103602,
123.493699384276)) ;
#57565=CARTESIAN_POINT('Ctrl Pts',(-20.6134756829108,-10.3379694299973,
123.477310647391)) ;
#57566=CARTESIAN_POINT('Ctrl Pts',(-20.9061303769722,-10.52790941594,123.232285620267)) ;
#57567=CARTESIAN_POINT('Ctrl Pts',(-20.6067552793287,-10.3479203355771,
123.268178977505)) ;
#57568=CARTESIAN_POINT('Ctrl Pts',(-20.8516285272166,-10.5379645179474,
122.973767430347)) ;
#57569=CARTESIAN_POINT('Ctrl Pts',(-20.5631517097427,-10.3579754375845,
123.061365248372)) ;
#57570=CARTESIAN_POINT('Ctrl Pts',(-20.755752145473,-10.5477861912685,122.734100762332)) ;
#57571=CARTESIAN_POINT('Ctrl Pts',(-20.4864480022253,-10.3677971109056,
122.869632334128)) ;
#57572=CARTESIAN_POINT('Ctrl Pts',(-20.6168357130529,-10.5578446623434,
122.509252277714)) ;
#57573=CARTESIAN_POINT('Ctrl Pts',(-20.3753148734437,-10.3778555819805,
122.689756047917)) ;
#57574=CARTESIAN_POINT('Ctrl Pts',(-20.4430403513938,-10.5677692735199,
122.314768071456)) ;
#57575=CARTESIAN_POINT('Ctrl Pts',(-20.2362698376991,-10.387780193157,122.534165626482)) ;
#57576=CARTESIAN_POINT('Ctrl Pts',(-20.1694406712993,-10.5810466124203,
122.098190251904)) ;
#57577=CARTESIAN_POINT('Ctrl Pts',(-20.0174235370575,-10.4010575320574,
122.360928563111)) ;
#57578=CARTESIAN_POINT('Ctrl Pts',(-19.8449850134819,-10.5943454916579,
121.958111265335)) ;
#57579=CARTESIAN_POINT('Ctrl Pts',(-19.7578454755217,-10.414356411295,122.248851541412)) ;
#57580=CARTESIAN_POINT('Ctrl Pts',(-19.5008057716341,-10.6075843638286,
121.907157355648)) ;
#57581=CARTESIAN_POINT('Ctrl Pts',(-19.4824812721784,-10.4275952834657,
122.208088431707)) ;
#57582=CARTESIAN_POINT('Ctrl Pts',(-19.2379220825872,-10.6175909819652,
121.913944971404)) ;
#57583=CARTESIAN_POINT('Ctrl Pts',(-19.2721785612158,-10.4376019016023,
122.213521362329)) ;
#57584=CARTESIAN_POINT('Ctrl Pts',(-18.9796997397484,-10.6276219270267,
121.966900411424)) ;
#57585=CARTESIAN_POINT('Ctrl Pts',(-19.0656000663898,-10.4476328466638,
122.255887759951)) ;
#57586=CARTESIAN_POINT('Ctrl Pts',(-18.7386663423424,-10.6374781003785,
122.061762842601)) ;
#57587=CARTESIAN_POINT('Ctrl Pts',(-18.8727746408769,-10.4574890200157,
122.33177976469)) ;
#57588=CARTESIAN_POINT('Ctrl Pts',(-18.5144394578762,-10.6474773713414,
122.198683103417)) ;
#57589=CARTESIAN_POINT('Ctrl Pts',(-18.6933942799492,-10.4674882909785,
122.44131783091)) ;
#57590=CARTESIAN_POINT('Ctrl Pts',(-18.3191873796767,-10.6573718230987,
122.370468477432)) ;
#57591=CARTESIAN_POINT('Ctrl Pts',(-18.5371942578644,-10.4773827427359,
122.578747654411)) ;
#57592=CARTESIAN_POINT('Ctrl Pts',(-18.1540827677519,-10.6674351389081,
122.576990252266)) ;
#57593=CARTESIAN_POINT('Ctrl Pts',(-18.4051122800728,-10.4874460585452,
122.743966484082)) ;
#57594=CARTESIAN_POINT('Ctrl Pts',(-18.0298636947034,-10.6772739956477,
122.80380319062)) ;
#57595=CARTESIAN_POINT('Ctrl Pts',(-18.3057391118683,-10.4972849152848,
122.925417599334)) ;
#57596=CARTESIAN_POINT('Ctrl Pts',(-17.9447485718205,-10.6873401174653,
123.054218033102)) ;
#57597=CARTESIAN_POINT('Ctrl Pts',(-18.2376490673584,-10.5073510371024,
123.125750218179)) ;
#57598=CARTESIAN_POINT('Ctrl Pts',(-17.9052474071487,-10.6972233451896,
123.310952604467)) ;
#57599=CARTESIAN_POINT('Ctrl Pts',(-18.2060503446323,-10.5172342648267,
123.331137917859)) ;
#57600=CARTESIAN_POINT('Ctrl Pts',(-17.9104088183902,-10.7072128064683,
123.573388107812)) ;
#57601=CARTESIAN_POINT('Ctrl Pts',(-18.2101816191011,-10.5272237261055,
123.541086174157)) ;
#57602=CARTESIAN_POINT('Ctrl Pts',(-17.9610292610865,-10.7171765168948,
123.830297049982)) ;
#57603=CARTESIAN_POINT('Ctrl Pts',(-18.2506800579227,-10.5371874365319,
123.746612765702)) ;
#57604=CARTESIAN_POINT('Ctrl Pts',(-18.055529675207,-10.7271715196257,124.075387412779)) ;
#57605=CARTESIAN_POINT('Ctrl Pts',(-18.3262823460712,-10.5471824392628,
123.942684211435)) ;
#57606=CARTESIAN_POINT('Ctrl Pts',(-18.1920485023394,-10.737207850636,124.30103460394)) ;
#57607=CARTESIAN_POINT('Ctrl Pts',(-18.4354992728269,-10.5572187702731,
124.12320085702)) ;
#57608=CARTESIAN_POINT('Ctrl Pts',(-18.3620830674316,-10.7470540799783,
124.496092551227)) ;
#57609=CARTESIAN_POINT('Ctrl Pts',(-18.5715282310147,-10.5670649996154,
124.279245472498)) ;
#57610=CARTESIAN_POINT('Ctrl Pts',(-18.5658978745921,-10.7570395782535,
124.661307439936)) ;
#57611=CARTESIAN_POINT('Ctrl Pts',(-18.7345812884953,-10.5770504978907,
124.411415684018)) ;
#57612=CARTESIAN_POINT('Ctrl Pts',(-18.7941275674691,-10.7669744812365,
124.788187738228)) ;
#57613=CARTESIAN_POINT('Ctrl Pts',(-18.9171658133098,-10.5869854008736,
124.51291799715)) ;
#57614=CARTESIAN_POINT('Ctrl Pts',(-19.0439620659958,-10.7770319843317,
124.874312872399)) ;
#57615=CARTESIAN_POINT('Ctrl Pts',(-19.1170341816332,-10.5970429039689,
124.58181616074)) ;
#57616=CARTESIAN_POINT('Ctrl Pts',(-19.2988377714799,-10.7868536407023,
124.915180256188)) ;
#57617=CARTESIAN_POINT('Ctrl Pts',(-19.3209344474807,-10.6068645603394,
124.614507954235)) ;
#57618=CARTESIAN_POINT('Ctrl Pts',(-19.5630543230624,-10.7969097033674,
124.911570311771)) ;
#57619=CARTESIAN_POINT('Ctrl Pts',(-19.5323077507347,-10.6169206230045,
124.611618015563)) ;
#57620=CARTESIAN_POINT('Ctrl Pts',(-19.819595446342,-10.8068503680706,124.862237558294)) ;
#57621=CARTESIAN_POINT('Ctrl Pts',(-19.7375400007717,-10.6268612877077,
124.572149858921)) ;
#57622=CARTESIAN_POINT('Ctrl Pts',(-20.0630665620373,-10.8167547720191,
124.77021482164)) ;
#57623=CARTESIAN_POINT('Ctrl Pts',(-19.9323158100592,-10.6367656916563,
124.498530010754)) ;
#57624=CARTESIAN_POINT('Ctrl Pts',(-20.2899670415844,-10.8268012570127,
124.635280761768)) ;
#57625=CARTESIAN_POINT('Ctrl Pts',(-20.1138352645202,-10.6468121766498,
124.390581038644)) ;
#57626=CARTESIAN_POINT('Ctrl Pts',(-20.4871895041345,-10.8366974848244,
124.465706330208)) ;
#57627=CARTESIAN_POINT('Ctrl Pts',(-20.2716116273665,-10.6567084044615,
124.254920337405)) ;
#57628=CARTESIAN_POINT('Ctrl Pts',(-20.6546848715982,-10.8467570683879,
124.261221540526)) ;
#57629=CARTESIAN_POINT('Ctrl Pts',(-20.4056065232405,-10.666767988025,124.091331180759)) ;
#57630=CARTESIAN_POINT('Ctrl Pts',(-20.7815048415044,-10.8566090780567,
124.035494716813)) ;
#57631=CARTESIAN_POINT('Ctrl Pts',(-20.5070605035221,-10.6766199976938,
123.910749362364)) ;
#57632=CARTESIAN_POINT('Ctrl Pts',(-20.8689878382938,-10.8665716094963,
123.788751735695)) ;
#57633=CARTESIAN_POINT('Ctrl Pts',(-20.5770451355397,-10.6865825291334,
123.713354624159)) ;
#57634=CARTESIAN_POINT('Ctrl Pts',(-20.912200798905,-10.8766031577357,123.528690516731)) ;
#57635=CARTESIAN_POINT('Ctrl Pts',(-20.6116136920761,-10.6966140773728,
123.505305293071)) ;
#57636=CARTESIAN_POINT('Ctrl Pts',(-20.9098873495447,-10.8864945689487,
123.268764662041)) ;
#57637=CARTESIAN_POINT('Ctrl Pts',(-20.6097611319996,-10.7065054885858,
123.297365172637)) ;
#57638=CARTESIAN_POINT('Ctrl Pts',(-20.8623452479891,-10.8965108226567,
123.009867420401)) ;
#57639=CARTESIAN_POINT('Ctrl Pts',(-20.5717257539026,-10.7165217422938,
123.090247714627)) ;
#57640=CARTESIAN_POINT('Ctrl Pts',(-20.7699148713601,-10.9065409255014,
122.763029266333)) ;
#57641=CARTESIAN_POINT('Ctrl Pts',(-20.4977797294624,-10.7265518451385,
122.89277779572)) ;
#57642=CARTESIAN_POINT('Ctrl Pts',(-20.6387642261451,-10.9163973744551,
122.539650565094)) ;
#57643=CARTESIAN_POINT('Ctrl Pts',(-20.3928580826567,-10.7364082940922,
122.714076343171)) ;
#57644=CARTESIAN_POINT('Ctrl Pts',(-20.4686808693851,-10.9263963852274,
122.339414946397)) ;
#57645=CARTESIAN_POINT('Ctrl Pts',(-20.2567901831118,-10.7464073048645,
122.553889022845)) ;
#57646=CARTESIAN_POINT('Ctrl Pts',(-20.2686322562331,-10.9362916021454,
122.17321802605)) ;
#57647=CARTESIAN_POINT('Ctrl Pts',(-20.0967507033617,-10.7563025217825,
122.420933115589)) ;
#57648=CARTESIAN_POINT('Ctrl Pts',(-20.0390441621644,-10.9463521175027,
122.042191046987)) ;
#57649=CARTESIAN_POINT('Ctrl Pts',(-19.9130792483847,-10.7663630371399,
122.316112859812)) ;
#57650=CARTESIAN_POINT('Ctrl Pts',(-19.7954165502139,-10.9562014108898,
121.954734482504)) ;
#57651=CARTESIAN_POINT('Ctrl Pts',(-19.7181774003615,-10.7762123305269,
122.246149405366)) ;
#57652=CARTESIAN_POINT('Ctrl Pts',(-19.5358374377705,-10.9662285865698,
121.909463378996)) ;
#57653=CARTESIAN_POINT('Ctrl Pts',(-19.5105138249597,-10.7862395062069,
122.209933979971)) ;
#57654=CARTESIAN_POINT('Ctrl Pts',(-19.2722869357793,-10.976257162197,121.910644966112)) ;
#57655=CARTESIAN_POINT('Ctrl Pts',(-19.2996733747243,-10.7962680818341,
122.210880867466)) ;
#57656=CARTESIAN_POINT('Ctrl Pts',(-19.0176264126342,-10.9861022557429,
121.956219772892)) ;
#57657=CARTESIAN_POINT('Ctrl Pts',(-19.0959461067893,-10.80611317538,122.247342053206)) ;
#57658=CARTESIAN_POINT('Ctrl Pts',(-18.7708903038592,-10.9960934971746,
122.045998590472)) ;
#57659=CARTESIAN_POINT('Ctrl Pts',(-18.8985578386737,-10.8161044168118,
122.319166355093)) ;
#57660=CARTESIAN_POINT('Ctrl Pts',(-18.5427482922778,-11.0061292783179,
122.178316886012)) ;
#57661=CARTESIAN_POINT('Ctrl Pts',(-18.7160448934344,-10.826140197955,122.425022334904)) ;
#57662=CARTESIAN_POINT('Ctrl Pts',(-18.3445251559911,-11.0159814840476,
122.344856285624)) ;
#57663=CARTESIAN_POINT('Ctrl Pts',(-18.5574679962225,-10.8359924036847,
122.558254360555)) ;
#57664=CARTESIAN_POINT('Ctrl Pts',(-18.1757880512695,-11.0259435781646,
122.545009574833)) ;
#57665=CARTESIAN_POINT('Ctrl Pts',(-18.422479486084,-10.8459544978017,122.718377561325)) ;
#57666=CARTESIAN_POINT('Ctrl Pts',(-18.0438458206682,-11.0359661389917,
122.7729601423)) ;
#57667=CARTESIAN_POINT('Ctrl Pts',(-18.3169268399301,-10.8559770586288,
122.900738711909)) ;
#57668=CARTESIAN_POINT('Ctrl Pts',(-17.9540915966108,-11.0458939106433,
123.017952668927)) ;
#57669=CARTESIAN_POINT('Ctrl Pts',(-18.245124831637,-10.8659048302804,123.096732704545)) ;
#57670=CARTESIAN_POINT('Ctrl Pts',(-17.9077456060715,-11.0559362947681,
123.277734456028)) ;
#57671=CARTESIAN_POINT('Ctrl Pts',(-18.2080492829974,-10.8759472144052,
123.304558492291)) ;
#57672=CARTESIAN_POINT('Ctrl Pts',(-17.9071113956414,-11.0658255188387,
123.537627775337)) ;
#57673=CARTESIAN_POINT('Ctrl Pts',(-18.2075431810581,-10.8858364384758,
123.512472408022)) ;
#57674=CARTESIAN_POINT('Ctrl Pts',(-17.9515732678051,-11.075814767006,123.796333212552)) ;
#57675=CARTESIAN_POINT('Ctrl Pts',(-18.2431137880875,-10.8958256866432,
123.719436394321)) ;
#57676=CARTESIAN_POINT('Ctrl Pts',(-18.0401957307403,-11.085773344048,124.042564530846)) ;
#57677=CARTESIAN_POINT('Ctrl Pts',(-18.3140127714057,-10.9057842636851,
123.916420715581)) ;
#57678=CARTESIAN_POINT('Ctrl Pts',(-18.168909061226,-11.0956729131393,124.268660685117)) ;
#57679=CARTESIAN_POINT('Ctrl Pts',(-18.4169840046767,-10.9156838327764,
124.097296505228)) ;
#57680=CARTESIAN_POINT('Ctrl Pts',(-18.337456729501,-11.1057208252233,124.471882073783)) ;
#57681=CARTESIAN_POINT('Ctrl Pts',(-18.5518230802635,-10.9257317448604,
124.259873062704)) ;
#57682=CARTESIAN_POINT('Ctrl Pts',(-18.5355938114042,-11.1156161795305,
124.640356432155)) ;
#57683=CARTESIAN_POINT('Ctrl Pts',(-18.7103328563198,-10.9356270991676,
124.394651291218)) ;
#57684=CARTESIAN_POINT('Ctrl Pts',(-18.7636640136148,-11.1256778300217,
124.774075513825)) ;
#57685=CARTESIAN_POINT('Ctrl Pts',(-18.8927897608012,-10.9456887496588,
124.50162580593)) ;
#57686=CARTESIAN_POINT('Ctrl Pts',(-19.006164366436,-11.1355224454842,124.864226909227)) ;
#57687=CARTESIAN_POINT('Ctrl Pts',(-19.0867894053353,-10.9555333651213,
124.573745602818)) ;
#57688=CARTESIAN_POINT('Ctrl Pts',(-19.2634346826531,-11.1454825243856,
124.912371167711)) ;
#57689=CARTESIAN_POINT('Ctrl Pts',(-19.2926054448866,-10.9654934440227,
124.612260162443)) ;
#57690=CARTESIAN_POINT('Ctrl Pts',(-19.527207804198,-11.1555207187439,124.914621442776)) ;
#57691=CARTESIAN_POINT('Ctrl Pts',(-19.5036240790433,-10.9755316383811,
124.614059468937)) ;
#57692=CARTESIAN_POINT('Ctrl Pts',(-19.7832249578582,-11.1653944341435,
124.872221302149)) ;
#57693=CARTESIAN_POINT('Ctrl Pts',(-19.7084367869545,-10.9854053537807,
124.580138714143)) ;
#57694=CARTESIAN_POINT('Ctrl Pts',(-20.0328232712046,-11.1754661436778,
124.784280775567)) ;
#57695=CARTESIAN_POINT('Ctrl Pts',(-19.9081154761896,-10.9954770633149,
124.509785425241)) ;
#57696=CARTESIAN_POINT('Ctrl Pts',(-20.2580073160466,-11.1852985841303,
124.657525797588)) ;
#57697=CARTESIAN_POINT('Ctrl Pts',(-20.0882613121544,-11.0053095037674,
124.408381348776)) ;
#57698=CARTESIAN_POINT('Ctrl Pts',(-20.4622563153842,-11.1953304050557,
124.490859965048)) ;
#57699=CARTESIAN_POINT('Ctrl Pts',(-20.2516602105671,-11.0153413246928,
124.275048161913)) ;
#57700=CARTESIAN_POINT('Ctrl Pts',(-20.6337047072471,-11.2053507749413,
124.290992198856)) ;
#57701=CARTESIAN_POINT('Ctrl Pts',(-20.388818355727,-11.0253616945784,124.115153420591)) ;
#57702=CARTESIAN_POINT('Ctrl Pts',(-20.7663802888455,-11.215217546075,124.068198059716)) ;
#57703=CARTESIAN_POINT('Ctrl Pts',(-20.4949578009106,-11.0352284657122,
123.936918629634)) ;
#57704=CARTESIAN_POINT('Ctrl Pts',(-20.8602333250101,-11.2252883172644,
123.820777914708)) ;
#57705=CARTESIAN_POINT('Ctrl Pts',(-20.5700397729981,-11.0452992369015,
123.738981987884)) ;
#57706=CARTESIAN_POINT('Ctrl Pts',(-20.9086197171465,-11.235131477786,123.566660443392)) ;
#57707=CARTESIAN_POINT('Ctrl Pts',(-20.608748082228,-11.0551423974231,123.535689006923)) ;
#57708=CARTESIAN_POINT('Ctrl Pts',(-20.9130575837451,-11.2451117109724,
123.304436329207)) ;
#57709=CARTESIAN_POINT('Ctrl Pts',(-20.6122979803846,-11.0651226306096,
123.325909958137)) ;
#57710=CARTESIAN_POINT('Ctrl Pts',(-20.871238578832,-11.2551302310076,123.044509679255)) ;
#57711=CARTESIAN_POINT('Ctrl Pts',(-20.5788422638188,-11.0751411506447,
123.117968711757)) ;
#57712=CARTESIAN_POINT('Ctrl Pts',(-20.7865977118334,-11.2650135393913,
122.798931493979)) ;
#57713=CARTESIAN_POINT('Ctrl Pts',(-20.5111294989851,-11.0850244590284,
122.921507117009)) ;
#57714=CARTESIAN_POINT('Ctrl Pts',(-20.6581795184354,-11.2750818235621,
122.567651782636)) ;
#57715=CARTESIAN_POINT('Ctrl Pts',(-20.4083944277967,-11.0950927431992,
122.736483258853)) ;
#57716=CARTESIAN_POINT('Ctrl Pts',(-20.4956768373956,-11.2849119502298,
122.366783576293)) ;
#57717=CARTESIAN_POINT('Ctrl Pts',(-20.278392801361,-11.1049228698669,122.575789859925)) ;
#57718=CARTESIAN_POINT('Ctrl Pts',(-20.2963683002106,-11.2949785224363,
122.192903170129)) ;
#57719=CARTESIAN_POINT('Ctrl Pts',(-20.1189455705143,-11.1149894420734,
122.436685510706)) ;
#57720=CARTESIAN_POINT('Ctrl Pts',(-20.0737183940731,-11.304868678677,122.058761956782)) ;
#57721=CARTESIAN_POINT('Ctrl Pts',(-19.9408262162374,-11.1248795983141,
122.329373218762)) ;
#57722=CARTESIAN_POINT('Ctrl Pts',(-19.8289002832035,-11.3148612062534,
121.963839656321)) ;
#57723=CARTESIAN_POINT('Ctrl Pts',(-19.7449718346838,-11.1348721258905,
122.253435573056)) ;
#57724=CARTESIAN_POINT('Ctrl Pts',(-19.5720596012938,-11.3248226961277,
121.913243325035)) ;
#57725=CARTESIAN_POINT('Ctrl Pts',(-19.53949961243,-11.1448336157648,122.212958778088)) ;
#57726=CARTESIAN_POINT('Ctrl Pts',(-19.3117087063765,-11.3347319180149,
121.907440658381)) ;
#57727=CARTESIAN_POINT('Ctrl Pts',(-19.3312196283681,-11.154742837652,122.208316707602)) ;
#57728=CARTESIAN_POINT('Ctrl Pts',(-19.0507261790839,-11.3447804978252,
121.947576761925)) ;
#57729=CARTESIAN_POINT('Ctrl Pts',(-19.1224334112309,-11.1647914174624,
122.240425692634)) ;
#57730=CARTESIAN_POINT('Ctrl Pts',(-18.8047397506185,-11.3546634722953,
122.030941792183)) ;
#57731=CARTESIAN_POINT('Ctrl Pts',(-18.9256451263576,-11.1746743919324,
122.307117480373)) ;
#57732=CARTESIAN_POINT('Ctrl Pts',(-18.5741327464813,-11.364658383438,122.156656022076)) ;
#57733=CARTESIAN_POINT('Ctrl Pts',(-18.7411596022947,-11.1846693030751,
122.407688711713)) ;
#57734=CARTESIAN_POINT('Ctrl Pts',(-18.3685394795987,-11.3746787700116,
122.321218804861)) ;
#57735=CARTESIAN_POINT('Ctrl Pts',(-18.5766849675727,-11.1946896896487,
122.539338955783)) ;
#57736=CARTESIAN_POINT('Ctrl Pts',(-18.1964679003152,-11.3845888738687,
122.516679816547)) ;
#57737=CARTESIAN_POINT('Ctrl Pts',(-18.4390281618024,-11.2045997935058,
122.69570718939)) ;
#57738=CARTESIAN_POINT('Ctrl Pts',(-18.0601098924679,-11.3945165860786,
122.739110167226)) ;
#57739=CARTESIAN_POINT('Ctrl Pts',(-18.3299418822673,-11.2145275057157,
122.873650852243)) ;
#57740=CARTESIAN_POINT('Ctrl Pts',(-17.9635464111682,-11.4045596958458,
122.984721718142)) ;
#57741=CARTESIAN_POINT('Ctrl Pts',(-18.2526908895868,-11.2245706154829,
123.070140194401)) ;
#57742=CARTESIAN_POINT('Ctrl Pts',(-17.9117458665147,-11.4144461163014,
123.239325516368)) ;
#57743=CARTESIAN_POINT('Ctrl Pts',(-18.2112504325607,-11.2344570359385,
123.273822340803)) ;
#57744=CARTESIAN_POINT('Ctrl Pts',(-17.9044206322636,-11.424439293907,123.501819128649)) ;
#57745=CARTESIAN_POINT('Ctrl Pts',(-18.2053899382535,-11.2444502135441,
123.483817059054)) ;
#57746=CARTESIAN_POINT('Ctrl Pts',(-17.9427031377925,-11.4343849568109,
123.760362733581)) ;
#57747=CARTESIAN_POINT('Ctrl Pts',(-18.2360155909013,-11.254395876448,123.690651513861)) ;
#57748=CARTESIAN_POINT('Ctrl Pts',(-18.0248064637638,-11.4443322530161,
124.008552115012)) ;
#57749=CARTESIAN_POINT('Ctrl Pts',(-18.3016977085877,-11.2643431726532,
123.889202714741)) ;
#57750=CARTESIAN_POINT('Ctrl Pts',(-18.1502567640289,-11.454380018594,124.240883955143)) ;
#57751=CARTESIAN_POINT('Ctrl Pts',(-18.402057739547,-11.2743909382311,124.075068526834)) ;
#57752=CARTESIAN_POINT('Ctrl Pts',(-18.31072897444,-11.4642282318116,124.443923603713)) ;
#57753=CARTESIAN_POINT('Ctrl Pts',(-18.5304345036023,-11.2842391514487,
124.237499615883)) ;
#57754=CARTESIAN_POINT('Ctrl Pts',(-18.5056290796381,-11.4741878046057,
124.618608195999)) ;
#57755=CARTESIAN_POINT('Ctrl Pts',(-18.6863538979281,-11.2941987242428,
124.377247496808)) ;
#57756=CARTESIAN_POINT('Ctrl Pts',(-18.7298566496538,-11.4842244256382,
124.757470221316)) ;
#57757=CARTESIAN_POINT('Ctrl Pts',(-18.8657357990191,-11.3042353452753,
124.488337605862)) ;
#57758=CARTESIAN_POINT('Ctrl Pts',(-18.9708633136617,-11.4941049404486,
124.854157638432)) ;
#57759=CARTESIAN_POINT('Ctrl Pts',(-19.0585400766373,-11.3141158600857,
124.565687764043)) ;
#57760=CARTESIAN_POINT('Ctrl Pts',(-19.2293390121453,-11.5041575917556,
124.90854357499)) ;
#57761=CARTESIAN_POINT('Ctrl Pts',(-19.265320722865,-11.3241685113927,124.609197170298)) ;
#57762=CARTESIAN_POINT('Ctrl Pts',(-19.4892814880954,-11.5140529900356,
124.917196362515)) ;
#57763=CARTESIAN_POINT('Ctrl Pts',(-19.4732739141341,-11.3340639096727,
124.61612002099)) ;
#57764=CARTESIAN_POINT('Ctrl Pts',(-19.7507413265183,-11.5241031117417,
124.880139860388)) ;
#57765=CARTESIAN_POINT('Ctrl Pts',(-19.6824420883012,-11.3441140313788,
124.586475461409)) ;
#57766=CARTESIAN_POINT('Ctrl Pts',(-19.9977235238706,-11.5339873912836,
124.799620909315)) ;
#57767=CARTESIAN_POINT('Ctrl Pts',(-19.8800272541223,-11.3539983109207,
124.522061213482)) ;
#57768=CARTESIAN_POINT('Ctrl Pts',(-20.2297217101426,-11.5439821725755,
124.676533838734)) ;
#57769=CARTESIAN_POINT('Ctrl Pts',(-20.0656260392352,-11.3639930922127,
124.423592342302)) ;
#57770=CARTESIAN_POINT('Ctrl Pts',(-20.4358226950316,-11.5539300177623,
124.515687379052)) ;
#57771=CARTESIAN_POINT('Ctrl Pts',(-20.2305069652934,-11.3739409373994,
124.294916057216)) ;
#57772=CARTESIAN_POINT('Ctrl Pts',(-20.6109276227123,-11.5638669811497,
124.321995034894)) ;
#57773=CARTESIAN_POINT('Ctrl Pts',(-20.37059121164,-11.3838779007868,124.139963144074)) ;
#57774=CARTESIAN_POINT('Ctrl Pts',(-20.7506923359331,-11.5738499458869,
124.099943607919)) ;
#57775=CARTESIAN_POINT('Ctrl Pts',(-20.482403674932,-11.3938608655241,123.962322680992)) ;
#57776=CARTESIAN_POINT('Ctrl Pts',(-20.8499100759965,-11.5838937973026,
123.855392878857)) ;
#57777=CARTESIAN_POINT('Ctrl Pts',(-20.561778696542,-11.4039047169397,123.766682270914)) ;
#57778=CARTESIAN_POINT('Ctrl Pts',(-20.9045834153395,-11.5937219986373,
123.60293017781)) ;
#57779=CARTESIAN_POINT('Ctrl Pts',(-20.6055180794411,-11.4137329182744,
123.5647134447)) ;
#57780=CARTESIAN_POINT('Ctrl Pts',(-20.9149654649752,-11.6037985712354,
123.338386769837)) ;
#57781=CARTESIAN_POINT('Ctrl Pts',(-20.6138247398722,-11.4238094908725,
123.353078412637)) ;
#57782=CARTESIAN_POINT('Ctrl Pts',(-20.8801663077808,-11.6136506512429,
123.081776137432)) ;
#57783=CARTESIAN_POINT('Ctrl Pts',(-20.5859865727851,-11.43366157088,123.147790745259)) ;
#57784=CARTESIAN_POINT('Ctrl Pts',(-20.7998144512249,-11.623723936247,122.829596800206)) ;
#57785=CARTESIAN_POINT('Ctrl Pts',(-20.5217060262302,-11.4437348558841,
122.946046639568)) ;
#57786=CARTESIAN_POINT('Ctrl Pts',(-20.6796373590905,-11.6335652879575,
122.60057140377)) ;
#57787=CARTESIAN_POINT('Ctrl Pts',(-20.4255657854105,-11.4535762075946,
122.762826748449)) ;
#57788=CARTESIAN_POINT('Ctrl Pts',(-20.5203770951846,-11.643526787354,122.39283222261)) ;
#57789=CARTESIAN_POINT('Ctrl Pts',(-20.2981587895807,-11.4635377069911,
122.59663487523)) ;
#57790=CARTESIAN_POINT('Ctrl Pts',(-20.3256964580967,-11.653562563484,122.21490632929)) ;
#57791=CARTESIAN_POINT('Ctrl Pts',(-20.1424150134632,-11.4735734831211,
122.454293226116)) ;
#57792=CARTESIAN_POINT('Ctrl Pts',(-20.1065035192901,-11.6634509901216,
122.07533899432)) ;
#57793=CARTESIAN_POINT('Ctrl Pts',(-19.9670619537043,-11.4834619097587,
122.34263870474)) ;
#57794=CARTESIAN_POINT('Ctrl Pts',(-19.8635046295888,-11.6734663121965,
121.974209274979)) ;
#57795=CARTESIAN_POINT('Ctrl Pts',(-19.7726633636097,-11.4934772318336,
122.261733686333)) ;
#57796=CARTESIAN_POINT('Ctrl Pts',(-19.6061275734712,-11.6834966610967,
121.917323321599)) ;
#57797=CARTESIAN_POINT('Ctrl Pts',(-19.5667619143694,-11.5035075807338,
122.216223718493)) ;
#57798=CARTESIAN_POINT('Ctrl Pts',(-19.3477206075241,-11.6933400367034,
121.905682077823)) ;
#57799=CARTESIAN_POINT('Ctrl Pts',(-19.3600373704475,-11.5133509563405,
122.206909440148)) ;
#57800=CARTESIAN_POINT('Ctrl Pts',(-19.0862848802727,-11.7033694736005,
121.939135039902)) ;
#57801=CARTESIAN_POINT('Ctrl Pts',(-19.1508885485966,-11.5233803932376,
122.233670378294)) ;
#57802=CARTESIAN_POINT('Ctrl Pts',(-18.834778258423,-11.7134013515334,122.018183059179)) ;
#57803=CARTESIAN_POINT('Ctrl Pts',(-18.9496827948867,-11.5334122711706,
122.296907572202)) ;
#57804=CARTESIAN_POINT('Ctrl Pts',(-18.6053133475109,-11.7232309746389,
122.136772150957)) ;
#57805=CARTESIAN_POINT('Ctrl Pts',(-18.7661111198526,-11.543241894276,122.391777125529)) ;
#57806=CARTESIAN_POINT('Ctrl Pts',(-18.3960907645237,-11.733220445792,122.295336373572)) ;
#57807=CARTESIAN_POINT('Ctrl Pts',(-18.5987322188273,-11.5532313654291,
122.518627168111)) ;
#57808=CARTESIAN_POINT('Ctrl Pts',(-18.2171052463347,-11.7432642945544,
122.489315908043)) ;
#57809=CARTESIAN_POINT('Ctrl Pts',(-18.4555426693397,-11.5632752141915,
122.673809908671)) ;
#57810=CARTESIAN_POINT('Ctrl Pts',(-18.0772224088806,-11.7530860000861,
122.706227559913)) ;
#57811=CARTESIAN_POINT('Ctrl Pts',(-18.3436356441143,-11.5730969197232,
122.847337557249)) ;
#57812=CARTESIAN_POINT('Ctrl Pts',(-17.974358275623,-11.7631210399139,122.949047320032)) ;
#57813=CARTESIAN_POINT('Ctrl Pts',(-18.2613427735164,-11.583131959551,123.041592794472)) ;
#57814=CARTESIAN_POINT('Ctrl Pts',(-17.9159869176276,-11.7731457468054,
123.205947428722)) ;
#57815=CARTESIAN_POINT('Ctrl Pts',(-18.2146441954026,-11.5931566664425,
123.247112562016)) ;
#57816=CARTESIAN_POINT('Ctrl Pts',(-17.9027824760765,-11.7829984511461,
123.464529062484)) ;
#57817=CARTESIAN_POINT('Ctrl Pts',(-18.2040790568452,-11.6030093707832,
123.453976982937)) ;
#57818=CARTESIAN_POINT('Ctrl Pts',(-17.9346582755181,-11.7929865733538,
123.72504475189)) ;
#57819=CARTESIAN_POINT('Ctrl Pts',(-18.2295779793896,-11.6129974929909,
123.662389596345)) ;
#57820=CARTESIAN_POINT('Ctrl Pts',(-18.0108208430666,-11.8029150434611,
123.974597684985)) ;
#57821=CARTESIAN_POINT('Ctrl Pts',(-18.290506276576,-11.6229259630982,123.862032045727)) ;
#57822=CARTESIAN_POINT('Ctrl Pts',(-18.129492517191,-11.8129040206283,124.20875545915)) ;
#57823=CARTESIAN_POINT('Ctrl Pts',(-18.3854419582014,-11.6329149402654,
124.049358946099)) ;
#57824=CARTESIAN_POINT('Ctrl Pts',(-18.2881378411285,-11.822941827908,124.419490767607)) ;
#57825=CARTESIAN_POINT('Ctrl Pts',(-18.5123568914905,-11.6429527475451,
124.217948275703)) ;
#57826=CARTESIAN_POINT('Ctrl Pts',(-18.4770035096972,-11.8327881287713,
124.596360779214)) ;
#57827=CARTESIAN_POINT('Ctrl Pts',(-18.6634476664908,-11.6527990484084,
124.359445074232)) ;
#57828=CARTESIAN_POINT('Ctrl Pts',(-18.6973386411338,-11.8428138721506,
124.740820127041)) ;
#57829=CARTESIAN_POINT('Ctrl Pts',(-18.8397147708248,-11.6628247917877,
124.47501413786)) ;
#57830=CARTESIAN_POINT('Ctrl Pts',(-18.9398076657194,-11.8528447385896,
124.844250930531)) ;
#57831=CARTESIAN_POINT('Ctrl Pts',(-19.0336893273778,-11.6728556582267,
124.557760414888)) ;
#57832=CARTESIAN_POINT('Ctrl Pts',(-19.1914647637144,-11.8626820973884,
124.903358127309)) ;
#57833=CARTESIAN_POINT('Ctrl Pts',(-19.2350138511474,-11.6826930170255,
124.605047798239)) ;
#57834=CARTESIAN_POINT('Ctrl Pts',(-19.4535879451844,-11.8726740583222,
124.918802859843)) ;
#57835=CARTESIAN_POINT('Ctrl Pts',(-19.4447121787566,-11.6926849779593,
124.617405527106)) ;
#57836=CARTESIAN_POINT('Ctrl Pts',(-19.7154151681285,-11.8827064208787,
124.887849956679)) ;
#57837=CARTESIAN_POINT('Ctrl Pts',(-19.6541742063547,-11.7027173405158,
124.592645060716)) ;
#57838=CARTESIAN_POINT('Ctrl Pts',(-19.9637513981786,-11.8925715814531,
124.813477415096)) ;
#57839=CARTESIAN_POINT('Ctrl Pts',(-19.8528431830511,-11.7125825010902,
124.533149033972)) ;
#57840=CARTESIAN_POINT('Ctrl Pts',(-20.1980246864583,-11.9025334860308,
124.696630723348)) ;
#57841=CARTESIAN_POINT('Ctrl Pts',(-20.0402625347496,-11.7225444056679,
124.439673577518)) ;
#57842=CARTESIAN_POINT('Ctrl Pts',(-20.4097188088187,-11.9125684161065,
124.539405883131)) ;
#57843=CARTESIAN_POINT('Ctrl Pts',(-20.2096190243359,-11.7325793357437,
124.313895264542)) ;
#57844=CARTESIAN_POINT('Ctrl Pts',(-20.5885436050965,-11.9224533629601,
124.350939834724)) ;
#57845=CARTESIAN_POINT('Ctrl Pts',(-20.3526800140608,-11.7424642825973,
124.163124141174)) ;
#57846=CARTESIAN_POINT('Ctrl Pts',(-20.7344544461953,-11.9325190392716,
124.130360829596)) ;
#57847=CARTESIAN_POINT('Ctrl Pts',(-20.4694104306545,-11.7525299589087,
123.986661948345)) ;
#57848=CARTESIAN_POINT('Ctrl Pts',(-20.8377538535721,-11.9423579589065,
123.89328858742)) ;
#57849=CARTESIAN_POINT('Ctrl Pts',(-20.5520516016734,-11.7623688785436,
123.797005487303)) ;
#57850=CARTESIAN_POINT('Ctrl Pts',(-20.9000168313516,-11.9524214686409,
123.636302931589)) ;
#57851=CARTESIAN_POINT('Ctrl Pts',(-20.6018640323336,-11.7724323882781,
123.591417349548)) ;
#57852=CARTESIAN_POINT('Ctrl Pts',(-20.9162207081352,-11.9623150818027,
123.376783859036)) ;
#57853=CARTESIAN_POINT('Ctrl Pts',(-20.6148291614224,-11.7823260014398,
123.383802596767)) ;
#57854=CARTESIAN_POINT('Ctrl Pts',(-20.8876645643203,-11.9722590886161,
123.117066234101)) ;
#57855=CARTESIAN_POINT('Ctrl Pts',(-20.5919863882844,-11.7922700082532,
123.176028481019)) ;
#57856=CARTESIAN_POINT('Ctrl Pts',(-20.8141243155986,-11.9822600429704,
122.8647086418)) ;
#57857=CARTESIAN_POINT('Ctrl Pts',(-20.5331562591136,-11.8022709626075,
122.974141872013)) ;
#57858=CARTESIAN_POINT('Ctrl Pts',(-20.6970504996991,-11.9922988006627,
122.628327621003)) ;
#57859=CARTESIAN_POINT('Ctrl Pts',(-20.4394990793776,-11.8123097202998,
122.78503611631)) ;
#57860=CARTESIAN_POINT('Ctrl Pts',(-20.5444825751892,-12.0021229848327,
122.420035361004)) ;
#57861=CARTESIAN_POINT('Ctrl Pts',(-20.3174467467038,-11.8221339044698,
122.618401417283)) ;
#57862=CARTESIAN_POINT('Ctrl Pts',(-20.3539293395536,-12.0121810504321,
122.236896566325)) ;
#57863=CARTESIAN_POINT('Ctrl Pts',(-20.1650056265507,-11.8321919700692,
122.471888771544)) ;
#57864=CARTESIAN_POINT('Ctrl Pts',(-20.1370409747147,-12.0221110972068,
122.091764368012)) ;
#57865=CARTESIAN_POINT('Ctrl Pts',(-19.9914963147766,-11.8421220168439,
122.355781349936)) ;
#57866=CARTESIAN_POINT('Ctrl Pts',(-19.8980237231667,-12.0320625395439,
121.985643564698)) ;
#57867=CARTESIAN_POINT('Ctrl Pts',(-19.8002835442428,-11.8520734591811,
122.270882756195)) ;
#57868=CARTESIAN_POINT('Ctrl Pts',(-19.6416983085707,-12.0421093367232,
121.922384338977)) ;
#57869=CARTESIAN_POINT('Ctrl Pts',(-19.5952237285874,-11.8621202563603,
122.220273262082)) ;
#57870=CARTESIAN_POINT('Ctrl Pts',(-19.3835093232675,-12.0519572774033,
121.904703348343)) ;
#57871=CARTESIAN_POINT('Ctrl Pts',(-19.3886730067727,-11.8719681970404,
122.206126303218)) ;
#57872=CARTESIAN_POINT('Ctrl Pts',(-19.1231275997313,-12.0619189087459,
121.931627958287)) ;
#57873=CARTESIAN_POINT('Ctrl Pts',(-19.1803674964563,-11.881929828383,122.227663754114)) ;
#57874=CARTESIAN_POINT('Ctrl Pts',(-18.8697470442625,-12.0719475681218,
122.004163670847)) ;
#57875=CARTESIAN_POINT('Ctrl Pts',(-18.9776624753786,-11.8919584877589,
122.28569018209)) ;
#57876=CARTESIAN_POINT('Ctrl Pts',(-18.6355935850335,-12.08185787101,122.118142693142)) ;
#57877=CARTESIAN_POINT('Ctrl Pts',(-18.7903388847647,-11.9018687906471,
122.376871325098)) ;
#57878=CARTESIAN_POINT('Ctrl Pts',(-18.4238474019827,-12.0917927655722,
122.270883953054)) ;
#57879=CARTESIAN_POINT('Ctrl Pts',(-18.6209407077585,-11.9118036852093,
122.49906244756)) ;
#57880=CARTESIAN_POINT('Ctrl Pts',(-18.2400799717895,-12.1018338642391,
122.460231143199)) ;
#57881=CARTESIAN_POINT('Ctrl Pts',(-18.4739251815215,-11.9218447838762,
122.650538612055)) ;
#57882=CARTESIAN_POINT('Ctrl Pts',(-18.0940875093298,-12.1117211467435,
122.675182672206)) ;
#57883=CARTESIAN_POINT('Ctrl Pts',(-18.3571294254557,-11.9317320663806,
122.822498468009)) ;
#57884=CARTESIAN_POINT('Ctrl Pts',(-17.9861176823212,-12.121712887254,122.914511116819)) ;
#57885=CARTESIAN_POINT('Ctrl Pts',(-18.2707515313325,-11.9417238068911,
123.013960245955)) ;
#57886=CARTESIAN_POINT('Ctrl Pts',(-17.921689729601,-12.1316634364894,123.16795292873)) ;
#57887=CARTESIAN_POINT('Ctrl Pts',(-18.2192070041483,-11.9516743561265,
123.216713069332)) ;
#57888=CARTESIAN_POINT('Ctrl Pts',(-17.9018892648507,-12.1415991141242,
123.428284203218)) ;
#57889=CARTESIAN_POINT('Ctrl Pts',(-18.203364387403,-11.9616100337613,123.424977867107)) ;
#57890=CARTESIAN_POINT('Ctrl Pts',(-17.9274444398076,-12.151584531917,123.689463440879)) ;
#57891=CARTESIAN_POINT('Ctrl Pts',(-18.2238062820509,-11.9715954515541,
123.633921427947)) ;
#57892=CARTESIAN_POINT('Ctrl Pts',(-17.9985764205707,-12.1616133247875,
123.943226816736)) ;
#57893=CARTESIAN_POINT('Ctrl Pts',(-18.2807096769127,-11.9816242444246,
123.836932670854)) ;
#57894=CARTESIAN_POINT('Ctrl Pts',(-18.1107411250608,-12.1714928360155,
124.177366527378)) ;
#57895=CARTESIAN_POINT('Ctrl Pts',(-18.3704394042732,-11.9915037556526,
124.024245403531)) ;
#57896=CARTESIAN_POINT('Ctrl Pts',(-18.263117466536,-12.1814863726884,124.391272663474)) ;
#57897=CARTESIAN_POINT('Ctrl Pts',(-18.4923386313118,-12.0014972923255,
124.195371583237)) ;
#57898=CARTESIAN_POINT('Ctrl Pts',(-18.4514152853576,-12.1915186409522,
124.575779592005)) ;
#57899=CARTESIAN_POINT('Ctrl Pts',(-18.6429752478029,-12.0115295605894,
124.342978676221)) ;
#57900=CARTESIAN_POINT('Ctrl Pts',(-18.6649582254987,-12.2013826029581,
124.722768521293)) ;
#57901=CARTESIAN_POINT('Ctrl Pts',(-18.813808386405,-12.0213935225952,124.460571699597)) ;
#57902=CARTESIAN_POINT('Ctrl Pts',(-18.9056381213548,-12.211452664303,124.832713751572)) ;
#57903=CARTESIAN_POINT('Ctrl Pts',(-19.0063512619196,-12.0314635839401,
124.548529868389)) ;
#57904=CARTESIAN_POINT('Ctrl Pts',(-19.1560012005742,-12.2212950286517,
124.897694900574)) ;
#57905=CARTESIAN_POINT('Ctrl Pts',(-19.2066412928752,-12.0413059482889,
124.600516988053)) ;
#57906=CARTESIAN_POINT('Ctrl Pts',(-19.4168488001017,-12.2312557011542,
124.919426126704)) ;
#57907=CARTESIAN_POINT('Ctrl Pts',(-19.4153192326186,-12.0512666207913,
124.617904150398)) ;
#57908=CARTESIAN_POINT('Ctrl Pts',(-19.6794781670334,-12.241293772222,124.894826056415)) ;
#57909=CARTESIAN_POINT('Ctrl Pts',(-19.6254228033852,-12.0613046918591,
124.598226319022)) ;
#57910=CARTESIAN_POINT('Ctrl Pts',(-19.9298584470305,-12.2511673871824,
124.826609084731)) ;
#57911=CARTESIAN_POINT('Ctrl Pts',(-19.82572781557,-12.0711783068196,124.543654773306)) ;
#57912=CARTESIAN_POINT('Ctrl Pts',(-20.1692027685541,-12.2612396217637,
124.713703674863)) ;
#57913=CARTESIAN_POINT('Ctrl Pts',(-20.0172039403952,-12.0812505414008,
124.45333259084)) ;
#57914=CARTESIAN_POINT('Ctrl Pts',(-20.3802336084559,-12.2710636402125,
124.56490174156)) ;
#57915=CARTESIAN_POINT('Ctrl Pts',(-20.1860304834579,-12.0910745598496,
124.334292311524)) ;
#57916=CARTESIAN_POINT('Ctrl Pts',(-20.5668505339034,-12.2811285611885,
124.3775468474)) ;
#57917=CARTESIAN_POINT('Ctrl Pts',(-20.3353241585353,-12.1011394808256,
124.184411132778)) ;
#57918=CARTESIAN_POINT('Ctrl Pts',(-20.7654710388387,-12.2943388594833,
124.092731380698)) ;
#57919=CARTESIAN_POINT('Ctrl Pts',(-20.4942292379436,-12.1143497791204,
123.9565547192)) ;
#57920=CARTESIAN_POINT('Ctrl Pts',(-20.8864681734945,-12.3076543062152,
123.760293059331)) ;
#57921=CARTESIAN_POINT('Ctrl Pts',(-20.5910323501045,-12.1276652258523,
123.690569694297)) ;
#57922=CARTESIAN_POINT('Ctrl Pts',(-20.9168412402485,-12.3209445514825,
123.412248798329)) ;
#57923=CARTESIAN_POINT('Ctrl Pts',(-20.6153241110925,-12.1409554711196,
123.412181858016)) ;
#57924=CARTESIAN_POINT('Ctrl Pts',(-20.8936136564304,-12.3309953010896,
123.149204261583)) ;
#57925=CARTESIAN_POINT('Ctrl Pts',(-20.5967459980804,-12.1510062207267,
123.20173670269)) ;
#57926=CARTESIAN_POINT('Ctrl Pts',(-20.8271599100472,-12.3408079080718,
122.900008574106)) ;
#57927=CARTESIAN_POINT('Ctrl Pts',(-20.5435845615401,-12.160818827709,123.002381693859)) ;
#57928=CARTESIAN_POINT('Ctrl Pts',(-20.7159339872492,-12.3508790060661,
122.659895486434)) ;
#57929=CARTESIAN_POINT('Ctrl Pts',(-20.4546048866285,-12.1708899257032,
122.810289464688)) ;
#57930=CARTESIAN_POINT('Ctrl Pts',(-20.5671825471141,-12.360768578841,122.446765213332)) ;
#57931=CARTESIAN_POINT('Ctrl Pts',(-20.3356088789073,-12.1807794984781,
122.639785845869)) ;
#57932=CARTESIAN_POINT('Ctrl Pts',(-20.3217335957846,-12.3740386856443,
122.199036770175)) ;
#57933=CARTESIAN_POINT('Ctrl Pts',(-20.1392327070889,-12.1940496052814,
122.441591581826)) ;
#57934=CARTESIAN_POINT('Ctrl Pts',(-19.9402799223287,-12.3906553725668,
121.976489963183)) ;
#57935=CARTESIAN_POINT('Ctrl Pts',(-19.8341061887492,-12.2106662922039,
122.263562894215)) ;
#57936=CARTESIAN_POINT('Ctrl Pts',(-19.5069560654083,-12.407229415883,121.897341845887)) ;
#57937=CARTESIAN_POINT('Ctrl Pts',(-19.4873858330109,-12.2272403355201,
122.200234744545)) ;
#57938=CARTESIAN_POINT('Ctrl Pts',(-19.1586250796142,-12.4205259833148,
121.925240968701)) ;
#57939=CARTESIAN_POINT('Ctrl Pts',(-19.2087707820573,-12.2405369029519,
122.222555129474)) ;
#57940=CARTESIAN_POINT('Ctrl Pts',(-18.9035497915594,-12.4305560468922,
121.991664800906)) ;
#57941=CARTESIAN_POINT('Ctrl Pts',(-19.0046999503751,-12.2505669665293,
122.275692101065)) ;
#57942=CARTESIAN_POINT('Ctrl Pts',(-18.6671468529052,-12.4404499387414,
122.099840645972)) ;
#57943=CARTESIAN_POINT('Ctrl Pts',(-18.8155801630729,-12.2604608583786,
122.362230133135)) ;
#57944=CARTESIAN_POINT('Ctrl Pts',(-18.3796682061191,-12.453702694527,122.296549637466)) ;
#57945=CARTESIAN_POINT('Ctrl Pts',(-18.5855889437377,-12.2737136141641,
122.519603145883)) ;
#57946=CARTESIAN_POINT('Ctrl Pts',(-18.0908280313655,-12.4704307995194,
122.634462100718)) ;
#57947=CARTESIAN_POINT('Ctrl Pts',(-18.3545219823308,-12.2904417191566,
122.789922698833)) ;
#57948=CARTESIAN_POINT('Ctrl Pts',(-17.9056069777788,-12.4902616359979,
123.128014485523)) ;
#57949=CARTESIAN_POINT('Ctrl Pts',(-18.2063394436304,-12.3102725556351,
123.184767136768)) ;
#57950=CARTESIAN_POINT('Ctrl Pts',(-17.8986058474029,-12.5101870278881,
123.65743523967)) ;
#57951=CARTESIAN_POINT('Ctrl Pts',(-18.2007363231524,-12.3301979475252,
123.608303576448)) ;
#57952=CARTESIAN_POINT('Ctrl Pts',(-18.0728134812496,-12.5301122412401,
124.157630024429)) ;
#57953=CARTESIAN_POINT('Ctrl Pts',(-18.3400999156776,-12.3501231608772,
124.00846101179)) ;
#57954=CARTESIAN_POINT('Ctrl Pts',(-18.4070561283902,-12.5500372547252,
124.568319257347)) ;
#57955=CARTESIAN_POINT('Ctrl Pts',(-18.6074925126866,-12.3700481743623,
124.337014427016)) ;
#57956=CARTESIAN_POINT('Ctrl Pts',(-18.8599799731256,-12.5699137264252,
124.840308096966)) ;
#57957=CARTESIAN_POINT('Ctrl Pts',(-18.9698314340081,-12.3899246460623,
124.554607919997)) ;
#57958=CARTESIAN_POINT('Ctrl Pts',(-19.3811313633293,-12.5898930443341,
124.942158139695)) ;
#57959=CARTESIAN_POINT('Ctrl Pts',(-19.3867523851537,-12.4099039639712,
124.636089848104)) ;
#57960=CARTESIAN_POINT('Ctrl Pts',(-19.9045262603243,-12.6098260479101,
124.859844414469)) ;
#57961=CARTESIAN_POINT('Ctrl Pts',(-19.8054692095567,-12.4298369675472,
124.570240637955)) ;
#57962=CARTESIAN_POINT('Ctrl Pts',(-20.3677432424192,-12.6297213179378,
124.6048789893)) ;
#57963=CARTESIAN_POINT('Ctrl Pts',(-20.1760444928505,-12.4497322375749,
124.366269105617)) ;
#57964=CARTESIAN_POINT('Ctrl Pts',(-20.7170498595964,-12.6496426558436,
124.206944794287)) ;
#57965=CARTESIAN_POINT('Ctrl Pts',(-20.4554911883008,-12.4696535754807,
124.047921837557)) ;
#57966=CARTESIAN_POINT('Ctrl Pts',(-20.9098403565593,-12.6696002791098,
123.712751204342)) ;
#57967=CARTESIAN_POINT('Ctrl Pts',(-20.6097246738742,-12.4896111987469,
123.652566906432)) ;
#57968=CARTESIAN_POINT('Ctrl Pts',(-20.922485985003,-12.689480111067,123.18461209717)) ;
#57969=CARTESIAN_POINT('Ctrl Pts',(-20.6198419805455,-12.5094910307041,
123.230054122359)) ;
#57970=CARTESIAN_POINT('Ctrl Pts',(-20.7554545445051,-12.7093619623639,
122.683172172836)) ;
#57971=CARTESIAN_POINT('Ctrl Pts',(-20.4862161995466,-12.529372882001,122.828900805559)) ;
#57972=CARTESIAN_POINT('Ctrl Pts',(-20.4235254244291,-12.7294329794677,
122.265649141046)) ;
#57973=CARTESIAN_POINT('Ctrl Pts',(-20.2206735911977,-12.5494438991048,
122.494883034392)) ;
#57974=CARTESIAN_POINT('Ctrl Pts',(-19.9749237655201,-12.7492402032208,
121.989968961482)) ;
#57975=CARTESIAN_POINT('Ctrl Pts',(-19.8617900839095,-12.5692511228579,
122.274337697005)) ;
#57976=CARTESIAN_POINT('Ctrl Pts',(-19.4550399386783,-12.7692213387896,
121.881799009553)) ;
#57977=CARTESIAN_POINT('Ctrl Pts',(-19.4458826423283,-12.5892322584267,
122.18780260183)) ;
#57978=CARTESIAN_POINT('Ctrl Pts',(-18.9310095255676,-12.7891488321288,
121.958350587305)) ;
#57979=CARTESIAN_POINT('Ctrl Pts',(-19.0266575304228,-12.6091597517659,
122.24904461452)) ;
#57980=CARTESIAN_POINT('Ctrl Pts',(-18.4660378435683,-12.8089694934866,
122.206286369213)) ;
#57981=CARTESIAN_POINT('Ctrl Pts',(-18.6546792788745,-12.6289804131237,
122.447395528075)) ;
#57982=CARTESIAN_POINT('Ctrl Pts',(-18.1095237058468,-12.8290666827084,
122.603786127405)) ;
#57983=CARTESIAN_POINT('Ctrl Pts',(-18.3694696834846,-12.6490776023455,
122.765395547961)) ;
#57984=CARTESIAN_POINT('Ctrl Pts',(-17.9128685242105,-12.8488303617167,
123.091145395877)) ;
#57985=CARTESIAN_POINT('Ctrl Pts',(-18.212146236786,-12.6688412813539,123.155285756016)) ;
#57986=CARTESIAN_POINT('Ctrl Pts',(-17.8934532250118,-12.8688876403898,
123.623648070234)) ;
#57987=CARTESIAN_POINT('Ctrl Pts',(-18.1966161448372,-12.6888985600269,
123.581287459871)) ;
#57988=CARTESIAN_POINT('Ctrl Pts',(-18.0551868058746,-12.8886830641372,
124.124451004221)) ;
#57989=CARTESIAN_POINT('Ctrl Pts',(-18.3260055893083,-12.7086939837743,
123.981930874229)) ;
#57990=CARTESIAN_POINT('Ctrl Pts',(-18.3794288064129,-12.9086467088648,
124.544379679826)) ;
#57991=CARTESIAN_POINT('Ctrl Pts',(-18.5854015952883,-12.7286576285019,
124.317872293328)) ;
#57992=CARTESIAN_POINT('Ctrl Pts',(-18.8287006511552,-12.9286302001389,
124.827680379695)) ;
#57993=CARTESIAN_POINT('Ctrl Pts',(-18.9448205353017,-12.748641119776,124.544510768176)) ;
#57994=CARTESIAN_POINT('Ctrl Pts',(-19.3429186866301,-12.9484376952882,
124.94073161998)) ;
#57995=CARTESIAN_POINT('Ctrl Pts',(-19.3561969576373,-12.7684486149253,
124.634949144309)) ;
#57996=CARTESIAN_POINT('Ctrl Pts',(-19.8693844497185,-12.9684202860083,
124.871533418394)) ;
#57997=CARTESIAN_POINT('Ctrl Pts',(-19.7773692207012,-12.7884312056454,
124.579587326227)) ;
#57998=CARTESIAN_POINT('Ctrl Pts',(-20.3384447754671,-12.9883029399995,
124.627871581349)) ;
#57999=CARTESIAN_POINT('Ctrl Pts',(-20.1526165530644,-12.8083138596367,
124.384654591439)) ;
#58000=CARTESIAN_POINT('Ctrl Pts',(-20.6976976848122,-13.0082611848626,
124.237731507644)) ;
#58001=CARTESIAN_POINT('Ctrl Pts',(-20.4400164509615,-12.8282721044997,
124.072539967842)) ;
#58002=CARTESIAN_POINT('Ctrl Pts',(-20.9017768869257,-13.0281367719042,
123.750397269444)) ;
#58003=CARTESIAN_POINT('Ctrl Pts',(-20.6032766081325,-12.8481476915413,
123.682670590867)) ;
#58004=CARTESIAN_POINT('Ctrl Pts',(-20.9278087943981,-13.0481176600395,
123.220011471926)) ;
#58005=CARTESIAN_POINT('Ctrl Pts',(-20.6240984650254,-12.8681285796766,
123.258361753543)) ;
#58006=CARTESIAN_POINT('Ctrl Pts',(-20.7712144053819,-13.0680528011505,
122.713763278227)) ;
#58007=CARTESIAN_POINT('Ctrl Pts',(-20.4988186174616,-12.8880637207876,
122.853363994619)) ;
#58008=CARTESIAN_POINT('Ctrl Pts',(-20.4520106816014,-13.0879648191615,
122.291696114272)) ;
#58009=CARTESIAN_POINT('Ctrl Pts',(-20.2434545045575,-12.9079757387987,
122.515712746724)) ;
#58010=CARTESIAN_POINT('Ctrl Pts',(-20.0087285877316,-13.1078530374051,
122.003722192709)) ;
#58011=CARTESIAN_POINT('Ctrl Pts',(-19.8888179313836,-12.9278639570422,
122.285335578687)) ;
#58012=CARTESIAN_POINT('Ctrl Pts',(-19.5791090604564,-13.124451341252,121.903703056221)) ;
#58013=CARTESIAN_POINT('Ctrl Pts',(-19.5451473403849,-12.9444622608891,
122.20532771232)) ;
#58014=CARTESIAN_POINT('Ctrl Pts',(-19.2304680801455,-13.1377239311548,
121.914976366624)) ;
#58015=CARTESIAN_POINT('Ctrl Pts',(-19.2662110826215,-12.957734850792,122.214345972793)) ;
#58016=CARTESIAN_POINT('Ctrl Pts',(-18.9730360739325,-13.1477313461057,
121.968723010403)) ;
#58017=CARTESIAN_POINT('Ctrl Pts',(-19.0602727214037,-12.9677422657428,
122.25734421058)) ;
#58018=CARTESIAN_POINT('Ctrl Pts',(-18.7289237747832,-13.1577386928383,
122.066570256317)) ;
#58019=CARTESIAN_POINT('Ctrl Pts',(-18.8649743141328,-12.9777496124754,
122.335631001214)) ;
#58020=CARTESIAN_POINT('Ctrl Pts',(-18.4326373531694,-13.1710050526399,
122.250316913842)) ;
#58021=CARTESIAN_POINT('Ctrl Pts',(-18.6279877739114,-12.991015972277,122.482594753417)) ;
#58022=CARTESIAN_POINT('Ctrl Pts',(-18.1316373287835,-13.1875197102629,
122.569692622284)) ;
#58023=CARTESIAN_POINT('Ctrl Pts',(-18.3871406493088,-13.0075306299,122.738147077933)) ;
#58024=CARTESIAN_POINT('Ctrl Pts',(-17.9558681007045,-13.2041171435055,
122.974265631492)) ;
#58025=CARTESIAN_POINT('Ctrl Pts',(-18.2465546550527,-13.0241280631426,
123.061762709622)) ;
#58026=CARTESIAN_POINT('Ctrl Pts',(-17.9045373896821,-13.2174651406505,
123.321302564893)) ;
#58027=CARTESIAN_POINT('Ctrl Pts',(-18.20548016203,-13.0374760602876,123.339423056025)) ;
#58028=CARTESIAN_POINT('Ctrl Pts',(-17.9113737957956,-13.2273608950021,
123.581262925382)) ;
#58029=CARTESIAN_POINT('Ctrl Pts',(-18.2109541050246,-13.0473718146392,
123.547385244145)) ;
#58030=CARTESIAN_POINT('Ctrl Pts',(-17.9634088821012,-13.2373488489335,
123.838506352538)) ;
#58031=CARTESIAN_POINT('Ctrl Pts',(-18.2525836755494,-13.0573597685706,
123.753181135679)) ;
#58032=CARTESIAN_POINT('Ctrl Pts',(-18.0589349739684,-13.2473060726382,
124.082144873651)) ;
#58033=CARTESIAN_POINT('Ctrl Pts',(-18.3290068212281,-13.0673169922753,
123.948090676495)) ;
#58034=CARTESIAN_POINT('Ctrl Pts',(-18.1964661586106,-13.2573416191949,
124.307146372465)) ;
#58035=CARTESIAN_POINT('Ctrl Pts',(-18.4390335973166,-13.077352538832,124.128090758229)) ;
#58036=CARTESIAN_POINT('Ctrl Pts',(-18.3682700533626,-13.267228730471,124.502082982706)) ;
#58037=CARTESIAN_POINT('Ctrl Pts',(-18.576478424902,-13.0872396501081,124.284038539208)) ;
#58038=CARTESIAN_POINT('Ctrl Pts',(-18.573168600081,-13.2772201355718,124.666246335832)) ;
#58039=CARTESIAN_POINT('Ctrl Pts',(-18.7403986257916,-13.0972310552089,
124.415367430382)) ;
#58040=CARTESIAN_POINT('Ctrl Pts',(-18.8024527486924,-13.2871657567866,
124.791696662128)) ;
#58041=CARTESIAN_POINT('Ctrl Pts',(-18.9238269941468,-13.1071766764237,
124.515725689855)) ;
#58042=CARTESIAN_POINT('Ctrl Pts',(-19.0499707909462,-13.2971150050549,
124.87596822317)) ;
#58043=CARTESIAN_POINT('Ctrl Pts',(-19.1218420945713,-13.117125924692,124.58314078008)) ;
#58044=CARTESIAN_POINT('Ctrl Pts',(-19.3109074952385,-13.3071615002235,
124.91606420447)) ;
#58045=CARTESIAN_POINT('Ctrl Pts',(-19.3305917563602,-13.1271724198607,
124.615215324585)) ;
#58046=CARTESIAN_POINT('Ctrl Pts',(-19.5697458477253,-13.3170128430151,
124.910614060128)) ;
#58047=CARTESIAN_POINT('Ctrl Pts',(-19.5376622956873,-13.1370237626522,
124.610852953311)) ;
#58048=CARTESIAN_POINT('Ctrl Pts',(-19.8268961278364,-13.3269846231424,
124.86034740168)) ;
#58049=CARTESIAN_POINT('Ctrl Pts',(-19.7433819968767,-13.1469955427795,
124.570637436565)) ;
#58050=CARTESIAN_POINT('Ctrl Pts',(-20.0720441858723,-13.3369798231201,
124.765921346646)) ;
#58051=CARTESIAN_POINT('Ctrl Pts',(-19.9394995773028,-13.1569907427572,
124.495094521128)) ;
#58052=CARTESIAN_POINT('Ctrl Pts',(-20.2977248332106,-13.3470138148161,
124.629595035348)) ;
#58053=CARTESIAN_POINT('Ctrl Pts',(-20.1200429020722,-13.1670247344533,
124.386031555564)) ;
#58054=CARTESIAN_POINT('Ctrl Pts',(-20.4930785404264,-13.3568692197886,
124.459519571124)) ;
#58055=CARTESIAN_POINT('Ctrl Pts',(-20.2763242533844,-13.1768801394258,
124.2499696171)) ;
#58056=CARTESIAN_POINT('Ctrl Pts',(-20.6585461151986,-13.3668685176344,
124.255447402342)) ;
#58057=CARTESIAN_POINT('Ctrl Pts',(-20.4086965325383,-13.1868794372715,
124.086710531574)) ;
#58058=CARTESIAN_POINT('Ctrl Pts',(-20.7850259763668,-13.3767636302396,
124.028196369691)) ;
#58059=CARTESIAN_POINT('Ctrl Pts',(-20.509878386038,-13.1967745498767,123.904908812571)) ;
#58060=CARTESIAN_POINT('Ctrl Pts',(-20.8714967332555,-13.3868242757746,
123.778389961119)) ;
#58061=CARTESIAN_POINT('Ctrl Pts',(-20.5790529024792,-13.2068351954117,
123.705062936695)) ;
#58062=CARTESIAN_POINT('Ctrl Pts',(-20.9125557494614,-13.3966731527638,
123.522828864941)) ;
#58063=CARTESIAN_POINT('Ctrl Pts',(-20.6118978858686,-13.2166840724009,
123.500614018673)) ;
#58064=CARTESIAN_POINT('Ctrl Pts',(-20.9092102411542,-13.4067018638574,
123.259309807964)) ;
#58065=CARTESIAN_POINT('Ctrl Pts',(-20.60921931471,-13.2267127834945,123.289798833326)) ;
#58066=CARTESIAN_POINT('Ctrl Pts',(-20.8594509750379,-13.4167312651135,
123.00048234628)) ;
#58067=CARTESIAN_POINT('Ctrl Pts',(-20.5694097280133,-13.2367421847506,
123.082737285215)) ;
#58068=CARTESIAN_POINT('Ctrl Pts',(-20.7678172835609,-13.4265714569095,
122.758667592175)) ;
#58069=CARTESIAN_POINT('Ctrl Pts',(-20.4961008807738,-13.2465823765466,
122.889286615854)) ;
#58070=CARTESIAN_POINT('Ctrl Pts',(-20.6338292437046,-13.4365748861025,
122.532528063033)) ;
#58071=CARTESIAN_POINT('Ctrl Pts',(-20.3889086516706,-13.2565858057396,
122.708376145626)) ;
#58072=CARTESIAN_POINT('Ctrl Pts',(-20.4628072717642,-13.4465603985687,
122.333446821148)) ;
#58073=CARTESIAN_POINT('Ctrl Pts',(-20.2520895182278,-13.2665713182058,
122.549112622993)) ;
#58074=CARTESIAN_POINT('Ctrl Pts',(-20.258572195235,-13.4566014949527,122.16640991458)) ;
#58075=CARTESIAN_POINT('Ctrl Pts',(-20.0887000684384,-13.2766124145898,
122.415484760473)) ;
#58076=CARTESIAN_POINT('Ctrl Pts',(-20.0331061121126,-13.4664446909037,
122.03957718795)) ;
#58077=CARTESIAN_POINT('Ctrl Pts',(-19.9083265551085,-13.2864556105408,
122.314020659262)) ;
#58078=CARTESIAN_POINT('Ctrl Pts',(-19.7857320971472,-13.4764310019581,
121.952101012445)) ;
#58079=CARTESIAN_POINT('Ctrl Pts',(-19.7104267699532,-13.2964419215952,
122.2440417256)) ;
#58080=CARTESIAN_POINT('Ctrl Pts',(-19.5282010411868,-13.4863656872158,
121.908939847016)) ;
#58081=CARTESIAN_POINT('Ctrl Pts',(-19.5044018436985,-13.3063766068529,
122.209514865674)) ;
#58082=CARTESIAN_POINT('Ctrl Pts',(-19.2639488168614,-13.4964232484328,
121.911409438826)) ;
#58083=CARTESIAN_POINT('Ctrl Pts',(-19.2929999897462,-13.31643416807,122.211492628297)) ;
#58084=CARTESIAN_POINT('Ctrl Pts',(-19.0100966675528,-13.5062448900414,
121.958214888149)) ;
#58085=CARTESIAN_POINT('Ctrl Pts',(-19.0899192590891,-13.3262558096786,
122.248938879444)) ;
#58086=CARTESIAN_POINT('Ctrl Pts',(-18.7623301682284,-13.5163009536324,
122.050058119956)) ;
#58087=CARTESIAN_POINT('Ctrl Pts',(-18.8917066650352,-13.3363118732695,
122.322415354375)) ;
#58088=CARTESIAN_POINT('Ctrl Pts',(-18.5371012425962,-13.5262416293942,
122.182417857288)) ;
#58089=CARTESIAN_POINT('Ctrl Pts',(-18.7115247897244,-13.3462525490313,
122.428304768289)) ;
#58090=CARTESIAN_POINT('Ctrl Pts',(-18.338478245611,-13.5361459881825,122.350628473911)) ;
#58091=CARTESIAN_POINT('Ctrl Pts',(-18.5526279681694,-13.3561569078197,
122.562874462125)) ;
#58092=CARTESIAN_POINT('Ctrl Pts',(-18.1698329826385,-13.5461926427583,
122.553733855565)) ;
#58093=CARTESIAN_POINT('Ctrl Pts',(-18.4177132105659,-13.3662035623955,
122.725360081205)) ;
#58094=CARTESIAN_POINT('Ctrl Pts',(-18.0407519036657,-13.5560882374012,
122.779526388176)) ;
#58095=CARTESIAN_POINT('Ctrl Pts',(-18.314450248629,-13.3760991570383,122.905994658498)) ;
#58096=CARTESIAN_POINT('Ctrl Pts',(-17.9513576421501,-13.5661501840581,
123.028342279855)) ;
#58097=CARTESIAN_POINT('Ctrl Pts',(-18.2429366010411,-13.3861611036952,
123.105048152778)) ;
#58098=CARTESIAN_POINT('Ctrl Pts',(-17.9074152113575,-13.5759998079902,
123.283436990171)) ;
#58099=CARTESIAN_POINT('Ctrl Pts',(-18.2077846559609,-13.3960107276274,
123.30912358981)) ;
#58100=CARTESIAN_POINT('Ctrl Pts',(-17.9075794490051,-13.5859630470201,
123.545245160118)) ;
#58101=CARTESIAN_POINT('Ctrl Pts',(-18.2079178311045,-13.4059739666572,
123.518569875125)) ;
#58102=CARTESIAN_POINT('Ctrl Pts',(-17.9538438452054,-13.5959876217959,
123.804601716854)) ;
#58103=CARTESIAN_POINT('Ctrl Pts',(-18.2449311618866,-13.415998541433,123.726054822038)) ;
#58104=CARTESIAN_POINT('Ctrl Pts',(-18.0433151854202,-13.6059061844836,
124.0494068293)) ;
#58105=CARTESIAN_POINT('Ctrl Pts',(-18.3165097898856,-13.4259171041207,
123.921897880132)) ;
#58106=CARTESIAN_POINT('Ctrl Pts',(-18.1745142883211,-13.6158983712076,
124.276882942804)) ;
#58107=CARTESIAN_POINT('Ctrl Pts',(-18.4214705117975,-13.4359092908447,
124.103877785203)) ;
#58108=CARTESIAN_POINT('Ctrl Pts',(-18.3442843563806,-13.6259331697918,
124.478655912716)) ;
#58109=CARTESIAN_POINT('Ctrl Pts',(-18.5572880000568,-13.4459440894289,
124.265295042287)) ;
#58110=CARTESIAN_POINT('Ctrl Pts',(-18.5426287178468,-13.6357883604655,
124.645217964009)) ;
#58111=CARTESIAN_POINT('Ctrl Pts',(-18.7159640464026,-13.4557992801026,
124.398542876088)) ;
#58112=CARTESIAN_POINT('Ctrl Pts',(-18.7699291705974,-13.6457877086185,
124.776978497853)) ;
#58113=CARTESIAN_POINT('Ctrl Pts',(-18.8978051604027,-13.4657986282556,
124.503949791851)) ;
#58114=CARTESIAN_POINT('Ctrl Pts',(-19.0140681533579,-13.6556828342936,
124.86662328346)) ;
#58115=CARTESIAN_POINT('Ctrl Pts',(-19.0931163563245,-13.4756937539307,
124.57566388753)) ;
#58116=CARTESIAN_POINT('Ctrl Pts',(-19.2742712713222,-13.6657433772417,
124.913241817981)) ;
#58117=CARTESIAN_POINT('Ctrl Pts',(-19.3012793296211,-13.4857542968788,
124.612957136434)) ;
#58118=CARTESIAN_POINT('Ctrl Pts',(-19.5331191647968,-13.6755926515086,
124.914103544901)) ;
#58119=CARTESIAN_POINT('Ctrl Pts',(-19.5083568152058,-13.4956035711457,
124.613644905364)) ;
#58120=CARTESIAN_POINT('Ctrl Pts',(-19.792878148494,-13.6856198760785,124.869872597639)) ;
#58121=CARTESIAN_POINT('Ctrl Pts',(-19.7161637833577,-13.5056307957156,
124.578258678487)) ;
#58122=CARTESIAN_POINT('Ctrl Pts',(-20.0408282968694,-13.6956482752663,
124.780544744153)) ;
#58123=CARTESIAN_POINT('Ctrl Pts',(-19.9145234061736,-13.5156591949034,
124.506794855646)) ;
#58124=CARTESIAN_POINT('Ctrl Pts',(-20.2655486146661,-13.7054940256798,
124.652339842706)) ;
#58125=CARTESIAN_POINT('Ctrl Pts',(-20.0942981282645,-13.5255049453169,
124.404230053982)) ;
#58126=CARTESIAN_POINT('Ctrl Pts',(-20.4679785318478,-13.7154828160805,
124.485209945321)) ;
#58127=CARTESIAN_POINT('Ctrl Pts',(-20.2562410584806,-13.5354937357177,
124.270525177274)) ;
#58128=CARTESIAN_POINT('Ctrl Pts',(-20.6387470354959,-13.7255277444802,
124.283933112254)) ;
#58129=CARTESIAN_POINT('Ctrl Pts',(-20.3928547958644,-13.5455386641174,
124.109502630356)) ;
#58130=CARTESIAN_POINT('Ctrl Pts',(-20.7695822850911,-13.7353522292692,
124.061344007578)) ;
#58131=CARTESIAN_POINT('Ctrl Pts',(-20.4975212694255,-13.5553631489063,
123.931431547031)) ;
#58132=CARTESIAN_POINT('Ctrl Pts',(-20.8622650301573,-13.7454096268104,
123.813853115559)) ;
#58133=CARTESIAN_POINT('Ctrl Pts',(-20.5716663117887,-13.5654205464475,
123.733438175729)) ;
#58134=CARTESIAN_POINT('Ctrl Pts',(-20.9096073544687,-13.7553357183966,
123.557318498504)) ;
#58135=CARTESIAN_POINT('Ctrl Pts',(-20.6095387227254,-13.5753466380337,
123.528210720789)) ;
#58136=CARTESIAN_POINT('Ctrl Pts',(-20.9123708210729,-13.7652905035412,
123.295734355723)) ;
#58137=CARTESIAN_POINT('Ctrl Pts',(-20.6117482517937,-13.5853014231783,
123.318943754624)) ;
#58138=CARTESIAN_POINT('Ctrl Pts',(-20.8690285856397,-13.7753278731988,
123.035549479101)) ;
#58139=CARTESIAN_POINT('Ctrl Pts',(-20.5770731610732,-13.5953387928359,
123.110795969221)) ;
#58140=CARTESIAN_POINT('Ctrl Pts',(-20.7826546061871,-13.7852166833204,
122.790448432935)) ;
#58141=CARTESIAN_POINT('Ctrl Pts',(-20.5079730348007,-13.6052276029575,
122.914716243319)) ;
#58142=CARTESIAN_POINT('Ctrl Pts',(-20.6541544832906,-13.7952060423715,
122.561546360115)) ;
#58143=CARTESIAN_POINT('Ctrl Pts',(-20.4051720120301,-13.6152169620086,
122.731595301545)) ;
#58144=CARTESIAN_POINT('Ctrl Pts',(-20.4882245281512,-13.8051645898276,
122.359184924028)) ;
#58145=CARTESIAN_POINT('Ctrl Pts',(-20.2724273390847,-13.6251755094647,
122.569707182105)) ;
#58146=CARTESIAN_POINT('Ctrl Pts',(-20.2912542115885,-13.8150641663786,
122.189215690163)) ;
#58147=CARTESIAN_POINT('Ctrl Pts',(-20.1148509292206,-13.6350750860157,
122.433733053993)) ;
#58148=CARTESIAN_POINT('Ctrl Pts',(-20.0644048944981,-13.8251120782093,
122.054135819925)) ;
#58149=CARTESIAN_POINT('Ctrl Pts',(-19.9333707741338,-13.6451229978464,
122.325669994257)) ;
#58150=CARTESIAN_POINT('Ctrl Pts',(-19.8213040212289,-13.8350074260699,
121.961702812424)) ;
#58151=CARTESIAN_POINT('Ctrl Pts',(-19.7388903925254,-13.655018345707,122.251724810852)) ;
#58152=CARTESIAN_POINT('Ctrl Pts',(-19.5616299165928,-13.845069102601,121.912040392459)) ;
#58153=CARTESIAN_POINT('Ctrl Pts',(-19.5311506601532,-13.6650800222382,
122.211995830886)) ;
#58154=CARTESIAN_POINT('Ctrl Pts',(-19.302943765994,-13.8549136203502,121.908260248801)) ;
#58155=CARTESIAN_POINT('Ctrl Pts',(-19.3242027824673,-13.6749245399873,
122.208972745531)) ;
#58156=CARTESIAN_POINT('Ctrl Pts',(-19.0443926106772,-13.864874064065,121.949016797608)) ;
#58157=CARTESIAN_POINT('Ctrl Pts',(-19.1173623421421,-13.6848849837021,
122.241578712485)) ;
#58158=CARTESIAN_POINT('Ctrl Pts',(-18.7951065533296,-13.8749108968832,
122.035163624274)) ;
#58159=CARTESIAN_POINT('Ctrl Pts',(-18.9179336758563,-13.6949218165203,
122.310497076572)) ;
#58160=CARTESIAN_POINT('Ctrl Pts',(-18.5679607592807,-13.88478969363,122.160911880469)) ;
#58161=CARTESIAN_POINT('Ctrl Pts',(-18.7362182015604,-13.7048006132671,
122.411095961693)) ;
#58162=CARTESIAN_POINT('Ctrl Pts',(-18.3623992980865,-13.8948490097584,
122.327074678705)) ;
#58163=CARTESIAN_POINT('Ctrl Pts',(-18.5717693261378,-13.7148599293955,
122.544026976484)) ;
#58164=CARTESIAN_POINT('Ctrl Pts',(-18.1920392191495,-13.9047194565116,
122.522692233472)) ;
#58165=CARTESIAN_POINT('Ctrl Pts',(-18.4354824658003,-13.7247303761487,
122.700520842774)) ;
#58166=CARTESIAN_POINT('Ctrl Pts',(-18.0559754687445,-13.9147120947696,
122.747289602296)) ;
#58167=CARTESIAN_POINT('Ctrl Pts',(-18.3266320713964,-13.7347230144067,
122.880198925302)) ;
#58168=CARTESIAN_POINT('Ctrl Pts',(-17.9611352243635,-13.9247441103175,
122.993260746216)) ;
#58169=CARTESIAN_POINT('Ctrl Pts',(-18.2507605487093,-13.7447550299547,
123.076976202334)) ;
#58170=CARTESIAN_POINT('Ctrl Pts',(-17.9107237978205,-13.9346099666241,
123.247603809028)) ;
#58171=CARTESIAN_POINT('Ctrl Pts',(-18.210432205314,-13.7546208862612,123.280449806178)) ;
#58172=CARTESIAN_POINT('Ctrl Pts',(-17.9051038745564,-13.9446792560932,
123.512124786768)) ;
#58173=CARTESIAN_POINT('Ctrl Pts',(-18.2059368701527,-13.7646901757304,
123.492066934925)) ;
#58174=CARTESIAN_POINT('Ctrl Pts',(-17.9445700338335,-13.9545228136445,
123.767790796992)) ;
#58175=CARTESIAN_POINT('Ctrl Pts',(-18.2375102230327,-13.7745337332817,
123.696598534101)) ;
#58176=CARTESIAN_POINT('Ctrl Pts',(-18.0281629110103,-13.9645029404324,
124.016370584098)) ;
#58177=CARTESIAN_POINT('Ctrl Pts',(-18.3043848156925,-13.7845138600695,
123.895462003248)) ;
#58178=CARTESIAN_POINT('Ctrl Pts',(-18.1545752563571,-13.9745214890323,
124.247305606012)) ;
#58179=CARTESIAN_POINT('Ctrl Pts',(-18.4055151504625,-13.7945324086694,
124.080209779767)) ;
#58180=CARTESIAN_POINT('Ctrl Pts',(-18.3165363213439,-13.9844047895555,
124.450385027953)) ;
#58181=CARTESIAN_POINT('Ctrl Pts',(-18.535083750399,-13.8044157091926,124.242672395031)) ;
#58182=CARTESIAN_POINT('Ctrl Pts',(-18.5149631927261,-13.9944730766036,
124.625337357405)) ;
#58183=CARTESIAN_POINT('Ctrl Pts',(-18.6938257640231,-13.8144839962408,
124.382634169633)) ;
#58184=CARTESIAN_POINT('Ctrl Pts',(-18.7353286473751,-14.0043031996223,
124.760223493667)) ;
#58185=CARTESIAN_POINT('Ctrl Pts',(-18.8701172488312,-13.8243141192594,
124.49054215336)) ;
#58186=CARTESIAN_POINT('Ctrl Pts',(-18.9813430292803,-14.0143697835476,
124.857357794633)) ;
#58187=CARTESIAN_POINT('Ctrl Pts',(-19.0669291407156,-13.8343807031847,
124.568249482507)) ;
#58188=CARTESIAN_POINT('Ctrl Pts',(-19.2360505050157,-14.0242598965621,
124.909235187301)) ;
#58189=CARTESIAN_POINT('Ctrl Pts',(-19.2706943553894,-13.8442708161992,
124.60975094901)) ;
#58190=CARTESIAN_POINT('Ctrl Pts',(-19.4985188781141,-14.0342525853247,
124.916724579482)) ;
#58191=CARTESIAN_POINT('Ctrl Pts',(-19.4806688914999,-13.8542635049618,
124.615742311681)) ;
#58192=CARTESIAN_POINT('Ctrl Pts',(-19.7574815058424,-14.0442134736805,
124.878462065094)) ;
#58193=CARTESIAN_POINT('Ctrl Pts',(-19.6878385846522,-13.8642243933176,
124.585132166976)) ;
#58194=CARTESIAN_POINT('Ctrl Pts',(-20.0049101277491,-14.0541314185605,
124.796606975513)) ;
#58195=CARTESIAN_POINT('Ctrl Pts',(-19.8857808233358,-13.8741423381976,
124.519648232361)) ;
#58196=CARTESIAN_POINT('Ctrl Pts',(-20.2366270328514,-14.0641391716567,
124.672163407092)) ;
#58197=CARTESIAN_POINT('Ctrl Pts',(-20.0711543039772,-13.8841500912938,
124.420093397815)) ;
#58198=CARTESIAN_POINT('Ctrl Pts',(-20.4433359395377,-14.0741702656157,
124.508602153767)) ;
#58199=CARTESIAN_POINT('Ctrl Pts',(-20.2365214217928,-13.8941811852529,
124.289244226254)) ;
#58200=CARTESIAN_POINT('Ctrl Pts',(-20.6157637308144,-14.0840182336437,
124.315591986878)) ;
#58201=CARTESIAN_POINT('Ctrl Pts',(-20.3744629095565,-13.9040291532808,
124.134836941808)) ;
#58202=CARTESIAN_POINT('Ctrl Pts',(-20.7551952257147,-14.0940801897696,
124.090948556963)) ;
#58203=CARTESIAN_POINT('Ctrl Pts',(-20.4860083127366,-13.9140911094067,
123.955121992217)) ;
#58204=CARTESIAN_POINT('Ctrl Pts',(-20.8516795936219,-14.1039774013707,
123.849406694872)) ;
#58205=CARTESIAN_POINT('Ctrl Pts',(-20.5631955167448,-13.9239883210078,
123.761889246969)) ;
#58206=CARTESIAN_POINT('Ctrl Pts',(-20.9057797422551,-14.1139085680353,
123.594099508417)) ;
#58207=CARTESIAN_POINT('Ctrl Pts',(-20.6064757368551,-13.9339194876725,
123.557644109238)) ;
#58208=CARTESIAN_POINT('Ctrl Pts',(-20.9145419978762,-14.1239507522395,
123.330350913867)) ;
#58209=CARTESIAN_POINT('Ctrl Pts',(-20.6134856993466,-13.9439616718766,
123.346645072015)) ;
#58210=CARTESIAN_POINT('Ctrl Pts',(-20.878134852128,-14.1338374204927,123.073090399106)) ;
#58211=CARTESIAN_POINT('Ctrl Pts',(-20.5843603024591,-13.9538483401298,
123.140837492851)) ;
#58212=CARTESIAN_POINT('Ctrl Pts',(-20.797171317607,-14.1438305324709,122.823288399636)) ;
#58213=CARTESIAN_POINT('Ctrl Pts',(-20.5195898212087,-13.963841452108,122.940995952471)) ;
#58214=CARTESIAN_POINT('Ctrl Pts',(-20.6745548235997,-14.1537762100867,
122.592473334251)) ;
#58215=CARTESIAN_POINT('Ctrl Pts',(-20.4214971012033,-13.9737871297239,
122.756344186729)) ;
#58216=CARTESIAN_POINT('Ctrl Pts',(-20.5141104749864,-14.1637235130717,
122.386083823547)) ;
#58217=CARTESIAN_POINT('Ctrl Pts',(-20.2931422359031,-13.9837344327088,
122.591232683106)) ;
#58218=CARTESIAN_POINT('Ctrl Pts',(-20.3181292651246,-14.1737712368185,
122.209146648077)) ;
#58219=CARTESIAN_POINT('Ctrl Pts',(-20.1363573513922,-13.9937821564556,
122.449682552309)) ;
#58220=CARTESIAN_POINT('Ctrl Pts',(-20.098946063385,-14.183619610581,122.071534647514)) ;
#58221=CARTESIAN_POINT('Ctrl Pts',(-19.961011947168,-14.0036305302181,122.339593209163)) ;
#58222=CARTESIAN_POINT('Ctrl Pts',(-19.8568324061559,-14.1935785830267,
121.972166958928)) ;
#58223=CARTESIAN_POINT('Ctrl Pts',(-19.767321602057,-14.0135895026638,122.260098632269)) ;
#58224=CARTESIAN_POINT('Ctrl Pts',(-19.5989991593622,-14.2036174449079,
121.916368996619)) ;
#58225=CARTESIAN_POINT('Ctrl Pts',(-19.5610549871586,-14.023628364545,122.215459749838)) ;
#58226=CARTESIAN_POINT('Ctrl Pts',(-19.339581937027,-14.2134960490797,121.905934350721)) ;
#58227=CARTESIAN_POINT('Ctrl Pts',(-19.3535221269257,-14.0335069687168,
122.207111469005)) ;
#58228=CARTESIAN_POINT('Ctrl Pts',(-19.0778376414756,-14.223547590283,121.941189793871)) ;
#58229=CARTESIAN_POINT('Ctrl Pts',(-19.1441263879232,-14.0435585099201,
122.235315233814)) ;
#58230=CARTESIAN_POINT('Ctrl Pts',(-18.8299973984445,-14.2334429882633,
122.020057862292)) ;
#58231=CARTESIAN_POINT('Ctrl Pts',(-18.9458547296678,-14.0534539079004,
122.298408839437)) ;
#58232=CARTESIAN_POINT('Ctrl Pts',(-18.5959941772312,-14.2434942208086,
122.142497343035)) ;
#58233=CARTESIAN_POINT('Ctrl Pts',(-18.7586516520923,-14.0635051404457,
122.396359920337)) ;
#58234=CARTESIAN_POINT('Ctrl Pts',(-18.3901717062413,-14.2533804114329,
122.301075810793)) ;
#58235=CARTESIAN_POINT('Ctrl Pts',(-18.5939939275408,-14.07339133107,122.523221635957)) ;
#58236=CARTESIAN_POINT('Ctrl Pts',(-18.2128046217201,-14.2633729507487,
122.494683384681)) ;
#58237=CARTESIAN_POINT('Ctrl Pts',(-18.4520997745653,-14.0833838703858,
122.678107034334)) ;
#58238=CARTESIAN_POINT('Ctrl Pts',(-18.0724208014174,-14.2733213966434,
122.715249428786)) ;
#58239=CARTESIAN_POINT('Ctrl Pts',(-18.339792292697,-14.0933323162805,122.854559084059)) ;
#58240=CARTESIAN_POINT('Ctrl Pts',(-17.9722554347127,-14.2832581991753,
122.956378922665)) ;
#58241=CARTESIAN_POINT('Ctrl Pts',(-18.2596593906044,-14.1032691188124,
123.047461874324)) ;
#58242=CARTESIAN_POINT('Ctrl Pts',(-17.9148800450432,-14.2932412066266,
123.212405357803)) ;
#58243=CARTESIAN_POINT('Ctrl Pts',(-18.2137581989984,-14.1132521262637,
123.252282614946)) ;
#58244=CARTESIAN_POINT('Ctrl Pts',(-17.9032450354326,-14.3032850480414,
123.476059954926)) ;
#58245=CARTESIAN_POINT('Ctrl Pts',(-18.2044493516429,-14.1232959676785,
123.463206407145)) ;
#58246=CARTESIAN_POINT('Ctrl Pts',(-17.9362327116183,-14.3131132466653,
123.732259863028)) ;
#58247=CARTESIAN_POINT('Ctrl Pts',(-18.2308383754507,-14.1331241663024,
123.668165314127)) ;
#58248=CARTESIAN_POINT('Ctrl Pts',(-18.0150012319065,-14.3231898401075,
123.985018013429)) ;
#58249=CARTESIAN_POINT('Ctrl Pts',(-18.2938523322178,-14.1432007597447,
123.870372464175)) ;
#58250=CARTESIAN_POINT('Ctrl Pts',(-18.1336866675862,-14.3330418394491,
124.215176688599)) ;
#58251=CARTESIAN_POINT('Ctrl Pts',(-18.3887993080397,-14.1530527590862,
124.054499001948)) ;
#58252=CARTESIAN_POINT('Ctrl Pts',(-18.2938233161721,-14.343115426273,124.425914520946)) ;
#58253=CARTESIAN_POINT('Ctrl Pts',(-18.5169079559941,-14.1631263459101,
124.223090181388)) ;
#58254=CARTESIAN_POINT('Ctrl Pts',(-18.4837016929012,-14.3529556513705,
124.601492972209)) ;
#58255=CARTESIAN_POINT('Ctrl Pts',(-18.6688091616826,-14.1729665710076,
124.363553020106)) ;
#58256=CARTESIAN_POINT('Ctrl Pts',(-18.703416961841,-14.3629213553991,124.743969337012)) ;
#58257=CARTESIAN_POINT('Ctrl Pts',(-18.844580419153,-14.1829322750362,124.47753501832)) ;
#58258=CARTESIAN_POINT('Ctrl Pts',(-18.946190326884,-14.3729479887057,124.846418837597)) ;
#58259=CARTESIAN_POINT('Ctrl Pts',(-19.0387986926441,-14.1929589083428,
124.559495739056)) ;
#58260=CARTESIAN_POINT('Ctrl Pts',(-19.2001264119849,-14.3828622844175,
124.904667897107)) ;
#58261=CARTESIAN_POINT('Ctrl Pts',(-19.2419467128813,-14.2028732040546,
124.60609605546)) ;
#58262=CARTESIAN_POINT('Ctrl Pts',(-19.4622585243968,-14.39285057311,124.918515058784)) ;
#58263=CARTESIAN_POINT('Ctrl Pts',(-19.4516521770258,-14.2128614927471,
124.617175109609)) ;
#58264=CARTESIAN_POINT('Ctrl Pts',(-19.7240472766002,-14.4028893062683,
124.886002641431)) ;
#58265=CARTESIAN_POINT('Ctrl Pts',(-19.6610834379714,-14.2229002259054,
124.591166382665)) ;
#58266=CARTESIAN_POINT('Ctrl Pts',(-19.9714422784701,-14.4127326380959,
124.810452799983)) ;
#58267=CARTESIAN_POINT('Ctrl Pts',(-19.8589988887457,-14.232743557733,124.530728061937)) ;
#58268=CARTESIAN_POINT('Ctrl Pts',(-20.2065561510804,-14.4227603639755,
124.691438006509)) ;
#58269=CARTESIAN_POINT('Ctrl Pts',(-20.0470906952005,-14.2427712836126,
124.435517495806)) ;
#58270=CARTESIAN_POINT('Ctrl Pts',(-20.4171057819061,-14.432792700364,124.532757562362)) ;
#58271=CARTESIAN_POINT('Ctrl Pts',(-20.2155312378511,-14.2528036200011,
124.308574138805)) ;
#58272=CARTESIAN_POINT('Ctrl Pts',(-20.5936350310893,-14.4426222006646,
124.34420163555)) ;
#58273=CARTESIAN_POINT('Ctrl Pts',(-20.3567549741227,-14.2626331203018,
124.15773110315)) ;
#58274=CARTESIAN_POINT('Ctrl Pts',(-20.7377126082824,-14.4526117045814,
124.124750610571)) ;
#58275=CARTESIAN_POINT('Ctrl Pts',(-20.4720182693449,-14.2726226242185,
123.982171262254)) ;
#58276=CARTESIAN_POINT('Ctrl Pts',(-20.8414417058682,-14.4626555450938,
123.882049023559)) ;
#58277=CARTESIAN_POINT('Ctrl Pts',(-20.5550029138087,-14.2826664647309,
123.788010448594)) ;
#58278=CARTESIAN_POINT('Ctrl Pts',(-20.900648035962,-14.4724772508619,123.63082704311)) ;
#58279=CARTESIAN_POINT('Ctrl Pts',(-20.602369249548,-14.292488170499,123.587034187836)) ;
#58280=CARTESIAN_POINT('Ctrl Pts',(-20.9162986354435,-14.4825122979942,
123.367582647658)) ;
#58281=CARTESIAN_POINT('Ctrl Pts',(-20.6148913940102,-14.3025232176314,
123.376438685901)) ;
#58282=CARTESIAN_POINT('Ctrl Pts',(-20.8853105895479,-14.4925369754311,
123.105964149167)) ;
#58283=CARTESIAN_POINT('Ctrl Pts',(-20.5901024698145,-14.3125478950683,
123.167143688753)) ;
#58284=CARTESIAN_POINT('Ctrl Pts',(-20.8111959911623,-14.5023897902856,
122.85787673168)) ;
#58285=CARTESIAN_POINT('Ctrl Pts',(-20.5308125817991,-14.3224007099227,
122.96867405913)) ;
#58286=CARTESIAN_POINT('Ctrl Pts',(-20.6939628548545,-14.5123774998931,
122.623068574786)) ;
#58287=CARTESIAN_POINT('Ctrl Pts',(-20.4370276691554,-14.3323884195303,
122.780826900379)) ;
#58288=CARTESIAN_POINT('Ctrl Pts',(-20.5386353139162,-14.5223075098872,
122.413370344863)) ;
#58289=CARTESIAN_POINT('Ctrl Pts',(-20.3127672606121,-14.3423184295243,
122.613067632083)) ;
#58290=CARTESIAN_POINT('Ctrl Pts',(-20.3483991859879,-14.5322972651064,
122.232456679631)) ;
#58291=CARTESIAN_POINT('Ctrl Pts',(-20.1605796814699,-14.3523081847435,
122.468335499922)) ;
#58292=CARTESIAN_POINT('Ctrl Pts',(-20.1286457021689,-14.5423238737893,
122.087070807904)) ;
#58293=CARTESIAN_POINT('Ctrl Pts',(-19.9847778210034,-14.3623347934264,
122.352025351931)) ;
#58294=CARTESIAN_POINT('Ctrl Pts',(-19.8905327192245,-14.5522078138111,
121.983318872916)) ;
#58295=CARTESIAN_POINT('Ctrl Pts',(-19.7942886798817,-14.3722187334482,
122.269022420981)) ;
#58296=CARTESIAN_POINT('Ctrl Pts',(-19.635462587809,-14.5621970413496,121.921242080345)) ;
#58297=CARTESIAN_POINT('Ctrl Pts',(-19.5902331362649,-14.3822079609867,
122.219359208042)) ;
#58298=CARTESIAN_POINT('Ctrl Pts',(-19.3720577988296,-14.5722399118733,
121.904853033029)) ;
#58299=CARTESIAN_POINT('Ctrl Pts',(-19.3795093430328,-14.3922508315104,
122.206246194466)) ;
#58300=CARTESIAN_POINT('Ctrl Pts',(-19.1152596800331,-14.5820722986287,
121.933419317847)) ;
#58301=CARTESIAN_POINT('Ctrl Pts',(-19.1740714024378,-14.4020832182658,
122.229097307701)) ;
#58302=CARTESIAN_POINT('Ctrl Pts',(-18.8630536665113,-14.5920655918003,
122.006599511882)) ;
#58303=CARTESIAN_POINT('Ctrl Pts',(-18.9723061434464,-14.4120765114374,
122.287639558264)) ;
#58304=CARTESIAN_POINT('Ctrl Pts',(-18.6267003875226,-14.6020975974487,
122.123410637976)) ;
#58305=CARTESIAN_POINT('Ctrl Pts',(-18.7832226648472,-14.4221085170859,
122.38108679379)) ;
#58306=CARTESIAN_POINT('Ctrl Pts',(-18.4175822404663,-14.6119628534177,
122.276618419926)) ;
#58307=CARTESIAN_POINT('Ctrl Pts',(-18.61592748227,-14.4319737730548,122.503651126042)) ;
#58308=CARTESIAN_POINT('Ctrl Pts',(-18.2359363520061,-14.6219247333252,
122.465143513999)) ;
#58309=CARTESIAN_POINT('Ctrl Pts',(-18.4706094571108,-14.4419356529623,
122.654469655171)) ;
#58310=CARTESIAN_POINT('Ctrl Pts',(-18.0890820796082,-14.6319596666871,
122.684159241081)) ;
#58311=CARTESIAN_POINT('Ctrl Pts',(-18.3531243943116,-14.4519705863242,
122.829681166478)) ;
#58312=CARTESIAN_POINT('Ctrl Pts',(-17.9836588830903,-14.6418446250664,
122.921611991648)) ;
#58313=CARTESIAN_POINT('Ctrl Pts',(-18.2687841767101,-14.4618555447035,
123.019642136378)) ;
#58314=CARTESIAN_POINT('Ctrl Pts',(-17.91999930049,-14.6519102519891,123.178306439075)) ;
#58315=CARTESIAN_POINT('Ctrl Pts',(-18.217854528994,-14.4719211716262,123.224997325049)) ;
#58316=CARTESIAN_POINT('Ctrl Pts',(-17.9020169238166,-14.6617493576534,
123.43628455332)) ;
#58317=CARTESIAN_POINT('Ctrl Pts',(-18.2034666313559,-14.4817602772905,
123.431379111336)) ;
#58318=CARTESIAN_POINT('Ctrl Pts',(-17.9293579840825,-14.6718121726588,
123.699271479237)) ;
#58319=CARTESIAN_POINT('Ctrl Pts',(-18.2253374197392,-14.4918230922959,
123.641768973016)) ;
#58320=CARTESIAN_POINT('Ctrl Pts',(-18.0009916819233,-14.6817083787074,
123.949301617982)) ;
#58321=CARTESIAN_POINT('Ctrl Pts',(-18.2826422983745,-14.5017192983446,
123.841793287146)) ;
#58322=CARTESIAN_POINT('Ctrl Pts',(-18.1147854788541,-14.6916492017327,
124.184415931245)) ;
#58323=CARTESIAN_POINT('Ctrl Pts',(-18.3736753208548,-14.5116601213698,
124.029885468125)) ;
#58324=CARTESIAN_POINT('Ctrl Pts',(-18.2686378473878,-14.7016537847114,
124.397645063482)) ;
#58325=CARTESIAN_POINT('Ctrl Pts',(-18.4967554534644,-14.5216647043485,
124.200469975829)) ;
#58326=CARTESIAN_POINT('Ctrl Pts',(-18.4576820792314,-14.7116746791561,
124.580965224182)) ;
#58327=CARTESIAN_POINT('Ctrl Pts',(-18.6479893550732,-14.5316855987932,
124.347127597631)) ;
#58328=CARTESIAN_POINT('Ctrl Pts',(-18.6727084410143,-14.7215665997455,
124.72705053099)) ;
#58329=CARTESIAN_POINT('Ctrl Pts',(-18.8200089755962,-14.5415775193826,
124.463997424165)) ;
#58330=CARTESIAN_POINT('Ctrl Pts',(-18.9120984381462,-14.7315600320909,
124.835009694246)) ;
#58331=CARTESIAN_POINT('Ctrl Pts',(-19.0115200042416,-14.551570951728,124.55036669427)) ;
#58332=CARTESIAN_POINT('Ctrl Pts',(-19.1654082297074,-14.7415056369908,
124.899373825222)) ;
#58333=CARTESIAN_POINT('Ctrl Pts',(-19.2141671271123,-14.5615165566279,
124.601860046211)) ;
#58334=CARTESIAN_POINT('Ctrl Pts',(-19.4260649276626,-14.7514529104723,
124.919311654018)) ;
#58335=CARTESIAN_POINT('Ctrl Pts',(-19.4226921583559,-14.5714638301094,
124.617812487927)) ;
#58336=CARTESIAN_POINT('Ctrl Pts',(-19.6888039980346,-14.7615008249487,
124.893135998467)) ;
#58337=CARTESIAN_POINT('Ctrl Pts',(-19.6328836382695,-14.5815117445858,
124.596874129132)) ;
#58338=CARTESIAN_POINT('Ctrl Pts',(-19.9380105597305,-14.771348465296,124.823369065413)) ;
#58339=CARTESIAN_POINT('Ctrl Pts',(-19.8322491726103,-14.5913593849331,
124.541062779856)) ;
#58340=CARTESIAN_POINT('Ctrl Pts',(-20.1743610165879,-14.7813101806726,
124.710840541122)) ;
#58341=CARTESIAN_POINT('Ctrl Pts',(-20.0213304109851,-14.6013211003097,
124.451042024514)) ;
#58342=CARTESIAN_POINT('Ctrl Pts',(-20.3888445239229,-14.7913388042454,
124.557674697892)) ;
#58343=CARTESIAN_POINT('Ctrl Pts',(-20.1929184772654,-14.6113497238825,
124.32851117537)) ;
#58344=CARTESIAN_POINT('Ctrl Pts',(-20.5713377846761,-14.8012491663118,
124.371890859621)) ;
#58345=CARTESIAN_POINT('Ctrl Pts',(-20.3389145561169,-14.6212600859489,
124.179885784323)) ;
#58346=CARTESIAN_POINT('Ctrl Pts',(-20.7197431781313,-14.8111838599642,
124.157087470465)) ;
#58347=CARTESIAN_POINT('Ctrl Pts',(-20.457640661641,-14.6311947796013,124.008044437838)) ;
#58348=CARTESIAN_POINT('Ctrl Pts',(-20.8295234845104,-14.8212257030921,
123.917131743842)) ;
#58349=CARTESIAN_POINT('Ctrl Pts',(-20.5454669287708,-14.6412366227292,
123.816080822821)) ;
#58350=CARTESIAN_POINT('Ctrl Pts',(-20.8951642259537,-14.8311102086625,
123.665780824477)) ;
#58351=CARTESIAN_POINT('Ctrl Pts',(-20.5979816634709,-14.6511211282996,
123.615000778527)) ;
#58352=CARTESIAN_POINT('Ctrl Pts',(-20.9167156314067,-14.8411123124477,
123.40385951735)) ;
#58353=CARTESIAN_POINT('Ctrl Pts',(-20.6152250273271,-14.6611232320848,
123.405463971272)) ;
#58354=CARTESIAN_POINT('Ctrl Pts',(-20.8928717590869,-14.8510306638627,
123.144264974598)) ;
#58355=CARTESIAN_POINT('Ctrl Pts',(-20.5961521920614,-14.6710415834998,
123.197788211826)) ;
#58356=CARTESIAN_POINT('Ctrl Pts',(-20.8233784416685,-14.8610783198836,
122.889574983756)) ;
#58357=CARTESIAN_POINT('Ctrl Pts',(-20.5405596778779,-14.6810892395207,
122.994035641784)) ;
#58358=CARTESIAN_POINT('Ctrl Pts',(-20.7129195792152,-14.8709495129118,
122.65480303298)) ;
#58359=CARTESIAN_POINT('Ctrl Pts',(-20.4521948362717,-14.6909604325489,
122.806217311393)) ;
#58360=CARTESIAN_POINT('Ctrl Pts',(-20.5605298604237,-14.8810152260553,
122.438669790613)) ;
#58361=CARTESIAN_POINT('Ctrl Pts',(-20.330284230218,-14.7010261456924,122.633308925959)) ;
#58362=CARTESIAN_POINT('Ctrl Pts',(-20.3770184511198,-14.890867686628,122.255919659017)) ;
#58363=CARTESIAN_POINT('Ctrl Pts',(-20.1834793625096,-14.7108786062651,
122.487109277975)) ;
#58364=CARTESIAN_POINT('Ctrl Pts',(-20.087542768723,-14.9042961493505,122.054287114174)) ;
#58365=CARTESIAN_POINT('Ctrl Pts',(-19.9518873140162,-14.7243070689876,
122.325790630287)) ;
#58366=CARTESIAN_POINT('Ctrl Pts',(-19.7606733441546,-14.9173770968676,
121.935403530529)) ;
#58367=CARTESIAN_POINT('Ctrl Pts',(-19.6903664132712,-14.7373880165047,
122.230682365548)) ;
#58368=CARTESIAN_POINT('Ctrl Pts',(-19.4080294143569,-14.9308515951022,
121.904239538084)) ;
#58369=CARTESIAN_POINT('Ctrl Pts',(-19.408296278235,-14.7508625147393,122.205756669958)) ;
#58370=CARTESIAN_POINT('Ctrl Pts',(-19.1506048230124,-14.9406836987116,
121.926886772641)) ;
#58371=CARTESIAN_POINT('Ctrl Pts',(-19.2023472618255,-14.7606946183488,
122.223870633588)) ;
#58372=CARTESIAN_POINT('Ctrl Pts',(-18.8974267387151,-14.9506496018383,
121.993755117999)) ;
#58373=CARTESIAN_POINT('Ctrl Pts',(-18.9998068131851,-14.7706605214754,
122.277363288063)) ;
#58374=CARTESIAN_POINT('Ctrl Pts',(-18.6583498545096,-14.9606770111485,
122.104643278367)) ;
#58375=CARTESIAN_POINT('Ctrl Pts',(-18.8085430338256,-14.7806879307857,
122.366073028994)) ;
#58376=CARTESIAN_POINT('Ctrl Pts',(-18.4446798401524,-14.9705880425151,
122.253516252991)) ;
#58377=CARTESIAN_POINT('Ctrl Pts',(-18.6376088003778,-14.7905989621522,
122.485164544284)) ;
#58378=CARTESIAN_POINT('Ctrl Pts',(-18.1971580268326,-14.9838323501362,
122.498300087744)) ;
#58379=CARTESIAN_POINT('Ctrl Pts',(-18.4395744217537,-14.8038432697733,
122.681015310389)) ;
#58380=CARTESIAN_POINT('Ctrl Pts',(-17.9735883960073,-15.0005328328073,
122.881645823256)) ;
#58381=CARTESIAN_POINT('Ctrl Pts',(-18.2607334713096,-14.8205437524445,
122.987646040595)) ;
#58382=CARTESIAN_POINT('Ctrl Pts',(-17.8949212635065,-15.0170396619631,
123.313331293313)) ;
#58383=CARTESIAN_POINT('Ctrl Pts',(-18.197786980337,-14.8370505816002,123.333061833224)) ;
#58384=CARTESIAN_POINT('Ctrl Pts',(-17.9226408363166,-15.0303502902007,
123.661981974254)) ;
#58385=CARTESIAN_POINT('Ctrl Pts',(-18.2199642568686,-14.8503612098378,
123.611928568434)) ;
#58386=CARTESIAN_POINT('Ctrl Pts',(-17.9885443792014,-15.0403428537408,
123.916213406476)) ;
#58387=CARTESIAN_POINT('Ctrl Pts',(-18.2726848749169,-14.8603537733779,
123.815325758311)) ;
#58388=CARTESIAN_POINT('Ctrl Pts',(-18.0982567045418,-15.0503729367423,
124.155839488556)) ;
#58389=CARTESIAN_POINT('Ctrl Pts',(-18.3604503472436,-14.8703838563795,
124.007021726878)) ;
#58390=CARTESIAN_POINT('Ctrl Pts',(-18.294281628791,-15.0635465407401,124.441261777876)) ;
#58391=CARTESIAN_POINT('Ctrl Pts',(-18.5172815099474,-14.8835574603772,
124.235376257215)) ;
#58392=CARTESIAN_POINT('Ctrl Pts',(-18.6299004804778,-15.0801842459715,
124.72893753815)) ;
#58393=CARTESIAN_POINT('Ctrl Pts',(-18.785763290496,-14.9001951656086,124.465502997211)) ;
#58394=CARTESIAN_POINT('Ctrl Pts',(-19.1244402677115,-15.1000660085389,
124.915683237853)) ;
#58395=CARTESIAN_POINT('Ctrl Pts',(-19.1813811513845,-14.9200769281761,
124.614910725455)) ;
#58396=CARTESIAN_POINT('Ctrl Pts',(-19.5680268436857,-15.1167623607554,
124.921075710828)) ;
#58397=CARTESIAN_POINT('Ctrl Pts',(-19.5363048231766,-14.9367732803926,
124.619219761806)) ;
#58398=CARTESIAN_POINT('Ctrl Pts',(-19.9032277012158,-15.1299193885445,
124.836006276955)) ;
#58399=CARTESIAN_POINT('Ctrl Pts',(-19.804416663056,-14.9499303081817,124.551173733196)) ;
#58400=CARTESIAN_POINT('Ctrl Pts',(-20.2240299227746,-15.1432967431881,
124.692326184051)) ;
#58401=CARTESIAN_POINT('Ctrl Pts',(-20.0610789329257,-14.9633076628252,
124.436222806107)) ;
#58402=CARTESIAN_POINT('Ctrl Pts',(-20.5648835408221,-15.1598275774469,
124.415004995461)) ;
#58403=CARTESIAN_POINT('Ctrl Pts',(-20.33374952369,-14.979838497084,124.214377150155)) ;
#58404=CARTESIAN_POINT('Ctrl Pts',(-20.8382356610329,-15.17979226719,123.960261264776)) ;
#58405=CARTESIAN_POINT('Ctrl Pts',(-20.5524388724161,-14.9998031868271,
123.850580630537)) ;
#58406=CARTESIAN_POINT('Ctrl Pts',(-20.9392779039823,-15.1997087606136,
123.440635012867)) ;
#58407=CARTESIAN_POINT('Ctrl Pts',(-20.6332747129782,-15.0197196802507,
123.434880576487)) ;
#58408=CARTESIAN_POINT('Ctrl Pts',(-20.8580805309166,-15.2195984799632,
122.918218801443)) ;
#58409=CARTESIAN_POINT('Ctrl Pts',(-20.5683198928512,-15.0396093996003,
123.016946176903)) ;
#58410=CARTESIAN_POINT('Ctrl Pts',(-20.6016712396196,-15.239605209611,122.45246543698)) ;
#58411=CARTESIAN_POINT('Ctrl Pts',(-20.363194945236,-15.0596161292481,122.644342199294)) ;
#58412=CARTESIAN_POINT('Ctrl Pts',(-20.2052118909962,-15.2594432632579,
122.104699832134)) ;
#58413=CARTESIAN_POINT('Ctrl Pts',(-20.0460282780659,-15.079454182895,122.366126875178)) ;
#58414=CARTESIAN_POINT('Ctrl Pts',(-19.7104197648505,-15.2794366014715,
121.911172706133)) ;
#58415=CARTESIAN_POINT('Ctrl Pts',(-19.6501953671741,-15.0994475211086,
122.211302958785)) ;
#58416=CARTESIAN_POINT('Ctrl Pts',(-19.1820210308814,-15.2993194008781,
121.898505004141)) ;
#58417=CARTESIAN_POINT('Ctrl Pts',(-19.2274754164287,-15.1193303205152,
122.201166461084)) ;
#58418=CARTESIAN_POINT('Ctrl Pts',(-18.6807320925926,-15.3192115817968,
122.06605896947)) ;
#58419=CARTESIAN_POINT('Ctrl Pts',(-18.8264426177306,-15.1392225014339,
122.335208221256)) ;
#58420=CARTESIAN_POINT('Ctrl Pts',(-18.2657076846686,-15.3391137602919,
122.394277865644)) ;
#58421=CARTESIAN_POINT('Ctrl Pts',(-18.494421510302,-15.159124679929,122.597782896425)) ;
#58422=CARTESIAN_POINT('Ctrl Pts',(-17.9866547281374,-15.3591510714956,
122.847707709371)) ;
#58423=CARTESIAN_POINT('Ctrl Pts',(-18.2711780423566,-15.1791619911328,
122.960525608524)) ;
#58424=CARTESIAN_POINT('Ctrl Pts',(-17.8794922157529,-15.3789635130365,
123.363506708324)) ;
#58425=CARTESIAN_POINT('Ctrl Pts',(-18.1854465971545,-15.1989744326736,
123.373166586324)) ;
#58426=CARTESIAN_POINT('Ctrl Pts',(-17.955834597053,-15.3990287537714,123.891058298143)) ;
#58427=CARTESIAN_POINT('Ctrl Pts',(-18.2465194339574,-15.2190396734085,
123.795207317988)) ;
#58428=CARTESIAN_POINT('Ctrl Pts',(-18.2036257717715,-15.4187859586272,
124.35431729337)) ;
#58429=CARTESIAN_POINT('Ctrl Pts',(-18.444753257949,-15.2387968782644,124.165817334642)) ;
#58430=CARTESIAN_POINT('Ctrl Pts',(-18.5991767273495,-15.4388192312729,
124.710349085039)) ;
#58431=CARTESIAN_POINT('Ctrl Pts',(-18.7611938046602,-15.2588301509101,
124.450642577608)) ;
#58432=CARTESIAN_POINT('Ctrl Pts',(-19.0875441524019,-15.4586321397268,
124.907957059452)) ;
#58433=CARTESIAN_POINT('Ctrl Pts',(-19.1518899723408,-15.2786430593639,
124.608729644721)) ;
#58434=CARTESIAN_POINT('Ctrl Pts',(-19.6183970906308,-15.4786282858542,
124.927914166445)) ;
#58435=CARTESIAN_POINT('Ctrl Pts',(-19.576572466702,-15.2986392054913,124.62469458261)) ;
#58436=CARTESIAN_POINT('Ctrl Pts',(-20.1213238855666,-15.4984900390767,
124.766723103207)) ;
#58437=CARTESIAN_POINT('Ctrl Pts',(-19.9789150179613,-15.3185009587138,
124.495740310664)) ;
#58438=CARTESIAN_POINT('Ctrl Pts',(-20.5429196526182,-15.5185585562048,
124.440174246411)) ;
#58439=CARTESIAN_POINT('Ctrl Pts',(-20.3161903555175,-15.3385694758419,
124.234500854143)) ;
#58440=CARTESIAN_POINT('Ctrl Pts',(-20.8242320696034,-15.5383894292016,
123.994315885912)) ;
#58441=CARTESIAN_POINT('Ctrl Pts',(-20.5412403549953,-15.3584003488387,
123.877812029321)) ;
#58442=CARTESIAN_POINT('Ctrl Pts',(-20.9383743235662,-15.5583113400183,
123.477399544044)) ;
#58443=CARTESIAN_POINT('Ctrl Pts',(-20.6325525210197,-15.3783222596554,
123.464277746288)) ;
#58444=CARTESIAN_POINT('Ctrl Pts',(-20.8690610707405,-15.5782407834536,
122.952175132017)) ;
#58445=CARTESIAN_POINT('Ctrl Pts',(-20.5770999180587,-15.3982517030907,
123.044097841455)) ;
#58446=CARTESIAN_POINT('Ctrl Pts',(-20.6251692263084,-15.59815045357,122.482655310939)) ;
#58447=CARTESIAN_POINT('Ctrl Pts',(-20.3819841289406,-15.4181613732071,
122.668482232618)) ;
#58448=CARTESIAN_POINT('Ctrl Pts',(-20.2369405024036,-15.6180238108329,
122.124408327086)) ;
#58449=CARTESIAN_POINT('Ctrl Pts',(-20.0713986144983,-15.43803473047,122.381885868014)) ;
#58450=CARTESIAN_POINT('Ctrl Pts',(-19.7469529682357,-15.6380153454508,
121.919076471871)) ;
#58451=CARTESIAN_POINT('Ctrl Pts',(-19.6794074858345,-15.4580262650879,
122.217622870441)) ;
#58452=CARTESIAN_POINT('Ctrl Pts',(-19.2195107524883,-15.6578809628615,
121.893213319316)) ;
#58453=CARTESIAN_POINT('Ctrl Pts',(-19.257452611772,-15.4778918824987,122.196935186946)) ;
#58454=CARTESIAN_POINT('Ctrl Pts',(-18.7119132760314,-15.6778618926898,
122.049260143643)) ;
#58455=CARTESIAN_POINT('Ctrl Pts',(-18.8513754816871,-15.4978728123269,
122.321775691797)) ;
#58456=CARTESIAN_POINT('Ctrl Pts',(-18.2892684219833,-15.6978003547729,
122.368964780256)) ;
#58457=CARTESIAN_POINT('Ctrl Pts',(-18.513261161945,-15.51781127441,122.577542114275)) ;
#58458=CARTESIAN_POINT('Ctrl Pts',(-18.0010412603232,-15.7176925479946,
122.812265657401)) ;
#58459=CARTESIAN_POINT('Ctrl Pts',(-18.2826819358055,-15.5377034676318,
122.932185207393)) ;
#58460=CARTESIAN_POINT('Ctrl Pts',(-17.8812058283193,-15.73766326303,123.329230583634)) ;
#58461=CARTESIAN_POINT('Ctrl Pts',(-18.1868169736697,-15.5576741826671,
123.345758094485)) ;
#58462=CARTESIAN_POINT('Ctrl Pts',(-17.9435942352086,-15.7574729346961,
123.852155946774)) ;
#58463=CARTESIAN_POINT('Ctrl Pts',(-18.236731360586,-15.5774838543332,123.764098868335)) ;
#58464=CARTESIAN_POINT('Ctrl Pts',(-18.1823832687672,-15.7774661513873,
124.326648974509)) ;
#58465=CARTESIAN_POINT('Ctrl Pts',(-18.4277666392234,-15.5974770710244,
124.143691534973)) ;
#58466=CARTESIAN_POINT('Ctrl Pts',(-18.5660086878683,-15.7973170635836,
124.689180060652)) ;
#58467=CARTESIAN_POINT('Ctrl Pts',(-18.7346680390251,-15.6173279832208,
124.433713872996)) ;
#58468=CARTESIAN_POINT('Ctrl Pts',(-19.0555605460036,-15.8173916699027,
124.900980308244)) ;
#58469=CARTESIAN_POINT('Ctrl Pts',(-19.126318602416,-15.6374025895398,124.603150145415)) ;
#58470=CARTESIAN_POINT('Ctrl Pts',(-19.493934124633,-15.833908301786,124.927054796924)) ;
#58471=CARTESIAN_POINT('Ctrl Pts',(-19.4769939508857,-15.6539192214231,
124.62400662122)) ;
#58472=CARTESIAN_POINT('Ctrl Pts',(-19.837342147255,-15.8472470094801,124.8571673599)) ;
#58473=CARTESIAN_POINT('Ctrl Pts',(-19.7517415685983,-15.6672579291172,
124.568093350014)) ;
#58474=CARTESIAN_POINT('Ctrl Pts',(-20.0781804979122,-15.8570893837884,
124.762739875852)) ;
#58475=CARTESIAN_POINT('Ctrl Pts',(-19.9444057990373,-15.6771003034255,
124.492551480651)) ;
#58476=CARTESIAN_POINT('Ctrl Pts',(-20.303796053823,-15.8671444037711,124.625272793233)) ;
#58477=CARTESIAN_POINT('Ctrl Pts',(-20.1249049700663,-15.6871553234083,
124.38256759213)) ;
#58478=CARTESIAN_POINT('Ctrl Pts',(-20.5648469001253,-15.8803765604287,
124.395495442102)) ;
#58479=CARTESIAN_POINT('Ctrl Pts',(-20.333709310747,-15.7003874800658,124.198785755722)) ;
#58480=CARTESIAN_POINT('Ctrl Pts',(-20.8101326079248,-15.8969915277738,
124.02832371329)) ;
#58481=CARTESIAN_POINT('Ctrl Pts',(-20.5299755608498,-15.717002447411,123.904990049025)) ;
#58482=CARTESIAN_POINT('Ctrl Pts',(-20.9150857051299,-15.913586114785,123.599951810518)) ;
#58483=CARTESIAN_POINT('Ctrl Pts',(-20.6139164049773,-15.7335970344222,
123.562338490809)) ;
#58484=CARTESIAN_POINT('Ctrl Pts',(-20.9083137993507,-15.9268196831404,
123.252228775196)) ;
#58485=CARTESIAN_POINT('Ctrl Pts',(-20.6085033810929,-15.7468306027775,
123.28412879026)) ;
#58486=CARTESIAN_POINT('Ctrl Pts',(-20.8574915953394,-15.9368633009491,
122.993254896173)) ;
#58487=CARTESIAN_POINT('Ctrl Pts',(-20.5678420886449,-15.7568742205862,
123.076956586024)) ;
#58488=CARTESIAN_POINT('Ctrl Pts',(-20.7640240610611,-15.9467502251839,
122.750807958911)) ;
#58489=CARTESIAN_POINT('Ctrl Pts',(-20.4930658151328,-15.766761144821,122.88299771998)) ;
#58490=CARTESIAN_POINT('Ctrl Pts',(-20.6288932481491,-15.9567408796307,
122.525730668388)) ;
#58491=CARTESIAN_POINT('Ctrl Pts',(-20.3849611673798,-15.7767517992678,
122.702938858516)) ;
#58492=CARTESIAN_POINT('Ctrl Pts',(-20.4571800169588,-15.9667026380847,
122.328129169805)) ;
#58493=CARTESIAN_POINT('Ctrl Pts',(-20.2475814010665,-15.7867135577218,
122.544854090362)) ;
#58494=CARTESIAN_POINT('Ctrl Pts',(-20.1849716448928,-15.9800425031519,
122.107130949398)) ;
#58495=CARTESIAN_POINT('Ctrl Pts',(-20.0298503330428,-15.800053422789,122.368082503893)) ;
#58496=CARTESIAN_POINT('Ctrl Pts',(-19.8618390549407,-15.9933512860652,
121.963354376013)) ;
#58497=CARTESIAN_POINT('Ctrl Pts',(-19.7713258119905,-15.8133622057023,
122.25304504801)) ;
#58498=CARTESIAN_POINT('Ctrl Pts',(-19.5194352459976,-16.0065470435093,
121.908483591951)) ;
#58499=CARTESIAN_POINT('Ctrl Pts',(-19.4973853555819,-15.8265579631464,
122.209149363533)) ;
#58500=CARTESIAN_POINT('Ctrl Pts',(-19.2576646411518,-16.0165089271858,
121.911843868139)) ;
#58501=CARTESIAN_POINT('Ctrl Pts',(-19.2879723775728,-15.8365198468229,
122.211840251455)) ;
#58502=CARTESIAN_POINT('Ctrl Pts',(-18.9984455353945,-16.0265520367004,
121.961426597411)) ;
#58503=CARTESIAN_POINT('Ctrl Pts',(-19.0805966476983,-15.8465629563375,
122.251508536236)) ;
#58504=CARTESIAN_POINT('Ctrl Pts',(-18.7563398527303,-16.0364042866996,
122.053197919852)) ;
#58505=CARTESIAN_POINT('Ctrl Pts',(-18.8869132360213,-15.8564152063368,
122.324927701526)) ;
#58506=CARTESIAN_POINT('Ctrl Pts',(-18.5308557513542,-16.0463758236501,
122.186642824529)) ;
#58507=CARTESIAN_POINT('Ctrl Pts',(-18.7065271150843,-15.8663867432872,
122.431685506008)) ;
#58508=CARTESIAN_POINT('Ctrl Pts',(-18.331455189681,-16.0563710891276,122.357680218404)) ;
#58509=CARTESIAN_POINT('Ctrl Pts',(-18.5470081927436,-15.8763820087648,
122.568517085258)) ;
#58510=CARTESIAN_POINT('Ctrl Pts',(-18.164426495201,-16.0664050620013,122.561684900348)) ;
#58511=CARTESIAN_POINT('Ctrl Pts',(-18.4133869982469,-15.8864159816384,
122.731722236848)) ;
#58512=CARTESIAN_POINT('Ctrl Pts',(-18.037271614364,-16.0762604767636,122.787340539645)) ;
#58513=CARTESIAN_POINT('Ctrl Pts',(-18.3116651407134,-15.8962713964007,
122.912247684701)) ;
#58514=CARTESIAN_POINT('Ctrl Pts',(-17.9496588451974,-16.0862597542724,
123.035027131255)) ;
#58515=CARTESIAN_POINT('Ctrl Pts',(-18.2415770550694,-15.9062706739096,
123.110397634539)) ;
#58516=CARTESIAN_POINT('Ctrl Pts',(-17.9065430994945,-16.0961549384354,
123.291508010341)) ;
#58517=CARTESIAN_POINT('Ctrl Pts',(-18.2070866753849,-15.9161658580725,
123.315582497717)) ;
#58518=CARTESIAN_POINT('Ctrl Pts',(-17.908679550301,-16.1062153180762,123.555839709386)) ;
#58519=CARTESIAN_POINT('Ctrl Pts',(-18.2087980556812,-15.9262262377133,
123.527047864045)) ;
#58520=CARTESIAN_POINT('Ctrl Pts',(-17.9555303866204,-16.1160651870843,
123.810434776852)) ;
#58521=CARTESIAN_POINT('Ctrl Pts',(-18.246280837973,-15.9360761067214,123.730723208321)) ;
#58522=CARTESIAN_POINT('Ctrl Pts',(-18.0469625663343,-16.1260967482922,
124.057672087697)) ;
#58523=CARTESIAN_POINT('Ctrl Pts',(-18.3194286080762,-15.9461076679293,
123.928512283029)) ;
#58524=CARTESIAN_POINT('Ctrl Pts',(-18.1801329408613,-16.1361071971745,
124.284566442434)) ;
#58525=CARTESIAN_POINT('Ctrl Pts',(-18.4259667878995,-15.9561181168116,
124.110026615654)) ;
#58526=CARTESIAN_POINT('Ctrl Pts',(-18.3486698658472,-16.1460139365915,
124.482977937529)) ;
#58527=CARTESIAN_POINT('Ctrl Pts',(-18.560797834217,-15.9660248562286,124.26875420935)) ;
#58528=CARTESIAN_POINT('Ctrl Pts',(-18.5494006644894,-16.1559519526599,
124.65002353466)) ;
#58529=CARTESIAN_POINT('Ctrl Pts',(-18.7213836797502,-15.9759628722971,
124.402388898548)) ;
#58530=CARTESIAN_POINT('Ctrl Pts',(-18.7775718601343,-16.1659571991111,
124.780727182674)) ;
#58531=CARTESIAN_POINT('Ctrl Pts',(-18.9039216373305,-15.9859681187482,
124.506949936595)) ;
#58532=CARTESIAN_POINT('Ctrl Pts',(-19.0257972538791,-16.1759912601674,
124.869646856981)) ;
#58533=CARTESIAN_POINT('Ctrl Pts',(-19.1025026967416,-15.9960021798045,
124.578083637669)) ;
#58534=CARTESIAN_POINT('Ctrl Pts',(-19.2807496064641,-16.1858363412255,
124.913723831211)) ;
#58535=CARTESIAN_POINT('Ctrl Pts',(-19.3064644940587,-16.0058472608626,
124.613343042249)) ;
#58536=CARTESIAN_POINT('Ctrl Pts',(-19.5431244270057,-16.195822147179,124.913341409534)) ;
#58537=CARTESIAN_POINT('Ctrl Pts',(-19.5163642183528,-16.0158330668161,
124.61303502158)) ;
#58538=CARTESIAN_POINT('Ctrl Pts',(-19.8002495182117,-16.2057569677332,
124.86781116894)) ;
#58539=CARTESIAN_POINT('Ctrl Pts',(-19.7220636745429,-16.0257678873703,
124.576608849091)) ;
#58540=CARTESIAN_POINT('Ctrl Pts',(-20.0484305675557,-16.2158144928654,
124.777029790826)) ;
#58541=CARTESIAN_POINT('Ctrl Pts',(-19.9206078848616,-16.0358254125025,
124.503981752975)) ;
#58542=CARTESIAN_POINT('Ctrl Pts',(-20.2719717473046,-16.2256361435168,
124.647952173762)) ;
#58543=CARTESIAN_POINT('Ctrl Pts',(-20.0994392637093,-16.0456470631539,
124.40071820774)) ;
#58544=CARTESIAN_POINT('Ctrl Pts',(-20.4747026404309,-16.2356922070215,
124.478471590715)) ;
#58545=CARTESIAN_POINT('Ctrl Pts',(-20.2616227752683,-16.0557031266586,
124.265132163495)) ;
#58546=CARTESIAN_POINT('Ctrl Pts',(-20.6426334922787,-16.2456328740854,
124.278356285801)) ;
#58547=CARTESIAN_POINT('Ctrl Pts',(-20.395965720866,-16.0656437937226,124.105038812576)) ;
#58548=CARTESIAN_POINT('Ctrl Pts',(-20.7734945781979,-16.2555372677514,
124.053362462488)) ;
#58549=CARTESIAN_POINT('Ctrl Pts',(-20.5006527028132,-16.0755481873885,
123.925043150666)) ;
#58550=CARTESIAN_POINT('Ctrl Pts',(-20.8644201156856,-16.2655837915144,
123.805527276489)) ;
#58551=CARTESIAN_POINT('Ctrl Pts',(-20.5733913233788,-16.0855947111516,
123.726774248411)) ;
#58552=CARTESIAN_POINT('Ctrl Pts',(-20.9104948421842,-16.2754798745308,
123.549534920301)) ;
#58553=CARTESIAN_POINT('Ctrl Pts',(-20.6102491311177,-16.0954907941679,
123.521980487086)) ;
#58554=CARTESIAN_POINT('Ctrl Pts',(-20.9113721563004,-16.2855465737608,
123.285041710437)) ;
#58555=CARTESIAN_POINT('Ctrl Pts',(-20.6109490499967,-16.105557493398,123.310385748136)) ;
#58556=CARTESIAN_POINT('Ctrl Pts',(-20.8676796982969,-16.2953701841619,
123.030571216678)) ;
#58557=CARTESIAN_POINT('Ctrl Pts',(-20.5759933528988,-16.115381103799,123.106810427065)) ;
#58558=CARTESIAN_POINT('Ctrl Pts',(-20.7788672822299,-16.3054260443394,
122.78172092023)) ;
#58559=CARTESIAN_POINT('Ctrl Pts',(-20.5049416634882,-16.1254369639765,
122.907730678547)) ;
#58560=CARTESIAN_POINT('Ctrl Pts',(-20.6494650621371,-16.3153591906443,
122.554983567681)) ;
#58561=CARTESIAN_POINT('Ctrl Pts',(-20.4014184363261,-16.1353701102815,
122.726342029914)) ;
#58562=CARTESIAN_POINT('Ctrl Pts',(-20.482907205734,-16.3253044464149,122.353620794924)) ;
#58563=CARTESIAN_POINT('Ctrl Pts',(-20.2681709878727,-16.1453153660521,
122.565253212726)) ;
#58564=CARTESIAN_POINT('Ctrl Pts',(-20.2832435137654,-16.3352877448534,
122.183387066587)) ;
#58565=CARTESIAN_POINT('Ctrl Pts',(-20.1084390193321,-16.1552986644905,
122.42906766522)) ;
#58566=CARTESIAN_POINT('Ctrl Pts',(-20.0556974557247,-16.345324925,122.050026596419)) ;
#58567=CARTESIAN_POINT('Ctrl Pts',(-19.9264011931984,-16.1653358446372,
122.322380816789)) ;
#58568=CARTESIAN_POINT('Ctrl Pts',(-19.8130492090875,-16.3551794777095,
121.959479734219)) ;
#58569=CARTESIAN_POINT('Ctrl Pts',(-19.7322826766303,-16.1751903973466,
122.249945218267)) ;
#58570=CARTESIAN_POINT('Ctrl Pts',(-19.5547543717417,-16.3651789961568,
121.911400782604)) ;
#58571=CARTESIAN_POINT('Ctrl Pts',(-19.5256466039838,-16.185189915794,122.211483732283)) ;
#58572=CARTESIAN_POINT('Ctrl Pts',(-19.2946925229401,-16.3750740786189,
121.908649507765)) ;
#58573=CARTESIAN_POINT('Ctrl Pts',(-19.3175976958741,-16.195084998256,122.209284348646)) ;
#58574=CARTESIAN_POINT('Ctrl Pts',(-19.0338948184868,-16.385134624125,121.951817978904)) ;
#58575=CARTESIAN_POINT('Ctrl Pts',(-19.1089596094464,-16.2051455437621,
122.243820773441)) ;
#58576=CARTESIAN_POINT('Ctrl Pts',(-18.7896903909749,-16.394983931373,122.037651600435)) ;
#58577=CARTESIAN_POINT('Ctrl Pts',(-18.9135973885813,-16.2149948510101,
122.312488912832)) ;
#58578=CARTESIAN_POINT('Ctrl Pts',(-18.5597221685601,-16.4050110214604,
122.166277137884)) ;
#58579=CARTESIAN_POINT('Ctrl Pts',(-18.729623508621,-16.2250219410975,122.415390653368)) ;
#58580=CARTESIAN_POINT('Ctrl Pts',(-18.3559738383633,-16.4150399255973,
122.333461717457)) ;
#58581=CARTESIAN_POINT('Ctrl Pts',(-18.5666258270769,-16.2350508452344,
122.549139604119)) ;
#58582=CARTESIAN_POINT('Ctrl Pts',(-18.1871403035161,-16.4248837906966,
122.529443722511)) ;
#58583=CARTESIAN_POINT('Ctrl Pts',(-18.4315607383292,-16.2448947103337,
122.705925518047)) ;
#58584=CARTESIAN_POINT('Ctrl Pts',(-18.0522973396058,-16.434879617405,122.754872248908)) ;
#58585=CARTESIAN_POINT('Ctrl Pts',(-18.3236876314131,-16.2548905370421,
122.886268932754)) ;
#58586=CARTESIAN_POINT('Ctrl Pts',(-17.9588203685943,-16.444904834054,123.001188739217)) ;
#58587=CARTESIAN_POINT('Ctrl Pts',(-18.2489074300727,-16.2649157536911,
123.083322689755)) ;
#58588=CARTESIAN_POINT('Ctrl Pts',(-17.909853990901,-16.4547946662116,123.256433493462)) ;
#58589=CARTESIAN_POINT('Ctrl Pts',(-18.2097358498301,-16.2748055858487,
123.287518087541)) ;
#58590=CARTESIAN_POINT('Ctrl Pts',(-17.9055514641145,-16.4647855222963,
123.518938743175)) ;
#58591=CARTESIAN_POINT('Ctrl Pts',(-18.2062951731,-16.2847964419335,123.497522159626)) ;
#58592=CARTESIAN_POINT('Ctrl Pts',(-17.9467544397181,-16.4747306168892,
123.777016725455)) ;
#58593=CARTESIAN_POINT('Ctrl Pts',(-18.2392588287559,-16.2947415365263,
123.70398393257)) ;
#58594=CARTESIAN_POINT('Ctrl Pts',(-18.0317409622789,-16.4846825206573,
124.02435926062)) ;
#58595=CARTESIAN_POINT('Ctrl Pts',(-18.3072491056377,-16.3046934402944,
123.901857190127)) ;
#58596=CARTESIAN_POINT('Ctrl Pts',(-18.1596521832206,-16.4947189201267,
124.255004193986)) ;
#58597=CARTESIAN_POINT('Ctrl Pts',(-18.4095792698802,-16.3147298397639,
124.086372598792)) ;
#58598=CARTESIAN_POINT('Ctrl Pts',(-18.3230928107259,-16.5046079902154,
124.45706017088)) ;
#58599=CARTESIAN_POINT('Ctrl Pts',(-18.5403322885734,-16.3246189098525,
124.248016015903)) ;
#58600=CARTESIAN_POINT('Ctrl Pts',(-18.5207993714946,-16.5145972795863,
124.62974295052)) ;
#58601=CARTESIAN_POINT('Ctrl Pts',(-18.6984981684148,-16.3346081992234,
124.386161255533)) ;
#58602=CARTESIAN_POINT('Ctrl Pts',(-18.7448946531672,-16.524555845796,124.764889240736)) ;
#58603=CARTESIAN_POINT('Ctrl Pts',(-18.8777747171326,-16.3445667654331,
124.494277080252)) ;
#58604=CARTESIAN_POINT('Ctrl Pts',(-18.9873964306672,-16.5344554170128,
124.859121187844)) ;
#58605=CARTESIAN_POINT('Ctrl Pts',(-19.0717758652844,-16.3544663366499,
124.569661399205)) ;
#58606=CARTESIAN_POINT('Ctrl Pts',(-19.2463751321028,-16.5445033314271,
124.910475054052)) ;
#58607=CARTESIAN_POINT('Ctrl Pts',(-19.2789592074066,-16.3645142510642,
124.610743469147)) ;
#58608=CARTESIAN_POINT('Ctrl Pts',(-19.5063926931676,-16.5543986742876,
124.916202482167)) ;
#58609=CARTESIAN_POINT('Ctrl Pts',(-19.4869725482659,-16.3744095939248,
124.615324365784)) ;
#58610=CARTESIAN_POINT('Ctrl Pts',(-19.7677103786567,-16.5644603682351,
124.876078188685)) ;
#58611=CARTESIAN_POINT('Ctrl Pts',(-19.696026799547,-16.3844712878722,124.583223879591)) ;
#58612=CARTESIAN_POINT('Ctrl Pts',(-20.0127402827111,-16.5743048213192,
124.793052261125)) ;
#58613=CARTESIAN_POINT('Ctrl Pts',(-19.8920493950965,-16.3943157409564,
124.516802517793)) ;
#58614=CARTESIAN_POINT('Ctrl Pts',(-20.2427297441495,-16.5842655062777,
124.668092227822)) ;
#58615=CARTESIAN_POINT('Ctrl Pts',(-20.0760402661694,-16.4042764259148,
124.416833962095)) ;
#58616=CARTESIAN_POINT('Ctrl Pts',(-20.4488151079738,-16.5943014387862,
124.503505578167)) ;
#58617=CARTESIAN_POINT('Ctrl Pts',(-20.2409080798894,-16.4143123584233,
124.285163870932)) ;
#58618=CARTESIAN_POINT('Ctrl Pts',(-20.6208188759846,-16.6041900544743,
124.308721850935)) ;
#58619=CARTESIAN_POINT('Ctrl Pts',(-20.3785099279013,-16.4242009741114,
124.129336942414)) ;
#58620=CARTESIAN_POINT('Ctrl Pts',(-20.7585722335098,-16.6142044636167,
124.084465548632)) ;
#58621=CARTESIAN_POINT('Ctrl Pts',(-20.4887119985352,-16.4342153832538,
123.949931533889)) ;
#58622=CARTESIAN_POINT('Ctrl Pts',(-20.8548321532337,-16.6242382725745,
123.839003471637)) ;
#58623=CARTESIAN_POINT('Ctrl Pts',(-20.5657191556869,-16.4442491922116,
123.753561447325)) ;
#58624=CARTESIAN_POINT('Ctrl Pts',(-20.9066678159083,-16.6340687268307,
123.585891332046)) ;
#58625=CARTESIAN_POINT('Ctrl Pts',(-20.6071867566373,-16.4540796464678,
123.551072756513)) ;
#58626=CARTESIAN_POINT('Ctrl Pts',(-20.9140293672991,-16.6441463944089,
123.321214560583)) ;
#58627=CARTESIAN_POINT('Ctrl Pts',(-20.6130753215692,-16.464157314046,123.33933095717)) ;
#58628=CARTESIAN_POINT('Ctrl Pts',(-20.8763072380744,-16.6539982625311,
123.065023312876)) ;
#58629=CARTESIAN_POINT('Ctrl Pts',(-20.5828971286681,-16.4740091821683,
123.134379095039)) ;
#58630=CARTESIAN_POINT('Ctrl Pts',(-20.7930831562176,-16.6640713000965,
122.81378563807)) ;
#58631=CARTESIAN_POINT('Ctrl Pts',(-20.5163171841745,-16.4840822197336,
122.933388811495)) ;
#58632=CARTESIAN_POINT('Ctrl Pts',(-20.6703077317123,-16.6739138534474,
122.586104119148)) ;
#58633=CARTESIAN_POINT('Ctrl Pts',(-20.4180968468373,-16.4939247730845,
122.751244883158)) ;
#58634=CARTESIAN_POINT('Ctrl Pts',(-20.5083311850613,-16.6838942489408,
122.3798384328)) ;
#58635=CARTESIAN_POINT('Ctrl Pts',(-20.288515456469,-16.5039051685779,122.586232769824)) ;
#58636=CARTESIAN_POINT('Ctrl Pts',(-20.3119093379596,-16.6939127269186,
122.204541346776)) ;
#58637=CARTESIAN_POINT('Ctrl Pts',(-20.1313776273068,-16.5139236465557,
122.445995481957)) ;
#58638=CARTESIAN_POINT('Ctrl Pts',(-20.0913143430655,-16.7037960412247,
122.067389838621)) ;
#58639=CARTESIAN_POINT('Ctrl Pts',(-19.9549021776647,-16.5238069608618,
122.336275060039)) ;
#58640=CARTESIAN_POINT('Ctrl Pts',(-19.8457714437164,-16.7138643437634,
121.968950139572)) ;
#58641=CARTESIAN_POINT('Ctrl Pts',(-19.7584674011895,-16.5338752634005,
122.25752355759)) ;
#58642=CARTESIAN_POINT('Ctrl Pts',(-19.5929691002655,-16.7236943910368,
121.915607289983)) ;
#58643=CARTESIAN_POINT('Ctrl Pts',(-19.5562266645258,-16.543705310674,122.214849855465)) ;
#58644=CARTESIAN_POINT('Ctrl Pts',(-19.3286263043383,-16.7337612624523,
121.906429428325)) ;
#58645=CARTESIAN_POINT('Ctrl Pts',(-19.3447521004645,-16.5537721820895,
122.207507801228)) ;
#58646=CARTESIAN_POINT('Ctrl Pts',(-19.0712701351498,-16.7436503012514,
121.942787563624)) ;
#58647=CARTESIAN_POINT('Ctrl Pts',(-19.1388680389634,-16.5636612208885,
122.236594472759)) ;
#58648=CARTESIAN_POINT('Ctrl Pts',(-18.8213494437771,-16.7536469993855,
122.023645715726)) ;
#58649=CARTESIAN_POINT('Ctrl Pts',(-18.9389316809213,-16.5736579190226,
122.301281090436)) ;
#58650=CARTESIAN_POINT('Ctrl Pts',(-18.5903042632975,-16.7635994250975,
122.146243992672)) ;
#58651=CARTESIAN_POINT('Ctrl Pts',(-18.7540959986369,-16.5836103447346,
122.399359670759)) ;
#58652=CARTESIAN_POINT('Ctrl Pts',(-18.3840928904313,-16.7735407273304,
122.306608387421)) ;
#58653=CARTESIAN_POINT('Ctrl Pts',(-18.5891273551198,-16.5935516469676,
122.52765094837)) ;
#58654=CARTESIAN_POINT('Ctrl Pts',(-18.2078769998902,-16.7835239664143,
122.501007316772)) ;
#58655=CARTESIAN_POINT('Ctrl Pts',(-18.4481547970743,-16.6035348860515,
122.683169946801)) ;
#58656=CARTESIAN_POINT('Ctrl Pts',(-18.0676897405683,-16.7935627679829,
122.724459360897)) ;
#58657=CARTESIAN_POINT('Ctrl Pts',(-18.3360050210743,-16.6135736876201,
122.861931768501)) ;
#58658=CARTESIAN_POINT('Ctrl Pts',(-17.9698306083083,-16.8034108741046,
122.964068373402)) ;
#58659=CARTESIAN_POINT('Ctrl Pts',(-18.2577181420015,-16.6234217937417,
123.053617920861)) ;
#58660=CARTESIAN_POINT('Ctrl Pts',(-17.91365079712,-16.8134710696799,123.222378870925)) ;
#58661=CARTESIAN_POINT('Ctrl Pts',(-18.2127741641893,-16.633481989317,123.260266584404)) ;
#58662=CARTESIAN_POINT('Ctrl Pts',(-17.9035805406861,-16.8233687529913,
123.482295776231)) ;
#58663=CARTESIAN_POINT('Ctrl Pts',(-18.2047179840723,-16.6433796726285,
123.468199309359)) ;
#58664=CARTESIAN_POINT('Ctrl Pts',(-17.938061631521,-16.8332997933653,123.740980891344)) ;
#58665=CARTESIAN_POINT('Ctrl Pts',(-18.2323025565366,-16.6533107130024,
123.675146859333)) ;
#58666=CARTESIAN_POINT('Ctrl Pts',(-18.018089634645,-16.8433420110219,123.992448629415)) ;
#58667=CARTESIAN_POINT('Ctrl Pts',(-18.2963248642871,-16.6633529306591,
123.876321254892)) ;
#58668=CARTESIAN_POINT('Ctrl Pts',(-18.1385099721154,-16.8532286717559,
124.222681786331)) ;
#58669=CARTESIAN_POINT('Ctrl Pts',(-18.3926605542748,-16.673239591393,124.06050710284)) ;
#58670=CARTESIAN_POINT('Ctrl Pts',(-18.2984195187527,-16.8632217803584,
124.430972590157)) ;
#58671=CARTESIAN_POINT('Ctrl Pts',(-18.5205878453715,-16.6832326999955,
124.227139806063)) ;
#58672=CARTESIAN_POINT('Ctrl Pts',(-18.4912243940808,-16.8731674789966,
124.607428923697)) ;
#58673=CARTESIAN_POINT('Ctrl Pts',(-18.6748312019824,-16.6931783986337,
124.368304761902)) ;
#58674=CARTESIAN_POINT('Ctrl Pts',(-18.7114963548054,-16.8831147012677,
124.748207213336)) ;
#58675=CARTESIAN_POINT('Ctrl Pts',(-18.8510481570175,-16.7031256209048,
124.480927500203)) ;
#58676=CARTESIAN_POINT('Ctrl Pts',(-18.9554062189626,-16.8931627268478,
124.849334419905)) ;
#58677=CARTESIAN_POINT('Ctrl Pts',(-19.0461761012947,-16.7131736464849,
124.561829660936)) ;
#58678=CARTESIAN_POINT('Ctrl Pts',(-19.2079801341472,-16.9030099739907,
124.905647599935)) ;
#58679=CARTESIAN_POINT('Ctrl Pts',(-19.2482340537887,-16.7230208936278,
124.606880351078)) ;
#58680=CARTESIAN_POINT('Ctrl Pts',(-19.4694948938835,-16.9129731510814,
124.918213293)) ;
#58681=CARTESIAN_POINT('Ctrl Pts',(-19.4574454686167,-16.7329840707186,
124.616933496724)) ;
#58682=CARTESIAN_POINT('Ctrl Pts',(-19.7309060814548,-16.9230028721148,
124.884564981777)) ;
#58683=CARTESIAN_POINT('Ctrl Pts',(-19.6665745634729,-16.743013791752,124.590015342495)) ;
#58684=CARTESIAN_POINT('Ctrl Pts',(-19.9794823375165,-16.9329073396477,
124.807315146919)) ;
#58685=CARTESIAN_POINT('Ctrl Pts',(-19.8654350540059,-16.7529182592849,
124.528216247189)) ;
#58686=CARTESIAN_POINT('Ctrl Pts',(-20.2136657521584,-16.9429318254775,
124.686737651366)) ;
#58687=CARTESIAN_POINT('Ctrl Pts',(-20.0527821064406,-16.7629427451146,
124.431754771356)) ;
#58688=CARTESIAN_POINT('Ctrl Pts',(-20.421015963903,-16.9528356606014,124.529379524787)) ;
#58689=CARTESIAN_POINT('Ctrl Pts',(-20.2186620983548,-16.7728465802385,
124.305869231909)) ;
#58690=CARTESIAN_POINT('Ctrl Pts',(-20.6005228715144,-16.9628868513114,
124.335656354932)) ;
#58691=CARTESIAN_POINT('Ctrl Pts',(-20.3622682531827,-16.7828977709485,
124.150891007985)) ;
#58692=CARTESIAN_POINT('Ctrl Pts',(-20.7413629698391,-16.9727712939697,
124.117369250282)) ;
#58693=CARTESIAN_POINT('Ctrl Pts',(-20.4749404514896,-16.7927822136068,
123.976262404854)) ;
#58694=CARTESIAN_POINT('Ctrl Pts',(-20.8436992076654,-16.9827643018216,
123.875549411217)) ;
#58695=CARTESIAN_POINT('Ctrl Pts',(-20.5568101194757,-16.8027752214587,
123.782806994121)) ;
#58696=CARTESIAN_POINT('Ctrl Pts',(-20.9021522987122,-16.9927126215379,
123.62071892228)) ;
#58697=CARTESIAN_POINT('Ctrl Pts',(-20.6035732565573,-16.812723541175,123.578943200647)) ;
#58698=CARTESIAN_POINT('Ctrl Pts',(-20.9158262169464,-17.0026494602473,
123.359970070186)) ;
#58699=CARTESIAN_POINT('Ctrl Pts',(-20.6145132340894,-16.8226603798844,
123.370344673644)) ;
#58700=CARTESIAN_POINT('Ctrl Pts',(-20.884191716522,-17.0126324491669,123.099507780396)) ;
#58701=CARTESIAN_POINT('Ctrl Pts',(-20.5892065993372,-16.832643368804,123.161974931273)) ;
#58702=CARTESIAN_POINT('Ctrl Pts',(-20.8069010684721,-17.022676328531,122.84716775239)) ;
#58703=CARTESIAN_POINT('Ctrl Pts',(-20.5273748335759,-16.8426872481681,
122.960102519886)) ;
#58704=CARTESIAN_POINT('Ctrl Pts',(-20.6900614936507,-17.0325043938894,
122.616789554295)) ;
#58705=CARTESIAN_POINT('Ctrl Pts',(-20.4339045684967,-16.8525153135265,
122.775800548252)) ;
#58706=CARTESIAN_POINT('Ctrl Pts',(-20.5312178370155,-17.0425814824443,
122.404977090048)) ;
#58707=CARTESIAN_POINT('Ctrl Pts',(-20.306830239219,-16.8625924020815,122.606349695402)) ;
#58708=CARTESIAN_POINT('Ctrl Pts',(-20.3423853676555,-17.0524316346006,
122.227828485222)) ;
#58709=CARTESIAN_POINT('Ctrl Pts',(-20.1557657033809,-16.8724425542378,
122.464630732549)) ;
#58710=CARTESIAN_POINT('Ctrl Pts',(-20.1207672096215,-17.062512115053,122.082830799905)) ;
#58711=CARTESIAN_POINT('Ctrl Pts',(-19.9784714607027,-16.8825230346901,
122.348631493821)) ;
#58712=CARTESIAN_POINT('Ctrl Pts',(-19.883737034747,-17.0723266128218,121.981011738217)) ;
#58713=CARTESIAN_POINT('Ctrl Pts',(-19.7888488634291,-16.8923375324589,
122.267175689381)) ;
#58714=CARTESIAN_POINT('Ctrl Pts',(-19.6263495978592,-17.0823949088419,
121.919989507403)) ;
#58715=CARTESIAN_POINT('Ctrl Pts',(-19.5829389187349,-16.9024058284791,
122.218356659132)) ;
#58716=CARTESIAN_POINT('Ctrl Pts',(-19.3665898868783,-17.0922937413247,
121.904909547411)) ;
#58717=CARTESIAN_POINT('Ctrl Pts',(-19.3751318865944,-16.9123046609618,
122.206291541471)) ;
#58718=CARTESIAN_POINT('Ctrl Pts',(-19.1042454569356,-17.1023466213392,
121.935528536243)) ;
#58719=CARTESIAN_POINT('Ctrl Pts',(-19.1652560101051,-16.9223575409764,
122.230785548798)) ;
#58720=CARTESIAN_POINT('Ctrl Pts',(-18.855638307516,-17.1122164368354,122.009652399298)) ;
#58721=CARTESIAN_POINT('Ctrl Pts',(-18.9663707255866,-16.9322273564725,
122.29008319219)) ;
#58722=CARTESIAN_POINT('Ctrl Pts',(-18.6189668205951,-17.1222891179182,
122.128093849741)) ;
#58723=CARTESIAN_POINT('Ctrl Pts',(-18.7770327094499,-16.9423000375553,
122.384835334691)) ;
#58724=CARTESIAN_POINT('Ctrl Pts',(-18.4114058096886,-17.1321215964892,
122.282028735497)) ;
#58725=CARTESIAN_POINT('Ctrl Pts',(-18.6109839479363,-16.9521325161263,
122.507981587497)) ;
#58726=CARTESIAN_POINT('Ctrl Pts',(-18.2296195608768,-17.1421522304753,
122.472896223419)) ;
#58727=CARTESIAN_POINT('Ctrl Pts',(-18.4655538438899,-16.9621631501124,
122.660674621782)) ;
#58728=CARTESIAN_POINT('Ctrl Pts',(-18.0843508674256,-17.1521837876944,
122.692895741896)) ;
#58729=CARTESIAN_POINT('Ctrl Pts',(-18.3493377687508,-16.9721947073315,
122.836673575722)) ;
#58730=CARTESIAN_POINT('Ctrl Pts',(-17.9811153912308,-17.1620134965661,
122.92966578504)) ;
#58731=CARTESIAN_POINT('Ctrl Pts',(-18.2667484984008,-16.9820244162032,
123.026088115789)) ;
#58732=CARTESIAN_POINT('Ctrl Pts',(-17.9188078334472,-17.1720029453682,
123.184684449035)) ;
#58733=CARTESIAN_POINT('Ctrl Pts',(-18.2169009623757,-16.9920138650053,
123.230102537214)) ;
#58734=CARTESIAN_POINT('Ctrl Pts',(-17.9023020185663,-17.1820467977682,
123.44810689289)) ;
#58735=CARTESIAN_POINT('Ctrl Pts',(-18.2036948702119,-17.0020577174053,
123.440840520039)) ;
#58736=CARTESIAN_POINT('Ctrl Pts',(-17.9306034522518,-17.1918685111003,
123.704655127921)) ;
#58737=CARTESIAN_POINT('Ctrl Pts',(-18.2263343758186,-17.0118794307374,
123.646078286481)) ;
#58738=CARTESIAN_POINT('Ctrl Pts',(-18.0039709952741,-17.201903516089,123.957951976954)) ;
#58739=CARTESIAN_POINT('Ctrl Pts',(-18.2850268365724,-17.0219144357261,
123.848716309395)) ;
#58740=CARTESIAN_POINT('Ctrl Pts',(-18.1207470223198,-17.2119283545366,
124.194108297233)) ;
#58741=CARTESIAN_POINT('Ctrl Pts',(-18.3784462993163,-17.0319392741737,
124.03764205884)) ;
#58742=CARTESIAN_POINT('Ctrl Pts',(-18.2736158124755,-17.2217805674918,
124.40306698223)) ;
#58743=CARTESIAN_POINT('Ctrl Pts',(-18.5007395422443,-17.0417914871289,
124.204809319358)) ;
#58744=CARTESIAN_POINT('Ctrl Pts',(-18.4627330156681,-17.2317705236856,
124.585121418507)) ;
#58745=CARTESIAN_POINT('Ctrl Pts',(-18.6520320121567,-17.0517814433227,
124.350453999726)) ;
#58746=CARTESIAN_POINT('Ctrl Pts',(-18.6792511906987,-17.2416986339689,
124.730700896654)) ;
#58747=CARTESIAN_POINT('Ctrl Pts',(-18.8252452509934,-17.061709553606,124.466918770551)) ;
#58748=CARTESIAN_POINT('Ctrl Pts',(-18.9190395513556,-17.2516872340484,
124.837500135833)) ;
#58749=CARTESIAN_POINT('Ctrl Pts',(-19.0170750943207,-17.0716981536855,
124.552359735373)) ;
#58750=CARTESIAN_POINT('Ctrl Pts',(-19.174783750514,-17.2617138259759,124.900929840425)) ;
#58751=CARTESIAN_POINT('Ctrl Pts',(-19.2216700660752,-17.081724745613,124.603105176145)) ;
#58752=CARTESIAN_POINT('Ctrl Pts',(-19.4339184087845,-17.2715989540401,
124.919007255833)) ;
#58753=CARTESIAN_POINT('Ctrl Pts',(-19.4289770822547,-17.0916098736772,
124.617568828664)) ;
#58754=CARTESIAN_POINT('Ctrl Pts',(-19.6951036459662,-17.2815900715136,
124.892117022616)) ;
#58755=CARTESIAN_POINT('Ctrl Pts',(-19.6379253382598,-17.1016009911507,
124.596058506662)) ;
#58756=CARTESIAN_POINT('Ctrl Pts',(-19.9487403100385,-17.2916306873654,
124.819396962872)) ;
#58757=CARTESIAN_POINT('Ctrl Pts',(-19.8408352281527,-17.1116416070025,
124.537884144439)) ;
#58758=CARTESIAN_POINT('Ctrl Pts',(-20.1811784262085,-17.3014636782191,
124.706518373388)) ;
#58759=CARTESIAN_POINT('Ctrl Pts',(-20.0267858395131,-17.1214745978562,
124.447583262725)) ;
#58760=CARTESIAN_POINT('Ctrl Pts',(-20.3943355471498,-17.3114568096694,
124.553138757061)) ;
#58761=CARTESIAN_POINT('Ctrl Pts',(-20.1973125961385,-17.1314677293065,
124.324881214405)) ;
#58762=CARTESIAN_POINT('Ctrl Pts',(-20.5779551582987,-17.3214888581048,
124.36395098382)) ;
#58763=CARTESIAN_POINT('Ctrl Pts',(-20.3442096485662,-17.1414997777419,
124.17353227877)) ;
#58764=CARTESIAN_POINT('Ctrl Pts',(-20.7237261254064,-17.3313541046472,
124.149582721403)) ;
#58765=CARTESIAN_POINT('Ctrl Pts',(-20.4608276825751,-17.1513650242843,
124.002039230348)) ;
#58766=CARTESIAN_POINT('Ctrl Pts',(-20.831788362086,-17.341315979474,123.911130472896)) ;
#58767=CARTESIAN_POINT('Ctrl Pts',(-20.5472792280348,-17.1613268991111,
123.811278448521)) ;
#58768=CARTESIAN_POINT('Ctrl Pts',(-20.8968589917748,-17.3513509425853,
123.655591647109)) ;
#58769=CARTESIAN_POINT('Ctrl Pts',(-20.5993376400282,-17.1713618622224,
123.606847845879)) ;
#58770=CARTESIAN_POINT('Ctrl Pts',(-20.9167197829666,-17.3612357870477,
123.396550342786)) ;
#58771=CARTESIAN_POINT('Ctrl Pts',(-20.6152282496205,-17.1812467066848,
123.399615406321)) ;
#58772=CARTESIAN_POINT('Ctrl Pts',(-20.8907754476135,-17.3713018398884,
123.133346946234)) ;
#58773=CARTESIAN_POINT('Ctrl Pts',(-20.5944747717883,-17.1913127595256,
123.189052373295)) ;
#58774=CARTESIAN_POINT('Ctrl Pts',(-20.8213961192781,-17.3811393557974,
122.88426085308)) ;
#58775=CARTESIAN_POINT('Ctrl Pts',(-20.5389734280671,-17.2011502754345,
122.989783496606)) ;
#58776=CARTESIAN_POINT('Ctrl Pts',(-20.7074934610674,-17.3912081039063,
122.645486865945)) ;
#58777=CARTESIAN_POINT('Ctrl Pts',(-20.4478531284103,-17.2112190235434,
122.798763308908)) ;
#58778=CARTESIAN_POINT('Ctrl Pts',(-20.5566061673441,-17.4010886209373,
122.434129920283)) ;
#58779=CARTESIAN_POINT('Ctrl Pts',(-20.3271452112243,-17.2210995405744,
122.629676886925)) ;
#58780=CARTESIAN_POINT('Ctrl Pts',(-20.3696663136538,-17.4110798078718,
122.249820531952)) ;
#58781=CARTESIAN_POINT('Ctrl Pts',(-20.1775948836073,-17.2310907275089,
122.482227931951)) ;
#58782=CARTESIAN_POINT('Ctrl Pts',(-20.1543475643769,-17.4210328741467,
122.101259878823)) ;
#58783=CARTESIAN_POINT('Ctrl Pts',(-20.0053412412653,-17.2410437937838,
122.363377768744)) ;
#58784=CARTESIAN_POINT('Ctrl Pts',(-19.9145466995836,-17.4310687116793,
121.991540433781)) ;
#58785=CARTESIAN_POINT('Ctrl Pts',(-19.8135014215866,-17.2510796313164,
122.275600286841)) ;
#58786=CARTESIAN_POINT('Ctrl Pts',(-19.6630503154042,-17.4409588378907,
121.925907930665)) ;
#58787=CARTESIAN_POINT('Ctrl Pts',(-19.6123051763993,-17.2609697575279,
122.223092308256)) ;
#58788=CARTESIAN_POINT('Ctrl Pts',(-19.4013697921715,-17.4509510197987,
121.904306259386)) ;
#58789=CARTESIAN_POINT('Ctrl Pts',(-19.4029610196723,-17.2709619394358,
122.205808818119)) ;
#58790=CARTESIAN_POINT('Ctrl Pts',(-19.1411178680801,-17.4608969597373,
121.928446401877)) ;
#58791=CARTESIAN_POINT('Ctrl Pts',(-19.1947594651076,-17.2809078793744,
122.22511876556)) ;
#58792=CARTESIAN_POINT('Ctrl Pts',(-18.88882641169,-17.4708441435014,121.996908692805)) ;
#58793=CARTESIAN_POINT('Ctrl Pts',(-18.9929258788226,-17.2908550631385,
122.279886435726)) ;
#58794=CARTESIAN_POINT('Ctrl Pts',(-18.6500049664529,-17.4808920818088,
122.109521528359)) ;
#58795=CARTESIAN_POINT('Ctrl Pts',(-18.8018677870459,-17.300903001446,122.369974738324)) ;
#58796=CARTESIAN_POINT('Ctrl Pts',(-18.4385276907917,-17.4907397165491,
122.258681232222)) ;
#58797=CARTESIAN_POINT('Ctrl Pts',(-18.6326849625005,-17.3107506361862,
122.489300526383)) ;
#58798=CARTESIAN_POINT('Ctrl Pts',(-18.2534782916843,-17.5007014305229,
122.443832320291)) ;
#58799=CARTESIAN_POINT('Ctrl Pts',(-18.4846439297647,-17.3207123501601,
122.637419744003)) ;
#58800=CARTESIAN_POINT('Ctrl Pts',(-18.1026371828242,-17.5107300653138,
122.659957308441)) ;
#58801=CARTESIAN_POINT('Ctrl Pts',(-18.3639692439427,-17.3307409849509,
122.810318436287)) ;
#58802=CARTESIAN_POINT('Ctrl Pts',(-17.9928588043532,-17.5206403839109,
122.896109111999)) ;
#58803=CARTESIAN_POINT('Ctrl Pts',(-18.2761445935121,-17.340651303548,122.999238788582)) ;
#58804=CARTESIAN_POINT('Ctrl Pts',(-17.9249170447996,-17.5305752402224,
123.148201377917)) ;
#58805=CARTESIAN_POINT('Ctrl Pts',(-18.2217890416061,-17.3505861598595,
123.200911914671)) ;
#58806=CARTESIAN_POINT('Ctrl Pts',(-17.9017863181592,-17.5406164761831,
123.41104640664)) ;
#58807=CARTESIAN_POINT('Ctrl Pts',(-18.2032822312824,-17.3606273958202,
123.411187703811)) ;
#58808=CARTESIAN_POINT('Ctrl Pts',(-17.9240826085059,-17.5505032477631,
123.669927416836)) ;
#58809=CARTESIAN_POINT('Ctrl Pts',(-18.221117014871,-17.3705141674002,123.618292577988)) ;
#58810=CARTESIAN_POINT('Ctrl Pts',(-17.991434789336,-17.5605034264693,123.923904177985)) ;
#58811=CARTESIAN_POINT('Ctrl Pts',(-18.274996565428,-17.3805143461064,123.821474510317)) ;
#58812=CARTESIAN_POINT('Ctrl Pts',(-18.1007768933539,-17.5704207046789,
124.160520976212)) ;
#58813=CARTESIAN_POINT('Ctrl Pts',(-18.3624681751621,-17.390431624316,124.010768829435)) ;
#58814=CARTESIAN_POINT('Ctrl Pts',(-18.2515125585857,-17.5804679510926,
124.377250917313)) ;
#58815=CARTESIAN_POINT('Ctrl Pts',(-18.4830548228013,-17.4004788707297,
124.184154022707)) ;
#58816=CARTESIAN_POINT('Ctrl Pts',(-18.4342365122274,-17.5903418400739,
124.561534748343)) ;
#58817=CARTESIAN_POINT('Ctrl Pts',(-18.6292323540018,-17.410352759711,124.331582640151)) ;
#58818=CARTESIAN_POINT('Ctrl Pts',(-18.6500768441802,-17.6004038576544,
124.714221581004)) ;
#58819=CARTESIAN_POINT('Ctrl Pts',(-18.8019032612626,-17.4204147772915,
124.453733907963)) ;
#58820=CARTESIAN_POINT('Ctrl Pts',(-18.8846741125319,-17.6102749193887,
124.82495821564)) ;
#58821=CARTESIAN_POINT('Ctrl Pts',(-18.9895801047362,-17.4302858390258,
124.542325248395)) ;
#58822=CARTESIAN_POINT('Ctrl Pts',(-19.1378416764729,-17.620268982749,124.894832090563)) ;
#58823=CARTESIAN_POINT('Ctrl Pts',(-19.1921135246435,-17.4402799023861,
124.598226499213)) ;
#58824=CARTESIAN_POINT('Ctrl Pts',(-19.4003404043878,-17.6303011407824,
124.919197850728)) ;
#58825=CARTESIAN_POINT('Ctrl Pts',(-19.4021122156701,-17.4503120604195,
124.617721341599)) ;
#58826=CARTESIAN_POINT('Ctrl Pts',(-19.6587556166457,-17.6401650170226,
124.898540308878)) ;
#58827=CARTESIAN_POINT('Ctrl Pts',(-19.6088446217045,-17.4601759366597,
124.601197540958)) ;
#58828=CARTESIAN_POINT('Ctrl Pts',(-19.9148657636072,-17.6502355316608,
124.832005118292)) ;
#58829=CARTESIAN_POINT('Ctrl Pts',(-19.8137332138143,-17.470246451298,124.54797155282)) ;
#58830=CARTESIAN_POINT('Ctrl Pts',(-20.150095477634,-17.6600761686018,124.724523892798)) ;
#58831=CARTESIAN_POINT('Ctrl Pts',(-20.0019179240621,-17.4800870882389,
124.461988673264)) ;
#58832=CARTESIAN_POINT('Ctrl Pts',(-20.3662817216806,-17.670043297442,124.576684081866)) ;
#58833=CARTESIAN_POINT('Ctrl Pts',(-20.1748686108959,-17.4900542170791,
124.343718154926)) ;
#58834=CARTESIAN_POINT('Ctrl Pts',(-20.5542290543161,-17.6800572705665,
124.392466662647)) ;
#58835=CARTESIAN_POINT('Ctrl Pts',(-20.3252263581462,-17.5000681902037,
124.196347578167)) ;
#58836=CARTESIAN_POINT('Ctrl Pts',(-20.7574242465171,-17.6933420044298,
124.108563216833)) ;
#58837=CARTESIAN_POINT('Ctrl Pts',(-20.487792909875,-17.5133529240669,123.969217895372)) ;
#58838=CARTESIAN_POINT('Ctrl Pts',(-20.8815792327918,-17.7065672691446,
123.779776387227)) ;
#58839=CARTESIAN_POINT('Ctrl Pts',(-20.5871211385938,-17.5265781887817,
123.706157444669)) ;
#58840=CARTESIAN_POINT('Ctrl Pts',(-20.9167156267444,-17.7198777916994,
123.431719811702)) ;
#58841=CARTESIAN_POINT('Ctrl Pts',(-20.6152233992077,-17.5398887113366,
123.427758937628)) ;
#58842=CARTESIAN_POINT('Ctrl Pts',(-20.8970403045933,-17.7299064366016,
123.168922156233)) ;
#58843=CARTESIAN_POINT('Ctrl Pts',(-20.599487173877,-17.5499173562387,123.217511388876)) ;
#58844=CARTESIAN_POINT('Ctrl Pts',(-20.833211337434,-17.7397874689555,122.917220164191)) ;
#58845=CARTESIAN_POINT('Ctrl Pts',(-20.5484257925112,-17.5597983885926,
123.016151680332)) ;
#58846=CARTESIAN_POINT('Ctrl Pts',(-20.7260717926928,-17.7497684416356,
122.677813694401)) ;
#58847=CARTESIAN_POINT('Ctrl Pts',(-20.4627150058846,-17.5697793612727,
122.824624299976)) ;
#58848=CARTESIAN_POINT('Ctrl Pts',(-20.5788081877206,-17.7597495692216,
122.460780265078)) ;
#58849=CARTESIAN_POINT('Ctrl Pts',(-20.3449101987234,-17.5797604888587,
122.650998991699)) ;
#58850=CARTESIAN_POINT('Ctrl Pts',(-20.3368568947388,-17.772992759483,122.21053545582)) ;
#58851=CARTESIAN_POINT('Ctrl Pts',(-20.1513291199415,-17.5930036791201,
122.450788794857)) ;
#58852=CARTESIAN_POINT('Ctrl Pts',(-19.9569936985326,-17.7896607548438,
121.982786748505)) ;
#58853=CARTESIAN_POINT('Ctrl Pts',(-19.8474794990023,-17.6096716744809,
122.26860190868)) ;
#58854=CARTESIAN_POINT('Ctrl Pts',(-19.5259606159641,-17.8061812548558,
121.898720902141)) ;
#58855=CARTESIAN_POINT('Ctrl Pts',(-19.5025885463891,-17.626192174493,122.201337274905)) ;
#58856=CARTESIAN_POINT('Ctrl Pts',(-19.1769501917683,-17.8194942711718,
121.922374301912)) ;
#58857=CARTESIAN_POINT('Ctrl Pts',(-19.2234321602598,-17.639505190809,122.220261939682)) ;
#58858=CARTESIAN_POINT('Ctrl Pts',(-18.9238414463951,-17.8294108294048,
121.984571342196)) ;
#58859=CARTESIAN_POINT('Ctrl Pts',(-19.0209334397387,-17.649421749042,122.270017435273)) ;
#58860=CARTESIAN_POINT('Ctrl Pts',(-18.6828367951169,-17.8394384977077,
122.090994480729)) ;
#58861=CARTESIAN_POINT('Ctrl Pts',(-18.8281336451652,-17.6594494173448,
122.355152451845)) ;
#58862=CARTESIAN_POINT('Ctrl Pts',(-18.394515897223,-17.8526190874524,122.283176068422)) ;
#58863=CARTESIAN_POINT('Ctrl Pts',(-18.5974653676165,-17.6726300070895,
122.50890583314)) ;
#58864=CARTESIAN_POINT('Ctrl Pts',(-18.1010163558912,-17.8693672265717,
122.617564692546)) ;
#58865=CARTESIAN_POINT('Ctrl Pts',(-18.3626740164398,-17.6893781462089,
122.776403445059)) ;
#58866=CARTESIAN_POINT('Ctrl Pts',(-17.909361184572,-17.8891619690823,123.107788785577)) ;
#58867=CARTESIAN_POINT('Ctrl Pts',(-18.2093429356618,-17.7091728887194,
123.168586034307)) ;
#58868=CARTESIAN_POINT('Ctrl Pts',(-17.8958042831171,-17.9092063618911,
123.640179567808)) ;
#58869=CARTESIAN_POINT('Ctrl Pts',(-18.198495043607,-17.7292172815282,123.594497346099)) ;
#58870=CARTESIAN_POINT('Ctrl Pts',(-18.0635490482974,-17.9290455441898,
124.140228438831)) ;
#58871=CARTESIAN_POINT('Ctrl Pts',(-18.3326878464618,-17.7490564638269,
123.994538700796)) ;
#58872=CARTESIAN_POINT('Ctrl Pts',(-18.3920994920008,-17.9489708678827,
124.555410464658)) ;
#58873=CARTESIAN_POINT('Ctrl Pts',(-18.5955264281991,-17.7689817875198,
124.3266864764)) ;
#58874=CARTESIAN_POINT('Ctrl Pts',(-18.842788696369,-17.9688945059342,124.833584548175)) ;
#58875=CARTESIAN_POINT('Ctrl Pts',(-18.9560768416233,-17.7889054255713,
124.549228339882)) ;
#58876=CARTESIAN_POINT('Ctrl Pts',(-19.3612051307133,-17.9888193793997,
124.941403037166)) ;
#58877=CARTESIAN_POINT('Ctrl Pts',(-19.3708100925674,-17.8088302990368,
124.635485728076)) ;
#58878=CARTESIAN_POINT('Ctrl Pts',(-19.8842672961237,-18.0086979864787,
124.866686275026)) ;
#58879=CARTESIAN_POINT('Ctrl Pts',(-19.7892612316858,-17.8287089061158,
124.575714277679)) ;
#58880=CARTESIAN_POINT('Ctrl Pts',(-20.3528378762813,-18.0286754293106,
124.616972672775)) ;
#58881=CARTESIAN_POINT('Ctrl Pts',(-20.1641187657695,-17.8486863489478,
124.375944971353)) ;
#58882=CARTESIAN_POINT('Ctrl Pts',(-20.7070199751766,-18.0486072773953,
124.222957551387)) ;
#58883=CARTESIAN_POINT('Ctrl Pts',(-20.4474662649599,-17.8686181970324,
124.060733674475)) ;
#58884=CARTESIAN_POINT('Ctrl Pts',(-20.9055702118375,-18.0685025457379,
123.732901280458)) ;
#58885=CARTESIAN_POINT('Ctrl Pts',(-20.6063082810486,-17.888513465375,123.668688213802)) ;
#58886=CARTESIAN_POINT('Ctrl Pts',(-20.9255908588565,-18.08842504415,123.203759760806)) ;
#58887=CARTESIAN_POINT('Ctrl Pts',(-20.622325941902,-17.9084359637871,123.245374181992)) ;
#58888=CARTESIAN_POINT('Ctrl Pts',(-20.7634037510858,-18.108384526026,122.69863823452)) ;
#58889=CARTESIAN_POINT('Ctrl Pts',(-20.4925770626071,-17.9283954456631,
122.84127622867)) ;
#58890=CARTESIAN_POINT('Ctrl Pts',(-20.4400561873198,-18.1282622784854,
122.280931726728)) ;
#58891=CARTESIAN_POINT('Ctrl Pts',(-20.2338986900793,-17.9482731981225,
122.507109352624)) ;
#58892=CARTESIAN_POINT('Ctrl Pts',(-19.9941357017279,-18.1481440692199,
121.997211525704)) ;
#58893=CARTESIAN_POINT('Ctrl Pts',(-19.8771609449229,-17.9681549888571,
122.280132520306)) ;
#58894=CARTESIAN_POINT('Ctrl Pts',(-19.473136676439,-18.1682174080709,121.882665391242)) ;
#58895=CARTESIAN_POINT('Ctrl Pts',(-19.4603626713499,-17.988228327708,122.188495684092)) ;
#58896=CARTESIAN_POINT('Ctrl Pts',(-18.9512092802025,-18.1880218753067,
121.951729931367)) ;
#58897=CARTESIAN_POINT('Ctrl Pts',(-19.0428183076886,-18.0080327949438,
122.243747774639)) ;
#58898=CARTESIAN_POINT('Ctrl Pts',(-18.4795781028299,-18.2080052157145,
122.195819043251)) ;
#58899=CARTESIAN_POINT('Ctrl Pts',(-18.665513625463,-18.0280161353516,122.43901994105)) ;
#58900=CARTESIAN_POINT('Ctrl Pts',(-18.1213593079001,-18.2279201803125,
122.585493056781)) ;
#58901=CARTESIAN_POINT('Ctrl Pts',(-18.3789384269809,-18.0479310999496,
122.750760357878)) ;
#58902=CARTESIAN_POINT('Ctrl Pts',(-17.9166900271828,-18.2477887150289,
123.072398846961)) ;
#58903=CARTESIAN_POINT('Ctrl Pts',(-18.2152038535447,-18.067799634666,123.140286849332)) ;
#58904=CARTESIAN_POINT('Ctrl Pts',(-17.891096129626,-18.2678410992406,123.604588275985)) ;
#58905=CARTESIAN_POINT('Ctrl Pts',(-18.1947300898754,-18.0878520188777,
123.566037963837)) ;
#58906=CARTESIAN_POINT('Ctrl Pts',(-18.0458895721995,-18.2876150630298,
124.107054946119)) ;
#58907=CARTESIAN_POINT('Ctrl Pts',(-18.3185671783008,-18.1076259826669,
123.968012895512)) ;
#58908=CARTESIAN_POINT('Ctrl Pts',(-18.3667637788578,-18.3076694420512,
124.53239666562)) ;
#58909=CARTESIAN_POINT('Ctrl Pts',(-18.5752679245152,-18.1276803616883,
124.308284615384)) ;
#58910=CARTESIAN_POINT('Ctrl Pts',(-18.8082021318572,-18.3274661796244,
124.819004328744)) ;
#58911=CARTESIAN_POINT('Ctrl Pts',(-18.9284212935939,-18.1474770992615,
124.537569929665)) ;
#58912=CARTESIAN_POINT('Ctrl Pts',(-19.3247749684746,-18.3474339919759,
124.940168786496)) ;
#58913=CARTESIAN_POINT('Ctrl Pts',(-19.3416804332519,-18.167444911613,124.634498827263)) ;
#58914=CARTESIAN_POINT('Ctrl Pts',(-19.8515753099783,-18.3673929680409,
124.876958419446)) ;
#58915=CARTESIAN_POINT('Ctrl Pts',(-19.7631206608013,-18.187403887678,124.583927892231)) ;
#58916=CARTESIAN_POINT('Ctrl Pts',(-20.323705737491,-18.3872878863183,124.638896796326)) ;
#58917=CARTESIAN_POINT('Ctrl Pts',(-20.140824401647,-18.2072988059554,124.393475677266)) ;
#58918=CARTESIAN_POINT('Ctrl Pts',(-20.6867396805035,-18.4071841987686,
124.254454112951)) ;
#58919=CARTESIAN_POINT('Ctrl Pts',(-20.4312497270068,-18.2271951184057,
124.085918852288)) ;
#58920=CARTESIAN_POINT('Ctrl Pts',(-20.8974889909594,-18.4270921321427,
123.769075405427)) ;
#58921=CARTESIAN_POINT('Ctrl Pts',(-20.5998462757639,-18.2471030517799,
123.697614033343)) ;
#58922=CARTESIAN_POINT('Ctrl Pts',(-20.9299591274622,-18.4470420224312,
123.239880881336)) ;
#58923=CARTESIAN_POINT('Ctrl Pts',(-20.6258188645366,-18.2670529420683,
123.274257946613)) ;
#58924=CARTESIAN_POINT('Ctrl Pts',(-20.7809301918273,-18.4669192529325,
122.732978965387)) ;
#58925=CARTESIAN_POINT('Ctrl Pts',(-20.5065921666265,-18.2869301725696,
122.868736840689)) ;
#58926=CARTESIAN_POINT('Ctrl Pts',(-20.4664719534886,-18.4869019218035,
122.305004321908)) ;
#58927=CARTESIAN_POINT('Ctrl Pts',(-20.2550218602243,-18.3069128414406,
122.526359509871)) ;
#58928=CARTESIAN_POINT('Ctrl Pts',(-20.0256670326121,-18.5068348083839,
122.011010324086)) ;
#58929=CARTESIAN_POINT('Ctrl Pts',(-19.9023778434081,-18.326845728021,122.291166823134)) ;
#58930=CARTESIAN_POINT('Ctrl Pts',(-19.5117084694408,-18.5267475544018,
121.884894904274)) ;
#58931=CARTESIAN_POINT('Ctrl Pts',(-19.4912012916676,-18.3467584740389,
122.190280271835)) ;
#58932=CARTESIAN_POINT('Ctrl Pts',(-19.0738118336098,-18.5433172757436,
121.93169130508)) ;
#58933=CARTESIAN_POINT('Ctrl Pts',(-19.140910274212,-18.3633281953808,122.227714621675)) ;
#58934=CARTESIAN_POINT('Ctrl Pts',(-18.7476501460358,-18.5566172870486,
122.057314468906)) ;
#58935=CARTESIAN_POINT('Ctrl Pts',(-18.8799531105504,-18.3766282066857,
122.32822609425)) ;
#58936=CARTESIAN_POINT('Ctrl Pts',(-18.4486656986035,-18.5698874747985,
122.23684236878)) ;
#58937=CARTESIAN_POINT('Ctrl Pts',(-18.6408115504094,-18.3898983944356,
122.471815668889)) ;
#58938=CARTESIAN_POINT('Ctrl Pts',(-18.1413722273347,-18.5865148571639,
122.554451895096)) ;
#58939=CARTESIAN_POINT('Ctrl Pts',(-18.3949285205775,-18.406525776801,122.72595265338)) ;
#58940=CARTESIAN_POINT('Ctrl Pts',(-17.9611265356219,-18.6031371469091,
122.957810899862)) ;
#58941=CARTESIAN_POINT('Ctrl Pts',(-18.2507608262965,-18.4231480665462,
123.048601618741)) ;
#58942=CARTESIAN_POINT('Ctrl Pts',(-17.9059528961361,-18.6163823613036,
123.301475150408)) ;
#58943=CARTESIAN_POINT('Ctrl Pts',(-18.2066124741129,-18.4363932809408,
123.323560293853)) ;
#58944=CARTESIAN_POINT('Ctrl Pts',(-17.9091768534027,-18.6262943262643,
123.561948497621)) ;
#58945=CARTESIAN_POINT('Ctrl Pts',(-18.2091963170387,-18.4463052459014,
123.53193369723)) ;
#58946=CARTESIAN_POINT('Ctrl Pts',(-17.9585883655337,-18.6363529494288,
123.821589557109)) ;
#58947=CARTESIAN_POINT('Ctrl Pts',(-18.2487269958253,-18.4563638690659,
123.739647432984)) ;
#58948=CARTESIAN_POINT('Ctrl Pts',(-18.0499609717764,-18.6461930635446,
124.06353698501)) ;
#58949=CARTESIAN_POINT('Ctrl Pts',(-18.3218274009337,-18.4662039831817,
123.933204397028)) ;
#58950=CARTESIAN_POINT('Ctrl Pts',(-18.1847150492908,-18.6562588485022,
124.291112489594)) ;
#58951=CARTESIAN_POINT('Ctrl Pts',(-18.4296324649852,-18.4762697681393,
124.11526364337)) ;
#58952=CARTESIAN_POINT('Ctrl Pts',(-18.3539469883158,-18.6661421662901,
124.488176476276)) ;
#58953=CARTESIAN_POINT('Ctrl Pts',(-18.5650197804419,-18.4861530859272,
124.272913430482)) ;
#58954=CARTESIAN_POINT('Ctrl Pts',(-18.5565725704209,-18.6761316041487,
124.655035297587)) ;
#58955=CARTESIAN_POINT('Ctrl Pts',(-18.7271216359093,-18.4961425237858,
124.406398725453)) ;
#58956=CARTESIAN_POINT('Ctrl Pts',(-18.7845837390266,-18.6860953182014,
124.783781642268)) ;
#58957=CARTESIAN_POINT('Ctrl Pts',(-18.9095316568693,-18.5061062378385,
124.509393835218)) ;
#58958=CARTESIAN_POINT('Ctrl Pts',(-19.0321760408685,-18.6960903298606,
124.871518685265)) ;
#58959=CARTESIAN_POINT('Ctrl Pts',(-19.1076061994151,-18.5161012494978,
124.579581328801)) ;
#58960=CARTESIAN_POINT('Ctrl Pts',(-19.2923475774158,-18.7061266215549,
124.914699798494)) ;
#58961=CARTESIAN_POINT('Ctrl Pts',(-19.3157437283926,-18.526137541192,124.614123995732)) ;
#58962=CARTESIAN_POINT('Ctrl Pts',(-19.5511061455371,-18.7159729992483,
124.912522869748)) ;
#58963=CARTESIAN_POINT('Ctrl Pts',(-19.5227505956409,-18.5359839188854,
124.612380200103)) ;
#58964=CARTESIAN_POINT('Ctrl Pts',(-19.8091754394204,-18.725957943399,124.865290742735)) ;
#58965=CARTESIAN_POINT('Ctrl Pts',(-19.7292055595761,-18.5459688630361,
124.574592283995)) ;
#58966=CARTESIAN_POINT('Ctrl Pts',(-20.0540693302501,-18.735894914529,124.774521245313)) ;
#58967=CARTESIAN_POINT('Ctrl Pts',(-19.9251198339151,-18.5559058341661,
124.50197459087)) ;
#58968=CARTESIAN_POINT('Ctrl Pts',(-20.2819125648932,-18.7459446991607,
124.64102455522)) ;
#58969=CARTESIAN_POINT('Ctrl Pts',(-20.1073932380398,-18.5659556187978,
124.395175312067)) ;
#58970=CARTESIAN_POINT('Ctrl Pts',(-20.4792864441643,-18.7557951612382,
124.473508135846)) ;
#58971=CARTESIAN_POINT('Ctrl Pts',(-20.2652908081466,-18.5758060808753,
124.261160516284)) ;
#58972=CARTESIAN_POINT('Ctrl Pts',(-20.6471074503595,-18.7657671747586,
124.272284173853)) ;
#58973=CARTESIAN_POINT('Ctrl Pts',(-20.3995458257233,-18.5857780943957,
124.100179977328)) ;
#58974=CARTESIAN_POINT('Ctrl Pts',(-20.7777500986428,-18.775762321878,124.044367513356)) ;
#58975=CARTESIAN_POINT('Ctrl Pts',(-20.5040579656922,-18.5957732415151,
123.917845587999)) ;
#58976=CARTESIAN_POINT('Ctrl Pts',(-20.86685809816,-18.7857962916141,123.796222100934)) ;
#58977=CARTESIAN_POINT('Ctrl Pts',(-20.5753422305749,-18.6058072112512,
123.719328523745)) ;
#58978=CARTESIAN_POINT('Ctrl Pts',(-20.9111412970602,-18.7956518372847,
123.541018035015)) ;
#58979=CARTESIAN_POINT('Ctrl Pts',(-20.6107665482665,-18.6156627569218,
123.515165073301)) ;
#58980=CARTESIAN_POINT('Ctrl Pts',(-20.9107995971931,-18.8056505942979,
123.278303845419)) ;
#58981=CARTESIAN_POINT('Ctrl Pts',(-20.6104909554121,-18.6256615139351,
123.304993798075)) ;
#58982=CARTESIAN_POINT('Ctrl Pts',(-20.8655454311932,-18.8155477295351,
123.022145216685)) ;
#58983=CARTESIAN_POINT('Ctrl Pts',(-20.5742854776814,-18.6355586491722,
123.100067482626)) ;
#58984=CARTESIAN_POINT('Ctrl Pts',(-20.7751653502272,-18.8256008253747,
122.773930212868)) ;
#58985=CARTESIAN_POINT('Ctrl Pts',(-20.5019793282326,-18.6456117450119,
122.901496230122)) ;
#58986=CARTESIAN_POINT('Ctrl Pts',(-20.6452882013384,-18.8354843341053,
122.54898577994)) ;
#58987=CARTESIAN_POINT('Ctrl Pts',(-20.3980758193706,-18.6554952537425,
122.72154200763)) ;
#58988=CARTESIAN_POINT('Ctrl Pts',(-20.4769328739096,-18.8454792067514,
122.347392525977)) ;
#58989=CARTESIAN_POINT('Ctrl Pts',(-20.2633899435099,-18.6654901263886,
122.56026886385)) ;
#58990=CARTESIAN_POINT('Ctrl Pts',(-20.2753461930725,-18.8554991683871,
122.177967546874)) ;
#58991=CARTESIAN_POINT('Ctrl Pts',(-20.1021192027833,-18.6755100880243,
122.424730580812)) ;
#58992=CARTESIAN_POINT('Ctrl Pts',(-20.0501362495513,-18.865404532187,122.047445707246)) ;
#58993=CARTESIAN_POINT('Ctrl Pts',(-19.9219503672684,-18.6854154518241,
122.320315127144)) ;
#58994=CARTESIAN_POINT('Ctrl Pts',(-19.8050116122211,-18.8753451197945,
121.957195984845)) ;
#58995=CARTESIAN_POINT('Ctrl Pts',(-19.7258501182768,-18.6953560394316,
122.248117437871)) ;
#58996=CARTESIAN_POINT('Ctrl Pts',(-19.5463105434524,-18.8853479378952,
121.910432554943)) ;
#58997=CARTESIAN_POINT('Ctrl Pts',(-19.5188889496675,-18.7053588575323,
122.21070880072)) ;
#58998=CARTESIAN_POINT('Ctrl Pts',(-19.2826245313416,-18.8953826496193,
121.909724812354)) ;
#58999=CARTESIAN_POINT('Ctrl Pts',(-19.307940120733,-18.7153935692564,122.21014477667)) ;
#59000=CARTESIAN_POINT('Ctrl Pts',(-19.0276297317745,-18.9052275563566,
121.953532899944)) ;
#59001=CARTESIAN_POINT('Ctrl Pts',(-19.1039450889391,-18.7252384759937,
122.245193267705)) ;
#59002=CARTESIAN_POINT('Ctrl Pts',(-18.7805173029334,-18.9152134089256,
122.041718002023)) ;
#59003=CARTESIAN_POINT('Ctrl Pts',(-18.906255967733,-18.7352243285627,122.315743268288)) ;
#59004=CARTESIAN_POINT('Ctrl Pts',(-18.5534655977386,-18.9251482173387,
122.170689853634)) ;
#59005=CARTESIAN_POINT('Ctrl Pts',(-18.7246158475465,-18.7451591369758,
122.418922408914)) ;
#59006=CARTESIAN_POINT('Ctrl Pts',(-18.3499886138001,-18.9352057444197,
122.33930838977)) ;
#59007=CARTESIAN_POINT('Ctrl Pts',(-18.5618355205911,-18.7552166640568,
122.553818905849)) ;
#59008=CARTESIAN_POINT('Ctrl Pts',(-18.1825491267777,-18.9450273994168,
122.535766487528)) ;
#59009=CARTESIAN_POINT('Ctrl Pts',(-18.4278858915271,-18.7650383190539,
122.710986228041)) ;
#59010=CARTESIAN_POINT('Ctrl Pts',(-18.0482437942149,-18.9550834435898,
122.76333018742)) ;
#59011=CARTESIAN_POINT('Ctrl Pts',(-18.3204432872126,-18.775094363227,122.893038272163)) ;
#59012=CARTESIAN_POINT('Ctrl Pts',(-17.9569846493071,-18.965024183635,123.008115620737)) ;
#59013=CARTESIAN_POINT('Ctrl Pts',(-18.2474379774065,-18.7850351032721,
123.08886708059)) ;
#59014=CARTESIAN_POINT('Ctrl Pts',(-17.9089873948513,-18.9749283047079,
123.26392514927)) ;
#59015=CARTESIAN_POINT('Ctrl Pts',(-18.2090421543443,-18.794939224345,123.293514641434)) ;
#59016=CARTESIAN_POINT('Ctrl Pts',(-17.9062567714271,-18.9849758458621,
123.527931134947)) ;
#59017=CARTESIAN_POINT('Ctrl Pts',(-18.2068596105166,-18.8049867654992,
123.504719530089)) ;
#59018=CARTESIAN_POINT('Ctrl Pts',(-17.9485884795945,-18.9948745974625,
123.784627499312)) ;
#59019=CARTESIAN_POINT('Ctrl Pts',(-18.2407268052107,-18.8148855170996,
123.710075859708)) ;
#59020=CARTESIAN_POINT('Ctrl Pts',(-18.0360231031298,-19.0049230764283,
124.033764662916)) ;
#59021=CARTESIAN_POINT('Ctrl Pts',(-18.3106763436582,-18.8249339960654,
123.909385048735)) ;
#59022=CARTESIAN_POINT('Ctrl Pts',(-18.163325670764,-19.014810573512,124.260307326459)) ;
#59023=CARTESIAN_POINT('Ctrl Pts',(-18.4125198128121,-18.8348214931492,
124.09061779922)) ;
#59024=CARTESIAN_POINT('Ctrl Pts',(-18.3293793931802,-19.0248036638101,
124.463720725707)) ;
#59025=CARTESIAN_POINT('Ctrl Pts',(-18.5453641388487,-18.8448145834472,
124.253347258974)) ;
#59026=CARTESIAN_POINT('Ctrl Pts',(-18.5275042406602,-19.0347558338704,
124.634466519872)) ;
#59027=CARTESIAN_POINT('Ctrl Pts',(-18.7038650100524,-18.8547667535075,
124.389942302569)) ;
#59028=CARTESIAN_POINT('Ctrl Pts',(-18.7517438317463,-19.0446942537849,
124.768323296831)) ;
#59029=CARTESIAN_POINT('Ctrl Pts',(-18.8832572996416,-18.864705173422,124.497025999753)) ;
#59030=CARTESIAN_POINT('Ctrl Pts',(-18.9969024435329,-19.0546793838705,
124.861939962815)) ;
#59031=CARTESIAN_POINT('Ctrl Pts',(-19.079384667915,-18.8746903035076,124.571917644386)) ;
#59032=CARTESIAN_POINT('Ctrl Pts',(-19.2559540582378,-19.0647160732846,
124.91143051181)) ;
#59033=CARTESIAN_POINT('Ctrl Pts',(-19.286626370737,-18.8847269929217,124.611508315008)) ;
#59034=CARTESIAN_POINT('Ctrl Pts',(-19.5149158429124,-19.0745707572771,
124.915534595951)) ;
#59035=CARTESIAN_POINT('Ctrl Pts',(-19.4937950895379,-18.8945816769142,
124.614789827494)) ;
#59036=CARTESIAN_POINT('Ctrl Pts',(-19.774403515448,-19.0845702413249,124.874379795706)) ;
#59037=CARTESIAN_POINT('Ctrl Pts',(-19.7013848578054,-18.9045811609621,
124.581864340682)) ;
#59038=CARTESIAN_POINT('Ctrl Pts',(-20.0203843648563,-19.0944653301018,
124.789921645643)) ;
#59039=CARTESIAN_POINT('Ctrl Pts',(-19.898168451651,-18.914476249739,124.514296469915)) ;
#59040=CARTESIAN_POINT('Ctrl Pts',(-20.2516876994953,-19.104525884748,124.66194576436)) ;
#59041=CARTESIAN_POINT('Ctrl Pts',(-20.0832104950723,-18.9245368043851,
124.41191423788)) ;
#59042=CARTESIAN_POINT('Ctrl Pts',(-20.4530733453116,-19.1143751491209,
124.499321729623)) ;
#59043=CARTESIAN_POINT('Ctrl Pts',(-20.2443173510078,-18.934386068758,124.281814281811)) ;
#59044=CARTESIAN_POINT('Ctrl Pts',(-20.6267212720183,-19.1244024015687,
124.301134264892)) ;
#59045=CARTESIAN_POINT('Ctrl Pts',(-20.3832345959501,-18.9444133212059,
124.123263308682)) ;
#59046=CARTESIAN_POINT('Ctrl Pts',(-20.7627508777503,-19.1344306991389,
124.075408616383)) ;
#59047=CARTESIAN_POINT('Ctrl Pts',(-20.4920569238612,-18.954441618776,123.942681905956)) ;
#59048=CARTESIAN_POINT('Ctrl Pts',(-20.8562554221649,-19.1442768281449,
123.834159661665)) ;
#59049=CARTESIAN_POINT('Ctrl Pts',(-20.5668588165386,-18.964287747782,123.749683032266)) ;
#59050=CARTESIAN_POINT('Ctrl Pts',(-20.9078510940648,-19.154270733507,123.576649296537)) ;
#59051=CARTESIAN_POINT('Ctrl Pts',(-20.6081339643689,-18.9742816531441,
123.543674604084)) ;
#59052=CARTESIAN_POINT('Ctrl Pts',(-20.9134974107354,-19.16429483119,123.313280162661)) ;
#59053=CARTESIAN_POINT('Ctrl Pts',(-20.6126495326501,-18.9843057508271,
123.332979224958)) ;
#59054=CARTESIAN_POINT('Ctrl Pts',(-20.8741896282484,-19.174184659044,123.056370784505)) ;
#59055=CARTESIAN_POINT('Ctrl Pts',(-20.5812020083466,-18.9941955786812,
123.127452614158)) ;
#59056=CARTESIAN_POINT('Ctrl Pts',(-20.7903778747057,-19.1841766404745,
122.807538053505)) ;
#59057=CARTESIAN_POINT('Ctrl Pts',(-20.5141513809669,-19.0041875601116,
122.928386999942)) ;
#59058=CARTESIAN_POINT('Ctrl Pts',(-20.665139925686,-19.1941236452403,122.578095153288)) ;
#59059=CARTESIAN_POINT('Ctrl Pts',(-20.41396002509,-19.0141345648774,122.744833684279)) ;
#59060=CARTESIAN_POINT('Ctrl Pts',(-20.5022911487532,-19.2040732966301,
122.373520731289)) ;
#59061=CARTESIAN_POINT('Ctrl Pts',(-20.2836802639546,-19.0240842162672,
122.581175227014)) ;
#59062=CARTESIAN_POINT('Ctrl Pts',(-20.3045468222314,-19.2141102996075,
122.198982921485)) ;
#59063=CARTESIAN_POINT('Ctrl Pts',(-20.125483863784,-19.0341212192446,122.441545883708)) ;
#59064=CARTESIAN_POINT('Ctrl Pts',(-20.0829020053588,-19.2239992080425,
122.063295386373)) ;
#59065=CARTESIAN_POINT('Ctrl Pts',(-19.9481679801292,-19.0440101276797,
122.332997314253)) ;
#59066=CARTESIAN_POINT('Ctrl Pts',(-19.8387974857453,-19.23398854052,121.96675176185)) ;
#59067=CARTESIAN_POINT('Ctrl Pts',(-19.7528840990243,-19.0539994601571,
122.255763553244)) ;
#59068=CARTESIAN_POINT('Ctrl Pts',(-19.5823918613755,-19.2439470959571,
121.91441371455)) ;
#59069=CARTESIAN_POINT('Ctrl Pts',(-19.547759698978,-19.0639580155942,122.213894361448)) ;
#59070=CARTESIAN_POINT('Ctrl Pts',(-19.3223367513905,-19.2538466671576,
121.906790613366)) ;
#59071=CARTESIAN_POINT('Ctrl Pts',(-19.3397162836837,-19.0738575867947,
122.20779695611)) ;
#59072=CARTESIAN_POINT('Ctrl Pts',(-19.0611077173987,-19.2638945924096,
121.945087876798)) ;
#59073=CARTESIAN_POINT('Ctrl Pts',(-19.1307330399337,-19.0839055120467,
122.23843585839)) ;
#59074=CARTESIAN_POINT('Ctrl Pts',(-18.814173133126,-19.2737898919356,122.026726025059)) ;
#59075=CARTESIAN_POINT('Ctrl Pts',(-18.9331863897438,-19.0938008115727,
122.303747125533)) ;
#59076=CARTESIAN_POINT('Ctrl Pts',(-18.5813585770366,-19.2838517483836,
122.152010675439)) ;
#59077=CARTESIAN_POINT('Ctrl Pts',(-18.7469349998699,-19.1038626680207,
122.403975871039)) ;
#59078=CARTESIAN_POINT('Ctrl Pts',(-18.3782635159342,-19.2936955948002,
122.312252866463)) ;
#59079=CARTESIAN_POINT('Ctrl Pts',(-18.5844604094953,-19.1137065144373,
122.53216976341)) ;
#59080=CARTESIAN_POINT('Ctrl Pts',(-18.203337799749,-19.3036585439283,122.507039819624)) ;
#59081=CARTESIAN_POINT('Ctrl Pts',(-18.4445206716217,-19.1236694635654,
122.687999590902)) ;
#59082=CARTESIAN_POINT('Ctrl Pts',(-18.0642605165968,-19.3136925803563,
122.731072713085)) ;
#59083=CARTESIAN_POINT('Ctrl Pts',(-18.3332595529383,-19.1337034999934,
122.867226472839)) ;
#59084=CARTESIAN_POINT('Ctrl Pts',(-17.9673787966871,-19.3235800073143,
122.972163161456)) ;
#59085=CARTESIAN_POINT('Ctrl Pts',(-18.2557552582931,-19.1435909269514,
123.060098390728)) ;
#59086=CARTESIAN_POINT('Ctrl Pts',(-17.9126484521056,-19.3335944416507,
123.229596243496)) ;
#59087=CARTESIAN_POINT('Ctrl Pts',(-18.2119716852264,-19.1536053612878,
123.266044996015)) ;
#59088=CARTESIAN_POINT('Ctrl Pts',(-17.9040917216401,-19.3436293862856,
123.493147352358)) ;
#59089=CARTESIAN_POINT('Ctrl Pts',(-18.2051271768608,-19.1636403059227,
123.476886022838)) ;
#59090=CARTESIAN_POINT('Ctrl Pts',(-17.9399787131204,-19.3534617363166,
123.749059430674)) ;
#59091=CARTESIAN_POINT('Ctrl Pts',(-18.2338373040545,-19.1734726559537,
123.681614412356)) ;
#59092=CARTESIAN_POINT('Ctrl Pts',(-18.0216292180747,-19.3635371754338,
124.000873856143)) ;
#59093=CARTESIAN_POINT('Ctrl Pts',(-18.2991584729874,-19.183548095071,123.883066086777)) ;
#59094=CARTESIAN_POINT('Ctrl Pts',(-18.1429328956799,-19.3733896406684,
124.229675102606)) ;
#59095=CARTESIAN_POINT('Ctrl Pts',(-18.396201496122,-19.1934005603056,124.066105849519)) ;
#59096=CARTESIAN_POINT('Ctrl Pts',(-18.3054527184388,-19.3834625182453,
124.438557806816)) ;
#59097=CARTESIAN_POINT('Ctrl Pts',(-18.5262180422587,-19.2034734378824,
124.23321192103)) ;
#59098=CARTESIAN_POINT('Ctrl Pts',(-18.497358063962,-19.3933051144378,124.61200943149)) ;
#59099=CARTESIAN_POINT('Ctrl Pts',(-18.6797418858111,-19.2133160340749,
124.371972008953)) ;
#59100=CARTESIAN_POINT('Ctrl Pts',(-18.7190343990807,-19.4032854985531,
124.75215735034)) ;
#59101=CARTESIAN_POINT('Ctrl Pts',(-18.8570829522641,-19.2232964181902,
124.4840898822)) ;
#59102=CARTESIAN_POINT('Ctrl Pts',(-18.9628028394866,-19.4133039792019,
124.851593565958)) ;
#59103=CARTESIAN_POINT('Ctrl Pts',(-19.0520979082859,-19.233314898839,124.56363837805)) ;
#59104=CARTESIAN_POINT('Ctrl Pts',(-19.2165815610938,-19.4231872942023,
124.906993128951)) ;
#59105=CARTESIAN_POINT('Ctrl Pts',(-19.2551201081469,-19.2431982138394,
124.607957472016)) ;
#59106=CARTESIAN_POINT('Ctrl Pts',(-19.48091038097,-19.4332555912927,124.917562972667)) ;
#59107=CARTESIAN_POINT('Ctrl Pts',(-19.4665835088432,-19.2532665109298,
124.616412951815)) ;
#59108=CARTESIAN_POINT('Ctrl Pts',(-19.7369866664886,-19.443085659665,124.883208337292)) ;
#59109=CARTESIAN_POINT('Ctrl Pts',(-19.6714432710506,-19.2630965793021,
124.588929081079)) ;
#59110=CARTESIAN_POINT('Ctrl Pts',(-19.9891462344239,-19.4531524521334,
124.803370268973)) ;
#59111=CARTESIAN_POINT('Ctrl Pts',(-19.8731711567886,-19.2731633717705,
124.525058292213)) ;
#59112=CARTESIAN_POINT('Ctrl Pts',(-20.2195097660386,-19.4630417856219,
124.682973671205)) ;
#59113=CARTESIAN_POINT('Ctrl Pts',(-20.0574610978455,-19.2830527052591,
124.428741164273)) ;
#59114=CARTESIAN_POINT('Ctrl Pts',(-20.4279957455821,-19.473043917038,124.522983695097)) ;
#59115=CARTESIAN_POINT('Ctrl Pts',(-20.2242496883146,-19.2930548366751,
124.300749114728)) ;
#59116=CARTESIAN_POINT('Ctrl Pts',(-20.6043330327823,-19.482967786659,124.330784900546)) ;
#59117=CARTESIAN_POINT('Ctrl Pts',(-20.3653190116598,-19.3029787062961,
124.146990434962)) ;
#59118=CARTESIAN_POINT('Ctrl Pts',(-20.7461987470963,-19.4930113021762,
124.108267757242)) ;
#59119=CARTESIAN_POINT('Ctrl Pts',(-20.4788115505222,-19.3130222218133,
123.968976491356)) ;
#59120=CARTESIAN_POINT('Ctrl Pts',(-20.8459623353145,-19.5028935150645,
123.868447779189)) ;
#59121=CARTESIAN_POINT('Ctrl Pts',(-20.5586220080263,-19.3229044347016,
123.77712130273)) ;
#59122=CARTESIAN_POINT('Ctrl Pts',(-20.9036081809755,-19.5129615922839,
123.610275746684)) ;
#59123=CARTESIAN_POINT('Ctrl Pts',(-20.6047386771519,-19.332972511921,123.570583349477)) ;
#59124=CARTESIAN_POINT('Ctrl Pts',(-20.9155157124554,-19.5228000970181,
123.351961006778)) ;
#59125=CARTESIAN_POINT('Ctrl Pts',(-20.6142646315837,-19.3428110166552,
123.363932740499)) ;
#59126=CARTESIAN_POINT('Ctrl Pts',(-20.8820171905211,-19.5328628654475,
123.089685129375)) ;
#59127=CARTESIAN_POINT('Ctrl Pts',(-20.5874658526555,-19.3528737850846,
123.154111733586)) ;
#59128=CARTESIAN_POINT('Ctrl Pts',(-20.8044967773862,-19.5427598587302,
122.841407511896)) ;
#59129=CARTESIAN_POINT('Ctrl Pts',(-20.5254497644867,-19.3627707783674,
122.955490404283)) ;
#59130=CARTESIAN_POINT('Ctrl Pts',(-20.6854165300552,-19.552691086365,122.609182603989)) ;
#59131=CARTESIAN_POINT('Ctrl Pts',(-20.4301860313907,-19.3727020060021,
122.769710887484)) ;
#59132=CARTESIAN_POINT('Ctrl Pts',(-20.5258305091892,-19.5627332450072,
122.399010178353)) ;
#59133=CARTESIAN_POINT('Ctrl Pts',(-20.3025172352716,-19.3827441646443,
122.601572722186)) ;
#59134=CARTESIAN_POINT('Ctrl Pts',(-20.3352897321001,-19.5726199545382,
122.222366967696)) ;
#59135=CARTESIAN_POINT('Ctrl Pts',(-20.1500853867411,-19.3926308741753,
122.460258598056)) ;
#59136=CARTESIAN_POINT('Ctrl Pts',(-20.1148863727174,-19.5826129269668,
122.079617245507)) ;
#59137=CARTESIAN_POINT('Ctrl Pts',(-19.9737630061899,-19.4026238466039,
122.346058647369)) ;
#59138=CARTESIAN_POINT('Ctrl Pts',(-19.8741264226561,-19.5925591215034,
121.977883229186)) ;
#59139=CARTESIAN_POINT('Ctrl Pts',(-19.7811555923769,-19.4125700411405,
122.264671358312)) ;
#59140=CARTESIAN_POINT('Ctrl Pts',(-19.6194821905471,-19.6025044963549,
121.918938430882)) ;
#59141=CARTESIAN_POINT('Ctrl Pts',(-19.5774407611386,-19.422515415992,122.217515208665)) ;
#59142=CARTESIAN_POINT('Ctrl Pts',(-19.3556280435181,-19.6125594157148,
121.905362356848)) ;
#59143=CARTESIAN_POINT('Ctrl Pts',(-19.3663572165396,-19.4325703353519,
122.206654013868)) ;
#59144=CARTESIAN_POINT('Ctrl Pts',(-19.0993869105069,-19.6223809351583,
121.936569596424)) ;
#59145=CARTESIAN_POINT('Ctrl Pts',(-19.1613655396477,-19.4423918547954,
122.231619200685)) ;
#59146=CARTESIAN_POINT('Ctrl Pts',(-18.8463008166757,-19.6324467039252,
122.013333704317)) ;
#59147=CARTESIAN_POINT('Ctrl Pts',(-18.9588962140942,-19.4524576235623,
122.29303006788)) ;
#59148=CARTESIAN_POINT('Ctrl Pts',(-18.6141847413824,-19.6423486255803,
122.131051371132)) ;
#59149=CARTESIAN_POINT('Ctrl Pts',(-18.7732037818426,-19.4623595452174,
122.387203418498)) ;
#59150=CARTESIAN_POINT('Ctrl Pts',(-18.4029852173609,-19.6523916844013,
122.289280682628)) ;
#59151=CARTESIAN_POINT('Ctrl Pts',(-18.604243687009,-19.4724026040384,122.513786518166)) ;
#59152=CARTESIAN_POINT('Ctrl Pts',(-18.2250106932067,-19.662297678444,122.479267826305)) ;
#59153=CARTESIAN_POINT('Ctrl Pts',(-18.4618641781161,-19.4823085980811,
122.665775345268)) ;
#59154=CARTESIAN_POINT('Ctrl Pts',(-18.0816334128682,-19.6722354515258,
122.697543077663)) ;
#59155=CARTESIAN_POINT('Ctrl Pts',(-18.3471620419146,-19.4922463711629,
122.840394715573)) ;
#59156=CARTESIAN_POINT('Ctrl Pts',(-17.9775290976188,-19.6822758152581,
122.939982086318)) ;
#59157=CARTESIAN_POINT('Ctrl Pts',(-18.2638779349782,-19.5022867348952,
123.034345802999)) ;
#59158=CARTESIAN_POINT('Ctrl Pts',(-17.9178270664722,-19.6921631589816,
123.192873036797)) ;
#59159=CARTESIAN_POINT('Ctrl Pts',(-18.2161158243129,-19.5121740786187,
123.236657594822)) ;
#59160=CARTESIAN_POINT('Ctrl Pts',(-17.9023535730957,-19.7021553895503,
123.454984271159)) ;
#59161=CARTESIAN_POINT('Ctrl Pts',(-18.2037362398585,-19.5221663091874,
123.446346372631)) ;
#59162=CARTESIAN_POINT('Ctrl Pts',(-17.9325684280021,-19.7121039173339,
123.714684335697)) ;
#59163=CARTESIAN_POINT('Ctrl Pts',(-18.2279072969856,-19.532114836971,123.654106084101)) ;
#59164=CARTESIAN_POINT('Ctrl Pts',(-18.0069653213655,-19.7220407010572,
123.964967568088)) ;
#59165=CARTESIAN_POINT('Ctrl Pts',(-18.2874238319089,-19.5420516206943,
123.854332429313)) ;
#59166=CARTESIAN_POINT('Ctrl Pts',(-18.1239596004005,-19.7320237018542,
124.199815869688)) ;
#59167=CARTESIAN_POINT('Ctrl Pts',(-18.3810183152476,-19.5520346214913,
124.042211309555)) ;
#59168=CARTESIAN_POINT('Ctrl Pts',(-18.2812582377019,-19.7420675886949,
124.411727571249)) ;
#59169=CARTESIAN_POINT('Ctrl Pts',(-18.5068566460487,-19.562078508332,124.21174128928)) ;
#59170=CARTESIAN_POINT('Ctrl Pts',(-18.4684715103472,-19.7518956122695,
124.589706055916)) ;
#59171=CARTESIAN_POINT('Ctrl Pts',(-18.6566257534126,-19.5719065319066,
124.3541239909)) ;
#59172=CARTESIAN_POINT('Ctrl Pts',(-18.6890566141087,-19.7619728604831,
124.736130030075)) ;
#59173=CARTESIAN_POINT('Ctrl Pts',(-18.8330935698082,-19.5819837801202,
124.471264200358)) ;
#59174=CARTESIAN_POINT('Ctrl Pts',(-18.9262775519246,-19.7718224157884,
124.839850242289)) ;
#59175=CARTESIAN_POINT('Ctrl Pts',(-19.0228689899652,-19.5918333354255,
124.554240926399)) ;
#59176=CARTESIAN_POINT('Ctrl Pts',(-19.1837052991682,-19.7819051239861,
124.902304787671)) ;
#59177=CARTESIAN_POINT('Ctrl Pts',(-19.2288112851542,-19.6019160436232,
124.604205685487)) ;
#59178=CARTESIAN_POINT('Ctrl Pts',(-19.4410933758794,-19.7917177169126,
124.918904855256)) ;
#59179=CARTESIAN_POINT('Ctrl Pts',(-19.434720478767,-19.6117286365497,124.61748677879)) ;
#59180=CARTESIAN_POINT('Ctrl Pts',(-19.7040333399795,-19.8017849091705,
124.890266579354)) ;
#59181=CARTESIAN_POINT('Ctrl Pts',(-19.6450728626718,-19.6217958288076,
124.594577333264)) ;
#59182=CARTESIAN_POINT('Ctrl Pts',(-19.9538529269052,-19.8116837386331,
124.817515981026)) ;
#59183=CARTESIAN_POINT('Ctrl Pts',(-19.8449282229179,-19.6316946582702,
124.536378184494)) ;
#59184=CARTESIAN_POINT('Ctrl Pts',(-20.1908446168851,-19.8217377298233,
124.700847328328)) ;
#59185=CARTESIAN_POINT('Ctrl Pts',(-20.0345222842642,-19.6417486494604,
124.443044266715)) ;
#59186=CARTESIAN_POINT('Ctrl Pts',(-20.4003396792968,-19.8316094546065,
124.547752149574)) ;
#59187=CARTESIAN_POINT('Ctrl Pts',(-20.2021184087781,-19.6516203742436,
124.32056963313)) ;
#59188=CARTESIAN_POINT('Ctrl Pts',(-20.5836646742585,-19.8416798967367,
124.356956666456)) ;
#59189=CARTESIAN_POINT('Ctrl Pts',(-20.3487795243232,-19.6616908163738,
124.167933928758)) ;
#59190=CARTESIAN_POINT('Ctrl Pts',(-20.7277380468266,-19.851512975167,124.142415105616)) ;
#59191=CARTESIAN_POINT('Ctrl Pts',(-20.4640387321514,-19.6715238948041,
123.996302256258)) ;
#59192=CARTESIAN_POINT('Ctrl Pts',(-20.8351448171807,-19.8615434486684,
123.901710971158)) ;
#59193=CARTESIAN_POINT('Ctrl Pts',(-20.5499655097051,-19.6815543683055,
123.803739479692)) ;
#59194=CARTESIAN_POINT('Ctrl Pts',(-20.8983935514118,-19.8715750479671,
123.645775745948)) ;
#59195=CARTESIAN_POINT('Ctrl Pts',(-20.6005657740463,-19.6915859676042,
123.598991547224)) ;
#59196=CARTESIAN_POINT('Ctrl Pts',(-20.9164189115037,-19.8814047490052,
123.388108112838)) ;
#59197=CARTESIAN_POINT('Ctrl Pts',(-20.6149874004344,-19.7014156686424,
123.392858551262)) ;
#59198=CARTESIAN_POINT('Ctrl Pts',(-20.889769707107,-19.8913941870617,123.126944309975)) ;
#59199=CARTESIAN_POINT('Ctrl Pts',(-20.5936696114577,-19.7114051066988,
123.183927490661)) ;
#59200=CARTESIAN_POINT('Ctrl Pts',(-20.817146145048,-19.9014380902778,122.873192498264)) ;
#59201=CARTESIAN_POINT('Ctrl Pts',(-20.5355721095239,-19.7214490099149,
122.980925533021)) ;
#59202=CARTESIAN_POINT('Ctrl Pts',(-20.7046073617645,-19.9112596110913,
122.640918152662)) ;
#59203=CARTESIAN_POINT('Ctrl Pts',(-20.4455429052235,-19.7312705307284,
122.795106281435)) ;
#59204=CARTESIAN_POINT('Ctrl Pts',(-20.5506673334166,-19.9212953353384,
122.426787436432)) ;
#59205=CARTESIAN_POINT('Ctrl Pts',(-20.3223921809841,-19.7413062549755,
122.623800668938)) ;
#59206=CARTESIAN_POINT('Ctrl Pts',(-20.3616469061169,-19.9313174892709,
122.243358309574)) ;
#59207=CARTESIAN_POINT('Ctrl Pts',(-20.1711768967696,-19.751328408908,122.477056260967)) ;
#59208=CARTESIAN_POINT('Ctrl Pts',(-20.1473968172802,-19.9411797210282,
122.097565987472)) ;
#59209=CARTESIAN_POINT('Ctrl Pts',(-19.9997783728668,-19.7611906406653,
122.360421503876)) ;
#59210=CARTESIAN_POINT('Ctrl Pts',(-19.9090443945828,-19.9511387914861,
121.989462309799)) ;
#59211=CARTESIAN_POINT('Ctrl Pts',(-19.8090974023785,-19.7711497111232,
122.273937084454)) ;
#59212=CARTESIAN_POINT('Ctrl Pts',(-19.653521817539,-19.9611739638623,121.924289992094)) ;
#59213=CARTESIAN_POINT('Ctrl Pts',(-19.6046796893941,-19.7811848834994,
122.221797596013)) ;
#59214=CARTESIAN_POINT('Ctrl Pts',(-19.3946113132475,-19.9710543490205,
121.904388967509)) ;
#59215=CARTESIAN_POINT('Ctrl Pts',(-19.397552035366,-19.7910652686577,122.205875089908)) ;
#59216=CARTESIAN_POINT('Ctrl Pts',(-19.1316102592397,-19.9811110636145,
121.930090607281)) ;
#59217=CARTESIAN_POINT('Ctrl Pts',(-19.1871508676461,-19.8011219832516,
122.226434670213)) ;
#59218=CARTESIAN_POINT('Ctrl Pts',(-18.8815248170591,-19.9909903321865,
121.999843996043)) ;
#59219=CARTESIAN_POINT('Ctrl Pts',(-18.9870826419165,-19.8110012518237,
122.282235527794)) ;
#59220=CARTESIAN_POINT('Ctrl Pts',(-18.6444106249268,-20.0009812896722,
122.112585153845)) ;
#59221=CARTESIAN_POINT('Ctrl Pts',(-18.7973905924176,-19.8209922093093,
122.372426718099)) ;
#59222=CARTESIAN_POINT('Ctrl Pts',(-18.4297462676032,-20.0110219483074,
122.266017180346)) ;
#59223=CARTESIAN_POINT('Ctrl Pts',(-18.6256580184065,-19.8310328679445,
122.495170938252)) ;
#59224=CARTESIAN_POINT('Ctrl Pts',(-18.2485010034738,-20.0208549280154,
122.450186849546)) ;
#59225=CARTESIAN_POINT('Ctrl Pts',(-18.4806610287741,-19.8408658476525,
122.642504838089)) ;
#59226=CARTESIAN_POINT('Ctrl Pts',(-18.0989811418267,-20.0308480612651,
122.666069459646)) ;
#59227=CARTESIAN_POINT('Ctrl Pts',(-18.361043590352,-19.8508589809022,122.815209731099)) ;
#59228=CARTESIAN_POINT('Ctrl Pts',(-17.9892812124725,-20.0408801136485,
122.905806909259)) ;
#59229=CARTESIAN_POINT('Ctrl Pts',(-18.2732819325311,-19.8608910332856,
123.006998938251)) ;
#59230=CARTESIAN_POINT('Ctrl Pts',(-17.9236747635864,-20.0507453425998,
123.15660297018)) ;
#59231=CARTESIAN_POINT('Ctrl Pts',(-18.2207950630936,-19.8707562622369,
123.207634737405)) ;
#59232=CARTESIAN_POINT('Ctrl Pts',(-17.9016652917606,-20.060707283843,123.417472522822)) ;
#59233=CARTESIAN_POINT('Ctrl Pts',(-18.2031854905323,-19.8807182034801,
123.416330009112)) ;
#59234=CARTESIAN_POINT('Ctrl Pts',(-17.9258798988399,-20.0707419988798,
123.680047914976)) ;
#59235=CARTESIAN_POINT('Ctrl Pts',(-18.2225552242478,-19.8907529185169,
123.626390529728)) ;
#59236=CARTESIAN_POINT('Ctrl Pts',(-17.9938945221677,-20.0806277692238,
123.930807070481)) ;
#59237=CARTESIAN_POINT('Ctrl Pts',(-18.2769648599555,-19.9006386888609,
123.82699794779)) ;
#59238=CARTESIAN_POINT('Ctrl Pts',(-18.1063688771636,-20.0906903666126,
124.17009418255)) ;
#59239=CARTESIAN_POINT('Ctrl Pts',(-18.3669425672961,-19.9107012862497,
124.018428597259)) ;
#59240=CARTESIAN_POINT('Ctrl Pts',(-18.2554062654784,-20.1005407784478,
124.381769206372)) ;
#59241=CARTESIAN_POINT('Ctrl Pts',(-18.4861705070814,-19.9205516980849,
124.187769342642)) ;
#59242=CARTESIAN_POINT('Ctrl Pts',(-18.4417280629167,-20.1105679477337,
124.568087270912)) ;
#59243=CARTESIAN_POINT('Ctrl Pts',(-18.635226462847,-19.9305788673709,124.336825291195)) ;
#59244=CARTESIAN_POINT('Ctrl Pts',(-18.6579883240975,-20.1205954284479,
124.71867494309)) ;
#59245=CARTESIAN_POINT('Ctrl Pts',(-18.808233509183,-19.940606348085,124.457297090605)) ;
#59246=CARTESIAN_POINT('Ctrl Pts',(-18.8924830333248,-20.1304384810272,
124.827831022184)) ;
#59247=CARTESIAN_POINT('Ctrl Pts',(-18.9958279396515,-19.9504494006643,
124.544623631068)) ;
#59248=CARTESIAN_POINT('Ctrl Pts',(-19.1460332396166,-20.1404323844658,
124.896285825858)) ;
#59249=CARTESIAN_POINT('Ctrl Pts',(-19.1986674699778,-19.9604433041029,
124.599389529279)) ;
#59250=CARTESIAN_POINT('Ctrl Pts',(-19.408537282864,-20.1504595072422,124.919271899717)) ;
#59251=CARTESIAN_POINT('Ctrl Pts',(-19.408670501884,-19.9704704268793,124.617780480819)) ;
#59252=CARTESIAN_POINT('Ctrl Pts',(-19.6674999586504,-20.1603502121343,
124.896966576094)) ;
#59253=CARTESIAN_POINT('Ctrl Pts',(-19.6158404984156,-19.9803611317714,
124.599938376062)) ;
#59254=CARTESIAN_POINT('Ctrl Pts',(-19.9213144643627,-20.1703422389846,
124.829720703187)) ;
#59255=CARTESIAN_POINT('Ctrl Pts',(-19.8188925751091,-19.9903531586217,
124.546143793371)) ;
#59256=CARTESIAN_POINT('Ctrl Pts',(-20.158473228304,-20.1802882204731,124.719860821045)) ;
#59257=CARTESIAN_POINT('Ctrl Pts',(-20.0086203263769,-20.0002991401102,
124.458257924358)) ;
#59258=CARTESIAN_POINT('Ctrl Pts',(-20.3732942470927,-20.190235393095,124.570897282398)) ;
#59259=CARTESIAN_POINT('Ctrl Pts',(-20.1804782620418,-20.0102463127322,
124.339088990223)) ;
#59260=CARTESIAN_POINT('Ctrl Pts',(-20.5606438303885,-20.2002833344212,
124.384839709342)) ;
#59261=CARTESIAN_POINT('Ctrl Pts',(-20.3303594683394,-20.0202942540583,
124.19024447105)) ;
#59262=CARTESIAN_POINT('Ctrl Pts',(-20.7099931677264,-20.210130968229,124.17349632098)) ;
#59263=CARTESIAN_POINT('Ctrl Pts',(-20.4498405454841,-20.0301418878661,
124.021171285439)) ;
#59264=CARTESIAN_POINT('Ctrl Pts',(-20.8223918370586,-20.220092682914,123.937083946774)) ;
#59265=CARTESIAN_POINT('Ctrl Pts',(-20.5397614600564,-20.0401036025511,
123.832042436741)) ;
#59266=CARTESIAN_POINT('Ctrl Pts',(-20.8921871412405,-20.2301213157925,
123.682935524378)) ;
#59267=CARTESIAN_POINT('Ctrl Pts',(-20.5955998340411,-20.0501322354297,
123.628724320913)) ;
#59268=CARTESIAN_POINT('Ctrl Pts',(-20.9165866653184,-20.2400316413277,
123.423658765384)) ;
#59269=CARTESIAN_POINT('Ctrl Pts',(-20.6151216495105,-20.0600425609648,
123.421303286286)) ;
#59270=CARTESIAN_POINT('Ctrl Pts',(-20.8962205046669,-20.2499664717994,
123.163371888268)) ;
#59271=CARTESIAN_POINT('Ctrl Pts',(-20.5988309868347,-20.0699773914365,
123.213073725564)) ;
#59272=CARTESIAN_POINT('Ctrl Pts',(-20.8300540056933,-20.2600078041814,
122.907927043714)) ;
#59273=CARTESIAN_POINT('Ctrl Pts',(-20.545899908751,-20.0800187238185,123.008717280529)) ;
#59274=CARTESIAN_POINT('Ctrl Pts',(-20.7222442141385,-20.2699006776202,
122.671362855132)) ;
#59275=CARTESIAN_POINT('Ctrl Pts',(-20.4596543888742,-20.0899115972573,
122.819465277106)) ;
#59276=CARTESIAN_POINT('Ctrl Pts',(-20.574403392537,-20.2798698434381,122.45507183945)) ;
#59277=CARTESIAN_POINT('Ctrl Pts',(-20.3413828139098,-20.0998807630752,
122.646430631496)) ;
#59278=CARTESIAN_POINT('Ctrl Pts',(-20.389867415721,-20.2898985771546,122.266945763663)) ;
#59279=CARTESIAN_POINT('Ctrl Pts',(-20.1937587117748,-20.1099094967917,
122.495930505573)) ;
#59280=CARTESIAN_POINT('Ctrl Pts',(-20.108189935514,-20.3030910959258,122.064717611353)) ;
#59281=CARTESIAN_POINT('Ctrl Pts',(-19.9684034754264,-20.1231020155629,
122.334134312511)) ;
#59282=CARTESIAN_POINT('Ctrl Pts',(-19.776200429425,-20.3164509639684,121.939098030054)) ;
#59283=CARTESIAN_POINT('Ctrl Pts',(-19.70278986189,-20.1364618836056,122.233638111856)) ;
#59284=CARTESIAN_POINT('Ctrl Pts',(-19.4302944299176,-20.3296763011173,
121.904585070859)) ;
#59285=CARTESIAN_POINT('Ctrl Pts',(-19.4261079855339,-20.1496872207544,
122.206033326473)) ;
#59286=CARTESIAN_POINT('Ctrl Pts',(-19.1686900557449,-20.3396575269579,
121.923502397448)) ;
#59287=CARTESIAN_POINT('Ctrl Pts',(-19.2168157977084,-20.1596684465951,
122.221163228254)) ;
#59288=CARTESIAN_POINT('Ctrl Pts',(-18.9130849261984,-20.3496930939408,
121.988403504327)) ;
#59289=CARTESIAN_POINT('Ctrl Pts',(-19.0123335164269,-20.1697040135779,
122.273082369404)) ;
#59290=CARTESIAN_POINT('Ctrl Pts',(-18.6765159440695,-20.3595561719029,
122.094373600289)) ;
#59291=CARTESIAN_POINT('Ctrl Pts',(-18.8230767411481,-20.17956709154,122.357856308508)) ;
#59292=CARTESIAN_POINT('Ctrl Pts',(-18.4574468061617,-20.369626470704,122.2427865665)) ;
#59293=CARTESIAN_POINT('Ctrl Pts',(-18.6478204417451,-20.1896373903411,
122.476584793139)) ;
#59294=CARTESIAN_POINT('Ctrl Pts',(-18.2717579005638,-20.3794687692718,
122.422851075719)) ;
#59295=CARTESIAN_POINT('Ctrl Pts',(-18.4992676185254,-20.1994796889089,
122.620634878705)) ;
#59296=CARTESIAN_POINT('Ctrl Pts',(-18.1175586647282,-20.3894294674416,
122.634360678073)) ;
#59297=CARTESIAN_POINT('Ctrl Pts',(-18.3759064506187,-20.2094403870787,
122.78984130679)) ;
#59298=CARTESIAN_POINT('Ctrl Pts',(-18.0020059072157,-20.3994675016211,
122.871483585782)) ;
#59299=CARTESIAN_POINT('Ctrl Pts',(-18.2834623026179,-20.2194784212582,
122.97953855026)) ;
#59300=CARTESIAN_POINT('Ctrl Pts',(-17.9300887193781,-20.4093412384676,
123.12082468391)) ;
#59301=CARTESIAN_POINT('Ctrl Pts',(-18.2259264014613,-20.2293521581047,
123.179011012652)) ;
#59302=CARTESIAN_POINT('Ctrl Pts',(-17.9020448474058,-20.4194130223928,
123.383973224126)) ;
#59303=CARTESIAN_POINT('Ctrl Pts',(-18.2034891482727,-20.2394239420299,
123.389529423009)) ;
#59304=CARTESIAN_POINT('Ctrl Pts',(-17.9195350319781,-20.429245143594,123.641783391188)) ;
#59305=CARTESIAN_POINT('Ctrl Pts',(-18.2174791482912,-20.2492560632311,
123.595778035105)) ;
#59306=CARTESIAN_POINT('Ctrl Pts',(-17.9820931576725,-20.4392781676194,
123.897898640785)) ;
#59307=CARTESIAN_POINT('Ctrl Pts',(-18.2675235858112,-20.2592890872566,
123.8006706467)) ;
#59308=CARTESIAN_POINT('Ctrl Pts',(-18.0886185614509,-20.4492940478161,
124.138604141846)) ;
#59309=CARTESIAN_POINT('Ctrl Pts',(-18.3527418295689,-20.2693049674532,
123.993235758513)) ;
#59310=CARTESIAN_POINT('Ctrl Pts',(-18.2329706508674,-20.4591775669103,
124.354523331879)) ;
#59311=CARTESIAN_POINT('Ctrl Pts',(-18.4682220840992,-20.2791884865474,
124.165972815499)) ;
#59312=CARTESIAN_POINT('Ctrl Pts',(-18.4143074091382,-20.469167979274,124.54434899152)) ;
#59313=CARTESIAN_POINT('Ctrl Pts',(-18.6132892508366,-20.2891788989111,
124.31783370646)) ;
#59314=CARTESIAN_POINT('Ctrl Pts',(-18.6951170310066,-20.4824311424774,
124.750853866765)) ;
#59315=CARTESIAN_POINT('Ctrl Pts',(-18.8379390825619,-20.3024420621145,
124.483045334698)) ;
#59316=CARTESIAN_POINT('Ctrl Pts',(-19.0235816254603,-20.4957087127286,
124.879780338446)) ;
#59317=CARTESIAN_POINT('Ctrl Pts',(-19.1007466138958,-20.3157196323657,
124.586193622694)) ;
#59318=CARTESIAN_POINT('Ctrl Pts',(-19.3717460245778,-20.5090390152352,
124.918788838269)) ;
#59319=CARTESIAN_POINT('Ctrl Pts',(-19.3792305302181,-20.3290499348723,
124.617392368579)) ;
#59320=CARTESIAN_POINT('Ctrl Pts',(-19.631378352144,-20.5189376970516,124.902811153565)) ;
#59321=CARTESIAN_POINT('Ctrl Pts',(-19.586946416879,-20.3389486166887,124.604614298726)) ;
#59322=CARTESIAN_POINT('Ctrl Pts',(-19.886681931356,-20.5289272120991,124.841743662503)) ;
#59323=CARTESIAN_POINT('Ctrl Pts',(-19.7911870921237,-20.3489381317363,
124.555761778186)) ;
#59324=CARTESIAN_POINT('Ctrl Pts',(-20.1265183759964,-20.5388752638742,
124.737689396078)) ;
#59325=CARTESIAN_POINT('Ctrl Pts',(-19.9830583085483,-20.3588861835113,
124.472519572636)) ;
#59326=CARTESIAN_POINT('Ctrl Pts',(-20.3446556457236,-20.5488166671527,
124.593959705977)) ;
#59327=CARTESIAN_POINT('Ctrl Pts',(-20.1575676024382,-20.3688275867898,
124.357539619825)) ;
#59328=CARTESIAN_POINT('Ctrl Pts',(-20.5987445476078,-20.5621033319336,
124.354427857962)) ;
#59329=CARTESIAN_POINT('Ctrl Pts',(-20.3608485152388,-20.3821142515707,
124.165903776339)) ;
#59330=CARTESIAN_POINT('Ctrl Pts',(-20.8307521720102,-20.5787137535884,
123.97887050718)) ;
#59331=CARTESIAN_POINT('Ctrl Pts',(-20.5464484061325,-20.3987246732255,
123.865472812429)) ;
#59332=CARTESIAN_POINT('Ctrl Pts',(-20.9389514260489,-20.5986250158392,
123.460821316337)) ;
#59333=CARTESIAN_POINT('Ctrl Pts',(-20.6330141894971,-20.4186359354763,
123.451029346131)) ;
#59334=CARTESIAN_POINT('Ctrl Pts',(-20.8639502681966,-20.6185691450041,
122.93604284961)) ;
#59335=CARTESIAN_POINT('Ctrl Pts',(-20.5730157436839,-20.4385800646412,
123.031206971255)) ;
#59336=CARTESIAN_POINT('Ctrl Pts',(-20.614611211859,-20.6384923076093,122.468951374548)) ;
#59337=CARTESIAN_POINT('Ctrl Pts',(-20.373547351219,-20.4585032272464,122.657531515704)) ;
#59338=CARTESIAN_POINT('Ctrl Pts',(-20.2219924331107,-20.6583824300158,
122.114827126927)) ;
#59339=CARTESIAN_POINT('Ctrl Pts',(-20.0594536357031,-20.4783933496529,
122.374229525961)) ;
#59340=CARTESIAN_POINT('Ctrl Pts',(-19.7292685932625,-20.6783873836159,
121.915230361568)) ;
#59341=CARTESIAN_POINT('Ctrl Pts',(-19.6652757291056,-20.498398303253,122.2145494258)) ;
#59342=CARTESIAN_POINT('Ctrl Pts',(-19.2022698837694,-20.6982256406315,
121.895490958203)) ;
#59343=CARTESIAN_POINT('Ctrl Pts',(-19.2436755852947,-20.5182365602686,
122.198755216504)) ;
#59344=CARTESIAN_POINT('Ctrl Pts',(-18.6962108824023,-20.718219941418,122.057473862947)) ;
#59345=CARTESIAN_POINT('Ctrl Pts',(-18.8388276085648,-20.5382308610552,
122.328339327978)) ;
#59346=CARTESIAN_POINT('Ctrl Pts',(-18.2783285952611,-20.7381051834625,
122.381075560874)) ;
#59347=CARTESIAN_POINT('Ctrl Pts',(-18.5045195347661,-20.5581161030996,
122.587219431288)) ;
#59348=CARTESIAN_POINT('Ctrl Pts',(-17.994854669319,-20.7579801299384,122.826813664133)) ;
#59349=CARTESIAN_POINT('Ctrl Pts',(-18.2777383070033,-20.5779910495756,
122.943810054151)) ;
#59350=CARTESIAN_POINT('Ctrl Pts',(-17.8799919148202,-20.7780131998795,
123.346775629798)) ;
#59351=CARTESIAN_POINT('Ctrl Pts',(-18.1858465680844,-20.5980241195166,
123.359778876185)) ;
#59352=CARTESIAN_POINT('Ctrl Pts',(-17.9496011378404,-20.7979017067799,
123.870729922687)) ;
#59353=CARTESIAN_POINT('Ctrl Pts',(-18.2415323136978,-20.617912626417,123.778943688252)) ;
#59354=CARTESIAN_POINT('Ctrl Pts',(-18.1918462219095,-20.8177565665612,
124.3396421318)) ;
#59355=CARTESIAN_POINT('Ctrl Pts',(-18.4353283966454,-20.6377674861983,
124.15407531908)) ;
#59356=CARTESIAN_POINT('Ctrl Pts',(-18.5838321068267,-20.8378074003489,
124.700496054133)) ;
#59357=CARTESIAN_POINT('Ctrl Pts',(-18.7489159490425,-20.657818319986,124.442758816039)) ;
#59358=CARTESIAN_POINT('Ctrl Pts',(-19.068464276831,-20.8575733422382,124.903648311882)) ;
#59359=CARTESIAN_POINT('Ctrl Pts',(-19.1366240867067,-20.6775842618753,
124.605282256728)) ;
#59360=CARTESIAN_POINT('Ctrl Pts',(-19.5995315082648,-20.8775860736975,
124.930591112169)) ;
#59361=CARTESIAN_POINT('Ctrl Pts',(-19.5614778234741,-20.6975969933346,
124.626836366824)) ;
#59362=CARTESIAN_POINT('Ctrl Pts',(-20.1049415619315,-20.8974789086411,
124.774856355301)) ;
#59363=CARTESIAN_POINT('Ctrl Pts',(-19.9658071300402,-20.7174898282782,
124.502248164714)) ;
#59364=CARTESIAN_POINT('Ctrl Pts',(-20.5274834956155,-20.9173859319806,
124.456638371314)) ;
#59365=CARTESIAN_POINT('Ctrl Pts',(-20.3038412440261,-20.7373968516177,
124.247672563111)) ;
#59366=CARTESIAN_POINT('Ctrl Pts',(-20.816830578431,-20.9373011968813,124.013259477076)) ;
#59367=CARTESIAN_POINT('Ctrl Pts',(-20.5353184953281,-20.7573121165184,
123.892968103574)) ;
#59368=CARTESIAN_POINT('Ctrl Pts',(-20.9375148304315,-20.957332889041,123.494752291647)) ;
#59369=CARTESIAN_POINT('Ctrl Pts',(-20.6318648818766,-20.7773438086781,
123.47816249865)) ;
#59370=CARTESIAN_POINT('Ctrl Pts',(-20.8746353856575,-20.977175935614,122.971063764451)) ;
#59371=CARTESIAN_POINT('Ctrl Pts',(-20.5815599743237,-20.7971868552511,
123.059210077434)) ;
#59372=CARTESIAN_POINT('Ctrl Pts',(-20.6370889547164,-20.9970924835138,
122.498095047724)) ;
#59373=CARTESIAN_POINT('Ctrl Pts',(-20.3915208071778,-20.8171034031509,
122.680835172587)) ;
#59374=CARTESIAN_POINT('Ctrl Pts',(-20.2519449229263,-21.0170247265051,
122.134274226715)) ;
#59375=CARTESIAN_POINT('Ctrl Pts',(-20.0834038045587,-20.8370356461422,
122.389779490593)) ;
#59376=CARTESIAN_POINT('Ctrl Pts',(-19.7666424548644,-21.0369285613144,
121.923791010191)) ;
#59377=CARTESIAN_POINT('Ctrl Pts',(-19.6951601330397,-20.8569394809515,
122.221394579836)) ;
#59378=CARTESIAN_POINT('Ctrl Pts',(-19.2387517746297,-21.0568289615019,
121.890890792397)) ;
#59379=CARTESIAN_POINT('Ctrl Pts',(-19.2728466143262,-20.876839881139,122.195076908479)) ;
#59380=CARTESIAN_POINT('Ctrl Pts',(-18.7299794806847,-21.0767786378812,
122.040270945825)) ;
#59381=CARTESIAN_POINT('Ctrl Pts',(-18.8658292110054,-20.8967895575183,
122.314583763135)) ;
#59382=CARTESIAN_POINT('Ctrl Pts',(-18.303166710287,-21.0967111621016,122.354115893689)) ;
#59383=CARTESIAN_POINT('Ctrl Pts',(-18.5243802930808,-20.9167220817387,
122.565662292929)) ;
#59384=CARTESIAN_POINT('Ctrl Pts',(-18.0088633209534,-21.1166311710878,
122.794268679534)) ;
#59385=CARTESIAN_POINT('Ctrl Pts',(-18.2889398325272,-20.9366420907249,
122.917786669233)) ;
#59386=CARTESIAN_POINT('Ctrl Pts',(-17.8822937308164,-21.136588077264,123.309313272766)) ;
#59387=CARTESIAN_POINT('Ctrl Pts',(-18.1876872095001,-20.9565989969011,
123.329823376665)) ;
#59388=CARTESIAN_POINT('Ctrl Pts',(-17.9384143246764,-21.1564739167655,
123.834958994811)) ;
#59389=CARTESIAN_POINT('Ctrl Pts',(-18.2325869694415,-20.9764848364026,
123.750340253762)) ;
#59390=CARTESIAN_POINT('Ctrl Pts',(-18.1714993859742,-21.1764450889013,
124.31171484266)) ;
#59391=CARTESIAN_POINT('Ctrl Pts',(-18.4190587792687,-20.9964560085384,
124.131743525052)) ;
#59392=CARTESIAN_POINT('Ctrl Pts',(-18.5499193847217,-21.1962592858857,
124.678080171936)) ;
#59393=CARTESIAN_POINT('Ctrl Pts',(-18.7217959353721,-21.0162702055228,
124.424833857205)) ;
#59394=CARTESIAN_POINT('Ctrl Pts',(-19.0342352621923,-21.2162404718539,
124.89571496393)) ;
#59395=CARTESIAN_POINT('Ctrl Pts',(-19.1092580929924,-21.0362513914911,
124.598937764021)) ;
#59396=CARTESIAN_POINT('Ctrl Pts',(-19.4736619237772,-21.2328159772432,
124.928069751188)) ;
#59397=CARTESIAN_POINT('Ctrl Pts',(-19.4607756982869,-21.0528268968803,
124.624819424069)) ;
#59398=CARTESIAN_POINT('Ctrl Pts',(-19.8173383619088,-21.2461254251068,
124.863112509641)) ;
#59399=CARTESIAN_POINT('Ctrl Pts',(-19.7357439277155,-21.0661363447439,
124.572846691441)) ;
#59400=CARTESIAN_POINT('Ctrl Pts',(-20.1458733462935,-21.2594931228834,
124.738714343657)) ;
#59401=CARTESIAN_POINT('Ctrl Pts',(-19.998523136109,-21.0795040425205,124.473349266923)) ;
#59402=CARTESIAN_POINT('Ctrl Pts',(-20.5018728442166,-21.2759836945493,
124.483060829662)) ;
#59403=CARTESIAN_POINT('Ctrl Pts',(-20.2833722640373,-21.0959946141864,
124.268798320229)) ;
#59404=CARTESIAN_POINT('Ctrl Pts',(-20.8018337601815,-21.2959039668821,
124.04687473534)) ;
#59405=CARTESIAN_POINT('Ctrl Pts',(-20.5233223409627,-21.1159148865192,
123.919846740881)) ;
#59406=CARTESIAN_POINT('Ctrl Pts',(-20.9126872837308,-21.3125210026031,
123.619326861712)) ;
#59407=CARTESIAN_POINT('Ctrl Pts',(-20.6120012338397,-21.1325319222402,
123.57783290666)) ;
#59408=CARTESIAN_POINT('Ctrl Pts',(-20.9100801364126,-21.3258118528842,
123.270041130568)) ;
#59409=CARTESIAN_POINT('Ctrl Pts',(-20.6099160373388,-21.1458227725213,
123.298380131864)) ;
#59410=CARTESIAN_POINT('Ctrl Pts',(-20.8627908877047,-21.3357808980387,
123.01239695694)) ;
#59411=CARTESIAN_POINT('Ctrl Pts',(-20.572081952972,-21.1557918176758,123.092270099761)) ;
#59412=CARTESIAN_POINT('Ctrl Pts',(-20.7725483587208,-21.3456842886722,
122.768260657611)) ;
#59413=CARTESIAN_POINT('Ctrl Pts',(-20.499885452573,-21.1656952083094,122.896960032138)) ;
#59414=CARTESIAN_POINT('Ctrl Pts',(-20.6391462593297,-21.355742074785,122.540122041422)) ;
#59415=CARTESIAN_POINT('Ctrl Pts',(-20.3931639432043,-21.1757529944221,
122.714452096665)) ;
#59416=CARTESIAN_POINT('Ctrl Pts',(-20.471796281269,-21.3655941114347,122.342544854426)) ;
#59417=CARTESIAN_POINT('Ctrl Pts',(-20.2592745302504,-21.1856050310718,
122.556386398767)) ;
#59418=CARTESIAN_POINT('Ctrl Pts',(-20.202086568455,-21.3789592355779,122.117585029651)) ;
#59419=CARTESIAN_POINT('Ctrl Pts',(-20.0435429434541,-21.198970155215,122.376446523523)) ;
#59420=CARTESIAN_POINT('Ctrl Pts',(-19.8829746642869,-21.3921852985409,
121.970083356066)) ;
#59421=CARTESIAN_POINT('Ctrl Pts',(-19.7882331633885,-21.2121962181781,
122.25842782825)) ;
#59422=CARTESIAN_POINT('Ctrl Pts',(-19.5386166648269,-21.4054889468232,
121.909867161857)) ;
#59423=CARTESIAN_POINT('Ctrl Pts',(-19.5127307955836,-21.2254998664603,
122.210256068313)) ;
#59424=CARTESIAN_POINT('Ctrl Pts',(-19.2760167649195,-21.4154804779862,
121.910107183642)) ;
#59425=CARTESIAN_POINT('Ctrl Pts',(-19.302654042271,-21.2354913976233,122.210450691306)) ;
#59426=CARTESIAN_POINT('Ctrl Pts',(-19.0163207496462,-21.4255199257855,
121.956500605478)) ;
#59427=CARTESIAN_POINT('Ctrl Pts',(-19.0948968590476,-21.2455308454226,
122.247567530299)) ;
#59428=CARTESIAN_POINT('Ctrl Pts',(-18.7732843139319,-21.4353637012994,
122.045159677628)) ;
#59429=CARTESIAN_POINT('Ctrl Pts',(-18.9004686755779,-21.2553746209365,
122.318496939825)) ;
#59430=CARTESIAN_POINT('Ctrl Pts',(-18.5458944197202,-21.445349342687,122.176053036341)) ;
#59431=CARTESIAN_POINT('Ctrl Pts',(-18.7185578856858,-21.2653602623241,
122.42321354917)) ;
#59432=CARTESIAN_POINT('Ctrl Pts',(-18.3455158402902,-21.4552861270488,
122.343559635745)) ;
#59433=CARTESIAN_POINT('Ctrl Pts',(-18.5582565294496,-21.2752970466859,
122.557220524187)) ;
#59434=CARTESIAN_POINT('Ctrl Pts',(-18.1755004123989,-21.4653359615162,
122.545621877111)) ;
#59435=CARTESIAN_POINT('Ctrl Pts',(-18.4222459430947,-21.2853468811533,
122.718871736199)) ;
#59436=CARTESIAN_POINT('Ctrl Pts',(-18.0455857951863,-21.4751864110193,
122.769542152888)) ;
#59437=CARTESIAN_POINT('Ctrl Pts',(-18.3183162510833,-21.2951973306564,
122.898009008209)) ;
#59438=CARTESIAN_POINT('Ctrl Pts',(-17.9548017337126,-21.4851584250014,
123.015333175436)) ;
#59439=CARTESIAN_POINT('Ctrl Pts',(-18.2456911442363,-21.3051693446385,
123.094642518288)) ;
#59440=CARTESIAN_POINT('Ctrl Pts',(-17.9079865989931,-21.4951535828485,
123.273832595304)) ;
#59441=CARTESIAN_POINT('Ctrl Pts',(-18.2082412561885,-21.3151645024856,
123.3014423916)) ;
#59442=CARTESIAN_POINT('Ctrl Pts',(-17.9070803718407,-21.5051875092122,
123.537489745388)) ;
#59443=CARTESIAN_POINT('Ctrl Pts',(-18.2075185318219,-21.3251984288494,
123.512368089065)) ;
#59444=CARTESIAN_POINT('Ctrl Pts',(-17.9507793758627,-21.5150432176446,
123.792798278233)) ;
#59445=CARTESIAN_POINT('Ctrl Pts',(-18.2424799133806,-21.3350541372817,
123.716614351345)) ;
#59446=CARTESIAN_POINT('Ctrl Pts',(-18.0390300008137,-21.5250413669833,
124.040230621142)) ;
#59447=CARTESIAN_POINT('Ctrl Pts',(-18.3130824917955,-21.3450522866204,
123.914559406275)) ;
#59448=CARTESIAN_POINT('Ctrl Pts',(-18.1674560178269,-21.5349407701568,
124.266510551616)) ;
#59449=CARTESIAN_POINT('Ctrl Pts',(-18.4158251303191,-21.354951689794,124.095582078707)) ;
#59450=CARTESIAN_POINT('Ctrl Pts',(-18.3356760700349,-21.5449919670453,
124.470114254987)) ;
#59451=CARTESIAN_POINT('Ctrl Pts',(-18.5504028849582,-21.3650028866824,
124.258463636638)) ;
#59452=CARTESIAN_POINT('Ctrl Pts',(-18.5333267197165,-21.5548742908582,
124.63859875685)) ;
#59453=CARTESIAN_POINT('Ctrl Pts',(-18.7085246479764,-21.3748852104953,
124.393249391773)) ;
#59454=CARTESIAN_POINT('Ctrl Pts',(-18.7594560018533,-21.5648691865148,
124.772199667984)) ;
#59455=CARTESIAN_POINT('Ctrl Pts',(-18.8894291059458,-21.3848801061519,
124.500128205226)) ;
#59456=CARTESIAN_POINT('Ctrl Pts',(-19.0061476935566,-21.5748902858973,
124.864395292257)) ;
#59457=CARTESIAN_POINT('Ctrl Pts',(-19.0867832058502,-21.3949012055344,
124.573882634977)) ;
#59458=CARTESIAN_POINT('Ctrl Pts',(-19.2621059878606,-21.5847975537594,
124.912011501582)) ;
#59459=CARTESIAN_POINT('Ctrl Pts',(-19.2915499957338,-21.4048084733965,
124.611973405595)) ;
#59460=CARTESIAN_POINT('Ctrl Pts',(-19.523241461829,-21.5947358975846,124.914993347183)) ;
#59461=CARTESIAN_POINT('Ctrl Pts',(-19.5004581837589,-21.4147468172218,
124.61435673395)) ;
#59462=CARTESIAN_POINT('Ctrl Pts',(-19.7826877608653,-21.6047393168851,
124.872466522298)) ;
#59463=CARTESIAN_POINT('Ctrl Pts',(-19.7080148132996,-21.4247502365222,
124.580333183701)) ;
#59464=CARTESIAN_POINT('Ctrl Pts',(-20.0313953526163,-21.6147738675922,
124.784868563439)) ;
#59465=CARTESIAN_POINT('Ctrl Pts',(-19.9069801784579,-21.4347847872293,
124.510252765367)) ;
#59466=CARTESIAN_POINT('Ctrl Pts',(-20.2570175361055,-21.6246188171978,
124.658232944476)) ;
#59467=CARTESIAN_POINT('Ctrl Pts',(-20.0874764875126,-21.4446297368349,
124.408942636223)) ;
#59468=CARTESIAN_POINT('Ctrl Pts',(-20.4603562191612,-21.6346046593107,
124.492418457877)) ;
#59469=CARTESIAN_POINT('Ctrl Pts',(-20.2501460171759,-21.4546155789478,
124.276289513827)) ;
#59470=CARTESIAN_POINT('Ctrl Pts',(-20.6311392301702,-21.6445394666798,
124.294885221514)) ;
#59471=CARTESIAN_POINT('Ctrl Pts',(-20.3867706983452,-21.4645503863169,
124.118261777518)) ;
#59472=CARTESIAN_POINT('Ctrl Pts',(-20.7664361277187,-21.6545970083931,
124.067883129677)) ;
#59473=CARTESIAN_POINT('Ctrl Pts',(-20.4950064705292,-21.4746079280302,
123.936658954064)) ;
#59474=CARTESIAN_POINT('Ctrl Pts',(-20.8584564948569,-21.6644186059052,
123.826712005177)) ;
#59475=CARTESIAN_POINT('Ctrl Pts',(-20.5686206343265,-21.4844295255424,
123.743721915454)) ;
#59476=CARTESIAN_POINT('Ctrl Pts',(-20.9088388978743,-21.6744748653857,
123.567314526484)) ;
#59477=CARTESIAN_POINT('Ctrl Pts',(-20.6089246277522,-21.4944857850228,
123.536203466964)) ;
#59478=CARTESIAN_POINT('Ctrl Pts',(-20.912905442173,-21.6844148016861,123.306120784318)) ;
#59479=CARTESIAN_POINT('Ctrl Pts',(-20.61217581895,-21.5044257213232,123.327248710015)) ;
#59480=CARTESIAN_POINT('Ctrl Pts',(-20.8724715625939,-21.6943219224305,
123.048933898916)) ;
#59481=CARTESIAN_POINT('Ctrl Pts',(-20.5798268670816,-21.5143328420676,
123.121499921516)) ;
#59482=CARTESIAN_POINT('Ctrl Pts',(-20.7867471086995,-21.7043648283558,
122.799333949718)) ;
#59483=CARTESIAN_POINT('Ctrl Pts',(-20.5112454371669,-21.5243757479929,
122.921820528242)) ;
#59484=CARTESIAN_POINT('Ctrl Pts',(-20.6607421010669,-21.714272609455,122.571477249608)) ;
#59485=CARTESIAN_POINT('Ctrl Pts',(-20.4104399317555,-21.5342835290921,
122.739536474708)) ;
#59486=CARTESIAN_POINT('Ctrl Pts',(-20.4957543255686,-21.7242829784574,
122.366574426333)) ;
#59487=CARTESIAN_POINT('Ctrl Pts',(-20.2784482779818,-21.5442938980945,
122.575615429182)) ;
#59488=CARTESIAN_POINT('Ctrl Pts',(-20.2969450012254,-21.7343138170262,
122.19348877084)) ;
#59489=CARTESIAN_POINT('Ctrl Pts',(-20.1193995041773,-21.5543247366633,
122.437148355907)) ;
#59490=CARTESIAN_POINT('Ctrl Pts',(-20.0753430040453,-21.7441666566659,
122.059562188914)) ;
#59491=CARTESIAN_POINT('Ctrl Pts',(-19.9421175002561,-21.564177576303,122.330009052223)) ;
#59492=CARTESIAN_POINT('Ctrl Pts',(-19.8307389892015,-21.7541546578309,
121.964427436421)) ;
#59493=CARTESIAN_POINT('Ctrl Pts',(-19.7464337668386,-21.574165577468,122.253902995604)) ;
#59494=CARTESIAN_POINT('Ctrl Pts',(-19.5748309877734,-21.76408347681,121.913501885889)) ;
#59495=CARTESIAN_POINT('Ctrl Pts',(-19.5417073934896,-21.5840943964472,
122.213164409837)) ;
#59496=CARTESIAN_POINT('Ctrl Pts',(-19.3124241042443,-21.7740711795323,
121.907308024055)) ;
#59497=CARTESIAN_POINT('Ctrl Pts',(-19.3317819920219,-21.5940820991695,
122.208211065179)) ;
#59498=CARTESIAN_POINT('Ctrl Pts',(-19.0517647367421,-21.784107179335,121.947395958042)) ;
#59499=CARTESIAN_POINT('Ctrl Pts',(-19.1232547049505,-21.6041180989721,
122.240283218186)) ;
#59500=CARTESIAN_POINT('Ctrl Pts',(-18.8063639187183,-21.7939620491364,
122.030208537148)) ;
#59501=CARTESIAN_POINT('Ctrl Pts',(-18.9269353053611,-21.6139729687736,
122.306534697317)) ;
#59502=CARTESIAN_POINT('Ctrl Pts',(-18.5756220536227,-21.80396147956,122.155848712853)) ;
#59503=CARTESIAN_POINT('Ctrl Pts',(-18.7423427130502,-21.6239723991971,
122.407048265854)) ;
#59504=CARTESIAN_POINT('Ctrl Pts',(-18.3721015982493,-21.8138565970253,
122.317772569663)) ;
#59505=CARTESIAN_POINT('Ctrl Pts',(-18.5795278239004,-21.6338675166624,
122.536588260672)) ;
#59506=CARTESIAN_POINT('Ctrl Pts',(-18.1969788650756,-21.8239170905422,
122.515789157084)) ;
#59507=CARTESIAN_POINT('Ctrl Pts',(-18.4394307367387,-21.6439280101794,
122.695002760507)) ;
#59508=CARTESIAN_POINT('Ctrl Pts',(-18.0616465449145,-21.8337665707434,
122.736447563643)) ;
#59509=CARTESIAN_POINT('Ctrl Pts',(-18.3311666894869,-21.6537774903805,
122.871529616356)) ;
#59510=CARTESIAN_POINT('Ctrl Pts',(-17.9643529997641,-21.8437930210072,
122.981307539562)) ;
#59511=CARTESIAN_POINT('Ctrl Pts',(-18.2533332210301,-21.6638039406443,
123.067418172796)) ;
#59512=CARTESIAN_POINT('Ctrl Pts',(-17.911737129383,-21.8538243114853,123.239620782822)) ;
#59513=CARTESIAN_POINT('Ctrl Pts',(-18.2112421016013,-21.6738352311224,
123.274069149451)) ;
#59514=CARTESIAN_POINT('Ctrl Pts',(-17.9043414975955,-21.8636656991371,
123.498138969836)) ;
#59515=CARTESIAN_POINT('Ctrl Pts',(-18.2053271327317,-21.6836766187742,
123.480882829659)) ;
#59516=CARTESIAN_POINT('Ctrl Pts',(-17.9420552180239,-21.8736691000283,
123.758271923707)) ;
#59517=CARTESIAN_POINT('Ctrl Pts',(-18.2354994952421,-21.6936800196655,
123.688988903637)) ;
#59518=CARTESIAN_POINT('Ctrl Pts',(-18.0243333212748,-21.8836534828195,
124.007465107845)) ;
#59519=CARTESIAN_POINT('Ctrl Pts',(-18.3013232846925,-21.7036644024566,
123.888342843706)) ;
#59520=CARTESIAN_POINT('Ctrl Pts',(-18.1494974495607,-21.8936925728329,
124.239670692868)) ;
#59521=CARTESIAN_POINT('Ctrl Pts',(-18.4014559474029,-21.71370349247,124.074106700481)) ;
#59522=CARTESIAN_POINT('Ctrl Pts',(-18.3096733742783,-21.9035383817421,
124.442892027175)) ;
#59523=CARTESIAN_POINT('Ctrl Pts',(-18.5295972153698,-21.7235493013792,
124.236682156643)) ;
#59524=CARTESIAN_POINT('Ctrl Pts',(-18.5050211085327,-21.9135228045611,
124.618000034142)) ;
#59525=CARTESIAN_POINT('Ctrl Pts',(-18.6858761220133,-21.7335337241982,
124.376767460048)) ;
#59526=CARTESIAN_POINT('Ctrl Pts',(-18.7268105926817,-21.9234624298023,
124.756042327652)) ;
#59527=CARTESIAN_POINT('Ctrl Pts',(-18.8633080134688,-21.7434733494394,
124.487199981582)) ;
#59528=CARTESIAN_POINT('Ctrl Pts',(-18.9716093217471,-21.9335021193209,
124.854379340595)) ;
#59529=CARTESIAN_POINT('Ctrl Pts',(-19.0591475870826,-21.7535130389581,
124.565868438061)) ;
#59530=CARTESIAN_POINT('Ctrl Pts',(-19.2258769015638,-21.9433903077395,
124.908032136323)) ;
#59531=CARTESIAN_POINT('Ctrl Pts',(-19.2625611888641,-21.7634012273766,
124.608789286634)) ;
#59532=CARTESIAN_POINT('Ctrl Pts',(-19.4882188467763,-21.9533798337416,
124.917301153433)) ;
#59533=CARTESIAN_POINT('Ctrl Pts',(-19.4724346146083,-21.7733907533787,
124.616203339472)) ;
#59534=CARTESIAN_POINT('Ctrl Pts',(-19.7473517520323,-21.9633383350968,
124.88079179001)) ;
#59535=CARTESIAN_POINT('Ctrl Pts',(-19.679740427849,-21.7833492547339,124.586994707607)) ;
#59536=CARTESIAN_POINT('Ctrl Pts',(-19.9949571853173,-21.9732379291004,
124.800926502595)) ;
#59537=CARTESIAN_POINT('Ctrl Pts',(-19.8778237805908,-21.7932488487375,
124.523101689369)) ;
#59538=CARTESIAN_POINT('Ctrl Pts',(-20.2282969934944,-21.9832858172217,
124.67739751358)) ;
#59539=CARTESIAN_POINT('Ctrl Pts',(-20.0644952773521,-21.8032967368588,
124.424277463967)) ;
#59540=CARTESIAN_POINT('Ctrl Pts',(-20.4336615725465,-21.9931812424672,
124.51780896921)) ;
#59541=CARTESIAN_POINT('Ctrl Pts',(-20.2287857314875,-21.8131921621044,
124.296606263855)) ;
#59542=CARTESIAN_POINT('Ctrl Pts',(-20.6111028161255,-22.0032426331678,
124.321832200981)) ;
#59543=CARTESIAN_POINT('Ctrl Pts',(-20.3707381429069,-21.8232535528049,
124.139823967692)) ;
#59544=CARTESIAN_POINT('Ctrl Pts',(-20.7488672563639,-22.0130882168545,
124.102810049072)) ;
#59545=CARTESIAN_POINT('Ctrl Pts',(-20.4809482739668,-21.8330991364916,
123.964606606129)) ;
#59546=CARTESIAN_POINT('Ctrl Pts',(-20.8484784322108,-22.0230511901637,
123.860702848364)) ;
#59547=CARTESIAN_POINT('Ctrl Pts',(-20.5606363386565,-21.8430621098008,
123.770920863267)) ;
#59548=CARTESIAN_POINT('Ctrl Pts',(-20.9045567467684,-22.0330768569895,
123.603259320304)) ;
#59549=CARTESIAN_POINT('Ctrl Pts',(-20.6054981356393,-21.8530877766266,
123.564965788728)) ;
#59550=CARTESIAN_POINT('Ctrl Pts',(-20.9151055478435,-22.0429913348558,
123.342939247587)) ;
#59551=CARTESIAN_POINT('Ctrl Pts',(-20.6139362973576,-21.8630022544929,
123.356710337489)) ;
#59552=CARTESIAN_POINT('Ctrl Pts',(-20.8805485313156,-22.0529798495308,
123.082714706942)) ;
#59553=CARTESIAN_POINT('Ctrl Pts',(-20.586289982988,-21.8729907691679,123.148530979108)) ;
#59554=CARTESIAN_POINT('Ctrl Pts',(-20.8003679518013,-22.0630239604462,
122.831264561867)) ;
#59555=CARTESIAN_POINT('Ctrl Pts',(-20.5221446448977,-21.8830348800833,
122.947370978964)) ;
#59556=CARTESIAN_POINT('Ctrl Pts',(-20.6809098953037,-22.0728520980408,
122.602235481647)) ;
#59557=CARTESIAN_POINT('Ctrl Pts',(-20.4265781234052,-21.8928630176779,
122.76414910543)) ;
#59558=CARTESIAN_POINT('Ctrl Pts',(-20.5196736795458,-22.0829286660997,
122.392249516455)) ;
#59559=CARTESIAN_POINT('Ctrl Pts',(-20.2975883848863,-21.9029395857368,
122.596160459755)) ;
#59560=CARTESIAN_POINT('Ctrl Pts',(-20.328782028387,-22.0927808280039,122.217258955797)) ;
#59561=CARTESIAN_POINT('Ctrl Pts',(-20.1448754008448,-21.912791747641,122.456169202449)) ;
#59562=CARTESIAN_POINT('Ctrl Pts',(-20.1057172725599,-22.1028537899607,
122.074824536988)) ;
#59563=CARTESIAN_POINT('Ctrl Pts',(-19.9664229786563,-21.9228647095978,
122.342221984015)) ;
#59564=CARTESIAN_POINT('Ctrl Pts',(-19.8668228113398,-22.1126963519636,
121.975615871429)) ;
#59565=CARTESIAN_POINT('Ctrl Pts',(-19.7753082232677,-21.9327072716007,
122.262856048578)) ;
#59566=CARTESIAN_POINT('Ctrl Pts',(-19.6110214816132,-22.1226767884574,
121.917755554155)) ;
#59567=CARTESIAN_POINT('Ctrl Pts',(-19.5706673154193,-21.9426877080945,
122.216568229645)) ;
#59568=CARTESIAN_POINT('Ctrl Pts',(-19.3480335183811,-22.1326950937818,
121.905648968687)) ;
#59569=CARTESIAN_POINT('Ctrl Pts',(-19.3602769131939,-21.9527060134189,
122.206883477632)) ;
#59570=CARTESIAN_POINT('Ctrl Pts',(-19.090340079734,-22.1425790577013,121.938406487101)) ;
#59571=CARTESIAN_POINT('Ctrl Pts',(-19.1541230782783,-21.9625899773384,
122.233089760099)) ;
#59572=CARTESIAN_POINT('Ctrl Pts',(-18.8377600204759,-22.1526449344398,
122.016875429429)) ;
#59573=CARTESIAN_POINT('Ctrl Pts',(-18.9520588488056,-21.9726558540769,
122.295865388187)) ;
#59574=CARTESIAN_POINT('Ctrl Pts',(-18.6078114382176,-22.1624840353007,
122.135152615212)) ;
#59575=CARTESIAN_POINT('Ctrl Pts',(-18.7681011911182,-21.9824949549378,
122.390486916667)) ;
#59576=CARTESIAN_POINT('Ctrl Pts',(-18.3974600457705,-22.1725171181664,
122.294091316826)) ;
#59577=CARTESIAN_POINT('Ctrl Pts',(-18.5998201180981,-21.9925280378036,
122.517638081399)) ;
#59578=CARTESIAN_POINT('Ctrl Pts',(-18.2185627413665,-22.1825388034419,
122.487389938133)) ;
#59579=CARTESIAN_POINT('Ctrl Pts',(-18.4567025086376,-22.002549723079,122.67227724618)) ;
#59580=CARTESIAN_POINT('Ctrl Pts',(-18.0778211454052,-22.1924054985404,
122.70513209668)) ;
#59581=CARTESIAN_POINT('Ctrl Pts',(-18.3441099857594,-22.0124164181775,
122.846470267623)) ;
#59582=CARTESIAN_POINT('Ctrl Pts',(-17.9754225074273,-22.2023653882749,
122.946017980769)) ;
#59583=CARTESIAN_POINT('Ctrl Pts',(-18.2621912862455,-22.0223763079121,
123.039178659271)) ;
#59584=CARTESIAN_POINT('Ctrl Pts',(-17.9163607642041,-22.2124003761004,
123.203010659034)) ;
#59585=CARTESIAN_POINT('Ctrl Pts',(-18.2149420385229,-22.0324112957375,
123.244772955829)) ;
#59586=CARTESIAN_POINT('Ctrl Pts',(-17.9025839574836,-22.2222870801747,
123.462494584695)) ;
#59587=CARTESIAN_POINT('Ctrl Pts',(-18.2039207061201,-22.0422979998118,
123.452359223595)) ;
#59588=CARTESIAN_POINT('Ctrl Pts',(-17.9346959980839,-22.2323522244076,
123.724996117154)) ;
#59589=CARTESIAN_POINT('Ctrl Pts',(-18.2296104579225,-22.0523631440447,
123.662360751984)) ;
#59590=CARTESIAN_POINT('Ctrl Pts',(-18.0099377691919,-22.2421915151362,
123.972415043862)) ;
#59591=CARTESIAN_POINT('Ctrl Pts',(-18.2898035447589,-22.0622024347733,
123.860294755891)) ;
#59592=CARTESIAN_POINT('Ctrl Pts',(-18.1292969690806,-22.2522540725746,
124.208342841471)) ;
#59593=CARTESIAN_POINT('Ctrl Pts',(-18.3852909705668,-22.0722649922117,
124.049037294054)) ;
#59594=CARTESIAN_POINT('Ctrl Pts',(-18.2854516849338,-22.2621511238267,
124.416351010826)) ;
#59595=CARTESIAN_POINT('Ctrl Pts',(-18.5102142588833,-22.0821620434638,
124.215443190149)) ;
#59596=CARTESIAN_POINT('Ctrl Pts',(-18.4753956190122,-22.272082330575,124.595319409224)) ;
#59597=CARTESIAN_POINT('Ctrl Pts',(-18.6621688310842,-22.0920932502121,
124.358617678543)) ;
#59598=CARTESIAN_POINT('Ctrl Pts',(-18.6961275311406,-22.2821245147938,
124.739948983585)) ;
#59599=CARTESIAN_POINT('Ctrl Pts',(-18.8387544167778,-22.1021354344309,
124.47432155666)) ;
#59600=CARTESIAN_POINT('Ctrl Pts',(-18.9348029986765,-22.2920111429047,
124.842623278117)) ;
#59601=CARTESIAN_POINT('Ctrl Pts',(-19.0296939129993,-22.1120220625418,
124.556460832634)) ;
#59602=CARTESIAN_POINT('Ctrl Pts',(-19.190281558459,-22.3020044154371,124.903358057767)) ;
#59603=CARTESIAN_POINT('Ctrl Pts',(-19.2340765313827,-22.1220153350742,
124.605048920887)) ;
#59604=CARTESIAN_POINT('Ctrl Pts',(-19.4511817330596,-22.3119494909786,
124.918648968524)) ;
#59605=CARTESIAN_POINT('Ctrl Pts',(-19.442796174619,-22.1319604106157,124.61728190834)) ;
#59606=CARTESIAN_POINT('Ctrl Pts',(-19.7109595708651,-22.3218990417068,
124.888897659172)) ;
#59607=CARTESIAN_POINT('Ctrl Pts',(-19.6506180532169,-22.141909961344,124.593481323135)) ;
#59608=CARTESIAN_POINT('Ctrl Pts',(-19.963792160214,-22.3319383765548,124.813587576149)) ;
#59609=CARTESIAN_POINT('Ctrl Pts',(-19.8528843512006,-22.1519492961919,
124.533233558072)) ;
#59610=CARTESIAN_POINT('Ctrl Pts',(-20.196245173065,-22.3418245154987,124.697521392829)) ;
#59611=CARTESIAN_POINT('Ctrl Pts',(-20.0388461770694,-22.1618354351359,
124.440381365318)) ;
#59612=CARTESIAN_POINT('Ctrl Pts',(-20.4075357060316,-22.3518226284724,
124.541405526169)) ;
#59613=CARTESIAN_POINT('Ctrl Pts',(-20.2078787966008,-22.1718335481096,
124.315489143515)) ;
#59614=CARTESIAN_POINT('Ctrl Pts',(-20.5872481934702,-22.3617423908249,
124.352530361773)) ;
#59615=CARTESIAN_POINT('Ctrl Pts',(-20.3516487449868,-22.181753310462,124.164389831893)) ;
#59616=CARTESIAN_POINT('Ctrl Pts',(-20.7332188476262,-22.3717817864375,
124.132782767646)) ;
#59617=CARTESIAN_POINT('Ctrl Pts',(-20.4684258066509,-22.1917927060747,
123.988591943343)) ;
#59618=CARTESIAN_POINT('Ctrl Pts',(-20.8373803848515,-22.3816909722258,
123.894117096644)) ;
#59619=CARTESIAN_POINT('Ctrl Pts',(-20.5517552368214,-22.2017018918629,
123.797660275818)) ;
#59620=CARTESIAN_POINT('Ctrl Pts',(-20.8993918232317,-22.3916261563833,
123.640499494821)) ;
#59621=CARTESIAN_POINT('Ctrl Pts',(-20.6013649575712,-22.2116370760204,
123.594766873805)) ;
#59622=CARTESIAN_POINT('Ctrl Pts',(-20.9163470243233,-22.4016672137692,
123.377183112359)) ;
#59623=CARTESIAN_POINT('Ctrl Pts',(-20.6149297759424,-22.2216781334063,
123.38411366101)) ;
#59624=CARTESIAN_POINT('Ctrl Pts',(-20.8879521472035,-22.4115543718025,
123.118900643946)) ;
#59625=CARTESIAN_POINT('Ctrl Pts',(-20.5922146560384,-22.2315652914396,
123.177488436444)) ;
#59626=CARTESIAN_POINT('Ctrl Pts',(-20.8147966666412,-22.4215466514784,
122.866729097642)) ;
#59627=CARTESIAN_POINT('Ctrl Pts',(-20.5336910860111,-22.2415575711155,
122.97575113261)) ;
#59628=CARTESIAN_POINT('Ctrl Pts',(-20.6993946933195,-22.4314951685235,
122.632124438289)) ;
#59629=CARTESIAN_POINT('Ctrl Pts',(-20.4413704002996,-22.2515060881606,
122.788067448919)) ;
#59630=CARTESIAN_POINT('Ctrl Pts',(-20.5455120187168,-22.4414319460939,
122.421182047729)) ;
#59631=CARTESIAN_POINT('Ctrl Pts',(-20.3182652644741,-22.261442865731,122.619313435312)) ;
#59632=CARTESIAN_POINT('Ctrl Pts',(-20.3566546113368,-22.4514149822408,
122.239043334206)) ;
#59633=CARTESIAN_POINT('Ctrl Pts',(-20.1671801441174,-22.2714259018779,
122.473601924756)) ;
#59634=CARTESIAN_POINT('Ctrl Pts',(-20.1374997937318,-22.4614587338345,
122.092007982459)) ;
#59635=CARTESIAN_POINT('Ctrl Pts',(-19.9918566291476,-22.2814696534717,
122.355972866551)) ;
#59636=CARTESIAN_POINT('Ctrl Pts',(-19.9014984819869,-22.4712872630471,
121.986966332369)) ;
#59637=CARTESIAN_POINT('Ctrl Pts',(-19.803057030311,-22.2912981826842,122.27193912262)) ;
#59638=CARTESIAN_POINT('Ctrl Pts',(-19.644672669795,-22.4813626239558,121.922812414429)) ;
#59639=CARTESIAN_POINT('Ctrl Pts',(-19.5975962939444,-22.3013735435929,
122.220614925738)) ;
#59640=CARTESIAN_POINT('Ctrl Pts',(-19.3862413607618,-22.491219222843,121.904531259593)) ;
#59641=CARTESIAN_POINT('Ctrl Pts',(-19.3908522878681,-22.3112301424801,
122.205989042091)) ;
#59642=CARTESIAN_POINT('Ctrl Pts',(-19.1232446773172,-22.5012822168609,
121.931678446646)) ;
#59643=CARTESIAN_POINT('Ctrl Pts',(-19.1804545703553,-22.321293136498,122.227705729695)) ;
#59644=CARTESIAN_POINT('Ctrl Pts',(-18.8735448281778,-22.5111601511503,
122.002791143889)) ;
#59645=CARTESIAN_POINT('Ctrl Pts',(-18.9806951761436,-22.3311710707875,
122.284594621574)) ;
#59646=CARTESIAN_POINT('Ctrl Pts',(-18.6369922199882,-22.5211607987084,
122.117182286071)) ;
#59647=CARTESIAN_POINT('Ctrl Pts',(-18.7914526693458,-22.3411717183456,
122.376106428338)) ;
#59648=CARTESIAN_POINT('Ctrl Pts',(-18.4254683343915,-22.5310786451465,
122.269531684477)) ;
#59649=CARTESIAN_POINT('Ctrl Pts',(-18.6222333099972,-22.3510895647836,
122.497984627214)) ;
#59650=CARTESIAN_POINT('Ctrl Pts',(-18.2412825269459,-22.5411297621521,
122.45879123557)) ;
#59651=CARTESIAN_POINT('Ctrl Pts',(-18.4748836852717,-22.3611406817893,
122.649391549011)) ;
#59652=CARTESIAN_POINT('Ctrl Pts',(-18.0951286476762,-22.5510004974627,
122.673148447113)) ;
#59653=CARTESIAN_POINT('Ctrl Pts',(-18.3579599995673,-22.3710114170999,
122.820875923692)) ;
#59654=CARTESIAN_POINT('Ctrl Pts',(-17.986241610246,-22.5610712047057,122.914310640418)) ;
#59655=CARTESIAN_POINT('Ctrl Pts',(-18.270849088114,-22.3810821243429,123.013805409563)) ;
#59656=CARTESIAN_POINT('Ctrl Pts',(-17.9222939724761,-22.5709042121576,
123.164699747312)) ;
#59657=CARTESIAN_POINT('Ctrl Pts',(-18.2196899694515,-22.3909151317947,
123.214115380671)) ;
#59658=CARTESIAN_POINT('Ctrl Pts',(-17.9016542679233,-22.5809347044599,
123.427471548306)) ;
#59659=CARTESIAN_POINT('Ctrl Pts',(-18.2031767454531,-22.400945624097,123.424332776703)) ;
#59660=CARTESIAN_POINT('Ctrl Pts',(-17.927723884169,-22.5909662995333,123.689813957202)) ;
#59661=CARTESIAN_POINT('Ctrl Pts',(-18.2240311522087,-22.4109772191704,
123.634206897862)) ;
#59662=CARTESIAN_POINT('Ctrl Pts',(-17.9969878123147,-22.6007959986715,
123.93865131243)) ;
#59663=CARTESIAN_POINT('Ctrl Pts',(-18.2794406618939,-22.4208069183087,
123.833276183553)) ;
#59664=CARTESIAN_POINT('Ctrl Pts',(-18.1095198729244,-22.6107854485531,
124.175829191989)) ;
#59665=CARTESIAN_POINT('Ctrl Pts',(-18.3694648327991,-22.4307963681902,
124.023019031505)) ;
#59666=CARTESIAN_POINT('Ctrl Pts',(-18.2628916857644,-22.6208293063688,
124.390633246382)) ;
#59667=CARTESIAN_POINT('Ctrl Pts',(-18.4921611832323,-22.4408402260059,
124.194863205091)) ;
#59668=CARTESIAN_POINT('Ctrl Pts',(-18.446692434265,-22.630650996959,124.571839161793)) ;
#59669=CARTESIAN_POINT('Ctrl Pts',(-18.6391999895716,-22.4506619165961,
124.339828335497)) ;
#59670=CARTESIAN_POINT('Ctrl Pts',(-18.6634124377873,-22.6406860874994,
124.722085054435)) ;
#59671=CARTESIAN_POINT('Ctrl Pts',(-18.8125751167322,-22.4606970071365,
124.460026463756)) ;
#59672=CARTESIAN_POINT('Ctrl Pts',(-18.9029886662497,-22.6507106064821,
124.831675526016)) ;
#59673=CARTESIAN_POINT('Ctrl Pts',(-19.0042354735576,-22.4707215261192,
124.547700237809)) ;
#59674=CARTESIAN_POINT('Ctrl Pts',(-19.1536198777574,-22.6605704518923,
124.897332264122)) ;
#59675=CARTESIAN_POINT('Ctrl Pts',(-19.204739284053,-22.4805813715294,124.600226994176)) ;
#59676=CARTESIAN_POINT('Ctrl Pts',(-19.4144244913002,-22.670530228208,124.919409092967)) ;
#59677=CARTESIAN_POINT('Ctrl Pts',(-19.4133825651792,-22.4905411478451,
124.617890170222)) ;
#59678=CARTESIAN_POINT('Ctrl Pts',(-19.6768496651292,-22.6805584255226,
124.895342097645)) ;
#59679=CARTESIAN_POINT('Ctrl Pts',(-19.6233228939347,-22.5005693451597,
124.598638241263)) ;
#59680=CARTESIAN_POINT('Ctrl Pts',(-19.9281559636117,-22.6904659678129,
124.827199646983)) ;
#59681=CARTESIAN_POINT('Ctrl Pts',(-19.8243678986999,-22.51047688745,124.544126081424)) ;
#59682=CARTESIAN_POINT('Ctrl Pts',(-20.1667897461997,-22.7004986183768,
124.715157775083)) ;
#59683=CARTESIAN_POINT('Ctrl Pts',(-20.0152757027157,-22.5205095380139,
124.454494146685)) ;
#59684=CARTESIAN_POINT('Ctrl Pts',(-20.3792168210052,-22.7103825748034,
124.56567950925)) ;
#59685=CARTESIAN_POINT('Ctrl Pts',(-20.1852178909652,-22.5303934944406,
124.334913312455)) ;
#59686=CARTESIAN_POINT('Ctrl Pts',(-20.5648833309736,-22.7203722761653,
124.380082284069)) ;
#59687=CARTESIAN_POINT('Ctrl Pts',(-20.333752327996,-22.5403831958024,124.18643693813)) ;
#59688=CARTESIAN_POINT('Ctrl Pts',(-20.7158142403492,-22.7304132714413,
124.163643559951)) ;
#59689=CARTESIAN_POINT('Ctrl Pts',(-20.454498551908,-22.5504241910784,124.013286914038)) ;
#59690=CARTESIAN_POINT('Ctrl Pts',(-20.8249543879318,-22.7402461607097,
123.929430163563)) ;
#59691=CARTESIAN_POINT('Ctrl Pts',(-20.5418120172613,-22.5602570803468,
123.825917666245)) ;
#59692=CARTESIAN_POINT('Ctrl Pts',(-20.8935867559205,-22.7502393190771,
123.675951817842)) ;
#59693=CARTESIAN_POINT('Ctrl Pts',(-20.5967197715693,-22.5702502387142,
123.623135597207)) ;
#59694=CARTESIAN_POINT('Ctrl Pts',(-20.9167106283028,-22.7602713614292,
123.413324039136)) ;
#59695=CARTESIAN_POINT('Ctrl Pts',(-20.6152207367782,-22.5802822810663,
123.413033509542)) ;
#59696=CARTESIAN_POINT('Ctrl Pts',(-20.8945827853963,-22.7701366053876,
123.155034786092)) ;
#59697=CARTESIAN_POINT('Ctrl Pts',(-20.5975204254551,-22.5901475250248,
123.206402523635)) ;
#59698=CARTESIAN_POINT('Ctrl Pts',(-20.82800234089,-22.7800984966336,122.901847296241)) ;
#59699=CARTESIAN_POINT('Ctrl Pts',(-20.5442580738547,-22.6001094162708,
123.003852212977)) ;
#59700=CARTESIAN_POINT('Ctrl Pts',(-20.7172881603951,-22.7901333966521,
122.662521920387)) ;
#59701=CARTESIAN_POINT('Ctrl Pts',(-20.4556884995148,-22.6101443162892,
122.812391063934)) ;
#59702=CARTESIAN_POINT('Ctrl Pts',(-20.5692752424808,-22.8000184770667,
122.449004039222)) ;
#59703=CARTESIAN_POINT('Ctrl Pts',(-20.3372800779245,-22.6200293967038,
122.641575980296)) ;
#59704=CARTESIAN_POINT('Ctrl Pts',(-20.3831352080727,-22.8100836491915,
122.261135086256)) ;
#59705=CARTESIAN_POINT('Ctrl Pts',(-20.1883694027549,-22.6300945688287,
122.491279318454)) ;
#59706=CARTESIAN_POINT('Ctrl Pts',(-20.1719153765991,-22.819930883915,122.111588554488)) ;
#59707=CARTESIAN_POINT('Ctrl Pts',(-20.0193951546591,-22.6399418035521,
122.37164074922)) ;
#59708=CARTESIAN_POINT('Ctrl Pts',(-19.9338810019722,-22.8299616952328,
121.998385955222)) ;
#59709=CARTESIAN_POINT('Ctrl Pts',(-19.8289685381442,-22.6499726148699,
122.281076763213)) ;
#59710=CARTESIAN_POINT('Ctrl Pts',(-19.6801542546242,-22.8399713111463,
121.928888950712)) ;
#59711=CARTESIAN_POINT('Ctrl Pts',(-19.6259877257716,-22.6599822307834,
122.225477204985)) ;
#59712=CARTESIAN_POINT('Ctrl Pts',(-19.4208786354196,-22.84988209055,121.904493618432)) ;
#59713=CARTESIAN_POINT('Ctrl Pts',(-19.4185677565269,-22.6698930101871,
122.20595890965)) ;
#59714=CARTESIAN_POINT('Ctrl Pts',(-19.1607322268354,-22.859811356339,121.924877430898)) ;
#59715=CARTESIAN_POINT('Ctrl Pts',(-19.2104507120868,-22.6798222759761,
122.222263811396)) ;
#59716=CARTESIAN_POINT('Ctrl Pts',(-18.9052696006217,-22.8698540496516,
121.991077325652)) ;
#59717=CARTESIAN_POINT('Ctrl Pts',(-19.0060800555527,-22.6898649692887,
122.275221687729)) ;
#59718=CARTESIAN_POINT('Ctrl Pts',(-18.6688210508467,-22.8797405823464,
122.098781259546)) ;
#59719=CARTESIAN_POINT('Ctrl Pts',(-18.8169206428243,-22.6997515019835,
122.361382756701)) ;
#59720=CARTESIAN_POINT('Ctrl Pts',(-18.4521283292672,-22.8897337274496,
122.247107144986)) ;
#59721=CARTESIAN_POINT('Ctrl Pts',(-18.6435653091888,-22.7097446470868,
122.480041629506)) ;
#59722=CARTESIAN_POINT('Ctrl Pts',(-18.2654318576276,-22.8996794081237,
122.430014319229)) ;
#59723=CARTESIAN_POINT('Ctrl Pts',(-18.4942067535944,-22.7196903277608,
122.626365697427)) ;
#59724=CARTESIAN_POINT('Ctrl Pts',(-18.1128639588266,-22.9096266657504,
122.642292140986)) ;
#59725=CARTESIAN_POINT('Ctrl Pts',(-18.372150743422,-22.7296375853876,122.796186542585)) ;
#59726=CARTESIAN_POINT('Ctrl Pts',(-17.9986015572507,-22.9196745678719,
122.880328253833)) ;
#59727=CARTESIAN_POINT('Ctrl Pts',(-18.280738856107,-22.739685487509,122.986614497746)) ;
#59728=CARTESIAN_POINT('Ctrl Pts',(-17.9286121291567,-22.9295222734936,
123.129473138919)) ;
#59729=CARTESIAN_POINT('Ctrl Pts',(-18.2247452886835,-22.7495331931307,
123.18592950677)) ;
#59730=CARTESIAN_POINT('Ctrl Pts',(-17.9018275042711,-22.9394837401277,
123.389866644002)) ;
#59731=CARTESIAN_POINT('Ctrl Pts',(-18.2033153717119,-22.7594946597648,
123.394243983057)) ;
#59732=CARTESIAN_POINT('Ctrl Pts',(-17.9211473399048,-22.9495132933959,
123.652733485376)) ;
#59733=CARTESIAN_POINT('Ctrl Pts',(-18.2187690258878,-22.769524213033,123.604537583863)) ;
#59734=CARTESIAN_POINT('Ctrl Pts',(-17.9848788717473,-22.9594201854233,
123.905158576402)) ;
#59735=CARTESIAN_POINT('Ctrl Pts',(-18.2697520510413,-22.7794311050604,
123.806478038071)) ;
#59736=CARTESIAN_POINT('Ctrl Pts',(-18.0914378078134,-22.9693678295363,
124.143845240036)) ;
#59737=CARTESIAN_POINT('Ctrl Pts',(-18.3549971072633,-22.7893787491735,
123.997428193049)) ;
#59738=CARTESIAN_POINT('Ctrl Pts',(-18.2384883382395,-22.9793678725652,
124.361682579422)) ;
#59739=CARTESIAN_POINT('Ctrl Pts',(-18.4726356373326,-22.7993787922023,
124.17169927459)) ;
#59740=CARTESIAN_POINT('Ctrl Pts',(-18.4221353271476,-22.9894066385592,
124.551044334108)) ;
#59741=CARTESIAN_POINT('Ctrl Pts',(-18.6195515901072,-22.8094175581963,
124.323190202852)) ;
#59742=CARTESIAN_POINT('Ctrl Pts',(-18.6310313255418,-22.9992317005814,
124.702816918751)) ;
#59743=CARTESIAN_POINT('Ctrl Pts',(-18.7866669492004,-22.8192426202186,
124.444610004211)) ;
#59744=CARTESIAN_POINT('Ctrl Pts',(-18.8683046803637,-23.0092862479078,
124.81903454041)) ;
#59745=CARTESIAN_POINT('Ctrl Pts',(-18.9764846127344,-22.8292971675449,
124.537586113637)) ;
#59746=CARTESIAN_POINT('Ctrl Pts',(-19.1194917233323,-23.019229491357,124.891049871198)) ;
#59747=CARTESIAN_POINT('Ctrl Pts',(-19.1774335457929,-22.8392404109942,
124.59520052088)) ;
#59748=CARTESIAN_POINT('Ctrl Pts',(-19.3782034066478,-23.0291316629649,
124.919048155738)) ;
#59749=CARTESIAN_POINT('Ctrl Pts',(-19.3844026140547,-22.849142582602,124.617601382244)) ;
#59750=CARTESIAN_POINT('Ctrl Pts',(-19.6417720055539,-23.0391844985751,
124.9012746228)) ;
#59751=CARTESIAN_POINT('Ctrl Pts',(-19.5952575647132,-22.8591954182122,
124.603384820688)) ;
#59752=CARTESIAN_POINT('Ctrl Pts',(-19.8937094829923,-23.0490575562606,
124.839234191459)) ;
#59753=CARTESIAN_POINT('Ctrl Pts',(-19.7968081119254,-22.8690684758978,
124.553754624461)) ;
#59754=CARTESIAN_POINT('Ctrl Pts',(-20.1342348698061,-23.0590528177863,
124.733693798384)) ;
#59755=CARTESIAN_POINT('Ctrl Pts',(-19.9892291535961,-22.8790637374234,
124.469324531308)) ;
#59756=CARTESIAN_POINT('Ctrl Pts',(-20.3531841875638,-23.0690781872068,
124.587158170132)) ;
#59757=CARTESIAN_POINT('Ctrl Pts',(-20.1643902941915,-22.8890891068439,
124.352097370289)) ;
#59758=CARTESIAN_POINT('Ctrl Pts',(-20.5410358788454,-23.0789680197334,
124.407538039965)) ;
#59759=CARTESIAN_POINT('Ctrl Pts',(-20.3146713621505,-22.8989789393705,
124.208404998467)) ;
#59760=CARTESIAN_POINT('Ctrl Pts',(-20.74814931711,-23.0922659905428,124.126127329763)) ;
#59761=CARTESIAN_POINT('Ctrl Pts',(-20.4803737638767,-22.9122769101799,
123.98326757738)) ;
#59762=CARTESIAN_POINT('Ctrl Pts',(-20.87663678955,-23.105464385652,123.799667857733)) ;
#59763=CARTESIAN_POINT('Ctrl Pts',(-20.58316718686,-22.9254753052891,123.722071594726)) ;
#59764=CARTESIAN_POINT('Ctrl Pts',(-20.9162580761209,-23.1188598279314,
123.449902418922)) ;
#59765=CARTESIAN_POINT('Ctrl Pts',(-20.6148571213026,-22.9388707475686,
123.442305273441)) ;
#59766=CARTESIAN_POINT('Ctrl Pts',(-20.9004717403109,-23.1287356661704,
123.190816756868)) ;
#59767=CARTESIAN_POINT('Ctrl Pts',(-20.6022321474832,-22.9487465858075,
123.235027218103)) ;
#59768=CARTESIAN_POINT('Ctrl Pts',(-20.8389416666321,-23.1387970687681,
122.933714939038)) ;
#59769=CARTESIAN_POINT('Ctrl Pts',(-20.5530100608366,-22.9588079884053,
123.029348080478)) ;
#59770=CARTESIAN_POINT('Ctrl Pts',(-20.7357971607144,-23.1486621257033,
122.69583283738)) ;
#59771=CARTESIAN_POINT('Ctrl Pts',(-20.4704951899831,-22.9686730453404,
122.839039863601)) ;
#59772=CARTESIAN_POINT('Ctrl Pts',(-20.5912157870178,-23.1586742216521,
122.476050346887)) ;
#59773=CARTESIAN_POINT('Ctrl Pts',(-20.3548367390331,-22.9786851412892,
122.663215848403)) ;
#59774=CARTESIAN_POINT('Ctrl Pts',(-20.3516936594044,-23.1719515307975,
122.222286259416)) ;
#59775=CARTESIAN_POINT('Ctrl Pts',(-20.1631968596537,-22.9919624504346,
122.460187975031)) ;
#59776=CARTESIAN_POINT('Ctrl Pts',(-19.9764398067608,-23.1885505563048,
121.990323874655)) ;
#59777=CARTESIAN_POINT('Ctrl Pts',(-19.8630376390117,-23.0085614759419,
122.27463286839)) ;
#59778=CARTESIAN_POINT('Ctrl Pts',(-19.5445846288261,-23.2051496043378,
121.900290049291)) ;
#59779=CARTESIAN_POINT('Ctrl Pts',(-19.5174874237851,-23.025160523975,122.202591932357)) ;
#59780=CARTESIAN_POINT('Ctrl Pts',(-19.197050432373,-23.2183930163688,121.919316506906)) ;
#59781=CARTESIAN_POINT('Ctrl Pts',(-19.2395130687559,-23.0384039360059,
122.217815974426)) ;
#59782=CARTESIAN_POINT('Ctrl Pts',(-18.9401631491161,-23.2284304440572,
121.979134289703)) ;
#59783=CARTESIAN_POINT('Ctrl Pts',(-19.0339916375281,-23.0484413636943,
122.26566763804)) ;
#59784=CARTESIAN_POINT('Ctrl Pts',(-18.7007825062615,-23.2383347460128,
122.08131781826)) ;
#59785=CARTESIAN_POINT('Ctrl Pts',(-18.8424912391791,-23.0583456656499,
122.347410849636)) ;
#59786=CARTESIAN_POINT('Ctrl Pts',(-18.4082618728628,-23.251601585988,122.271030307521)) ;
#59787=CARTESIAN_POINT('Ctrl Pts',(-18.60846034993,-23.0716125056251,122.499189722715)) ;
#59788=CARTESIAN_POINT('Ctrl Pts',(-18.1123399887699,-23.2682277840779,
122.599191193754)) ;
#59789=CARTESIAN_POINT('Ctrl Pts',(-18.37173453001,-23.088238703715,122.761707661206)) ;
#59790=CARTESIAN_POINT('Ctrl Pts',(-17.9131297581632,-23.2881468994613,
123.089717711788)) ;
#59791=CARTESIAN_POINT('Ctrl Pts',(-18.2123565653371,-23.1081578190985,
123.154114524712)) ;
#59792=CARTESIAN_POINT('Ctrl Pts',(-17.8962057487813,-23.3047533225956,
123.530754190466)) ;
#59793=CARTESIAN_POINT('Ctrl Pts',(-18.1988208182487,-23.1247642422327,
123.506996945006)) ;
#59794=CARTESIAN_POINT('Ctrl Pts',(-17.9736383080703,-23.3180495430913,
123.871481315084)) ;
#59795=CARTESIAN_POINT('Ctrl Pts',(-18.260758884604,-23.1380604627284,123.779530840826)) ;
#59796=CARTESIAN_POINT('Ctrl Pts',(-18.1080876895051,-23.3313183754327,
124.193291225439)) ;
#59797=CARTESIAN_POINT('Ctrl Pts',(-18.3683238288418,-23.1513292950698,
124.03699746914)) ;
#59798=CARTESIAN_POINT('Ctrl Pts',(-18.3795904845808,-23.3480096234658,
124.544002089629)) ;
#59799=CARTESIAN_POINT('Ctrl Pts',(-18.5855160258156,-23.1680205431029,
124.317555357592)) ;
#59800=CARTESIAN_POINT('Ctrl Pts',(-18.8243580038784,-23.3678193551386,
124.825895671555)) ;
#59801=CARTESIAN_POINT('Ctrl Pts',(-18.9413318339364,-23.1878302747757,
124.543077599675)) ;
#59802=CARTESIAN_POINT('Ctrl Pts',(-19.3426692477421,-23.3877969624672,
124.941057197669)) ;
#59803=CARTESIAN_POINT('Ctrl Pts',(-19.3559797197809,-23.2078078821043,
124.635208534349)) ;
#59804=CARTESIAN_POINT('Ctrl Pts',(-19.8676443126626,-23.407723271525,124.871649885225)) ;
#59805=CARTESIAN_POINT('Ctrl Pts',(-19.7759608640312,-23.2277341911621,
124.579685870567)) ;
#59806=CARTESIAN_POINT('Ctrl Pts',(-20.3358743901566,-23.4275401316897,
124.630155280585)) ;
#59807=CARTESIAN_POINT('Ctrl Pts',(-20.1505472945724,-23.2475510513268,
124.386491407269)) ;
#59808=CARTESIAN_POINT('Ctrl Pts',(-20.6978674016167,-23.4476399472837,
124.237525821763)) ;
#59809=CARTESIAN_POINT('Ctrl Pts',(-20.4401428874829,-23.2676508669208,
124.072390151263)) ;
#59810=CARTESIAN_POINT('Ctrl Pts',(-20.9010174941863,-23.4673969111663,
123.753071870117)) ;
#59811=CARTESIAN_POINT('Ctrl Pts',(-20.6026658029561,-23.2874078308034,
123.684825804928)) ;
#59812=CARTESIAN_POINT('Ctrl Pts',(-20.9280426935608,-23.4874338372357,
123.221391133714)) ;
#59813=CARTESIAN_POINT('Ctrl Pts',(-20.6242875973045,-23.3074447568728,
123.259481619139)) ;
#59814=CARTESIAN_POINT('Ctrl Pts',(-20.772426096765,-23.5073034196172,122.716597558778)) ;
#59815=CARTESIAN_POINT('Ctrl Pts',(-20.4997956703775,-23.3273143392544,
122.855645015619)) ;
#59816=CARTESIAN_POINT('Ctrl Pts',(-20.4545393933605,-23.5272079913704,
122.293853597091)) ;
#59817=CARTESIAN_POINT('Ctrl Pts',(-20.245486515064,-23.3472189110075,122.517448272747)) ;
#59818=CARTESIAN_POINT('Ctrl Pts',(-20.0102149504557,-23.5471605935689,
122.004204373971)) ;
#59819=CARTESIAN_POINT('Ctrl Pts',(-19.8900270498159,-23.367171513206,122.28572785493)) ;
#59820=CARTESIAN_POINT('Ctrl Pts',(-19.4949902616942,-23.5670700845392,
121.884042017214)) ;
#59821=CARTESIAN_POINT('Ctrl Pts',(-19.477846400596,-23.3870810041763,122.189596888272)) ;
#59822=CARTESIAN_POINT('Ctrl Pts',(-18.9708122647659,-23.5869214532386,
121.94527950064)) ;
#59823=CARTESIAN_POINT('Ctrl Pts',(-19.0585021151188,-23.4069323728757,
122.23858718962)) ;
#59824=CARTESIAN_POINT('Ctrl Pts',(-18.4941229340544,-23.6070016493746,
122.185035924344)) ;
#59825=CARTESIAN_POINT('Ctrl Pts',(-18.6771515404996,-23.4270125690117,
122.43039179208)) ;
#59826=CARTESIAN_POINT('Ctrl Pts',(-18.1327837985555,-23.62680259295,122.567847534588)) ;
#59827=CARTESIAN_POINT('Ctrl Pts',(-18.3880785930256,-23.4468135125871,
122.736642978161)) ;
#59828=CARTESIAN_POINT('Ctrl Pts',(-17.9208269264055,-23.6467865694595,
123.054772698368)) ;
#59829=CARTESIAN_POINT('Ctrl Pts',(-18.2185138580659,-23.4667974890966,
123.126183626084)) ;
#59830=CARTESIAN_POINT('Ctrl Pts',(-17.8886839110732,-23.6667025324351,
123.583127051767)) ;
#59831=CARTESIAN_POINT('Ctrl Pts',(-18.1928000784033,-23.4867134520722,
123.548868146991)) ;
#59832=CARTESIAN_POINT('Ctrl Pts',(-18.0370543006657,-23.686572967257,124.090087584522)) ;
#59833=CARTESIAN_POINT('Ctrl Pts',(-18.3114982241245,-23.5065838868942,
123.954437479053)) ;
#59834=CARTESIAN_POINT('Ctrl Pts',(-18.3529120736301,-23.7066232524901,
124.519105466772)) ;
#59835=CARTESIAN_POINT('Ctrl Pts',(-18.5641852225777,-23.5266341721272,
124.297650597675)) ;
#59836=CARTESIAN_POINT('Ctrl Pts',(-18.789984541274,-23.7263972212494,124.811340607854)) ;
#59837=CARTESIAN_POINT('Ctrl Pts',(-18.9138460145566,-23.5464081408865,
124.531438476037)) ;
#59838=CARTESIAN_POINT('Ctrl Pts',(-19.3073372095614,-23.746453679369,124.93893490729)) ;
#59839=CARTESIAN_POINT('Ctrl Pts',(-19.3277281762554,-23.5664645990061,
124.633511759487)) ;
#59840=CARTESIAN_POINT('Ctrl Pts',(-19.8306051755044,-23.76624856236,124.882843707526)) ;
#59841=CARTESIAN_POINT('Ctrl Pts',(-19.7463441186502,-23.5862594819971,
124.588636471734)) ;
#59842=CARTESIAN_POINT('Ctrl Pts',(-20.3078444224997,-23.7862152176623,
124.651011447722)) ;
#59843=CARTESIAN_POINT('Ctrl Pts',(-20.1281345081567,-23.6062261372994,
124.40316804433)) ;
#59844=CARTESIAN_POINT('Ctrl Pts',(-20.6767016461882,-23.8061741877388,
124.269621393362)) ;
#59845=CARTESIAN_POINT('Ctrl Pts',(-20.4232185854534,-23.6261851073759,
124.09805398004)) ;
#59846=CARTESIAN_POINT('Ctrl Pts',(-20.892884068729,-23.8260702753289,123.787054530312)) ;
#59847=CARTESIAN_POINT('Ctrl Pts',(-20.5961622166163,-23.6460811949661,
123.711998606436)) ;
#59848=CARTESIAN_POINT('Ctrl Pts',(-20.9320464014087,-23.8459684452405,
123.259690813219)) ;
#59849=CARTESIAN_POINT('Ctrl Pts',(-20.6274889756677,-23.6659793648776,
123.290106706066)) ;
#59850=CARTESIAN_POINT('Ctrl Pts',(-20.7893616368976,-23.8658742806076,
122.750190072207)) ;
#59851=CARTESIAN_POINT('Ctrl Pts',(-20.5133377383693,-23.6858852002447,
122.882506513553)) ;
#59852=CARTESIAN_POINT('Ctrl Pts',(-20.4807327588592,-23.8858242055455,
122.319088447684)) ;
#59853=CARTESIAN_POINT('Ctrl Pts',(-20.2664316366618,-23.7058351251827,
122.537627039628)) ;
#59854=CARTESIAN_POINT('Ctrl Pts',(-20.0452649316201,-23.9057033954559,
122.019778092239)) ;
#59855=CARTESIAN_POINT('Ctrl Pts',(-19.9180547884745,-23.725714315093,122.298181446568)) ;
#59856=CARTESIAN_POINT('Ctrl Pts',(-19.5313379424967,-23.9256847197365,
121.886108846057)) ;
#59857=CARTESIAN_POINT('Ctrl Pts',(-19.5069121971362,-23.7456956393736,
122.191249793125)) ;
#59858=CARTESIAN_POINT('Ctrl Pts',(-19.0038793190178,-23.9456145039448,
121.936000230857)) ;
#59859=CARTESIAN_POINT('Ctrl Pts',(-19.084945405429,-23.765625423582,122.231166579714)) ;
#59860=CARTESIAN_POINT('Ctrl Pts',(-18.5255093850671,-23.9655344933356,
122.162577000674)) ;
#59861=CARTESIAN_POINT('Ctrl Pts',(-18.70225086222,-23.7855454129728,122.412432333271)) ;
#59862=CARTESIAN_POINT('Ctrl Pts',(-18.1533588423712,-23.9853896886896,
122.536910497568)) ;
#59863=CARTESIAN_POINT('Ctrl Pts',(-18.4045331019949,-23.8054006083268,
122.711900044301)) ;
#59864=CARTESIAN_POINT('Ctrl Pts',(-17.9297252155865,-24.005435690349,123.020349675099)) ;
#59865=CARTESIAN_POINT('Ctrl Pts',(-18.225629991919,-23.8254466099861,123.098661705087)) ;
#59866=CARTESIAN_POINT('Ctrl Pts',(-17.8922881637436,-24.0219354375588,
123.457418896112)) ;
#59867=CARTESIAN_POINT('Ctrl Pts',(-18.1956840852011,-23.8419463571959,
123.448290621712)) ;
#59868=CARTESIAN_POINT('Ctrl Pts',(-17.9536182369137,-24.0353240420069,
123.803823185436)) ;
#59869=CARTESIAN_POINT('Ctrl Pts',(-18.2447511118131,-23.855334961644,123.725437823404)) ;
#59870=CARTESIAN_POINT('Ctrl Pts',(-18.0424306542549,-24.0451858703418,
124.047300970856)) ;
#59871=CARTESIAN_POINT('Ctrl Pts',(-18.3158010379649,-23.8651967899789,
123.920212948107)) ;
#59872=CARTESIAN_POINT('Ctrl Pts',(-18.1728224348044,-24.0551520130994,
124.274441107709)) ;
#59873=CARTESIAN_POINT('Ctrl Pts',(-18.4201247042669,-23.8751629327365,
124.101932317986)) ;
#59874=CARTESIAN_POINT('Ctrl Pts',(-18.398315477012,-24.0685137592243,124.543527593381)) ;
#59875=CARTESIAN_POINT('Ctrl Pts',(-18.600479724246,-23.8885246788614,124.317163946771)) ;
#59876=CARTESIAN_POINT('Ctrl Pts',(-18.7557534014151,-24.0849680881794,
124.795766078304)) ;
#59877=CARTESIAN_POINT('Ctrl Pts',(-18.8864880582342,-23.9049790078165,
124.518993913012)) ;
#59878=CARTESIAN_POINT('Ctrl Pts',(-19.1855079887731,-24.1017353332277,
124.913045707015)) ;
#59879=CARTESIAN_POINT('Ctrl Pts',(-19.2302449597953,-23.9217462528648,
124.61279458323)) ;
#59880=CARTESIAN_POINT('Ctrl Pts',(-19.5321625871901,-24.1149218985017,
124.914163508115)) ;
#59881=CARTESIAN_POINT('Ctrl Pts',(-19.5076007478974,-23.9349328181389,
124.613694249745)) ;
#59882=CARTESIAN_POINT('Ctrl Pts',(-19.7909027433267,-24.1249113572463,
124.870218955293)) ;
#59883=CARTESIAN_POINT('Ctrl Pts',(-19.7145860227272,-23.9449222768835,
124.578534711631)) ;
#59884=CARTESIAN_POINT('Ctrl Pts',(-20.0373293987813,-24.1348651297274,
124.782335916118)) ;
#59885=CARTESIAN_POINT('Ctrl Pts',(-19.9117282978741,-23.9548760493646,
124.508226619746)) ;
#59886=CARTESIAN_POINT('Ctrl Pts',(-20.2667248444726,-24.1449129462601,
124.651640371251)) ;
#59887=CARTESIAN_POINT('Ctrl Pts',(-20.0952430132553,-23.9649238658972,
124.403668150689)) ;
#59888=CARTESIAN_POINT('Ctrl Pts',(-20.4660081191832,-24.1547544793826,
124.486757064472)) ;
#59889=CARTESIAN_POINT('Ctrl Pts',(-20.2546683482556,-23.9747653990197,
124.27175978153)) ;
#59890=CARTESIAN_POINT('Ctrl Pts',(-20.6364815530708,-24.1647407216023,
124.287296273843)) ;
#59891=CARTESIAN_POINT('Ctrl Pts',(-20.3910452989074,-23.9847516412394,
124.112189719401)) ;
#59892=CARTESIAN_POINT('Ctrl Pts',(-20.7692271456916,-24.1746773450272,
124.062380424929)) ;
#59893=CARTESIAN_POINT('Ctrl Pts',(-20.497239809877,-23.9946882646643,123.932255945756)) ;
#59894=CARTESIAN_POINT('Ctrl Pts',(-20.8617993883025,-24.1847272224102,
123.815064619583)) ;
#59895=CARTESIAN_POINT('Ctrl Pts',(-20.5712954677108,-24.0047381420473,
123.734402552555)) ;
#59896=CARTESIAN_POINT('Ctrl Pts',(-20.9092661000716,-24.1945776611878,
123.560575071859)) ;
#59897=CARTESIAN_POINT('Ctrl Pts',(-20.6092666006814,-24.0145885808249,
123.53081059359)) ;
#59898=CARTESIAN_POINT('Ctrl Pts',(-20.9125392723098,-24.2045496751565,
123.298574461719)) ;
#59899=CARTESIAN_POINT('Ctrl Pts',(-20.6118828876205,-24.0245605947936,
123.3212101705)) ;
#59900=CARTESIAN_POINT('Ctrl Pts',(-20.8701252717379,-24.2145448437826,
123.039316830709)) ;
#59901=CARTESIAN_POINT('Ctrl Pts',(-20.5779494825875,-24.0345557634197,
123.113804490714)) ;
#59902=CARTESIAN_POINT('Ctrl Pts',(-20.7827267210347,-24.2245787270438,
122.790564493814)) ;
#59903=CARTESIAN_POINT('Ctrl Pts',(-20.5080285227167,-24.0445896466809,
122.914803398227)) ;
#59904=CARTESIAN_POINT('Ctrl Pts',(-20.6560814228119,-24.2344345971071,
122.564616215145)) ;
#59905=CARTESIAN_POINT('Ctrl Pts',(-20.4067104191487,-24.0544455167443,
122.734046035466)) ;
#59906=CARTESIAN_POINT('Ctrl Pts',(-20.4901252098502,-24.2444321430243,
122.3609792939)) ;
#59907=CARTESIAN_POINT('Ctrl Pts',(-20.2739437686294,-24.0644430626614,
122.571137967992)) ;
#59908=CARTESIAN_POINT('Ctrl Pts',(-20.293135035734,-24.2543402699236,122.190698398529)) ;
#59909=CARTESIAN_POINT('Ctrl Pts',(-20.1163503191905,-24.0743511895607,
122.434915056073)) ;
#59910=CARTESIAN_POINT('Ctrl Pts',(-20.0674961654377,-24.2643506414457,
122.055437128195)) ;
#59911=CARTESIAN_POINT('Ctrl Pts',(-19.9358381408742,-24.0843615610829,
122.326707954225)) ;
#59912=CARTESIAN_POINT('Ctrl Pts',(-19.8211172047256,-24.2743810841931,
121.961778537735)) ;
#59913=CARTESIAN_POINT('Ctrl Pts',(-19.7387341883922,-24.0943920038303,
122.251783172163)) ;
#59914=CARTESIAN_POINT('Ctrl Pts',(-19.5670147878812,-24.2842290367464,
121.912623318456)) ;
#59915=CARTESIAN_POINT('Ctrl Pts',(-19.5354521536671,-24.1042399563836,
122.212461213181)) ;
#59916=CARTESIAN_POINT('Ctrl Pts',(-19.3026436245788,-24.2942917057674,
121.908036631008)) ;
#59917=CARTESIAN_POINT('Ctrl Pts',(-19.3239551506336,-24.1143026254045,
122.208794046212)) ;
#59918=CARTESIAN_POINT('Ctrl Pts',(-19.0458393133714,-24.3041860812313,
121.948921771872)) ;
#59919=CARTESIAN_POINT('Ctrl Pts',(-19.1185123080235,-24.1241970008685,
122.24150428493)) ;
#59920=CARTESIAN_POINT('Ctrl Pts',(-18.7986820358757,-24.3141278795495,
122.033501629842)) ;
#59921=CARTESIAN_POINT('Ctrl Pts',(-18.9207873807656,-24.1341387991866,
122.309170130401)) ;
#59922=CARTESIAN_POINT('Ctrl Pts',(-18.5684608876012,-24.3241303732768,
122.160425707919)) ;
#59923=CARTESIAN_POINT('Ctrl Pts',(-18.7366115490919,-24.1441412929139,
122.410711225786)) ;
#59924=CARTESIAN_POINT('Ctrl Pts',(-18.3634159135229,-24.3341651717837,
122.326219304177)) ;
#59925=CARTESIAN_POINT('Ctrl Pts',(-18.572576923515,-24.1541760914208,122.543347798557)) ;
#59926=CARTESIAN_POINT('Ctrl Pts',(-18.1931997744196,-24.3440100557631,
122.521073096174)) ;
#59927=CARTESIAN_POINT('Ctrl Pts',(-18.4364059140593,-24.1640209754002,
122.699231890635)) ;
#59928=CARTESIAN_POINT('Ctrl Pts',(-18.0570939034257,-24.3539959125811,
122.745386068162)) ;
#59929=CARTESIAN_POINT('Ctrl Pts',(-18.3275230654761,-24.1740068322182,
122.878683238655)) ;
#59930=CARTESIAN_POINT('Ctrl Pts',(-17.9622837121039,-24.3639307267559,
122.988691099202)) ;
#59931=CARTESIAN_POINT('Ctrl Pts',(-18.2516769244132,-24.183941646393,123.07332776623)) ;
#59932=CARTESIAN_POINT('Ctrl Pts',(-17.9107758866694,-24.3739882265412,
123.247885388004)) ;
#59933=CARTESIAN_POINT('Ctrl Pts',(-18.2104726941361,-24.1939991461783,
123.28068369653)) ;
#59934=CARTESIAN_POINT('Ctrl Pts',(-17.904793545213,-24.3838099849595,123.505950068629)) ;
#59935=CARTESIAN_POINT('Ctrl Pts',(-18.2056888745737,-24.2038209045966,
123.487134859051)) ;
#59936=CARTESIAN_POINT('Ctrl Pts',(-17.9441385895894,-24.3938656427435,
123.767234420915)) ;
#59937=CARTESIAN_POINT('Ctrl Pts',(-18.2371668835213,-24.2138765623806,
123.696162133941)) ;
#59938=CARTESIAN_POINT('Ctrl Pts',(-18.0277646258523,-24.4038078249235,
124.014774122479)) ;
#59939=CARTESIAN_POINT('Ctrl Pts',(-18.3040695599417,-24.2238187445607,
123.894192987516)) ;
#59940=CARTESIAN_POINT('Ctrl Pts',(-18.1519307759585,-24.4137130336182,
124.243545142332)) ;
#59941=CARTESIAN_POINT('Ctrl Pts',(-18.4034039803286,-24.2337239532553,
124.077208506641)) ;
#59942=CARTESIAN_POINT('Ctrl Pts',(-18.3162322484998,-24.4237548245807,
124.450038000876)) ;
#59943=CARTESIAN_POINT('Ctrl Pts',(-18.5348467279855,-24.2437657442178,
124.242401635478)) ;
#59944=CARTESIAN_POINT('Ctrl Pts',(-18.5112465951366,-24.4336625990529,
124.622564118162)) ;
#59945=CARTESIAN_POINT('Ctrl Pts',(-18.6908591806819,-24.25367351869,124.380420796196)) ;
#59946=CARTESIAN_POINT('Ctrl Pts',(-18.7353216882572,-24.4436740992805,
124.760445262885)) ;
#59947=CARTESIAN_POINT('Ctrl Pts',(-18.8701201999352,-24.2636850189176,
124.490724088854)) ;
#59948=CARTESIAN_POINT('Ctrl Pts',(-18.9806475911732,-24.4537068596732,
124.857016709312)) ;
#59949=CARTESIAN_POINT('Ctrl Pts',(-19.0663816751917,-24.2737177793103,
124.567979438308)) ;
#59950=CARTESIAN_POINT('Ctrl Pts',(-19.2342398512447,-24.4635574288081,
124.909018469813)) ;
#59951=CARTESIAN_POINT('Ctrl Pts',(-19.2692552091276,-24.2835683484452,
124.609578862469)) ;
#59952=CARTESIAN_POINT('Ctrl Pts',(-19.496593073052,-24.473546038338,124.916794312844)) ;
#59953=CARTESIAN_POINT('Ctrl Pts',(-19.4791376938432,-24.2935569579751,
124.615797717518)) ;
#59954=CARTESIAN_POINT('Ctrl Pts',(-19.7547810174037,-24.4834746943621,
124.879120015881)) ;
#59955=CARTESIAN_POINT('Ctrl Pts',(-19.685687402309,-24.3034856139992,124.585656541612)) ;
#59956=CARTESIAN_POINT('Ctrl Pts',(-20.0041249025158,-24.4934624405399,
124.797121058112)) ;
#59957=CARTESIAN_POINT('Ctrl Pts',(-19.8851618270809,-24.313473360177,124.520055766498)) ;
#59958=CARTESIAN_POINT('Ctrl Pts',(-20.2363287243684,-24.5034984294756,
124.672094532501)) ;
#59959=CARTESIAN_POINT('Ctrl Pts',(-20.0709240851037,-24.3235093491128,
124.42003291363)) ;
#59960=CARTESIAN_POINT('Ctrl Pts',(-20.4398532893897,-24.5133532992892,
124.511915768883)) ;
#59961=CARTESIAN_POINT('Ctrl Pts',(-20.23374208075,-24.3333642189264,124.291888988596)) ;
#59962=CARTESIAN_POINT('Ctrl Pts',(-20.6152286146219,-24.523352740531,124.316286380148)) ;
#59963=CARTESIAN_POINT('Ctrl Pts',(-20.3740410150847,-24.3433636601681,
124.135384433191)) ;
#59964=CARTESIAN_POINT('Ctrl Pts',(-20.7528077611867,-24.5332478147111,
124.095579716367)) ;
#59965=CARTESIAN_POINT('Ctrl Pts',(-20.4841026378956,-24.3532587343482,
123.958818739032)) ;
#59966=CARTESIAN_POINT('Ctrl Pts',(-20.8515452176625,-24.5433084705508,
123.850362627596)) ;
#59967=CARTESIAN_POINT('Ctrl Pts',(-20.5630911554068,-24.3633193901879,
123.762644277068)) ;
#59968=CARTESIAN_POINT('Ctrl Pts',(-20.90521146566,-24.5531573447464,123.597149046186)) ;
#59969=CARTESIAN_POINT('Ctrl Pts',(-20.6060224056543,-24.3731682643835,
123.560073894341)) ;
#59970=CARTESIAN_POINT('Ctrl Pts',(-20.9149218984342,-24.5631860567097,
123.333787858284)) ;
#59971=CARTESIAN_POINT('Ctrl Pts',(-20.6137892700435,-24.3831969763468,
123.349384859398)) ;
#59972=CARTESIAN_POINT('Ctrl Pts',(-20.8780431867244,-24.5732154572928,
123.072813707619)) ;
#59973=CARTESIAN_POINT('Ctrl Pts',(-20.5842846871539,-24.3932263769299,
123.140605706527)) ;
#59974=CARTESIAN_POINT('Ctrl Pts',(-20.7984988600526,-24.5830556509096,
122.826757371458)) ;
#59975=CARTESIAN_POINT('Ctrl Pts',(-20.5206480690799,-24.4030665705467,
122.943761971265)) ;
#59976=CARTESIAN_POINT('Ctrl Pts',(-20.675875973219,-24.5930590734848,122.594259198633)) ;
#59977=CARTESIAN_POINT('Ctrl Pts',(-20.4225485501973,-24.4130699931219,
122.757764169377)) ;
#59978=CARTESIAN_POINT('Ctrl Pts',(-20.5149236678703,-24.6030446105779,
122.386952011327)) ;
#59979=CARTESIAN_POINT('Ctrl Pts',(-20.2937856775477,-24.423055530215,122.591919429252)) ;
#59980=CARTESIAN_POINT('Ctrl Pts',(-20.319214882974,-24.6130856150647,122.210004150072)) ;
#59981=CARTESIAN_POINT('Ctrl Pts',(-20.1372175724213,-24.4330965347018,
122.450362171703)) ;
#59982=CARTESIAN_POINT('Ctrl Pts',(-20.100298824301,-24.6229291540059,122.072161974285)) ;
#59983=CARTESIAN_POINT('Ctrl Pts',(-19.9620847673465,-24.442940073643,122.340090125974)) ;
#59984=CARTESIAN_POINT('Ctrl Pts',(-19.8575938757749,-24.6329141849967,
121.972533729906)) ;
#59985=CARTESIAN_POINT('Ctrl Pts',(-19.7679204996431,-24.4529251046338,
122.260388809874)) ;
#59986=CARTESIAN_POINT('Ctrl Pts',(-19.6023947114749,-24.6428536475187,
121.916697509575)) ;
#59987=CARTESIAN_POINT('Ctrl Pts',(-19.5637613212233,-24.4628645671558,
122.215721172914)) ;
#59988=CARTESIAN_POINT('Ctrl Pts',(-19.3388001962216,-24.6528933797425,
121.905974359338)) ;
#59989=CARTESIAN_POINT('Ctrl Pts',(-19.3528855389491,-24.4729042993796,
122.207143937649)) ;
#59990=CARTESIAN_POINT('Ctrl Pts',(-19.0812413725031,-24.6627815600597,
121.940528367606)) ;
#59991=CARTESIAN_POINT('Ctrl Pts',(-19.1468393800042,-24.4827924796968,
122.23478829755)) ;
#59992=CARTESIAN_POINT('Ctrl Pts',(-18.830930339593,-24.6727710757622,122.019607849904)) ;
#59993=CARTESIAN_POINT('Ctrl Pts',(-18.9465910651468,-24.4927819953993,
122.298052933552)) ;
#59994=CARTESIAN_POINT('Ctrl Pts',(-18.5989667873706,-24.6827296264169,
122.140752466296)) ;
#59995=CARTESIAN_POINT('Ctrl Pts',(-18.7610210868457,-24.502740546054,122.394969531165)) ;
#59996=CARTESIAN_POINT('Ctrl Pts',(-18.3923783177254,-24.6926290335219,
122.298887165231)) ;
#59997=CARTESIAN_POINT('Ctrl Pts',(-18.5957515114888,-24.5126399531591,
122.521477699572)) ;
#59998=CARTESIAN_POINT('Ctrl Pts',(-18.2138481637525,-24.7026776199382,
122.493414575767)) ;
#59999=CARTESIAN_POINT('Ctrl Pts',(-18.4529280643294,-24.5226885395753,
122.677100488762)) ;
#60000=CARTESIAN_POINT('Ctrl Pts',(-18.0737497675781,-24.7125704389027,
122.712471449112)) ;
#60001=CARTESIAN_POINT('Ctrl Pts',(-18.3408506079003,-24.5325813585398,
122.852345913931)) ;
#60002=CARTESIAN_POINT('Ctrl Pts',(-17.9721440404555,-24.7226415564325,
122.95679058556)) ;
#60003=CARTESIAN_POINT('Ctrl Pts',(-18.2595668744231,-24.5426524760696,
123.047801904658)) ;
#60004=CARTESIAN_POINT('Ctrl Pts',(-17.9156039987701,-24.7324572503985,
123.208514840523)) ;
#60005=CARTESIAN_POINT('Ctrl Pts',(-18.214336048054,-24.5524681700357,123.249180320883)) ;
#60006=CARTESIAN_POINT('Ctrl Pts',(-17.9029486725744,-24.7425236278958,
123.472689210429)) ;
#60007=CARTESIAN_POINT('Ctrl Pts',(-18.2042126493569,-24.562534547533,123.460520152789)) ;
#60008=CARTESIAN_POINT('Ctrl Pts',(-17.935892095498,-24.7524226139777,123.730795685717)) ;
#60009=CARTESIAN_POINT('Ctrl Pts',(-18.2305681821553,-24.5724335336148,
123.667004510187)) ;
#60010=CARTESIAN_POINT('Ctrl Pts',(-18.0142279454651,-24.7624767939712,
123.983068491379)) ;
#60011=CARTESIAN_POINT('Ctrl Pts',(-18.2932377609771,-24.5824877136083,
123.868822703197)) ;
#60012=CARTESIAN_POINT('Ctrl Pts',(-18.1327982653444,-24.7723476069039,
124.213846997016)) ;
#60013=CARTESIAN_POINT('Ctrl Pts',(-18.3880943171351,-24.592358526541,124.053444317472)) ;
#60014=CARTESIAN_POINT('Ctrl Pts',(-18.2927953165878,-24.7824215077577,
124.424680232047)) ;
#60015=CARTESIAN_POINT('Ctrl Pts',(-18.5160928152564,-24.6024324273948,
124.222110690457)) ;
#60016=CARTESIAN_POINT('Ctrl Pts',(-18.4819523062821,-24.7922416631444,
124.600316090913)) ;
#60017=CARTESIAN_POINT('Ctrl Pts',(-18.6674179941489,-24.6122525827815,
124.36261799151)) ;
#60018=CARTESIAN_POINT('Ctrl Pts',(-18.7041959809352,-24.8023203700966,
124.744270009316)) ;
#60019=CARTESIAN_POINT('Ctrl Pts',(-18.8452136184264,-24.6223312897337,
124.477780764093)) ;
#60020=CARTESIAN_POINT('Ctrl Pts',(-18.9426453970189,-24.8121719586354,
124.845254460228)) ;
#60021=CARTESIAN_POINT('Ctrl Pts',(-19.0359724337194,-24.6321828782725,
124.558567311492)) ;
#60022=CARTESIAN_POINT('Ctrl Pts',(-19.200521069137,-24.8222450751604,124.904809172551)) ;
#60023=CARTESIAN_POINT('Ctrl Pts',(-19.2422734477073,-24.6422559947975,
124.606210577257)) ;
#60024=CARTESIAN_POINT('Ctrl Pts',(-19.4588424041164,-24.8320875922562,
124.91832832477)) ;
#60025=CARTESIAN_POINT('Ctrl Pts',(-19.4489294152064,-24.6520985118933,
124.617025231616)) ;
#60026=CARTESIAN_POINT('Ctrl Pts',(-19.7192553917927,-24.8420680538102,
124.887225976131)) ;
#60027=CARTESIAN_POINT('Ctrl Pts',(-19.6572595128658,-24.6620789734473,
124.592142995155)) ;
#60028=CARTESIAN_POINT('Ctrl Pts',(-19.9711242826029,-24.8520863038009,
124.810604842072)) ;
#60029=CARTESIAN_POINT('Ctrl Pts',(-19.8587544824804,-24.6720972234381,
124.530845590783)) ;
#60030=CARTESIAN_POINT('Ctrl Pts',(-20.2029896410635,-24.8619704639947,
124.693474375189)) ;
#60031=CARTESIAN_POINT('Ctrl Pts',(-20.0442458164623,-24.6819813836318,
124.437141271385)) ;
#60032=CARTESIAN_POINT('Ctrl Pts',(-20.4147243951242,-24.8720356109697,
124.535001991824)) ;
#60033=CARTESIAN_POINT('Ctrl Pts',(-20.2136336325646,-24.6920465306068,
124.310362857701)) ;
#60034=CARTESIAN_POINT('Ctrl Pts',(-20.5918496186671,-24.8818774346105,
124.346514930548)) ;
#60035=CARTESIAN_POINT('Ctrl Pts',(-20.3553327465534,-24.7018883542476,
124.159573817455)) ;
#60036=CARTESIAN_POINT('Ctrl Pts',(-20.7368372685072,-24.8919069070713,
124.126420308641)) ;
#60037=CARTESIAN_POINT('Ctrl Pts',(-20.4713227600886,-24.7119178267085,
123.983497953276)) ;
#60038=CARTESIAN_POINT('Ctrl Pts',(-20.8407071584653,-24.9019337623334,
123.884255455993)) ;
#60039=CARTESIAN_POINT('Ctrl Pts',(-20.5544183607699,-24.7219446819705,
123.789765854984)) ;
#60040=CARTESIAN_POINT('Ctrl Pts',(-20.9004509562917,-24.9117770124439,
123.632574419147)) ;
#60041=CARTESIAN_POINT('Ctrl Pts',(-20.6022129291242,-24.731787932081,123.588422099066)) ;
#60042=CARTESIAN_POINT('Ctrl Pts',(-20.916260611242,-24.9218254520271,123.368993380643)) ;
#60043=CARTESIAN_POINT('Ctrl Pts',(-20.614860543706,-24.7418363716642,123.377557052921)) ;
#60044=CARTESIAN_POINT('Ctrl Pts',(-20.8859488523691,-24.931774946275,123.109292637768)) ;
#60045=CARTESIAN_POINT('Ctrl Pts',(-20.59061096289,-24.7517858659121,123.169796946132)) ;
#60046=CARTESIAN_POINT('Ctrl Pts',(-20.812063374515,-24.941682802001,122.85961242254)) ;
#60047=CARTESIAN_POINT('Ctrl Pts',(-20.531502761985,-24.7616937216381,122.970053477872)) ;
#60048=CARTESIAN_POINT('Ctrl Pts',(-20.6939388264685,-24.9517422786509,
122.623150935641)) ;
#60049=CARTESIAN_POINT('Ctrl Pts',(-20.4370029110324,-24.771753198288,122.7808840852)) ;
#60050=CARTESIAN_POINT('Ctrl Pts',(-20.5402177796958,-24.9615830880596,
122.415150839327)) ;
#60051=CARTESIAN_POINT('Ctrl Pts',(-20.3140267650596,-24.7815940076967,
122.614484958291)) ;
#60052=CARTESIAN_POINT('Ctrl Pts',(-20.3487716521003,-24.9716452383604,
122.232796879525)) ;
#60053=CARTESIAN_POINT('Ctrl Pts',(-20.1608697005257,-24.7916561579975,
122.46860153275)) ;
#60054=CARTESIAN_POINT('Ctrl Pts',(-20.1319979378848,-24.981542399483,122.089055106717)) ;
#60055=CARTESIAN_POINT('Ctrl Pts',(-19.9874513995793,-24.8015533191201,
122.353608554069)) ;
#60056=CARTESIAN_POINT('Ctrl Pts',(-19.8931048762682,-24.991473573887,121.983991783669)) ;
#60057=CARTESIAN_POINT('Ctrl Pts',(-19.7963375692776,-24.8114844935241,
122.269557920393)) ;
#60058=CARTESIAN_POINT('Ctrl Pts',(-19.6366938542377,-25.001515777612,121.921591372385)) ;
#60059=CARTESIAN_POINT('Ctrl Pts',(-19.5912086257086,-24.8215266972492,
122.219637404033)) ;
#60060=CARTESIAN_POINT('Ctrl Pts',(-19.3774193320319,-25.0114023600425,
121.904731667752)) ;
#60061=CARTESIAN_POINT('Ctrl Pts',(-19.3837898885551,-24.8314132796796,
122.206149496955)) ;
#60062=CARTESIAN_POINT('Ctrl Pts',(-19.116345118076,-25.0213957957908,121.933019786069)) ;
#60063=CARTESIAN_POINT('Ctrl Pts',(-19.1749306450464,-24.8414067154279,
122.228779665525)) ;
#60064=CARTESIAN_POINT('Ctrl Pts',(-18.8653899853733,-25.031340264149,122.0059331557)) ;
#60065=CARTESIAN_POINT('Ctrl Pts',(-18.9741669200582,-24.8513511837861,
122.287109951159)) ;
#60066=CARTESIAN_POINT('Ctrl Pts',(-18.6305081904514,-25.0412920803945,
122.120959221121)) ;
#60067=CARTESIAN_POINT('Ctrl Pts',(-18.7862616983895,-24.8613030000317,
122.379130236719)) ;
#60068=CARTESIAN_POINT('Ctrl Pts',(-18.4175106984375,-25.051329516509,122.276526693865)) ;
#60069=CARTESIAN_POINT('Ctrl Pts',(-18.6158633904333,-24.8713404361461,
122.503584006888)) ;
#60070=CARTESIAN_POINT('Ctrl Pts',(-18.2373294887089,-25.0612144756854,
122.463677159572)) ;
#60071=CARTESIAN_POINT('Ctrl Pts',(-18.4717187211798,-24.8812253953225,
122.653303473347)) ;
#60072=CARTESIAN_POINT('Ctrl Pts',(-18.0904935273236,-25.0712125938973,
122.681519130343)) ;
#60073=CARTESIAN_POINT('Ctrl Pts',(-18.3542496121446,-24.8912235135344,
122.82757667031)) ;
#60074=CARTESIAN_POINT('Ctrl Pts',(-17.9843474113932,-25.0811335264093,
122.919675638714)) ;
#60075=CARTESIAN_POINT('Ctrl Pts',(-18.2693324840715,-24.9011444460464,
123.018101090549)) ;
#60076=CARTESIAN_POINT('Ctrl Pts',(-17.9203421285094,-25.0911748266313,
123.175657289294)) ;
#60077=CARTESIAN_POINT('Ctrl Pts',(-18.2181276878849,-24.9111857462685,
123.222886415152)) ;
#60078=CARTESIAN_POINT('Ctrl Pts',(-17.9020926498255,-25.1010817450213,
123.435363279085)) ;
#60079=CARTESIAN_POINT('Ctrl Pts',(-18.2035276252548,-24.9210926646584,
123.430650454951)) ;
#60080=CARTESIAN_POINT('Ctrl Pts',(-17.9285484881312,-25.1110175367304,
123.69512331008)) ;
#60081=CARTESIAN_POINT('Ctrl Pts',(-18.2246915312731,-24.9310284563675,
123.638458030304)) ;
#60082=CARTESIAN_POINT('Ctrl Pts',(-18.0007127842541,-25.1210584313083,
123.948921149935)) ;
#60083=CARTESIAN_POINT('Ctrl Pts',(-18.2824223843685,-24.9410693509454,
123.841496622937)) ;
#60084=CARTESIAN_POINT('Ctrl Pts',(-18.1139247515408,-25.1309456330221,
124.18280063066)) ;
#60085=CARTESIAN_POINT('Ctrl Pts',(-18.3729909704001,-24.9509565526592,
124.028599762318)) ;
#60086=CARTESIAN_POINT('Ctrl Pts',(-18.2672700656794,-25.1409379007837,
124.395937506852)) ;
#60087=CARTESIAN_POINT('Ctrl Pts',(-18.4956664766225,-24.9609488204208,
124.199109598826)) ;
#60088=CARTESIAN_POINT('Ctrl Pts',(-18.4545445264848,-25.1508864218055,
124.578379945049)) ;
#60089=CARTESIAN_POINT('Ctrl Pts',(-18.6454851891911,-24.9708973414426,
124.345063807)) ;
#60090=CARTESIAN_POINT('Ctrl Pts',(-18.6701593794825,-25.1608231953832,
124.72564450551)) ;
#60091=CARTESIAN_POINT('Ctrl Pts',(-18.8179761594363,-24.9808341150203,
124.462875886773)) ;
#60092=CARTESIAN_POINT('Ctrl Pts',(-18.9090898746252,-25.1708062435242,
124.834059046402)) ;
#60093=CARTESIAN_POINT('Ctrl Pts',(-19.0091199773882,-24.9908171631614,
124.549608297516)) ;
#60094=CARTESIAN_POINT('Ctrl Pts',(-19.1648198261409,-25.1808499511343,
124.899256681723)) ;
#60095=CARTESIAN_POINT('Ctrl Pts',(-19.2137038781447,-25.0008608707714,
124.601767252083)) ;
#60096=CARTESIAN_POINT('Ctrl Pts',(-19.4223677819913,-25.1906786442876,
124.919232914373)) ;
#60097=CARTESIAN_POINT('Ctrl Pts',(-19.4197410212802,-25.0106895639247,
124.617749120168)) ;
#60098=CARTESIAN_POINT('Ctrl Pts',(-19.6858526790546,-25.200753393417,124.893750955826)) ;
#60099=CARTESIAN_POINT('Ctrl Pts',(-19.6305293633067,-25.0207643130542,
124.59736453674)) ;
#60100=CARTESIAN_POINT('Ctrl Pts',(-19.9356579462158,-25.2106187192126,
124.824304856564)) ;
#60101=CARTESIAN_POINT('Ctrl Pts',(-19.8303729649698,-25.0306296388497,
124.541808869368)) ;
#60102=CARTESIAN_POINT('Ctrl Pts',(-20.173585469303,-25.2206408935695,124.711387601586)) ;
#60103=CARTESIAN_POINT('Ctrl Pts',(-20.0207155100975,-25.0406518132067,
124.451476093775)) ;
#60104=CARTESIAN_POINT('Ctrl Pts',(-20.3880226560733,-25.2306669467765,
124.558270853384)) ;
#60105=CARTESIAN_POINT('Ctrl Pts',(-20.1922658914238,-25.0506778664136,
124.328983483751)) ;
#60106=CARTESIAN_POINT('Ctrl Pts',(-20.5697163878782,-25.2405206436227,
124.373799671678)) ;
#60107=CARTESIAN_POINT('Ctrl Pts',(-20.3376209782561,-25.0605315632599,
124.181408007588)) ;
#60108=CARTESIAN_POINT('Ctrl Pts',(-20.7188606913848,-25.2504800483757,
124.15871963452)) ;
#60109=CARTESIAN_POINT('Ctrl Pts',(-20.4569372775264,-25.0704909680128,
124.009344986073)) ;
#60110=CARTESIAN_POINT('Ctrl Pts',(-20.8288249195141,-25.2605182940806,
123.91895416316)) ;
#60111=CARTESIAN_POINT('Ctrl Pts',(-20.5449097751489,-25.0805292137177,
123.817532999354)) ;
#60112=CARTESIAN_POINT('Ctrl Pts',(-20.8948612313139,-25.2703924782426,
123.667978712676)) ;
#60113=CARTESIAN_POINT('Ctrl Pts',(-20.5977398529196,-25.0904033978798,
123.616753747338)) ;
#60114=CARTESIAN_POINT('Ctrl Pts',(-20.9167246661195,-25.2804622613806,
123.404296836379)) ;
#60115=CARTESIAN_POINT('Ctrl Pts',(-20.6152318948764,-25.1004731810177,
123.405808073507)) ;
#60116=CARTESIAN_POINT('Ctrl Pts',(-20.8931748950452,-25.2902955164013,
123.146942101532)) ;
#60117=CARTESIAN_POINT('Ctrl Pts',(-20.5963934691841,-25.1103064360384,
123.199925185877)) ;
#60118=CARTESIAN_POINT('Ctrl Pts',(-20.824664603496,-25.300325942533,122.892421113422)) ;
#60119=CARTESIAN_POINT('Ctrl Pts',(-20.5415866267975,-25.1203368621701,
122.996307948949)) ;
#60120=CARTESIAN_POINT('Ctrl Pts',(-20.7122848539056,-25.31035755472,122.653938383803)) ;
#60121=CARTESIAN_POINT('Ctrl Pts',(-20.4516839742709,-25.1303684743571,
122.805521151809)) ;
#60122=CARTESIAN_POINT('Ctrl Pts',(-20.5637225648046,-25.3201872515746,
122.442640422475)) ;
#60123=CARTESIAN_POINT('Ctrl Pts',(-20.3328358819854,-25.1401981712117,
122.636482800151)) ;
#60124=CARTESIAN_POINT('Ctrl Pts',(-20.3782914259255,-25.3301766934771,
122.2568129731)) ;
#60125=CARTESIAN_POINT('Ctrl Pts',(-20.1844921808869,-25.1501876131142,
122.487819833207)) ;
#60126=CARTESIAN_POINT('Ctrl Pts',(-20.1618642262399,-25.3402205854928,
122.105737145019)) ;
#60127=CARTESIAN_POINT('Ctrl Pts',(-20.0113511467643,-25.1602315051299,
122.366957925949)) ;
#60128=CARTESIAN_POINT('Ctrl Pts',(-19.9280150892264,-25.350042147262,121.996514020556)) ;
#60129=CARTESIAN_POINT('Ctrl Pts',(-19.8242733908789,-25.1700530668991,
122.279578452109)) ;
#60130=CARTESIAN_POINT('Ctrl Pts',(-19.6734892886853,-25.3600777188862,
121.927457195706)) ;
#60131=CARTESIAN_POINT('Ctrl Pts',(-19.6206531100156,-25.1800886385233,
122.224331363423)) ;
#60132=CARTESIAN_POINT('Ctrl Pts',(-19.4109364974854,-25.370106993168,121.904446478748)) ;
#60133=CARTESIAN_POINT('Ctrl Pts',(-19.410610970347,-25.1901179128051,122.205921274802)) ;
#60134=CARTESIAN_POINT('Ctrl Pts',(-19.153425698316,-25.3799408302867,121.92623667871)) ;
#60135=CARTESIAN_POINT('Ctrl Pts',(-19.2046030736676,-25.1999517499238,
122.223351721254)) ;
#60136=CARTESIAN_POINT('Ctrl Pts',(-18.8979973838901,-25.3899932263748,
121.99356443242)) ;
#60137=CARTESIAN_POINT('Ctrl Pts',(-19.0002598327071,-25.2100041460119,
122.277212317537)) ;
#60138=CARTESIAN_POINT('Ctrl Pts',(-18.6610161340933,-25.3999299933253,
122.103265136597)) ;
#60139=CARTESIAN_POINT('Ctrl Pts',(-18.8106744978957,-25.2199409129625,
122.364971228474)) ;
#60140=CARTESIAN_POINT('Ctrl Pts',(-18.4463642084405,-25.4098642283046,
122.251846102408)) ;
#60141=CARTESIAN_POINT('Ctrl Pts',(-18.6389522789307,-25.2298751479417,
122.483834331329)) ;
#60142=CARTESIAN_POINT('Ctrl Pts',(-18.2592125481551,-25.4198879916314,
122.437210228712)) ;
#60143=CARTESIAN_POINT('Ctrl Pts',(-18.4892297234926,-25.2398989112685,
122.632124410148)) ;
#60144=CARTESIAN_POINT('Ctrl Pts',(-18.1090179641426,-25.429774333016,122.649196677396)) ;
#60145=CARTESIAN_POINT('Ctrl Pts',(-18.3690729553001,-25.2497852526532,
122.801712072819)) ;
#60146=CARTESIAN_POINT('Ctrl Pts',(-17.9962023976865,-25.439763381783,122.886228834323)) ;
#60147=CARTESIAN_POINT('Ctrl Pts',(-18.2788188754758,-25.2597743014202,
122.991336884264)) ;
#60148=CARTESIAN_POINT('Ctrl Pts',(-17.92642324804,-25.4498046024804,123.140706746069)) ;
#60149=CARTESIAN_POINT('Ctrl Pts',(-18.2229938254166,-25.2698155221175,
123.194918814878)) ;
#60150=CARTESIAN_POINT('Ctrl Pts',(-17.9019779830715,-25.4596372426583,
123.397935296118)) ;
#60151=CARTESIAN_POINT('Ctrl Pts',(-18.2034358520446,-25.2796481622954,
123.400700720434)) ;
#60152=CARTESIAN_POINT('Ctrl Pts',(-17.9221548130397,-25.4696311719663,
123.659787613403)) ;
#60153=CARTESIAN_POINT('Ctrl Pts',(-18.2195753605606,-25.2896420916034,
123.610182627543)) ;
#60154=CARTESIAN_POINT('Ctrl Pts',(-17.9882634627547,-25.4796603796468,
123.914920831953)) ;
#60155=CARTESIAN_POINT('Ctrl Pts',(-18.2724604733462,-25.2996712992839,
123.814289688043)) ;
#60156=CARTESIAN_POINT('Ctrl Pts',(-18.095614902813,-25.4895361913509,124.151219574805)) ;
#60157=CARTESIAN_POINT('Ctrl Pts',(-18.3583396441264,-25.309547110988,124.003328991269)) ;
#60158=CARTESIAN_POINT('Ctrl Pts',(-18.243932354423,-25.4995354183223,124.368086107195)) ;
#60159=CARTESIAN_POINT('Ctrl Pts',(-18.4769919264261,-25.3195463379594,
124.176823257669)) ;
#60160=CARTESIAN_POINT('Ctrl Pts',(-18.4258762775159,-25.509444899478,124.554446462771)) ;
#60161=CARTESIAN_POINT('Ctrl Pts',(-18.6225453691918,-25.3294558191151,
124.325912669467)) ;
#60162=CARTESIAN_POINT('Ctrl Pts',(-18.6404489287507,-25.5194981297789,
124.708521879958)) ;
#60163=CARTESIAN_POINT('Ctrl Pts',(-18.7942023889779,-25.339509049416,124.449174675351)) ;
#60164=CARTESIAN_POINT('Ctrl Pts',(-18.8741769469546,-25.52936874633,124.821053391255)) ;
#60165=CARTESIAN_POINT('Ctrl Pts',(-18.981183490012,-25.3493796659671,124.539201487123)) ;
#60166=CARTESIAN_POINT('Ctrl Pts',(-19.127535526737,-25.539390408062,124.892923586668)) ;
#60167=CARTESIAN_POINT('Ctrl Pts',(-19.1838697832088,-25.3594013276991,
124.596699645032)) ;
#60168=CARTESIAN_POINT('Ctrl Pts',(-19.3896325300281,-25.5494132212431,
124.919115026202)) ;
#60169=CARTESIAN_POINT('Ctrl Pts',(-19.3935471728134,-25.3694241408802,
124.617654797419)) ;
#60170=CARTESIAN_POINT('Ctrl Pts',(-19.6482244565105,-25.5592803857031,
124.900141299359)) ;
#60171=CARTESIAN_POINT('Ctrl Pts',(-19.6004204014471,-25.3792913053402,
124.602477906034)) ;
#60172=CARTESIAN_POINT('Ctrl Pts',(-19.902976585568,-25.569273827923,124.83632140457)) ;
#60173=CARTESIAN_POINT('Ctrl Pts',(-19.8042225357259,-25.3892847475601,
124.551424072953)) ;
#60174=CARTESIAN_POINT('Ctrl Pts',(-20.1434775002714,-25.5793055015233,
124.728362358273)) ;
#60175=CARTESIAN_POINT('Ctrl Pts',(-19.9966241166619,-25.3993164211604,
124.465058726285)) ;
#60176=CARTESIAN_POINT('Ctrl Pts',(-20.3582214202011,-25.5891719366363,
124.583046155646)) ;
#60177=CARTESIAN_POINT('Ctrl Pts',(-20.1684200947875,-25.4091828562734,
124.348807744366)) ;
#60178=CARTESIAN_POINT('Ctrl Pts',(-20.5470220993217,-25.5991593871694,
124.400775187836)) ;
#60179=CARTESIAN_POINT('Ctrl Pts',(-20.3194620631275,-25.4191703068065,
124.202992587349)) ;
#60180=CARTESIAN_POINT('Ctrl Pts',(-20.7008042109663,-25.6091043169973,
124.189419968421)) ;
#60181=CARTESIAN_POINT('Ctrl Pts',(-20.4424893892085,-25.4291152366345,
124.033909833955)) ;
#60182=CARTESIAN_POINT('Ctrl Pts',(-20.8165443609091,-25.6191492120525,
123.952204828847)) ;
#60183=CARTESIAN_POINT('Ctrl Pts',(-20.535083449004,-25.4391601316896,123.844138651969)) ;
#60184=CARTESIAN_POINT('Ctrl Pts',(-20.8882445301737,-25.6290112737383,
123.70313575114)) ;
#60185=CARTESIAN_POINT('Ctrl Pts',(-20.5924455729224,-25.4490221933754,
123.644884316791)) ;
#60186=CARTESIAN_POINT('Ctrl Pts',(-20.9164870894924,-25.6390029965252,
123.442107956851)) ;
#60187=CARTESIAN_POINT('Ctrl Pts',(-20.6150418055074,-25.4590139161623,
123.436062394398)) ;
#60188=CARTESIAN_POINT('Ctrl Pts',(-20.8989852870473,-25.6489352107651,
123.181683998695)) ;
#60189=CARTESIAN_POINT('Ctrl Pts',(-20.6010425682798,-25.4689461304023,
123.227723257091)) ;
#60190=CARTESIAN_POINT('Ctrl Pts',(-20.8370703423436,-25.6588745293309,
122.927926047669)) ;
#60191=CARTESIAN_POINT('Ctrl Pts',(-20.5515128122733,-25.478885448968,123.024716500619)) ;
#60192=CARTESIAN_POINT('Ctrl Pts',(-20.7307098426691,-25.6689187041067,
122.686357803622)) ;
#60193=CARTESIAN_POINT('Ctrl Pts',(-20.4664264490109,-25.4889296237439,
122.831461026835)) ;
#60194=CARTESIAN_POINT('Ctrl Pts',(-20.5866715410215,-25.6787892581717,
122.47063867262)) ;
#60195=CARTESIAN_POINT('Ctrl Pts',(-20.351197775471,-25.4988001778088,122.658884659411)) ;
#60196=CARTESIAN_POINT('Ctrl Pts',(-20.4061979028758,-25.6887542405259,
122.280888722177)) ;
#60197=CARTESIAN_POINT('Ctrl Pts',(-20.2068205491805,-25.508765160163,122.507083201106)) ;
#60198=CARTESIAN_POINT('Ctrl Pts',(-20.1938959519348,-25.6987849434157,
122.124661424676)) ;
#60199=CARTESIAN_POINT('Ctrl Pts',(-20.0369803529524,-25.5187958630528,
122.382099587623)) ;
#60200=CARTESIAN_POINT('Ctrl Pts',(-19.9610841220414,-25.7086772834409,
122.008927766554)) ;
#60201=CARTESIAN_POINT('Ctrl Pts',(-19.8507319966017,-25.528688203078,122.289510701505)) ;
#60202=CARTESIAN_POINT('Ctrl Pts',(-19.7077317559287,-25.7187305166009,
121.934171888619)) ;
#60203=CARTESIAN_POINT('Ctrl Pts',(-19.6480507770561,-25.538741436238,122.229703850899)) ;
#60204=CARTESIAN_POINT('Ctrl Pts',(-19.4496748815431,-25.7286117610776,
121.904882259363)) ;
#60205=CARTESIAN_POINT('Ctrl Pts',(-19.4416056279945,-25.5486226807147,
122.206269922949)) ;
#60206=CARTESIAN_POINT('Ctrl Pts',(-19.1865495494831,-25.7386448819486,
121.920889891667)) ;
#60207=CARTESIAN_POINT('Ctrl Pts',(-19.2311052788292,-25.5586558015858,
122.219073772921)) ;
#60208=CARTESIAN_POINT('Ctrl Pts',(-18.933934095788,-25.7485260922237,121.981208015015)) ;
#60209=CARTESIAN_POINT('Ctrl Pts',(-19.029012442334,-25.5685370118608,122.26732607008)) ;
#60210=CARTESIAN_POINT('Ctrl Pts',(-18.6913224502721,-25.758588167993,122.086259918764)) ;
#60211=CARTESIAN_POINT('Ctrl Pts',(-18.8349222926242,-25.5785990876302,
122.351365495269)) ;
#60212=CARTESIAN_POINT('Ctrl Pts',(-18.4750177696445,-25.7684452263748,
122.228841554689)) ;
#60213=CARTESIAN_POINT('Ctrl Pts',(-18.6618773148377,-25.5884561460119,
122.465428920654)) ;
#60214=CARTESIAN_POINT('Ctrl Pts',(-18.2838238477272,-25.7784397816638,
122.408857735709)) ;
#60215=CARTESIAN_POINT('Ctrl Pts',(-18.5089206655225,-25.5984507013009,
122.60944020259)) ;
#60216=CARTESIAN_POINT('Ctrl Pts',(-18.1277492566093,-25.7883656691993,
122.617897877619)) ;
#60217=CARTESIAN_POINT('Ctrl Pts',(-18.3840591928632,-25.6083765888364,
122.77667098702)) ;
#60218=CARTESIAN_POINT('Ctrl Pts',(-18.0091260993972,-25.7983906891946,
122.853105228335)) ;
#60219=CARTESIAN_POINT('Ctrl Pts',(-18.2891587030672,-25.6184016088317,
122.964835791046)) ;
#60220=CARTESIAN_POINT('Ctrl Pts',(-17.9340157762588,-25.8082880662982,
123.102124235181)) ;
#60221=CARTESIAN_POINT('Ctrl Pts',(-18.2290682857916,-25.6282989859354,
123.164050416227)) ;
#60222=CARTESIAN_POINT('Ctrl Pts',(-17.9024264992633,-25.8182783033791,
123.362756958186)) ;
#60223=CARTESIAN_POINT('Ctrl Pts',(-18.2037946795891,-25.6382892230162,
123.372556307197)) ;
#60224=CARTESIAN_POINT('Ctrl Pts',(-17.9171433202812,-25.8283149161879,
123.62609402293)) ;
#60225=CARTESIAN_POINT('Ctrl Pts',(-18.2155658929526,-25.648325835825,123.583225962692)) ;
#60226=CARTESIAN_POINT('Ctrl Pts',(-17.9758333009536,-25.8381647996059,
123.878206838358)) ;
#60227=CARTESIAN_POINT('Ctrl Pts',(-18.2625157992265,-25.658175719243,123.784916942111)) ;
#60228=CARTESIAN_POINT('Ctrl Pts',(-18.0784917995666,-25.8481684165084,
124.120189945079)) ;
#60229=CARTESIAN_POINT('Ctrl Pts',(-18.3446404819217,-25.6681793361455,
123.978504135792)) ;
#60230=CARTESIAN_POINT('Ctrl Pts',(-18.2215613397651,-25.8581578282735,
124.340338256903)) ;
#60231=CARTESIAN_POINT('Ctrl Pts',(-18.4590946437798,-25.6781687479106,
124.154624345632)) ;
#60232=CARTESIAN_POINT('Ctrl Pts',(-18.4012825635189,-25.8681765896183,
124.532704279284)) ;
#60233=CARTESIAN_POINT('Ctrl Pts',(-18.6028685580281,-25.6881875092555,
124.308517112761)) ;
#60234=CARTESIAN_POINT('Ctrl Pts',(-18.6786331146531,-25.8813952649994,
124.7419424)) ;
#60235=CARTESIAN_POINT('Ctrl Pts',(-18.8247543705837,-25.7014061846365,
124.475917413394)) ;
#60236=CARTESIAN_POINT('Ctrl Pts',(-19.0063037436624,-25.8947055722441,
124.875037990649)) ;
#60237=CARTESIAN_POINT('Ctrl Pts',(-19.0869232033359,-25.7147164918812,
124.582399636663)) ;
#60238=CARTESIAN_POINT('Ctrl Pts',(-19.3515492793032,-25.9079432384701,
124.918059062423)) ;
#60239=CARTESIAN_POINT('Ctrl Pts',(-19.3630728386149,-25.7279541581072,
124.616808324183)) ;
#60240=CARTESIAN_POINT('Ctrl Pts',(-19.6119358669547,-25.9178629338808,
124.905712873478)) ;
#60241=CARTESIAN_POINT('Ctrl Pts',(-19.5713918638856,-25.7378738535179,
124.606935541768)) ;
#60242=CARTESIAN_POINT('Ctrl Pts',(-19.8695568706956,-25.9279158008794,
124.847282646854)) ;
#60243=CARTESIAN_POINT('Ctrl Pts',(-19.7774862246626,-25.7479267205165,
124.560193132552)) ;
#60244=CARTESIAN_POINT('Ctrl Pts',(-20.1084811470634,-25.9377712092086,
124.747272818571)) ;
#60245=CARTESIAN_POINT('Ctrl Pts',(-19.9686281873536,-25.7577821288458,
124.480186034087)) ;
#60246=CARTESIAN_POINT('Ctrl Pts',(-20.3306652047621,-25.9478098408852,
124.60508116567)) ;
#60247=CARTESIAN_POINT('Ctrl Pts',(-20.1463738336963,-25.7678207605223,
124.366438470224)) ;
#60248=CARTESIAN_POINT('Ctrl Pts',(-20.5876341488702,-25.9611120231522,
124.368071353018)) ;
#60249=CARTESIAN_POINT('Ctrl Pts',(-20.3519625615486,-25.7811229427894,
124.176812457001)) ;
#60250=CARTESIAN_POINT('Ctrl Pts',(-20.8234715239028,-25.9776570362351,
123.996893725382)) ;
#60251=CARTESIAN_POINT('Ctrl Pts',(-20.5406208335467,-25.7976679558722,
123.87990862136)) ;
#60252=CARTESIAN_POINT('Ctrl Pts',(-20.9191905979447,-25.9943090523113,
123.56485434143)) ;
#60253=CARTESIAN_POINT('Ctrl Pts',(-20.6172087980807,-25.8143199719484,
123.534214776845)) ;
#60254=CARTESIAN_POINT('Ctrl Pts',(-20.9040855806235,-26.0075321432166,
123.217655815596)) ;
#60255=CARTESIAN_POINT('Ctrl Pts',(-20.6051216995438,-25.8275430628537,
123.256506511511)) ;
#60256=CARTESIAN_POINT('Ctrl Pts',(-20.8481710288913,-26.0174931027759,
122.961938491828)) ;
#60257=CARTESIAN_POINT('Ctrl Pts',(-20.5603924152172,-25.837504022413,123.051921427646)) ;
#60258=CARTESIAN_POINT('Ctrl Pts',(-20.7477672743641,-26.027517899527,122.718386742879)) ;
#60259=CARTESIAN_POINT('Ctrl Pts',(-20.4800725252395,-25.8475288191641,
122.857083778402)) ;
#60260=CARTESIAN_POINT('Ctrl Pts',(-20.561933381812,-26.0407423469228,122.424679164752)) ;
#60261=CARTESIAN_POINT('Ctrl Pts',(-20.3313987756676,-25.8607532665599,
122.622107468328)) ;
#60262=CARTESIAN_POINT('Ctrl Pts',(-20.2373134506599,-26.0573761316219,
122.124643357412)) ;
#60263=CARTESIAN_POINT('Ctrl Pts',(-20.0717139940136,-25.877387051259,122.382085646915)) ;
#60264=CARTESIAN_POINT('Ctrl Pts',(-19.7495611853889,-26.0772787983468,
121.919792632271)) ;
#60265=CARTESIAN_POINT('Ctrl Pts',(-19.6815098776299,-25.897289717984,122.218198920366)) ;
#60266=CARTESIAN_POINT('Ctrl Pts',(-19.22136228124,-26.0971790261287,121.892991857284)) ;
#60267=CARTESIAN_POINT('Ctrl Pts',(-19.2589510054893,-25.9171899457658,
122.196756056214)) ;
#60268=CARTESIAN_POINT('Ctrl Pts',(-18.715147674176,-26.1170965136602,122.047840068895)) ;
#60269=CARTESIAN_POINT('Ctrl Pts',(-18.8539776981445,-25.9371074332973,
122.320631958508)) ;
#60270=CARTESIAN_POINT('Ctrl Pts',(-18.2916834899083,-26.1370260394771,
122.366086543322)) ;
#60271=CARTESIAN_POINT('Ctrl Pts',(-18.5152044325254,-25.9570369591142,
122.575227523537)) ;
#60272=CARTESIAN_POINT('Ctrl Pts',(-18.0018457091614,-26.1569883073634,
122.810521281011)) ;
#60273=CARTESIAN_POINT('Ctrl Pts',(-18.283332009678,-25.9769992270005,122.930774214087)) ;
#60274=CARTESIAN_POINT('Ctrl Pts',(-17.8814876928622,-26.1768785023156,
123.325213587121)) ;
#60275=CARTESIAN_POINT('Ctrl Pts',(-18.1870431423497,-25.9968894219527,
123.342528513262)) ;
#60276=CARTESIAN_POINT('Ctrl Pts',(-17.942686360803,-26.1967687470618,123.850425839036)) ;
#60277=CARTESIAN_POINT('Ctrl Pts',(-18.2360005788665,-26.016779666699,123.762699536368)) ;
#60278=CARTESIAN_POINT('Ctrl Pts',(-18.182532872639,-26.2168431196243,124.326942241085)) ;
#60279=CARTESIAN_POINT('Ctrl Pts',(-18.4278757324527,-26.0368540392614,
124.143912810045)) ;
#60280=CARTESIAN_POINT('Ctrl Pts',(-18.5649877790472,-26.2366284969846,
124.687956672163)) ;
#60281=CARTESIAN_POINT('Ctrl Pts',(-18.7338401401723,-26.0566394166217,
124.432727122548)) ;
#60282=CARTESIAN_POINT('Ctrl Pts',(-19.0512197803277,-26.2565903710517,
124.900124064153)) ;
#60283=CARTESIAN_POINT('Ctrl Pts',(-19.1228258509435,-26.0766012906889,
124.602461970491)) ;
#60284=CARTESIAN_POINT('Ctrl Pts',(-19.5812880978387,-26.2765703465422,
124.932395779744)) ;
#60285=CARTESIAN_POINT('Ctrl Pts',(-19.5468805975335,-26.0965812661794,
124.628280541388)) ;
#60286=CARTESIAN_POINT('Ctrl Pts',(-20.0865875254388,-26.2963827764202,
124.784090581285)) ;
#60287=CARTESIAN_POINT('Ctrl Pts',(-19.9511225306785,-26.1163936960573,
124.50963622777)) ;
#60288=CARTESIAN_POINT('Ctrl Pts',(-20.5148410357087,-26.3163628845105,
124.470248873448)) ;
#60289=CARTESIAN_POINT('Ctrl Pts',(-20.2937255891069,-26.1363738041476,
124.258562667596)) ;
#60290=CARTESIAN_POINT('Ctrl Pts',(-20.8089496480924,-26.3362572681077,
124.030690459046)) ;
#60291=CARTESIAN_POINT('Ctrl Pts',(-20.5290131148898,-26.1562681877448,
123.906914797705)) ;
#60292=CARTESIAN_POINT('Ctrl Pts',(-20.9360216455939,-26.3561841960849,
123.516657893152)) ;
#60293=CARTESIAN_POINT('Ctrl Pts',(-20.6306703947907,-26.1761951157221,
123.495687702575)) ;
#60294=CARTESIAN_POINT('Ctrl Pts',(-20.8808211228342,-26.3760790533862,
122.990653193015)) ;
#60295=CARTESIAN_POINT('Ctrl Pts',(-20.5865088182755,-26.1960899730233,
123.074882896028)) ;
#60296=CARTESIAN_POINT('Ctrl Pts',(-20.647350202661,-26.3961182469898,122.512000068605)) ;
#60297=CARTESIAN_POINT('Ctrl Pts',(-20.3997313810415,-26.2161291666269,
122.691961220065)) ;
#60298=CARTESIAN_POINT('Ctrl Pts',(-20.2682064549475,-26.4159582149006,
122.145440895336)) ;
#60299=CARTESIAN_POINT('Ctrl Pts',(-20.0964143290626,-26.2359691345377,
122.398713470548)) ;
#60300=CARTESIAN_POINT('Ctrl Pts',(-19.7855675978371,-26.4358730318646,
121.928243360252)) ;
#60301=CARTESIAN_POINT('Ctrl Pts',(-19.7103017055272,-26.2558839515018,
122.224956789686)) ;
#60302=CARTESIAN_POINT('Ctrl Pts',(-19.2570238059739,-26.4558152772609,
121.889095738746)) ;
#60303=CARTESIAN_POINT('Ctrl Pts',(-19.2874659515853,-26.275826196898,122.193640519728)) ;
#60304=CARTESIAN_POINT('Ctrl Pts',(-18.748249738879,-26.4756873253754,122.031335489932)) ;
#60305=CARTESIAN_POINT('Ctrl Pts',(-18.8804462675257,-26.2956982450125,
122.307434864793)) ;
#60306=CARTESIAN_POINT('Ctrl Pts',(-18.3160101803626,-26.4956983903295,
122.340952921604)) ;
#60307=CARTESIAN_POINT('Ctrl Pts',(-18.5346560494726,-26.3157093099666,
122.555130681776)) ;
#60308=CARTESIAN_POINT('Ctrl Pts',(-18.0174531568864,-26.5155099146331,
122.774978345867)) ;
#60309=CARTESIAN_POINT('Ctrl Pts',(-18.2958118673303,-26.3355208342703,
122.902353753564)) ;
#60310=CARTESIAN_POINT('Ctrl Pts',(-17.883457283048,-26.5356051265965,123.29177843999)) ;
#60311=CARTESIAN_POINT('Ctrl Pts',(-18.188618039186,-26.3556160462336,123.315793821141)) ;
#60312=CARTESIAN_POINT('Ctrl Pts',(-17.9332038026506,-26.5553858505163,
123.815368387734)) ;
#60313=CARTESIAN_POINT('Ctrl Pts',(-18.2284182371962,-26.3753967701534,
123.734667085211)) ;
#60314=CARTESIAN_POINT('Ctrl Pts',(-18.1597535329976,-26.5753769261591,
124.295760856938)) ;
#60315=CARTESIAN_POINT('Ctrl Pts',(-18.409661050836,-26.3953878457962,124.118979676145)) ;
#60316=CARTESIAN_POINT('Ctrl Pts',(-18.5350790245251,-26.5952588652021,
124.667951356014)) ;
#60317=CARTESIAN_POINT('Ctrl Pts',(-18.7099242517618,-26.4152697848392,
124.416730225271)) ;
#60318=CARTESIAN_POINT('Ctrl Pts',(-19.0161267182173,-26.6152114697054,
124.89094908574)) ;
#60319=CARTESIAN_POINT('Ctrl Pts',(-19.0947641449975,-26.4352223893425,
124.595125248235)) ;
#60320=CARTESIAN_POINT('Ctrl Pts',(-19.5431138580635,-26.635110338436,124.936289536443)) ;
#60321=CARTESIAN_POINT('Ctrl Pts',(-19.5163546351924,-26.4551212580731,
124.631394176078)) ;
#60322=CARTESIAN_POINT('Ctrl Pts',(-20.0538241489415,-26.6550037382456,
124.799784245693)) ;
#60323=CARTESIAN_POINT('Ctrl Pts',(-19.9249224379141,-26.4750146578827,
124.522185551533)) ;
#60324=CARTESIAN_POINT('Ctrl Pts',(-20.4882718449817,-26.6749128690856,
124.497507103209)) ;
#60325=CARTESIAN_POINT('Ctrl Pts',(-20.2724781151579,-26.4949237887228,
124.280362392057)) ;
#60326=CARTESIAN_POINT('Ctrl Pts',(-20.7946862216762,-26.6949449688492,
124.062171882771)) ;
#60327=CARTESIAN_POINT('Ctrl Pts',(-20.5176077611612,-26.5149558884863,
123.932084425509)) ;
#60328=CARTESIAN_POINT('Ctrl Pts',(-20.9099487231253,-26.7114770420187,
123.638071483004)) ;
#60329=CARTESIAN_POINT('Ctrl Pts',(-20.6098098769218,-26.5314879616558,
123.592826514406)) ;
#60330=CARTESIAN_POINT('Ctrl Pts',(-20.9115489477632,-26.7248123826246,
123.287684923675)) ;
#60331=CARTESIAN_POINT('Ctrl Pts',(-20.6110911397521,-26.5448233022617,
123.312495827901)) ;
#60332=CARTESIAN_POINT('Ctrl Pts',(-20.8682561091955,-26.7346549411643,
123.032650001442)) ;
#60333=CARTESIAN_POINT('Ctrl Pts',(-20.5764556671409,-26.5546658608015,
123.108474233604)) ;
#60334=CARTESIAN_POINT('Ctrl Pts',(-20.77977083026,-26.7447068480142,122.78379500435)) ;
#60335=CARTESIAN_POINT('Ctrl Pts',(-20.5056588060069,-26.5647177676514,
122.909381558418)) ;
#60336=CARTESIAN_POINT('Ctrl Pts',(-20.6078481493321,-26.7579553624051,
122.480989791618)) ;
#60337=CARTESIAN_POINT('Ctrl Pts',(-20.368152466766,-26.5779662820423,122.667181160605)) ;
#60338=CARTESIAN_POINT('Ctrl Pts',(-20.2986718809481,-26.7745545373529,
122.166348506659)) ;
#60339=CARTESIAN_POINT('Ctrl Pts',(-20.120762032831,-26.59456545699,122.415419305003)) ;
#60340=CARTESIAN_POINT('Ctrl Pts',(-19.9009478345017,-26.7911433231479,
121.976048097058)) ;
#60341=CARTESIAN_POINT('Ctrl Pts',(-19.8026233502208,-26.6111542427851,
122.263209553901)) ;
#60342=CARTESIAN_POINT('Ctrl Pts',(-19.5580496300445,-26.8044191394899,
121.911724128209)) ;
#60343=CARTESIAN_POINT('Ctrl Pts',(-19.5282751818262,-26.624430059127,122.211739560136)) ;
#60344=CARTESIAN_POINT('Ctrl Pts',(-19.2959531359205,-26.8143929902837,
121.908486613091)) ;
#60345=CARTESIAN_POINT('Ctrl Pts',(-19.3186038165586,-26.6344039099208,
122.209154538032)) ;
#60346=CARTESIAN_POINT('Ctrl Pts',(-19.0359115386452,-26.8244220223761,
121.951317775132)) ;
#60347=CARTESIAN_POINT('Ctrl Pts',(-19.1105694160277,-26.6444329420132,
122.243420903689)) ;
#60348=CARTESIAN_POINT('Ctrl Pts',(-18.7905877643252,-26.834312147878,122.037189062032)) ;
#60349=CARTESIAN_POINT('Ctrl Pts',(-18.9143114743061,-26.6543230675151,
122.312120264419)) ;
#60350=CARTESIAN_POINT('Ctrl Pts',(-18.5614228030226,-26.8443046261495,
122.165337470072)) ;
#60351=CARTESIAN_POINT('Ctrl Pts',(-18.7309805312086,-26.6643155457866,
122.414640877474)) ;
#60352=CARTESIAN_POINT('Ctrl Pts',(-18.3586851596353,-26.8542558412469,
122.330580371171)) ;
#60353=CARTESIAN_POINT('Ctrl Pts',(-18.5687918791563,-26.674266760884,122.546836944886)) ;
#60354=CARTESIAN_POINT('Ctrl Pts',(-18.1862556413636,-26.8643043430019,
122.530537857795)) ;
#60355=CARTESIAN_POINT('Ctrl Pts',(-18.4308500085545,-26.6843152626391,
122.706804337278)) ;
#60356=CARTESIAN_POINT('Ctrl Pts',(-18.0536640724743,-26.8741456926187,
122.752611956706)) ;
#60357=CARTESIAN_POINT('Ctrl Pts',(-18.3247786705187,-26.6941566122558,
122.884464800855)) ;
#60358=CARTESIAN_POINT('Ctrl Pts',(-17.9597894559771,-26.8841319836389,
122.997630523713)) ;
#60359=CARTESIAN_POINT('Ctrl Pts',(-18.2496811140076,-26.7041429032761,
123.080480402911)) ;
#60360=CARTESIAN_POINT('Ctrl Pts',(-17.9099883261813,-26.8940685953675,
123.254005646133)) ;
#60361=CARTESIAN_POINT('Ctrl Pts',(-18.2098424357147,-26.7140795150047,
123.285580874397)) ;
#60362=CARTESIAN_POINT('Ctrl Pts',(-17.9055405282516,-26.9041184707351,
123.518041545854)) ;
#60363=CARTESIAN_POINT('Ctrl Pts',(-18.2062864585873,-26.7241293903722,
123.496809585011)) ;
#60364=CARTESIAN_POINT('Ctrl Pts',(-17.9459982769325,-26.9139689292705,
123.7737392886)) ;
#60365=CARTESIAN_POINT('Ctrl Pts',(-18.2386548730221,-26.7339798489077,
123.70136733283)) ;
#60366=CARTESIAN_POINT('Ctrl Pts',(-18.0306120394359,-26.9239408662233,
124.021720774531)) ;
#60367=CARTESIAN_POINT('Ctrl Pts',(-18.3063479820366,-26.7439517858604,
123.89975170688)) ;
#60368=CARTESIAN_POINT('Ctrl Pts',(-18.1573679303231,-26.9339363231554,
124.251828560722)) ;
#60369=CARTESIAN_POINT('Ctrl Pts',(-18.4077546301214,-26.7539472427925,
124.083836797404)) ;
#60370=CARTESIAN_POINT('Ctrl Pts',(-18.3229646348335,-26.9439691302085,
124.456964358552)) ;
#60371=CARTESIAN_POINT('Ctrl Pts',(-18.540233729948,-26.7639800498456,124.24794399399)) ;
#60372=CARTESIAN_POINT('Ctrl Pts',(-18.5180312778613,-26.9538290167985,
124.627530238962)) ;
#60373=CARTESIAN_POINT('Ctrl Pts',(-18.6962883826648,-26.7738399364356,
124.384394886845)) ;
#60374=CARTESIAN_POINT('Ctrl Pts',(-18.7423698226788,-26.9638180973637,
124.763794005457)) ;
#60375=CARTESIAN_POINT('Ctrl Pts',(-18.8757603004552,-26.7838290170008,
124.493403950581)) ;
#60376=CARTESIAN_POINT('Ctrl Pts',(-18.9855793301611,-26.9737495765729,
124.858494603905)) ;
#60377=CARTESIAN_POINT('Ctrl Pts',(-19.07032857135,-26.79376049621,124.569162300801)) ;
#60378=CARTESIAN_POINT('Ctrl Pts',(-19.2428644372235,-26.9837354360188,
124.910233267454)) ;
#60379=CARTESIAN_POINT('Ctrl Pts',(-19.2761570014402,-26.8037463556559,
124.610551055388)) ;
#60380=CARTESIAN_POINT('Ctrl Pts',(-19.5065740592286,-26.993773586666,124.916079842677)) ;
#60381=CARTESIAN_POINT('Ctrl Pts',(-19.4871247473151,-26.8137845063031,
124.615226085904)) ;
#60382=CARTESIAN_POINT('Ctrl Pts',(-19.7624778086568,-27.0036216771704,
124.877322071397)) ;
#60383=CARTESIAN_POINT('Ctrl Pts',(-19.691847097787,-26.8236325968075,124.584217745267)) ;
#60384=CARTESIAN_POINT('Ctrl Pts',(-20.0130872707028,-27.0136825856884,
124.793163184846)) ;
#60385=CARTESIAN_POINT('Ctrl Pts',(-19.892334005724,-26.8336935053255,124.51688855541)) ;
#60386=CARTESIAN_POINT('Ctrl Pts',(-20.2414042796906,-27.0235774328464,
124.668672645301)) ;
#60387=CARTESIAN_POINT('Ctrl Pts',(-20.0749863296734,-26.8435883524835,
124.417294323175)) ;
#60388=CARTESIAN_POINT('Ctrl Pts',(-20.4459889974729,-27.0335191048914,
124.506241389245)) ;
#60389=CARTESIAN_POINT('Ctrl Pts',(-20.238652605061,-26.8535300245285,124.287347771796)) ;
#60390=CARTESIAN_POINT('Ctrl Pts',(-20.6204448444618,-27.0435216320169,
124.309576543544)) ;
#60391=CARTESIAN_POINT('Ctrl Pts',(-20.3782156448559,-26.863532551654,124.130014531869)) ;
#60392=CARTESIAN_POINT('Ctrl Pts',(-20.758164805552,-27.0535564232043,124.084711962413)) ;
#60393=CARTESIAN_POINT('Ctrl Pts',(-20.4883897705064,-26.8735673428414,
123.950121722146)) ;
#60394=CARTESIAN_POINT('Ctrl Pts',(-20.8533381771542,-27.0634013030634,
123.8441219504)) ;
#60395=CARTESIAN_POINT('Ctrl Pts',(-20.5645263213738,-26.8834122227005,
123.757649351723)) ;
#60396=CARTESIAN_POINT('Ctrl Pts',(-20.9065073830601,-27.0733871836819,
123.587189440378)) ;
#60397=CARTESIAN_POINT('Ctrl Pts',(-20.6070596196296,-26.893398103319,123.552103047888)) ;
#60398=CARTESIAN_POINT('Ctrl Pts',(-20.9144081114304,-27.0833219067751,
123.326185418482)) ;
#60399=CARTESIAN_POINT('Ctrl Pts',(-20.6133781382632,-26.9033328264122,
123.343300030194)) ;
#60400=CARTESIAN_POINT('Ctrl Pts',(-20.8761775034525,-27.0933797470863,
123.064696003703)) ;
#60401=CARTESIAN_POINT('Ctrl Pts',(-20.5827915712378,-26.9133906667234,
123.134108707124)) ;
#60402=CARTESIAN_POINT('Ctrl Pts',(-20.7954566740253,-27.1032002344828,
122.819537535272)) ;
#60403=CARTESIAN_POINT('Ctrl Pts',(-20.5182131694661,-26.9232111541199,
122.937983169382)) ;
#60404=CARTESIAN_POINT('Ctrl Pts',(-20.6708300595228,-27.1132606358279,
122.586414372848)) ;
#60405=CARTESIAN_POINT('Ctrl Pts',(-20.418510079688,-26.9332715554651,122.751485490579)) ;
#60406=CARTESIAN_POINT('Ctrl Pts',(-20.5094030853154,-27.1231916013808,
122.381316698631)) ;
#60407=CARTESIAN_POINT('Ctrl Pts',(-20.2893670916496,-26.943202521018,122.587408842451)) ;
#60408=CARTESIAN_POINT('Ctrl Pts',(-20.3150919759397,-27.1331304637173,
122.206830149708)) ;
#60409=CARTESIAN_POINT('Ctrl Pts',(-20.133917119692,-26.9531413833544,122.44782126066)) ;
#60410=CARTESIAN_POINT('Ctrl Pts',(-20.0924353593602,-27.1431161946435,
122.067902692524)) ;
#60411=CARTESIAN_POINT('Ctrl Pts',(-19.9557909146957,-26.9631271142806,
122.336681000983)) ;
#60412=CARTESIAN_POINT('Ctrl Pts',(-19.8480377025175,-27.1531405800709,
121.969643385179)) ;
#60413=CARTESIAN_POINT('Ctrl Pts',(-19.7602720483066,-26.9731514997081,
122.258075383028)) ;
#60414=CARTESIAN_POINT('Ctrl Pts',(-19.59343508194,-27.1630438644242,121.915568323419)) ;
#60415=CARTESIAN_POINT('Ctrl Pts',(-19.5565899913194,-26.9830547840613,
122.214817300124)) ;
#60416=CARTESIAN_POINT('Ctrl Pts',(-19.3292573389903,-27.1731038690022,
121.90646877428)) ;
#60417=CARTESIAN_POINT('Ctrl Pts',(-19.3452475890792,-26.9931147886393,
122.207539583563)) ;
#60418=CARTESIAN_POINT('Ctrl Pts',(-19.0730690560541,-27.1829471380713,
121.942410469089)) ;
#60419=CARTESIAN_POINT('Ctrl Pts',(-19.1402979129544,-27.0029580577084,
122.236294726187)) ;
#60420=CARTESIAN_POINT('Ctrl Pts',(-18.8231985706705,-27.192937703679,122.02288556215)) ;
#60421=CARTESIAN_POINT('Ctrl Pts',(-18.9404022136018,-27.0129486233161,
122.300676481672)) ;
#60422=CARTESIAN_POINT('Ctrl Pts',(-18.5925284415636,-27.2028658354578,
122.144814465017)) ;
#60423=CARTESIAN_POINT('Ctrl Pts',(-18.7558673038755,-27.022876755095,122.398221026076)) ;
#60424=CARTESIAN_POINT('Ctrl Pts',(-18.3850125185332,-27.2128537225387,
122.305545417301)) ;
#60425=CARTESIAN_POINT('Ctrl Pts',(-18.5898557473657,-27.0328646421759,
122.526807075092)) ;
#60426=CARTESIAN_POINT('Ctrl Pts',(-18.2080550368114,-27.2228896721074,
122.501085855653)) ;
#60427=CARTESIAN_POINT('Ctrl Pts',(-18.4482910618857,-27.0429005917445,
122.683240696432)) ;
#60428=CARTESIAN_POINT('Ctrl Pts',(-18.0698877945043,-27.2327445584862,
122.720150718132)) ;
#60429=CARTESIAN_POINT('Ctrl Pts',(-18.3377591347981,-27.0527554781234,
122.858492893348)) ;
#60430=CARTESIAN_POINT('Ctrl Pts',(-17.9701127120356,-27.2427439728341,
122.963197940076)) ;
#60431=CARTESIAN_POINT('Ctrl Pts',(-18.2579406678591,-27.0627548924712,
123.05293121135)) ;
#60432=CARTESIAN_POINT('Ctrl Pts',(-17.9143476221429,-27.2526391380246,
123.217227543753)) ;
#60433=CARTESIAN_POINT('Ctrl Pts',(-18.2133303139703,-27.0726500576617,
123.256154668995)) ;
#60434=CARTESIAN_POINT('Ctrl Pts',(-17.9033877648429,-27.2626994567166,
123.481339637183)) ;
#60435=CARTESIAN_POINT('Ctrl Pts',(-18.2045640578609,-27.0827103763537,
123.467444605589)) ;
#60436=CARTESIAN_POINT('Ctrl Pts',(-17.937576742963,-27.2725495884926,123.737946697359)) ;
#60437=CARTESIAN_POINT('Ctrl Pts',(-18.2319167231407,-27.0925605081298,
123.672729209851)) ;
#60438=CARTESIAN_POINT('Ctrl Pts',(-18.0166306722375,-27.2825801589429,
123.989393136718)) ;
#60439=CARTESIAN_POINT('Ctrl Pts',(-18.2951613035429,-27.10259107858,123.873885960265)) ;
#60440=CARTESIAN_POINT('Ctrl Pts',(-18.1384764760697,-27.2925943096157,
124.222663794495)) ;
#60441=CARTESIAN_POINT('Ctrl Pts',(-18.3926393637792,-27.1126052292528,
124.060501732075)) ;
#60442=CARTESIAN_POINT('Ctrl Pts',(-18.2966929164752,-27.3024872431611,
124.428958569241)) ;
#60443=CARTESIAN_POINT('Ctrl Pts',(-18.5192133357134,-27.1224981627982,
124.225536119169)) ;
#60444=CARTESIAN_POINT('Ctrl Pts',(-18.4899718704159,-27.3124767571514,
124.60656373873)) ;
#60445=CARTESIAN_POINT('Ctrl Pts',(-18.673837373234,-27.1324876767885,124.367619065612)) ;
#60446=CARTESIAN_POINT('Ctrl Pts',(-18.7103215045909,-27.3224305278038,
124.74758509881)) ;
#60447=CARTESIAN_POINT('Ctrl Pts',(-18.8501175596139,-27.1424414474409,
124.480434760865)) ;
#60448=CARTESIAN_POINT('Ctrl Pts',(-18.9541222140896,-27.3324782964644,
124.848911596832)) ;
#60449=CARTESIAN_POINT('Ctrl Pts',(-19.0451588376447,-27.1524892161015,
124.561494652999)) ;
#60450=CARTESIAN_POINT('Ctrl Pts',(-19.2065092981465,-27.3423200229042,
124.905498197986)) ;
#60451=CARTESIAN_POINT('Ctrl Pts',(-19.2470678872194,-27.1623309425413,
124.606762343776)) ;
#60452=CARTESIAN_POINT('Ctrl Pts',(-19.4685730601993,-27.3523055397269,
124.918145048951)) ;
#60453=CARTESIAN_POINT('Ctrl Pts',(-19.456718762585,-27.172316459364,124.616878517439)) ;
#60454=CARTESIAN_POINT('Ctrl Pts',(-19.727737905255,-27.3622448714225,124.885335148688)) ;
#60455=CARTESIAN_POINT('Ctrl Pts',(-19.6640500453479,-27.1822557910596,
124.590629385903)) ;
#60456=CARTESIAN_POINT('Ctrl Pts',(-19.9797167083431,-27.37228464112,124.807206664709)) ;
#60457=CARTESIAN_POINT('Ctrl Pts',(-19.8656328181808,-27.1922955607571,
124.528125331113)) ;
#60458=CARTESIAN_POINT('Ctrl Pts',(-20.210851339288,-27.3821728023688,124.688432935281)) ;
#60459=CARTESIAN_POINT('Ctrl Pts',(-20.0505392887375,-27.2021837220059,
124.433105562087)) ;
#60460=CARTESIAN_POINT('Ctrl Pts',(-20.4202523049205,-27.3921623568712,
124.530127299133)) ;
#60461=CARTESIAN_POINT('Ctrl Pts',(-20.2180592277372,-27.2121732765083,
124.306460234651)) ;
#60462=CARTESIAN_POINT('Ctrl Pts',(-20.5982841261054,-27.4021207713948,
124.338329003495)) ;
#60463=CARTESIAN_POINT('Ctrl Pts',(-20.360483568371,-27.222131691032,124.153021035403)) ;
#60464=CARTESIAN_POINT('Ctrl Pts',(-20.7400208952278,-27.4120206842242,
124.120151747141)) ;
#60465=CARTESIAN_POINT('Ctrl Pts',(-20.473871715113,-27.2320316038613,123.9784792444)) ;
#60466=CARTESIAN_POINT('Ctrl Pts',(-20.8431437130591,-27.4220673838741,
123.877134998684)) ;
#60467=CARTESIAN_POINT('Ctrl Pts',(-20.5563690459131,-27.2420783035112,
123.784065268537)) ;
#60468=CARTESIAN_POINT('Ctrl Pts',(-20.9018126855217,-27.4319672441797,
123.623637353348)) ;
#60469=CARTESIAN_POINT('Ctrl Pts',(-20.6033030544183,-27.2519781638168,
123.581267614642)) ;
#60470=CARTESIAN_POINT('Ctrl Pts',(-20.9158681861848,-27.4420186483852,
123.359908517845)) ;
#60471=CARTESIAN_POINT('Ctrl Pts',(-20.614546450276,-27.2620295680223,123.370284295332)) ;
#60472=CARTESIAN_POINT('Ctrl Pts',(-20.8845444215458,-27.4518996853063,
123.102102763115)) ;
#60473=CARTESIAN_POINT('Ctrl Pts',(-20.5894865476393,-27.2719106049434,
123.164040624998)) ;
#60474=CARTESIAN_POINT('Ctrl Pts',(-20.8083897017697,-27.4618995174838,
122.850639705419)) ;
#60475=CARTESIAN_POINT('Ctrl Pts',(-20.5285619312095,-27.2819104371209,
122.962870552448)) ;
#60476=CARTESIAN_POINT('Ctrl Pts',(-20.6908521995959,-27.4718175204687,
122.61796100732)) ;
#60477=CARTESIAN_POINT('Ctrl Pts',(-20.43453143348,-27.2918284401058,122.776728527516)) ;
#60478=CARTESIAN_POINT('Ctrl Pts',(-20.5325862276468,-27.4818688263432,
122.406544566139)) ;
#60479=CARTESIAN_POINT('Ctrl Pts',(-20.3079178321186,-27.3018797459804,
122.607595752983)) ;
#60480=CARTESIAN_POINT('Ctrl Pts',(-20.3436360267876,-27.4917386497348,
122.228783160696)) ;
#60481=CARTESIAN_POINT('Ctrl Pts',(-20.1567577854576,-27.3117495693719,
122.465387842878)) ;
#60482=CARTESIAN_POINT('Ctrl Pts',(-20.1222882553386,-27.5018128157851,
122.083664260692)) ;
#60483=CARTESIAN_POINT('Ctrl Pts',(-19.9796788329855,-27.3218237354222,
122.349293214515)) ;
#60484=CARTESIAN_POINT('Ctrl Pts',(-19.8852542608473,-27.5116328999267,
121.981478176074)) ;
#60485=CARTESIAN_POINT('Ctrl Pts',(-19.7900524902871,-27.3316438195639,
122.267545514143)) ;
#60486=CARTESIAN_POINT('Ctrl Pts',(-19.6276445348726,-27.5217116266626,
121.920220233275)) ;
#60487=CARTESIAN_POINT('Ctrl Pts',(-19.5839641856869,-27.3417225462997,
122.218539730451)) ;
#60488=CARTESIAN_POINT('Ctrl Pts',(-19.3691479103184,-27.5315632073121,
121.904877852358)) ;
#60489=CARTESIAN_POINT('Ctrl Pts',(-19.3771679014181,-27.3515741269492,
122.206266540335)) ;
#60490=CARTESIAN_POINT('Ctrl Pts',(-19.1062132173581,-27.5416363356105,
121.935078088023)) ;
#60491=CARTESIAN_POINT('Ctrl Pts',(-19.1668198669398,-27.3616472552476,
122.230427363407)) ;
#60492=CARTESIAN_POINT('Ctrl Pts',(-18.8582685980059,-27.5514788135019,
122.008806224884)) ;
#60493=CARTESIAN_POINT('Ctrl Pts',(-18.9684654319779,-27.3714897331391,
122.289410133124)) ;
#60494=CARTESIAN_POINT('Ctrl Pts',(-18.6232876861483,-27.5614594201,122.125286522871)) ;
#60495=CARTESIAN_POINT('Ctrl Pts',(-18.7804810973601,-27.3814703397371,
122.382594611719)) ;
#60496=CARTESIAN_POINT('Ctrl Pts',(-18.4116002704639,-27.5714771291188,
122.281782687979)) ;
#60497=CARTESIAN_POINT('Ctrl Pts',(-18.6111314675826,-27.3914880487559,
122.507791959957)) ;
#60498=CARTESIAN_POINT('Ctrl Pts',(-18.2323009870814,-27.5813633081562,
122.469819398542)) ;
#60499=CARTESIAN_POINT('Ctrl Pts',(-18.4676929146779,-27.4013742277934,
122.65822097498)) ;
#60500=CARTESIAN_POINT('Ctrl Pts',(-18.0858887221731,-27.5914209207286,
122.689836404072)) ;
#60501=CARTESIAN_POINT('Ctrl Pts',(-18.3505632824027,-27.4114318403657,
122.834234999918)) ;
#60502=CARTESIAN_POINT('Ctrl Pts',(-17.981772680714,-27.6012973141007,122.927596725681)) ;
#60503=CARTESIAN_POINT('Ctrl Pts',(-18.2672711670262,-27.4213082337378,
123.024442556299)) ;
#60504=CARTESIAN_POINT('Ctrl Pts',(-17.9191542665853,-27.6112923422511,
123.182674524743)) ;
#60505=CARTESIAN_POINT('Ctrl Pts',(-18.2171766775005,-27.4313032618883,
123.228504708676)) ;
#60506=CARTESIAN_POINT('Ctrl Pts',(-17.9021807329972,-27.6213130890971,
123.445473162291)) ;
#60507=CARTESIAN_POINT('Ctrl Pts',(-18.2035981738734,-27.4413240087343,
123.4387436757)) ;
#60508=CARTESIAN_POINT('Ctrl Pts',(-17.930448869701,-27.6312151577635,123.704146901839)) ;
#60509=CARTESIAN_POINT('Ctrl Pts',(-18.2262128505501,-27.4512260774006,
123.645681876394)) ;
#60510=CARTESIAN_POINT('Ctrl Pts',(-18.0034825912362,-27.6412058975832,
123.956332064129)) ;
#60511=CARTESIAN_POINT('Ctrl Pts',(-18.2846399233845,-27.4612168172203,
123.847429782292)) ;
#60512=CARTESIAN_POINT('Ctrl Pts',(-18.1190427862629,-27.6511690937935,
124.191258163438)) ;
#60513=CARTESIAN_POINT('Ctrl Pts',(-18.3770881012001,-27.4711800134306,
124.035370248739)) ;
#60514=CARTESIAN_POINT('Ctrl Pts',(-18.2722240570765,-27.6610732780936,
124.401708795378)) ;
#60515=CARTESIAN_POINT('Ctrl Pts',(-18.4996327056077,-27.4810841977308,
124.203730123677)) ;
#60516=CARTESIAN_POINT('Ctrl Pts',(-18.4626904000373,-27.6711337384845,
124.585014918484)) ;
#60517=CARTESIAN_POINT('Ctrl Pts',(-18.6520060497622,-27.4911446581216,
124.350375149966)) ;
#60518=CARTESIAN_POINT('Ctrl Pts',(-18.6771667745688,-27.6809742843553,
124.729554078274)) ;
#60519=CARTESIAN_POINT('Ctrl Pts',(-18.8235861793774,-27.5009852039924,
124.466005811902)) ;
#60520=CARTESIAN_POINT('Ctrl Pts',(-18.9186090603338,-27.6910365050671,
124.83730737481)) ;
#60521=CARTESIAN_POINT('Ctrl Pts',(-19.016740247443,-27.5110474247042,124.552208638131)) ;
#60522=CARTESIAN_POINT('Ctrl Pts',(-19.1709926750529,-27.7009336480836,
124.900195583727)) ;
#60523=CARTESIAN_POINT('Ctrl Pts',(-19.2186463603094,-27.5209445677207,
124.602519015299)) ;
#60524=CARTESIAN_POINT('Ctrl Pts',(-19.4312729665485,-27.7108648245008,
124.919233320648)) ;
#60525=CARTESIAN_POINT('Ctrl Pts',(-19.4268700019089,-27.5308757441379,
124.617749388828)) ;
#60526=CARTESIAN_POINT('Ctrl Pts',(-19.6937795868889,-27.7209070382794,
124.892204557255)) ;
#60527=CARTESIAN_POINT('Ctrl Pts',(-19.636875479684,-27.5409179579165,124.59612651213)) ;
#60528=CARTESIAN_POINT('Ctrl Pts',(-19.9437421483585,-27.7307935784821,
124.821306255689)) ;
#60529=CARTESIAN_POINT('Ctrl Pts',(-19.836844746594,-27.5508044981193,124.539408302028)) ;
#60530=CARTESIAN_POINT('Ctrl Pts',(-20.180282407611,-27.7407871730876,124.707252644134)) ;
#60531=CARTESIAN_POINT('Ctrl Pts',(-20.0260769445174,-27.5607980927247,
124.448165758018)) ;
#60532=CARTESIAN_POINT('Ctrl Pts',(-20.3923713220577,-27.7507310482451,
124.554570637425)) ;
#60533=CARTESIAN_POINT('Ctrl Pts',(-20.1957478479467,-27.5707419678822,
124.326020684454)) ;
#60534=CARTESIAN_POINT('Ctrl Pts',(-20.5752568933734,-27.7606915843599,
124.367331130021)) ;
#60535=CARTESIAN_POINT('Ctrl Pts',(-20.3420563159796,-27.5807025039971,
124.176229618266)) ;
#60536=CARTESIAN_POINT('Ctrl Pts',(-20.7235437790341,-27.7706881876827,
124.150451479886)) ;
#60537=CARTESIAN_POINT('Ctrl Pts',(-20.4606861037265,-27.5906991073198,
124.002726235317)) ;
#60538=CARTESIAN_POINT('Ctrl Pts',(-20.8319614750394,-27.7807212706372,
123.910121632712)) ;
#60539=CARTESIAN_POINT('Ctrl Pts',(-20.5474206058342,-27.6007321902743,
123.810462391625)) ;
#60540=CARTESIAN_POINT('Ctrl Pts',(-20.8961417940296,-27.7905724393387,
123.65932892789)) ;
#60541=CARTESIAN_POINT('Ctrl Pts',(-20.5987649851893,-27.6105833589758,
123.609829391344)) ;
#60542=CARTESIAN_POINT('Ctrl Pts',(-20.9167937428057,-27.8005349300376,
123.398350225034)) ;
#60543=CARTESIAN_POINT('Ctrl Pts',(-20.6152871158748,-27.6205458496747,
123.401046845239)) ;
#60544=CARTESIAN_POINT('Ctrl Pts',(-20.8913248727649,-27.8105633584554,
123.136032193867)) ;
#60545=CARTESIAN_POINT('Ctrl Pts',(-20.5949125321571,-27.6305742780925,
123.191192291486)) ;
#60546=CARTESIAN_POINT('Ctrl Pts',(-20.8216156440544,-27.8204737258199,
122.885112920422)) ;
#60547=CARTESIAN_POINT('Ctrl Pts',(-20.5391458591745,-27.640484645457,122.990457403175)) ;
#60548=CARTESIAN_POINT('Ctrl Pts',(-20.7097290522174,-27.830408593435,122.649216253135)) ;
#60549=CARTESIAN_POINT('Ctrl Pts',(-20.4496374549925,-27.6504195130721,
122.801740241644)) ;
#60550=CARTESIAN_POINT('Ctrl Pts',(-20.5567753117552,-27.840449735414,122.434208642636)) ;
#60551=CARTESIAN_POINT('Ctrl Pts',(-20.3272749058312,-27.6604606550512,
122.629733654314)) ;
#60552=CARTESIAN_POINT('Ctrl Pts',(-20.371806724897,-27.8503368716172,122.251718186914)) ;
#60553=CARTESIAN_POINT('Ctrl Pts',(-20.1793011160621,-27.6703477912543,
122.483741378946)) ;
#60554=CARTESIAN_POINT('Ctrl Pts',(-20.1559638841929,-27.8603291540206,
122.102205529793)) ;
#60555=CARTESIAN_POINT('Ctrl Pts',(-20.006627433317,-27.6803400736577,122.364130687556)) ;
#60556=CARTESIAN_POINT('Ctrl Pts',(-19.9184230348256,-27.8702776819858,
121.99297454764)) ;
#60557=CARTESIAN_POINT('Ctrl Pts',(-19.816595474273,-27.6902886016229,122.276745372545)) ;
#60558=CARTESIAN_POINT('Ctrl Pts',(-19.665953180287,-27.8802144131479,121.926377817828)) ;
#60559=CARTESIAN_POINT('Ctrl Pts',(-19.6146203057764,-27.7002253327851,
122.223467276849)) ;
#60560=CARTESIAN_POINT('Ctrl Pts',(-19.4045120642448,-27.8901976240079,
121.904196807196)) ;
#60561=CARTESIAN_POINT('Ctrl Pts',(-19.4054676973117,-27.710208543645,122.205721541653)) ;
#60562=CARTESIAN_POINT('Ctrl Pts',(-19.1417251311674,-27.9002407231578,
121.92835440127)) ;
#60563=CARTESIAN_POINT('Ctrl Pts',(-19.1952379245654,-27.7202516427949,
122.225046799241)) ;
#60564=CARTESIAN_POINT('Ctrl Pts',(-18.892293224786,-27.9100716874327,121.995765252508)) ;
#60565=CARTESIAN_POINT('Ctrl Pts',(-18.9956932551907,-27.7300826070698,
122.278974240053)) ;
#60566=CARTESIAN_POINT('Ctrl Pts',(-18.6525836805033,-27.9201445398186,
122.107953193368)) ;
#60567=CARTESIAN_POINT('Ctrl Pts',(-18.8039248906843,-27.7401554594558,
122.368723808351)) ;
#60568=CARTESIAN_POINT('Ctrl Pts',(-18.4404518362338,-27.9300086675304,
122.256983728471)) ;
#60569=CARTESIAN_POINT('Ctrl Pts',(-18.6342195866533,-27.7500195871675,
122.487946889381)) ;
#60570=CARTESIAN_POINT('Ctrl Pts',(-18.2540538810711,-27.9400308696653,
122.44303741669)) ;
#60571=CARTESIAN_POINT('Ctrl Pts',(-18.4851003818533,-27.7600417893024,
122.636789047312)) ;
#60572=CARTESIAN_POINT('Ctrl Pts',(-18.1032133230383,-27.9500580626337,
122.659116134907)) ;
#60573=CARTESIAN_POINT('Ctrl Pts',(-18.3644270759834,-27.7700689822708,
122.809651490149)) ;
#60574=CARTESIAN_POINT('Ctrl Pts',(-17.9937284543403,-27.9599136566007,
122.893810711294)) ;
#60575=CARTESIAN_POINT('Ctrl Pts',(-18.2768385935525,-27.7799245762378,
122.997405800576)) ;
#60576=CARTESIAN_POINT('Ctrl Pts',(-17.9252066477856,-27.969870828466,123.146353412769)) ;
#60577=CARTESIAN_POINT('Ctrl Pts',(-18.2220200039114,-27.7898817481031,
123.199439298674)) ;
#60578=CARTESIAN_POINT('Ctrl Pts',(-17.9018363926086,-27.9799096724644,
123.409110487333)) ;
#60579=CARTESIAN_POINT('Ctrl Pts',(-18.2033226182715,-27.7999205921015,
123.409644963665)) ;
#60580=CARTESIAN_POINT('Ctrl Pts',(-17.9236207437678,-27.98978369634,123.667708642615)) ;
#60581=CARTESIAN_POINT('Ctrl Pts',(-18.2207487591916,-27.8097946159771,
123.616522787693)) ;
#60582=CARTESIAN_POINT('Ctrl Pts',(-17.9912807797275,-27.9998535223304,
123.923499029241)) ;
#60583=CARTESIAN_POINT('Ctrl Pts',(-18.2748756263371,-27.8198644419675,
123.821155692994)) ;
#60584=CARTESIAN_POINT('Ctrl Pts',(-18.0996170115864,-28.0096867662276,
124.158124720439)) ;
#60585=CARTESIAN_POINT('Ctrl Pts',(-18.3615429995661,-27.8296976858648,
124.008855863308)) ;
#60586=CARTESIAN_POINT('Ctrl Pts',(-18.249371382821,-28.0197171940007,124.375030745284)) ;
#60587=CARTESIAN_POINT('Ctrl Pts',(-18.481345335379,-27.8397281136378,124.182381569428)) ;
#60588=CARTESIAN_POINT('Ctrl Pts',(-18.4350962680924,-28.0297488107458,
124.562139179243)) ;
#60589=CARTESIAN_POINT('Ctrl Pts',(-18.6299243679393,-27.8497597303829,
124.332069278655)) ;
#60590=CARTESIAN_POINT('Ctrl Pts',(-18.6458160519967,-28.0395784877265,
124.711519341739)) ;
#60591=CARTESIAN_POINT('Ctrl Pts',(-18.798498550654,-27.8595894073637,124.451573974288)) ;
#60592=CARTESIAN_POINT('Ctrl Pts',(-18.8827549500496,-28.0495680045665,
124.824558143869)) ;
#60593=CARTESIAN_POINT('Ctrl Pts',(-18.9880488657586,-27.8695789242036,
124.542006370576)) ;
#60594=CARTESIAN_POINT('Ctrl Pts',(-19.1372585887124,-28.0596116167062,
124.894470815532)) ;
#60595=CARTESIAN_POINT('Ctrl Pts',(-19.1916515109275,-27.8796225363434,
124.597937922925)) ;
#60596=CARTESIAN_POINT('Ctrl Pts',(-19.3942099817878,-28.0694342230415,
124.91912779169)) ;
#60597=CARTESIAN_POINT('Ctrl Pts',(-19.3972114824336,-27.8894451426787,
124.617664945199)) ;
#60598=CARTESIAN_POINT('Ctrl Pts',(-19.6572218646034,-28.0794724529408,
124.898947663021)) ;
#60599=CARTESIAN_POINT('Ctrl Pts',(-19.6076212137935,-27.8994833725779,
124.601522486604)) ;
#60600=CARTESIAN_POINT('Ctrl Pts',(-19.9119170104515,-28.0894834877327,
124.832984826371)) ;
#60601=CARTESIAN_POINT('Ctrl Pts',(-19.8113776795567,-27.9094944073698,
124.548753715423)) ;
#60602=CARTESIAN_POINT('Ctrl Pts',(-20.1487320477206,-28.0993812186998,
124.725423875281)) ;
#60603=CARTESIAN_POINT('Ctrl Pts',(-20.000829845105,-27.919392138337,124.462706670356)) ;
#60604=CARTESIAN_POINT('Ctrl Pts',(-20.3654611748462,-28.1093708465503,
124.5772951408)) ;
#60605=CARTESIAN_POINT('Ctrl Pts',(-20.1742139780183,-27.9293817661874,
124.344205147162)) ;
#60606=CARTESIAN_POINT('Ctrl Pts',(-20.5524779416027,-28.1193266369963,
124.394341663434)) ;
#60607=CARTESIAN_POINT('Ctrl Pts',(-20.3238283305594,-27.9393375566334,
124.197843770989)) ;
#60608=CARTESIAN_POINT('Ctrl Pts',(-20.7048656204767,-28.1292540355584,
124.182581520283)) ;
#60609=CARTESIAN_POINT('Ctrl Pts',(-20.4457396528893,-27.9492649551955,
124.028437013102)) ;
#60610=CARTESIAN_POINT('Ctrl Pts',(-20.8192132351186,-28.1392796306682,
123.945237856592)) ;
#60611=CARTESIAN_POINT('Ctrl Pts',(-20.5372193152296,-27.9592905503054,
123.838562820331)) ;
#60612=CARTESIAN_POINT('Ctrl Pts',(-20.8897744387993,-28.1491654813378,
123.695212486568)) ;
#60613=CARTESIAN_POINT('Ctrl Pts',(-20.5936698151312,-27.9691764009749,
123.638543566476)) ;
#60614=CARTESIAN_POINT('Ctrl Pts',(-20.9167426862714,-28.159154661182,123.434089007642)) ;
#60615=CARTESIAN_POINT('Ctrl Pts',(-20.6152462522755,-27.9791655808191,
123.429645100009)) ;
#60616=CARTESIAN_POINT('Ctrl Pts',(-20.8973138529512,-28.1691958482856,
123.170934263122)) ;
#60617=CARTESIAN_POINT('Ctrl Pts',(-20.5997049495287,-27.9892067679227,
123.219121101024)) ;
#60618=CARTESIAN_POINT('Ctrl Pts',(-20.8342467261708,-28.1790284917615,
122.920361624849)) ;
#60619=CARTESIAN_POINT('Ctrl Pts',(-20.5492532207289,-27.9990394113987,
123.018663281372)) ;
#60620=CARTESIAN_POINT('Ctrl Pts',(-20.7275828726051,-28.189022441471,122.680368443651)) ;
#60621=CARTESIAN_POINT('Ctrl Pts',(-20.463923962656,-28.0090333611081,122.826668031653)) ;
#60622=CARTESIAN_POINT('Ctrl Pts',(-20.5798888066981,-28.1990515642475,
122.462081994114)) ;
#60623=CARTESIAN_POINT('Ctrl Pts',(-20.3457702502389,-28.0190624838847,
122.652037809533)) ;
#60624=CARTESIAN_POINT('Ctrl Pts',(-20.3996251641318,-28.2089276951662,
122.275347174546)) ;
#60625=CARTESIAN_POINT('Ctrl Pts',(-20.2015610992789,-28.0289386148033,
122.502648999522)) ;
#60626=CARTESIAN_POINT('Ctrl Pts',(-20.1873021799441,-28.2189257301832,
122.120642324747)) ;
#60627=CARTESIAN_POINT('Ctrl Pts',(-20.0317039475205,-28.0389366498204,
122.37888357736)) ;
#60628=CARTESIAN_POINT('Ctrl Pts',(-19.9533587455655,-28.2288396599419,
122.005916898594)) ;
#60629=CARTESIAN_POINT('Ctrl Pts',(-19.8445504140462,-28.0488505795791,
122.287101605949)) ;
#60630=CARTESIAN_POINT('Ctrl Pts',(-19.6998517913933,-28.2388828476797,
121.932573093305)) ;
#60631=CARTESIAN_POINT('Ctrl Pts',(-19.6417453532736,-28.0588937673169,
122.228424618319)) ;
#60632=CARTESIAN_POINT('Ctrl Pts',(-19.4411734358199,-28.2487826898201,
121.904743447238)) ;
#60633=CARTESIAN_POINT('Ctrl Pts',(-19.4348032777468,-28.0687936094572,
122.206158949824)) ;
#60634=CARTESIAN_POINT('Ctrl Pts',(-19.1791693222562,-28.2587739566281,
121.921854204058)) ;
#60635=CARTESIAN_POINT('Ctrl Pts',(-19.2251999469823,-28.0787848762652,
122.219845480099)) ;
#60636=CARTESIAN_POINT('Ctrl Pts',(-18.923180998322,-28.2688060587601,121.984895781452)) ;
#60637=CARTESIAN_POINT('Ctrl Pts',(-19.0204087941554,-28.0888169783972,
122.270276784581)) ;
#60638=CARTESIAN_POINT('Ctrl Pts',(-18.6858684267657,-28.2786729397148,
122.08935619064)) ;
#60639=CARTESIAN_POINT('Ctrl Pts',(-18.830558338332,-28.098683859352,122.353843037551)) ;
#60640=CARTESIAN_POINT('Ctrl Pts',(-18.4672132264588,-28.288664731003,122.234743944374)) ;
#60641=CARTESIAN_POINT('Ctrl Pts',(-18.6556330730798,-28.1086756506401,
122.470151422643)) ;
#60642=CARTESIAN_POINT('Ctrl Pts',(-18.276712974157,-28.2986968469145,122.416985014583)) ;
#60643=CARTESIAN_POINT('Ctrl Pts',(-18.5032314387329,-28.1187077665516,
122.615942781619)) ;
#60644=CARTESIAN_POINT('Ctrl Pts',(-18.1230016340979,-28.3085631637145,
122.625798315029)) ;
#60645=CARTESIAN_POINT('Ctrl Pts',(-18.380260910136,-28.1285740833517,122.782991837959)) ;
#60646=CARTESIAN_POINT('Ctrl Pts',(-18.0061033569078,-28.3185506451881,
122.86075275285)) ;
#60647=CARTESIAN_POINT('Ctrl Pts',(-18.2867404042396,-28.1385615648253,
122.970954341277)) ;
#60648=CARTESIAN_POINT('Ctrl Pts',(-17.931940003922,-28.328495569567,123.111391293711)) ;
#60649=CARTESIAN_POINT('Ctrl Pts',(-18.2274077034628,-28.1485064892042,
123.171464381746)) ;
#60650=CARTESIAN_POINT('Ctrl Pts',(-17.902279648867,-28.3385404554777,123.373664123611)) ;
#60651=CARTESIAN_POINT('Ctrl Pts',(-18.2036772802856,-28.1585513751149,
123.381282418945)) ;
#60652=CARTESIAN_POINT('Ctrl Pts',(-17.9180879856087,-28.3484025591903,
123.632366059909)) ;
#60653=CARTESIAN_POINT('Ctrl Pts',(-18.2163217656105,-28.1684134788274,
123.588243760099)) ;
#60654=CARTESIAN_POINT('Ctrl Pts',(-17.978845222314,-28.3583941230148,123.887787950721)) ;
#60655=CARTESIAN_POINT('Ctrl Pts',(-18.2649253910361,-28.1784050426519,
123.792581709161)) ;
#60656=CARTESIAN_POINT('Ctrl Pts',(-18.0825235360191,-28.3683269310777,
124.127337211337)) ;
#60657=CARTESIAN_POINT('Ctrl Pts',(-18.3478659549648,-28.1883378507148,
123.984221828264)) ;
#60658=CARTESIAN_POINT('Ctrl Pts',(-18.2257556811439,-28.378264033314,124.345706898237)) ;
#60659=CARTESIAN_POINT('Ctrl Pts',(-18.4624497295589,-28.1982749529511,
124.158918686381)) ;
#60660=CARTESIAN_POINT('Ctrl Pts',(-18.4070352870554,-28.3883164795844,
124.537830699298)) ;
#60661=CARTESIAN_POINT('Ctrl Pts',(-18.6074717934068,-28.2083273992215,
124.312619238854)) ;
#60662=CARTESIAN_POINT('Ctrl Pts',(-18.6143836431893,-28.398162595166,124.692645379455)) ;
#60663=CARTESIAN_POINT('Ctrl Pts',(-18.7733489636727,-28.2181735148031,
124.436472636285)) ;
#60664=CARTESIAN_POINT('Ctrl Pts',(-18.8499799673712,-28.4082106148809,
124.811841582492)) ;
#60665=CARTESIAN_POINT('Ctrl Pts',(-18.9618249984737,-28.228221534518,124.531831597543)) ;
#60666=CARTESIAN_POINT('Ctrl Pts',(-19.1001636769322,-28.4181525665098,
124.887173703346)) ;
#60667=CARTESIAN_POINT('Ctrl Pts',(-19.1619712108279,-28.238163486147,124.592099400923)) ;
#60668=CARTESIAN_POINT('Ctrl Pts',(-19.3594558684256,-28.4280913475089,
124.91855224253)) ;
#60669=CARTESIAN_POINT('Ctrl Pts',(-19.3694046064628,-28.248102267146,124.61720445296)) ;
#60670=CARTESIAN_POINT('Ctrl Pts',(-19.6225169288426,-28.438117396235,124.904110048364)) ;
#60671=CARTESIAN_POINT('Ctrl Pts',(-19.5798535127197,-28.2581283158721,
124.60565295931)) ;
#60672=CARTESIAN_POINT('Ctrl Pts',(-19.8756354818284,-28.4480042566432,
124.845353062354)) ;
#60673=CARTESIAN_POINT('Ctrl Pts',(-19.7823488152932,-28.2680151762803,
124.55864953328)) ;
#60674=CARTESIAN_POINT('Ctrl Pts',(-20.1181752200281,-28.458035531775,124.742190925089)) ;
#60675=CARTESIAN_POINT('Ctrl Pts',(-19.9763812831176,-28.2780464514121,
124.476122110811)) ;
#60676=CARTESIAN_POINT('Ctrl Pts',(-20.3360779496977,-28.4679185090754,
124.600777052286)) ;
#60677=CARTESIAN_POINT('Ctrl Pts',(-20.1507052303913,-28.2879294287125,
124.362992221081)) ;
#60678=CARTESIAN_POINT('Ctrl Pts',(-20.5293776948737,-28.4779753624826,
124.420644314917)) ;
#60679=CARTESIAN_POINT('Ctrl Pts',(-20.3053443489214,-28.2979862821197,
124.218890369488)) ;
#60680=CARTESIAN_POINT('Ctrl Pts',(-20.7382563360483,-28.4911436035585,
124.144618303968)) ;
#60681=CARTESIAN_POINT('Ctrl Pts',(-20.4724604249661,-28.3111545231956,
123.998058237581)) ;
#60682=CARTESIAN_POINT('Ctrl Pts',(-20.8725696183407,-28.504544632785,123.814898572995)) ;
#60683=CARTESIAN_POINT('Ctrl Pts',(-20.5799131718557,-28.3245555524222,
123.734258095252)) ;
#60684=CARTESIAN_POINT('Ctrl Pts',(-20.9154664864313,-28.5177575495159,
123.470229804426)) ;
#60685=CARTESIAN_POINT('Ctrl Pts',(-20.6142236339119,-28.337768469153,123.458566993245)) ;
#60686=CARTESIAN_POINT('Ctrl Pts',(-20.9031228604222,-28.5276859439691,
123.209668872578)) ;
#60687=CARTESIAN_POINT('Ctrl Pts',(-20.6043529645336,-28.3476968636062,
123.250109340891)) ;
#60688=CARTESIAN_POINT('Ctrl Pts',(-20.8455899283561,-28.5376674440972,
122.953713451803)) ;
#60689=CARTESIAN_POINT('Ctrl Pts',(-20.5583282472634,-28.3576783637344,
123.045346890605)) ;
#60690=CARTESIAN_POINT('Ctrl Pts',(-20.7435726949857,-28.5477079873673,
122.710393832338)) ;
#60691=CARTESIAN_POINT('Ctrl Pts',(-20.4767166760668,-28.3677189070045,
122.850689784726)) ;
#60692=CARTESIAN_POINT('Ctrl Pts',(-20.6038530329981,-28.5575573191504,
122.492510433972)) ;
#60693=CARTESIAN_POINT('Ctrl Pts',(-20.3649427782715,-28.3775682387876,
122.676381961247)) ;
#60694=CARTESIAN_POINT('Ctrl Pts',(-20.4263234254277,-28.5675527236221,
122.298921849287)) ;
#60695=CARTESIAN_POINT('Ctrl Pts',(-20.2229202780013,-28.3875636432592,
122.521509270193)) ;
#60696=CARTESIAN_POINT('Ctrl Pts',(-20.2171504397288,-28.5775690510707,
122.139134607576)) ;
#60697=CARTESIAN_POINT('Ctrl Pts',(-20.0555849188895,-28.3975799707078,
122.393679028551)) ;
#60698=CARTESIAN_POINT('Ctrl Pts',(-19.9087920777924,-28.5907927082372,
121.978832990271)) ;
#60699=CARTESIAN_POINT('Ctrl Pts',(-19.8088913174118,-28.4108036278744,
122.265428956437)) ;
#60700=CARTESIAN_POINT('Ctrl Pts',(-19.5639959876032,-28.6040869996266,
121.90200706357)) ;
#60701=CARTESIAN_POINT('Ctrl Pts',(-19.5330215630254,-28.4240979192637,
122.203967911005)) ;
#60702=CARTESIAN_POINT('Ctrl Pts',(-19.2151418343695,-28.6173713505581,
121.916882629654)) ;
#60703=CARTESIAN_POINT('Ctrl Pts',(-19.2539858779433,-28.4373822701952,
122.215868656955)) ;
#60704=CARTESIAN_POINT('Ctrl Pts',(-18.9592277477311,-28.6273437316199,
121.973142750752)) ;
#60705=CARTESIAN_POINT('Ctrl Pts',(-19.0492444708714,-28.447354651257,122.260874150028)) ;
#60706=CARTESIAN_POINT('Ctrl Pts',(-18.7182849243588,-28.6372521112455,
122.071948770313)) ;
#60707=CARTESIAN_POINT('Ctrl Pts',(-18.8564918768448,-28.4572630308826,
122.33991702492)) ;
#60708=CARTESIAN_POINT('Ctrl Pts',(-18.4950390577731,-28.6473061099936,
122.213201780035)) ;
#60709=CARTESIAN_POINT('Ctrl Pts',(-18.6778931410017,-28.4673170296307,
122.452918687146)) ;
#60710=CARTESIAN_POINT('Ctrl Pts',(-18.3032620688519,-28.6571683071099,
122.38756772639)) ;
#60711=CARTESIAN_POINT('Ctrl Pts',(-18.5244716495436,-28.477179226747,122.592405885585)) ;
#60712=CARTESIAN_POINT('Ctrl Pts',(-18.0882237967221,-28.670515433484,122.664637872146)) ;
#60713=CARTESIAN_POINT('Ctrl Pts',(-18.352430803744,-28.4905263531211,122.814082073788)) ;
#60714=CARTESIAN_POINT('Ctrl Pts',(-17.9176634712148,-28.6870523991254,
123.069772556873)) ;
#60715=CARTESIAN_POINT('Ctrl Pts',(-18.2159875992731,-28.5070633187626,
123.138150149593)) ;
#60716=CARTESIAN_POINT('Ctrl Pts',(-17.8947632869084,-28.7036870032994,
123.511208297081)) ;
#60717=CARTESIAN_POINT('Ctrl Pts',(-18.1976653221791,-28.5236979229365,
123.491362432851)) ;
#60718=CARTESIAN_POINT('Ctrl Pts',(-17.9677541226804,-28.716976796542,123.852806493769)) ;
#60719=CARTESIAN_POINT('Ctrl Pts',(-18.256052534024,-28.5369877161791,123.764590263567)) ;
#60720=CARTESIAN_POINT('Ctrl Pts',(-18.0656567609654,-28.7269294278014,
124.095304375433)) ;
#60721=CARTESIAN_POINT('Ctrl Pts',(-18.3343741827955,-28.5469403474385,
123.9586001496)) ;
#60722=CARTESIAN_POINT('Ctrl Pts',(-18.2039394803118,-28.7368813951061,
124.317317362258)) ;
#60723=CARTESIAN_POINT('Ctrl Pts',(-18.444996651739,-28.5568923147432,124.136207458359)) ;
#60724=CARTESIAN_POINT('Ctrl Pts',(-18.4387363200913,-28.7502486535699,
124.578542730155)) ;
#60725=CARTESIAN_POINT('Ctrl Pts',(-18.6328430825618,-28.570259573207,124.345197322045)) ;
#60726=CARTESIAN_POINT('Ctrl Pts',(-18.8064292376097,-28.7667654655191,
124.818587725884)) ;
#60727=CARTESIAN_POINT('Ctrl Pts',(-18.9269842710425,-28.5867763851562,
124.537227610055)) ;
#60728=CARTESIAN_POINT('Ctrl Pts',(-19.3245222155934,-28.7867913605254,
124.939922033055)) ;
#60729=CARTESIAN_POINT('Ctrl Pts',(-19.3414616488824,-28.6068022801626,
124.634301067543)) ;
#60730=CARTESIAN_POINT('Ctrl Pts',(-19.8475073460439,-28.8066020906556,
124.877979440127)) ;
#60731=CARTESIAN_POINT('Ctrl Pts',(-19.7598502986681,-28.6266130102927,
124.58474931514)) ;
#60732=CARTESIAN_POINT('Ctrl Pts',(-20.3222930272887,-28.8265793067854,
124.640387404646)) ;
#60733=CARTESIAN_POINT('Ctrl Pts',(-20.1396805393653,-28.6465902264226,
124.39467832848)) ;
#60734=CARTESIAN_POINT('Ctrl Pts',(-20.6858890813368,-28.8465061821807,
124.255335344324)) ;
#60735=CARTESIAN_POINT('Ctrl Pts',(-20.4305598381238,-28.6665171018178,
124.086638285115)) ;
#60736=CARTESIAN_POINT('Ctrl Pts',(-20.896748937638,-28.866327643657,123.772474684031)) ;
#60737=CARTESIAN_POINT('Ctrl Pts',(-20.5992504644692,-28.6863385632941,
123.700349310091)) ;
#60738=CARTESIAN_POINT('Ctrl Pts',(-20.930240651337,-28.8864019614663,123.240064582413)) ;
#60739=CARTESIAN_POINT('Ctrl Pts',(-20.6260460784137,-28.7064128811034,
123.27442205142)) ;
#60740=CARTESIAN_POINT('Ctrl Pts',(-20.7811745275789,-28.9062499304742,
122.733886817119)) ;
#60741=CARTESIAN_POINT('Ctrl Pts',(-20.5067950359757,-28.7262608501113,
122.869477923346)) ;
#60742=CARTESIAN_POINT('Ctrl Pts',(-20.4677973260097,-28.9261969645374,
122.306404432572)) ;
#60743=CARTESIAN_POINT('Ctrl Pts',(-20.2560944036663,-28.7462078841745,
122.527490503496)) ;
#60744=CARTESIAN_POINT('Ctrl Pts',(-20.0282780332881,-28.9460929155096,
122.012300463532)) ;
#60745=CARTESIAN_POINT('Ctrl Pts',(-19.9044790239162,-28.7661038351467,
122.292205334614)) ;
#60746=CARTESIAN_POINT('Ctrl Pts',(-19.5150711784553,-28.9659883951278,
121.885006525189)) ;
#60747=CARTESIAN_POINT('Ctrl Pts',(-19.4939126765269,-28.7859993147649,
122.190368780619)) ;
#60748=CARTESIAN_POINT('Ctrl Pts',(-18.987543756163,-28.9859445060926,121.940541079356)) ;
#60749=CARTESIAN_POINT('Ctrl Pts',(-19.0718901729245,-28.8059554257297,
122.234795557163)) ;
#60750=CARTESIAN_POINT('Ctrl Pts',(-18.5120357100849,-29.0058490541326,
122.172247469475)) ;
#60751=CARTESIAN_POINT('Ctrl Pts',(-18.6914823057681,-28.8258599737697,
122.420160465214)) ;
#60752=CARTESIAN_POINT('Ctrl Pts',(-18.1436273509991,-29.0257231784517,
122.550925494824)) ;
#60753=CARTESIAN_POINT('Ctrl Pts',(-18.3967545360288,-28.8457340980888,
122.723104052043)) ;
#60754=CARTESIAN_POINT('Ctrl Pts',(-17.9253569901024,-29.0457777084507,
123.037111210492)) ;
#60755=CARTESIAN_POINT('Ctrl Pts',(-18.2221384159378,-28.8657886280878,
123.112051915873)) ;
#60756=CARTESIAN_POINT('Ctrl Pts',(-17.8864107136343,-29.0655852222107,
123.562230606204)) ;
#60757=CARTESIAN_POINT('Ctrl Pts',(-18.1909813694771,-28.8855961418478,
123.532149866875)) ;
#60758=CARTESIAN_POINT('Ctrl Pts',(-18.0291344865639,-29.0855685779784,
124.073742812752)) ;
#60759=CARTESIAN_POINT('Ctrl Pts',(-18.3051612924804,-28.9055794976156,
123.941359571674)) ;
#60760=CARTESIAN_POINT('Ctrl Pts',(-18.3375275327191,-29.1054868805624,
124.504029337498)) ;
#60761=CARTESIAN_POINT('Ctrl Pts',(-18.5518768788528,-28.9254978001995,
124.285589192693)) ;
#60762=CARTESIAN_POINT('Ctrl Pts',(-18.7724331767996,-29.1253550960081,
124.803732067651)) ;
#60763=CARTESIAN_POINT('Ctrl Pts',(-18.8998033875348,-28.9453660156452,
124.525350924034)) ;
#60764=CARTESIAN_POINT('Ctrl Pts',(-19.2881479519155,-29.1454054128044,
124.937374691163)) ;
#60765=CARTESIAN_POINT('Ctrl Pts',(-19.3123750642973,-28.9654163324415,
124.632263609282)) ;
#60766=CARTESIAN_POINT('Ctrl Pts',(-19.8116842876558,-29.1651814746869,
124.888368150055)) ;
#60767=CARTESIAN_POINT('Ctrl Pts',(-19.7312061711631,-28.985192394324,124.59305641669)) ;
#60768=CARTESIAN_POINT('Ctrl Pts',(-20.2935470559368,-29.1852360803793,
124.661024000669)) ;
#60769=CARTESIAN_POINT('Ctrl Pts',(-20.1166950466578,-29.0052470000165,
124.411179407397)) ;
#60770=CARTESIAN_POINT('Ctrl Pts',(-20.6641709204212,-29.2050297695352,
124.287435707295)) ;
#60771=CARTESIAN_POINT('Ctrl Pts',(-20.413193887911,-29.0250406891723,124.112305976162)) ;
#60772=CARTESIAN_POINT('Ctrl Pts',(-20.8881946382118,-29.2249964611296,
123.806481690324)) ;
#60773=CARTESIAN_POINT('Ctrl Pts',(-20.592410427374,-29.0450073807667,123.727541366071)) ;
#60774=CARTESIAN_POINT('Ctrl Pts',(-20.9338249693073,-29.2449565068806,
123.277844260743)) ;
#60775=CARTESIAN_POINT('Ctrl Pts',(-20.62891209658,-29.0649674265177,123.304630928054)) ;
#60776=CARTESIAN_POINT('Ctrl Pts',(-20.7971171356574,-29.2648547670308,
122.766988876807)) ;
#60777=CARTESIAN_POINT('Ctrl Pts',(-20.5195428530867,-29.084865686668,122.895946613903)) ;
#60778=CARTESIAN_POINT('Ctrl Pts',(-20.4948597929885,-29.28474968258,122.33314837501)) ;
#60779=CARTESIAN_POINT('Ctrl Pts',(-20.2777339778196,-29.1047606022171,
122.548875457773)) ;
#60780=CARTESIAN_POINT('Ctrl Pts',(-20.0626359964947,-29.3046598629936,
122.027845909722)) ;
#60781=CARTESIAN_POINT('Ctrl Pts',(-19.9319525576066,-29.1246707826307,
122.304635941344)) ;
#60782=CARTESIAN_POINT('Ctrl Pts',(-19.5515593327172,-29.3245956621079,
121.887948224382)) ;
#60783=CARTESIAN_POINT('Ctrl Pts',(-19.5230899669336,-29.144606581745,122.19272116096)) ;
#60784=CARTESIAN_POINT('Ctrl Pts',(-19.0233846938744,-29.344533523762,121.930820617086)) ;
#60785=CARTESIAN_POINT('Ctrl Pts',(-19.1005502612154,-29.1645444433991,
122.227022574999)) ;
#60786=CARTESIAN_POINT('Ctrl Pts',(-18.5418309889796,-29.3644525703997,
122.150865733304)) ;
#60787=CARTESIAN_POINT('Ctrl Pts',(-18.7153085362879,-29.1844634900368,
122.403062807844)) ;
#60788=CARTESIAN_POINT('Ctrl Pts',(-18.1636813294162,-29.3844014684538,
122.522511403366)) ;
#60789=CARTESIAN_POINT('Ctrl Pts',(-18.4127914568634,-29.2044123880909,
122.700380148177)) ;
#60790=CARTESIAN_POINT('Ctrl Pts',(-17.9354075384507,-29.4043072958969,
122.999821271264)) ;
#60791=CARTESIAN_POINT('Ctrl Pts',(-18.2301756194061,-29.224318215534,123.082237846385)) ;
#60792=CARTESIAN_POINT('Ctrl Pts',(-17.8918934979895,-29.4208899912622,
123.438338526591)) ;
#60793=CARTESIAN_POINT('Ctrl Pts',(-18.195368494416,-29.2409009108993,123.4330280738)) ;
#60794=CARTESIAN_POINT('Ctrl Pts',(-17.9480247352152,-29.4341642049858,
123.782679410161)) ;
#60795=CARTESIAN_POINT('Ctrl Pts',(-18.2402760241612,-29.2541751246229,
123.708522277928)) ;
#60796=CARTESIAN_POINT('Ctrl Pts',(-18.0352295821613,-29.4442109241851,
124.031850013628)) ;
#60797=CARTESIAN_POINT('Ctrl Pts',(-18.3100397891959,-29.2642218438223,
123.907851739695)) ;
#60798=CARTESIAN_POINT('Ctrl Pts',(-18.1615379687603,-29.4540549588308,
124.257627504343)) ;
#60799=CARTESIAN_POINT('Ctrl Pts',(-18.4110966944545,-29.2740658784679,
124.088481420666)) ;
#60800=CARTESIAN_POINT('Ctrl Pts',(-18.3825117400926,-29.4673893437353,
124.529570908532)) ;
#60801=CARTESIAN_POINT('Ctrl Pts',(-18.587837079466,-29.2874002633725,124.305998087073)) ;
#60802=CARTESIAN_POINT('Ctrl Pts',(-18.7397290349317,-29.4839765610351,
124.788022651488)) ;
#60803=CARTESIAN_POINT('Ctrl Pts',(-18.8736672821377,-29.3039874806722,
124.512799388885)) ;
#60804=CARTESIAN_POINT('Ctrl Pts',(-19.1646822605817,-29.500609773073,124.90971077457)) ;
#60805=CARTESIAN_POINT('Ctrl Pts',(-19.2135860980992,-29.3206206927101,
124.610126710635)) ;
#60806=CARTESIAN_POINT('Ctrl Pts',(-19.5137203885275,-29.5138922153452,
124.915596996125)) ;
#60807=CARTESIAN_POINT('Ctrl Pts',(-19.4928464224192,-29.3339031349823,
124.614841247233)) ;
#60808=CARTESIAN_POINT('Ctrl Pts',(-19.7708729287446,-29.5237981032594,
124.875254844356)) ;
#60809=CARTESIAN_POINT('Ctrl Pts',(-19.6985621395063,-29.3438090228965,
124.582563747932)) ;
#60810=CARTESIAN_POINT('Ctrl Pts',(-20.0193014854552,-29.5337865213645,
124.790472867222)) ;
#60811=CARTESIAN_POINT('Ctrl Pts',(-19.8973061999821,-29.3537974410017,
124.51473599808)) ;
#60812=CARTESIAN_POINT('Ctrl Pts',(-20.2499022751864,-29.5438099486033,
124.663153811252)) ;
#60813=CARTESIAN_POINT('Ctrl Pts',(-20.0817838661683,-29.3638208682404,
124.412880687566)) ;
#60814=CARTESIAN_POINT('Ctrl Pts',(-20.4525327560064,-29.5537143797203,
124.499823981593)) ;
#60815=CARTESIAN_POINT('Ctrl Pts',(-20.2438922431529,-29.3737252993574,
124.282207749836)) ;
#60816=CARTESIAN_POINT('Ctrl Pts',(-20.6825120254526,-29.5669775323307,
124.237867726831)) ;
#60817=CARTESIAN_POINT('Ctrl Pts',(-20.4278473773578,-29.3869884519678,
124.072677218546)) ;
#60818=CARTESIAN_POINT('Ctrl Pts',(-20.8392151516731,-29.5803024302346,
123.9203381995)) ;
#60819=CARTESIAN_POINT('Ctrl Pts',(-20.553226732279,-29.4003133498717,123.818635845126)) ;
#60820=CARTESIAN_POINT('Ctrl Pts',(-20.9074394904579,-29.5935581738502,
123.578684401647)) ;
#60821=CARTESIAN_POINT('Ctrl Pts',(-20.6078059447763,-29.4135690934873,
123.545295374543)) ;
#60822=CARTESIAN_POINT('Ctrl Pts',(-20.9137330388378,-29.6035175472975,
123.317072430943)) ;
#60823=CARTESIAN_POINT('Ctrl Pts',(-20.6128379811963,-29.4235284669346,
123.336009184031)) ;
#60824=CARTESIAN_POINT('Ctrl Pts',(-20.8748846541773,-29.6134613712245,
123.058630457453)) ;
#60825=CARTESIAN_POINT('Ctrl Pts',(-20.5817571955094,-29.4334722908616,
123.129255093572)) ;
#60826=CARTESIAN_POINT('Ctrl Pts',(-20.7906838438031,-29.6235093153718,
122.808386846984)) ;
#60827=CARTESIAN_POINT('Ctrl Pts',(-20.5143943808657,-29.4435202350089,
122.929061213128)) ;
#60828=CARTESIAN_POINT('Ctrl Pts',(-20.666972739531,-29.6333602865899,122.580969032646)) ;
#60829=CARTESIAN_POINT('Ctrl Pts',(-20.4154235694875,-29.4533712062271,
122.747128058925)) ;
#60830=CARTESIAN_POINT('Ctrl Pts',(-20.504231739043,-29.643332104032,122.37561747521)) ;
#60831=CARTESIAN_POINT('Ctrl Pts',(-20.285229061277,-29.4633430236691,122.582848300707)) ;
#60832=CARTESIAN_POINT('Ctrl Pts',(-20.3077646577954,-29.6533275263241,
122.20121873475)) ;
#60833=CARTESIAN_POINT('Ctrl Pts',(-20.1280539536979,-29.4733384459612,
122.443331024174)) ;
#60834=CARTESIAN_POINT('Ctrl Pts',(-20.0830517816903,-29.6633605914478,
122.063322483088)) ;
#60835=CARTESIAN_POINT('Ctrl Pts',(-19.9482825016034,-29.4833715110849,
122.333015964112)) ;
#60836=CARTESIAN_POINT('Ctrl Pts',(-19.8419990547799,-29.673225924113,121.967921099706)) ;
#60837=CARTESIAN_POINT('Ctrl Pts',(-19.7554396557229,-29.4932368437501,
122.256697012164)) ;
#60838=CARTESIAN_POINT('Ctrl Pts',(-19.5857362753535,-29.6831864667106,
121.914563791572)) ;
#60839=CARTESIAN_POINT('Ctrl Pts',(-19.5504291017455,-29.5031973863477,
122.214013362556)) ;
#60840=CARTESIAN_POINT('Ctrl Pts',(-19.3221856204255,-29.6932201522123,
121.906899471747)) ;
#60841=CARTESIAN_POINT('Ctrl Pts',(-19.3395885271886,-29.5132310718494,
122.207884142788)) ;
#60842=CARTESIAN_POINT('Ctrl Pts',(-19.0650645565921,-29.7031049842026,
121.944106565339)) ;
#60843=CARTESIAN_POINT('Ctrl Pts',(-19.1338922165619,-29.5231159038397,
122.237651976139)) ;
#60844=CARTESIAN_POINT('Ctrl Pts',(-18.8138468784926,-29.7131724109624,
122.026926609439)) ;
#60845=CARTESIAN_POINT('Ctrl Pts',(-18.9329187385003,-29.5331833305995,
122.303910131109)) ;
#60846=CARTESIAN_POINT('Ctrl Pts',(-18.5859272208204,-29.7230109001213,
122.149077864787)) ;
#60847=CARTESIAN_POINT('Ctrl Pts',(-18.7505843444716,-29.5430218197584,
122.401632918194)) ;
#60848=CARTESIAN_POINT('Ctrl Pts',(-18.3778786570836,-29.7330743813114,
122.312276880641)) ;
#60849=CARTESIAN_POINT('Ctrl Pts',(-18.5841468108762,-29.5530853009485,
122.532193870255)) ;
#60850=CARTESIAN_POINT('Ctrl Pts',(-18.2044212593036,-29.7429685391265,
122.506008820073)) ;
#60851=CARTESIAN_POINT('Ctrl Pts',(-18.4453827052769,-29.5629794587636,
122.687180688913)) ;
#60852=CARTESIAN_POINT('Ctrl Pts',(-18.0660044708574,-29.7529103958708,
122.727551566468)) ;
#60853=CARTESIAN_POINT('Ctrl Pts',(-18.334651204385,-29.5729213155079,122.864415841661)) ;
#60854=CARTESIAN_POINT('Ctrl Pts',(-17.9674436496093,-29.7629128735422,
122.971267274101)) ;
#60855=CARTESIAN_POINT('Ctrl Pts',(-18.255804547113,-29.5829237931793,123.059389144256)) ;
#60856=CARTESIAN_POINT('Ctrl Pts',(-17.9129372902024,-29.7729476778465,
123.229259453664)) ;
#60857=CARTESIAN_POINT('Ctrl Pts',(-18.2122015796833,-29.5929585974836,
123.265783349704)) ;
#60858=CARTESIAN_POINT('Ctrl Pts',(-17.9037873257415,-29.7827925546922,
123.487828320676)) ;
#60859=CARTESIAN_POINT('Ctrl Pts',(-18.2048837514533,-29.6028034743293,
123.472638064826)) ;
#60860=CARTESIAN_POINT('Ctrl Pts',(-17.9396889314393,-29.7927784342477,
123.747736250522)) ;
#60861=CARTESIAN_POINT('Ctrl Pts',(-18.2336070824238,-29.6127893538848,
123.680563995791)) ;
#60862=CARTESIAN_POINT('Ctrl Pts',(-18.0196096204046,-29.8027131646062,
123.996330158484)) ;
#60863=CARTESIAN_POINT('Ctrl Pts',(-18.2975455112086,-29.6227240842433,
123.879438242773)) ;
#60864=CARTESIAN_POINT('Ctrl Pts',(-18.1431663387283,-29.8127709769191,
124.229931834435)) ;
#60865=CARTESIAN_POINT('Ctrl Pts',(-18.3963927784555,-29.6327818965562,
124.066318691056)) ;
#60866=CARTESIAN_POINT('Ctrl Pts',(-18.3012830487912,-29.8225915690435,
124.433951656902)) ;
#60867=CARTESIAN_POINT('Ctrl Pts',(-18.5228873635076,-29.6426024886806,
124.229532798967)) ;
#60868=CARTESIAN_POINT('Ctrl Pts',(-18.4969190824133,-29.8326581546532,
124.611938648179)) ;
#60869=CARTESIAN_POINT('Ctrl Pts',(-18.679397626606,-29.6526690742904,124.37192099675)) ;
#60870=CARTESIAN_POINT('Ctrl Pts',(-18.7169004533599,-29.8425577352351,
124.750929340355)) ;
#60871=CARTESIAN_POINT('Ctrl Pts',(-18.8553834510956,-29.6625686548722,
124.483111642557)) ;
#60872=CARTESIAN_POINT('Ctrl Pts',(-18.9612300162177,-29.8526093349133,
124.851178041536)) ;
#60873=CARTESIAN_POINT('Ctrl Pts',(-19.050847943237,-29.6726202545505,124.563308795822)) ;
#60874=CARTESIAN_POINT('Ctrl Pts',(-19.2147547487882,-29.8624835213303,
124.90669960071)) ;
#60875=CARTESIAN_POINT('Ctrl Pts',(-19.2536676428027,-29.6824944409674,
124.607724013081)) ;
#60876=CARTESIAN_POINT('Ctrl Pts',(-19.4787496446823,-29.8725399972112,
124.917720031893)) ;
#60877=CARTESIAN_POINT('Ctrl Pts',(-19.4648637461611,-29.6925509168483,
124.616538418507)) ;
#60878=CARTESIAN_POINT('Ctrl Pts',(-19.7365039466463,-29.8824329285138,
124.883386677831)) ;
#60879=CARTESIAN_POINT('Ctrl Pts',(-19.6710664653841,-29.7024438481509,
124.589069887457)) ;
#60880=CARTESIAN_POINT('Ctrl Pts',(-19.9885582400929,-29.8924957072264,
124.803550123632)) ;
#60881=CARTESIAN_POINT('Ctrl Pts',(-19.8727094596313,-29.7125066268636,
124.52519876481)) ;
#60882=CARTESIAN_POINT('Ctrl Pts',(-20.2179182729383,-29.9023382328076,
124.683922711731)) ;
#60883=CARTESIAN_POINT('Ctrl Pts',(-20.0561959904771,-29.7223491524447,
124.429495469086)) ;
#60884=CARTESIAN_POINT('Ctrl Pts',(-20.4264420362186,-29.9123289982325,
124.524451584241)) ;
#60885=CARTESIAN_POINT('Ctrl Pts',(-20.2230137897094,-29.7323399178696,
124.301917213795)) ;
#60886=CARTESIAN_POINT('Ctrl Pts',(-20.6029907905239,-29.9222570742305,
124.332343420825)) ;
#60887=CARTESIAN_POINT('Ctrl Pts',(-20.3642511922906,-29.7422679938676,
124.148229742484)) ;
#60888=CARTESIAN_POINT('Ctrl Pts',(-20.7447343008597,-29.9322449846175,
124.11142218186)) ;
#60889=CARTESIAN_POINT('Ctrl Pts',(-20.4776444559696,-29.7522559042547,
123.971491933959)) ;
#60890=CARTESIAN_POINT('Ctrl Pts',(-20.8460304545597,-29.9422808967425,
123.867929241378)) ;
#60891=CARTESIAN_POINT('Ctrl Pts',(-20.5586797287902,-29.7622918163796,
123.776696819529)) ;
#60892=CARTESIAN_POINT('Ctrl Pts',(-20.9028976475888,-29.9521359095901,
123.61524963978)) ;
#60893=CARTESIAN_POINT('Ctrl Pts',(-20.6041716209895,-29.7721468292273,
123.574553473142)) ;
#60894=CARTESIAN_POINT('Ctrl Pts',(-20.9155677101948,-29.9621348555064,
123.352835793816)) ;
#60895=CARTESIAN_POINT('Ctrl Pts',(-20.6143059849255,-29.7821457751435,
123.364622425134)) ;
#60896=CARTESIAN_POINT('Ctrl Pts',(-20.8830605294398,-29.9720317679544,
123.094753953415)) ;
#60897=CARTESIAN_POINT('Ctrl Pts',(-20.5882986910333,-29.7920426875915,
123.158157729796)) ;
#60898=CARTESIAN_POINT('Ctrl Pts',(-20.805069403928,-29.9820855660479,122.84235819033)) ;
#60899=CARTESIAN_POINT('Ctrl Pts',(-20.5259041888426,-29.802096485685,122.956241456897)) ;
#60900=CARTESIAN_POINT('Ctrl Pts',(-20.6865523391872,-29.9919664868746,
122.611290225832)) ;
#60901=CARTESIAN_POINT('Ctrl Pts',(-20.4310894079275,-29.8119774065117,
122.771388421395)) ;
#60902=CARTESIAN_POINT('Ctrl Pts',(-20.5281670015566,-30.0019710128723,
122.40148341337)) ;
#60903=CARTESIAN_POINT('Ctrl Pts',(-20.3043799645414,-29.8219819325095,
122.603543955252)) ;
#60904=CARTESIAN_POINT('Ctrl Pts',(-20.3360451640396,-30.0119549764898,
122.222739387201)) ;
#60905=CARTESIAN_POINT('Ctrl Pts',(-20.1506815650826,-29.8319658961269,
122.460549974152)) ;
#60906=CARTESIAN_POINT('Ctrl Pts',(-20.1144958155581,-30.0219946170411,
122.079517699187)) ;
#60907=CARTESIAN_POINT('Ctrl Pts',(-19.9734411337302,-29.8420055366782,
122.345973905275)) ;
#60908=CARTESIAN_POINT('Ctrl Pts',(-19.8762838854574,-30.0318386426558,
121.978637774701)) ;
#60909=CARTESIAN_POINT('Ctrl Pts',(-19.7828718281963,-29.8518495622929,
122.265271730029)) ;
#60910=CARTESIAN_POINT('Ctrl Pts',(-19.6205810796489,-30.0418296484732,
121.919049659348)) ;
#60911=CARTESIAN_POINT('Ctrl Pts',(-19.5783094204032,-29.8618405681103,
122.217602616233)) ;
#60912=CARTESIAN_POINT('Ctrl Pts',(-19.3571576412147,-30.0518674400053,
121.905299416152)) ;
#60913=CARTESIAN_POINT('Ctrl Pts',(-19.3675704851451,-29.8718783596425,
122.206603915684)) ;
#60914=CARTESIAN_POINT('Ctrl Pts',(-19.1003268169004,-30.0617118397937,
121.936426083733)) ;
#60915=CARTESIAN_POINT('Ctrl Pts',(-19.1621069272286,-29.8817227594309,
122.231506534638)) ;
#60916=CARTESIAN_POINT('Ctrl Pts',(-18.8491638611297,-30.0716966403505,
122.012238721689)) ;
#60917=CARTESIAN_POINT('Ctrl Pts',(-18.9611771300981,-29.8917075599876,
122.292157833579)) ;
#60918=CARTESIAN_POINT('Ctrl Pts',(-18.6159274223169,-30.0816361637616,
122.129904287764)) ;
#60919=CARTESIAN_POINT('Ctrl Pts',(-18.774588942654,-29.9016470833988,122.386291228805)) ;
#60920=CARTESIAN_POINT('Ctrl Pts',(-18.4046377386934,-30.0916758828626,
122.287871780247)) ;
#60921=CARTESIAN_POINT('Ctrl Pts',(-18.6055578744043,-29.9116868024998,
122.512666327168)) ;
#60922=CARTESIAN_POINT('Ctrl Pts',(-18.2265933390173,-30.1015640547819,
122.477161788335)) ;
#60923=CARTESIAN_POINT('Ctrl Pts',(-18.4631237804811,-29.921574974419,122.664098660573)) ;
#60924=CARTESIAN_POINT('Ctrl Pts',(-18.0822626446461,-30.1115536171989,
122.696428624441)) ;
#60925=CARTESIAN_POINT('Ctrl Pts',(-18.3476602845798,-29.931564536836,122.839512622054)) ;
#60926=CARTESIAN_POINT('Ctrl Pts',(-17.9786995241896,-30.1215119893936,
122.936755300708)) ;
#60927=CARTESIAN_POINT('Ctrl Pts',(-18.2648110278588,-29.9415229090307,
123.031774118599)) ;
#60928=CARTESIAN_POINT('Ctrl Pts',(-17.9181786121953,-30.1314120636243,
123.189791746356)) ;
#60929=CARTESIAN_POINT('Ctrl Pts',(-18.2163954912986,-29.9514229832614,
123.234202841237)) ;
#60930=CARTESIAN_POINT('Ctrl Pts',(-17.9023177046355,-30.1414581599979,
123.453303427384)) ;
#60931=CARTESIAN_POINT('Ctrl Pts',(-18.2037078197734,-29.961469079635,123.445012405779)) ;
#60932=CARTESIAN_POINT('Ctrl Pts',(-17.9320269697077,-30.151366743995,123.712002752069)) ;
#60933=CARTESIAN_POINT('Ctrl Pts',(-18.2274762127078,-29.9713776636321,
123.651971093748)) ;
#60934=CARTESIAN_POINT('Ctrl Pts',(-18.0064982865296,-30.1613773225859,
123.964313150607)) ;
#60935=CARTESIAN_POINT('Ctrl Pts',(-18.2870541704328,-29.981388242223,123.853819106392)) ;
#60936=CARTESIAN_POINT('Ctrl Pts',(-18.1243449648106,-30.1714064806987,
124.200064581345)) ;
#60937=CARTESIAN_POINT('Ctrl Pts',(-18.3813325117191,-29.9914174003359,
124.042419843847)) ;
#60938=CARTESIAN_POINT('Ctrl Pts',(-18.2782623863857,-30.1812593625368,
124.408253321648)) ;
#60939=CARTESIAN_POINT('Ctrl Pts',(-18.5044666446186,-30.0012702821739,
124.208969431975)) ;
#60940=CARTESIAN_POINT('Ctrl Pts',(-18.4674836005063,-30.1912189236878,
124.589086196399)) ;
#60941=CARTESIAN_POINT('Ctrl Pts',(-18.6558438971189,-30.0112298433249,
124.35363489223)) ;
#60942=CARTESIAN_POINT('Ctrl Pts',(-18.687199388826,-30.2012573582769,124.735052040734)) ;
#60943=CARTESIAN_POINT('Ctrl Pts',(-18.8316171435154,-30.021268277914,124.470406880302)) ;
#60944=CARTESIAN_POINT('Ctrl Pts',(-18.9248025261078,-30.211130630504,124.839385850343)) ;
#60945=CARTESIAN_POINT('Ctrl Pts',(-19.0216991485207,-30.0311415501411,
124.553872836708)) ;
#60946=CARTESIAN_POINT('Ctrl Pts',(-19.1819439103011,-30.2212038724976,
124.902021223868)) ;
#60947=CARTESIAN_POINT('Ctrl Pts',(-19.2274127817706,-30.0412147921347,
124.603980422162)) ;
#60948=CARTESIAN_POINT('Ctrl Pts',(-19.4395127810917,-30.2310242040306,
124.918975069592)) ;
#60949=CARTESIAN_POINT('Ctrl Pts',(-19.433466684621,-30.0510351236678,124.617542685309)) ;
#60950=CARTESIAN_POINT('Ctrl Pts',(-19.7027659038404,-30.2411028652574,
124.890467615748)) ;
#60951=CARTESIAN_POINT('Ctrl Pts',(-19.6440694852678,-30.0611137848945,
124.594736008976)) ;
#60952=CARTESIAN_POINT('Ctrl Pts',(-19.9514865660436,-30.2509544605516,
124.818398357271)) ;
#60953=CARTESIAN_POINT('Ctrl Pts',(-19.8430448190709,-30.0709653801888,
124.537080268754)) ;
#60954=CARTESIAN_POINT('Ctrl Pts',(-20.1891444820223,-30.2610275957804,
124.701927251076)) ;
#60955=CARTESIAN_POINT('Ctrl Pts',(-20.0331712033916,-30.0810385154176,
124.44390269208)) ;
#60956=CARTESIAN_POINT('Ctrl Pts',(-20.398106604193,-30.2708700313055,124.549458419366)) ;
#60957=CARTESIAN_POINT('Ctrl Pts',(-20.2003396262217,-30.0908809509426,
124.321927803439)) ;
#60958=CARTESIAN_POINT('Ctrl Pts',(-20.5805436587888,-30.2808508004389,
124.361037704408)) ;
#60959=CARTESIAN_POINT('Ctrl Pts',(-20.3462888173977,-30.100861720076,124.171191137294)) ;
#60960=CARTESIAN_POINT('Ctrl Pts',(-20.7276313527105,-30.2908679016827,
124.142726286126)) ;
#60961=CARTESIAN_POINT('Ctrl Pts',(-20.4639585479526,-30.1108788213199,
123.99654171188)) ;
#60962=CARTESIAN_POINT('Ctrl Pts',(-20.8336603363903,-30.3007563492846,
123.905461600815)) ;
#60963=CARTESIAN_POINT('Ctrl Pts',(-20.5487810297276,-30.1207672689217,
123.806730589124)) ;
#60964=CARTESIAN_POINT('Ctrl Pts',(-20.897966874934,-30.3108120634654,123.649176787978)) ;
#60965=CARTESIAN_POINT('Ctrl Pts',(-20.6002259506018,-30.1308229831026,
123.601702402648)) ;
#60966=CARTESIAN_POINT('Ctrl Pts',(-20.916501105489,-30.3206872698793,123.390311340077)) ;
#60967=CARTESIAN_POINT('Ctrl Pts',(-20.6150528932545,-30.1406981895164,
123.39461094526)) ;
#60968=CARTESIAN_POINT('Ctrl Pts',(-20.8901135577961,-30.330682322352,123.128988240062)) ;
#60969=CARTESIAN_POINT('Ctrl Pts',(-20.5939426563615,-30.1506932419891,
123.185552627896)) ;
#60970=CARTESIAN_POINT('Ctrl Pts',(-20.8181453544106,-30.3407042063141,
122.87563748445)) ;
#60971=CARTESIAN_POINT('Ctrl Pts',(-20.5363677699957,-30.1607151259512,
122.982872078019)) ;
#60972=CARTESIAN_POINT('Ctrl Pts',(-20.7048988527743,-30.3506081788434,
122.641302484579)) ;
#60973=CARTESIAN_POINT('Ctrl Pts',(-20.4457706757612,-30.1706190984805,
122.795404879528)) ;
#60974=CARTESIAN_POINT('Ctrl Pts',(-20.5516896929561,-30.3605966755043,
122.428164932682)) ;
#60975=CARTESIAN_POINT('Ctrl Pts',(-20.3232033327596,-30.1806075951414,
122.624895080866)) ;
#60976=CARTESIAN_POINT('Ctrl Pts',(-20.3641515811051,-30.3705604727523,
122.245458339291)) ;
#60977=CARTESIAN_POINT('Ctrl Pts',(-20.17317296099,-30.1905713923894,122.478730202668)) ;
#60978=CARTESIAN_POINT('Ctrl Pts',(-20.1493641423966,-30.3804644960603,
122.098426355358)) ;
#60979=CARTESIAN_POINT('Ctrl Pts',(-20.0013436095708,-30.2004754156974,
122.361105071754)) ;
#60980=CARTESIAN_POINT('Ctrl Pts',(-19.9085262576648,-30.3905249993819,
121.989448658708)) ;
#60981=CARTESIAN_POINT('Ctrl Pts',(-19.8086730047828,-30.2105359190191,
122.273922884312)) ;
#60982=CARTESIAN_POINT('Ctrl Pts',(-19.6580405512922,-30.4003655345218,
121.925039834791)) ;
#60983=CARTESIAN_POINT('Ctrl Pts',(-19.6082855766348,-30.2203764541589,
122.222396127967)) ;
#60984=CARTESIAN_POINT('Ctrl Pts',(-19.3944577950573,-30.4104277552264,
121.904320740095)) ;
#60985=CARTESIAN_POINT('Ctrl Pts',(-19.3974190827422,-30.2304386748635,
122.205820754266)) ;
#60986=CARTESIAN_POINT('Ctrl Pts',(-19.1355824753204,-30.4203249090026,
121.929541442186)) ;
#60987=CARTESIAN_POINT('Ctrl Pts',(-19.1903196245163,-30.2403358286398,
122.225997234219)) ;
#60988=CARTESIAN_POINT('Ctrl Pts',(-18.8839449757999,-30.4302560423881,
121.998725090014)) ;
#60989=CARTESIAN_POINT('Ctrl Pts',(-18.9890101207813,-30.2502669620252,
122.281343781079)) ;
#60990=CARTESIAN_POINT('Ctrl Pts',(-18.6456264180008,-30.4402984175338,
122.112067478881)) ;
#60991=CARTESIAN_POINT('Ctrl Pts',(-18.7983550586508,-30.260309337171,122.372017626633)) ;
#60992=CARTESIAN_POINT('Ctrl Pts',(-18.4338243469554,-30.4501843553,122.26253329312)) ;
#60993=CARTESIAN_POINT('Ctrl Pts',(-18.6289139946321,-30.2701952749371,
122.492389609933)) ;
#60994=CARTESIAN_POINT('Ctrl Pts',(-18.2490727524169,-30.4601801982848,
122.449233759781)) ;
#60995=CARTESIAN_POINT('Ctrl Pts',(-18.4811126123803,-30.2801911179219,
122.641749654634)) ;
#60996=CARTESIAN_POINT('Ctrl Pts',(-18.1003554686225,-30.4701221761634,
122.664059702261)) ;
#60997=CARTESIAN_POINT('Ctrl Pts',(-18.3621388222961,-30.2901330958005,
122.813609831262)) ;
#60998=CARTESIAN_POINT('Ctrl Pts',(-17.9906956060769,-30.4800815506444,
122.901684237793)) ;
#60999=CARTESIAN_POINT('Ctrl Pts',(-18.2744107413088,-30.3000924702815,
123.003708954726)) ;
#61000=CARTESIAN_POINT('Ctrl Pts',(-17.9235701573867,-30.4900781664782,
123.15569235127)) ;
#61001=CARTESIAN_POINT('Ctrl Pts',(-18.2207100063737,-30.3100890861153,
123.206915221358)) ;
#61002=CARTESIAN_POINT('Ctrl Pts',(-17.9018377987369,-30.5001123850517,
123.418476175523)) ;
#61003=CARTESIAN_POINT('Ctrl Pts',(-18.203323782619,-30.3201233046888,123.417142364106)) ;
#61004=CARTESIAN_POINT('Ctrl Pts',(-17.9253133851979,-30.5099654522623,
123.676335153502)) ;
#61005=CARTESIAN_POINT('Ctrl Pts',(-18.2221037452179,-30.3299763718994,
123.623428491503)) ;
#61006=CARTESIAN_POINT('Ctrl Pts',(-17.9932051454583,-30.5199257101399,
123.929113114964)) ;
#61007=CARTESIAN_POINT('Ctrl Pts',(-18.2764164755412,-30.339936629777,123.825650660064)) ;
#61008=CARTESIAN_POINT('Ctrl Pts',(-18.1050124820995,-30.5299547368455,
124.167789386581)) ;
#61009=CARTESIAN_POINT('Ctrl Pts',(-18.3658619051834,-30.3499656564826,
124.016591970179)) ;
#61010=CARTESIAN_POINT('Ctrl Pts',(-18.2546907015098,-30.5398649438799,
124.380895877564)) ;
#61011=CARTESIAN_POINT('Ctrl Pts',(-18.4856036341333,-30.3598758635171,
124.18707690079)) ;
#61012=CARTESIAN_POINT('Ctrl Pts',(-18.4390851726062,-30.5497998545275,
124.565733591977)) ;
#61013=CARTESIAN_POINT('Ctrl Pts',(-18.633118334194,-30.3698107741647,124.334947200933)) ;
#61014=CARTESIAN_POINT('Ctrl Pts',(-18.6551854058701,-30.5598409847068,
124.71713937099)) ;
#61015=CARTESIAN_POINT('Ctrl Pts',(-18.805998270169,-30.3798519043439,124.456072442656)) ;
#61016=CARTESIAN_POINT('Ctrl Pts',(-18.8905691522215,-30.5697281250767,
124.827187732175)) ;
#61017=CARTESIAN_POINT('Ctrl Pts',(-18.994304219969,-30.3897390447139,124.544111408934)) ;
#61018=CARTESIAN_POINT('Ctrl Pts',(-19.1440074490238,-30.5797204026127,
124.895826199179)) ;
#61019=CARTESIAN_POINT('Ctrl Pts',(-19.1970544909255,-30.3997313222498,
124.599022913111)) ;
#61020=CARTESIAN_POINT('Ctrl Pts',(-19.4044083048242,-30.589668945881,124.919242868932)) ;
#61021=CARTESIAN_POINT('Ctrl Pts',(-19.405374674023,-30.4096798655181,124.61775698852)) ;
#61022=CARTESIAN_POINT('Ctrl Pts',(-19.6646066985077,-30.5996056206982,
124.897490650973)) ;
#61023=CARTESIAN_POINT('Ctrl Pts',(-19.6135329527055,-30.4196165403353,
124.600356125457)) ;
#61024=CARTESIAN_POINT('Ctrl Pts',(-19.9183885696594,-30.6095890416346,
124.830870140857)) ;
#61025=CARTESIAN_POINT('Ctrl Pts',(-19.816558494324,-30.4295999612717,124.547060681517)) ;
#61026=CARTESIAN_POINT('Ctrl Pts',(-20.1579384638186,-30.6196313568238,
124.720177686834)) ;
#61027=CARTESIAN_POINT('Ctrl Pts',(-20.0081988873676,-30.4396422764609,
124.458507428981)) ;
#61028=CARTESIAN_POINT('Ctrl Pts',(-20.3705238609549,-30.629471674263,124.572936951925)) ;
#61029=CARTESIAN_POINT('Ctrl Pts',(-20.1782668479969,-30.4494825939001,
124.340716237617)) ;
#61030=CARTESIAN_POINT('Ctrl Pts',(-20.5582851075911,-30.6395013783205,
124.387959911787)) ;
#61031=CARTESIAN_POINT('Ctrl Pts',(-20.3284766672307,-30.4595122979576,
124.192735318187)) ;
#61032=CARTESIAN_POINT('Ctrl Pts',(-20.7103623023063,-30.649522335043,124.172970910553)) ;
#61033=CARTESIAN_POINT('Ctrl Pts',(-20.450139188978,-30.4695332546801,124.020744631255)) ;
#61034=CARTESIAN_POINT('Ctrl Pts',(-20.8216762306296,-30.6593888773466,
123.938777584491)) ;
#61035=CARTESIAN_POINT('Ctrl Pts',(-20.5391909126625,-30.4793997969837,
123.833391248542)) ;
#61036=CARTESIAN_POINT('Ctrl Pts',(-20.8920560097773,-30.6694599772918,
123.683674797178)) ;
#61037=CARTESIAN_POINT('Ctrl Pts',(-20.5954958516475,-30.4894708969289,
123.629309014543)) ;
#61038=CARTESIAN_POINT('Ctrl Pts',(-20.9165006065021,-30.6793020514693,
123.426182698946)) ;
#61039=CARTESIAN_POINT('Ctrl Pts',(-20.6150525003073,-30.4993129711065,
123.423316470327)) ;
#61040=CARTESIAN_POINT('Ctrl Pts',(-20.8965796706122,-30.6892628460564,
123.165188338066)) ;
#61041=CARTESIAN_POINT('Ctrl Pts',(-20.5991170611532,-30.5092737656935,
123.214521207781)) ;
#61042=CARTESIAN_POINT('Ctrl Pts',(-20.8306367978976,-30.6993007189572,
122.909788435439)) ;
#61043=CARTESIAN_POINT('Ctrl Pts',(-20.5463638720667,-30.5193116385943,
123.010200889343)) ;
#61044=CARTESIAN_POINT('Ctrl Pts',(-20.7235512011237,-30.7091750045013,
122.673393853135)) ;
#61045=CARTESIAN_POINT('Ctrl Pts',(-20.4606968923866,-30.5291859241384,
122.821085433644)) ;
#61046=CARTESIAN_POINT('Ctrl Pts',(-20.5741723489282,-30.7192447549152,
122.45500866596)) ;
#61047=CARTESIAN_POINT('Ctrl Pts',(-20.3411947055965,-30.5392556745523,
122.646376333744)) ;
#61048=CARTESIAN_POINT('Ctrl Pts',(-20.3935486500737,-30.7290780394499,
122.270181067719)) ;
#61049=CARTESIAN_POINT('Ctrl Pts',(-20.1966973937778,-30.549088959087,122.498514076006)) ;
#61050=CARTESIAN_POINT('Ctrl Pts',(-20.1798297267143,-30.7391083802499,
122.115914599699)) ;
#61051=CARTESIAN_POINT('Ctrl Pts',(-20.0257230530562,-30.559119299887,122.375099677665)) ;
#61052=CARTESIAN_POINT('Ctrl Pts',(-19.9421798972545,-30.7491403042495,
122.001770363478)) ;
#61053=CARTESIAN_POINT('Ctrl Pts',(-19.8356036909516,-30.5691512238866,
122.28378308955)) ;
#61054=CARTESIAN_POINT('Ctrl Pts',(-19.6936420289257,-30.7589688391854,
121.931532551847)) ;
#61055=CARTESIAN_POINT('Ctrl Pts',(-19.6367747626622,-30.5789797588226,
122.227591754788)) ;
#61056=CARTESIAN_POINT('Ctrl Pts',(-19.4324272173847,-30.7689626169501,
121.904361062443)) ;
#61057=CARTESIAN_POINT('Ctrl Pts',(-19.4278031940052,-30.5889735365872,
122.205853025448)) ;
#61058=CARTESIAN_POINT('Ctrl Pts',(-19.1696001927807,-30.7789903274356,
121.923539411999)) ;
#61059=CARTESIAN_POINT('Ctrl Pts',(-19.2175414369296,-30.5990012470728,
122.221194254643)) ;
#61060=CARTESIAN_POINT('Ctrl Pts',(-18.9175710994844,-30.7888787382696,
121.986850390428)) ;
#61061=CARTESIAN_POINT('Ctrl Pts',(-19.0159184367103,-30.6088896579067,
122.271841400405)) ;
#61062=CARTESIAN_POINT('Ctrl Pts',(-18.6780751168425,-30.7988555888051,
122.09348195838)) ;
#61063=CARTESIAN_POINT('Ctrl Pts',(-18.8243211846636,-30.6188665084423,
122.357145104466)) ;
#61064=CARTESIAN_POINT('Ctrl Pts',(-18.4603462228554,-30.8088473853556,
122.240311680779)) ;
#61065=CARTESIAN_POINT('Ctrl Pts',(-18.6501372714632,-30.6288583049927,
122.474607479311)) ;
#61066=CARTESIAN_POINT('Ctrl Pts',(-18.2708493730239,-30.8188833914493,
122.42371347671)) ;
#61067=CARTESIAN_POINT('Ctrl Pts',(-18.4985386630892,-30.6388943110864,
122.621327853477)) ;
#61068=CARTESIAN_POINT('Ctrl Pts',(-18.1185854663055,-30.8287341257121,
122.633088418445)) ;
#61069=CARTESIAN_POINT('Ctrl Pts',(-18.376726707459,-30.6487450453492,122.788826190101)) ;
#61070=CARTESIAN_POINT('Ctrl Pts',(-18.0029869058182,-30.8387253842403,
122.868789450594)) ;
#61071=CARTESIAN_POINT('Ctrl Pts',(-18.2842463850415,-30.6587363038774,
122.97738614376)) ;
#61072=CARTESIAN_POINT('Ctrl Pts',(-17.9304364001845,-30.8486432791435,
123.119155041273)) ;
#61073=CARTESIAN_POINT('Ctrl Pts',(-18.2262044469805,-30.6686541987806,
123.177677695621)) ;
#61074=CARTESIAN_POINT('Ctrl Pts',(-17.9020877614499,-30.8586714208065,
123.3811332833)) ;
#61075=CARTESIAN_POINT('Ctrl Pts',(-18.2035238003672,-30.6786823404437,
123.387260129306)) ;
#61076=CARTESIAN_POINT('Ctrl Pts',(-17.9193001864898,-30.8685565889224,
123.640341140622)) ;
#61077=CARTESIAN_POINT('Ctrl Pts',(-18.2172919455385,-30.6885675085595,
123.594625944928)) ;
#61078=CARTESIAN_POINT('Ctrl Pts',(-17.9812908655851,-30.8785459524284,
123.895432047551)) ;
#61079=CARTESIAN_POINT('Ctrl Pts',(-18.2668826491316,-30.6985568720655,
123.798698988406)) ;
#61080=CARTESIAN_POINT('Ctrl Pts',(-18.0876859531419,-30.8885870874385,
124.136901868337)) ;
#61081=CARTESIAN_POINT('Ctrl Pts',(-18.3519971252596,-30.7085980070756,
123.991875626918)) ;
#61082=CARTESIAN_POINT('Ctrl Pts',(-18.2309896742768,-30.8984197556265,
124.35190954771)) ;
#61083=CARTESIAN_POINT('Ctrl Pts',(-18.4666381458969,-30.7184306752636,
124.163882156588)) ;
#61084=CARTESIAN_POINT('Ctrl Pts',(-18.4118327452605,-30.908413658581,124.542354351649)) ;
#61085=CARTESIAN_POINT('Ctrl Pts',(-18.6113111190892,-30.7284245782181,
124.316239274634)) ;
#61086=CARTESIAN_POINT('Ctrl Pts',(-18.6240784848063,-30.9184429436655,
124.698611210536)) ;
#61087=CARTESIAN_POINT('Ctrl Pts',(-18.78110661491,-30.7384538633026,124.441246278568)) ;
#61088=CARTESIAN_POINT('Ctrl Pts',(-18.856433654806,-30.9283184721074,124.814232093926)) ;
#61089=CARTESIAN_POINT('Ctrl Pts',(-18.96698940901,-30.7483293917445,124.533744474627)) ;
#61090=CARTESIAN_POINT('Ctrl Pts',(-19.1083519713591,-30.9383187547235,
124.888948210804)) ;
#61091=CARTESIAN_POINT('Ctrl Pts',(-19.168523414082,-30.7583296743606,124.593519235513)) ;
#61092=CARTESIAN_POINT('Ctrl Pts',(-19.3671515658204,-30.9482307707805,
124.918740815708)) ;
#61093=CARTESIAN_POINT('Ctrl Pts',(-19.3755624914892,-30.7682416904176,
124.617355261869)) ;
#61094=CARTESIAN_POINT('Ctrl Pts',(-19.6305583756846,-30.9582728461195,
124.903010863025)) ;
#61095=CARTESIAN_POINT('Ctrl Pts',(-19.5862881163539,-30.7782837657566,
124.604773299001)) ;
#61096=CARTESIAN_POINT('Ctrl Pts',(-19.8836271403426,-30.9681726787756,
124.842636496997)) ;
#61097=CARTESIAN_POINT('Ctrl Pts',(-19.7887432076105,-30.7881835984127,
124.55647584906)) ;
#61098=CARTESIAN_POINT('Ctrl Pts',(-20.1248202353029,-30.9781650793536,
124.738811837685)) ;
#61099=CARTESIAN_POINT('Ctrl Pts',(-19.9816984157365,-30.7981759989908,
124.473418063959)) ;
#61100=CARTESIAN_POINT('Ctrl Pts',(-20.3449819506173,-30.988199101113,124.593690835872)) ;
#61101=CARTESIAN_POINT('Ctrl Pts',(-20.157828908641,-30.8082100207501,124.357322942106)) ;
#61102=CARTESIAN_POINT('Ctrl Pts',(-20.5335886314549,-30.9980637119542,
124.415853378407)) ;
#61103=CARTESIAN_POINT('Ctrl Pts',(-20.3087153229984,-30.8180746315913,
124.215054797051)) ;
#61104=CARTESIAN_POINT('Ctrl Pts',(-20.6909778265813,-31.0080561114154,
124.205652827145)) ;
#61105=CARTESIAN_POINT('Ctrl Pts',(-20.4346283289395,-30.8280670310525,
124.046895699291)) ;
#61106=CARTESIAN_POINT('Ctrl Pts',(-20.8094832862645,-31.0180880647483,
123.970160489407)) ;
#61107=CARTESIAN_POINT('Ctrl Pts',(-20.5294345476933,-30.8380989843854,
123.85850276039)) ;
#61108=CARTESIAN_POINT('Ctrl Pts',(-20.8844320812118,-31.0279544236899,
123.721940205726)) ;
#61109=CARTESIAN_POINT('Ctrl Pts',(-20.5893954864046,-30.8479653433271,
123.659927538539)) ;
#61110=CARTESIAN_POINT('Ctrl Pts',(-20.9159397608911,-31.0379418991757,
123.461410041658)) ;
#61111=CARTESIAN_POINT('Ctrl Pts',(-20.6146037560401,-30.8579528188129,
123.451503763144)) ;
#61112=CARTESIAN_POINT('Ctrl Pts',(-20.9019287886433,-31.0478868053642,
123.200405236579)) ;
#61113=CARTESIAN_POINT('Ctrl Pts',(-20.6033971453962,-30.8678977250013,
123.242699989987)) ;
#61114=CARTESIAN_POINT('Ctrl Pts',(-20.8420850390457,-31.0579317700244,
122.943333258433)) ;
#61115=CARTESIAN_POINT('Ctrl Pts',(-20.5555242372743,-30.8779426896616,
123.037041905058)) ;
#61116=CARTESIAN_POINT('Ctrl Pts',(-20.7406003647243,-31.0677935769293,
122.704848430439)) ;
#61117=CARTESIAN_POINT('Ctrl Pts',(-20.4743386257341,-30.8878044965664,
122.846253507543)) ;
#61118=CARTESIAN_POINT('Ctrl Pts',(-20.597822144092,-31.0777862492351,122.484491140274)) ;
#61119=CARTESIAN_POINT('Ctrl Pts',(-20.3601179413071,-30.8977971688722,
122.669966539594)) ;
#61120=CARTESIAN_POINT('Ctrl Pts',(-20.4200444703197,-31.0877149201804,
122.293491951008)) ;
#61121=CARTESIAN_POINT('Ctrl Pts',(-20.2178975346058,-30.9077258398175,
122.517165820862)) ;
#61122=CARTESIAN_POINT('Ctrl Pts',(-20.2115893827837,-31.0976674624057,
122.135563380117)) ;
#61123=CARTESIAN_POINT('Ctrl Pts',(-20.0511349097933,-30.9176783820428,
122.390821266279)) ;
#61124=CARTESIAN_POINT('Ctrl Pts',(-19.9777608298293,-31.1076688184016,
122.015498299379)) ;
#61125=CARTESIAN_POINT('Ctrl Pts',(-19.864073138811,-30.9276797380387,122.29476724589)) ;
#61126=CARTESIAN_POINT('Ctrl Pts',(-19.7258837090503,-31.1176974306763,
121.93800176093)) ;
#61127=CARTESIAN_POINT('Ctrl Pts',(-19.6625721285863,-30.9377083503134,
122.2327679101)) ;
#61128=CARTESIAN_POINT('Ctrl Pts',(-19.468678402315,-31.1275617652258,121.905569609794)) ;
#61129=CARTESIAN_POINT('Ctrl Pts',(-19.4568083670694,-30.9475726848629,
122.206820002847)) ;
#61130=CARTESIAN_POINT('Ctrl Pts',(-19.2064222623212,-31.1375540893024,
121.918044378445)) ;
#61131=CARTESIAN_POINT('Ctrl Pts',(-19.2470034110608,-30.9575650089395,
122.21679756988)) ;
#61132=CARTESIAN_POINT('Ctrl Pts',(-18.9518724580088,-31.1474815816683,
121.975353810798)) ;
#61133=CARTESIAN_POINT('Ctrl Pts',(-19.043363176175,-30.9674925013054,122.262642901527)) ;
#61134=CARTESIAN_POINT('Ctrl Pts',(-18.7087875925179,-31.1575089402191,
122.076985697164)) ;
#61135=CARTESIAN_POINT('Ctrl Pts',(-18.8488944626726,-30.9775198598562,
122.343946315082)) ;
#61136=CARTESIAN_POINT('Ctrl Pts',(-18.4899494031481,-31.1673953582702,
122.217086576)) ;
#61137=CARTESIAN_POINT('Ctrl Pts',(-18.6738227767691,-30.9874062779074,
122.456025072437)) ;
#61138=CARTESIAN_POINT('Ctrl Pts',(-18.2959218218459,-31.1774270930056,
122.395489361766)) ;
#61139=CARTESIAN_POINT('Ctrl Pts',(-18.5185992246313,-30.9974380126427,
122.59874560302)) ;
#61140=CARTESIAN_POINT('Ctrl Pts',(-18.1379570317836,-31.1873086742489,
122.601654224087)) ;
#61141=CARTESIAN_POINT('Ctrl Pts',(-18.3922256360828,-31.007319593886,122.763676083483)) ;
#61142=CARTESIAN_POINT('Ctrl Pts',(-18.0159864387997,-31.1973706522812,
122.836214609579)) ;
#61143=CARTESIAN_POINT('Ctrl Pts',(-18.2946471919646,-31.0173815719183,
122.951323289987)) ;
#61144=CARTESIAN_POINT('Ctrl Pts',(-17.9380997062694,-31.2072277306429,
123.083299705092)) ;
#61145=CARTESIAN_POINT('Ctrl Pts',(-18.2323356602816,-31.02723865028,123.148990682481)) ;
#61146=CARTESIAN_POINT('Ctrl Pts',(-17.9033134792368,-31.2172223037489,
123.343589981846)) ;
#61147=CARTESIAN_POINT('Ctrl Pts',(-18.204504458958,-31.037233223386,123.357222569661)) ;
#61148=CARTESIAN_POINT('Ctrl Pts',(-17.9140838363557,-31.2271481000365,
123.604243273479)) ;
#61149=CARTESIAN_POINT('Ctrl Pts',(-18.2131185010766,-31.0471590196736,
123.565745298409)) ;
#61150=CARTESIAN_POINT('Ctrl Pts',(-17.9704288396952,-31.2371734672062,
123.861581949243)) ;
#61151=CARTESIAN_POINT('Ctrl Pts',(-18.2581923330531,-31.0571843868434,
123.77161667508)) ;
#61152=CARTESIAN_POINT('Ctrl Pts',(-18.0692181290173,-31.2470695468601,
124.102157307068)) ;
#61153=CARTESIAN_POINT('Ctrl Pts',(-18.3372216027186,-31.0670804664972,
123.964077752132)) ;
#61154=CARTESIAN_POINT('Ctrl Pts',(-18.2092168773112,-31.2570646265657,
124.324401074987)) ;
#61155=CARTESIAN_POINT('Ctrl Pts',(-18.4492191754673,-31.0770755462028,
124.141874372406)) ;
#61156=CARTESIAN_POINT('Ctrl Pts',(-18.3865390046239,-31.2670897143815,
124.519239586884)) ;
#61157=CARTESIAN_POINT('Ctrl Pts',(-18.5910734554309,-31.0871006340186,
124.297744917431)) ;
#61158=CARTESIAN_POINT('Ctrl Pts',(-18.6602990640863,-31.2802735367488,
124.731576473087)) ;
#61159=CARTESIAN_POINT('Ctrl Pts',(-18.8100883440291,-31.1002844563859,
124.46762529973)) ;
#61160=CARTESIAN_POINT('Ctrl Pts',(-18.9862948594309,-31.2935956548947,
124.869711357312)) ;
#61161=CARTESIAN_POINT('Ctrl Pts',(-19.0709153826081,-31.1136065745318,
124.578138411476)) ;
#61162=CARTESIAN_POINT('Ctrl Pts',(-19.3347015527575,-31.3069748645223,
124.917347223178)) ;
#61163=CARTESIAN_POINT('Ctrl Pts',(-19.3495941692662,-31.1269857841594,
124.616238563571)) ;
#61164=CARTESIAN_POINT('Ctrl Pts',(-19.5930836021212,-31.3168131017665,
124.908057132309)) ;
#61165=CARTESIAN_POINT('Ctrl Pts',(-19.5563095018621,-31.1368240214036,
124.608810852484)) ;
#61166=CARTESIAN_POINT('Ctrl Pts',(-19.8519437779237,-31.3268860250252,
124.852876717695)) ;
#61167=CARTESIAN_POINT('Ctrl Pts',(-19.7633952063794,-31.1468969446624,
124.564668365869)) ;
#61168=CARTESIAN_POINT('Ctrl Pts',(-20.0920602272961,-31.3367426664803,
124.755670606679)) ;
#61169=CARTESIAN_POINT('Ctrl Pts',(-19.9554908730702,-31.1567535861175,
124.486904328256)) ;
#61170=CARTESIAN_POINT('Ctrl Pts',(-20.3148623984286,-31.3467280419864,
124.617067390045)) ;
#61171=CARTESIAN_POINT('Ctrl Pts',(-20.1337308377886,-31.1667389616235,
124.376027861451)) ;
#61172=CARTESIAN_POINT('Ctrl Pts',(-20.5745088879433,-31.3600120734468,
124.383813942974)) ;
#61173=CARTESIAN_POINT('Ctrl Pts',(-20.3414635227013,-31.180022993084,124.18940523939)) ;
#61174=CARTESIAN_POINT('Ctrl Pts',(-20.8154916492515,-31.3765308653172,
124.016626072661)) ;
#61175=CARTESIAN_POINT('Ctrl Pts',(-20.5342357532926,-31.1965417849543,
123.895695702942)) ;
#61176=CARTESIAN_POINT('Ctrl Pts',(-20.9173070492714,-31.3933165823238,
123.582394229583)) ;
#61177=CARTESIAN_POINT('Ctrl Pts',(-20.6157025962168,-31.2133275019609,
123.548246263072)) ;
#61178=CARTESIAN_POINT('Ctrl Pts',(-20.906515294897,-31.4064297308328,123.237879258058)) ;
#61179=CARTESIAN_POINT('Ctrl Pts',(-20.6070652302265,-31.2264406504699,
123.272686121829)) ;
#61180=CARTESIAN_POINT('Ctrl Pts',(-20.8536524123544,-31.416465279913,122.97954630541)) ;
#61181=CARTESIAN_POINT('Ctrl Pts',(-20.56477758318,-31.2364761995501,123.066008431127)) ;
#61182=CARTESIAN_POINT('Ctrl Pts',(-20.7561932613821,-31.4264813360924,
122.73500867879)) ;
#61183=CARTESIAN_POINT('Ctrl Pts',(-20.4868138633641,-31.2464922557295,
122.870382595949)) ;
#61184=CARTESIAN_POINT('Ctrl Pts',(-20.5747356330736,-31.4396593719584,
122.440107128178)) ;
#61185=CARTESIAN_POINT('Ctrl Pts',(-20.3416392942912,-31.2596702915955,
122.634448243853)) ;
#61186=CARTESIAN_POINT('Ctrl Pts',(-20.2550642401252,-31.4562612491455,
122.135837120638)) ;
#61187=CARTESIAN_POINT('Ctrl Pts',(-20.0859155602014,-31.2762721687826,
122.391041933051)) ;
#61188=CARTESIAN_POINT('Ctrl Pts',(-19.7659328719897,-31.4763243937614,
121.923514400748)) ;
#61189=CARTESIAN_POINT('Ctrl Pts',(-19.6946085896363,-31.2963353133985,
122.221176679855)) ;
#61190=CARTESIAN_POINT('Ctrl Pts',(-19.2406043647874,-31.4961252838451,
121.89094955361)) ;
#61191=CARTESIAN_POINT('Ctrl Pts',(-19.2743458623151,-31.3161362034822,
122.195122232715)) ;
#61192=CARTESIAN_POINT('Ctrl Pts',(-18.731841866447,-31.5160684091238,122.039356586224)) ;
#61193=CARTESIAN_POINT('Ctrl Pts',(-18.8673343450499,-31.3360793287609,
122.313844690629)) ;
#61194=CARTESIAN_POINT('Ctrl Pts',(-18.3053752399663,-31.5359664542434,
122.352092202936)) ;
#61195=CARTESIAN_POINT('Ctrl Pts',(-18.5261587181132,-31.3559773738805,
122.564031167843)) ;
#61196=CARTESIAN_POINT('Ctrl Pts',(-18.0102664114479,-31.5558522138702,
122.790649876929)) ;
#61197=CARTESIAN_POINT('Ctrl Pts',(-18.2900689875788,-31.3758631335073,
122.914876579139)) ;
#61198=CARTESIAN_POINT('Ctrl Pts',(-17.8822137797069,-31.57591738905,123.30830329177)) ;
#61199=CARTESIAN_POINT('Ctrl Pts',(-18.1876243873306,-31.3959283086872,
123.328998110787)) ;
#61200=CARTESIAN_POINT('Ctrl Pts',(-17.9380242803409,-31.5957440321528,
123.832388879101)) ;
#61201=CARTESIAN_POINT('Ctrl Pts',(-18.2322702877505,-31.41575495179,123.748268249303)) ;
#61202=CARTESIAN_POINT('Ctrl Pts',(-18.1688732800194,-31.6156527416012,
124.308361931682)) ;
#61203=CARTESIAN_POINT('Ctrl Pts',(-18.4169480416883,-31.4356636612383,
124.129048386258)) ;
#61204=CARTESIAN_POINT('Ctrl Pts',(-18.5492284834963,-31.635604578633,124.678079899656)) ;
#61205=CARTESIAN_POINT('Ctrl Pts',(-18.7212312265001,-31.4556154982701,
124.424824341634)) ;
#61206=CARTESIAN_POINT('Ctrl Pts',(-19.0344540490019,-31.6556130533361,
124.895564294001)) ;
#61207=CARTESIAN_POINT('Ctrl Pts',(-19.1094107625724,-31.4756239729733,
124.598813645085)) ;
#61208=CARTESIAN_POINT('Ctrl Pts',(-19.5593044714881,-31.6754145120976,
124.934638681105)) ;
#61209=CARTESIAN_POINT('Ctrl Pts',(-19.529293065133,-31.4954254317348,124.630074897987)) ;
#61210=CARTESIAN_POINT('Ctrl Pts',(-20.0703188207212,-31.6953714003336,
124.792477849082)) ;
#61211=CARTESIAN_POINT('Ctrl Pts',(-19.9381052599703,-31.5153823199707,
124.516346913691)) ;
#61212=CARTESIAN_POINT('Ctrl Pts',(-20.502014723073,-31.7153552377477,124.483083841928)) ;
#61213=CARTESIAN_POINT('Ctrl Pts',(-20.2834628020649,-31.5353661573848,
124.268832576871)) ;
#61214=CARTESIAN_POINT('Ctrl Pts',(-20.8005129693209,-31.7351636769686,
124.049324638335)) ;
#61215=CARTESIAN_POINT('Ctrl Pts',(-20.5222631468944,-31.5551745966057,
123.921823569577)) ;
#61216=CARTESIAN_POINT('Ctrl Pts',(-20.9347328465596,-31.7551493863488,
123.535538119656)) ;
#61217=CARTESIAN_POINT('Ctrl Pts',(-20.629639166781,-31.5751603059859,123.510794112745)) ;
#61218=CARTESIAN_POINT('Ctrl Pts',(-20.8859933951321,-31.7750189093641,
123.009476827453)) ;
#61219=CARTESIAN_POINT('Ctrl Pts',(-20.5906472054233,-31.5950298290012,
123.089943545706)) ;
#61220=CARTESIAN_POINT('Ctrl Pts',(-20.6589290212962,-31.7950396484813,
122.528458277174)) ;
#61221=CARTESIAN_POINT('Ctrl Pts',(-20.4089954572022,-31.6150505681184,
122.705129026127)) ;
#61222=CARTESIAN_POINT('Ctrl Pts',(-20.2856318116993,-31.8148437134583,
122.157092625036)) ;
#61223=CARTESIAN_POINT('Ctrl Pts',(-20.1103554752544,-31.6348546330954,
122.408035494353)) ;
#61224=CARTESIAN_POINT('Ctrl Pts',(-19.8021889396994,-31.834905677189,121.932500294498)) ;
#61225=CARTESIAN_POINT('Ctrl Pts',(-19.7236013288936,-31.6549165968261,
122.228362959859)) ;
#61226=CARTESIAN_POINT('Ctrl Pts',(-19.2768672597706,-31.8547388574775,
121.88738259078)) ;
#61227=CARTESIAN_POINT('Ctrl Pts',(-19.3033420853306,-31.6747497771146,
122.192269707988)) ;
#61228=CARTESIAN_POINT('Ctrl Pts',(-18.7652950498868,-31.8746580548036,
122.02333953517)) ;
#61229=CARTESIAN_POINT('Ctrl Pts',(-18.894083985732,-31.6946689744407,122.301037293139)) ;
#61230=CARTESIAN_POINT('Ctrl Pts',(-18.3305352276764,-31.8945960799169,
122.32632493169)) ;
#61231=CARTESIAN_POINT('Ctrl Pts',(-18.5462767220526,-31.714606999554,122.543427492195)) ;
#61232=CARTESIAN_POINT('Ctrl Pts',(-18.0255423060835,-31.914474125973,122.757789608184)) ;
#61233=CARTESIAN_POINT('Ctrl Pts',(-18.3022836422757,-31.7344850456101,
122.888601425754)) ;
#61234=CARTESIAN_POINT('Ctrl Pts',(-17.8853325731395,-31.934458860261,123.270040998411)) ;
#61235=CARTESIAN_POINT('Ctrl Pts',(-18.190118198044,-31.7544697798982,123.298403291928)) ;
#61236=CARTESIAN_POINT('Ctrl Pts',(-17.928106557493,-31.9543696769395,123.797659471924)) ;
#61237=CARTESIAN_POINT('Ctrl Pts',(-18.2243400264694,-31.7743805965766,
123.720498525304)) ;
#61238=CARTESIAN_POINT('Ctrl Pts',(-18.1495333782431,-31.9743686524582,
124.280744001209)) ;
#61239=CARTESIAN_POINT('Ctrl Pts',(-18.4014839037645,-31.7943795720954,
124.106965091444)) ;
#61240=CARTESIAN_POINT('Ctrl Pts',(-18.5185878611027,-31.9941735731034,
124.656228575391)) ;
#61241=CARTESIAN_POINT('Ctrl Pts',(-18.6967305737938,-31.8141844927406,
124.407351675959)) ;
#61242=CARTESIAN_POINT('Ctrl Pts',(-18.9973682960231,-32.0141575333947,
124.885894562646)) ;
#61243=CARTESIAN_POINT('Ctrl Pts',(-19.0797564164797,-31.8341684530318,
124.59108154804)) ;
#61244=CARTESIAN_POINT('Ctrl Pts',(-19.5234477413584,-32.0340437371186,
124.937928873616)) ;
#61245=CARTESIAN_POINT('Ctrl Pts',(-19.5006209678039,-31.8540546567557,
124.632705726637)) ;
#61246=CARTESIAN_POINT('Ctrl Pts',(-20.0373301585634,-32.0539929154418,
124.807521706156)) ;
#61247=CARTESIAN_POINT('Ctrl Pts',(-19.9117263038171,-31.8740038350789,
124.528376628622)) ;
#61248=CARTESIAN_POINT('Ctrl Pts',(-20.4747803851015,-32.0738947146813,
124.510171457429)) ;
#61249=CARTESIAN_POINT('Ctrl Pts',(-20.261684750146,-31.8939056343185,124.290492599356)) ;
#61250=CARTESIAN_POINT('Ctrl Pts',(-20.7850691732621,-32.0937733197337,
124.082510674293)) ;
#61251=CARTESIAN_POINT('Ctrl Pts',(-20.5099133229686,-31.9137842393708,
123.948363354658)) ;
#61252=CARTESIAN_POINT('Ctrl Pts',(-20.9316880819048,-32.1138056794594,
123.570639458984)) ;
#61253=CARTESIAN_POINT('Ctrl Pts',(-20.6272030682315,-31.9338165990965,
123.538857703905)) ;
#61254=CARTESIAN_POINT('Ctrl Pts',(-20.9004840928426,-32.1303874054155,
123.13101387148)) ;
#61255=CARTESIAN_POINT('Ctrl Pts',(-20.6022414356194,-31.9503983250526,
123.18718139994)) ;
#61256=CARTESIAN_POINT('Ctrl Pts',(-20.7882628387208,-32.1435815757134,
122.802971043195)) ;
#61257=CARTESIAN_POINT('Ctrl Pts',(-20.5124528334552,-31.9635924953505,
122.924720353763)) ;
#61258=CARTESIAN_POINT('Ctrl Pts',(-20.6197762199004,-32.1568937538066,
122.496386987847)) ;
#61259=CARTESIAN_POINT('Ctrl Pts',(-20.3776944292789,-31.9769046734437,
122.679499995801)) ;
#61260=CARTESIAN_POINT('Ctrl Pts',(-20.3152084467147,-32.1734599333999,
122.178383590941)) ;
#61261=CARTESIAN_POINT('Ctrl Pts',(-20.1339927311637,-31.9934708530371,
122.425047213569)) ;
#61262=CARTESIAN_POINT('Ctrl Pts',(-19.9191951145893,-32.1900881282601,
121.982318684066)) ;
#61263=CARTESIAN_POINT('Ctrl Pts',(-19.8172191413778,-32.0100990478972,
122.268225564694)) ;
#61264=CARTESIAN_POINT('Ctrl Pts',(-19.5767420543761,-32.2033767099699,
121.913670003331)) ;
#61265=CARTESIAN_POINT('Ctrl Pts',(-19.5432298830773,-32.023387629607,122.21329620248)) ;
#61266=CARTESIAN_POINT('Ctrl Pts',(-19.3148866166845,-32.2133449580735,
121.907334290486)) ;
#61267=CARTESIAN_POINT('Ctrl Pts',(-19.3337508380696,-32.0333558777106,
122.208232314246)) ;
#61268=CARTESIAN_POINT('Ctrl Pts',(-19.0572238635977,-32.2232597143296,
121.946033185605)) ;
#61269=CARTESIAN_POINT('Ctrl Pts',(-19.1276189170704,-32.0432706339667,
122.239193494291)) ;
#61270=CARTESIAN_POINT('Ctrl Pts',(-18.8076409322538,-32.2332728649808,
122.029433371392)) ;
#61271=CARTESIAN_POINT('Ctrl Pts',(-18.9279556714256,-32.0532837846179,
122.305913714308)) ;
#61272=CARTESIAN_POINT('Ctrl Pts',(-18.5765593857256,-32.2432855721828,
122.155251712162)) ;
#61273=CARTESIAN_POINT('Ctrl Pts',(-18.7430841787746,-32.0632964918199,
122.406578419691)) ;
#61274=CARTESIAN_POINT('Ctrl Pts',(-18.3044914721772,-32.2565048608741,
122.371339808174)) ;
#61275=CARTESIAN_POINT('Ctrl Pts',(-18.5254677230784,-32.0765157805112,
122.579410561966)) ;
#61276=CARTESIAN_POINT('Ctrl Pts',(-18.0412520385267,-32.2731235418722,
122.725865756024)) ;
#61277=CARTESIAN_POINT('Ctrl Pts',(-18.3148360322381,-32.0931344615093,
122.863088795251)) ;
#61278=CARTESIAN_POINT('Ctrl Pts',(-17.9146049570504,-32.2896884496456,
123.147620680735)) ;
#61279=CARTESIAN_POINT('Ctrl Pts',(-18.2135427847506,-32.1096993692827,
123.200444214174)) ;
#61280=CARTESIAN_POINT('Ctrl Pts',(-17.904363104532,-32.3030869212564,123.499558748901)) ;
#61281=CARTESIAN_POINT('Ctrl Pts',(-18.2053428096442,-32.1230978408936,
123.482028671522)) ;
#61282=CARTESIAN_POINT('Ctrl Pts',(-17.9415874189062,-32.3129281767434,
123.755505137551)) ;
#61283=CARTESIAN_POINT('Ctrl Pts',(-18.2351264004454,-32.1329390963805,
123.686778655729)) ;
#61284=CARTESIAN_POINT('Ctrl Pts',(-18.0233154440135,-32.3229144923316,
124.004839610842)) ;
#61285=CARTESIAN_POINT('Ctrl Pts',(-18.3005104402209,-32.1429254119687,
123.886247298971)) ;
#61286=CARTESIAN_POINT('Ctrl Pts',(-18.1464078763225,-32.332851099918,124.2351797327)) ;
#61287=CARTESIAN_POINT('Ctrl Pts',(-18.3989864852805,-32.1528620195551,
124.070517791497)) ;
#61288=CARTESIAN_POINT('Ctrl Pts',(-18.3095220075479,-32.3429009672863,
124.44285330986)) ;
#61289=CARTESIAN_POINT('Ctrl Pts',(-18.5294795023595,-32.1629118869234,
124.23665535116)) ;
#61290=CARTESIAN_POINT('Ctrl Pts',(-18.5022200305885,-32.3527514619611,
124.615730119443)) ;
#61291=CARTESIAN_POINT('Ctrl Pts',(-18.6836393679515,-32.1727623815982,
124.374955019593)) ;
#61292=CARTESIAN_POINT('Ctrl Pts',(-18.7243070867326,-32.3627232623556,
124.754758703636)) ;
#61293=CARTESIAN_POINT('Ctrl Pts',(-18.8613101252405,-32.1827341819927,
124.486175940165)) ;
#61294=CARTESIAN_POINT('Ctrl Pts',(-18.9678327868554,-32.3727192293814,
124.853354582418)) ;
#61295=CARTESIAN_POINT('Ctrl Pts',(-19.0561314683988,-32.1927301490186,
124.565050536217)) ;
#61296=CARTESIAN_POINT('Ctrl Pts',(-19.225851948996,-32.3827566887626,124.90802999486)) ;
#61297=CARTESIAN_POINT('Ctrl Pts',(-19.2625472401696,-32.2027676083997,
124.608788652274)) ;
#61298=CARTESIAN_POINT('Ctrl Pts',(-19.4843048557896,-32.3925973896634,
124.917387851395)) ;
#61299=CARTESIAN_POINT('Ctrl Pts',(-19.4693094439586,-32.2126083093005,
124.616272690437)) ;
#61300=CARTESIAN_POINT('Ctrl Pts',(-19.7458762676805,-32.4026454109307,
124.881367125265)) ;
#61301=CARTESIAN_POINT('Ctrl Pts',(-19.6785662481788,-32.2226563305678,
124.587453906341)) ;
#61302=CARTESIAN_POINT('Ctrl Pts',(-19.9945882738061,-32.4125928040134,
124.800883482138)) ;
#61303=CARTESIAN_POINT('Ctrl Pts',(-19.8775350535338,-32.2326037236505,
124.523064890071)) ;
#61304=CARTESIAN_POINT('Ctrl Pts',(-20.2250646863654,-32.4225029500598,
124.679595400653)) ;
#61305=CARTESIAN_POINT('Ctrl Pts',(-20.0619149780218,-32.2425138696969,
124.426032565424)) ;
#61306=CARTESIAN_POINT('Ctrl Pts',(-20.4338556734805,-32.4325618639094,
124.517526668951)) ;
#61307=CARTESIAN_POINT('Ctrl Pts',(-20.2289464252875,-32.2525727835465,
124.296375807091)) ;
#61308=CARTESIAN_POINT('Ctrl Pts',(-20.6077963923764,-32.4424026341987,
124.326112710777)) ;
#61309=CARTESIAN_POINT('Ctrl Pts',(-20.3680971502017,-32.2624135538358,
124.143243405943)) ;
#61310=CARTESIAN_POINT('Ctrl Pts',(-20.749200205045,-32.4524655037773,124.102692225348)) ;
#61311=CARTESIAN_POINT('Ctrl Pts',(-20.4812183762259,-32.2724764234145,
123.964505819681)) ;
#61312=CARTESIAN_POINT('Ctrl Pts',(-20.8478072363101,-32.4623598269078,
123.862073047581)) ;
#61313=CARTESIAN_POINT('Ctrl Pts',(-20.5601018691605,-32.2823707465449,
123.772009890152)) ;
#61314=CARTESIAN_POINT('Ctrl Pts',(-20.9040808602051,-32.4723016340023,
123.606978235594)) ;
#61315=CARTESIAN_POINT('Ctrl Pts',(-20.6051186298419,-32.2923125536394,
123.567933786065)) ;
#61316=CARTESIAN_POINT('Ctrl Pts',(-20.9153764258059,-32.4823041449576,
123.34432986247)) ;
#61317=CARTESIAN_POINT('Ctrl Pts',(-20.6141529513669,-32.3023150645948,
123.357815062894)) ;
#61318=CARTESIAN_POINT('Ctrl Pts',(-20.8803820948059,-32.492338865776,123.082976331004)) ;
#61319=CARTESIAN_POINT('Ctrl Pts',(-20.5861553344511,-32.3123497854131,
123.148732512367)) ;
#61320=CARTESIAN_POINT('Ctrl Pts',(-20.8024460213099,-32.5021840432817,
122.836257068615)) ;
#61321=CARTESIAN_POINT('Ctrl Pts',(-20.5238045816804,-32.3221949629189,
122.951358176035)) ;
#61322=CARTESIAN_POINT('Ctrl Pts',(-20.6816420858177,-32.5121688036828,
122.603373026614)) ;
#61323=CARTESIAN_POINT('Ctrl Pts',(-20.427159646758,-32.3321797233199,122.765052018463)) ;
#61324=CARTESIAN_POINT('Ctrl Pts',(-20.523022050828,-32.5221077099992,122.395822102444)) ;
#61325=CARTESIAN_POINT('Ctrl Pts',(-20.3002621303212,-32.3421186296363,
122.59901272905)) ;
#61326=CARTESIAN_POINT('Ctrl Pts',(-20.3287624729339,-32.5321499376349,
122.217239391601)) ;
#61327=CARTESIAN_POINT('Ctrl Pts',(-20.1448530337361,-32.3521608572721,
122.456148061873)) ;
#61328=CARTESIAN_POINT('Ctrl Pts',(-20.1099755420916,-32.5420351492193,
122.077133850417)) ;
#61329=CARTESIAN_POINT('Ctrl Pts',(-19.9698227394801,-32.3620460688564,
122.344065585937)) ;
#61330=CARTESIAN_POINT('Ctrl Pts',(-19.8676198087422,-32.5520340794212,
121.975708802829)) ;
#61331=CARTESIAN_POINT('Ctrl Pts',(-19.7759374551782,-32.3720449990584,
122.262927442215)) ;
#61332=CARTESIAN_POINT('Ctrl Pts',(-19.6133877400118,-32.5619515023317,
121.918164610241)) ;
#61333=CARTESIAN_POINT('Ctrl Pts',(-19.5725517025332,-32.3819624219688,
122.216894103057)) ;
#61334=CARTESIAN_POINT('Ctrl Pts',(-19.3496802081964,-32.5719994344104,
121.905528177764)) ;
#61335=CARTESIAN_POINT('Ctrl Pts',(-19.3615855024817,-32.3920103540475,
122.206786949623)) ;
#61336=CARTESIAN_POINT('Ctrl Pts',(-19.0921154350541,-32.5818768102198,
121.938063647421)) ;
#61337=CARTESIAN_POINT('Ctrl Pts',(-19.1555344414447,-32.4018877298569,
122.232817207828)) ;
#61338=CARTESIAN_POINT('Ctrl Pts',(-18.8397271603765,-32.5919307033877,
122.016043063102)) ;
#61339=CARTESIAN_POINT('Ctrl Pts',(-18.9536242958656,-32.4119416230248,
122.295202630568)) ;
#61340=CARTESIAN_POINT('Ctrl Pts',(-18.6083164557563,-32.601824326641,122.134675324029)) ;
#61341=CARTESIAN_POINT('Ctrl Pts',(-18.7684970311458,-32.4218352462781,
122.390109938702)) ;
#61342=CARTESIAN_POINT('Ctrl Pts',(-18.3975309341739,-32.611886920264,122.29427674415)) ;
#61343=CARTESIAN_POINT('Ctrl Pts',(-18.5998696580958,-32.4318978399011,
122.517792698231)) ;
#61344=CARTESIAN_POINT('Ctrl Pts',(-18.221443696393,-32.6217294942531,122.483777412127)) ;
#61345=CARTESIAN_POINT('Ctrl Pts',(-18.4590017343272,-32.4417404138902,
122.669394019431)) ;
#61346=CARTESIAN_POINT('Ctrl Pts',(-18.0783294582589,-32.631720251136,122.703848805901)) ;
#61347=CARTESIAN_POINT('Ctrl Pts',(-18.3445119383423,-32.4517311707731,
122.845452004202)) ;
#61348=CARTESIAN_POINT('Ctrl Pts',(-17.9762694762357,-32.6416483128939,
122.943971098664)) ;
#61349=CARTESIAN_POINT('Ctrl Pts',(-18.2628657760219,-32.4616592325311,
123.037550188827)) ;
#61350=CARTESIAN_POINT('Ctrl Pts',(-17.9166533727178,-32.6516362887831,
123.19959535074)) ;
#61351=CARTESIAN_POINT('Ctrl Pts',(-18.2151746225017,-32.4716472084202,
123.242049843833)) ;
#61352=CARTESIAN_POINT('Ctrl Pts',(-17.9027006002209,-32.6616719531395,
123.462944824449)) ;
#61353=CARTESIAN_POINT('Ctrl Pts',(-18.2040142137418,-32.4816828727767,
123.452729587914)) ;
#61354=CARTESIAN_POINT('Ctrl Pts',(-17.9337120201421,-32.6715278915592,
123.720099296854)) ;
#61355=CARTESIAN_POINT('Ctrl Pts',(-18.2288249953322,-32.4915388111963,
123.658452229222)) ;
#61356=CARTESIAN_POINT('Ctrl Pts',(-18.0095431011939,-32.6815233829561,
123.971557376319)) ;
#61357=CARTESIAN_POINT('Ctrl Pts',(-18.2894914284038,-32.5015343025932,
123.859618092693)) ;
#61358=CARTESIAN_POINT('Ctrl Pts',(-18.1268171255641,-32.6914331879096,
124.20409067232)) ;
#61359=CARTESIAN_POINT('Ctrl Pts',(-18.3833118888715,-32.5114441075467,
124.045643510793)) ;
#61360=CARTESIAN_POINT('Ctrl Pts',(-18.2839493311189,-32.7014454101763,
124.41513539528)) ;
#61361=CARTESIAN_POINT('Ctrl Pts',(-18.509018896985,-32.5214563298134,124.214478314619)) ;
#61362=CARTESIAN_POINT('Ctrl Pts',(-18.4759885042275,-32.7114732908691,
124.595595889866)) ;
#61363=CARTESIAN_POINT('Ctrl Pts',(-18.6626514215253,-32.5314842105063,
124.358845523371)) ;
#61364=CARTESIAN_POINT('Ctrl Pts',(-18.6924294796709,-32.7213296868517,
124.737869480862)) ;
#61365=CARTESIAN_POINT('Ctrl Pts',(-18.8358044087005,-32.5413406064889,
124.472662626393)) ;
#61366=CARTESIAN_POINT('Ctrl Pts',(-18.9341360919731,-32.7313544840317,
124.842659911602)) ;
#61367=CARTESIAN_POINT('Ctrl Pts',(-19.0291703120113,-32.5513654036688,
124.556493611938)) ;
#61368=CARTESIAN_POINT('Ctrl Pts',(-19.1906775296738,-32.7413854140155,
124.903298738838)) ;
#61369=CARTESIAN_POINT('Ctrl Pts',(-19.2344038900453,-32.5613963336526,
124.605003114696)) ;
#61370=CARTESIAN_POINT('Ctrl Pts',(-19.4489157332629,-32.7512300165242,
124.918654695543)) ;
#61371=CARTESIAN_POINT('Ctrl Pts',(-19.4409936483921,-32.5712409361613,
124.617286306339)) ;
#61372=CARTESIAN_POINT('Ctrl Pts',(-19.7098139114528,-32.7612208677483,
124.889204775659)) ;
#61373=CARTESIAN_POINT('Ctrl Pts',(-19.6497118803502,-32.5812317873854,
124.593725014445)) ;
#61374=CARTESIAN_POINT('Ctrl Pts',(-19.962644010255,-32.7712587007595,124.813987935703)) ;
#61375=CARTESIAN_POINT('Ctrl Pts',(-19.8519756339455,-32.5912696203966,
124.533550073541)) ;
#61376=CARTESIAN_POINT('Ctrl Pts',(-20.1942400544308,-32.7811030892249,
124.698686780465)) ;
#61377=CARTESIAN_POINT('Ctrl Pts',(-20.037251000993,-32.6011140088621,124.441308307128)) ;
#61378=CARTESIAN_POINT('Ctrl Pts',(-20.4055373690367,-32.7910878935945,
124.543175419173)) ;
#61379=CARTESIAN_POINT('Ctrl Pts',(-20.2062879201296,-32.6110988132316,
124.316898288086)) ;
#61380=CARTESIAN_POINT('Ctrl Pts',(-20.5859328054878,-32.8010274130773,
124.354225945988)) ;
#61381=CARTESIAN_POINT('Ctrl Pts',(-20.3506030458168,-32.6210383327145,
124.16573814407)) ;
#61382=CARTESIAN_POINT('Ctrl Pts',(-20.7321570744506,-32.8110671440787,
124.134645385839)) ;
#61383=CARTESIAN_POINT('Ctrl Pts',(-20.4675814518196,-32.6310780637158,
123.990072882451)) ;
#61384=CARTESIAN_POINT('Ctrl Pts',(-20.8365696228075,-32.820955272325,123.896678841576)) ;
#61385=CARTESIAN_POINT('Ctrl Pts',(-20.551110037506,-32.6409661919621,123.79969981623)) ;
#61386=CARTESIAN_POINT('Ctrl Pts',(-20.8991776003898,-32.8309449975335,
123.641744550588)) ;
#61387=CARTESIAN_POINT('Ctrl Pts',(-20.6011952561969,-32.6509559171706,
123.595752273945)) ;
#61388=CARTESIAN_POINT('Ctrl Pts',(-20.9163259243604,-32.840902762235,123.380631029218)) ;
#61389=CARTESIAN_POINT('Ctrl Pts',(-20.6149126952404,-32.6609136818721,
123.386861725222)) ;
#61390=CARTESIAN_POINT('Ctrl Pts',(-20.8886398161754,-32.850805103647,123.121875613575)) ;
#61391=CARTESIAN_POINT('Ctrl Pts',(-20.5927628294816,-32.6708160232841,
123.179858200967)) ;
#61392=CARTESIAN_POINT('Ctrl Pts',(-20.8153934381563,-32.8608492993534,
122.868304834852)) ;
#61393=CARTESIAN_POINT('Ctrl Pts',(-20.5341646599949,-32.6808602189905,
122.977001723796)) ;
#61394=CARTESIAN_POINT('Ctrl Pts',(-20.7008271858602,-32.8707567001127,
122.634494488512)) ;
#61395=CARTESIAN_POINT('Ctrl Pts',(-20.4425109923345,-32.6907676197498,
122.789954502378)) ;
#61396=CARTESIAN_POINT('Ctrl Pts',(-20.5461862319884,-32.880767299987,122.421673048565)) ;
#61397=CARTESIAN_POINT('Ctrl Pts',(-20.3187974795829,-32.7007782196241,
122.619697941561)) ;
#61398=CARTESIAN_POINT('Ctrl Pts',(-20.356212767659,-32.8907975958992,122.238939688487)) ;
#61399=CARTESIAN_POINT('Ctrl Pts',(-20.1668179033373,-32.7108085155363,
122.473511971535)) ;
#61400=CARTESIAN_POINT('Ctrl Pts',(-20.1414444851523,-32.9006523755489,
122.094253937587)) ;
#61401=CARTESIAN_POINT('Ctrl Pts',(-19.9950035629509,-32.720663295186,122.35776475964)) ;
#61402=CARTESIAN_POINT('Ctrl Pts',(-19.9026572208542,-32.9106097037664,
121.987223818498)) ;
#61403=CARTESIAN_POINT('Ctrl Pts',(-19.8039737675108,-32.7306206234035,
122.272141549309)) ;
#61404=CARTESIAN_POINT('Ctrl Pts',(-19.6467435512146,-32.9206487366733,
121.923215339529)) ;
#61405=CARTESIAN_POINT('Ctrl Pts',(-19.5992424816828,-32.7406596563104,
122.220935620064)) ;
#61406=CARTESIAN_POINT('Ctrl Pts',(-19.3879265897767,-32.9305218485626,
121.90443588022)) ;
#61407=CARTESIAN_POINT('Ctrl Pts',(-19.3921897535148,-32.7505327681997,
122.205912911945)) ;
#61408=CARTESIAN_POINT('Ctrl Pts',(-19.1246518188088,-32.9405951335897,
121.93148651026)) ;
#61409=CARTESIAN_POINT('Ctrl Pts',(-19.18156967997,-32.7606060532268,122.227554264233)) ;
#61410=CARTESIAN_POINT('Ctrl Pts',(-18.8762664627294,-32.9504154533265,
122.001727342518)) ;
#61411=CARTESIAN_POINT('Ctrl Pts',(-18.9828627923026,-32.7704263729636,
122.283747296942)) ;
#61412=CARTESIAN_POINT('Ctrl Pts',(-18.6377418415184,-32.9604941187049,
122.116709479966)) ;
#61413=CARTESIAN_POINT('Ctrl Pts',(-18.7920430490926,-32.780505038342,122.375733780278)) ;
#61414=CARTESIAN_POINT('Ctrl Pts',(-18.4274927507125,-32.9703457091887,
122.267875972372)) ;
#61415=CARTESIAN_POINT('Ctrl Pts',(-18.623845014994,-32.7903566288258,122.496666887985)) ;
#61416=CARTESIAN_POINT('Ctrl Pts',(-18.2425317134073,-32.9804188595076,
122.457180219424)) ;
#61417=CARTESIAN_POINT('Ctrl Pts',(-18.4758763682574,-32.8004297791447,
122.648110955056)) ;
#61418=CARTESIAN_POINT('Ctrl Pts',(-18.0966577530102,-32.9902612394826,
122.670798846665)) ;
#61419=CARTESIAN_POINT('Ctrl Pts',(-18.3591783416525,-32.8102721591198,
122.819005262211)) ;
#61420=CARTESIAN_POINT('Ctrl Pts',(-17.987823954365,-33.0002422157257,122.90942173405)) ;
#61421=CARTESIAN_POINT('Ctrl Pts',(-18.272111762497,-32.8202531353628,123.009903514452)) ;
#61422=CARTESIAN_POINT('Ctrl Pts',(-17.9222646672302,-33.010258544081,123.164359426917)) ;
#61423=CARTESIAN_POINT('Ctrl Pts',(-18.2196648233517,-32.8302694637181,
123.213853781775)) ;
#61424=CARTESIAN_POINT('Ctrl Pts',(-17.9018796513175,-33.0201563410721,
123.423653833823)) ;
#61425=CARTESIAN_POINT('Ctrl Pts',(-18.2033572916693,-32.8401672607093,
123.421288551752)) ;
#61426=CARTESIAN_POINT('Ctrl Pts',(-17.9266701886612,-33.0301688978042,
123.685622214838)) ;
#61427=CARTESIAN_POINT('Ctrl Pts',(-18.2231900289858,-32.8501798174413,
123.630863208958)) ;
#61428=CARTESIAN_POINT('Ctrl Pts',(-17.9972994489001,-33.0402009326507,
123.939603199681)) ;
#61429=CARTESIAN_POINT('Ctrl Pts',(-18.2796939144183,-32.8602118522878,
123.834047973384)) ;
#61430=CARTESIAN_POINT('Ctrl Pts',(-18.1082062116321,-33.0500403334661,
124.173202825564)) ;
#61431=CARTESIAN_POINT('Ctrl Pts',(-18.3684190950603,-32.8700512531033,
124.020926481006)) ;
#61432=CARTESIAN_POINT('Ctrl Pts',(-18.2612411137015,-33.0601061191177,
124.388920029464)) ;
#61433=CARTESIAN_POINT('Ctrl Pts',(-18.4908474005065,-32.8801170387548,
124.193500344908)) ;
#61434=CARTESIAN_POINT('Ctrl Pts',(-18.4462566311347,-33.0699965742323,
124.571505176903)) ;
#61435=CARTESIAN_POINT('Ctrl Pts',(-18.6388594192354,-32.8900074938694,
124.339567673731)) ;
#61436=CARTESIAN_POINT('Ctrl Pts',(-18.6620084681289,-33.0799886928681,
124.721150558715)) ;
#61437=CARTESIAN_POINT('Ctrl Pts',(-18.8114608287963,-32.8999996125052,
124.459283763965)) ;
#61438=CARTESIAN_POINT('Ctrl Pts',(-18.8998759883332,-33.0899515196311,
124.830519144683)) ;
#61439=CARTESIAN_POINT('Ctrl Pts',(-19.0017545994413,-32.9099624392683,
124.546778293489)) ;
#61440=CARTESIAN_POINT('Ctrl Pts',(-19.1514920073142,-33.099855802904,124.897179406725)) ;
#61441=CARTESIAN_POINT('Ctrl Pts',(-19.2030466974503,-32.9198667225411,
124.600106275238)) ;
#61442=CARTESIAN_POINT('Ctrl Pts',(-19.4149143853563,-33.1099162368511,
124.919252762117)) ;
#61443=CARTESIAN_POINT('Ctrl Pts',(-19.4137848897019,-32.9299271564882,
124.617764888164)) ;
#61444=CARTESIAN_POINT('Ctrl Pts',(-19.6725102686655,-33.1197567895243,
124.896100987741)) ;
#61445=CARTESIAN_POINT('Ctrl Pts',(-19.6198604236689,-32.9397677091614,
124.599243563997)) ;
#61446=CARTESIAN_POINT('Ctrl Pts',(-19.9278232585217,-33.12981900947,124.827395120368)) ;
#61447=CARTESIAN_POINT('Ctrl Pts',(-19.824111120568,-32.9498299291071,124.544278865711)) ;
#61448=CARTESIAN_POINT('Ctrl Pts',(-20.1633223010035,-33.1397161487486,
124.716975844118)) ;
#61449=CARTESIAN_POINT('Ctrl Pts',(-20.0125096303553,-32.9597270683857,
124.455943788509)) ;
#61450=CARTESIAN_POINT('Ctrl Pts',(-20.377287539303,-33.1496473408836,124.567550900585)) ;
#61451=CARTESIAN_POINT('Ctrl Pts',(-20.1836814780393,-32.9696582605208,
124.336404350332)) ;
#61452=CARTESIAN_POINT('Ctrl Pts',(-20.5639122193513,-33.1596894955287,
124.380978396875)) ;
#61453=CARTESIAN_POINT('Ctrl Pts',(-20.3329814474512,-32.9797004151658,
124.187146334296)) ;
#61454=CARTESIAN_POINT('Ctrl Pts',(-20.7131557897439,-33.169576256548,124.168279265478)) ;
#61455=CARTESIAN_POINT('Ctrl Pts',(-20.4523759687857,-32.9895871761851,
124.016987866727)) ;
#61456=CARTESIAN_POINT('Ctrl Pts',(-20.8247334245669,-33.1795755582652,
123.930412036511)) ;
#61457=CARTESIAN_POINT('Ctrl Pts',(-20.5416382872207,-32.9995864779024,
123.826694322003)) ;
#61458=CARTESIAN_POINT('Ctrl Pts',(-20.8929652906654,-33.189496356432,123.678753341723)) ;
#61459=CARTESIAN_POINT('Ctrl Pts',(-20.5962239379931,-33.0095072760691,
123.625368054938)) ;
#61460=CARTESIAN_POINT('Ctrl Pts',(-20.9167545830113,-33.1995304100287,
123.416173818305)) ;
#61461=CARTESIAN_POINT('Ctrl Pts',(-20.6152557226043,-33.0195413296658,
123.415304354511)) ;
#61462=CARTESIAN_POINT('Ctrl Pts',(-20.894986412613,-33.2094535275951,123.156274431571)) ;
#61463=CARTESIAN_POINT('Ctrl Pts',(-20.5978416138883,-33.0294644472322,
123.207385423938)) ;
#61464=CARTESIAN_POINT('Ctrl Pts',(-20.8274911534907,-33.2195096510942,
122.900802570426)) ;
#61465=CARTESIAN_POINT('Ctrl Pts',(-20.5438456966334,-33.0395205707314,
123.003007611585)) ;
#61466=CARTESIAN_POINT('Ctrl Pts',(-20.7190711618733,-33.2293550927491,
122.665874666496)) ;
#61467=CARTESIAN_POINT('Ctrl Pts',(-20.4571105336298,-33.0493660123862,
122.815066148446)) ;
#61468=CARTESIAN_POINT('Ctrl Pts',(-20.5704789953411,-33.2393173938732,
122.450351068691)) ;
#61469=CARTESIAN_POINT('Ctrl Pts',(-20.3382375063864,-33.0593283135103,
122.64264722283)) ;
#61470=CARTESIAN_POINT('Ctrl Pts',(-20.3852299651721,-33.2493458731483,
122.262882911342)) ;
#61471=CARTESIAN_POINT('Ctrl Pts',(-20.1900385985285,-33.0693567927855,
122.492672276396)) ;
#61472=CARTESIAN_POINT('Ctrl Pts',(-20.172852355375,-33.259256226658,122.112168058019)) ;
#61473=CARTESIAN_POINT('Ctrl Pts',(-20.020137396195,-33.0792671462951,122.37210035673)) ;
#61474=CARTESIAN_POINT('Ctrl Pts',(-19.9372239609423,-33.2691910988352,
121.999716737927)) ;
#61475=CARTESIAN_POINT('Ctrl Pts',(-19.8316354638329,-33.0892020184723,
122.282138886147)) ;
#61476=CARTESIAN_POINT('Ctrl Pts',(-19.6829095119979,-33.2792322364209,
121.92938034057)) ;
#61477=CARTESIAN_POINT('Ctrl Pts',(-19.6281839338197,-33.099243156058,122.225869101484)) ;
#61478=CARTESIAN_POINT('Ctrl Pts',(-19.4242673412634,-33.2891193856355,
121.904471017884)) ;
#61479=CARTESIAN_POINT('Ctrl Pts',(-19.4212710912674,-33.1091303052726,
122.205941031457)) ;
#61480=CARTESIAN_POINT('Ctrl Pts',(-19.1624743734912,-33.2991116203865,
121.924625120071)) ;
#61481=CARTESIAN_POINT('Ctrl Pts',(-19.2118368178498,-33.1191225400237,
122.222063502103)) ;
#61482=CARTESIAN_POINT('Ctrl Pts',(-18.9092537722081,-33.3090603259495,
121.989726729914)) ;
#61483=CARTESIAN_POINT('Ctrl Pts',(-19.009260561855,-33.1290712455866,122.274143925144)) ;
#61484=CARTESIAN_POINT('Ctrl Pts',(-18.6713579683458,-33.3189963943732,
122.097309682469)) ;
#61485=CARTESIAN_POINT('Ctrl Pts',(-18.8189440248541,-33.1390073140103,
122.360209282463)) ;
#61486=CARTESIAN_POINT('Ctrl Pts',(-18.454473086345,-33.328982078589,122.245077547478)) ;
#61487=CARTESIAN_POINT('Ctrl Pts',(-18.6454357542757,-33.1489929982261,
122.478422680742)) ;
#61488=CARTESIAN_POINT('Ctrl Pts',(-18.2658309062383,-33.3390225051576,
122.429534786724)) ;
#61489=CARTESIAN_POINT('Ctrl Pts',(-18.494521322166,-33.1590334247948,122.625987962609)) ;
#61490=CARTESIAN_POINT('Ctrl Pts',(-18.1148023371037,-33.3488616186214,
122.639409270607)) ;
#61491=CARTESIAN_POINT('Ctrl Pts',(-18.3736983361703,-33.1688725382585,
122.793886113984)) ;
#61492=CARTESIAN_POINT('Ctrl Pts',(-17.9997997485683,-33.3588913527972,
122.876570796198)) ;
#61493=CARTESIAN_POINT('Ctrl Pts',(-18.2816952521632,-33.1789022724343,
122.983614938204)) ;
#61494=CARTESIAN_POINT('Ctrl Pts',(-17.9284390777351,-33.3689134523031,
123.130086625313)) ;
#61495=CARTESIAN_POINT('Ctrl Pts',(-18.2246058215283,-33.1889243719402,
123.186427373328)) ;
#61496=CARTESIAN_POINT('Ctrl Pts',(-17.9019339658882,-33.3787818921965,
123.388080969439)) ;
#61497=CARTESIAN_POINT('Ctrl Pts',(-18.2034007565293,-33.1987928118337,
123.3928218386)) ;
#61498=CARTESIAN_POINT('Ctrl Pts',(-17.9210110195692,-33.3888507568821,
123.651967424913)) ;
#61499=CARTESIAN_POINT('Ctrl Pts',(-18.2186613497739,-33.2088616765193,
123.603931380545)) ;
#61500=CARTESIAN_POINT('Ctrl Pts',(-17.9841657910811,-33.3986934299808,
123.902803793652)) ;
#61501=CARTESIAN_POINT('Ctrl Pts',(-18.2691838719648,-33.2187043496179,
123.804599731666)) ;
#61502=CARTESIAN_POINT('Ctrl Pts',(-18.0903011027806,-33.4086540641432,
124.142069897794)) ;
#61503=CARTESIAN_POINT('Ctrl Pts',(-18.3540908116242,-33.2286649837803,
123.996012840234)) ;
#61504=CARTESIAN_POINT('Ctrl Pts',(-18.237930321801,-33.4186919798213,124.360664605472)) ;
#61505=CARTESIAN_POINT('Ctrl Pts',(-18.4721932743968,-33.2387028994585,
124.170889351092)) ;
#61506=CARTESIAN_POINT('Ctrl Pts',(-18.4179673638906,-33.4285662546808,
124.547577121921)) ;
#61507=CARTESIAN_POINT('Ctrl Pts',(-18.6162214263879,-33.2485771743179,
124.320419667571)) ;
#61508=CARTESIAN_POINT('Ctrl Pts',(-18.6318294560732,-33.4386360050559,
124.703362669157)) ;
#61509=CARTESIAN_POINT('Ctrl Pts',(-18.7873105748439,-33.258646924693,124.445049300282)) ;
#61510=CARTESIAN_POINT('Ctrl Pts',(-18.8639015606415,-33.4484693004304,
124.817067545813)) ;
#61511=CARTESIAN_POINT('Ctrl Pts',(-18.9729667662246,-33.2684802200675,
124.536013921811)) ;
#61512=CARTESIAN_POINT('Ctrl Pts',(-19.116928618104,-33.45849959791,124.890896842844)) ;
#61513=CARTESIAN_POINT('Ctrl Pts',(-19.1753880699453,-33.2785105175472,
124.595078779856)) ;
#61514=CARTESIAN_POINT('Ctrl Pts',(-19.3790808832761,-33.4685316843515,
124.918905806779)) ;
#61515=CARTESIAN_POINT('Ctrl Pts',(-19.3851098109455,-33.2885426039886,
124.617487248845)) ;
#61516=CARTESIAN_POINT('Ctrl Pts',(-19.6367776217658,-33.4783596128404,
124.901904690569)) ;
#61517=CARTESIAN_POINT('Ctrl Pts',(-19.5912662774906,-33.2983705324775,
124.603887836004)) ;
#61518=CARTESIAN_POINT('Ctrl Pts',(-19.8920737335198,-33.4883556539512,
124.840047977085)) ;
#61519=CARTESIAN_POINT('Ctrl Pts',(-19.7955034173776,-33.3083665735883,
124.554404008552)) ;
#61520=CARTESIAN_POINT('Ctrl Pts',(-20.133272867296,-33.4983814660524,124.734019156174)) ;
#61521=CARTESIAN_POINT('Ctrl Pts',(-19.9884633393389,-33.3183923856895,
124.469582272309)) ;
#61522=CARTESIAN_POINT('Ctrl Pts',(-20.3495536621585,-33.5082687009472,
124.590024685913)) ;
#61523=CARTESIAN_POINT('Ctrl Pts',(-20.1614882643308,-33.3282796205843,
124.35438833044)) ;
#61524=CARTESIAN_POINT('Ctrl Pts',(-20.5395336848334,-33.5182455671582,
124.409369154937)) ;
#61525=CARTESIAN_POINT('Ctrl Pts',(-20.3134732405899,-33.3382564867954,
124.209865210489)) ;
#61526=CARTESIAN_POINT('Ctrl Pts',(-20.6955808166486,-33.52823851103,124.198113299847)) ;
#61527=CARTESIAN_POINT('Ctrl Pts',(-20.4383121677193,-33.3482494306672,
124.040861581618)) ;
#61528=CARTESIAN_POINT('Ctrl Pts',(-20.8127780411408,-33.5382764337014,
123.961814580438)) ;
#61529=CARTESIAN_POINT('Ctrl Pts',(-20.5320713666861,-33.3582873533385,
123.851823229752)) ;
#61530=CARTESIAN_POINT('Ctrl Pts',(-20.8861474399005,-33.5481248979631,
123.713603887042)) ;
#61531=CARTESIAN_POINT('Ctrl Pts',(-20.5907682089124,-33.3681358176002,
123.653255920477)) ;
#61532=CARTESIAN_POINT('Ctrl Pts',(-20.9161879631416,-33.5581167647071,
123.452790730188)) ;
#61533=CARTESIAN_POINT('Ctrl Pts',(-20.6148023084948,-33.3781276843442,
123.444605723383)) ;
#61534=CARTESIAN_POINT('Ctrl Pts',(-20.9007460375611,-33.5680344967483,
123.192586764787)) ;
#61535=CARTESIAN_POINT('Ctrl Pts',(-20.6024505212769,-33.3880454163854,
123.236442905293)) ;
#61536=CARTESIAN_POINT('Ctrl Pts',(-20.8397673980302,-33.5780626816436,
122.936230922789)) ;
#61537=CARTESIAN_POINT('Ctrl Pts',(-20.5536692986984,-33.3980736012807,
123.031357801439)) ;
#61538=CARTESIAN_POINT('Ctrl Pts',(-20.7367825952507,-33.5879478396924,
122.697737712798)) ;
#61539=CARTESIAN_POINT('Ctrl Pts',(-20.4712833051947,-33.4079587593295,
122.840563075759)) ;
#61540=CARTESIAN_POINT('Ctrl Pts',(-20.5929810834346,-33.5979372002341,
122.478112272451)) ;
#61541=CARTESIAN_POINT('Ctrl Pts',(-20.3562437228865,-33.4179481198712,
122.664861808084)) ;
#61542=CARTESIAN_POINT('Ctrl Pts',(-20.4118953447041,-33.6079783571685,
122.28618599598)) ;
#61543=CARTESIAN_POINT('Ctrl Pts',(-20.211376372118,-33.4279892768056,122.511319516605)) ;
#61544=CARTESIAN_POINT('Ctrl Pts',(-20.2048905331621,-33.6178109406236,
122.131549195167)) ;
#61545=CARTESIAN_POINT('Ctrl Pts',(-20.0457742371618,-33.4378218602607,
122.387609057188)) ;
#61546=CARTESIAN_POINT('Ctrl Pts',(-19.9707238077735,-33.6278051605856,
122.012626278824)) ;
#61547=CARTESIAN_POINT('Ctrl Pts',(-19.8584418276612,-33.4478160802227,
122.292469026325)) ;
#61548=CARTESIAN_POINT('Ctrl Pts',(-19.718447243707,-33.6378332623729,121.936421881646)) ;
#61549=CARTESIAN_POINT('Ctrl Pts',(-19.6566211029712,-33.45784418201,122.231503711827)) ;
#61550=CARTESIAN_POINT('Ctrl Pts',(-19.4606834132683,-33.647713206996,121.905273090565)) ;
#61551=CARTESIAN_POINT('Ctrl Pts',(-19.450410798269,-33.4677241266331,122.206582828695)) ;
#61552=CARTESIAN_POINT('Ctrl Pts',(-19.1985284829144,-33.657703533553,121.919105510909)) ;
#61553=CARTESIAN_POINT('Ctrl Pts',(-19.2406868632452,-33.4777144531901,
122.217646778312)) ;
#61554=CARTESIAN_POINT('Ctrl Pts',(-18.9440006247662,-33.6676444652073,
121.977957452937)) ;
#61555=CARTESIAN_POINT('Ctrl Pts',(-19.037064402286,-33.4876553848444,122.264726340451)) ;
#61556=CARTESIAN_POINT('Ctrl Pts',(-18.7022824096691,-33.6776315837102,
122.080244334494)) ;
#61557=CARTESIAN_POINT('Ctrl Pts',(-18.8436891442797,-33.4976425033473,
122.346553933699)) ;
#61558=CARTESIAN_POINT('Ctrl Pts',(-18.481234424871,-33.6876649166074,122.223936502288)) ;
#61559=CARTESIAN_POINT('Ctrl Pts',(-18.6668496639801,-33.5076758362445,
122.461506021483)) ;
#61560=CARTESIAN_POINT('Ctrl Pts',(-18.2913247035046,-33.6975310210521,
122.400490262853)) ;
#61561=CARTESIAN_POINT('Ctrl Pts',(-18.514920867317,-33.5175419406893,122.602747196414)) ;
#61562=CARTESIAN_POINT('Ctrl Pts',(-18.1317726324715,-33.7075971349325,
122.611443969021)) ;
#61563=CARTESIAN_POINT('Ctrl Pts',(-18.3872775066212,-33.5276080545696,
122.771509020567)) ;
#61564=CARTESIAN_POINT('Ctrl Pts',(-18.0137527035476,-33.7174531467009,
122.84201884311)) ;
#61565=CARTESIAN_POINT('Ctrl Pts',(-18.2928599689319,-33.537464066338,122.955967544122)) ;
#61566=CARTESIAN_POINT('Ctrl Pts',(-17.9357556600526,-33.7274478503322,
123.0928133731)) ;
#61567=CARTESIAN_POINT('Ctrl Pts',(-18.2304603236921,-33.5474587699693,
123.156602459403)) ;
#61568=CARTESIAN_POINT('Ctrl Pts',(-17.9029259941155,-33.7374791860571,
123.354378720209)) ;
#61569=CARTESIAN_POINT('Ctrl Pts',(-18.2041945366287,-33.5574901056942,
123.365854477829)) ;
#61570=CARTESIAN_POINT('Ctrl Pts',(-17.9153845549704,-33.7473457112607,
123.613370405302)) ;
#61571=CARTESIAN_POINT('Ctrl Pts',(-18.2141592554439,-33.5673566308979,
123.573047516046)) ;
#61572=CARTESIAN_POINT('Ctrl Pts',(-17.9729030336068,-33.7573331393065,
123.869417371802)) ;
#61573=CARTESIAN_POINT('Ctrl Pts',(-18.2601719160976,-33.5773440589437,
123.777885465428)) ;
#61574=CARTESIAN_POINT('Ctrl Pts',(-18.0734724275908,-33.767278068993,124.110676065872)) ;
#61575=CARTESIAN_POINT('Ctrl Pts',(-18.3406253653803,-33.5872889886301,
123.970893079309)) ;
#61576=CARTESIAN_POINT('Ctrl Pts',(-18.2159131529908,-33.7773229871015,
124.332886434286)) ;
#61577=CARTESIAN_POINT('Ctrl Pts',(-18.4545761429792,-33.5973339067386,
124.14866254757)) ;
#61578=CARTESIAN_POINT('Ctrl Pts',(-18.3913760380472,-33.7871849567154,
124.523645046325)) ;
#61579=CARTESIAN_POINT('Ctrl Pts',(-18.5949446249841,-33.6071958763525,
124.301270653746)) ;
#61580=CARTESIAN_POINT('Ctrl Pts',(-18.5996633149286,-33.7971770247366,
124.683493416082)) ;
#61581=CARTESIAN_POINT('Ctrl Pts',(-18.7615730437336,-33.6171879443737,
124.429151053145)) ;
#61582=CARTESIAN_POINT('Ctrl Pts',(-18.8311757134717,-33.8071079501112,
124.803984732102)) ;
#61583=CARTESIAN_POINT('Ctrl Pts',(-18.9467817879391,-33.6271188697483,
124.525545974419)) ;
#61584=CARTESIAN_POINT('Ctrl Pts',(-19.0804210325099,-33.8170585783346,
124.883010582507)) ;
#61585=CARTESIAN_POINT('Ctrl Pts',(-19.1461772488705,-33.6370694979717,
124.588768739218)) ;
#61586=CARTESIAN_POINT('Ctrl Pts',(-19.3409209971923,-33.8270588173937,
124.917887617961)) ;
#61587=CARTESIAN_POINT('Ctrl Pts',(-19.3545768691479,-33.6470697370308,
124.616672564472)) ;
#61588=CARTESIAN_POINT('Ctrl Pts',(-19.6042058083092,-33.8370872727629,
124.906594290871)) ;
#61589=CARTESIAN_POINT('Ctrl Pts',(-19.5652047628629,-33.6570981924,124.607640132786)) ;
#61590=CARTESIAN_POINT('Ctrl Pts',(-19.8574687091397,-33.8469533073462,
124.851055548244)) ;
#61591=CARTESIAN_POINT('Ctrl Pts',(-19.767815408138,-33.6669642269833,124.563211299104)) ;
#61592=CARTESIAN_POINT('Ctrl Pts',(-20.1004399415462,-33.8569456290936,
124.751536396934)) ;
#61593=CARTESIAN_POINT('Ctrl Pts',(-19.9621930061691,-33.6769565487307,
124.483598313414)) ;
#61594=CARTESIAN_POINT('Ctrl Pts',(-20.3211678423663,-33.8668779187706,
124.612195664073)) ;
#61595=CARTESIAN_POINT('Ctrl Pts',(-20.1387771157398,-33.6868888384077,
124.372126818241)) ;
#61596=CARTESIAN_POINT('Ctrl Pts',(-20.5158504184365,-33.8768795637414,
124.435627299884)) ;
#61597=CARTESIAN_POINT('Ctrl Pts',(-20.2945221175348,-33.6968904833785,
124.230877050889)) ;
#61598=CARTESIAN_POINT('Ctrl Pts',(-20.730134344151,-33.8901921971574,124.159073181011)) ;
#61599=CARTESIAN_POINT('Ctrl Pts',(-20.4659641625927,-33.7102031167945,
124.009619650892)) ;
#61600=CARTESIAN_POINT('Ctrl Pts',(-20.8667466130496,-33.903423946539,123.835025634149)) ;
#61601=CARTESIAN_POINT('Ctrl Pts',(-20.5752544036822,-33.7234348661761,
123.750361646045)) ;
#61602=CARTESIAN_POINT('Ctrl Pts',(-20.9147529608524,-33.916747211356,123.488209575824)) ;
#61603=CARTESIAN_POINT('Ctrl Pts',(-20.613652637114,-33.7367581309931,123.47295053957)) ;
#61604=CARTESIAN_POINT('Ctrl Pts',(-20.9055507233818,-33.9266229175737,
123.228839180932)) ;
#61605=CARTESIAN_POINT('Ctrl Pts',(-20.6062950688991,-33.7466338372108,
123.265445862905)) ;
#61606=CARTESIAN_POINT('Ctrl Pts',(-20.8511725357474,-33.9366125086737,
122.972045792766)) ;
#61607=CARTESIAN_POINT('Ctrl Pts',(-20.5627941970681,-33.7566234283109,
123.060012946144)) ;
#61608=CARTESIAN_POINT('Ctrl Pts',(-20.7537843023225,-33.9465396051291,
122.72999873487)) ;
#61609=CARTESIAN_POINT('Ctrl Pts',(-20.4848858225803,-33.7665505247663,
122.866373858558)) ;
#61610=CARTESIAN_POINT('Ctrl Pts',(-20.6145413556846,-33.9565647536337,
122.506380398598)) ;
#61611=CARTESIAN_POINT('Ctrl Pts',(-20.3734933698443,-33.7765756732709,
122.687478231554)) ;
#61612=CARTESIAN_POINT('Ctrl Pts',(-20.4409482369391,-33.9664604077804,
122.312726536766)) ;
#61613=CARTESIAN_POINT('Ctrl Pts',(-20.2346204969347,-33.7864713274175,
122.532553555553)) ;
#61614=CARTESIAN_POINT('Ctrl Pts',(-20.234405044289,-33.9764639421586,122.150141791109)) ;
#61615=CARTESIAN_POINT('Ctrl Pts',(-20.0693873459231,-33.7964748617957,
122.402484058768)) ;
#61616=CARTESIAN_POINT('Ctrl Pts',(-20.0031251936759,-33.9864490805987,
122.026110363717)) ;
#61617=CARTESIAN_POINT('Ctrl Pts',(-19.8843645383385,-33.8064600002358,
122.303256977614)) ;
#61618=CARTESIAN_POINT('Ctrl Pts',(-19.7525232072214,-33.996485005194,121.943972168262)) ;
#61619=CARTESIAN_POINT('Ctrl Pts',(-19.6838837485256,-33.8164959248312,
122.237544337022)) ;
#61620=CARTESIAN_POINT('Ctrl Pts',(-19.4963012262117,-34.0063362806217,
121.906976170342)) ;
#61621=CARTESIAN_POINT('Ctrl Pts',(-19.4789062849549,-33.8263472002588,
122.207945321101)) ;
#61622=CARTESIAN_POINT('Ctrl Pts',(-19.2338112579742,-34.0163285417831,
121.914396519971)) ;
#61623=CARTESIAN_POINT('Ctrl Pts',(-19.2689142641197,-33.8363394614202,
122.213879435451)) ;
#61624=CARTESIAN_POINT('Ctrl Pts',(-18.9755284714672,-34.0263684258007,
121.968182550343)) ;
#61625=CARTESIAN_POINT('Ctrl Pts',(-19.0622876995497,-33.8463793454378,
122.256906084154)) ;
#61626=CARTESIAN_POINT('Ctrl Pts',(-18.7352293588995,-34.0362032003031,
122.063406918151)) ;
#61627=CARTESIAN_POINT('Ctrl Pts',(-18.8700473962123,-33.8562141199402,
122.333083630202)) ;
#61628=CARTESIAN_POINT('Ctrl Pts',(-18.5097194264488,-34.0462795813234,
122.202115742426)) ;
#61629=CARTESIAN_POINT('Ctrl Pts',(-18.6896381792612,-33.8662905009605,
122.444048990142)) ;
#61630=CARTESIAN_POINT('Ctrl Pts',(-18.3161370097982,-34.056125854474,122.37385617066)) ;
#61631=CARTESIAN_POINT('Ctrl Pts',(-18.534771813737,-33.8761367741112,122.581439034222)) ;
#61632=CARTESIAN_POINT('Ctrl Pts',(-18.0973641720853,-34.0694903757593,
122.648596301571)) ;
#61633=CARTESIAN_POINT('Ctrl Pts',(-18.3597451619224,-33.8895012953964,
122.801233992996)) ;
#61634=CARTESIAN_POINT('Ctrl Pts',(-17.9574233667404,-34.0826966201937,
122.97048578706)) ;
#61635=CARTESIAN_POINT('Ctrl Pts',(-18.2477846414627,-33.9027075398308,
123.058779978968)) ;
#61636=CARTESIAN_POINT('Ctrl Pts',(-17.9048166903989,-34.0959615748709,
123.315069758424)) ;
#61637=CARTESIAN_POINT('Ctrl Pts',(-18.2057090036201,-33.9159724945081,
123.334400438449)) ;
#61638=CARTESIAN_POINT('Ctrl Pts',(-17.9110068532374,-34.1059938554226,
123.57864144408)) ;
#61639=CARTESIAN_POINT('Ctrl Pts',(-18.2106566732483,-33.9260047750597,
123.545267055076)) ;
#61640=CARTESIAN_POINT('Ctrl Pts',(-17.9622064695877,-34.1159025889405,
123.833943902984)) ;
#61641=CARTESIAN_POINT('Ctrl Pts',(-18.2516149524503,-33.9359135085776,
123.749507096678)) ;
#61642=CARTESIAN_POINT('Ctrl Pts',(-18.0566040745096,-34.125840139808,124.077443630493)) ;
#61643=CARTESIAN_POINT('Ctrl Pts',(-18.3271318142154,-33.9458510594451,
123.944309004323)) ;
#61644=CARTESIAN_POINT('Ctrl Pts',(-18.1932746081133,-34.1358699874019,
124.302786499422)) ;
#61645=CARTESIAN_POINT('Ctrl Pts',(-18.4364641738599,-33.9558809070391,
124.124582034141)) ;
#61646=CARTESIAN_POINT('Ctrl Pts',(-18.4222258929034,-34.1491051273224,
124.564718290271)) ;
#61647=CARTESIAN_POINT('Ctrl Pts',(-18.6196353445962,-33.9691160469595,
124.334139139703)) ;
#61648=CARTESIAN_POINT('Ctrl Pts',(-18.7900532730984,-34.1657735916935,
124.811391878838)) ;
#61649=CARTESIAN_POINT('Ctrl Pts',(-18.9138856664441,-33.9857845113307,
124.531468849858)) ;
#61650=CARTESIAN_POINT('Ctrl Pts',(-19.3028100031656,-34.1856446035674,
124.938674734945)) ;
#61651=CARTESIAN_POINT('Ctrl Pts',(-19.3240782602018,-34.0056555232046,
124.633306456755)) ;
#61652=CARTESIAN_POINT('Ctrl Pts',(-19.7442781237528,-34.2023516879504,
124.8920557054)) ;
#61653=CARTESIAN_POINT('Ctrl Pts',(-19.6773043553831,-34.0223626075875,
124.596000463399)) ;
#61654=CARTESIAN_POINT('Ctrl Pts',(-20.0675644892654,-34.215528969261,124.767792583565)) ;
#61655=CARTESIAN_POINT('Ctrl Pts',(-19.935888328374,-34.0355398888981,124.496604100906)) ;
#61656=CARTESIAN_POINT('Ctrl Pts',(-20.3669683527793,-34.2287964297751,
124.589169379259)) ;
#61657=CARTESIAN_POINT('Ctrl Pts',(-20.1754272032707,-34.0488073494122,
124.353698951168)) ;
#61658=CARTESIAN_POINT('Ctrl Pts',(-20.6747925423891,-34.2454103204623,
124.272577564532)) ;
#61659=CARTESIAN_POINT('Ctrl Pts',(-20.4216796479605,-34.0654212400994,
124.100434565729)) ;
#61660=CARTESIAN_POINT('Ctrl Pts',(-20.8925501699724,-34.2653591198897,
123.789095141607)) ;
#61661=CARTESIAN_POINT('Ctrl Pts',(-20.5958914715679,-34.0853700395268,
123.713647108598)) ;
#61662=CARTESIAN_POINT('Ctrl Pts',(-20.9320934628038,-34.2852802314206,
123.26117694893)) ;
#61663=CARTESIAN_POINT('Ctrl Pts',(-20.627528243359,-34.1052911510577,123.29131282389)) ;
#61664=CARTESIAN_POINT('Ctrl Pts',(-20.7905220573564,-34.3051466795934,
122.752407298956)) ;
#61665=CARTESIAN_POINT('Ctrl Pts',(-20.5142733449368,-34.1251575992306,
122.884295234101)) ;
#61666=CARTESIAN_POINT('Ctrl Pts',(-20.4811847888518,-34.3251730262106,
122.319328242786)) ;
#61667=CARTESIAN_POINT('Ctrl Pts',(-20.2668055516656,-34.1451839458477,
122.537830873447)) ;
#61668=CARTESIAN_POINT('Ctrl Pts',(-20.0460469289995,-34.3450350706001,
122.020279911706)) ;
#61669=CARTESIAN_POINT('Ctrl Pts',(-19.9186955596424,-34.1650459902372,
122.298589641338)) ;
#61670=CARTESIAN_POINT('Ctrl Pts',(-19.5332082975654,-34.3649803732812,
121.886348768634)) ;
#61671=CARTESIAN_POINT('Ctrl Pts',(-19.5084245595147,-34.1849912929184,
122.191442818576)) ;
#61672=CARTESIAN_POINT('Ctrl Pts',(-19.0066946739163,-34.3848756803401,
121.93543015809)) ;
#61673=CARTESIAN_POINT('Ctrl Pts',(-19.0872124491375,-34.2048865999772,
122.230706348824)) ;
#61674=CARTESIAN_POINT('Ctrl Pts',(-18.528179666335,-34.4047689505077,122.160351280735)) ;
#61675=CARTESIAN_POINT('Ctrl Pts',(-18.7043988887934,-34.2247798701449,
122.410642726589)) ;
#61676=CARTESIAN_POINT('Ctrl Pts',(-18.1538942485171,-34.4247345431882,
122.53647446393)) ;
#61677=CARTESIAN_POINT('Ctrl Pts',(-18.404969560696,-34.2447454628253,122.711540862601)) ;
#61678=CARTESIAN_POINT('Ctrl Pts',(-17.9310744457826,-34.444609866873,123.015467619857)) ;
#61679=CARTESIAN_POINT('Ctrl Pts',(-18.2267125107953,-34.2646207865101,
123.094736487549)) ;
#61680=CARTESIAN_POINT('Ctrl Pts',(-17.8843177630335,-34.464584929448,123.544333074597)) ;
#61681=CARTESIAN_POINT('Ctrl Pts',(-18.1893069457108,-34.2845958490851,
123.517829108664)) ;
#61682=CARTESIAN_POINT('Ctrl Pts',(-18.0214586110986,-34.4845373390791,
124.056594429955)) ;
#61683=CARTESIAN_POINT('Ctrl Pts',(-18.2990194229785,-34.3045482587162,
123.927638867659)) ;
#61684=CARTESIAN_POINT('Ctrl Pts',(-18.3225640751946,-34.5043733933152,
124.489356119812)) ;
#61685=CARTESIAN_POINT('Ctrl Pts',(-18.5399052793811,-34.3243843129523,
124.27384976748)) ;
#61686=CARTESIAN_POINT('Ctrl Pts',(-18.7560161142767,-34.5243513047327,
124.796045846229)) ;
#61687=CARTESIAN_POINT('Ctrl Pts',(-18.8866675828867,-34.3443622243698,
124.519201026929)) ;
#61688=CARTESIAN_POINT('Ctrl Pts',(-19.2667030759239,-34.5442693542362,
124.935377333597)) ;
#61689=CARTESIAN_POINT('Ctrl Pts',(-19.2952182947917,-34.3642802738733,
124.630665776378)) ;
#61690=CARTESIAN_POINT('Ctrl Pts',(-19.7932159078448,-34.5641374980043,
124.893556756045)) ;
#61691=CARTESIAN_POINT('Ctrl Pts',(-19.7164298223103,-34.3841484176414,
124.597207716313)) ;
#61692=CARTESIAN_POINT('Ctrl Pts',(-20.2777146690572,-34.5841883545916,
124.671918199537)) ;
#61693=CARTESIAN_POINT('Ctrl Pts',(-20.1040278270987,-34.4041992742287,
124.419895848041)) ;
#61694=CARTESIAN_POINT('Ctrl Pts',(-20.6529658815064,-34.6039687910475,
124.303496686845)) ;
#61695=CARTESIAN_POINT('Ctrl Pts',(-20.4042291464414,-34.4239797106846,
124.125155886527)) ;
#61696=CARTESIAN_POINT('Ctrl Pts',(-20.8834863290637,-34.6239988467253,
123.823760909331)) ;
#61697=CARTESIAN_POINT('Ctrl Pts',(-20.5886433844177,-34.4440097663624,
123.74136659525)) ;
#61698=CARTESIAN_POINT('Ctrl Pts',(-20.9351889705778,-34.6438799519001,
123.297798988631)) ;
#61699=CARTESIAN_POINT('Ctrl Pts',(-20.6300035954088,-34.4638908715372,
123.32059580445)) ;
#61700=CARTESIAN_POINT('Ctrl Pts',(-20.805790334357,-34.6637604142679,122.785553366895)) ;
#61701=CARTESIAN_POINT('Ctrl Pts',(-20.5264818601808,-34.483771333905,122.910799001557)) ;
#61702=CARTESIAN_POINT('Ctrl Pts',(-20.5076352220214,-34.6837455614122,
122.345932910046)) ;
#61703=CARTESIAN_POINT('Ctrl Pts',(-20.2879554585398,-34.5037564810494,
122.559104093687)) ;
#61704=CARTESIAN_POINT('Ctrl Pts',(-20.0793236955457,-34.7036361399486,
122.036027427117)) ;
#61705=CARTESIAN_POINT('Ctrl Pts',(-19.9453039222835,-34.5236470595857,
122.311181522728)) ;
#61706=CARTESIAN_POINT('Ctrl Pts',(-19.5711560383436,-34.723530159823,121.889965636303)) ;
#61707=CARTESIAN_POINT('Ctrl Pts',(-19.5387682446119,-34.5435410794601,
122.1943349732)) ;
#61708=CARTESIAN_POINT('Ctrl Pts',(-19.0429893283783,-34.7434516045494,
121.925987779891)) ;
#61709=CARTESIAN_POINT('Ctrl Pts',(-19.1162346135711,-34.5634625241865,
122.223156059284)) ;
#61710=CARTESIAN_POINT('Ctrl Pts',(-18.5587933443279,-34.7633497426048,
122.139065599401)) ;
#61711=CARTESIAN_POINT('Ctrl Pts',(-18.7288788359676,-34.583360662242,122.393621850554)) ;
#61712=CARTESIAN_POINT('Ctrl Pts',(-18.1739396124289,-34.7834204978209,
122.508326536902)) ;
#61713=CARTESIAN_POINT('Ctrl Pts',(-18.4209985757421,-34.603431417458,122.689032837873)) ;
#61714=CARTESIAN_POINT('Ctrl Pts',(-17.9412291317738,-34.8032060478722,
122.980030562384)) ;
#61715=CARTESIAN_POINT('Ctrl Pts',(-18.234833032526,-34.6232169675093,123.066398644646)) ;
#61716=CARTESIAN_POINT('Ctrl Pts',(-17.8816194222905,-34.8231891227495,
123.507694573191)) ;
#61717=CARTESIAN_POINT('Ctrl Pts',(-18.1871490553495,-34.6432000423866,
123.488530272471)) ;
#61718=CARTESIAN_POINT('Ctrl Pts',(-18.0060182323476,-34.8430982053954,
124.022021160858)) ;
#61719=CARTESIAN_POINT('Ctrl Pts',(-18.2866725880628,-34.6631091250326,
123.899991117196)) ;
#61720=CARTESIAN_POINT('Ctrl Pts',(-18.2964865246401,-34.8629567645182,
124.462795926968)) ;
#61721=CARTESIAN_POINT('Ctrl Pts',(-18.5190486895846,-34.6829676841553,
124.252608470384)) ;
#61722=CARTESIAN_POINT('Ctrl Pts',(-18.7241036774144,-34.8830002083569,
124.780319588221)) ;
#61723=CARTESIAN_POINT('Ctrl Pts',(-18.8611532239642,-34.703011127994,124.506625843281)) ;
#61724=CARTESIAN_POINT('Ctrl Pts',(-19.1443314362236,-34.8995002730861,
124.906184977463)) ;
#61725=CARTESIAN_POINT('Ctrl Pts',(-19.1973104768277,-34.7195111927232,
124.607308957452)) ;
#61726=CARTESIAN_POINT('Ctrl Pts',(-19.4959856145689,-34.912890012935,124.916808895163)) ;
#61727=CARTESIAN_POINT('Ctrl Pts',(-19.4786571226114,-34.7329009325721,
124.615810467763)) ;
#61728=CARTESIAN_POINT('Ctrl Pts',(-19.7523697501484,-34.9227469141434,
124.879642738554)) ;
#61729=CARTESIAN_POINT('Ctrl Pts',(-19.6837596469558,-34.7427578337805,
124.586074466439)) ;
#61730=CARTESIAN_POINT('Ctrl Pts',(-20.0018598351797,-34.9327384399899,
124.79795143579)) ;
#61731=CARTESIAN_POINT('Ctrl Pts',(-19.8833526563097,-34.752749359627,124.520719090591)) ;
#61732=CARTESIAN_POINT('Ctrl Pts',(-20.2319445660988,-34.9426631204409,
124.675054574799)) ;
#61733=CARTESIAN_POINT('Ctrl Pts',(-20.0674176841992,-34.762674040078,124.4224015819)) ;
#61734=CARTESIAN_POINT('Ctrl Pts',(-20.438971803788,-34.9526737104853,124.512809926613)) ;
#61735=CARTESIAN_POINT('Ctrl Pts',(-20.2330436587693,-34.7726846301224,
124.292596602303)) ;
#61736=CARTESIAN_POINT('Ctrl Pts',(-20.6720998991134,-34.9659329711889,
124.253723717875)) ;
#61737=CARTESIAN_POINT('Ctrl Pts',(-20.4195165683706,-34.7859438908261,
124.085363349355)) ;
#61738=CARTESIAN_POINT('Ctrl Pts',(-20.8329350805989,-34.9792840463392,
123.937545082256)) ;
#61739=CARTESIAN_POINT('Ctrl Pts',(-20.5482036204118,-34.7992949659763,
123.832398938157)) ;
#61740=CARTESIAN_POINT('Ctrl Pts',(-20.9051329385635,-34.992490355574,123.598017654249)) ;
#61741=CARTESIAN_POINT('Ctrl Pts',(-20.605960739995,-34.8125012752111,123.56076258238)) ;
#61742=CARTESIAN_POINT('Ctrl Pts',(-20.914842890768,-35.0024771891643,123.335798885094)) ;
#61743=CARTESIAN_POINT('Ctrl Pts',(-20.6137261079857,-34.8224881088014,
123.350990280824)) ;
#61744=CARTESIAN_POINT('Ctrl Pts',(-20.8791149640092,-35.0124299166604,
123.076657694403)) ;
#61745=CARTESIAN_POINT('Ctrl Pts',(-20.5851416344258,-34.8324408362975,
123.143676914264)) ;
#61746=CARTESIAN_POINT('Ctrl Pts',(-20.7979778136165,-35.022478013502,122.825409407708)) ;
#61747=CARTESIAN_POINT('Ctrl Pts',(-20.5202297765397,-34.8424889331391,
122.942679247368)) ;
#61748=CARTESIAN_POINT('Ctrl Pts',(-20.6772333062096,-35.0323194703738,
122.596674503416)) ;
#61749=CARTESIAN_POINT('Ctrl Pts',(-20.4236321706692,-34.8523303900109,
122.759692291335)) ;
#61750=CARTESIAN_POINT('Ctrl Pts',(-20.5167579761239,-35.0423057372873,
122.389083764502)) ;
#61751=CARTESIAN_POINT('Ctrl Pts',(-20.2952501539374,-34.8623166569244,
122.593621150654)) ;
#61752=CARTESIAN_POINT('Ctrl Pts',(-20.3236651757576,-35.0522423381877,
122.213233449278)) ;
#61753=CARTESIAN_POINT('Ctrl Pts',(-20.1407744379203,-34.8722532578248,
122.452942601343)) ;
#61754=CARTESIAN_POINT('Ctrl Pts',(-20.1004431975683,-35.0622922809748,
122.072138574706)) ;
#61755=CARTESIAN_POINT('Ctrl Pts',(-19.9621956872849,-34.8823032006119,
122.340068638975)) ;
#61756=CARTESIAN_POINT('Ctrl Pts',(-19.861002389051,-35.0721424806605,121.973740369883)) ;
#61757=CARTESIAN_POINT('Ctrl Pts',(-19.7706422695711,-34.8921534002976,
122.261352199334)) ;
#61758=CARTESIAN_POINT('Ctrl Pts',(-19.6051578614204,-35.0821153855926,
121.917057183094)) ;
#61759=CARTESIAN_POINT('Ctrl Pts',(-19.5659662526582,-34.9021263052297,
122.216007866642)) ;
#61760=CARTESIAN_POINT('Ctrl Pts',(-19.3426236375317,-35.0921137600722,
121.905710783946)) ;
#61761=CARTESIAN_POINT('Ctrl Pts',(-19.3559388367088,-34.9121246797094,
122.206932993469)) ;
#61762=CARTESIAN_POINT('Ctrl Pts',(-19.0816040718578,-35.1021339339422,
121.940379135869)) ;
#61763=CARTESIAN_POINT('Ctrl Pts',(-19.1471235237251,-34.9221448535794,
122.234669903381)) ;
#61764=CARTESIAN_POINT('Ctrl Pts',(-18.8334713868321,-35.1120349778842,
122.018687487834)) ;
#61765=CARTESIAN_POINT('Ctrl Pts',(-18.9486181859309,-34.9320458975213,
122.297318684873)) ;
#61766=CARTESIAN_POINT('Ctrl Pts',(-18.600476033389,-35.1220237816085,122.139585076272)) ;
#61767=CARTESIAN_POINT('Ctrl Pts',(-18.7622230038763,-34.9420347012456,
122.394038699726)) ;
#61768=CARTESIAN_POINT('Ctrl Pts',(-18.3926205883172,-35.1319892484403,
122.298870811014)) ;
#61769=CARTESIAN_POINT('Ctrl Pts',(-18.5959400898762,-34.9520001680775,
122.521469007001)) ;
#61770=CARTESIAN_POINT('Ctrl Pts',(-18.2161904041538,-35.1418928107133,
122.490230413735)) ;
#61771=CARTESIAN_POINT('Ctrl Pts',(-18.4547977047164,-34.9619037303504,
122.674558035766)) ;
#61772=CARTESIAN_POINT('Ctrl Pts',(-18.0736527312663,-35.1519534885913,
122.712860272288)) ;
#61773=CARTESIAN_POINT('Ctrl Pts',(-18.3407694238614,-34.9719644082284,
122.852663144503)) ;
#61774=CARTESIAN_POINT('Ctrl Pts',(-17.9738293172813,-35.1617937865408,
122.951450001417)) ;
#61775=CARTESIAN_POINT('Ctrl Pts',(-18.2609128496764,-34.9818047061779,
123.043535471726)) ;
#61776=CARTESIAN_POINT('Ctrl Pts',(-17.9153656043643,-35.1718567814502,
123.209316008984)) ;
#61777=CARTESIAN_POINT('Ctrl Pts',(-18.2141439991331,-34.9918677010873,
123.249828796046)) ;
#61778=CARTESIAN_POINT('Ctrl Pts',(-17.9029906881241,-35.1817510755973,
123.469061216247)) ;
#61779=CARTESIAN_POINT('Ctrl Pts',(-18.2042462718512,-35.0017619952345,
123.457624801608)) ;
#61780=CARTESIAN_POINT('Ctrl Pts',(-17.9353509724904,-35.1916928732942,
123.728277083016)) ;
#61781=CARTESIAN_POINT('Ctrl Pts',(-18.230136599556,-35.0117037929313,123.664997019035)) ;
#61782=CARTESIAN_POINT('Ctrl Pts',(-18.0126256104855,-35.2016954508233,
123.979555436209)) ;
#61783=CARTESIAN_POINT('Ctrl Pts',(-18.2919583264141,-35.0217063704604,
123.866019011557)) ;
#61784=CARTESIAN_POINT('Ctrl Pts',(-18.1330779756745,-35.2117299147444,
124.214117512253)) ;
#61785=CARTESIAN_POINT('Ctrl Pts',(-18.3883221539504,-35.0317408343815,
124.053667693136)) ;
#61786=CARTESIAN_POINT('Ctrl Pts',(-18.2891276130123,-35.2215760532655,
124.420521008391)) ;
#61787=CARTESIAN_POINT('Ctrl Pts',(-18.5131632916011,-35.0415869729026,
124.218788844697)) ;
#61788=CARTESIAN_POINT('Ctrl Pts',(-18.4808245709193,-35.2315572265025,
124.59951775017)) ;
#61789=CARTESIAN_POINT('Ctrl Pts',(-18.6665221721677,-35.0515681461396,
124.361984625144)) ;
#61790=CARTESIAN_POINT('Ctrl Pts',(-18.7001113066703,-35.2415095204597,
124.742060651056)) ;
#61791=CARTESIAN_POINT('Ctrl Pts',(-18.8419525117809,-35.0615204400968,
124.476017085114)) ;
#61792=CARTESIAN_POINT('Ctrl Pts',(-18.9418196622479,-35.2515083155943,
124.845159871712)) ;
#61793=CARTESIAN_POINT('Ctrl Pts',(-19.0353199196314,-35.0715192352314,
124.558494551332)) ;
#61794=CARTESIAN_POINT('Ctrl Pts',(-19.1988694220206,-35.2615474238551,
124.904462676824)) ;
#61795=CARTESIAN_POINT('Ctrl Pts',(-19.2409602470283,-35.0815583434922,
124.605934759269)) ;
#61796=CARTESIAN_POINT('Ctrl Pts',(-19.4566932433114,-35.2713723652943,
124.918494235156)) ;
#61797=CARTESIAN_POINT('Ctrl Pts',(-19.4472187973089,-35.0913832849314,
124.617157941595)) ;
#61798=CARTESIAN_POINT('Ctrl Pts',(-19.7190507496054,-35.2814270523687,
124.887257605285)) ;
#61799=CARTESIAN_POINT('Ctrl Pts',(-19.6571046535086,-35.1014379720058,
124.592166657345)) ;
#61800=CARTESIAN_POINT('Ctrl Pts',(-19.9690783925131,-35.2913698573088,
124.811356103697)) ;
#61801=CARTESIAN_POINT('Ctrl Pts',(-19.8571259192075,-35.1113807769459,
124.531443580824)) ;
#61802=CARTESIAN_POINT('Ctrl Pts',(-20.2015729912878,-35.3012736433053,
124.694371844272)) ;
#61803=CARTESIAN_POINT('Ctrl Pts',(-20.0431203471688,-35.1212845629424,
124.437854636998)) ;
#61804=CARTESIAN_POINT('Ctrl Pts',(-20.4131178490129,-35.3113204598701,
124.536438012286)) ;
#61805=CARTESIAN_POINT('Ctrl Pts',(-20.2123551289518,-35.1313313795072,
124.311505953245)) ;
#61806=CARTESIAN_POINT('Ctrl Pts',(-20.5915179796175,-35.3212159793488,
124.347180770753)) ;
#61807=CARTESIAN_POINT('Ctrl Pts',(-20.3550735141645,-35.1412268989859,
124.160099180785)) ;
#61808=CARTESIAN_POINT('Ctrl Pts',(-20.7367072779153,-35.3312780646732,
124.126231712253)) ;
#61809=CARTESIAN_POINT('Ctrl Pts',(-20.4712234236235,-35.1512889843104,
123.983338754042)) ;
#61810=CARTESIAN_POINT('Ctrl Pts',(-20.8392082177454,-35.3411207756312,
123.888720096976)) ;
#61811=CARTESIAN_POINT('Ctrl Pts',(-20.5532221538063,-35.1611316952683,
123.793329345071)) ;
#61812=CARTESIAN_POINT('Ctrl Pts',(-20.9004009016988,-35.3511114929372,
123.633439183849)) ;
#61813=CARTESIAN_POINT('Ctrl Pts',(-20.6021745071673,-35.1711224125743,
123.589104328749)) ;
#61814=CARTESIAN_POINT('Ctrl Pts',(-20.9161968438839,-35.3610395760338,
123.373005745111)) ;
#61815=CARTESIAN_POINT('Ctrl Pts',(-20.6148094255355,-35.1810504956709,
123.38075785787)) ;
#61816=CARTESIAN_POINT('Ctrl Pts',(-20.8868090725257,-35.3710275061455,
123.112172972253)) ;
#61817=CARTESIAN_POINT('Ctrl Pts',(-20.5912974941036,-35.1910384257827,
123.172091979698)) ;
#61818=CARTESIAN_POINT('Ctrl Pts',(-20.8118024544747,-35.3810633322728,
122.859341843818)) ;
#61819=CARTESIAN_POINT('Ctrl Pts',(-20.5312904395145,-35.20107425191,122.969827526995)) ;
#61820=CARTESIAN_POINT('Ctrl Pts',(-20.6965136129544,-35.3909186693864,
122.627413231324)) ;
#61821=CARTESIAN_POINT('Ctrl Pts',(-20.4390581291398,-35.2109295890236,
122.784286070346)) ;
#61822=CARTESIAN_POINT('Ctrl Pts',(-20.5408432692029,-35.4009164042366,
122.415802979033)) ;
#61823=CARTESIAN_POINT('Ctrl Pts',(-20.3145205770678,-35.2209273238737,
122.614998959278)) ;
#61824=CARTESIAN_POINT('Ctrl Pts',(-20.3525343320192,-35.4108243082211,
122.235974665639)) ;
#61825=CARTESIAN_POINT('Ctrl Pts',(-20.1638726660472,-35.2308352278582,
122.471137872087)) ;
#61826=CARTESIAN_POINT('Ctrl Pts',(-20.1338538119606,-35.4208353827695,
122.089706748638)) ;
#61827=CARTESIAN_POINT('Ctrl Pts',(-19.9889274042967,-35.2408463024066,
122.354124872877)) ;
#61828=CARTESIAN_POINT('Ctrl Pts',(-19.8924829761476,-35.4308632383051,
121.983948431218)) ;
#61829=CARTESIAN_POINT('Ctrl Pts',(-19.7958300154897,-35.2508741579423,
122.26951973446)) ;
#61830=CARTESIAN_POINT('Ctrl Pts',(-19.6408783355081,-35.4407208322104,
121.922312589415)) ;
#61831=CARTESIAN_POINT('Ctrl Pts',(-19.5945467001667,-35.2607317518475,
122.220212798044)) ;
#61832=CARTESIAN_POINT('Ctrl Pts',(-19.3779878358377,-35.4507475190485,
121.904471410872)) ;
#61833=CARTESIAN_POINT('Ctrl Pts',(-19.3842341773709,-35.2707584386856,
122.205941341526)) ;
#61834=CARTESIAN_POINT('Ctrl Pts',(-19.116007159778,-35.4607761882022,121.933207053321)) ;
#61835=CARTESIAN_POINT('Ctrl Pts',(-19.1746497551832,-35.2807871078393,
122.228931467457)) ;
#61836=CARTESIAN_POINT('Ctrl Pts',(-18.8675097602884,-35.4706213964836,
122.005176454278)) ;
#61837=CARTESIAN_POINT('Ctrl Pts',(-18.975853120482,-35.2906323161207,122.286508201954)) ;
#61838=CARTESIAN_POINT('Ctrl Pts',(-18.6315240046396,-35.4806120854467,
122.120258716243)) ;
#61839=CARTESIAN_POINT('Ctrl Pts',(-18.787065262531,-35.3006230050839,122.3785751853)) ;
#61840=CARTESIAN_POINT('Ctrl Pts',(-18.4184551336644,-35.490649961729,122.275766762544)) ;
#61841=CARTESIAN_POINT('Ctrl Pts',(-18.6166109641243,-35.3106608813661,
122.502982897611)) ;
#61842=CARTESIAN_POINT('Ctrl Pts',(-18.2388143581137,-35.5004943393712,
122.461939201288)) ;
#61843=CARTESIAN_POINT('Ctrl Pts',(-18.472900009195,-35.3205052590084,122.651921150758)) ;
#61844=CARTESIAN_POINT('Ctrl Pts',(-18.0917605510307,-35.5104791437627,
122.679207506938)) ;
#61845=CARTESIAN_POINT('Ctrl Pts',(-18.3552581535845,-35.3304900633998,
122.825736359485)) ;
#61846=CARTESIAN_POINT('Ctrl Pts',(-17.9850190706446,-35.5204186739812,
122.917641507292)) ;
#61847=CARTESIAN_POINT('Ctrl Pts',(-18.2698663114521,-35.3404295936183,
123.016483683079)) ;
#61848=CARTESIAN_POINT('Ctrl Pts',(-17.9207300902949,-35.5304583620181,
123.173500108613)) ;
#61849=CARTESIAN_POINT('Ctrl Pts',(-18.2184363504254,-35.3504692816552,
123.221170992911)) ;
#61850=CARTESIAN_POINT('Ctrl Pts',(-17.9019975600655,-35.5403466513864,
123.43269321979)) ;
#61851=CARTESIAN_POINT('Ctrl Pts',(-18.2034516388014,-35.3603575710235,
123.428524836043)) ;
#61852=CARTESIAN_POINT('Ctrl Pts',(-17.928329013415,-35.5503357750712,123.693863790479)) ;
#61853=CARTESIAN_POINT('Ctrl Pts',(-18.2245179343512,-35.3703466947083,
123.637461006412)) ;
#61854=CARTESIAN_POINT('Ctrl Pts',(-17.9995984433313,-35.5602957847458,
123.945708092075)) ;
#61855=CARTESIAN_POINT('Ctrl Pts',(-18.2815345383664,-35.3803067043829,
123.83893578616)) ;
#61856=CARTESIAN_POINT('Ctrl Pts',(-18.1122794989603,-35.57019621445,124.180223126085)) ;
#61857=CARTESIAN_POINT('Ctrl Pts',(-18.3716800348444,-35.3902071340872,
124.026546724073)) ;
#61858=CARTESIAN_POINT('Ctrl Pts',(-18.2661525939819,-35.5802392958568,
124.394633262475)) ;
#61859=CARTESIAN_POINT('Ctrl Pts',(-18.4947794676731,-35.4002502154939,
124.198074338897)) ;
#61860=CARTESIAN_POINT('Ctrl Pts',(-18.4523813317248,-35.5901466897644,
124.576598857662)) ;
#61861=CARTESIAN_POINT('Ctrl Pts',(-18.6437627318548,-35.4101576094016,
124.343645597368)) ;
#61862=CARTESIAN_POINT('Ctrl Pts',(-18.6693558214365,-35.6001584207536,
124.725406064343)) ;
#61863=CARTESIAN_POINT('Ctrl Pts',(-18.817342832175,-35.4201693403907,124.462690554545)) ;
#61864=CARTESIAN_POINT('Ctrl Pts',(-18.9095840015776,-35.6101906384684,
124.834028669225)) ;
#61865=CARTESIAN_POINT('Ctrl Pts',(-19.0095258944054,-35.4302015581055,
124.549587692303)) ;
#61866=CARTESIAN_POINT('Ctrl Pts',(-19.1603393482666,-35.6200431477146,
124.898453661677)) ;
#61867=CARTESIAN_POINT('Ctrl Pts',(-19.2101294376099,-35.4400540673517,
124.601126473367)) ;
#61868=CARTESIAN_POINT('Ctrl Pts',(-19.4211928177086,-35.6300010842576,
124.919386454323)) ;
#61869=CARTESIAN_POINT('Ctrl Pts',(-19.4188119019026,-35.4500120038947,
124.617871878894)) ;
#61870=CARTESIAN_POINT('Ctrl Pts',(-19.6837654584528,-35.6400399542659,
124.894038281209)) ;
#61871=CARTESIAN_POINT('Ctrl Pts',(-19.6288700585704,-35.460050873903,124.59759241855)) ;
#61872=CARTESIAN_POINT('Ctrl Pts',(-19.9339392913664,-35.6499131094241,
124.825100619419)) ;
#61873=CARTESIAN_POINT('Ctrl Pts',(-19.8290080447909,-35.4699240290612,
124.542441760864)) ;
#61874=CARTESIAN_POINT('Ctrl Pts',(-20.1729716447795,-35.6599863842738,
124.711483830272)) ;
#61875=CARTESIAN_POINT('Ctrl Pts',(-20.0202338855392,-35.4799973039109,
124.451547444271)) ;
#61876=CARTESIAN_POINT('Ctrl Pts',(-20.3835167615202,-35.6698067014512,
124.562152640001)) ;
#61877=CARTESIAN_POINT('Ctrl Pts',(-20.1886685395271,-35.4898176210883,
124.332082614018)) ;
#61878=CARTESIAN_POINT('Ctrl Pts',(-20.5697933970036,-35.6798853872447,
124.373961088606)) ;
#61879=CARTESIAN_POINT('Ctrl Pts',(-20.337689632591,-35.4998963068818,124.1815286286)) ;
#61880=CARTESIAN_POINT('Ctrl Pts',(-20.7173141230226,-35.6897368986278,
124.161139832778)) ;
#61881=CARTESIAN_POINT('Ctrl Pts',(-20.4557050752507,-35.5097478182649,
124.011272119984)) ;
#61882=CARTESIAN_POINT('Ctrl Pts',(-20.8282376597634,-35.6998103449344,
123.920835993557)) ;
#61883=CARTESIAN_POINT('Ctrl Pts',(-20.5444435077093,-35.5198212645716,
123.81902847826)) ;
#61884=CARTESIAN_POINT('Ctrl Pts',(-20.8941975462152,-35.7096516200591,
123.670739828049)) ;
#61885=CARTESIAN_POINT('Ctrl Pts',(-20.5972105412205,-35.5296625396963,
123.618952491442)) ;
#61886=CARTESIAN_POINT('Ctrl Pts',(-20.9168565666188,-35.7196367197159,
123.409346913405)) ;
#61887=CARTESIAN_POINT('Ctrl Pts',(-20.6153373392901,-35.539647639353,123.409838356451)) ;
#61888=CARTESIAN_POINT('Ctrl Pts',(-20.8933643885283,-35.7296441958502,
123.147392528966)) ;
#61889=CARTESIAN_POINT('Ctrl Pts',(-20.5965431125166,-35.5496551154873,
123.200274949627)) ;
#61890=CARTESIAN_POINT('Ctrl Pts',(-20.8255661487373,-35.7395667835592,
122.89561863727)) ;
#61891=CARTESIAN_POINT('Ctrl Pts',(-20.5423042616246,-35.5595777031963,
122.998856548276)) ;
#61892=CARTESIAN_POINT('Ctrl Pts',(-20.7147391058567,-35.7495533878325,
122.657703592569)) ;
#61893=CARTESIAN_POINT('Ctrl Pts',(-20.4536424122356,-35.5695643074696,
122.80852482131)) ;
#61894=CARTESIAN_POINT('Ctrl Pts',(-20.5631005957844,-35.7595935161666,
122.44181432373)) ;
#61895=CARTESIAN_POINT('Ctrl Pts',(-20.3323311466458,-35.5796044358037,
122.635813545013)) ;
#61896=CARTESIAN_POINT('Ctrl Pts',(-20.380378834698,-35.7694329507,122.258824742576)) ;
#61897=CARTESIAN_POINT('Ctrl Pts',(-20.1861543576817,-35.5894438703371,
122.489422939203)) ;
#61898=CARTESIAN_POINT('Ctrl Pts',(-20.1640017994239,-35.779497005191,122.106806406757)) ;
#61899=CARTESIAN_POINT('Ctrl Pts',(-20.0130523328328,-35.5995079248281,
122.36780830073)) ;
#61900=CARTESIAN_POINT('Ctrl Pts',(-19.9285321533398,-35.7893879244282,
121.996676734452)) ;
#61901=CARTESIAN_POINT('Ctrl Pts',(-19.8246772528639,-35.6093988440653,
122.279705175091)) ;
#61902=CARTESIAN_POINT('Ctrl Pts',(-19.67513790255,-35.7993799177342,121.927884966154)) ;
#61903=CARTESIAN_POINT('Ctrl Pts',(-19.6219619807546,-35.6193908373713,
122.224671942912)) ;
#61904=CARTESIAN_POINT('Ctrl Pts',(-19.4143822634357,-35.8093427816935,
121.904446853395)) ;
#61905=CARTESIAN_POINT('Ctrl Pts',(-19.4133578143958,-35.6293537013306,
122.205921690293)) ;
#61906=CARTESIAN_POINT('Ctrl Pts',(-19.1549680514992,-35.8192470415113,
121.925855666197)) ;
#61907=CARTESIAN_POINT('Ctrl Pts',(-19.2058271969419,-35.6392579611484,
122.223048715094)) ;
#61908=CARTESIAN_POINT('Ctrl Pts',(-18.8993526736226,-35.8293075320827,
121.993232864711)) ;
#61909=CARTESIAN_POINT('Ctrl Pts',(-19.001334645375,-35.6493184517198,122.276950638567)) ;
#61910=CARTESIAN_POINT('Ctrl Pts',(-18.6643671184913,-35.8391478817137,
122.101269435871)) ;
#61911=CARTESIAN_POINT('Ctrl Pts',(-18.8133472746285,-35.6591588013508,
122.363379411723)) ;
#61912=CARTESIAN_POINT('Ctrl Pts',(-18.4467771153745,-35.8492108572037,
122.251492745729)) ;
#61913=CARTESIAN_POINT('Ctrl Pts',(-18.6392749852965,-35.6692217768408,
122.483558171074)) ;
#61914=CARTESIAN_POINT('Ctrl Pts',(-18.2618359407232,-35.8591051773471,
122.434298711921)) ;
#61915=CARTESIAN_POINT('Ctrl Pts',(-18.491322616233,-35.6791160969842,122.629802358124)) ;
#61916=CARTESIAN_POINT('Ctrl Pts',(-18.1101865601334,-35.8690468904787,
122.646995887001)) ;
#61917=CARTESIAN_POINT('Ctrl Pts',(-18.3700032496171,-35.6890578101158,
122.799959569415)) ;
#61918=CARTESIAN_POINT('Ctrl Pts',(-17.9969449047293,-35.8790497802728,
122.884263259516)) ;
#61919=CARTESIAN_POINT('Ctrl Pts',(-18.2794097634867,-35.69906069991,122.989773283224)) ;
#61920=CARTESIAN_POINT('Ctrl Pts',(-17.9268443214871,-35.8890896374333,
123.138590645404)) ;
#61921=CARTESIAN_POINT('Ctrl Pts',(-18.2233291597186,-35.7091005570704,
123.193235305604)) ;
#61922=CARTESIAN_POINT('Ctrl Pts',(-17.9019122829128,-35.8989138182709,
123.395574782342)) ;
#61923=CARTESIAN_POINT('Ctrl Pts',(-18.2033834027197,-35.7189247379081,
123.398821321961)) ;
#61924=CARTESIAN_POINT('Ctrl Pts',(-17.9220883778628,-35.9089707917741,
123.659068393619)) ;
#61925=CARTESIAN_POINT('Ctrl Pts',(-18.2195239554329,-35.7289817114113,
123.609616505664)) ;
#61926=CARTESIAN_POINT('Ctrl Pts',(-17.9871986049093,-35.9188989159612,
123.911729558089)) ;
#61927=CARTESIAN_POINT('Ctrl Pts',(-18.271611742449,-35.7389098355983,123.811744931268)) ;
#61928=CARTESIAN_POINT('Ctrl Pts',(-18.0948259751119,-35.9288526110346,
124.150136156797)) ;
#61929=CARTESIAN_POINT('Ctrl Pts',(-18.3577130663129,-35.7488635306717,
124.002469995443)) ;
#61930=CARTESIAN_POINT('Ctrl Pts',(-18.2438917115577,-35.9388988046099,
124.368025599995)) ;
#61931=CARTESIAN_POINT('Ctrl Pts',(-18.4769654839936,-35.758909724247,124.176781901697)) ;
#61932=CARTESIAN_POINT('Ctrl Pts',(-18.4247087145349,-35.9487469069698,
124.553177298368)) ;
#61933=CARTESIAN_POINT('Ctrl Pts',(-18.6216180178333,-35.7687578266069,
124.324902741368)) ;
#61934=CARTESIAN_POINT('Ctrl Pts',(-18.6368680943373,-35.9587084951974,
124.706511430656)) ;
#61935=CARTESIAN_POINT('Ctrl Pts',(-18.7913448718134,-35.7787194148345,
124.44757032455)) ;
#61936=CARTESIAN_POINT('Ctrl Pts',(-18.8741832744797,-35.9687371653537,
124.821161297278)) ;
#61937=CARTESIAN_POINT('Ctrl Pts',(-18.9811968587923,-35.7887480849908,
124.539290720976)) ;
#61938=CARTESIAN_POINT('Ctrl Pts',(-19.1247583602108,-35.9786474682354,
124.892091064519)) ;
#61939=CARTESIAN_POINT('Ctrl Pts',(-19.1816561053087,-35.7986583878725,
124.59603486579)) ;
#61940=CARTESIAN_POINT('Ctrl Pts',(-19.3844352240823,-35.9885823520433,
124.919183512007)) ;
#61941=CARTESIAN_POINT('Ctrl Pts',(-19.3893969971606,-35.8085932716804,
124.617709476599)) ;
#61942=CARTESIAN_POINT('Ctrl Pts',(-19.6476231191508,-35.9986234937339,
124.900335055066)) ;
#61943=CARTESIAN_POINT('Ctrl Pts',(-19.5999475089394,-35.8186344133711,
124.602631349119)) ;
#61944=CARTESIAN_POINT('Ctrl Pts',(-19.8996824512963,-36.0085106148979,
124.837232249301)) ;
#61945=CARTESIAN_POINT('Ctrl Pts',(-19.8015943370243,-35.828521534535,124.552149980266)) ;
#61946=CARTESIAN_POINT('Ctrl Pts',(-20.1396295182809,-36.0185029577464,
124.730608252142)) ;
#61947=CARTESIAN_POINT('Ctrl Pts',(-19.9935521670757,-35.8385138773836,
124.466851580924)) ;
#61948=CARTESIAN_POINT('Ctrl Pts',(-20.3564426703236,-36.0284512589704,
124.584508836111)) ;
#61949=CARTESIAN_POINT('Ctrl Pts',(-20.1670027663451,-35.8484621786075,
124.34997293713)) ;
#61950=CARTESIAN_POINT('Ctrl Pts',(-20.5446351269655,-36.0383888366525,
124.403471920414)) ;
#61951=CARTESIAN_POINT('Ctrl Pts',(-20.3175569672634,-35.8583997562896,
124.205144391475)) ;
#61952=CARTESIAN_POINT('Ctrl Pts',(-20.6995297067376,-36.0483754111031,
124.191598913458)) ;
#61953=CARTESIAN_POINT('Ctrl Pts',(-20.4414732773456,-35.8683863307402,
124.035646689111)) ;
#61954=CARTESIAN_POINT('Ctrl Pts',(-20.8154914356218,-36.0584042210115,
123.954937669147)) ;
#61955=CARTESIAN_POINT('Ctrl Pts',(-20.5342434668736,-35.8784151406487,
123.846318005785)) ;
#61956=CARTESIAN_POINT('Ctrl Pts',(-20.887745257479,-36.0682825423183,123.705606150759)) ;
#61957=CARTESIAN_POINT('Ctrl Pts',(-20.5920471744882,-35.8882934619554,
123.646853866704)) ;
#61958=CARTESIAN_POINT('Ctrl Pts',(-20.9165435264159,-36.0782741896657,
123.444611225449)) ;
#61959=CARTESIAN_POINT('Ctrl Pts',(-20.6150868306485,-35.8982851093029,
123.438058194467)) ;
#61960=CARTESIAN_POINT('Ctrl Pts',(-20.8989774525734,-36.0883087131035,
123.181512331536)) ;
#61961=CARTESIAN_POINT('Ctrl Pts',(-20.6010349029805,-35.9083196327406,
123.227578932499)) ;
#61962=CARTESIAN_POINT('Ctrl Pts',(-20.8375844347476,-36.0981720699821,
122.929660650926)) ;
#61963=CARTESIAN_POINT('Ctrl Pts',(-20.55192174251,-35.9181829896192,123.026098230027)) ;
#61964=CARTESIAN_POINT('Ctrl Pts',(-20.7312794061574,-36.1082422966624,
122.687347241547)) ;
#61965=CARTESIAN_POINT('Ctrl Pts',(-20.4668785833512,-35.9282532162995,
122.832246790872)) ;
#61966=CARTESIAN_POINT('Ctrl Pts',(-20.5878041611143,-36.1180846047971,
122.472130151302)) ;
#61967=CARTESIAN_POINT('Ctrl Pts',(-20.3520998563727,-35.9380955244342,
122.660073387355)) ;
#61968=CARTESIAN_POINT('Ctrl Pts',(-20.4077016432791,-36.1280453368205,
122.282190824122)) ;
#61969=CARTESIAN_POINT('Ctrl Pts',(-20.2080190009201,-35.9480562564576,
122.50812127463)) ;
#61970=CARTESIAN_POINT('Ctrl Pts',(-20.1954179813049,-36.1380832260186,
122.125622966376)) ;
#61971=CARTESIAN_POINT('Ctrl Pts',(-20.0381926818535,-35.9580941456557,
122.382865981336)) ;
#61972=CARTESIAN_POINT('Ctrl Pts',(-19.9632011127719,-36.1479575089374,
122.009756791366)) ;
#61973=CARTESIAN_POINT('Ctrl Pts',(-19.852420481698,-35.9679684285746,122.290172259536)) ;
#61974=CARTESIAN_POINT('Ctrl Pts',(-19.7095295605332,-36.1580272535549,
121.93454430428)) ;
#61975=CARTESIAN_POINT('Ctrl Pts',(-19.6494833349554,-35.978038173192,122.230000967982)) ;
#61976=CARTESIAN_POINT('Ctrl Pts',(-19.4527844206973,-36.1678605639005,
121.90508124975)) ;
#61977=CARTESIAN_POINT('Ctrl Pts',(-19.4440883880503,-35.9878714835377,
122.206429346442)) ;
#61978=CARTESIAN_POINT('Ctrl Pts',(-19.1896400044963,-36.1778908072532,
121.920204651437)) ;
#61979=CARTESIAN_POINT('Ctrl Pts',(-19.2335727027001,-35.9979017268903,
122.218526613797)) ;
#61980=CARTESIAN_POINT('Ctrl Pts',(-18.9332371754208,-36.1879230952316,
121.981571396722)) ;
#61981=CARTESIAN_POINT('Ctrl Pts',(-19.0284500699383,-36.0079340148687,
122.267618766793)) ;
#61982=CARTESIAN_POINT('Ctrl Pts',(-18.6960884547325,-36.1977502716997,
122.083816541885)) ;
#61983=CARTESIAN_POINT('Ctrl Pts',(-18.838731476733,-36.0177611913368,122.349413165543)) ;
#61984=CARTESIAN_POINT('Ctrl Pts',(-18.4761127317123,-36.2077556545666,
122.22778364051)) ;
#61985=CARTESIAN_POINT('Ctrl Pts',(-18.6627501158308,-36.0277665742037,
122.464585522614)) ;
#61986=CARTESIAN_POINT('Ctrl Pts',(-18.2849106465945,-36.2177382935593,
122.407469430057)) ;
#61987=CARTESIAN_POINT('Ctrl Pts',(-18.5097875384203,-36.0377492131964,
122.60833293523)) ;
#61988=CARTESIAN_POINT('Ctrl Pts',(-18.127151161634,-36.2277823606959,122.619049599079)) ;
#61989=CARTESIAN_POINT('Ctrl Pts',(-18.3835787128746,-36.047793280333,122.777596301397)) ;
#61990=CARTESIAN_POINT('Ctrl Pts',(-18.0107408057579,-36.2376035794999,
122.849407145954)) ;
#61991=CARTESIAN_POINT('Ctrl Pts',(-18.2904495064269,-36.057614499137,122.961880755855)) ;
#61992=CARTESIAN_POINT('Ctrl Pts',(-17.9338160941293,-36.247640418438,123.101693464145)) ;
#61993=CARTESIAN_POINT('Ctrl Pts',(-18.2289081204975,-36.0676513380751,
123.163709405385)) ;
#61994=CARTESIAN_POINT('Ctrl Pts',(-17.902648663204,-36.2576648305357,123.363283148383)) ;
#61995=CARTESIAN_POINT('Ctrl Pts',(-18.2039726598348,-36.0776757501728,
123.372980991972)) ;
#61996=CARTESIAN_POINT('Ctrl Pts',(-17.9165495303506,-36.267516914941,123.621816862721)) ;
#61997=CARTESIAN_POINT('Ctrl Pts',(-18.2150916816491,-36.0875278345781,
123.579807245692)) ;
#61998=CARTESIAN_POINT('Ctrl Pts',(-17.9755567901383,-36.2775078116842,
123.877618050233)) ;
#61999=CARTESIAN_POINT('Ctrl Pts',(-18.2622957977157,-36.0975187313213,
123.784448445474)) ;
#62000=CARTESIAN_POINT('Ctrl Pts',(-18.0772031608818,-36.2874258035851,
124.117648747743)) ;
#62001=CARTESIAN_POINT('Ctrl Pts',(-18.3436111230473,-36.1074367232222,
123.976473257481)) ;
#62002=CARTESIAN_POINT('Ctrl Pts',(-18.2204755143682,-36.2974539190421,
124.338803226218)) ;
#62003=CARTESIAN_POINT('Ctrl Pts',(-18.4582275584006,-36.1174648386792,
124.153397810827)) ;
#62004=CARTESIAN_POINT('Ctrl Pts',(-18.3973504809565,-36.3073390949842,
124.529066690562)) ;
#62005=CARTESIAN_POINT('Ctrl Pts',(-18.5997258423448,-36.1273500146213,
124.30560934978)) ;
#62006=CARTESIAN_POINT('Ctrl Pts',(-18.6063723872479,-36.3173284533911,
124.687887703223)) ;
#62007=CARTESIAN_POINT('Ctrl Pts',(-18.7669421404985,-36.1373393730282,
124.43266756716)) ;
#62008=CARTESIAN_POINT('Ctrl Pts',(-18.8412552934419,-36.3273696009714,
124.808127004772)) ;
#62009=CARTESIAN_POINT('Ctrl Pts',(-18.9548477220754,-36.1473805206085,
124.528860620491)) ;
#62010=CARTESIAN_POINT('Ctrl Pts',(-19.088082204701,-36.3372022239778,124.884553235414)) ;
#62011=CARTESIAN_POINT('Ctrl Pts',(-19.1523079763883,-36.157213143615,124.590003139103)) ;
#62012=CARTESIAN_POINT('Ctrl Pts',(-19.3485418518654,-36.3471962950886,
124.918229067231)) ;
#62013=CARTESIAN_POINT('Ctrl Pts',(-19.3606753488184,-36.1672072147257,
124.616945728324)) ;
#62014=CARTESIAN_POINT('Ctrl Pts',(-19.6117962054243,-36.3572249527295,
124.905606556835)) ;
#62015=CARTESIAN_POINT('Ctrl Pts',(-19.571278932422,-36.1772358723666,124.606849593265)) ;
#62016=CARTESIAN_POINT('Ctrl Pts',(-19.8651977309864,-36.3671092789223,
124.848586979554)) ;
#62017=CARTESIAN_POINT('Ctrl Pts',(-19.7740000730835,-36.1871201985594,
124.561235916018)) ;
#62018=CARTESIAN_POINT('Ctrl Pts',(-20.1070919688669,-36.3770750224129,
124.748197481995)) ;
#62019=CARTESIAN_POINT('Ctrl Pts',(-19.9675160571563,-36.19708594205,124.480926240918)) ;
#62020=CARTESIAN_POINT('Ctrl Pts',(-20.3290461476334,-36.3871034015441,
124.606136879299)) ;
#62021=CARTESIAN_POINT('Ctrl Pts',(-20.1450804639494,-36.2071143211812,
124.367279397955)) ;
#62022=CARTESIAN_POINT('Ctrl Pts',(-20.5207969131445,-36.397004247751,124.430224963369)) ;
#62023=CARTESIAN_POINT('Ctrl Pts',(-20.2984821301222,-36.2170151673881,
124.226551616459)) ;
#62024=CARTESIAN_POINT('Ctrl Pts',(-20.6815114754316,-36.4070629051681,
124.220415524595)) ;
#62025=CARTESIAN_POINT('Ctrl Pts',(-20.4270554231223,-36.2270738248052,
124.058705203557)) ;
#62026=CARTESIAN_POINT('Ctrl Pts',(-20.8012013743605,-36.41692046795,123.990625446808)) ;
#62027=CARTESIAN_POINT('Ctrl Pts',(-20.5228088997045,-36.2369313875871,
123.874874540363)) ;
#62028=CARTESIAN_POINT('Ctrl Pts',(-20.8809810994181,-36.4269888705032,
123.738394192383)) ;
#62029=CARTESIAN_POINT('Ctrl Pts',(-20.5866346717548,-36.2469997901403,
123.673090038089)) ;
#62030=CARTESIAN_POINT('Ctrl Pts',(-20.9150001537344,-36.4368442692428,
123.481625971228)) ;
#62031=CARTESIAN_POINT('Ctrl Pts',(-20.6138518770455,-36.2568551888799,
123.467676224677)) ;
#62032=CARTESIAN_POINT('Ctrl Pts',(-20.9045521214138,-36.4468391363167,
123.219187981031)) ;
#62033=CARTESIAN_POINT('Ctrl Pts',(-20.6054955832144,-36.2668500559538,
123.257725827146)) ;
#62034=CARTESIAN_POINT('Ctrl Pts',(-20.8479327596291,-36.4568704313002,
122.961723074886)) ;
#62035=CARTESIAN_POINT('Ctrl Pts',(-20.5602021162859,-36.2768813509373,
123.051753458956)) ;
#62036=CARTESIAN_POINT('Ctrl Pts',(-20.7495006730971,-36.4667369560267,
122.721841789066)) ;
#62037=CARTESIAN_POINT('Ctrl Pts',(-20.4814585578185,-36.2867478756638,
122.859848009329)) ;
#62038=CARTESIAN_POINT('Ctrl Pts',(-20.609591909687,-36.4767244267224,122.499818683266)) ;
#62039=CARTESIAN_POINT('Ctrl Pts',(-20.36953342095,-36.2967353463596,122.68222845983)) ;
#62040=CARTESIAN_POINT('Ctrl Pts',(-20.4340715146542,-36.4866691862863,
122.306140896146)) ;
#62041=CARTESIAN_POINT('Ctrl Pts',(-20.2291188313566,-36.3066801059234,
122.527284917964)) ;
#62042=CARTESIAN_POINT('Ctrl Pts',(-20.2254502142119,-36.4967147422351,
122.144429454285)) ;
#62043=CARTESIAN_POINT('Ctrl Pts',(-20.0622230962988,-36.3167256618723,
122.397914055264)) ;
#62044=CARTESIAN_POINT('Ctrl Pts',(-19.9963181527322,-36.5065743306102,
122.023404639029)) ;
#62045=CARTESIAN_POINT('Ctrl Pts',(-19.8789187628921,-36.3265852502474,
122.301092445277)) ;
#62046=CARTESIAN_POINT('Ctrl Pts',(-19.7463087037596,-36.5165752857463,
121.942510562632)) ;
#62047=CARTESIAN_POINT('Ctrl Pts',(-19.6789119467519,-36.3365862053834,
122.236375109967)) ;
#62048=CARTESIAN_POINT('Ctrl Pts',(-19.4885136890261,-36.5264795130239,
121.906393185174)) ;
#62049=CARTESIAN_POINT('Ctrl Pts',(-19.472676448649,-36.346490432661,122.207479050223)) ;
#62050=CARTESIAN_POINT('Ctrl Pts',(-19.2248160077214,-36.536521589919,121.915638023373)) ;
#62051=CARTESIAN_POINT('Ctrl Pts',(-19.2617182336787,-36.3565325095561,
122.214872707114)) ;
#62052=CARTESIAN_POINT('Ctrl Pts',(-18.9700774883834,-36.5464292026052,
121.969685726458)) ;
#62053=CARTESIAN_POINT('Ctrl Pts',(-19.0579271360362,-36.3664401222423,
122.258108661664)) ;
#62054=CARTESIAN_POINT('Ctrl Pts',(-18.7250847627801,-36.5564837332209,
122.068538595468)) ;
#62055=CARTESIAN_POINT('Ctrl Pts',(-18.8619321279312,-36.376494652858,122.337188894249)) ;
#62056=CARTESIAN_POINT('Ctrl Pts',(-18.5051552713082,-36.5663445197698,
122.205642071035)) ;
#62057=CARTESIAN_POINT('Ctrl Pts',(-18.6859875392954,-36.3863554394069,
122.446869671373)) ;
#62058=CARTESIAN_POINT('Ctrl Pts',(-18.309504624998,-36.5763382748409,122.380772756738)) ;
#62059=CARTESIAN_POINT('Ctrl Pts',(-18.5294655677005,-36.396349194478,122.586972503952)) ;
#62060=CARTESIAN_POINT('Ctrl Pts',(-18.1481936177485,-36.5862636350808,
122.585788118924)) ;
#62061=CARTESIAN_POINT('Ctrl Pts',(-18.4004150621657,-36.406274554718,122.750983322731)) ;
#62062=CARTESIAN_POINT('Ctrl Pts',(-18.0236841922653,-36.5962915644761,
122.818002834881)) ;
#62063=CARTESIAN_POINT('Ctrl Pts',(-18.300805562702,-36.4163024841132,122.936753987693)) ;
#62064=CARTESIAN_POINT('Ctrl Pts',(-17.9422706636189,-36.6061778312754,
123.064758942346)) ;
#62065=CARTESIAN_POINT('Ctrl Pts',(-18.2356726313687,-36.4261887509125,
123.134158078855)) ;
#62066=CARTESIAN_POINT('Ctrl Pts',(-17.9042663342486,-36.6162096001737,
123.325585129761)) ;
#62067=CARTESIAN_POINT('Ctrl Pts',(-18.2052669459445,-36.4362205198108,
123.342818652238)) ;
#62068=CARTESIAN_POINT('Ctrl Pts',(-17.9117588182437,-36.6260911960173,
123.585201643652)) ;
#62069=CARTESIAN_POINT('Ctrl Pts',(-18.2112586694567,-36.4461021156544,
123.55051186725)) ;
#62070=CARTESIAN_POINT('Ctrl Pts',(-17.9650896020763,-36.6361530814852,
123.844142860244)) ;
#62071=CARTESIAN_POINT('Ctrl Pts',(-18.2539211167218,-36.4561640011224,
123.757665267779)) ;
#62072=CARTESIAN_POINT('Ctrl Pts',(-18.0605371633806,-36.6460105155041,
124.084996144572)) ;
#62073=CARTESIAN_POINT('Ctrl Pts',(-18.3302769065666,-36.4660214351412,
123.950348570272)) ;
#62074=CARTESIAN_POINT('Ctrl Pts',(-18.1977180729179,-36.6560037585461,
124.308890236601)) ;
#62075=CARTESIAN_POINT('Ctrl Pts',(-18.4400203090856,-36.4760146781832,
124.129465536782)) ;
#62076=CARTESIAN_POINT('Ctrl Pts',(-18.3706217888367,-36.6659345194324,
124.504384734692)) ;
#62077=CARTESIAN_POINT('Ctrl Pts',(-18.5783393320726,-36.4859454390695,
124.285860564829)) ;
#62078=CARTESIAN_POINT('Ctrl Pts',(-18.6449288885869,-36.6792835116296,
124.7231001116)) ;
#62079=CARTESIAN_POINT('Ctrl Pts',(-18.797794429001,-36.4992944312667,124.46084539929)) ;
#62080=CARTESIAN_POINT('Ctrl Pts',(-18.9682246085567,-36.692551884446,124.863897618014)) ;
#62081=CARTESIAN_POINT('Ctrl Pts',(-19.0564576791259,-36.5125628040832,
124.573487208325)) ;
#62082=CARTESIAN_POINT('Ctrl Pts',(-19.3133563776516,-36.7058348258304,
124.916340475203)) ;
#62083=CARTESIAN_POINT('Ctrl Pts',(-19.3325181777442,-36.5258457454675,
124.615432945298)) ;
#62084=CARTESIAN_POINT('Ctrl Pts',(-19.5771730601609,-36.7158776116726,
124.9098870958)) ;
#62085=CARTESIAN_POINT('Ctrl Pts',(-19.5435804546175,-36.5358885313097,
124.610274688818)) ;
#62086=CARTESIAN_POINT('Ctrl Pts',(-19.8309776235917,-36.7257275542247,
124.858999538569)) ;
#62087=CARTESIAN_POINT('Ctrl Pts',(-19.7466221103153,-36.5457384738618,
124.569566509396)) ;
#62088=CARTESIAN_POINT('Ctrl Pts',(-20.0759163398289,-36.7357247871437,
124.764028514352)) ;
#62089=CARTESIAN_POINT('Ctrl Pts',(-19.9425753637021,-36.5557357067808,
124.493590557892)) ;
#62090=CARTESIAN_POINT('Ctrl Pts',(-20.3008516831836,-36.7457396824782,
124.627366616209)) ;
#62091=CARTESIAN_POINT('Ctrl Pts',(-20.1225212573089,-36.5657506021153,
124.384267868071)) ;
#62092=CARTESIAN_POINT('Ctrl Pts',(-20.5625371625823,-36.7589793591164,
124.398087289449)) ;
#62093=CARTESIAN_POINT('Ctrl Pts',(-20.3318880358835,-36.5789902787535,
124.200821860388)) ;
#62094=CARTESIAN_POINT('Ctrl Pts',(-20.8079029753691,-36.7755265835217,
124.033128787356)) ;
#62095=CARTESIAN_POINT('Ctrl Pts',(-20.5281632731602,-36.5955375031589,
123.908899479938)) ;
#62096=CARTESIAN_POINT('Ctrl Pts',(-20.9148689308505,-36.7921740206528,
123.60379676647)) ;
#62097=CARTESIAN_POINT('Ctrl Pts',(-20.6137528357625,-36.6121849402899,
123.56536784602)) ;
#62098=CARTESIAN_POINT('Ctrl Pts',(-20.9083945687103,-36.805463518131,123.254597757722)) ;
#62099=CARTESIAN_POINT('Ctrl Pts',(-20.6085683029633,-36.6254744377682,
123.286061935331)) ;
#62100=CARTESIAN_POINT('Ctrl Pts',(-20.8593749513475,-36.8153369259534,
122.99980702422)) ;
#62101=CARTESIAN_POINT('Ctrl Pts',(-20.56935600526,-36.6353478455905,123.082217773299)) ;
#62102=CARTESIAN_POINT('Ctrl Pts',(-20.7652312032613,-36.8253893035461,
122.752998369539)) ;
#62103=CARTESIAN_POINT('Ctrl Pts',(-20.4940428185494,-36.6454002231832,
122.884773343294)) ;
#62104=CARTESIAN_POINT('Ctrl Pts',(-20.6315577727922,-36.835292957087,122.529670136184)) ;
#62105=CARTESIAN_POINT('Ctrl Pts',(-20.3871046825718,-36.6553038767241,
122.706108244707)) ;
#62106=CARTESIAN_POINT('Ctrl Pts',(-20.4609498467479,-36.8452372260823,
122.331765024518)) ;
#62107=CARTESIAN_POINT('Ctrl Pts',(-20.250623548332,-36.6652481457194,122.547784435435)) ;
#62108=CARTESIAN_POINT('Ctrl Pts',(-20.1896663855523,-36.858568234415,122.109990345323)) ;
#62109=CARTESIAN_POINT('Ctrl Pts',(-20.0335788518521,-36.6785791540521,
122.3703552458)) ;
#62110=CARTESIAN_POINT('Ctrl Pts',(-19.7868089891935,-36.8751898149393,
121.928852787723)) ;
#62111=CARTESIAN_POINT('Ctrl Pts',(-19.7113302438444,-36.6952007345764,
122.22544992753)) ;
#62112=CARTESIAN_POINT('Ctrl Pts',(-19.3483970122196,-36.8917324856377,
121.895325330693)) ;
#62113=CARTESIAN_POINT('Ctrl Pts',(-19.3605382150688,-36.7117434052748,
122.198625176032)) ;
#62114=CARTESIAN_POINT('Ctrl Pts',(-19.0036058959069,-36.9050816452006,
121.959959179237)) ;
#62115=CARTESIAN_POINT('Ctrl Pts',(-19.084756195026,-36.7250925648377,122.250326885057)) ;
#62116=CARTESIAN_POINT('Ctrl Pts',(-18.678061892058,-36.9183097953601,122.081981867065)) ;
#62117=CARTESIAN_POINT('Ctrl Pts',(-18.8243006830399,-36.7383207149972,
122.347949900398)) ;
#62118=CARTESIAN_POINT('Ctrl Pts',(-18.3181836591371,-36.9349404724976,
122.338513488551)) ;
#62119=CARTESIAN_POINT('Ctrl Pts',(-18.536409956563,-36.7549513921347,122.553165511551)) ;
#62120=CARTESIAN_POINT('Ctrl Pts',(-18.0180562107992,-36.9548434117857,
122.774198058464)) ;
#62121=CARTESIAN_POINT('Ctrl Pts',(-18.2963005856459,-36.7748543314228,
122.901714217013)) ;
#62122=CARTESIAN_POINT('Ctrl Pts',(-17.884130698863,-36.974746278389,123.285845641894)) ;
#62123=CARTESIAN_POINT('Ctrl Pts',(-18.1891582490799,-36.7947571980261,
123.311031567695)) ;
#62124=CARTESIAN_POINT('Ctrl Pts',(-17.9320811341198,-36.9946594434938,
123.813046654327)) ;
#62125=CARTESIAN_POINT('Ctrl Pts',(-18.2275157048257,-36.8146703631309,
123.732793421951)) ;
#62126=CARTESIAN_POINT('Ctrl Pts',(-18.159115508631,-37.0146952726351,124.294661831118)) ;
#62127=CARTESIAN_POINT('Ctrl Pts',(-18.4091406225134,-36.8347061922723,
124.118086406354)) ;
#62128=CARTESIAN_POINT('Ctrl Pts',(-18.5326928560836,-37.0345138475132,
124.666191700449)) ;
#62129=CARTESIAN_POINT('Ctrl Pts',(-18.7080017265223,-36.8545247671503,
124.415313158299)) ;
#62130=CARTESIAN_POINT('Ctrl Pts',(-19.0136563927245,-37.0544841485552,
124.890270639901)) ;
#62131=CARTESIAN_POINT('Ctrl Pts',(-19.0927719398134,-36.8744950681923,
124.594578398497)) ;
#62132=CARTESIAN_POINT('Ctrl Pts',(-19.5404829664515,-37.0743756809197,
124.936789595179)) ;
#62133=CARTESIAN_POINT('Ctrl Pts',(-19.5142340085164,-36.8943866005569,
124.63179555628)) ;
#62134=CARTESIAN_POINT('Ctrl Pts',(-20.0545360586126,-37.0943987787363,
124.799534983068)) ;
#62135=CARTESIAN_POINT('Ctrl Pts',(-19.9254767467742,-36.9144096983734,
124.52199379209)) ;
#62136=CARTESIAN_POINT('Ctrl Pts',(-20.4863256454403,-37.1141955316562,
124.498745537816)) ;
#62137=CARTESIAN_POINT('Ctrl Pts',(-20.2709110786742,-36.9342064512933,
124.281362358102)) ;
#62138=CARTESIAN_POINT('Ctrl Pts',(-20.7931678599209,-37.134156620145,124.066005974626)) ;
#62139=CARTESIAN_POINT('Ctrl Pts',(-20.5163858339727,-36.9541675397821,
123.93517078883)) ;
#62140=CARTESIAN_POINT('Ctrl Pts',(-20.9329957734479,-37.1541348890772,
123.553712501942)) ;
#62141=CARTESIAN_POINT('Ctrl Pts',(-20.6282493161937,-36.9741458087143,
123.525336142619)) ;
#62142=CARTESIAN_POINT('Ctrl Pts',(-20.8907271345775,-37.1739549038682,
123.028678283237)) ;
#62143=CARTESIAN_POINT('Ctrl Pts',(-20.5944348575025,-36.9939658235053,
123.105306484844)) ;
#62144=CARTESIAN_POINT('Ctrl Pts',(-20.6717362479,-37.19389331312,122.546084069936)) ;
#62145=CARTESIAN_POINT('Ctrl Pts',(-20.4192415860018,-37.0139042327571,
122.719230493431)) ;
#62146=CARTESIAN_POINT('Ctrl Pts',(-20.298300215747,-37.2139404305124,122.165933042875)) ;
#62147=CARTESIAN_POINT('Ctrl Pts',(-20.1204933529623,-37.0339513501496,
122.415110073134)) ;
#62148=CARTESIAN_POINT('Ctrl Pts',(-19.8223796112928,-37.2337866763463,
121.938614397227)) ;
#62149=CARTESIAN_POINT('Ctrl Pts',(-19.7397550078523,-37.0537975959834,
122.233254223609)) ;
#62150=CARTESIAN_POINT('Ctrl Pts',(-19.2975051439848,-37.2536356448583,
121.885263707638)) ;
#62151=CARTESIAN_POINT('Ctrl Pts',(-19.3198535804931,-37.0736465644954,
122.190574646049)) ;
#62152=CARTESIAN_POINT('Ctrl Pts',(-18.7809853427193,-37.2736859471696,
122.01617607887)) ;
#62153=CARTESIAN_POINT('Ctrl Pts',(-18.9066385592989,-37.0936968668067,
122.295305374503)) ;
#62154=CARTESIAN_POINT('Ctrl Pts',(-18.3447935795883,-37.2935208696008,
122.312469305322)) ;
#62155=CARTESIAN_POINT('Ctrl Pts',(-18.5576842939248,-37.113531789238,122.532341920129)) ;
#62156=CARTESIAN_POINT('Ctrl Pts',(-18.0337656489116,-37.3134512708267,
122.741007439741)) ;
#62157=CARTESIAN_POINT('Ctrl Pts',(-18.3088629320483,-37.1334621904638,
122.875174080636)) ;
#62158=CARTESIAN_POINT('Ctrl Pts',(-17.8872187178112,-37.3333362161856,
123.249003693809)) ;
#62159=CARTESIAN_POINT('Ctrl Pts',(-18.1916271520052,-37.1533471358227,
123.28157263407)) ;
#62160=CARTESIAN_POINT('Ctrl Pts',(-17.9240043991043,-37.353408824337,123.781130410511)) ;
#62161=CARTESIAN_POINT('Ctrl Pts',(-18.2210576286058,-37.1734197439741,
123.707273187308)) ;
#62162=CARTESIAN_POINT('Ctrl Pts',(-18.1371306277917,-37.3732001406651,
124.262126611238)) ;
#62163=CARTESIAN_POINT('Ctrl Pts',(-18.3915613312149,-37.1932110603022,
124.092070982679)) ;
#62164=CARTESIAN_POINT('Ctrl Pts',(-18.5035285318798,-37.3931649304323,
124.645891221234)) ;
#62165=CARTESIAN_POINT('Ctrl Pts',(-18.6846818764584,-37.2131758500695,
124.399080894642)) ;
#62166=CARTESIAN_POINT('Ctrl Pts',(-18.979960539183,-37.4131478861826,124.8806328502)) ;
#62167=CARTESIAN_POINT('Ctrl Pts',(-19.0658287233952,-37.2331588058198,
124.586871974143)) ;
#62168=CARTESIAN_POINT('Ctrl Pts',(-19.5032077670167,-37.4329564081588,
124.93927814081)) ;
#62169=CARTESIAN_POINT('Ctrl Pts',(-19.4844282141108,-37.2529673277959,
124.633785395356)) ;
#62170=CARTESIAN_POINT('Ctrl Pts',(-20.0196196742879,-37.4529419828946,
124.815366561225)) ;
#62171=CARTESIAN_POINT('Ctrl Pts',(-19.8975570540621,-37.2729529025317,
124.534652928844)) ;
#62172=CARTESIAN_POINT('Ctrl Pts',(-20.4606042546842,-37.472824622963,124.523953283866)) ;
#62173=CARTESIAN_POINT('Ctrl Pts',(-20.2503434533714,-37.2928355426001,
124.301519156789)) ;
#62174=CARTESIAN_POINT('Ctrl Pts',(-20.7770251297192,-37.4927799350949,
124.098432867934)) ;
#62175=CARTESIAN_POINT('Ctrl Pts',(-20.5034774694716,-37.312790854732,123.961100528127)) ;
#62176=CARTESIAN_POINT('Ctrl Pts',(-20.9290068708027,-37.5126542917027,
123.592447664143)) ;
#62177=CARTESIAN_POINT('Ctrl Pts',(-20.6250594668182,-37.3326652113398,
123.556310724529)) ;
#62178=CARTESIAN_POINT('Ctrl Pts',(-20.8993899561854,-37.5326364985638,
123.062239130214)) ;
#62179=CARTESIAN_POINT('Ctrl Pts',(-20.6013622688047,-37.3526474182009,
123.132144083971)) ;
#62180=CARTESIAN_POINT('Ctrl Pts',(-20.690825481049,-37.5525675765137,122.575167631245)) ;
#62181=CARTESIAN_POINT('Ctrl Pts',(-20.4345064463008,-37.3725784961509,
122.742488126059)) ;
#62182=CARTESIAN_POINT('Ctrl Pts',(-20.3288457045334,-37.5724945513687,
122.188694790906)) ;
#62183=CARTESIAN_POINT('Ctrl Pts',(-20.1449218052122,-37.3925054710058,
122.433312456316)) ;
#62184=CARTESIAN_POINT('Ctrl Pts',(-19.8592684233419,-37.5923270103176,
121.94907564169)) ;
#62185=CARTESIAN_POINT('Ctrl Pts',(-19.7692491705873,-37.4123379299547,
122.241620182198)) ;
#62186=CARTESIAN_POINT('Ctrl Pts',(-19.4200658004663,-37.6089846944928,
121.894159881209)) ;
#62187=CARTESIAN_POINT('Ctrl Pts',(-19.4179129229134,-37.4289956141299,
122.197692407191)) ;
#62188=CARTESIAN_POINT('Ctrl Pts',(-19.0750788995633,-37.6222339183999,
121.941806794377)) ;
#62189=CARTESIAN_POINT('Ctrl Pts',(-19.1418999521506,-37.442244838037,122.235812007745)) ;
#62190=CARTESIAN_POINT('Ctrl Pts',(-18.8237258577179,-37.6322829398511,
122.022687580734)) ;
#62191=CARTESIAN_POINT('Ctrl Pts',(-18.9408249160599,-37.4522938594882,
122.300516750014)) ;
#62192=CARTESIAN_POINT('Ctrl Pts',(-18.5945663208798,-37.6421429480816,
122.143620577139)) ;
#62193=CARTESIAN_POINT('Ctrl Pts',(-18.7574893710446,-37.4621538677187,
122.397273180662)) ;
#62194=CARTESIAN_POINT('Ctrl Pts',(-18.318087679396,-37.6554264613062,122.356789242169)) ;
#62195=CARTESIAN_POINT('Ctrl Pts',(-18.5363454539202,-37.4754373809433,
122.567770274827)) ;
#62196=CARTESIAN_POINT('Ctrl Pts',(-18.0500066419728,-37.672072380307,122.708670183428)) ;
#62197=CARTESIAN_POINT('Ctrl Pts',(-18.3218393587194,-37.4920832999442,
122.849331203031)) ;
#62198=CARTESIAN_POINT('Ctrl Pts',(-17.9182173116251,-37.6886263581231,
123.1284860917)) ;
#62199=CARTESIAN_POINT('Ctrl Pts',(-18.2164325852077,-37.5086372777602,
123.185138398988)) ;
#62200=CARTESIAN_POINT('Ctrl Pts',(-17.9032980831102,-37.7019860870947,
123.479244069035)) ;
#62201=CARTESIAN_POINT('Ctrl Pts',(-18.2044905709866,-37.5219970067318,
123.465776425923)) ;
#62202=CARTESIAN_POINT('Ctrl Pts',(-17.9373186787806,-37.7118791388914,
123.737005381468)) ;
#62203=CARTESIAN_POINT('Ctrl Pts',(-18.2317111977967,-37.5318900585285,
123.671978909914)) ;
#62204=CARTESIAN_POINT('Ctrl Pts',(-18.0159935017335,-37.7218691041725,
123.987433562175)) ;
#62205=CARTESIAN_POINT('Ctrl Pts',(-18.2946526703774,-37.5418800238096,
123.872322439341)) ;
#62206=CARTESIAN_POINT('Ctrl Pts',(-18.1363891804887,-37.7318209850333,
124.219643590471)) ;
#62207=CARTESIAN_POINT('Ctrl Pts',(-18.3909713400926,-37.5518319046704,
124.058088956669)) ;
#62208=CARTESIAN_POINT('Ctrl Pts',(-18.2969510924967,-37.7418693367251,
124.42924502608)) ;
#62209=CARTESIAN_POINT('Ctrl Pts',(-18.5194225674474,-37.5618802563622,
124.225768799345)) ;
#62210=CARTESIAN_POINT('Ctrl Pts',(-18.4872912316246,-37.7517106208313,
124.60436691775)) ;
#62211=CARTESIAN_POINT('Ctrl Pts',(-18.6716962379228,-37.5717215404684,
124.365864646808)) ;
#62212=CARTESIAN_POINT('Ctrl Pts',(-18.7080075972399,-37.761697323957,124.746264446467)) ;
#62213=CARTESIAN_POINT('Ctrl Pts',(-18.848270497138,-37.5817082435941,124.479380739021)) ;
#62214=CARTESIAN_POINT('Ctrl Pts',(-18.9487838243805,-37.7716323527744,
124.847344520004)) ;
#62215=CARTESIAN_POINT('Ctrl Pts',(-19.0408922983168,-37.5916432724115,
124.560242693313)) ;
#62216=CARTESIAN_POINT('Ctrl Pts',(-19.2065084133453,-37.7816881476813,
124.905549326523)) ;
#62217=CARTESIAN_POINT('Ctrl Pts',(-19.2470724255386,-37.6016990673184,
124.606804323034)) ;
#62218=CARTESIAN_POINT('Ctrl Pts',(-19.4645118314012,-37.7915165109706,
124.918239663582)) ;
#62219=CARTESIAN_POINT('Ctrl Pts',(-19.4534751612069,-37.6115274306077,
124.61695433475)) ;
#62220=CARTESIAN_POINT('Ctrl Pts',(-19.7268395348764,-37.8015774808685,
124.885556198697)) ;
#62221=CARTESIAN_POINT('Ctrl Pts',(-19.6633370066296,-37.6215884005056,
124.590805332165)) ;
#62222=CARTESIAN_POINT('Ctrl Pts',(-19.975820977289,-37.8114917597583,124.808729302256)) ;
#62223=CARTESIAN_POINT('Ctrl Pts',(-19.8625213953459,-37.6315026793954,
124.529341692583)) ;
#62224=CARTESIAN_POINT('Ctrl Pts',(-20.2101091148539,-37.8215007542265,
124.689174409311)) ;
#62225=CARTESIAN_POINT('Ctrl Pts',(-20.0499508319165,-37.6415116738637,
124.433695808887)) ;
#62226=CARTESIAN_POINT('Ctrl Pts',(-20.4201860704738,-37.8315305887903,
124.529999912084)) ;
#62227=CARTESIAN_POINT('Ctrl Pts',(-20.2180110082682,-37.6515415084274,
124.306354429914)) ;
#62228=CARTESIAN_POINT('Ctrl Pts',(-20.596742436033,-37.8413888188625,124.340392518913)) ;
#62229=CARTESIAN_POINT('Ctrl Pts',(-20.3592543312716,-37.6613997384997,
124.154667125539)) ;
#62230=CARTESIAN_POINT('Ctrl Pts',(-20.7399359738029,-37.8513875246049,
124.120135025723)) ;
#62231=CARTESIAN_POINT('Ctrl Pts',(-20.4738072491821,-37.6713984442421,
123.978459973914)) ;
#62232=CARTESIAN_POINT('Ctrl Pts',(-20.8419611023496,-37.8612821805237,
123.880914135963)) ;
#62233=CARTESIAN_POINT('Ctrl Pts',(-20.5554252348265,-37.6812931001609,
123.787082588274)) ;
#62234=CARTESIAN_POINT('Ctrl Pts',(-20.9018013798977,-37.8713452449077,
123.62337316206)) ;
#62235=CARTESIAN_POINT('Ctrl Pts',(-20.603295299142,-37.6913561645448,123.581049278094)) ;
#62236=CARTESIAN_POINT('Ctrl Pts',(-20.9159903077687,-37.8811849031876,
123.365144028715)) ;
#62237=CARTESIAN_POINT('Ctrl Pts',(-20.6146442263728,-37.7011958228247,
123.374466181267)) ;
#62238=CARTESIAN_POINT('Ctrl Pts',(-20.8847687942713,-37.8912480702694,
123.102580743054)) ;
#62239=CARTESIAN_POINT('Ctrl Pts',(-20.589664844702,-37.7112589899066,123.16441577383)) ;
#62240=CARTESIAN_POINT('Ctrl Pts',(-20.809484036126,-37.9011423153965,122.853677895888)) ;
#62241=CARTESIAN_POINT('Ctrl Pts',(-20.5294350133251,-37.7211532350337,
122.965294385449)) ;
#62242=CARTESIAN_POINT('Ctrl Pts',(-20.6922226402162,-37.9110841370011,
122.620247034589)) ;
#62243=CARTESIAN_POINT('Ctrl Pts',(-20.4356240768759,-37.7310950566383,
122.778550847944)) ;
#62244=CARTESIAN_POINT('Ctrl Pts',(-20.5352958890887,-37.9210866679192,
122.40933067988)) ;
#62245=CARTESIAN_POINT('Ctrl Pts',(-20.3100810068094,-37.7410975875563,
122.60981908937)) ;
#62246=CARTESIAN_POINT('Ctrl Pts',(-20.3432724835516,-37.9311212943767,
122.228617908719)) ;
#62247=CARTESIAN_POINT('Ctrl Pts',(-20.1564607864245,-37.7511322140138,
122.465250443075)) ;
#62248=CARTESIAN_POINT('Ctrl Pts',(-20.1271504515569,-37.9409668293631,
122.086359667686)) ;
#62249=CARTESIAN_POINT('Ctrl Pts',(-19.9835623661803,-37.7609777490003,
122.351445878483)) ;
#62250=CARTESIAN_POINT('Ctrl Pts',(-19.8865382083941,-37.9509502542022,
121.981841696408)) ;
#62251=CARTESIAN_POINT('Ctrl Pts',(-19.7910718730727,-37.7709611738393,
122.267833461775)) ;
#62252=CARTESIAN_POINT('Ctrl Pts',(-19.6322370248592,-37.9609006445672,
121.920936388949)) ;
#62253=CARTESIAN_POINT('Ctrl Pts',(-19.5876306530056,-37.7809115642044,
122.219111287148)) ;
#62254=CARTESIAN_POINT('Ctrl Pts',(-19.3699906918077,-37.9708982848643,
121.904681189327)) ;
#62255=CARTESIAN_POINT('Ctrl Pts',(-19.3778335442572,-37.7909092045014,
122.206109169459)) ;
#62256=CARTESIAN_POINT('Ctrl Pts',(-19.1079206636273,-37.9809373654275,
121.934852971173)) ;
#62257=CARTESIAN_POINT('Ctrl Pts',(-19.1681777138388,-37.8009482850646,
122.230248687512)) ;
#62258=CARTESIAN_POINT('Ctrl Pts',(-18.860240682653,-37.9907635161966,122.007929238581)) ;
#62259=CARTESIAN_POINT('Ctrl Pts',(-18.9700348973941,-37.8107744358337,
122.288711477367)) ;
#62260=CARTESIAN_POINT('Ctrl Pts',(-18.6234287247367,-38.0008200911257,
122.125206427547)) ;
#62261=CARTESIAN_POINT('Ctrl Pts',(-18.7805861344579,-37.8208310107629,
122.382535045153)) ;
#62262=CARTESIAN_POINT('Ctrl Pts',(-18.4132844279037,-38.010760630506,122.280394942276)) ;
#62263=CARTESIAN_POINT('Ctrl Pts',(-18.6124721241605,-37.8307715501431,
122.506687339545)) ;
#62264=CARTESIAN_POINT('Ctrl Pts',(-18.2333456791287,-38.0206650234824,
122.468461282899)) ;
#62265=CARTESIAN_POINT('Ctrl Pts',(-18.4685228183294,-37.8406759431195,
122.657141441045)) ;
#62266=CARTESIAN_POINT('Ctrl Pts',(-18.0868734496572,-38.0307116776873,
122.68809334047)) ;
#62267=CARTESIAN_POINT('Ctrl Pts',(-18.3513466170776,-37.8507225973244,
122.832848242214)) ;
#62268=CARTESIAN_POINT('Ctrl Pts',(-17.9821139835232,-38.0406072396257,
122.926149688474)) ;
#62269=CARTESIAN_POINT('Ctrl Pts',(-18.2675409920432,-37.8606181592628,
123.023293667874)) ;
#62270=CARTESIAN_POINT('Ctrl Pts',(-17.9192592235961,-38.0506693174713,
123.182952338498)) ;
#62271=CARTESIAN_POINT('Ctrl Pts',(-18.2172590200462,-37.8706802371084,
123.228736387907)) ;
#62272=CARTESIAN_POINT('Ctrl Pts',(-17.9021734628791,-38.060512015885,123.441072933946)) ;
#62273=CARTESIAN_POINT('Ctrl Pts',(-18.2035923555535,-37.8805229355222,
123.43523229754)) ;
#62274=CARTESIAN_POINT('Ctrl Pts',(-17.9299628607559,-38.0705027908465,
123.702111270586)) ;
#62275=CARTESIAN_POINT('Ctrl Pts',(-18.2258256600623,-37.8905137104836,
123.644062635813)) ;
#62276=CARTESIAN_POINT('Ctrl Pts',(-18.0022482230094,-38.0804306558656,
123.952806457239)) ;
#62277=CARTESIAN_POINT('Ctrl Pts',(-18.2836555848188,-37.9004415755027,
123.844617906558)) ;
#62278=CARTESIAN_POINT('Ctrl Pts',(-18.1172694269985,-38.0904194006318,
124.188763665487)) ;
#62279=CARTESIAN_POINT('Ctrl Pts',(-18.3756740525521,-37.9104303202689,
124.033382779807)) ;
#62280=CARTESIAN_POINT('Ctrl Pts',(-18.2725063779841,-38.1004521862187,
124.401872836885)) ;
#62281=CARTESIAN_POINT('Ctrl Pts',(-18.4998651103405,-37.9204631058559,
124.203869099965)) ;
#62282=CARTESIAN_POINT('Ctrl Pts',(-18.4590525160662,-38.1103188708394,
124.581942987114)) ;
#62283=CARTESIAN_POINT('Ctrl Pts',(-18.6491027477406,-37.9303297904765,
124.347923469176)) ;
#62284=CARTESIAN_POINT('Ctrl Pts',(-18.6756943059788,-38.1202807630025,
124.728918023254)) ;
#62285=CARTESIAN_POINT('Ctrl Pts',(-18.8224168656527,-37.9402916826396,
124.46550199026)) ;
#62286=CARTESIAN_POINT('Ctrl Pts',(-18.9164378070942,-38.1303142399151,
124.836426983259)) ;
#62287=CARTESIAN_POINT('Ctrl Pts',(-19.0150124287312,-37.9503251595522,
124.551507627464)) ;
#62288=CARTESIAN_POINT('Ctrl Pts',(-19.1683321359747,-38.1401985811634,
124.899959302381)) ;
#62289=CARTESIAN_POINT('Ctrl Pts',(-19.2165276738214,-37.9602095008005,
124.602331745054)) ;
#62290=CARTESIAN_POINT('Ctrl Pts',(-19.4320465863447,-38.1502615232845,
124.919128358715)) ;
#62291=CARTESIAN_POINT('Ctrl Pts',(-19.4274995576439,-37.9702724429217,
124.617665373635)) ;
#62292=CARTESIAN_POINT('Ctrl Pts',(-19.6895940464433,-38.1601119249041,
124.892904733968)) ;
#62293=CARTESIAN_POINT('Ctrl Pts',(-19.6335365291386,-37.9801228445412,
124.596684955515)) ;
#62294=CARTESIAN_POINT('Ctrl Pts',(-19.9432929414163,-38.1701388136938,
124.821745925476)) ;
#62295=CARTESIAN_POINT('Ctrl Pts',(-19.8364952746785,-37.9901497333309,
124.539756471089)) ;
#62296=CARTESIAN_POINT('Ctrl Pts',(-20.1805416769707,-38.18016742865,124.706967424635)) ;
#62297=CARTESIAN_POINT('Ctrl Pts',(-20.0262936087495,-38.0001783482871,
124.447932190044)) ;
#62298=CARTESIAN_POINT('Ctrl Pts',(-20.3906137720793,-38.19001265177,124.555971632204)) ;
#62299=CARTESIAN_POINT('Ctrl Pts',(-20.1943496685895,-38.0100235714072,
124.327134842774)) ;
#62300=CARTESIAN_POINT('Ctrl Pts',(-20.574464611682,-38.200003335576,124.368535624673)) ;
#62301=CARTESIAN_POINT('Ctrl Pts',(-20.3414292436618,-38.0200142552131,
124.177185180511)) ;
#62302=CARTESIAN_POINT('Ctrl Pts',(-20.7231886883335,-38.2100412176484,
124.1506774248)) ;
#62303=CARTESIAN_POINT('Ctrl Pts',(-20.4604073258307,-38.0300521372856,
124.002897686156)) ;
#62304=CARTESIAN_POINT('Ctrl Pts',(-20.8301490996899,-38.2198855772873,
123.915113415464)) ;
#62305=CARTESIAN_POINT('Ctrl Pts',(-20.5459739843948,-38.0398964969244,
123.814446751513)) ;
#62306=CARTESIAN_POINT('Ctrl Pts',(-20.8959919668574,-38.229870447902,123.661153850813)) ;
#62307=CARTESIAN_POINT('Ctrl Pts',(-20.5986469676164,-38.0498813675391,
123.611278966283)) ;
#62308=CARTESIAN_POINT('Ctrl Pts',(-20.9167692456538,-38.2398097312307,
123.400748772405)) ;
#62309=CARTESIAN_POINT('Ctrl Pts',(-20.6152674855689,-38.0598206508678,
123.402955237377)) ;
#62310=CARTESIAN_POINT('Ctrl Pts',(-20.8916876625912,-38.2498503406038,
123.138114322854)) ;
#62311=CARTESIAN_POINT('Ctrl Pts',(-20.5952009193857,-38.0698612602409,
123.192847680362)) ;
#62312=CARTESIAN_POINT('Ctrl Pts',(-20.8226462971584,-38.259735191517,122.887662089246)) ;
#62313=CARTESIAN_POINT('Ctrl Pts',(-20.5399668195097,-38.0797461111542,
122.992486951818)) ;
#62314=CARTESIAN_POINT('Ctrl Pts',(-20.710161993773,-38.2697371476858,122.650150261944)) ;
#62315=CARTESIAN_POINT('Ctrl Pts',(-20.44997835604,-38.089748067323,122.802478099931)) ;
#62316=CARTESIAN_POINT('Ctrl Pts',(-20.5595370994859,-38.2796557444063,
122.437376954978)) ;
#62317=CARTESIAN_POINT('Ctrl Pts',(-20.3294778457341,-38.0996666640434,
122.632260578575)) ;
#62318=CARTESIAN_POINT('Ctrl Pts',(-20.3718806509748,-38.2897025664821,
122.251710845181)) ;
#62319=CARTESIAN_POINT('Ctrl Pts',(-20.1793517557982,-38.1097134861192,
122.483728389381)) ;
#62320=CARTESIAN_POINT('Ctrl Pts',(-20.1586361996875,-38.2995768475948,
122.103781930093)) ;
#62321=CARTESIAN_POINT('Ctrl Pts',(-20.0087562603686,-38.1195877672319,
122.365386632677)) ;
#62322=CARTESIAN_POINT('Ctrl Pts',(-19.9188009996355,-38.3096310476394,
121.993039914093)) ;
#62323=CARTESIAN_POINT('Ctrl Pts',(-19.8168874663292,-38.1296419672765,
122.276793896463)) ;
#62324=CARTESIAN_POINT('Ctrl Pts',(-19.6673495935004,-38.3195264772746,
121.926560229075)) ;
#62325=CARTESIAN_POINT('Ctrl Pts',(-19.615726790868,-38.1395373969118,122.223611339034)) ;
#62326=CARTESIAN_POINT('Ctrl Pts',(-19.403909575533,-38.329588105592,121.904328761475)) ;
#62327=CARTESIAN_POINT('Ctrl Pts',(-19.4049744286583,-38.1495990252291,
122.20582716044)) ;
#62328=CARTESIAN_POINT('Ctrl Pts',(-19.1462446840125,-38.3394327344219,
121.927632920062)) ;
#62329=CARTESIAN_POINT('Ctrl Pts',(-19.1988436604768,-38.159443654059,122.224471403124)) ;
#62330=CARTESIAN_POINT('Ctrl Pts',(-18.8933810810859,-38.3493927820275,
121.99520301882)) ;
#62331=CARTESIAN_POINT('Ctrl Pts',(-18.9965533361364,-38.1694037016646,
122.278528153739)) ;
#62332=CARTESIAN_POINT('Ctrl Pts',(-18.6544538829586,-38.3594310882016,
122.106985936773)) ;
#62333=CARTESIAN_POINT('Ctrl Pts',(-18.8054118480748,-38.1794420078387,
122.367955372878)) ;
#62334=CARTESIAN_POINT('Ctrl Pts',(-18.4417836193016,-38.3693043876342,
122.255686315727)) ;
#62335=CARTESIAN_POINT('Ctrl Pts',(-18.6352768308471,-38.1893153072714,
122.486915811868)) ;
#62336=CARTESIAN_POINT('Ctrl Pts',(-18.254572634365,-38.3793776492205,122.442761738888)) ;
#62337=CARTESIAN_POINT('Ctrl Pts',(-18.4855083791044,-38.1993885688576,
122.636576970832)) ;
#62338=CARTESIAN_POINT('Ctrl Pts',(-18.1061577776451,-38.3891978751772,
122.653952116024)) ;
#62339=CARTESIAN_POINT('Ctrl Pts',(-18.3667778089366,-38.2092087948143,
122.805528675082)) ;
#62340=CARTESIAN_POINT('Ctrl Pts',(-17.9936243510384,-38.3992769391167,
122.893649468812)) ;
#62341=CARTESIAN_POINT('Ctrl Pts',(-18.2767515207265,-38.2192878587538,
122.997287189187)) ;
#62342=CARTESIAN_POINT('Ctrl Pts',(-17.9258375544917,-38.4091270291365,
123.143539427592)) ;
#62343=CARTESIAN_POINT('Ctrl Pts',(-18.2225229861537,-38.2291379487737,
123.197198298179)) ;
#62344=CARTESIAN_POINT('Ctrl Pts',(-17.9018026838566,-38.4192057827503,
123.40723841002)) ;
#62345=CARTESIAN_POINT('Ctrl Pts',(-18.2032956687307,-38.2392167023874,
123.408157924605)) ;
#62346=CARTESIAN_POINT('Ctrl Pts',(-17.923166969544,-38.4290272500098,123.664509279081)) ;
#62347=CARTESIAN_POINT('Ctrl Pts',(-18.2203875531494,-38.2490381696469,
123.613973301711)) ;
#62348=CARTESIAN_POINT('Ctrl Pts',(-17.9900867207186,-38.4390928483674,
123.920355248471)) ;
#62349=CARTESIAN_POINT('Ctrl Pts',(-18.2739238795727,-38.2591037680045,
123.818650252036)) ;
#62350=CARTESIAN_POINT('Ctrl Pts',(-18.0987428644432,-38.4489955041421,
124.156888509072)) ;
#62351=CARTESIAN_POINT('Ctrl Pts',(-18.3608489306835,-38.2690064237792,
124.007875995514)) ;
#62352=CARTESIAN_POINT('Ctrl Pts',(-18.2488988281451,-38.4590463299717,
124.374113939604)) ;
#62353=CARTESIAN_POINT('Ctrl Pts',(-18.4809742059933,-38.2790572496089,
124.181656254911)) ;
#62354=CARTESIAN_POINT('Ctrl Pts',(-18.4311282813033,-38.4689205343106,
124.558922029202)) ;
#62355=CARTESIAN_POINT('Ctrl Pts',(-18.6267574017553,-38.2889314539477,
124.329501781547)) ;
#62356=CARTESIAN_POINT('Ctrl Pts',(-18.6468226000741,-38.4789929843497,
124.712247945028)) ;
#62357=CARTESIAN_POINT('Ctrl Pts',(-18.7993133663225,-38.2990039039868,
124.452162386081)) ;
#62358=CARTESIAN_POINT('Ctrl Pts',(-18.8800743167778,-38.4888220011232,
124.823318123614)) ;
#62359=CARTESIAN_POINT('Ctrl Pts',(-18.985913767497,-38.3088329207603,124.54101769674)) ;
#62360=CARTESIAN_POINT('Ctrl Pts',(-19.1349034186575,-38.498888847038,124.894192497804)) ;
#62361=CARTESIAN_POINT('Ctrl Pts',(-19.18977742163,-38.3188997666751,124.597717046058)) ;
#62362=CARTESIAN_POINT('Ctrl Pts',(-19.3936404772055,-38.5087790183398,
124.919135574597)) ;
#62363=CARTESIAN_POINT('Ctrl Pts',(-19.3967662609791,-38.3287899379769,
124.6176711408)) ;
#62364=CARTESIAN_POINT('Ctrl Pts',(-19.6554475745632,-38.5187712119636,
124.899143715405)) ;
#62365=CARTESIAN_POINT('Ctrl Pts',(-19.6062117573264,-38.3387821316008,
124.601677525334)) ;
#62366=CARTESIAN_POINT('Ctrl Pts',(-19.9090056650285,-38.5287340225871,
124.833945501294)) ;
#62367=CARTESIAN_POINT('Ctrl Pts',(-19.8090578249638,-38.3487449422242,
124.549518845411)) ;
#62368=CARTESIAN_POINT('Ctrl Pts',(-20.1462891748571,-38.5386382954305,
124.726937805208)) ;
#62369=CARTESIAN_POINT('Ctrl Pts',(-19.9988839326754,-38.3586492150676,
124.463912964312)) ;
#62370=CARTESIAN_POINT('Ctrl Pts',(-20.3646057034677,-38.5486987872351,
124.577884540204)) ;
#62371=CARTESIAN_POINT('Ctrl Pts',(-20.173537335335,-38.3687097068723,124.344670113735)) ;
#62372=CARTESIAN_POINT('Ctrl Pts',(-20.549872151261,-38.5585391189074,124.397423633048)) ;
#62373=CARTESIAN_POINT('Ctrl Pts',(-20.3217496440126,-38.3785500385446,
124.200302203012)) ;
#62374=CARTESIAN_POINT('Ctrl Pts',(-20.7046268368384,-38.5686021649992,
124.183029887266)) ;
#62375=CARTESIAN_POINT('Ctrl Pts',(-20.4455536256558,-38.3886130846363,
124.028787005913)) ;
#62376=CARTESIAN_POINT('Ctrl Pts',(-20.8177037943771,-38.5784962206943,
123.948871113631)) ;
#62377=CARTESIAN_POINT('Ctrl Pts',(-20.5360148493182,-38.3985071403314,
123.841460727974)) ;
#62378=CARTESIAN_POINT('Ctrl Pts',(-20.889425745872,-38.5884389210173,123.697654055537)) ;
#62379=CARTESIAN_POINT('Ctrl Pts',(-20.5933924604119,-38.4084498406544,
123.640487633951)) ;
#62380=CARTESIAN_POINT('Ctrl Pts',(-20.9166674415414,-38.5984446619449,
123.436101061356)) ;
#62381=CARTESIAN_POINT('Ctrl Pts',(-20.6151860207473,-38.418455581582,123.431245328084)) ;
#62382=CARTESIAN_POINT('Ctrl Pts',(-20.8977588227754,-38.6084655724604,
123.173448091062)) ;
#62383=CARTESIAN_POINT('Ctrl Pts',(-20.6000592553857,-38.4284764920975,
123.221122910589)) ;
#62384=CARTESIAN_POINT('Ctrl Pts',(-20.8346540510326,-38.6183563079104,
122.921298084122)) ;
#62385=CARTESIAN_POINT('Ctrl Pts',(-20.5495758458622,-38.4383672275475,
123.019403663293)) ;
#62386=CARTESIAN_POINT('Ctrl Pts',(-20.7280091756525,-38.6283478486392,
122.68137528438)) ;
#62387=CARTESIAN_POINT('Ctrl Pts',(-20.4642602954684,-38.4483587682763,
122.827465455942)) ;
#62388=CARTESIAN_POINT('Ctrl Pts',(-20.5819003598894,-38.6382957090609,
122.46460048107)) ;
#62389=CARTESIAN_POINT('Ctrl Pts',(-20.3473737456245,-38.458306628698,122.654045845982)) ;
#62390=CARTESIAN_POINT('Ctrl Pts',(-20.400753356158,-38.6482423782472,122.276140396852)) ;
#62391=CARTESIAN_POINT('Ctrl Pts',(-20.2024567640308,-38.4682532978843,
122.503277819394)) ;
#62392=CARTESIAN_POINT('Ctrl Pts',(-20.1873323482229,-38.6582904543828,
122.12067245961)) ;
#62393=CARTESIAN_POINT('Ctrl Pts',(-20.0317199988072,-38.4783013740199,
122.378903072768)) ;
#62394=CARTESIAN_POINT('Ctrl Pts',(-19.9549752001431,-38.6681380523884,
122.006738756206)) ;
#62395=CARTESIAN_POINT('Ctrl Pts',(-19.8458354617128,-38.4881489720256,
122.287756243606)) ;
#62396=CARTESIAN_POINT('Ctrl Pts',(-19.703727329421,-38.6780997754729,121.933263220706)) ;
#62397=CARTESIAN_POINT('Ctrl Pts',(-19.6448376844739,-38.49811069511,122.228975335749)) ;
#62398=CARTESIAN_POINT('Ctrl Pts',(-19.4417254602095,-38.6881284105559,
121.904664952716)) ;
#62399=CARTESIAN_POINT('Ctrl Pts',(-19.435236168815,-38.508139330193,122.206096194811)) ;
#62400=CARTESIAN_POINT('Ctrl Pts',(-19.181862671313,-38.6980387188739,121.921702009282)) ;
#62401=CARTESIAN_POINT('Ctrl Pts',(-19.2273466015253,-38.5180496385111,
122.219725252916)) ;
#62402=CARTESIAN_POINT('Ctrl Pts',(-18.9280968782032,-38.7079736160098,
121.98309499747)) ;
#62403=CARTESIAN_POINT('Ctrl Pts',(-19.0243343132026,-38.5279845356469,
122.268838827757)) ;
#62404=CARTESIAN_POINT('Ctrl Pts',(-18.6864010149185,-38.7180146989524,
122.088952068271)) ;
#62405=CARTESIAN_POINT('Ctrl Pts',(-18.830977224545,-38.5380256185895,122.353523948551)) ;
#62406=CARTESIAN_POINT('Ctrl Pts',(-18.4700029594323,-38.7279020417806,
122.232792348805)) ;
#62407=CARTESIAN_POINT('Ctrl Pts',(-18.6578590879055,-38.5479129614178,
122.468595134658)) ;
#62408=CARTESIAN_POINT('Ctrl Pts',(-18.2795943518185,-38.73789355672,122.413563464237)) ;
#62409=CARTESIAN_POINT('Ctrl Pts',(-18.5055317681181,-38.5579044763571,
122.613211332423)) ;
#62410=CARTESIAN_POINT('Ctrl Pts',(-18.1241690742749,-38.7478449479164,
122.623883939098)) ;
#62411=CARTESIAN_POINT('Ctrl Pts',(-18.3811911759621,-38.5678558675536,
122.781466905472)) ;
#62412=CARTESIAN_POINT('Ctrl Pts',(-18.0074429397806,-38.7577774812491,
122.857344924824)) ;
#62413=CARTESIAN_POINT('Ctrl Pts',(-18.2878097133205,-38.5777884008862,
122.968234824021)) ;
#62414=CARTESIAN_POINT('Ctrl Pts',(-17.9324451631841,-38.7677746391485,
123.109116894518)) ;
#62415=CARTESIAN_POINT('Ctrl Pts',(-18.2278106582551,-38.5877855587856,
123.1696520247)) ;
#62416=CARTESIAN_POINT('Ctrl Pts',(-17.9022350151,-38.777759649312,123.369808873099)) ;
#62417=CARTESIAN_POINT('Ctrl Pts',(-18.2036416362819,-38.5977705689491,
123.378205317584)) ;
#62418=CARTESIAN_POINT('Ctrl Pts',(-17.918220476194,-38.7878024758818,123.633203162121)) ;
#62419=CARTESIAN_POINT('Ctrl Pts',(-18.2164291783058,-38.6078133955189,
123.588920944231)) ;
#62420=CARTESIAN_POINT('Ctrl Pts',(-17.9778363800637,-38.7976327101868,
123.884601181613)) ;
#62421=CARTESIAN_POINT('Ctrl Pts',(-18.2641206846296,-38.6176436298239,
123.790038464492)) ;
#62422=CARTESIAN_POINT('Ctrl Pts',(-18.0826097273411,-38.8077087354214,
124.127718361036)) ;
#62423=CARTESIAN_POINT('Ctrl Pts',(-18.3479385732616,-38.6277196550586,
123.984532923754)) ;
#62424=CARTESIAN_POINT('Ctrl Pts',(-18.22472296995,-38.8175609719123,124.344203206639)) ;
#62425=CARTESIAN_POINT('Ctrl Pts',(-18.4616277604428,-38.6375718915494,
124.157720543777)) ;
#62426=CARTESIAN_POINT('Ctrl Pts',(-18.4060166292549,-38.8276341783464,
124.537031920896)) ;
#62427=CARTESIAN_POINT('Ctrl Pts',(-18.6066621150346,-38.6476450979836,
124.311984493962)) ;
#62428=CARTESIAN_POINT('Ctrl Pts',(-18.6132523458117,-38.8374756878536,
124.691787453132)) ;
#62429=CARTESIAN_POINT('Ctrl Pts',(-18.7724492132766,-38.6574866074907,
124.435789153201)) ;
#62430=CARTESIAN_POINT('Ctrl Pts',(-18.8465449135048,-38.8474366346334,
124.810489310294)) ;
#62431=CARTESIAN_POINT('Ctrl Pts',(-18.9590823935704,-38.6674475542705,
124.530751641621)) ;
#62432=CARTESIAN_POINT('Ctrl Pts',(-19.0989906357663,-38.8574744634334,
124.886965770252)) ;
#62433=CARTESIAN_POINT('Ctrl Pts',(-19.1610387331382,-38.6774853830706,
124.591933962578)) ;
#62434=CARTESIAN_POINT('Ctrl Pts',(-19.3565960865171,-38.8673487731879,
124.918417832295)) ;
#62435=CARTESIAN_POINT('Ctrl Pts',(-19.3671221354591,-38.687359692825,124.617096782375)) ;
#62436=CARTESIAN_POINT('Ctrl Pts',(-19.620809364879,-38.8774184708611,124.90438027923)) ;
#62437=CARTESIAN_POINT('Ctrl Pts',(-19.5784931043603,-38.6974293904982,
124.605867998489)) ;
#62438=CARTESIAN_POINT('Ctrl Pts',(-19.8726090818737,-38.8872519421485,
124.846200103951)) ;
#62439=CARTESIAN_POINT('Ctrl Pts',(-19.779932174487,-38.7072628617856,124.559325358216)) ;
#62440=CARTESIAN_POINT('Ctrl Pts',(-20.1154997478902,-38.8972815886784,
124.743876964785)) ;
#62441=CARTESIAN_POINT('Ctrl Pts',(-19.9742453375795,-38.7172925083155,
124.477468165888)) ;
#62442=CARTESIAN_POINT('Ctrl Pts',(-20.336613329244,-38.9073161030058,124.600184240686)) ;
#62443=CARTESIAN_POINT('Ctrl Pts',(-20.1511369670628,-38.7273270226429,
124.362515034824)) ;
#62444=CARTESIAN_POINT('Ctrl Pts',(-20.525819561072,-38.9171413884767,124.424489904963)) ;
#62445=CARTESIAN_POINT('Ctrl Pts',(-20.3025021660536,-38.7371523081138,
124.221961312577)) ;
#62446=CARTESIAN_POINT('Ctrl Pts',(-20.684908264894,-38.9271456300252,124.215225042705)) ;
#62447=CARTESIAN_POINT('Ctrl Pts',(-20.4297743088031,-38.7471565496623,
124.054550406334)) ;
#62448=CARTESIAN_POINT('Ctrl Pts',(-20.8049240326916,-38.9371282751043,
123.981897983475)) ;
#62449=CARTESIAN_POINT('Ctrl Pts',(-20.5257881879668,-38.7571391947414,
123.867889603181)) ;
#62450=CARTESIAN_POINT('Ctrl Pts',(-20.8827806719574,-38.9471734721958,
123.729693087427)) ;
#62451=CARTESIAN_POINT('Ctrl Pts',(-20.5880749231069,-38.7671843918329,
123.666125997018)) ;
#62452=CARTESIAN_POINT('Ctrl Pts',(-20.915373446422,-38.9569965879559,123.473607472964)) ;
#62453=CARTESIAN_POINT('Ctrl Pts',(-20.6141505414293,-38.7770075075931,
123.461258688752)) ;
#62454=CARTESIAN_POINT('Ctrl Pts',(-20.9034051256726,-38.9670311997562,
123.210183840102)) ;
#62455=CARTESIAN_POINT('Ctrl Pts',(-20.6045775434522,-38.7870421193933,
123.250519622744)) ;
#62456=CARTESIAN_POINT('Ctrl Pts',(-20.8452141569218,-38.9770562085294,
122.953236014192)) ;
#62457=CARTESIAN_POINT('Ctrl Pts',(-20.5580262508377,-38.7970671281665,
123.044961006179)) ;
#62458=CARTESIAN_POINT('Ctrl Pts',(-20.7455751866615,-38.9869081333709,
122.714273478739)) ;
#62459=CARTESIAN_POINT('Ctrl Pts',(-20.4783168903162,-38.8069190530081,
122.853791094508)) ;
#62460=CARTESIAN_POINT('Ctrl Pts',(-20.6043472152323,-38.9968990716936,
122.492979055733)) ;
#62461=CARTESIAN_POINT('Ctrl Pts',(-20.3653360237467,-38.8169099913308,
122.676754754454)) ;
#62462=CARTESIAN_POINT('Ctrl Pts',(-20.4282184151075,-39.0068170568401,
122.300819554238)) ;
#62463=CARTESIAN_POINT('Ctrl Pts',(-20.2244345676972,-38.8268279764772,
122.523026321021)) ;
#62464=CARTESIAN_POINT('Ctrl Pts',(-20.2191838999621,-39.0168451577356,
122.140380206335)) ;
#62465=CARTESIAN_POINT('Ctrl Pts',(-20.0572079946836,-38.8368560773727,
122.394673443587)) ;
#62466=CARTESIAN_POINT('Ctrl Pts',(-19.988823563365,-39.0267303986782,122.020299045368)) ;
#62467=CARTESIAN_POINT('Ctrl Pts',(-19.8729210602191,-38.8467413183153,
122.298607226252)) ;
#62468=CARTESIAN_POINT('Ctrl Pts',(-19.7387023265392,-39.0367195116448,
121.940602617723)) ;
#62469=CARTESIAN_POINT('Ctrl Pts',(-19.6728247564175,-38.8567304312819,
122.234848346961)) ;
#62470=CARTESIAN_POINT('Ctrl Pts',(-19.477101074724,-39.0467615759856,121.905935512538)) ;
#62471=CARTESIAN_POINT('Ctrl Pts',(-19.4635439135823,-38.8667724956227,
122.207112896485)) ;
#62472=CARTESIAN_POINT('Ctrl Pts',(-19.2190051557775,-39.0565907773901,
121.91648957557)) ;
#62473=CARTESIAN_POINT('Ctrl Pts',(-19.2570678745084,-38.8766016970272,
122.215554268652)) ;
#62474=CARTESIAN_POINT('Ctrl Pts',(-18.96201942726,-39.0665976181483,121.972124528539)) ;
#62475=CARTESIAN_POINT('Ctrl Pts',(-19.0514789416566,-38.8866085377854,
122.260060324957)) ;
#62476=CARTESIAN_POINT('Ctrl Pts',(-18.7190580246925,-39.0765851423402,
122.071516726106)) ;
#62477=CARTESIAN_POINT('Ctrl Pts',(-18.8571092146858,-38.8965960619773,
122.339572267112)) ;
#62478=CARTESIAN_POINT('Ctrl Pts',(-18.4962632862226,-39.0866147881488,
122.21229469891)) ;
#62479=CARTESIAN_POINT('Ctrl Pts',(-18.6788723982506,-38.9066257077859,
122.452193065279)) ;
#62480=CARTESIAN_POINT('Ctrl Pts',(-18.3040742602747,-39.0964888188876,
122.386670421096)) ;
#62481=CARTESIAN_POINT('Ctrl Pts',(-18.5251202815215,-38.9164997385247,
122.591691852851)) ;
#62482=CARTESIAN_POINT('Ctrl Pts',(-18.142850412755,-39.1064881417517,122.594116058602)) ;
#62483=CARTESIAN_POINT('Ctrl Pts',(-18.3961396994837,-38.9264990613888,
122.757647081838)) ;
#62484=CARTESIAN_POINT('Ctrl Pts',(-18.0209136491181,-39.1163989773273,
122.824305926561)) ;
#62485=CARTESIAN_POINT('Ctrl Pts',(-18.2985886964444,-38.9364098969644,
122.941797703191)) ;
#62486=CARTESIAN_POINT('Ctrl Pts',(-17.939756418586,-39.1264532253013,123.075703741562)) ;
#62487=CARTESIAN_POINT('Ctrl Pts',(-18.2336609864209,-38.9464641449384,
123.142915426417)) ;
#62488=CARTESIAN_POINT('Ctrl Pts',(-17.9038739773889,-39.136311969564,123.332330097261)) ;
#62489=CARTESIAN_POINT('Ctrl Pts',(-18.2049530965617,-38.9563228892011,
123.348215715669)) ;
#62490=CARTESIAN_POINT('Ctrl Pts',(-17.9131303556298,-39.146380055637,123.596708290308)) ;
#62491=CARTESIAN_POINT('Ctrl Pts',(-18.2123561545412,-38.9663909752741,
123.559718464088)) ;
#62492=CARTESIAN_POINT('Ctrl Pts',(-17.9670211523186,-39.1562355388165,
123.850053708663)) ;
#62493=CARTESIAN_POINT('Ctrl Pts',(-18.2554666875822,-38.9762464584537,
123.762394736116)) ;
#62494=CARTESIAN_POINT('Ctrl Pts',(-18.0647131560755,-39.1662303846107,
124.093854715308)) ;
#62495=CARTESIAN_POINT('Ctrl Pts',(-18.3336182833703,-38.9862413042478,
123.957436260119)) ;
#62496=CARTESIAN_POINT('Ctrl Pts',(-18.2042478281487,-39.1762616802733,
124.31751521221)) ;
#62497=CARTESIAN_POINT('Ctrl Pts',(-18.4452442635705,-38.9962725999104,
124.136365752348)) ;
#62498=CARTESIAN_POINT('Ctrl Pts',(-18.3772981542013,-39.1861282235631,
124.510610102635)) ;
#62499=CARTESIAN_POINT('Ctrl Pts',(-18.5836826763418,-39.0061391432003,
124.290842767909)) ;
#62500=CARTESIAN_POINT('Ctrl Pts',(-18.5834523133935,-39.1961156193265,
124.672993813445)) ;
#62501=CARTESIAN_POINT('Ctrl Pts',(-18.7486045943314,-39.0161265389636,
124.420751367233)) ;
#62502=CARTESIAN_POINT('Ctrl Pts',(-18.8136849281219,-39.2060606600565,
124.796745724654)) ;
#62503=CARTESIAN_POINT('Ctrl Pts',(-18.9327894986595,-39.0260715796936,
124.519754710555)) ;
#62504=CARTESIAN_POINT('Ctrl Pts',(-19.0643744385041,-39.2161051662732,
124.879300115833)) ;
#62505=CARTESIAN_POINT('Ctrl Pts',(-19.1333404484933,-39.0361160859103,
124.585800271082)) ;
#62506=CARTESIAN_POINT('Ctrl Pts',(-19.3209006976939,-39.2259686724105,
124.916631731165)) ;
#62507=CARTESIAN_POINT('Ctrl Pts',(-19.3385608066028,-39.0459795920477,
124.61566765999)) ;
#62508=CARTESIAN_POINT('Ctrl Pts',(-19.5833595972504,-39.2359615332466,
124.909220187151)) ;
#62509=CARTESIAN_POINT('Ctrl Pts',(-19.5485279119773,-39.0559724528837,
124.609740630112)) ;
#62510=CARTESIAN_POINT('Ctrl Pts',(-19.838927622203,-39.2458877269655,124.856807196961)) ;
#62511=CARTESIAN_POINT('Ctrl Pts',(-19.7529826014343,-39.0658986466027,
124.567812433635)) ;
#62512=CARTESIAN_POINT('Ctrl Pts',(-20.0837340012441,-39.2559066529981,
124.759990302351)) ;
#62513=CARTESIAN_POINT('Ctrl Pts',(-19.9488284801805,-39.0759175726352,
124.490360989848)) ;
#62514=CARTESIAN_POINT('Ctrl Pts',(-20.3058732169499,-39.2658216523657,
124.623740322462)) ;
#62515=CARTESIAN_POINT('Ctrl Pts',(-20.1265408661882,-39.0858325720028,
124.381362989768)) ;
#62516=CARTESIAN_POINT('Ctrl Pts',(-20.5036398438425,-39.275876423923,124.448561261991)) ;
#62517=CARTESIAN_POINT('Ctrl Pts',(-20.2847556360216,-39.0958873435601,
124.241221409002)) ;
#62518=CARTESIAN_POINT('Ctrl Pts',(-20.6649559413948,-39.2857353862206,
124.245785908657)) ;
#62519=CARTESIAN_POINT('Ctrl Pts',(-20.4138101229452,-39.1057463058577,
124.079002680325)) ;
#62520=CARTESIAN_POINT('Ctrl Pts',(-20.7907073337683,-39.2957296300584,
124.015257630016)) ;
#62521=CARTESIAN_POINT('Ctrl Pts',(-20.5144131818237,-39.1157405496955,
123.894581187682)) ;
#62522=CARTESIAN_POINT('Ctrl Pts',(-20.8740852786362,-39.3056548594826,
123.76807558954)) ;
#62523=CARTESIAN_POINT('Ctrl Pts',(-20.5811176317263,-39.1256657791198,
123.696836372389)) ;
#62524=CARTESIAN_POINT('Ctrl Pts',(-20.9136831801555,-39.3156828233741,
123.507578576389)) ;
#62525=CARTESIAN_POINT('Ctrl Pts',(-20.6127981700986,-39.1356937430112,
123.488439150127)) ;
#62526=CARTESIAN_POINT('Ctrl Pts',(-20.9078028794062,-39.3255690830045,
123.247805458002)) ;
#62527=CARTESIAN_POINT('Ctrl Pts',(-20.6080961812906,-39.1455800026416,
123.280620698185)) ;
#62528=CARTESIAN_POINT('Ctrl Pts',(-20.8563083055305,-39.3356008460823,
122.989304179214)) ;
#62529=CARTESIAN_POINT('Ctrl Pts',(-20.5669027458931,-39.1556117657195,
123.07381928786)) ;
#62530=CARTESIAN_POINT('Ctrl Pts',(-20.7623452754649,-39.3454824723765,
122.747171858518)) ;
#62531=CARTESIAN_POINT('Ctrl Pts',(-20.4917344390515,-39.1654933920136,
122.880112663831)) ;
#62532=CARTESIAN_POINT('Ctrl Pts',(-20.6254181998426,-39.3555442418626,
122.521020260046)) ;
#62533=CARTESIAN_POINT('Ctrl Pts',(-20.3821947440194,-39.1755551614998,
122.699190275451)) ;
#62534=CARTESIAN_POINT('Ctrl Pts',(-20.4548438165245,-39.3654021093581,
122.326007790114)) ;
#62535=CARTESIAN_POINT('Ctrl Pts',(-20.2457369371644,-39.1854130289952,
122.543178822639)) ;
#62536=CARTESIAN_POINT('Ctrl Pts',(-20.2506752048756,-39.3753937344755,
122.160957633342)) ;
#62537=CARTESIAN_POINT('Ctrl Pts',(-20.0824034879034,-39.1954046541126,
122.41113697398)) ;
#62538=CARTESIAN_POINT('Ctrl Pts',(-20.0221459359135,-39.3853305335837,
122.034581725534)) ;
#62539=CARTESIAN_POINT('Ctrl Pts',(-19.8995811564876,-39.2053414532208,
122.310034285515)) ;
#62540=CARTESIAN_POINT('Ctrl Pts',(-19.7739378812529,-39.3953213631411,
121.948989845805)) ;
#62541=CARTESIAN_POINT('Ctrl Pts',(-19.7010154745598,-39.2153322827782,
122.241558685224)) ;
#62542=CARTESIAN_POINT('Ctrl Pts',(-19.5137457792809,-39.4053445988542,
121.90796320333)) ;
#62543=CARTESIAN_POINT('Ctrl Pts',(-19.4928622206853,-39.2253555184914,
122.208735172086)) ;
#62544=CARTESIAN_POINT('Ctrl Pts',(-19.2537240353539,-39.4152409468834,
121.912457737756)) ;
#62545=CARTESIAN_POINT('Ctrl Pts',(-19.284844725392,-39.2352518665205,122.212328561207)) ;
#62546=CARTESIAN_POINT('Ctrl Pts',(-18.9959028450578,-39.4252305093859,
121.961952758598)) ;
#62547=CARTESIAN_POINT('Ctrl Pts',(-19.0785873514741,-39.245241429023,122.251922433717)) ;
#62548=CARTESIAN_POINT('Ctrl Pts',(-18.7495601440801,-39.4352708170704,
122.056425100597)) ;
#62549=CARTESIAN_POINT('Ctrl Pts',(-18.8815126089877,-39.2552817367076,
122.327498082193)) ;
#62550=CARTESIAN_POINT('Ctrl Pts',(-18.5275396488835,-39.4451131204176,
122.189149904879)) ;
#62551=CARTESIAN_POINT('Ctrl Pts',(-18.7038944864329,-39.2651240400548,
122.433676503167)) ;
#62552=CARTESIAN_POINT('Ctrl Pts',(-18.3281491908963,-39.4551368286967,
122.361220908179)) ;
#62553=CARTESIAN_POINT('Ctrl Pts',(-18.544382291125,-39.2751477483338,122.571330259957)) ;
#62554=CARTESIAN_POINT('Ctrl Pts',(-18.1083641388758,-39.4683590061644,
122.630415698339)) ;
#62555=CARTESIAN_POINT('Ctrl Pts',(-18.3685442466138,-39.2883699258015,
122.786691064912)) ;
#62556=CARTESIAN_POINT('Ctrl Pts',(-17.9628051141578,-39.4816515912237,
122.952220149241)) ;
#62557=CARTESIAN_POINT('Ctrl Pts',(-18.2520900201739,-39.3016625108608,
123.0441667538)) ;
#62558=CARTESIAN_POINT('Ctrl Pts',(-17.9061735340481,-39.4949364471453,
123.296785705772)) ;
#62559=CARTESIAN_POINT('Ctrl Pts',(-18.2067947639732,-39.3149473667824,
123.319772623799)) ;
#62560=CARTESIAN_POINT('Ctrl Pts',(-17.9090249687646,-39.5049086743181,
123.558791097656)) ;
#62561=CARTESIAN_POINT('Ctrl Pts',(-18.2090712941876,-39.3249195939552,
123.529386330433)) ;
#62562=CARTESIAN_POINT('Ctrl Pts',(-17.956586488933,-39.5148172907571,123.814831513861)) ;
#62563=CARTESIAN_POINT('Ctrl Pts',(-18.2471189493616,-39.3348282103942,
123.734216637461)) ;
#62564=CARTESIAN_POINT('Ctrl Pts',(-18.0492936761947,-39.5248704961408,
124.062190998726)) ;
#62565=CARTESIAN_POINT('Ctrl Pts',(-18.321283555231,-39.3448814157779,123.93210607372)) ;
#62566=CARTESIAN_POINT('Ctrl Pts',(-18.1809125138042,-39.5347356299011,
124.285566478985)) ;
#62567=CARTESIAN_POINT('Ctrl Pts',(-18.4265731937417,-39.3547465495382,
124.110805222555)) ;
#62568=CARTESIAN_POINT('Ctrl Pts',(-18.4080910892468,-39.5480746875274,
124.552496993327)) ;
#62569=CARTESIAN_POINT('Ctrl Pts',(-18.6083336756882,-39.3680856071645,
124.324363766932)) ;
#62570=CARTESIAN_POINT('Ctrl Pts',(-18.7706176279161,-39.5646438748606,
124.802631868927)) ;
#62571=CARTESIAN_POINT('Ctrl Pts',(-18.8983168389849,-39.3846547944977,
124.524458515266)) ;
#62572=CARTESIAN_POINT('Ctrl Pts',(-19.1984775012585,-39.5812890147116,
124.914837427631)) ;
#62573=CARTESIAN_POINT('Ctrl Pts',(-19.2406669700555,-39.4012999343487,
124.614238150144)) ;
#62574=CARTESIAN_POINT('Ctrl Pts',(-19.5473160626107,-39.594561317185,124.912945050677)) ;
#62575=CARTESIAN_POINT('Ctrl Pts',(-19.5196867817272,-39.4145722368221,
124.6127192198)) ;
#62576=CARTESIAN_POINT('Ctrl Pts',(-19.8054003621908,-39.6045422806326,
124.866324423649)) ;
#62577=CARTESIAN_POINT('Ctrl Pts',(-19.7261653890183,-39.4245532002698,
124.575425593905)) ;
#62578=CARTESIAN_POINT('Ctrl Pts',(-20.0506098849888,-39.6144841127019,
124.776085831053)) ;
#62579=CARTESIAN_POINT('Ctrl Pts',(-19.9223292887017,-39.4344950323391,
124.503237755022)) ;
#62580=CARTESIAN_POINT('Ctrl Pts',(-20.3531494019142,-39.6278036819174,
124.600140541929)) ;
#62581=CARTESIAN_POINT('Ctrl Pts',(-20.1643723390079,-39.4478146015545,
124.362474577121)) ;
#62582=CARTESIAN_POINT('Ctrl Pts',(-20.6634916788334,-39.6443338368501,
124.289002055755)) ;
#62583=CARTESIAN_POINT('Ctrl Pts',(-20.4126378083465,-39.4643447564872,
124.11357553459)) ;
#62584=CARTESIAN_POINT('Ctrl Pts',(-20.8878880488286,-39.6643555623422,
123.80663214029)) ;
#62585=CARTESIAN_POINT('Ctrl Pts',(-20.5921614310952,-39.4843664819793,
123.727677884978)) ;
#62586=CARTESIAN_POINT('Ctrl Pts',(-20.9340458411,-39.684166958949,123.281975948021)) ;
#62587=CARTESIAN_POINT('Ctrl Pts',(-20.6290900257531,-39.5041778785861,
123.307952866676)) ;
#62588=CARTESIAN_POINT('Ctrl Pts',(-20.7981256340549,-39.7041522076579,
122.768612564933)) ;
#62589=CARTESIAN_POINT('Ctrl Pts',(-20.5203568572082,-39.524163127295,122.897261068082)) ;
#62590=CARTESIAN_POINT('Ctrl Pts',(-20.4961474222789,-39.7240462702938,
122.334473379802)) ;
#62591=CARTESIAN_POINT('Ctrl Pts',(-20.2787761236903,-39.5440571899309,
122.549947532651)) ;
#62592=CARTESIAN_POINT('Ctrl Pts',(-20.0638627446628,-39.7439779494674,
122.028277249774)) ;
#62593=CARTESIAN_POINT('Ctrl Pts',(-19.9329493834132,-39.5639888691045,
122.304988270493)) ;
#62594=CARTESIAN_POINT('Ctrl Pts',(-19.552105313075,-39.7639420039394,121.888081012904)) ;
#62595=CARTESIAN_POINT('Ctrl Pts',(-19.523543821286,-39.5839529235765,122.192828836387)) ;
#62596=CARTESIAN_POINT('Ctrl Pts',(-19.0253744540023,-39.7838229057023,
121.930361827111)) ;
#62597=CARTESIAN_POINT('Ctrl Pts',(-19.1021578729861,-39.6038338253394,
122.226651390255)) ;
#62598=CARTESIAN_POINT('Ctrl Pts',(-18.5431348409718,-39.8037615673107,
122.150015941344)) ;
#62599=CARTESIAN_POINT('Ctrl Pts',(-18.7163648705892,-39.6237724869478,
122.402373239355)) ;
#62600=CARTESIAN_POINT('Ctrl Pts',(-18.1655278033416,-39.823658092566,122.520218221338)) ;
#62601=CARTESIAN_POINT('Ctrl Pts',(-18.4142773121928,-39.6436690122031,
122.698534606389)) ;
#62602=CARTESIAN_POINT('Ctrl Pts',(-17.9361396477719,-39.8435531310203,
122.99666905445)) ;
#62603=CARTESIAN_POINT('Ctrl Pts',(-18.2307652509137,-39.6635640506575,
123.079695848156)) ;
#62604=CARTESIAN_POINT('Ctrl Pts',(-17.883006132507,-39.8635169543264,123.524568225147)) ;
#62605=CARTESIAN_POINT('Ctrl Pts',(-18.1882574093228,-39.6835278739635,
123.502015493419)) ;
#62606=CARTESIAN_POINT('Ctrl Pts',(-18.0122595317287,-39.8833910784555,
124.036771136618)) ;
#62607=CARTESIAN_POINT('Ctrl Pts',(-18.2916598855057,-39.7034019980926,
123.911779438151)) ;
#62608=CARTESIAN_POINT('Ctrl Pts',(-18.3096308451413,-39.9033661541827,
124.476606505038)) ;
#62609=CARTESIAN_POINT('Ctrl Pts',(-18.5295569287949,-39.7233770738199,
124.263648070586)) ;
#62610=CARTESIAN_POINT('Ctrl Pts',(-18.7392016865621,-39.9233197235393,
124.787593898478)) ;
#62611=CARTESIAN_POINT('Ctrl Pts',(-18.8732138714757,-39.7433306431764,
124.512438635764)) ;
#62612=CARTESIAN_POINT('Ctrl Pts',(-19.245888696071,-39.9431576337272,124.933442271979)) ;
#62613=CARTESIAN_POINT('Ctrl Pts',(-19.278565608068,-39.7631685533643,124.629117598788)) ;
#62614=CARTESIAN_POINT('Ctrl Pts',(-19.7756254405552,-39.9631334622981,
124.897944226643)) ;
#62615=CARTESIAN_POINT('Ctrl Pts',(-19.702355195912,-39.7831443819352,124.600718333619)) ;
#62616=CARTESIAN_POINT('Ctrl Pts',(-20.259776971264,-39.9830515070084,124.68390775287)) ;
#62617=CARTESIAN_POINT('Ctrl Pts',(-20.0896770292724,-39.8030624266455,
124.429488092088)) ;
#62618=CARTESIAN_POINT('Ctrl Pts',(-20.6419438140887,-40.002921752796,124.319255201488)) ;
#62619=CARTESIAN_POINT('Ctrl Pts',(-20.3954104744399,-39.8229326724332,
124.137764014872)) ;
#62620=CARTESIAN_POINT('Ctrl Pts',(-20.8780281936789,-40.0229707558956,
123.841688417852)) ;
#62621=CARTESIAN_POINT('Ctrl Pts',(-20.584276553681,-39.8429816755327,123.755710427859)) ;
#62622=CARTESIAN_POINT('Ctrl Pts',(-20.9367938161444,-40.0427499971364,
123.319128562746)) ;
#62623=CARTESIAN_POINT('Ctrl Pts',(-20.6312875872331,-39.8627609167736,
123.337660188172)) ;
#62624=CARTESIAN_POINT('Ctrl Pts',(-20.8129964068986,-40.0627800608453,
122.801479468829)) ;
#62625=CARTESIAN_POINT('Ctrl Pts',(-20.5322475926192,-39.8827909804824,
122.92354173138)) ;
#62626=CARTESIAN_POINT('Ctrl Pts',(-20.5213204071413,-40.0826623457473,
122.360731282124)) ;
#62627=CARTESIAN_POINT('Ctrl Pts',(-20.2989045254631,-39.9026732653844,
122.570943408871)) ;
#62628=CARTESIAN_POINT('Ctrl Pts',(-20.0977276287473,-40.1025446466403,
122.044872252735)) ;
#62629=CARTESIAN_POINT('Ctrl Pts',(-19.9600279171563,-39.9225555662774,
122.31825773152)) ;
#62630=CARTESIAN_POINT('Ctrl Pts',(-19.5891047472004,-40.1225277562586,
121.891899364651)) ;
#62631=CARTESIAN_POINT('Ctrl Pts',(-19.5531287369363,-39.9425386758957,
122.195882009548)) ;
#62632=CARTESIAN_POINT('Ctrl Pts',(-19.0612514000338,-40.1424181516365,
121.921603035673)) ;
#62633=CARTESIAN_POINT('Ctrl Pts',(-19.1308454119986,-39.9624290712736,
122.219647817995)) ;
#62634=CARTESIAN_POINT('Ctrl Pts',(-18.5748477163413,-40.1623149416708,
122.128947492388)) ;
#62635=CARTESIAN_POINT('Ctrl Pts',(-18.7417230650517,-39.9823258613079,
122.385526589855)) ;
#62636=CARTESIAN_POINT('Ctrl Pts',(-18.1875342172556,-40.1822319956124,
122.489841093225)) ;
#62637=CARTESIAN_POINT('Ctrl Pts',(-18.4318742437841,-40.0022429152495,
122.674244288826)) ;
#62638=CARTESIAN_POINT('Ctrl Pts',(-17.9457158456868,-40.2022355438159,
122.963405930333)) ;
#62639=CARTESIAN_POINT('Ctrl Pts',(-18.2384227101736,-40.022246463453,123.05309765344)) ;
#62640=CARTESIAN_POINT('Ctrl Pts',(-17.8810209349113,-40.2221738374685,
123.489343815251)) ;
#62641=CARTESIAN_POINT('Ctrl Pts',(-18.1866699625709,-40.0421847571056,
123.473848687239)) ;
#62642=CARTESIAN_POINT('Ctrl Pts',(-17.9977400537545,-40.2419953249014,
124.003081008329)) ;
#62643=CARTESIAN_POINT('Ctrl Pts',(-18.2800496556778,-40.0620062445386,
123.884838604969)) ;
#62644=CARTESIAN_POINT('Ctrl Pts',(-18.2845312148424,-40.2619737178923,
124.449892679348)) ;
#62645=CARTESIAN_POINT('Ctrl Pts',(-18.5094838885054,-40.0819846375294,
124.242285370891)) ;
#62646=CARTESIAN_POINT('Ctrl Pts',(-18.7051945465058,-40.281872099506,124.770559205405)) ;
#62647=CARTESIAN_POINT('Ctrl Pts',(-18.8460248106455,-40.1018830191431,
124.498817503231)) ;
#62648=CARTESIAN_POINT('Ctrl Pts',(-19.1255703487818,-40.2984550302359,
124.902674539461)) ;
#62649=CARTESIAN_POINT('Ctrl Pts',(-19.1823032071528,-40.118465949873,124.604500927526)) ;
#62650=CARTESIAN_POINT('Ctrl Pts',(-19.4741295857763,-40.3117292658247,
124.917986772684)) ;
#62651=CARTESIAN_POINT('Ctrl Pts',(-19.461172160329,-40.1317401854619,124.616752617202)) ;
#62652=CARTESIAN_POINT('Ctrl Pts',(-19.7358425463294,-40.3217756832809,
124.883469686194)) ;
#62653=CARTESIAN_POINT('Ctrl Pts',(-19.6705356336101,-40.1417866029181,
124.589137624141)) ;
#62654=CARTESIAN_POINT('Ctrl Pts',(-19.9826774778135,-40.3316209085002,
124.805881778584)) ;
#62655=CARTESIAN_POINT('Ctrl Pts',(-19.8680131815929,-40.1516318281373,
124.527058888594)) ;
#62656=CARTESIAN_POINT('Ctrl Pts',(-20.293982933582,-40.3449558795396,124.645032731908)) ;
#62657=CARTESIAN_POINT('Ctrl Pts',(-20.117012406976,-40.1649667991767,124.398409704518)) ;
#62658=CARTESIAN_POINT('Ctrl Pts',(-20.6198884114383,-40.3615387363322,
124.348182656226)) ;
#62659=CARTESIAN_POINT('Ctrl Pts',(-20.3777873723934,-40.1815496559694,
124.160882593775)) ;
#62660=CARTESIAN_POINT('Ctrl Pts',(-20.8256972515988,-40.3781817386816,
123.956743051151)) ;
#62661=CARTESIAN_POINT('Ctrl Pts',(-20.5424028051594,-40.1981926583188,
123.84776904717)) ;
#62662=CARTESIAN_POINT('Ctrl Pts',(-20.9027340822747,-40.3914254697133,
123.617264907875)) ;
#62663=CARTESIAN_POINT('Ctrl Pts',(-20.6040438274232,-40.2114363893504,
123.576158441857)) ;
#62664=CARTESIAN_POINT('Ctrl Pts',(-20.9155780417739,-40.4014798643879,
123.353409333891)) ;
#62665=CARTESIAN_POINT('Ctrl Pts',(-20.6143139039399,-40.221490784025,123.365079497654)) ;
#62666=CARTESIAN_POINT('Ctrl Pts',(-20.8834362366564,-40.4113209257765,
123.096754250363)) ;
#62667=CARTESIAN_POINT('Ctrl Pts',(-20.5885990123171,-40.2313318454136,
123.159754036855)) ;
#62668=CARTESIAN_POINT('Ctrl Pts',(-20.805749324976,-40.421387150133,122.843935791926)) ;
#62669=CARTESIAN_POINT('Ctrl Pts',(-20.5264471820404,-40.2413980697701,
122.957500455723)) ;
#62670=CARTESIAN_POINT('Ctrl Pts',(-20.6874567828035,-40.4312677630526,
122.61274782886)) ;
#62671=CARTESIAN_POINT('Ctrl Pts',(-20.431811178883,-40.2512786826897,122.77255090532)) ;
#62672=CARTESIAN_POINT('Ctrl Pts',(-20.5294818312083,-40.4412610562122,
122.403016184153)) ;
#62673=CARTESIAN_POINT('Ctrl Pts',(-20.3054294355456,-40.2612719758493,
122.604767012198)) ;
#62674=CARTESIAN_POINT('Ctrl Pts',(-20.3383061144584,-40.4512120644359,
122.224524733115)) ;
#62675=CARTESIAN_POINT('Ctrl Pts',(-20.1524873435744,-40.271222984073,122.461975496637)) ;
#62676=CARTESIAN_POINT('Ctrl Pts',(-20.116847152072,-40.4612605787978,122.080752823443)) ;
#62677=CARTESIAN_POINT('Ctrl Pts',(-19.9753190159199,-40.281271498435,122.34695989764)) ;
#62678=CARTESIAN_POINT('Ctrl Pts',(-19.8788615309096,-40.4711020848605,
121.979450513905)) ;
#62679=CARTESIAN_POINT('Ctrl Pts',(-19.7849296059222,-40.2911130044976,
122.265920106906)) ;
#62680=CARTESIAN_POINT('Ctrl Pts',(-19.623405666514,-40.4810877374902,121.919608247054)) ;
#62681=CARTESIAN_POINT('Ctrl Pts',(-19.5805644621411,-40.3010986571273,
122.218048512511)) ;
#62682=CARTESIAN_POINT('Ctrl Pts',(-19.3625879444289,-40.4910267463351,
121.904994593026)) ;
#62683=CARTESIAN_POINT('Ctrl Pts',(-19.3719102147239,-40.3110376659722,
122.206359844841)) ;
#62684=CARTESIAN_POINT('Ctrl Pts',(-19.1006071741867,-40.5010676716281,
121.936267236992)) ;
#62685=CARTESIAN_POINT('Ctrl Pts',(-19.1623259175616,-40.3210785912652,
122.231380198729)) ;
#62686=CARTESIAN_POINT('Ctrl Pts',(-18.8517347176778,-40.510957993383,122.011275192603)) ;
#62687=CARTESIAN_POINT('Ctrl Pts',(-18.9632286807816,-40.3309689130201,
122.291388701103)) ;
#62688=CARTESIAN_POINT('Ctrl Pts',(-18.6170528304471,-40.5209539667164,
122.129240595666)) ;
#62689=CARTESIAN_POINT('Ctrl Pts',(-18.775484242593,-40.3409648863536,122.385763008815)) ;
#62690=CARTESIAN_POINT('Ctrl Pts',(-18.4077408551288,-40.5308853662985,
122.285152304524)) ;
#62691=CARTESIAN_POINT('Ctrl Pts',(-18.6080360869343,-40.3508962859356,
122.510494122467)) ;
#62692=CARTESIAN_POINT('Ctrl Pts',(-18.2270702114119,-40.5408909067755,
122.476201697503)) ;
#62693=CARTESIAN_POINT('Ctrl Pts',(-18.463501244713,-40.3609018264127,122.663335132753)) ;
#62694=CARTESIAN_POINT('Ctrl Pts',(-18.0823350470843,-40.5509238907068,
122.696568451517)) ;
#62695=CARTESIAN_POINT('Ctrl Pts',(-18.3477150174073,-40.370934810344,122.839629750178)) ;
#62696=CARTESIAN_POINT('Ctrl Pts',(-17.9794720037659,-40.5607795215337,
122.934283776559)) ;
#62697=CARTESIAN_POINT('Ctrl Pts',(-18.2654267150485,-40.3807904411708,
123.029802727258)) ;
#62698=CARTESIAN_POINT('Ctrl Pts',(-17.9182550889907,-40.5707789237268,
123.189781090327)) ;
#62699=CARTESIAN_POINT('Ctrl Pts',(-18.2164553726085,-40.390789843364,123.234201028577)) ;
#62700=CARTESIAN_POINT('Ctrl Pts',(-17.9021932202681,-40.5806733930879,
123.44934937898)) ;
#62701=CARTESIAN_POINT('Ctrl Pts',(-18.2036080982215,-40.400684312725,123.441855585745)) ;
#62702=CARTESIAN_POINT('Ctrl Pts',(-17.932011300945,-40.5907365072521,123.712065167649)) ;
#62703=CARTESIAN_POINT('Ctrl Pts',(-18.2274647737821,-40.4107474268893,
123.65202799485)) ;
#62704=CARTESIAN_POINT('Ctrl Pts',(-18.0050786320666,-40.6005761529685,
123.960147159055)) ;
#62705=CARTESIAN_POINT('Ctrl Pts',(-18.2859206557208,-40.4205870726056,
123.850492648776)) ;
#62706=CARTESIAN_POINT('Ctrl Pts',(-18.122387240134,-40.6106393205242,124.197113300157)) ;
#62707=CARTESIAN_POINT('Ctrl Pts',(-18.3797695138113,-40.4306502401614,
124.04006462666)) ;
#62708=CARTESIAN_POINT('Ctrl Pts',(-18.2766451104993,-40.6205335763191,
124.406457589584)) ;
#62709=CARTESIAN_POINT('Ctrl Pts',(-18.5031774204624,-40.4405444959563,
124.207538542366)) ;
#62710=CARTESIAN_POINT('Ctrl Pts',(-18.4652776966857,-40.6304753547788,
124.587171422744)) ;
#62711=CARTESIAN_POINT('Ctrl Pts',(-18.6540848187046,-40.4504862744159,
124.352107914679)) ;
#62712=CARTESIAN_POINT('Ctrl Pts',(-18.6837565652639,-40.640478047609,124.733392656185)) ;
#62713=CARTESIAN_POINT('Ctrl Pts',(-18.8288690428585,-40.4604889672461,
124.469083093928)) ;
#62714=CARTESIAN_POINT('Ctrl Pts',(-18.9251772147638,-40.6505120695628,
124.839403238279)) ;
#62715=CARTESIAN_POINT('Ctrl Pts',(-19.0220064463768,-40.4705229891999,
124.553889578956)) ;
#62716=CARTESIAN_POINT('Ctrl Pts',(-19.176509623626,-40.6603598606518,124.901116406676)) ;
#62717=CARTESIAN_POINT('Ctrl Pts',(-19.2230724433567,-40.480370780289,124.603257935975)) ;
#62718=CARTESIAN_POINT('Ctrl Pts',(-19.4381766703649,-40.6703413852009,
124.919060383607)) ;
#62719=CARTESIAN_POINT('Ctrl Pts',(-19.4324060828598,-40.490352304838,124.617611036855)) ;
#62720=CARTESIAN_POINT('Ctrl Pts',(-19.6981676204706,-40.6802906086918,
124.891345054652)) ;
#62721=CARTESIAN_POINT('Ctrl Pts',(-19.6403984071711,-40.5003015283289,
124.595436730586)) ;
#62722=CARTESIAN_POINT('Ctrl Pts',(-19.9507242764533,-40.6902882649084,
124.818869487459)) ;
#62723=CARTESIAN_POINT('Ctrl Pts',(-19.8424430882566,-40.5102991845455,
124.537454338467)) ;
#62724=CARTESIAN_POINT('Ctrl Pts',(-20.1876076661773,-40.7003284779634,
124.702714148648)) ;
#62725=CARTESIAN_POINT('Ctrl Pts',(-20.0319489184708,-40.5203393976006,
124.444528159668)) ;
#62726=CARTESIAN_POINT('Ctrl Pts',(-20.39657947432,-40.7101565252397,124.550916691026)) ;
#62727=CARTESIAN_POINT('Ctrl Pts',(-20.1991246693014,-40.5301674448768,
124.323088910881)) ;
#62728=CARTESIAN_POINT('Ctrl Pts',(-20.5804267072164,-40.7202108722721,
124.361171005036)) ;
#62729=CARTESIAN_POINT('Ctrl Pts',(-20.346201090862,-40.5402217919092,124.171290919494)) ;
#62730=CARTESIAN_POINT('Ctrl Pts',(-20.7265146724235,-40.7301520086006,
124.144583500037)) ;
#62731=CARTESIAN_POINT('Ctrl Pts',(-20.4630696218111,-40.5501629282377,
123.998019996052)) ;
#62732=CARTESIAN_POINT('Ctrl Pts',(-20.833118168353,-40.7400562416803,123.907137322024)) ;
#62733=CARTESIAN_POINT('Ctrl Pts',(-20.5483504786271,-40.5600671613174,
123.808062650785)) ;
#62734=CARTESIAN_POINT('Ctrl Pts',(-20.8976239886845,-40.7501029385239,
123.651145500443)) ;
#62735=CARTESIAN_POINT('Ctrl Pts',(-20.5999532571857,-40.5701138581611,
123.603268634691)) ;
#62736=CARTESIAN_POINT('Ctrl Pts',(-20.9166549329738,-40.7599984898042,
123.391755647878)) ;
#62737=CARTESIAN_POINT('Ctrl Pts',(-20.6151760608745,-40.5800094094413,
123.395757077431)) ;
#62738=CARTESIAN_POINT('Ctrl Pts',(-20.8899239295474,-40.7700605676437,
123.128727559493)) ;
#62739=CARTESIAN_POINT('Ctrl Pts',(-20.5937893272539,-40.5900714872808,
123.18533465587)) ;
#62740=CARTESIAN_POINT('Ctrl Pts',(-20.8196225925667,-40.7799032767398,
122.879777795718)) ;
#62741=CARTESIAN_POINT('Ctrl Pts',(-20.5375466154367,-40.5999141963769,
122.98617602963)) ;
#62742=CARTESIAN_POINT('Ctrl Pts',(-20.7060594583057,-40.7898940089782,
122.643100332516)) ;
#62743=CARTESIAN_POINT('Ctrl Pts',(-20.4466945356706,-40.6099049286153,
122.796834968904)) ;
#62744=CARTESIAN_POINT('Ctrl Pts',(-20.554024482547,-40.799822034207,122.43106134549)) ;
#62745=CARTESIAN_POINT('Ctrl Pts',(-20.3250653085112,-40.6198329538441,
122.627205154481)) ;
#62746=CARTESIAN_POINT('Ctrl Pts',(-20.3666704074435,-40.8098101808575,
122.247223536498)) ;
#62747=CARTESIAN_POINT('Ctrl Pts',(-20.1751809297172,-40.6298211004947,
122.480136252607)) ;
#62748=CARTESIAN_POINT('Ctrl Pts',(-20.1490005900659,-40.8198451986975,
122.098346117619)) ;
#62749=CARTESIAN_POINT('Ctrl Pts',(-20.0010440055564,-40.6398561183346,
122.361035777316)) ;
#62750=CARTESIAN_POINT('Ctrl Pts',(-19.9129860527782,-40.8297099958027,
121.991128079681)) ;
#62751=CARTESIAN_POINT('Ctrl Pts',(-19.8122322768596,-40.6497209154398,
122.275263239916)) ;
#62752=CARTESIAN_POINT('Ctrl Pts',(-19.6596753422036,-40.8396707281588,
121.925143350382)) ;
#62753=CARTESIAN_POINT('Ctrl Pts',(-19.6095835667024,-40.6596816477959,
122.222477106731)) ;
#62754=CARTESIAN_POINT('Ctrl Pts',(-19.3968323127543,-40.8497041905558,
121.904431778563)) ;
#62755=CARTESIAN_POINT('Ctrl Pts',(-19.3993089374676,-40.6697151101929,
122.205909546887)) ;
#62756=CARTESIAN_POINT('Ctrl Pts',(-19.1381719931737,-40.8595897247672,
121.928871855677)) ;
#62757=CARTESIAN_POINT('Ctrl Pts',(-19.1923814686727,-40.6796006444043,
122.225463173289)) ;
#62758=CARTESIAN_POINT('Ctrl Pts',(-18.8832051234913,-40.8696545654472,
121.999096373019)) ;
#62759=CARTESIAN_POINT('Ctrl Pts',(-18.9884082093164,-40.6896654850843,
122.281644418991)) ;
#62760=CARTESIAN_POINT('Ctrl Pts',(-18.6493502439054,-40.8795026971761,
122.110000505807)) ;
#62761=CARTESIAN_POINT('Ctrl Pts',(-18.8013257528878,-40.6995136168132,
122.370368822003)) ;
#62762=CARTESIAN_POINT('Ctrl Pts',(-18.4340900376583,-40.8895301941662,
122.261979815528)) ;
#62763=CARTESIAN_POINT('Ctrl Pts',(-18.6291184182037,-40.7095411138033,
122.49195350058)) ;
#62764=CARTESIAN_POINT('Ctrl Pts',(-18.2489515312442,-40.8995586462113,
122.449550693022)) ;
#62765=CARTESIAN_POINT('Ctrl Pts',(-18.4810087252179,-40.7195695658484,
122.642011378484)) ;
#62766=CARTESIAN_POINT('Ctrl Pts',(-18.1015397641077,-40.9094039127754,
122.662154181766)) ;
#62767=CARTESIAN_POINT('Ctrl Pts',(-18.3630810732943,-40.7294148324125,
122.812094300653)) ;
#62768=CARTESIAN_POINT('Ctrl Pts',(-17.9910357650172,-40.9193945857163,
122.900318312532)) ;
#62769=CARTESIAN_POINT('Ctrl Pts',(-18.2746791939818,-40.7394055053534,
123.002626045039)) ;
#62770=CARTESIAN_POINT('Ctrl Pts',(-17.9238150126673,-40.9294324678048,
123.155391668012)) ;
#62771=CARTESIAN_POINT('Ctrl Pts',(-18.2209040160254,-40.7494433874419,
123.206685215275)) ;
#62772=CARTESIAN_POINT('Ctrl Pts',(-17.9018757959936,-40.9392768382444,
123.413170064838)) ;
#62773=CARTESIAN_POINT('Ctrl Pts',(-18.2033541255179,-40.7592877578816,
123.41290711647)) ;
#62774=CARTESIAN_POINT('Ctrl Pts',(-17.9248387222201,-40.9492616656398,
123.674518463669)) ;
#62775=CARTESIAN_POINT('Ctrl Pts',(-18.2217257460994,-40.7692725852769,
123.621985522676)) ;
#62776=CARTESIAN_POINT('Ctrl Pts',(-17.9924288980122,-40.9592011110451,
123.926859519996)) ;
#62777=CARTESIAN_POINT('Ctrl Pts',(-18.2757990048026,-40.7792120306822,
123.823857616306)) ;
#62778=CARTESIAN_POINT('Ctrl Pts',(-18.1039644977268,-40.969241115331,124.165936540769)) ;
#62779=CARTESIAN_POINT('Ctrl Pts',(-18.3650287084099,-40.7892520349681,
124.015118795446)) ;
#62780=CARTESIAN_POINT('Ctrl Pts',(-18.2528993475112,-40.9791282245166,
124.378873025714)) ;
#62781=CARTESIAN_POINT('Ctrl Pts',(-18.4841771835395,-40.7991391441538,
124.185466648641)) ;
#62782=CARTESIAN_POINT('Ctrl Pts',(-18.4383623409919,-40.9891282844191,
124.564995129704)) ;
#62783=CARTESIAN_POINT('Ctrl Pts',(-18.6325483359507,-40.8091392040562,
124.334363415602)) ;
#62784=CARTESIAN_POINT('Ctrl Pts',(-18.6514890497464,-40.9990457003338,
124.715068772833)) ;
#62785=CARTESIAN_POINT('Ctrl Pts',(-18.8030498870585,-40.8190566199709,
124.454421071669)) ;
#62786=CARTESIAN_POINT('Ctrl Pts',(-18.8904730960395,-41.0090925150746,
124.827199842309)) ;
#62787=CARTESIAN_POINT('Ctrl Pts',(-18.9942377675479,-40.8291034347117,
124.54412495723)) ;
#62788=CARTESIAN_POINT('Ctrl Pts',(-19.1409580665125,-41.0189679922713,
124.895235368087)) ;
#62789=CARTESIAN_POINT('Ctrl Pts',(-19.1946252220464,-40.8389789119084,
124.59855210373)) ;
#62790=CARTESIAN_POINT('Ctrl Pts',(-19.4040773768789,-41.0290240879925,
124.919312459321)) ;
#62791=CARTESIAN_POINT('Ctrl Pts',(-19.4051209742534,-40.8490350076296,
124.617812738242)) ;
#62792=CARTESIAN_POINT('Ctrl Pts',(-19.6632167072632,-41.0389172500076,
124.897783110469)) ;
#62793=CARTESIAN_POINT('Ctrl Pts',(-19.612431616485,-40.8589281696447,124.600588287946)) ;
#62794=CARTESIAN_POINT('Ctrl Pts',(-19.918917313857,-41.0489794860302,124.830551760871)) ;
#62795=CARTESIAN_POINT('Ctrl Pts',(-19.816992096317,-40.8689904056673,124.546802153709)) ;
#62796=CARTESIAN_POINT('Ctrl Pts',(-20.1539134835327,-41.0588239516591,
124.722342924619)) ;
#62797=CARTESIAN_POINT('Ctrl Pts',(-20.0049876465229,-40.8788348712962,
124.460234605023)) ;
#62798=CARTESIAN_POINT('Ctrl Pts',(-20.3695735130956,-41.0687840443633,
124.574029278927)) ;
#62799=CARTESIAN_POINT('Ctrl Pts',(-20.1775149195478,-40.8887949640004,
124.34158324237)) ;
#62800=CARTESIAN_POINT('Ctrl Pts',(-20.5573002807056,-41.0788223333443,
124.388718288801)) ;
#62801=CARTESIAN_POINT('Ctrl Pts',(-20.3276957826536,-40.8988332529814,
124.193333707095)) ;
#62802=CARTESIAN_POINT('Ctrl Pts',(-20.7079273846869,-41.0886956564505,
124.177407956231)) ;
#62803=CARTESIAN_POINT('Ctrl Pts',(-20.4481962954603,-40.9087065760876,
124.024285712482)) ;
#62804=CARTESIAN_POINT('Ctrl Pts',(-20.8217196875643,-41.0987688405356,
123.938460528923)) ;
#62805=CARTESIAN_POINT('Ctrl Pts',(-20.5392295466057,-40.9187797601727,
123.833127110571)) ;
#62806=CARTESIAN_POINT('Ctrl Pts',(-20.8908771120928,-41.1085893528235,
123.689767340494)) ;
#62807=CARTESIAN_POINT('Ctrl Pts',(-20.5945544458289,-40.9286002724607,
123.634173561183)) ;
#62808=CARTESIAN_POINT('Ctrl Pts',(-20.9166985130199,-41.1186673489393,
123.426252975594)) ;
#62809=CARTESIAN_POINT('Ctrl Pts',(-20.615210932042,-40.9386782685765,123.423361632516)) ;
#62810=CARTESIAN_POINT('Ctrl Pts',(-20.8968766070843,-41.1285214239226,
123.167997632845)) ;
#62811=CARTESIAN_POINT('Ctrl Pts',(-20.5993528292853,-40.9485323435597,
123.21675844281)) ;
#62812=CARTESIAN_POINT('Ctrl Pts',(-20.8314512990001,-41.1385853055063,
122.911802236426)) ;
#62813=CARTESIAN_POINT('Ctrl Pts',(-20.5470119442779,-40.9585962251434,
123.011802002189)) ;
#62814=CARTESIAN_POINT('Ctrl Pts',(-20.7244059189189,-41.14846873148,122.675111707094)) ;
#62815=CARTESIAN_POINT('Ctrl Pts',(-20.461375448032,-40.9684796511172,122.822450609287)) ;
#62816=CARTESIAN_POINT('Ctrl Pts',(-20.5765499860383,-41.1584693354011,
122.457899543958)) ;
#62817=CARTESIAN_POINT('Ctrl Pts',(-20.3430903518895,-40.9784802550382,
122.648681253808)) ;
#62818=CARTESIAN_POINT('Ctrl Pts',(-20.3947593959915,-41.168389119739,122.270998373932)) ;
#62819=CARTESIAN_POINT('Ctrl Pts',(-20.1976579864223,-40.9884000393761,
122.499161080854)) ;
#62820=CARTESIAN_POINT('Ctrl Pts',(-20.1805968421938,-41.1784364700958,
122.116644490037)) ;
#62821=CARTESIAN_POINT('Ctrl Pts',(-20.0263275114058,-40.998447389733,122.37567824904)) ;
#62822=CARTESIAN_POINT('Ctrl Pts',(-19.9469565780985,-41.1883138123301,
122.003445575771)) ;
#62823=CARTESIAN_POINT('Ctrl Pts',(-19.8394159581554,-41.0083247319672,
122.285119878453)) ;
#62824=CARTESIAN_POINT('Ctrl Pts',(-19.6924393110652,-41.1983836934047,
121.931197405337)) ;
#62825=CARTESIAN_POINT('Ctrl Pts',(-19.6358017081943,-41.0183946130419,
122.227321635127)) ;
#62826=CARTESIAN_POINT('Ctrl Pts',(-19.4354489668085,-41.2082133986064,
121.904602386854)) ;
#62827=CARTESIAN_POINT('Ctrl Pts',(-19.430210627212,-41.0282243182436,122.206046078659)) ;
#62828=CARTESIAN_POINT('Ctrl Pts',(-19.1716002965813,-41.2182800597728,
121.923118301563)) ;
#62829=CARTESIAN_POINT('Ctrl Pts',(-19.2191313901848,-41.03829097941,122.220859076658)) ;
#62830=CARTESIAN_POINT('Ctrl Pts',(-18.9194385507973,-41.2281702816401,
121.986221032481)) ;
#62831=CARTESIAN_POINT('Ctrl Pts',(-19.0174028771925,-41.0481812012773,
122.271341336615)) ;
#62832=CARTESIAN_POINT('Ctrl Pts',(-18.6794263982386,-41.2381624577503,
122.092694865169)) ;
#62833=CARTESIAN_POINT('Ctrl Pts',(-18.825393369095,-41.0581733773874,122.356520462696)) ;
#62834=CARTESIAN_POINT('Ctrl Pts',(-18.462319115849,-41.2481252878629,122.239006352315)) ;
#62835=CARTESIAN_POINT('Ctrl Pts',(-18.6517079609517,-41.0681362075001,
122.473569619426)) ;
#62836=CARTESIAN_POINT('Ctrl Pts',(-18.2745423237503,-41.2580295002633,
122.419265967195)) ;
#62837=CARTESIAN_POINT('Ctrl Pts',(-18.5014870946545,-41.0780404199004,
122.617776816636)) ;
#62838=CARTESIAN_POINT('Ctrl Pts',(-18.1187135739592,-41.2680902143511,
122.632804079682)) ;
#62839=CARTESIAN_POINT('Ctrl Pts',(-18.3768240055462,-41.0881011339882,
122.788607593364)) ;
#62840=CARTESIAN_POINT('Ctrl Pts',(-18.0045368875343,-41.2779297173339,
122.864848022296)) ;
#62841=CARTESIAN_POINT('Ctrl Pts',(-18.2854831831512,-41.097940636971,122.974241688555)) ;
#62842=CARTESIAN_POINT('Ctrl Pts',(-17.9304874746578,-41.2879958559003,
123.11875522056)) ;
#62843=CARTESIAN_POINT('Ctrl Pts',(-18.2262435039461,-41.1080067755374,
123.177367738535)) ;
#62844=CARTESIAN_POINT('Ctrl Pts',(-17.902263224335,-41.2978783703863,123.376958924445)) ;
#62845=CARTESIAN_POINT('Ctrl Pts',(-18.2036641643928,-41.1178892900235,
123.383929797729)) ;
#62846=CARTESIAN_POINT('Ctrl Pts',(-17.9189692034043,-41.3078706697419,
123.638973965491)) ;
#62847=CARTESIAN_POINT('Ctrl Pts',(-18.2170287674167,-41.127881589379,123.593541666519)) ;
#62848=CARTESIAN_POINT('Ctrl Pts',(-17.9806273077311,-41.3178237366953,
123.893199304568)) ;
#62849=CARTESIAN_POINT('Ctrl Pts',(-18.2663549772125,-41.1378346563324,
123.796921581805)) ;
#62850=CARTESIAN_POINT('Ctrl Pts',(-18.0864278200169,-41.3278584449005,
124.134724121174)) ;
#62851=CARTESIAN_POINT('Ctrl Pts',(-18.3509952924776,-41.1478693645376,
123.990141608418)) ;
#62852=CARTESIAN_POINT('Ctrl Pts',(-18.2302862077972,-41.3377466658047,
124.351140926558)) ;
#62853=CARTESIAN_POINT('Ctrl Pts',(-18.4660813609323,-41.1577575854418,
124.163274450491)) ;
#62854=CARTESIAN_POINT('Ctrl Pts',(-18.411128140004,-41.3477410888351,124.541587743708)) ;
#62855=CARTESIAN_POINT('Ctrl Pts',(-18.6107545669795,-41.1677520084722,
124.31563199722)) ;
#62856=CARTESIAN_POINT('Ctrl Pts',(-18.6213277144287,-41.3576864282813,
124.696900401289)) ;
#62857=CARTESIAN_POINT('Ctrl Pts',(-18.7789136746949,-41.1776973479184,
124.439882070568)) ;
#62858=CARTESIAN_POINT('Ctrl Pts',(-18.8551198560532,-41.3676337728926,
124.813866561764)) ;
#62859=CARTESIAN_POINT('Ctrl Pts',(-18.9659467888428,-41.1876446925297,
124.533455168981)) ;
#62860=CARTESIAN_POINT('Ctrl Pts',(-19.1082663812488,-41.3776816683036,
124.888923688486)) ;
#62861=CARTESIAN_POINT('Ctrl Pts',(-19.1684641030672,-41.1976925879407,
124.593501257939)) ;
#62862=CARTESIAN_POINT('Ctrl Pts',(-19.3653576889217,-41.387529313783,124.918508593892)) ;
#62863=CARTESIAN_POINT('Ctrl Pts',(-19.374135991281,-41.2075402334201,124.617169451887)) ;
#62864=CARTESIAN_POINT('Ctrl Pts',(-19.6267063239456,-41.397491027697,124.903644555584)) ;
#62865=CARTESIAN_POINT('Ctrl Pts',(-19.5832145704097,-41.2175019473341,
124.605278846852)) ;
#62866=CARTESIAN_POINT('Ctrl Pts',(-19.8831669773239,-41.4075196519879,
124.842893155659)) ;
#62867=CARTESIAN_POINT('Ctrl Pts',(-19.7883832884811,-41.227530571625,124.556678216363)) ;
#62868=CARTESIAN_POINT('Ctrl Pts',(-20.1223364379903,-41.4174300126446,
124.739853154527)) ;
#62869=CARTESIAN_POINT('Ctrl Pts',(-19.9797184280272,-41.2374409322817,
124.474246990679)) ;
#62870=CARTESIAN_POINT('Ctrl Pts',(-20.3409126898904,-41.4273647112179,
124.597063389142)) ;
#62871=CARTESIAN_POINT('Ctrl Pts',(-20.1545793763586,-41.247375630855,124.360016063863)) ;
#62872=CARTESIAN_POINT('Ctrl Pts',(-20.5332339905114,-41.4374065360721,
124.416390285309)) ;
#62873=CARTESIAN_POINT('Ctrl Pts',(-20.3084369714252,-41.2574174557092,
124.215477948896)) ;
#62874=CARTESIAN_POINT('Ctrl Pts',(-20.6889942202741,-41.4472911098165,
124.208484214558)) ;
#62875=CARTESIAN_POINT('Ctrl Pts',(-20.4330452122912,-41.2673020294536,
124.049154187181)) ;
#62876=CARTESIAN_POINT('Ctrl Pts',(-20.8079337346372,-41.4572929591797,
123.974137087454)) ;
#62877=CARTESIAN_POINT('Ctrl Pts',(-20.5281974668487,-41.2773038788168,
123.861676944645)) ;
#62878=CARTESIAN_POINT('Ctrl Pts',(-20.8839492756787,-41.4672122607537,
123.724761737193)) ;
#62879=CARTESIAN_POINT('Ctrl Pts',(-20.5890105118696,-41.2872231803909,
123.662177488703)) ;
#62880=CARTESIAN_POINT('Ctrl Pts',(-20.9159063783837,-41.477256369099,123.462776779803)) ;
#62881=CARTESIAN_POINT('Ctrl Pts',(-20.6145770325687,-41.2972672887361,
123.452589454882)) ;
#62882=CARTESIAN_POINT('Ctrl Pts',(-20.9021882404978,-41.4871407925413,
123.203374700093)) ;
#62883=CARTESIAN_POINT('Ctrl Pts',(-20.6036034091239,-41.3071517121784,
123.245068567429)) ;
#62884=CARTESIAN_POINT('Ctrl Pts',(-20.8434269167983,-41.4971571544507,
122.946788139686)) ;
#62885=CARTESIAN_POINT('Ctrl Pts',(-20.5565953052322,-41.3171680740879,
123.039799101921)) ;
#62886=CARTESIAN_POINT('Ctrl Pts',(-20.740169246239,-41.5071938099561,122.704103736706)) ;
#62887=CARTESIAN_POINT('Ctrl Pts',(-20.4739898809288,-41.3272047295932,
122.845651168886)) ;
#62888=CARTESIAN_POINT('Ctrl Pts',(-20.5998669968465,-41.5170239401454,
122.487161714525)) ;
#62889=CARTESIAN_POINT('Ctrl Pts',(-20.3617495279934,-41.3370348597826,
122.672097974141)) ;
#62890=CARTESIAN_POINT('Ctrl Pts',(-20.4197517580595,-41.5270999932353,
122.293140547087)) ;
#62891=CARTESIAN_POINT('Ctrl Pts',(-20.2176578409717,-41.3471109128724,
122.516880105175)) ;
#62892=CARTESIAN_POINT('Ctrl Pts',(-20.2133740001492,-41.5369522224211,
122.136713686681)) ;
#62893=CARTESIAN_POINT('Ctrl Pts',(-20.0525570462563,-41.3569631420582,
122.391738386618)) ;
#62894=CARTESIAN_POINT('Ctrl Pts',(-19.9779921555952,-41.5470254302204,
122.015693380369)) ;
#62895=CARTESIAN_POINT('Ctrl Pts',(-19.8642517827859,-41.3670363498575,
122.294921027755)) ;
#62896=CARTESIAN_POINT('Ctrl Pts',(-19.7309096530658,-41.5568669415718,
121.939233606283)) ;
#62897=CARTESIAN_POINT('Ctrl Pts',(-19.6665870925325,-41.3768778612089,
122.233752494711)) ;
#62898=CARTESIAN_POINT('Ctrl Pts',(-19.4713417220652,-41.5668278796093,
121.905469506213)) ;
#62899=CARTESIAN_POINT('Ctrl Pts',(-19.4589332355636,-41.3868387992465,
122.206739977289)) ;
#62900=CARTESIAN_POINT('Ctrl Pts',(-19.2078592032353,-41.5768657415343,
121.917907090772)) ;
#62901=CARTESIAN_POINT('Ctrl Pts',(-19.2481470590052,-41.3968766611714,
122.216688878807)) ;
#62902=CARTESIAN_POINT('Ctrl Pts',(-18.9545877190135,-41.5867399275314,
121.974495320736)) ;
#62903=CARTESIAN_POINT('Ctrl Pts',(-19.0455303831215,-41.4067508471685,
122.261958038974)) ;
#62904=CARTESIAN_POINT('Ctrl Pts',(-18.7103088483806,-41.5968100871093,
122.076174219164)) ;
#62905=CARTESIAN_POINT('Ctrl Pts',(-18.8501065384056,-41.4168210067464,
122.343300089057)) ;
#62906=CARTESIAN_POINT('Ctrl Pts',(-18.4925316287136,-41.6066418345351,
122.215244290512)) ;
#62907=CARTESIAN_POINT('Ctrl Pts',(-18.675884926045,-41.4266527541722,122.454554491954)) ;
#62908=CARTESIAN_POINT('Ctrl Pts',(-18.2978201733905,-41.6166779146064,
122.393114575387)) ;
#62909=CARTESIAN_POINT('Ctrl Pts',(-18.5201147167768,-41.4366888342435,
122.596849707631)) ;
#62910=CARTESIAN_POINT('Ctrl Pts',(-18.1377661291796,-41.6266949614589,
122.602121409424)) ;
#62911=CARTESIAN_POINT('Ctrl Pts',(-18.3920704452954,-41.446705881096,122.764054368868)) ;
#62912=CARTESIAN_POINT('Ctrl Pts',(-18.0176363964437,-41.6365772196255,
122.832366722384)) ;
#62913=CARTESIAN_POINT('Ctrl Pts',(-18.2959657432194,-41.4565881392626,
122.948249322725)) ;
#62914=CARTESIAN_POINT('Ctrl Pts',(-17.9381960769655,-41.6465649024218,
123.082493245792)) ;
#62915=CARTESIAN_POINT('Ctrl Pts',(-18.2324121300775,-41.466575822059,123.148349941612)) ;
#62916=CARTESIAN_POINT('Ctrl Pts',(-17.9033168942799,-41.6565115591386,
123.341584277109)) ;
#62917=CARTESIAN_POINT('Ctrl Pts',(-18.2045073339234,-41.4765224787757,
123.355622202973)) ;
#62918=CARTESIAN_POINT('Ctrl Pts',(-17.9143411683041,-41.6665686172188,
123.605613842751)) ;
#62919=CARTESIAN_POINT('Ctrl Pts',(-18.2133253006572,-41.4865795368559,
123.56684609059)) ;
#62920=CARTESIAN_POINT('Ctrl Pts',(-17.969355045573,-41.6763867967682,123.857706729659)) ;
#62921=CARTESIAN_POINT('Ctrl Pts',(-18.2573346904217,-41.4963977164053,
123.768519739504)) ;
#62922=CARTESIAN_POINT('Ctrl Pts',(-18.0688075005491,-41.6864227312072,
124.101962973962)) ;
#62923=CARTESIAN_POINT('Ctrl Pts',(-18.3368951443602,-41.5064336508443,
123.963925444336)) ;
#62924=CARTESIAN_POINT('Ctrl Pts',(-18.2096507194806,-41.6964473856362,
124.324600663781)) ;
#62925=CARTESIAN_POINT('Ctrl Pts',(-18.4495684418936,-41.5164583052733,
124.142036426713)) ;
#62926=CARTESIAN_POINT('Ctrl Pts',(-18.3835301012507,-41.7062994052157,
124.51642843277)) ;
#62927=CARTESIAN_POINT('Ctrl Pts',(-18.5886701972633,-41.5263103248528,
124.295499139978)) ;
#62928=CARTESIAN_POINT('Ctrl Pts',(-18.5906854588075,-41.7162903189306,
124.677682956406)) ;
#62929=CARTESIAN_POINT('Ctrl Pts',(-18.7543933282232,-41.5363012385678,
124.424504019859)) ;
#62930=CARTESIAN_POINT('Ctrl Pts',(-18.8209758181354,-41.7262083077702,
124.799801736939)) ;
#62931=CARTESIAN_POINT('Ctrl Pts',(-18.9386244015868,-41.5462192274073,
124.522200358764)) ;
#62932=CARTESIAN_POINT('Ctrl Pts',(-19.0716562721303,-41.736236418501,124.88101516819)) ;
#62933=CARTESIAN_POINT('Ctrl Pts',(-19.1391682539512,-41.5562473381381,
124.587172769983)) ;
#62934=CARTESIAN_POINT('Ctrl Pts',(-19.3289219205496,-41.7461216164094,
124.917060930178)) ;
#62935=CARTESIAN_POINT('Ctrl Pts',(-19.3449799461922,-41.5661325360465,
124.616011040601)) ;
#62936=CARTESIAN_POINT('Ctrl Pts',(-19.5912951011556,-41.7561108916774,
124.908434150028)) ;
#62937=CARTESIAN_POINT('Ctrl Pts',(-19.554878426075,-41.5761218113145,124.609111482984)) ;
#62938=CARTESIAN_POINT('Ctrl Pts',(-19.8493960390687,-41.7661523498469,
124.853543536914)) ;
#62939=CARTESIAN_POINT('Ctrl Pts',(-19.7613596181265,-41.586163269484,124.565200709918)) ;
#62940=CARTESIAN_POINT('Ctrl Pts',(-20.089121327571,-41.7759838136352,124.757174104887)) ;
#62941=CARTESIAN_POINT('Ctrl Pts',(-19.9531398219293,-41.5959947332723,
124.488107167589)) ;
#62942=CARTESIAN_POINT('Ctrl Pts',(-20.3126159520966,-41.7859887459391,
124.618753527264)) ;
#62943=CARTESIAN_POINT('Ctrl Pts',(-20.1319364892421,-41.6059996655762,
124.377372384104)) ;
#62944=CARTESIAN_POINT('Ctrl Pts',(-20.5082790000552,-41.7959751098338,
124.44379651089)) ;
#62945=CARTESIAN_POINT('Ctrl Pts',(-20.2884681052533,-41.615986029471,124.237408279578)) ;
#62946=CARTESIAN_POINT('Ctrl Pts',(-20.6710896620277,-41.8060047387197,
124.236556568521)) ;
#62947=CARTESIAN_POINT('Ctrl Pts',(-20.4187181302531,-41.6260156583568,
124.071617471286)) ;
#62948=CARTESIAN_POINT('Ctrl Pts',(-20.7938478463196,-41.8158799608281,
124.007888084102)) ;
#62949=CARTESIAN_POINT('Ctrl Pts',(-20.5169261213944,-41.6358908804652,
123.88868407081)) ;
#62950=CARTESIAN_POINT('Ctrl Pts',(-20.8763477233689,-41.8258811732252,
123.758394357555)) ;
#62951=CARTESIAN_POINT('Ctrl Pts',(-20.5829278694143,-41.6458920928623,
123.689089793448)) ;
#62952=CARTESIAN_POINT('Ctrl Pts',(-20.9141799974451,-41.8357897524607,
123.500723797923)) ;
#62953=CARTESIAN_POINT('Ctrl Pts',(-20.6131956146695,-41.6558006720979,
123.482954012209)) ;
#62954=CARTESIAN_POINT('Ctrl Pts',(-20.9065096443018,-41.8458446050167,
123.236647196744)) ;
#62955=CARTESIAN_POINT('Ctrl Pts',(-20.607061323779,-41.6658555246539,123.271692585024)) ;
#62956=CARTESIAN_POINT('Ctrl Pts',(-20.8544198064542,-41.8557031872915,
122.982817801589)) ;
#62957=CARTESIAN_POINT('Ctrl Pts',(-20.5653915448547,-41.6757141069286,
123.068629169974)) ;
#62958=CARTESIAN_POINT('Ctrl Pts',(-20.7572019522211,-41.8657713167342,
122.736787999825)) ;
#62959=CARTESIAN_POINT('Ctrl Pts',(-20.4876191232104,-41.6857822363713,
122.871804461378)) ;
#62960=CARTESIAN_POINT('Ctrl Pts',(-20.6216170476226,-41.8756267884233,
122.516096462903)) ;
#62961=CARTESIAN_POINT('Ctrl Pts',(-20.3791532034229,-41.6956377080604,
122.695250586501)) ;
#62962=CARTESIAN_POINT('Ctrl Pts',(-20.4479526497867,-41.8856216368096,
122.319060073039)) ;
#62963=CARTESIAN_POINT('Ctrl Pts',(-20.2402233360119,-41.7056325564467,
122.537620125504)) ;
#62964=CARTESIAN_POINT('Ctrl Pts',(-20.2416008599543,-41.895652933594,122.155008415797)) ;
#62965=CARTESIAN_POINT('Ctrl Pts',(-20.0751431938009,-41.7156638532311,
122.406377179865)) ;
#62966=CARTESIAN_POINT('Ctrl Pts',(-20.0138985646584,-41.9055194698041,
122.030978291943)) ;
#62967=CARTESIAN_POINT('Ctrl Pts',(-19.8929827296992,-41.7255303894412,
122.307151422635)) ;
#62968=CARTESIAN_POINT('Ctrl Pts',(-19.7652803949844,-41.9155068927649,
121.946967065513)) ;
#62969=CARTESIAN_POINT('Ctrl Pts',(-19.6940889763465,-41.7355178124021,
122.23994043297)) ;
#62970=CARTESIAN_POINT('Ctrl Pts',(-19.5069103967345,-41.9254518317847,
121.907424800281)) ;
#62971=CARTESIAN_POINT('Ctrl Pts',(-19.4873934887718,-41.7454627514218,
122.208304514196)) ;
#62972=CARTESIAN_POINT('Ctrl Pts',(-19.2430300937842,-41.9354967176447,
121.913529165086)) ;
#62973=CARTESIAN_POINT('Ctrl Pts',(-19.2762891837712,-41.7555076372818,
122.213185853992)) ;
#62974=CARTESIAN_POINT('Ctrl Pts',(-18.9887092821943,-41.9453652527309,
121.964316287629)) ;
#62975=CARTESIAN_POINT('Ctrl Pts',(-19.072832435962,-41.7653761723681,122.253813365681)) ;
#62976=CARTESIAN_POINT('Ctrl Pts',(-18.7444398718667,-41.9553311207376,
122.058732418128)) ;
#62977=CARTESIAN_POINT('Ctrl Pts',(-18.8774162150229,-41.7753420403747,
122.329344164061)) ;
#62978=CARTESIAN_POINT('Ctrl Pts',(-18.5191258960405,-41.9653537681901,
122.195167959833)) ;
#62979=CARTESIAN_POINT('Ctrl Pts',(-18.6971639262968,-41.7853646878272,
122.438490705683)) ;
#62980=CARTESIAN_POINT('Ctrl Pts',(-18.322858065799,-41.9752774071977,122.366864085304)) ;
#62981=CARTESIAN_POINT('Ctrl Pts',(-18.5401483567963,-41.7952883268348,
122.575845826025)) ;
#62982=CARTESIAN_POINT('Ctrl Pts',(-18.1585632397569,-41.9852201322034,
122.570050124167)) ;
#62983=CARTESIAN_POINT('Ctrl Pts',(-18.4087108446553,-41.8052310518406,
122.738393149906)) ;
#62984=CARTESIAN_POINT('Ctrl Pts',(-18.0310264117004,-41.9952657382553,
122.80116942064)) ;
#62985=CARTESIAN_POINT('Ctrl Pts',(-18.3066794495729,-41.8152766578924,
122.923287501502)) ;
#62986=CARTESIAN_POINT('Ctrl Pts',(-17.9468424318338,-42.0051271607764,
123.046286075553)) ;
#62987=CARTESIAN_POINT('Ctrl Pts',(-18.2393302260419,-41.8251380804135,
123.119379900334)) ;
#62988=CARTESIAN_POINT('Ctrl Pts',(-17.9055231594074,-42.0151207292256,
123.305597710692)) ;
#62989=CARTESIAN_POINT('Ctrl Pts',(-18.2062726013886,-41.8351316488627,
123.326828797274)) ;
#62990=CARTESIAN_POINT('Ctrl Pts',(-17.9096925519482,-42.0250461999809,
123.56643384868)) ;
#62991=CARTESIAN_POINT('Ctrl Pts',(-18.2096058544786,-41.845057119618,123.535497626538)) ;
#62992=CARTESIAN_POINT('Ctrl Pts',(-17.9595713839581,-42.0350738739368,
123.825153894762)) ;
#62993=CARTESIAN_POINT('Ctrl Pts',(-18.2495067533621,-41.8550847935739,
123.742474085264)) ;
#62994=CARTESIAN_POINT('Ctrl Pts',(-18.0520856877186,-42.0449610519785,
124.067987197481)) ;
#62995=CARTESIAN_POINT('Ctrl Pts',(-18.3235158644063,-41.8649719716156,
123.93674127071)) ;
#62996=CARTESIAN_POINT('Ctrl Pts',(-18.187066988808,-42.0549894313466,124.294288291678)) ;
#62997=CARTESIAN_POINT('Ctrl Pts',(-18.4314996700195,-41.8750003509838,
124.117783890498)) ;
#62998=CARTESIAN_POINT('Ctrl Pts',(-18.3569254897191,-42.0648836740681,
124.491191503969)) ;
#62999=CARTESIAN_POINT('Ctrl Pts',(-18.5673820062169,-41.8848945937052,
124.275305521873)) ;
#63000=CARTESIAN_POINT('Ctrl Pts',(-18.6285705558117,-42.078236590719,124.71326978042)) ;
#63001=CARTESIAN_POINT('Ctrl Pts',(-18.7847096513815,-41.8982475103561,
124.452982209414)) ;
#63002=CARTESIAN_POINT('Ctrl Pts',(-18.948377526286,-42.0914391084657,124.857795814166)) ;
#63003=CARTESIAN_POINT('Ctrl Pts',(-19.0405786175282,-41.9114500281029,
124.568605567899)) ;
#63004=CARTESIAN_POINT('Ctrl Pts',(-19.2946442505059,-42.1047950137467,
124.914924015773)) ;
#63005=CARTESIAN_POINT('Ctrl Pts',(-19.3175485758015,-41.9248059333838,
124.614299551762)) ;
#63006=CARTESIAN_POINT('Ctrl Pts',(-19.5547381910601,-42.1146916623845,
124.912293117139)) ;
#63007=CARTESIAN_POINT('Ctrl Pts',(-19.5256324094928,-41.9347025820217,
124.612199382613)) ;
#63008=CARTESIAN_POINT('Ctrl Pts',(-19.8142993016192,-42.124739800437,124.86390602345)) ;
#63009=CARTESIAN_POINT('Ctrl Pts',(-19.7332792909241,-41.9447507200741,
124.573491312428)) ;
#63010=CARTESIAN_POINT('Ctrl Pts',(-20.0576759368903,-42.1346307606148,
124.772616402038)) ;
#63011=CARTESIAN_POINT('Ctrl Pts',(-19.9279820995287,-41.9546416802519,
124.500461812852)) ;
#63012=CARTESIAN_POINT('Ctrl Pts',(-20.2841432703349,-42.1446235964915,
124.639664036342)) ;
#63013=CARTESIAN_POINT('Ctrl Pts',(-20.1091567936653,-41.9646345161287,
124.394101924367)) ;
#63014=CARTESIAN_POINT('Ctrl Pts',(-20.4846006078538,-42.1546626914931,
124.468172605259)) ;
#63015=CARTESIAN_POINT('Ctrl Pts',(-20.269524451752,-41.9746736111302,124.256910062148)) ;
#63016=CARTESIAN_POINT('Ctrl Pts',(-20.6493590677972,-42.1645000473443,
124.268925825602)) ;
#63017=CARTESIAN_POINT('Ctrl Pts',(-20.4013316292031,-41.9845109669814,
124.097515752566)) ;
#63018=CARTESIAN_POINT('Ctrl Pts',(-20.8232941424064,-42.177892995275,123.963015567167)) ;
#63019=CARTESIAN_POINT('Ctrl Pts',(-20.5404892049295,-41.9979039149121,
123.85277973288)) ;
#63020=CARTESIAN_POINT('Ctrl Pts',(-20.9119427186459,-42.1910596717019,
123.624389608226)) ;
#63021=CARTESIAN_POINT('Ctrl Pts',(-20.6114090656495,-42.0110705913391,
123.581847590379)) ;
#63022=CARTESIAN_POINT('Ctrl Pts',(-20.9103198254801,-42.2044444531087,
123.272710611957)) ;
#63023=CARTESIAN_POINT('Ctrl Pts',(-20.6101088464383,-42.0244553727458,
123.300551791675)) ;
#63024=CARTESIAN_POINT('Ctrl Pts',(-20.8642332429121,-42.2143062357526,
123.017641919768)) ;
#63025=CARTESIAN_POINT('Ctrl Pts',(-20.5732425041568,-42.0343171553897,
123.096486611068)) ;
#63026=CARTESIAN_POINT('Ctrl Pts',(-20.7737441303443,-42.2243053837056,
122.771002649473)) ;
#63027=CARTESIAN_POINT('Ctrl Pts',(-20.5008532527009,-42.0443163033428,
122.899177173043)) ;
#63028=CARTESIAN_POINT('Ctrl Pts',(-20.6432311626779,-42.2342081763227,
122.545797674276)) ;
#63029=CARTESIAN_POINT('Ctrl Pts',(-20.3964433972298,-42.0542190959598,
122.71901073462)) ;
#63030=CARTESIAN_POINT('Ctrl Pts',(-20.4731343577102,-42.2442577562136,
122.343862138749)) ;
#63031=CARTESIAN_POINT('Ctrl Pts',(-20.2603721024993,-42.0642686758508,
122.557463185732)) ;
#63032=CARTESIAN_POINT('Ctrl Pts',(-20.2076003346992,-42.2574448300231,
122.12099560958)) ;
#63033=CARTESIAN_POINT('Ctrl Pts',(-20.0479240767754,-42.0774557496602,
122.379158188714)) ;
#63034=CARTESIAN_POINT('Ctrl Pts',(-19.8041265873875,-42.2741976199943,
121.933081385993)) ;
#63035=CARTESIAN_POINT('Ctrl Pts',(-19.7251863995672,-42.0942085396314,
122.228834129982)) ;
#63036=CARTESIAN_POINT('Ctrl Pts',(-19.3673812946828,-42.290686272089,121.894819463525)) ;
#63037=CARTESIAN_POINT('Ctrl Pts',(-19.3757249718531,-42.1106971917261,
122.198219603723)) ;
#63038=CARTESIAN_POINT('Ctrl Pts',(-19.0216618585074,-42.3040430982724,
121.955010874022)) ;
#63039=CARTESIAN_POINT('Ctrl Pts',(-19.0992014122385,-42.1240540179095,
122.246369156977)) ;
#63040=CARTESIAN_POINT('Ctrl Pts',(-18.7769948829387,-42.3139394831503,
122.043336388622)) ;
#63041=CARTESIAN_POINT('Ctrl Pts',(-18.9034558730959,-42.1339504027875,
122.31702867763)) ;
#63042=CARTESIAN_POINT('Ctrl Pts',(-18.5489107993243,-42.3239459976708,
122.174062497428)) ;
#63043=CARTESIAN_POINT('Ctrl Pts',(-18.7209920470431,-42.1439569173079,
122.421605740756)) ;
#63044=CARTESIAN_POINT('Ctrl Pts',(-18.2820313956166,-42.3371361211872,
122.395439854909)) ;
#63045=CARTESIAN_POINT('Ctrl Pts',(-18.5074779287399,-42.1571470408243,
122.598716881194)) ;
#63046=CARTESIAN_POINT('Ctrl Pts',(-18.0248416307128,-42.3539026823368,
122.759167368776)) ;
#63047=CARTESIAN_POINT('Ctrl Pts',(-18.3017330244153,-42.1739136019739,
122.889684714368)) ;
#63048=CARTESIAN_POINT('Ctrl Pts',(-17.886048515107,-42.3736871710448,123.266512292216)) ;
#63049=CARTESIAN_POINT('Ctrl Pts',(-18.190691850351,-42.1936980906819,123.295564709079)) ;
#63050=CARTESIAN_POINT('Ctrl Pts',(-17.9274046621304,-42.3936326186413,
123.794881011967)) ;
#63051=CARTESIAN_POINT('Ctrl Pts',(-18.2237744875469,-42.2136435382784,
123.718259302305)) ;
#63052=CARTESIAN_POINT('Ctrl Pts',(-18.1467300052869,-42.4135442807972,
124.276525572974)) ;
#63053=CARTESIAN_POINT('Ctrl Pts',(-18.3992319711091,-42.2335552004343,
124.103577050796)) ;
#63054=CARTESIAN_POINT('Ctrl Pts',(-18.5161004763561,-42.4334364728161,
124.654913018434)) ;
#63055=CARTESIAN_POINT('Ctrl Pts',(-18.6947270610426,-42.2534473924532,
124.40628936176)) ;
#63056=CARTESIAN_POINT('Ctrl Pts',(-18.9961947812989,-42.4534776033707,
124.885472692553)) ;
#63057=CARTESIAN_POINT('Ctrl Pts',(-19.0788009536354,-42.2734885230078,
124.590739459069)) ;
#63058=CARTESIAN_POINT('Ctrl Pts',(-19.5204288936076,-42.4732959379863,
124.938073341943)) ;
#63059=CARTESIAN_POINT('Ctrl Pts',(-19.4981894659672,-42.2933068576234,
124.632822663084)) ;
#63060=CARTESIAN_POINT('Ctrl Pts',(-20.0350303911064,-42.4932685032059,
124.808520139639)) ;
#63061=CARTESIAN_POINT('Ctrl Pts',(-19.9098714983823,-42.313279422843,124.529182116314)) ;
#63062=CARTESIAN_POINT('Ctrl Pts',(-20.473087584271,-42.5131577193775,124.512279231662)) ;
#63063=CARTESIAN_POINT('Ctrl Pts',(-20.2603191389922,-42.3331686390146,
124.292190423348)) ;
#63064=CARTESIAN_POINT('Ctrl Pts',(-20.7853676285003,-42.5331812937002,
124.081500341418)) ;
#63065=CARTESIAN_POINT('Ctrl Pts',(-20.510144598529,-42.3531922133373,123.947568642154)) ;
#63066=CARTESIAN_POINT('Ctrl Pts',(-20.9306728526506,-42.5529784567885,
123.575689148436)) ;
#63067=CARTESIAN_POINT('Ctrl Pts',(-20.6263909037281,-42.3729893764256,
123.542918090147)) ;
#63068=CARTESIAN_POINT('Ctrl Pts',(-20.8956352696577,-42.5729439506122,
123.046309019479)) ;
#63069=CARTESIAN_POINT('Ctrl Pts',(-20.5983617160724,-42.3929548702494,
123.119413476898)) ;
#63070=CARTESIAN_POINT('Ctrl Pts',(-20.6814765719901,-42.5928976583536,
122.560980844406)) ;
#63071=CARTESIAN_POINT('Ctrl Pts',(-20.4270354944749,-42.4129085779908,
122.731150136192)) ;
#63072=CARTESIAN_POINT('Ctrl Pts',(-20.3156068294175,-42.6128050350802,
122.178926648595)) ;
#63073=CARTESIAN_POINT('Ctrl Pts',(-20.1343395078316,-42.4328159547174,
122.425505382769)) ;
#63074=CARTESIAN_POINT('Ctrl Pts',(-19.8430795028509,-42.6326572466288,
121.943950043858)) ;
#63075=CARTESIAN_POINT('Ctrl Pts',(-19.7563159223275,-42.4526681662659,
122.237523311971)) ;
#63076=CARTESIAN_POINT('Ctrl Pts',(-19.3129641321421,-42.6527296335745,
121.884197616228)) ;
#63077=CARTESIAN_POINT('Ctrl Pts',(-19.3322245789558,-42.4727405532116,
122.189721484159)) ;
#63078=CARTESIAN_POINT('Ctrl Pts',(-18.8004818960636,-42.6725675032148,
122.008159120081)) ;
#63079=CARTESIAN_POINT('Ctrl Pts',(-18.9222366927177,-42.4925784228519,
122.288891090315)) ;
#63080=CARTESIAN_POINT('Ctrl Pts',(-18.3595239816206,-42.6924181577679,
122.297834685126)) ;
#63081=CARTESIAN_POINT('Ctrl Pts',(-18.5694695547567,-42.5124290774051,
122.52063348008)) ;
#63082=CARTESIAN_POINT('Ctrl Pts',(-18.0413332378271,-42.7124700921084,
122.725319925752)) ;
#63083=CARTESIAN_POINT('Ctrl Pts',(-18.3149181158026,-42.5324810117455,
122.862621797376)) ;
#63084=CARTESIAN_POINT('Ctrl Pts',(-17.8898151802692,-42.7323032796744,
123.230332622468)) ;
#63085=CARTESIAN_POINT('Ctrl Pts',(-18.1937042468816,-42.5523141993116,
123.266634019015)) ;
#63086=CARTESIAN_POINT('Ctrl Pts',(-17.9188018275413,-42.7522324919051,
123.759028000003)) ;
#63087=CARTESIAN_POINT('Ctrl Pts',(-18.2168953694706,-42.5722434115422,
123.689590983492)) ;
#63088=CARTESIAN_POINT('Ctrl Pts',(-18.1255818945999,-42.7721174571195,
124.245626671825)) ;
#63089=CARTESIAN_POINT('Ctrl Pts',(-18.3823217704082,-42.5921283767566,
124.078870010309)) ;
#63090=CARTESIAN_POINT('Ctrl Pts',(-18.4898112910282,-42.7921911982641,
124.635336040243)) ;
#63091=CARTESIAN_POINT('Ctrl Pts',(-18.6737062691616,-42.6122021179012,
124.390635650376)) ;
#63092=CARTESIAN_POINT('Ctrl Pts',(-18.9586591560268,-42.8119843800445,
124.874120892103)) ;
#63093=CARTESIAN_POINT('Ctrl Pts',(-19.0487871981899,-42.6319952996816,
124.581662463708)) ;
#63094=CARTESIAN_POINT('Ctrl Pts',(-19.4849952307029,-42.8319470880472,
124.940716397595)) ;
#63095=CARTESIAN_POINT('Ctrl Pts',(-19.4698566611138,-42.6519580076843,
124.634936088449)) ;
#63096=CARTESIAN_POINT('Ctrl Pts',(-20.0027532085215,-42.8519300397896,
124.822320272742)) ;
#63097=CARTESIAN_POINT('Ctrl Pts',(-19.8840626043544,-42.6719409594268,
124.540216680374)) ;
#63098=CARTESIAN_POINT('Ctrl Pts',(-20.4457748038711,-42.8717406595618,
124.537685736192)) ;
#63099=CARTESIAN_POINT('Ctrl Pts',(-20.2384794300186,-42.6917515791989,
124.312505791514)) ;
#63100=CARTESIAN_POINT('Ctrl Pts',(-20.7682626054881,-42.8917243755947,
124.115808826861)) ;
#63101=CARTESIAN_POINT('Ctrl Pts',(-20.496467127968,-42.7117352952318,123.975002213064)) ;
#63102=CARTESIAN_POINT('Ctrl Pts',(-20.9266062652679,-42.911605839492,123.611535793601)) ;
#63103=CARTESIAN_POINT('Ctrl Pts',(-20.6231390533387,-42.7316167591292,
123.571582135576)) ;
#63104=CARTESIAN_POINT('Ctrl Pts',(-20.9036603572419,-42.9315611693364,
123.081759157368)) ;
#63105=CARTESIAN_POINT('Ctrl Pts',(-20.6047789224965,-42.7515720889735,
123.147760755325)) ;
#63106=CARTESIAN_POINT('Ctrl Pts',(-20.7024014511106,-42.9514366301419,
122.593252469761)) ;
#63107=CARTESIAN_POINT('Ctrl Pts',(-20.4437676559676,-42.771447549779,122.756956211372)) ;
#63108=CARTESIAN_POINT('Ctrl Pts',(-20.3449003201343,-42.9714209501934,
122.200502446689)) ;
#63109=CARTESIAN_POINT('Ctrl Pts',(-20.1577657851218,-42.7914318698305,
122.442758885575)) ;
#63110=CARTESIAN_POINT('Ctrl Pts',(-19.8758679528504,-42.991348982983,121.954198379585)) ;
#63111=CARTESIAN_POINT('Ctrl Pts',(-19.7825308096546,-42.8113599026202,
122.24571839476)) ;
#63112=CARTESIAN_POINT('Ctrl Pts',(-19.438573167792,-43.0079577449228,121.894584975642)) ;
#63113=CARTESIAN_POINT('Ctrl Pts',(-19.4327162628233,-42.82796866456,122.198032510649)) ;
#63114=CARTESIAN_POINT('Ctrl Pts',(-19.0946716817039,-43.0211453836129,
121.937615803098)) ;
#63115=CARTESIAN_POINT('Ctrl Pts',(-19.1575750804821,-42.84115630325,122.232458887897)) ;
#63116=CARTESIAN_POINT('Ctrl Pts',(-18.8437153066299,-43.031131817973,122.014331380066)) ;
#63117=CARTESIAN_POINT('Ctrl Pts',(-18.9568164411077,-42.8511427376102,
122.293831610718)) ;
#63118=CARTESIAN_POINT('Ctrl Pts',(-18.6094527009105,-43.0411411919324,
122.133980200505)) ;
#63119=CARTESIAN_POINT('Ctrl Pts',(-18.7693988622901,-42.8611521115695,
122.38956024232)) ;
#63120=CARTESIAN_POINT('Ctrl Pts',(-18.3305857336724,-43.0544312254977,
122.344252306569)) ;
#63121=CARTESIAN_POINT('Ctrl Pts',(-18.5463444103637,-42.8744421451348,
122.55774111295)) ;
#63122=CARTESIAN_POINT('Ctrl Pts',(-18.0587919012148,-43.0710252131601,
122.691613440136)) ;
#63123=CARTESIAN_POINT('Ctrl Pts',(-18.3288675517154,-42.8910361327973,
122.835684012626)) ;
#63124=CARTESIAN_POINT('Ctrl Pts',(-17.9215463024505,-43.0876574684357,
123.111805424013)) ;
#63125=CARTESIAN_POINT('Ctrl Pts',(-18.2190954252728,-42.9076683880728,
123.171796586433)) ;
#63126=CARTESIAN_POINT('Ctrl Pts',(-17.9026645543824,-43.1008998521035,
123.459298795023)) ;
#63127=CARTESIAN_POINT('Ctrl Pts',(-18.203983606276,-42.9209107717406,123.449819411052)) ;
#63128=CARTESIAN_POINT('Ctrl Pts',(-17.9331154384697,-43.1108140603309,
123.718057560274)) ;
#63129=CARTESIAN_POINT('Ctrl Pts',(-18.2283482599857,-42.9308249799681,
123.656820588526)) ;
#63130=CARTESIAN_POINT('Ctrl Pts',(-18.0093888248284,-43.1208706996026,
123.971069080689)) ;
#63131=CARTESIAN_POINT('Ctrl Pts',(-18.2893690473881,-42.9408816192397,
123.859230933456)) ;
#63132=CARTESIAN_POINT('Ctrl Pts',(-18.1256799001394,-43.1307165060227,
124.202224696424)) ;
#63133=CARTESIAN_POINT('Ctrl Pts',(-18.3824021684236,-42.9507274256599,
124.044152714525)) ;
#63134=CARTESIAN_POINT('Ctrl Pts',(-18.2830849970775,-43.1407615056559,
124.414117164475)) ;
#63135=CARTESIAN_POINT('Ctrl Pts',(-18.5083351697391,-42.960772425293,124.21367093415)) ;
#63136=CARTESIAN_POINT('Ctrl Pts',(-18.537043251934,-43.1540425280286,124.65350405423)) ;
#63137=CARTESIAN_POINT('Ctrl Pts',(-18.7114678288813,-42.9740534476658,
124.405150550178)) ;
#63138=CARTESIAN_POINT('Ctrl Pts',(-18.8452649773422,-43.1672399745533,
124.820961905211)) ;
#63139=CARTESIAN_POINT('Ctrl Pts',(-18.9580634355738,-42.9872508941904,
124.539134958599)) ;
#63140=CARTESIAN_POINT('Ctrl Pts',(-19.1881152200042,-43.1806542723603,
124.902985565981)) ;
#63141=CARTESIAN_POINT('Ctrl Pts',(-19.232360308715,-43.0006651919974,124.604753983446)) ;
#63142=CARTESIAN_POINT('Ctrl Pts',(-19.4462101896744,-43.190493337763,124.918723959337)) ;
#63143=CARTESIAN_POINT('Ctrl Pts',(-19.4388332239247,-43.0105042574002,
124.617341843955)) ;
#63144=CARTESIAN_POINT('Ctrl Pts',(-19.7069166424415,-43.2004765440407,
124.889671060815)) ;
#63145=CARTESIAN_POINT('Ctrl Pts',(-19.6473989352599,-43.0204874636778,
124.594097446698)) ;
#63146=CARTESIAN_POINT('Ctrl Pts',(-19.9578281238234,-43.2104277789535,
124.815931888651)) ;
#63147=CARTESIAN_POINT('Ctrl Pts',(-19.8481272005172,-43.0304386985906,
124.535103914391)) ;
#63148=CARTESIAN_POINT('Ctrl Pts',(-20.1934350689946,-43.2204287786551,
124.699450981921)) ;
#63149=CARTESIAN_POINT('Ctrl Pts',(-20.0366117625381,-43.0404396982923,
124.441917204073)) ;
#63150=CARTESIAN_POINT('Ctrl Pts',(-20.4056235278496,-43.2304601244425,
124.543033701341)) ;
#63151=CARTESIAN_POINT('Ctrl Pts',(-20.206361135427,-43.0504710440796,124.316781584499)) ;
#63152=CARTESIAN_POINT('Ctrl Pts',(-20.5844761556059,-43.2403138891475,
124.355767995576)) ;
#63153=CARTESIAN_POINT('Ctrl Pts',(-20.3494415434613,-43.0603248087846,
124.166967530126)) ;
#63154=CARTESIAN_POINT('Ctrl Pts',(-20.7303004788071,-43.2502845428158,
124.138111587072)) ;
#63155=CARTESIAN_POINT('Ctrl Pts',(-20.4660990801308,-43.0702954624529,
123.992841228193)) ;
#63156=CARTESIAN_POINT('Ctrl Pts',(-20.836417878929,-43.260281786473,123.897736472941)) ;
#63157=CARTESIAN_POINT('Ctrl Pts',(-20.5509909214164,-43.0802927061101,
123.800540288638)) ;
#63158=CARTESIAN_POINT('Ctrl Pts',(-20.8990697974022,-43.2703152424172,
123.641641842364)) ;
#63159=CARTESIAN_POINT('Ctrl Pts',(-20.6011102563004,-43.0903261620543,
123.595664077152)) ;
#63160=CARTESIAN_POINT('Ctrl Pts',(-20.9164201484356,-43.2801707467176,
123.383205983392)) ;
#63161=CARTESIAN_POINT('Ctrl Pts',(-20.6149882875894,-43.1001816663547,
123.388915428103)) ;
#63162=CARTESIAN_POINT('Ctrl Pts',(-20.8885847142338,-43.2901701830037,
123.121956715712)) ;
#63163=CARTESIAN_POINT('Ctrl Pts',(-20.5927177264753,-43.1101811026408,
123.17991632247)) ;
#63164=CARTESIAN_POINT('Ctrl Pts',(-20.8168337005953,-43.3000646425196,
122.871985466953)) ;
#63165=CARTESIAN_POINT('Ctrl Pts',(-20.5353148477446,-43.1200755621567,
122.979940136269)) ;
#63166=CARTESIAN_POINT('Ctrl Pts',(-20.7007964614407,-43.3101277619712,
122.634405971093)) ;
#63167=CARTESIAN_POINT('Ctrl Pts',(-20.4424830472007,-43.1301386816084,
122.789877488713)) ;
#63168=CARTESIAN_POINT('Ctrl Pts',(-20.5489034190072,-43.3199673963832,
122.425092863815)) ;
#63169=CARTESIAN_POINT('Ctrl Pts',(-20.3209670269666,-43.1399783160204,
122.622428563072)) ;
#63170=CARTESIAN_POINT('Ctrl Pts',(-20.3590408300149,-43.330030603869,122.2410636791)) ;
#63171=CARTESIAN_POINT('Ctrl Pts',(-20.1690754107749,-43.1500415235061,
122.475206756355)) ;
#63172=CARTESIAN_POINT('Ctrl Pts',(-20.1436111274021,-43.3399247112482,
122.095429795694)) ;
#63173=CARTESIAN_POINT('Ctrl Pts',(-19.9967306388888,-43.1599356308853,
122.358701616965)) ;
#63174=CARTESIAN_POINT('Ctrl Pts',(-19.9053553865041,-43.3498670434406,
121.988285686092)) ;
#63175=CARTESIAN_POINT('Ctrl Pts',(-19.8061253596654,-43.1698779630777,
122.272988371083)) ;
#63176=CARTESIAN_POINT('Ctrl Pts',(-19.6505873376339,-43.3598676697556,
121.923617759925)) ;
#63177=CARTESIAN_POINT('Ctrl Pts',(-19.6023104651923,-43.1798785893927,
122.221256110046)) ;
#63178=CARTESIAN_POINT('Ctrl Pts',(-19.3874126433953,-43.3699094040375,
121.904584247529)) ;
#63179=CARTESIAN_POINT('Ctrl Pts',(-19.391770525899,-43.1899203236746,122.206031467427)) ;
#63180=CARTESIAN_POINT('Ctrl Pts',(-19.1304837624484,-43.3797348299866,
121.930388446646)) ;
#63181=CARTESIAN_POINT('Ctrl Pts',(-19.1862281367957,-43.1997457496237,
122.226676884756)) ;
#63182=CARTESIAN_POINT('Ctrl Pts',(-18.876016923458,-43.3897916565143,122.001672516022)) ;
#63183=CARTESIAN_POINT('Ctrl Pts',(-18.9826551632411,-43.2098025761514,
122.283706165014)) ;
#63184=CARTESIAN_POINT('Ctrl Pts',(-18.6409865992809,-43.3997190896358,
122.114930897131)) ;
#63185=CARTESIAN_POINT('Ctrl Pts',(-18.7946320604858,-43.219730009273,122.374314665372)) ;
#63186=CARTESIAN_POINT('Ctrl Pts',(-18.428277440835,-43.4096690820421,122.267013929381)) ;
#63187=CARTESIAN_POINT('Ctrl Pts',(-18.6244661072569,-43.2296800016792,
122.495982618452)) ;
#63188=CARTESIAN_POINT('Ctrl Pts',(-18.2436237169547,-43.4197242831161,
122.456000772691)) ;
#63189=CARTESIAN_POINT('Ctrl Pts',(-18.4767445661238,-43.2397352027532,
122.647173618493)) ;
#63190=CARTESIAN_POINT('Ctrl Pts',(-18.0976352137637,-43.4295465571684,
122.668893815947)) ;
#63191=CARTESIAN_POINT('Ctrl Pts',(-18.3599557989295,-43.2495574768055,
122.817488687827)) ;
#63192=CARTESIAN_POINT('Ctrl Pts',(-17.987876075402,-43.4396024511276,122.909259308021)) ;
#63193=CARTESIAN_POINT('Ctrl Pts',(-18.272150254971,-43.2596133707647,123.009781985742)) ;
#63194=CARTESIAN_POINT('Ctrl Pts',(-17.9227225617815,-43.4495431729727,
123.162245934171)) ;
#63195=CARTESIAN_POINT('Ctrl Pts',(-18.2200294874287,-43.2695540926099,
123.212171536294)) ;
#63196=CARTESIAN_POINT('Ctrl Pts',(-17.9017472036595,-43.4594475170593,
123.421680109374)) ;
#63197=CARTESIAN_POINT('Ctrl Pts',(-18.2032511636437,-43.2794584366965,
123.41971860684)) ;
#63198=CARTESIAN_POINT('Ctrl Pts',(-17.926651728431,-43.4694941843588,123.684496298927)) ;
#63199=CARTESIAN_POINT('Ctrl Pts',(-18.2231767399461,-43.2895051039959,
123.629971456514)) ;
#63200=CARTESIAN_POINT('Ctrl Pts',(-17.9955444787495,-43.4793897428087,
123.935293204385)) ;
#63201=CARTESIAN_POINT('Ctrl Pts',(-18.2782926706353,-43.2994006624459,
123.830608021522)) ;
#63202=CARTESIAN_POINT('Ctrl Pts',(-18.1087774586024,-43.4894518215134,
124.174200467457)) ;
#63203=CARTESIAN_POINT('Ctrl Pts',(-18.3688808575243,-43.3094627411505,
124.021733139343)) ;
#63204=CARTESIAN_POINT('Ctrl Pts',(-18.258354480537,-43.4992945199792,124.38525663974)) ;
#63205=CARTESIAN_POINT('Ctrl Pts',(-18.4885436261305,-43.3193054396163,
124.19057641101)) ;
#63206=CARTESIAN_POINT('Ctrl Pts',(-18.4445910638163,-43.5092852938737,
124.570269448432)) ;
#63207=CARTESIAN_POINT('Ctrl Pts',(-18.6375340693141,-43.3292962135108,
124.338585274364)) ;
#63208=CARTESIAN_POINT('Ctrl Pts',(-18.6588280253988,-43.5192131631086,
124.719179491474)) ;
#63209=CARTESIAN_POINT('Ctrl Pts',(-18.8089243549263,-43.3392240827457,
124.457711595414)) ;
#63210=CARTESIAN_POINT('Ctrl Pts',(-18.8969249830435,-43.5292018920784,
124.829722059016)) ;
#63211=CARTESIAN_POINT('Ctrl Pts',(-18.9994025173376,-43.3492128117156,
124.546144008221)) ;
#63212=CARTESIAN_POINT('Ctrl Pts',(-19.1519853155007,-43.5392412940622,
124.897107996918)) ;
#63213=CARTESIAN_POINT('Ctrl Pts',(-19.2034513317484,-43.3592522136993,
124.600051019993)) ;
#63214=CARTESIAN_POINT('Ctrl Pts',(-19.4096395220042,-43.549081461799,124.91925607013)) ;
#63215=CARTESIAN_POINT('Ctrl Pts',(-19.4095740497206,-43.3690923814361,
124.617767680726)) ;
#63216=CARTESIAN_POINT('Ctrl Pts',(-19.6726790143965,-43.5591296721735,
124.896233588286)) ;
#63217=CARTESIAN_POINT('Ctrl Pts',(-19.6200056228297,-43.3791405918106,
124.599348022425)) ;
#63218=CARTESIAN_POINT('Ctrl Pts',(-19.9250688422305,-43.5690768424612,
124.828171804027)) ;
#63219=CARTESIAN_POINT('Ctrl Pts',(-19.8219167126913,-43.3890877620984,
124.544896996661)) ;
#63220=CARTESIAN_POINT('Ctrl Pts',(-20.1612764162791,-43.5789876907163,
124.718431010593)) ;
#63221=CARTESIAN_POINT('Ctrl Pts',(-20.0108816130576,-43.3989986103534,
124.457103131757)) ;
#63222=CARTESIAN_POINT('Ctrl Pts',(-20.3778135163567,-43.5890440183941,
124.566965650242)) ;
#63223=CARTESIAN_POINT('Ctrl Pts',(-20.1841104958632,-43.4090549380312,
124.335929390239)) ;
#63224=CARTESIAN_POINT('Ctrl Pts',(-20.561112631005,-43.5988944311626,124.384166137477)) ;
#63225=CARTESIAN_POINT('Ctrl Pts',(-20.3307480642774,-43.4189053507997,
124.189689229524)) ;
#63226=CARTESIAN_POINT('Ctrl Pts',(-20.7130674436225,-43.6089213169963,
124.168903399289)) ;
#63227=CARTESIAN_POINT('Ctrl Pts',(-20.4523107179373,-43.4289322366334,
124.017478157488)) ;
#63228=CARTESIAN_POINT('Ctrl Pts',(-20.8247441401648,-43.6189499326271,
123.930180059024)) ;
#63229=CARTESIAN_POINT('Ctrl Pts',(-20.5416506341111,-43.4389608522643,
123.82649874937)) ;
#63230=CARTESIAN_POINT('Ctrl Pts',(-20.8924859435401,-43.6287951560046,
123.680497788512)) ;
#63231=CARTESIAN_POINT('Ctrl Pts',(-20.5958423726042,-43.4488060756417,
123.626753399107)) ;
#63232=CARTESIAN_POINT('Ctrl Pts',(-20.9168945752152,-43.6387858381062,
123.419083293922)) ;
#63233=CARTESIAN_POINT('Ctrl Pts',(-20.6153678869585,-43.4587967577433,
123.417621830856)) ;
#63234=CARTESIAN_POINT('Ctrl Pts',(-20.8948561360059,-43.6488237267386,
123.156223171646)) ;
#63235=CARTESIAN_POINT('Ctrl Pts',(-20.5977356311787,-43.4688346463758,
123.207333751848)) ;
#63236=CARTESIAN_POINT('Ctrl Pts',(-20.8292438813552,-43.6586680618418,
122.905971997117)) ;
#63237=CARTESIAN_POINT('Ctrl Pts',(-20.5452447033601,-43.4786789814789,
123.00713407774)) ;
#63238=CARTESIAN_POINT('Ctrl Pts',(-20.7201211840109,-43.6686530240393,
122.667383970185)) ;
#63239=CARTESIAN_POINT('Ctrl Pts',(-20.4579454445687,-43.4886639436764,
122.816264379379)) ;
#63240=CARTESIAN_POINT('Ctrl Pts',(-20.5719738572654,-43.6785919655727,
122.452232949088)) ;
#63241=CARTESIAN_POINT('Ctrl Pts',(-20.3394267805854,-43.4986028852098,
122.644144644649)) ;
#63242=CARTESIAN_POINT('Ctrl Pts',(-20.3868068904669,-43.6886338505441,
122.264249292356)) ;
#63243=CARTESIAN_POINT('Ctrl Pts',(-20.1912922023766,-43.5086447701812,
122.493758541871)) ;
#63244=CARTESIAN_POINT('Ctrl Pts',(-20.1751934660884,-43.6985203984524,
122.113473137318)) ;
#63245=CARTESIAN_POINT('Ctrl Pts',(-20.0220013410477,-43.5185313180895,
122.373139073177)) ;
#63246=CARTESIAN_POINT('Ctrl Pts',(-19.9382875919748,-43.7085143239524,
122.000193047115)) ;
#63247=CARTESIAN_POINT('Ctrl Pts',(-19.8324762632877,-43.5285252435895,
122.282516123217)) ;
#63248=CARTESIAN_POINT('Ctrl Pts',(-19.6867374287566,-43.7184504150789,
121.930037797555)) ;
#63249=CARTESIAN_POINT('Ctrl Pts',(-19.631236272687,-43.538461334716,122.226393150879)) ;
#63250=CARTESIAN_POINT('Ctrl Pts',(-19.4244597082895,-43.7284796840588,
121.904445450491)) ;
#63251=CARTESIAN_POINT('Ctrl Pts',(-19.4214139225834,-43.5484906036959,
122.205920422987)) ;
#63252=CARTESIAN_POINT('Ctrl Pts',(-19.1654713412245,-43.7383620666181,
121.924160359803)) ;
#63253=CARTESIAN_POINT('Ctrl Pts',(-19.2142241183985,-43.5583729862552,
122.221693371168)) ;
#63254=CARTESIAN_POINT('Ctrl Pts',(-18.909564469388,-43.748414583706,121.989548406113)) ;
#63255=CARTESIAN_POINT('Ctrl Pts',(-19.0094986897132,-43.5684255033431,
122.274004889728)) ;
#63256=CARTESIAN_POINT('Ctrl Pts',(-18.672555542748,-43.7583087045299,122.096577505371)) ;
#63257=CARTESIAN_POINT('Ctrl Pts',(-18.8198926461261,-43.578319624167,122.359628808823)) ;
#63258=CARTESIAN_POINT('Ctrl Pts',(-18.4541166120411,-43.7683706839503,
122.245521781435)) ;
#63259=CARTESIAN_POINT('Ctrl Pts',(-18.6451418602276,-43.5883816035874,
122.478785221664)) ;
#63260=CARTESIAN_POINT('Ctrl Pts',(-18.2688956918944,-43.7782152171792,
122.426149066543)) ;
#63261=CARTESIAN_POINT('Ctrl Pts',(-18.4969665901332,-43.5982261368164,
122.623287037953)) ;
#63262=CARTESIAN_POINT('Ctrl Pts',(-18.1153222214896,-43.7881752960855,
122.63809537997)) ;
#63263=CARTESIAN_POINT('Ctrl Pts',(-18.3741086705153,-43.6081862157226,
122.792844257825)) ;
#63264=CARTESIAN_POINT('Ctrl Pts',(-18.0004538039104,-43.7982135726581,
122.875554226971)) ;
#63265=CARTESIAN_POINT('Ctrl Pts',(-18.2822147043336,-43.6182244922952,
122.982811851236)) ;
#63266=CARTESIAN_POINT('Ctrl Pts',(-17.9292494152414,-43.8080869591959,
123.125095646778)) ;
#63267=CARTESIAN_POINT('Ctrl Pts',(-18.225252205665,-43.6280978788331,123.182444339761)) ;
#63268=CARTESIAN_POINT('Ctrl Pts',(-17.902000155212,-43.818159901963,123.388344568531)) ;
#63269=CARTESIAN_POINT('Ctrl Pts',(-18.2034535746662,-43.6381708216001,
123.393043900429)) ;
#63270=CARTESIAN_POINT('Ctrl Pts',(-17.9200947062017,-43.8279813160913,
123.645856942376)) ;
#63271=CARTESIAN_POINT('Ctrl Pts',(-18.2179298642884,-43.6479922357285,
123.599052510802)) ;
#63272=CARTESIAN_POINT('Ctrl Pts',(-17.9839061111706,-43.8380559461636,
123.902752660032)) ;
#63273=CARTESIAN_POINT('Ctrl Pts',(-18.2689797188223,-43.6580668658008,
123.804569272354)) ;
#63274=CARTESIAN_POINT('Ctrl Pts',(-18.0892674357171,-43.8479225834805,
124.139701464723)) ;
#63275=CARTESIAN_POINT('Ctrl Pts',(-18.353269010714,-43.6679335031176,123.99412714447)) ;
#63276=CARTESIAN_POINT('Ctrl Pts',(-18.2358881550822,-43.8579461288523,
124.358516056916)) ;
#63277=CARTESIAN_POINT('Ctrl Pts',(-18.4705660406864,-43.6779570484894,
124.169178557313)) ;
#63278=CARTESIAN_POINT('Ctrl Pts',(-18.4187926357899,-43.8679718803695,
124.54817037461)) ;
#63279=CARTESIAN_POINT('Ctrl Pts',(-18.6168901651521,-43.6879828000066,
124.320901587011)) ;
#63280=CARTESIAN_POINT('Ctrl Pts',(-18.6279123309116,-43.8778254673789,
124.700856473428)) ;
#63281=CARTESIAN_POINT('Ctrl Pts',(-18.7841853999482,-43.697836387016,124.443049376181)) ;
#63282=CARTESIAN_POINT('Ctrl Pts',(-18.8629865023443,-43.8878024276068,
124.816974766263)) ;
#63283=CARTESIAN_POINT('Ctrl Pts',(-18.9722446774819,-43.7078133472439,
124.535943532528)) ;
#63284=CARTESIAN_POINT('Ctrl Pts',(-19.1158727506149,-43.8978235706353,
124.890405499117)) ;
#63285=CARTESIAN_POINT('Ctrl Pts',(-19.1745538313907,-43.7178344902724,
124.594687628449)) ;
#63286=CARTESIAN_POINT('Ctrl Pts',(-19.3740398930884,-43.9077061766552,
124.918943559724)) ;
#63287=CARTESIAN_POINT('Ctrl Pts',(-19.3810867133437,-43.7277170962923,
124.617517603467)) ;
#63288=CARTESIAN_POINT('Ctrl Pts',(-19.6380282810842,-43.9177746472879,
124.901808568913)) ;
#63289=CARTESIAN_POINT('Ctrl Pts',(-19.5922777253755,-43.737785566925,124.603809182427)) ;
#63290=CARTESIAN_POINT('Ctrl Pts',(-19.889104080618,-43.9276047304716,124.840852015822)) ;
#63291=CARTESIAN_POINT('Ctrl Pts',(-19.7931370891346,-43.7476156501087,
124.555043909552)) ;
#63292=CARTESIAN_POINT('Ctrl Pts',(-20.1315321754818,-43.937671290152,124.735084209406)) ;
#63293=CARTESIAN_POINT('Ctrl Pts',(-19.9870797585783,-43.7576822097891,
124.470429312396)) ;
#63294=CARTESIAN_POINT('Ctrl Pts',(-20.3480256593167,-43.9475615399812,
124.591215461382)) ;
#63295=CARTESIAN_POINT('Ctrl Pts',(-20.1602736880261,-43.7675724596183,
124.355334538994)) ;
#63296=CARTESIAN_POINT('Ctrl Pts',(-20.5385520107773,-43.95755370573,124.41054400151)) ;
#63297=CARTESIAN_POINT('Ctrl Pts',(-20.3126945474677,-43.7775646253671,
124.210797386208)) ;
#63298=CARTESIAN_POINT('Ctrl Pts',(-20.6941599747678,-43.9675165493261,
124.199999732193)) ;
#63299=CARTESIAN_POINT('Ctrl Pts',(-20.4371805360489,-43.7875274689632,
124.042362141687)) ;
#63300=CARTESIAN_POINT('Ctrl Pts',(-20.8107661786076,-43.9774207181539,
123.967284902334)) ;
#63301=CARTESIAN_POINT('Ctrl Pts',(-20.5304651300537,-43.797431637791,123.856190933871)) ;
#63302=CARTESIAN_POINT('Ctrl Pts',(-20.8861267321908,-43.9874815930482,
123.713900101275)) ;
#63303=CARTESIAN_POINT('Ctrl Pts',(-20.5907535610701,-43.8074925126853,
123.653482792957)) ;
#63304=CARTESIAN_POINT('Ctrl Pts',(-20.9160480543138,-43.9973204963776,
123.457038808334)) ;
#63305=CARTESIAN_POINT('Ctrl Pts',(-20.6146904768429,-43.8173314160147,
123.44799493269)) ;
#63306=CARTESIAN_POINT('Ctrl Pts',(-20.9008215569112,-44.0073888727515,
123.192934464757)) ;
#63307=CARTESIAN_POINT('Ctrl Pts',(-20.6025093217577,-43.8273997923886,
123.236711133605)) ;
#63308=CARTESIAN_POINT('Ctrl Pts',(-20.8409996767229,-44.0172694893841,
122.940227571329)) ;
#63309=CARTESIAN_POINT('Ctrl Pts',(-20.5546520629352,-43.8372804090212,
123.034546490848)) ;
#63310=CARTESIAN_POINT('Ctrl Pts',(-20.7375752826336,-44.0272606496131,
122.698940269794)) ;
#63311=CARTESIAN_POINT('Ctrl Pts',(-20.4719127723535,-43.8472715692502,
122.841516743795)) ;
#63312=CARTESIAN_POINT('Ctrl Pts',(-20.5943672382838,-44.0372137230452,
122.480025241818)) ;
#63313=CARTESIAN_POINT('Ctrl Pts',(-20.357346713871,-43.8572246426823,122.666384965214)) ;
#63314=CARTESIAN_POINT('Ctrl Pts',(-20.413814021043,-44.0472495586578,122.28781904818)) ;
#63315=CARTESIAN_POINT('Ctrl Pts',(-20.212904171313,-43.867260478295,122.512619815452)) ;
#63316=CARTESIAN_POINT('Ctrl Pts',(-20.2057716275745,-44.057139685388,122.132010547474)) ;
#63317=CARTESIAN_POINT('Ctrl Pts',(-20.0464710629452,-43.8771506050251,
122.387973367554)) ;
#63318=CARTESIAN_POINT('Ctrl Pts',(-19.9716606492844,-44.0671318671573,
122.013118819397)) ;
#63319=CARTESIAN_POINT('Ctrl Pts',(-19.8591825691405,-43.8871427867944,
122.292859783673)) ;
#63320=CARTESIAN_POINT('Ctrl Pts',(-19.721585969689,-44.0770778071318,121.93711664901)) ;
#63321=CARTESIAN_POINT('Ctrl Pts',(-19.6591233631449,-43.8970887267689,
122.232057912344)) ;
#63322=CARTESIAN_POINT('Ctrl Pts',(-19.4621316011703,-44.0870249908912,
121.905158079447)) ;
#63323=CARTESIAN_POINT('Ctrl Pts',(-19.4515603759915,-43.9070359105284,
122.206490695908)) ;
#63324=CARTESIAN_POINT('Ctrl Pts',(-19.1984633098486,-44.0970729291816,
121.91916626143)) ;
#63325=CARTESIAN_POINT('Ctrl Pts',(-19.2406255245606,-43.9170838488187,
122.217696907762)) ;
#63326=CARTESIAN_POINT('Ctrl Pts',(-18.9462999517132,-44.1069205639951,
121.977344862777)) ;
#63327=CARTESIAN_POINT('Ctrl Pts',(-19.0388958389278,-43.9269314836323,
122.264239147175)) ;
#63328=CARTESIAN_POINT('Ctrl Pts',(-18.7050030349617,-44.1168822776931,
122.078833023626)) ;
#63329=CARTESIAN_POINT('Ctrl Pts',(-18.8458584060323,-43.9368931973302,
122.345428976242)) ;
#63330=CARTESIAN_POINT('Ctrl Pts',(-18.4836721334991,-44.1269109135143,
122.221925767037)) ;
#63331=CARTESIAN_POINT('Ctrl Pts',(-18.6687933369296,-43.9469218331514,
122.459902775154)) ;
#63332=CARTESIAN_POINT('Ctrl Pts',(-18.2927904240574,-44.136821228266,122.39907817817)) ;
#63333=CARTESIAN_POINT('Ctrl Pts',(-18.5160881141208,-43.9568321479032,
122.601623829949)) ;
#63334=CARTESIAN_POINT('Ctrl Pts',(-18.1346189321038,-44.1467560989287,
122.60679979726)) ;
#63335=CARTESIAN_POINT('Ctrl Pts',(-18.3895506742922,-43.9667670185658,
122.767800273057)) ;
#63336=CARTESIAN_POINT('Ctrl Pts',(-18.0138706731733,-44.1567972813305,
122.841409864127)) ;
#63337=CARTESIAN_POINT('Ctrl Pts',(-18.2929514212946,-43.9768082009676,
122.955488165132)) ;
#63338=CARTESIAN_POINT('Ctrl Pts',(-17.9366823755265,-44.1666842527952,
123.089522740013)) ;
#63339=CARTESIAN_POINT('Ctrl Pts',(-18.2312003631439,-43.9866951724323,
123.153977453905)) ;
#63340=CARTESIAN_POINT('Ctrl Pts',(-17.903048419426,-44.1766836850578,123.350101781409)) ;
#63341=CARTESIAN_POINT('Ctrl Pts',(-18.2042924372665,-43.9966946046949,
123.36244046689)) ;
#63342=CARTESIAN_POINT('Ctrl Pts',(-17.9149014701427,-44.1866037503144,
123.610552838708)) ;
#63343=CARTESIAN_POINT('Ctrl Pts',(-18.213774030704,-44.0066146699516,123.570800751409)) ;
#63344=CARTESIAN_POINT('Ctrl Pts',(-17.9724055290717,-44.1966406028986,
123.867950986159)) ;
#63345=CARTESIAN_POINT('Ctrl Pts',(-18.2597764896288,-44.0166515225357,
123.776719574248)) ;
#63346=CARTESIAN_POINT('Ctrl Pts',(-18.072489495965,-44.2065532622386,124.10845708331)) ;
#63347=CARTESIAN_POINT('Ctrl Pts',(-18.33984264497,-44.0265641818757,123.969124165985)) ;
#63348=CARTESIAN_POINT('Ctrl Pts',(-18.2134492761814,-44.2165444741535,
124.329987229818)) ;
#63349=CARTESIAN_POINT('Ctrl Pts',(-18.4526095642665,-44.0365553937906,
124.146348659042)) ;
#63350=CARTESIAN_POINT('Ctrl Pts',(-18.3920400927921,-44.2265861155566,
124.524226386298)) ;
#63351=CARTESIAN_POINT('Ctrl Pts',(-18.5954817048883,-44.0465970351937,
124.301740649263)) ;
#63352=CARTESIAN_POINT('Ctrl Pts',(-18.5968513118657,-44.2364149097636,
124.681658511536)) ;
#63353=CARTESIAN_POINT('Ctrl Pts',(-18.7593291698146,-44.0564258294008,
124.427686424433)) ;
#63354=CARTESIAN_POINT('Ctrl Pts',(-18.8315253713429,-44.2464913208849,
124.804205426187)) ;
#63355=CARTESIAN_POINT('Ctrl Pts',(-18.9470682569457,-44.066502240522,124.525725008789)) ;
#63356=CARTESIAN_POINT('Ctrl Pts',(-19.0783578845555,-44.2563434539274,
124.882525081973)) ;
#63357=CARTESIAN_POINT('Ctrl Pts',(-19.1445330139973,-44.0763543735645,
124.588381422117)) ;
#63358=CARTESIAN_POINT('Ctrl Pts',(-19.3406710042076,-44.2664166882687,
124.917774928891)) ;
#63359=CARTESIAN_POINT('Ctrl Pts',(-19.3543836827224,-44.0864276079058,
124.616582420438)) ;
#63360=CARTESIAN_POINT('Ctrl Pts',(-19.5990935689742,-44.2762581895953,
124.907117526406)) ;
#63361=CARTESIAN_POINT('Ctrl Pts',(-19.5611207373312,-44.0962691092324,
124.608057610087)) ;
#63362=CARTESIAN_POINT('Ctrl Pts',(-19.8549900005199,-44.2862191411901,
124.852048007979)) ;
#63363=CARTESIAN_POINT('Ctrl Pts',(-19.7658378370726,-44.1062300608272,
124.56400332464)) ;
#63364=CARTESIAN_POINT('Ctrl Pts',(-20.0991093096047,-44.2962569589108,
124.752132918042)) ;
#63365=CARTESIAN_POINT('Ctrl Pts',(-19.9611338268518,-44.1162678785479,
124.484072297486)) ;
#63366=CARTESIAN_POINT('Ctrl Pts',(-20.3188305768388,-44.3061313081678,
124.61402724624)) ;
#63367=CARTESIAN_POINT('Ctrl Pts',(-20.1369108352661,-44.1261422278049,
124.373589272937)) ;
#63368=CARTESIAN_POINT('Ctrl Pts',(-20.5149750943613,-44.31620085891,124.436460091646)) ;
#63369=CARTESIAN_POINT('Ctrl Pts',(-20.2938275119669,-44.1362117785471,
124.231536305792)) ;
#63370=CARTESIAN_POINT('Ctrl Pts',(-20.6736665782886,-44.3260348784186,
124.232462693714)) ;
#63371=CARTESIAN_POINT('Ctrl Pts',(-20.4207810991636,-44.1460457980557,
124.068340001014)) ;
#63372=CARTESIAN_POINT('Ctrl Pts',(-20.7975823820433,-44.3360690329981,
123.999722159393)) ;
#63373=CARTESIAN_POINT('Ctrl Pts',(-20.5199150654758,-44.1560799526353,
123.88214817752)) ;
#63374=CARTESIAN_POINT('Ctrl Pts',(-20.8784453196383,-44.3460849588206,
123.749227159064)) ;
#63375=CARTESIAN_POINT('Ctrl Pts',(-20.5846066615164,-44.1660958784577,
123.681752589755)) ;
#63376=CARTESIAN_POINT('Ctrl Pts',(-20.914563804666,-44.3559672140149,123.492051220715)) ;
#63377=CARTESIAN_POINT('Ctrl Pts',(-20.613502746607,-44.175978133652,123.476012754182)) ;
#63378=CARTESIAN_POINT('Ctrl Pts',(-20.9057075528016,-44.3659560205258,
123.229734225039)) ;
#63379=CARTESIAN_POINT('Ctrl Pts',(-20.6064192252653,-44.1859669401629,
123.266159268691)) ;
#63380=CARTESIAN_POINT('Ctrl Pts',(-20.8518375941005,-44.3759045877885,
122.973864298052)) ;
#63381=CARTESIAN_POINT('Ctrl Pts',(-20.563324813657,-44.1959155074256,123.061463372867)) ;
#63382=CARTESIAN_POINT('Ctrl Pts',(-20.7530825570645,-44.3859593930905,
122.728813985344)) ;
#63383=CARTESIAN_POINT('Ctrl Pts',(-20.4843220736738,-44.2059703127276,
122.86542241497)) ;
#63384=CARTESIAN_POINT('Ctrl Pts',(-20.616855401469,-44.3957781763541,122.509662800884)) ;
#63385=CARTESIAN_POINT('Ctrl Pts',(-20.3753421837085,-44.2157890959912,
122.690101516828)) ;
#63386=CARTESIAN_POINT('Ctrl Pts',(-20.4413805689007,-44.4058139487147,
122.312790934125)) ;
#63387=CARTESIAN_POINT('Ctrl Pts',(-20.2349635031074,-44.2258248683518,
122.532602849493)) ;
#63388=CARTESIAN_POINT('Ctrl Pts',(-20.2341379246685,-44.4158386477433,
122.150140067367)) ;
#63389=CARTESIAN_POINT('Ctrl Pts',(-20.0691703136329,-44.2358495673804,
122.402480945821)) ;
#63390=CARTESIAN_POINT('Ctrl Pts',(-20.0060783372853,-44.4256906510024,
122.027581366541)) ;
#63391=CARTESIAN_POINT('Ctrl Pts',(-19.8867241261111,-44.2457015706395,
122.304432930007)) ;
#63392=CARTESIAN_POINT('Ctrl Pts',(-19.7568956897588,-44.4356815853996,
121.944970803461)) ;
#63393=CARTESIAN_POINT('Ctrl Pts',(-19.6873786743973,-44.2556925050367,
122.238342904726)) ;
#63394=CARTESIAN_POINT('Ctrl Pts',(-19.4990141869541,-44.4455995078307,
121.906980973465)) ;
#63395=CARTESIAN_POINT('Ctrl Pts',(-19.4810741764347,-44.2656104274678,
122.207949395468)) ;
#63396=CARTESIAN_POINT('Ctrl Pts',(-19.2356052976764,-44.455627863513,121.914367687928)) ;
#63397=CARTESIAN_POINT('Ctrl Pts',(-19.2703469878274,-44.2756387831502,
122.213857026739)) ;
#63398=CARTESIAN_POINT('Ctrl Pts',(-18.9811319610234,-44.4655121480236,
121.966499520298)) ;
#63399=CARTESIAN_POINT('Ctrl Pts',(-19.0667685443539,-44.2855230676607,
122.255560647816)) ;
#63400=CARTESIAN_POINT('Ctrl Pts',(-18.7367176525546,-44.4755048319315,
122.06251590164)) ;
#63401=CARTESIAN_POINT('Ctrl Pts',(-18.871236522365,-44.2955157515686,122.332371983472)) ;
#63402=CARTESIAN_POINT('Ctrl Pts',(-18.5121188960608,-44.4855335689392,
122.20040107881)) ;
#63403=CARTESIAN_POINT('Ctrl Pts',(-18.6915565682666,-44.3055444885763,
122.442678613519)) ;
#63404=CARTESIAN_POINT('Ctrl Pts',(-18.3174591681186,-44.4954189655681,
122.372439116343)) ;
#63405=CARTESIAN_POINT('Ctrl Pts',(-18.5358279827225,-44.3154298852052,
122.580307299376)) ;
#63406=CARTESIAN_POINT('Ctrl Pts',(-18.1536797930773,-44.505406850982,122.577508760622)) ;
#63407=CARTESIAN_POINT('Ctrl Pts',(-18.4048030832296,-44.3254177706191,
122.744361731314)) ;
#63408=CARTESIAN_POINT('Ctrl Pts',(-18.0283271818904,-44.5153575536426,
122.807042074314)) ;
#63409=CARTESIAN_POINT('Ctrl Pts',(-18.3045194438468,-44.3353684732797,
122.927987235333)) ;
#63410=CARTESIAN_POINT('Ctrl Pts',(-17.9441368874462,-44.52539787174,123.057070192369)) ;
#63411=CARTESIAN_POINT('Ctrl Pts',(-18.2371653982975,-44.3454087913771,
123.128009182656)) ;
#63412=CARTESIAN_POINT('Ctrl Pts',(-17.9050280766287,-44.5352724370732,
123.313629339727)) ;
#63413=CARTESIAN_POINT('Ctrl Pts',(-18.2058765291738,-44.3552833567104,
123.333255668068)) ;
#63414=CARTESIAN_POINT('Ctrl Pts',(-17.9108009163294,-44.5452720971343,
123.576303554644)) ;
#63415=CARTESIAN_POINT('Ctrl Pts',(-18.2104928246366,-44.3652830167714,
123.543394997243)) ;
#63416=CARTESIAN_POINT('Ctrl Pts',(-17.9614015776546,-44.555181092302,123.831785012484)) ;
#63417=CARTESIAN_POINT('Ctrl Pts',(-18.2509713159387,-44.3751920119392,
123.747780179525)) ;
#63418=CARTESIAN_POINT('Ctrl Pts',(-18.0570243118767,-44.5652358334653,
124.078057381489)) ;
#63419=CARTESIAN_POINT('Ctrl Pts',(-18.3274676754747,-44.3852467531024,
123.944798879371)) ;
#63420=CARTESIAN_POINT('Ctrl Pts',(-18.1910740418543,-44.5750944453791,
124.299808917657)) ;
#63421=CARTESIAN_POINT('Ctrl Pts',(-18.4347054549292,-44.3951053650162,
124.122200713057)) ;
#63422=CARTESIAN_POINT('Ctrl Pts',(-18.3650377633451,-44.5851625676584,
124.499103963352)) ;
#63423=CARTESIAN_POINT('Ctrl Pts',(-18.5738749680476,-44.4051734872955,
124.281638189971)) ;
#63424=CARTESIAN_POINT('Ctrl Pts',(-18.5666736485935,-44.5950180383616,
124.661680062319)) ;
#63425=CARTESIAN_POINT('Ctrl Pts',(-18.7351820039692,-44.4150289579987,
124.411700348019)) ;
#63426=CARTESIAN_POINT('Ctrl Pts',(-18.7962745857909,-44.605012897855,124.789218966965)) ;
#63427=CARTESIAN_POINT('Ctrl Pts',(-18.9188616496907,-44.4250238174921,
124.513733295613)) ;
#63428=CARTESIAN_POINT('Ctrl Pts',(-19.0456348868395,-44.6150441511969,
124.874734939455)) ;
#63429=CARTESIAN_POINT('Ctrl Pts',(-19.1183492174815,-44.435055070834,124.582148031688)) ;
#63430=CARTESIAN_POINT('Ctrl Pts',(-19.3017226630708,-44.62491085007,124.915389460278)) ;
#63431=CARTESIAN_POINT('Ctrl Pts',(-19.3232187005312,-44.4449217697071,
124.614673670169)) ;
#63432=CARTESIAN_POINT('Ctrl Pts',(-19.5641051552104,-44.6348976658212,
124.911339609303)) ;
#63433=CARTESIAN_POINT('Ctrl Pts',(-19.5331246292621,-44.4549085854583,
124.611435943813)) ;
#63434=CARTESIAN_POINT('Ctrl Pts',(-19.8208626335505,-44.6448448710167,
124.862095013778)) ;
#63435=CARTESIAN_POINT('Ctrl Pts',(-19.7385308356951,-44.4648557906538,
124.572042423977)) ;
#63436=CARTESIAN_POINT('Ctrl Pts',(-20.0674296681808,-44.6548878591429,
124.76803108169)) ;
#63437=CARTESIAN_POINT('Ctrl Pts',(-19.9357852426788,-44.4748987787801,
124.496793284832)) ;
#63438=CARTESIAN_POINT('Ctrl Pts',(-20.2900606909374,-44.6647552137644,
124.635070010698)) ;
#63439=CARTESIAN_POINT('Ctrl Pts',(-20.1138908853131,-44.4847661334015,
124.390426455139)) ;
#63440=CARTESIAN_POINT('Ctrl Pts',(-20.4886282483647,-44.6747211070625,
124.464326907893)) ;
#63441=CARTESIAN_POINT('Ctrl Pts',(-20.2727462890408,-44.4947320266996,
124.253833725483)) ;
#63442=CARTESIAN_POINT('Ctrl Pts',(-20.6553026894128,-44.6847448844386,
124.260328412907)) ;
#63443=CARTESIAN_POINT('Ctrl Pts',(-20.4060875193306,-44.5047558040757,
124.090636341466)) ;
#63444=CARTESIAN_POINT('Ctrl Pts',(-20.7828007334005,-44.6946704323703,
124.032794984382)) ;
#63445=CARTESIAN_POINT('Ctrl Pts',(-20.5080877807566,-44.5146813520074,
123.908610839297)) ;
#63446=CARTESIAN_POINT('Ctrl Pts',(-20.8695762747895,-44.7046109087913,
123.786387153745)) ;
#63447=CARTESIAN_POINT('Ctrl Pts',(-20.5775102739201,-44.5246218284284,
123.711485441995)) ;
#63448=CARTESIAN_POINT('Ctrl Pts',(-20.912400649323,-44.7146571184542,123.525895807852)) ;
#63449=CARTESIAN_POINT('Ctrl Pts',(-20.6117719585213,-44.5346680380913,
123.503092741529)) ;
#63450=CARTESIAN_POINT('Ctrl Pts',(-20.9096780311405,-44.724518375116,123.26674378884)) ;
#63451=CARTESIAN_POINT('Ctrl Pts',(-20.6095960943389,-44.5445292947531,
123.295771314812)) ;
#63452=CARTESIAN_POINT('Ctrl Pts',(-20.8618140135343,-44.7345120033913,
123.008558951118)) ;
#63453=CARTESIAN_POINT('Ctrl Pts',(-20.5713071019526,-44.5545229230284,
123.089223095259)) ;
#63454=CARTESIAN_POINT('Ctrl Pts',(-20.7705763697433,-44.7444374007015,
122.764165937578)) ;
#63455=CARTESIAN_POINT('Ctrl Pts',(-20.498319127258,-44.5644483203386,122.893707997254)) ;
#63456=CARTESIAN_POINT('Ctrl Pts',(-20.6369673169243,-44.7544653086117,
122.537064718162)) ;
#63457=CARTESIAN_POINT('Ctrl Pts',(-20.3914338502099,-44.5744762282489,
122.712025924337)) ;
#63458=CARTESIAN_POINT('Ctrl Pts',(-20.4685272889073,-44.7643516242809,
122.33921389434)) ;
#63459=CARTESIAN_POINT('Ctrl Pts',(-20.2566836019861,-44.584362543918,122.553743877924)) ;
#63460=CARTESIAN_POINT('Ctrl Pts',(-20.2655021977993,-44.7743832191847,
122.171124667766)) ;
#63461=CARTESIAN_POINT('Ctrl Pts',(-20.0942650101056,-44.5943941388218,
122.419270793338)) ;
#63462=CARTESIAN_POINT('Ctrl Pts',(-20.0398318506451,-44.7842654621364,
122.042531241798)) ;
#63463=CARTESIAN_POINT('Ctrl Pts',(-19.9137298912166,-44.6042763817735,
122.316394121493)) ;
#63464=CARTESIAN_POINT('Ctrl Pts',(-19.790980965489,-44.7943249331663,121.953425884434)) ;
#63465=CARTESIAN_POINT('Ctrl Pts',(-19.7146500072838,-44.6143358528034,
122.24510773456)) ;
#63466=CARTESIAN_POINT('Ctrl Pts',(-19.5353894138272,-44.8041913778294,
121.909764540214)) ;
#63467=CARTESIAN_POINT('Ctrl Pts',(-19.5101771563229,-44.6242022974665,
122.210176441665)) ;
#63468=CARTESIAN_POINT('Ctrl Pts',(-19.2734974473692,-44.8141575022781,
121.910332881293)) ;
#63469=CARTESIAN_POINT('Ctrl Pts',(-19.300663601662,-44.6341684219152,122.210628864892)) ;
#63470=CARTESIAN_POINT('Ctrl Pts',(-19.0140941942044,-44.8241877456692,
121.957079096099)) ;
#63471=CARTESIAN_POINT('Ctrl Pts',(-19.0931406459017,-44.6441986653064,
122.248023646285)) ;
#63472=CARTESIAN_POINT('Ctrl Pts',(-18.7699778546539,-44.8340807806223,
122.04657166839)) ;
#63473=CARTESIAN_POINT('Ctrl Pts',(-18.8978469009694,-44.6540917002594,
122.319615481204)) ;
#63474=CARTESIAN_POINT('Ctrl Pts',(-18.5415249218624,-44.8441316948591,
122.179088598224)) ;
#63475=CARTESIAN_POINT('Ctrl Pts',(-18.7150830028236,-44.6641426144963,
122.425627556527)) ;
#63476=CARTESIAN_POINT('Ctrl Pts',(-18.3427444001931,-44.8540215210837,
122.346531093265)) ;
#63477=CARTESIAN_POINT('Ctrl Pts',(-18.5560590226922,-44.6740324407208,
122.55957796272)) ;
#63478=CARTESIAN_POINT('Ctrl Pts',(-18.1174461021876,-44.8673563361306,
122.614979487024)) ;
#63479=CARTESIAN_POINT('Ctrl Pts',(-18.3758085267228,-44.6873672557678,
122.774344354257)) ;
#63480=CARTESIAN_POINT('Ctrl Pts',(-17.9686335760902,-44.8806334273021,
122.934896659141)) ;
#63481=CARTESIAN_POINT('Ctrl Pts',(-18.2567530298792,-44.7006443469392,
123.030306574973)) ;
#63482=CARTESIAN_POINT('Ctrl Pts',(-17.9076731562678,-44.8938817159004,
123.277709414345)) ;
#63483=CARTESIAN_POINT('Ctrl Pts',(-18.2079946998203,-44.7138926355375,
123.304511413503)) ;
#63484=CARTESIAN_POINT('Ctrl Pts',(-17.9074623164892,-44.9039365573945,
123.541899571283)) ;
#63485=CARTESIAN_POINT('Ctrl Pts',(-18.2078213171443,-44.7239474770316,
123.515872463229)) ;
#63486=CARTESIAN_POINT('Ctrl Pts',(-17.9516919899064,-44.913767546702,123.796479325853)) ;
#63487=CARTESIAN_POINT('Ctrl Pts',(-18.2432033587368,-44.7337784663392,
123.719534329518)) ;
#63488=CARTESIAN_POINT('Ctrl Pts',(-18.0414310833544,-44.9238441110252,
124.045563596302)) ;
#63489=CARTESIAN_POINT('Ctrl Pts',(-18.3149935556506,-44.7438550306624,
123.918803730498)) ;
#63490=CARTESIAN_POINT('Ctrl Pts',(-18.1701298255741,-44.9336934361592,
124.270160085588)) ;
#63491=CARTESIAN_POINT('Ctrl Pts',(-18.4179464132743,-44.7537043557963,
124.098479058977)) ;
#63492=CARTESIAN_POINT('Ctrl Pts',(-18.3940753258795,-44.9470414357965,
124.540160290177)) ;
#63493=CARTESIAN_POINT('Ctrl Pts',(-18.5971230250769,-44.7670523554336,
124.314496251429)) ;
#63494=CARTESIAN_POINT('Ctrl Pts',(-18.7539725180923,-44.963626195333,124.794623795617)) ;
#63495=CARTESIAN_POINT('Ctrl Pts',(-18.8849990055932,-44.7836371149701,
124.518050456276)) ;
#63496=CARTESIAN_POINT('Ctrl Pts',(-19.1783954643001,-44.9801947466811,
124.911954796591)) ;
#63497=CARTESIAN_POINT('Ctrl Pts',(-19.2246019623236,-44.8002056663183,
124.611932785891)) ;
#63498=CARTESIAN_POINT('Ctrl Pts',(-19.5295000394639,-44.9935545715001,
124.914496420765)) ;
#63499=CARTESIAN_POINT('Ctrl Pts',(-19.5054328311711,-44.8135654911373,
124.613960044086)) ;
#63500=CARTESIAN_POINT('Ctrl Pts',(-19.7862085515421,-45.0034599803308,
124.87135192276)) ;
#63501=CARTESIAN_POINT('Ctrl Pts',(-19.7108114579357,-44.8234708999679,
124.579447577859)) ;
#63502=CARTESIAN_POINT('Ctrl Pts',(-20.0329770475992,-45.0134200069148,
124.784181635824)) ;
#63503=CARTESIAN_POINT('Ctrl Pts',(-19.9082219143351,-44.833430926552,124.509714796774)) ;
#63504=CARTESIAN_POINT('Ctrl Pts',(-20.3365929403509,-45.0266775911001,
124.613239797289)) ;
#63505=CARTESIAN_POINT('Ctrl Pts',(-20.151128683135,-44.8466885107373,124.372952796465)) ;
#63506=CARTESIAN_POINT('Ctrl Pts',(-20.6530388478672,-45.0433288025948,
124.303846929761)) ;
#63507=CARTESIAN_POINT('Ctrl Pts',(-20.4042740591769,-44.8633397222319,
124.125452733239)) ;
#63508=CARTESIAN_POINT('Ctrl Pts',(-20.8822225928719,-45.0632470167051,
123.826665489803)) ;
#63509=CARTESIAN_POINT('Ctrl Pts',(-20.5876289589755,-44.8832579363422,
123.743704995004)) ;
#63510=CARTESIAN_POINT('Ctrl Pts',(-20.9358462100671,-45.0831247799259,
123.300999284693)) ;
#63511=CARTESIAN_POINT('Ctrl Pts',(-20.6305301436153,-44.9031356995631,
123.323172734801)) ;
#63512=CARTESIAN_POINT('Ctrl Pts',(-20.8055712371326,-45.1031374477131,
122.785395465323)) ;
#63513=CARTESIAN_POINT('Ctrl Pts',(-20.5263138314019,-44.9231483673502,
122.910688665346)) ;
#63514=CARTESIAN_POINT('Ctrl Pts',(-20.5104525719544,-45.1229499703797,
122.349160972193)) ;
#63515=CARTESIAN_POINT('Ctrl Pts',(-20.2902207745244,-44.9429608900168,
122.561698343085)) ;
#63516=CARTESIAN_POINT('Ctrl Pts',(-20.081167872577,-45.1429332703796,122.036595982268)) ;
#63517=CARTESIAN_POINT('Ctrl Pts',(-19.946794629083,-44.9629441900167,122.311643931763)) ;
#63518=CARTESIAN_POINT('Ctrl Pts',(-19.5729808270998,-45.1628275474809,
121.890260817414)) ;
#63519=CARTESIAN_POINT('Ctrl Pts',(-19.5402450431835,-44.982838467118,122.194572859151)) ;
#63520=CARTESIAN_POINT('Ctrl Pts',(-19.0443792388159,-45.1827603092387,
121.925363493254)) ;
#63521=CARTESIAN_POINT('Ctrl Pts',(-19.1173630609288,-45.0027712288758,
122.222652560923)) ;
#63522=CARTESIAN_POINT('Ctrl Pts',(-18.5588123388653,-45.2027263150034,
122.139444767471)) ;
#63523=CARTESIAN_POINT('Ctrl Pts',(-18.7289082955966,-45.0227372346405,
122.393915435072)) ;
#63524=CARTESIAN_POINT('Ctrl Pts',(-18.1768400075753,-45.2226048471683,
122.504512707876)) ;
#63525=CARTESIAN_POINT('Ctrl Pts',(-18.4233281318735,-45.0426157668054,
122.685968958821)) ;
#63526=CARTESIAN_POINT('Ctrl Pts',(-17.9412382746725,-45.2425445138286,
122.979165174917)) ;
#63527=CARTESIAN_POINT('Ctrl Pts',(-18.2348448067827,-45.0625554334657,
123.065690634958)) ;
#63528=CARTESIAN_POINT('Ctrl Pts',(-17.8817201357155,-45.262439388474,123.504633155352)) ;
#63529=CARTESIAN_POINT('Ctrl Pts',(-18.1872285519615,-45.0824503081111,
123.48606590208)) ;
#63530=CARTESIAN_POINT('Ctrl Pts',(-18.0046155637013,-45.2823465277673,
124.019136501102)) ;
#63531=CARTESIAN_POINT('Ctrl Pts',(-18.2855439122614,-45.1023574474044,
123.897669917515)) ;
#63532=CARTESIAN_POINT('Ctrl Pts',(-18.2951592685282,-45.3022570758458,
124.461637555377)) ;
#63533=CARTESIAN_POINT('Ctrl Pts',(-18.5179788419764,-45.1222679954829,
124.251671936744)) ;
#63534=CARTESIAN_POINT('Ctrl Pts',(-18.7231289192442,-45.322325661203,124.779793280886)) ;
#63535=CARTESIAN_POINT('Ctrl Pts',(-18.8603532666718,-45.1423365808401,
124.506196853283)) ;
#63536=CARTESIAN_POINT('Ctrl Pts',(-19.2267990765381,-45.3421074585177,
124.931211593154)) ;
#63537=CARTESIAN_POINT('Ctrl Pts',(-19.2632917257971,-45.1621183781549,
124.627332840506)) ;
#63538=CARTESIAN_POINT('Ctrl Pts',(-19.7575625515052,-45.3621150054623,
124.902127405188)) ;
#63539=CARTESIAN_POINT('Ctrl Pts',(-19.6879025560016,-45.1821259250994,
124.604065538221)) ;
#63540=CARTESIAN_POINT('Ctrl Pts',(-20.2423289587424,-45.3819367437651,
124.695488931146)) ;
#63541=CARTESIAN_POINT('Ctrl Pts',(-20.0757176520892,-45.2019476634022,
124.438753696871)) ;
#63542=CARTESIAN_POINT('Ctrl Pts',(-20.6310564599377,-45.4019167636693,
124.333814619466)) ;
#63543=CARTESIAN_POINT('Ctrl Pts',(-20.3866992414769,-45.2219276833064,
124.149413465804)) ;
#63544=CARTESIAN_POINT('Ctrl Pts',(-20.8717000555941,-45.4218342149315,
123.862278018821)) ;
#63545=CARTESIAN_POINT('Ctrl Pts',(-20.579213919715,-45.2418451345686,123.77218297004)) ;
#63546=CARTESIAN_POINT('Ctrl Pts',(-20.9380767680918,-45.4417091361042,
123.338188475184)) ;
#63547=CARTESIAN_POINT('Ctrl Pts',(-20.6323140215928,-45.2617200557413,
123.352909817565)) ;
#63548=CARTESIAN_POINT('Ctrl Pts',(-20.8204289201312,-45.461733504655,122.819174893006)) ;
#63549=CARTESIAN_POINT('Ctrl Pts',(-20.5381943820615,-45.2817444242922,
122.937699557393)) ;
#63550=CARTESIAN_POINT('Ctrl Pts',(-20.5348026192168,-45.4816001890285,
122.374971928378)) ;
#63551=CARTESIAN_POINT('Ctrl Pts',(-20.3096913007445,-45.3016111086656,
122.582336913759)) ;
#63552=CARTESIAN_POINT('Ctrl Pts',(-20.113737828752,-45.5015440108747,122.053072103722)) ;
#63553=CARTESIAN_POINT('Ctrl Pts',(-19.9728377986509,-45.3215549305118,
122.324818360673)) ;
#63554=CARTESIAN_POINT('Ctrl Pts',(-19.6089136734289,-45.5214513801262,
121.894620584429)) ;
#63555=CARTESIAN_POINT('Ctrl Pts',(-19.5689770139582,-45.3414622997634,
122.198058922414)) ;
#63556=CARTESIAN_POINT('Ctrl Pts',(-19.0811541092211,-45.5413260778729,
121.916926618997)) ;
#63557=CARTESIAN_POINT('Ctrl Pts',(-19.1467684454857,-45.3613369975101,
122.215906404225)) ;
#63558=CARTESIAN_POINT('Ctrl Pts',(-18.5899663032709,-45.5613080203947,
122.11896949238)) ;
#63559=CARTESIAN_POINT('Ctrl Pts',(-18.7538191655351,-45.3813189400318,
122.377543293856)) ;
#63560=CARTESIAN_POINT('Ctrl Pts',(-18.1991325996576,-45.5812106873055,
122.475351878754)) ;
#63561=CARTESIAN_POINT('Ctrl Pts',(-18.4411535104022,-45.4012216069426,
122.662651767787)) ;
#63562=CARTESIAN_POINT('Ctrl Pts',(-17.9525130136247,-45.6010660448442,
122.94198968938)) ;
#63563=CARTESIAN_POINT('Ctrl Pts',(-18.2438603264457,-45.4210769644813,
123.035964382293)) ;
#63564=CARTESIAN_POINT('Ctrl Pts',(-17.8797853306708,-45.6211300835602,
123.470193368152)) ;
#63565=CARTESIAN_POINT('Ctrl Pts',(-18.1856815073262,-45.4411410031973,
123.458527308833)) ;
#63566=CARTESIAN_POINT('Ctrl Pts',(-17.9907738386166,-45.6409852632853,
123.986308188026)) ;
#63567=CARTESIAN_POINT('Ctrl Pts',(-18.2744755604141,-45.4609961829224,
123.871419313323)) ;
#63568=CARTESIAN_POINT('Ctrl Pts',(-18.2724161799833,-45.6609653679497,
124.436265927067)) ;
#63569=CARTESIAN_POINT('Ctrl Pts',(-18.4997930441946,-45.4809762875868,
124.231383659367)) ;
#63570=CARTESIAN_POINT('Ctrl Pts',(-18.6870078952182,-45.6807744731195,
124.761025281335)) ;
#63571=CARTESIAN_POINT('Ctrl Pts',(-18.8314673456426,-45.5007853927566,
124.491189117074)) ;
#63572=CARTESIAN_POINT('Ctrl Pts',(-19.1916999501427,-45.7007670934602,
124.926741074859)) ;
#63573=CARTESIAN_POINT('Ctrl Pts',(-19.235230041018,-45.5207780130973,124.623756847041)) ;
#63574=CARTESIAN_POINT('Ctrl Pts',(-19.6312118173371,-45.7173065759643,
124.913196409966)) ;
#63575=CARTESIAN_POINT('Ctrl Pts',(-19.5868155436623,-45.5373174956014,
124.612921459841)) ;
#63576=CARTESIAN_POINT('Ctrl Pts',(-19.9674993568783,-45.7306708940285,
124.812112387644)) ;
#63577=CARTESIAN_POINT('Ctrl Pts',(-19.8558719099428,-45.5506818136656,
124.532044502846)) ;
#63578=CARTESIAN_POINT('Ctrl Pts',(-20.2779790594621,-45.74388849653,124.656227492421)) ;
#63579=CARTESIAN_POINT('Ctrl Pts',(-20.1042094374621,-45.5638994161671,
124.407362610249)) ;
#63580=CARTESIAN_POINT('Ctrl Pts',(-20.6088613725694,-45.7605460908078,
124.362235325753)) ;
#63581=CARTESIAN_POINT('Ctrl Pts',(-20.3689615158667,-45.5805570104449,
124.172135807522)) ;
#63582=CARTESIAN_POINT('Ctrl Pts',(-20.8603771681575,-45.7804117928495,
123.897882285973)) ;
#63583=CARTESIAN_POINT('Ctrl Pts',(-20.5701552926539,-45.6004227124867,
123.800652558022)) ;
#63584=CARTESIAN_POINT('Ctrl Pts',(-20.9262145451772,-45.7970415195396,
123.460911151536)) ;
#63585=CARTESIAN_POINT('Ctrl Pts',(-20.6228240067414,-45.6170524391767,
123.451100564137)) ;
#63586=CARTESIAN_POINT('Ctrl Pts',(-20.8869828199733,-45.8103306346774,
123.113835882224)) ;
#63587=CARTESIAN_POINT('Ctrl Pts',(-20.5914361114732,-45.6303415543145,
123.17341573683)) ;
#63588=CARTESIAN_POINT('Ctrl Pts',(-20.813137221631,-45.8202949816545,122.862628158048)) ;
#63589=CARTESIAN_POINT('Ctrl Pts',(-20.532359431995,-45.6403059012916,122.97245700907)) ;
#63590=CARTESIAN_POINT('Ctrl Pts',(-20.6973720958994,-45.830223349656,122.628822672111)) ;
#63591=CARTESIAN_POINT('Ctrl Pts',(-20.4397374777452,-45.6502342692931,
122.785404651052)) ;
#63592=CARTESIAN_POINT('Ctrl Pts',(-20.491036246019,-45.8435067827447,122.347203200446)) ;
#63593=CARTESIAN_POINT('Ctrl Pts',(-20.2747057229162,-45.6635177023819,
122.560148879039)) ;
#63594=CARTESIAN_POINT('Ctrl Pts',(-20.145826084982,-45.8601588604851,122.070280119537)) ;
#63595=CARTESIAN_POINT('Ctrl Pts',(-19.9984819208062,-45.6801697801222,
122.338567916265)) ;
#63596=CARTESIAN_POINT('Ctrl Pts',(-19.7294257177558,-45.8767102297859,
121.928426697341)) ;
#63597=CARTESIAN_POINT('Ctrl Pts',(-19.6654083759465,-45.696721149423,122.22511130924)) ;
#63598=CARTESIAN_POINT('Ctrl Pts',(-19.3810452958569,-45.8899976579349,
121.904492705596)) ;
#63599=CARTESIAN_POINT('Ctrl Pts',(-19.386670912546,-45.710008577572,122.205956446535)) ;
#63600=CARTESIAN_POINT('Ctrl Pts',(-19.1186091401649,-45.900042197635,121.932658291026)) ;
#63601=CARTESIAN_POINT('Ctrl Pts',(-19.1767289258844,-45.7200531172721,
122.228493281736)) ;
#63602=CARTESIAN_POINT('Ctrl Pts',(-18.8700233535146,-45.9098850394588,
122.00419504513)) ;
#63603=CARTESIAN_POINT('Ctrl Pts',(-18.9778591118884,-45.7298959590959,
122.285724283644)) ;
#63604=CARTESIAN_POINT('Ctrl Pts',(-18.6340661750229,-45.9198693237057,
122.118877741184)) ;
#63605=CARTESIAN_POINT('Ctrl Pts',(-18.7890948938155,-45.7398802433429,
122.377472601013)) ;
#63606=CARTESIAN_POINT('Ctrl Pts',(-18.4223444457942,-45.9298189691049,
122.272320772615)) ;
#63607=CARTESIAN_POINT('Ctrl Pts',(-18.6197187508759,-45.749829888742,122.500228781122)) ;
#63608=CARTESIAN_POINT('Ctrl Pts',(-18.2393318883207,-45.9398187307933,
122.460918444187)) ;
#63609=CARTESIAN_POINT('Ctrl Pts',(-18.4733104024896,-45.7598296504304,
122.65110845724)) ;
#63610=CARTESIAN_POINT('Ctrl Pts',(-18.0917505487203,-45.9498500767522,
122.679344429148)) ;
#63611=CARTESIAN_POINT('Ctrl Pts',(-18.3552472195982,-45.7698609963893,
122.825850469655)) ;
#63612=CARTESIAN_POINT('Ctrl Pts',(-17.9858757132729,-45.9597050312293,
122.915697062005)) ;
#63613=CARTESIAN_POINT('Ctrl Pts',(-18.2705494534768,-45.7797159508665,
123.014933412963)) ;
#63614=CARTESIAN_POINT('Ctrl Pts',(-17.9213083460971,-45.9696775692299,
123.1696585988)) ;
#63615=CARTESIAN_POINT('Ctrl Pts',(-18.218897762685,-45.789688488867,123.218103106479)) ;
#63616=CARTESIAN_POINT('Ctrl Pts',(-17.9017881316978,-45.9796725629648,
123.43163061832)) ;
#63617=CARTESIAN_POINT('Ctrl Pts',(-18.2032838339912,-45.7996834826019,
123.427680825471)) ;
#63618=CARTESIAN_POINT('Ctrl Pts',(-17.9284695515831,-45.9897066217589,
123.693939039804)) ;
#63619=CARTESIAN_POINT('Ctrl Pts',(-18.2246312126076,-45.809717541396,123.637527304085)) ;
#63620=CARTESIAN_POINT('Ctrl Pts',(-17.9986278342862,-45.9995619645819,
123.943270201395)) ;
#63621=CARTESIAN_POINT('Ctrl Pts',(-18.2807599457767,-45.819572884219,123.83699144443)) ;
#63622=CARTESIAN_POINT('Ctrl Pts',(-18.1123057056934,-46.0095614439275,
124.180132595263)) ;
#63623=CARTESIAN_POINT('Ctrl Pts',(-18.3717042256828,-45.8295723635646,
124.026480327799)) ;
#63624=CARTESIAN_POINT('Ctrl Pts',(-18.2635910838762,-46.0194558926828,
124.391666206078)) ;
#63625=CARTESIAN_POINT('Ctrl Pts',(-18.4927342046914,-45.8394668123199,
124.195705758367)) ;
#63626=CARTESIAN_POINT('Ctrl Pts',(-18.4524598572534,-46.0295190121173,
124.576699295059)) ;
#63627=CARTESIAN_POINT('Ctrl Pts',(-18.6438307990039,-45.8495299317544,
124.343730662622)) ;
#63628=CARTESIAN_POINT('Ctrl Pts',(-18.6656547763294,-46.0393586573585,
124.723094304069)) ;
#63629=CARTESIAN_POINT('Ctrl Pts',(-18.8143877068013,-45.8593695769957,
124.460844668667)) ;
#63630=CARTESIAN_POINT('Ctrl Pts',(-18.9061641632514,-46.0494218215446,
124.832954725746)) ;
#63631=CARTESIAN_POINT('Ctrl Pts',(-19.0067961563735,-45.8694327411817,
124.5487310367)) ;
#63632=CARTESIAN_POINT('Ctrl Pts',(-19.1579188977088,-46.0593160912934,
124.898075179652)) ;
#63633=CARTESIAN_POINT('Ctrl Pts',(-19.2082002369437,-45.8793270109305,
124.600825207935)) ;
#63634=CARTESIAN_POINT('Ctrl Pts',(-19.4182795982721,-46.0692578173072,
124.919290922679)) ;
#63635=CARTESIAN_POINT('Ctrl Pts',(-19.4164887608804,-45.8892687369444,
124.617795648672)) ;
#63636=CARTESIAN_POINT('Ctrl Pts',(-19.6800549445947,-46.0792607059666,
124.894933738321)) ;
#63637=CARTESIAN_POINT('Ctrl Pts',(-19.6259087706948,-45.8992716256037,
124.598307788373)) ;
#63638=CARTESIAN_POINT('Ctrl Pts',(-19.9343703358343,-46.0893005547606,
124.824788939864)) ;
#63639=CARTESIAN_POINT('Ctrl Pts',(-19.8293605316926,-45.9093114743977,
124.542189846149)) ;
#63640=CARTESIAN_POINT('Ctrl Pts',(-20.1678185633982,-46.0991247702215,
124.714495173511)) ;
#63641=CARTESIAN_POINT('Ctrl Pts',(-20.0161177505501,-45.9191356898586,
124.453953133522)) ;
#63642=CARTESIAN_POINT('Ctrl Pts',(-20.3837390423242,-46.109181613715,124.562135863679)) ;
#63643=CARTESIAN_POINT('Ctrl Pts',(-20.1888529869787,-45.9291925333521,
124.332063944319)) ;
#63644=CARTESIAN_POINT('Ctrl Pts',(-20.5673296043918,-46.119110223111,124.376727071012)) ;
#63645=CARTESIAN_POINT('Ctrl Pts',(-20.3357237457142,-45.9391211427481,
124.183735605175)) ;
#63646=CARTESIAN_POINT('Ctrl Pts',(-20.7168895335636,-46.1290621071489,
124.162174744986)) ;
#63647=CARTESIAN_POINT('Ctrl Pts',(-20.4553698831515,-45.949073026786,124.012092764765)) ;
#63648=CARTESIAN_POINT('Ctrl Pts',(-20.8275975547341,-46.1391150599565,
123.922329195858)) ;
#63649=CARTESIAN_POINT('Ctrl Pts',(-20.5439344348876,-45.9591259795936,
123.820215369618)) ;
#63650=CARTESIAN_POINT('Ctrl Pts',(-20.8939114402365,-46.1489379364227,
123.672837152796)) ;
#63651=CARTESIAN_POINT('Ctrl Pts',(-20.5969834127684,-45.9689488560598,
123.620621818295)) ;
#63652=CARTESIAN_POINT('Ctrl Pts',(-20.9168785394599,-46.1589936689928,
123.409601144836)) ;
#63653=CARTESIAN_POINT('Ctrl Pts',(-20.6153551246797,-45.9790045886299,
123.410032751232)) ;
#63654=CARTESIAN_POINT('Ctrl Pts',(-20.893591540016,-46.1689344339805,123.149398558187)) ;
#63655=CARTESIAN_POINT('Ctrl Pts',(-20.5967235160762,-45.9889453536176,
123.201871130652)) ;
#63656=CARTESIAN_POINT('Ctrl Pts',(-20.8265158340173,-46.1788387668861,
122.89790937762)) ;
#63657=CARTESIAN_POINT('Ctrl Pts',(-20.5430611920399,-45.9988496865232,
123.000680697245)) ;
#63658=CARTESIAN_POINT('Ctrl Pts',(-20.7150751051334,-46.1888854357668,
122.658590446776)) ;
#63659=CARTESIAN_POINT('Ctrl Pts',(-20.4539067994353,-46.0088963554039,
122.809226303556)) ;
#63660=CARTESIAN_POINT('Ctrl Pts',(-20.5662066575866,-46.1987809990726,
122.445321690522)) ;
#63661=CARTESIAN_POINT('Ctrl Pts',(-20.3348107319398,-46.0187919187097,
122.638612781793)) ;
#63662=CARTESIAN_POINT('Ctrl Pts',(-20.379536426161,-46.2088430567729,122.258099155572)) ;
#63663=CARTESIAN_POINT('Ctrl Pts',(-20.1854730795545,-46.02885397641,122.488836010064)) ;
#63664=CARTESIAN_POINT('Ctrl Pts',(-20.1679385535702,-46.2186858344004,
122.109285146216)) ;
#63665=CARTESIAN_POINT('Ctrl Pts',(-20.0161942548949,-46.0386967540375,
122.369786757822)) ;
#63666=CARTESIAN_POINT('Ctrl Pts',(-19.9305238988353,-46.2286763126523,
121.997288664891)) ;
#63667=CARTESIAN_POINT('Ctrl Pts',(-19.8262618842319,-46.0486872322894,
122.280191270744)) ;
#63668=CARTESIAN_POINT('Ctrl Pts',(-19.6787697821799,-46.2386052852958,
121.928664786175)) ;
#63669=CARTESIAN_POINT('Ctrl Pts',(-19.6248584943409,-46.0586162049329,
122.225294020736)) ;
#63670=CARTESIAN_POINT('Ctrl Pts',(-19.4173499655239,-46.2485964221754,
121.904240994676)) ;
#63671=CARTESIAN_POINT('Ctrl Pts',(-19.4157226100633,-46.0686073418125,
122.205756739917)) ;
#63672=CARTESIAN_POINT('Ctrl Pts',(-19.1548721753511,-46.2586185396643,
121.92596250925)) ;
#63673=CARTESIAN_POINT('Ctrl Pts',(-19.2057405118503,-46.0786294593014,
122.22313574868)) ;
#63674=CARTESIAN_POINT('Ctrl Pts',(-18.9031822162054,-46.2685190500665,
121.991878228814)) ;
#63675=CARTESIAN_POINT('Ctrl Pts',(-19.0043894985658,-46.0885299697036,
122.275869893625)) ;
#63676=CARTESIAN_POINT('Ctrl Pts',(-18.6644805817943,-46.2785080428126,
122.101090338779)) ;
#63677=CARTESIAN_POINT('Ctrl Pts',(-18.8134290284549,-46.0985189624497,
122.363241059296)) ;
#63678=CARTESIAN_POINT('Ctrl Pts',(-18.4489924497402,-46.2884732868632,
122.249880282488)) ;
#63679=CARTESIAN_POINT('Ctrl Pts',(-18.6410397168517,-46.1084842065003,
122.482274286718)) ;
#63680=CARTESIAN_POINT('Ctrl Pts',(-18.2633002251361,-46.2983775513764,
122.43228474134)) ;
#63681=CARTESIAN_POINT('Ctrl Pts',(-18.4924874591841,-46.1183884710135,
122.628198618205)) ;
#63682=CARTESIAN_POINT('Ctrl Pts',(-18.1099129937586,-46.3084356430746,
122.64751373004)) ;
#63683=CARTESIAN_POINT('Ctrl Pts',(-18.3697789069092,-46.1284465627118,
122.800382913545)) ;
#63684=CARTESIAN_POINT('Ctrl Pts',(-17.9983877780156,-46.318285583503,122.881119052211)) ;
#63685=CARTESIAN_POINT('Ctrl Pts',(-18.2805605437885,-46.1382965031402,
122.98726711269)) ;
#63686=CARTESIAN_POINT('Ctrl Pts',(-17.9272509867176,-46.3283125946766,
123.13482951254)) ;
#63687=CARTESIAN_POINT('Ctrl Pts',(-18.2236525328705,-46.1483235143137,
123.190235911234)) ;
#63688=CARTESIAN_POINT('Ctrl Pts',(-17.901925769436,-46.3383411812886,123.397163125626)) ;
#63689=CARTESIAN_POINT('Ctrl Pts',(-18.2033939634236,-46.1583521009257,
123.400103012758)) ;
#63690=CARTESIAN_POINT('Ctrl Pts',(-17.9216676872438,-46.3481863954013,
123.655117412453)) ;
#63691=CARTESIAN_POINT('Ctrl Pts',(-18.2191889474225,-46.1681973150384,
123.606465432505)) ;
#63692=CARTESIAN_POINT('Ctrl Pts',(-17.9861726596863,-46.3581771435809,
123.909622518266)) ;
#63693=CARTESIAN_POINT('Ctrl Pts',(-18.2707942272682,-46.178188063218,123.810069025763)) ;
#63694=CARTESIAN_POINT('Ctrl Pts',(-18.0949209308514,-46.3682147771664,
124.149940691054)) ;
#63695=CARTESIAN_POINT('Ctrl Pts',(-18.3577942543388,-46.1882256968035,
124.002323042482)) ;
#63696=CARTESIAN_POINT('Ctrl Pts',(-18.2405394895734,-46.3780600663792,
124.363798772761)) ;
#63697=CARTESIAN_POINT('Ctrl Pts',(-18.4742897414031,-46.1980709860163,
124.173407939844)) ;
#63698=CARTESIAN_POINT('Ctrl Pts',(-18.4231399414147,-46.3880414671851,
124.552075901713)) ;
#63699=CARTESIAN_POINT('Ctrl Pts',(-18.6203708816344,-46.2080523868222,
124.324028590119)) ;
#63700=CARTESIAN_POINT('Ctrl Pts',(-18.6350962163679,-46.397993700175,124.705303329863)) ;
#63701=CARTESIAN_POINT('Ctrl Pts',(-18.7899363575204,-46.2180046198121,
124.446609255118)) ;
#63702=CARTESIAN_POINT('Ctrl Pts',(-18.8714017008727,-46.4079925116317,
124.820247929086)) ;
#63703=CARTESIAN_POINT('Ctrl Pts',(-18.9789811859863,-46.2280034312688,
124.538563781757)) ;
#63704=CARTESIAN_POINT('Ctrl Pts',(-19.1251985398827,-46.4180316155623,
124.892209201477)) ;
#63705=CARTESIAN_POINT('Ctrl Pts',(-19.1820191456136,-46.2380425351995,
124.596131542575)) ;
#63706=CARTESIAN_POINT('Ctrl Pts',(-19.3820108279109,-46.4278565579816,
124.918993385592)) ;
#63707=CARTESIAN_POINT('Ctrl Pts',(-19.387468008186,-46.2478674776188,124.61755756467)) ;
#63708=CARTESIAN_POINT('Ctrl Pts',(-19.64559328927,-46.4379112454576,124.900789356719)) ;
#63709=CARTESIAN_POINT('Ctrl Pts',(-19.5983341049394,-46.2579221650947,
124.602993203772)) ;
#63710=CARTESIAN_POINT('Ctrl Pts',(-19.8990733415374,-46.4478540478144,
124.837364781521)) ;
#63711=CARTESIAN_POINT('Ctrl Pts',(-19.8011174177466,-46.2678649674515,
124.552252461191)) ;
#63712=CARTESIAN_POINT('Ctrl Pts',(-20.1370762828401,-46.4577578437542,
124.732039090923)) ;
#63713=CARTESIAN_POINT('Ctrl Pts',(-19.9915187270784,-46.2777687633913,
124.467991228943)) ;
#63714=CARTESIAN_POINT('Ctrl Pts',(-20.3561848751386,-46.4678046231292,
124.584777991393)) ;
#63715=CARTESIAN_POINT('Ctrl Pts',(-20.1668051376118,-46.2878155427663,
124.350181357414)) ;
#63716=CARTESIAN_POINT('Ctrl Pts',(-20.5437352889847,-46.4777002814238,
124.40458454613)) ;
#63717=CARTESIAN_POINT('Ctrl Pts',(-20.3168442299365,-46.2977112010609,
124.206026364736)) ;
#63718=CARTESIAN_POINT('Ctrl Pts',(-20.6997061794261,-46.4877618486744,
124.191114977027)) ;
#63719=CARTESIAN_POINT('Ctrl Pts',(-20.4416202696434,-46.3077727683115,
124.035249895047)) ;
#63720=CARTESIAN_POINT('Ctrl Pts',(-20.8137834732747,-46.4976064931117,
123.958907813317)) ;
#63721=CARTESIAN_POINT('Ctrl Pts',(-20.5328807279198,-46.3176174127489,
123.849484665839)) ;
#63722=CARTESIAN_POINT('Ctrl Pts',(-20.8875519244176,-46.5075665393544,
123.707782162122)) ;
#63723=CARTESIAN_POINT('Ctrl Pts',(-20.5918946247474,-46.3275774589915,
123.648584272298)) ;
#63724=CARTESIAN_POINT('Ctrl Pts',(-20.9163089327259,-46.5176048353728,
123.445571143073)) ;
#63725=CARTESIAN_POINT('Ctrl Pts',(-20.6148993352014,-46.3376157550099,
123.438815228034)) ;
#63726=CARTESIAN_POINT('Ctrl Pts',(-20.8998770457403,-46.5274781767911,
123.186591367245)) ;
#63727=CARTESIAN_POINT('Ctrl Pts',(-20.6017530884054,-46.3474890964282,
123.231632356186)) ;
#63728=CARTESIAN_POINT('Ctrl Pts',(-20.8374336990215,-46.5375512805904,
122.92940409922)) ;
#63729=CARTESIAN_POINT('Ctrl Pts',(-20.5517975371544,-46.3575622002275,
123.025882403029)) ;
#63730=CARTESIAN_POINT('Ctrl Pts',(-20.7341962066025,-46.5473720957093,
122.692815045796)) ;
#63731=CARTESIAN_POINT('Ctrl Pts',(-20.4692073631793,-46.3673830153464,
122.836612591769)) ;
#63732=CARTESIAN_POINT('Ctrl Pts',(-20.5880342149854,-46.5574489607873,
122.472055591262)) ;
#63733=CARTESIAN_POINT('Ctrl Pts',(-20.3522770187593,-46.3774598804244,
122.660005096316)) ;
#63734=CARTESIAN_POINT('Ctrl Pts',(-20.4094709146945,-46.5673137004426,
122.28408059887)) ;
#63735=CARTESIAN_POINT('Ctrl Pts',(-20.2094265518685,-46.3873246200797,
122.509626284042)) ;
#63736=CARTESIAN_POINT('Ctrl Pts',(-20.1980943113753,-46.5773361036839,
122.126973882739)) ;
#63737=CARTESIAN_POINT('Ctrl Pts',(-20.0403249282567,-46.397347023321,122.383941308971)) ;
#63738=CARTESIAN_POINT('Ctrl Pts',(-19.962253273062,-46.5873618279724,122.009494285123)) ;
#63739=CARTESIAN_POINT('Ctrl Pts',(-19.8516517311113,-46.4073727476095,
122.289958211651)) ;
#63740=CARTESIAN_POINT('Ctrl Pts',(-19.7140632034375,-46.5972166109937,
121.935594664619)) ;
#63741=CARTESIAN_POINT('Ctrl Pts',(-19.6531005311567,-46.4172275306308,
122.230839367749)) ;
#63742=CARTESIAN_POINT('Ctrl Pts',(-19.453631099447,-46.607195454717,121.904856532763)) ;
#63743=CARTESIAN_POINT('Ctrl Pts',(-19.4447550642986,-46.4272063743541,
122.206249292798)) ;
#63744=CARTESIAN_POINT('Ctrl Pts',(-19.1908123744642,-46.6172143469536,
121.920317600805)) ;
#63745=CARTESIAN_POINT('Ctrl Pts',(-19.2345001020312,-46.4372252665907,
122.218618661177)) ;
#63746=CARTESIAN_POINT('Ctrl Pts',(-18.9379696064049,-46.6270975559946,
121.979840758629)) ;
#63747=CARTESIAN_POINT('Ctrl Pts',(-19.0322268301204,-46.4471084756317,
122.266237355114)) ;
#63748=CARTESIAN_POINT('Ctrl Pts',(-18.6949496716682,-46.6371658653348,
122.084353104064)) ;
#63749=CARTESIAN_POINT('Ctrl Pts',(-18.8378107414872,-46.4571767849719,
122.349847736102)) ;
#63750=CARTESIAN_POINT('Ctrl Pts',(-18.4787605240765,-46.6469959906675,
122.225836194928)) ;
#63751=CARTESIAN_POINT('Ctrl Pts',(-18.6648606358559,-46.4670069103046,
122.463033810365)) ;
#63752=CARTESIAN_POINT('Ctrl Pts',(-18.2857214966169,-46.6570625430445,
122.406651152196)) ;
#63753=CARTESIAN_POINT('Ctrl Pts',(-18.5104293493474,-46.4770734626816,
122.607686172701)) ;
#63754=CARTESIAN_POINT('Ctrl Pts',(-18.1298739186722,-46.6669527799382,
122.614687511568)) ;
#63755=CARTESIAN_POINT('Ctrl Pts',(-18.3857520197668,-46.4869636995753,
122.774114761019)) ;
#63756=CARTESIAN_POINT('Ctrl Pts',(-18.0108157653476,-46.6769450047322,
122.848713195629)) ;
#63757=CARTESIAN_POINT('Ctrl Pts',(-18.2905057011773,-46.4969559243693,
122.96133522007)) ;
#63758=CARTESIAN_POINT('Ctrl Pts',(-17.9346569102099,-46.6869076250832,
123.099193972045)) ;
#63759=CARTESIAN_POINT('Ctrl Pts',(-18.2295789196735,-46.5069185447203,
123.161719551088)) ;
#63760=CARTESIAN_POINT('Ctrl Pts',(-17.9026865142012,-46.6968126278463,
123.35753421386)) ;
#63761=CARTESIAN_POINT('Ctrl Pts',(-18.2040027337092,-46.5168235474834,
123.368391006395)) ;
#63762=CARTESIAN_POINT('Ctrl Pts',(-17.9164439568202,-46.7068703902444,
123.621460054285)) ;
#63763=CARTESIAN_POINT('Ctrl Pts',(-18.2150087894346,-46.5268813098816,
123.579531944023)) ;
#63764=CARTESIAN_POINT('Ctrl Pts',(-17.9743972615009,-46.7167209096232,
123.873771940566)) ;
#63765=CARTESIAN_POINT('Ctrl Pts',(-18.2613712111539,-46.5367318292604,
123.781380349578)) ;
#63766=CARTESIAN_POINT('Ctrl Pts',(-18.076585890768,-46.7267524866214,124.116760874155)) ;
#63767=CARTESIAN_POINT('Ctrl Pts',(-18.343122043701,-46.5467634062585,123.97577162832)) ;
#63768=CARTESIAN_POINT('Ctrl Pts',(-18.2195527491891,-46.7367622217263,
124.337596888945)) ;
#63769=CARTESIAN_POINT('Ctrl Pts',(-18.4574955266173,-46.5567731413635,
124.15244040257)) ;
#63770=CARTESIAN_POINT('Ctrl Pts',(-18.3966970018907,-46.7466717983526,
124.528446109055)) ;
#63771=CARTESIAN_POINT('Ctrl Pts',(-18.5992104071735,-46.5666827179897,
124.30511928162)) ;
#63772=CARTESIAN_POINT('Ctrl Pts',(-18.6042842738298,-46.7565991842093,
124.686473857333)) ;
#63773=CARTESIAN_POINT('Ctrl Pts',(-18.7652796215495,-46.5766101038464,
124.431541287681)) ;
#63774=CARTESIAN_POINT('Ctrl Pts',(-18.8389799600762,-46.7666441186995,
124.807271873775)) ;
#63775=CARTESIAN_POINT('Ctrl Pts',(-18.9530362508393,-46.5866550383367,
124.528179918756)) ;
#63776=CARTESIAN_POINT('Ctrl Pts',(-19.0870750670697,-46.7765300508875,
124.884401576548)) ;
#63777=CARTESIAN_POINT('Ctrl Pts',(-19.1515114465665,-46.5965409705246,
124.589883612155)) ;
#63778=CARTESIAN_POINT('Ctrl Pts',(-19.3475046537344,-46.7865233568405,
124.918084459445)) ;
#63779=CARTESIAN_POINT('Ctrl Pts',(-19.3598549143501,-46.6065342764777,
124.616830206673)) ;
#63780=CARTESIAN_POINT('Ctrl Pts',(-19.6085865453895,-46.7964689946224,
124.905990634094)) ;
#63781=CARTESIAN_POINT('Ctrl Pts',(-19.5687199653506,-46.6164799142595,
124.607155453148)) ;
#63782=CARTESIAN_POINT('Ctrl Pts',(-19.8637733413823,-46.8064162629683,
124.84925888775)) ;
#63783=CARTESIAN_POINT('Ctrl Pts',(-19.7728690447604,-46.6264271826054,
124.561770566073)) ;
#63784=CARTESIAN_POINT('Ctrl Pts',(-20.1075420667063,-46.8164641651054,
124.747800719658)) ;
#63785=CARTESIAN_POINT('Ctrl Pts',(-19.9678843424592,-46.6364750847425,
124.480604273047)) ;
#63786=CARTESIAN_POINT('Ctrl Pts',(-20.3256846821778,-46.8263118599456,
124.608569806517)) ;
#63787=CARTESIAN_POINT('Ctrl Pts',(-20.1423977064483,-46.6463227795827,
124.369220481856)) ;
#63788=CARTESIAN_POINT('Ctrl Pts',(-20.5190914280319,-46.83627336969,124.432171593144)) ;
#63789=CARTESIAN_POINT('Ctrl Pts',(-20.297123242795,-46.6562842893271,124.2281026054)) ;
#63790=CARTESIAN_POINT('Ctrl Pts',(-20.6797539090321,-46.8463027612989,
124.223227378211)) ;
#63791=CARTESIAN_POINT('Ctrl Pts',(-20.42565368723,-46.666313680936,124.060947484944)) ;
#63792=CARTESIAN_POINT('Ctrl Pts',(-20.8003366055072,-46.8562102568536,
123.992472885729)) ;
#63793=CARTESIAN_POINT('Ctrl Pts',(-20.5221200032968,-46.6762211764908,
123.876344781865)) ;
#63794=CARTESIAN_POINT('Ctrl Pts',(-20.8798121649612,-46.8661556485166,
123.743517315993)) ;
#63795=CARTESIAN_POINT('Ctrl Pts',(-20.5857009581305,-46.6861665681538,
123.6771809766)) ;
#63796=CARTESIAN_POINT('Ctrl Pts',(-20.915214625767,-46.876157566114,123.48303667498)) ;
#63797=CARTESIAN_POINT('Ctrl Pts',(-20.614023626857,-46.6961684857511,123.468796661138)) ;
#63798=CARTESIAN_POINT('Ctrl Pts',(-20.9043274469187,-46.8861976336662,
123.219443241607)) ;
#63799=CARTESIAN_POINT('Ctrl Pts',(-20.605314478917,-46.7062085533033,123.257921751627)) ;
#63800=CARTESIAN_POINT('Ctrl Pts',(-20.8496146260734,-46.896021945106,122.967111685229)) ;
#63801=CARTESIAN_POINT('Ctrl Pts',(-20.5615452065626,-46.7160328647431,
123.056057541106)) ;
#63802=CARTESIAN_POINT('Ctrl Pts',(-20.7499690603553,-46.9060781862621,
122.722378928017)) ;
#63803=CARTESIAN_POINT('Ctrl Pts',(-20.481829431188,-46.7260891058992,122.860270789842)) ;
#63804=CARTESIAN_POINT('Ctrl Pts',(-20.6108065948018,-46.9160091079977,
122.501569334543)) ;
#63805=CARTESIAN_POINT('Ctrl Pts',(-20.3705003850126,-46.7360200276349,
122.683623170689)) ;
#63806=CARTESIAN_POINT('Ctrl Pts',(-20.4356383205666,-46.925952344074,122.307725777461)) ;
#63807=CARTESIAN_POINT('Ctrl Pts',(-20.2303667445202,-46.7459632637111,
122.528548091162)) ;
#63808=CARTESIAN_POINT('Ctrl Pts',(-20.2287819479061,-46.9359336280864,
122.146383450111)) ;
#63809=CARTESIAN_POINT('Ctrl Pts',(-20.0648823935122,-46.7559445477236,
122.399473615786)) ;
#63810=CARTESIAN_POINT('Ctrl Pts',(-19.9954418662365,-46.9459779297121,
122.023069093696)) ;
#63811=CARTESIAN_POINT('Ctrl Pts',(-19.8782105832335,-46.7659888493492,
122.300821320702)) ;
#63812=CARTESIAN_POINT('Ctrl Pts',(-19.7497569427276,-46.9558060109315,
121.943291660823)) ;
#63813=CARTESIAN_POINT('Ctrl Pts',(-19.6816640439892,-46.7758169305687,
122.236998801319)) ;
#63814=CARTESIAN_POINT('Ctrl Pts',(-19.4875976586509,-46.9658826137807,
121.90636263565)) ;
#63815=CARTESIAN_POINT('Ctrl Pts',(-19.4719364151813,-46.7858935334178,
122.207454534728)) ;
#63816=CARTESIAN_POINT('Ctrl Pts',(-19.228788648694,-46.9757346928992,121.915184765414)) ;
#63817=CARTESIAN_POINT('Ctrl Pts',(-19.2648901580032,-46.7957456125364,
122.214511170181)) ;
#63818=CARTESIAN_POINT('Ctrl Pts',(-18.9698079849325,-46.9858079512082,
121.969772870616)) ;
#63819=CARTESIAN_POINT('Ctrl Pts',(-19.0577050887598,-46.8058188708453,
122.258180656131)) ;
#63820=CARTESIAN_POINT('Ctrl Pts',(-18.7298606158885,-46.9956494105884,
122.066316849577)) ;
#63821=CARTESIAN_POINT('Ctrl Pts',(-18.8657477611846,-46.8156603302256,
122.335414457744)) ;
#63822=CARTESIAN_POINT('Ctrl Pts',(-18.507158497528,-47.0056105060008,122.203869923558)) ;
#63823=CARTESIAN_POINT('Ctrl Pts',(-18.6875856641331,-46.8256214256379,
122.445455650075)) ;
#63824=CARTESIAN_POINT('Ctrl Pts',(-18.3105700406655,-47.0156477903975,
122.379722097263)) ;
#63825=CARTESIAN_POINT('Ctrl Pts',(-18.5303140387269,-46.8356587100347,
122.586136582411)) ;
#63826=CARTESIAN_POINT('Ctrl Pts',(-18.1497383800558,-47.0255241291328,
122.583459652795)) ;
#63827=CARTESIAN_POINT('Ctrl Pts',(-18.4016482050606,-46.8455350487699,
122.749125213228)) ;
#63828=CARTESIAN_POINT('Ctrl Pts',(-18.0243973839348,-47.0355862552861,
122.816248967698)) ;
#63829=CARTESIAN_POINT('Ctrl Pts',(-18.3013741678358,-46.8555971749232,
122.935356256442)) ;
#63830=CARTESIAN_POINT('Ctrl Pts',(-17.942900261197,-47.0454544292626,123.062469015826)) ;
#63831=CARTESIAN_POINT('Ctrl Pts',(-18.2361754986026,-46.8654653488997,
123.132331099916)) ;
#63832=CARTESIAN_POINT('Ctrl Pts',(-17.9043551712799,-47.0554599777664,
123.322528432364)) ;
#63833=CARTESIAN_POINT('Ctrl Pts',(-18.2053380449325,-46.8754708974035,
123.340378359643)) ;
#63834=CARTESIAN_POINT('Ctrl Pts',(-17.911626244223,-47.065442609662,123.58480879542)) ;
#63835=CARTESIAN_POINT('Ctrl Pts',(-18.2111535111412,-46.8854535292991,
123.55020250964)) ;
#63836=CARTESIAN_POINT('Ctrl Pts',(-17.964905818864,-47.0754865520838,123.843296984547)) ;
#63837=CARTESIAN_POINT('Ctrl Pts',(-18.2537758946358,-46.8954974717209,
123.756993455038)) ;
#63838=CARTESIAN_POINT('Ctrl Pts',(-18.0598529385593,-47.0853147001109,
124.083485382796)) ;
#63839=CARTESIAN_POINT('Ctrl Pts',(-18.3297319083217,-46.9053256197481,
123.949143731469)) ;
#63840=CARTESIAN_POINT('Ctrl Pts',(-18.1965689479448,-47.0953045674853,
124.307600675723)) ;
#63841=CARTESIAN_POINT('Ctrl Pts',(-18.4391033021549,-46.9153154871225,
124.128436666438)) ;
#63842=CARTESIAN_POINT('Ctrl Pts',(-18.3715713484641,-47.1053483064408,
124.505180389695)) ;
#63843=CARTESIAN_POINT('Ctrl Pts',(-18.5791042261939,-46.925359226078,124.286501476418)) ;
#63844=CARTESIAN_POINT('Ctrl Pts',(-18.5733188648744,-47.1151700549788,
124.666164420579)) ;
#63845=CARTESIAN_POINT('Ctrl Pts',(-18.7405004989235,-46.9351809746159,
124.41528928464)) ;
#63846=CARTESIAN_POINT('Ctrl Pts',(-18.8045645528301,-47.1252050325885,
124.792922450378)) ;
#63847=CARTESIAN_POINT('Ctrl Pts',(-18.9254963238758,-46.9452159522256,
124.516697207204)) ;
#63848=CARTESIAN_POINT('Ctrl Pts',(-19.0542980945525,-47.1352299453462,
124.876825162639)) ;
#63849=CARTESIAN_POINT('Ctrl Pts',(-19.1252826902165,-46.9552408649833,
124.583820828544)) ;
#63850=CARTESIAN_POINT('Ctrl Pts',(-19.3102255315884,-47.14508188844,124.915973693937)) ;
#63851=CARTESIAN_POINT('Ctrl Pts',(-19.3300235960743,-46.9650928080772,
124.615141143761)) ;
#63852=CARTESIAN_POINT('Ctrl Pts',(-19.5726863790115,-47.1550728497691,
124.910409512825)) ;
#63853=CARTESIAN_POINT('Ctrl Pts',(-19.5399921733102,-46.9750837694063,
124.61069150596)) ;
#63854=CARTESIAN_POINT('Ctrl Pts',(-19.8284072327233,-47.1649907246376,
124.859887472714)) ;
#63855=CARTESIAN_POINT('Ctrl Pts',(-19.7445687433349,-46.9850016442747,
124.570275659941)) ;
#63856=CARTESIAN_POINT('Ctrl Pts',(-20.074151105226,-47.1750192436388,124.764752235649)) ;
#63857=CARTESIAN_POINT('Ctrl Pts',(-19.9411644966269,-46.9950301632759,
124.494169084387)) ;
#63858=CARTESIAN_POINT('Ctrl Pts',(-20.2964844789698,-47.1849029224366,
124.630459757665)) ;
#63859=CARTESIAN_POINT('Ctrl Pts',(-20.1190316002392,-47.0049138420738,
124.386736915918)) ;
#63860=CARTESIAN_POINT('Ctrl Pts',(-20.4946972413566,-47.1948978658764,
124.458122754185)) ;
#63861=CARTESIAN_POINT('Ctrl Pts',(-20.2776029447661,-47.0149087855135,
124.248868788224)) ;
#63862=CARTESIAN_POINT('Ctrl Pts',(-20.6601527760735,-47.2049247196988,
124.253049913782)) ;
#63863=CARTESIAN_POINT('Ctrl Pts',(-20.4099687724888,-47.0249356393359,
124.084811622413)) ;
#63864=CARTESIAN_POINT('Ctrl Pts',(-20.7859931800233,-47.2148088840377,
124.025810555363)) ;
#63865=CARTESIAN_POINT('Ctrl Pts',(-20.5106424360365,-47.0348198036749,
123.90302151066)) ;
#63866=CARTESIAN_POINT('Ctrl Pts',(-20.8716717234267,-47.2247969820801,
123.777738571855)) ;
#63867=CARTESIAN_POINT('Ctrl Pts',(-20.5791870192374,-47.0448079017172,
123.704564663885)) ;
#63868=CARTESIAN_POINT('Ctrl Pts',(-20.912975435298,-47.2347480885372,123.519483140428)) ;
#63869=CARTESIAN_POINT('Ctrl Pts',(-20.6122318336066,-47.0547590081743,
123.497960883868)) ;
#63870=CARTESIAN_POINT('Ctrl Pts',(-20.908624300372,-47.2447931397053,123.255561025828)) ;
#63871=CARTESIAN_POINT('Ctrl Pts',(-20.6087528155346,-47.0648040593424,
123.286823089854)) ;
#63872=CARTESIAN_POINT('Ctrl Pts',(-20.8595658745191,-47.2546549000636,
123.001088343712)) ;
#63873=CARTESIAN_POINT('Ctrl Pts',(-20.5695080656259,-47.0746658197007,
123.083245164195)) ;
#63874=CARTESIAN_POINT('Ctrl Pts',(-20.7668750532524,-47.264617716894,122.756231591829)) ;
#63875=CARTESIAN_POINT('Ctrl Pts',(-20.4953573697405,-47.0846286365312,
122.887359233057)) ;
#63876=CARTESIAN_POINT('Ctrl Pts',(-20.6317297453688,-47.2746523981748,
122.529807845383)) ;
#63877=CARTESIAN_POINT('Ctrl Pts',(-20.3872427942103,-47.0946633178119,
122.706219207797)) ;
#63878=CARTESIAN_POINT('Ctrl Pts',(-20.4621990513068,-47.2845374279556,
122.332938364002)) ;
#63879=CARTESIAN_POINT('Ctrl Pts',(-20.2516200615866,-47.1045483475927,
122.548722648107)) ;
#63880=CARTESIAN_POINT('Ctrl Pts',(-20.2574099722437,-47.2946030213536,
122.16558837992)) ;
#63881=CARTESIAN_POINT('Ctrl Pts',(-20.0877899799016,-47.1146139409907,
122.414841027643)) ;
#63882=CARTESIAN_POINT('Ctrl Pts',(-20.0319196599626,-47.3044421897151,
122.038978242884)) ;
#63883=CARTESIAN_POINT('Ctrl Pts',(-19.9073992209969,-47.1244531093522,
122.313551415424)) ;
#63884=CARTESIAN_POINT('Ctrl Pts',(-19.7825183008089,-47.3145047874566,
121.95118250225)) ;
#63885=CARTESIAN_POINT('Ctrl Pts',(-19.7078787262288,-47.1345157070937,
122.243312822989)) ;
#63886=CARTESIAN_POINT('Ctrl Pts',(-19.5258624977633,-47.3244017998635,
121.909002521009)) ;
#63887=CARTESIAN_POINT('Ctrl Pts',(-19.502554784226,-47.1444127195006,122.209566874311)) ;
#63888=CARTESIAN_POINT('Ctrl Pts',(-19.2648924723534,-47.3343331216891,
121.911168475374)) ;
#63889=CARTESIAN_POINT('Ctrl Pts',(-19.2937789864561,-47.1543440413262,
122.211297494334)) ;
#63890=CARTESIAN_POINT('Ctrl Pts',(-19.0054588236434,-47.3443748844436,
121.959423773206)) ;
#63891=CARTESIAN_POINT('Ctrl Pts',(-19.0862316578282,-47.1643858040807,
122.249899661236)) ;
#63892=CARTESIAN_POINT('Ctrl Pts',(-18.7620408415515,-47.3542630833343,
122.050409572673)) ;
#63893=CARTESIAN_POINT('Ctrl Pts',(-18.8914968446578,-47.1742740029714,
122.322686186617)) ;
#63894=CARTESIAN_POINT('Ctrl Pts',(-18.5355442147587,-47.3642570219342,
122.18331150089)) ;
#63895=CARTESIAN_POINT('Ctrl Pts',(-18.7102985172249,-47.1842679415713,
122.429005819235)) ;
#63896=CARTESIAN_POINT('Ctrl Pts',(-18.3366094811848,-47.374197842971,122.352654796007)) ;
#63897=CARTESIAN_POINT('Ctrl Pts',(-18.551149473623,-47.1942087626082,122.564478686452)) ;
#63898=CARTESIAN_POINT('Ctrl Pts',(-18.1695526330089,-47.3841572252593,
122.554106932035)) ;
#63899=CARTESIAN_POINT('Ctrl Pts',(-18.417502400572,-47.2041681448964,122.725638889882)) ;
#63900=CARTESIAN_POINT('Ctrl Pts',(-18.0393553532008,-47.3941549849116,
122.782338451518)) ;
#63901=CARTESIAN_POINT('Ctrl Pts',(-18.3133427031119,-47.2141659045487,
122.908222957332)) ;
#63902=CARTESIAN_POINT('Ctrl Pts',(-17.9507774145601,-47.4041911211139,
123.03075086766)) ;
#63903=CARTESIAN_POINT('Ctrl Pts',(-18.2424783105885,-47.224202040751,123.106952144432)) ;
#63904=CARTESIAN_POINT('Ctrl Pts',(-17.9071905133116,-47.4140419186048,
123.285921661673)) ;
#63905=CARTESIAN_POINT('Ctrl Pts',(-18.2076066786079,-47.2340528382419,
123.311088103092)) ;
#63906=CARTESIAN_POINT('Ctrl Pts',(-17.9078079177087,-47.4240027836811,
123.547672833049)) ;
#63907=CARTESIAN_POINT('Ctrl Pts',(-18.2080983638521,-47.2440137033182,
123.520488944659)) ;
#63908=CARTESIAN_POINT('Ctrl Pts',(-17.9544972057267,-47.4340316513115,
123.807067402969)) ;
#63909=CARTESIAN_POINT('Ctrl Pts',(-18.2454476048845,-47.2540425709486,
123.728004959381)) ;
#63910=CARTESIAN_POINT('Ctrl Pts',(-18.0443558522348,-47.4439418874479,
124.051493099895)) ;
#63911=CARTESIAN_POINT('Ctrl Pts',(-18.3173323750563,-47.263952807085,123.923546127263)) ;
#63912=CARTESIAN_POINT('Ctrl Pts',(-18.1750338402729,-47.4538768407624,
124.27752403088)) ;
#63913=CARTESIAN_POINT('Ctrl Pts',(-18.4218727658216,-47.2738877603996,
124.10437190683)) ;
#63914=CARTESIAN_POINT('Ctrl Pts',(-18.3449402389459,-47.463917771172,124.479398422713)) ;
#63915=CARTESIAN_POINT('Ctrl Pts',(-18.5577961461573,-47.2839286908091,
124.265872834734)) ;
#63916=CARTESIAN_POINT('Ctrl Pts',(-18.5441394208993,-47.4738056679536,
124.646262687843)) ;
#63917=CARTESIAN_POINT('Ctrl Pts',(-18.717153951654,-47.2938165875907,124.399365886383)) ;
#63918=CARTESIAN_POINT('Ctrl Pts',(-18.7713398491585,-47.4837951196123,
124.777752129253)) ;
#63919=CARTESIAN_POINT('Ctrl Pts',(-18.8989131176986,-47.3038060392494,
124.504559363541)) ;
#63920=CARTESIAN_POINT('Ctrl Pts',(-19.0172406224052,-47.4937542099777,
124.867323859579)) ;
#63921=CARTESIAN_POINT('Ctrl Pts',(-19.0956328934438,-47.3137651296148,
124.576218838424)) ;
#63922=CARTESIAN_POINT('Ctrl Pts',(-19.2732681589925,-47.503651522284,124.913214982479)) ;
#63923=CARTESIAN_POINT('Ctrl Pts',(-19.3004544847699,-47.3236624419211,
124.612933948275)) ;
#63924=CARTESIAN_POINT('Ctrl Pts',(-19.5375180334294,-47.5137079481842,
124.913840318976)) ;
#63925=CARTESIAN_POINT('Ctrl Pts',(-19.5118543105369,-47.3337188678213,
124.613436469234)) ;
#63926=CARTESIAN_POINT('Ctrl Pts',(-19.7931038035126,-47.523577950774,124.86953541503)) ;
#63927=CARTESIAN_POINT('Ctrl Pts',(-19.7163232953093,-47.3435888704111,
124.577994777982)) ;
#63928=CARTESIAN_POINT('Ctrl Pts',(-20.0405538778607,-47.5335818839512,
124.780842159389)) ;
#63929=CARTESIAN_POINT('Ctrl Pts',(-19.9142841000956,-47.3535928035883,
124.507042257219)) ;
#63930=CARTESIAN_POINT('Ctrl Pts',(-20.2684557085201,-47.5435691444151,
124.650592871632)) ;
#63931=CARTESIAN_POINT('Ctrl Pts',(-20.096606520165,-47.3635800640522,124.402844965088)) ;
#63932=CARTESIAN_POINT('Ctrl Pts',(-20.470938720581,-47.5535961960008,124.482002870623)) ;
#63933=CARTESIAN_POINT('Ctrl Pts',(-20.2585947483738,-47.3736071156379,
124.267974120626)) ;
#63934=CARTESIAN_POINT('Ctrl Pts',(-20.6389889194383,-47.5634872858269,
124.283677447582)) ;
#63935=CARTESIAN_POINT('Ctrl Pts',(-20.3930350147794,-47.383498205464,124.109317524504)) ;
#63936=CARTESIAN_POINT('Ctrl Pts',(-20.8155222736475,-47.576785040608,123.982153459967)) ;
#63937=CARTESIAN_POINT('Ctrl Pts',(-20.5342723572746,-47.3967959602451,
123.86808831075)) ;
#63938=CARTESIAN_POINT('Ctrl Pts',(-20.9091627271371,-47.5899831002161,
123.644050843664)) ;
#63939=CARTESIAN_POINT('Ctrl Pts',(-20.6091851817961,-47.4099940198532,
123.597577609492)) ;
#63940=CARTESIAN_POINT('Ctrl Pts',(-20.911961468793,-47.6033798407853,123.29203099922)) ;
#63941=CARTESIAN_POINT('Ctrl Pts',(-20.6114219138469,-47.4233907604224,
123.316008249511)) ;
#63942=CARTESIAN_POINT('Ctrl Pts',(-20.8692234169841,-47.6132507528587,
123.036128094905)) ;
#63943=CARTESIAN_POINT('Ctrl Pts',(-20.5772346237464,-47.4332616724959,
123.111276038365)) ;
#63944=CARTESIAN_POINT('Ctrl Pts',(-20.7809529679,-47.6233243146269,122.78661751852)) ;
#63945=CARTESIAN_POINT('Ctrl Pts',(-20.5066201804174,-47.443335234264,122.911669620032)) ;
#63946=CARTESIAN_POINT('Ctrl Pts',(-20.6541739490141,-47.6331457272152,
122.561735103917)) ;
#63947=CARTESIAN_POINT('Ctrl Pts',(-20.405198506557,-47.4531566468523,122.731761296753)) ;
#63948=CARTESIAN_POINT('Ctrl Pts',(-20.4863320285724,-47.6432197444462,
122.357091382162)) ;
#63949=CARTESIAN_POINT('Ctrl Pts',(-20.2709276233739,-47.4632306640834,
122.568046598626)) ;
#63950=CARTESIAN_POINT('Ctrl Pts',(-20.2240587467137,-47.6563785314108,
122.131615915309)) ;
#63951=CARTESIAN_POINT('Ctrl Pts',(-20.0611061721674,-47.4763894510479,
122.387657331464)) ;
#63952=CARTESIAN_POINT('Ctrl Pts',(-19.904396611808,-47.669744634505,121.976897634996)) ;
#63953=CARTESIAN_POINT('Ctrl Pts',(-19.8053424387584,-47.4897555541421,
122.263873680573)) ;
#63954=CARTESIAN_POINT('Ctrl Pts',(-19.5604802159987,-47.683058569394,121.912018372431)) ;
#63955=CARTESIAN_POINT('Ctrl Pts',(-19.5302562121692,-47.5030694890312,
122.211981762191)) ;
#63956=CARTESIAN_POINT('Ctrl Pts',(-19.3003815270742,-47.6929586088415,
121.908333183184)) ;
#63957=CARTESIAN_POINT('Ctrl Pts',(-19.322167620802,-47.5129695284786,122.209028724385)) ;
#63958=CARTESIAN_POINT('Ctrl Pts',(-19.0418005240808,-47.702923011976,121.949706846036)) ;
#63959=CARTESIAN_POINT('Ctrl Pts',(-19.1153050560258,-47.5229339316132,
122.242126300754)) ;
#63960=CARTESIAN_POINT('Ctrl Pts',(-18.7927924422109,-47.7129529790972,
122.036134213176)) ;
#63961=CARTESIAN_POINT('Ctrl Pts',(-18.9160968262407,-47.5329638987343,
122.311266676217)) ;
#63962=CARTESIAN_POINT('Ctrl Pts',(-18.5654632174081,-47.7228552557062,
122.162745640329)) ;
#63963=CARTESIAN_POINT('Ctrl Pts',(-18.734234498539,-47.5428661753434,122.412551849973)) ;
#63964=CARTESIAN_POINT('Ctrl Pts',(-18.2943866086344,-47.7361211848754,
122.382011147429)) ;
#63965=CARTESIAN_POINT('Ctrl Pts',(-18.5173605390981,-47.5561321045125,
122.587974585937)) ;
#63966=CARTESIAN_POINT('Ctrl Pts',(-18.0346303797176,-47.7527427159818,
122.739250673809)) ;
#63967=CARTESIAN_POINT('Ctrl Pts',(-18.3095657843141,-47.5727536356189,
122.873754271504)) ;
#63968=CARTESIAN_POINT('Ctrl Pts',(-17.8876997701404,-47.7726175446265,
123.246720784385)) ;
#63969=CARTESIAN_POINT('Ctrl Pts',(-18.192010176043,-47.5926284642636,123.27971738618)) ;
#63970=CARTESIAN_POINT('Ctrl Pts',(-17.917000592734,-47.7892907527283,123.68884871812)) ;
#63971=CARTESIAN_POINT('Ctrl Pts',(-18.2154597786599,-47.6093016723655,
123.63347188355)) ;
#63972=CARTESIAN_POINT('Ctrl Pts',(-18.0293936752082,-47.8025418777096,
124.018462677686)) ;
#63973=CARTESIAN_POINT('Ctrl Pts',(-18.305361509496,-47.6225527973467,123.897116801206)) ;
#63974=CARTESIAN_POINT('Ctrl Pts',(-18.1961054880451,-47.8157841965304,
124.323995100748)) ;
#63975=CARTESIAN_POINT('Ctrl Pts',(-18.4387378061925,-47.6357951161676,
124.141559984397)) ;
#63976=CARTESIAN_POINT('Ctrl Pts',(-18.5033373266895,-47.8325174368699,
124.645448284564)) ;
#63977=CARTESIAN_POINT('Ctrl Pts',(-18.6845128198436,-47.652528356507,124.398713602975)) ;
#63978=CARTESIAN_POINT('Ctrl Pts',(-18.9757346113331,-47.8523465850579,
124.879336049279)) ;
#63979=CARTESIAN_POINT('Ctrl Pts',(-19.0624327890952,-47.672357504695,124.585830613588)) ;
#63980=CARTESIAN_POINT('Ctrl Pts',(-19.5017537468954,-47.8722712801585,
124.939516678205)) ;
#63981=CARTESIAN_POINT('Ctrl Pts',(-19.4832476587856,-47.6922821997956,
124.633977069387)) ;
#63982=CARTESIAN_POINT('Ctrl Pts',(-20.016875861944,-47.8921945087419,124.816493222092)) ;
#63983=CARTESIAN_POINT('Ctrl Pts',(-19.8953467115458,-47.7122054283791,
124.535561030838)) ;
#63984=CARTESIAN_POINT('Ctrl Pts',(-20.4591503180632,-47.912121647868,124.525228376918)) ;
#63985=CARTESIAN_POINT('Ctrl Pts',(-20.2491681384619,-47.7321325675052,
124.302550855083)) ;
#63986=CARTESIAN_POINT('Ctrl Pts',(-20.7752836476955,-47.9319981104837,
124.101934449769)) ;
#63987=CARTESIAN_POINT('Ctrl Pts',(-20.5020771966928,-47.7520090301208,
123.963916114928)) ;
#63988=CARTESIAN_POINT('Ctrl Pts',(-20.9290246638759,-47.951975339089,123.593724361099)) ;
#63989=CARTESIAN_POINT('Ctrl Pts',(-20.6250718773028,-47.7719862587261,
123.557348393509)) ;
#63990=CARTESIAN_POINT('Ctrl Pts',(-20.899749641412,-47.9719101970627,123.064652071563)) ;
#63991=CARTESIAN_POINT('Ctrl Pts',(-20.6016537118098,-47.7919211166998,
123.134089837888)) ;
#63992=CARTESIAN_POINT('Ctrl Pts',(-20.6926191392148,-47.9918066459935,
122.578134849579)) ;
#63993=CARTESIAN_POINT('Ctrl Pts',(-20.4359502844163,-47.8118175656306,
122.744874452236)) ;
#63994=CARTESIAN_POINT('Ctrl Pts',(-20.3318393279067,-48.0117279300601,
122.190571444876)) ;
#63995=CARTESIAN_POINT('Ctrl Pts',(-20.147326663776,-47.8317388496972,122.434822343269)) ;
#63996=CARTESIAN_POINT('Ctrl Pts',(-19.859543379667,-48.0316845797311,121.949105900427)) ;
#63997=CARTESIAN_POINT('Ctrl Pts',(-19.7694899560227,-47.8516954993682,
122.241648817227)) ;
#63998=CARTESIAN_POINT('Ctrl Pts',(-19.3354077539481,-48.0515618728427,
121.883411775971)) ;
#63999=CARTESIAN_POINT('Ctrl Pts',(-19.3501800444516,-47.8715727924798,
122.189092575261)) ;
#64000=CARTESIAN_POINT('Ctrl Pts',(-18.8196458602332,-48.0714483450711,
121.999233714919)) ;
#64001=CARTESIAN_POINT('Ctrl Pts',(-18.9375691001692,-47.8914592647082,
122.281750583357)) ;
#64002=CARTESIAN_POINT('Ctrl Pts',(-18.3709126385938,-48.0915099109951,
122.287270877205)) ;
#64003=CARTESIAN_POINT('Ctrl Pts',(-18.578583226595,-47.9115208306322,122.512179806311)) ;
#64004=CARTESIAN_POINT('Ctrl Pts',(-18.0514008754144,-48.1113503185359,
122.706744756814)) ;
#64005=CARTESIAN_POINT('Ctrl Pts',(-18.3229724703465,-47.931361238173,122.847760542803)) ;
#64006=CARTESIAN_POINT('Ctrl Pts',(-17.8920053839532,-48.1312016425088,
123.209726070964)) ;
#64007=CARTESIAN_POINT('Ctrl Pts',(-18.1954566722783,-47.9512125621459,
123.250147612826)) ;
#64008=CARTESIAN_POINT('Ctrl Pts',(-17.9148449517258,-48.1512549124602,
123.742150506195)) ;
#64009=CARTESIAN_POINT('Ctrl Pts',(-18.2137292815851,-47.9712658320974,
123.676086505446)) ;
#64010=CARTESIAN_POINT('Ctrl Pts',(-18.1156214422887,-48.1710755698436,
124.229345578872)) ;
#64011=CARTESIAN_POINT('Ctrl Pts',(-18.3743523078456,-47.9910864894807,
124.065843886977)) ;
#64012=CARTESIAN_POINT('Ctrl Pts',(-18.4724496628158,-48.1910469911741,
124.622086302263)) ;
#64013=CARTESIAN_POINT('Ctrl Pts',(-18.659816387674,-48.0110579108112,124.380035522052)) ;
#64014=CARTESIAN_POINT('Ctrl Pts',(-18.9403084788893,-48.2109404835378,
124.86880464151)) ;
#64015=CARTESIAN_POINT('Ctrl Pts',(-19.03410518183,-48.0309514031749,124.577408955661)) ;
#64016=CARTESIAN_POINT('Ctrl Pts',(-19.4674642242549,-48.2309645697788,
124.941135895711)) ;
#64017=CARTESIAN_POINT('Ctrl Pts',(-19.4558298576854,-48.050975489416,124.635271999274)) ;
#64018=CARTESIAN_POINT('Ctrl Pts',(-19.982186864098,-48.2507694488917,124.830704772301)) ;
#64019=CARTESIAN_POINT('Ctrl Pts',(-19.867609211054,-48.0707803685288,124.546924581979)) ;
#64020=CARTESIAN_POINT('Ctrl Pts',(-20.4325013285474,-48.2707284645896,
124.550337764469)) ;
#64021=CARTESIAN_POINT('Ctrl Pts',(-20.227859532346,-48.0907393842267,124.32262844544)) ;
#64022=CARTESIAN_POINT('Ctrl Pts',(-20.7595855617661,-48.2907144882186,
124.131795730191)) ;
#64023=CARTESIAN_POINT('Ctrl Pts',(-20.4895249857821,-48.1107254078558,
123.987793147059)) ;
#64024=CARTESIAN_POINT('Ctrl Pts',(-20.9237469669242,-48.3105229839791,
123.631516939085)) ;
#64025=CARTESIAN_POINT('Ctrl Pts',(-20.6208517088242,-48.1305339036163,
123.587567868658)) ;
#64026=CARTESIAN_POINT('Ctrl Pts',(-20.9078563777569,-48.3305056230847,
123.100761863428)) ;
#64027=CARTESIAN_POINT('Ctrl Pts',(-20.6081359619185,-48.1505165427219,
123.162963825818)) ;
#64028=CARTESIAN_POINT('Ctrl Pts',(-20.7125774921877,-48.3503870708787,
122.609609792286)) ;
#64029=CARTESIAN_POINT('Ctrl Pts',(-20.4519095117402,-48.1703979905159,
122.770042764306)) ;
#64030=CARTESIAN_POINT('Ctrl Pts',(-20.3605699834758,-48.3703435376163,
122.212992650453)) ;
#64031=CARTESIAN_POINT('Ctrl Pts',(-20.1703007092997,-48.1903544572534,
122.452751209908)) ;
#64032=CARTESIAN_POINT('Ctrl Pts',(-19.8961915070511,-48.3902209345718,
121.960894036844)) ;
#64033=CARTESIAN_POINT('Ctrl Pts',(-19.7987956286007,-48.210231854209,122.2510753083)) ;
#64034=CARTESIAN_POINT('Ctrl Pts',(-19.3710944052881,-48.4102028807471,
121.881710834972)) ;
#64035=CARTESIAN_POINT('Ctrl Pts',(-19.3787173826546,-48.2302138003843,
122.1877323754)) ;
#64036=CARTESIAN_POINT('Ctrl Pts',(-18.8517658005324,-48.4301319797839,
121.986485155074)) ;
#64037=CARTESIAN_POINT('Ctrl Pts',(-18.9632548451584,-48.250142899421,122.271556232587)) ;
#64038=CARTESIAN_POINT('Ctrl Pts',(-18.3995108077568,-48.4500606029965,
122.262000851826)) ;
#64039=CARTESIAN_POINT('Ctrl Pts',(-18.6014532429342,-48.2700715226336,
122.491970142446)) ;
#64040=CARTESIAN_POINT('Ctrl Pts',(-18.0691275875861,-48.4698949271029,
122.672852581631)) ;
#64041=CARTESIAN_POINT('Ctrl Pts',(-18.337147399175,-48.28990584674,122.820662663942)) ;
#64042=CARTESIAN_POINT('Ctrl Pts',(-17.9257131670204,-48.4865472144863,
123.091471777967)) ;
#64043=CARTESIAN_POINT('Ctrl Pts',(-18.2224260058625,-48.3065581341234,
123.155533896471)) ;
#64044=CARTESIAN_POINT('Ctrl Pts',(-17.9020712050957,-48.4998077155085,
123.439203218313)) ;
#64045=CARTESIAN_POINT('Ctrl Pts',(-18.2035092593179,-48.3198186351457,
123.433741819018)) ;
#64046=CARTESIAN_POINT('Ctrl Pts',(-17.9295520562288,-48.5098091927098,
123.700586123899)) ;
#64047=CARTESIAN_POINT('Ctrl Pts',(-18.2254971398453,-48.3298201123469,
123.642843255364)) ;
#64048=CARTESIAN_POINT('Ctrl Pts',(-18.002650404669,-48.5198412135693,123.953887639431)) ;
#64049=CARTESIAN_POINT('Ctrl Pts',(-18.2839780158191,-48.3398521332064,
123.845485394046)) ;
#64050=CARTESIAN_POINT('Ctrl Pts',(-18.116381192127,-48.5297047572949,124.186799307421)) ;
#64051=CARTESIAN_POINT('Ctrl Pts',(-18.3749628126578,-48.349715676932,124.031812191722)) ;
#64052=CARTESIAN_POINT('Ctrl Pts',(-18.2698960730485,-48.539673470965,124.399078392856)) ;
#64053=CARTESIAN_POINT('Ctrl Pts',(-18.4977838735188,-48.3596843906021,
124.201640071483)) ;
#64054=CARTESIAN_POINT('Ctrl Pts',(-18.5219675225796,-48.5530192183687,
124.642888173834)) ;
#64055=CARTESIAN_POINT('Ctrl Pts',(-18.6994062245984,-48.3730301380058,
124.396656830868)) ;
#64056=CARTESIAN_POINT('Ctrl Pts',(-18.8271260677206,-48.5661697734414,
124.813370160914)) ;
#64057=CARTESIAN_POINT('Ctrl Pts',(-18.9435542458751,-48.3861806930785,
124.533062412033)) ;
#64058=CARTESIAN_POINT('Ctrl Pts',(-19.1680417733709,-48.5795551539912,
124.899907926004)) ;
#64059=CARTESIAN_POINT('Ctrl Pts',(-19.2163009890961,-48.3995660736284,
124.602291912706)) ;
#64060=CARTESIAN_POINT('Ctrl Pts',(-19.4272046606678,-48.5894430899841,
124.919132760716)) ;
#64061=CARTESIAN_POINT('Ctrl Pts',(-19.4236288223874,-48.4094540096212,
124.617669122976)) ;
#64062=CARTESIAN_POINT('Ctrl Pts',(-19.6884474342547,-48.5994342797967,
124.893240945766)) ;
#64063=CARTESIAN_POINT('Ctrl Pts',(-19.6326235030201,-48.4194451994339,
124.596953556144)) ;
#64064=CARTESIAN_POINT('Ctrl Pts',(-19.9403393905158,-48.609386378335,124.822747843543)) ;
#64065=CARTESIAN_POINT('Ctrl Pts',(-19.834136251256,-48.4293972979721,124.540556882283)) ;
#64066=CARTESIAN_POINT('Ctrl Pts',(-20.1782692262088,-48.6194326347855,
124.708388111913)) ;
#64067=CARTESIAN_POINT('Ctrl Pts',(-20.0244791282803,-48.4394435544226,
124.449067115827)) ;
#64068=CARTESIAN_POINT('Ctrl Pts',(-20.3886560573569,-48.6292820821796,
124.557608789877)) ;
#64069=CARTESIAN_POINT('Ctrl Pts',(-20.1927872963318,-48.4492930018168,
124.328441805435)) ;
#64070=CARTESIAN_POINT('Ctrl Pts',(-20.572326095922,-48.6392447346748,124.371049479693)) ;
#64071=CARTESIAN_POINT('Ctrl Pts',(-20.3397216706453,-48.4592556543119,
124.179192818539)) ;
#64072=CARTESIAN_POINT('Ctrl Pts',(-20.7214277473186,-48.6492678203169,
124.153918077393)) ;
#64073=CARTESIAN_POINT('Ctrl Pts',(-20.4590011009063,-48.469278739954,124.005486461818)) ;
#64074=CARTESIAN_POINT('Ctrl Pts',(-20.8297802315917,-48.6591929360738,
123.916635975645)) ;
#64075=CARTESIAN_POINT('Ctrl Pts',(-20.5456810096503,-48.479203855711,123.815659897724)) ;
#64076=CARTESIAN_POINT('Ctrl Pts',(-20.8960112318138,-48.6692454144736,
123.660930444406)) ;
#64077=CARTESIAN_POINT('Ctrl Pts',(-20.5986636102316,-48.4892563341108,
123.611094951253)) ;
#64078=CARTESIAN_POINT('Ctrl Pts',(-20.9165980681484,-48.6790969131764,
123.402843889694)) ;
#64079=CARTESIAN_POINT('Ctrl Pts',(-20.6151308203117,-48.4991078328135,
123.404625622349)) ;
#64080=CARTESIAN_POINT('Ctrl Pts',(-20.8924457354999,-48.6890686523789,
123.141945824781)) ;
#64081=CARTESIAN_POINT('Ctrl Pts',(-20.5958067228006,-48.509079572016,123.195907470545)) ;
#64082=CARTESIAN_POINT('Ctrl Pts',(-20.8231457686488,-48.6990638601446,
122.888545055584)) ;
#64083=CARTESIAN_POINT('Ctrl Pts',(-20.5403646013204,-48.5190747797817,
122.993187508509)) ;
#64084=CARTESIAN_POINT('Ctrl Pts',(-20.71020152793,-48.7090978616136,122.650301300846)) ;
#64085=CARTESIAN_POINT('Ctrl Pts',(-20.4500071819512,-48.5291087812508,
122.802593499085)) ;
#64086=CARTESIAN_POINT('Ctrl Pts',(-20.5606310889083,-48.718953219706,122.438836911348)) ;
#64087=CARTESIAN_POINT('Ctrl Pts',(-20.3303491093556,-48.5389641393431,
122.633423436185)) ;
#64088=CARTESIAN_POINT('Ctrl Pts',(-20.3742255768515,-48.7289526952993,
122.253690036881)) ;
#64089=CARTESIAN_POINT('Ctrl Pts',(-20.1812231766611,-48.5489636149364,
122.485307572519)) ;
#64090=CARTESIAN_POINT('Ctrl Pts',(-20.1608603226581,-48.7388471437944,
122.104999075767)) ;
#64091=CARTESIAN_POINT('Ctrl Pts',(-20.0105298816174,-48.5588580634315,
122.366356738769)) ;
#64092=CARTESIAN_POINT('Ctrl Pts',(-19.9209501103882,-48.7489102680221,
121.993860313604)) ;
#64093=CARTESIAN_POINT('Ctrl Pts',(-19.8186007515957,-48.5689211876593,
122.277447732973)) ;
#64094=CARTESIAN_POINT('Ctrl Pts',(-19.6710512311322,-48.7587498943507,
121.927273469944)) ;
#64095=CARTESIAN_POINT('Ctrl Pts',(-19.6186814015643,-48.5787608139879,
122.224180469347)) ;
#64096=CARTESIAN_POINT('Ctrl Pts',(-19.4076398792598,-48.7688131293937,
121.904256633562)) ;
#64097=CARTESIAN_POINT('Ctrl Pts',(-19.4079520936183,-48.5888240490308,
122.205769170456)) ;
#64098=CARTESIAN_POINT('Ctrl Pts',(-19.1486188793919,-48.7787071346277,
121.927163232832)) ;
#64099=CARTESIAN_POINT('Ctrl Pts',(-19.2007357506879,-48.5987180542649,
122.224096613958)) ;
#64100=CARTESIAN_POINT('Ctrl Pts',(-18.8961432339119,-48.7886498478435,
121.99432181877)) ;
#64101=CARTESIAN_POINT('Ctrl Pts',(-18.9987559919676,-48.6086607674806,
122.27782549784)) ;
#64102=CARTESIAN_POINT('Ctrl Pts',(-18.6575880747036,-48.7986555876417,
122.104972809918)) ;
#64103=CARTESIAN_POINT('Ctrl Pts',(-18.8079128155078,-48.6186665072788,
122.366348201292)) ;
#64104=CARTESIAN_POINT('Ctrl Pts',(-18.4417397385889,-48.8086764897881,
122.255816146101)) ;
#64105=CARTESIAN_POINT('Ctrl Pts',(-18.6352354003947,-48.6286874094252,
122.487024632224)) ;
#64106=CARTESIAN_POINT('Ctrl Pts',(-18.2575608011542,-48.818567259837,122.439229061463)) ;
#64107=CARTESIAN_POINT('Ctrl Pts',(-18.4878939926653,-48.6385781794741,
122.633756241431)) ;
#64108=CARTESIAN_POINT('Ctrl Pts',(-18.106193675921,-48.8285586706167,122.653759103654)) ;
#64109=CARTESIAN_POINT('Ctrl Pts',(-18.3668020674057,-48.6485695902538,
122.805381400602)) ;
#64110=CARTESIAN_POINT('Ctrl Pts',(-17.9949337392161,-48.8385070162812,
122.890328842219)) ;
#64111=CARTESIAN_POINT('Ctrl Pts',(-18.2777961188115,-48.6585179359183,
122.994637890624)) ;
#64112=CARTESIAN_POINT('Ctrl Pts',(-17.9259246879504,-48.8484518743424,
123.142417551886)) ;
#64113=CARTESIAN_POINT('Ctrl Pts',(-18.2225909149543,-48.6684627939795,
123.196309167332)) ;
#64114=CARTESIAN_POINT('Ctrl Pts',(-17.9018586345267,-48.8585067097353,
123.405524737978)) ;
#64115=CARTESIAN_POINT('Ctrl Pts',(-18.2033401477523,-48.6785176293724,
123.406795195145)) ;
#64116=CARTESIAN_POINT('Ctrl Pts',(-17.9228907005279,-48.8683290818368,
123.662811089171)) ;
#64117=CARTESIAN_POINT('Ctrl Pts',(-18.2201677808873,-48.6883400014739,
123.612623483924)) ;
#64118=CARTESIAN_POINT('Ctrl Pts',(-17.9893599290882,-48.8783849492805,
123.918552606262)) ;
#64119=CARTESIAN_POINT('Ctrl Pts',(-18.2733451048243,-48.6983958689176,
123.817216284864)) ;
#64120=CARTESIAN_POINT('Ctrl Pts',(-18.0984022475195,-48.8883256791384,
124.155949320405)) ;
#64121=CARTESIAN_POINT('Ctrl Pts',(-18.360580702555,-48.7083365987755,124.007132560782)) ;
#64122=CARTESIAN_POINT('Ctrl Pts',(-18.2457897778608,-48.8982300176895,
124.370478803514)) ;
#64123=CARTESIAN_POINT('Ctrl Pts',(-18.4784920796112,-48.7182409373267,
124.178754699922)) ;
#64124=CARTESIAN_POINT('Ctrl Pts',(-18.4309099578703,-48.908276699118,124.558689346407)) ;
#64125=CARTESIAN_POINT('Ctrl Pts',(-18.6265896773682,-48.7282876187551,
124.329321820861)) ;
#64126=CARTESIAN_POINT('Ctrl Pts',(-18.6425771224679,-48.9181722065873,
124.709824664085)) ;
#64127=CARTESIAN_POINT('Ctrl Pts',(-18.7959241464339,-48.7381831262244,
124.450228239053)) ;
#64128=CARTESIAN_POINT('Ctrl Pts',(-18.8811535876977,-48.9282344750859,
124.823761366572)) ;
#64129=CARTESIAN_POINT('Ctrl Pts',(-18.986786280884,-48.748245394723,124.541375925979)) ;
#64130=CARTESIAN_POINT('Ctrl Pts',(-19.1303382919628,-48.9380764653565,
124.893166471091)) ;
#64131=CARTESIAN_POINT('Ctrl Pts',(-19.18613388542,-48.7580873849936,124.596897991502)) ;
#64132=CARTESIAN_POINT('Ctrl Pts',(-19.3916192445913,-48.9480698822375,
124.919216288475)) ;
#64133=CARTESIAN_POINT('Ctrl Pts',(-19.3951586909665,-48.7680808018746,
124.617736026515)) ;
#64134=CARTESIAN_POINT('Ctrl Pts',(-19.6517180268275,-48.9579943700896,
124.899657271309)) ;
#64135=CARTESIAN_POINT('Ctrl Pts',(-19.6032371787446,-48.7780052897268,
124.602087041937)) ;
#64136=CARTESIAN_POINT('Ctrl Pts',(-19.9064040385048,-48.9679940039981,
124.835026142014)) ;
#64137=CARTESIAN_POINT('Ctrl Pts',(-19.8069854638334,-48.7880049236352,
124.550380450082)) ;
#64138=CARTESIAN_POINT('Ctrl Pts',(-20.145734566015,-48.9779801142549,124.72728379971)) ;
#64139=CARTESIAN_POINT('Ctrl Pts',(-19.9984490348426,-48.797991033892,124.464185028181)) ;
#64140=CARTESIAN_POINT('Ctrl Pts',(-20.363595758635,-48.988016065442,124.578693439179)) ;
#64141=CARTESIAN_POINT('Ctrl Pts',(-20.1727370240025,-48.8080269850791,
124.345311205248)) ;
#64142=CARTESIAN_POINT('Ctrl Pts',(-20.5492835774246,-48.9978727037768,
124.398066759077)) ;
#64143=CARTESIAN_POINT('Ctrl Pts',(-20.321285535719,-48.8178836234139,124.200809123624)) ;
#64144=CARTESIAN_POINT('Ctrl Pts',(-20.7032232576622,-49.0078716638548,
124.185175408038)) ;
#64145=CARTESIAN_POINT('Ctrl Pts',(-20.4444358521844,-48.8278825834919,
124.030495143245)) ;
#64146=CARTESIAN_POINT('Ctrl Pts',(-20.8169628556699,-49.0177668941686,
123.951284538968)) ;
#64147=CARTESIAN_POINT('Ctrl Pts',(-20.5354258074483,-48.8377778138057,
123.84338226399)) ;
#64148=CARTESIAN_POINT('Ctrl Pts',(-20.8895070310717,-49.0278274066372,
123.697088016909)) ;
#64149=CARTESIAN_POINT('Ctrl Pts',(-20.5934596252462,-48.8478383262744,
123.640024411145)) ;
#64150=CARTESIAN_POINT('Ctrl Pts',(-20.9163903855367,-49.0376766981834,
123.439638200355)) ;
#64151=CARTESIAN_POINT('Ctrl Pts',(-20.6149646209664,-48.8576876178205,
123.434065220729)) ;
#64152=CARTESIAN_POINT('Ctrl Pts',(-20.8985020837487,-49.0477038841156,
123.176748817994)) ;
#64153=CARTESIAN_POINT('Ctrl Pts',(-20.6006524960591,-48.8677148037527,
123.223753784893)) ;
#64154=CARTESIAN_POINT('Ctrl Pts',(-20.8345541010092,-49.0577324205749,
122.921071960557)) ;
#64155=CARTESIAN_POINT('Ctrl Pts',(-20.5494925272255,-48.8777433402121,
123.019212637237)) ;
#64156=CARTESIAN_POINT('Ctrl Pts',(-20.7296054273253,-49.0675776605399,
122.68460614522)) ;
#64157=CARTESIAN_POINT('Ctrl Pts',(-20.4655325601765,-48.887588580177,122.830041421681)) ;
#64158=CARTESIAN_POINT('Ctrl Pts',(-20.5836317515741,-49.0775683554631,
122.466374760989)) ;
#64159=CARTESIAN_POINT('Ctrl Pts',(-20.3487525572943,-48.8975792751002,
122.655457213119)) ;
#64160=CARTESIAN_POINT('Ctrl Pts',(-20.4007099669352,-49.0876061762217,
122.276320211683)) ;
#64161=CARTESIAN_POINT('Ctrl Pts',(-20.202413975225,-48.9076170958588,122.503414537184)) ;
#64162=CARTESIAN_POINT('Ctrl Pts',(-20.1919240683842,-49.0974507699987,
122.123545795109)) ;
#64163=CARTESIAN_POINT('Ctrl Pts',(-20.0353851785869,-48.9174616896358,
122.381196695483)) ;
#64164=CARTESIAN_POINT('Ctrl Pts',(-19.9567693977097,-49.1074347653747,
122.00723791885)) ;
#64165=CARTESIAN_POINT('Ctrl Pts',(-19.8472610587631,-48.9274456850118,
122.288151648235)) ;
#64166=CARTESIAN_POINT('Ctrl Pts',(-19.705830459049,-49.1173838139361,121.933802445044)) ;
#64167=CARTESIAN_POINT('Ctrl Pts',(-19.646509912876,-48.9373947335732,122.229404623023)) ;
#64168=CARTESIAN_POINT('Ctrl Pts',(-19.4445921214419,-49.1273862529106,
121.904618015651)) ;
#64169=CARTESIAN_POINT('Ctrl Pts',(-19.437519186954,-48.9473971725478,122.206058321962)) ;
#64170=CARTESIAN_POINT('Ctrl Pts',(-19.1817922313132,-49.137407494207,121.921624060379)) ;
#64171=CARTESIAN_POINT('Ctrl Pts',(-19.2272793333639,-48.9574184138441,
122.219664472921)) ;
#64172=CARTESIAN_POINT('Ctrl Pts',(-18.9291459751133,-49.1473001726465,
121.982897915693)) ;
#64173=CARTESIAN_POINT('Ctrl Pts',(-19.025163319022,-48.9673110922836,122.268684604712)) ;
#64174=CARTESIAN_POINT('Ctrl Pts',(-18.6884670363836,-49.1572902265941,
122.087747388181)) ;
#64175=CARTESIAN_POINT('Ctrl Pts',(-18.8326207934705,-48.9773011462313,
122.352565175257)) ;
#64176=CARTESIAN_POINT('Ctrl Pts',(-18.4704519830292,-49.1672485877426,
122.232485671817)) ;
#64177=CARTESIAN_POINT('Ctrl Pts',(-18.6582097022475,-48.9872595073797,
122.468356610712)) ;
#64178=CARTESIAN_POINT('Ctrl Pts',(-18.2815383415692,-49.1771482146274,
122.411369259889)) ;
#64179=CARTESIAN_POINT('Ctrl Pts',(-18.5070800263305,-48.9971591342646,
122.611463763631)) ;
#64180=CARTESIAN_POINT('Ctrl Pts',(-18.1243345330828,-49.1871961114308,
122.623486945981)) ;
#64181=CARTESIAN_POINT('Ctrl Pts',(-18.3813177411218,-49.0072070310679,
122.781158694447)) ;
#64182=CARTESIAN_POINT('Ctrl Pts',(-18.0079271717103,-49.1970914690668,
122.856062333984)) ;
#64183=CARTESIAN_POINT('Ctrl Pts',(-18.2881931003449,-49.0171023887039,
122.967218812396)) ;
#64184=CARTESIAN_POINT('Ctrl Pts',(-17.9324068931307,-49.2071531215235,
123.109426695893)) ;
#64185=CARTESIAN_POINT('Ctrl Pts',(-18.2277777834536,-49.0271640411606,
123.169910844373)) ;
#64186=CARTESIAN_POINT('Ctrl Pts',(-17.9026375541845,-49.2169977257954,
123.366423552934)) ;
#64187=CARTESIAN_POINT('Ctrl Pts',(-18.2039634417627,-49.0370086454325,
123.375507396247)) ;
#64188=CARTESIAN_POINT('Ctrl Pts',(-17.9171858178237,-49.2269578474934,
123.62775607521)) ;
#64189=CARTESIAN_POINT('Ctrl Pts',(-18.2156028245757,-49.0469687671305,
123.584573004918)) ;
#64190=CARTESIAN_POINT('Ctrl Pts',(-17.9778519477484,-49.2369958818559,
123.884464098742)) ;
#64191=CARTESIAN_POINT('Ctrl Pts',(-18.2641366483863,-49.0570068014931,
123.789939339049)) ;
#64192=CARTESIAN_POINT('Ctrl Pts',(-18.0800477463435,-49.2468701944424,
124.123014445666)) ;
#64193=CARTESIAN_POINT('Ctrl Pts',(-18.3458936691752,-49.0668811140795,
123.980778477681)) ;
#64194=CARTESIAN_POINT('Ctrl Pts',(-18.2248917333607,-49.2569396752251,
124.344424493672)) ;
#64195=CARTESIAN_POINT('Ctrl Pts',(-18.4617697106575,-49.0769505948622,
124.157906347072)) ;
#64196=CARTESIAN_POINT('Ctrl Pts',(-18.4016886197062,-49.2667740112422,
124.532954912051)) ;
#64197=CARTESIAN_POINT('Ctrl Pts',(-18.6032069775405,-49.0867849308793,
124.308729299601)) ;
#64198=CARTESIAN_POINT('Ctrl Pts',(-18.612254092902,-49.2768069689704,124.691612235755)) ;
#64199=CARTESIAN_POINT('Ctrl Pts',(-18.7716597901353,-49.0968178886076,
124.435654741883)) ;
#64200=CARTESIAN_POINT('Ctrl Pts',(-18.8472145112584,-49.2868273675456,
124.810505656813)) ;
#64201=CARTESIAN_POINT('Ctrl Pts',(-18.9596285027308,-49.1068382871827,
124.530768800945)) ;
#64202=CARTESIAN_POINT('Ctrl Pts',(-19.0951813191321,-49.2966929413168,
124.886249263445)) ;
#64203=CARTESIAN_POINT('Ctrl Pts',(-19.158001200267,-49.116703860954,124.59136281955)) ;
#64204=CARTESIAN_POINT('Ctrl Pts',(-19.3577881565911,-49.3067618159729,
124.918435602837)) ;
#64205=CARTESIAN_POINT('Ctrl Pts',(-19.3680870720684,-49.12677273561,124.617111322248)) ;
#64206=CARTESIAN_POINT('Ctrl Pts',(-19.6161749842658,-49.3166072468784,
124.904881658473)) ;
#64207=CARTESIAN_POINT('Ctrl Pts',(-19.5747953751554,-49.1366181665155,
124.606267622671)) ;
#64208=CARTESIAN_POINT('Ctrl Pts',(-19.8718870581051,-49.3265868717491,
124.846704436863)) ;
#64209=CARTESIAN_POINT('Ctrl Pts',(-19.7793647044864,-49.1465977913862,
124.55972551948)) ;
#64210=CARTESIAN_POINT('Ctrl Pts',(-20.1143655069739,-49.3366055546632,
124.74415269252)) ;
#64211=CARTESIAN_POINT('Ctrl Pts',(-19.9733472699668,-49.1566164743003,
124.477683643661)) ;
#64212=CARTESIAN_POINT('Ctrl Pts',(-20.3326993754849,-49.346488819847,124.603431043373)) ;
#64213=CARTESIAN_POINT('Ctrl Pts',(-20.148013421792,-49.1664997394842,124.365106482365)) ;
#64214=CARTESIAN_POINT('Ctrl Pts',(-20.5267164375359,-49.3565571139384,
124.423600519391)) ;
#64215=CARTESIAN_POINT('Ctrl Pts',(-20.3032270348823,-49.1765680335755,
124.221241540364)) ;
#64216=CARTESIAN_POINT('Ctrl Pts',(-20.6830755384687,-49.3663872441237,
124.217913860219)) ;
#64217=CARTESIAN_POINT('Ctrl Pts',(-20.4283133065888,-49.1863981637609,
124.056692994351)) ;
#64218=CARTESIAN_POINT('Ctrl Pts',(-20.8044543031149,-49.3764537923389,
123.982913211132)) ;
#64219=CARTESIAN_POINT('Ctrl Pts',(-20.5254162463695,-49.196464711976,123.868692079819)) ;
#64220=CARTESIAN_POINT('Ctrl Pts',(-20.881675014768,-49.3863440410275,123.734710364339)) ;
#64221=CARTESIAN_POINT('Ctrl Pts',(-20.5871922922867,-49.2063549606646,
123.670130518056)) ;
#64222=CARTESIAN_POINT('Ctrl Pts',(-20.9155298639726,-49.3963362228035,
123.474333218862)) ;
#64223=CARTESIAN_POINT('Ctrl Pts',(-20.6142760088709,-49.2163471424406,
123.461828953088)) ;
#64224=CARTESIAN_POINT('Ctrl Pts',(-20.9034492216854,-49.4062990034313,
123.212805454271)) ;
#64225=CARTESIAN_POINT('Ctrl Pts',(-20.6046113070106,-49.2263099230684,
123.252607116101)) ;
#64226=CARTESIAN_POINT('Ctrl Pts',(-20.847109080545,-49.4162034081051,122.958679801309)) ;
#64227=CARTESIAN_POINT('Ctrl Pts',(-20.5595393178523,-49.2362143277422,
123.04930733304)) ;
#64228=CARTESIAN_POINT('Ctrl Pts',(-20.7457693980106,-49.4262634025841,
122.714534227944)) ;
#64229=CARTESIAN_POINT('Ctrl Pts',(-20.4784673873757,-49.2462743222212,
122.853990658576)) ;
#64230=CARTESIAN_POINT('Ctrl Pts',(-20.6067290420419,-49.4361120245539,
122.496219298933)) ;
#64231=CARTESIAN_POINT('Ctrl Pts',(-20.3672356811197,-49.256122944191,122.679339680775)) ;
#64232=CARTESIAN_POINT('Ctrl Pts',(-20.4291275579387,-49.4461424639657,
122.301465539573)) ;
#64233=CARTESIAN_POINT('Ctrl Pts',(-20.2251545164189,-49.2661533836029,
122.523536525192)) ;
#64234=CARTESIAN_POINT('Ctrl Pts',(-20.2204806965298,-49.4561521796005,
122.141233524308)) ;
#64235=CARTESIAN_POINT('Ctrl Pts',(-20.0582370435673,-49.2761630992376,
122.395350947196)) ;
#64236=CARTESIAN_POINT('Ctrl Pts',(-19.9896519589518,-49.4660629322931,
122.020664911616)) ;
#64237=CARTESIAN_POINT('Ctrl Pts',(-19.8735747112757,-49.2860738519302,
122.298896350739)) ;
#64238=CARTESIAN_POINT('Ctrl Pts',(-19.7410945155268,-49.4759922052395,
121.941224683221)) ;
#64239=CARTESIAN_POINT('Ctrl Pts',(-19.674729389547,-49.2960031248766,122.235344147617)) ;
#64240=CARTESIAN_POINT('Ctrl Pts',(-19.4795590978915,-49.4860348966322,
121.90597303431)) ;
#64241=CARTESIAN_POINT('Ctrl Pts',(-19.4655009066754,-49.3060458162693,
122.207142650007)) ;
#64242=CARTESIAN_POINT('Ctrl Pts',(-19.219942862055,-49.4959214298497,121.916333239462)) ;
#64243=CARTESIAN_POINT('Ctrl Pts',(-19.2578087796181,-49.3159323494868,
122.215430581112)) ;
#64244=CARTESIAN_POINT('Ctrl Pts',(-18.9632658837388,-49.5059145747817,
121.971768765229)) ;
#64245=CARTESIAN_POINT('Ctrl Pts',(-19.0524672904058,-49.3259254944189,
122.259778662686)) ;
#64246=CARTESIAN_POINT('Ctrl Pts',(-18.7212920167133,-49.5158602556182,
122.070557018529)) ;
#64247=CARTESIAN_POINT('Ctrl Pts',(-18.8588885297617,-49.3358711752553,
122.338808821512)) ;
#64248=CARTESIAN_POINT('Ctrl Pts',(-18.499816284014,-49.5258075127667,122.209435357243)) ;
#64249=CARTESIAN_POINT('Ctrl Pts',(-18.6817081096544,-49.3458184324039,
122.449910892272)) ;
#64250=CARTESIAN_POINT('Ctrl Pts',(-18.3040709556974,-49.5358554166387,
122.386637839566)) ;
#64251=CARTESIAN_POINT('Ctrl Pts',(-18.5251114670603,-49.3558663362759,
122.591672756877)) ;
#64252=CARTESIAN_POINT('Ctrl Pts',(-18.1451172426182,-49.5457031157367,
122.590856449756)) ;
#64253=CARTESIAN_POINT('Ctrl Pts',(-18.3979488685203,-49.3657140353738,
122.755046516047)) ;
#64254=CARTESIAN_POINT('Ctrl Pts',(-18.0219137176075,-49.5556646067154,
122.821817640682)) ;
#64255=CARTESIAN_POINT('Ctrl Pts',(-18.2993856846161,-49.3756755263525,
122.939814861468)) ;
#64256=CARTESIAN_POINT('Ctrl Pts',(-17.940459021946,-49.5656940691293,123.072489705636)) ;
#64257=CARTESIAN_POINT('Ctrl Pts',(-18.2342214104261,-49.3857049887665,
123.140352429838)) ;
#64258=CARTESIAN_POINT('Ctrl Pts',(-17.9040753303837,-49.5756013002292,
123.330287135663)) ;
#64259=CARTESIAN_POINT('Ctrl Pts',(-18.2051140105785,-49.3956122198664,
123.346589589261)) ;
#64260=CARTESIAN_POINT('Ctrl Pts',(-17.9125098782815,-49.5855476789066,
123.591516015328)) ;
#64261=CARTESIAN_POINT('Ctrl Pts',(-18.2118609481446,-49.4055585985438,
123.555572243342)) ;
#64262=CARTESIAN_POINT('Ctrl Pts',(-17.9664056109614,-49.5955524477155,
123.848870528812)) ;
#64263=CARTESIAN_POINT('Ctrl Pts',(-18.2549768267066,-49.4155633673526,
123.761455926636)) ;
#64264=CARTESIAN_POINT('Ctrl Pts',(-18.0645967713653,-49.6055735687357,
124.09321890463)) ;
#64265=CARTESIAN_POINT('Ctrl Pts',(-18.3335291813953,-49.4255844883728,
123.95693488968)) ;
#64266=CARTESIAN_POINT('Ctrl Pts',(-18.201669169235,-49.6154644345883,124.314070124033)) ;
#64267=CARTESIAN_POINT('Ctrl Pts',(-18.4431860779359,-49.4354753542255,
124.133615557219)) ;
#64268=CARTESIAN_POINT('Ctrl Pts',(-18.3764527037186,-49.6254552433476,
124.509963682935)) ;
#64269=CARTESIAN_POINT('Ctrl Pts',(-18.5830121977067,-49.4454661629847,
124.290330807483)) ;
#64270=CARTESIAN_POINT('Ctrl Pts',(-18.5818191091062,-49.6354059015279,
124.671858407225)) ;
#64271=CARTESIAN_POINT('Ctrl Pts',(-18.747304497956,-49.4554168211651,124.41984693504)) ;
#64272=CARTESIAN_POINT('Ctrl Pts',(-18.8116465771157,-49.64534211117,124.795748611683)) ;
#64273=CARTESIAN_POINT('Ctrl Pts',(-18.9311656103158,-49.4653530308072,
124.518959622352)) ;
#64274=CARTESIAN_POINT('Ctrl Pts',(-19.0606091019556,-49.6553252778949,
124.878578886078)) ;
#64275=CARTESIAN_POINT('Ctrl Pts',(-19.1303351363198,-49.475336197532,124.585224676569)) ;
#64276=CARTESIAN_POINT('Ctrl Pts',(-19.3217571085356,-49.6653690751052,
124.916663479526)) ;
#64277=CARTESIAN_POINT('Ctrl Pts',(-19.3392535710715,-49.4853799947423,
124.615693198187)) ;
#64278=CARTESIAN_POINT('Ctrl Pts',(-19.5799756953038,-49.6751972912734,
124.909602892924)) ;
#64279=CARTESIAN_POINT('Ctrl Pts',(-19.5458273138333,-49.4952082109106,
124.610045737877)) ;
#64280=CARTESIAN_POINT('Ctrl Pts',(-19.8393726054235,-49.6852738587427,
124.85664781919)) ;
#64281=CARTESIAN_POINT('Ctrl Pts',(-19.7533453820382,-49.5052847783798,
124.567682597387)) ;
#64282=CARTESIAN_POINT('Ctrl Pts',(-20.0802989166778,-49.6951259444321,
124.761703259049)) ;
#64283=CARTESIAN_POINT('Ctrl Pts',(-19.9460858927394,-49.5151368640692,
124.491728274294)) ;
#64284=CARTESIAN_POINT('Ctrl Pts',(-20.3060674976311,-49.7051992118375,
124.623574721995)) ;
#64285=CARTESIAN_POINT('Ctrl Pts',(-20.1267015988155,-49.5252101314746,
124.381226205106)) ;
#64286=CARTESIAN_POINT('Ctrl Pts',(-20.4998566127892,-49.7150406282611,
124.452283158232)) ;
#64287=CARTESIAN_POINT('Ctrl Pts',(-20.2817328184751,-49.5350515478982,
124.244194445969)) ;
#64288=CARTESIAN_POINT('Ctrl Pts',(-20.6636690759953,-49.7250018864038,
124.248115309277)) ;
#64289=CARTESIAN_POINT('Ctrl Pts',(-20.412783592269,-49.545012806041,124.080861225897)) ;
#64290=CARTESIAN_POINT('Ctrl Pts',(-20.7900512077694,-49.7350385628358,
124.016618869433)) ;
#64291=CARTESIAN_POINT('Ctrl Pts',(-20.5138903779245,-49.5550494824729,
123.895664546268)) ;
#64292=CARTESIAN_POINT('Ctrl Pts',(-20.8734168716423,-49.7449171706996,
123.770739635616)) ;
#64293=CARTESIAN_POINT('Ctrl Pts',(-20.5805838585332,-49.5649280903367,
123.698962322209)) ;
#64294=CARTESIAN_POINT('Ctrl Pts',(-20.9135969834897,-49.7549773993384,
123.509473505377)) ;
#64295=CARTESIAN_POINT('Ctrl Pts',(-20.6127292533526,-49.5749883189755,
123.489949387837)) ;
#64296=CARTESIAN_POINT('Ctrl Pts',(-20.9079881465136,-49.7648443834992,
123.250206599961)) ;
#64297=CARTESIAN_POINT('Ctrl Pts',(-20.6082434986379,-49.5848553031363,
123.282536664813)) ;
#64298=CARTESIAN_POINT('Ctrl Pts',(-20.8572486896229,-49.7748499497519,
122.992248525013)) ;
#64299=CARTESIAN_POINT('Ctrl Pts',(-20.5676533267145,-49.594860869389,123.076169999909)) ;
#64300=CARTESIAN_POINT('Ctrl Pts',(-20.762604793769,-49.7848337381665,122.747500893272)) ;
#64301=CARTESIAN_POINT('Ctrl Pts',(-20.4919395690296,-49.6048446578036,
122.88037156088)) ;
#64302=CARTESIAN_POINT('Ctrl Pts',(-20.6258474889343,-49.7948795949691,
122.521714953431)) ;
#64303=CARTESIAN_POINT('Ctrl Pts',(-20.3825347960662,-49.6148905146063,
122.699742010315)) ;
#64304=CARTESIAN_POINT('Ctrl Pts',(-20.4560100049214,-49.8047054721851,
122.327215170071)) ;
#64305=CARTESIAN_POINT('Ctrl Pts',(-20.246666541654,-49.6247163918222,122.544142037423)) ;
#64306=CARTESIAN_POINT('Ctrl Pts',(-20.2521537953988,-49.8146959480264,
122.161777820883)) ;
#64307=CARTESIAN_POINT('Ctrl Pts',(-20.0835826717048,-49.6347068676635,
122.411791024612)) ;
#64308=CARTESIAN_POINT('Ctrl Pts',(-20.0211126978458,-49.8247395239252,
122.03417835331)) ;
#64309=CARTESIAN_POINT('Ctrl Pts',(-19.8987503848234,-49.6447504435623,
122.30971013817)) ;
#64310=CARTESIAN_POINT('Ctrl Pts',(-19.7771162248852,-49.8345613162232,
121.950011278901)) ;
#64311=CARTESIAN_POINT('Ctrl Pts',(-19.7035546511395,-49.6545722358604,
122.242375346219)) ;
#64312=CARTESIAN_POINT('Ctrl Pts',(-19.5167805110166,-49.8445962818491,
121.907971037279)) ;
#64313=CARTESIAN_POINT('Ctrl Pts',(-19.4952862619387,-49.6646072014862,
122.208741497832)) ;
#64314=CARTESIAN_POINT('Ctrl Pts',(-19.25336832143,-49.8546211987822,121.912502122807)) ;
#64315=CARTESIAN_POINT('Ctrl Pts',(-19.2845564644904,-49.6746321184193,
122.212364842142)) ;
#64316=CARTESIAN_POINT('Ctrl Pts',(-18.9991000929311,-49.8644731371583,
121.961278882292)) ;
#64317=CARTESIAN_POINT('Ctrl Pts',(-19.0811423664437,-49.6844840567954,
122.251384496068)) ;
#64318=CARTESIAN_POINT('Ctrl Pts',(-18.7536426685323,-49.8744641131831,
122.054376600934)) ;
#64319=CARTESIAN_POINT('Ctrl Pts',(-18.8847759503893,-49.6944750328202,
122.325861028897)) ;
#64320=CARTESIAN_POINT('Ctrl Pts',(-18.5295831349131,-49.8843819339867,
122.187580190448)) ;
#64321=CARTESIAN_POINT('Ctrl Pts',(-18.7055278321113,-49.7043928536238,
122.432422178777)) ;
#64322=CARTESIAN_POINT('Ctrl Pts',(-18.3298664401693,-49.8944106545513,
122.359492881508)) ;
#64323=CARTESIAN_POINT('Ctrl Pts',(-18.5457533183806,-49.7144215741884,
122.569951033302)) ;
#64324=CARTESIAN_POINT('Ctrl Pts',(-18.1652873217021,-49.9042935811605,
122.56043375668)) ;
#64325=CARTESIAN_POINT('Ctrl Pts',(-18.4140890357409,-49.7243045007976,
122.730702147218)) ;
#64326=CARTESIAN_POINT('Ctrl Pts',(-18.0361983461571,-49.91429786628,122.789426912467)) ;
#64327=CARTESIAN_POINT('Ctrl Pts',(-18.3108162891678,-49.7343087859171,
122.913895707216)) ;
#64328=CARTESIAN_POINT('Ctrl Pts',(-17.949014297203,-49.9242815474878,123.036925185848)) ;
#64329=CARTESIAN_POINT('Ctrl Pts',(-18.2410673737591,-49.7442924671249,
123.111893582383)) ;
#64330=CARTESIAN_POINT('Ctrl Pts',(-17.9061915789435,-49.9343225462177,
123.297274155865)) ;
#64331=CARTESIAN_POINT('Ctrl Pts',(-18.2068074268591,-49.7543334658549,
123.32017254399)) ;
#64332=CARTESIAN_POINT('Ctrl Pts',(-17.9087977233851,-49.9441549910849,
123.555650792521)) ;
#64333=CARTESIAN_POINT('Ctrl Pts',(-18.2088904958492,-49.764165910722,123.526873108748)) ;
#64334=CARTESIAN_POINT('Ctrl Pts',(-17.9562480238635,-49.9541499895152,
123.81397987155)) ;
#64335=CARTESIAN_POINT('Ctrl Pts',(-18.2468487951362,-49.7741609091523,
123.733536626353)) ;
#64336=CARTESIAN_POINT('Ctrl Pts',(-18.0487030674048,-49.9641815382648,
124.060868717992)) ;
#64337=CARTESIAN_POINT('Ctrl Pts',(-18.3208110873252,-49.7841924579019,
123.93104838714)) ;
#64338=CARTESIAN_POINT('Ctrl Pts',(-18.1801084382992,-49.9740469165703,
124.284334653721)) ;
#64339=CARTESIAN_POINT('Ctrl Pts',(-18.4259334333969,-49.7940578362074,
124.109821606921)) ;
#64340=CARTESIAN_POINT('Ctrl Pts',(-18.3494144439518,-49.9840087640306,
124.484014610873)) ;
#64341=CARTESIAN_POINT('Ctrl Pts',(-18.56137656749,-49.8040196836677,124.269566724914)) ;
#64342=CARTESIAN_POINT('Ctrl Pts',(-18.5525546909306,-49.9940437048448,
124.652146083478)) ;
#64343=CARTESIAN_POINT('Ctrl Pts',(-18.7238875347409,-49.814054624482,124.404073431929)) ;
#64344=CARTESIAN_POINT('Ctrl Pts',(-18.7782043027359,-50.003928665862,124.780909685819)) ;
#64345=CARTESIAN_POINT('Ctrl Pts',(-18.9044058329455,-49.8239395854991,
124.507085842024)) ;
#64346=CARTESIAN_POINT('Ctrl Pts',(-19.0271970940224,-50.0139942747808,
124.870056934491)) ;
#64347=CARTESIAN_POINT('Ctrl Pts',(-19.1035994992475,-49.8340051944179,
124.578405575516)) ;
#64348=CARTESIAN_POINT('Ctrl Pts',(-19.2820603187455,-50.0238334498225,
124.913884244235)) ;
#64349=CARTESIAN_POINT('Ctrl Pts',(-19.3074891770789,-49.8438443694597,
124.613469338266)) ;
#64350=CARTESIAN_POINT('Ctrl Pts',(-19.5464617510403,-50.0338960053224,
124.913133557086)) ;
#64351=CARTESIAN_POINT('Ctrl Pts',(-19.5190104339783,-49.8539069249596,
124.61287087145)) ;
#64352=CARTESIAN_POINT('Ctrl Pts',(-19.8024340996347,-50.0437931800154,
124.866966630769)) ;
#64353=CARTESIAN_POINT('Ctrl Pts',(-19.7237883101448,-49.8638040996525,
124.575939415286)) ;
#64354=CARTESIAN_POINT('Ctrl Pts',(-20.0476128622874,-50.0537238949387,
124.777581121014)) ;
#64355=CARTESIAN_POINT('Ctrl Pts',(-19.9199318279951,-49.8737348145758,
124.504433101703)) ;
#64356=CARTESIAN_POINT('Ctrl Pts',(-20.2759720546877,-50.0637679230163,
124.645229703549)) ;
#64357=CARTESIAN_POINT('Ctrl Pts',(-20.1026202614428,-49.8837788426534,
124.398553782836)) ;
#64358=CARTESIAN_POINT('Ctrl Pts',(-20.4748580560086,-50.0736541248696,
124.478049522978)) ;
#64359=CARTESIAN_POINT('Ctrl Pts',(-20.2617301731961,-49.8936650445067,
124.264811487387)) ;
#64360=CARTESIAN_POINT('Ctrl Pts',(-20.6437749690615,-50.0836472913365,
124.277011182732)) ;
#64361=CARTESIAN_POINT('Ctrl Pts',(-20.396865308046,-49.9036582109736,124.103982270604)) ;
#64362=CARTESIAN_POINT('Ctrl Pts',(-20.7746102355523,-50.0935867623236,
124.050904663364)) ;
#64363=CARTESIAN_POINT('Ctrl Pts',(-20.5015353032639,-49.9135976819608,
123.92309830424)) ;
#64364=CARTESIAN_POINT('Ctrl Pts',(-20.8649209945911,-50.1036032766778,
123.803687664981)) ;
#64365=CARTESIAN_POINT('Ctrl Pts',(-20.5737859376745,-49.9236141963149,
123.725325490292)) ;
#64366=CARTESIAN_POINT('Ctrl Pts',(-20.9107662307901,-50.1135333031546,
123.546758707773)) ;
#64367=CARTESIAN_POINT('Ctrl Pts',(-20.610464245172,-49.9335442227918,123.519782903442)) ;
#64368=CARTESIAN_POINT('Ctrl Pts',(-20.9111940114087,-50.1235858386641,
123.282611468914)) ;
#64369=CARTESIAN_POINT('Ctrl Pts',(-20.6108086511653,-49.9435967583012,
123.308465098402)) ;
#64370=CARTESIAN_POINT('Ctrl Pts',(-20.8668229607071,-50.1334322418838,
123.02768188537)) ;
#64371=CARTESIAN_POINT('Ctrl Pts',(-20.5753140241265,-49.9534431615209,
123.104521371413)) ;
#64372=CARTESIAN_POINT('Ctrl Pts',(-20.7786326898469,-50.1433942847378,
122.781207115451)) ;
#64373=CARTESIAN_POINT('Ctrl Pts',(-20.5047639491462,-49.963405204375,122.907340893886)) ;
#64374=CARTESIAN_POINT('Ctrl Pts',(-20.6478070135381,-50.1534228355285,
122.552412487854)) ;
#64375=CARTESIAN_POINT('Ctrl Pts',(-20.400105350936,-49.9734337551656,122.724304121501)) ;
#64376=CARTESIAN_POINT('Ctrl Pts',(-20.4813154002532,-50.1633331612461,
122.352163354463)) ;
#64377=CARTESIAN_POINT('Ctrl Pts',(-20.2669138792127,-49.9833440808833,
122.564103520818)) ;
#64378=CARTESIAN_POINT('Ctrl Pts',(-20.2825162867384,-50.1732680730757,
122.182913771946)) ;
#64379=CARTESIAN_POINT('Ctrl Pts',(-20.107876126385,-49.9932789927128,122.42870221035)) ;
#64380=CARTESIAN_POINT('Ctrl Pts',(-20.0548359115821,-50.1833090798438,
122.049558725394)) ;
#64381=CARTESIAN_POINT('Ctrl Pts',(-19.9257329909012,-50.0033199994809,
122.322016258521)) ;
#64382=CARTESIAN_POINT('Ctrl Pts',(-19.8112788264307,-50.193196712676,121.958995011386)) ;
#64383=CARTESIAN_POINT('Ctrl Pts',(-19.7308882259912,-50.0132076323131,
122.249563225972)) ;
#64384=CARTESIAN_POINT('Ctrl Pts',(-19.5531495649687,-50.203187143774,121.911155500967)) ;
#64385=CARTESIAN_POINT('Ctrl Pts',(-19.5243852785124,-50.0231980634112,
122.211289414015)) ;
#64386=CARTESIAN_POINT('Ctrl Pts',(-19.2915318676096,-50.2131425803313,
121.909011127631)) ;
#64387=CARTESIAN_POINT('Ctrl Pts',(-19.3150912261265,-50.0331534999684,
122.209571651062)) ;
#64388=CARTESIAN_POINT('Ctrl Pts',(-19.0346123538421,-50.2230535284306,
121.951656547324)) ;
#64389=CARTESIAN_POINT('Ctrl Pts',(-19.1095552462161,-50.0430644480677,
122.243685801554)) ;
#64390=CARTESIAN_POINT('Ctrl Pts',(-18.7863546985664,-50.2330656045283,
122.038872975967)) ;
#64391=CARTESIAN_POINT('Ctrl Pts',(-18.9109485915979,-50.0530765241654,
122.31345662738)) ;
#64392=CARTESIAN_POINT('Ctrl Pts',(-18.5569655230889,-50.2430929266033,
122.168505406507)) ;
#64393=CARTESIAN_POINT('Ctrl Pts',(-18.727435583092,-50.0631038462404,122.417161230504)) ;
#64394=CARTESIAN_POINT('Ctrl Pts',(-18.3565173091822,-50.2529517015574,
122.332725267675)) ;
#64395=CARTESIAN_POINT('Ctrl Pts',(-18.5670778973102,-50.0729626211945,
122.548532925854)) ;
#64396=CARTESIAN_POINT('Ctrl Pts',(-18.126853897068,-50.2663778943698,122.600443072369)) ;
#64397=CARTESIAN_POINT('Ctrl Pts',(-18.3833334664102,-50.086388814007,122.762717346392)) ;
#64398=CARTESIAN_POINT('Ctrl Pts',(-17.975652168747,-50.2794619101513,122.913754436189)) ;
#64399=CARTESIAN_POINT('Ctrl Pts',(-18.2623681321715,-50.0994728297884,
123.013391525604)) ;
#64400=CARTESIAN_POINT('Ctrl Pts',(-17.909201931477,-50.2929353589065,123.261460162963)) ;
#64401=CARTESIAN_POINT('Ctrl Pts',(-18.2092179634923,-50.1129462785436,
123.291511896051)) ;
#64402=CARTESIAN_POINT('Ctrl Pts',(-17.9058612706939,-50.3027683167123,
123.519872041659)) ;
#64403=CARTESIAN_POINT('Ctrl Pts',(-18.2065406001334,-50.1227792363495,
123.498250245797)) ;
#64404=CARTESIAN_POINT('Ctrl Pts',(-17.9468858271895,-50.312731590163,123.778444889116)) ;
#64405=CARTESIAN_POINT('Ctrl Pts',(-18.2393587805037,-50.1327425098001,
123.705106558061)) ;
#64406=CARTESIAN_POINT('Ctrl Pts',(-18.0333597051189,-50.322768663981,124.027627149675)) ;
#64407=CARTESIAN_POINT('Ctrl Pts',(-18.3085355866663,-50.1427795836181,
123.904453627933)) ;
#64408=CARTESIAN_POINT('Ctrl Pts',(-18.1593001786209,-50.3326436669926,
124.254558222492)) ;
#64409=CARTESIAN_POINT('Ctrl Pts',(-18.409286108333,-50.1526545866297,124.085999460383)) ;
#64410=CARTESIAN_POINT('Ctrl Pts',(-18.3258841681713,-50.3427113466188,
124.460049111905)) ;
#64411=CARTESIAN_POINT('Ctrl Pts',(-18.5425518166163,-50.1627222662559,
124.250393776869)) ;
#64412=CARTESIAN_POINT('Ctrl Pts',(-18.5210703743217,-50.3525521968365,
124.629743114865)) ;
#64413=CARTESIAN_POINT('Ctrl Pts',(-18.6986983036897,-50.1725631164736,
124.386149592484)) ;
#64414=CARTESIAN_POINT('Ctrl Pts',(-18.8210606852671,-50.3658883953125,
124.810877501075)) ;
#64415=CARTESIAN_POINT('Ctrl Pts',(-18.9386954921332,-50.1858993149496,
124.531065583499)) ;
#64416=CARTESIAN_POINT('Ctrl Pts',(-19.1585310682997,-50.3791059191269,
124.908576997203)) ;
#64417=CARTESIAN_POINT('Ctrl Pts',(-19.2087060042156,-50.199116838764,124.609228123008)) ;
#64418=CARTESIAN_POINT('Ctrl Pts',(-19.5088595130066,-50.3924408456182,
124.916046147867)) ;
#64419=CARTESIAN_POINT('Ctrl Pts',(-19.4889209379206,-50.2124517652553,
124.615199985815)) ;
#64420=CARTESIAN_POINT('Ctrl Pts',(-19.7681867122454,-50.4024239462128,
124.876091752188)) ;
#64421=CARTESIAN_POINT('Ctrl Pts',(-19.696392649381,-50.2224348658499,124.583239677521)) ;
#64422=CARTESIAN_POINT('Ctrl Pts',(-20.0179829922131,-50.4124687221124,
124.790847910221)) ;
#64423=CARTESIAN_POINT('Ctrl Pts',(-19.896227454566,-50.2324796417495,124.515046638421)) ;
#64424=CARTESIAN_POINT('Ctrl Pts',(-20.2442444733831,-50.4222866452983,
124.666833014598)) ;
#64425=CARTESIAN_POINT('Ctrl Pts',(-20.0772393601815,-50.2422975649354,
124.415835165722)) ;
#64426=CARTESIAN_POINT('Ctrl Pts',(-20.4505999318951,-50.4323359592536,
124.502045800867)) ;
#64427=CARTESIAN_POINT('Ctrl Pts',(-20.2423227107125,-50.2523468788908,
124.284011299718)) ;
#64428=CARTESIAN_POINT('Ctrl Pts',(-20.6812147142531,-50.4456396998762,
124.239319481561)) ;
#64429=CARTESIAN_POINT('Ctrl Pts',(-20.4268261522775,-50.2656506195133,
124.073810794489)) ;
#64430=CARTESIAN_POINT('Ctrl Pts',(-20.8766371020504,-50.4621298953529,
123.846918741757)) ;
#64431=CARTESIAN_POINT('Ctrl Pts',(-20.5831565547659,-50.28214081499,123.759929216494)) ;
#64432=CARTESIAN_POINT('Ctrl Pts',(-20.9269267933237,-50.4788490602775,
123.405534034858)) ;
#64433=CARTESIAN_POINT('Ctrl Pts',(-20.6233943759952,-50.2988599799146,
123.406758446571)) ;
#64434=CARTESIAN_POINT('Ctrl Pts',(-20.8757804021482,-50.4920100539476,
123.063406602128)) ;
#64435=CARTESIAN_POINT('Ctrl Pts',(-20.5824794341171,-50.3120209735847,
123.13310677555)) ;
#64436=CARTESIAN_POINT('Ctrl Pts',(-20.7933286314175,-50.5020062760529,
122.814013822185)) ;
#64437=CARTESIAN_POINT('Ctrl Pts',(-20.5165192334636,-50.32201719569,122.933581356952)) ;
#64438=CARTESIAN_POINT('Ctrl Pts',(-20.66794702487,-50.5120301155866,122.58234791319)) ;
#64439=CARTESIAN_POINT('Ctrl Pts',(-20.4162173324879,-50.3320410352238,
122.748251908727)) ;
#64440=CARTESIAN_POINT('Ctrl Pts',(-20.4530703195707,-50.5252234375799,
122.310222407941)) ;
#64441=CARTESIAN_POINT('Ctrl Pts',(-20.2443087067898,-50.345234357217,122.530542413722)) ;
#64442=CARTESIAN_POINT('Ctrl Pts',(-20.0984605249334,-50.5418826093572,
122.04515035663)) ;
#64443=CARTESIAN_POINT('Ctrl Pts',(-19.9606321286751,-50.3618935289943,
122.318489942363)) ;
#64444=CARTESIAN_POINT('Ctrl Pts',(-19.5917715291836,-50.5617927848429,
121.89245685484)) ;
#64445=CARTESIAN_POINT('Ctrl Pts',(-19.5552782569538,-50.38180370448,122.196329454903)) ;
#64446=CARTESIAN_POINT('Ctrl Pts',(-19.0638261203489,-50.5816827726873,
121.920703930916)) ;
#64447=CARTESIAN_POINT('Ctrl Pts',(-19.132921841017,-50.4016936923244,122.218924915738)) ;
#64448=CARTESIAN_POINT('Ctrl Pts',(-18.5747132438789,-50.6016882207021,
122.12899945876)) ;
#64449=CARTESIAN_POINT('Ctrl Pts',(-18.7416302351988,-50.4216991403392,
122.385558456999)) ;
#64450=CARTESIAN_POINT('Ctrl Pts',(-18.1887817456848,-50.6215246147294,
122.488396023025)) ;
#64451=CARTESIAN_POINT('Ctrl Pts',(-18.4328823682395,-50.4415355343665,
122.673074725378)) ;
#64452=CARTESIAN_POINT('Ctrl Pts',(-17.9465286197536,-50.6415324086261,
122.961624501261)) ;
#64453=CARTESIAN_POINT('Ctrl Pts',(-18.2390777138567,-50.4615433282632,
123.051656336489)) ;
#64454=CARTESIAN_POINT('Ctrl Pts',(-17.880692353325,-50.66135904492,123.484550765059)) ;
#64455=CARTESIAN_POINT('Ctrl Pts',(-18.1864063185633,-50.4813699645572,
123.469998611925)) ;
#64456=CARTESIAN_POINT('Ctrl Pts',(-17.9971845806245,-50.6813379878739,
124.002602226816)) ;
#64457=CARTESIAN_POINT('Ctrl Pts',(-18.2795984569262,-50.501348907511,123.884440399758)) ;
#64458=CARTESIAN_POINT('Ctrl Pts',(-18.2835587250181,-50.701269789743,124.448196582327)) ;
#64459=CARTESIAN_POINT('Ctrl Pts',(-18.5086966003631,-50.5212807093801,
124.240917422711)) ;
#64460=CARTESIAN_POINT('Ctrl Pts',(-18.7016353948024,-50.7210940902405,
124.769140330186)) ;
#64461=CARTESIAN_POINT('Ctrl Pts',(-18.843158485295,-50.5411050098776,124.497674650865)) ;
#64462=CARTESIAN_POINT('Ctrl Pts',(-19.2109425558882,-50.7411900915803,
124.929317666213)) ;
#64463=CARTESIAN_POINT('Ctrl Pts',(-19.2506040110265,-50.5612010112175,
124.625816398005)) ;
#64464=CARTESIAN_POINT('Ctrl Pts',(-19.7359254653028,-50.7609485076843,
124.90700825648)) ;
#64465=CARTESIAN_POINT('Ctrl Pts',(-19.6705889099247,-50.5809594273214,
124.607973339329)) ;
#64466=CARTESIAN_POINT('Ctrl Pts',(-20.2295077365795,-50.7810422005684,
124.703903011743)) ;
#64467=CARTESIAN_POINT('Ctrl Pts',(-20.0654722041603,-50.6010531202055,
124.445475287471)) ;
#64468=CARTESIAN_POINT('Ctrl Pts',(-20.4872438678407,-50.7941531664751,
124.469055541275)) ;
#64469=CARTESIAN_POINT('Ctrl Pts',(-20.2716279488377,-50.6141640861122,
124.257625239002)) ;
#64470=CARTESIAN_POINT('Ctrl Pts',(-20.5950497967257,-50.8008665412629,
124.330315451401)) ;
#64471=CARTESIAN_POINT('Ctrl Pts',(-20.357892637621,-50.6208774609001,124.146615798218)) ;
#64472=CARTESIAN_POINT('',(-18.1577260363418,-12.,123.523171848835)) ;
#64473=CARTESIAN_POINT('Ctrl Pts',(-17.9274924084134,-12.1498929727495,
123.644402320537)) ;
#64474=CARTESIAN_POINT('Ctrl Pts',(-17.9447322736189,-12.1380608032114,
123.631287153522)) ;
#64475=CARTESIAN_POINT('Ctrl Pts',(-17.9630111136594,-12.1257315979358,
123.61865820345)) ;
#64476=CARTESIAN_POINT('Ctrl Pts',(-17.9820336742706,-12.1130842288466,
123.606705870659)) ;
#64477=CARTESIAN_POINT('Ctrl Pts',(-18.0012480997282,-12.1003092961987,
123.594632984565)) ;
#64478=CARTESIAN_POINT('Ctrl Pts',(-18.0212209537106,-12.0872097491302,
123.583250489011)) ;
#64479=CARTESIAN_POINT('Ctrl Pts',(-18.0416342610097,-12.073969917745,123.572702334622)) ;
#64480=CARTESIAN_POINT('Ctrl Pts',(-18.0628845294966,-12.0601872431625,
123.561721697849)) ;
#64481=CARTESIAN_POINT('Ctrl Pts',(-18.0846116965369,-12.046252544725,123.551645261562)) ;
#64482=CARTESIAN_POINT('Ctrl Pts',(-18.1064482931762,-12.0323737605024,
123.542577794954)) ;
#64483=CARTESIAN_POINT('Ctrl Pts',(-18.1235331135845,-12.0215150841324,
123.535483464225)) ;
#64484=CARTESIAN_POINT('Ctrl Pts',(-18.1406846749009,-12.0106906348965,
123.52900545476)) ;
#64485=CARTESIAN_POINT('Ctrl Pts',(-18.1577260360659,-11.9999999999988,
123.52317184888)) ;
#64486=CARTESIAN_POINT('Ctrl Pts',(-18.1577260360659,-11.9999999999988,
123.52317184888)) ;
#64487=CARTESIAN_POINT('Ctrl Pts',(-18.1523700395754,-11.9999999999989,
123.490912584228)) ;
#64488=CARTESIAN_POINT('Ctrl Pts',(-18.1482641940248,-12.,123.458366720246)) ;
#64489=CARTESIAN_POINT('Ctrl Pts',(-18.1454318173621,-12.,123.425634822543)) ;
#64490=CARTESIAN_POINT('Ctrl Pts',(-18.1391124983055,-12.,123.352606645309)) ;
#64491=CARTESIAN_POINT('Ctrl Pts',(-18.139130762036,-12.,123.278629626742)) ;
#64492=CARTESIAN_POINT('Ctrl Pts',(-18.1456716811646,-12.,123.204576506712)) ;
#64493=CARTESIAN_POINT('Ctrl Pts',(-18.1517101445967,-12.,123.136211946846)) ;
#64494=CARTESIAN_POINT('Ctrl Pts',(-18.1633098563508,-11.9999999994,123.067757580192)) ;
#64495=CARTESIAN_POINT('Ctrl Pts',(-18.180582178177,-11.9999999999304,123.000096158631)) ;
#64496=CARTESIAN_POINT('Ctrl Pts',(-18.1819709423,-11.9999999999731,122.994655908286)) ;
#64497=CARTESIAN_POINT('Ctrl Pts',(-18.1833963771835,-12.,122.989220812084)) ;
#64498=CARTESIAN_POINT('Ctrl Pts',(-18.1848585399242,-12.,122.983791343577)) ;
#64499=CARTESIAN_POINT('Ctrl Pts',(-18.2003846048102,-12.,122.926138198693)) ;
#64500=CARTESIAN_POINT('Ctrl Pts',(-18.2200467363594,-12.0000000052168,
122.869141588207)) ;
#64501=CARTESIAN_POINT('Ctrl Pts',(-18.2435971844896,-12.0000000018168,
122.813603051952)) ;
#64502=CARTESIAN_POINT('Ctrl Pts',(-18.2497774297557,-12.0000000009246,
122.799028306967)) ;
#64503=CARTESIAN_POINT('Ctrl Pts',(-18.2562253303416,-12.,122.784554225748)) ;
#64504=CARTESIAN_POINT('Ctrl Pts',(-18.2629361382999,-12.,122.770195825027)) ;
#64505=CARTESIAN_POINT('Ctrl Pts',(-18.2951446697432,-12.,122.701282662267)) ;
#64506=CARTESIAN_POINT('Ctrl Pts',(-18.3334226087301,-12.,122.635003694009)) ;
#64507=CARTESIAN_POINT('Ctrl Pts',(-18.3779347229611,-12.,122.57166047214)) ;
#64508=CARTESIAN_POINT('Ctrl Pts',(-18.4098344464478,-12.,122.526265385942)) ;
#64509=CARTESIAN_POINT('Ctrl Pts',(-18.4449399291145,-12.0000000149114,
122.482373487453)) ;
#64510=CARTESIAN_POINT('Ctrl Pts',(-18.482822642223,-12.0000000073334,122.440677242729)) ;
#64511=CARTESIAN_POINT('Ctrl Pts',(-18.4976553716752,-12.0000000043663,
122.424351349823)) ;
#64512=CARTESIAN_POINT('Ctrl Pts',(-18.5129135125104,-12.,122.408362500768)) ;
#64513=CARTESIAN_POINT('Ctrl Pts',(-18.5285699207533,-12.,122.392753917874)) ;
#64514=CARTESIAN_POINT('Ctrl Pts',(-18.5841047825192,-12.,122.337388697449)) ;
#64515=CARTESIAN_POINT('Ctrl Pts',(-18.6446065470671,-12.,122.28685455902)) ;
#64516=CARTESIAN_POINT('Ctrl Pts',(-18.7093690801587,-12.,122.241689425851)) ;
#64517=CARTESIAN_POINT('Ctrl Pts',(-18.7739954385736,-12.,122.19661926036)) ;
#64518=CARTESIAN_POINT('Ctrl Pts',(-18.8429277799953,-12.,122.156848889559)) ;
#64519=CARTESIAN_POINT('Ctrl Pts',(-18.9158209517903,-12.,122.123023408323)) ;
#64520=CARTESIAN_POINT('Ctrl Pts',(-18.97041252654,-12.,122.097690633773)) ;
#64521=CARTESIAN_POINT('Ctrl Pts',(-19.0272216439489,-12.0000000102563,
122.07569526255)) ;
#64522=CARTESIAN_POINT('Ctrl Pts',(-19.0855066103726,-12.0000000043775,
122.057451417983)) ;
#64523=CARTESIAN_POINT('Ctrl Pts',(-19.1048218044881,-12.0000000024293,
122.051405546794)) ;
#64524=CARTESIAN_POINT('Ctrl Pts',(-19.1242986823222,-12.,122.045771825291)) ;
#64525=CARTESIAN_POINT('Ctrl Pts',(-19.1439090623038,-12.,122.040565761127)) ;
#64526=CARTESIAN_POINT('Ctrl Pts',(-19.2140201463212,-12.,122.02195302632)) ;
#64527=CARTESIAN_POINT('Ctrl Pts',(-19.2857743787866,-12.0000000003845,
122.008825196783)) ;
#64528=CARTESIAN_POINT('Ctrl Pts',(-19.3581616094974,-12.0000000000663,
122.001266834043)) ;
#64529=CARTESIAN_POINT('Ctrl Pts',(-19.3669843878261,-12.0000000000275,
122.000345597544)) ;
#64530=CARTESIAN_POINT('Ctrl Pts',(-19.3758165065751,-12.,121.999507090169)) ;
#64531=CARTESIAN_POINT('Ctrl Pts',(-19.3846560842804,-12.,121.998751458056)) ;
#64532=CARTESIAN_POINT('Ctrl Pts',(-19.4614572885066,-12.,121.99218627382)) ;
#64533=CARTESIAN_POINT('Ctrl Pts',(-19.538903862666,-11.9999999928402,121.991868832861)) ;
#64534=CARTESIAN_POINT('Ctrl Pts',(-19.6170404757029,-11.9999999993994,
121.998118870204)) ;
#64535=CARTESIAN_POINT('Ctrl Pts',(-19.6215372909564,-11.9999999997768,
121.998478564106)) ;
#64536=CARTESIAN_POINT('Ctrl Pts',(-19.6260364054519,-12.,121.998860014342)) ;
#64537=CARTESIAN_POINT('Ctrl Pts',(-19.630537832746,-12.,121.999263283676)) ;
#64538=CARTESIAN_POINT('Ctrl Pts',(-19.6881089405452,-12.,122.004420906088)) ;
#64539=CARTESIAN_POINT('Ctrl Pts',(-19.7460667548092,-12.0000000189751,
122.013148289636)) ;
#64540=CARTESIAN_POINT('Ctrl Pts',(-19.8035599226054,-12.0000000101354,
122.02543377879)) ;
#64541=CARTESIAN_POINT('Ctrl Pts',(-19.8284255246479,-12.0000000063122,
122.030747211601)) ;
#64542=CARTESIAN_POINT('Ctrl Pts',(-19.8532035599087,-12.,122.036726116961)) ;
#64543=CARTESIAN_POINT('Ctrl Pts',(-19.8778221613683,-12.,122.043369085461)) ;
#64544=CARTESIAN_POINT('Ctrl Pts',(-19.9591906752725,-12.,122.065325185429)) ;
#64545=CARTESIAN_POINT('Ctrl Pts',(-20.0387357146672,-12.,122.094515610606)) ;
#64546=CARTESIAN_POINT('Ctrl Pts',(-20.1155608588238,-12.,122.13054538147)) ;
#64547=CARTESIAN_POINT('Ctrl Pts',(-20.1922295232036,-12.,122.166501765807)) ;
#64548=CARTESIAN_POINT('Ctrl Pts',(-20.2662621433006,-12.,122.209300999016)) ;
#64549=CARTESIAN_POINT('Ctrl Pts',(-20.3368145274386,-12.,122.259002783194)) ;
#64550=CARTESIAN_POINT('Ctrl Pts',(-20.3861836086094,-12.,122.293781642156)) ;
#64551=CARTESIAN_POINT('Ctrl Pts',(-20.4338172518609,-12.0000000080963,
122.331920190157)) ;
#64552=CARTESIAN_POINT('Ctrl Pts',(-20.4789726009455,-12.0000000042853,
122.372781155038)) ;
#64553=CARTESIAN_POINT('Ctrl Pts',(-20.49821889138,-12.0000000026609,122.390197076152)) ;
#64554=CARTESIAN_POINT('Ctrl Pts',(-20.5170145004755,-12.,122.408107114264)) ;
#64555=CARTESIAN_POINT('Ctrl Pts',(-20.5352999373477,-12.,122.426459820579)) ;
#64556=CARTESIAN_POINT('Ctrl Pts',(-20.548691568813,-12.,122.439900717894)) ;
#64557=CARTESIAN_POINT('Ctrl Pts',(-20.5618056963188,-12.,122.453575160092)) ;
#64558=CARTESIAN_POINT('Ctrl Pts',(-20.5746457983858,-12.,122.467488525849)) ;
#64559=CARTESIAN_POINT('Origin',(-20.3808735729049,-12.,126.250122109236)) ;
#64560=CARTESIAN_POINT('',(-20.8451118552234,-12.,123.237406292887)) ;
#64561=CARTESIAN_POINT('Origin',(-20.3808735729049,-12.,126.250122109236)) ;
#64562=CARTESIAN_POINT('',(-18.1577260363418,-12.,123.523171848835)) ;
#64563=CARTESIAN_POINT('',(-20.4601832664426,-12.,122.734993854115)) ;
#64564=CARTESIAN_POINT('Ctrl Pts',(-20.8283303706881,10.,122.926041870813)) ;
#64565=CARTESIAN_POINT('Ctrl Pts',(-20.5445170967909,9.82001091963712,123.023196933748)) ;
#64566=CARTESIAN_POINT('Ctrl Pts',(-20.8845408159969,10.0066268508181,123.090165629856)) ;
#64567=CARTESIAN_POINT('Ctrl Pts',(-20.5894888524673,9.82663777045524,123.154521539138)) ;
#64568=CARTESIAN_POINT('Ctrl Pts',(-20.9394617690737,10.0198574772991,123.437507823531)) ;
#64569=CARTESIAN_POINT('Ctrl Pts',(-20.633420846741,9.83986839693625,123.432353293108)) ;
#64570=CARTESIAN_POINT('Ctrl Pts',(-20.8387858493119,10.0398330985578,123.958797508285)) ;
#64571=CARTESIAN_POINT('Ctrl Pts',(-20.5528814274113,9.85984401819488,123.849407562291)) ;
#64572=CARTESIAN_POINT('Ctrl Pts',(-20.5666727975867,10.0597504334597,124.412849839357)) ;
#64573=CARTESIAN_POINT('Ctrl Pts',(-20.3351890331055,9.87976135309682,124.212644574099)) ;
#64574=CARTESIAN_POINT('Ctrl Pts',(-20.157556275784,10.0796237101757,124.747029739186)) ;
#64575=CARTESIAN_POINT('Ctrl Pts',(-20.007894029438,9.89963462981282,124.479989709356)) ;
#64576=CARTESIAN_POINT('Ctrl Pts',(-19.6551315118144,10.0996482003397,124.922482691163)) ;
#64577=CARTESIAN_POINT('Ctrl Pts',(-19.6059539581694,9.91965911997678,124.6203502007)) ;
#64578=CARTESIAN_POINT('Ctrl Pts',(-19.1270395366036,10.1195160414904,124.915890798164)) ;
#64579=CARTESIAN_POINT('Ctrl Pts',(-19.183479078867,9.9395269611275,124.615075206311)) ;
#64580=CARTESIAN_POINT('Ctrl Pts',(-18.6307952228403,10.1394616923699,124.72957580943)) ;
#64581=CARTESIAN_POINT('Ctrl Pts',(-18.7864838467008,9.95947261200706,124.466021078065)) ;
#64582=CARTESIAN_POINT('Ctrl Pts',(-18.2288224078826,10.1593670929869,124.385607616877)) ;
#64583=CARTESIAN_POINT('Ctrl Pts',(-18.4649063275282,9.97937801262402,124.19084435197)) ;
#64584=CARTESIAN_POINT('Ctrl Pts',(-17.9678535157127,10.1792413208033,123.926349000794)) ;
#64585=CARTESIAN_POINT('Ctrl Pts',(-18.2561329793354,9.99925224044038,123.823435269459)) ;
#64586=CARTESIAN_POINT('Ctrl Pts',(-17.878734209588,10.1992271116809,123.402675114316)) ;
#64587=CARTESIAN_POINT('Ctrl Pts',(-18.1848402358937,10.019238031318,123.404495614569)) ;
#64588=CARTESIAN_POINT('Ctrl Pts',(-17.973517700436,10.2191213543406,122.882519965019)) ;
#64589=CARTESIAN_POINT('Ctrl Pts',(-18.2606699231879,10.0391322739778,122.988371207676)) ;
#64590=CARTESIAN_POINT('Ctrl Pts',(-18.2387528910803,10.2390000704127,122.425502981447)) ;
#64591=CARTESIAN_POINT('Ctrl Pts',(-18.4728612986517,10.0590109900498,122.62275860733)) ;
#64592=CARTESIAN_POINT('Ctrl Pts',(-18.647614090005,10.2590395202573,122.084258749108)) ;
#64593=CARTESIAN_POINT('Ctrl Pts',(-18.7999520972875,10.0790504398944,122.349765888777)) ;
#64594=CARTESIAN_POINT('Ctrl Pts',(-19.1441721121047,10.2789026817952,121.90452088182)) ;
#64595=CARTESIAN_POINT('Ctrl Pts',(-19.1972003931787,10.0989136014323,122.205978444044)) ;
#64596=CARTESIAN_POINT('Ctrl Pts',(-19.6750232066901,10.2988820498094,121.904721686728)) ;
#64597=CARTESIAN_POINT('Ctrl Pts',(-19.6218814079036,10.1188929694465,122.206142590273)) ;
#64598=CARTESIAN_POINT('Ctrl Pts',(-20.1701799765179,10.3186926303322,122.084083785786)) ;
#64599=CARTESIAN_POINT('Ctrl Pts',(-20.0180064135448,10.1387035499693,122.349636107043)) ;
#64600=CARTESIAN_POINT('Ctrl Pts',(-20.578226084171,10.3386735586178,122.423812224567)) ;
#64601=CARTESIAN_POINT('Ctrl Pts',(-20.3444408940403,10.1586844782549,122.621421767106)) ;
#64602=CARTESIAN_POINT('Ctrl Pts',(-20.8444469588477,10.3585662304872,122.880680954098)) ;
#64603=CARTESIAN_POINT('Ctrl Pts',(-20.5574140513056,10.1785771501243,122.986919611144)) ;
#64604=CARTESIAN_POINT('Ctrl Pts',(-20.9398341757817,10.3784925607743,123.40162915944)) ;
#64605=CARTESIAN_POINT('Ctrl Pts',(-20.6337210673662,10.1985034804115,123.403677177554)) ;
#64606=CARTESIAN_POINT('Ctrl Pts',(-20.8510572230715,10.3984631148666,123.924927290891)) ;
#64607=CARTESIAN_POINT('Ctrl Pts',(-20.5626906127405,10.2184740345037,123.822322291595)) ;
#64608=CARTESIAN_POINT('Ctrl Pts',(-20.6345446351863,10.4149949539542,124.307272603886)) ;
#64609=CARTESIAN_POINT('Ctrl Pts',(-20.3894922234183,10.2350058735914,124.128174543065)) ;
#64610=CARTESIAN_POINT('Ctrl Pts',(-20.3891097552813,10.4283346927818,124.557601822174)) ;
#64611=CARTESIAN_POINT('Ctrl Pts',(-20.1931290434829,10.2483456124189,124.328455837242)) ;
#64612=CARTESIAN_POINT('Ctrl Pts',(-20.1744300570267,10.4383669350004,124.710615084593)) ;
#64613=CARTESIAN_POINT('Ctrl Pts',(-20.0213869924123,10.2583778546375,124.450860682641)) ;
#64614=CARTESIAN_POINT('Ctrl Pts',(-19.9407404802418,10.4482246356439,124.822421617883)) ;
#64615=CARTESIAN_POINT('Ctrl Pts',(-19.8344327400403,10.268235555281,124.540305070127)) ;
#64616=CARTESIAN_POINT('Ctrl Pts',(-19.6879423525307,10.4582165002831,124.893352629427)) ;
#64617=CARTESIAN_POINT('Ctrl Pts',(-19.6321963403517,10.2782274199202,124.597047919264)) ;
#64618=CARTESIAN_POINT('Ctrl Pts',(-19.4284710425139,10.4681390500432,124.919080315321)) ;
#64619=CARTESIAN_POINT('Ctrl Pts',(-19.4246096943487,10.2881499696804,124.61762631767)) ;
#64620=CARTESIAN_POINT('Ctrl Pts',(-19.0804105140851,10.4814168235367,124.893583985624)) ;
#64621=CARTESIAN_POINT('Ctrl Pts',(-19.14620736525,10.3014277431738,124.597234554234)) ;
#64622=CARTESIAN_POINT('Ctrl Pts',(-18.7455859092888,10.4947641624773,124.776616835755)) ;
#64623=CARTESIAN_POINT('Ctrl Pts',(-18.8783191462352,10.3147750821144,124.503658407746)) ;
#64624=CARTESIAN_POINT('Ctrl Pts',(-18.4584522382473,10.5079713942705,124.581549246914)) ;
#64625=CARTESIAN_POINT('Ctrl Pts',(-18.648603078249,10.3279823139076,124.347593121025)) ;
#64626=CARTESIAN_POINT('Ctrl Pts',(-18.269958838059,10.5179585103602,124.398989341533)) ;
#64627=CARTESIAN_POINT('Ctrl Pts',(-18.497812104421,10.3379694299973,124.201545371492)) ;
#64628=CARTESIAN_POINT('Ctrl Pts',(-18.1163933969716,10.52790941594,124.187269395838)) ;
#64629=CARTESIAN_POINT('Ctrl Pts',(-18.3749610183035,10.3479203355771,124.032167599002)) ;
#64630=CARTESIAN_POINT('Ctrl Pts',(-18.0010345813923,10.5379645179474,123.949583784548)) ;
#64631=CARTESIAN_POINT('Ctrl Pts',(-18.2826761214566,10.3579754375845,123.842018479487)) ;
#64632=CARTESIAN_POINT('Ctrl Pts',(-17.9299233421522,10.5477861912685,123.701439503961)) ;
#64633=CARTESIAN_POINT('Ctrl Pts',(-18.2257894437957,10.3677971109056,123.643501792389)) ;
#64634=CARTESIAN_POINT('Ctrl Pts',(-17.9019040586336,10.5578446623434,123.43862866708)) ;
#64635=CARTESIAN_POINT('Ctrl Pts',(-18.2033755364028,10.3778555819805,123.43325511011)) ;
#64636=CARTESIAN_POINT('Ctrl Pts',(-17.9200547531203,10.5677692735199,123.178437417212)) ;
#64637=CARTESIAN_POINT('Ctrl Pts',(-18.2179011304931,10.387780193157,123.22509433493)) ;
#64638=CARTESIAN_POINT('Ctrl Pts',(-18.0035329037317,10.5810466124203,122.839624585047)) ;
#64639=CARTESIAN_POINT('Ctrl Pts',(-18.2846726619434,10.4010575320574,122.954084471608)) ;
#64640=CARTESIAN_POINT('Ctrl Pts',(-18.174078890485,10.5943454916579,122.53009645584)) ;
#64641=CARTESIAN_POINT('Ctrl Pts',(-18.4211116702471,10.414356411295,122.706442742821)) ;
#64642=CARTESIAN_POINT('Ctrl Pts',(-18.4148290889509,10.6075843638286,122.278909287836)) ;
#64643=CARTESIAN_POINT('Ctrl Pts',(-18.61372828438,10.4275952834657,122.505480269817)) ;
#64644=CARTESIAN_POINT('Ctrl Pts',(-18.6267237904145,10.6175909819652,122.123170592624)) ;
#64645=CARTESIAN_POINT('Ctrl Pts',(-18.7832424340302,10.4376019016023,122.380894154854)) ;
#64646=CARTESIAN_POINT('Ctrl Pts',(-18.8632279358434,10.6276219270267,122.006771081612)) ;
#64647=CARTESIAN_POINT('Ctrl Pts',(-18.9724474943499,10.4476328466638,122.287775782223)) ;
#64648=CARTESIAN_POINT('Ctrl Pts',(-19.1118308518252,10.6374781003785,121.93402103227)) ;
#64649=CARTESIAN_POINT('Ctrl Pts',(-19.1713300681509,10.4574890200157,122.229578162461)) ;
#64650=CARTESIAN_POINT('Ctrl Pts',(-19.3729271808616,10.6474773713414,121.904805274484)) ;
#64651=CARTESIAN_POINT('Ctrl Pts',(-19.3802073636504,10.4674882909785,122.206207726809)) ;
#64652=CARTESIAN_POINT('Ctrl Pts',(-19.63249343999,10.6573718230987,121.920897070182)) ;
#64653=CARTESIAN_POINT('Ctrl Pts',(-19.5878600087485,10.4773827427359,122.219083373213)) ;
#64654=CARTESIAN_POINT('Ctrl Pts',(-19.8895240952696,10.6674351389081,121.982913347126)) ;
#64655=CARTESIAN_POINT('Ctrl Pts',(-19.7934840442871,10.4874460585452,122.268698557826)) ;
#64656=CARTESIAN_POINT('Ctrl Pts',(-20.1266813029374,10.6772739956477,122.086019825898)) ;
#64657=CARTESIAN_POINT('Ctrl Pts',(-19.9832086272329,10.4972849152848,122.351185625972)) ;
#64658=CARTESIAN_POINT('Ctrl Pts',(-20.3474018172676,10.6873401174653,122.231740902041)) ;
#64659=CARTESIAN_POINT('Ctrl Pts',(-20.1597838722231,10.5073510371024,122.46776433411)) ;
#64660=CARTESIAN_POINT('Ctrl Pts',(-20.5359503275351,10.6972233451896,122.410409425907)) ;
#64661=CARTESIAN_POINT('Ctrl Pts',(-20.3106209609387,10.5172342648267,122.6107005406)) ;
#64662=CARTESIAN_POINT('Ctrl Pts',(-20.6926994160287,10.7072128064683,122.620953380555)) ;
#64663=CARTESIAN_POINT('Ctrl Pts',(-20.4360184466383,10.5272237261055,122.779136903454)) ;
#64664=CARTESIAN_POINT('Ctrl Pts',(-20.8101391925705,10.7171765168948,122.854988704109)) ;
#64665=CARTESIAN_POINT('Ctrl Pts',(-20.5299682760089,10.5371874365319,122.966365995585)) ;
#64666=CARTESIAN_POINT('Ctrl Pts',(-20.8856615342042,10.7271715196257,123.106575647569)) ;
#64667=CARTESIAN_POINT('Ctrl Pts',(-20.5903840854433,10.5471824392628,123.167636082224)) ;
#64668=CARTESIAN_POINT('Ctrl Pts',(-20.9160649147156,10.737207850636,123.368548316933)) ;
#64669=CARTESIAN_POINT('Ctrl Pts',(-20.6147046374483,10.5572187702731,123.377214485628)) ;
#64670=CARTESIAN_POINT('Ctrl Pts',(-20.901237668564,10.7470540799783,123.626888226543)) ;
#64671=CARTESIAN_POINT('Ctrl Pts',(-20.6028407406531,10.5670649996154,123.583885836904)) ;
#64672=CARTESIAN_POINT('Ctrl Pts',(-20.8414280631531,10.7570395782535,123.88234711985)) ;
#64673=CARTESIAN_POINT('Ctrl Pts',(-20.5549910573095,10.5770504978907,123.788252351213)) ;
#64674=CARTESIAN_POINT('Ctrl Pts',(-20.7388329136923,10.7669744812365,124.122475498249)) ;
#64675=CARTESIAN_POINT('Ctrl Pts',(-20.4729131488679,10.5869854008736,123.98035400456)) ;
#64676=CARTESIAN_POINT('Ctrl Pts',(-20.5941893977946,10.7770319843317,124.343638489499)) ;
#64677=CARTESIAN_POINT('Ctrl Pts',(-20.3571965368945,10.5970429039689,124.157283333151)) ;
#64678=CARTESIAN_POINT('Ctrl Pts',(-20.4178270374552,10.7868536407023,124.532127444505)) ;
#64679=CARTESIAN_POINT('Ctrl Pts',(-20.216105589301,10.6068645603394,124.308072644051)) ;
#64680=CARTESIAN_POINT('Ctrl Pts',(-20.2068264505713,10.7969097033674,124.691194003415)) ;
#64681=CARTESIAN_POINT('Ctrl Pts',(-20.0473038554878,10.6169206230045,124.435324362058)) ;
#64682=CARTESIAN_POINT('Ctrl Pts',(-19.9738709151238,10.8068503680706,124.809425923824)) ;
#64683=CARTESIAN_POINT('Ctrl Pts',(-19.8609387422743,10.6268612877077,124.529907956941)) ;
#64684=CARTESIAN_POINT('Ctrl Pts',(-19.7250819168071,10.8167547720191,124.885913848072)) ;
#64685=CARTESIAN_POINT('Ctrl Pts',(-19.6619073830525,10.6367656916563,124.591096321636)) ;
#64686=CARTESIAN_POINT('Ctrl Pts',(-19.4630900672441,10.8268012570127,124.918337587752)) ;
#64687=CARTESIAN_POINT('Ctrl Pts',(-19.4523135810077,10.6468121766498,124.617033381453)) ;
#64688=CARTESIAN_POINT('Ctrl Pts',(-19.2033217042056,10.8366974848244,124.905200421478)) ;
#64689=CARTESIAN_POINT('Ctrl Pts',(-19.2444994521855,10.6567084044615,124.606521750019)) ;
#64690=CARTESIAN_POINT('Ctrl Pts',(-18.9456501548748,10.8467570683879,124.846258925075)) ;
#64691=CARTESIAN_POINT('Ctrl Pts',(-19.0383625055845,10.666767988025,124.559366649145)) ;
#64692=CARTESIAN_POINT('Ctrl Pts',(-18.7071032762899,10.8566090780567,124.745604613553)) ;
#64693=CARTESIAN_POINT('Ctrl Pts',(-18.8475263594419,10.6766199976938,124.478841692918)) ;
#64694=CARTESIAN_POINT('Ctrl Pts',(-18.4867618466311,10.8665716094963,124.604236201826)) ;
#64695=CARTESIAN_POINT('Ctrl Pts',(-18.6712543942556,10.6865825291334,124.36574560245)) ;
#64696=CARTESIAN_POINT('Ctrl Pts',(-18.2932415519936,10.8766031577357,124.425213596724)) ;
#64697=CARTESIAN_POINT('Ctrl Pts',(-18.5164393722649,10.6966140773728,124.222526126703)) ;
#64698=CARTESIAN_POINT('Ctrl Pts',(-18.1357799386366,10.8864945689487,124.218398117847)) ;
#64699=CARTESIAN_POINT('Ctrl Pts',(-18.3904718496513,10.7065054885858,124.057073085295)) ;
#64700=CARTESIAN_POINT('Ctrl Pts',(-18.0146891209222,10.8965108226567,123.984678099418)) ;
#64701=CARTESIAN_POINT('Ctrl Pts',(-18.2936007418435,10.7165217422938,123.870096295635)) ;
#64702=CARTESIAN_POINT('Ctrl Pts',(-17.9364599064937,10.9065409255014,123.732978598351)) ;
#64703=CARTESIAN_POINT('Ctrl Pts',(-18.2310191023128,10.7265518451385,123.66873611636)) ;
#64704=CARTESIAN_POINT('Ctrl Pts',(-17.9032046926023,10.9163973744551,123.476088297528)) ;
#64705=CARTESIAN_POINT('Ctrl Pts',(-18.2044167490604,10.7364082940922,123.463224374815)) ;
#64706=CARTESIAN_POINT('Ctrl Pts',(-17.9148974747618,10.9263963852274,123.213627004979)) ;
#64707=CARTESIAN_POINT('Ctrl Pts',(-18.2137726540653,10.7464073048645,123.253255524932)) ;
#64708=CARTESIAN_POINT('Ctrl Pts',(-17.9711291549323,10.9362916021454,122.959700121601)) ;
#64709=CARTESIAN_POINT('Ctrl Pts',(-18.2587594621295,10.7563025217825,123.050114944414)) ;
#64710=CARTESIAN_POINT('Ctrl Pts',(-18.0722565351528,10.9463521175027,122.715462501341)) ;
#64711=CARTESIAN_POINT('Ctrl Pts',(-18.3396629540108,10.7663630371399,122.854725296797)) ;
#64712=CARTESIAN_POINT('Ctrl Pts',(-18.2111793287984,10.9562014108898,122.497051143162)) ;
#64713=CARTESIAN_POINT('Ctrl Pts',(-18.4508020993981,10.7762123305269,122.679997778405)) ;
#64714=CARTESIAN_POINT('Ctrl Pts',(-18.388559678523,10.9662285865698,122.302199917963)) ;
#64715=CARTESIAN_POINT('Ctrl Pts',(-18.5927074978848,10.7862395062069,122.524117774987)) ;
#64716=CARTESIAN_POINT('Ctrl Pts',(-18.5975457775489,10.976257162197,122.141622604304)) ;
#64717=CARTESIAN_POINT('Ctrl Pts',(-18.7598974069773,10.7962680818341,122.395657172665)) ;
#64718=CARTESIAN_POINT('Ctrl Pts',(-18.8267122580128,10.9861022557429,122.021573575598)) ;
#64719=CARTESIAN_POINT('Ctrl Pts',(-18.9432305035226,10.80611317538,122.299619713947)) ;
#64720=CARTESIAN_POINT('Ctrl Pts',(-19.0767061726053,10.9960934971746,121.941311591283)) ;
#64721=CARTESIAN_POINT('Ctrl Pts',(-19.1432259108285,10.8161044168118,122.235411491827)) ;
#64722=CARTESIAN_POINT('Ctrl Pts',(-19.3380760888337,11.0061292783179,121.906059986019)) ;
#64723=CARTESIAN_POINT('Ctrl Pts',(-19.3523221423469,10.826140197955,122.20721167611)) ;
#64724=CARTESIAN_POINT('Ctrl Pts',(-19.5967752495355,11.0159814840476,121.916185579079)) ;
#64725=CARTESIAN_POINT('Ctrl Pts',(-19.5592805072898,10.8359924036847,122.215313538143)) ;
#64726=CARTESIAN_POINT('Ctrl Pts',(-19.8527735772293,11.0259435781646,121.970943280899)) ;
#64727=CARTESIAN_POINT('Ctrl Pts',(-19.7640785909624,10.8459544978017,122.259120868789)) ;
#64728=CARTESIAN_POINT('Ctrl Pts',(-20.0967309229679,11.0359661389917,122.070215768955)) ;
#64729=CARTESIAN_POINT('Ctrl Pts',(-19.9592439949302,10.8559770586288,122.338540107306)) ;
#64730=CARTESIAN_POINT('Ctrl Pts',(-20.3177943873502,11.0458939106433,122.208809071659)) ;
#64731=CARTESIAN_POINT('Ctrl Pts',(-20.1360936655196,10.8659048302804,122.449415566975)) ;
#64732=CARTESIAN_POINT('Ctrl Pts',(-20.513619210783,11.0559362947681,122.385690857822)) ;
#64733=CARTESIAN_POINT('Ctrl Pts',(-20.2927527608326,10.8759472144052,122.590922041084)) ;
#64734=CARTESIAN_POINT('Ctrl Pts',(-20.6733901753496,11.0658255188387,122.590674219405)) ;
#64735=CARTESIAN_POINT('Ctrl Pts',(-20.4205680784334,10.8858364384758,122.754908921902)) ;
#64736=CARTESIAN_POINT('Ctrl Pts',(-20.7967974985103,11.075814767006,122.822355021181)) ;
#64737=CARTESIAN_POINT('Ctrl Pts',(-20.5192928376293,10.8958256866432,122.940253955908)) ;
#64738=CARTESIAN_POINT('Ctrl Pts',(-20.8776639039544,11.085773344048,123.07124139589)) ;
#64739=CARTESIAN_POINT('Ctrl Pts',(-20.5839847120867,10.9057842636851,123.139363096927)) ;
#64740=CARTESIAN_POINT('Ctrl Pts',(-20.9145104547189,11.0956729131393,123.328785419539)) ;
#64741=CARTESIAN_POINT('Ctrl Pts',(-20.6134608083522,10.9156838327764,123.34539776855)) ;
#64742=CARTESIAN_POINT('Ctrl Pts',(-20.9058609614056,11.1057208252233,123.592665004876)) ;
#64743=CARTESIAN_POINT('Ctrl Pts',(-20.6065401309608,10.9257317448604,123.556501576119)) ;
#64744=CARTESIAN_POINT('Ctrl Pts',(-20.8525354819136,11.1156161795305,123.847220118537)) ;
#64745=CARTESIAN_POINT('Ctrl Pts',(-20.5638788889721,10.9356270991676,123.760144740549)) ;
#64746=CARTESIAN_POINT('Ctrl Pts',(-20.7542573598821,11.1256778300217,124.092654877015)) ;
#64747=CARTESIAN_POINT('Ctrl Pts',(-20.485255344439,10.9456887496588,123.95649240933)) ;
#64748=CARTESIAN_POINT('Ctrl Pts',(-20.6178768119318,11.1355224454842,124.31250491989)) ;
#64749=CARTESIAN_POINT('Ctrl Pts',(-20.3761506014328,10.9555333651213,124.132371010177)) ;
#64750=CARTESIAN_POINT('Ctrl Pts',(-20.4440816600714,11.1454825243856,124.508211665868)) ;
#64751=CARTESIAN_POINT('Ctrl Pts',(-20.2371141294296,10.9654934440227,124.288935606726)) ;
#64752=CARTESIAN_POINT('Ctrl Pts',(-20.2370227832588,11.1555207187439,124.671637321506)) ;
#64753=CARTESIAN_POINT('Ctrl Pts',(-20.0714663599296,10.9755316383811,124.419675493237)) ;
#64754=CARTESIAN_POINT('Ctrl Pts',(-20.0087297938616,11.1653944341435,124.795026404838)) ;
#64755=CARTESIAN_POINT('Ctrl Pts',(-19.8888323768802,10.9854053537807,124.518385630322)) ;
#64756=CARTESIAN_POINT('Ctrl Pts',(-19.7576006730884,11.1754661436778,124.87849507525)) ;
#64757=CARTESIAN_POINT('Ctrl Pts',(-19.6879285180809,10.9954770633149,124.585159904661)) ;
#64758=CARTESIAN_POINT('Ctrl Pts',(-19.5019775459593,11.1852985841303,124.916330182897)) ;
#64759=CARTESIAN_POINT('Ctrl Pts',(-19.4834310649531,11.0053095037674,124.61542705853)) ;
#64760=CARTESIAN_POINT('Ctrl Pts',(-19.2384391664689,11.1953304050557,124.909797495667)) ;
#64761=CARTESIAN_POINT('Ctrl Pts',(-19.2726002800821,11.0153413246928,124.610200312681)) ;
#64762=CARTESIAN_POINT('Ctrl Pts',(-18.9804733109709,11.2053507749413,124.856926970494)) ;
#64763=CARTESIAN_POINT('Ctrl Pts',(-19.0662277209886,11.0253616945784,124.567903126728)) ;
#64764=CARTESIAN_POINT('Ctrl Pts',(-18.7390964607104,11.215217546075,124.762178595596)) ;
#64765=CARTESIAN_POINT('Ctrl Pts',(-18.8731273657641,11.0352284657122,124.492104212861)) ;
#64766=CARTESIAN_POINT('Ctrl Pts',(-18.5133063352698,11.2252883172644,124.624178813688)) ;
#64767=CARTESIAN_POINT('Ctrl Pts',(-18.6924953042277,11.0452992369015,124.381703691916)) ;
#64768=CARTESIAN_POINT('Ctrl Pts',(-18.3193404016488,11.235131477786,124.453023478491)) ;
#64769=CARTESIAN_POINT('Ctrl Pts',(-18.5373238034759,11.0551423974231,124.24477971788)) ;
#64770=CARTESIAN_POINT('Ctrl Pts',(-18.1551353492722,11.2451117109724,124.248529269541)) ;
#64771=CARTESIAN_POINT('Ctrl Pts',(-18.4059602224555,11.0651226306096,124.081184300254)) ;
#64772=CARTESIAN_POINT('Ctrl Pts',(-18.028891195577,11.2551302310076,124.017503067163)) ;
#64773=CARTESIAN_POINT('Ctrl Pts',(-18.3049653496854,11.0751411506447,123.896363082341)) ;
#64774=CARTESIAN_POINT('Ctrl Pts',(-17.94527872475,11.2650135393913,123.771572840937)) ;
#64775=CARTESIAN_POINT('Ctrl Pts',(-18.2380760136292,11.0850244590284,123.699619611155)) ;
#64776=CARTESIAN_POINT('Ctrl Pts',(-17.9050223248742,11.2750818235621,123.510113552435)) ;
#64777=CARTESIAN_POINT('Ctrl Pts',(-18.2058712472604,11.0950927431992,123.490451793453)) ;
#64778=CARTESIAN_POINT('Ctrl Pts',(-17.9103370638304,11.2849119502298,123.251798025967)) ;
#64779=CARTESIAN_POINT('Ctrl Pts',(-18.2101233434264,11.1049228698669,123.283800611474)) ;
#64780=CARTESIAN_POINT('Ctrl Pts',(-17.9612752714376,11.2949785224363,122.992253063296)) ;
#64781=CARTESIAN_POINT('Ctrl Pts',(-18.2508742115829,11.1149894420734,123.07616437634)) ;
#64782=CARTESIAN_POINT('Ctrl Pts',(-18.0550114914209,11.304868678677,122.749806436418)) ;
#64783=CARTESIAN_POINT('Ctrl Pts',(-18.3258631525923,11.1248795983141,122.882207960884)) ;
#64784=CARTESIAN_POINT('Ctrl Pts',(-18.1902998279982,11.3148612062534,122.524765958901)) ;
#64785=CARTESIAN_POINT('Ctrl Pts',(-18.4340938564837,11.1348721258905,122.702175798357)) ;
#64786=CARTESIAN_POINT('Ctrl Pts',(-18.362252777776,11.3248226961277,122.327384835979)) ;
#64787=CARTESIAN_POINT('Ctrl Pts',(-18.57165612635,11.1448336157648,122.544271311536)) ;
#64788=CARTESIAN_POINT('Ctrl Pts',(-18.5644303505552,11.3347319180149,122.163249256382)) ;
#64789=CARTESIAN_POINT('Ctrl Pts',(-18.7333976447445,11.154742837652,122.412963346025)) ;
#64790=CARTESIAN_POINT('Ctrl Pts',(-18.7952595963488,11.3447804978252,122.035028175252)) ;
#64791=CARTESIAN_POINT('Ctrl Pts',(-18.9180612583401,11.1647914174624,122.310386442191)) ;
#64792=CARTESIAN_POINT('Ctrl Pts',(-19.0407305551564,11.3546634722953,121.950157334317)) ;
#64793=CARTESIAN_POINT('Ctrl Pts',(-19.1144372025468,11.1746743919324,122.242490108327)) ;
#64794=CARTESIAN_POINT('Ctrl Pts',(-19.3000011957523,11.364658383438,121.908176471057)) ;
#64795=CARTESIAN_POINT('Ctrl Pts',(-19.3218535588989,11.1846693030751,122.208905345717)) ;
#64796=CARTESIAN_POINT('Ctrl Pts',(-19.5633130308643,11.3746787700116,121.912223489131)) ;
#64797=CARTESIAN_POINT('Ctrl Pts',(-19.532503054688,11.1946896896487,122.212142961274)) ;
#64798=CARTESIAN_POINT('Ctrl Pts',(-19.8190707586081,11.3845888738687,121.961229817149)) ;
#64799=CARTESIAN_POINT('Ctrl Pts',(-19.7371085224044,11.2045997935058,122.251347849191)) ;
#64800=CARTESIAN_POINT('Ctrl Pts',(-20.0631345837218,11.3945165860786,122.053434027889)) ;
#64801=CARTESIAN_POINT('Ctrl Pts',(-19.9323591038037,11.2145275057157,122.325110807346)) ;
#64802=CARTESIAN_POINT('Ctrl Pts',(-20.2899581915959,11.4045596958458,122.18834359306)) ;
#64803=CARTESIAN_POINT('Ctrl Pts',(-20.1138182163407,11.2245706154829,122.433038412383)) ;
#64804=CARTESIAN_POINT('Ctrl Pts',(-20.4869200798739,11.4144461163014,122.357790944953)) ;
#64805=CARTESIAN_POINT('Ctrl Pts',(-20.2713871970456,11.2344570359385,122.568595575828)) ;
#64806=CARTESIAN_POINT('Ctrl Pts',(-20.653571934063,11.424439293907,122.560728657171)) ;
#64807=CARTESIAN_POINT('Ctrl Pts',(-20.4047088177741,11.2444502135441,122.730945421941)) ;
#64808=CARTESIAN_POINT('Ctrl Pts',(-20.7817631202176,11.4343849568109,122.788494689918)) ;
#64809=CARTESIAN_POINT('Ctrl Pts',(-20.5072617816881,11.254395876448,122.913157693448)) ;
#64810=CARTESIAN_POINT('Ctrl Pts',(-20.8689810112581,11.4443322530161,123.034933251578)) ;
#64811=CARTESIAN_POINT('Ctrl Pts',(-20.5770363372179,11.2643431726532,123.11030796952)) ;
#64812=CARTESIAN_POINT('Ctrl Pts',(-20.9122274632139,11.454380018594,123.295405142899)) ;
#64813=CARTESIAN_POINT('Ctrl Pts',(-20.611633872492,11.2743909382311,123.318685623006)) ;
#64814=CARTESIAN_POINT('Ctrl Pts',(-20.909847955661,11.4642282318116,123.554192250672)) ;
#64815=CARTESIAN_POINT('Ctrl Pts',(-20.6097306740805,11.2842391514487,123.525714196094)) ;
#64816=CARTESIAN_POINT('Ctrl Pts',(-20.8628861917845,11.4741878046057,123.811671085768)) ;
#64817=CARTESIAN_POINT('Ctrl Pts',(-20.5721619350103,11.2941987242428,123.731697005072)) ;
#64818=CARTESIAN_POINT('Ctrl Pts',(-20.7707963194684,11.4842244256382,124.058815012756)) ;
#64819=CARTESIAN_POINT('Ctrl Pts',(-20.4984904591295,11.3042353452753,123.929412437981)) ;
#64820=CARTESIAN_POINT('Ctrl Pts',(-20.6396015638057,11.4941049404486,124.282914554949)) ;
#64821=CARTESIAN_POINT('Ctrl Pts',(-20.3935356247347,11.3141158600857,124.108691603462)) ;
#64822=CARTESIAN_POINT('Ctrl Pts',(-20.4686789714687,11.5041575917556,124.484292270277)) ;
#64823=CARTESIAN_POINT('Ctrl Pts',(-20.2567978844015,11.3241685113927,124.26979434849)) ;
#64824=CARTESIAN_POINT('Ctrl Pts',(-20.2685707709031,11.5140529900356,124.650429772369)) ;
#64825=CARTESIAN_POINT('Ctrl Pts',(-20.0967123281824,11.3340639096727,124.402704356806)) ;
#64826=CARTESIAN_POINT('Ctrl Pts',(-20.0392516106828,11.5241031117417,124.781376915193)) ;
#64827=CARTESIAN_POINT('Ctrl Pts',(-19.9132571537407,11.3441140313788,124.50746276443)) ;
#64828=CARTESIAN_POINT('Ctrl Pts',(-19.794737934636,11.5339873912836,124.869107009898)) ;
#64829=CARTESIAN_POINT('Ctrl Pts',(-19.7176472402292,11.3539983109207,124.577647198776)) ;
#64830=CARTESIAN_POINT('Ctrl Pts',(-19.5359779545354,11.5439821725755,124.914016452958)) ;
#64831=CARTESIAN_POINT('Ctrl Pts',(-19.5106395508264,11.3639930922127,124.613575518455)) ;
#64832=CARTESIAN_POINT('Ctrl Pts',(-19.2745423776044,11.5539300177623,124.913217278818)) ;
#64833=CARTESIAN_POINT('Ctrl Pts',(-19.3014915210338,11.3739409373994,124.612936961295)) ;
#64834=CARTESIAN_POINT('Ctrl Pts',(-19.0174715357979,11.5638669811497,124.867467500935)) ;
#64835=CARTESIAN_POINT('Ctrl Pts',(-19.0958351968564,11.3838779007868,124.576338085747)) ;
#64836=CARTESIAN_POINT('Ctrl Pts',(-18.7709478903475,11.5738499458869,124.77765044511)) ;
#64837=CARTESIAN_POINT('Ctrl Pts',(-18.8986161489032,11.3938608655241,124.504485401762)) ;
#64838=CARTESIAN_POINT('Ctrl Pts',(-18.5426769439724,11.5838937973026,124.645205762056)) ;
#64839=CARTESIAN_POINT('Ctrl Pts',(-18.7159988423959,11.4039047169397,124.398530300539)) ;
#64840=CARTESIAN_POINT('Ctrl Pts',(-18.3447570490132,11.5937219986373,124.479210868658)) ;
#64841=CARTESIAN_POINT('Ctrl Pts',(-18.5576631821431,11.4137329182744,124.265735876442)) ;
#64842=CARTESIAN_POINT('Ctrl Pts',(-18.1744334770806,11.6037985712354,124.27652667465)) ;
#64843=CARTESIAN_POINT('Ctrl Pts',(-18.4214033306732,11.4238094908725,124.103588905207)) ;
#64844=CARTESIAN_POINT('Ctrl Pts',(-18.0446742700679,11.6136506512429,124.052422800966)) ;
#64845=CARTESIAN_POINT('Ctrl Pts',(-18.3175955633479,11.43366157088,123.924307178956)) ;
#64846=CARTESIAN_POINT('Ctrl Pts',(-17.9536271837052,11.623723936247,123.80390465869)) ;
#64847=CARTESIAN_POINT('Ctrl Pts',(-18.2447567627859,11.4437348558841,123.725492737883)) ;
#64848=CARTESIAN_POINT('Ctrl Pts',(-17.9082400349615,11.6335652879575,123.549277141686)) ;
#64849=CARTESIAN_POINT('Ctrl Pts',(-18.2084461725825,11.4535762075946,123.521791939049)) ;
#64850=CARTESIAN_POINT('Ctrl Pts',(-17.9067818389188,11.643526787354,123.287519099378)) ;
#64851=CARTESIAN_POINT('Ctrl Pts',(-18.2072783316507,11.4635377069911,123.312385832505)) ;
#64852=CARTESIAN_POINT('Ctrl Pts',(-17.951583816689,11.653562563484,123.027613430416)) ;
#64853=CARTESIAN_POINT('Ctrl Pts',(-18.2431187615393,11.4735734831211,123.104461008452)) ;
#64854=CARTESIAN_POINT('Ctrl Pts',(-18.0392630064654,11.6634509901216,122.782997517006)) ;
#64855=CARTESIAN_POINT('Ctrl Pts',(-18.3132606925425,11.4834619097587,122.908768552732)) ;
#64856=CARTESIAN_POINT('Ctrl Pts',(-18.169309686562,11.6734663121965,122.55416670281)) ;
#64857=CARTESIAN_POINT('Ctrl Pts',(-18.4172968626864,11.4934772318336,122.72570323888)) ;
#64858=CARTESIAN_POINT('Ctrl Pts',(-18.337832034103,11.6834966610967,122.351486710983)) ;
#64859=CARTESIAN_POINT('Ctrl Pts',(-18.5521138475697,11.5035075807338,122.563558413002)) ;
#64860=CARTESIAN_POINT('Ctrl Pts',(-18.5348954406339,11.6933400367034,122.18392868398)) ;
#64861=CARTESIAN_POINT('Ctrl Pts',(-18.7097629733351,11.5133509563405,122.429511607795)) ;
#64862=CARTESIAN_POINT('Ctrl Pts',(-18.7619871989816,11.7033694736005,122.05014873987)) ;
#64863=CARTESIAN_POINT('Ctrl Pts',(-18.8914356924309,11.5233803932376,122.322486374189)) ;
#64864=CARTESIAN_POINT('Ctrl Pts',(-19.0091747229,11.7134013515334,121.958483598159)) ;
#64865=CARTESIAN_POINT('Ctrl Pts',(-19.0891853235092,11.5334122711706,122.24915301597)) ;
#64866=CARTESIAN_POINT('Ctrl Pts',(-19.2631763810942,11.7232309746389,121.91157223852)) ;
#64867=CARTESIAN_POINT('Ctrl Pts',(-19.2923853954677,11.543241894276,122.211622724481)) ;
#64868=CARTESIAN_POINT('Ctrl Pts',(-19.5256800788775,11.733220445792,121.908654949481)) ;
#64869=CARTESIAN_POINT('Ctrl Pts',(-19.5023881948005,11.5532313654291,122.209287326421)) ;
#64870=CARTESIAN_POINT('Ctrl Pts',(-19.7859934259949,11.7432642945544,121.95225353693)) ;
#64871=CARTESIAN_POINT('Ctrl Pts',(-19.7106392257516,11.5632752141915,122.244164799925)) ;
#64872=CARTESIAN_POINT('Ctrl Pts',(-20.0294606191008,11.7530860000861,122.037936667196)) ;
#64873=CARTESIAN_POINT('Ctrl Pts',(-19.9054125518466,11.5730969197232,122.312709519324)) ;
#64874=CARTESIAN_POINT('Ctrl Pts',(-20.2595522204667,11.7631210399139,122.166778899388)) ;
#64875=CARTESIAN_POINT('Ctrl Pts',(-20.0894867189853,11.583131959551,122.415781895507)) ;
#64876=CARTESIAN_POINT('Ctrl Pts',(-20.4631137171743,11.7731457468054,122.334014058184)) ;
#64877=CARTESIAN_POINT('Ctrl Pts',(-20.2523368993887,11.5931566664425,122.549568855976)) ;
#64878=CARTESIAN_POINT('Ctrl Pts',(-20.6320140503155,11.7829984511461,122.530257519376)) ;
#64879=CARTESIAN_POINT('Ctrl Pts',(-20.3874578756258,11.6030093707832,122.706561953202)) ;
#64880=CARTESIAN_POINT('Ctrl Pts',(-20.7664764699797,11.7929865733538,122.755655719711)) ;
#64881=CARTESIAN_POINT('Ctrl Pts',(-20.4950292060904,11.6129974929909,122.886879510142)) ;
#64882=CARTESIAN_POINT('Ctrl Pts',(-20.8592244692304,11.8029150434611,122.999531121806)) ;
#64883=CARTESIAN_POINT('Ctrl Pts',(-20.5692290568483,11.6229259630982,123.081978836487)) ;
#64884=CARTESIAN_POINT('Ctrl Pts',(-20.9089464870837,11.8129040206283,123.257291767332)) ;
#64885=CARTESIAN_POINT('Ctrl Pts',(-20.609008398413,11.6329149402654,123.288186875209)) ;
#64886=CARTESIAN_POINT('Ctrl Pts',(-20.912726728438,11.822941827908,123.521040547069)) ;
#64887=CARTESIAN_POINT('Ctrl Pts',(-20.6120343028068,11.6429527475451,123.499185942152)) ;
#64888=CARTESIAN_POINT('Ctrl Pts',(-20.8718727620384,11.8327881287713,123.776548267499)) ;
#64889=CARTESIAN_POINT('Ctrl Pts',(-20.5793530040237,11.6527990484084,123.703591663681)) ;
#64890=CARTESIAN_POINT('Ctrl Pts',(-20.7862889531826,11.8428138721506,124.025729898005)) ;
#64891=CARTESIAN_POINT('Ctrl Pts',(-20.5108877193562,11.6628247917877,123.902937607542)) ;
#64892=CARTESIAN_POINT('Ctrl Pts',(-20.6580711492051,11.8528447385896,124.256054351195)) ;
#64893=CARTESIAN_POINT('Ctrl Pts',(-20.4083150016841,11.6728556582267,124.087198055119)) ;
#64894=CARTESIAN_POINT('Ctrl Pts',(-20.4954300469777,11.8626820973884,124.456984258248)) ;
#64895=CARTESIAN_POINT('Ctrl Pts',(-20.2782040287213,11.6826930170255,124.24794255801)) ;
#64896=CARTESIAN_POINT('Ctrl Pts',(-20.2977609080492,11.8726740583222,124.62982526479)) ;
#64897=CARTESIAN_POINT('Ctrl Pts',(-20.1200700801293,11.6926849779593,124.386216765177)) ;
#64898=CARTESIAN_POINT('Ctrl Pts',(-20.0718918884167,11.8827064208787,124.765820716401)) ;
#64899=CARTESIAN_POINT('Ctrl Pts',(-19.9393758049619,11.7027173405158,124.495014745963)) ;
#64900=CARTESIAN_POINT('Ctrl Pts',(-19.830074922632,11.8925715814531,124.859237594725)) ;
#64901=CARTESIAN_POINT('Ctrl Pts',(-19.7459234677896,11.7125825010902,124.569749829709)) ;
#64902=CARTESIAN_POINT('Ctrl Pts',(-19.5733413955139,11.9025334860308,124.910472534242)) ;
#64903=CARTESIAN_POINT('Ctrl Pts',(-19.5405372387899,11.7225444056679,124.610739722214)) ;
#64904=CARTESIAN_POINT('Ctrl Pts',(-19.3097054567228,11.9125684161065,124.915962853087)) ;
#64905=CARTESIAN_POINT('Ctrl Pts',(-19.3296285015763,11.7325793357437,124.615133939698)) ;
#64906=CARTESIAN_POINT('Ctrl Pts',(-19.0528979312036,11.9224533629601,124.876622619197)) ;
#64907=CARTESIAN_POINT('Ctrl Pts',(-19.1241826214947,11.7424642825973,124.583663814499)) ;
#64908=CARTESIAN_POINT('Ctrl Pts',(-18.8024198540435,11.9325190392716,124.791735612442)) ;
#64909=CARTESIAN_POINT('Ctrl Pts',(-18.9237994015907,11.7525299589087,124.515756076817)) ;
#64910=CARTESIAN_POINT('Ctrl Pts',(-18.5755065294971,11.9423579589065,124.667701912514)) ;
#64911=CARTESIAN_POINT('Ctrl Pts',(-18.7422682586687,11.7623688785436,124.416531178168)) ;
#64912=CARTESIAN_POINT('Ctrl Pts',(-18.3688173844643,11.9524214686409,124.502784044984)) ;
#64913=CARTESIAN_POINT('Ctrl Pts',(-18.576915561043,11.7724323882781,124.284598445225)) ;
#64914=CARTESIAN_POINT('Ctrl Pts',(-18.1969723593472,11.9623150818027,124.307637940785)) ;
#64915=CARTESIAN_POINT('Ctrl Pts',(-18.4394382482953,11.7823260014398,124.128483203739)) ;
#64916=CARTESIAN_POINT('Ctrl Pts',(-18.0603757685369,11.9722590886161,124.08490476088)) ;
#64917=CARTESIAN_POINT('Ctrl Pts',(-18.3301592733883,11.7922700082532,123.950297959954)) ;
#64918=CARTESIAN_POINT('Ctrl Pts',(-17.9638367967476,11.9822600429704,123.840420099808)) ;
#64919=CARTESIAN_POINT('Ctrl Pts',(-18.2529261323973,11.8022709626075,123.754711076634)) ;
#64920=CARTESIAN_POINT('Ctrl Pts',(-17.9114896578375,11.9922988006627,123.58188181945)) ;
#64921=CARTESIAN_POINT('Ctrl Pts',(-18.2110463657214,11.8123097202998,123.547880858099)) ;
#64922=CARTESIAN_POINT('Ctrl Pts',(-17.9044041219212,12.0021229848327,123.323787975382)) ;
#64923=CARTESIAN_POINT('Ctrl Pts',(-18.2053758050296,11.8221339044698,123.341406308645)) ;
#64924=CARTESIAN_POINT('Ctrl Pts',(-17.9427499485555,12.0121810504321,123.062292370625)) ;
#64925=CARTESIAN_POINT('Ctrl Pts',(-18.2360503193674,11.8321919700692,123.132209452442)) ;
#64926=CARTESIAN_POINT('Ctrl Pts',(-18.0251977237691,12.0221110972068,122.814691316201)) ;
#64927=CARTESIAN_POINT('Ctrl Pts',(-18.3020064298566,11.8421220168439,122.934128140568)) ;
#64928=CARTESIAN_POINT('Ctrl Pts',(-18.1490393731302,12.0320625395439,122.584356522223)) ;
#64929=CARTESIAN_POINT('Ctrl Pts',(-18.4010777391838,11.8520734591811,122.749859395245)) ;
#64930=CARTESIAN_POINT('Ctrl Pts',(-18.3128249788135,12.0421093367232,122.377284739554)) ;
#64931=CARTESIAN_POINT('Ctrl Pts',(-18.5321045207289,11.8621202563603,122.584200615192)) ;
#64932=CARTESIAN_POINT('Ctrl Pts',(-18.5060148098008,12.0519572774033,122.205087588693)) ;
#64933=CARTESIAN_POINT('Ctrl Pts',(-18.6866546893362,11.8719681970404,122.446441468451)) ;
#64934=CARTESIAN_POINT('Ctrl Pts',(-18.7282729224672,12.0619189087459,122.066794754727)) ;
#64935=CARTESIAN_POINT('Ctrl Pts',(-18.8644599124411,11.881929828383,122.335805352937)) ;
#64936=CARTESIAN_POINT('Ctrl Pts',(-18.9729503385559,12.0719475681218,121.968835081685)) ;
#64937=CARTESIAN_POINT('Ctrl Pts',(-19.0602009883113,11.8919584877589,122.257435568384)) ;
#64938=CARTESIAN_POINT('Ctrl Pts',(-19.227831787757,12.08185787101,121.915407496624)) ;
#64939=CARTESIAN_POINT('Ctrl Pts',(-19.2641055266912,11.9018687906471,122.214691356274)) ;
#64940=CARTESIAN_POINT('Ctrl Pts',(-19.4887612039821,12.0917927655722,121.906342273827)) ;
#64941=CARTESIAN_POINT('Ctrl Pts',(-19.472848876618,11.9118036852093,122.207436933983)) ;
#64942=CARTESIAN_POINT('Ctrl Pts',(-19.7500144690061,12.1018338642391,121.943349818059)) ;
#64943=CARTESIAN_POINT('Ctrl Pts',(-19.6818517658866,11.9218447838762,122.23704074526)) ;
#64944=CARTESIAN_POINT('Ctrl Pts',(-19.9971083719985,12.1117211467435,122.023739879768)) ;
#64945=CARTESIAN_POINT('Ctrl Pts',(-19.8795274617952,11.9317320663806,122.301350619632)) ;
#64946=CARTESIAN_POINT('Ctrl Pts',(-20.2290950029525,12.121712887254,122.146694306298)) ;
#64947=CARTESIAN_POINT('Ctrl Pts',(-20.0651177734983,11.9417238068911,122.399712142644)) ;
#64948=CARTESIAN_POINT('Ctrl Pts',(-20.4353231818005,12.1316634364894,122.307485013012)) ;
#64949=CARTESIAN_POINT('Ctrl Pts',(-20.230101643679,11.9516743561265,122.528342886444)) ;
#64950=CARTESIAN_POINT('Ctrl Pts',(-20.6105080303125,12.1415991141242,122.501068844292)) ;
#64951=CARTESIAN_POINT('Ctrl Pts',(-20.3702511605467,11.9616100337613,122.683208400421)) ;
#64952=CARTESIAN_POINT('Ctrl Pts',(-20.750371753253,12.151584531917,122.723117938316)) ;
#64953=CARTESIAN_POINT('Ctrl Pts',(-20.4821440178031,11.9715954515541,122.860846434547)) ;
#64954=CARTESIAN_POINT('Ctrl Pts',(-20.8496752814087,12.1616133247875,122.967237619846)) ;
#64955=CARTESIAN_POINT('Ctrl Pts',(-20.5615889029913,11.9816242444246,123.056141266303)) ;
#64956=CARTESIAN_POINT('Ctrl Pts',(-20.9045281450594,12.1714928360155,123.220996340645)) ;
#64957=CARTESIAN_POINT('Ctrl Pts',(-20.6054733938422,11.9915037556526,123.259147756982)) ;
#64958=CARTESIAN_POINT('Ctrl Pts',(-20.9152054113298,12.1814863726884,123.483408955597)) ;
#64959=CARTESIAN_POINT('Ctrl Pts',(-20.6140174445098,12.0014972923255,123.469077721808)) ;
#64960=CARTESIAN_POINT('Ctrl Pts',(-20.8794802827671,12.1915186409522,123.744603500789)) ;
#64961=CARTESIAN_POINT('Ctrl Pts',(-20.5854395864625,12.0115295605894,123.678033578765)) ;
#64962=CARTESIAN_POINT('Ctrl Pts',(-20.8008139737887,12.2013826029581,123.991621606298)) ;
#64963=CARTESIAN_POINT('Ctrl Pts',(-20.522508650298,12.0213935225952,123.875648805063)) ;
#64964=CARTESIAN_POINT('Ctrl Pts',(-20.678002189668,12.211452664303,124.225997440401)) ;
#64965=CARTESIAN_POINT('Ctrl Pts',(-20.4242612619508,12.0314635839401,124.063150402527)) ;
#64966=CARTESIAN_POINT('Ctrl Pts',(-20.5199833626838,12.2212950286517,124.430776031763)) ;
#64967=CARTESIAN_POINT('Ctrl Pts',(-20.2978478905724,12.0413059482889,124.22697474946)) ;
#64968=CARTESIAN_POINT('Ctrl Pts',(-20.327174746647,12.2312557011542,124.607803018266)) ;
#64969=CARTESIAN_POINT('Ctrl Pts',(-20.1436024451247,12.0512666207913,124.368597976752)) ;
#64970=CARTESIAN_POINT('Ctrl Pts',(-20.1045650508631,12.241293772222,124.749310160051)) ;
#64971=CARTESIAN_POINT('Ctrl Pts',(-19.9655159909283,12.0613046918591,124.48180549562)) ;
#64972=CARTESIAN_POINT('Ctrl Pts',(-19.8649051459857,12.2511673871824,124.84884392232)) ;
#64973=CARTESIAN_POINT('Ctrl Pts',(-19.7737886892284,12.0711783068196,124.561434593888)) ;
#64974=CARTESIAN_POINT('Ctrl Pts',(-19.6065797304044,12.2612396217637,124.906300997495)) ;
#64975=CARTESIAN_POINT('Ctrl Pts',(-19.5671291439869,12.0812505414008,124.607402358508)) ;
#64976=CARTESIAN_POINT('Ctrl Pts',(-19.3486297183306,12.2710636402125,124.918040759663)) ;
#64977=CARTESIAN_POINT('Ctrl Pts',(-19.3607684323741,12.0910745598496,124.616796316392)) ;
#64978=CARTESIAN_POINT('Ctrl Pts',(-19.0863456687476,12.2811285611885,124.884353810211)) ;
#64979=CARTESIAN_POINT('Ctrl Pts',(-19.1509427633031,12.1011394808256,124.589849001883)) ;
#64980=CARTESIAN_POINT('Ctrl Pts',(-18.7548496615759,12.2943388594833,124.781008020348)) ;
#64981=CARTESIAN_POINT('Ctrl Pts',(-18.8857366261165,12.1143497791204,124.507174493907)) ;
#64982=CARTESIAN_POINT('Ctrl Pts',(-18.4555083325038,12.3076543062152,124.592460114452)) ;
#64983=CARTESIAN_POINT('Ctrl Pts',(-18.646238230641,12.1276652258523,124.356312323164)) ;
#64984=CARTESIAN_POINT('Ctrl Pts',(-18.2182158984291,12.3209445514825,124.336043204847)) ;
#64985=CARTESIAN_POINT('Ctrl Pts',(-18.4564387255934,12.1409554711196,124.15121228678)) ;
#64986=CARTESIAN_POINT('Ctrl Pts',(-18.0753697674858,12.3309953010896,124.113946532571)) ;
#64987=CARTESIAN_POINT('Ctrl Pts',(-18.3421528585355,12.1510062207267,123.973529844557)) ;
#64988=CARTESIAN_POINT('Ctrl Pts',(-17.9751686262583,12.3408079080718,123.876303265546)) ;
#64989=CARTESIAN_POINT('Ctrl Pts',(-18.261991656828,12.160818827709,123.783417405138)) ;
#64990=CARTESIAN_POINT('Ctrl Pts',(-17.9159132713503,12.3508790060661,123.61839959421)) ;
#64991=CARTESIAN_POINT('Ctrl Pts',(-18.2145854546591,12.1708899257032,123.577093729689)) ;
#64992=CARTESIAN_POINT('Ctrl Pts',(-17.9028470180164,12.360768578841,123.358821518713)) ;
#64993=CARTESIAN_POINT('Ctrl Pts',(-18.2041287543014,12.1807794984781,123.369434895776)) ;
#64994=CARTESIAN_POINT('Ctrl Pts',(-17.9449900324593,12.3740386856443,123.012644489447)) ;
#64995=CARTESIAN_POINT('Ctrl Pts',(-18.2378495546872,12.1940496052814,123.092473752692)) ;
#64996=CARTESIAN_POINT('Ctrl Pts',(-18.1100382420715,12.3906553725668,122.603018959482)) ;
#64997=CARTESIAN_POINT('Ctrl Pts',(-18.3698647094851,12.2106662922039,122.764802568865)) ;
#64998=CARTESIAN_POINT('Ctrl Pts',(-18.403953809166,12.407229415883,122.274921978595)) ;
#64999=CARTESIAN_POINT('Ctrl Pts',(-18.6050396625321,12.2272403355201,122.502279805884)) ;
#65000=CARTESIAN_POINT('Ctrl Pts',(-18.6963080999561,12.4205259833148,122.083501484983)) ;
#65001=CARTESIAN_POINT('Ctrl Pts',(-18.838884457567,12.2405369029519,122.349174750329)) ;
#65002=CARTESIAN_POINT('Ctrl Pts',(-18.9385791929077,12.4305560468922,121.979673523522)) ;
#65003=CARTESIAN_POINT('Ctrl Pts',(-19.0327084258361,12.2505669665293,122.266104229579)) ;
#65004=CARTESIAN_POINT('Ctrl Pts',(-19.1916818709481,12.4404499387414,121.920281628208)) ;
#65005=CARTESIAN_POINT('Ctrl Pts',(-19.2351869221464,12.2604608583786,122.218590195066)) ;
#65006=CARTESIAN_POINT('Ctrl Pts',(-19.5394009792638,12.453702694527,121.899549493621)) ;
#65007=CARTESIAN_POINT('Ctrl Pts',(-19.5133723354866,12.2737136141641,122.202003998467)) ;
#65008=CARTESIAN_POINT('Ctrl Pts',(-19.9747293753154,12.4704307995194,121.989564308867)) ;
#65009=CARTESIAN_POINT('Ctrl Pts',(-19.8616245760486,12.2904417191566,122.274010791926)) ;
#65010=CARTESIAN_POINT('Ctrl Pts',(-20.423556659189,12.4902616359979,122.266069036656)) ;
#65011=CARTESIAN_POINT('Ctrl Pts',(-20.2206924545975,12.3102725556351,122.495213082915)) ;
#65012=CARTESIAN_POINT('Ctrl Pts',(-20.7535327226879,12.5101870278881,122.680135635484)) ;
#65013=CARTESIAN_POINT('Ctrl Pts',(-20.4846749563749,12.3301979475252,122.826464874533)) ;
#65014=CARTESIAN_POINT('Ctrl Pts',(-20.9224041261077,12.5301122412401,123.18215712058)) ;
#65015=CARTESIAN_POINT('Ctrl Pts',(-20.6197750512931,12.3501231608772,123.228081791924)) ;
#65016=CARTESIAN_POINT('Ctrl Pts',(-20.9099617273115,12.5500372547252,123.711523704258)) ;
#65017=CARTESIAN_POINT('Ctrl Pts',(-20.6098235773023,12.3700481743623,123.651575730201)) ;
#65018=CARTESIAN_POINT('Ctrl Pts',(-20.7187360422604,12.5699137264252,124.204018044716)) ;
#65019=CARTESIAN_POINT('Ctrl Pts',(-20.4568446351546,12.3899246460623,124.045573021246)) ;
#65020=CARTESIAN_POINT('Ctrl Pts',(-20.3693300643289,12.5898930443341,124.603877601687)) ;
#65021=CARTESIAN_POINT('Ctrl Pts',(-20.1773211406971,12.4099039639712,124.365462064758)) ;
#65022=CARTESIAN_POINT('Ctrl Pts',(-19.9052905888142,12.6098260479101,124.859582769263)) ;
#65023=CARTESIAN_POINT('Ctrl Pts',(-19.8060899284359,12.4298369675472,124.570028153243)) ;
#65024=CARTESIAN_POINT('Ctrl Pts',(-19.3829989743676,12.6297213179378,124.941977004567)) ;
#65025=CARTESIAN_POINT('Ctrl Pts',(-19.388255790433,12.4497322375749,124.635945220169)) ;
#65026=CARTESIAN_POINT('Ctrl Pts',(-18.8631060156455,12.6496426558436,124.841587523865)) ;
#65027=CARTESIAN_POINT('Ctrl Pts',(-18.9723403696999,12.4696535754807,124.555634564112)) ;
#65028=CARTESIAN_POINT('Ctrl Pts',(-18.4079042835162,12.6696002791098,124.569214868981)) ;
#65029=CARTESIAN_POINT('Ctrl Pts',(-18.6081780879779,12.4896111987469,124.337737060207)) ;
#65030=CARTESIAN_POINT('Ctrl Pts',(-18.0742532724176,12.689480111067,124.15962015315)) ;
#65031=CARTESIAN_POINT('Ctrl Pts',(-18.3412557256098,12.5094910307041,124.010060596195)) ;
#65032=CARTESIAN_POINT('Ctrl Pts',(-17.8989480657597,12.7093619623639,123.661012507451)) ;
#65033=CARTESIAN_POINT('Ctrl Pts',(-18.2010112129469,12.529372882001,123.611173006021)) ;
#65034=CARTESIAN_POINT('Ctrl Pts',(-17.9053743363839,12.7294329794677,123.127663535506)) ;
#65035=CARTESIAN_POINT('Ctrl Pts',(-18.206152086956,12.5494438991048,123.184494766924)) ;
#65036=CARTESIAN_POINT('Ctrl Pts',(-18.0909224032866,12.7492402032208,122.634900991628)) ;
#65037=CARTESIAN_POINT('Ctrl Pts',(-18.3545915317239,12.5692511228579,122.79028245245)) ;
#65038=CARTESIAN_POINT('Ctrl Pts',(-18.4354537167374,12.7692213387896,122.230824135122)) ;
#65039=CARTESIAN_POINT('Ctrl Pts',(-18.630217413786,12.5892322584267,122.467021418923)) ;
#65040=CARTESIAN_POINT('Ctrl Pts',(-18.8964641846084,12.7891488321288,121.970176160961)) ;
#65041=CARTESIAN_POINT('Ctrl Pts',(-18.9990268654917,12.6091597517659,122.258503153768)) ;
#65042=CARTESIAN_POINT('Ctrl Pts',(-19.415834432645,12.8089694934866,121.881151656097)) ;
#65043=CARTESIAN_POINT('Ctrl Pts',(-19.4145251819836,12.6289804131237,122.187284802725)) ;
#65044=CARTESIAN_POINT('Ctrl Pts',(-19.9411566590933,12.8290666827084,121.976780870031)) ;
#65045=CARTESIAN_POINT('Ctrl Pts',(-19.8347817388246,12.6490776023455,122.26378939332)) ;
#65046=CARTESIAN_POINT('Ctrl Pts',(-20.3952240684518,12.8488303617167,122.241384544964)) ;
#65047=CARTESIAN_POINT('Ctrl Pts',(-20.1980368260556,12.6688412813539,122.475474968688)) ;
#65048=CARTESIAN_POINT('Ctrl Pts',(-20.7368987004041,12.8688876403898,122.650278783027)) ;
#65049=CARTESIAN_POINT('Ctrl Pts',(-20.471374567732,12.6888985600269,122.802591330888)) ;
#65050=CARTESIAN_POINT('Ctrl Pts',(-20.915999998585,12.8886830641372,123.145136393717)) ;
#65051=CARTESIAN_POINT('Ctrl Pts',(-20.6146542216816,12.7086939837743,123.198479843696)) ;
#65052=CARTESIAN_POINT('Ctrl Pts',(-20.9171224626081,12.9086467088648,123.675675466344)) ;
#65053=CARTESIAN_POINT('Ctrl Pts',(-20.6155493596477,12.7286576285019,123.62291137376)) ;
#65054=CARTESIAN_POINT('Ctrl Pts',(-20.7357148689362,12.9286302001389,124.174870580485)) ;
#65055=CARTESIAN_POINT('Ctrl Pts',(-20.4704208498852,12.748641119776,124.022266714748)) ;
#65056=CARTESIAN_POINT('Ctrl Pts',(-20.3986521463145,12.9484376952882,124.579332558867)) ;
#65057=CARTESIAN_POINT('Ctrl Pts',(-20.2007674929157,12.7684486149253,124.345835452123)) ;
#65058=CARTESIAN_POINT('Ctrl Pts',(-19.9402235763069,12.9684202860083,124.847283742868)) ;
#65059=CARTESIAN_POINT('Ctrl Pts',(-19.8340229155712,12.7884312056454,124.560193612836)) ;
#65060=CARTESIAN_POINT('Ctrl Pts',(-19.4202416053834,12.9883029399995,124.942191223807)) ;
#65061=CARTESIAN_POINT('Ctrl Pts',(-19.4180360713643,12.8083138596367,124.636116448561)) ;
#65062=CARTESIAN_POINT('Ctrl Pts',(-18.8972653738817,13.0082611848626,124.854056149815)) ;
#65063=CARTESIAN_POINT('Ctrl Pts',(-18.9996554343786,12.8282721044997,124.565604873839)) ;
#65064=CARTESIAN_POINT('Ctrl Pts',(-18.4373467193133,13.0281367719042,124.594021898923)) ;
#65065=CARTESIAN_POINT('Ctrl Pts',(-18.6317218256589,12.8481476915413,124.357573939608)) ;
#65066=CARTESIAN_POINT('Ctrl Pts',(-18.0917408140289,13.0481176600395,124.190855292359)) ;
#65067=CARTESIAN_POINT('Ctrl Pts',(-18.355239878661,12.8681285796766,124.035038248343)) ;
#65068=CARTESIAN_POINT('Ctrl Pts',(-17.9052414355018,13.0680528011505,123.694844185524)) ;
#65069=CARTESIAN_POINT('Ctrl Pts',(-18.2060442903282,12.8880637207876,123.63822733448)) ;
#65070=CARTESIAN_POINT('Ctrl Pts',(-17.8988271166947,13.0879648191615,123.165702838927)) ;
#65071=CARTESIAN_POINT('Ctrl Pts',(-18.200915253109,12.9079757387987,123.21491552465)) ;
#65072=CARTESIAN_POINT('Ctrl Pts',(-18.072637630343,13.1078530374051,122.666485551976)) ;
#65073=CARTESIAN_POINT('Ctrl Pts',(-18.3399734826579,12.9278639570422,122.815536572551)) ;
#65074=CARTESIAN_POINT('Ctrl Pts',(-18.3508356377982,13.124451341252,122.324166060085)) ;
#65075=CARTESIAN_POINT('Ctrl Pts',(-18.562516670019,12.9444622608891,122.54170220006)) ;
#65076=CARTESIAN_POINT('Ctrl Pts',(-18.6332461345771,13.1377239311548,122.119417599801)) ;
#65077=CARTESIAN_POINT('Ctrl Pts',(-18.7884633789187,12.957734850792,122.37788874013)) ;
#65078=CARTESIAN_POINT('Ctrl Pts',(-18.8696106143661,13.1477313461057,122.004127651261)) ;
#65079=CARTESIAN_POINT('Ctrl Pts',(-18.9775498041114,12.9677422657428,122.285661949653)) ;
#65080=CARTESIAN_POINT('Ctrl Pts',(-19.1224757065835,13.1577386928383,121.931849416177)) ;
#65081=CARTESIAN_POINT('Ctrl Pts',(-19.1798541601348,12.9777496124754,122.22784121804)) ;
#65082=CARTESIAN_POINT('Ctrl Pts',(-19.4692111889447,13.1710050526399,121.895476582139)) ;
#65083=CARTESIAN_POINT('Ctrl Pts',(-19.4571883101494,12.991015972277,122.198742524881)) ;
#65084=CARTESIAN_POINT('Ctrl Pts',(-19.9027886653172,13.1875197102629,121.963391453896)) ;
#65085=CARTESIAN_POINT('Ctrl Pts',(-19.8041192330616,13.0075306299,122.253086454829)) ;
#65086=CARTESIAN_POINT('Ctrl Pts',(-20.2896179416635,13.2041171435055,122.175375538865)) ;
#65087=CARTESIAN_POINT('Ctrl Pts',(-20.1135332169725,13.0241280631426,122.422657930658)) ;
#65088=CARTESIAN_POINT('Ctrl Pts',(-20.5428541366256,13.2174651406505,122.418153018463)) ;
#65089=CARTESIAN_POINT('Ctrl Pts',(-20.3161488901095,13.0374760602876,122.61689817093)) ;
#65090=CARTESIAN_POINT('Ctrl Pts',(-20.6967627804406,13.2273608950021,122.62776755716)) ;
#65091=CARTESIAN_POINT('Ctrl Pts',(-20.4392682594011,13.0473718146392,122.784587934019)) ;
#65092=CARTESIAN_POINT('Ctrl Pts',(-20.8132896637095,13.2373488489335,122.862934128972)) ;
#65093=CARTESIAN_POINT('Ctrl Pts',(-20.5324892841562,13.0573597685706,122.972723020215)) ;
#65094=CARTESIAN_POINT('Ctrl Pts',(-20.887111769064,13.2473060726382,123.114002366625)) ;
#65095=CARTESIAN_POINT('Ctrl Pts',(-20.591544390908,13.0673169922753,123.17357799442)) ;
#65096=CARTESIAN_POINT('Ctrl Pts',(-20.9163194697392,13.2573416191949,123.376085199788)) ;
#65097=CARTESIAN_POINT('Ctrl Pts',(-20.6149084219131,13.077352538832,123.383244498507)) ;
#65098=CARTESIAN_POINT('Ctrl Pts',(-20.9000197111728,13.267228730471,123.635413520908)) ;
#65099=CARTESIAN_POINT('Ctrl Pts',(-20.6018663387177,13.0872396501081,123.590707013406)) ;
#65100=CARTESIAN_POINT('Ctrl Pts',(-20.8387093067046,13.2772201355718,123.890705618829)) ;
#65101=CARTESIAN_POINT('Ctrl Pts',(-20.5528158398965,13.0972310552089,123.794940111806)) ;
#65102=CARTESIAN_POINT('Ctrl Pts',(-20.7344045824693,13.2871657567866,124.130350209159)) ;
#65103=CARTESIAN_POINT('Ctrl Pts',(-20.4693700045889,13.1071766764237,123.986654845543)) ;
#65104=CARTESIAN_POINT('Ctrl Pts',(-20.5904556480587,13.2971150050549,124.348628887742)) ;
#65105=CARTESIAN_POINT('Ctrl Pts',(-20.3542090074305,13.117125924692,124.161276491165)) ;
#65106=CARTESIAN_POINT('Ctrl Pts',(-20.4088310489179,13.3071615002235,124.540222615066)) ;
#65107=CARTESIAN_POINT('Ctrl Pts',(-20.208907719291,13.1271724198607,124.314549885357)) ;
#65108=CARTESIAN_POINT('Ctrl Pts',(-20.2009526790891,13.3170128430151,124.69453910851)) ;
#65109=CARTESIAN_POINT('Ctrl Pts',(-20.0426037537448,13.1370237626522,124.438001210113)) ;
#65110=CARTESIAN_POINT('Ctrl Pts',(-19.9669434550335,13.3269846231424,124.812406349802)) ;
#65111=CARTESIAN_POINT('Ctrl Pts',(-19.85539544562,13.1469955427795,124.532292952135)) ;
#65112=CARTESIAN_POINT('Ctrl Pts',(-19.7153564891379,13.3369798231201,124.888022808457)) ;
#65113=CARTESIAN_POINT('Ctrl Pts',(-19.6541252878157,13.1569907427572,124.592783951486)) ;
#65114=CARTESIAN_POINT('Ctrl Pts',(-19.4534753611638,13.3470138148161,124.918598821052)) ;
#65115=CARTESIAN_POINT('Ctrl Pts',(-19.4446201537456,13.1670247344533,124.617242515926)) ;
#65116=CARTESIAN_POINT('Ctrl Pts',(-19.1948766730221,13.3568692197886,124.903920505576)) ;
#65117=CARTESIAN_POINT('Ctrl Pts',(-19.2377415186523,13.1768801394258,124.605497635822)) ;
#65118=CARTESIAN_POINT('Ctrl Pts',(-18.9390603846793,13.3668685176344,124.844062381727)) ;
#65119=CARTESIAN_POINT('Ctrl Pts',(-19.0330890674642,13.1868794372715,124.557608978315)) ;
#65120=CARTESIAN_POINT('Ctrl Pts',(-18.6998481883594,13.3767636302396,124.741995186928)) ;
#65121=CARTESIAN_POINT('Ctrl Pts',(-18.8417203716604,13.1967745498767,124.475953269536)) ;
#65122=CARTESIAN_POINT('Ctrl Pts',(-18.4784292945889,13.3868242757746,124.597585675323)) ;
#65123=CARTESIAN_POINT('Ctrl Pts',(-18.6645864484423,13.2068351954117,124.360423788125)) ;
#65124=CARTESIAN_POINT('Ctrl Pts',(-18.2893688821215,13.3966731527638,124.420799145494)) ;
#65125=CARTESIAN_POINT('Ctrl Pts',(-18.5133398551408,13.2166840724009,124.218993165454)) ;
#65126=CARTESIAN_POINT('Ctrl Pts',(-18.1305208053495,13.4067018638574,124.210511784196)) ;
#65127=CARTESIAN_POINT('Ctrl Pts',(-18.3862631410708,13.2267127834945,124.050761997541)) ;
#65128=CARTESIAN_POINT('Ctrl Pts',(-18.0112247910287,13.4167312651135,123.975488167396)) ;
#65129=CARTESIAN_POINT('Ctrl Pts',(-18.2908283055355,13.2367421847506,123.862742104803)) ;
#65130=CARTESIAN_POINT('Ctrl Pts',(-17.9354445009214,13.4265714569095,123.72824647118)) ;
#65131=CARTESIAN_POINT('Ctrl Pts',(-18.2302062650651,13.2465823765466,123.664948483144)) ;
#65132=CARTESIAN_POINT('Ctrl Pts',(-17.9027395319079,13.4365748861025,123.467435684465)) ;
#65133=CARTESIAN_POINT('Ctrl Pts',(-18.2040444166883,13.2565858057396,123.456299663574)) ;
#65134=CARTESIAN_POINT('Ctrl Pts',(-17.9158814573718,13.4465603985687,123.205311390375)) ;
#65135=CARTESIAN_POINT('Ctrl Pts',(-18.2145600879431,13.2665713182058,123.24660043712)) ;
#65136=CARTESIAN_POINT('Ctrl Pts',(-17.9749065837832,13.4566014949527,122.948155155583)) ;
#65137=CARTESIAN_POINT('Ctrl Pts',(-18.2617823053095,13.2766124145898,123.040875912254)) ;
#65138=CARTESIAN_POINT('Ctrl Pts',(-18.0753470360815,13.4664446909037,122.709757985454)) ;
#65139=CARTESIAN_POINT('Ctrl Pts',(-18.3421364530239,13.2864556105408,122.850159423479)) ;
#65140=CARTESIAN_POINT('Ctrl Pts',(-18.217218281521,13.4764310019581,122.489035231126)) ;
#65141=CARTESIAN_POINT('Ctrl Pts',(-18.455635132101,13.2964419215952,122.673582454515)) ;
#65142=CARTESIAN_POINT('Ctrl Pts',(-18.3942732512551,13.4863656872158,122.297106419642)) ;
#65143=CARTESIAN_POINT('Ctrl Pts',(-18.5972804423146,13.3063766068529,122.520040993049)) ;
#65144=CARTESIAN_POINT('Ctrl Pts',(-18.6046031877743,13.4964232484328,122.137116873894)) ;
#65145=CARTESIAN_POINT('Ctrl Pts',(-18.7655457306992,13.31643416807,122.392050961701)) ;
#65146=CARTESIAN_POINT('Ctrl Pts',(-18.8338850495127,13.5062448900414,122.018535713195)) ;
#65147=CARTESIAN_POINT('Ctrl Pts',(-18.9489715980104,13.3262558096786,122.297188133943)) ;
#65148=CARTESIAN_POINT('Ctrl Pts',(-19.0859583258846,13.5163009536324,121.939273611562)) ;
#65149=CARTESIAN_POINT('Ctrl Pts',(-19.1506308986353,13.3363118732695,122.233780316748)) ;
#65150=CARTESIAN_POINT('Ctrl Pts',(-19.3450516698222,13.5262416293942,121.905839973782)) ;
#65151=CARTESIAN_POINT('Ctrl Pts',(-19.3579055692691,13.3462525490313,122.207035465221)) ;
#65152=CARTESIAN_POINT('Ctrl Pts',(-19.6050909750196,13.5361459881825,121.917041144644)) ;
#65153=CARTESIAN_POINT('Ctrl Pts',(-19.565936503742,13.3561569078197,122.215998316432)) ;
#65154=CARTESIAN_POINT('Ctrl Pts',(-19.862825851585,13.5461926427583,121.97418792217)) ;
#65155=CARTESIAN_POINT('Ctrl Pts',(-19.7721240620941,13.3662035623955,122.261717666906)) ;
#65156=CARTESIAN_POINT('Ctrl Pts',(-20.1031997643857,13.5560882374012,122.073508487898)) ;
#65157=CARTESIAN_POINT('Ctrl Pts',(-19.9644220277355,13.3760991570383,122.341175720192)) ;
#65158=CARTESIAN_POINT('Ctrl Pts',(-20.3263218440362,13.5661501840581,122.215343672236)) ;
#65159=CARTESIAN_POINT('Ctrl Pts',(-20.1429187779707,13.3861611036952,122.454645564345)) ;
#65160=CARTESIAN_POINT('Ctrl Pts',(-20.5173749645332,13.5759998079902,122.38999462014)) ;
#65161=CARTESIAN_POINT('Ctrl Pts',(-20.295759491306,13.3960107276274,122.594367286313)) ;
#65162=CARTESIAN_POINT('Ctrl Pts',(-20.6776884554839,13.5859630470201,122.596980439567)) ;
#65163=CARTESIAN_POINT('Ctrl Pts',(-20.4240087199095,13.4059739666572,122.759956837706)) ;
#65164=CARTESIAN_POINT('Ctrl Pts',(-20.8000704181908,13.5959876217959,122.830280403309)) ;
#65165=CARTESIAN_POINT('Ctrl Pts',(-20.5219126738478,13.415998541433,122.946597684399)) ;
#65166=CARTESIAN_POINT('Ctrl Pts',(-20.8793920083737,13.6059061844836,123.07855998187)) ;
#65167=CARTESIAN_POINT('Ctrl Pts',(-20.5853680842003,13.4259171041207,123.145221485307)) ;
#65168=CARTESIAN_POINT('Ctrl Pts',(-20.9151199375489,13.6158983712076,123.338717822216)) ;
#65169=CARTESIAN_POINT('Ctrl Pts',(-20.6139486858676,13.4359092908447,123.353347860863)) ;
#65170=CARTESIAN_POINT('Ctrl Pts',(-20.9046168525977,13.6259331697918,123.6022019633)) ;
#65171=CARTESIAN_POINT('Ctrl Pts',(-20.605544399225,13.4459440894289,123.564135168279)) ;
#65172=CARTESIAN_POINT('Ctrl Pts',(-20.8499556627768,13.6357883604655,123.855372966742)) ;
#65173=CARTESIAN_POINT('Ctrl Pts',(-20.5618138995585,13.4557992801026,123.766670884377)) ;
#65174=CARTESIAN_POINT('Ctrl Pts',(-20.7510855573927,13.6457877086185,124.098788324435)) ;
#65175=CARTESIAN_POINT('Ctrl Pts',(-20.4827162949927,13.4657986282556,123.961402436991)) ;
#65176=CARTESIAN_POINT('Ctrl Pts',(-20.6130996723433,13.6556828342936,124.319242233489)) ;
#65177=CARTESIAN_POINT('Ctrl Pts',(-20.3723265173656,13.4756937539307,124.137764200893)) ;
#65178=CARTESIAN_POINT('Ctrl Pts',(-20.4360519660016,13.6657433772417,124.515540628893)) ;
#65179=CARTESIAN_POINT('Ctrl Pts',(-20.2306870063593,13.4857542968788,124.294801963191)) ;
#65180=CARTESIAN_POINT('Ctrl Pts',(-20.2320341456861,13.6755926515086,124.674850714962)) ;
#65181=CARTESIAN_POINT('Ctrl Pts',(-20.0674724171004,13.4956035711457,124.422248249584)) ;
#65182=CARTESIAN_POINT('Ctrl Pts',(-19.9996623311131,13.6856198760785,124.799086161189)) ;
#65183=CARTESIAN_POINT('Ctrl Pts',(-19.8815742380617,13.5056307957156,124.521635311594)) ;
#65184=CARTESIAN_POINT('Ctrl Pts',(-19.7489854254844,13.6956482752663,124.880448501815)) ;
#65185=CARTESIAN_POINT('Ctrl Pts',(-19.6810321616281,13.5156591949034,124.586723663228)) ;
#65186=CARTESIAN_POINT('Ctrl Pts',(-19.4928401900497,13.7054940256798,124.916853671087)) ;
#65187=CARTESIAN_POINT('Ctrl Pts',(-19.4761166444092,13.5255049453169,124.615846163914)) ;
#65188=CARTESIAN_POINT('Ctrl Pts',(-19.230454887784,13.7154828160805,124.908839488335)) ;
#65189=CARTESIAN_POINT('Ctrl Pts',(-19.2662086080236,13.5354937357177,124.609433445062)) ;
#65190=CARTESIAN_POINT('Ctrl Pts',(-18.9721627761797,13.7255277444802,124.854438840815)) ;
#65191=CARTESIAN_POINT('Ctrl Pts',(-19.0595750986044,13.5455386641174,124.565911420256)) ;
#65192=CARTESIAN_POINT('Ctrl Pts',(-18.7323658376547,13.7353522292692,124.758724681303)) ;
#65193=CARTESIAN_POINT('Ctrl Pts',(-18.8677390346098,13.5553631489063,124.489339193207)) ;
#65194=CARTESIAN_POINT('Ctrl Pts',(-18.507457139982,13.7454096268104,124.619951807237)) ;
#65195=CARTESIAN_POINT('Ctrl Pts',(-18.6878125850875,13.5654205464475,124.378319667226)) ;
#65196=CARTESIAN_POINT('Ctrl Pts',(-18.3128349524813,13.7553357183966,124.44624656969)) ;
#65197=CARTESIAN_POINT('Ctrl Pts',(-18.5321161260099,13.5753466380337,124.239354778128)) ;
#65198=CARTESIAN_POINT('Ctrl Pts',(-18.1503452309715,13.7652905035412,124.241231958245)) ;
#65199=CARTESIAN_POINT('Ctrl Pts',(-18.4021255453027,13.5853014231783,124.075342601526)) ;
#65200=CARTESIAN_POINT('Ctrl Pts',(-18.0251465109341,13.7753278731988,124.009068223143)) ;
#65201=CARTESIAN_POINT('Ctrl Pts',(-18.3019676694534,13.5953387928359,123.889610906895)) ;
#65202=CARTESIAN_POINT('Ctrl Pts',(-17.9431959784106,13.7852166833204,123.762452941019)) ;
#65203=CARTESIAN_POINT('Ctrl Pts',(-18.2364086692508,13.6052276029575,123.692318981433)) ;
#65204=CARTESIAN_POINT('Ctrl Pts',(-17.9044614031139,13.7952060423715,123.502822293364)) ;
#65205=CARTESIAN_POINT('Ctrl Pts',(-18.2054221786113,13.6152169620086,123.484614462953)) ;
#65206=CARTESIAN_POINT('Ctrl Pts',(-17.9115693386521,13.8051645898276,123.241226463732)) ;
#65207=CARTESIAN_POINT('Ctrl Pts',(-18.2111097180374,13.6251755094647,123.275338178328)) ;
#65208=CARTESIAN_POINT('Ctrl Pts',(-17.9630567197968,13.8150641663786,122.986205100608)) ;
#65209=CARTESIAN_POINT('Ctrl Pts',(-18.2523005182494,13.6350750860157,123.071321986717)) ;
#65210=CARTESIAN_POINT('Ctrl Pts',(-18.0595361492998,13.8251120782093,122.740443216478)) ;
#65211=CARTESIAN_POINT('Ctrl Pts',(-18.329485128724,13.6451229978464,122.874712710548)) ;
#65212=CARTESIAN_POINT('Ctrl Pts',(-18.1949930036132,13.8350074260699,122.518422190268)) ;
#65213=CARTESIAN_POINT('Ctrl Pts',(-18.4378511109109,13.655018345707,122.697097049966)) ;
#65214=CARTESIAN_POINT('Ctrl Pts',(-18.3697572977927,13.845069102601,122.320042659935)) ;
#65215=CARTESIAN_POINT('Ctrl Pts',(-18.5776634866624,13.6650800222382,122.538393906198)) ;
#65216=CARTESIAN_POINT('Ctrl Pts',(-18.5718588198519,13.8549136203502,122.158525512922)) ;
#65217=CARTESIAN_POINT('Ctrl Pts',(-18.7393445112275,13.6749245399873,122.409181641225)) ;
#65218=CARTESIAN_POINT('Ctrl Pts',(-18.8011469810602,13.864874064065,122.032284729829)) ;
#65219=CARTESIAN_POINT('Ctrl Pts',(-18.9227751038679,13.6848849837021,122.308189886519)) ;
#65220=CARTESIAN_POINT('Ctrl Pts',(-19.0509301231226,13.8749108968832,121.947590007007)) ;
#65221=CARTESIAN_POINT('Ctrl Pts',(-19.1226020288338,13.6949218165203,122.240434931693)) ;
#65222=CARTESIAN_POINT('Ctrl Pts',(-19.3074865101994,13.88478969363,121.907757156992)) ;
#65223=CARTESIAN_POINT('Ctrl Pts',(-19.3278463927919,13.7048006132671,122.208569584531)) ;
#65224=CARTESIAN_POINT('Ctrl Pts',(-19.5717537455678,13.8948490097584,121.91308802529)) ;
#65225=CARTESIAN_POINT('Ctrl Pts',(-19.5392604248098,13.7148599293955,122.212835072421)) ;
#65226=CARTESIAN_POINT('Ctrl Pts',(-19.8262549511952,13.9047194565116,121.963266910915)) ;
#65227=CARTESIAN_POINT('Ctrl Pts',(-19.7428603300386,13.7247303761487,122.252978777756)) ;
#65228=CARTESIAN_POINT('Ctrl Pts',(-20.0714142577279,13.9147120947696,122.057363864517)) ;
#65229=CARTESIAN_POINT('Ctrl Pts',(-19.9389874113429,13.7347230144067,122.328256860103)) ;
#65230=CARTESIAN_POINT('Ctrl Pts',(-20.2970965036502,13.9247441103175,122.193613633218)) ;
#65231=CARTESIAN_POINT('Ctrl Pts',(-20.1195328981886,13.7447550299547,122.437257373362)) ;
#65232=CARTESIAN_POINT('Ctrl Pts',(-20.4928009018349,13.9346099666241,122.363706237578)) ;
#65233=CARTESIAN_POINT('Ctrl Pts',(-20.2760952675698,13.7546208862612,122.573331276944)) ;
#65234=CARTESIAN_POINT('Ctrl Pts',(-20.6593476164435,13.9446792560932,122.569291069351)) ;
#65235=CARTESIAN_POINT('Ctrl Pts',(-20.4093323747788,13.7646901757304,122.737799786026)) ;
#65236=CARTESIAN_POINT('Ctrl Pts',(-20.7848399902421,13.9545228136445,122.795508554596)) ;
#65237=CARTESIAN_POINT('Ctrl Pts',(-20.509725196703,13.7745337332817,122.91877307958)) ;
#65238=CARTESIAN_POINT('Ctrl Pts',(-20.871120064522,13.9645029404324,123.043168459414)) ;
#65239=CARTESIAN_POINT('Ctrl Pts',(-20.578748805291,13.7845138600695,123.116900896814)) ;
#65240=CARTESIAN_POINT('Ctrl Pts',(-20.9127502836893,13.9745214890323,123.303126129535)) ;
#65241=CARTESIAN_POINT('Ctrl Pts',(-20.6120524706176,13.7945324086694,123.324867123436)) ;
#65242=CARTESIAN_POINT('Ctrl Pts',(-20.9092186327094,13.9844047895555,123.562857078074)) ;
#65243=CARTESIAN_POINT('Ctrl Pts',(-20.609226783806,13.8044157091926,123.532650998994)) ;
#65244=CARTESIAN_POINT('Ctrl Pts',(-20.8596340362664,13.9944730766036,123.822708783211)) ;
#65245=CARTESIAN_POINT('Ctrl Pts',(-20.5695586439728,13.8144839962408,123.740532609343)) ;
#65246=CARTESIAN_POINT('Ctrl Pts',(-20.7681595371697,14.0043031996223,124.064344085627)) ;
#65247=CARTESIAN_POINT('Ctrl Pts',(-20.4963791721871,13.8243141192594,123.933839581481)) ;
#65248=CARTESIAN_POINT('Ctrl Pts',(-20.6332814623007,14.0143697835476,124.291865630646)) ;
#65249=CARTESIAN_POINT('Ctrl Pts',(-20.3884763385761,13.8343807031847,124.11585696606)) ;
#65250=CARTESIAN_POINT('Ctrl Pts',(-20.4637992773007,14.0242598965621,124.488951781943)) ;
#65251=CARTESIAN_POINT('Ctrl Pts',(-20.2528909214938,13.8442708161992,124.273525063999)) ;
#65252=CARTESIAN_POINT('Ctrl Pts',(-20.2609821100153,14.0342525853247,124.655717889191)) ;
#65253=CARTESIAN_POINT('Ctrl Pts',(-20.090637223389,13.8542635049618,124.406937730911)) ;
#65254=CARTESIAN_POINT('Ctrl Pts',(-20.0328972096088,14.0442134736805,124.784181661414)) ;
#65255=CARTESIAN_POINT('Ctrl Pts',(-19.9081695446619,13.8642243933176,124.509708392774)) ;
#65256=CARTESIAN_POINT('Ctrl Pts',(-19.7872119388903,14.0541314185605,124.87112949854)) ;
#65257=CARTESIAN_POINT('Ctrl Pts',(-19.7116219327022,13.8741423381976,124.579266367016)) ;
#65258=CARTESIAN_POINT('Ctrl Pts',(-19.527842932523,14.0641391716567,124.914794637581)) ;
#65259=CARTESIAN_POINT('Ctrl Pts',(-19.5041267743093,13.8841500912938,124.614198467582)) ;
#65260=CARTESIAN_POINT('Ctrl Pts',(-19.2642632651857,14.0741702656157,124.912222739613)) ;
#65261=CARTESIAN_POINT('Ctrl Pts',(-19.2932629428853,13.8941811852529,124.612140811124)) ;
#65262=CARTESIAN_POINT('Ctrl Pts',(-19.0097259981526,14.0840182336437,124.865371406458)) ;
#65263=CARTESIAN_POINT('Ctrl Pts',(-19.0896342385044,13.9040291532808,124.57465995883)) ;
#65264=CARTESIAN_POINT('Ctrl Pts',(-18.7618772164016,14.0940801897696,124.773301901415)) ;
#65265=CARTESIAN_POINT('Ctrl Pts',(-18.89135492329,13.9140911094067,124.501004319296)) ;
#65266=CARTESIAN_POINT('Ctrl Pts',(-18.5376101429091,14.1039774013707,124.641559789166)) ;
#65267=CARTESIAN_POINT('Ctrl Pts',(-18.7119419501136,13.9239883210078,124.395611039838)) ;
#65268=CARTESIAN_POINT('Ctrl Pts',(-18.3384000135968,14.1139085680353,124.472965869001)) ;
#65269=CARTESIAN_POINT('Ctrl Pts',(-18.5525741413936,13.9339194876725,124.26073644889)) ;
#65270=CARTESIAN_POINT('Ctrl Pts',(-18.169843513441,14.1239507522395,124.269917095288)) ;
#65271=CARTESIAN_POINT('Ctrl Pts',(-18.4177287173971,13.9439616718766,124.098297399059)) ;
#65272=CARTESIAN_POINT('Ctrl Pts',(-18.0409566998773,14.1338374204927,124.044314253981)) ;
#65273=CARTESIAN_POINT('Ctrl Pts',(-18.3146195241724,13.9538483401298,123.91781597991)) ;
#65274=CARTESIAN_POINT('Ctrl Pts',(-17.9518498698231,14.1438305324709,123.797299870393)) ;
#65275=CARTESIAN_POINT('Ctrl Pts',(-18.2433338227016,13.963841452108,123.720204732081)) ;
#65276=CARTESIAN_POINT('Ctrl Pts',(-17.9072936184703,14.1537762100867,123.539763194409)) ;
#65277=CARTESIAN_POINT('Ctrl Pts',(-18.2076886217236,13.9737871297239,123.514175908959)) ;
#65278=CARTESIAN_POINT('Ctrl Pts',(-17.9075982211722,14.1637235130717,123.278346044345)) ;
#65279=CARTESIAN_POINT('Ctrl Pts',(-18.2079318833263,13.9837344327088,123.305042647858)) ;
#65280=CARTESIAN_POINT('Ctrl Pts',(-17.9540338467725,14.1737712368185,123.018424649771)) ;
#65281=CARTESIAN_POINT('Ctrl Pts',(-18.245080078658,13.9937821564556,123.097105274778)) ;
#65282=CARTESIAN_POINT('Ctrl Pts',(-18.0429036250617,14.183619610581,122.775359841272)) ;
#65283=CARTESIAN_POINT('Ctrl Pts',(-18.3161751445601,14.0036305302181,122.90265434045)) ;
#65284=CARTESIAN_POINT('Ctrl Pts',(-18.1733306008267,14.1935785830267,122.54846390798)) ;
#65285=CARTESIAN_POINT('Ctrl Pts',(-18.4205160052355,14.0135895026638,122.721137613016)) ;
#65286=CARTESIAN_POINT('Ctrl Pts',(-18.3428801887918,14.2036174449079,122.346364098552)) ;
#65287=CARTESIAN_POINT('Ctrl Pts',(-18.5561553752817,14.023628364545,122.559457349719)) ;
#65288=CARTESIAN_POINT('Ctrl Pts',(-18.5414813532127,14.2134960490797,122.179140432255)) ;
#65289=CARTESIAN_POINT('Ctrl Pts',(-18.7150352359828,14.0335069687168,122.425678533261)) ;
#65290=CARTESIAN_POINT('Ctrl Pts',(-18.7699215575239,14.223547590283,122.046595739492)) ;
#65291=CARTESIAN_POINT('Ctrl Pts',(-18.8977872771299,14.0435585099201,122.319642127634)) ;
#65292=CARTESIAN_POINT('Ctrl Pts',(-19.0141015690712,14.2334429882633,121.957035255779)) ;
#65293=CARTESIAN_POINT('Ctrl Pts',(-19.0931303423171,14.0534539079004,122.247993398259)) ;
#65294=CARTESIAN_POINT('Ctrl Pts',(-19.2740491001981,14.2434942208086,121.910385335695)) ;
#65295=CARTESIAN_POINT('Ctrl Pts',(-19.3010884541272,14.0635051404457,122.210672757379)) ;
#65296=CARTESIAN_POINT('Ctrl Pts',(-19.5338747027506,14.2533804114329,121.909562985904)) ;
#65297=CARTESIAN_POINT('Ctrl Pts',(-19.5089480881137,14.07339133107,122.210014195614)) ;
#65298=CARTESIAN_POINT('Ctrl Pts',(-19.7926811889532,14.2633729507487,121.953859464746)) ;
#65299=CARTESIAN_POINT('Ctrl Pts',(-19.7159932556982,14.0833838703858,122.245450559124)) ;
#65300=CARTESIAN_POINT('Ctrl Pts',(-20.0387837794866,14.2733213966434,122.042123340413)) ;
#65301=CARTESIAN_POINT('Ctrl Pts',(-19.9128751830492,14.0933323162805,122.316060778059)) ;
#65302=CARTESIAN_POINT('Ctrl Pts',(-20.2657069288235,14.2832581991753,122.171283774759)) ;
#65303=CARTESIAN_POINT('Ctrl Pts',(-20.0944136903199,14.1032691188124,122.419388116494)) ;
#65304=CARTESIAN_POINT('Ctrl Pts',(-20.4679459835233,14.2932412066266,122.338438899069)) ;
#65305=CARTESIAN_POINT('Ctrl Pts',(-20.2562053796479,14.1132521262637,122.55311135473)) ;
#65306=CARTESIAN_POINT('Ctrl Pts',(-20.6387149774407,14.3032850480414,122.539652891498)) ;
#65307=CARTESIAN_POINT('Ctrl Pts',(-20.3928213084693,14.1232959676785,122.714082124582)) ;
#65308=CARTESIAN_POINT('Ctrl Pts',(-20.7696539436816,14.3131132466653,122.762322078436)) ;
#65309=CARTESIAN_POINT('Ctrl Pts',(-20.4975727394675,14.1331241663024,122.892215983891)) ;
#65310=CARTESIAN_POINT('Ctrl Pts',(-20.8623069213888,14.3231898401075,123.010327296333)) ;
#65311=CARTESIAN_POINT('Ctrl Pts',(-20.5716961867102,14.1432007597447,123.090620129128)) ;
#65312=CARTESIAN_POINT('Ctrl Pts',(-20.909567306365,14.3330418394491,123.264936220785)) ;
#65313=CARTESIAN_POINT('Ctrl Pts',(-20.6095053328595,14.1530527590862,123.294306109493)) ;
#65314=CARTESIAN_POINT('Ctrl Pts',(-20.9121706248892,14.343115426273,123.529600919858)) ;
#65315=CARTESIAN_POINT('Ctrl Pts',(-20.6115890777029,14.1631263459101,123.506038179509)) ;
#65316=CARTESIAN_POINT('Ctrl Pts',(-20.8697248958235,14.3529556513705,123.784708643342)) ;
#65317=CARTESIAN_POINT('Ctrl Pts',(-20.5776337239948,14.1729665710076,123.710123503099)) ;
#65318=CARTESIAN_POINT('Ctrl Pts',(-20.7834156858806,14.3629213553991,124.031943418832)) ;
#65319=CARTESIAN_POINT('Ctrl Pts',(-20.5085876682656,14.1829322750362,123.907911452828)) ;
#65320=CARTESIAN_POINT('Ctrl Pts',(-20.6543560175008,14.3729479887057,124.26167893838)) ;
#65321=CARTESIAN_POINT('Ctrl Pts',(-20.405340950833,14.1929589083428,124.091700497226)) ;
#65322=CARTESIAN_POINT('Ctrl Pts',(-20.4893881315526,14.3828622844175,124.463327357308)) ;
#65323=CARTESIAN_POINT('Ctrl Pts',(-20.273367967042,14.2028732040546,124.253019557366)) ;
#65324=CARTESIAN_POINT('Ctrl Pts',(-20.29073289972,14.39285057311,124.634911409917)) ;
#65325=CARTESIAN_POINT('Ctrl Pts',(-20.1144447718736,14.2128614927471,124.390287707971)) ;
#65326=CARTESIAN_POINT('Ctrl Pts',(-20.0639385669575,14.4028893062683,124.769650931547)) ;
#65327=CARTESIAN_POINT('Ctrl Pts',(-19.933009840498,14.2229002259054,124.498080437852)) ;
#65328=CARTESIAN_POINT('Ctrl Pts',(-19.8221438934761,14.4127326380959,124.861560677325)) ;
#65329=CARTESIAN_POINT('Ctrl Pts',(-19.7395754882741,14.232743557733,124.571609123733)) ;
#65330=CARTESIAN_POINT('Ctrl Pts',(-19.5634174500474,14.4227603639755,124.911597480083)) ;
#65331=CARTESIAN_POINT('Ctrl Pts',(-19.532594551231,14.2427712836126,124.611640002553)) ;
#65332=CARTESIAN_POINT('Ctrl Pts',(-19.2997938732283,14.432792700364,124.915236180486)) ;
#65333=CARTESIAN_POINT('Ctrl Pts',(-19.3216956393782,14.2528036200011,124.614552265305)) ;
#65334=CARTESIAN_POINT('Ctrl Pts',(-19.0447452472327,14.4426222006646,124.874418148553)) ;
#65335=CARTESIAN_POINT('Ctrl Pts',(-19.1176575176957,14.2626331203018,124.581899394182)) ;
#65336=CARTESIAN_POINT('Ctrl Pts',(-18.796407103076,14.4526117045814,124.789299015739)) ;
#65337=CARTESIAN_POINT('Ctrl Pts',(-18.9189866276755,14.2726226242185,124.513805617526)) ;
#65338=CARTESIAN_POINT('Ctrl Pts',(-18.5657044122553,14.4626555450938,124.661080239922)) ;
#65339=CARTESIAN_POINT('Ctrl Pts',(-18.734423674689,14.2826664647309,124.411231794536)) ;
#65340=CARTESIAN_POINT('Ctrl Pts',(-18.3649628204512,14.4724772508619,124.498843726449)) ;
#65341=CARTESIAN_POINT('Ctrl Pts',(-18.5738302074953,14.292488170499,124.281444409)) ;
#65342=CARTESIAN_POINT('Ctrl Pts',(-18.1912720235427,14.4825122979942,124.300414746533)) ;
#65343=CARTESIAN_POINT('Ctrl Pts',(-18.4348762631959,14.3025232176314,124.122702256751)) ;
#65344=CARTESIAN_POINT('Ctrl Pts',(-18.055432254409,14.4925369754311,124.074689127998)) ;
#65345=CARTESIAN_POINT('Ctrl Pts',(-18.3262031311123,14.3125478950683,123.942122532093)) ;
#65346=CARTESIAN_POINT('Ctrl Pts',(-17.9619640242889,14.5023897902856,123.833226852752)) ;
#65347=CARTESIAN_POINT('Ctrl Pts',(-18.2514273185047,14.3224007099227,123.748954049798)) ;
#65348=CARTESIAN_POINT('Ctrl Pts',(-17.9107066774369,14.5123774998931,123.575833839664)) ;
#65349=CARTESIAN_POINT('Ctrl Pts',(-18.210419791455,14.3323884195303,123.543040117254)) ;
#65350=CARTESIAN_POINT('Ctrl Pts',(-17.9049402191342,14.5223075098872,123.314937805648)) ;
#65351=CARTESIAN_POINT('Ctrl Pts',(-18.2058049219443,14.3423184295243,123.33432374461)) ;
#65352=CARTESIAN_POINT('Ctrl Pts',(-17.9443990827381,14.5322972651064,123.055394867544)) ;
#65353=CARTESIAN_POINT('Ctrl Pts',(-18.237370231834,14.3523081847435,123.126689256779)) ;
#65354=CARTESIAN_POINT('Ctrl Pts',(-18.0289554645481,14.5423238737893,122.80583753216)) ;
#65355=CARTESIAN_POINT('Ctrl Pts',(-18.3050137161035,14.3623347934264,122.927042810016)) ;
#65356=CARTESIAN_POINT('Ctrl Pts',(-18.1535342537274,14.5522078138111,122.577928818094)) ;
#65357=CARTESIAN_POINT('Ctrl Pts',(-18.4046749159261,14.3722187334482,122.744715509039)) ;
#65358=CARTESIAN_POINT('Ctrl Pts',(-18.3170525414426,14.5621970413496,122.372560685954)) ;
#65359=CARTESIAN_POINT('Ctrl Pts',(-18.5354880122314,14.3822079609867,122.580419941737)) ;
#65360=CARTESIAN_POINT('Ctrl Pts',(-18.5151557257719,14.5722399118733,122.198188061704)) ;
#65361=CARTESIAN_POINT('Ctrl Pts',(-18.6939694414926,14.3922508315104,122.440920462388)) ;
#65362=CARTESIAN_POINT('Ctrl Pts',(-18.7355880780577,14.5820722986287,122.063388638443)) ;
#65363=CARTESIAN_POINT('Ctrl Pts',(-18.8703137118598,14.4020832182658,122.333079750593)) ;
#65364=CARTESIAN_POINT('Ctrl Pts',(-18.9797323076057,14.5920655918003,121.966658037112)) ;
#65365=CARTESIAN_POINT('Ctrl Pts',(-19.0656282824221,14.4120765114374,122.255693489777)) ;
#65366=CARTESIAN_POINT('Ctrl Pts',(-19.2380876823601,14.6020975974487,121.914120317295)) ;
#65367=CARTESIAN_POINT('Ctrl Pts',(-19.2723122376113,14.4221085170859,122.213661473719)) ;
#65368=CARTESIAN_POINT('Ctrl Pts',(-19.4972262784199,14.6119628534177,121.907034280981)) ;
#65369=CARTESIAN_POINT('Ctrl Pts',(-19.479622479628,14.4319737730548,122.207990741055)) ;
#65370=CARTESIAN_POINT('Ctrl Pts',(-19.7562992627137,14.6219247333252,121.944692330567)) ;
#65371=CARTESIAN_POINT('Ctrl Pts',(-19.6868809582063,14.4419356529623,122.238115153452)) ;
#65372=CARTESIAN_POINT('Ctrl Pts',(-20.0065648350329,14.6319596666871,122.027765848265)) ;
#65373=CARTESIAN_POINT('Ctrl Pts',(-19.8870940599284,14.4519705863242,122.304572113767)) ;
#65374=CARTESIAN_POINT('Ctrl Pts',(-20.2353895991265,14.6418446250664,122.150798715635)) ;
#65375=CARTESIAN_POINT('Ctrl Pts',(-20.0701544291512,14.4618555447035,122.402996417728)) ;
#65376=CARTESIAN_POINT('Ctrl Pts',(-20.4430039039663,14.6519102519891,122.314630587451)) ;
#65377=CARTESIAN_POINT('Ctrl Pts',(-20.2362472126455,14.4719211716262,122.534060408975)) ;
#65378=CARTESIAN_POINT('Ctrl Pts',(-20.6153099874822,14.6617493576534,122.507469086936)) ;
#65379=CARTESIAN_POINT('Ctrl Pts',(-20.3740932248574,14.4817602772905,122.688329427988)) ;
#65380=CARTESIAN_POINT('Ctrl Pts',(-20.7548702754188,14.6718121726588,122.732041086105)) ;
#65381=CARTESIAN_POINT('Ctrl Pts',(-20.4857432796024,14.4918230922959,122.867986018619)) ;
#65382=CARTESIAN_POINT('Ctrl Pts',(-20.8514895076296,14.6817083787074,122.973518167656)) ;
#65383=CARTESIAN_POINT('Ctrl Pts',(-20.5630404332213,14.5017192983446,123.061166569921)) ;
#65384=CARTESIAN_POINT('Ctrl Pts',(-20.905652298732,14.6916492017327,123.229045388477)) ;
#65385=CARTESIAN_POINT('Ctrl Pts',(-20.6063727060311,14.5116601213698,123.265587688841)) ;
#65386=CARTESIAN_POINT('Ctrl Pts',(-20.9147482972179,14.7016537847114,123.49182757385)) ;
#65387=CARTESIAN_POINT('Ctrl Pts',(-20.6136516339194,14.5216647043485,123.475813306976)) ;
#65388=CARTESIAN_POINT('Ctrl Pts',(-20.8777060565819,14.7116746791561,123.752541737872)) ;
#65389=CARTESIAN_POINT('Ctrl Pts',(-20.584019929086,14.5316855987932,123.684384908824)) ;
#65390=CARTESIAN_POINT('Ctrl Pts',(-20.7973137583484,14.7215665997455,123.999754867603)) ;
#65391=CARTESIAN_POINT('Ctrl Pts',(-20.5197082201853,14.5415775193826,123.882155761826)) ;
#65392=CARTESIAN_POINT('Ctrl Pts',(-20.6743041569518,14.7315600320909,124.231770792966)) ;
#65393=CARTESIAN_POINT('Ctrl Pts',(-20.4213024934147,14.551570951728,124.067769440875)) ;
#65394=CARTESIAN_POINT('Ctrl Pts',(-20.5135786631871,14.7415056369908,124.437867633095)) ;
#65395=CARTESIAN_POINT('Ctrl Pts',(-20.2927239143119,14.5615165566279,124.232648095339)) ;
#65396=CARTESIAN_POINT('Ctrl Pts',(-20.3198218573511,14.7514529104723,124.613360457444)) ;
#65397=CARTESIAN_POINT('Ctrl Pts',(-20.137720063294,14.5714638301094,124.373043875978)) ;
#65398=CARTESIAN_POINT('Ctrl Pts',(-20.0961599099383,14.7615008249487,124.753689774848)) ;
#65399=CARTESIAN_POINT('Ctrl Pts',(-19.9587916558263,14.5815117445858,124.485309178269)) ;
#65400=CARTESIAN_POINT('Ctrl Pts',(-19.8564776376663,14.771348465296,124.851279444888)) ;
#65401=CARTESIAN_POINT('Ctrl Pts',(-19.7670469592938,14.5913593849331,124.563382825184)) ;
#65402=CARTESIAN_POINT('Ctrl Pts',(-19.6007489896213,14.7813101806726,124.907199618394)) ;
#65403=CARTESIAN_POINT('Ctrl Pts',(-19.5624646160184,14.6013211003097,124.608121129999)) ;
#65404=CARTESIAN_POINT('Ctrl Pts',(-19.3373962978428,14.7913388042454,124.917606836282)) ;
#65405=CARTESIAN_POINT('Ctrl Pts',(-19.3517825852773,14.6113497238825,124.616449119218)) ;
#65406=CARTESIAN_POINT('Ctrl Pts',(-19.0793336231031,14.8012491663118,124.882634265756)) ;
#65407=CARTESIAN_POINT('Ctrl Pts',(-19.1453323129572,14.6212600859489,124.58847329103)) ;
#65408=CARTESIAN_POINT('Ctrl Pts',(-18.8304237660988,14.8111838599642,124.803839977348)) ;
#65409=CARTESIAN_POINT('Ctrl Pts',(-18.9462038486766,14.6311947796013,124.52544003625)) ;
#65410=CARTESIAN_POINT('Ctrl Pts',(-18.5966220485025,14.8212257030921,124.681499373881)) ;
#65411=CARTESIAN_POINT('Ctrl Pts',(-18.7591614689245,14.6412366227292,124.427569556202)) ;
#65412=CARTESIAN_POINT('Ctrl Pts',(-18.390716860511,14.8311102086625,124.523104155642)) ;
#65413=CARTESIAN_POINT('Ctrl Pts',(-18.5944360498318,14.6511211282996,124.300855240205)) ;
#65414=CARTESIAN_POINT('Ctrl Pts',(-18.2131739736385,14.8411123124477,124.329336878928)) ;
#65415=CARTESIAN_POINT('Ctrl Pts',(-18.4524001167752,14.6611232320848,124.145842979682)) ;
#65416=CARTESIAN_POINT('Ctrl Pts',(-18.0729290956816,14.8510306638627,124.109588770675)) ;
#65417=CARTESIAN_POINT('Ctrl Pts',(-18.3402023497202,14.6710415834998,123.970045780687)) ;
#65418=CARTESIAN_POINT('Ctrl Pts',(-17.9717628132547,14.8610783198836,123.865741080711)) ;
#65419=CARTESIAN_POINT('Ctrl Pts',(-18.2592672790845,14.6810892395207,123.774968483768)) ;
#65420=CARTESIAN_POINT('Ctrl Pts',(-17.9151745106479,14.8709495129118,123.612528140335)) ;
#65421=CARTESIAN_POINT('Ctrl Pts',(-18.2139943885735,14.6909604325489,123.572398901037)) ;
#65422=CARTESIAN_POINT('Ctrl Pts',(-17.9031429831484,14.8810152260553,123.34834743098)) ;
#65423=CARTESIAN_POINT('Ctrl Pts',(-18.204367144922,14.7010261456924,123.361053634231)) ;
#65424=CARTESIAN_POINT('Ctrl Pts',(-17.9361624249687,14.890867686628,123.091474379834)) ;
#65425=CARTESIAN_POINT('Ctrl Pts',(-18.2307796125064,14.7108786062651,123.155558165158)) ;
#65426=CARTESIAN_POINT('Ctrl Pts',(-18.0413449335706,14.9042961493505,122.754742299802)) ;
#65427=CARTESIAN_POINT('Ctrl Pts',(-18.3149269800469,14.7243070689876,122.88615548597)) ;
#65428=CARTESIAN_POINT('Ctrl Pts',(-18.2267874470069,14.9173770968676,122.460483907588)) ;
#65429=CARTESIAN_POINT('Ctrl Pts',(-18.4633001749267,14.7373880165047,122.65073212564)) ;
#65430=CARTESIAN_POINT('Ctrl Pts',(-18.4863543902938,14.9308515951022,122.219747666857)) ;
#65431=CARTESIAN_POINT('Ctrl Pts',(-18.6709215324032,14.7508625147393,122.458175060593)) ;
#65432=CARTESIAN_POINT('Ctrl Pts',(-18.7036544341988,14.9406836987116,122.079886991967)) ;
#65433=CARTESIAN_POINT('Ctrl Pts',(-18.8447666073225,14.7606946183488,122.346277773026)) ;
#65434=CARTESIAN_POINT('Ctrl Pts',(-18.9446987351203,14.9506496018383,121.977572951031)) ;
#65435=CARTESIAN_POINT('Ctrl Pts',(-19.0375992137508,14.7706605214754,122.264426179784)) ;
#65436=CARTESIAN_POINT('Ctrl Pts',(-19.2015765911018,14.9606770111485,121.918685704724)) ;
#65437=CARTESIAN_POINT('Ctrl Pts',(-19.2431028113862,14.7806879307857,122.217314368209)) ;
#65438=CARTESIAN_POINT('Ctrl Pts',(-19.4616556588049,14.9705880425151,121.905384721623)) ;
#65439=CARTESIAN_POINT('Ctrl Pts',(-19.4511604538144,14.7905989621522,122.206669246989)) ;
#65440=CARTESIAN_POINT('Ctrl Pts',(-19.8072618039374,14.9838323501362,121.947128778354)) ;
#65441=CARTESIAN_POINT('Ctrl Pts',(-19.7276732696558,14.8038432697733,122.24007284524)) ;
#65442=CARTESIAN_POINT('Ctrl Pts',(-20.2188550941679,15.0005328328073,122.113045312188)) ;
#65443=CARTESIAN_POINT('Ctrl Pts',(-20.0569081396409,14.8205437524445,122.372778876184)) ;
#65444=CARTESIAN_POINT('Ctrl Pts',(-20.5455679441702,15.0170396619631,122.405960959497)) ;
#65445=CARTESIAN_POINT('Ctrl Pts',(-20.3183298372832,14.8370505816002,122.607156832751)) ;
#65446=CARTESIAN_POINT('Ctrl Pts',(-20.7373262391937,15.0303502902007,122.698457845509)) ;
#65447=CARTESIAN_POINT('Ctrl Pts',(-20.4717022185341,14.8503612098378,122.841112812095)) ;
#65448=CARTESIAN_POINT('Ctrl Pts',(-20.8410482037776,15.0403428537408,122.939743261889)) ;
#65449=CARTESIAN_POINT('Ctrl Pts',(-20.5546889224827,14.8603537733779,123.034149304461)) ;
#65450=CARTESIAN_POINT('Ctrl Pts',(-20.9012011780977,15.0503729367423,123.196334518998)) ;
#65451=CARTESIAN_POINT('Ctrl Pts',(-20.6028117682902,14.8703838563795,123.239415751326)) ;
#65452=CARTESIAN_POINT('Ctrl Pts',(-20.9212136813736,15.0635465407401,123.542009444152)) ;
#65453=CARTESIAN_POINT('Ctrl Pts',(-20.6188231356047,14.8835574603772,123.515975765134)) ;
#65454=CARTESIAN_POINT('Ctrl Pts',(-20.8322977307926,15.0801842459715,123.97501211203)) ;
#65455=CARTESIAN_POINT('Ctrl Pts',(-20.5476923868234,14.9001951656086,123.862358789437)) ;
#65456=CARTESIAN_POINT('Ctrl Pts',(-20.5559470864143,15.1000660085389,124.425649304088)) ;
#65457=CARTESIAN_POINT('Ctrl Pts',(-20.3266297541307,14.9200769281761,124.222868808078)) ;
#65458=CARTESIAN_POINT('Ctrl Pts',(-20.2087222530336,15.1167623607554,124.70175262575)) ;
#65459=CARTESIAN_POINT('Ctrl Pts',(-20.0488038623269,14.9367732803926,124.443780904704)) ;
#65460=CARTESIAN_POINT('Ctrl Pts',(-19.8917080630513,15.1299193885445,124.839949683673)) ;
#65461=CARTESIAN_POINT('Ctrl Pts',(-19.7952369425697,14.9499303081817,124.554316138444)) ;
#65462=CARTESIAN_POINT('Ctrl Pts',(-19.5501536847632,15.1432967431881,124.92300774244)) ;
#65463=CARTESIAN_POINT('Ctrl Pts',(-19.5219730467639,14.9633076628252,124.620769728734)) ;
#65464=CARTESIAN_POINT('Ctrl Pts',(-19.1108554066313,15.1598275774469,124.912748434119)) ;
#65465=CARTESIAN_POINT('Ctrl Pts',(-19.170551068665,14.979838497084,124.612563667479)) ;
#65466=CARTESIAN_POINT('Ctrl Pts',(-18.616168502824,15.17979226719,124.720920100906)) ;
#65467=CARTESIAN_POINT('Ctrl Pts',(-18.7747945577077,14.9998031868271,124.45910447757)) ;
#65468=CARTESIAN_POINT('Ctrl Pts',(-18.2178819295255,15.1997087606136,124.372224270615)) ;
#65469=CARTESIAN_POINT('Ctrl Pts',(-18.4561642627655,15.0197196802507,124.180149816018)) ;
#65470=CARTESIAN_POINT('Ctrl Pts',(-17.9618943674429,15.2195984799632,123.909642300137)) ;
#65471=CARTESIAN_POINT('Ctrl Pts',(-18.2513709039393,15.0396093996003,123.810084995758)) ;
#65472=CARTESIAN_POINT('Ctrl Pts',(-17.8790867340295,15.239605209611,123.384461553137)) ;
#65473=CARTESIAN_POINT('Ctrl Pts',(-18.1851220450662,15.0596161292481,123.389940905044)) ;
#65474=CARTESIAN_POINT('Ctrl Pts',(-17.9792551414852,15.2594432632579,122.866690154571)) ;
#65475=CARTESIAN_POINT('Ctrl Pts',(-18.2652543890131,15.079454182895,122.975722039237)) ;
#65476=CARTESIAN_POINT('Ctrl Pts',(-18.2516493430185,15.2794366014715,122.410539526417)) ;
#65477=CARTESIAN_POINT('Ctrl Pts',(-18.4831677681727,15.0994475211086,122.610800270065)) ;
#65478=CARTESIAN_POINT('Ctrl Pts',(-18.661435692982,15.2993194008781,122.076711965965)) ;
#65479=CARTESIAN_POINT('Ctrl Pts',(-18.8109961779416,15.1193303205152,122.34373578517)) ;
#65480=CARTESIAN_POINT('Ctrl Pts',(-19.1602442446391,15.3192115817968,121.901912195536)) ;
#65481=CARTESIAN_POINT('Ctrl Pts',(-19.2100434562284,15.1392225014339,122.203893842988)) ;
#65482=CARTESIAN_POINT('Ctrl Pts',(-19.6893450348153,15.3391137602919,121.906937811211)) ;
#65483=CARTESIAN_POINT('Ctrl Pts',(-19.6333250670439,15.159124679929,122.207913017499)) ;
#65484=CARTESIAN_POINT('Ctrl Pts',(-20.1877316480936,15.3591510714956,122.094234259217)) ;
#65485=CARTESIAN_POINT('Ctrl Pts',(-20.0320345164081,15.1791619911328,122.357748581197)) ;
#65486=CARTESIAN_POINT('Ctrl Pts',(-20.5885091138174,15.3789635130365,122.4361550605)) ;
#65487=CARTESIAN_POINT('Ctrl Pts',(-20.352658713179,15.1989744326736,122.631285748145)) ;
#65488=CARTESIAN_POINT('Ctrl Pts',(-20.8514802727897,15.3990287537714,122.899819819407)) ;
#65489=CARTESIAN_POINT('Ctrl Pts',(-20.5630361534512,15.2190396734085,123.002216473756)) ;
#65490=CARTESIAN_POINT('Ctrl Pts',(-20.939569466923,15.4187859586272,123.417748054594)) ;
#65491=CARTESIAN_POINT('Ctrl Pts',(-20.6335085384984,15.2387968782644,123.416561832562)) ;
#65492=CARTESIAN_POINT('Ctrl Pts',(-20.8451846342489,15.4388192312729,123.941494843128)) ;
#65493=CARTESIAN_POINT('Ctrl Pts',(-20.5580007277665,15.2588301509101,123.835558979513)) ;
#65494=CARTESIAN_POINT('Ctrl Pts',(-20.5803681949361,15.4586321397268,124.396932991369)) ;
#65495=CARTESIAN_POINT('Ctrl Pts',(-20.3461462373689,15.2786430593639,124.199911406604)) ;
#65496=CARTESIAN_POINT('Ctrl Pts',(-20.1731096405733,15.4786282858542,124.738024765008)) ;
#65497=CARTESIAN_POINT('Ctrl Pts',(-20.0203388220478,15.2986392054913,124.472784322776)) ;
#65498=CARTESIAN_POINT('Ctrl Pts',(-19.6769061894164,15.4984900390767,124.918856330261)) ;
#65499=CARTESIAN_POINT('Ctrl Pts',(-19.6233743087396,15.3185009587138,124.617449135294)) ;
#65500=CARTESIAN_POINT('Ctrl Pts',(-19.1436360482035,15.5185585562048,124.919177517765)) ;
#65501=CARTESIAN_POINT('Ctrl Pts',(-19.1967589767419,15.3385694758419,124.617705010039)) ;
#65502=CARTESIAN_POINT('Ctrl Pts',(-18.6481039856445,15.5383894292016,124.739248841471)) ;
#65503=CARTESIAN_POINT('Ctrl Pts',(-18.8003319653689,15.3584003488387,124.473760421146)) ;
#65504=CARTESIAN_POINT('Ctrl Pts',(-18.2411262734598,15.5583113400183,124.400722475563)) ;
#65505=CARTESIAN_POINT('Ctrl Pts',(-18.4747503480826,15.3783222596554,124.202937369334)) ;
#65506=CARTESIAN_POINT('Ctrl Pts',(-17.9740267390617,15.5782407834536,123.943204335233)) ;
#65507=CARTESIAN_POINT('Ctrl Pts',(-18.2610720716113,15.3982517030907,123.836921334488)) ;
#65508=CARTESIAN_POINT('Ctrl Pts',(-17.8790194223619,15.59815045357,123.422718308582)) ;
#65509=CARTESIAN_POINT('Ctrl Pts',(-18.1850681984714,15.4181613732071,123.42053129134)) ;
#65510=CARTESIAN_POINT('Ctrl Pts',(-17.9662605748662,15.6180238108329,122.901708304058)) ;
#65511=CARTESIAN_POINT('Ctrl Pts',(-18.254863873094,15.43803473047,123.00372270003)) ;
#65512=CARTESIAN_POINT('Ctrl Pts',(-18.2276238439571,15.6380153454508,122.439173769157)) ;
#65513=CARTESIAN_POINT('Ctrl Pts',(-18.4639568825122,15.4580262650879,122.633696362136)) ;
#65514=CARTESIAN_POINT('Ctrl Pts',(-18.6285678009232,15.6578809628615,122.095505124988)) ;
#65515=CARTESIAN_POINT('Ctrl Pts',(-18.7847146580216,15.4778918824987,122.358763014861)) ;
#65516=CARTESIAN_POINT('Ctrl Pts',(-19.1253095706751,15.6778618926898,121.907746174012)) ;
#65517=CARTESIAN_POINT('Ctrl Pts',(-19.1821092675839,15.4978728123269,122.208558782164)) ;
#65518=CARTESIAN_POINT('Ctrl Pts',(-19.6552143908038,15.6978003547729,121.901373660419)) ;
#65519=CARTESIAN_POINT('Ctrl Pts',(-19.6060335509028,15.51781127441,122.203463873449)) ;
#65520=CARTESIAN_POINT('Ctrl Pts',(-20.1546433032014,15.7176925479946,122.075043824401)) ;
#65521=CARTESIAN_POINT('Ctrl Pts',(-20.0055761682767,15.5377034676318,122.342403428384)) ;
#65522=CARTESIAN_POINT('Ctrl Pts',(-20.5661496331982,15.73766326303,122.410119645807)) ;
#65523=CARTESIAN_POINT('Ctrl Pts',(-20.3347791384015,15.5576741826671,122.610466906619)) ;
#65524=CARTESIAN_POINT('Ctrl Pts',(-20.8373123753955,15.7574729346961,122.861577302707)) ;
#65525=CARTESIAN_POINT('Ctrl Pts',(-20.5517067350592,15.5774838543332,122.97163565789)) ;
#65526=CARTESIAN_POINT('Ctrl Pts',(-20.9393997364478,15.7774661513873,123.382866096592)) ;
#65527=CARTESIAN_POINT('Ctrl Pts',(-20.6333723462591,15.5974770710244,123.388667788783)) ;
#65528=CARTESIAN_POINT('Ctrl Pts',(-20.8584216081124,15.7973170635836,123.904440437728)) ;
#65529=CARTESIAN_POINT('Ctrl Pts',(-20.5685874513888,15.6173279832208,123.805925914107)) ;
#65530=CARTESIAN_POINT('Ctrl Pts',(-20.6013666268889,15.8173916699027,124.371819409561)) ;
#65531=CARTESIAN_POINT('Ctrl Pts',(-20.3629338879566,15.6374025895398,124.17983155202)) ;
#65532=CARTESIAN_POINT('Ctrl Pts',(-20.2709357008999,15.833908301786,124.661071335312)) ;
#65533=CARTESIAN_POINT('Ctrl Pts',(-20.098605819619,15.6539192214231,124.411216220692)) ;
#65534=CARTESIAN_POINT('Ctrl Pts',(-19.9567400193657,15.8472470094801,124.816295036982)) ;
#65535=CARTESIAN_POINT('Ctrl Pts',(-19.8472304865429,15.6672579291172,124.535405548964)) ;
#65536=CARTESIAN_POINT('Ctrl Pts',(-19.7085577801769,15.8570893837884,124.889269258747)) ;
#65537=CARTESIAN_POINT('Ctrl Pts',(-19.6486898643955,15.6771003034255,124.593781066732)) ;
#65538=CARTESIAN_POINT('Ctrl Pts',(-19.4460289923727,15.8671444037711,124.918903925048)) ;
#65539=CARTESIAN_POINT('Ctrl Pts',(-19.438655254333,15.6871553234083,124.617484843905)) ;
#65540=CARTESIAN_POINT('Ctrl Pts',(-19.0989283678214,15.8803765604287,124.897309206157)) ;
#65541=CARTESIAN_POINT('Ctrl Pts',(-19.1610280086618,15.7003874800658,124.600218444694)) ;
#65542=CARTESIAN_POINT('Ctrl Pts',(-18.680086550223,15.8969915277738,124.757481852894)) ;
#65543=CARTESIAN_POINT('Ctrl Pts',(-18.8258890338263,15.717002447411,124.488333567479)) ;
#65544=CARTESIAN_POINT('Ctrl Pts',(-18.3346327392559,15.913586114785,124.48329340641)) ;
#65545=CARTESIAN_POINT('Ctrl Pts',(-18.549571248321,15.7335970344222,124.26900587412)) ;
#65546=CARTESIAN_POINT('Ctrl Pts',(-18.1268897362054,15.9268196831404,124.204366870051)) ;
#65547=CARTESIAN_POINT('Ctrl Pts',(-18.3833541247988,15.7468306027775,124.045842691326)) ;
#65548=CARTESIAN_POINT('Ctrl Pts',(-18.0083439444997,15.9368633009491,123.968576154149)) ;
#65549=CARTESIAN_POINT('Ctrl Pts',(-18.288524508184,15.7568742205862,123.857213407479)) ;
#65550=CARTESIAN_POINT('Ctrl Pts',(-17.9336253681816,15.9467502251839,123.719711066793)) ;
#65551=CARTESIAN_POINT('Ctrl Pts',(-18.228750615402,15.766761144821,123.658118921018)) ;
#65552=CARTESIAN_POINT('Ctrl Pts',(-17.9024744065932,15.9567408796307,123.459039355824)) ;
#65553=CARTESIAN_POINT('Ctrl Pts',(-18.2038316647778,15.7767517992678,123.44958390152)) ;
#65554=CARTESIAN_POINT('Ctrl Pts',(-17.9170694041595,15.9667026380847,123.197660756749)) ;
#65555=CARTESIAN_POINT('Ctrl Pts',(-18.2155127307376,15.7867135577218,123.240472575159)) ;
#65556=CARTESIAN_POINT('Ctrl Pts',(-17.9967391763496,15.9800425031519,122.856207482281)) ;
#65557=CARTESIAN_POINT('Ctrl Pts',(-18.2792369334935,15.800053422789,122.967353118238)) ;
#65558=CARTESIAN_POINT('Ctrl Pts',(-18.1639736695918,15.9933512860652,122.544568270991)) ;
#65559=CARTESIAN_POINT('Ctrl Pts',(-18.4130291807897,15.8133622057023,122.718017643817)) ;
#65560=CARTESIAN_POINT('Ctrl Pts',(-18.4009205226991,16.0065470435093,122.291373958012)) ;
#65561=CARTESIAN_POINT('Ctrl Pts',(-18.6026009981143,15.8265579631464,122.515452269556)) ;
#65562=CARTESIAN_POINT('Ctrl Pts',(-18.6098352782094,16.0165089271858,122.133609050801)) ;
#65563=CARTESIAN_POINT('Ctrl Pts',(-18.7697316665217,15.8365198468229,122.389244599765)) ;
#65564=CARTESIAN_POINT('Ctrl Pts',(-18.8450601920169,16.0265520367004,122.013933523829)) ;
#65565=CARTESIAN_POINT('Ctrl Pts',(-18.9579132372001,15.8465629563375,122.293505565848)) ;
#65566=CARTESIAN_POINT('Ctrl Pts',(-19.0926161288735,16.0364042866996,121.938083702946)) ;
#65567=CARTESIAN_POINT('Ctrl Pts',(-19.1559583816547,15.8564152063368,122.232828069619)) ;
#65568=CARTESIAN_POINT('Ctrl Pts',(-19.3525761374353,16.0463758236501,121.90535120371)) ;
#65569=CARTESIAN_POINT('Ctrl Pts',(-19.3639266242928,15.8663867432872,122.206644267402)) ;
#65570=CARTESIAN_POINT('Ctrl Pts',(-19.6149622143192,16.0563710891276,121.918309627861)) ;
#65571=CARTESIAN_POINT('Ctrl Pts',(-19.5738352989783,15.8763820087648,122.217013257549)) ;
#65572=CARTESIAN_POINT('Ctrl Pts',(-19.8719707676213,16.0664050620013,121.977157725234)) ;
#65573=CARTESIAN_POINT('Ctrl Pts',(-19.7794416116365,15.8864159816384,122.264093925763)) ;
#65574=CARTESIAN_POINT('Ctrl Pts',(-20.1107386746183,16.0762604767636,122.077550542983)) ;
#65575=CARTESIAN_POINT('Ctrl Pts',(-19.9704548934143,15.8962713964007,122.344410174474)) ;
#65576=CARTESIAN_POINT('Ctrl Pts',(-20.3317609231274,16.0862597542724,122.219585083318)) ;
#65577=CARTESIAN_POINT('Ctrl Pts',(-20.1472714239141,15.9062706739096,122.458039646496)) ;
#65578=CARTESIAN_POINT('Ctrl Pts',(-20.5230102658078,16.0961549384354,122.395838020282)) ;
#65579=CARTESIAN_POINT('Ctrl Pts',(-20.3002692442417,15.9161658580725,122.599043480994)) ;
#65580=CARTESIAN_POINT('Ctrl Pts',(-20.6833117694189,16.1062153180762,122.606026601043)) ;
#65581=CARTESIAN_POINT('Ctrl Pts',(-20.4285086974711,15.9262262377133,122.76719571147)) ;
#65582=CARTESIAN_POINT('Ctrl Pts',(-20.8023123453152,16.1160651870843,122.835923343469)) ;
#65583=CARTESIAN_POINT('Ctrl Pts',(-20.5237070533521,15.9360761067214,122.951113839647)) ;
#65584=CARTESIAN_POINT('Ctrl Pts',(-20.8815749658397,16.1260967482922,123.087326542233)) ;
#65585=CARTESIAN_POINT('Ctrl Pts',(-20.5871150742216,15.9461076679293,123.152237028848)) ;
#65586=CARTESIAN_POINT('Ctrl Pts',(-20.9153886455586,16.1361071971745,123.3482327168)) ;
#65587=CARTESIAN_POINT('Ctrl Pts',(-20.6141638267646,15.9561181168116,123.360962211071)) ;
#65588=CARTESIAN_POINT('Ctrl Pts',(-20.9038000062041,16.1460139365915,123.608304860459)) ;
#65589=CARTESIAN_POINT('Ctrl Pts',(-20.604890742972,15.9660248562286,123.569019582891)) ;
#65590=CARTESIAN_POINT('Ctrl Pts',(-20.8475493442764,16.1559519526599,123.863320444448)) ;
#65591=CARTESIAN_POINT('Ctrl Pts',(-20.5598881638927,15.9759628722971,123.773031376224)) ;
#65592=CARTESIAN_POINT('Ctrl Pts',(-20.7473434745622,16.1659571991111,124.106434248665)) ;
#65593=CARTESIAN_POINT('Ctrl Pts',(-20.4797215247247,15.9859681187482,123.967521547182)) ;
#65594=CARTESIAN_POINT('Ctrl Pts',(-20.6056840713685,16.1759912601674,124.328819428175)) ;
#65595=CARTESIAN_POINT('Ctrl Pts',(-20.3663921647497,15.9960021798045,124.145428536233)) ;
#65596=CARTESIAN_POINT('Ctrl Pts',(-20.4312280688443,16.1858363412255,124.519891626386)) ;
#65597=CARTESIAN_POINT('Ctrl Pts',(-20.2268260969221,16.0058472608626,124.298284524298)) ;
#65598=CARTESIAN_POINT('Ctrl Pts',(-20.2236607634961,16.195822147179,124.680379963816)) ;
#65599=CARTESIAN_POINT('Ctrl Pts',(-20.0607710803416,16.0158330668161,124.426673466983)) ;
#65600=CARTESIAN_POINT('Ctrl Pts',(-19.9925740517516,16.2057569677332,124.801974564811)) ;
#65601=CARTESIAN_POINT('Ctrl Pts',(-19.8759009849248,16.0257678873703,124.523947205164)) ;
#65602=CARTESIAN_POINT('Ctrl Pts',(-19.7408239243177,16.2158144928654,124.88232980859)) ;
#65603=CARTESIAN_POINT('Ctrl Pts',(-19.674500158399,16.0358254125025,124.588229439226)) ;
#65604=CARTESIAN_POINT('Ctrl Pts',(-19.4850756391553,16.2256361435168,124.917322735119)) ;
#65605=CARTESIAN_POINT('Ctrl Pts',(-19.4699018773493,16.0456470631539,124.616221674339)) ;
#65606=CARTESIAN_POINT('Ctrl Pts',(-19.2210119356238,16.2356922070215,124.90763544783)) ;
#65607=CARTESIAN_POINT('Ctrl Pts',(-19.258650898185,16.0557031266586,124.608469860502)) ;
#65608=CARTESIAN_POINT('Ctrl Pts',(-18.965674000184,16.2456328740854,124.852413667813)) ;
#65609=CARTESIAN_POINT('Ctrl Pts',(-19.0543812431617,16.0656437937226,124.564290497931)) ;
#65610=CARTESIAN_POINT('Ctrl Pts',(-18.7243829673979,16.2555372677514,124.754815092852)) ;
#65611=CARTESIAN_POINT('Ctrl Pts',(-18.8613495382106,16.0755481873885,124.486210004982)) ;
#65612=CARTESIAN_POINT('Ctrl Pts',(-18.5006518515227,16.2655837915144,124.614693286642)) ;
#65613=CARTESIAN_POINT('Ctrl Pts',(-18.6823656136091,16.0855947111516,124.374110855756)) ;
#65614=CARTESIAN_POINT('Ctrl Pts',(-18.3073636533246,16.2754798745308,124.440639733717)) ;
#65615=CARTESIAN_POINT('Ctrl Pts',(-18.5277366902723,16.0954907941679,124.234866901715)) ;
#65616=CARTESIAN_POINT('Ctrl Pts',(-18.1445816442607,16.2855465737608,124.232170442766)) ;
#65617=CARTESIAN_POINT('Ctrl Pts',(-18.3975125052179,16.105557493398,124.068090149545)) ;
#65618=CARTESIAN_POINT('Ctrl Pts',(-18.0231616074987,16.2953701841619,124.004307681981)) ;
#65619=CARTESIAN_POINT('Ctrl Pts',(-18.3003785015697,16.115381103799,123.885799728941)) ;
#65620=CARTESIAN_POINT('Ctrl Pts',(-17.9408403240638,16.3054260443394,123.753235338654)) ;
#65621=CARTESIAN_POINT('Ctrl Pts',(-18.2345231623342,16.1254369639765,123.684941163944)) ;
#65622=CARTESIAN_POINT('Ctrl Pts',(-17.904145201317,16.3153591906443,123.494762458891)) ;
#65623=CARTESIAN_POINT('Ctrl Pts',(-18.2051689666766,16.1353701102815,123.478162945526)) ;
#65624=CARTESIAN_POINT('Ctrl Pts',(-17.9123613233359,16.3253044464149,123.233570994404)) ;
#65625=CARTESIAN_POINT('Ctrl Pts',(-18.2117436421572,16.1453153660521,123.269210168122)) ;
#65626=CARTESIAN_POINT('Ctrl Pts',(-17.9658149650056,16.3352877448534,122.976690048544)) ;
#65627=CARTESIAN_POINT('Ctrl Pts',(-18.2545082370437,16.1552986644905,123.063705923525)) ;
#65628=CARTESIAN_POINT('Ctrl Pts',(-18.0638986666255,16.345324925,122.731859880856)) ;
#65629=CARTESIAN_POINT('Ctrl Pts',(-18.3329769087346,16.1653358446372,122.867842396204)) ;
#65630=CARTESIAN_POINT('Ctrl Pts',(-18.2001537297579,16.3551794777095,122.511606700127)) ;
#65631=CARTESIAN_POINT('Ctrl Pts',(-18.4419820544397,16.1751903973466,122.691641395589)) ;
#65632=CARTESIAN_POINT('Ctrl Pts',(-18.3747984971053,16.3651789961568,122.315323705892)) ;
#65633=CARTESIAN_POINT('Ctrl Pts',(-18.5816990552253,16.185189915794,122.534616199794)) ;
#65634=CARTESIAN_POINT('Ctrl Pts',(-18.5786176379803,16.3750740786189,122.153776522294)) ;
#65635=CARTESIAN_POINT('Ctrl Pts',(-18.7447549194951,16.195084998256,122.405380095778)) ;
#65636=CARTESIAN_POINT('Ctrl Pts',(-18.8111591522696,16.385134624125,122.028064933009)) ;
#65637=CARTESIAN_POINT('Ctrl Pts',(-18.9307890798417,16.2051455437621,122.304812173805)) ;
#65638=CARTESIAN_POINT('Ctrl Pts',(-19.0567347651697,16.394983931373,121.946236873333)) ;
#65639=CARTESIAN_POINT('Ctrl Pts',(-19.1272492874052,16.2149948510101,122.239351517279)) ;
#65640=CARTESIAN_POINT('Ctrl Pts',(-19.3172847594668,16.4050110214604,121.906948036796)) ;
#65641=CARTESIAN_POINT('Ctrl Pts',(-19.3356895344519,16.2250219410975,122.207921911425)) ;
#65642=CARTESIAN_POINT('Ctrl Pts',(-19.5807454043777,16.4150399255973,121.91419747043)) ;
#65643=CARTESIAN_POINT('Ctrl Pts',(-19.5464580626688,16.2350508452344,122.213723077586)) ;
#65644=CARTESIAN_POINT('Ctrl Pts',(-19.8342636546748,16.4248837906966,121.965599859095)) ;
#65645=CARTESIAN_POINT('Ctrl Pts',(-19.7492714785227,16.2448947103337,122.254846299181)) ;
#65646=CARTESIAN_POINT('Ctrl Pts',(-20.0789676317228,16.434879617405,122.0611017389)) ;
#65647=CARTESIAN_POINT('Ctrl Pts',(-19.9450340249279,16.2548905370421,122.331249046834)) ;
#65648=CARTESIAN_POINT('Ctrl Pts',(-20.3037842341569,16.444904834054,122.198459857618)) ;
#65649=CARTESIAN_POINT('Ctrl Pts',(-20.1248865660534,16.2649157536911,122.441136831011)) ;
#65650=CARTESIAN_POINT('Ctrl Pts',(-20.4988993121104,16.4547946662116,122.370150559373)) ;
#65651=CARTESIAN_POINT('Ctrl Pts',(-20.2809771772072,16.2748055858487,122.578490004565)) ;
#65652=CARTESIAN_POINT('Ctrl Pts',(-20.6631697043296,16.4647855222963,122.574949866266)) ;
#65653=CARTESIAN_POINT('Ctrl Pts',(-20.4123923501296,16.2847964419335,122.742330173249)) ;
#65654=CARTESIAN_POINT('Ctrl Pts',(-20.7887677400445,16.4747306168892,122.804137700936)) ;
#65655=CARTESIAN_POINT('Ctrl Pts',(-20.512869395449,16.2947415365263,122.925680738138)) ;
#65656=CARTESIAN_POINT('Ctrl Pts',(-20.8731883104183,16.4846825206573,123.051673973059)) ;
#65657=CARTESIAN_POINT('Ctrl Pts',(-20.5804045428109,16.3046934402944,123.123709795798)) ;
#65658=CARTESIAN_POINT('Ctrl Pts',(-20.9134563188917,16.4947189201267,123.312320962728)) ;
#65659=CARTESIAN_POINT('Ctrl Pts',(-20.612617681498,16.3147298397639,123.332227690102)) ;
#65660=CARTESIAN_POINT('Ctrl Pts',(-20.9081282976239,16.5046079902154,123.572149884728)) ;
#65661=CARTESIAN_POINT('Ctrl Pts',(-20.6083540200427,16.3246189098525,123.540090066167)) ;
#65662=CARTESIAN_POINT('Ctrl Pts',(-20.8577220598271,16.5145972795863,123.829766727629)) ;
#65663=CARTESIAN_POINT('Ctrl Pts',(-20.5680279279272,16.3346081992234,123.746183149683)) ;
#65664=CARTESIAN_POINT('Ctrl Pts',(-20.76345961891,16.524555845796,124.073893348995)) ;
#65665=CARTESIAN_POINT('Ctrl Pts',(-20.4926169796923,16.3445667654331,123.941483690802)) ;
#65666=CARTESIAN_POINT('Ctrl Pts',(-20.6295786198911,16.5344554170128,124.296968784774)) ;
#65667=CARTESIAN_POINT('Ctrl Pts',(-20.3855116377468,16.3544663366499,124.119942892736)) ;
#65668=CARTESIAN_POINT('Ctrl Pts',(-20.4564004098396,16.5445033314271,124.49625876178)) ;
#65669=CARTESIAN_POINT('Ctrl Pts',(-20.246968141716,16.3645142510642,124.279374299401)) ;
#65670=CARTESIAN_POINT('Ctrl Pts',(-20.254440134761,16.5543986742876,124.660130610446)) ;
#65671=CARTESIAN_POINT('Ctrl Pts',(-20.0853998401919,16.3744095939248,124.410470518004)) ;
#65672=CARTESIAN_POINT('Ctrl Pts',(-20.0233532789183,16.5644603682351,124.788566418278)) ;
#65673=CARTESIAN_POINT('Ctrl Pts',(-19.9005296298809,16.3844712878722,124.513218396484)) ;
#65674=CARTESIAN_POINT('Ctrl Pts',(-19.7788459931032,16.5743048213192,124.873119039239)) ;
#65675=CARTESIAN_POINT('Ctrl Pts',(-19.7049244705946,16.3943157409564,124.580859189868)) ;
#65676=CARTESIAN_POINT('Ctrl Pts',(-19.5205255375102,16.5842655062777,124.915317433973)) ;
#65677=CARTESIAN_POINT('Ctrl Pts',(-19.4982683335334,16.4042764259148,124.614617059786)) ;
#65678=CARTESIAN_POINT('Ctrl Pts',(-19.2568102129339,16.5943014387862,124.911553126493)) ;
#65679=CARTESIAN_POINT('Ctrl Pts',(-19.2872959783146,16.4143123584233,124.611604711671)) ;
#65680=CARTESIAN_POINT('Ctrl Pts',(-19.0015211293968,16.6041900544743,124.863040443295)) ;
#65681=CARTESIAN_POINT('Ctrl Pts',(-19.0830656658347,16.4242009741114,124.572793892405)) ;
#65682=CARTESIAN_POINT('Ctrl Pts',(-18.7552356821971,16.6142044636167,124.770248444018)) ;
#65683=CARTESIAN_POINT('Ctrl Pts',(-18.8860375696502,16.4342153832538,124.498559626099)) ;
#65684=CARTESIAN_POINT('Ctrl Pts',(-18.5287435554736,16.6242382725745,124.635270964711)) ;
#65685=CARTESIAN_POINT('Ctrl Pts',(-18.7048442231239,16.4442491922116,124.390576829673)) ;
#65686=CARTESIAN_POINT('Ctrl Pts',(-18.3326680459431,16.6340687268307,124.467023867572)) ;
#65687=CARTESIAN_POINT('Ctrl Pts',(-18.5479851753716,16.4540796464678,124.255979389229)) ;
#65688=CARTESIAN_POINT('Ctrl Pts',(-18.164649593129,16.6441463944089,124.262383242805)) ;
#65689=CARTESIAN_POINT('Ctrl Pts',(-18.4135707132439,16.464157314046,124.092266173035)) ;
#65690=CARTESIAN_POINT('Ctrl Pts',(-18.037457177748,16.6539982625311,124.03681949593)) ;
#65691=CARTESIAN_POINT('Ctrl Pts',(-18.3118178639604,16.4740091821683,123.911815773256)) ;
#65692=CARTESIAN_POINT('Ctrl Pts',(-17.949256848314,16.6640713000965,123.787285292001)) ;
#65693=CARTESIAN_POINT('Ctrl Pts',(-18.241258048914,16.4840822197336,123.712187880445)) ;
#65694=CARTESIAN_POINT('Ctrl Pts',(-17.9067465102641,16.6739138534474,123.53212739955)) ;
#65695=CARTESIAN_POINT('Ctrl Pts',(-18.2072505652693,16.4939247730845,123.508062584724)) ;
#65696=CARTESIAN_POINT('Ctrl Pts',(-17.908337764321,16.6838942489408,123.269869124294)) ;
#65697=CARTESIAN_POINT('Ctrl Pts',(-18.208523956492,16.5039051685779,123.29825621506)) ;
#65698=CARTESIAN_POINT('Ctrl Pts',(-17.9561266808866,16.6939127269186,123.010973721011)) ;
#65699=CARTESIAN_POINT('Ctrl Pts',(-18.2467556009483,16.5139236465557,123.091139978071)) ;
#65700=CARTESIAN_POINT('Ctrl Pts',(-18.046394284067,16.7037960412247,122.767407615452)) ;
#65701=CARTESIAN_POINT('Ctrl Pts',(-18.3189697326464,16.5238069608618,122.896288048403)) ;
#65702=CARTESIAN_POINT('Ctrl Pts',(-18.1800998015951,16.7138643437634,122.539143460683)) ;
#65703=CARTESIAN_POINT('Ctrl Pts',(-18.4259346651635,16.5338752634005,122.713676647449)) ;
#65704=CARTESIAN_POINT('Ctrl Pts',(-18.3471784469217,16.7236943910368,122.342066798614)) ;
#65705=CARTESIAN_POINT('Ctrl Pts',(-18.5595970360175,16.543705310674,122.556016471638)) ;
#65706=CARTESIAN_POINT('Ctrl Pts',(-18.5504420735912,16.7337612624523,122.172817736648)) ;
#65707=CARTESIAN_POINT('Ctrl Pts',(-18.7222083400755,16.5537721820895,122.420617207245)) ;
#65708=CARTESIAN_POINT('Ctrl Pts',(-18.7760904676618,16.7436503012514,122.043833574538)) ;
#65709=CARTESIAN_POINT('Ctrl Pts',(-18.9027264648716,16.5636612208885,122.317430542113)) ;
#65710=CARTESIAN_POINT('Ctrl Pts',(-19.0231340623094,16.7536469993855,121.95457073187)) ;
#65711=CARTESIAN_POINT('Ctrl Pts',(-19.1003612452814,16.5736579190226,122.246020463371)) ;
#65712=CARTESIAN_POINT('Ctrl Pts',(-19.2808414151497,16.7635994250975,121.909859064209)) ;
#65713=CARTESIAN_POINT('Ctrl Pts',(-19.306526737126,16.5836103447346,122.210251379847)) ;
#65714=CARTESIAN_POINT('Ctrl Pts',(-19.5420687997964,16.7735407273304,121.910209653822)) ;
#65715=CARTESIAN_POINT('Ctrl Pts',(-19.515508139504,16.5935516469676,122.210531942016)) ;
#65716=CARTESIAN_POINT('Ctrl Pts',(-19.8004505578449,16.7835239664143,121.955836958364)) ;
#65717=CARTESIAN_POINT('Ctrl Pts',(-19.7222133350524,16.6035348860515,122.247033765642)) ;
#65718=CARTESIAN_POINT('Ctrl Pts',(-20.0481664431086,16.7935627679829,122.04650185724)) ;
#65719=CARTESIAN_POINT('Ctrl Pts',(-19.9203861326362,16.6135736876201,122.319565851317)) ;
#65720=CARTESIAN_POINT('Ctrl Pts',(-20.27233537467,16.8034108741046,122.175874106053)) ;
#65721=CARTESIAN_POINT('Ctrl Pts',(-20.0997202925184,16.6234217937417,122.423063076114)) ;
#65722=CARTESIAN_POINT('Ctrl Pts',(-20.4750293998556,16.8134710696799,122.345566817946)) ;
#65723=CARTESIAN_POINT('Ctrl Pts',(-20.2618757772164,16.633481989317,122.55881737648)) ;
#65724=CARTESIAN_POINT('Ctrl Pts',(-20.6422713390571,16.8233687529913,122.544786148084)) ;
#65725=CARTESIAN_POINT('Ctrl Pts',(-20.3956688189713,16.6433796726285,122.718192224318)) ;
#65726=CARTESIAN_POINT('Ctrl Pts',(-20.7735531876702,16.8332997933653,122.770334392659)) ;
#65727=CARTESIAN_POINT('Ctrl Pts',(-20.5006942028639,16.6533107130024,122.898630207615)) ;
#65728=CARTESIAN_POINT('Ctrl Pts',(-20.864420100794,16.8433420110219,123.018091751125)) ;
#65729=CARTESIAN_POINT('Ctrl Pts',(-20.5733879339271,16.6633529306591,123.096836198398)) ;
#65730=CARTESIAN_POINT('Ctrl Pts',(-20.9103551819919,16.8532286717559,123.273822728003)) ;
#65731=CARTESIAN_POINT('Ctrl Pts',(-20.61013604196,16.673239591393,123.30142008903)) ;
#65732=CARTESIAN_POINT('Ctrl Pts',(-20.9116383536201,16.8632217803584,123.536414570098)) ;
#65733=CARTESIAN_POINT('Ctrl Pts',(-20.6111628897148,16.6832326999955,123.511493398078)) ;
#65734=CARTESIAN_POINT('Ctrl Pts',(-20.8674180471858,16.8731674789966,123.794009449891)) ;
#65735=CARTESIAN_POINT('Ctrl Pts',(-20.5757870061501,16.6931783986337,123.717568881039)) ;
#65736=CARTESIAN_POINT('Ctrl Pts',(-20.7796283027966,16.8831147012677,124.04024353424)) ;
#65737=CARTESIAN_POINT('Ctrl Pts',(-20.5055557607933,16.7031256209048,123.91455585675)) ;
#65738=CARTESIAN_POINT('Ctrl Pts',(-20.6488602156385,16.8931627268478,124.269630633099)) ;
#65739=CARTESIAN_POINT('Ctrl Pts',(-20.4009414915831,16.7131736464849,124.0980658808)) ;
#65740=CARTESIAN_POINT('Ctrl Pts',(-20.4837823786232,16.9030099739907,124.468914512535)) ;
#65741=CARTESIAN_POINT('Ctrl Pts',(-20.2688802436977,16.7230208936278,124.257492376889)) ;
#65742=CARTESIAN_POINT('Ctrl Pts',(-20.2848296697992,16.9129731510814,124.639107596571)) ;
#65743=CARTESIAN_POINT('Ctrl Pts',(-20.1097187494631,16.7329840707186,124.393647070472)) ;
#65744=CARTESIAN_POINT('Ctrl Pts',(-20.0576375877666,16.9230028721148,124.772718133945)) ;
#65745=CARTESIAN_POINT('Ctrl Pts',(-19.9279652726105,16.743013791752,124.500535980068)) ;
#65746=CARTESIAN_POINT('Ctrl Pts',(-19.8138676646833,16.9329073396477,124.864008421836)) ;
#65747=CARTESIAN_POINT('Ctrl Pts',(-19.7329502140236,16.7529182592849,124.573568505699)) ;
#65748=CARTESIAN_POINT('Ctrl Pts',(-19.5549188176407,16.9429318254775,124.912240141092)) ;
#65749=CARTESIAN_POINT('Ctrl Pts',(-19.5257912019944,16.7629427451146,124.612154489046)) ;
#65750=CARTESIAN_POINT('Ctrl Pts',(-19.2946338276999,16.9528356606014,124.914963066489)) ;
#65751=CARTESIAN_POINT('Ctrl Pts',(-19.3175639397184,16.7728465802385,124.614333480641)) ;
#65752=CARTESIAN_POINT('Ctrl Pts',(-19.0340655773043,16.9628868513114,124.871886584455)) ;
#65753=CARTESIAN_POINT('Ctrl Pts',(-19.1091090337395,16.7828977709485,124.579872926838)) ;
#65754=CARTESIAN_POINT('Ctrl Pts',(-18.7889990253017,16.9727712939697,124.785703184415)) ;
#65755=CARTESIAN_POINT('Ctrl Pts',(-18.9130563598052,16.7927822136068,124.510927134029)) ;
#65756=CARTESIAN_POINT('Ctrl Pts',(-18.5599373549121,16.9827643018216,124.657327597577)) ;
#65757=CARTESIAN_POINT('Ctrl Pts',(-18.7298067701624,16.8027752214587,124.408227443796)) ;
#65758=CARTESIAN_POINT('Ctrl Pts',(-18.3575795915092,16.9927126215379,124.491777975001)) ;
#65759=CARTESIAN_POINT('Ctrl Pts',(-18.5679204008152,16.812723541175,124.275788625095)) ;
#65760=CARTESIAN_POINT('Ctrl Pts',(-18.186980138861,17.0026494602473,124.294109650112)) ;
#65761=CARTESIAN_POINT('Ctrl Pts',(-18.4314405125063,16.8226603798844,124.117654920075)) ;
#65762=CARTESIAN_POINT('Ctrl Pts',(-18.0523597654586,17.0126324491669,124.06890152174)) ;
#65763=CARTESIAN_POINT('Ctrl Pts',(-18.3237435055854,16.832643368804,123.93748907981)) ;
#65764=CARTESIAN_POINT('Ctrl Pts',(-17.9587951854769,17.022676328531,123.82213239202)) ;
#65765=CARTESIAN_POINT('Ctrl Pts',(-18.2488910084418,16.8426872481681,123.740073929916)) ;
#65766=CARTESIAN_POINT('Ctrl Pts',(-17.9099416408422,17.0325043938894,123.568481191394)) ;
#65767=CARTESIAN_POINT('Ctrl Pts',(-18.2098074301906,16.8525153135265,123.537154287906)) ;
#65768=CARTESIAN_POINT('Ctrl Pts',(-17.9056580144789,17.0425814824443,123.303759681484)) ;
#65769=CARTESIAN_POINT('Ctrl Pts',(-18.2063795179285,16.8625924020815,123.325376748704)) ;
#65770=CARTESIAN_POINT('Ctrl Pts',(-17.9463150166963,17.0524316346006,123.048052157451)) ;
#65771=CARTESIAN_POINT('Ctrl Pts',(-18.2389039336585,16.8724425542378,123.120811549314)) ;
#65772=CARTESIAN_POINT('Ctrl Pts',(-18.032582786432,17.062512115053,122.797658849589)) ;
#65773=CARTESIAN_POINT('Ctrl Pts',(-18.3079172569512,16.8825230346901,122.920496215202)) ;
#65774=CARTESIAN_POINT('Ctrl Pts',(-18.1574904407852,17.0723266128218,122.571941098829)) ;
#65775=CARTESIAN_POINT('Ctrl Pts',(-18.4078418212507,16.8923375324589,122.739922521317)) ;
#65776=CARTESIAN_POINT('Ctrl Pts',(-18.3234861663821,17.0823949088419,122.36598619016)) ;
#65777=CARTESIAN_POINT('Ctrl Pts',(-18.5406376345855,16.9024058284791,122.575157613041)) ;
#65778=CARTESIAN_POINT('Ctrl Pts',(-18.5195111943069,17.0922937413247,122.194881832912)) ;
#65779=CARTESIAN_POINT('Ctrl Pts',(-18.697456370269,16.9123046609618,122.438273670192)) ;
#65780=CARTESIAN_POINT('Ctrl Pts',(-18.7455842875903,17.1023466213392,122.058305557914)) ;
#65781=CARTESIAN_POINT('Ctrl Pts',(-18.878314382243,16.9223575409764,122.329011510998)) ;
#65782=CARTESIAN_POINT('Ctrl Pts',(-18.9874629412991,17.1122164368354,121.964526142813)) ;
#65783=CARTESIAN_POINT('Ctrl Pts',(-19.0718160746585,16.9322273564725,122.253987102022)) ;
#65784=CARTESIAN_POINT('Ctrl Pts',(-19.2470688770235,17.1222891179182,121.913081725806)) ;
#65785=CARTESIAN_POINT('Ctrl Pts',(-19.2795008526622,16.9423000375553,122.212830257528)) ;
#65786=CARTESIAN_POINT('Ctrl Pts',(-19.505422587486,17.1321215964892,121.907524515032)) ;
#65787=CARTESIAN_POINT('Ctrl Pts',(-19.4861827690057,16.9521325161263,122.208383209402)) ;
#65788=CARTESIAN_POINT('Ctrl Pts',(-19.7660419704814,17.1421522304753,121.946947546496)) ;
#65789=CARTESIAN_POINT('Ctrl Pts',(-19.6946785626933,16.9621631501124,122.239920201912)) ;
#65790=CARTESIAN_POINT('Ctrl Pts',(-20.0156574864725,17.1521837876944,122.031770159067)) ;
#65791=CARTESIAN_POINT('Ctrl Pts',(-19.8943714558458,16.9721947073315,122.307777083162)) ;
#65792=CARTESIAN_POINT('Ctrl Pts',(-20.2423350956265,17.1620134965661,122.155604235088)) ;
#65793=CARTESIAN_POINT('Ctrl Pts',(-20.075713330144,16.9820244162032,122.406842617996)) ;
#65794=CARTESIAN_POINT('Ctrl Pts',(-20.4478540416198,17.1720029453682,122.318940433098)) ;
#65795=CARTESIAN_POINT('Ctrl Pts',(-20.2401293518006,16.9920138650053,122.537510260585)) ;
#65796=CARTESIAN_POINT('Ctrl Pts',(-20.6223297569369,17.1820467977682,122.516986010216)) ;
#65797=CARTESIAN_POINT('Ctrl Pts',(-20.379711079171,17.0020577174053,122.69594586157)) ;
#65798=CARTESIAN_POINT('Ctrl Pts',(-20.7571853342976,17.1918685111003,122.737058592109)) ;
#65799=CARTESIAN_POINT('Ctrl Pts',(-20.4875963345862,17.0118794307374,122.872002271996)) ;
#65800=CARTESIAN_POINT('Ctrl Pts',(-20.8544363834582,17.201903516089,122.982179630652)) ;
#65801=CARTESIAN_POINT('Ctrl Pts',(-20.5653987506376,17.0219144357261,123.068098568077)) ;
#65802=CARTESIAN_POINT('Ctrl Pts',(-20.9068811373926,17.2119283545366,123.240357855693)) ;
#65803=CARTESIAN_POINT('Ctrl Pts',(-20.6073560524299,17.0319392741737,123.274640863138)) ;
#65804=CARTESIAN_POINT('Ctrl Pts',(-20.9141373279082,17.2217805674918,123.499162698651)) ;
#65805=CARTESIAN_POINT('Ctrl Pts',(-20.6131626102164,17.0417914871289,123.481683887994)) ;
#65806=CARTESIAN_POINT('Ctrl Pts',(-20.8762617532287,17.2317705236856,123.758921385039)) ;
#65807=CARTESIAN_POINT('Ctrl Pts',(-20.5828638652605,17.0517814433227,123.689490938947)) ;
#65808=CARTESIAN_POINT('Ctrl Pts',(-20.7943806135892,17.2416986339689,124.006649024893)) ;
#65809=CARTESIAN_POINT('Ctrl Pts',(-20.5173607099962,17.061709553606,123.887673192447)) ;
#65810=CARTESIAN_POINT('Ctrl Pts',(-20.670345385213,17.2516872340484,124.237992487124)) ;
#65811=CARTESIAN_POINT('Ctrl Pts',(-20.4181341594561,17.0716981536855,124.07274868766)) ;
#65812=CARTESIAN_POINT('Ctrl Pts',(-20.5071235397933,17.2617138259759,124.444842800166)) ;
#65813=CARTESIAN_POINT('Ctrl Pts',(-20.2875580171586,17.081724745613,124.23823002585)) ;
#65814=CARTESIAN_POINT('Ctrl Pts',(-20.3134293623449,17.2715989540401,124.617932746978)) ;
#65815=CARTESIAN_POINT('Ctrl Pts',(-20.1326042907807,17.0916098736772,124.376702907249)) ;
#65816=CARTESIAN_POINT('Ctrl Pts',(-20.0905573668405,17.2815900715136,124.756745161351)) ;
#65817=CARTESIAN_POINT('Ctrl Pts',(-19.9543077846783,17.1016009911507,124.487754352768)) ;
#65818=CARTESIAN_POINT('Ctrl Pts',(-19.8455645964301,17.2916306873654,124.854716110604)) ;
#65819=CARTESIAN_POINT('Ctrl Pts',(-19.7583141598722,17.1116416070025,124.566132786485)) ;
#65820=CARTESIAN_POINT('Ctrl Pts',(-19.5927130154484,17.3014636782191,124.907962066392)) ;
#65821=CARTESIAN_POINT('Ctrl Pts',(-19.5560340209557,17.1214745978562,124.60873119612)) ;
#65822=CARTESIAN_POINT('Ctrl Pts',(-19.330277450202,17.3114568096694,124.917387511024)) ;
#65823=CARTESIAN_POINT('Ctrl Pts',(-19.3460857391731,17.1314677293065,124.616273501047)) ;
#65824=CARTESIAN_POINT('Ctrl Pts',(-19.0692386893252,17.3214888581048,124.88041535309)) ;
#65825=CARTESIAN_POINT('Ctrl Pts',(-19.1372544392363,17.1414997777419,124.58669762411)) ;
#65826=CARTESIAN_POINT('Ctrl Pts',(-18.822677257513,17.3313541046472,124.800350459875)) ;
#65827=CARTESIAN_POINT('Ctrl Pts',(-18.9400052547958,17.1513650242843,124.522647715831)) ;
#65828=CARTESIAN_POINT('Ctrl Pts',(-18.5911545600622,17.341315979474,124.678145049276)) ;
#65829=CARTESIAN_POINT('Ctrl Pts',(-18.7547863323555,17.1613268991111,124.424885267182)) ;
#65830=CARTESIAN_POINT('Ctrl Pts',(-18.38313341919,17.3513509425853,124.516091097511)) ;
#65831=CARTESIAN_POINT('Ctrl Pts',(-18.5883681924007,17.1713618622224,124.295243637103)) ;
#65832=CARTESIAN_POINT('Ctrl Pts',(-18.2086914290502,17.3612357870477,124.323563591818)) ;
#65833=CARTESIAN_POINT('Ctrl Pts',(-18.4488134084025,17.1812467066848,124.1412233211)) ;
#65834=CARTESIAN_POINT('Ctrl Pts',(-18.0678947666769,17.3713018398884,124.099676485538)) ;
#65835=CARTESIAN_POINT('Ctrl Pts',(-18.3361743120959,17.1913127595256,123.962114606341)) ;
#65836=CARTESIAN_POINT('Ctrl Pts',(-17.9700726313909,17.3811393557974,123.860326944384)) ;
#65837=CARTESIAN_POINT('Ctrl Pts',(-18.2579149281125,17.2011502754345,123.770636270255)) ;
#65838=CARTESIAN_POINT('Ctrl Pts',(-17.9137531151006,17.3912081039063,123.601841075206)) ;
#65839=CARTESIAN_POINT('Ctrl Pts',(-18.2128572598282,17.2112190235434,123.563847905866)) ;
#65840=CARTESIAN_POINT('Ctrl Pts',(-17.9034613928053,17.4010886209373,123.342355402501)) ;
#65841=CARTESIAN_POINT('Ctrl Pts',(-18.2046218361467,17.2210995405744,123.356259859083)) ;
#65842=CARTESIAN_POINT('Ctrl Pts',(-17.9382344928248,17.4110798078718,123.082149155382)) ;
#65843=CARTESIAN_POINT('Ctrl Pts',(-18.2324382019981,17.2310907275089,123.148094673223)) ;
#65844=CARTESIAN_POINT('Ctrl Pts',(-18.0173408799565,17.4210328741467,122.832800782693)) ;
#65845=CARTESIAN_POINT('Ctrl Pts',(-18.2957212338474,17.2410437937838,122.948615510215)) ;
#65846=CARTESIAN_POINT('Ctrl Pts',(-18.1395964065383,17.4310687116793,122.599142062341)) ;
#65847=CARTESIAN_POINT('Ctrl Pts',(-18.3935237856952,17.2510796313164,122.761687546562)) ;
#65848=CARTESIAN_POINT('Ctrl Pts',(-18.2981116221672,17.4409588378907,122.393154239559)) ;
#65849=CARTESIAN_POINT('Ctrl Pts',(-18.5203340659042,17.2609697575279,122.596896255148)) ;
#65850=CARTESIAN_POINT('Ctrl Pts',(-18.4916578231572,17.4509510197987,122.215719190812)) ;
#65851=CARTESIAN_POINT('Ctrl Pts',(-18.6751695002837,17.2709619394358,122.454946675199)) ;
#65852=CARTESIAN_POINT('Ctrl Pts',(-18.7121069676179,17.4608969597373,122.075305569039)) ;
#65853=CARTESIAN_POINT('Ctrl Pts',(-18.8515275002128,17.2809078793744,122.342614056364)) ;
#65854=CARTESIAN_POINT('Ctrl Pts',(-18.9534274542707,17.4708441435014,121.974794440461)) ;
#65855=CARTESIAN_POINT('Ctrl Pts',(-19.0445828970662,17.2908550631385,122.262203186491)) ;
#65856=CARTESIAN_POINT('Ctrl Pts',(-19.211160386698,17.4808920818088,121.917426601221)) ;
#65857=CARTESIAN_POINT('Ctrl Pts',(-19.2507687776007,17.300903001446,122.216306788302)) ;
#65858=CARTESIAN_POINT('Ctrl Pts',(-19.4696824314095,17.4907397165491,121.905695967141)) ;
#65859=CARTESIAN_POINT('Ctrl Pts',(-19.4575859964064,17.3107506361862,122.206920105047)) ;
#65860=CARTESIAN_POINT('Ctrl Pts',(-19.7293772423961,17.5007014305229,121.938602055784)) ;
#65861=CARTESIAN_POINT('Ctrl Pts',(-19.6653420282454,17.3207123501601,122.233242742379)) ;
#65862=CARTESIAN_POINT('Ctrl Pts',(-19.9810217545707,17.5107300653138,122.016948020053)) ;
#65863=CARTESIAN_POINT('Ctrl Pts',(-19.8666582637803,17.3307409849509,122.295917385593)) ;
#65864=CARTESIAN_POINT('Ctrl Pts',(-20.2124907996332,17.5206403839109,122.136283881726)) ;
#65865=CARTESIAN_POINT('Ctrl Pts',(-20.0518343705786,17.340651303548,122.391384019584)) ;
#65866=CARTESIAN_POINT('Ctrl Pts',(-20.4206686080383,17.5305752402224,122.293854796919)) ;
#65867=CARTESIAN_POINT('Ctrl Pts',(-20.2183778909395,17.3505861598595,122.517438895075)) ;
#65868=CARTESIAN_POINT('Ctrl Pts',(-20.6000255828736,17.5406164761831,122.487384162176)) ;
#65869=CARTESIAN_POINT('Ctrl Pts',(-20.3618650889074,17.3606273958202,122.672260836499)) ;
#65870=CARTESIAN_POINT('Ctrl Pts',(-20.7410561133952,17.5505032477631,122.70562002418)) ;
#65871=CARTESIAN_POINT('Ctrl Pts',(-20.4746913307344,17.3705141674002,122.846848200213)) ;
#65872=CARTESIAN_POINT('Ctrl Pts',(-20.8434772707178,17.5605034264693,122.947591960567)) ;
#65873=CARTESIAN_POINT('Ctrl Pts',(-20.5566303111727,17.3805143461064,123.040424818321)) ;
#65874=CARTESIAN_POINT('Ctrl Pts',(-20.9020786278622,17.5704207046789,123.201578349681)) ;
#65875=CARTESIAN_POINT('Ctrl Pts',(-20.6035135750036,17.390431624316,123.24361335474)) ;
#65876=CARTESIAN_POINT('Ctrl Pts',(-20.91578288945,17.5804679510926,123.465216930615)) ;
#65877=CARTESIAN_POINT('Ctrl Pts',(-20.6144792336198,17.4004788707297,123.454524044763)) ;
#65878=CARTESIAN_POINT('Ctrl Pts',(-20.8843256015444,17.5903418400739,123.722819361991)) ;
#65879=CARTESIAN_POINT('Ctrl Pts',(-20.5893156441907,17.410352759711,123.660606216813)) ;
#65880=CARTESIAN_POINT('Ctrl Pts',(-20.8073356878369,17.6004038576544,123.975747950634)) ;
#65881=CARTESIAN_POINT('Ctrl Pts',(-20.527725890698,17.4204147772915,123.862949679042)) ;
#65882=CARTESIAN_POINT('Ctrl Pts',(-20.6898154915697,17.6102749193887,124.207021563565)) ;
#65883=CARTESIAN_POINT('Ctrl Pts',(-20.4337117468578,17.4302858390258,124.047969580495)) ;
#65884=CARTESIAN_POINT('Ctrl Pts',(-20.5325789116341,17.620268982749,124.417385133982)) ;
#65885=CARTESIAN_POINT('Ctrl Pts',(-20.307924299848,17.4402799023861,124.216261749645)) ;
#65886=CARTESIAN_POINT('Ctrl Pts',(-20.3400800616733,17.6303011407824,124.597505830153)) ;
#65887=CARTESIAN_POINT('Ctrl Pts',(-20.1539268192864,17.4503120604195,124.360359893607)) ;
#65888=CARTESIAN_POINT('Ctrl Pts',(-20.1232165512678,17.6401650170226,124.739545873156)) ;
#65889=CARTESIAN_POINT('Ctrl Pts',(-19.9804371926355,17.4601759366597,124.473993837202)) ;
#65890=CARTESIAN_POINT('Ctrl Pts',(-19.8800594521067,17.6502355316608,124.843920027478)) ;
#65891=CARTESIAN_POINT('Ctrl Pts',(-19.7859124646786,17.470246451298,124.557495161762)) ;
#65892=CARTESIAN_POINT('Ctrl Pts',(-19.6283095577294,17.6600761686018,124.90314183829)) ;
#65893=CARTESIAN_POINT('Ctrl Pts',(-19.5845130945949,17.4800870882389,124.60487484599)) ;
#65894=CARTESIAN_POINT('Ctrl Pts',(-19.366875274711,17.670043297442,124.918801259543)) ;
#65895=CARTESIAN_POINT('Ctrl Pts',(-19.375365146763,17.4900542170791,124.61740447096)) ;
#65896=CARTESIAN_POINT('Ctrl Pts',(-19.1054626465016,17.6800572705665,124.888408905222)) ;
#65897=CARTESIAN_POINT('Ctrl Pts',(-19.1662371963715,17.5000681902037,124.593093168698)) ;
#65898=CARTESIAN_POINT('Ctrl Pts',(-18.7709105569482,17.6933420044298,124.788587304081)) ;
#65899=CARTESIAN_POINT('Ctrl Pts',(-18.8985830635496,17.5133529240669,124.513236786793)) ;
#65900=CARTESIAN_POINT('Ctrl Pts',(-18.4713115759659,17.7065672691446,124.604860086354)) ;
#65901=CARTESIAN_POINT('Ctrl Pts',(-18.6588815387832,17.5265781887817,124.36623312436)) ;
#65902=CARTESIAN_POINT('Ctrl Pts',(-18.23024753484,17.7198777916994,124.351352544017)) ;
#65903=CARTESIAN_POINT('Ctrl Pts',(-18.4660643742217,17.5398887113366,124.163459835131)) ;
#65904=CARTESIAN_POINT('Ctrl Pts',(-18.0847456433107,17.7299064366016,124.131627885447)) ;
#65905=CARTESIAN_POINT('Ctrl Pts',(-18.3496538990184,17.5499173562387,123.987675132136)) ;
#65906=CARTESIAN_POINT('Ctrl Pts',(-17.9809344252587,17.7397874689555,123.893612632043)) ;
#65907=CARTESIAN_POINT('Ctrl Pts',(-18.2666046634578,17.5597983885926,123.797265517451)) ;
#65908=CARTESIAN_POINT('Ctrl Pts',(-17.9188829813947,17.7497684416356,123.638771587196)) ;
#65909=CARTESIAN_POINT('Ctrl Pts',(-18.2169614863476,17.5697793612727,123.593391459913)) ;
#65910=CARTESIAN_POINT('Ctrl Pts',(-17.9022490540845,17.7597495692216,123.377020959202)) ;
#65911=CARTESIAN_POINT('Ctrl Pts',(-18.2036504220169,17.5797604888587,123.383995815664)) ;
#65912=CARTESIAN_POINT('Ctrl Pts',(-17.940086062115,17.772992759483,123.030998917188)) ;
#65913=CARTESIAN_POINT('Ctrl Pts',(-18.233927074126,17.5930036791201,123.10715455913)) ;
#65914=CARTESIAN_POINT('Ctrl Pts',(-18.1006895820262,17.7896607548438,122.618237447441)) ;
#65915=CARTESIAN_POINT('Ctrl Pts',(-18.3623849444853,17.6096716744809,122.776980015619)) ;
#65916=CARTESIAN_POINT('Ctrl Pts',(-18.3897812209932,17.8061812548558,122.28765824502)) ;
#65917=CARTESIAN_POINT('Ctrl Pts',(-18.5937018866241,17.626192174493,122.512467686169)) ;
#65918=CARTESIAN_POINT('Ctrl Pts',(-18.6800705190158,17.8194942711718,122.092466331838)) ;
#65919=CARTESIAN_POINT('Ctrl Pts',(-18.8258934626634,17.639505190809,122.356347530936)) ;
#65920=CARTESIAN_POINT('Ctrl Pts',(-18.9181973224567,17.8294108294048,121.986503440751)) ;
#65921=CARTESIAN_POINT('Ctrl Pts',(-19.016402860702,17.649421749042,122.271568344734)) ;
#65922=CARTESIAN_POINT('Ctrl Pts',(-19.1738622433935,17.8394384977077,121.92290647105)) ;
#65923=CARTESIAN_POINT('Ctrl Pts',(-19.2209295533305,17.6594494173448,122.220690413991)) ;
#65924=CARTESIAN_POINT('Ctrl Pts',(-19.5194723945054,17.8526190874524,121.898080551952)) ;
#65925=CARTESIAN_POINT('Ctrl Pts',(-19.4974317792493,17.6726300070895,122.200829004453)) ;
#65926=CARTESIAN_POINT('Ctrl Pts',(-19.9563231936178,17.8693672265717,121.982455382444)) ;
#65927=CARTESIAN_POINT('Ctrl Pts',(-19.8468977311799,17.6893781462089,122.268323444308)) ;
#65928=CARTESIAN_POINT('Ctrl Pts',(-20.4081951552472,17.8891619690823,122.252387033747)) ;
#65929=CARTESIAN_POINT('Ctrl Pts',(-20.2084028189433,17.7091728887194,122.484267129473)) ;
#65930=CARTESIAN_POINT('Ctrl Pts',(-20.7451718132866,17.9092063618911,122.66478304066)) ;
#65931=CARTESIAN_POINT('Ctrl Pts',(-20.4779852136411,17.7292172815282,122.814181443718)) ;
#65932=CARTESIAN_POINT('Ctrl Pts',(-20.9190608630453,17.9290455441898,123.162728597956)) ;
#65933=CARTESIAN_POINT('Ctrl Pts',(-20.6171002151294,17.7490564638269,123.212537829593)) ;
#65934=CARTESIAN_POINT('Ctrl Pts',(-20.9138698455996,17.9489708678827,123.692157121899)) ;
#65935=CARTESIAN_POINT('Ctrl Pts',(-20.6129501230136,17.7689817875198,123.636081264938)) ;
#65936=CARTESIAN_POINT('Ctrl Pts',(-20.7282004987486,17.9688945059342,124.188169695646)) ;
#65937=CARTESIAN_POINT('Ctrl Pts',(-20.4644169876035,17.7889054255713,124.032892793635)) ;
#65938=CARTESIAN_POINT('Ctrl Pts',(-20.3846133570625,17.9888193793997,124.591069561661)) ;
#65939=CARTESIAN_POINT('Ctrl Pts',(-20.1895487840061,17.8088302990368,124.355214802049)) ;
#65940=CARTESIAN_POINT('Ctrl Pts',(-19.9254924402877,18.0086979864787,124.852574068712)) ;
#65941=CARTESIAN_POINT('Ctrl Pts',(-19.8222521396401,17.8287089061158,124.564420818094)) ;
#65942=CARTESIAN_POINT('Ctrl Pts',(-19.4021887856867,18.0286754293106,124.94239921452)) ;
#65943=CARTESIAN_POINT('Ctrl Pts',(-19.403609335955,17.8486863489478,124.636282835405)) ;
#65944=CARTESIAN_POINT('Ctrl Pts',(-18.8808448567372,18.0486072773953,124.848094480769)) ;
#65945=CARTESIAN_POINT('Ctrl Pts',(-18.9865332449473,17.8686181970324,124.560840796153)) ;
#65946=CARTESIAN_POINT('Ctrl Pts',(-18.4236271458194,18.0685025457379,124.582520931676)) ;
#65947=CARTESIAN_POINT('Ctrl Pts',(-18.620757360624,17.888513465375,124.348382725567)) ;
#65948=CARTESIAN_POINT('Ctrl Pts',(-18.083533966346,18.08842504415,124.176653707817)) ;
#65949=CARTESIAN_POINT('Ctrl Pts',(-18.3486814135184,17.9084359637871,124.023689002201)) ;
#65950=CARTESIAN_POINT('Ctrl Pts',(-17.9021445000866,18.108384526026,123.678105539859)) ;
#65951=CARTESIAN_POINT('Ctrl Pts',(-18.2035687540983,17.9283954456631,123.624850383669)) ;
#65952=CARTESIAN_POINT('Ctrl Pts',(-17.901677043034,18.1282622784854,123.149870596743)) ;
#65953=CARTESIAN_POINT('Ctrl Pts',(-18.2031940192158,17.9482731981225,123.202260912629)) ;
#65954=CARTESIAN_POINT('Ctrl Pts',(-18.0801792550787,18.1481440692199,122.65239779122)) ;
#65955=CARTESIAN_POINT('Ctrl Pts',(-18.3459964494123,17.9681549888571,122.804281306169)) ;
#65956=CARTESIAN_POINT('Ctrl Pts',(-18.4216843162061,18.1682174080709,122.242598944837)) ;
#65957=CARTESIAN_POINT('Ctrl Pts',(-18.6191997939776,17.988228327708,122.476442865587)) ;
#65958=CARTESIAN_POINT('Ctrl Pts',(-18.8764446818162,18.1880218753067,121.977323375824)) ;
#65959=CARTESIAN_POINT('Ctrl Pts',(-18.983010300815,18.0080327949438,122.26422127326)) ;
#65960=CARTESIAN_POINT('Ctrl Pts',(-19.3987200282656,18.2080052157145,121.881178045719)) ;
#65961=CARTESIAN_POINT('Ctrl Pts',(-19.4008309101687,18.0280161353516,122.187305861256)) ;
#65962=CARTESIAN_POINT('Ctrl Pts',(-19.9205934708167,18.2279201803125,121.969578565073)) ;
#65963=CARTESIAN_POINT('Ctrl Pts',(-19.8183305317221,18.0479310999496,122.258027130134)) ;
#65964=CARTESIAN_POINT('Ctrl Pts',(-20.3807158505364,18.2477887150289,122.228912632756)) ;
#65965=CARTESIAN_POINT('Ctrl Pts',(-20.1864289023512,18.067799634666,122.465496375139)) ;
#65966=CARTESIAN_POINT('Ctrl Pts',(-20.7270809482803,18.2678410992406,122.6337729235)) ;
#65967=CARTESIAN_POINT('Ctrl Pts',(-20.4635196475679,18.0878520188777,122.789385098956)) ;
#65968=CARTESIAN_POINT('Ctrl Pts',(-20.9126860426018,18.2876150630298,123.125692137824)) ;
#65969=CARTESIAN_POINT('Ctrl Pts',(-20.6120028561782,18.1076259826669,123.182923161825)) ;
#65970=CARTESIAN_POINT('Ctrl Pts',(-20.919787056096,18.3076694420512,123.658444810698)) ;
#65971=CARTESIAN_POINT('Ctrl Pts',(-20.6176815610967,18.1276803616883,123.609124837985)) ;
#65972=CARTESIAN_POINT('Ctrl Pts',(-20.7465962162573,18.3274661796244,124.155452562203)) ;
#65973=CARTESIAN_POINT('Ctrl Pts',(-20.4791262659657,18.1474770992615,124.006732040671)) ;
#65974=CARTESIAN_POINT('Ctrl Pts',(-20.4126446942546,18.3474339919759,124.567768827108)) ;
#65975=CARTESIAN_POINT('Ctrl Pts',(-20.2119627251939,18.167444911613,124.336583477204)) ;
#65976=CARTESIAN_POINT('Ctrl Pts',(-19.9576212451287,18.3673929680409,124.840656736435)) ;
#65977=CARTESIAN_POINT('Ctrl Pts',(-19.8479423832508,18.187403887678,124.554891689415)) ;
#65978=CARTESIAN_POINT('Ctrl Pts',(-19.4386451944303,18.3872878863183,124.941871042673)) ;
#65979=CARTESIAN_POINT('Ctrl Pts',(-19.4327602304496,18.2072988059554,124.635860461353)) ;
#65980=CARTESIAN_POINT('Ctrl Pts',(-18.9161726453232,18.4071841987686,124.860555263088)) ;
#65981=CARTESIAN_POINT('Ctrl Pts',(-19.0147819951874,18.2271951184057,124.570804600373)) ;
#65982=CARTESIAN_POINT('Ctrl Pts',(-18.4521815633956,18.4270921321427,124.606153931591)) ;
#65983=CARTESIAN_POINT('Ctrl Pts',(-18.6435902854391,18.2471030517799,124.367280294003)) ;
#65984=CARTESIAN_POINT('Ctrl Pts',(-18.1022181077,18.4470420224312,124.207874213592)) ;
#65985=CARTESIAN_POINT('Ctrl Pts',(-18.3636220163142,18.2670529420683,124.048653992795)) ;
#65986=CARTESIAN_POINT('Ctrl Pts',(-17.9093397630461,18.4669192529325,123.715982843254)) ;
#65987=CARTESIAN_POINT('Ctrl Pts',(-18.2093224069639,18.2869301725696,123.655139058645)) ;
#65988=CARTESIAN_POINT('Ctrl Pts',(-17.8955552161801,18.4869019218035,123.185081472576)) ;
#65989=CARTESIAN_POINT('Ctrl Pts',(-18.1982991666636,18.3069128414406,123.230417568849)) ;
#65990=CARTESIAN_POINT('Ctrl Pts',(-18.0637189576036,18.5068348083839,122.682625101242)) ;
#65991=CARTESIAN_POINT('Ctrl Pts',(-18.3328317622398,18.326845728021,122.82845440733)) ;
#65992=CARTESIAN_POINT('Ctrl Pts',(-18.3925705510188,18.5267475544018,122.267998602716)) ;
#65993=CARTESIAN_POINT('Ctrl Pts',(-18.5959242479568,18.3467584740389,122.496751834392)) ;
#65994=CARTESIAN_POINT('Ctrl Pts',(-18.767281881698,18.5433172757436,122.036622749478)) ;
#65995=CARTESIAN_POINT('Ctrl Pts',(-18.8956708387233,18.3633281953808,122.311665074245)) ;
#65996=CARTESIAN_POINT('Ctrl Pts',(-19.1020056145289,18.5566172870486,121.936011376313)) ;
#65997=CARTESIAN_POINT('Ctrl Pts',(-19.1634797346767,18.3766282066857,122.231169157369)) ;
#65998=CARTESIAN_POINT('Ctrl Pts',(-19.4482877506077,18.5698874747985,121.89465138511)) ;
#65999=CARTESIAN_POINT('Ctrl Pts',(-19.4404490281102,18.3898983944356,122.198083477283)) ;
#66000=CARTESIAN_POINT('Ctrl Pts',(-19.8857560482088,18.5865148571639,121.957313792384)) ;
#66001=CARTESIAN_POINT('Ctrl Pts',(-19.7904920476466,18.406525776801,122.248222840253)) ;
#66002=CARTESIAN_POINT('Ctrl Pts',(-20.2753787251303,18.6031371469091,122.165595250357)) ;
#66003=CARTESIAN_POINT('Ctrl Pts',(-20.1021439506729,18.4231480665462,122.414835475618)) ;
#66004=CARTESIAN_POINT('Ctrl Pts',(-20.5295847929134,18.6163823613036,122.403352527217)) ;
#66005=CARTESIAN_POINT('Ctrl Pts',(-20.3055329796882,18.4363932809408,122.60505706455)) ;
#66006=CARTESIAN_POINT('Ctrl Pts',(-20.6866624263127,18.6262943262643,122.611158628173)) ;
#66007=CARTESIAN_POINT('Ctrl Pts',(-20.4311881581819,18.4463052459014,122.771300643665)) ;
#66008=CARTESIAN_POINT('Ctrl Pts',(-20.8067318368115,18.6363529494288,122.846612050245)) ;
#66009=CARTESIAN_POINT('Ctrl Pts',(-20.5272430699789,18.4563638690659,122.959664983458)) ;
#66010=CARTESIAN_POINT('Ctrl Pts',(-20.882799746978,18.6461930635446,123.093798587262)) ;
#66011=CARTESIAN_POINT('Ctrl Pts',(-20.5880949652043,18.4662039831817,123.157414861851)) ;
#66012=CARTESIAN_POINT('Ctrl Pts',(-20.9157793856879,18.6562588485022,123.356213554678)) ;
#66013=CARTESIAN_POINT('Ctrl Pts',(-20.6144765429298,18.4762697681393,123.367347025587)) ;
#66014=CARTESIAN_POINT('Ctrl Pts',(-20.9028157443252,18.6661421662901,123.615646798569)) ;
#66015=CARTESIAN_POINT('Ctrl Pts',(-20.6041033763825,18.4861530859272,123.574893593804)) ;
#66016=CARTESIAN_POINT('Ctrl Pts',(-20.8449533316139,18.6761316041487,123.871675964814)) ;
#66017=CARTESIAN_POINT('Ctrl Pts',(-20.5578112681338,18.4961425237858,123.779716386074)) ;
#66018=CARTESIAN_POINT('Ctrl Pts',(-20.7436744284095,18.6860953182014,124.113145006398)) ;
#66019=CARTESIAN_POINT('Ctrl Pts',(-20.4767860825283,18.5061062378385,123.972890731368)) ;
#66020=CARTESIAN_POINT('Ctrl Pts',(-20.6017905558508,18.6960903298606,124.334207674781)) ;
#66021=CARTESIAN_POINT('Ctrl Pts',(-20.3632771185327,18.5161012494978,124.149739604004)) ;
#66022=CARTESIAN_POINT('Ctrl Pts',(-20.4226612590053,18.7061266215549,124.527770408748)) ;
#66023=CARTESIAN_POINT('Ctrl Pts',(-20.2199720814813,18.526137541192,124.304588217699)) ;
#66024=CARTESIAN_POINT('Ctrl Pts',(-20.2168518529892,18.7159729992483,124.684624557531)) ;
#66025=CARTESIAN_POINT('Ctrl Pts',(-20.0553231661172,18.5359839188854,124.430069764472)) ;
#66026=CARTESIAN_POINT('Ctrl Pts',(-19.9839760536042,18.725957943399,124.805452933041)) ;
#66027=CARTESIAN_POINT('Ctrl Pts',(-19.8690215418316,18.5459688630361,124.526730426201)) ;
#66028=CARTESIAN_POINT('Ctrl Pts',(-19.7348307743134,18.735894914529,124.883803103654)) ;
#66029=CARTESIAN_POINT('Ctrl Pts',(-19.6697046968684,18.5559058341661,124.589408393291)) ;
#66030=CARTESIAN_POINT('Ctrl Pts',(-19.4729748038764,18.7459446991607,124.917940423187)) ;
#66031=CARTESIAN_POINT('Ctrl Pts',(-19.4602196750584,18.5659556187978,124.616716001048)) ;
#66032=CARTESIAN_POINT('Ctrl Pts',(-19.21434799551,18.7557951612382,124.906522324717)) ;
#66033=CARTESIAN_POINT('Ctrl Pts',(-19.2533184225446,18.5758060808753,124.607579270633)) ;
#66034=CARTESIAN_POINT('Ctrl Pts',(-18.9584174462669,18.7657671747586,124.850357148989)) ;
#66035=CARTESIAN_POINT('Ctrl Pts',(-19.0485745563845,18.5857780943957,124.562644952603)) ;
#66036=CARTESIAN_POINT('Ctrl Pts',(-18.7155078312172,18.775762321878,124.750315034863)) ;
#66037=CARTESIAN_POINT('Ctrl Pts',(-18.8542477777451,18.5957732415151,124.48260921036)) ;
#66038=CARTESIAN_POINT('Ctrl Pts',(-18.493022848757,18.7857962916141,124.608834245128)) ;
#66039=CARTESIAN_POINT('Ctrl Pts',(-18.6762610286674,18.6058072112512,124.369422690082)) ;
#66040=CARTESIAN_POINT('Ctrl Pts',(-18.3016334315015,18.7956518372847,124.434305714712)) ;
#66041=CARTESIAN_POINT('Ctrl Pts',(-18.5231511449158,18.6156627569218,124.229798335907)) ;
#66042=CARTESIAN_POINT('Ctrl Pts',(-18.140904940295,18.8056505942979,124.226495189743)) ;
#66043=CARTESIAN_POINT('Ctrl Pts',(-18.394570163324,18.6256615139351,124.063548607924)) ;
#66044=CARTESIAN_POINT('Ctrl Pts',(-18.019684455447,18.8155477295351,123.99634137885)) ;
#66045=CARTESIAN_POINT('Ctrl Pts',(-18.2975958304662,18.6355586491722,123.87942470902)) ;
#66046=CARTESIAN_POINT('Ctrl Pts',(-17.93899129175,18.8256008253747,123.744810345997)) ;
#66047=CARTESIAN_POINT('Ctrl Pts',(-18.2330434068114,18.6456117450119,123.678199198287)) ;
#66048=CARTESIAN_POINT('Ctrl Pts',(-17.9037702162779,18.8354843341053,123.487463211661)) ;
#66049=CARTESIAN_POINT('Ctrl Pts',(-18.2048687720169,18.6554952537425,123.472321440138)) ;
#66050=CARTESIAN_POINT('Ctrl Pts',(-17.9132654845491,18.8454792067514,123.224988077224)) ;
#66051=CARTESIAN_POINT('Ctrl Pts',(-18.2124671563329,18.6654901263886,123.262341496769)) ;
#66052=CARTESIAN_POINT('Ctrl Pts',(-17.9687343278623,18.8554991683871,122.967567757792)) ;
#66053=CARTESIAN_POINT('Ctrl Pts',(-18.2568443761274,18.6755100880243,123.056405729243)) ;
#66054=CARTESIAN_POINT('Ctrl Pts',(-18.0667115840973,18.865404532187,122.726412358638)) ;
#66055=CARTESIAN_POINT('Ctrl Pts',(-18.3352281137652,18.6854154518241,122.863482464888)) ;
#66056=CARTESIAN_POINT('Ctrl Pts',(-18.2051056278125,18.8753451197945,122.504876382137)) ;
#66057=CARTESIAN_POINT('Ctrl Pts',(-18.4459450547457,18.6953560394316,122.68625500378)) ;
#66058=CARTESIAN_POINT('Ctrl Pts',(-18.3808775940096,18.8853479378952,122.309383985207)) ;
#66059=CARTESIAN_POINT('Ctrl Pts',(-18.5865641665979,18.7053588575323,122.529862558861)) ;
#66060=CARTESIAN_POINT('Ctrl Pts',(-18.5888129419843,18.8953826496193,122.147230647452)) ;
#66061=CARTESIAN_POINT('Ctrl Pts',(-18.7529137900349,18.7153935692564,122.40014159165)) ;
#66062=CARTESIAN_POINT('Ctrl Pts',(-18.8171608789422,18.9052275563566,122.025580674038)) ;
#66063=CARTESIAN_POINT('Ctrl Pts',(-18.9355927397188,18.7252384759937,122.302823704996)) ;
#66064=CARTESIAN_POINT('Ctrl Pts',(-19.066475495053,18.9152134089256,121.943828689904)) ;
#66065=CARTESIAN_POINT('Ctrl Pts',(-19.1350449591221,18.7352243285627,122.237424137714)) ;
#66066=CARTESIAN_POINT('Ctrl Pts',(-19.3249330398174,18.9251482173387,121.906600838846)) ;
#66067=CARTESIAN_POINT('Ctrl Pts',(-19.3418110288155,18.7451591369758,122.207643930442)) ;
#66068=CARTESIAN_POINT('Ctrl Pts',(-19.5890580305708,18.9352057444197,121.915149697282)) ;
#66069=CARTESIAN_POINT('Ctrl Pts',(-19.5531110478041,18.7552166640568,122.214485107576)) ;
#66070=CARTESIAN_POINT('Ctrl Pts',(-19.8417664438443,18.9450273994168,121.967782613312)) ;
#66071=CARTESIAN_POINT('Ctrl Pts',(-19.7552767463782,18.7650383190539,122.256593308813)) ;
#66072=CARTESIAN_POINT('Ctrl Pts',(-20.0873540689241,18.9550834435898,122.065301218056)) ;
#66073=CARTESIAN_POINT('Ctrl Pts',(-19.9517461977428,18.775094363227,122.334610067724)) ;
#66074=CARTESIAN_POINT('Ctrl Pts',(-20.3094798342934,18.965024183635,122.20280861514)) ;
#66075=CARTESIAN_POINT('Ctrl Pts',(-20.1294455077566,18.7850351032721,122.444617579698)) ;
#66076=CARTESIAN_POINT('Ctrl Pts',(-20.5041752042223,18.9749283047079,122.375539516404)) ;
#66077=CARTESIAN_POINT('Ctrl Pts',(-20.2852002006892,18.794939224345,122.582803465436)) ;
#66078=CARTESIAN_POINT('Ctrl Pts',(-20.6681231446912,18.9849758458621,122.58248803559)) ;
#66079=CARTESIAN_POINT('Ctrl Pts',(-20.416357069613,18.8049867654992,122.748363557921)) ;
#66080=CARTESIAN_POINT('Ctrl Pts',(-20.7919825435621,18.9948745974625,122.811275811282)) ;
#66081=CARTESIAN_POINT('Ctrl Pts',(-20.5154426771701,18.8148855170996,122.931394296776)) ;
#66082=CARTESIAN_POINT('Ctrl Pts',(-20.8755683816824,19.0049230764283,123.061730492506)) ;
#66083=CARTESIAN_POINT('Ctrl Pts',(-20.5823095619046,18.8249339960654,123.131758740942)) ;
#66084=CARTESIAN_POINT('Ctrl Pts',(-20.9138033739238,19.014810573512,123.318762800787)) ;
#66085=CARTESIAN_POINT('Ctrl Pts',(-20.612895591588,18.8348214931492,123.33738436397)) ;
#66086=CARTESIAN_POINT('Ctrl Pts',(-20.9072423074913,19.0248036638101,123.581265757207)) ;
#66087=CARTESIAN_POINT('Ctrl Pts',(-20.6076449012029,18.8448145834472,123.547386559869)) ;
#66088=CARTESIAN_POINT('Ctrl Pts',(-20.8553184944048,19.0347558338704,123.837608299615)) ;
#66089=CARTESIAN_POINT('Ctrl Pts',(-20.5661040904152,18.8547667535075,123.752459944652)) ;
#66090=CARTESIAN_POINT('Ctrl Pts',(-20.7601517684657,19.0446942537849,124.080804362951)) ;
#66091=CARTESIAN_POINT('Ctrl Pts',(-20.4899691655713,18.864705173422,123.947015810628)) ;
#66092=CARTESIAN_POINT('Ctrl Pts',(-20.6237942335491,19.0546793838705,124.305021774752)) ;
#66093=CARTESIAN_POINT('Ctrl Pts',(-20.3808817246997,18.8746903035076,124.126388699509)) ;
#66094=CARTESIAN_POINT('Ctrl Pts',(-20.4494165139908,19.0647160732846,124.502884010772)) ;
#66095=CARTESIAN_POINT('Ctrl Pts',(-20.2413781403973,18.8847269929217,124.284677342677)) ;
#66096=CARTESIAN_POINT('Ctrl Pts',(-20.2472957009717,19.0745707572771,124.664826057112)) ;
#66097=CARTESIAN_POINT('Ctrl Pts',(-20.0796809747905,18.8945816769142,124.414229158598)) ;
#66098=CARTESIAN_POINT('Ctrl Pts',(-20.0170234288064,19.0845702413249,124.791326058903)) ;
#66099=CARTESIAN_POINT('Ctrl Pts',(-19.8954624401579,18.9045811609621,124.515427632247)) ;
#66100=CARTESIAN_POINT('Ctrl Pts',(-19.7708869846679,19.0944653301018,124.875329679388)) ;
#66101=CARTESIAN_POINT('Ctrl Pts',(-19.6985533150144,18.914476249739,124.582628795942)) ;
#66102=CARTESIAN_POINT('Ctrl Pts',(-19.5096800897201,19.104525884748,124.915950078661)) ;
#66103=CARTESIAN_POINT('Ctrl Pts',(-19.4895873565871,18.9245368043851,124.61512352611)) ;
#66104=CARTESIAN_POINT('Ctrl Pts',(-19.2508813050788,19.1143751491209,124.910856545189)) ;
#66105=CARTESIAN_POINT('Ctrl Pts',(-19.2825491948916,18.934386068758,124.611047106101)) ;
#66106=CARTESIAN_POINT('Ctrl Pts',(-18.99220707569,19.1244024015687,124.86066175785)) ;
#66107=CARTESIAN_POINT('Ctrl Pts',(-19.0756100641405,18.9444133212059,124.570889813033)) ;
#66108=CARTESIAN_POINT('Ctrl Pts',(-18.7463833099064,19.1344306991389,124.765652294078)) ;
#66109=CARTESIAN_POINT('Ctrl Pts',(-18.8789515818906,18.954441618776,124.49488071212)) ;
#66110=CARTESIAN_POINT('Ctrl Pts',(-18.5246504442198,19.1442768281449,124.632315524006)) ;
#66111=CARTESIAN_POINT('Ctrl Pts',(-18.7015668443456,18.964287747782,124.388210457223)) ;
#66112=CARTESIAN_POINT('Ctrl Pts',(-18.3260692253604,19.154270733507,124.460445802928)) ;
#66113=CARTESIAN_POINT('Ctrl Pts',(-18.54270288402,18.9742816531441,124.250713721188)) ;
#66114=CARTESIAN_POINT('Ctrl Pts',(-18.1602075359614,19.16429483119,124.255787351941)) ;
#66115=CARTESIAN_POINT('Ctrl Pts',(-18.4100146618778,18.9843057508271,124.0869859934)) ;
#66116=CARTESIAN_POINT('Ctrl Pts',(-18.0338280399953,19.174184659044,124.028684394348)) ;
#66117=CARTESIAN_POINT('Ctrl Pts',(-18.3089126375273,18.9941955786812,123.905303536338)) ;
#66118=CARTESIAN_POINT('Ctrl Pts',(-17.947565914458,19.1841766404745,123.780690475578)) ;
#66119=CARTESIAN_POINT('Ctrl Pts',(-18.2399042544237,19.0041875601116,123.706908101772)) ;
#66120=CARTESIAN_POINT('Ctrl Pts',(-17.9059220811503,19.1941236452403,123.522631607328)) ;
#66121=CARTESIAN_POINT('Ctrl Pts',(-18.2065905909474,19.0141345648774,123.500461190172)) ;
#66122=CARTESIAN_POINT('Ctrl Pts',(-17.9092390395663,19.2040732966301,123.261175270493)) ;
#66123=CARTESIAN_POINT('Ctrl Pts',(-18.2092454041741,19.0240842162672,123.291296521161)) ;
#66124=CARTESIAN_POINT('Ctrl Pts',(-17.958538306793,19.2141102996075,123.002069408009)) ;
#66125=CARTESIAN_POINT('Ctrl Pts',(-18.2486861142578,19.0341212192446,123.084011970538)) ;
#66126=CARTESIAN_POINT('Ctrl Pts',(-18.0505326598567,19.2239992080425,122.759016798404)) ;
#66127=CARTESIAN_POINT('Ctrl Pts',(-18.3222825144302,19.0440101276797,122.88957101701)) ;
#66128=CARTESIAN_POINT('Ctrl Pts',(-18.1842635126106,19.23398854052,122.533132432072)) ;
#66129=CARTESIAN_POINT('Ctrl Pts',(-18.429268104139,19.0539994601571,122.708864261039)) ;
#66130=CARTESIAN_POINT('Ctrl Pts',(-18.3548053010277,19.2439470959571,122.334641591459)) ;
#66131=CARTESIAN_POINT('Ctrl Pts',(-18.5657022198966,19.0639580155942,122.550072634139)) ;
#66132=CARTESIAN_POINT('Ctrl Pts',(-18.5556335270977,19.2538466671576,122.169248739393)) ;
#66133=CARTESIAN_POINT('Ctrl Pts',(-18.7263649283418,19.0738575867947,122.417759614696)) ;
#66134=CARTESIAN_POINT('Ctrl Pts',(-18.7855306745994,19.2638945924096,122.039423510114)) ;
#66135=CARTESIAN_POINT('Ctrl Pts',(-18.910283328349,19.0839055120467,122.313900283675)) ;
#66136=CARTESIAN_POINT('Ctrl Pts',(-19.0306926009335,19.2737898919356,121.952607002251)) ;
#66137=CARTESIAN_POINT('Ctrl Pts',(-19.1064125243075,19.0938008115727,122.244448292274)) ;
#66138=CARTESIAN_POINT('Ctrl Pts',(-19.2914444276105,19.2838517483836,121.908933829335)) ;
#66139=CARTESIAN_POINT('Ctrl Pts',(-19.3150144124183,19.1038626680207,122.209510720343)) ;
#66140=CARTESIAN_POINT('Ctrl Pts',(-19.5501343610573,19.2936955948002,121.911097613413)) ;
#66141=CARTESIAN_POINT('Ctrl Pts',(-19.5219652921603,19.1137065144373,122.211242751695)) ;
#66142=CARTESIAN_POINT('Ctrl Pts',(-19.8077343935755,19.3036585439283,121.957822195286)) ;
#66143=CARTESIAN_POINT('Ctrl Pts',(-19.7280448206616,19.1236694635654,122.248623138328)) ;
#66144=CARTESIAN_POINT('Ctrl Pts',(-20.0549291177178,19.3136925803563,122.049626315006)) ;
#66145=CARTESIAN_POINT('Ctrl Pts',(-19.9258003882064,19.1337034999934,122.322067316074)) ;
#66146=CARTESIAN_POINT('Ctrl Pts',(-20.2792335465816,19.3235800073143,122.18076820435)) ;
#66147=CARTESIAN_POINT('Ctrl Pts',(-20.1052428067102,19.1435909269514,122.426981141854)) ;
#66148=CARTESIAN_POINT('Ctrl Pts',(-20.4802444747173,19.3335944416507,122.350655841088)) ;
#66149=CARTESIAN_POINT('Ctrl Pts',(-20.2660510795986,19.1536053612878,122.562891792175)) ;
#66150=CARTESIAN_POINT('Ctrl Pts',(-20.6485175407954,19.3436293862856,122.553674509814)) ;
#66151=CARTESIAN_POINT('Ctrl Pts',(-20.4006689258585,19.1636403059227,122.725307374417)) ;
#66152=CARTESIAN_POINT('Ctrl Pts',(-20.7769890298325,19.3534617363166,122.777893029322)) ;
#66153=CARTESIAN_POINT('Ctrl Pts',(-20.5034449148929,19.1734726559537,122.904681511226)) ;
#66154=CARTESIAN_POINT('Ctrl Pts',(-20.8667862746344,19.3635371754338,123.026918659849)) ;
#66155=CARTESIAN_POINT('Ctrl Pts',(-20.5752821883899,19.183548095071,123.103902590368)) ;
#66156=CARTESIAN_POINT('Ctrl Pts',(-20.9111458115105,19.3733896406684,123.282059452494)) ;
#66157=CARTESIAN_POINT('Ctrl Pts',(-20.6107689973514,19.1934005603056,123.308014298688)) ;
#66158=CARTESIAN_POINT('Ctrl Pts',(-20.9107290324318,19.3834625182453,123.546718673386)) ;
#66159=CARTESIAN_POINT('Ctrl Pts',(-20.6104349741825,19.2034734378824,123.519742024396)) ;
#66160=CARTESIAN_POINT('Ctrl Pts',(-20.8653781808651,19.3933051144378,123.801387925564)) ;
#66161=CARTESIAN_POINT('Ctrl Pts',(-20.5741538923526,19.2133160340749,123.723476203268)) ;
#66162=CARTESIAN_POINT('Ctrl Pts',(-20.7760923678515,19.4032854985531,124.047984519831)) ;
#66163=CARTESIAN_POINT('Ctrl Pts',(-20.5027249602154,19.2232964181902,123.920753112728)) ;
#66164=CARTESIAN_POINT('Ctrl Pts',(-20.6443997501556,19.4133039792019,124.275948701137)) ;
#66165=CARTESIAN_POINT('Ctrl Pts',(-20.3973704129932,19.233314898839,124.103124205952)) ;
#66166=CARTESIAN_POINT('Ctrl Pts',(-20.4778099653252,19.4231872942023,124.475248963833)) ;
#66167=CARTESIAN_POINT('Ctrl Pts',(-20.2640988584677,19.2431982138394,124.262563499982)) ;
#66168=CARTESIAN_POINT('Ctrl Pts',(-20.2754104277972,19.4332555912927,124.645589428262)) ;
#66169=CARTESIAN_POINT('Ctrl Pts',(-20.1021787138093,19.2532665109298,124.398835770553)) ;
#66170=CARTESIAN_POINT('Ctrl Pts',(-20.0520012191522,19.443085659665,124.775372441285)) ;
#66171=CARTESIAN_POINT('Ctrl Pts',(-19.9234522479264,19.2630965793021,124.502661276645)) ;
#66172=CARTESIAN_POINT('Ctrl Pts',(-19.8038135625138,19.4531524521334,124.86681341649)) ;
#66173=CARTESIAN_POINT('Ctrl Pts',(-19.7249017349538,19.2731633717705,124.575813934512)) ;
#66174=CARTESIAN_POINT('Ctrl Pts',(-19.5479941097252,19.4630417856219,124.912847154411)) ;
#66175=CARTESIAN_POINT('Ctrl Pts',(-19.5202469635521,19.2830527052591,124.612640501714)) ;
#66176=CARTESIAN_POINT('Ctrl Pts',(-19.2851987471319,19.473043917038,124.914186378401)) ;
#66177=CARTESIAN_POINT('Ctrl Pts',(-19.3100107840446,19.2930548366751,124.613711708274)) ;
#66178=CARTESIAN_POINT('Ctrl Pts',(-19.0280693627692,19.482967786659,124.870372052193)) ;
#66179=CARTESIAN_POINT('Ctrl Pts',(-19.1043078948215,19.3029787062961,124.578660218181)) ;
#66180=CARTESIAN_POINT('Ctrl Pts',(-18.7796000674895,19.4930113021762,124.781474531052)) ;
#66181=CARTESIAN_POINT('Ctrl Pts',(-18.9055323440351,19.3130222218133,124.507542000366)) ;
#66182=CARTESIAN_POINT('Ctrl Pts',(-18.5537969176444,19.5028935150645,124.653102676941)) ;
#66183=CARTESIAN_POINT('Ctrl Pts',(-18.7248906370469,19.3229044347016,124.404844891224)) ;
#66184=CARTESIAN_POINT('Ctrl Pts',(-18.3500292628219,19.5129615922839,124.484417808806)) ;
#66185=CARTESIAN_POINT('Ctrl Pts',(-18.5618763184921,19.332972511921,124.269896733581)) ;
#66186=CARTESIAN_POINT('Ctrl Pts',(-18.1823173295114,19.5228000970181,124.287590469283)) ;
#66187=CARTESIAN_POINT('Ctrl Pts',(-18.4277075526952,19.3428110166552,124.112435753387)) ;
#66188=CARTESIAN_POINT('Ctrl Pts',(-18.04805852035,19.5328628654475,124.059806889975)) ;
#66189=CARTESIAN_POINT('Ctrl Pts',(-18.3203002879426,19.3528737850846,123.930208672601)) ;
#66190=CARTESIAN_POINT('Ctrl Pts',(-17.9571650618813,19.5427598587302,123.816107138229)) ;
#66191=CARTESIAN_POINT('Ctrl Pts',(-18.247585798284,19.3627707783674,123.735249623978)) ;
#66192=CARTESIAN_POINT('Ctrl Pts',(-17.9089504191746,19.552691086365,123.559623490826)) ;
#66193=CARTESIAN_POINT('Ctrl Pts',(-18.2090139678198,19.3727020060021,123.530063314493)) ;
#66194=CARTESIAN_POINT('Ctrl Pts',(-17.9062584823097,19.5627332450072,123.295743025407)) ;
#66195=CARTESIAN_POINT('Ctrl Pts',(-18.2068602643135,19.3827441646443,123.318958777135)) ;
#66196=CARTESIAN_POINT('Ctrl Pts',(-17.9485751372052,19.5726199545382,123.039387974114)) ;
#66197=CARTESIAN_POINT('Ctrl Pts',(-18.240713249619,19.3926308741753,123.113875561071)) ;
#66198=CARTESIAN_POINT('Ctrl Pts',(-18.035260566707,19.5826129269668,122.791515506251)) ;
#66199=CARTESIAN_POINT('Ctrl Pts',(-18.3100612446795,19.4026238466039,122.915577638234)) ;
#66200=CARTESIAN_POINT('Ctrl Pts',(-18.1631676695922,19.5925591215034,122.563579250553)) ;
#66201=CARTESIAN_POINT('Ctrl Pts',(-18.4123864487675,19.4125700411405,122.733228908367)) ;
#66202=CARTESIAN_POINT('Ctrl Pts',(-18.3282687771438,19.6025044963549,122.360947075224)) ;
#66203=CARTESIAN_POINT('Ctrl Pts',(-18.5444667060827,19.422515415992,122.571123262125)) ;
#66204=CARTESIAN_POINT('Ctrl Pts',(-18.5284509193618,19.6125594157148,122.188521930226)) ;
#66205=CARTESIAN_POINT('Ctrl Pts',(-18.7046123935706,19.4325703353519,122.433182741857)) ;
#66206=CARTESIAN_POINT('Ctrl Pts',(-18.750061582201,19.6223809351583,122.056150769602)) ;
#66207=CARTESIAN_POINT('Ctrl Pts',(-18.8818995815922,19.4423918547954,122.327286088883)) ;
#66208=CARTESIAN_POINT('Ctrl Pts',(-18.9970975872,19.6324467039252,121.961712899097)) ;
#66209=CARTESIAN_POINT('Ctrl Pts',(-19.0795284847268,19.4524576235623,122.251735185212)) ;
#66210=CARTESIAN_POINT('Ctrl Pts',(-19.2526602063055,19.6423486255803,121.912488218236)) ;
#66211=CARTESIAN_POINT('Ctrl Pts',(-19.2839777620693,19.4623595452174,122.212355084193)) ;
#66212=CARTESIAN_POINT('Ctrl Pts',(-19.5165208729935,19.6523916844013,121.908094752818)) ;
#66213=CARTESIAN_POINT('Ctrl Pts',(-19.4950664570593,19.4724026040384,122.208839744185)) ;
#66214=CARTESIAN_POINT('Ctrl Pts',(-19.7735886685139,19.662297678444,121.949158051718)) ;
#66215=CARTESIAN_POINT('Ctrl Pts',(-19.7007200621191,19.4823085980811,122.241689749395)) ;
#66216=CARTESIAN_POINT('Ctrl Pts',(-20.0206528799151,19.6722354515258,122.033777229908)) ;
#66217=CARTESIAN_POINT('Ctrl Pts',(-19.8983711686072,19.4922463711629,122.30938424429)) ;
#66218=CARTESIAN_POINT('Ctrl Pts',(-20.2514911587077,19.6822758152581,122.161558568198)) ;
#66219=CARTESIAN_POINT('Ctrl Pts',(-20.0830422357934,19.5022867348952,122.411608819251)) ;
#66220=CARTESIAN_POINT('Ctrl Pts',(-20.4536472526372,19.6921631589816,122.324810150255)) ;
#66221=CARTESIAN_POINT('Ctrl Pts',(-20.2447669012231,19.5121740786187,122.542209021845)) ;
#66222=CARTESIAN_POINT('Ctrl Pts',(-20.6265036649569,19.7021553895503,122.522452222942)) ;
#66223=CARTESIAN_POINT('Ctrl Pts',(-20.3830525266567,19.5221663091874,122.700322030319)) ;
#66224=CARTESIAN_POINT('Ctrl Pts',(-20.7617787531808,19.7121039173339,122.746188030278)) ;
#66225=CARTESIAN_POINT('Ctrl Pts',(-20.4912730421252,19.532114836971,122.879309900702)) ;
#66226=CARTESIAN_POINT('Ctrl Pts',(-20.856369565108,19.7220407010572,122.989558473137)) ;
#66227=CARTESIAN_POINT('Ctrl Pts',(-20.5669463183877,19.5420516206943,123.074005464355)) ;
#66228=CARTESIAN_POINT('Ctrl Pts',(-20.9078402627332,19.7320237018542,123.246836830907)) ;
#66229=CARTESIAN_POINT('Ctrl Pts',(-20.6081237656465,19.5520346214913,123.279827763413)) ;
#66230=CARTESIAN_POINT('Ctrl Pts',(-20.9134056044351,19.7420675886949,123.510689929292)) ;
#66231=CARTESIAN_POINT('Ctrl Pts',(-20.6125768755946,19.562078508332,123.490910375999)) ;
#66232=CARTESIAN_POINT('Ctrl Pts',(-20.8745366916682,19.7518956122695,123.766060949729)) ;
#66233=CARTESIAN_POINT('Ctrl Pts',(-20.5814828864297,19.5719065319066,123.69520619847)) ;
#66234=CARTESIAN_POINT('Ctrl Pts',(-20.7899593277774,19.7619728604831,124.016948250578)) ;
#66235=CARTESIAN_POINT('Ctrl Pts',(-20.513821837292,19.5819837801202,123.895916689788)) ;
#66236=CARTESIAN_POINT('Ctrl Pts',(-20.6660660069028,19.7718224157884,124.244285226899)) ;
#66237=CARTESIAN_POINT('Ctrl Pts',(-20.4147085725534,19.5918333354255,124.077785895298)) ;
#66238=CARTESIAN_POINT('Ctrl Pts',(-20.5009161893016,19.7819051239861,124.451396677659)) ;
#66239=CARTESIAN_POINT('Ctrl Pts',(-20.2825893295826,19.6019160436232,124.243476002834)) ;
#66240=CARTESIAN_POINT('Ctrl Pts',(-20.307696830118,19.7917177169126,124.622248846254)) ;
#66241=CARTESIAN_POINT('Ctrl Pts',(-20.1280154809097,19.6117286365497,124.380157782015)) ;
#66242=CARTESIAN_POINT('Ctrl Pts',(-20.0823669714035,19.8017849091705,124.760755273323)) ;
#66243=CARTESIAN_POINT('Ctrl Pts',(-19.9477519880674,19.6217958288076,124.490964105197)) ;
#66244=CARTESIAN_POINT('Ctrl Pts',(-19.8403718039497,19.8116837386331,124.856362880226)) ;
#66245=CARTESIAN_POINT('Ctrl Pts',(-19.7541569135087,19.6316946582702,124.567451052078)) ;
#66246=CARTESIAN_POINT('Ctrl Pts',(-19.581599257843,19.8217377298233,124.90940442077)) ;
#66247=CARTESIAN_POINT('Ctrl Pts',(-19.5471389315843,19.6417486494604,124.609885512907)) ;
#66248=CARTESIAN_POINT('Ctrl Pts',(-19.3222318233483,19.8316094546065,124.916810422138)) ;
#66249=CARTESIAN_POINT('Ctrl Pts',(-19.339645850064,19.6516203742436,124.615811552476)) ;
#66250=CARTESIAN_POINT('Ctrl Pts',(-19.0604406240858,19.8416798967367,124.878387276188)) ;
#66251=CARTESIAN_POINT('Ctrl Pts',(-19.1302124239704,19.6616908163738,124.585074260848)) ;
#66252=CARTESIAN_POINT('Ctrl Pts',(-18.8151144576531,19.851512975167,124.797145106877)) ;
#66253=CARTESIAN_POINT('Ctrl Pts',(-18.9339520539141,19.6715238948041,124.52008208332)) ;
#66254=CARTESIAN_POINT('Ctrl Pts',(-18.5827297027157,19.8615434486684,124.672758530689)) ;
#66255=CARTESIAN_POINT('Ctrl Pts',(-18.7480434996773,19.6815543683055,124.420574076199)) ;
#66256=CARTESIAN_POINT('Ctrl Pts',(-18.3759053294246,19.8715750479671,124.509274829673)) ;
#66257=CARTESIAN_POINT('Ctrl Pts',(-18.5825831437698,19.6915859676042,124.289788093677)) ;
#66258=CARTESIAN_POINT('Ctrl Pts',(-18.2037555511074,19.8814047490052,124.31670801897)) ;
#66259=CARTESIAN_POINT('Ctrl Pts',(-18.4448629441187,19.7014156686424,124.135736342827)) ;
#66260=CARTESIAN_POINT('Ctrl Pts',(-18.0647658072952,19.8913941870617,124.094000670336)) ;
#66261=CARTESIAN_POINT('Ctrl Pts',(-18.3336698936195,19.7114051066988,123.957571414372)) ;
#66262=CARTESIAN_POINT('Ctrl Pts',(-17.9666480383149,19.9014380902778,123.848976044792)) ;
#66263=CARTESIAN_POINT('Ctrl Pts',(-18.2551743019667,19.7214490099149,123.761552138209)) ;
#66264=CARTESIAN_POINT('Ctrl Pts',(-17.9132339251412,19.9112596110913,123.596462120658)) ;
#66265=CARTESIAN_POINT('Ctrl Pts',(-18.212441709217,19.7312705307284,123.559542293389)) ;
#66266=CARTESIAN_POINT('Ctrl Pts',(-17.9036546813369,19.9212953353384,123.332913768264)) ;
#66267=CARTESIAN_POINT('Ctrl Pts',(-18.2047766510836,19.7413062549755,123.348703585753)) ;
#66268=CARTESIAN_POINT('Ctrl Pts',(-17.9406113337571,19.9313174892709,123.072128085455)) ;
#66269=CARTESIAN_POINT('Ctrl Pts',(-18.2343404591825,19.751328408908,123.140074813286)) ;
#66270=CARTESIAN_POINT('Ctrl Pts',(-18.0205697573143,19.9411797210282,122.825622198603)) ;
#66271=CARTESIAN_POINT('Ctrl Pts',(-18.2983054242486,19.7611906406653,122.942870341222)) ;
#66272=CARTESIAN_POINT('Ctrl Pts',(-18.1426708877126,19.9511387914861,122.594127929803)) ;
#66273=CARTESIAN_POINT('Ctrl Pts',(-18.3959846585781,19.7711497111232,122.757674351822)) ;
#66274=CARTESIAN_POINT('Ctrl Pts',(-18.3046496822276,19.9611739638623,122.386036391047)) ;
#66275=CARTESIAN_POINT('Ctrl Pts',(-18.525566417151,19.7811848834994,122.591200043048)) ;
#66276=CARTESIAN_POINT('Ctrl Pts',(-18.4970491714254,19.9710543490205,122.211642765681)) ;
#66277=CARTESIAN_POINT('Ctrl Pts',(-18.6794843828221,19.7910652686577,122.451684269361)) ;
#66278=CARTESIAN_POINT('Ctrl Pts',(-18.720627652709,19.9811110636145,122.070778322321)) ;
#66279=CARTESIAN_POINT('Ctrl Pts',(-18.8583463631659,19.8011219832516,122.338991147531)) ;
#66280=CARTESIAN_POINT('Ctrl Pts',(-18.960996130641,19.9909903321865,121.972639347132)) ;
#66281=CARTESIAN_POINT('Ctrl Pts',(-19.0506399085198,19.8110012518237,122.260478581221)) ;
#66282=CARTESIAN_POINT('Ctrl Pts',(-19.2174586026876,20.0009812896722,121.916419162101)) ;
#66283=CARTESIAN_POINT('Ctrl Pts',(-19.2558093721547,19.8209922093093,122.21550063503)) ;
#66284=CARTESIAN_POINT('Ctrl Pts',(-19.4811173295918,20.0110219483074,121.906111456795)) ;
#66285=CARTESIAN_POINT('Ctrl Pts',(-19.4667363549532,19.8310328679445,122.207252696804)) ;
#66286=CARTESIAN_POINT('Ctrl Pts',(-19.7372046092749,20.0208549280154,121.940573290861)) ;
#66287=CARTESIAN_POINT('Ctrl Pts',(-19.6716056688886,19.8408658476525,122.234820236614)) ;
#66288=CARTESIAN_POINT('Ctrl Pts',(-19.9876565139675,20.0308480612651,122.019537420732)) ;
#66289=CARTESIAN_POINT('Ctrl Pts',(-19.871967684399,19.8508589809022,122.297989646812)) ;
#66290=CARTESIAN_POINT('Ctrl Pts',(-20.2212609501245,20.0408801136485,122.141754795336)) ;
#66291=CARTESIAN_POINT('Ctrl Pts',(-20.0588521268464,19.8608910332856,122.395761901234)) ;
#66292=CARTESIAN_POINT('Ctrl Pts',(-20.4267990069944,20.0507453425998,122.29973257063)) ;
#66293=CARTESIAN_POINT('Ctrl Pts',(-20.2232832806594,19.8707562622369,122.522142243935)) ;
#66294=CARTESIAN_POINT('Ctrl Pts',(-20.6040593213488,20.060707283843,122.492388017739)) ;
#66295=CARTESIAN_POINT('Ctrl Pts',(-20.3650928817087,19.8807182034801,122.676265086268)) ;
#66296=CARTESIAN_POINT('Ctrl Pts',(-20.7458379853386,20.0707419988798,122.71471883926)) ;
#66297=CARTESIAN_POINT('Ctrl Pts',(-20.4785174821517,19.8907529185169,122.854128710767)) ;
#66298=CARTESIAN_POINT('Ctrl Pts',(-20.8457638320152,20.0806277692238,122.954554133205)) ;
#66299=CARTESIAN_POINT('Ctrl Pts',(-20.5584598470704,19.9006386888609,123.045995755698)) ;
#66300=CARTESIAN_POINT('Ctrl Pts',(-20.9035264743855,20.0906903666126,123.212570178599)) ;
#66301=CARTESIAN_POINT('Ctrl Pts',(-20.6046719531102,19.9107012862497,123.252408261689)) ;
#66302=CARTESIAN_POINT('Ctrl Pts',(-20.9154749497781,20.1005407784478,123.471173528851)) ;
#66303=CARTESIAN_POINT('Ctrl Pts',(-20.6142327359483,19.9205516980849,123.459290308044)) ;
#66304=CARTESIAN_POINT('Ctrl Pts',(-20.8824212203225,20.1105679477337,123.732588303383)) ;
#66305=CARTESIAN_POINT('Ctrl Pts',(-20.5877918409855,19.9305788673709,123.668422402238)) ;
#66306=CARTESIAN_POINT('Ctrl Pts',(-20.8038130480593,20.1205954284479,123.984115444725)) ;
#66307=CARTESIAN_POINT('Ctrl Pts',(-20.5249072402036,19.940606348085,123.86964471591)) ;
#66308=CARTESIAN_POINT('Ctrl Pts',(-20.6854052876472,20.1304384810272,124.214077225316)) ;
#66309=CARTESIAN_POINT('Ctrl Pts',(-20.4301831161523,19.9504494006643,124.053614646428)) ;
#66310=CARTESIAN_POINT('Ctrl Pts',(-20.5269966913248,20.1404323844658,124.423553915828)) ;
#66311=CARTESIAN_POINT('Ctrl Pts',(-20.3034580001774,19.9604433041029,124.221197233981)) ;
#66312=CARTESIAN_POINT('Ctrl Pts',(-20.3336481312429,20.1504595072422,124.602587618317)) ;
#66313=CARTESIAN_POINT('Ctrl Pts',(-20.1487805945953,19.9704704268793,124.364425725248)) ;
#66314=CARTESIAN_POINT('Ctrl Pts',(-20.1153421998912,20.1603502121343,124.743661057522)) ;
#66315=CARTESIAN_POINT('Ctrl Pts',(-19.9741372834993,19.9803611317714,124.477286090543)) ;
#66316=CARTESIAN_POINT('Ctrl Pts',(-19.873563628878,20.1703422389846,124.846066786522)) ;
#66317=CARTESIAN_POINT('Ctrl Pts',(-19.7807153501285,19.9903531586217,124.559212634884)) ;
#66318=CARTESIAN_POINT('Ctrl Pts',(-19.618831660715,20.1802882204731,124.904591118333)) ;
#66319=CARTESIAN_POINT('Ctrl Pts',(-19.5769304388928,20.0002991401102,124.60603416333)) ;
#66320=CARTESIAN_POINT('Ctrl Pts',(-19.3577875500338,20.190235393095,124.918525903528)) ;
#66321=CARTESIAN_POINT('Ctrl Pts',(-19.3680954272052,20.0102463127322,124.61718417711)) ;
#66322=CARTESIAN_POINT('Ctrl Pts',(-19.0957195762214,20.2002833344212,124.886313111744)) ;
#66323=CARTESIAN_POINT('Ctrl Pts',(-19.1584407747982,20.0202942540583,124.591416103589)) ;
#66324=CARTESIAN_POINT('Ctrl Pts',(-18.8481841830687,20.210130968229,124.810831448379)) ;
#66325=CARTESIAN_POINT('Ctrl Pts',(-18.9604121247911,20.0301418878661,124.531032963021)) ;
#66326=CARTESIAN_POINT('Ctrl Pts',(-18.6144848557031,20.220092682914,124.692895466025)) ;
#66327=CARTESIAN_POINT('Ctrl Pts',(-18.7734517428529,20.0401036025511,124.436686220242)) ;
#66328=CARTESIAN_POINT('Ctrl Pts',(-18.4035822760522,20.2301213157925,124.534835645106)) ;
#66329=CARTESIAN_POINT('Ctrl Pts',(-18.6047283766993,20.0501322354297,124.310240160807)) ;
#66330=CARTESIAN_POINT('Ctrl Pts',(-18.2254094105789,20.2400316413277,124.34490354003)) ;
#66331=CARTESIAN_POINT('Ctrl Pts',(-18.4621885771613,20.0600425609648,124.158296117052)) ;
#66332=CARTESIAN_POINT('Ctrl Pts',(-18.0819921054121,20.2499664717994,124.126739575367)) ;
#66333=CARTESIAN_POINT('Ctrl Pts',(-18.347452906344,20.0699773914365,123.983766287248)) ;
#66334=CARTESIAN_POINT('Ctrl Pts',(-17.9777343205273,20.2600078041814,123.884334153632)) ;
#66335=CARTESIAN_POINT('Ctrl Pts',(-18.2640446533727,20.0800187238185,123.789842799783)) ;
#66336=CARTESIAN_POINT('Ctrl Pts',(-17.9179543452334,20.2699006776202,123.631328380915)) ;
#66337=CARTESIAN_POINT('Ctrl Pts',(-18.2162184451713,20.0899115972573,123.587439083643)) ;
#66338=CARTESIAN_POINT('Ctrl Pts',(-17.9022315156781,20.2798698434381,123.369810686241)) ;
#66339=CARTESIAN_POINT('Ctrl Pts',(-18.2036382029103,20.0998807630752,123.37822414266)) ;
#66340=CARTESIAN_POINT('Ctrl Pts',(-17.9327660607719,20.2898985771546,123.108061591331)) ;
#66341=CARTESIAN_POINT('Ctrl Pts',(-18.2280625915591,20.1099094967917,123.168828314924)) ;
#66342=CARTESIAN_POINT('Ctrl Pts',(-18.0314212956118,20.3030910959258,122.775637805959)) ;
#66343=CARTESIAN_POINT('Ctrl Pts',(-18.3069888734284,20.1231020155629,122.902870362102)) ;
#66344=CARTESIAN_POINT('Ctrl Pts',(-18.2167817772954,20.3164509639684,122.472918789065)) ;
#66345=CARTESIAN_POINT('Ctrl Pts',(-18.455294322149,20.1364618836056,122.660681237817)) ;
#66346=CARTESIAN_POINT('Ctrl Pts',(-18.4689719567282,20.3296763011173,122.233665328807)) ;
#66347=CARTESIAN_POINT('Ctrl Pts',(-18.657015967816,20.1496872207544,122.469309185131)) ;
#66348=CARTESIAN_POINT('Ctrl Pts',(-18.6872891439649,20.3396575269579,122.0882957323)) ;
#66349=CARTESIAN_POINT('Ctrl Pts',(-18.8316741569079,20.1596684465951,122.353005054526)) ;
#66350=CARTESIAN_POINT('Ctrl Pts',(-18.9290457583576,20.3496930939408,121.982939786469)) ;
#66351=CARTESIAN_POINT('Ctrl Pts',(-19.0250769393784,20.1697040135779,122.268720036234)) ;
#66352=CARTESIAN_POINT('Ctrl Pts',(-19.1809279027677,20.3595561719029,121.921703115503)) ;
#66353=CARTESIAN_POINT('Ctrl Pts',(-19.2265826009953,20.17956709154,122.219728036107)) ;
#66354=CARTESIAN_POINT('Ctrl Pts',(-19.4449915418395,20.369626470704,121.904729894139)) ;
#66355=CARTESIAN_POINT('Ctrl Pts',(-19.4378331366122,20.1896373903411,122.206147360686)) ;
#66356=CARTESIAN_POINT('Ctrl Pts',(-19.7020745055463,20.3794687692718,121.933224576347)) ;
#66357=CARTESIAN_POINT('Ctrl Pts',(-19.6434999173445,20.1994796889089,122.228940862857)) ;
#66358=CARTESIAN_POINT('Ctrl Pts',(-19.9535442296739,20.3894294674416,122.005865433082)) ;
#66359=CARTESIAN_POINT('Ctrl Pts',(-19.844676334268,20.2094403870787,122.287051467107)) ;
#66360=CARTESIAN_POINT('Ctrl Pts',(-20.1901714045228,20.3994675016211,122.122429978516)) ;
#66361=CARTESIAN_POINT('Ctrl Pts',(-20.0339789452335,20.2194784212582,122.380301057783)) ;
#66362=CARTESIAN_POINT('Ctrl Pts',(-20.3998046709007,20.4093412384676,122.275390622965)) ;
#66363=CARTESIAN_POINT('Ctrl Pts',(-20.2016870029984,20.2293521581047,122.502667926402)) ;
#66364=CARTESIAN_POINT('Ctrl Pts',(-20.5832300951106,20.4194130223928,122.466148916955)) ;
#66365=CARTESIAN_POINT('Ctrl Pts',(-20.3484287872655,20.2394239420299,122.655272907251)) ;
#66366=CARTESIAN_POINT('Ctrl Pts',(-20.7274022481108,20.429245143594,122.680593266604)) ;
#66367=CARTESIAN_POINT('Ctrl Pts',(-20.4637684999712,20.2492560632311,122.826827448914)) ;
#66368=CARTESIAN_POINT('Ctrl Pts',(-20.83492227229,20.4392781676194,122.921317142792)) ;
#66369=CARTESIAN_POINT('Ctrl Pts',(-20.549786401994,20.2592890872566,123.019405611083)) ;
#66370=CARTESIAN_POINT('Ctrl Pts',(-20.8982551027824,20.4492940478161,123.176808341218)) ;
#66371=CARTESIAN_POINT('Ctrl Pts',(-20.6004547451558,20.2693049674532,123.223797857408)) ;
#66372=CARTESIAN_POINT('Ctrl Pts',(-20.9165069215087,20.4591775669103,123.435894221683)) ;
#66373=CARTESIAN_POINT('Ctrl Pts',(-20.615058364723,20.2791884865474,123.43106704069)) ;
#66374=CARTESIAN_POINT('Ctrl Pts',(-20.8895420040221,20.469167979274,123.697025786576)) ;
#66375=CARTESIAN_POINT('Ctrl Pts',(-20.5934884233315,20.2891788989111,123.639971206989)) ;
#66376=CARTESIAN_POINT('Ctrl Pts',(-20.7941934591565,20.4824311424774,124.032297261989)) ;
#66377=CARTESIAN_POINT('Ctrl Pts',(-20.5172126368922,20.3024420621145,123.908195802062)) ;
#66378=CARTESIAN_POINT('Ctrl Pts',(-20.61364497499,20.4957087127286,124.335469275498)) ;
#66379=CARTESIAN_POINT('Ctrl Pts',(-20.3727498733357,20.3157196323657,124.15076100523)) ;
#66380=CARTESIAN_POINT('Ctrl Pts',(-20.3624251620307,20.5090390152352,124.579659196355)) ;
#66381=CARTESIAN_POINT('Ctrl Pts',(-20.1718067039307,20.3290499348723,124.346077405116)) ;
#66382=CARTESIAN_POINT('Ctrl Pts',(-20.1474678125217,20.5189376970516,124.726143222167)) ;
#66383=CARTESIAN_POINT('Ctrl Pts',(-19.9998354017675,20.3389486166887,124.463273991554)) ;
#66384=CARTESIAN_POINT('Ctrl Pts',(-19.9082988338251,20.5289272120991,124.834343756603)) ;
#66385=CARTESIAN_POINT('Ctrl Pts',(-19.8085028501753,20.3489381317363,124.549834241605)) ;
#66386=CARTESIAN_POINT('Ctrl Pts',(-19.6550087594271,20.5388752638742,124.899096739163)) ;
#66387=CARTESIAN_POINT('Ctrl Pts',(-19.6058699022926,20.3588861835113,124.601638844772)) ;
#66388=CARTESIAN_POINT('Ctrl Pts',(-19.3945515389815,20.5488166671527,124.919199688652)) ;
#66389=CARTESIAN_POINT('Ctrl Pts',(-19.3975068666403,20.3688275867898,124.617723886778)) ;
#66390=CARTESIAN_POINT('Ctrl Pts',(-19.0469745337114,20.5621033319336,124.885630332357)) ;
#66391=CARTESIAN_POINT('Ctrl Pts',(-19.1194311731786,20.3821142515707,124.590866211464)) ;
#66392=CARTESIAN_POINT('Ctrl Pts',(-18.6334863377988,20.5787137535884,124.731039345078)) ;
#66393=CARTESIAN_POINT('Ctrl Pts',(-18.788654663985,20.3987246732255,124.467201404259)) ;
#66394=CARTESIAN_POINT('Ctrl Pts',(-18.2305106418667,20.5986250158392,124.387975748647)) ;
#66395=CARTESIAN_POINT('Ctrl Pts',(-18.4662665446094,20.4186359354763,124.192751186382)) ;
#66396=CARTESIAN_POINT('Ctrl Pts',(-17.9681790722083,20.6185691450041,123.927324296484)) ;
#66397=CARTESIAN_POINT('Ctrl Pts',(-18.2563995729899,20.4385800646412,123.824231859657)) ;
#66398=CARTESIAN_POINT('Ctrl Pts',(-17.8789643904274,20.6384923076093,123.405418987404)) ;
#66399=CARTESIAN_POINT('Ctrl Pts',(-18.1850241788991,20.4585032272464,123.406707562409)) ;
#66400=CARTESIAN_POINT('Ctrl Pts',(-17.9722011638597,20.6583824300158,122.884976490813)) ;
#66401=CARTESIAN_POINT('Ctrl Pts',(-18.2596109762183,20.4783933496529,122.990352318436)) ;
#66402=CARTESIAN_POINT('Ctrl Pts',(-18.2392413285999,20.6783873836159,122.425297035635)) ;
#66403=CARTESIAN_POINT('Ctrl Pts',(-18.4732405399828,20.498398303253,122.622607344408)) ;
#66404=CARTESIAN_POINT('Ctrl Pts',(-18.6435876221089,20.6982256406315,122.086739272797)) ;
#66405=CARTESIAN_POINT('Ctrl Pts',(-18.7967168578306,20.5182365602686,122.35175829032)) ;
#66406=CARTESIAN_POINT('Ctrl Pts',(-19.1427514572152,20.718219941418,121.904613931299)) ;
#66407=CARTESIAN_POINT('Ctrl Pts',(-19.1960471830647,20.5382308610552,122.206055793577)) ;
#66408=CARTESIAN_POINT('Ctrl Pts',(-19.6712810445263,20.7381051834625,121.904239572849)) ;
#66409=CARTESIAN_POINT('Ctrl Pts',(-19.6188718571092,20.5581161030996,122.205753939832)) ;
#66410=CARTESIAN_POINT('Ctrl Pts',(-20.168447470455,20.7579801299384,122.082748587511)) ;
#66411=CARTESIAN_POINT('Ctrl Pts',(-20.0166067329943,20.5779910495756,122.348559983418)) ;
#66412=CARTESIAN_POINT('Ctrl Pts',(-20.5778609764888,20.7780131998795,122.423240113376)) ;
#66413=CARTESIAN_POINT('Ctrl Pts',(-20.3441382911306,20.5980241195166,122.620951670167)) ;
#66414=CARTESIAN_POINT('Ctrl Pts',(-20.8439482662448,20.7979017067799,122.879935963145)) ;
#66415=CARTESIAN_POINT('Ctrl Pts',(-20.5570102575303,20.617912626417,122.986308438082)) ;
#66416=CARTESIAN_POINT('Ctrl Pts',(-20.9398845189848,20.8177565665612,123.398932664504)) ;
#66417=CARTESIAN_POINT('Ctrl Pts',(-20.6337603893495,20.6377674861983,123.401507281384)) ;
#66418=CARTESIAN_POINT('Ctrl Pts',(-20.8512719992327,20.8378074003489,123.924305207163)) ;
#66419=CARTESIAN_POINT('Ctrl Pts',(-20.5628715067338,20.657818319986,123.821804891128)) ;
#66420=CARTESIAN_POINT('Ctrl Pts',(-20.5928049104702,20.8575733422382,124.381835472892)) ;
#66421=CARTESIAN_POINT('Ctrl Pts',(-20.3560969395519,20.6775842618753,124.187831867116)) ;
#66422=CARTESIAN_POINT('Ctrl Pts',(-20.1896580437569,20.8775860736975,124.728578782344)) ;
#66423=CARTESIAN_POINT('Ctrl Pts',(-20.0335794046623,20.6975969933346,124.465226382195)) ;
#66424=CARTESIAN_POINT('Ctrl Pts',(-19.6948360554275,20.8974789086411,124.915243821142)) ;
#66425=CARTESIAN_POINT('Ctrl Pts',(-19.6377205723978,20.7174898282782,124.61455887421)) ;
#66426=CARTESIAN_POINT('Ctrl Pts',(-19.1659236264529,20.9173859319806,124.922728039924)) ;
#66427=CARTESIAN_POINT('Ctrl Pts',(-19.2145894369091,20.7373968516177,124.620545637084)) ;
#66428=CARTESIAN_POINT('Ctrl Pts',(-18.6655619227043,20.9373011968813,124.749682544139)) ;
#66429=CARTESIAN_POINT('Ctrl Pts',(-18.8142995780805,20.7573121165184,124.482107923995)) ;
#66430=CARTESIAN_POINT('Ctrl Pts',(-18.2524397020174,20.957332889041,124.413908184194)) ;
#66431=CARTESIAN_POINT('Ctrl Pts',(-18.4838026915331,20.7773438086781,124.21348792732)) ;
#66432=CARTESIAN_POINT('Ctrl Pts',(-17.9811972981208,20.977175935614,123.961546540794)) ;
#66433=CARTESIAN_POINT('Ctrl Pts',(-18.2668088563855,20.7971868552511,123.8515965203)) ;
#66434=CARTESIAN_POINT('Ctrl Pts',(-17.8790621516814,20.9970924835138,123.442223784006)) ;
#66435=CARTESIAN_POINT('Ctrl Pts',(-18.1851023793624,20.8171034031509,123.436137129649)) ;
#66436=CARTESIAN_POINT('Ctrl Pts',(-17.9604499278885,21.0170247265051,122.918699625149)) ;
#66437=CARTESIAN_POINT('Ctrl Pts',(-18.2502146020831,20.8370356461422,123.017317483767)) ;
#66438=CARTESIAN_POINT('Ctrl Pts',(-18.2149540834011,21.0369285613144,122.454965536719)) ;
#66439=CARTESIAN_POINT('Ctrl Pts',(-18.4538202863488,20.8569394809515,122.646330486718)) ;
#66440=CARTESIAN_POINT('Ctrl Pts',(-18.6119399166127,21.0568289615019,122.105461255144)) ;
#66441=CARTESIAN_POINT('Ctrl Pts',(-18.7714112568372,20.876839881139,122.366728442058)) ;
#66442=CARTESIAN_POINT('Ctrl Pts',(-19.1055245267092,21.0767786378812,121.91171422936)) ;
#66443=CARTESIAN_POINT('Ctrl Pts',(-19.1662802778635,20.8967895575183,122.211733244875)) ;
#66444=CARTESIAN_POINT('Ctrl Pts',(-19.6351319246211,21.0967111621016,121.898157078062)) ;
#66445=CARTESIAN_POINT('Ctrl Pts',(-19.5899667460685,20.9167220817387,122.200890351572)) ;
#66446=CARTESIAN_POINT('Ctrl Pts',(-20.1374331359232,21.1166311710878,122.065615887878)) ;
#66447=CARTESIAN_POINT('Ctrl Pts',(-19.9918072525265,20.9366420907249,122.334860475937)) ;
#66448=CARTESIAN_POINT('Ctrl Pts',(-20.5530840765956,21.136588077264,122.395047352195)) ;
#66449=CARTESIAN_POINT('Ctrl Pts',(-20.3243262285862,20.9565989969011,122.598408332127)) ;
#66450=CARTESIAN_POINT('Ctrl Pts',(-20.8308668599276,21.1564739167655,122.844813593085)) ;
#66451=CARTESIAN_POINT('Ctrl Pts',(-20.5465500430235,20.9764848364026,122.958223574526)) ;
#66452=CARTESIAN_POINT('Ctrl Pts',(-20.9388483133597,21.1764450889013,123.364394953387)) ;
#66453=CARTESIAN_POINT('Ctrl Pts',(-20.6329313716892,20.9964560085384,123.373889855656)) ;
#66454=CARTESIAN_POINT('Ctrl Pts',(-20.8643333248033,21.1962592858857,123.885809151916)) ;
#66455=CARTESIAN_POINT('Ctrl Pts',(-20.5733172829464,21.0162702055228,123.791020397466)) ;
#66456=CARTESIAN_POINT('Ctrl Pts',(-20.6149914724651,21.2162404718539,124.35458992427)) ;
#66457=CARTESIAN_POINT('Ctrl Pts',(-20.3738339226301,21.0362513914911,124.166047707023)) ;
#66458=CARTESIAN_POINT('Ctrl Pts',(-20.2875771231592,21.2328159772432,124.649450004713)) ;
#66459=CARTESIAN_POINT('Ctrl Pts',(-20.1119198605758,21.0528268968803,124.401919518092)) ;
#66460=CARTESIAN_POINT('Ctrl Pts',(-19.976190695121,21.2461254251068,124.808734121278)) ;
#66461=CARTESIAN_POINT('Ctrl Pts',(-19.8627850672793,21.0661363447439,124.529357922434)) ;
#66462=CARTESIAN_POINT('Ctrl Pts',(-19.6403422561752,21.2594931228834,124.911767929916)) ;
#66463=CARTESIAN_POINT('Ctrl Pts',(-19.5941577979202,21.0795040425205,124.611771756262)) ;
#66464=CARTESIAN_POINT('Ctrl Pts',(-19.2023540010426,21.2759836945493,124.927912591737)) ;
#66465=CARTESIAN_POINT('Ctrl Pts',(-19.2437108124987,21.0959946141864,124.62469560568)) ;
#66466=CARTESIAN_POINT('Ctrl Pts',(-18.6980130161789,21.2959039668821,124.76705541604)) ;
#66467=CARTESIAN_POINT('Ctrl Pts',(-18.8402511097492,21.1159148865192,124.495996295646)) ;
#66468=CARTESIAN_POINT('Ctrl Pts',(-18.3484015779916,21.3125210026031,124.497134075246)) ;
#66469=CARTESIAN_POINT('Ctrl Pts',(-18.5605800541927,21.1325319222402,124.280076149471)) ;
#66470=CARTESIAN_POINT('Ctrl Pts',(-18.1364098503999,21.3258118528842,124.219524949621)) ;
#66471=CARTESIAN_POINT('Ctrl Pts',(-18.3909714359101,21.1458227725213,124.057970053224)) ;
#66472=CARTESIAN_POINT('Ctrl Pts',(-18.0158871388316,21.3357808980387,123.986950081581)) ;
#66473=CARTESIAN_POINT('Ctrl Pts',(-18.2945586408566,21.1557918176758,123.871912706625)) ;
#66474=CARTESIAN_POINT('Ctrl Pts',(-17.9375848219816,21.3456842886722,123.7387264045)) ;
#66475=CARTESIAN_POINT('Ctrl Pts',(-18.2319181148261,21.1656952083094,123.673331434388)) ;
#66476=CARTESIAN_POINT('Ctrl Pts',(-17.9031917373362,21.355742074785,123.476694986446)) ;
#66477=CARTESIAN_POINT('Ctrl Pts',(-18.2044053250832,21.1757529944221,123.463708741263)) ;
#66478=CARTESIAN_POINT('Ctrl Pts',(-17.9143537185253,21.3655941114347,123.218009520766)) ;
#66479=CARTESIAN_POINT('Ctrl Pts',(-18.2133399425486,21.1856050310718,123.256751469431)) ;
#66480=CARTESIAN_POINT('Ctrl Pts',(-17.9896212280947,21.3789592355779,122.874956968011)) ;
#66481=CARTESIAN_POINT('Ctrl Pts',(-18.2735425071571,21.198970155215,122.982353715324)) ;
#66482=CARTESIAN_POINT('Ctrl Pts',(-18.1513956643206,21.3921852985409,122.562838107837)) ;
#66483=CARTESIAN_POINT('Ctrl Pts',(-18.4029674268594,21.2121962181781,122.732632497982)) ;
#66484=CARTESIAN_POINT('Ctrl Pts',(-18.3866109363659,21.4054889468232,122.304222180962)) ;
#66485=CARTESIAN_POINT('Ctrl Pts',(-18.5911529954546,21.2254998664603,122.525730915353)) ;
#66486=CARTESIAN_POINT('Ctrl Pts',(-18.5942688365872,21.4154804779862,122.143483381919)) ;
#66487=CARTESIAN_POINT('Ctrl Pts',(-18.7572784100833,21.2354913976233,122.397143875669)) ;
#66488=CARTESIAN_POINT('Ctrl Pts',(-18.8279161165822,21.4255199257855,122.020995347853)) ;
#66489=CARTESIAN_POINT('Ctrl Pts',(-18.9441978151252,21.2455308454226,122.299154881713)) ;
#66490=CARTESIAN_POINT('Ctrl Pts',(-19.0743002770801,21.4353637012994,121.942115783865)) ;
#66491=CARTESIAN_POINT('Ctrl Pts',(-19.1413056995706,21.2553746209365,122.236053522357)) ;
#66492=CARTESIAN_POINT('Ctrl Pts',(-19.3342026170286,21.445349342687,121.90619908811)) ;
#66493=CARTESIAN_POINT('Ctrl Pts',(-19.3492278602432,21.2653602623241,122.207322374569)) ;
#66494=CARTESIAN_POINT('Ctrl Pts',(-19.5951977714836,21.4552861270488,121.915768063468)) ;
#66495=CARTESIAN_POINT('Ctrl Pts',(-19.5580238317526,21.2752970466859,122.214979818382)) ;
#66496=CARTESIAN_POINT('Ctrl Pts',(-19.8533761099886,21.4653359615162,121.971250859302)) ;
#66497=CARTESIAN_POINT('Ctrl Pts',(-19.7645659845222,21.2853468811533,122.259368252402)) ;
#66498=CARTESIAN_POINT('Ctrl Pts',(-20.0932613278945,21.4751864110193,122.068581121297)) ;
#66499=CARTESIAN_POINT('Ctrl Pts',(-19.9564732213435,21.2951973306564,122.337234519556)) ;
#66500=CARTESIAN_POINT('Ctrl Pts',(-20.3156279272745,21.4851584250014,122.207174295959)) ;
#66501=CARTESIAN_POINT('Ctrl Pts',(-20.1343652320431,21.3051693446385,122.448110919028)) ;
#66502=CARTESIAN_POINT('Ctrl Pts',(-20.5110376061981,21.4951535828485,122.382755229701)) ;
#66503=CARTESIAN_POINT('Ctrl Pts',(-20.290691427895,21.3151645024856,122.588577292965)) ;
#66504=CARTESIAN_POINT('Ctrl Pts',(-20.6733301023097,21.5051875092122,122.590546133602)) ;
#66505=CARTESIAN_POINT('Ctrl Pts',(-20.4205236271332,21.3251984288494,122.754811381595)) ;
#66506=CARTESIAN_POINT('Ctrl Pts',(-20.7952585397872,21.5150432176446,122.819075138393)) ;
#66507=CARTESIAN_POINT('Ctrl Pts',(-20.5180643101211,21.3350541372817,122.937635474695)) ;
#66508=CARTESIAN_POINT('Ctrl Pts',(-20.8771547988309,21.5250413669833,123.068682710145)) ;
#66509=CARTESIAN_POINT('Ctrl Pts',(-20.5835791727783,21.3450522866204,123.13732215833)) ;
#66510=CARTESIAN_POINT('Ctrl Pts',(-20.9143410126104,21.5349407701568,123.326195883179)) ;
#66511=CARTESIAN_POINT('Ctrl Pts',(-20.6133259222408,21.354951689794,123.343332810001)) ;
#66512=CARTESIAN_POINT('Ctrl Pts',(-20.9061846999684,21.5449919670453,123.590176807784)) ;
#66513=CARTESIAN_POINT('Ctrl Pts',(-20.6067986577069,21.3650028866824,123.554517489311)) ;
#66514=CARTESIAN_POINT('Ctrl Pts',(-20.853249823519,21.5548742908582,123.844441837906)) ;
#66515=CARTESIAN_POINT('Ctrl Pts',(-20.5644486425954,21.3748852104953,123.7579288163)) ;
#66516=CARTESIAN_POINT('Ctrl Pts',(-20.7564330306425,21.5648691865148,124.088593766656)) ;
#66517=CARTESIAN_POINT('Ctrl Pts',(-20.4869932187418,21.3848801061519,123.953249478274)) ;
#66518=CARTESIAN_POINT('Ctrl Pts',(-20.6179931768872,21.5748902858973,124.312627761359)) ;
#66519=CARTESIAN_POINT('Ctrl Pts',(-20.3762394774589,21.3949012055344,124.132475496053)) ;
#66520=CARTESIAN_POINT('Ctrl Pts',(-20.4449112034606,21.5847975537594,124.507113190861)) ;
#66521=CARTESIAN_POINT('Ctrl Pts',(-20.2377724303908,21.4048084733965,124.288062198318)) ;
#66522=CARTESIAN_POINT('Ctrl Pts',(-20.2403849662515,21.5947358975846,124.669500522451)) ;
#66523=CARTESIAN_POINT('Ctrl Pts',(-20.0741502752422,21.4147468172218,124.417970248963)) ;
#66524=CARTESIAN_POINT('Ctrl Pts',(-20.0093045735368,21.6047393168851,124.79489097273)) ;
#66525=CARTESIAN_POINT('Ctrl Pts',(-19.8892850037941,21.4247502365222,124.518280706296)) ;
#66526=CARTESIAN_POINT('Ctrl Pts',(-19.7590892507398,21.6147738675922,124.878084487071)) ;
#66527=CARTESIAN_POINT('Ctrl Pts',(-19.6891120481609,21.4347847872293,124.584833462809)) ;
#66528=CARTESIAN_POINT('Ctrl Pts',(-19.5031930456652,21.6246188171978,124.916282417656)) ;
#66529=CARTESIAN_POINT('Ctrl Pts',(-19.4843952188806,21.4446297368349,124.615389634999)) ;
#66530=CARTESIAN_POINT('Ctrl Pts',(-19.2408957415365,21.6346046593107,124.909864611199)) ;
#66531=CARTESIAN_POINT('Ctrl Pts',(-19.274557555605,21.4546155789478,124.610253310096)) ;
#66532=CARTESIAN_POINT('Ctrl Pts',(-18.9848863453834,21.6445394666798,124.858431106566)) ;
#66533=CARTESIAN_POINT('Ctrl Pts',(-19.0697507008442,21.4645503863169,124.569104541095)) ;
#66534=CARTESIAN_POINT('Ctrl Pts',(-18.738859338082,21.6545970083931,124.761963952245)) ;
#66535=CARTESIAN_POINT('Ctrl Pts',(-18.8729297698642,21.4746079280302,124.491928838993)) ;
#66536=CARTESIAN_POINT('Ctrl Pts',(-18.5183469904694,21.6644186059052,124.627779140097)) ;
#66537=CARTESIAN_POINT('Ctrl Pts',(-18.696521489678,21.4844295255424,124.384579574157)) ;
#66538=CARTESIAN_POINT('Ctrl Pts',(-18.3195680415686,21.6744748653857,124.453674665829)) ;
#66539=CARTESIAN_POINT('Ctrl Pts',(-18.5374995695825,21.4944857850228,124.245294444731)) ;
#66540=CARTESIAN_POINT('Ctrl Pts',(-18.1562878546674,21.6844148016861,124.249767117428)) ;
#66541=CARTESIAN_POINT('Ctrl Pts',(-18.4068771805631,21.5044257213232,124.082167340354)) ;
#66542=CARTESIAN_POINT('Ctrl Pts',(-18.0306281552504,21.6943219224305,124.021754765608)) ;
#66543=CARTESIAN_POINT('Ctrl Pts',(-18.3063513226383,21.5143328420676,123.899756895081)) ;
#66544=CARTESIAN_POINT('Ctrl Pts',(-17.9454073048491,21.7043648283558,123.771982422679)) ;
#66545=CARTESIAN_POINT('Ctrl Pts',(-18.2381764644056,21.5243757479929,123.699938324042)) ;
#66546=CARTESIAN_POINT('Ctrl Pts',(-17.9053416812303,21.714272609455,123.51470692144)) ;
#66547=CARTESIAN_POINT('Ctrl Pts',(-18.2061259509787,21.5342835290921,123.494118036696)) ;
#66548=CARTESIAN_POINT('Ctrl Pts',(-17.9101476585179,21.7242829784574,123.251680239082)) ;
#66549=CARTESIAN_POINT('Ctrl Pts',(-18.2099726089032,21.5442938980945,123.283696771005)) ;
#66550=CARTESIAN_POINT('Ctrl Pts',(-17.9611784249865,21.7343138170262,122.993069233019)) ;
#66551=CARTESIAN_POINT('Ctrl Pts',(-18.25079914997,21.5543247366633,123.076808307396)) ;
#66552=CARTESIAN_POINT('Ctrl Pts',(-18.0542181019441,21.7441666566659,122.751434398998)) ;
#66553=CARTESIAN_POINT('Ctrl Pts',(-18.3252324147839,21.564177576303,122.883501741555)) ;
#66554=CARTESIAN_POINT('Ctrl Pts',(-18.1892070598107,21.7541546578309,122.526357242308)) ;
#66555=CARTESIAN_POINT('Ctrl Pts',(-18.433225062823,21.574165577468,122.703441075812)) ;
#66556=CARTESIAN_POINT('Ctrl Pts',(-18.3602212353183,21.76408347681,122.32928753721)) ;
#66557=CARTESIAN_POINT('Ctrl Pts',(-18.5700375178516,21.5840943964472,122.545786794347)) ;
#66558=CARTESIAN_POINT('Ctrl Pts',(-18.5637837492857,21.7740711795323,122.163582862095)) ;
#66559=CARTESIAN_POINT('Ctrl Pts',(-18.7328885150387,21.5940820991695,122.413224497597)) ;
#66560=CARTESIAN_POINT('Ctrl Pts',(-18.7943281092038,21.784107179335,122.035521757821)) ;
#66561=CARTESIAN_POINT('Ctrl Pts',(-18.9173249461088,21.6041180989721,122.310777167978)) ;
#66562=CARTESIAN_POINT('Ctrl Pts',(-19.038997751584,21.7939620491364,121.950573239043)) ;
#66563=CARTESIAN_POINT('Ctrl Pts',(-19.1130605360951,21.6139729687736,122.242820240775)) ;
#66564=CARTESIAN_POINT('Ctrl Pts',(-19.2983295791008,21.80396147956,121.908451210414)) ;
#66565=CARTESIAN_POINT('Ctrl Pts',(-19.3205261622003,21.6239723991971,122.209124297681)) ;
#66566=CARTESIAN_POINT('Ctrl Pts',(-19.5583862373949,21.8138565970253,121.911683181411)) ;
#66567=CARTESIAN_POINT('Ctrl Pts',(-19.5285708804354,21.6338675166624,122.21171149709)) ;
#66568=CARTESIAN_POINT('Ctrl Pts',(-19.8181211650492,21.8239170905422,121.96083913654)) ;
#66569=CARTESIAN_POINT('Ctrl Pts',(-19.7363587075279,21.6439280101794,122.251037906807)) ;
#66570=CARTESIAN_POINT('Ctrl Pts',(-20.0602885784198,21.8337665707434,122.052271697296)) ;
#66571=CARTESIAN_POINT('Ctrl Pts',(-19.930091288856,21.6537774903805,122.324185167146)) ;
#66572=CARTESIAN_POINT('Ctrl Pts',(-20.2872285089844,21.8437930210072,122.186139952124)) ;
#66573=CARTESIAN_POINT('Ctrl Pts',(-20.1116425053652,21.6638039406443,122.431281064082)) ;
#66574=CARTESIAN_POINT('Ctrl Pts',(-20.4871079315352,21.8538243114853,122.35801891506)) ;
#66575=CARTESIAN_POINT('Ctrl Pts',(-20.2715450314613,21.6738352311224,122.568785502684)) ;
#66576=CARTESIAN_POINT('Ctrl Pts',(-20.6513791646752,21.8636656991371,122.557772038563)) ;
#66577=CARTESIAN_POINT('Ctrl Pts',(-20.4029602709634,21.6836766187742,122.728588256116)) ;
#66578=CARTESIAN_POINT('Ctrl Pts',(-20.7809938111829,21.8736691000283,122.786445434062)) ;
#66579=CARTESIAN_POINT('Ctrl Pts',(-20.5066507156167,21.6936800196655,122.91152759353)) ;
#66580=CARTESIAN_POINT('Ctrl Pts',(-20.8686887483206,21.8836534828195,123.033784325657)) ;
#66581=CARTESIAN_POINT('Ctrl Pts',(-20.5768052604981,21.7036644024566,123.109399027828)) ;
#66582=CARTESIAN_POINT('Ctrl Pts',(-20.9120839655183,21.8936925728329,123.293981074003)) ;
#66583=CARTESIAN_POINT('Ctrl Pts',(-20.6115199849103,21.71370349247,123.317556776986)) ;
#66584=CARTESIAN_POINT('Ctrl Pts',(-20.9100499298834,21.9035383817421,123.552730180815)) ;
#66585=CARTESIAN_POINT('Ctrl Pts',(-20.609891351577,21.7235493013792,123.524555112863)) ;
#66586=CARTESIAN_POINT('Ctrl Pts',(-20.8629939222876,21.9135228045611,123.810817924676)) ;
#66587=CARTESIAN_POINT('Ctrl Pts',(-20.5722453017055,21.7335337241982,123.73102487777)) ;
#66588=CARTESIAN_POINT('Ctrl Pts',(-20.7723283116897,21.9234624298023,124.05581995963)) ;
#66589=CARTESIAN_POINT('Ctrl Pts',(-20.4997117680828,21.7434733494394,123.927025654345)) ;
#66590=CARTESIAN_POINT('Ctrl Pts',(-20.6391479210158,21.9335021193209,124.283546922036)) ;
#66591=CARTESIAN_POINT('Ctrl Pts',(-20.3931662819036,21.7535130389581,124.109206674248)) ;
#66592=CARTESIAN_POINT('Ctrl Pts',(-20.4711013650952,21.9433903077395,124.481766445994)) ;
#66593=CARTESIAN_POINT('Ctrl Pts',(-20.2587285516933,21.7634012273766,124.267780913417)) ;
#66594=CARTESIAN_POINT('Ctrl Pts',(-20.2694747065142,21.9533798337416,124.649861363959)) ;
#66595=CARTESIAN_POINT('Ctrl Pts',(-20.097426616492,21.7733907533787,124.402255850537)) ;
#66596=CARTESIAN_POINT('Ctrl Pts',(-20.0423296292845,21.9633383350968,124.779814856002)) ;
#66597=CARTESIAN_POINT('Ctrl Pts',(-19.915710259167,21.7833492547339,124.506217429302)) ;
#66598=CARTESIAN_POINT('Ctrl Pts',(-19.7977240449736,21.9732379291004,124.868443422786)) ;
#66599=CARTESIAN_POINT('Ctrl Pts',(-19.7200260940079,21.7932488487375,124.577119050715)) ;
#66600=CARTESIAN_POINT('Ctrl Pts',(-19.5376330731142,21.9832858172217,124.913825837491)) ;
#66601=CARTESIAN_POINT('Ctrl Pts',(-19.5119529591425,21.8032967368588,124.61342395089)) ;
#66602=CARTESIAN_POINT('Ctrl Pts',(-19.2775503015537,21.9931812424672,124.913569399124)) ;
#66603=CARTESIAN_POINT('Ctrl Pts',(-19.3038874739033,21.8131921621044,124.613217771097)) ;
#66604=CARTESIAN_POINT('Ctrl Pts',(-19.017233305932,22.0032426331678,124.86744619023)) ;
#66605=CARTESIAN_POINT('Ctrl Pts',(-19.0956337981961,21.8232535528049,124.576318149791)) ;
#66606=CARTESIAN_POINT('Ctrl Pts',(-18.7741467328486,22.0130882168545,124.778797095436)) ;
#66607=CARTESIAN_POINT('Ctrl Pts',(-18.9011658833268,21.8330991364916,124.505398287498)) ;
#66608=CARTESIAN_POINT('Ctrl Pts',(-18.5470623486079,22.0230511901637,124.648524437436)) ;
#66609=CARTESIAN_POINT('Ctrl Pts',(-18.7194990790042,21.8430621098008,124.401179638259)) ;
#66610=CARTESIAN_POINT('Ctrl Pts',(-18.3449798305692,22.0330768569895,124.479454619294)) ;
#66611=CARTESIAN_POINT('Ctrl Pts',(-18.5578335854537,21.8530877766266,124.265923060778)) ;
#66612=CARTESIAN_POINT('Ctrl Pts',(-18.1771126653133,22.0429913348558,124.28020996493)) ;
#66613=CARTESIAN_POINT('Ctrl Pts',(-18.4235409199083,21.8630022544929,124.106527278134)) ;
#66614=CARTESIAN_POINT('Ctrl Pts',(-18.0449474119808,22.0529798495308,124.053398711337)) ;
#66615=CARTESIAN_POINT('Ctrl Pts',(-18.317809439298,21.8729907691679,123.925078062203)) ;
#66616=CARTESIAN_POINT('Ctrl Pts',(-17.954211848732,22.0630239604462,123.805561752125)) ;
#66617=CARTESIAN_POINT('Ctrl Pts',(-18.2452217507632,21.8830348800833,123.726808050528)) ;
#66618=CARTESIAN_POINT('Ctrl Pts',(-17.9082542485454,22.0728520980408,123.551371969022)) ;
#66619=CARTESIAN_POINT('Ctrl Pts',(-18.2084565831269,21.8928630176779,123.523457276199)) ;
#66620=CARTESIAN_POINT('Ctrl Pts',(-17.9069805912369,22.0829286660997,123.286627562761)) ;
#66621=CARTESIAN_POINT('Ctrl Pts',(-18.2074383400266,21.9029395857368,123.311661381763)) ;
#66622=CARTESIAN_POINT('Ctrl Pts',(-17.9505873022016,22.0927808280039,123.031363437666)) ;
#66623=CARTESIAN_POINT('Ctrl Pts',(-18.2423241725982,21.912791747641,123.107451229462)) ;
#66624=CARTESIAN_POINT('Ctrl Pts',(-18.0395690380517,22.1028537899607,122.782109150564)) ;
#66625=CARTESIAN_POINT('Ctrl Pts',(-18.3135102432881,21.9228647095978,122.908047671536)) ;
#66626=CARTESIAN_POINT('Ctrl Pts',(-18.1675496052933,22.1126963519636,122.557311692099)) ;
#66627=CARTESIAN_POINT('Ctrl Pts',(-18.4158946651662,21.9327072716007,122.728210991207)) ;
#66628=CARTESIAN_POINT('Ctrl Pts',(-18.3342296705409,22.1226767884574,122.354827390352)) ;
#66629=CARTESIAN_POINT('Ctrl Pts',(-18.5492388606532,21.9426877080945,122.566223989023)) ;
#66630=CARTESIAN_POINT('Ctrl Pts',(-18.5346278830778,22.1326950937818,122.184094281001)) ;
#66631=CARTESIAN_POINT('Ctrl Pts',(-18.7095577721264,21.9527060134189,122.429637890191)) ;
#66632=CARTESIAN_POINT('Ctrl Pts',(-18.7583362356547,22.1425790577013,122.052058163512)) ;
#66633=CARTESIAN_POINT('Ctrl Pts',(-18.8885238944235,21.9625899773384,122.32400976912)) ;
#66634=CARTESIAN_POINT('Ctrl Pts',(-19.0060171333251,22.1526449344398,121.959277593487)) ;
#66635=CARTESIAN_POINT('Ctrl Pts',(-19.0866690470502,21.9726558540769,122.249785576266)) ;
#66636=CARTESIAN_POINT('Ctrl Pts',(-19.2602098520566,22.1624840353007,121.911823353389)) ;
#66637=CARTESIAN_POINT('Ctrl Pts',(-19.2900221324471,21.9824949549378,122.211822750592)) ;
#66638=CARTESIAN_POINT('Ctrl Pts',(-19.5238350449174,22.1725171181664,121.908510218283)) ;
#66639=CARTESIAN_POINT('Ctrl Pts',(-19.5009223790608,21.9925280378036,122.209172428358)) ;
#66640=CARTESIAN_POINT('Ctrl Pts',(-19.7836614016497,22.1825388034419,121.951624796669)) ;
#66641=CARTESIAN_POINT('Ctrl Pts',(-19.7087834435619,22.002549723079,122.243664446075)) ;
#66642=CARTESIAN_POINT('Ctrl Pts',(-20.0283161574298,22.1924054985404,122.037437936202)) ;
#66643=CARTESIAN_POINT('Ctrl Pts',(-19.9045062201637,22.0124164181775,122.312314862293)) ;
#66644=CARTESIAN_POINT('Ctrl Pts',(-20.2568547840646,22.2023653882749,122.165037255751)) ;
#66645=CARTESIAN_POINT('Ctrl Pts',(-20.0873367614171,22.0223763079121,122.414394197747)) ;
#66646=CARTESIAN_POINT('Ctrl Pts',(-20.4610185638516,22.2124003761004,122.331922477437)) ;
#66647=CARTESIAN_POINT('Ctrl Pts',(-20.2506677635409,22.0324112957375,122.547902586744)) ;
#66648=CARTESIAN_POINT('Ctrl Pts',(-20.6309241388541,22.2222870801747,122.528528183517)) ;
#66649=CARTESIAN_POINT('Ctrl Pts',(-20.3865915994159,22.0422979998118,122.705186531169)) ;
#66650=CARTESIAN_POINT('Ctrl Pts',(-20.766416856272,22.2323522244076,122.755640405164)) ;
#66651=CARTESIAN_POINT('Ctrl Pts',(-20.4949858643928,22.0523631440447,122.88687662059)) ;
#66652=CARTESIAN_POINT('Ctrl Pts',(-20.8585847061565,22.2421915151362,122.997265190441)) ;
#66653=CARTESIAN_POINT('Ctrl Pts',(-20.5687197080449,22.0622024347733,123.080175347708)) ;
#66654=CARTESIAN_POINT('Ctrl Pts',(-20.9088481489483,22.2522540725746,123.256845872699)) ;
#66655=CARTESIAN_POINT('Ctrl Pts',(-20.6089305940997,22.0722649922117,123.287840171023)) ;
#66656=CARTESIAN_POINT('Ctrl Pts',(-20.9129252441028,22.2621511238267,123.516913308371)) ;
#66657=CARTESIAN_POINT('Ctrl Pts',(-20.6121922611426,22.0821620434638,123.495893317472)) ;
#66658=CARTESIAN_POINT('Ctrl Pts',(-20.8725051637196,22.272082330575,123.774739999813)) ;
#66659=CARTESIAN_POINT('Ctrl Pts',(-20.5798565101102,22.0920932502121,123.702154136205)) ;
#66660=CARTESIAN_POINT('Ctrl Pts',(-20.786712131682,22.2821245147938,124.024299304319)) ;
#66661=CARTESIAN_POINT('Ctrl Pts',(-20.5112221742166,22.1021354344309,123.901801786887)) ;
#66662=CARTESIAN_POINT('Ctrl Pts',(-20.6610284500015,22.2920111429047,124.25170115506)) ;
#66663=CARTESIAN_POINT('Ctrl Pts',(-20.4106758246915,22.1120220625418,124.083722603376)) ;
#66664=CARTESIAN_POINT('Ctrl Pts',(-20.4963649928319,22.3020044154371,124.45625910245)) ;
#66665=CARTESIAN_POINT('Ctrl Pts',(-20.2789454023778,22.1220153350742,124.247369029717)) ;
#66666=CARTESIAN_POINT('Ctrl Pts',(-20.2995680280399,22.3119494909786,124.628229064092)) ;
#66667=CARTESIAN_POINT('Ctrl Pts',(-20.1215083814713,22.1319604106157,124.384944899341)) ;
#66668=CARTESIAN_POINT('Ctrl Pts',(-20.0760548364874,22.3218990417068,124.763918115327)) ;
#66669=CARTESIAN_POINT('Ctrl Pts',(-19.9426984210111,22.141909961344,124.493496265617)) ;
#66670=CARTESIAN_POINT('Ctrl Pts',(-19.8301102215282,22.3319383765548,124.859349625922)) ;
#66671=CARTESIAN_POINT('Ctrl Pts',(-19.7459427347351,22.1519492961919,124.569841851037)) ;
#66672=CARTESIAN_POINT('Ctrl Pts',(-19.5752934234394,22.3418245154987,124.910085821145)) ;
#66673=CARTESIAN_POINT('Ctrl Pts',(-19.5420902200881,22.1618354351359,124.610431044817)) ;
#66674=CARTESIAN_POINT('Ctrl Pts',(-19.3126560173104,22.3518226284724,124.916205138615)) ;
#66675=CARTESIAN_POINT('Ctrl Pts',(-19.3319804315117,22.1718335481096,124.615326989773)) ;
#66676=CARTESIAN_POINT('Ctrl Pts',(-19.0548963059002,22.3617423908249,124.877085616116)) ;
#66677=CARTESIAN_POINT('Ctrl Pts',(-19.1257731976824,22.181753310462,124.584031994196)) ;
#66678=CARTESIAN_POINT('Ctrl Pts',(-18.8048804750818,22.3717817864375,124.792892259255)) ;
#66679=CARTESIAN_POINT('Ctrl Pts',(-18.9257602220697,22.1917927060747,124.51667778619)) ;
#66680=CARTESIAN_POINT('Ctrl Pts',(-18.5763093840162,22.3816909722258,124.668127742339)) ;
#66681=CARTESIAN_POINT('Ctrl Pts',(-18.7429037235827,22.2017018918629,124.41686698238)) ;
#66682=CARTESIAN_POINT('Ctrl Pts',(-18.3718830460784,22.3916261563833,124.505717216813)) ;
#66683=CARTESIAN_POINT('Ctrl Pts',(-18.5793626191556,22.2116370760204,124.286939448208)) ;
#66684=CARTESIAN_POINT('Ctrl Pts',(-18.1971172156532,22.4016672137692,124.308030847448)) ;
#66685=CARTESIAN_POINT('Ctrl Pts',(-18.4395493697844,22.2216781334063,124.128790671233)) ;
#66686=CARTESIAN_POINT('Ctrl Pts',(-18.0612726927552,22.4115543718025,124.086530580778)) ;
#66687=CARTESIAN_POINT('Ctrl Pts',(-18.330873593402,22.2315652914396,123.951591529793)) ;
#66688=CARTESIAN_POINT('Ctrl Pts',(-17.9645436848904,22.4215466514784,123.842428732897)) ;
#66689=CARTESIAN_POINT('Ctrl Pts',(-18.2534897026088,22.2415575711155,123.756310497809)) ;
#66690=CARTESIAN_POINT('Ctrl Pts',(-17.9119640315032,22.4314951685235,123.586318714181)) ;
#66691=CARTESIAN_POINT('Ctrl Pts',(-18.211425301115,22.2515060881606,123.551423064664)) ;
#66692=CARTESIAN_POINT('Ctrl Pts',(-17.9042933598069,22.4414319460939,123.325324977717)) ;
#66693=CARTESIAN_POINT('Ctrl Pts',(-18.2052879085007,22.261442865731,123.342628610746)) ;
#66694=CARTESIAN_POINT('Ctrl Pts',(-17.9419119920911,22.4514149822408,123.065658904093)) ;
#66695=CARTESIAN_POINT('Ctrl Pts',(-18.235381847005,22.2714259018779,123.134895818999)) ;
#66696=CARTESIAN_POINT('Ctrl Pts',(-18.0249844510094,22.4614587338345,122.815165001349)) ;
#66697=CARTESIAN_POINT('Ctrl Pts',(-18.3018390701171,22.2814696534717,122.934500290776)) ;
#66698=CARTESIAN_POINT('Ctrl Pts',(-18.1471041894676,22.4712872630471,122.587531223368)) ;
#66699=CARTESIAN_POINT('Ctrl Pts',(-18.3995334548748,22.2912981826842,122.752393822393)) ;
#66700=CARTESIAN_POINT('Ctrl Pts',(-18.310736925562,22.4813626239558,122.379445782567)) ;
#66701=CARTESIAN_POINT('Ctrl Pts',(-18.5304390610458,22.3013735435929,122.585924577045)) ;
#66702=CARTESIAN_POINT('Ctrl Pts',(-18.5037504475988,22.491219222843,122.2066258693)) ;
#66703=CARTESIAN_POINT('Ctrl Pts',(-18.684848467763,22.3112301424801,122.447668526044)) ;
#66704=CARTESIAN_POINT('Ctrl Pts',(-18.7282113464719,22.5012822168609,122.066906399844)) ;
#66705=CARTESIAN_POINT('Ctrl Pts',(-18.8644168289928,22.321293136498,122.335891884029)) ;
#66706=CARTESIAN_POINT('Ctrl Pts',(-18.9691081441337,22.5111601511503,121.970077874885)) ;
#66707=CARTESIAN_POINT('Ctrl Pts',(-19.0571331080001,22.3311710707875,122.258428360996)) ;
#66708=CARTESIAN_POINT('Ctrl Pts',(-19.2261379991879,22.5211607987084,121.915505689096)) ;
#66709=CARTESIAN_POINT('Ctrl Pts',(-19.2627566457403,22.3411717183456,122.214769480072)) ;
#66710=CARTESIAN_POINT('Ctrl Pts',(-19.4866516087189,22.5310786451465,121.906267040837)) ;
#66711=CARTESIAN_POINT('Ctrl Pts',(-19.4711669227681,22.3510895647836,122.207377364757)) ;
#66712=CARTESIAN_POINT('Ctrl Pts',(-19.7481817747748,22.5411297621521,121.942948938101)) ;
#66713=CARTESIAN_POINT('Ctrl Pts',(-19.6803913883822,22.3611406817893,122.236721714525)) ;
#66714=CARTESIAN_POINT('Ctrl Pts',(-19.9950390178656,22.5510004974627,122.022770439589)) ;
#66715=CARTESIAN_POINT('Ctrl Pts',(-19.8778767883679,22.3710114170999,122.300577456873)) ;
#66716=CARTESIAN_POINT('Ctrl Pts',(-20.2288742155722,22.5610712047057,122.146611832965)) ;
#66717=CARTESIAN_POINT('Ctrl Pts',(-20.0649457944915,22.3810821243429,122.399649573841)) ;
#66718=CARTESIAN_POINT('Ctrl Pts',(-20.432852059648,22.5709042121576,122.305284591667)) ;
#66719=CARTESIAN_POINT('Ctrl Pts',(-20.2281280611383,22.3909151317947,122.526586124132)) ;
#66720=CARTESIAN_POINT('Ctrl Pts',(-20.6101957114275,22.5809347044599,122.50028265826)) ;
#66721=CARTESIAN_POINT('Ctrl Pts',(-20.3700041091279,22.400945624097,122.682583647088)) ;
#66722=CARTESIAN_POINT('Ctrl Pts',(-20.7503657377508,22.5909662995333,122.723566173364)) ;
#66723=CARTESIAN_POINT('Ctrl Pts',(-20.4821412655094,22.4109772191704,122.861209824262)) ;
#66724=CARTESIAN_POINT('Ctrl Pts',(-20.848126630718,22.6007959986715,122.962648437251)) ;
#66725=CARTESIAN_POINT('Ctrl Pts',(-20.5603509034017,22.4208069183087,123.052474161789)) ;
#66726=CARTESIAN_POINT('Ctrl Pts',(-20.904551077241,22.6107854485531,123.219033095629)) ;
#66727=CARTESIAN_POINT('Ctrl Pts',(-20.6054919617955,22.4307963681902,123.257581413107)) ;
#66728=CARTESIAN_POINT('Ctrl Pts',(-20.9149919746047,22.6208293063688,123.482765312887)) ;
#66729=CARTESIAN_POINT('Ctrl Pts',(-20.6138461187708,22.4408402260059,123.46856724786)) ;
#66730=CARTESIAN_POINT('Ctrl Pts',(-20.8807975538298,22.630650996959,123.738595413769)) ;
#66731=CARTESIAN_POINT('Ctrl Pts',(-20.5864922425363,22.4506619165961,123.673230544663)) ;
#66732=CARTESIAN_POINT('Ctrl Pts',(-20.8016166335874,22.6406860874994,123.990134218036)) ;
#66733=CARTESIAN_POINT('Ctrl Pts',(-20.5231490649285,22.4606970071365,123.874462168931)) ;
#66734=CARTESIAN_POINT('Ctrl Pts',(-20.6794595798729,22.6507106064821,124.223553358068)) ;
#66735=CARTESIAN_POINT('Ctrl Pts',(-20.4254247725794,22.4707215261192,124.061198201126)) ;
#66736=CARTESIAN_POINT('Ctrl Pts',(-20.5216428899484,22.6605704518923,124.429030130044)) ;
#66737=CARTESIAN_POINT('Ctrl Pts',(-20.2991731733227,22.4805813715294,124.22557998796)) ;
#66738=CARTESIAN_POINT('Ctrl Pts',(-20.3290800370369,22.670530228208,124.606303874563)) ;
#66739=CARTESIAN_POINT('Ctrl Pts',(-20.1451242645067,22.4905411478451,124.367400086112)) ;
#66740=CARTESIAN_POINT('Ctrl Pts',(-20.1069583810948,22.6805584255226,124.748107125882)) ;
#66741=CARTESIAN_POINT('Ctrl Pts',(-19.9674278116215,22.5005693451597,124.480844120942)) ;
#66742=CARTESIAN_POINT('Ctrl Pts',(-19.8666123895492,22.6904659678129,124.848267265594)) ;
#66743=CARTESIAN_POINT('Ctrl Pts',(-19.7751521487821,22.51047688745,124.5609736348)) ;
#66744=CARTESIAN_POINT('Ctrl Pts',(-19.6093776535577,22.7004986183768,124.905971284957)) ;
#66745=CARTESIAN_POINT('Ctrl Pts',(-19.569364702959,22.5205095380139,124.607138561972)) ;
#66746=CARTESIAN_POINT('Ctrl Pts',(-19.349909838197,22.7103825748034,124.918032249207)) ;
#66747=CARTESIAN_POINT('Ctrl Pts',(-19.3617911229907,22.5303934944406,124.616789062543)) ;
#66748=CARTESIAN_POINT('Ctrl Pts',(-19.0894539708058,22.7203722761653,124.88515179817)) ;
#66749=CARTESIAN_POINT('Ctrl Pts',(-19.1534263193822,22.5403831958024,124.590486565815)) ;
#66750=CARTESIAN_POINT('Ctrl Pts',(-18.8375462307077,22.7304132714413,124.806612946757)) ;
#66751=CARTESIAN_POINT('Ctrl Pts',(-18.9518995301889,22.5504241910784,124.527657156544)) ;
#66752=CARTESIAN_POINT('Ctrl Pts',(-18.6077694357356,22.7402461607097,124.68841772116)) ;
#66753=CARTESIAN_POINT('Ctrl Pts',(-18.7680779300007,22.5602570803468,124.4331029628)) ;
#66754=CARTESIAN_POINT('Ctrl Pts',(-18.3981964690907,22.7502393190771,124.530174726569)) ;
#66755=CARTESIAN_POINT('Ctrl Pts',(-18.6004184592641,22.5702502387142,124.306510187023)) ;
#66756=CARTESIAN_POINT('Ctrl Pts',(-18.2189780474116,22.7602713614292,124.336812835409)) ;
#66757=CARTESIAN_POINT('Ctrl Pts',(-18.457042329262,22.5802822810663,124.151821925346)) ;
#66758=CARTESIAN_POINT('Ctrl Pts',(-18.078177052041,22.7701366053876,124.11914781899)) ;
#66759=CARTESIAN_POINT('Ctrl Pts',(-18.3444002370286,22.5901475250248,123.97769144434)) ;
#66760=CARTESIAN_POINT('Ctrl Pts',(-17.9756297430813,22.7800984966336,123.878272519234)) ;
#66761=CARTESIAN_POINT('Ctrl Pts',(-18.262360610908,22.6001094162708,123.784992180742)) ;
#66762=CARTESIAN_POINT('Ctrl Pts',(-17.9164527324428,22.7901333966521,123.621304920688)) ;
#66763=CARTESIAN_POINT('Ctrl Pts',(-18.2150170837711,22.6101443162892,123.579418516256)) ;
#66764=CARTESIAN_POINT('Ctrl Pts',(-17.9025653496462,22.8000184770667,123.361873137659)) ;
#66765=CARTESIAN_POINT('Ctrl Pts',(-18.2039051888414,22.6200293967038,123.371873646667)) ;
#66766=CARTESIAN_POINT('Ctrl Pts',(-17.9345250196897,22.8100836491915,123.099344214703)) ;
#66767=CARTESIAN_POINT('Ctrl Pts',(-18.229470937305,22.6300945688287,123.161850152158)) ;
#66768=CARTESIAN_POINT('Ctrl Pts',(-18.0097882001565,22.819930883915,122.851728714304)) ;
#66769=CARTESIAN_POINT('Ctrl Pts',(-18.2896793803027,22.6399418035521,122.963757680924)) ;
#66770=CARTESIAN_POINT('Ctrl Pts',(-18.1285132437623,22.8299616952328,122.616400101498)) ;
#66771=CARTESIAN_POINT('Ctrl Pts',(-18.3846575488646,22.6499726148699,122.775493825297)) ;
#66772=CARTESIAN_POINT('Ctrl Pts',(-18.2864226563192,22.8399713111463,122.40599165732)) ;
#66773=CARTESIAN_POINT('Ctrl Pts',(-18.5109834183892,22.6599822307834,122.607165884196)) ;
#66774=CARTESIAN_POINT('Ctrl Pts',(-18.4763564295643,22.84988209055,122.227822802769)) ;
#66775=CARTESIAN_POINT('Ctrl Pts',(-18.6629287774965,22.6698930101871,122.464629519222)) ;
#66776=CARTESIAN_POINT('Ctrl Pts',(-18.6944202111758,22.859811356339,122.084505529354)) ;
#66777=CARTESIAN_POINT('Ctrl Pts',(-18.8373784211579,22.6798222759761,122.349974053439)) ;
#66778=CARTESIAN_POINT('Ctrl Pts',(-18.9368601501301,22.8698540496516,121.980263237278)) ;
#66779=CARTESIAN_POINT('Ctrl Pts',(-19.0313295614933,22.6898649692887,122.266578267691)) ;
#66780=CARTESIAN_POINT('Ctrl Pts',(-19.1897096706424,22.8797405823464,121.920470478153)) ;
#66781=CARTESIAN_POINT('Ctrl Pts',(-19.2336083570812,22.6997515019835,122.218742067114)) ;
#66782=CARTESIAN_POINT('Ctrl Pts',(-19.4518420605083,22.8897337274496,121.904884777647)) ;
#66783=CARTESIAN_POINT('Ctrl Pts',(-19.4433140578841,22.7097446470868,122.206271347572)) ;
#66784=CARTESIAN_POINT('Ctrl Pts',(-19.7114632832621,22.8996794081237,121.935008316747)) ;
#66785=CARTESIAN_POINT('Ctrl Pts',(-19.6510111009045,22.7196903277608,122.230368013377)) ;
#66786=CARTESIAN_POINT('Ctrl Pts',(-19.9621146837926,22.9096266657504,122.009255961602)) ;
#66787=CARTESIAN_POINT('Ctrl Pts',(-19.8515326922247,22.7296375853876,122.289763976907)) ;
#66788=CARTESIAN_POINT('Ctrl Pts',(-20.1982818352397,22.9196745678719,122.127332902665)) ;
#66789=CARTESIAN_POINT('Ctrl Pts',(-20.0404673939253,22.739685487509,122.38422358596)) ;
#66790=CARTESIAN_POINT('Ctrl Pts',(-20.4062715090379,22.9295222734936,122.281319880695)) ;
#66791=CARTESIAN_POINT('Ctrl Pts',(-20.2068601821527,22.7495331931307,122.507411217)) ;
#66792=CARTESIAN_POINT('Ctrl Pts',(-20.5870134936696,22.9394837401277,122.470672801482)) ;
#66793=CARTESIAN_POINT('Ctrl Pts',(-20.3514553209462,22.7594946597648,122.658891935936)) ;
#66794=CARTESIAN_POINT('Ctrl Pts',(-20.7328386955894,22.9495132933959,122.690234279952)) ;
#66795=CARTESIAN_POINT('Ctrl Pts',(-20.4681173105457,22.769524213033,122.834539862625)) ;
#66796=CARTESIAN_POINT('Ctrl Pts',(-20.8371700436695,22.9594201854233,122.928761227148)) ;
#66797=CARTESIAN_POINT('Ctrl Pts',(-20.5515843614637,22.7794311050604,123.025360373342)) ;
#66798=CARTESIAN_POINT('Ctrl Pts',(-20.8992391770811,22.9693678295363,123.182677656175)) ;
#66799=CARTESIAN_POINT('Ctrl Pts',(-20.6012418268376,22.7893787491735,123.228492885336)) ;
#66800=CARTESIAN_POINT('Ctrl Pts',(-20.9165341377211,22.9793678725652,123.444932969306)) ;
#66801=CARTESIAN_POINT('Ctrl Pts',(-20.6150800337761,22.7993787922023,123.438296931167)) ;
#66802=CARTESIAN_POINT('Ctrl Pts',(-20.8874593437994,22.9894066385592,123.707113721901)) ;
#66803=CARTESIAN_POINT('Ctrl Pts',(-20.5918224275554,22.8094175581963,123.648041733911)) ;
#66804=CARTESIAN_POINT('Ctrl Pts',(-20.8153966815368,22.9992317005814,123.955064177239)) ;
#66805=CARTESIAN_POINT('Ctrl Pts',(-20.5341744977842,22.8192426202186,123.846402585896)) ;
#66806=CARTESIAN_POINT('Ctrl Pts',(-20.6991206973961,23.0092862479078,124.192308936938)) ;
#66807=CARTESIAN_POINT('Ctrl Pts',(-20.4411557498176,22.8292971675449,124.036199358367)) ;
#66808=CARTESIAN_POINT('Ctrl Pts',(-20.5447615013441,23.019229491357,124.403151003466)) ;
#66809=CARTESIAN_POINT('Ctrl Pts',(-20.3176702602204,22.8392404109942,124.204874274932)) ;
#66810=CARTESIAN_POINT('Ctrl Pts',(-20.357481348229,23.0291316629649,124.583821375332)) ;
#66811=CARTESIAN_POINT('Ctrl Pts',(-20.1678477266094,22.849142582602,124.349412166951)) ;
#66812=CARTESIAN_POINT('Ctrl Pts',(-20.1383129462667,23.0391844985751,124.731298547748)) ;
#66813=CARTESIAN_POINT('Ctrl Pts',(-19.9925143364415,22.8591954182122,124.4673957384)) ;
#66814=CARTESIAN_POINT('Ctrl Pts',(-19.9012076725115,23.0490575562606,124.836667408501)) ;
#66815=CARTESIAN_POINT('Ctrl Pts',(-19.8028309876301,22.8690684758978,124.551692871464)) ;
#66816=CARTESIAN_POINT('Ctrl Pts',(-19.6464624451115,23.0590528177863,124.90066823185)) ;
#66817=CARTESIAN_POINT('Ctrl Pts',(-19.5990355883761,22.8790637374234,124.602895734181)) ;
#66818=CARTESIAN_POINT('Ctrl Pts',(-19.3836439744441,23.0690781872068,124.919051527796)) ;
#66819=CARTESIAN_POINT('Ctrl Pts',(-19.3887803013881,22.8890891068439,124.617604464544)) ;
#66820=CARTESIAN_POINT('Ctrl Pts',(-19.1251242692714,23.0789680197334,124.892233416081)) ;
#66821=CARTESIAN_POINT('Ctrl Pts',(-19.1819670497776,22.8989789393705,124.59615274981)) ;
#66822=CARTESIAN_POINT('Ctrl Pts',(-18.7890035337137,23.0922659905428,124.796782825436)) ;
#66823=CARTESIAN_POINT('Ctrl Pts',(-18.9130558291102,22.9122769101799,124.519792421691)) ;
#66824=CARTESIAN_POINT('Ctrl Pts',(-18.4874072190834,23.105464385652,124.617549791502)) ;
#66825=CARTESIAN_POINT('Ctrl Pts',(-18.6717586476981,22.9254753052891,124.376385659626)) ;
#66826=CARTESIAN_POINT('Ctrl Pts',(-18.2417519026231,23.1188598279314,124.365440342986)) ;
#66827=CARTESIAN_POINT('Ctrl Pts',(-18.4752682092803,22.9388707475686,124.1747301264)) ;
#66828=CARTESIAN_POINT('Ctrl Pts',(-18.0954516814504,23.1287356661704,124.151032241541)) ;
#66829=CARTESIAN_POINT('Ctrl Pts',(-18.3582189589316,22.9487465858075,124.003198627306)) ;
#66830=CARTESIAN_POINT('Ctrl Pts',(-17.9865146772214,23.1387970687681,123.910158781384)) ;
#66831=CARTESIAN_POINT('Ctrl Pts',(-18.2710692167074,22.9588079884053,123.810502898505)) ;
#66832=CARTESIAN_POINT('Ctrl Pts',(-17.922240462111,23.1486621257033,123.658970587668)) ;
#66833=CARTESIAN_POINT('Ctrl Pts',(-18.2196477108387,22.9686730453404,123.60955078964)) ;
#66834=CARTESIAN_POINT('Ctrl Pts',(-17.9018022904604,23.1586742216521,123.396691351192)) ;
#66835=CARTESIAN_POINT('Ctrl Pts',(-18.2032931318325,22.9786851412892,123.399733036954)) ;
#66836=CARTESIAN_POINT('Ctrl Pts',(-17.9355630207714,23.1719515307975,123.049376976604)) ;
#66837=CARTESIAN_POINT('Ctrl Pts',(-18.230309065925,22.9919624504346,123.121854826151)) ;
#66838=CARTESIAN_POINT('Ctrl Pts',(-18.0899419028751,23.1885505563048,122.636110521846)) ;
#66839=CARTESIAN_POINT('Ctrl Pts',(-18.3537865821073,23.0085614759419,122.791280237995)) ;
#66840=CARTESIAN_POINT('Ctrl Pts',(-18.3760258329839,23.2051496043378,122.300311520429)) ;
#66841=CARTESIAN_POINT('Ctrl Pts',(-18.5826974346445,23.025160523975,122.522589580736)) ;
#66842=CARTESIAN_POINT('Ctrl Pts',(-18.6623130734036,23.2183930163688,122.102367993719)) ;
#66843=CARTESIAN_POINT('Ctrl Pts',(-18.8116871062911,23.0384039360059,122.364269513183)) ;
#66844=CARTESIAN_POINT('Ctrl Pts',(-18.9019676656497,23.2284304440572,121.992209381467)) ;
#66845=CARTESIAN_POINT('Ctrl Pts',(-19.0034183798067,23.0484413636943,122.27613348672)) ;
#66846=CARTESIAN_POINT('Ctrl Pts',(-19.1537511180854,23.2383347460128,121.926257438649)) ;
#66847=CARTESIAN_POINT('Ctrl Pts',(-19.2048396762017,23.0583456656499,122.223371601155)) ;
#66848=CARTESIAN_POINT('Ctrl Pts',(-19.5011668383559,23.251601585988,121.896906683047)) ;
#66849=CARTESIAN_POINT('Ctrl Pts',(-19.4827890606653,23.0716125056251,122.199889201105)) ;
#66850=CARTESIAN_POINT('Ctrl Pts',(-19.9361152832958,23.2682277840779,121.974875772965)) ;
#66851=CARTESIAN_POINT('Ctrl Pts',(-19.8307319806188,23.088238703715,122.262263124349)) ;
#66852=CARTESIAN_POINT('Ctrl Pts',(-20.394142712814,23.2881468994613,122.240416456631)) ;
#66853=CARTESIAN_POINT('Ctrl Pts',(-20.1971528580598,23.1081578190985,122.474678337376)) ;
#66854=CARTESIAN_POINT('Ctrl Pts',(-20.6777956763041,23.3047533225956,122.578559316856)) ;
#66855=CARTESIAN_POINT('Ctrl Pts',(-20.4241051196912,23.1247642422327,122.745236815236)) ;
#66856=CARTESIAN_POINT('Ctrl Pts',(-20.8254141685684,23.3180495430913,122.895260367424)) ;
#66857=CARTESIAN_POINT('Ctrl Pts',(-20.5421769247472,23.1380604627284,122.998554989249)) ;
#66858=CARTESIAN_POINT('Ctrl Pts',(-20.9163840285696,23.3313183754327,123.231954203337)) ;
#66859=CARTESIAN_POINT('Ctrl Pts',(-20.614959974584,23.1513292950698,123.26792816828)) ;
#66860=CARTESIAN_POINT('Ctrl Pts',(-20.9167633041339,23.3480096234658,123.675476169135)) ;
#66861=CARTESIAN_POINT('Ctrl Pts',(-20.6152647077734,23.1680205431029,123.622731052057)) ;
#66862=CARTESIAN_POINT('Ctrl Pts',(-20.7380527826187,23.3678193551386,124.170798980292)) ;
#66863=CARTESIAN_POINT('Ctrl Pts',(-20.4722993945024,23.1878302747757,124.018996228655)) ;
#66864=CARTESIAN_POINT('Ctrl Pts',(-20.3990487800684,23.3877969624672,124.579436972735)) ;
#66865=CARTESIAN_POINT('Ctrl Pts',(-20.2010981192601,23.2078078821043,124.345907297091)) ;
#66866=CARTESIAN_POINT('Ctrl Pts',(-19.9416700356385,23.407723271525,124.846309372867)) ;
#66867=CARTESIAN_POINT('Ctrl Pts',(-19.8351962131263,23.2277341911621,124.559408404364)) ;
#66868=CARTESIAN_POINT('Ctrl Pts',(-19.423672280542,23.4275401316897,124.942420637845)) ;
#66869=CARTESIAN_POINT('Ctrl Pts',(-19.4207968852883,23.2475510513268,124.636299832249)) ;
#66870=CARTESIAN_POINT('Ctrl Pts',(-18.897005210854,23.4476399472837,124.853997620555)) ;
#66871=CARTESIAN_POINT('Ctrl Pts',(-18.9994637104009,23.2676508669208,124.565563970077)) ;
#66872=CARTESIAN_POINT('Ctrl Pts',(-18.4395858732156,23.4673969111663,124.595670036021)) ;
#66873=CARTESIAN_POINT('Ctrl Pts',(-18.6335252687433,23.2874078308034,124.358902707329)) ;
#66874=CARTESIAN_POINT('Ctrl Pts',(-18.0924014778527,23.4874338372357,124.192088863914)) ;
#66875=CARTESIAN_POINT('Ctrl Pts',(-18.3557767077419,23.3074447568728,124.036039090244)) ;
#66876=CARTESIAN_POINT('Ctrl Pts',(-17.9060208621862,23.5073034196172,123.697826439083)) ;
#66877=CARTESIAN_POINT('Ctrl Pts',(-18.206670079505,23.3273143392544,123.64062860021)) ;
#66878=CARTESIAN_POINT('Ctrl Pts',(-17.8981510516399,23.5272079913704,123.168957382108)) ;
#66879=CARTESIAN_POINT('Ctrl Pts',(-18.2003731028714,23.3472189110075,123.217532238313)) ;
#66880=CARTESIAN_POINT('Ctrl Pts',(-18.0717585757874,23.5471605935689,122.667777463739)) ;
#66881=CARTESIAN_POINT('Ctrl Pts',(-18.3392584148753,23.367171513206,122.816587536918)) ;
#66882=CARTESIAN_POINT('Ctrl Pts',(-18.4052588840874,23.5670700845392,122.257079257931)) ;
#66883=CARTESIAN_POINT('Ctrl Pts',(-18.6060587086755,23.3870810041763,122.488027567399)) ;
#66884=CARTESIAN_POINT('Ctrl Pts',(-18.8570010753677,23.5869214532386,121.984239388305)) ;
#66885=CARTESIAN_POINT('Ctrl Pts',(-18.9674541463767,23.4069323728757,122.269754763327)) ;
#66886=CARTESIAN_POINT('Ctrl Pts',(-19.3806182677798,23.6070016493746,121.881570519937)) ;
#66887=CARTESIAN_POINT('Ctrl Pts',(-19.3863468682687,23.4270125690117,122.187619790065)) ;
#66888=CARTESIAN_POINT('Ctrl Pts',(-19.9007519851589,23.62680259295,121.962636023239)) ;
#66889=CARTESIAN_POINT('Ctrl Pts',(-19.8024563004733,23.4468135125871,122.252472687978)) ;
#66890=CARTESIAN_POINT('Ctrl Pts',(-20.366645013507,23.6467865694595,122.217519363045)) ;
#66891=CARTESIAN_POINT('Ctrl Pts',(-20.1751704371761,23.4667974890966,122.456380235725)) ;
#66892=CARTESIAN_POINT('Ctrl Pts',(-20.7158350928187,23.6667025324351,122.615335633075)) ;
#66893=CARTESIAN_POINT('Ctrl Pts',(-20.4545226369622,23.4867134520722,122.774634459819)) ;
#66894=CARTESIAN_POINT('Ctrl Pts',(-20.909269753505,23.686572967257,123.106869748193)) ;
#66895=CARTESIAN_POINT('Ctrl Pts',(-20.6092694713509,23.5065838868942,123.167863591692)) ;
#66896=CARTESIAN_POINT('Ctrl Pts',(-20.922587690353,23.7066232524901,123.639453176953)) ;
#66897=CARTESIAN_POINT('Ctrl Pts',(-20.6199224768603,23.5266341721272,123.593929874628)) ;
#66898=CARTESIAN_POINT('Ctrl Pts',(-20.7562955195823,23.7263972212494,124.138232320058)) ;
#66899=CARTESIAN_POINT('Ctrl Pts',(-20.4868863698106,23.5464081408865,123.992954730668)) ;
#66900=CARTESIAN_POINT('Ctrl Pts',(-20.4256681461167,23.746453679369,124.556107455173)) ;
#66901=CARTESIAN_POINT('Ctrl Pts',(-20.2223831283312,23.5664645990061,124.327253151564)) ;
#66902=CARTESIAN_POINT('Ctrl Pts',(-19.9777988611578,23.76624856236,124.832456311627)) ;
#66903=CARTESIAN_POINT('Ctrl Pts',(-19.8640850333811,23.5862594819971,124.548331359068)) ;
#66904=CARTESIAN_POINT('Ctrl Pts',(-19.4586032621524,23.7862152176623,124.941723989977)) ;
#66905=CARTESIAN_POINT('Ctrl Pts',(-19.4487277454471,23.6062261372994,124.635742813942)) ;
#66906=CARTESIAN_POINT('Ctrl Pts',(-18.9333997951415,23.8061741877388,124.86638911577)) ;
#66907=CARTESIAN_POINT('Ctrl Pts',(-19.0285650781102,23.6261851073759,124.575472274884)) ;
#66908=CARTESIAN_POINT('Ctrl Pts',(-18.466838553606,23.8260702753289,124.617539311619)) ;
#66909=CARTESIAN_POINT('Ctrl Pts',(-18.6553167537536,23.6460811949661,124.376389529742)) ;
#66910=CARTESIAN_POINT('Ctrl Pts',(-18.1127087822637,23.8459684452405,124.224807490326)) ;
#66911=CARTESIAN_POINT('Ctrl Pts',(-18.3720148240515,23.6659793648776,124.062201436306)) ;
#66912=CARTESIAN_POINT('Ctrl Pts',(-17.9132245363324,23.8658742806076,123.734750368409)) ;
#66913=CARTESIAN_POINT('Ctrl Pts',(-18.2124303796564,23.6858852002447,123.670153955737)) ;
#66914=CARTESIAN_POINT('Ctrl Pts',(-17.8929172316979,23.8858242055455,123.204950398228)) ;
#66915=CARTESIAN_POINT('Ctrl Pts',(-18.1961880248625,23.7058351251827,123.246313584245)) ;
#66916=CARTESIAN_POINT('Ctrl Pts',(-18.0536055022471,23.9057033954559,122.701563671004)) ;
#66917=CARTESIAN_POINT('Ctrl Pts',(-18.3247423344152,23.725714315093,122.843604744158)) ;
#66918=CARTESIAN_POINT('Ctrl Pts',(-18.3778029519875,23.9256847197365,122.280987362701)) ;
#66919=CARTESIAN_POINT('Ctrl Pts',(-18.584103378577,23.7456956393736,122.507146042841)) ;
#66920=CARTESIAN_POINT('Ctrl Pts',(-18.8251843464588,23.9456145039448,121.997171158723)) ;
#66921=CARTESIAN_POINT('Ctrl Pts',(-18.9420106639801,23.765625423582,122.280096052287)) ;
#66922=CARTESIAN_POINT('Ctrl Pts',(-19.3420527237489,23.9655344933356,121.8830575886)) ;
#66923=CARTESIAN_POINT('Ctrl Pts',(-19.3555069146509,23.7855454129728,122.188809484294)) ;
#66924=CARTESIAN_POINT('Ctrl Pts',(-19.8655341729859,23.9853896886896,121.950798016933)) ;
#66925=CARTESIAN_POINT('Ctrl Pts',(-19.7742905208817,23.8054006083268,122.243004187493)) ;
#66926=CARTESIAN_POINT('Ctrl Pts',(-20.3385180584329,24.005435690349,122.195770834828)) ;
#66927=CARTESIAN_POINT('Ctrl Pts',(-20.1526809568724,23.8254466099861,122.438992919313)) ;
#66928=CARTESIAN_POINT('Ctrl Pts',(-20.6359495242104,24.0219354375588,122.518207743344)) ;
#66929=CARTESIAN_POINT('Ctrl Pts',(-20.3906069626951,23.8419463571959,122.696923825608)) ;
#66930=CARTESIAN_POINT('Ctrl Pts',(-20.7997715920691,24.0353240420069,122.829526935845)) ;
#66931=CARTESIAN_POINT('Ctrl Pts',(-20.5216768386143,23.855334961644,122.945999782161)) ;
#66932=CARTESIAN_POINT('Ctrl Pts',(-20.8788004514205,24.0451858703418,123.076353832387)) ;
#66933=CARTESIAN_POINT('Ctrl Pts',(-20.5848955788943,23.8651967899789,123.143455681254)) ;
#66934=CARTESIAN_POINT('Ctrl Pts',(-20.9149604443776,24.0551520130994,123.335751428972)) ;
#66935=CARTESIAN_POINT('Ctrl Pts',(-20.6138199293417,23.8751629327365,123.350985772304)) ;
#66936=CARTESIAN_POINT('Ctrl Pts',(-20.9016757192965,24.0685137592243,123.68657640661)) ;
#66937=CARTESIAN_POINT('Ctrl Pts',(-20.6032002770534,23.8885246788614,123.631591920217)) ;
#66938=CARTESIAN_POINT('Ctrl Pts',(-20.7738010339285,24.0849680881794,124.104947280262)) ;
#66939=CARTESIAN_POINT('Ctrl Pts',(-20.5008787101127,23.9049790078165,123.966355119094)) ;
#66940=CARTESIAN_POINT('Ctrl Pts',(-20.506074005893,24.1017353332277,124.460989068715)) ;
#66941=CARTESIAN_POINT('Ctrl Pts',(-20.2867199296873,23.9217462528648,124.251141688073)) ;
#66942=CARTESIAN_POINT('Ctrl Pts',(-20.2328267963323,24.1149218985017,124.674311881725)) ;
#66943=CARTESIAN_POINT('Ctrl Pts',(-20.0681001136612,23.9349328181389,124.421823903416)) ;
#66944=CARTESIAN_POINT('Ctrl Pts',(-20.0014355866622,24.1249113572463,124.798149275947)) ;
#66945=CARTESIAN_POINT('Ctrl Pts',(-19.8829901714832,23.9449222768835,124.520886542304)) ;
#66946=CARTESIAN_POINT('Ctrl Pts',(-19.7528479925732,24.1348651297274,124.879719694348)) ;
#66947=CARTESIAN_POINT('Ctrl Pts',(-19.6841183272593,23.9548760493646,124.586142147501)) ;
#66948=CARTESIAN_POINT('Ctrl Pts',(-19.4914820582763,24.1449129462601,124.917021763208)) ;
#66949=CARTESIAN_POINT('Ctrl Pts',(-19.4750256307248,23.9649238658972,124.615981190194)) ;
#66950=CARTESIAN_POINT('Ctrl Pts',(-19.2329600579686,24.1547544793826,124.90885452434)) ;
#66951=CARTESIAN_POINT('Ctrl Pts',(-19.268207989371,23.9747653990197,124.609445249634)) ;
#66952=CARTESIAN_POINT('Ctrl Pts',(-18.9760140363379,24.1647407216023,124.855708116863)) ;
#66953=CARTESIAN_POINT('Ctrl Pts',(-19.0626517155432,23.9847516412394,124.566925893019)) ;
#66954=CARTESIAN_POINT('Ctrl Pts',(-18.7332816198796,24.1746773450272,124.759326036302)) ;
#66955=CARTESIAN_POINT('Ctrl Pts',(-18.8684666629235,23.9946882646643,124.489818160608)) ;
#66956=CARTESIAN_POINT('Ctrl Pts',(-18.5085675410313,24.1847272224102,124.620623799681)) ;
#66957=CARTESIAN_POINT('Ctrl Pts',(-18.6886966289881,24.0047381420473,124.378854470344)) ;
#66958=CARTESIAN_POINT('Ctrl Pts',(-18.3151003354371,24.1945776611878,124.448610838)) ;
#66959=CARTESIAN_POINT('Ctrl Pts',(-18.5339244352023,24.0145885808249,124.241242476954)) ;
#66960=CARTESIAN_POINT('Ctrl Pts',(-18.1519526133633,24.2045496751565,124.243579488805)) ;
#66961=CARTESIAN_POINT('Ctrl Pts',(-18.4034080760509,24.0245605947936,124.077216069596)) ;
#66962=CARTESIAN_POINT('Ctrl Pts',(-18.0265886284109,24.2145448437826,124.012717326557)) ;
#66963=CARTESIAN_POINT('Ctrl Pts',(-18.303118890646,24.0345557634197,123.892525324631)) ;
#66964=CARTESIAN_POINT('Ctrl Pts',(-17.9432101173695,24.2245787270438,123.762588848226)) ;
#66965=CARTESIAN_POINT('Ctrl Pts',(-18.2364182327103,24.0445896466809,123.692421857217)) ;
#66966=CARTESIAN_POINT('Ctrl Pts',(-17.9048199953682,24.2344345971071,123.506429025599)) ;
#66967=CARTESIAN_POINT('Ctrl Pts',(-18.2057083811246,24.0544455167443,123.487493852008)) ;
#66968=CARTESIAN_POINT('Ctrl Pts',(-17.9111670277577,24.2444321430243,123.243809194865)) ;
#66969=CARTESIAN_POINT('Ctrl Pts',(-18.2107882352827,24.0644430626614,123.277398119021)) ;
#66970=CARTESIAN_POINT('Ctrl Pts',(-17.9624791058961,24.2543402699236,122.988529382377)) ;
#66971=CARTESIAN_POINT('Ctrl Pts',(-18.2518400388648,24.0743511895607,123.073174891986)) ;
#66972=CARTESIAN_POINT('Ctrl Pts',(-18.0578908532251,24.2643506414457,122.743365948088)) ;
#66973=CARTESIAN_POINT('Ctrl Pts',(-18.3281714650137,24.0843615610829,122.877044994232)) ;
#66974=CARTESIAN_POINT('Ctrl Pts',(-18.1951870356825,24.2743810841931,122.518367543358)) ;
#66975=CARTESIAN_POINT('Ctrl Pts',(-18.4380103114372,24.0943920038303,122.697047441839)) ;
#66976=CARTESIAN_POINT('Ctrl Pts',(-18.3658593160879,24.2842290367464,122.323803295538)) ;
#66977=CARTESIAN_POINT('Ctrl Pts',(-18.574549574067,24.1042399563836,122.541397733003)) ;
#66978=CARTESIAN_POINT('Ctrl Pts',(-18.5719589574334,24.2942917057674,122.158164871478)) ;
#66979=CARTESIAN_POINT('Ctrl Pts',(-18.7394306821448,24.1143026254045,122.408888674427)) ;
#66980=CARTESIAN_POINT('Ctrl Pts',(-18.7999455381362,24.3041860812313,122.033096218261)) ;
#66981=CARTESIAN_POINT('Ctrl Pts',(-18.9218207704429,24.1241970008685,122.308835803467)) ;
#66982=CARTESIAN_POINT('Ctrl Pts',(-19.0470862012802,24.3141278795495,121.948467825779)) ;
#66983=CARTESIAN_POINT('Ctrl Pts',(-19.1195337945076,24.1341387991866,122.24113518591)) ;
#66984=CARTESIAN_POINT('Ctrl Pts',(-19.306793360523,24.3241303732768,121.9076794678)) ;
#66985=CARTESIAN_POINT('Ctrl Pts',(-19.3272997862454,24.1441412929139,122.208506614045)) ;
#66986=CARTESIAN_POINT('Ctrl Pts',(-19.5704262020177,24.3341651717837,121.913035104117)) ;
#66987=CARTESIAN_POINT('Ctrl Pts',(-19.5382060289476,24.1541760914208,122.212793292696)) ;
#66988=CARTESIAN_POINT('Ctrl Pts',(-19.8243456090835,24.3440100557631,121.962698662003)) ;
#66989=CARTESIAN_POINT('Ctrl Pts',(-19.7413407004111,24.1640209754002,122.252526140925)) ;
#66990=CARTESIAN_POINT('Ctrl Pts',(-20.069363913774,24.3539959125811,122.056545067836)) ;
#66991=CARTESIAN_POINT('Ctrl Pts',(-19.937354478382,24.1740068322182,122.327605165077)) ;
#66992=CARTESIAN_POINT('Ctrl Pts',(-20.2933885436929,24.3639307267559,122.190706447143)) ;
#66993=CARTESIAN_POINT('Ctrl Pts',(-20.1165729005004,24.183941646393,122.434935898804)) ;
#66994=CARTESIAN_POINT('Ctrl Pts',(-20.4929322997301,24.3739882265412,122.363960667453)) ;
#66995=CARTESIAN_POINT('Ctrl Pts',(-20.2762066070936,24.1939991461783,122.573540913657)) ;
#66996=CARTESIAN_POINT('Ctrl Pts',(-20.6558088061112,24.3838099849595,122.564221525997)) ;
#66997=CARTESIAN_POINT('Ctrl Pts',(-20.4065058327547,24.2038209045966,122.733750399107)) ;
#66998=CARTESIAN_POINT('Ctrl Pts',(-20.7848399620391,24.3938656427435,122.794804496023)) ;
#66999=CARTESIAN_POINT('Ctrl Pts',(-20.5097290712294,24.2138765623806,122.918217820985)) ;
#67000=CARTESIAN_POINT('Ctrl Pts',(-20.8704564403244,24.4038078249235,123.041662828752)) ;
#67001=CARTESIAN_POINT('Ctrl Pts',(-20.5782202377542,24.2238187445607,123.11570490205)) ;
#67002=CARTESIAN_POINT('Ctrl Pts',(-20.9125354801232,24.4137130336182,123.298533938)) ;
#67003=CARTESIAN_POINT('Ctrl Pts',(-20.6118814893409,24.2337239532553,123.321201684156)) ;
#67004=CARTESIAN_POINT('Ctrl Pts',(-20.909246248355,24.4237548245807,123.562396507273)) ;
#67005=CARTESIAN_POINT('Ctrl Pts',(-20.6092481539301,24.2437657442178,123.532291786414)) ;
#67006=CARTESIAN_POINT('Ctrl Pts',(-20.8608714359243,24.4336625990529,123.818239689833)) ;
#67007=CARTESIAN_POINT('Ctrl Pts',(-20.5705464711203,24.25367351869,123.736965560673)) ;
#67008=CARTESIAN_POINT('Ctrl Pts',(-20.7683009426795,24.4436740992805,124.064515066611)) ;
#67009=CARTESIAN_POINT('Ctrl Pts',(-20.496488335269,24.2636850189176,123.933985158452)) ;
#67010=CARTESIAN_POINT('Ctrl Pts',(-20.6336219825576,24.4537068596732,124.291169915681)) ;
#67011=CARTESIAN_POINT('Ctrl Pts',(-20.388743464398,24.2737177793103,124.115308070656)) ;
#67012=CARTESIAN_POINT('Ctrl Pts',(-20.4650972755638,24.4635574288081,124.487670909562)) ;
#67013=CARTESIAN_POINT('Ctrl Pts',(-20.2539226994214,24.2835683484452,124.272507129792)) ;
#67014=CARTESIAN_POINT('Ctrl Pts',(-20.262546647733,24.473546038338,124.654592807145)) ;
#67015=CARTESIAN_POINT('Ctrl Pts',(-20.0918811554699,24.2935569579751,124.40604315333)) ;
#67016=CARTESIAN_POINT('Ctrl Pts',(-20.035434390892,24.4834746943621,124.783046651201)) ;
#67017=CARTESIAN_POINT('Ctrl Pts',(-19.910190795979,24.3034856139992,124.508804458404)) ;
#67018=CARTESIAN_POINT('Ctrl Pts',(-19.788147480938,24.4934624405399,124.871054527459)) ;
#67019=CARTESIAN_POINT('Ctrl Pts',(-19.7123608220074,24.313473360177,124.579209069275)) ;
#67020=CARTESIAN_POINT('Ctrl Pts',(-19.5280364525962,24.5034984294756,124.914557400059)) ;
#67021=CARTESIAN_POINT('Ctrl Pts',(-19.5042716307132,24.3235093491128,124.614009587492)) ;
#67022=CARTESIAN_POINT('Ctrl Pts',(-19.2690459880752,24.5133532992892,124.912706949231)) ;
#67023=CARTESIAN_POINT('Ctrl Pts',(-19.2970800077781,24.3333642189264,124.612527489391)) ;
#67024=CARTESIAN_POINT('Ctrl Pts',(-19.0105743992336,24.523352740531,124.865592193593)) ;
#67025=CARTESIAN_POINT('Ctrl Pts',(-19.0903031443664,24.3433636601681,124.574834047047)) ;
#67026=CARTESIAN_POINT('Ctrl Pts',(-18.7666019329129,24.5332478147111,124.775498416424)) ;
#67027=CARTESIAN_POINT('Ctrl Pts',(-18.8951262877469,24.3532587343482,124.502757699957)) ;
#67028=CARTESIAN_POINT('Ctrl Pts',(-18.5383021509909,24.5433084705508,124.642232833805)) ;
#67029=CARTESIAN_POINT('Ctrl Pts',(-18.7124871214675,24.3633193901879,124.39614372167)) ;
#67030=CARTESIAN_POINT('Ctrl Pts',(-18.3407179161461,24.5531573447464,124.475027408876)) ;
#67031=CARTESIAN_POINT('Ctrl Pts',(-18.5544214106381,24.3731682643835,124.262378691614)) ;
#67032=CARTESIAN_POINT('Ctrl Pts',(-18.1716495641239,24.5631860567097,124.272865839476)) ;
#67033=CARTESIAN_POINT('Ctrl Pts',(-18.4191678481287,24.3831969763468,124.100648461118)) ;
#67034=CARTESIAN_POINT('Ctrl Pts',(-18.0408595712216,24.5732154572928,124.044039432676)) ;
#67035=CARTESIAN_POINT('Ctrl Pts',(-18.3145372315862,24.3932263769299,123.917586479356)) ;
#67036=CARTESIAN_POINT('Ctrl Pts',(-17.9529267054046,24.5830556509096,123.80085466428)) ;
#67037=CARTESIAN_POINT('Ctrl Pts',(-18.2441926703123,24.4030665705467,123.723039009644)) ;
#67038=CARTESIAN_POINT('Ctrl Pts',(-17.9073440510645,24.5930590734848,123.541984051105)) ;
#67039=CARTESIAN_POINT('Ctrl Pts',(-18.2077279538104,24.4130699931219,123.515942359835)) ;
#67040=CARTESIAN_POINT('Ctrl Pts',(-17.9074876720707,24.6030446105779,123.279530447817)) ;
#67041=CARTESIAN_POINT('Ctrl Pts',(-18.2078442820345,24.423055530215,123.305979644887)) ;
#67042=CARTESIAN_POINT('Ctrl Pts',(-17.953701474388,24.6130856150647,123.019767558698)) ;
#67043=CARTESIAN_POINT('Ctrl Pts',(-18.2448168072216,24.4330965347018,123.098169488521)) ;
#67044=CARTESIAN_POINT('Ctrl Pts',(-18.0422190940517,24.6229291540059,122.776684574555)) ;
#67045=CARTESIAN_POINT('Ctrl Pts',(-18.3156319085525,24.442940073643,122.903704466201)) ;
#67046=CARTESIAN_POINT('Ctrl Pts',(-18.1729536422505,24.6329141849967,122.549220386111)) ;
#67047=CARTESIAN_POINT('Ctrl Pts',(-18.42022057525,24.4529251046338,122.72173393716)) ;
#67048=CARTESIAN_POINT('Ctrl Pts',(-18.3403982888488,24.6428536475187,122.348704583029)) ;
#67049=CARTESIAN_POINT('Ctrl Pts',(-18.5541769923721,24.4628645671558,122.56132244681)) ;
#67050=CARTESIAN_POINT('Ctrl Pts',(-18.5421236161833,24.6528933797425,122.178692975382)) ;
#67051=CARTESIAN_POINT('Ctrl Pts',(-18.7155581760706,24.4729042993796,122.425314071837)) ;
#67052=CARTESIAN_POINT('Ctrl Pts',(-18.766826532383,24.6627815600597,122.048158969798)) ;
#67053=CARTESIAN_POINT('Ctrl Pts',(-18.8953205045771,24.4827924796968,122.320888330278)) ;
#67054=CARTESIAN_POINT('Ctrl Pts',(-19.0130885634454,24.6727710757622,121.957251380598)) ;
#67055=CARTESIAN_POINT('Ctrl Pts',(-19.0923303688238,24.4927819953993,122.248163402219)) ;
#67056=CARTESIAN_POINT('Ctrl Pts',(-19.2706307855915,24.6827296264169,121.910828202634)) ;
#67057=CARTESIAN_POINT('Ctrl Pts',(-19.2983640185096,24.502740546054,122.211026103761)) ;
#67058=CARTESIAN_POINT('Ctrl Pts',(-19.5307897392351,24.6926290335219,121.909185754216)) ;
#67059=CARTESIAN_POINT('Ctrl Pts',(-19.5064904836855,24.5126399531591,122.209713204043)) ;
#67060=CARTESIAN_POINT('Ctrl Pts',(-19.7910790035536,24.7026776199382,121.953496342207)) ;
#67061=CARTESIAN_POINT('Ctrl Pts',(-19.7147218884372,24.5226885395753,122.245162768907)) ;
#67062=CARTESIAN_POINT('Ctrl Pts',(-20.0360311856884,24.7125704389027,122.040742561825)) ;
#67063=CARTESIAN_POINT('Ctrl Pts',(-19.9106825930213,24.5325813585398,122.31496045899)) ;
#67064=CARTESIAN_POINT('Ctrl Pts',(-20.2660472328048,24.7226415564325,122.171540812148)) ;
#67065=CARTESIAN_POINT('Ctrl Pts',(-20.0946951781208,24.5426524760696,122.419600117649)) ;
#67066=CARTESIAN_POINT('Ctrl Pts',(-20.4649896868534,24.7324572503985,122.33580820644)) ;
#67067=CARTESIAN_POINT('Ctrl Pts',(-20.2538475822672,24.5524681700357,122.55101399222)) ;
#67068=CARTESIAN_POINT('Ctrl Pts',(-20.6368834830163,24.7425236278958,122.536807653796)) ;
#67069=CARTESIAN_POINT('Ctrl Pts',(-20.3913621437234,24.562534547533,122.711814344018)) ;
#67070=CARTESIAN_POINT('Ctrl Pts',(-20.7690258159267,24.7524226139777,122.760956322212)) ;
#67071=CARTESIAN_POINT('Ctrl Pts',(-20.4970748780025,24.5724335336148,122.891133115402)) ;
#67072=CARTESIAN_POINT('Ctrl Pts',(-20.8617232642626,24.7624767939712,123.008312860307)) ;
#67073=CARTESIAN_POINT('Ctrl Pts',(-20.5712320948138,24.5824877136083,123.089018856006)) ;
#67074=CARTESIAN_POINT('Ctrl Pts',(-20.9094544648808,24.7723476069039,123.263341038962)) ;
#67075=CARTESIAN_POINT('Ctrl Pts',(-20.6094160886339,24.592358526541,123.293040642391)) ;
#67076=CARTESIAN_POINT('Ctrl Pts',(-20.9122265609454,24.7824215077577,123.527995577717)) ;
#67077=CARTESIAN_POINT('Ctrl Pts',(-20.6116329563875,24.6024324273948,123.504764628738)) ;
#67078=CARTESIAN_POINT('Ctrl Pts',(-20.8703860648763,24.7922416631444,123.782706579754)) ;
#67079=CARTESIAN_POINT('Ctrl Pts',(-20.5781600363798,24.6122525827815,123.708532082081)) ;
#67080=CARTESIAN_POINT('Ctrl Pts',(-20.7829843523247,24.8023203700966,124.032658419494)) ;
#67081=CARTESIAN_POINT('Ctrl Pts',(-20.5082379034631,24.6223312897337,123.90849368722)) ;
#67082=CARTESIAN_POINT('Ctrl Pts',(-20.6564437174401,24.8121719586354,124.258586397133)) ;
#67083=CARTESIAN_POINT('Ctrl Pts',(-20.4070053415969,24.6321828782725,124.08923482883)) ;
#67084=CARTESIAN_POINT('Ctrl Pts',(-20.4891628443996,24.8222450751604,124.463680852311)) ;
#67085=CARTESIAN_POINT('Ctrl Pts',(-20.2731799578671,24.6422559947975,124.253310286516)) ;
#67086=CARTESIAN_POINT('Ctrl Pts',(-20.2933179390205,24.8320875922562,124.632670356776)) ;
#67087=CARTESIAN_POINT('Ctrl Pts',(-20.116504494174,24.6520985118933,124.388500688278)) ;
#67088=CARTESIAN_POINT('Ctrl Pts',(-20.0684748873038,24.8420680538102,124.767681031673)) ;
#67089=CARTESIAN_POINT('Ctrl Pts',(-19.9366300648084,24.6620789734473,124.496508766413)) ;
#67090=CARTESIAN_POINT('Ctrl Pts',(-19.8224883546883,24.8520863038009,124.861485946865)) ;
#67091=CARTESIAN_POINT('Ctrl Pts',(-19.7398406470911,24.6720972234381,124.571552218075)) ;
#67092=CARTESIAN_POINT('Ctrl Pts',(-19.5674837085229,24.8619704639947,124.911020996683)) ;
#67093=CARTESIAN_POINT('Ctrl Pts',(-19.535837716226,24.6819813836318,124.611179716792)) ;
#67094=CARTESIAN_POINT('Ctrl Pts',(-19.3030511330044,24.8720356109697,124.915550386411)) ;
#67095=CARTESIAN_POINT('Ctrl Pts',(-19.3242913349557,24.6920465306068,124.614802835819)) ;
#67096=CARTESIAN_POINT('Ctrl Pts',(-19.0475737608601,24.8818774346105,124.875152002711)) ;
#67097=CARTESIAN_POINT('Ctrl Pts',(-19.1199106517723,24.7018883542476,124.582483957355)) ;
#67098=CARTESIAN_POINT('Ctrl Pts',(-18.7981220481967,24.8919069070713,124.790082006543)) ;
#67099=CARTESIAN_POINT('Ctrl Pts',(-18.9203492635413,24.7119178267085,124.514427763563)) ;
#67100=CARTESIAN_POINT('Ctrl Pts',(-18.5676370265376,24.9019337623334,124.662373648599)) ;
#67101=CARTESIAN_POINT('Ctrl Pts',(-18.7359613597194,24.7219446819705,124.41226071562)) ;
#67102=CARTESIAN_POINT('Ctrl Pts',(-18.3661893963596,24.9117770124439,124.500103756191)) ;
#67103=CARTESIAN_POINT('Ctrl Pts',(-18.5748042848117,24.731787932081,124.282445362066)) ;
#67104=CARTESIAN_POINT('Ctrl Pts',(-18.1921666070184,24.9218254520271,124.30150622892)) ;
#67105=CARTESIAN_POINT('Ctrl Pts',(-18.4355860078039,24.7418363716642,124.123567103051)) ;
#67106=CARTESIAN_POINT('Ctrl Pts',(-18.056967678217,24.931774946275,124.077710500125)) ;
#67107=CARTESIAN_POINT('Ctrl Pts',(-18.3274273007974,24.7517858659121,123.944530798796)) ;
#67108=CARTESIAN_POINT('Ctrl Pts',(-17.9623422828139,24.941682802001,123.835129981)) ;
#67109=CARTESIAN_POINT('Ctrl Pts',(-18.25172727253,24.7616937216381,123.750467050901)) ;
#67110=CARTESIAN_POINT('Ctrl Pts',(-17.9107761380726,24.9517422786509,123.575884197323)) ;
#67111=CARTESIAN_POINT('Ctrl Pts',(-18.2104744001724,24.771753198288,123.543070133189)) ;
#67112=CARTESIAN_POINT('Ctrl Pts',(-17.9047808645182,24.9615830880596,123.317314560702)) ;
#67113=CARTESIAN_POINT('Ctrl Pts',(-18.2056782172109,24.7815940076967,123.336215598447)) ;
#67114=CARTESIAN_POINT('Ctrl Pts',(-17.9443132377084,24.9716452383604,123.055891956674)) ;
#67115=CARTESIAN_POINT('Ctrl Pts',(-18.237304086214,24.7916561579975,123.127077212028)) ;
#67116=CARTESIAN_POINT('Ctrl Pts',(-18.027522505227,24.981542399483,122.809459900675)) ;
#67117=CARTESIAN_POINT('Ctrl Pts',(-18.3038712398251,24.8015533191201,122.929932325436)) ;
#67118=CARTESIAN_POINT('Ctrl Pts',(-18.15191407074,24.991473573887,122.580036852208)) ;
#67119=CARTESIAN_POINT('Ctrl Pts',(-18.4033840182732,24.8114844935241,122.746394285566)) ;
#67120=CARTESIAN_POINT('Ctrl Pts',(-18.3162936300384,25.001515777612,122.373591256392)) ;
#67121=CARTESIAN_POINT('Ctrl Pts',(-18.5348876504328,24.8215266972492,122.581237583697)) ;
#67122=CARTESIAN_POINT('Ctrl Pts',(-18.5108445770742,25.0114023600425,122.201377852405)) ;
#67123=CARTESIAN_POINT('Ctrl Pts',(-18.6905276243258,24.8314132796796,122.443467286876)) ;
#67124=CARTESIAN_POINT('Ctrl Pts',(-18.7344855027603,25.0213957957908,122.063738108185)) ;
#67125=CARTESIAN_POINT('Ctrl Pts',(-18.8694400641659,24.8414067154279,122.333355312054)) ;
#67126=CARTESIAN_POINT('Ctrl Pts',(-18.9774777481212,25.031340264149,121.967563232072)) ;
#67127=CARTESIAN_POINT('Ctrl Pts',(-19.0638333079419,24.8513511837861,122.256415320713)) ;
#67128=CARTESIAN_POINT('Ctrl Pts',(-19.2335763972328,25.0412920803945,121.914516693683)) ;
#67129=CARTESIAN_POINT('Ctrl Pts',(-19.2687117105756,24.8613030000317,122.213977773435)) ;
#67130=CARTESIAN_POINT('Ctrl Pts',(-19.4972265998584,25.051329516509,121.906917954592)) ;
#67131=CARTESIAN_POINT('Ctrl Pts',(-19.4796319935927,24.8713404361461,122.207898425137)) ;
#67132=CARTESIAN_POINT('Ctrl Pts',(-19.7542997604475,25.0612144756854,121.944387345544)) ;
#67133=CARTESIAN_POINT('Ctrl Pts',(-19.6852897308738,24.8812253953225,122.237873404825)) ;
#67134=CARTESIAN_POINT('Ctrl Pts',(-20.0038315528282,25.0712125938973,122.026544562977)) ;
#67135=CARTESIAN_POINT('Ctrl Pts',(-19.8849152007323,24.8912235135344,122.303598670447)) ;
#67136=CARTESIAN_POINT('Ctrl Pts',(-20.2336588620757,25.0811335264093,122.149690526495)) ;
#67137=CARTESIAN_POINT('Ctrl Pts',(-20.0687767521282,24.9011444460464,122.402114675573)) ;
#67138=CARTESIAN_POINT('Ctrl Pts',(-20.4411095234431,25.0911748266313,122.31274727971)) ;
#67139=CARTESIAN_POINT('Ctrl Pts',(-20.2347377340864,24.9111857462685,122.532559732178)) ;
#67140=CARTESIAN_POINT('Ctrl Pts',(-20.6146855652456,25.1010817450213,122.506787487702)) ;
#67141=CARTESIAN_POINT('Ctrl Pts',(-20.3735984857151,24.9210926646584,122.687791010339)) ;
#67142=CARTESIAN_POINT('Ctrl Pts',(-20.7529678400047,25.1110175367304,122.728267052382)) ;
#67143=CARTESIAN_POINT('Ctrl Pts',(-20.4842246343113,24.9310284563675,122.86497383834)) ;
#67144=CARTESIAN_POINT('Ctrl Pts',(-20.8514767358832,25.1210584313083,122.973046599286)) ;
#67145=CARTESIAN_POINT('Ctrl Pts',(-20.5630324089093,24.9410693509454,123.060797371555)) ;
#67146=CARTESIAN_POINT('Ctrl Pts',(-20.9053425589782,25.1309456330221,123.227241473632)) ;
#67147=CARTESIAN_POINT('Ctrl Pts',(-20.6061255751286,24.9509565526592,123.264152313877)) ;
#67148=CARTESIAN_POINT('Ctrl Pts',(-20.9147827032288,25.1409379007837,123.489640019812)) ;
#67149=CARTESIAN_POINT('Ctrl Pts',(-20.6136784849478,24.9609488204208,123.474070959372)) ;
#67150=CARTESIAN_POINT('Ctrl Pts',(-20.8786010725189,25.1508864218055,123.748576028363)) ;
#67151=CARTESIAN_POINT('Ctrl Pts',(-20.5847340147397,24.9708973414426,123.681219445159)) ;
#67152=CARTESIAN_POINT('Ctrl Pts',(-20.7984664179347,25.1608231953832,123.997081667606)) ;
#67153=CARTESIAN_POINT('Ctrl Pts',(-20.5206272762469,24.9808341150203,123.880023738464)) ;
#67154=CARTESIAN_POINT('Ctrl Pts',(-20.6760989906385,25.1708062435242,124.229175844446)) ;
#67155=CARTESIAN_POINT('Ctrl Pts',(-20.4227342680816,24.9908171631614,124.065699340434)) ;
#67156=CARTESIAN_POINT('Ctrl Pts',(-20.5139718407011,25.1808499511343,124.437414474404)) ;
#67157=CARTESIAN_POINT('Ctrl Pts',(-20.2930331145472,25.0008608707714,124.232290876119)) ;
#67158=CARTESIAN_POINT('Ctrl Pts',(-20.3226951495202,25.1906786442876,124.611032523133)) ;
#67159=CARTESIAN_POINT('Ctrl Pts',(-20.1400132673799,25.0106895639247,124.371185263449)) ;
#67160=CARTESIAN_POINT('Ctrl Pts',(-20.098868954127,25.200753393417,124.752367074633)) ;
#67161=CARTESIAN_POINT('Ctrl Pts',(-19.9609525783771,25.0207643130542,124.484253941825)) ;
#67162=CARTESIAN_POINT('Ctrl Pts',(-19.858910190644,25.2106187192126,124.850577176108)) ;
#67163=CARTESIAN_POINT('Ctrl Pts',(-19.7689867940253,25.0306296388497,124.562822605687)) ;
#67164=CARTESIAN_POINT('Ctrl Pts',(-19.6016970937392,25.2206408935695,124.907156637884)) ;
#67165=CARTESIAN_POINT('Ctrl Pts',(-19.5632165305531,25.0406518132067,124.608087310509)) ;
#67166=CARTESIAN_POINT('Ctrl Pts',(-19.33841109203,25.2306669467765,124.91757426496)) ;
#67167=CARTESIAN_POINT('Ctrl Pts',(-19.3525877130776,25.0506778664136,124.616422422536)) ;
#67168=CARTESIAN_POINT('Ctrl Pts',(-19.0817846505437,25.2405206436227,124.883149004069)) ;
#67169=CARTESIAN_POINT('Ctrl Pts',(-19.1472873801373,25.0605315632599,124.588883436946)) ;
#67170=CARTESIAN_POINT('Ctrl Pts',(-18.8321213569949,25.2504800483757,124.804588928289)) ;
#67171=CARTESIAN_POINT('Ctrl Pts',(-18.9475566863649,25.0704909680128,124.526036697892)) ;
#67172=CARTESIAN_POINT('Ctrl Pts',(-18.5982908950502,25.2605182940806,124.68251138002)) ;
#67173=CARTESIAN_POINT('Ctrl Pts',(-18.7604916748522,25.0805292137177,124.428375651128)) ;
#67174=CARTESIAN_POINT('Ctrl Pts',(-18.3923032184799,25.2703924782426,124.52465527997)) ;
#67175=CARTESIAN_POINT('Ctrl Pts',(-18.5957014002325,25.0904033978798,124.302092277131)) ;
#67176=CARTESIAN_POINT('Ctrl Pts',(-18.2134348354326,25.2804622613806,124.32968799242)) ;
#67177=CARTESIAN_POINT('Ctrl Pts',(-18.4526055652732,25.1004731810177,124.146119103615)) ;
#67178=CARTESIAN_POINT('Ctrl Pts',(-18.0743301698985,25.2902955164013,124.111890050986)) ;
#67179=CARTESIAN_POINT('Ctrl Pts',(-18.341321285219,25.1103064360384,123.971882314404)) ;
#67180=CARTESIAN_POINT('Ctrl Pts',(-17.9724906536207,25.300325942533,123.868778335182)) ;
#67181=CARTESIAN_POINT('Ctrl Pts',(-18.2598482995309,25.1203368621701,123.777393441329)) ;
#67182=CARTESIAN_POINT('Ctrl Pts',(-17.9151462002579,25.31035755472,123.611455902983)) ;
#67183=CARTESIAN_POINT('Ctrl Pts',(-18.213971454411,25.1303684743571,123.571535713818)) ;
#67184=CARTESIAN_POINT('Ctrl Pts',(-17.9030533678709,25.3201872515746,123.353441667699)) ;
#67185=CARTESIAN_POINT('Ctrl Pts',(-18.2042958249843,25.1401981712117,123.365125405049)) ;
#67186=CARTESIAN_POINT('Ctrl Pts',(-17.935703946638,25.3301766934771,123.092960405583)) ;
#67187=CARTESIAN_POINT('Ctrl Pts',(-18.2304147144429,25.1501876131142,123.156740340782)) ;
#67188=CARTESIAN_POINT('Ctrl Pts',(-18.01414488107,25.3402205854928,122.840945210804)) ;
#67189=CARTESIAN_POINT('Ctrl Pts',(-18.293166125743,25.1602315051299,122.955127645986)) ;
#67190=CARTESIAN_POINT('Ctrl Pts',(-18.1320014123289,25.350042147262,122.611326074322)) ;
#67191=CARTESIAN_POINT('Ctrl Pts',(-18.3874495259112,25.1700530668991,122.771432519081)) ;
#67192=CARTESIAN_POINT('Ctrl Pts',(-18.290812004256,25.3600777188862,122.400775785575)) ;
#67193=CARTESIAN_POINT('Ctrl Pts',(-18.5144967171378,25.1800886385233,122.602991221329)) ;
#67194=CARTESIAN_POINT('Ctrl Pts',(-18.4841839838092,25.370106993168,122.221692735608)) ;
#67195=CARTESIAN_POINT('Ctrl Pts',(-18.6691932985931,25.1901179128051,122.459723641306)) ;
#67196=CARTESIAN_POINT('Ctrl Pts',(-18.7010269361118,25.3799408302867,122.081101987193)) ;
#67197=CARTESIAN_POINT('Ctrl Pts',(-18.8426660234848,25.1999517499238,122.347250143643)) ;
#67198=CARTESIAN_POINT('Ctrl Pts',(-18.9441309444256,25.3899932263748,121.977771975232)) ;
#67199=CARTESIAN_POINT('Ctrl Pts',(-19.037148711284,25.2100041460119,122.264584503233)) ;
#67200=CARTESIAN_POINT('Ctrl Pts',(-19.1986250893084,25.3999299933253,121.919230643914)) ;
#67201=CARTESIAN_POINT('Ctrl Pts',(-19.2407432792532,25.2199409129625,122.21774992714)) ;
#67202=CARTESIAN_POINT('Ctrl Pts',(-19.459301128586,25.4098642283046,121.905097168243)) ;
#67203=CARTESIAN_POINT('Ctrl Pts',(-19.4492836234959,25.2298751479417,122.206441411335)) ;
#67204=CARTESIAN_POINT('Ctrl Pts',(-19.72078773703,25.4198879916314,121.936883279556)) ;
#67205=CARTESIAN_POINT('Ctrl Pts',(-19.6584731310004,25.2398989112685,122.231868582496)) ;
#67206=CARTESIAN_POINT('Ctrl Pts',(-19.9693851432808,25.429774333016,122.012355109386)) ;
#67207=CARTESIAN_POINT('Ctrl Pts',(-19.8573510090563,25.2497852526532,122.292244189265)) ;
#67208=CARTESIAN_POINT('Ctrl Pts',(-20.2037937296493,25.439763381783,122.130525368287)) ;
#67209=CARTESIAN_POINT('Ctrl Pts',(-20.0448786033805,25.2597743014202,122.38677867719)) ;
#67210=CARTESIAN_POINT('Ctrl Pts',(-20.4148854638875,25.4498046024804,122.288855457116)) ;
#67211=CARTESIAN_POINT('Ctrl Pts',(-20.213753113731,25.2698155221175,122.513441372726)) ;
#67212=CARTESIAN_POINT('Ctrl Pts',(-20.5918392755866,25.4596372426583,122.477141002139)) ;
#67213=CARTESIAN_POINT('Ctrl Pts',(-20.3553169822991,25.2796481622954,122.664067990868)) ;
#67214=CARTESIAN_POINT('Ctrl Pts',(-20.7363655379612,25.4696311719663,122.696425976588)) ;
#67215=CARTESIAN_POINT('Ctrl Pts',(-20.4709395700862,25.2896420916034,122.839494814172)) ;
#67216=CARTESIAN_POINT('Ctrl Pts',(-20.8404780632738,25.4796603796468,122.93854969465)) ;
#67217=CARTESIAN_POINT('Ctrl Pts',(-20.5542313158732,25.2996712992839,123.033193065027)) ;
#67218=CARTESIAN_POINT('Ctrl Pts',(-20.9004575630717,25.4895361913509,123.191064817286)) ;
#67219=CARTESIAN_POINT('Ctrl Pts',(-20.6022166706708,25.309547110988,123.235204193094)) ;
#67220=CARTESIAN_POINT('Ctrl Pts',(-20.9161564441938,25.4995354183223,123.453329386861)) ;
#67221=CARTESIAN_POINT('Ctrl Pts',(-20.6147777399727,25.3195463379594,123.445015642034)) ;
#67222=CARTESIAN_POINT('Ctrl Pts',(-20.8865881009697,25.509444899478,123.712094698215)) ;
#67223=CARTESIAN_POINT('Ctrl Pts',(-20.5911250962336,25.3294558191151,123.65202774278)) ;
#67224=CARTESIAN_POINT('Ctrl Pts',(-20.81145089258,25.5194981297789,123.965343699702)) ;
#67225=CARTESIAN_POINT('Ctrl Pts',(-20.5310172244404,25.339509049416,123.854627590473)) ;
#67226=CARTESIAN_POINT('Ctrl Pts',(-20.6957175422055,25.52936874633,124.197502953534)) ;
#67227=CARTESIAN_POINT('Ctrl Pts',(-20.438432564313,25.3493796659671,124.040355455078)) ;
#67228=CARTESIAN_POINT('Ctrl Pts',(-20.5395534186836,25.539390408062,124.409561109384)) ;
#67229=CARTESIAN_POINT('Ctrl Pts',(-20.3135029430388,25.3594013276991,124.210003211742)) ;
#67230=CARTESIAN_POINT('Ctrl Pts',(-20.3484908449209,25.5494132212431,124.590878299816)) ;
#67231=CARTESIAN_POINT('Ctrl Pts',(-20.1606542784881,25.3694241408802,124.355058414572)) ;
#67232=CARTESIAN_POINT('Ctrl Pts',(-20.1325195803171,25.5592803857031,124.734357216796)) ;
#67233=CARTESIAN_POINT('Ctrl Pts',(-19.987878794653,25.3792913053402,124.469843008238)) ;
#67234=CARTESIAN_POINT('Ctrl Pts',(-19.8920996177146,25.569273827923,124.840044812153)) ;
#67235=CARTESIAN_POINT('Ctrl Pts',(-19.7955437603287,25.3892847475601,124.554394994497)) ;
#67236=CARTESIAN_POINT('Ctrl Pts',(-19.6358915111173,25.5793055015233,124.902119378316)) ;
#67237=CARTESIAN_POINT('Ctrl Pts',(-19.5905777624909,25.3993164211604,124.604056661626)) ;
#67238=CARTESIAN_POINT('Ctrl Pts',(-19.377143513442,25.5891719366363,124.918889100785)) ;
#67239=CARTESIAN_POINT('Ctrl Pts',(-19.3835799123551,25.4091828562734,124.617474520486)) ;
#67240=CARTESIAN_POINT('Ctrl Pts',(-19.1162493958071,25.5991593871694,124.890557819024)) ;
#67241=CARTESIAN_POINT('Ctrl Pts',(-19.1748644832375,25.4191703068065,124.594811646345)) ;
#67242=CARTESIAN_POINT('Ctrl Pts',(-18.8652039002789,25.6091043169973,124.817783333034)) ;
#67243=CARTESIAN_POINT('Ctrl Pts',(-18.9740276649419,25.4291152366345,124.536594184406)) ;
#67244=CARTESIAN_POINT('Ctrl Pts',(-18.6283721225821,25.6191492120525,124.701260743701)) ;
#67245=CARTESIAN_POINT('Ctrl Pts',(-18.784561279619,25.4391601316896,124.443378036371)) ;
#67246=CARTESIAN_POINT('Ctrl Pts',(-18.419077049514,25.6290112737383,124.548382059341)) ;
#67247=CARTESIAN_POINT('Ctrl Pts',(-18.6171242178969,25.4490221933754,124.321077040016)) ;
#67248=CARTESIAN_POINT('Ctrl Pts',(-18.2367942709095,25.6390029965252,124.359421375143)) ;
#67249=CARTESIAN_POINT('Ctrl Pts',(-18.4712964601253,25.4590139161623,124.169910079133)) ;
#67250=CARTESIAN_POINT('Ctrl Pts',(-18.091029495205,25.6489352107651,124.142904444548)) ;
#67251=CARTESIAN_POINT('Ctrl Pts',(-18.3546829152542,25.4689461304023,123.996697908865)) ;
#67252=CARTESIAN_POINT('Ctrl Pts',(-17.9844458363519,25.6588745293309,123.904437503963)) ;
#67253=CARTESIAN_POINT('Ctrl Pts',(-18.2694140074215,25.478885448968,123.805925391818)) ;
#67254=CARTESIAN_POINT('Ctrl Pts',(-17.9204539831751,25.6689187041067,123.648365609469)) ;
#67255=CARTESIAN_POINT('Ctrl Pts',(-18.2182183772246,25.4889296237439,123.60106842999)) ;
#67256=CARTESIAN_POINT('Ctrl Pts',(-17.9020768058315,25.6787892581717,123.389630116784)) ;
#67257=CARTESIAN_POINT('Ctrl Pts',(-18.2035144291742,25.4988001778088,123.394080402049)) ;
#67258=CARTESIAN_POINT('Ctrl Pts',(-17.9284060681277,25.6887542405259,123.1290873224)) ;
#67259=CARTESIAN_POINT('Ctrl Pts',(-18.2245755901221,25.508765160163,123.185646014976)) ;
#67260=CARTESIAN_POINT('Ctrl Pts',(-18.000430199717,25.6987849434157,122.875529417126)) ;
#67261=CARTESIAN_POINT('Ctrl Pts',(-18.2821927290592,25.5187958630528,122.98279912396)) ;
#67262=CARTESIAN_POINT('Ctrl Pts',(-18.1134771988756,25.7086772834409,122.641401239108)) ;
#67263=CARTESIAN_POINT('Ctrl Pts',(-18.3726282522614,25.528688203078,122.795495711768)) ;
#67264=CARTESIAN_POINT('Ctrl Pts',(-18.2678679863379,25.7187305166009,122.427066576845)) ;
#67265=CARTESIAN_POINT('Ctrl Pts',(-18.4961390336313,25.538741436238,122.624026697012)) ;
#67266=CARTESIAN_POINT('Ctrl Pts',(-18.4538393268546,25.7286117610776,122.245777047898)) ;
#67267=CARTESIAN_POINT('Ctrl Pts',(-18.6449144658524,25.5486226807147,122.478993530744)) ;
#67268=CARTESIAN_POINT('Ctrl Pts',(-18.6715752593228,25.7386448819486,122.097176077592)) ;
#67269=CARTESIAN_POINT('Ctrl Pts',(-18.8191018953641,25.5586558015858,122.360110920692)) ;
#67270=CARTESIAN_POINT('Ctrl Pts',(-18.9081608033064,25.7485260922237,121.990030737852)) ;
#67271=CARTESIAN_POINT('Ctrl Pts',(-19.0083693555972,25.5685370118608,122.274392619025)) ;
#67272=CARTESIAN_POINT('Ctrl Pts',(-19.1642552672847,25.758588167993,121.924365385186)) ;
#67273=CARTESIAN_POINT('Ctrl Pts',(-19.2132442996693,25.5785990876302,122.2218581685)) ;
#67274=CARTESIAN_POINT('Ctrl Pts',(-19.4225607860531,25.7684452263748,121.904478285387)) ;
#67275=CARTESIAN_POINT('Ctrl Pts',(-19.4198885350739,25.5884561460119,122.205946244612)) ;
#67276=CARTESIAN_POINT('Ctrl Pts',(-19.6839642883553,25.7784397816638,121.929561151871)) ;
#67277=CARTESIAN_POINT('Ctrl Pts',(-19.6290115124918,25.5984507013009,122.226010297302)) ;
#67278=CARTESIAN_POINT('Ctrl Pts',(-19.9354025958823,25.7883656691993,121.999101330404)) ;
#67279=CARTESIAN_POINT('Ctrl Pts',(-19.8301627662093,25.6083765888364,122.281640286907)) ;
#67280=CARTESIAN_POINT('Ctrl Pts',(-20.1732821454297,25.7983906891946,122.112270545144)) ;
#67281=CARTESIAN_POINT('Ctrl Pts',(-20.020467298116,25.6184016088317,122.372173604384)) ;
#67282=CARTESIAN_POINT('Ctrl Pts',(-20.3852412939983,25.8082880662982,122.26301982624)) ;
#67283=CARTESIAN_POINT('Ctrl Pts',(-20.1900359672413,25.6282989859354,122.49277124775)) ;
#67284=CARTESIAN_POINT('Ctrl Pts',(-20.5699265939808,25.8182783033791,122.449617357553)) ;
#67285=CARTESIAN_POINT('Ctrl Pts',(-20.3377857573925,25.6382892230162,122.64204770688)) ;
#67286=CARTESIAN_POINT('Ctrl Pts',(-20.7196773404664,25.8283149161879,122.666729559919)) ;
#67287=CARTESIAN_POINT('Ctrl Pts',(-20.4575881296598,25.648325835825,122.815736096847)) ;
#67288=CARTESIAN_POINT('Ctrl Pts',(-20.8278012350198,25.8381647996059,122.901920140004)) ;
#67289=CARTESIAN_POINT('Ctrl Pts',(-20.5440893331541,25.658175719243,123.003887861845)) ;
#67290=CARTESIAN_POINT('Ctrl Pts',(-20.8949727103039,25.8481684165084,123.156051177432)) ;
#67291=CARTESIAN_POINT('Ctrl Pts',(-20.5978286197024,25.6681793361455,123.207191954639)) ;
#67292=CARTESIAN_POINT('Ctrl Pts',(-20.9168297433397,25.8581578282735,123.417692998704)) ;
#67293=CARTESIAN_POINT('Ctrl Pts',(-20.6153163642316,25.6781687479106,123.416505743654)) ;
#67294=CARTESIAN_POINT('Ctrl Pts',(-20.8926982525151,25.8681765896183,123.67984195633)) ;
#67295=CARTESIAN_POINT('Ctrl Pts',(-20.5960135622755,25.6881875092555,123.626222991465)) ;
#67296=CARTESIAN_POINT('Ctrl Pts',(-20.8017581311539,25.8813952649994,124.015153473732)) ;
#67297=CARTESIAN_POINT('Ctrl Pts',(-20.5232632286193,25.7014061846365,123.894483244612)) ;
#67298=CARTESIAN_POINT('Ctrl Pts',(-20.6243920028856,25.8947055722441,124.321133430442)) ;
#67299=CARTESIAN_POINT('Ctrl Pts',(-20.3813483028792,25.7147164918812,124.139291566757)) ;
#67300=CARTESIAN_POINT('Ctrl Pts',(-20.3779377392562,25.9079432384701,124.566705392269)) ;
#67301=CARTESIAN_POINT('Ctrl Pts',(-20.1842168620273,25.7279541581072,124.335714004042)) ;
#67302=CARTESIAN_POINT('Ctrl Pts',(-20.1646098417396,25.9178629338808,124.716521317829)) ;
#67303=CARTESIAN_POINT('Ctrl Pts',(-20.0135493900519,25.7378738535179,124.455576016923)) ;
#67304=CARTESIAN_POINT('Ctrl Pts',(-19.9252257840937,25.9279158008794,124.828226044214)) ;
#67305=CARTESIAN_POINT('Ctrl Pts',(-19.8220451597961,25.7479267205165,124.544939701704)) ;
#67306=CARTESIAN_POINT('Ctrl Pts',(-19.6751350635831,25.9377712092086,124.895616007158)) ;
#67307=CARTESIAN_POINT('Ctrl Pts',(-19.6219710432747,25.7577821288458,124.598853833472)) ;
#67308=CARTESIAN_POINT('Ctrl Pts',(-19.4124225556355,25.9478098408852,124.919414322609)) ;
#67309=CARTESIAN_POINT('Ctrl Pts',(-19.4118058300607,25.7678207605223,124.617896055851)) ;
#67310=CARTESIAN_POINT('Ctrl Pts',(-19.0641152659986,25.9611120231522,124.889602889987)) ;
#67311=CARTESIAN_POINT('Ctrl Pts',(-19.1331381422336,25.7811229427894,124.594040874612)) ;
#67312=CARTESIAN_POINT('Ctrl Pts',(-18.6502847526992,25.9776570362351,124.740819809691)) ;
#67313=CARTESIAN_POINT('Ctrl Pts',(-18.8021063710032,25.7976679558722,124.475037523198)) ;
#67314=CARTESIAN_POINT('Ctrl Pts',(-18.3098802866931,25.9943090523113,124.458074394266)) ;
#67315=CARTESIAN_POINT('Ctrl Pts',(-18.5297345562069,25.8143199719484,124.248799717003)) ;
#67316=CARTESIAN_POINT('Ctrl Pts',(-18.1090436808664,26.0075321432166,124.174455573223)) ;
#67317=CARTESIAN_POINT('Ctrl Pts',(-18.369098690815,25.8275430628537,124.021942719457)) ;
#67318=CARTESIAN_POINT('Ctrl Pts',(-17.9965176539852,26.0174931027759,123.938117510176)) ;
#67319=CARTESIAN_POINT('Ctrl Pts',(-18.2790691278245,25.837504022413,123.832864843426)) ;
#67320=CARTESIAN_POINT('Ctrl Pts',(-17.9266031351628,26.027517899527,123.684128674994)) ;
#67321=CARTESIAN_POINT('Ctrl Pts',(-18.223137350365,25.8475288191641,123.629678646653)) ;
#67322=CARTESIAN_POINT('Ctrl Pts',(-17.8934600554389,26.0407423469228,123.338151922398)) ;
#67323=CARTESIAN_POINT('Ctrl Pts',(-18.1966218500974,25.8607532665599,123.352885080339)) ;
#67324=CARTESIAN_POINT('Ctrl Pts',(-17.9661098980233,26.0573761316219,122.902122581917)) ;
#67325=CARTESIAN_POINT('Ctrl Pts',(-18.2547370849816,25.877387051259,123.004073841914)) ;
#67326=CARTESIAN_POINT('Ctrl Pts',(-18.2260016702492,26.0772787983468,122.441338078492)) ;
#67327=CARTESIAN_POINT('Ctrl Pts',(-18.4626485568475,25.897289717984,122.6354399701)) ;
#67328=CARTESIAN_POINT('Ctrl Pts',(-18.6269689740633,26.0971790261287,122.096464789941)) ;
#67329=CARTESIAN_POINT('Ctrl Pts',(-18.7834208261286,25.9171899457658,122.359539719814)) ;
#67330=CARTESIAN_POINT('Ctrl Pts',(-19.1218834344603,26.1170965136602,121.908606135804)) ;
#67331=CARTESIAN_POINT('Ctrl Pts',(-19.1793520415274,25.9371074332973,122.209249695182)) ;
#67332=CARTESIAN_POINT('Ctrl Pts',(-19.6515421009118,26.1370260394771,121.900579250022)) ;
#67333=CARTESIAN_POINT('Ctrl Pts',(-19.6030795010678,25.9570369591142,122.202825735213)) ;
#67334=CARTESIAN_POINT('Ctrl Pts',(-20.1529386123422,26.1569883073634,122.074158377623)) ;
#67335=CARTESIAN_POINT('Ctrl Pts',(-20.0041977734396,25.9769992270005,122.341686821222)) ;
#67336=CARTESIAN_POINT('Ctrl Pts',(-20.5634651727886,26.1768785023156,122.407118082729)) ;
#67337=CARTESIAN_POINT('Ctrl Pts',(-20.3326212396169,25.9968894219527,122.608053440236)) ;
#67338=CARTESIAN_POINT('Ctrl Pts',(-20.8369695350651,26.1967687470618,122.859653772299)) ;
#67339=CARTESIAN_POINT('Ctrl Pts',(-20.5514266616668,26.016779666699,122.970082039285)) ;
#67340=CARTESIAN_POINT('Ctrl Pts',(-20.9394612388346,26.2168431196243,123.383189522101)) ;
#67341=CARTESIAN_POINT('Ctrl Pts',(-20.6334217424483,26.0368540392614,123.388909499368)) ;
#67342=CARTESIAN_POINT('Ctrl Pts',(-20.858478621002,26.2366284969846,123.902848054689)) ;
#67343=CARTESIAN_POINT('Ctrl Pts',(-20.5686369629156,26.0566394166217,123.80463880822)) ;
#67344=CARTESIAN_POINT('Ctrl Pts',(-20.604272042101,26.2565903710517,124.368482650199)) ;
#67345=CARTESIAN_POINT('Ctrl Pts',(-20.3652721856668,26.0766012906889,124.177147290224)) ;
#67346=CARTESIAN_POINT('Ctrl Pts',(-20.2051802401964,26.2765703465422,124.718824795122)) ;
#67347=CARTESIAN_POINT('Ctrl Pts',(-20.0459994054117,26.0965812661794,124.457422009913)) ;
#67348=CARTESIAN_POINT('Ctrl Pts',(-19.7149987089246,26.2963827764202,124.911292999828)) ;
#67349=CARTESIAN_POINT('Ctrl Pts',(-19.6538521960381,26.1163936960573,124.611397916623)) ;
#67350=CARTESIAN_POINT('Ctrl Pts',(-19.1842547999823,26.3163628845105,124.925735636618)) ;
#67351=CARTESIAN_POINT('Ctrl Pts',(-19.2292567523326,26.1363738041476,124.622952026166)) ;
#67352=CARTESIAN_POINT('Ctrl Pts',(-18.6824717518944,26.3362572681077,124.758627144309)) ;
#67353=CARTESIAN_POINT('Ctrl Pts',(-18.8278291137582,26.1562681877448,124.489264722442)) ;
#67354=CARTESIAN_POINT('Ctrl Pts',(-18.2670439988586,26.3561841960849,124.430303289928)) ;
#67355=CARTESIAN_POINT('Ctrl Pts',(-18.4954865238769,26.1761951157221,124.226604620263)) ;
#67356=CARTESIAN_POINT('Ctrl Pts',(-17.9883141683562,26.3760790533862,123.980817223551)) ;
#67357=CARTESIAN_POINT('Ctrl Pts',(-18.2725029335029,26.1960899730233,123.867014230406)) ;
#67358=CARTESIAN_POINT('Ctrl Pts',(-17.8794749235701,26.3961182469898,123.459500138785)) ;
#67359=CARTESIAN_POINT('Ctrl Pts',(-18.1854325963948,26.2161291666269,123.449960783738)) ;
#67360=CARTESIAN_POINT('Ctrl Pts',(-17.9544430376458,26.4159582149006,122.937489228161)) ;
#67361=CARTESIAN_POINT('Ctrl Pts',(-18.2454084587968,26.2359691345377,123.032350471907)) ;
#67362=CARTESIAN_POINT('Ctrl Pts',(-18.2027276437108,26.4358730318646,122.470081707864)) ;
#67363=CARTESIAN_POINT('Ctrl Pts',(-18.4440381844851,26.2558839515018,122.658424577818)) ;
#67364=CARTESIAN_POINT('Ctrl Pts',(-18.596400995126,26.4558152772609,122.115240379138)) ;
#67365=CARTESIAN_POINT('Ctrl Pts',(-18.7589785547177,26.275826196898,122.374552517246)) ;
#67366=CARTESIAN_POINT('Ctrl Pts',(-19.0856111707764,26.4756873253754,121.915849802114)) ;
#67367=CARTESIAN_POINT('Ctrl Pts',(-19.1503485944393,26.2956982450125,122.215041802279)) ;
#67368=CARTESIAN_POINT('Ctrl Pts',(-19.6169161682822,26.4956983903295,121.895626311636)) ;
#67369=CARTESIAN_POINT('Ctrl Pts',(-19.57539261041,26.3157093099666,122.198865364486)) ;
#67370=CARTESIAN_POINT('Ctrl Pts',(-20.118823655691,26.5155099146331,122.055636433992)) ;
#67371=CARTESIAN_POINT('Ctrl Pts',(-19.9769191395575,26.3355208342703,122.326876501952)) ;
#67372=CARTESIAN_POINT('Ctrl Pts',(-20.5414187886625,26.5356051265965,122.381904092641)) ;
#67373=CARTESIAN_POINT('Ctrl Pts',(-20.3149929725486,26.3556160462336,122.587892382152)) ;
#67374=CARTESIAN_POINT('Ctrl Pts',(-20.8229786362358,26.5553858505163,122.826139617815)) ;
#67375=CARTESIAN_POINT('Ctrl Pts',(-20.5402392941985,26.3753967701534,122.943283661868)) ;
#67376=CARTESIAN_POINT('Ctrl Pts',(-20.9383530388371,26.5753769261591,123.344589665565)) ;
#67377=CARTESIAN_POINT('Ctrl Pts',(-20.6325355740105,26.3953878457962,123.358044462546)) ;
#67378=CARTESIAN_POINT('Ctrl Pts',(-20.86985320622,26.5952588652021,123.868710610695)) ;
#67379=CARTESIAN_POINT('Ctrl Pts',(-20.577732355409,26.4152697848392,123.777341477282)) ;
#67380=CARTESIAN_POINT('Ctrl Pts',(-20.6263804833536,26.6152114697054,124.339726432393)) ;
#67381=CARTESIAN_POINT('Ctrl Pts',(-20.3829508664611,26.4352223893425,124.154152702177)) ;
#67382=CARTESIAN_POINT('Ctrl Pts',(-20.2377323609478,26.635110338436,124.698507478413)) ;
#67383=CARTESIAN_POINT('Ctrl Pts',(-20.0720296498314,26.4551212580731,124.441175303376)) ;
#67384=CARTESIAN_POINT('Ctrl Pts',(-19.750506384729,26.6550037382456,124.903616092832)) ;
#67385=CARTESIAN_POINT('Ctrl Pts',(-19.6822465171285,26.4750146578827,124.605258460819)) ;
#67386=CARTESIAN_POINT('Ctrl Pts',(-19.2219548120851,26.6749128690856,124.930993209538)) ;
#67387=CARTESIAN_POINT('Ctrl Pts',(-19.2594063325904,26.4949237887228,124.627157492375)) ;
#67388=CARTESIAN_POINT('Ctrl Pts',(-18.7130356342311,26.6949449688492,124.774763267432)) ;
#67389=CARTESIAN_POINT('Ctrl Pts',(-18.8522664567341,26.5149558884863,124.502164665301)) ;
#67390=CARTESIAN_POINT('Ctrl Pts',(-18.3620528555376,26.7114770420187,124.510268121194)) ;
#67391=CARTESIAN_POINT('Ctrl Pts',(-18.5715001976287,26.5314879616558,124.290581423656)) ;
#67392=CARTESIAN_POINT('Ctrl Pts',(-18.1460617747501,26.7248123826246,124.234367496516)) ;
#67393=CARTESIAN_POINT('Ctrl Pts',(-18.3986933386626,26.5448233022617,124.069844646193)) ;
#67394=CARTESIAN_POINT('Ctrl Pts',(-18.0239800547126,26.7346549411643,124.006303612785)) ;
#67395=CARTESIAN_POINT('Ctrl Pts',(-18.3010327997462,26.5546658608015,123.887397815469)) ;
#67396=CARTESIAN_POINT('Ctrl Pts',(-17.9413973813911,26.7447068480142,123.755428033597)) ;
#67397=CARTESIAN_POINT('Ctrl Pts',(-18.2349681691499,26.5647177676514,123.686685201408)) ;
#67398=CARTESIAN_POINT('Ctrl Pts',(-17.891686149238,26.7579553624051,123.410787353362)) ;
#67399=CARTESIAN_POINT('Ctrl Pts',(-18.1952008751101,26.5779662820423,123.411026738166)) ;
#67400=CARTESIAN_POINT('Ctrl Pts',(-17.9431815127596,26.7745545373529,122.972680824458)) ;
#67401=CARTESIAN_POINT('Ctrl Pts',(-18.2364062949001,26.59456545699,123.060472645166)) ;
#67402=CARTESIAN_POINT('Ctrl Pts',(-18.1408483242503,26.7911433231479,122.578566000262)) ;
#67403=CARTESIAN_POINT('Ctrl Pts',(-18.3945264353871,26.6111542427851,122.745229800877)) ;
#67404=CARTESIAN_POINT('Ctrl Pts',(-18.3723926843041,26.8044191394899,122.317598644227)) ;
#67405=CARTESIAN_POINT('Ctrl Pts',(-18.5797786876683,26.624430059127,122.536429224287)) ;
#67406=CARTESIAN_POINT('Ctrl Pts',(-18.5775216542846,26.8143929902837,122.15442033865)) ;
#67407=CARTESIAN_POINT('Ctrl Pts',(-18.7438803146688,26.6344039099208,122.405894095803)) ;
#67408=CARTESIAN_POINT('Ctrl Pts',(-18.8092589677791,26.8244220223761,122.028905565457)) ;
#67409=CARTESIAN_POINT('Ctrl Pts',(-18.9292719326846,26.6444329420132,122.305482723991)) ;
#67410=CARTESIAN_POINT('Ctrl Pts',(-19.0557421895212,26.834312147878,121.946421302957)) ;
#67411=CARTESIAN_POINT('Ctrl Pts',(-19.1264590870646,26.6543230675151,122.239497816618)) ;
#67412=CARTESIAN_POINT('Ctrl Pts',(-19.3153650354541,26.8443046261495,121.907247691411)) ;
#67413=CARTESIAN_POINT('Ctrl Pts',(-19.3341577092669,26.6643155457866,122.208161046948)) ;
#67414=CARTESIAN_POINT('Ctrl Pts',(-19.5768371046668,26.8542558412469,121.913582155201)) ;
#67415=CARTESIAN_POINT('Ctrl Pts',(-19.5433352791444,26.674266760884,122.213230894477)) ;
#67416=CARTESIAN_POINT('Ctrl Pts',(-19.8356332457282,26.8643043430019,121.965922317603)) ;
#67417=CARTESIAN_POINT('Ctrl Pts',(-19.7503716736977,26.6843152626391,122.255105201927)) ;
#67418=CARTESIAN_POINT('Ctrl Pts',(-20.0765024472187,26.8741456926187,122.060153190044)) ;
#67419=CARTESIAN_POINT('Ctrl Pts',(-19.9430662458474,26.6941566122558,122.330492010687)) ;
#67420=CARTESIAN_POINT('Ctrl Pts',(-20.3008378724975,26.8841319836389,122.196241980051)) ;
#67421=CARTESIAN_POINT('Ctrl Pts',(-20.1225333562957,26.7041429032761,122.439364943551)) ;
#67422=CARTESIAN_POINT('Ctrl Pts',(-20.4973053062689,26.8940685953675,122.368314358404)) ;
#67423=CARTESIAN_POINT('Ctrl Pts',(-20.2797057735737,26.7140795150047,122.577024505294)) ;
#67424=CARTESIAN_POINT('Ctrl Pts',(-20.662628518743,26.9041184707351,122.574234184223)) ;
#67425=CARTESIAN_POINT('Ctrl Pts',(-20.4119625510863,26.7241293903722,122.741761744443)) ;
#67426=CARTESIAN_POINT('Ctrl Pts',(-20.7873567686691,26.9139689292705,122.801084418396)) ;
#67427=CARTESIAN_POINT('Ctrl Pts',(-20.5117431267573,26.7339798489077,122.92324293676)) ;
#67428=CARTESIAN_POINT('Ctrl Pts',(-20.8724634669083,26.9239408662233,123.048897162386)) ;
#67429=CARTESIAN_POINT('Ctrl Pts',(-20.5798263274072,26.7439517858604,123.121493774499)) ;
#67430=CARTESIAN_POINT('Ctrl Pts',(-20.9133152577875,26.9339363231554,123.308411671272)) ;
#67431=CARTESIAN_POINT('Ctrl Pts',(-20.6125055330845,26.7539472427925,123.329105668054)) ;
#67432=CARTESIAN_POINT('Ctrl Pts',(-20.9081708679061,26.9439691302085,123.571995622508)) ;
#67433=CARTESIAN_POINT('Ctrl Pts',(-20.6083877656907,26.7639800498456,123.539972753807)) ;
#67434=CARTESIAN_POINT('Ctrl Pts',(-20.8585534427238,26.9538290167985,123.826321841959)) ;
#67435=CARTESIAN_POINT('Ctrl Pts',(-20.5686916578816,26.7738399364356,123.743433118056)) ;
#67436=CARTESIAN_POINT('Ctrl Pts',(-20.7647835915375,26.9638180973637,124.071480590036)) ;
#67437=CARTESIAN_POINT('Ctrl Pts',(-20.4936737272855,26.7838290170008,123.939559239062)) ;
#67438=CARTESIAN_POINT('Ctrl Pts',(-20.6306305349959,26.9737495765729,124.29536007837)) ;
#67439=CARTESIAN_POINT('Ctrl Pts',(-20.3863494522034,26.79376049621,124.118661555198)) ;
#67440=CARTESIAN_POINT('Ctrl Pts',(-20.4590264458182,26.9837354360188,124.493916247248)) ;
#67441=CARTESIAN_POINT('Ctrl Pts',(-20.2490645750113,26.8037463556559,124.277504981672)) ;
#67442=CARTESIAN_POINT('Ctrl Pts',(-20.254221659418,26.993773586666,124.66014484481)) ;
#67443=CARTESIAN_POINT('Ctrl Pts',(-20.0852193413478,26.8137845063031,124.410486127387)) ;
#67444=CARTESIAN_POINT('Ctrl Pts',(-20.0282504284219,27.0036216771704,124.786342691733)) ;
#67445=CARTESIAN_POINT('Ctrl Pts',(-19.9044415680484,26.8236325968075,124.511442329042)) ;
#67446=CARTESIAN_POINT('Ctrl Pts',(-19.7786397745395,27.0136825856884,124.873419336829)) ;
#67447=CARTESIAN_POINT('Ctrl Pts',(-19.7047522927702,26.8336935053255,124.581101595474)) ;
#67448=CARTESIAN_POINT('Ctrl Pts',(-19.5219286374244,27.0235774328464,124.914963808306)) ;
#67449=CARTESIAN_POINT('Ctrl Pts',(-19.4993832936596,26.8435883524835,124.614334963387)) ;
#67450=CARTESIAN_POINT('Ctrl Pts',(-19.2607200330095,27.0335191048914,124.911983091372)) ;
#67451=CARTESIAN_POINT('Ctrl Pts',(-19.2904166467755,26.8535300245285,124.611948249213)) ;
#67452=CARTESIAN_POINT('Ctrl Pts',(-19.002340474553,27.0435216320169,124.863486618766)) ;
#67453=CARTESIAN_POINT('Ctrl Pts',(-19.0837134587159,26.863532551654,124.573148990088)) ;
#67454=CARTESIAN_POINT('Ctrl Pts',(-18.755708647713,27.0535564232043,124.770193481186)) ;
#67455=CARTESIAN_POINT('Ctrl Pts',(-18.8864087522121,26.8735673428414,124.498512445791)) ;
#67456=CARTESIAN_POINT('Ctrl Pts',(-18.53306086531,27.0634013030634,124.63840012197)) ;
#67457=CARTESIAN_POINT('Ctrl Pts',(-18.7082920013057,26.8834122227005,124.393076157916)) ;
#67458=CARTESIAN_POINT('Ctrl Pts',(-18.3335903392706,27.0733871836819,124.467951336687)) ;
#67459=CARTESIAN_POINT('Ctrl Pts',(-18.5487170321478,26.893398103319,124.256715629541)) ;
#67460=CARTESIAN_POINT('Ctrl Pts',(-18.1673965821684,27.0833219067751,124.266543402248)) ;
#67461=CARTESIAN_POINT('Ctrl Pts',(-18.4157637799795,26.9033328264122,124.095588174979)) ;
#67462=CARTESIAN_POINT('Ctrl Pts',(-18.0373591121067,27.0933797470863,124.03648134582)) ;
#67463=CARTESIAN_POINT('Ctrl Pts',(-18.3117355760186,26.9133906667234,123.911537419721)) ;
#67464=CARTESIAN_POINT('Ctrl Pts',(-17.9509061764655,27.1032002344828,123.793285094069)) ;
#67465=CARTESIAN_POINT('Ctrl Pts',(-18.242575359153,26.9232111541199,123.716980330585)) ;
#67466=CARTESIAN_POINT('Ctrl Pts',(-17.9065238901742,27.1132606358279,123.532692664086)) ;
#67467=CARTESIAN_POINT('Ctrl Pts',(-18.2070714726686,26.9332715554651,123.508505957209)) ;
#67468=CARTESIAN_POINT('Ctrl Pts',(-17.9083966530251,27.1231916013808,123.271694164607)) ;
#67469=CARTESIAN_POINT('Ctrl Pts',(-18.2085717099821,26.943202521018,123.299707472759)) ;
#67470=CARTESIAN_POINT('Ctrl Pts',(-17.9550143490479,27.1331304637173,123.014732779571)) ;
#67471=CARTESIAN_POINT('Ctrl Pts',(-18.2458677394245,26.9531413833544,123.094139009809)) ;
#67472=CARTESIAN_POINT('Ctrl Pts',(-18.0458227293772,27.1431161946435,122.768499870868)) ;
#67473=CARTESIAN_POINT('Ctrl Pts',(-18.3185162096812,26.9631271142806,122.897153472277)) ;
#67474=CARTESIAN_POINT('Ctrl Pts',(-18.1787338062467,27.1531405800709,122.54108010085)) ;
#67475=CARTESIAN_POINT('Ctrl Pts',(-18.4248467768607,26.9731514997081,122.715218646662)) ;
#67476=CARTESIAN_POINT('Ctrl Pts',(-18.3467863406668,27.1630438644242,122.342321573022)) ;
#67477=CARTESIAN_POINT('Ctrl Pts',(-18.5592899783311,26.9830547840613,122.556213402555)) ;
#67478=CARTESIAN_POINT('Ctrl Pts',(-18.5499675318017,27.1731038690022,122.173235543931)) ;
#67479=CARTESIAN_POINT('Ctrl Pts',(-18.7218362738242,26.9931147886393,122.420945971278)) ;
#67480=CARTESIAN_POINT('Ctrl Pts',(-18.7744378365037,27.1829471380713,122.044638016558)) ;
#67481=CARTESIAN_POINT('Ctrl Pts',(-18.9014128616889,27.0029580577084,122.318069943643)) ;
#67482=CARTESIAN_POINT('Ctrl Pts',(-19.0212070083882,27.192937703679,121.955103241881)) ;
#67483=CARTESIAN_POINT('Ctrl Pts',(-19.0988286849585,27.0129486233161,122.246443874494)) ;
#67484=CARTESIAN_POINT('Ctrl Pts',(-19.2782077784814,27.2028658354578,121.910092465526)) ;
#67485=CARTESIAN_POINT('Ctrl Pts',(-19.3044292293712,27.022876755095,122.210437108631)) ;
#67486=CARTESIAN_POINT('Ctrl Pts',(-19.5406906769413,27.2128537225387,121.909933250644)) ;
#67487=CARTESIAN_POINT('Ctrl Pts',(-19.5144154029953,27.0328646421759,122.210311478194)) ;
#67488=CARTESIAN_POINT('Ctrl Pts',(-19.8003580009036,27.2228896721074,121.956008127035)) ;
#67489=CARTESIAN_POINT('Ctrl Pts',(-19.7221490136593,27.0429005917445,122.247173180015)) ;
#67490=CARTESIAN_POINT('Ctrl Pts',(-20.0437890490973,27.2327445584862,122.044444124203)) ;
#67491=CARTESIAN_POINT('Ctrl Pts',(-19.9168925651677,27.0527554781234,122.317923364294)) ;
#67492=CARTESIAN_POINT('Ctrl Pts',(-20.2715790260407,27.2427439728341,122.175359156114)) ;
#67493=CARTESIAN_POINT('Ctrl Pts',(-20.0991236143385,27.0627548924712,122.422656796826)) ;
#67494=CARTESIAN_POINT('Ctrl Pts',(-20.47132188163,27.2526391380246,122.341923187153)) ;
#67495=CARTESIAN_POINT('Ctrl Pts',(-20.2589164031302,27.0726500576617,122.555908896478)) ;
#67496=CARTESIAN_POINT('Ctrl Pts',(-20.6418377253297,27.2626994567166,122.543912452748)) ;
#67497=CARTESIAN_POINT('Ctrl Pts',(-20.3953279507184,27.0827103763537,122.717501514616)) ;
#67498=CARTESIAN_POINT('Ctrl Pts',(-20.7720769168341,27.2725495884926,122.767639569015)) ;
#67499=CARTESIAN_POINT('Ctrl Pts',(-20.4995174924838,27.0925605081298,122.89648329143)) ;
#67500=CARTESIAN_POINT('Ctrl Pts',(-20.8637005068752,27.2825801589429,123.014783157539)) ;
#67501=CARTESIAN_POINT('Ctrl Pts',(-20.5728149832003,27.10259107858,123.094198725936)) ;
#67502=CARTESIAN_POINT('Ctrl Pts',(-20.9103706252309,27.2925943096157,123.273787983254)) ;
#67503=CARTESIAN_POINT('Ctrl Pts',(-20.6101494956889,27.1126052292528,123.301402858841)) ;
#67504=CARTESIAN_POINT('Ctrl Pts',(-20.911768495837,27.3024872431611,123.533764947733)) ;
#67505=CARTESIAN_POINT('Ctrl Pts',(-20.6112662665047,27.1224981627982,123.509383800559)) ;
#67506=CARTESIAN_POINT('Ctrl Pts',(-20.8678776029836,27.3124767571514,123.792558185261)) ;
#67507=CARTESIAN_POINT('Ctrl Pts',(-20.5761521325388,27.1324876767885,123.716417986733)) ;
#67508=CARTESIAN_POINT('Ctrl Pts',(-20.7801754400193,27.3224305278038,124.03903194835)) ;
#67509=CARTESIAN_POINT('Ctrl Pts',(-20.505989170069,27.1424414474409,123.913596190151)) ;
#67510=CARTESIAN_POINT('Ctrl Pts',(-20.6496157399914,27.3324782964644,124.26850963764)) ;
#67511=CARTESIAN_POINT('Ctrl Pts',(-20.4015400481253,27.1524892161015,124.097177744708)) ;
#67512=CARTESIAN_POINT('Ctrl Pts',(-20.4848531000536,27.3423200229042,124.467895083723)) ;
#67513=CARTESIAN_POINT('Ctrl Pts',(-20.2697294497831,27.1623309425413,124.256684466489)) ;
#67514=CARTESIAN_POINT('Ctrl Pts',(-20.2855162962699,27.3523055397269,124.638488743857)) ;
#67515=CARTESIAN_POINT('Ctrl Pts',(-20.1102593118314,27.172316459364,124.393158279408)) ;
#67516=CARTESIAN_POINT('Ctrl Pts',(-20.0606131128351,27.3622448714225,124.771385186807)) ;
#67517=CARTESIAN_POINT('Ctrl Pts',(-19.9303364915707,27.1822557910596,124.499474112979)) ;
#67518=CARTESIAN_POINT('Ctrl Pts',(-19.8136159800649,27.37228464112,124.864066326302)) ;
#67519=CARTESIAN_POINT('Ctrl Pts',(-19.7327382216027,27.1922955607571,124.57361785765)) ;
#67520=CARTESIAN_POINT('Ctrl Pts',(-19.5581817302825,27.3821728023688,124.911855032732)) ;
#67521=CARTESIAN_POINT('Ctrl Pts',(-19.5283913156951,27.2021837220059,124.61184744574)) ;
#67522=CARTESIAN_POINT('Ctrl Pts',(-19.2956955404914,27.3921623568712,124.915085978907)) ;
#67523=CARTESIAN_POINT('Ctrl Pts',(-19.318402520903,27.2121732765083,124.614431045079)) ;
#67524=CARTESIAN_POINT('Ctrl Pts',(-19.0374725439821,27.4021207713948,124.872626590807)) ;
#67525=CARTESIAN_POINT('Ctrl Pts',(-19.1118246609645,27.222131691032,124.580462405806)) ;
#67526=CARTESIAN_POINT('Ctrl Pts',(-18.7917647458714,27.4120206842242,124.787079499337)) ;
#67527=CARTESIAN_POINT('Ctrl Pts',(-18.9152594335383,27.2320316038613,124.51202396635)) ;
#67528=CARTESIAN_POINT('Ctrl Pts',(-18.5613480077617,27.4220673838741,124.658240132733)) ;
#67529=CARTESIAN_POINT('Ctrl Pts',(-18.7309264191264,27.2420783035112,124.40895145111)) ;
#67530=CARTESIAN_POINT('Ctrl Pts',(-18.3596364546277,27.4319672441797,124.493876043428)) ;
#67531=CARTESIAN_POINT('Ctrl Pts',(-18.5695583841052,27.2519781638168,124.277459828361)) ;
#67532=CARTESIAN_POINT('Ctrl Pts',(-18.186909253097,27.4420186483852,124.294086730336)) ;
#67533=CARTESIAN_POINT('Ctrl Pts',(-18.4313772630263,27.2620295680223,124.117627563925)) ;
#67534=CARTESIAN_POINT('Ctrl Pts',(-18.0536713291326,27.4518996853063,124.071168267617)) ;
#67535=CARTESIAN_POINT('Ctrl Pts',(-18.3247881999234,27.2719106049434,123.939292985394)) ;
#67536=CARTESIAN_POINT('Ctrl Pts',(-17.9597465513536,27.4618995174838,123.825788262627)) ;
#67537=CARTESIAN_POINT('Ctrl Pts',(-18.24964927092,27.2819104371209,123.742988761484)) ;
#67538=CARTESIAN_POINT('Ctrl Pts',(-17.9100347106082,27.4718175204687,123.56989145949)) ;
#67539=CARTESIAN_POINT('Ctrl Pts',(-18.2098807623671,27.2918284401058,123.538271752722)) ;
#67540=CARTESIAN_POINT('Ctrl Pts',(-17.9055372820663,27.4818688263432,123.305836914717)) ;
#67541=CARTESIAN_POINT('Ctrl Pts',(-18.2062837024167,27.3018797459804,123.327027911082)) ;
#67542=CARTESIAN_POINT('Ctrl Pts',(-17.9459117765369,27.4917386497348,123.049572996332)) ;
#67543=CARTESIAN_POINT('Ctrl Pts',(-18.2385839520129,27.3117495693719,123.122017805772)) ;
#67544=CARTESIAN_POINT('Ctrl Pts',(-18.0318915985893,27.5018128157851,122.799249602971)) ;
#67545=CARTESIAN_POINT('Ctrl Pts',(-18.3073686920026,27.3218237354222,122.921759028966)) ;
#67546=CARTESIAN_POINT('Ctrl Pts',(-18.1565773494833,27.5116328999267,122.573239483822)) ;
#67547=CARTESIAN_POINT('Ctrl Pts',(-18.4071173341134,27.3316438195639,122.740952378761)) ;
#67548=CARTESIAN_POINT('Ctrl Pts',(-18.3226042808018,27.5217116266626,122.366962086733)) ;
#67549=CARTESIAN_POINT('Ctrl Pts',(-18.5399396427468,27.3417225462997,122.575930590935)) ;
#67550=CARTESIAN_POINT('Ctrl Pts',(-18.5174703780383,27.5315632073121,122.196424414338)) ;
#67551=CARTESIAN_POINT('Ctrl Pts',(-18.6958321561076,27.3515741269492,122.439501639971)) ;
#67552=CARTESIAN_POINT('Ctrl Pts',(-18.7437532834736,27.5416363356105,122.05915550415)) ;
#67553=CARTESIAN_POINT('Ctrl Pts',(-18.8768590906674,27.3616472552476,122.329686841586)) ;
#67554=CARTESIAN_POINT('Ctrl Pts',(-18.9848658829686,27.5514788135019,121.965469396346)) ;
#67555=CARTESIAN_POINT('Ctrl Pts',(-19.0697483336544,27.3714897331391,122.25473893346)) ;
#67556=CARTESIAN_POINT('Ctrl Pts',(-19.2419340497948,27.5614594201,121.913511275121)) ;
#67557=CARTESIAN_POINT('Ctrl Pts',(-19.2754027022882,27.3814703397371,122.213172868281)) ;
#67558=CARTESIAN_POINT('Ctrl Pts',(-19.505118136635,27.5714771291188,121.907449255122)) ;
#67559=CARTESIAN_POINT('Ctrl Pts',(-19.4859499875362,27.3914880487559,122.208323766678)) ;
#67560=CARTESIAN_POINT('Ctrl Pts',(-19.7620374996728,27.5813633081562,121.946159440311)) ;
#67561=CARTESIAN_POINT('Ctrl Pts',(-19.6914845708838,27.4013742277934,122.239292171034)) ;
#67562=CARTESIAN_POINT('Ctrl Pts',(-20.0125674013974,27.5914209207286,122.030295059284)) ;
#67563=CARTESIAN_POINT('Ctrl Pts',(-19.8919086080025,27.4114318403657,122.306601108605)) ;
#67564=CARTESIAN_POINT('Ctrl Pts',(-20.2405477178494,27.6012973141007,122.154372035112)) ;
#67565=CARTESIAN_POINT('Ctrl Pts',(-20.0742918644194,27.4213082337378,122.405862575282)) ;
#67566=CARTESIAN_POINT('Ctrl Pts',(-20.4463485472987,27.6112923422511,122.317564461287)) ;
#67567=CARTESIAN_POINT('Ctrl Pts',(-20.2389322836839,27.4313032618883,122.53641659574)) ;
#67568=CARTESIAN_POINT('Ctrl Pts',(-20.6208115759906,27.6213130890971,122.51483046535)) ;
#67569=CARTESIAN_POINT('Ctrl Pts',(-20.3785024861279,27.4413240087343,122.694229642115)) ;
#67570=CARTESIAN_POINT('Ctrl Pts',(-20.7569960330264,27.6312151577635,122.736562250952)) ;
#67571=CARTESIAN_POINT('Ctrl Pts',(-20.4874494348297,27.4512260774006,122.871614548114)) ;
#67572=CARTESIAN_POINT('Ctrl Pts',(-20.8538296011518,27.6412058975832,122.980600241119)) ;
#67573=CARTESIAN_POINT('Ctrl Pts',(-20.5649160765477,27.4612168172203,123.066844821881)) ;
#67574=CARTESIAN_POINT('Ctrl Pts',(-20.9064812123952,27.6511690937935,123.237061229662)) ;
#67575=CARTESIAN_POINT('Ctrl Pts',(-20.6070370952218,27.4711800134306,123.272013299712)) ;
#67576=CARTESIAN_POINT('Ctrl Pts',(-20.9144047817725,27.6610732780936,123.497236530681)) ;
#67577=CARTESIAN_POINT('Ctrl Pts',(-20.6133758900281,27.4810841977308,123.480152789572)) ;
#67578=CARTESIAN_POINT('Ctrl Pts',(-20.8762301626549,27.6711337384845,123.758811110914)) ;
#67579=CARTESIAN_POINT('Ctrl Pts',(-20.5828360598664,27.4911446581216,123.689412720083)) ;
#67580=CARTESIAN_POINT('Ctrl Pts',(-20.7953249519176,27.6809742843553,124.004465402187)) ;
#67581=CARTESIAN_POINT('Ctrl Pts',(-20.5181122497151,27.5009852039924,123.88593503245)) ;
#67582=CARTESIAN_POINT('Ctrl Pts',(-20.6705674371017,27.6910365050671,124.237576347375)) ;
#67583=CARTESIAN_POINT('Ctrl Pts',(-20.4183061644665,27.5110474247042,124.072424084696)) ;
#67584=CARTESIAN_POINT('Ctrl Pts',(-20.5096693378974,27.7009336480836,124.441939302609)) ;
#67585=CARTESIAN_POINT('Ctrl Pts',(-20.2895881841943,27.5209445677207,124.235913821433)) ;
#67586=CARTESIAN_POINT('Ctrl Pts',(-20.315658373556,27.7108648245008,124.61649018712)) ;
#67587=CARTESIAN_POINT('Ctrl Pts',(-20.1343799929666,27.5308757441379,124.375554311888)) ;
#67588=CARTESIAN_POINT('Ctrl Pts',(-20.091657303987,27.7209070382794,124.756002912722)) ;
#67589=CARTESIAN_POINT('Ctrl Pts',(-19.9551790760134,27.5409179579165,124.487164709501)) ;
#67590=CARTESIAN_POINT('Ctrl Pts',(-19.8506842942627,27.7307935784821,124.85316185408)) ;
#67591=CARTESIAN_POINT('Ctrl Pts',(-19.7624015506141,27.5508044981193,124.564891723896)) ;
#67592=CARTESIAN_POINT('Ctrl Pts',(-19.5938710456304,27.7407871730876,124.907993194414)) ;
#67593=CARTESIAN_POINT('Ctrl Pts',(-19.5569511707671,27.5607980927247,124.608757063164)) ;
#67594=CARTESIAN_POINT('Ctrl Pts',(-19.3327071093546,27.7507310482451,124.917315275339)) ;
#67595=CARTESIAN_POINT('Ctrl Pts',(-19.3480205279212,27.5707419678822,124.616215008341)) ;
#67596=CARTESIAN_POINT('Ctrl Pts',(-19.0734423500519,27.7606915843599,124.881432829596)) ;
#67597=CARTESIAN_POINT('Ctrl Pts',(-19.1406090425669,27.5807025039971,124.587509484983)) ;
#67598=CARTESIAN_POINT('Ctrl Pts',(-18.823353749831,27.7706881876827,124.800925220385)) ;
#67599=CARTESIAN_POINT('Ctrl Pts',(-18.9405381483672,27.5906991073198,124.523103835156)) ;
#67600=CARTESIAN_POINT('Ctrl Pts',(-18.5903995182117,27.7807212706372,124.677453935382)) ;
#67601=CARTESIAN_POINT('Ctrl Pts',(-18.7541745110723,27.6007321902743,124.424327045669)) ;
#67602=CARTESIAN_POINT('Ctrl Pts',(-18.3859904696139,27.7905724393387,124.518604840361)) ;
#67603=CARTESIAN_POINT('Ctrl Pts',(-18.5906478871506,27.6105833589758,124.297248765221)) ;
#67604=CARTESIAN_POINT('Ctrl Pts',(-18.2097360022858,27.8005349300376,124.325031213336)) ;
#67605=CARTESIAN_POINT('Ctrl Pts',(-18.4496441165959,27.6205458496747,124.142390542805)) ;
#67606=CARTESIAN_POINT('Ctrl Pts',(-18.0691061956658,27.8105633584554,124.102135115778)) ;
#67607=CARTESIAN_POINT('Ctrl Pts',(-18.3371397875157,27.6305742780925,123.964073876923)) ;
#67608=CARTESIAN_POINT('Ctrl Pts',(-17.9704213296521,27.8204737258199,123.861134793012)) ;
#67609=CARTESIAN_POINT('Ctrl Pts',(-18.2581916587335,27.640484645457,123.771274472976)) ;
#67610=CARTESIAN_POINT('Ctrl Pts',(-17.9142719852206,27.830408593435,123.606158130962)) ;
#67611=CARTESIAN_POINT('Ctrl Pts',(-18.2132716018524,27.6504195130721,123.567293812213)) ;
#67612=CARTESIAN_POINT('Ctrl Pts',(-17.9033759753097,27.840449735414,123.342521266579)) ;
#67613=CARTESIAN_POINT('Ctrl Pts',(-18.2045541379343,27.6604606550512,123.356384198053)) ;
#67614=CARTESIAN_POINT('Ctrl Pts',(-17.9377060396121,27.8503368716172,123.084960416994)) ;
#67615=CARTESIAN_POINT('Ctrl Pts',(-18.2320173908359,27.6703477912543,123.150336250561)) ;
#67616=CARTESIAN_POINT('Ctrl Pts',(-18.0166431581778,27.8603291540206,122.834538577221)) ;
#67617=CARTESIAN_POINT('Ctrl Pts',(-18.2951662729315,27.6803400736577,122.94999869318)) ;
#67618=CARTESIAN_POINT('Ctrl Pts',(-18.137412126526,27.8702776819858,122.602650848213)) ;
#67619=CARTESIAN_POINT('Ctrl Pts',(-18.3917805539364,27.6902886016229,122.764488533233)) ;
#67620=CARTESIAN_POINT('Ctrl Pts',(-18.2961056898845,27.8802144131479,122.395304507949)) ;
#67621=CARTESIAN_POINT('Ctrl Pts',(-18.5187344032728,27.7002253327851,122.598611336762)) ;
#67622=CARTESIAN_POINT('Ctrl Pts',(-18.4891076721817,27.8901976240079,122.217558370946)) ;
#67623=CARTESIAN_POINT('Ctrl Pts',(-18.6731351964962,27.710208543645,122.456413869143)) ;
#67624=CARTESIAN_POINT('Ctrl Pts',(-18.7115707177152,27.9002407231578,122.075605016214)) ;
#67625=CARTESIAN_POINT('Ctrl Pts',(-18.8511053106445,27.7202516427949,122.342850400546)) ;
#67626=CARTESIAN_POINT('Ctrl Pts',(-18.9499871891245,27.9100716874327,121.976015433695)) ;
#67627=CARTESIAN_POINT('Ctrl Pts',(-19.041837051544,27.7300826070698,122.263178278936)) ;
#67628=CARTESIAN_POINT('Ctrl Pts',(-19.2081615249894,27.9201445398186,121.917767583989)) ;
#67629=CARTESIAN_POINT('Ctrl Pts',(-19.2483766156714,27.7401554594558,122.216578932533)) ;
#67630=CARTESIAN_POINT('Ctrl Pts',(-19.4671216625185,27.9300086675304,121.905533740892)) ;
#67631=CARTESIAN_POINT('Ctrl Pts',(-19.4555437647533,27.7500195871675,122.206790898622)) ;
#67632=CARTESIAN_POINT('Ctrl Pts',(-19.7284352632182,27.9400308696653,121.938326646805)) ;
#67633=CARTESIAN_POINT('Ctrl Pts',(-19.6645948238701,27.7600417893024,122.233024081806)) ;
#67634=CARTESIAN_POINT('Ctrl Pts',(-19.980050984628,27.9500580626337,122.016636385366)) ;
#67635=CARTESIAN_POINT('Ctrl Pts',(-19.8658877542819,27.7700689822708,122.295670925777)) ;
#67636=CARTESIAN_POINT('Ctrl Pts',(-20.2103950643466,27.9599136566007,122.135000592785)) ;
#67637=CARTESIAN_POINT('Ctrl Pts',(-20.0501626545512,27.7799245762378,122.39036086436)) ;
#67638=CARTESIAN_POINT('Ctrl Pts',(-20.4193072748828,27.969870828466,122.29257198083)) ;
#67639=CARTESIAN_POINT('Ctrl Pts',(-20.2172929209471,27.7898817481031,122.5164167495)) ;
#67640=CARTESIAN_POINT('Ctrl Pts',(-20.5987996284151,27.9799096724644,122.485885053549)) ;
#67641=CARTESIAN_POINT('Ctrl Pts',(-20.3608877406853,27.7999205921015,122.67106648784)) ;
#67642=CARTESIAN_POINT('Ctrl Pts',(-20.7400613604965,27.98978369634,122.703583668428)) ;
#67643=CARTESIAN_POINT('Ctrl Pts',(-20.4738977561458,27.8097946159771,122.845224005242)) ;
#67644=CARTESIAN_POINT('Ctrl Pts',(-20.8433506853364,27.9998535223304,122.947177423952)) ;
#67645=CARTESIAN_POINT('Ctrl Pts',(-20.5565304991962,27.8198644419675,123.040098768756)) ;
#67646=CARTESIAN_POINT('Ctrl Pts',(-20.9015266940339,28.0096867662276,123.198973980949)) ;
#67647=CARTESIAN_POINT('Ctrl Pts',(-20.6030723456922,27.8296976858648,123.241534723945)) ;
#67648=CARTESIAN_POINT('Ctrl Pts',(-20.9161142994382,28.0197171940007,123.462150342134)) ;
#67649=CARTESIAN_POINT('Ctrl Pts',(-20.6147438907103,27.8397281136378,123.452075801618)) ;
#67650=CARTESIAN_POINT('Ctrl Pts',(-20.8840166201033,28.0297488107458,123.72382387547)) ;
#67651=CARTESIAN_POINT('Ctrl Pts',(-20.5890670287782,27.8497597303829,123.661414851897)) ;
#67652=CARTESIAN_POINT('Ctrl Pts',(-20.80904662986,28.0395784877265,123.971001465148)) ;
#67653=CARTESIAN_POINT('Ctrl Pts',(-20.5290926826595,27.8595894073637,123.859156362875)) ;
#67654=CARTESIAN_POINT('Ctrl Pts',(-20.6910868706554,28.0495680045665,124.205529304447)) ;
#67655=CARTESIAN_POINT('Ctrl Pts',(-20.4347263402333,27.8695789242036,124.046779212421)) ;
#67656=CARTESIAN_POINT('Ctrl Pts',(-20.5328182779669,28.0596116167062,124.416742316167)) ;
#67657=CARTESIAN_POINT('Ctrl Pts',(-20.308112543254,27.8796225363434,124.215750577102)) ;
#67658=CARTESIAN_POINT('Ctrl Pts',(-20.3448814894554,28.0694342230415,124.593693576125)) ;
#67659=CARTESIAN_POINT('Ctrl Pts',(-20.1577648989237,27.8894451426787,124.357312023611)) ;
#67660=CARTESIAN_POINT('Ctrl Pts',(-20.124678185504,28.0794724529408,124.73892784558)) ;
#67661=CARTESIAN_POINT('Ctrl Pts',(-19.9816030855766,27.8994833725779,124.473500876513)) ;
#67662=CARTESIAN_POINT('Ctrl Pts',(-19.8829899980489,28.0894834877327,124.842887131756)) ;
#67663=CARTESIAN_POINT('Ctrl Pts',(-19.7882531778609,27.9094944073698,124.556669703237)) ;
#67664=CARTESIAN_POINT('Ctrl Pts',(-19.6299384968335,28.0993812186998,124.903017471924)) ;
#67665=CARTESIAN_POINT('Ctrl Pts',(-19.5858129211223,27.919392138337,124.60477541441)) ;
#67666=CARTESIAN_POINT('Ctrl Pts',(-19.3678981582499,28.1093708465503,124.918781274721)) ;
#67667=CARTESIAN_POINT('Ctrl Pts',(-19.3761808908369,27.9293817661874,124.617388123224)) ;
#67668=CARTESIAN_POINT('Ctrl Pts',(-19.1079954571358,28.1193266369963,124.888817431813)) ;
#67669=CARTESIAN_POINT('Ctrl Pts',(-19.1682588492881,27.9393375566334,124.593418735249)) ;
#67670=CARTESIAN_POINT('Ctrl Pts',(-18.8578037171305,28.1292540355584,124.814868421456)) ;
#67671=CARTESIAN_POINT('Ctrl Pts',(-18.968105356819,27.9492649551955,124.534261321663)) ;
#67672=CARTESIAN_POINT('Ctrl Pts',(-18.6219935808609,28.1392796306682,124.697390886151)) ;
#67673=CARTESIAN_POINT('Ctrl Pts',(-18.7794564590463,27.9592905503054,124.440280839266)) ;
#67674=CARTESIAN_POINT('Ctrl Pts',(-18.413012495007,28.1491654813378,124.543058534145)) ;
#67675=CARTESIAN_POINT('Ctrl Pts',(-18.612271014501,27.9691764009749,124.316816723086)) ;
#67676=CARTESIAN_POINT('Ctrl Pts',(-18.2316780606301,28.159154661182,124.353241304876)) ;
#67677=CARTESIAN_POINT('Ctrl Pts',(-18.4672022077259,27.9791655808191,124.164964317004)) ;
#67678=CARTESIAN_POINT('Ctrl Pts',(-18.085762555499,28.1691958482856,124.133385523761)) ;
#67679=CARTESIAN_POINT('Ctrl Pts',(-18.3504682851199,27.9892067679227,123.989080612378)) ;
#67680=CARTESIAN_POINT('Ctrl Pts',(-17.9820414176768,28.1790284917615,123.896729581303)) ;
#67681=CARTESIAN_POINT('Ctrl Pts',(-18.2674899943736,27.9990394113987,123.799757297218)) ;
#67682=CARTESIAN_POINT('Ctrl Pts',(-17.9192545217861,28.189022441471,123.641716424028)) ;
#67683=CARTESIAN_POINT('Ctrl Pts',(-18.2172586037933,28.0090333611081,123.595747332759)) ;
#67684=CARTESIAN_POINT('Ctrl Pts',(-17.9021928664862,28.1990515642475,123.378711840277)) ;
#67685=CARTESIAN_POINT('Ctrl Pts',(-18.2036074112526,28.0190624838847,123.385343770105)) ;
#67686=CARTESIAN_POINT('Ctrl Pts',(-17.9302039422221,28.2089276951662,123.120680343544)) ;
#67687=CARTESIAN_POINT('Ctrl Pts',(-18.2260142937599,28.0289386148033,123.178918899042)) ;
#67688=CARTESIAN_POINT('Ctrl Pts',(-18.0031776926144,28.2189257301832,122.86831261201)) ;
#67689=CARTESIAN_POINT('Ctrl Pts',(-18.2843913725109,28.0389366498204,122.977024252251)) ;
#67690=CARTESIAN_POINT('Ctrl Pts',(-18.117736776842,28.2288396599419,122.634287677194)) ;
#67691=CARTESIAN_POINT('Ctrl Pts',(-18.376036681339,28.0488505795791,122.789803759949)) ;
#67692=CARTESIAN_POINT('Ctrl Pts',(-18.2731150794606,28.2388828476797,122.420974122389)) ;
#67693=CARTESIAN_POINT('Ctrl Pts',(-18.5003377353294,28.0588937673169,122.619151688384)) ;
#67694=CARTESIAN_POINT('Ctrl Pts',(-18.4604722427515,28.2487826898201,122.24045743561)) ;
#67695=CARTESIAN_POINT('Ctrl Pts',(-18.6502217887544,28.0687936094572,122.474737169911)) ;
#67696=CARTESIAN_POINT('Ctrl Pts',(-18.6779981948743,28.2587739566281,122.093415286291)) ;
#67697=CARTESIAN_POINT('Ctrl Pts',(-18.8242413102653,28.0787848762652,122.357101786154)) ;
#67698=CARTESIAN_POINT('Ctrl Pts',(-18.918918044841,28.2688060587601,121.986355077235)) ;
#67699=CARTESIAN_POINT('Ctrl Pts',(-19.0169763807828,28.0888169783972,122.271451769572)) ;
#67700=CARTESIAN_POINT('Ctrl Pts',(-19.1704626082505,28.2786729397148,121.923469734543)) ;
#67701=CARTESIAN_POINT('Ctrl Pts',(-19.2182110752363,28.098683859352,122.221141611949)) ;
#67702=CARTESIAN_POINT('Ctrl Pts',(-19.432345213223,28.288664731003,121.904359612356)) ;
#67703=CARTESIAN_POINT('Ctrl Pts',(-19.4277169183523,28.1086756506401,122.20585140049)) ;
#67704=CARTESIAN_POINT('Ctrl Pts',(-19.694564039776,28.2986968469145,121.93162572317)) ;
#67705=CARTESIAN_POINT('Ctrl Pts',(-19.6374921940647,28.1187077665516,122.227662228157)) ;
#67706=CARTESIAN_POINT('Ctrl Pts',(-19.943995852301,28.3085631637145,122.002434913296)) ;
#67707=CARTESIAN_POINT('Ctrl Pts',(-19.8370378243453,28.1285740833517,122.284307435928)) ;
#67708=CARTESIAN_POINT('Ctrl Pts',(-20.1803573809643,28.3185506451881,122.116461326157)) ;
#67709=CARTESIAN_POINT('Ctrl Pts',(-20.0261278945652,28.1385615648253,122.375526584252)) ;
#67710=CARTESIAN_POINT('Ctrl Pts',(-20.3925607131235,28.328495569567,122.269070719418)) ;
#67711=CARTESIAN_POINT('Ctrl Pts',(-20.1958916697619,28.1485064892042,122.497612235911)) ;
#67712=CARTESIAN_POINT('Ctrl Pts',(-20.5767268496923,28.3385404554777,122.458146387094)) ;
#67713=CARTESIAN_POINT('Ctrl Pts',(-20.343226130455,28.1585513751149,122.648871279974)) ;
#67714=CARTESIAN_POINT('Ctrl Pts',(-20.7227745276264,28.3484025591903,122.672264744843)) ;
#67715=CARTESIAN_POINT('Ctrl Pts',(-20.4600658712918,28.1684134788274,122.820164463442)) ;
#67716=CARTESIAN_POINT('Ctrl Pts',(-20.8312927348308,28.3583941230148,122.911337082898)) ;
#67717=CARTESIAN_POINT('Ctrl Pts',(-20.5468824144814,28.1784050426519,123.011421352625)) ;
#67718=CARTESIAN_POINT('Ctrl Pts',(-20.8961668071842,28.3683269310777,123.164169825498)) ;
#67719=CARTESIAN_POINT('Ctrl Pts',(-20.5987837570556,28.1883378507148,123.213686829248)) ;
#67720=CARTESIAN_POINT('Ctrl Pts',(-20.9168053566465,28.378264033314,123.424505796562)) ;
#67721=CARTESIAN_POINT('Ctrl Pts',(-20.615296810215,28.1982749529511,123.421955292323)) ;
#67722=CARTESIAN_POINT('Ctrl Pts',(-20.8912939664117,28.3883164795844,123.687418366482)) ;
#67723=CARTESIAN_POINT('Ctrl Pts',(-20.5948899052389,28.2083273992215,123.632285549448)) ;
#67724=CARTESIAN_POINT('Ctrl Pts',(-20.8223185569164,28.398162595166,123.936824298385)) ;
#67725=CARTESIAN_POINT('Ctrl Pts',(-20.5397117877283,28.2181735148031,123.831810673226)) ;
#67726=CARTESIAN_POINT('Ctrl Pts',(-20.709193147176,28.4082106148809,124.175395051952)) ;
#67727=CARTESIAN_POINT('Ctrl Pts',(-20.4492134944853,28.228221534518,124.022668227718)) ;
#67728=CARTESIAN_POINT('Ctrl Pts',(-20.5576594223878,28.4181525665098,124.388243230741)) ;
#67729=CARTESIAN_POINT('Ctrl Pts',(-20.3279884025434,28.238163486147,124.192947972631)) ;
#67730=CARTESIAN_POINT('Ctrl Pts',(-20.3719920554206,28.4280913475089,124.571940487482)) ;
#67731=CARTESIAN_POINT('Ctrl Pts',(-20.1794561524199,28.248102267146,124.339907313728)) ;
#67732=CARTESIAN_POINT('Ctrl Pts',(-20.155266255181,28.438117396235,124.721739105602)) ;
#67733=CARTESIAN_POINT('Ctrl Pts',(-20.0060768524774,28.2581283158721,124.45974803094)) ;
#67734=CARTESIAN_POINT('Ctrl Pts',(-19.9192398618305,28.4480042566432,124.830426395165)) ;
#67735=CARTESIAN_POINT('Ctrl Pts',(-19.8172566995611,28.2680151762803,124.546699853667)) ;
#67736=CARTESIAN_POINT('Ctrl Pts',(-19.6643603212813,28.458035531775,124.897541005947)) ;
#67737=CARTESIAN_POINT('Ctrl Pts',(-19.6133539336829,28.2780464514121,124.600393764835)) ;
#67738=CARTESIAN_POINT('Ctrl Pts',(-19.405507635062,28.4679185090754,124.919330220156)) ;
#67739=CARTESIAN_POINT('Ctrl Pts',(-19.4062711317406,28.2879294287125,124.617827171934)) ;
#67740=CARTESIAN_POINT('Ctrl Pts',(-19.14236864725,28.4779753624826,124.895445755536)) ;
#67741=CARTESIAN_POINT('Ctrl Pts',(-19.1957631355811,28.2979862821197,124.598722613177)) ;
#67742=CARTESIAN_POINT('Ctrl Pts',(-18.8081529113529,28.4911436035585,124.80533200887)) ;
#67743=CARTESIAN_POINT('Ctrl Pts',(-18.9283732060215,28.3111545231956,124.526630734819)) ;
#67744=CARTESIAN_POINT('Ctrl Pts',(-18.4999549682012,28.504544632785,124.627092881207)) ;
#67745=CARTESIAN_POINT('Ctrl Pts',(-18.681798248427,28.3245555524222,124.384021484789)) ;
#67746=CARTESIAN_POINT('Ctrl Pts',(-18.2548346129752,28.5177575495159,124.381018273064)) ;
#67747=CARTESIAN_POINT('Ctrl Pts',(-18.4857344323844,28.337768469153,124.187192189279)) ;
#67748=CARTESIAN_POINT('Ctrl Pts',(-18.1049098192041,28.5276859439691,124.167554176501)) ;
#67749=CARTESIAN_POINT('Ctrl Pts',(-18.3657857952432,28.3476968636062,124.016416466804)) ;
#67750=CARTESIAN_POINT('Ctrl Pts',(-17.9935167509591,28.5376674440972,123.930036177092)) ;
#67751=CARTESIAN_POINT('Ctrl Pts',(-18.2766712098695,28.3576783637344,123.826404555807)) ;
#67752=CARTESIAN_POINT('Ctrl Pts',(-17.9250194853092,28.5477079873673,123.675241990111)) ;
#67753=CARTESIAN_POINT('Ctrl Pts',(-18.2218707823498,28.3677189070045,123.622569449493)) ;
#67754=CARTESIAN_POINT('Ctrl Pts',(-17.9019033242933,28.5575573191504,123.417442838969)) ;
#67755=CARTESIAN_POINT('Ctrl Pts',(-18.2033757289784,28.3775682387876,123.416330378134)) ;
#67756=CARTESIAN_POINT('Ctrl Pts',(-17.9235537436292,28.5675527236221,123.155670875178)) ;
#67757=CARTESIAN_POINT('Ctrl Pts',(-18.2206940100474,28.3875636432592,123.206912092977)) ;
#67758=CARTESIAN_POINT('Ctrl Pts',(-17.990923682755,28.5775690510707,122.901217359065)) ;
#67759=CARTESIAN_POINT('Ctrl Pts',(-18.2745872927144,28.3975799707078,123.003350782383)) ;
#67760=CARTESIAN_POINT('Ctrl Pts',(-18.1363563321866,28.5907927082372,122.585573838039)) ;
#67761=CARTESIAN_POINT('Ctrl Pts',(-18.3909334946143,28.4108036278744,122.750824793006)) ;
#67762=CARTESIAN_POINT('Ctrl Pts',(-18.361738888197,28.6040869996266,122.313564150216)) ;
#67763=CARTESIAN_POINT('Ctrl Pts',(-18.5712653371683,28.4240979192637,122.533196651324)) ;
#67764=CARTESIAN_POINT('Ctrl Pts',(-18.6465253994931,28.6173713505581,122.111531614028)) ;
#67765=CARTESIAN_POINT('Ctrl Pts',(-18.7990570818657,28.4373822701952,122.371600047551)) ;
#67766=CARTESIAN_POINT('Ctrl Pts',(-18.8832307222806,28.6273437316199,121.999158080089)) ;
#67767=CARTESIAN_POINT('Ctrl Pts',(-18.9884277554392,28.447354651257,122.281692950129)) ;
#67768=CARTESIAN_POINT('Ctrl Pts',(-19.1341788049863,28.6372521112455,121.929579826141)) ;
#67769=CARTESIAN_POINT('Ctrl Pts',(-19.1891837168037,28.4572630308826,122.22602983351)) ;
#67770=CARTESIAN_POINT('Ctrl Pts',(-19.3971551455222,28.6473061099936,121.904389073441)) ;
#67771=CARTESIAN_POINT('Ctrl Pts',(-19.3995659464143,28.4673170296307,122.205875390456)) ;
#67772=CARTESIAN_POINT('Ctrl Pts',(-19.6555567772795,28.6571683071099,121.924649710965)) ;
#67773=CARTESIAN_POINT('Ctrl Pts',(-19.6062837665613,28.477179226747,122.222079569028)) ;
#67774=CARTESIAN_POINT('Ctrl Pts',(-19.9952798306344,28.670515433484,122.011813758423)) ;
#67775=CARTESIAN_POINT('Ctrl Pts',(-19.8780825920856,28.4905263531211,122.291820399844)) ;
#67776=CARTESIAN_POINT('Ctrl Pts',(-20.3783371558031,28.6870523991254,122.227433848027)) ;
#67777=CARTESIAN_POINT('Ctrl Pts',(-20.1845001448543,28.5070633187626,122.464288220489)) ;
#67778=CARTESIAN_POINT('Ctrl Pts',(-20.6669572705968,28.7036870032994,122.562229846375)) ;
#67779=CARTESIAN_POINT('Ctrl Pts',(-20.4154369512327,28.5236979229365,122.73217404382)) ;
#67780=CARTESIAN_POINT('Ctrl Pts',(-20.818619503667,28.716976796542,122.876897221786)) ;
#67781=CARTESIAN_POINT('Ctrl Pts',(-20.536739963039,28.5369877161791,122.983864515057)) ;
#67782=CARTESIAN_POINT('Ctrl Pts',(-20.8898646071741,28.7269294278014,123.12852052043)) ;
#67783=CARTESIAN_POINT('Ctrl Pts',(-20.5937435077852,28.5469403474385,123.185172022197)) ;
#67784=CARTESIAN_POINT('Ctrl Pts',(-20.916646989976,28.7368813951061,123.388702342932)) ;
#67785=CARTESIAN_POINT('Ctrl Pts',(-20.6151704550531,28.5568923147432,123.393312774312)) ;
#67786=CARTESIAN_POINT('Ctrl Pts',(-20.891192739327,28.7502486535699,123.739016958567)) ;
#67787=CARTESIAN_POINT('Ctrl Pts',(-20.5948058393565,28.570259573207,123.673577519016)) ;
#67788=CARTESIAN_POINT('Ctrl Pts',(-20.7477418810432,28.7667654655191,124.154036877155)) ;
#67789=CARTESIAN_POINT('Ctrl Pts',(-20.4800520421779,28.5867763851562,124.005580886931)) ;
#67790=CARTESIAN_POINT('Ctrl Pts',(-20.4126932064644,28.7867913605254,124.567418944492)) ;
#67791=CARTESIAN_POINT('Ctrl Pts',(-20.2120144196254,28.6068022801626,124.336293127083)) ;
#67792=CARTESIAN_POINT('Ctrl Pts',(-19.9614615275447,28.8066020906556,124.838970603354)) ;
#67793=CARTESIAN_POINT('Ctrl Pts',(-19.8510300684342,28.6266130102927,124.553536623259)) ;
#67794=CARTESIAN_POINT('Ctrl Pts',(-19.4406750274565,28.8265793067854,124.942183198345)) ;
#67795=CARTESIAN_POINT('Ctrl Pts',(-19.4344011473137,28.6465902264226,124.636109825958)) ;
#67796=CARTESIAN_POINT('Ctrl Pts',(-18.9173848458449,28.8465061821807,124.860730356123)) ;
#67797=CARTESIAN_POINT('Ctrl Pts',(-19.015768045154,28.6665171018178,124.570950325204)) ;
#67798=CARTESIAN_POINT('Ctrl Pts',(-18.4548495376105,28.866327643657,124.608386572972)) ;
#67799=CARTESIAN_POINT('Ctrl Pts',(-18.6457373585372,28.6863385632941,124.36907662557)) ;
#67800=CARTESIAN_POINT('Ctrl Pts',(-18.1021082199431,28.8864019614663,124.20819190284)) ;
#67801=CARTESIAN_POINT('Ctrl Pts',(-18.3635430360855,28.7064128811034,124.048922914079)) ;
#67802=CARTESIAN_POINT('Ctrl Pts',(-17.9097030414757,28.9062499304742,123.716849978485)) ;
#67803=CARTESIAN_POINT('Ctrl Pts',(-18.2096162521416,28.7262608501113,123.655848998423)) ;
#67804=CARTESIAN_POINT('Ctrl Pts',(-17.8953659112392,28.9261969645374,123.187000088179)) ;
#67805=CARTESIAN_POINT('Ctrl Pts',(-18.1981447291151,28.7462078841745,123.231968583052)) ;
#67806=CARTESIAN_POINT('Ctrl Pts',(-18.0624463345147,28.9460929155096,122.685244684184)) ;
#67807=CARTESIAN_POINT('Ctrl Pts',(-18.3318078029622,28.7661038351467,122.830562717796)) ;
#67808=CARTESIAN_POINT('Ctrl Pts',(-18.3899816868081,28.9659883951278,122.270147568337)) ;
#67809=CARTESIAN_POINT('Ctrl Pts',(-18.5938359071739,28.7859993147649,122.498483387)) ;
#67810=CARTESIAN_POINT('Ctrl Pts',(-18.8408757372252,28.9859445060926,121.990748528834)) ;
#67811=CARTESIAN_POINT('Ctrl Pts',(-18.9545510633946,28.8059554257297,122.274963123727)) ;
#67812=CARTESIAN_POINT('Ctrl Pts',(-19.3586261760562,29.0058490541326,121.882442313881)) ;
#67813=CARTESIAN_POINT('Ctrl Pts',(-19.3687524196573,28.8258599737697,122.188317114002)) ;
#67814=CARTESIAN_POINT('Ctrl Pts',(-19.8818129365437,29.0257231784517,121.95590917428)) ;
#67815=CARTESIAN_POINT('Ctrl Pts',(-19.7873033983275,28.8457340980888,122.24709086078)) ;
#67816=CARTESIAN_POINT('Ctrl Pts',(-20.3522418344828,29.0457777084507,122.206339109689)) ;
#67817=CARTESIAN_POINT('Ctrl Pts',(-20.1636459491141,28.8657886280878,122.447434352417)) ;
#67818=CARTESIAN_POINT('Ctrl Pts',(-20.7048254925126,29.0655852222107,122.597429836113)) ;
#67819=CARTESIAN_POINT('Ctrl Pts',(-20.4457143874069,28.8855961418478,122.760308841788)) ;
#67820=CARTESIAN_POINT('Ctrl Pts',(-20.9055115949536,29.0855685779784,123.089100356984)) ;
#67821=CARTESIAN_POINT('Ctrl Pts',(-20.6062625174432,28.9055794976156,123.153645765125)) ;
#67822=CARTESIAN_POINT('Ctrl Pts',(-20.9255057422183,29.1054868805624,123.618111697477)) ;
#67823=CARTESIAN_POINT('Ctrl Pts',(-20.622257172822,28.9254978001995,123.576855858986)) ;
#67824=CARTESIAN_POINT('Ctrl Pts',(-20.7655021762044,29.1253550960081,124.121463964361)) ;
#67825=CARTESIAN_POINT('Ctrl Pts',(-20.4942524673024,28.9453660156452,123.979538536319)) ;
#67826=CARTESIAN_POINT('Ctrl Pts',(-20.4398756731327,29.1454054128044,124.543114839599)) ;
#67827=CARTESIAN_POINT('Ctrl Pts',(-20.2337505118372,28.9654163324415,124.316858031653)) ;
#67828=CARTESIAN_POINT('Ctrl Pts',(-19.9961359923068,29.1651814746869,124.82522657557)) ;
#67829=CARTESIAN_POINT('Ctrl Pts',(-19.878755955537,28.985192394324,124.542547120948)) ;
#67830=CARTESIAN_POINT('Ctrl Pts',(-19.4760372478541,29.1852360803793,124.9408742549)) ;
#67831=CARTESIAN_POINT('Ctrl Pts',(-19.4626769826316,29.0052470000165,124.63506310846)) ;
#67832=CARTESIAN_POINT('Ctrl Pts',(-18.9542188864203,29.2050297695352,124.872787108227)) ;
#67833=CARTESIAN_POINT('Ctrl Pts',(-19.0452207775086,29.0250406891723,124.580591027841)) ;
#67834=CARTESIAN_POINT('Ctrl Pts',(-18.4824497195716,29.2249964611296,124.630017164074)) ;
#67835=CARTESIAN_POINT('Ctrl Pts',(-18.667806512202,29.0450073807667,124.386372476876)) ;
#67836=CARTESIAN_POINT('Ctrl Pts',(-18.1224282621344,29.2449565068806,124.240242601981)) ;
#67837=CARTESIAN_POINT('Ctrl Pts',(-18.3797910944419,29.0649674265177,124.074550845858)) ;
#67838=CARTESIAN_POINT('Ctrl Pts',(-17.9173907834527,29.2648547670308,123.752777846934)) ;
#67839=CARTESIAN_POINT('Ctrl Pts',(-18.2157634593431,29.084865686668,123.68457721216)) ;
#67840=CARTESIAN_POINT('Ctrl Pts',(-17.8903701259974,29.28474968258,123.224718223152)) ;
#67841=CARTESIAN_POINT('Ctrl Pts',(-18.1941500680826,29.1047606022171,123.262128658022)) ;
#67842=CARTESIAN_POINT('Ctrl Pts',(-18.0448227791641,29.3046598629936,122.718584462674)) ;
#67843=CARTESIAN_POINT('Ctrl Pts',(-18.3177155786987,29.1246707826307,122.857222129875)) ;
#67844=CARTESIAN_POINT('Ctrl Pts',(-18.3629508949474,29.3245956621079,122.294833096222)) ;
#67845=CARTESIAN_POINT('Ctrl Pts',(-18.5722211306576,29.144606581745,122.518222926126)) ;
#67846=CARTESIAN_POINT('Ctrl Pts',(-18.8065966645385,29.344533523762,122.005031573975)) ;
#67847=CARTESIAN_POINT('Ctrl Pts',(-18.9271398869184,29.1645444433991,122.28638447727)) ;
#67848=CARTESIAN_POINT('Ctrl Pts',(-19.3219781329333,29.3644525703997,121.88380547982)) ;
#67849=CARTESIAN_POINT('Ctrl Pts',(-19.339446619592,29.1844634900368,122.189407632627)) ;
#67850=CARTESIAN_POINT('Ctrl Pts',(-19.8485530096058,29.3844014684538,121.945745518254)) ;
#67851=CARTESIAN_POINT('Ctrl Pts',(-19.7607049211448,29.2044123880909,122.238961921839)) ;
#67852=CARTESIAN_POINT('Ctrl Pts',(-20.3214474198052,29.4043072958969,122.18303123303)) ;
#67853=CARTESIAN_POINT('Ctrl Pts',(-20.1390239324075,29.224318215534,122.428800199034)) ;
#67854=CARTESIAN_POINT('Ctrl Pts',(-20.6245684184595,29.4208899912622,122.502888255951)) ;
#67855=CARTESIAN_POINT('Ctrl Pts',(-20.381503037069,29.2409009108993,122.684669703668)) ;
#67856=CARTESIAN_POINT('Ctrl Pts',(-20.791234180934,29.4341642049858,122.809390920718)) ;
#67857=CARTESIAN_POINT('Ctrl Pts',(-20.5148468140483,29.2541751246229,122.929890379545)) ;
#67858=CARTESIAN_POINT('Ctrl Pts',(-20.8750220852076,29.4442109241851,123.05973121324)) ;
#67859=CARTESIAN_POINT('Ctrl Pts',(-20.5818729237177,29.2642218438223,123.13015699649)) ;
#67860=CARTESIAN_POINT('Ctrl Pts',(-20.9135737768039,29.4540549588308,123.315549607641)) ;
#67861=CARTESIAN_POINT('Ctrl Pts',(-20.6127109316255,29.2740658784679,123.334824035889)) ;
#67862=CARTESIAN_POINT('Ctrl Pts',(-20.9056110532671,29.4673893437353,123.665862635849)) ;
#67863=CARTESIAN_POINT('Ctrl Pts',(-20.6063479581414,29.2874002633725,123.615020710436)) ;
#67864=CARTESIAN_POINT('Ctrl Pts',(-20.7817183691016,29.4839765610351,124.089008121444)) ;
#67865=CARTESIAN_POINT('Ctrl Pts',(-20.5072137252115,29.3039874806722,123.953603177572)) ;
#67866=CARTESIAN_POINT('Ctrl Pts',(-20.5204871039959,29.500609773073,124.445591168462)) ;
#67867=CARTESIAN_POINT('Ctrl Pts',(-20.2982490932776,29.3206206927101,124.238824480431)) ;
#67868=CARTESIAN_POINT('Ctrl Pts',(-20.2482786094575,29.5138922153452,124.664142759317)) ;
#67869=CARTESIAN_POINT('Ctrl Pts',(-20.0804621387608,29.3339031349823,124.413688421931)) ;
#67870=CARTESIAN_POINT('Ctrl Pts',(-20.0203496111071,29.5237981032594,124.789853895898)) ;
#67871=CARTESIAN_POINT('Ctrl Pts',(-19.8981216151747,29.3438090228965,124.514250475789)) ;
#67872=CARTESIAN_POINT('Ctrl Pts',(-19.7720804977814,29.5337865213645,124.875101645455)) ;
#67873=CARTESIAN_POINT('Ctrl Pts',(-19.699504035617,29.3537974410017,124.582447706781)) ;
#67874=CARTESIAN_POINT('Ctrl Pts',(-19.5118312861888,29.5438099486033,124.9158105401)) ;
#67875=CARTESIAN_POINT('Ctrl Pts',(-19.4913069695219,29.3638208682404,124.615012953148)) ;
#67876=CARTESIAN_POINT('Ctrl Pts',(-19.2516162816116,29.5537143797203,124.910922144998)) ;
#67877=CARTESIAN_POINT('Ctrl Pts',(-19.2831262502567,29.3737252993574,124.611097513249)) ;
#67878=CARTESIAN_POINT('Ctrl Pts',(-18.9093488133413,29.5669775323307,124.844857601197)) ;
#67879=CARTESIAN_POINT('Ctrl Pts',(-19.0093557497466,29.3869884519678,124.558255787372)) ;
#67880=CARTESIAN_POINT('Ctrl Pts',(-18.5909285364746,29.5803024302346,124.689972489664)) ;
#67881=CARTESIAN_POINT('Ctrl Pts',(-18.7545953313426,29.4003133498717,124.434343999134)) ;
#67882=CARTESIAN_POINT('Ctrl Pts',(-18.3276416499704,29.5935581738502,124.461801734779)) ;
#67883=CARTESIAN_POINT('Ctrl Pts',(-18.5439553434392,29.4135690934873,124.251793461498)) ;
#67884=CARTESIAN_POINT('Ctrl Pts',(-18.1623453454126,29.6035175472975,124.258928464813)) ;
#67885=CARTESIAN_POINT('Ctrl Pts',(-18.4117225892705,29.4235284669346,124.089495803923)) ;
#67886=CARTESIAN_POINT('Ctrl Pts',(-18.0346636089127,29.6134613712245,124.030895956569)) ;
#67887=CARTESIAN_POINT('Ctrl Pts',(-18.3095785285436,29.4334722908616,123.907068119568)) ;
#67888=CARTESIAN_POINT('Ctrl Pts',(-17.9478442966657,29.6235093153718,123.781548712612)) ;
#67889=CARTESIAN_POINT('Ctrl Pts',(-18.2401254083158,29.4435202350089,123.707589793291)) ;
#67890=CARTESIAN_POINT('Ctrl Pts',(-17.906234953778,29.6333602865899,123.526025793516)) ;
#67891=CARTESIAN_POINT('Ctrl Pts',(-18.2068401299479,29.4533712062271,123.503171143586)) ;
#67892=CARTESIAN_POINT('Ctrl Pts',(-17.9089904954044,29.643332104032,123.264021399714)) ;
#67893=CARTESIAN_POINT('Ctrl Pts',(-18.2090468245195,29.4633430236691,123.293567757575)) ;
#67894=CARTESIAN_POINT('Ctrl Pts',(-17.9573656877064,29.6533275263241,123.005808163303)) ;
#67895=CARTESIAN_POINT('Ctrl Pts',(-18.2477491698236,29.4733384459612,123.086997640274)) ;
#67896=CARTESIAN_POINT('Ctrl Pts',(-18.0504309097234,29.6633605914478,122.75912999775)) ;
#67897=CARTESIAN_POINT('Ctrl Pts',(-18.3222034468051,29.4833715110849,122.88965593636)) ;
#67898=CARTESIAN_POINT('Ctrl Pts',(-18.1824501820335,29.673225924113,122.536018472183)) ;
#67899=CARTESIAN_POINT('Ctrl Pts',(-18.4278207101303,29.4932368437501,122.711168011498)) ;
#67900=CARTESIAN_POINT('Ctrl Pts',(-18.352254460823,29.6831864667106,122.336809734032)) ;
#67901=CARTESIAN_POINT('Ctrl Pts',(-18.5636657405991,29.5031973863477,122.551802554504)) ;
#67902=CARTESIAN_POINT('Ctrl Pts',(-18.5558196647205,29.6932201522123,122.169242143868)) ;
#67903=CARTESIAN_POINT('Ctrl Pts',(-18.7265193140521,29.5132310718494,122.417750218351)) ;
#67904=CARTESIAN_POINT('Ctrl Pts',(-18.7818025397086,29.7031049842026,122.041072921772)) ;
#67905=CARTESIAN_POINT('Ctrl Pts',(-18.9073065097523,29.5231159038397,122.315216877536)) ;
#67906=CARTESIAN_POINT('Ctrl Pts',(-19.0310733364163,29.7131724109624,121.952565569517)) ;
#67907=CARTESIAN_POINT('Ctrl Pts',(-19.1067239210886,29.5331833305995,122.24441307792)) ;
#67908=CARTESIAN_POINT('Ctrl Pts',(-19.286036901977,29.7230109001213,121.909416064618)) ;
#67909=CARTESIAN_POINT('Ctrl Pts',(-19.3106948134357,29.5430218197584,122.209895699158)) ;
#67910=CARTESIAN_POINT('Ctrl Pts',(-19.550453199473,29.7330743813114,121.910880737687)) ;
#67911=CARTESIAN_POINT('Ctrl Pts',(-19.5222278763447,29.5530853009485,122.211069619433)) ;
#67912=CARTESIAN_POINT('Ctrl Pts',(-19.8062464008285,29.7429685391265,121.957671456219)) ;
#67913=CARTESIAN_POINT('Ctrl Pts',(-19.7268617815842,29.5629794587636,122.248504306379)) ;
#67914=CARTESIAN_POINT('Ctrl Pts',(-20.0513931602021,29.7529103958708,122.047912589705)) ;
#67915=CARTESIAN_POINT('Ctrl Pts',(-19.9229782497092,29.5729213155079,122.320699150998)) ;
#67916=CARTESIAN_POINT('Ctrl Pts',(-20.27863327422,29.7629128735422,122.180100002924)) ;
#67917=CARTESIAN_POINT('Ctrl Pts',(-20.1047692120472,29.5829237931793,122.426450889047)) ;
#67918=CARTESIAN_POINT('Ctrl Pts',(-20.4798098359431,29.7729476778465,122.350566712122)) ;
#67919=CARTESIAN_POINT('Ctrl Pts',(-20.265709069093,29.5929585974836,122.562825920578)) ;
#67920=CARTESIAN_POINT('Ctrl Pts',(-20.64549843004,29.7827925546922,122.549284780308)) ;
#67921=CARTESIAN_POINT('Ctrl Pts',(-20.3982580187208,29.6028034743293,122.721801389537)) ;
#67922=CARTESIAN_POINT('Ctrl Pts',(-20.7764071388104,29.7927784342477,122.776669844146)) ;
#67923=CARTESIAN_POINT('Ctrl Pts',(-20.5029831155846,29.6127893538848,122.903710368416)) ;
#67924=CARTESIAN_POINT('Ctrl Pts',(-20.8655976909384,29.8027131646062,123.022090489185)) ;
#67925=CARTESIAN_POINT('Ctrl Pts',(-20.5743335346531,29.6227240842433,123.100047340193)) ;
#67926=CARTESIAN_POINT('Ctrl Pts',(-20.911118673284,29.8127709769191,123.2824053866)) ;
#67927=CARTESIAN_POINT('Ctrl Pts',(-20.6107482780399,29.6327818965562,123.308299712704)) ;
#67928=CARTESIAN_POINT('Ctrl Pts',(-20.9112011989042,29.8225915690435,123.540523528446)) ;
#67929=CARTESIAN_POINT('Ctrl Pts',(-20.610812264355,29.6426024886806,123.514793589066)) ;
#67930=CARTESIAN_POINT('Ctrl Pts',(-20.8656816934186,29.8326581546532,123.801062971402)) ;
#67931=CARTESIAN_POINT('Ctrl Pts',(-20.5743946700159,29.6526690742904,123.723224921033)) ;
#67932=CARTESIAN_POINT('Ctrl Pts',(-20.7770260888292,29.8425577352351,124.045706385067)) ;
#67933=CARTESIAN_POINT('Ctrl Pts',(-20.503468442044,29.6625686548722,123.918938590259)) ;
#67934=CARTESIAN_POINT('Ctrl Pts',(-20.6453879764234,29.8526093349133,124.274656477308)) ;
#67935=CARTESIAN_POINT('Ctrl Pts',(-20.398156179075,29.6726202545505,124.102097751505)) ;
#67936=CARTESIAN_POINT('Ctrl Pts',(-20.4790736605817,29.8624835213303,124.473897491922)) ;
#67937=CARTESIAN_POINT('Ctrl Pts',(-20.2651035506588,29.6824944409674,124.261488905988)) ;
#67938=CARTESIAN_POINT('Ctrl Pts',(-20.2772141277769,29.8725399972112,124.644389380226)) ;
#67939=CARTESIAN_POINT('Ctrl Pts',(-20.1036145883348,29.6925509168483,124.39788099837)) ;
#67940=CARTESIAN_POINT('Ctrl Pts',(-20.0524919644059,29.8824329285138,124.775217544899)) ;
#67941=CARTESIAN_POINT('Ctrl Pts',(-19.9238362960661,29.7024438481509,124.502541627271)) ;
#67942=CARTESIAN_POINT('Ctrl Pts',(-19.8043884253136,29.8924957072264,124.866595201475)) ;
#67943=CARTESIAN_POINT('Ctrl Pts',(-19.7253526612113,29.7125066268636,124.57564199753)) ;
#67944=CARTESIAN_POINT('Ctrl Pts',(-19.5498333322758,29.9023382328076,124.91262179111)) ;
#67945=CARTESIAN_POINT('Ctrl Pts',(-19.5217089312482,29.7223491524447,124.612461273201)) ;
#67946=CARTESIAN_POINT('Ctrl Pts',(-19.2873260771025,29.9123289982325,124.914394172825)) ;
#67947=CARTESIAN_POINT('Ctrl Pts',(-19.3117032550328,29.7323399178696,124.613877366799)) ;
#67948=CARTESIAN_POINT('Ctrl Pts',(-19.0300851291776,29.9222570742305,124.870781057726)) ;
#67949=CARTESIAN_POINT('Ctrl Pts',(-19.1059111853094,29.7422679938676,124.578985150407)) ;
#67950=CARTESIAN_POINT('Ctrl Pts',(-18.7826904157509,29.9322449846175,124.783069756764)) ;
#67951=CARTESIAN_POINT('Ctrl Pts',(-18.9079961342318,29.7522559042547,124.508814517184)) ;
#67952=CARTESIAN_POINT('Ctrl Pts',(-18.5534253143983,29.9422808967425,124.652734665094)) ;
#67953=CARTESIAN_POINT('Ctrl Pts',(-18.7245848901154,29.7622918163796,124.404544830416)) ;
#67954=CARTESIAN_POINT('Ctrl Pts',(-18.3536388771245,29.9521359095901,124.487912827377)) ;
#67955=CARTESIAN_POINT('Ctrl Pts',(-18.5647574170873,29.7721468292273,124.272686483657)) ;
#67956=CARTESIAN_POINT('Ctrl Pts',(-18.1828123336801,29.9621348555064,124.288313606199)) ;
#67957=CARTESIAN_POINT('Ctrl Pts',(-18.4280975323811,29.7821457751435,124.113006096126)) ;
#67958=CARTESIAN_POINT('Ctrl Pts',(-18.0503403718914,29.9720317679544,124.064451745925)) ;
#67959=CARTESIAN_POINT('Ctrl Pts',(-18.3221216633801,29.7920426875915,123.933916272445)) ;
#67960=CARTESIAN_POINT('Ctrl Pts',(-17.9572951648542,29.9820855660479,123.817209301492)) ;
#67961=CARTESIAN_POINT('Ctrl Pts',(-18.2476869703767,29.802096485685,123.736121602035)) ;
#67962=CARTESIAN_POINT('Ctrl Pts',(-17.9093444927588,29.9919664868746,123.56198502385)) ;
#67963=CARTESIAN_POINT('Ctrl Pts',(-18.2093281437484,29.8119774065117,123.53194254377)) ;
#67964=CARTESIAN_POINT('Ctrl Pts',(-17.9059278138796,30.0019710128723,123.299129283876)) ;
#67965=CARTESIAN_POINT('Ctrl Pts',(-18.2065963307077,29.8219819325095,123.321658010208)) ;
#67966=CARTESIAN_POINT('Ctrl Pts',(-17.9482064112771,30.0119549764898,123.040145215749)) ;
#67967=CARTESIAN_POINT('Ctrl Pts',(-18.2404207028938,29.8319658961269,123.114471165854)) ;
#67968=CARTESIAN_POINT('Ctrl Pts',(-18.035508186737,30.0219946170411,122.791197498885)) ;
#67969=CARTESIAN_POINT('Ctrl Pts',(-18.3102636613557,29.8420055366782,122.915313421293)) ;
#67970=CARTESIAN_POINT('Ctrl Pts',(-18.161925212928,30.0318386426558,122.565497657734)) ;
#67971=CARTESIAN_POINT('Ctrl Pts',(-18.411398175043,29.8518495622929,122.734755088774)) ;
#67972=CARTESIAN_POINT('Ctrl Pts',(-18.3274685805744,30.0418296484732,122.361708399386)) ;
#67973=CARTESIAN_POINT('Ctrl Pts',(-18.5438338428557,29.8618405681103,122.571724671418)) ;
#67974=CARTESIAN_POINT('Ctrl Pts',(-18.5272036340267,30.0518674400053,122.189409573137)) ;
#67975=CARTESIAN_POINT('Ctrl Pts',(-18.7036229469901,29.8718783596425,122.433886677935)) ;
#67976=CARTESIAN_POINT('Ctrl Pts',(-18.749230903998,30.0617118397937,122.056613364073)) ;
#67977=CARTESIAN_POINT('Ctrl Pts',(-18.8812446799317,29.8817227594309,122.327651401076)) ;
#67978=CARTESIAN_POINT('Ctrl Pts',(-18.994164126273,30.0716966403505,121.962602178295)) ;
#67979=CARTESIAN_POINT('Ctrl Pts',(-19.0771915377067,29.8917075599876,122.252443739457)) ;
#67980=CARTESIAN_POINT('Ctrl Pts',(-19.2505801464928,30.0816361637616,121.912649736868)) ;
#67981=CARTESIAN_POINT('Ctrl Pts',(-19.2823241699332,29.9016470833988,122.212483121513)) ;
#67982=CARTESIAN_POINT('Ctrl Pts',(-19.5143516088782,30.0916758828626,121.907994125418)) ;
#67983=CARTESIAN_POINT('Ctrl Pts',(-19.4933414803542,29.9116868024998,122.208759920945)) ;
#67984=CARTESIAN_POINT('Ctrl Pts',(-19.7710473972636,30.1015640547819,121.948463714533)) ;
#67985=CARTESIAN_POINT('Ctrl Pts',(-19.6986971847122,29.921574974419,122.241136724367)) ;
#67986=CARTESIAN_POINT('Ctrl Pts',(-20.0194726827981,30.1115536171989,122.033282181041)) ;
#67987=CARTESIAN_POINT('Ctrl Pts',(-19.897436877706,29.931564536836,122.30899253618)) ;
#67988=CARTESIAN_POINT('Ctrl Pts',(-20.2485888048623,30.1215119893936,122.159725978258)) ;
#67989=CARTESIAN_POINT('Ctrl Pts',(-20.0807288910839,29.9415229090307,122.410148456545)) ;
#67990=CARTESIAN_POINT('Ctrl Pts',(-20.451481155513,30.1314120636243,122.322590700227)) ;
#67991=CARTESIAN_POINT('Ctrl Pts',(-20.2430415629541,29.9514229832614,122.540440622386)) ;
#67992=CARTESIAN_POINT('Ctrl Pts',(-20.6255019413428,30.1414581599979,122.521102011054)) ;
#67993=CARTESIAN_POINT('Ctrl Pts',(-20.3822574929672,29.961469079635,122.699250490915)) ;
#67994=CARTESIAN_POINT('Ctrl Pts',(-20.7605632740528,30.151366743995,122.743737177707)) ;
#67995=CARTESIAN_POINT('Ctrl Pts',(-20.4903053110624,29.9713776636321,122.877358615472)) ;
#67996=CARTESIAN_POINT('Ctrl Pts',(-20.8563375787038,30.1613773225859,122.988755129718)) ;
#67997=CARTESIAN_POINT('Ctrl Pts',(-20.5669238525766,29.981388242223,123.073373289288)) ;
#67998=CARTESIAN_POINT('Ctrl Pts',(-20.9076881587369,30.1714064806987,123.247269528944)) ;
#67999=CARTESIAN_POINT('Ctrl Pts',(-20.6080032779403,29.9914174003359,123.28018509895)) ;
#68000=CARTESIAN_POINT('Ctrl Pts',(-20.913643859901,30.1812593625368,123.506108579083)) ;
#68001=CARTESIAN_POINT('Ctrl Pts',(-20.6127668237937,30.0012702821739,123.4872553494)) ;
#68002=CARTESIAN_POINT('Ctrl Pts',(-20.8749374874299,30.1912189236878,123.764965708006)) ;
#68003=CARTESIAN_POINT('Ctrl Pts',(-20.5818009891085,30.0112298433249,123.694340561445)) ;
#68004=CARTESIAN_POINT('Ctrl Pts',(-20.7907663164554,30.2012573582769,124.014958246547)) ;
#68005=CARTESIAN_POINT('Ctrl Pts',(-20.5144631445051,30.021268277914,123.89433442643)) ;
#68006=CARTESIAN_POINT('Ctrl Pts',(-20.6669470046296,30.211130630504,124.243014320118)) ;
#68007=CARTESIAN_POINT('Ctrl Pts',(-20.4154074251945,30.0311415501411,124.07677811357)) ;
#68008=CARTESIAN_POINT('Ctrl Pts',(-20.5021342923516,30.2212038724976,124.450093173102)) ;
#68009=CARTESIAN_POINT('Ctrl Pts',(-20.2835564026306,30.0412147921347,124.242440954527)) ;
#68010=CARTESIAN_POINT('Ctrl Pts',(-20.3089888716899,30.2310242040306,124.621335698669)) ;
#68011=CARTESIAN_POINT('Ctrl Pts',(-20.1290405109537,30.0510351236678,124.379433600609)) ;
#68012=CARTESIAN_POINT('Ctrl Pts',(-20.0834917211719,30.2411028652574,124.760137415769)) ;
#68013=CARTESIAN_POINT('Ctrl Pts',(-19.9486421144359,30.0611137848945,124.49047459601)) ;
#68014=CARTESIAN_POINT('Ctrl Pts',(-19.8427824861803,30.2509544605516,124.855609977345)) ;
#68015=CARTESIAN_POINT('Ctrl Pts',(-19.7560754671688,30.0709653801888,124.566851648864)) ;
#68016=CARTESIAN_POINT('Ctrl Pts',(-19.5836045391597,30.2610275957804,124.909215904106)) ;
#68017=CARTESIAN_POINT('Ctrl Pts',(-19.5487326449223,30.0810385154176,124.609735875249)) ;
#68018=CARTESIAN_POINT('Ctrl Pts',(-19.3250420856673,30.2708700313055,124.916790254833)) ;
#68019=CARTESIAN_POINT('Ctrl Pts',(-19.3418837978834,30.0908809509426,124.615794714185)) ;
#68020=CARTESIAN_POINT('Ctrl Pts',(-19.0654078751379,30.2808508004389,124.879699535808)) ;
#68021=CARTESIAN_POINT('Ctrl Pts',(-19.1341767293187,30.100861720076,124.58612178724)) ;
#68022=CARTESIAN_POINT('Ctrl Pts',(-18.8153894691253,30.2908679016827,124.797325621791)) ;
#68023=CARTESIAN_POINT('Ctrl Pts',(-18.9341621618172,30.1108788213199,124.520222166044)) ;
#68024=CARTESIAN_POINT('Ctrl Pts',(-18.5862012535222,30.3007563492846,124.674812609811)) ;
#68025=CARTESIAN_POINT('Ctrl Pts',(-18.75081252989,30.1207672689217,124.422211818588)) ;
#68026=CARTESIAN_POINT('Ctrl Pts',(-18.378326748722,30.3108120634654,124.511700910524)) ;
#68027=CARTESIAN_POINT('Ctrl Pts',(-18.5845129649496,30.1308229831026,124.29172200353)) ;
#68028=CARTESIAN_POINT('Ctrl Pts',(-18.2050407985295,30.3206872698793,124.31849941652)) ;
#68029=CARTESIAN_POINT('Ctrl Pts',(-18.4458851060229,30.1406981895164,124.137161249517)) ;
#68030=CARTESIAN_POINT('Ctrl Pts',(-18.065746667546,30.330682322352,124.095826539079)) ;
#68031=CARTESIAN_POINT('Ctrl Pts',(-18.3344500579577,30.1506932419891,123.959022954298)) ;
#68032=CARTESIAN_POINT('Ctrl Pts',(-17.9673568014916,30.3407042063141,123.851520456621)) ;
#68033=CARTESIAN_POINT('Ctrl Pts',(-18.2557384543419,30.1607151259512,123.763577933142)) ;
#68034=CARTESIAN_POINT('Ctrl Pts',(-17.9132391133063,30.3506081788434,123.596944459868)) ;
#68035=CARTESIAN_POINT('Ctrl Pts',(-18.2124447103049,30.1706190984805,123.559917834642)) ;
#68036=CARTESIAN_POINT('Ctrl Pts',(-17.9036909635563,30.3605966755043,123.334628818861)) ;
#68037=CARTESIAN_POINT('Ctrl Pts',(-18.2048063513031,30.1806075951414,123.350065504462)) ;
#68038=CARTESIAN_POINT('Ctrl Pts',(-17.9399190541115,30.3705604727523,123.075322497842)) ;
#68039=CARTESIAN_POINT('Ctrl Pts',(-18.2337889737254,30.1905713923894,123.142620833117)) ;
#68040=CARTESIAN_POINT('Ctrl Pts',(-18.019542401481,30.3804644960603,122.827507706759)) ;
#68041=CARTESIAN_POINT('Ctrl Pts',(-18.2974874574404,30.2004754156974,122.944369728192)) ;
#68042=CARTESIAN_POINT('Ctrl Pts',(-18.1430719623568,30.3905249993819,122.593799613876)) ;
#68043=CARTESIAN_POINT('Ctrl Pts',(-18.3963113223776,30.2105359190191,122.757403048071)) ;
#68044=CARTESIAN_POINT('Ctrl Pts',(-18.3015384279696,30.4003655345218,122.38939813401)) ;
#68045=CARTESIAN_POINT('Ctrl Pts',(-18.5230837819883,30.2203764541589,122.593882800201)) ;
#68046=CARTESIAN_POINT('Ctrl Pts',(-18.4971286724099,30.4104277552264,122.211494771059)) ;
#68047=CARTESIAN_POINT('Ctrl Pts',(-18.6795561458151,30.2304386748635,122.451559855394)) ;
#68048=CARTESIAN_POINT('Ctrl Pts',(-18.7171521979687,30.4203249090026,122.072778646605)) ;
#68049=CARTESIAN_POINT('Ctrl Pts',(-18.8555742859337,30.2403358286398,122.340587380024)) ;
#68050=CARTESIAN_POINT('Ctrl Pts',(-18.9583979844501,30.4302560423881,121.973238309069)) ;
#68051=CARTESIAN_POINT('Ctrl Pts',(-19.0485702956595,30.2502669620252,122.260955120397)) ;
#68052=CARTESIAN_POINT('Ctrl Pts',(-19.216180617271,30.4402984175338,121.916755158295)) ;
#68053=CARTESIAN_POINT('Ctrl Pts',(-19.2547965323524,30.260309337171,122.215768415683)) ;
#68054=CARTESIAN_POINT('Ctrl Pts',(-19.4757597411927,30.4501843553,121.905857590778)) ;
#68055=CARTESIAN_POINT('Ctrl Pts',(-19.4624589536106,30.2701952749371,122.207050197027)) ;
#68056=CARTESIAN_POINT('Ctrl Pts',(-19.7361687240311,30.4601801982848,121.940170527014)) ;
#68057=CARTESIAN_POINT('Ctrl Pts',(-19.6707860227431,30.2801911179219,122.234500220989)) ;
#68058=CARTESIAN_POINT('Ctrl Pts',(-19.9853388632678,30.4701221761634,122.018791502423)) ;
#68059=CARTESIAN_POINT('Ctrl Pts',(-19.8701217511132,30.2901330958005,122.297396567724)) ;
#68060=CARTESIAN_POINT('Ctrl Pts',(-20.2176167858868,30.4800815506444,122.139363771227)) ;
#68061=CARTESIAN_POINT('Ctrl Pts',(-20.0559439306465,30.3000924702815,122.393853866718)) ;
#68062=CARTESIAN_POINT('Ctrl Pts',(-20.4263236161457,30.4900781664782,122.298948878856)) ;
#68063=CARTESIAN_POINT('Ctrl Pts',(-20.2229095545966,30.3100890861153,122.521521545282)) ;
#68064=CARTESIAN_POINT('Ctrl Pts',(-20.6045380695498,30.5001123850517,122.493286837832)) ;
#68065=CARTESIAN_POINT('Ctrl Pts',(-20.3654814345688,30.3201233046888,122.676991771903)) ;
#68066=CARTESIAN_POINT('Ctrl Pts',(-20.7440103711108,30.5099654522623,122.711437778196)) ;
#68067=CARTESIAN_POINT('Ctrl Pts',(-20.477059029593,30.3299763718994,122.851511380086)) ;
#68068=CARTESIAN_POINT('Ctrl Pts',(-20.8452704862501,30.5199257101399,122.952793072304)) ;
#68069=CARTESIAN_POINT('Ctrl Pts',(-20.5580675344423,30.339936629777,123.044595041422)) ;
#68070=CARTESIAN_POINT('Ctrl Pts',(-20.9031858777252,30.5299547368455,123.209917654151)) ;
#68071=CARTESIAN_POINT('Ctrl Pts',(-20.604400374506,30.3499656564826,123.250294668849)) ;
#68072=CARTESIAN_POINT('Ctrl Pts',(-20.9155052003231,30.5398649438799,123.470044892547)) ;
#68073=CARTESIAN_POINT('Ctrl Pts',(-20.6142563408965,30.3598758635171,123.458395733584)) ;
#68074=CARTESIAN_POINT('Ctrl Pts',(-20.8830672767706,30.5497998545275,123.729108750999)) ;
#68075=CARTESIAN_POINT('Ctrl Pts',(-20.5883067737471,30.3698107741647,123.665646384641)) ;
#68076=CARTESIAN_POINT('Ctrl Pts',(-20.8050869196827,30.5598409847068,123.981184304442)) ;
#68077=CARTESIAN_POINT('Ctrl Pts',(-20.5259230651749,30.3798519043439,123.867307162557)) ;
#68078=CARTESIAN_POINT('Ctrl Pts',(-20.6865234424483,30.5697281250767,124.212396007676)) ;
#68079=CARTESIAN_POINT('Ctrl Pts',(-20.4310732809217,30.3897390447139,124.052276102492)) ;
#68080=CARTESIAN_POINT('Ctrl Pts',(-20.5283158328247,30.5797204026127,124.421949250781)) ;
#68081=CARTESIAN_POINT('Ctrl Pts',(-20.3045079305415,30.3997313222498,124.219919049695)) ;
#68082=CARTESIAN_POINT('Ctrl Pts',(-20.336893127493,30.589668945881,124.600034325977)) ;
#68083=CARTESIAN_POINT('Ctrl Pts',(-20.1513706158548,30.4096798655181,124.362387386942)) ;
#68084=CARTESIAN_POINT('Ctrl Pts',(-20.117949669728,30.5996056206982,124.742302120517)) ;
#68085=CARTESIAN_POINT('Ctrl Pts',(-19.9762167528585,30.4196165403353,124.476202075347)) ;
#68086=CARTESIAN_POINT('Ctrl Pts',(-19.8765801266705,30.6095890416346,124.845182022236)) ;
#68087=CARTESIAN_POINT('Ctrl Pts',(-19.7831216739518,30.4295999612717,124.558506786004)) ;
#68088=CARTESIAN_POINT('Ctrl Pts',(-19.619448424608,30.6196313568238,124.904513792509)) ;
#68089=CARTESIAN_POINT('Ctrl Pts',(-19.577416370328,30.4396422764609,124.605973056573)) ;
#68090=CARTESIAN_POINT('Ctrl Pts',(-19.3612267210301,30.629471674263,124.918439915204)) ;
#68091=CARTESIAN_POINT('Ctrl Pts',(-19.3708401454886,30.4494825939001,124.617114839488)) ;
#68092=CARTESIAN_POINT('Ctrl Pts',(-19.0994956244019,30.6395013783205,124.887333257162)) ;
#68093=CARTESIAN_POINT('Ctrl Pts',(-19.1614550554373,30.4595122979576,124.592230579924)) ;
#68094=CARTESIAN_POINT('Ctrl Pts',(-18.84757050077,30.649522335043,124.810642476183)) ;
#68095=CARTESIAN_POINT('Ctrl Pts',(-18.9599146662731,30.4695332546801,124.530878830767)) ;
#68096=CARTESIAN_POINT('Ctrl Pts',(-18.6160882477537,30.6593888773466,124.69379526334)) ;
#68097=CARTESIAN_POINT('Ctrl Pts',(-18.7747291880007,30.4793997969837,124.437402426566)) ;
#68098=CARTESIAN_POINT('Ctrl Pts',(-18.4041389450964,30.6694599772918,124.535339469786)) ;
#68099=CARTESIAN_POINT('Ctrl Pts',(-18.6051688617141,30.4894708969289,124.310638472156)) ;
#68100=CARTESIAN_POINT('Ctrl Pts',(-18.2270241518516,30.6793020514693,124.346845255088)) ;
#68101=CARTESIAN_POINT('Ctrl Pts',(-18.4634769547701,30.4993129711065,124.159844592022)) ;
#68102=CARTESIAN_POINT('Ctrl Pts',(-18.0828214570917,30.6892628460564,124.128395071014)) ;
#68103=CARTESIAN_POINT('Ctrl Pts',(-18.3481139027231,30.5092737656935,123.98508542601)) ;
#68104=CARTESIAN_POINT('Ctrl Pts',(-17.9784145006715,30.6993007189572,123.886162207482)) ;
#68105=CARTESIAN_POINT('Ctrl Pts',(-18.2645872182837,30.5193116385943,123.791299501671)) ;
#68106=CARTESIAN_POINT('Ctrl Pts',(-17.9181661940265,30.7091750045013,123.63373426702)) ;
#68107=CARTESIAN_POINT('Ctrl Pts',(-18.216387518212,30.5291859241384,123.589358233217)) ;
#68108=CARTESIAN_POINT('Ctrl Pts',(-17.9023753757216,30.7192447549152,123.369619175597)) ;
#68109=CARTESIAN_POINT('Ctrl Pts',(-18.203753574066,30.5392556745523,123.378065957705)) ;
#68110=CARTESIAN_POINT('Ctrl Pts',(-17.9318397718058,30.7290780394499,123.112874144442)) ;
#68111=CARTESIAN_POINT('Ctrl Pts',(-18.2273236794525,30.549088959087,123.172670800708)) ;
#68112=CARTESIAN_POINT('Ctrl Pts',(-18.0061852690051,30.7391083802499,122.859997359419)) ;
#68113=CARTESIAN_POINT('Ctrl Pts',(-18.2867986965905,30.559119299887,122.970368894539)) ;
#68114=CARTESIAN_POINT('Ctrl Pts',(-18.1240293775023,30.7491403042495,122.624160309324)) ;
#68115=CARTESIAN_POINT('Ctrl Pts',(-18.381072852259,30.5691512238866,122.781698614195)) ;
#68116=CARTESIAN_POINT('Ctrl Pts',(-18.2773844645063,30.7589688391854,122.416346355351)) ;
#68117=CARTESIAN_POINT('Ctrl Pts',(-18.5037551769327,30.5789797588226,122.615447430621)) ;
#68118=CARTESIAN_POINT('Ctrl Pts',(-18.4671493140597,30.7689626169501,122.234795344671)) ;
#68119=CARTESIAN_POINT('Ctrl Pts',(-18.6555658924433,30.5889735365872,122.470205578814)) ;
#68120=CARTESIAN_POINT('Ctrl Pts',(-18.6865926220814,30.7789903274356,122.088882738916)) ;
#68121=CARTESIAN_POINT('Ctrl Pts',(-18.8311197585545,30.5990012470728,122.353474263841)) ;
#68122=CARTESIAN_POINT('Ctrl Pts',(-18.924548918543,30.7888787382696,121.984461740876)) ;
#68123=CARTESIAN_POINT('Ctrl Pts',(-19.0214835756871,30.6088896579067,122.269936340011)) ;
#68124=CARTESIAN_POINT('Ctrl Pts',(-19.1791493957345,30.7988555888051,121.921954029357)) ;
#68125=CARTESIAN_POINT('Ctrl Pts',(-19.2251633755617,30.6188665084423,122.219928660186)) ;
#68126=CARTESIAN_POINT('Ctrl Pts',(-19.4411836962534,30.8088473853556,121.904551040875)) ;
#68127=CARTESIAN_POINT('Ctrl Pts',(-19.4347905867356,30.6288583049927,122.206004671625)) ;
#68128=CARTESIAN_POINT('Ctrl Pts',(-19.7033209422536,30.8188833914493,121.933349289194)) ;
#68129=CARTESIAN_POINT('Ctrl Pts',(-19.6445006241245,30.6388943110864,122.229041739031)) ;
#68130=CARTESIAN_POINT('Ctrl Pts',(-19.9519531581678,30.8287341257121,122.005489324719)) ;
#68131=CARTESIAN_POINT('Ctrl Pts',(-19.84340606214,30.6487450453492,122.286751981054)) ;
#68132=CARTESIAN_POINT('Ctrl Pts',(-20.1877451626918,30.8387253842403,122.12090221111)) ;
#68133=CARTESIAN_POINT('Ctrl Pts',(-20.0320402961377,30.6587363038774,122.379080697725)) ;
#68134=CARTESIAN_POINT('Ctrl Pts',(-20.3985067246429,30.8486432791435,122.274284311981)) ;
#68135=CARTESIAN_POINT('Ctrl Pts',(-20.2006501933195,30.6686541987806,122.50178471108)) ;
#68136=CARTESIAN_POINT('Ctrl Pts',(-20.5814557895788,30.8586714208065,122.463931047394)) ;
#68137=CARTESIAN_POINT('Ctrl Pts',(-20.3470107187746,30.6786823404437,122.653500909386)) ;
#68138=CARTESIAN_POINT('Ctrl Pts',(-20.726703975958,30.8685565889224,122.679309656422)) ;
#68139=CARTESIAN_POINT('Ctrl Pts',(-20.4632103980333,30.6885675085595,122.82580232508)) ;
#68140=CARTESIAN_POINT('Ctrl Pts',(-20.8340446604117,30.8785459524284,122.918876333056)) ;
#68141=CARTESIAN_POINT('Ctrl Pts',(-20.5490845941834,30.6985568720655,123.017454790216)) ;
#68142=CARTESIAN_POINT('Ctrl Pts',(-20.8979488651774,30.8885870874385,123.174891648262)) ;
#68143=CARTESIAN_POINT('Ctrl Pts',(-20.6002096966955,30.7085980070756,123.222266683441)) ;
#68144=CARTESIAN_POINT('Ctrl Pts',(-20.916470523059,30.8984197556265,123.432614768819)) ;
#68145=CARTESIAN_POINT('Ctrl Pts',(-20.6150288055355,30.7184306752636,123.42844428619)) ;
#68146=CARTESIAN_POINT('Ctrl Pts',(-20.8902751541959,30.908413658581,123.693933046635)) ;
#68147=CARTESIAN_POINT('Ctrl Pts',(-20.5940744640968,30.7284245782181,123.637499006698)) ;
#68148=CARTESIAN_POINT('Ctrl Pts',(-20.8183135578191,30.9184429436655,123.947479863912)) ;
#68149=CARTESIAN_POINT('Ctrl Pts',(-20.5365069824791,30.7384538633026,123.840336987593)) ;
#68150=CARTESIAN_POINT('Ctrl Pts',(-20.705558307434,30.9283184721074,124.181239071671)) ;
#68151=CARTESIAN_POINT('Ctrl Pts',(-20.4463047552757,30.7483293917445,124.027344708354)) ;
#68152=CARTESIAN_POINT('Ctrl Pts',(-20.55227636311,30.9383187547235,124.394663488926)) ;
#68153=CARTESIAN_POINT('Ctrl Pts',(-20.3236808563954,30.7583296743606,124.198085320578)) ;
#68154=CARTESIAN_POINT('Ctrl Pts',(-20.3660263502005,30.9482307707805,124.576805636963)) ;
#68155=CARTESIAN_POINT('Ctrl Pts',(-20.1746825091219,30.7682416904176,124.343800207381)) ;
#68156=CARTESIAN_POINT('Ctrl Pts',(-20.148238159027,30.9582728461195,124.725798531691)) ;
#68157=CARTESIAN_POINT('Ctrl Pts',(-20.0004530415488,30.7782837657566,124.462996211481)) ;
#68158=CARTESIAN_POINT('Ctrl Pts',(-19.9112599341149,30.9681726787756,124.833177229003)) ;
#68159=CARTESIAN_POINT('Ctrl Pts',(-19.8108716507074,30.7881835984127,124.548900832387)) ;
#68160=CARTESIAN_POINT('Ctrl Pts',(-19.6570385216495,30.9781650793536,124.898943043692)) ;
#68161=CARTESIAN_POINT('Ctrl Pts',(-19.6074951324964,30.7981759989908,124.601515467701)) ;
#68162=CARTESIAN_POINT('Ctrl Pts',(-19.3941289164041,30.988199101113,124.91918719167)) ;
#68163=CARTESIAN_POINT('Ctrl Pts',(-19.3971675920454,30.8082100207501,124.617712800097)) ;
#68164=CARTESIAN_POINT('Ctrl Pts',(-19.1361050769742,30.9980637119542,124.894240456014)) ;
#68165=CARTESIAN_POINT('Ctrl Pts',(-19.1907487911247,30.8180746315913,124.597757506025)) ;
#68166=CARTESIAN_POINT('Ctrl Pts',(-18.8829168166101,31.0080561114154,124.824588928341)) ;
#68167=CARTESIAN_POINT('Ctrl Pts',(-18.9881977022827,30.8280670310525,124.542038356411)) ;
#68168=CARTESIAN_POINT('Ctrl Pts',(-18.6449556256928,31.0180880647483,124.711122383822)) ;
#68169=CARTESIAN_POINT('Ctrl Pts',(-18.7978278575721,30.8380989843854,124.451266991065)) ;
#68170=CARTESIAN_POINT('Ctrl Pts',(-18.433613598993,31.0279544236899,124.56090527812)) ;
#68171=CARTESIAN_POINT('Ctrl Pts',(-18.6287533485745,30.8479653433271,124.331095266806)) ;
#68172=CARTESIAN_POINT('Ctrl Pts',(-18.2490556295149,31.0379418991757,124.374338785496)) ;
#68173=CARTESIAN_POINT('Ctrl Pts',(-18.4811055111565,30.8579528188129,124.181843656717)) ;
#68174=CARTESIAN_POINT('Ctrl Pts',(-18.1001763827017,31.0478868053642,124.159502137119)) ;
#68175=CARTESIAN_POINT('Ctrl Pts',(-18.3620004446378,30.8678977250013,124.009975722139)) ;
#68176=CARTESIAN_POINT('Ctrl Pts',(-17.9899251037199,31.0579317700244,123.919685682728)) ;
#68177=CARTESIAN_POINT('Ctrl Pts',(-18.2737974607781,30.8779426896616,123.818123443375)) ;
#68178=CARTESIAN_POINT('Ctrl Pts',(-17.9239698947395,31.0677935769293,123.669038395262)) ;
#68179=CARTESIAN_POINT('Ctrl Pts',(-18.221031284142,30.8878044965664,123.617606494588)) ;
#68180=CARTESIAN_POINT('Ctrl Pts',(-17.9017545884407,31.0777862492351,123.407409964502)) ;
#68181=CARTESIAN_POINT('Ctrl Pts',(-18.2032568478911,30.8977971688722,123.408304011957)) ;
#68182=CARTESIAN_POINT('Ctrl Pts',(-17.9251878868137,31.0877149201804,123.147532162219)) ;
#68183=CARTESIAN_POINT('Ctrl Pts',(-18.2220012797528,30.9077258398175,123.200401751263)) ;
#68184=CARTESIAN_POINT('Ctrl Pts',(-17.9931295756622,31.0976674624057,122.894987346514)) ;
#68185=CARTESIAN_POINT('Ctrl Pts',(-18.2763524482962,30.9176783820428,122.998365442682)) ;
#68186=CARTESIAN_POINT('Ctrl Pts',(-18.1043255909368,31.1076688184016,122.656813330348)) ;
#68187=CARTESIAN_POINT('Ctrl Pts',(-18.3653072153254,30.9276797380387,122.807825340817)) ;
#68188=CARTESIAN_POINT('Ctrl Pts',(-18.2558710625769,31.1176974306763,122.441217023634)) ;
#68189=CARTESIAN_POINT('Ctrl Pts',(-18.486541760213,30.9377083503134,122.63534705266)) ;
#68190=CARTESIAN_POINT('Ctrl Pts',(-18.4392436560099,31.1275617652258,122.257966085798)) ;
#68191=CARTESIAN_POINT('Ctrl Pts',(-18.6332381127442,30.9475726848629,122.488744871235)) ;
#68192=CARTESIAN_POINT('Ctrl Pts',(-18.6541277020736,31.1375540893024,122.107106052772)) ;
#68193=CARTESIAN_POINT('Ctrl Pts',(-18.805144006808,30.9575650089395,122.368055041523)) ;
#68194=CARTESIAN_POINT('Ctrl Pts',(-18.8903979931826,31.1474815816683,121.99639777191)) ;
#68195=CARTESIAN_POINT('Ctrl Pts',(-18.9941591920697,30.9674925013054,122.279486427225)) ;
#68196=CARTESIAN_POINT('Ctrl Pts',(-19.1447705223875,31.1575089402191,121.927739862365)) ;
#68197=CARTESIAN_POINT('Ctrl Pts',(-19.1976565800842,30.9775198598562,122.224557940461)) ;
#68198=CARTESIAN_POINT('Ctrl Pts',(-19.403557785468,31.1673953582702,121.904339822956)) ;
#68199=CARTESIAN_POINT('Ctrl Pts',(-19.40468609459,30.9874062779074,122.205835676203)) ;
#68200=CARTESIAN_POINT('Ctrl Pts',(-19.6662117593913,31.1774270930056,121.926411212978)) ;
#68201=CARTESIAN_POINT('Ctrl Pts',(-19.6148094082564,30.9974380126427,122.223490535075)) ;
#68202=CARTESIAN_POINT('Ctrl Pts',(-19.9173816828502,31.1873086742489,121.992520931665)) ;
#68203=CARTESIAN_POINT('Ctrl Pts',(-19.815745871323,31.007319593886,122.276376119868)) ;
#68204=CARTESIAN_POINT('Ctrl Pts',(-20.1575099536661,31.1973706522812,122.103127502672)) ;
#68205=CARTESIAN_POINT('Ctrl Pts',(-20.0078493692217,31.0173815719183,122.364859298836)) ;
#68206=CARTESIAN_POINT('Ctrl Pts',(-20.3704779128565,31.2072277306429,122.250647114545)) ;
#68207=CARTESIAN_POINT('Ctrl Pts',(-20.1782250129861,31.02723865028,122.482873132973)) ;
#68208=CARTESIAN_POINT('Ctrl Pts',(-20.557479635411,31.2172223037489,122.435014859895)) ;
#68209=CARTESIAN_POINT('Ctrl Pts',(-20.3278279402508,31.037233223386,122.630365704853)) ;
#68210=CARTESIAN_POINT('Ctrl Pts',(-20.7087042530508,31.2271481000365,122.647587798087)) ;
#68211=CARTESIAN_POINT('Ctrl Pts',(-20.4488094657624,31.0471590196736,122.8004227559)) ;
#68212=CARTESIAN_POINT('Ctrl Pts',(-20.8218837391766,31.2371734672062,122.885470873075)) ;
#68213=CARTESIAN_POINT('Ctrl Pts',(-20.539355037212,31.0571843868434,122.99072823021)) ;
#68214=CARTESIAN_POINT('Ctrl Pts',(-20.8912500206041,31.2470695468601,123.136118325641)) ;
#68215=CARTESIAN_POINT('Ctrl Pts',(-20.594850255258,31.0670804664972,123.191245492355)) ;
#68216=CARTESIAN_POINT('Ctrl Pts',(-20.916817797818,31.2570646265657,123.397534145115)) ;
#68217=CARTESIAN_POINT('Ctrl Pts',(-20.6153065879517,31.0770755462028,123.400378543151)) ;
#68218=CARTESIAN_POINT('Ctrl Pts',(-20.8960973227342,31.2670897143815,123.660166672547)) ;
#68219=CARTESIAN_POINT('Ctrl Pts',(-20.5987327498281,31.0871006340186,123.610482259063)) ;
#68220=CARTESIAN_POINT('Ctrl Pts',(-20.809893476644,31.2802735367488,123.995726533553)) ;
#68221=CARTESIAN_POINT('Ctrl Pts',(-20.5297709305419,31.1002844563859,123.87894293253)) ;
#68222=CARTESIAN_POINT('Ctrl Pts',(-20.6369390480152,31.2935956548947,124.30466223955)) ;
#68223=CARTESIAN_POINT('Ctrl Pts',(-20.3913865526123,31.1136065745318,124.126114241275)) ;
#68224=CARTESIAN_POINT('Ctrl Pts',(-20.3908148582284,31.3069748645223,124.555818133117)) ;
#68225=CARTESIAN_POINT('Ctrl Pts',(-20.1945187656795,31.1269857841594,124.327003669048)) ;
#68226=CARTESIAN_POINT('Ctrl Pts',(-20.1809438414753,31.3168131017665,124.706820601801)) ;
#68227=CARTESIAN_POINT('Ctrl Pts',(-20.0266169655379,31.1368240214036,124.447815030813)) ;
#68228=CARTESIAN_POINT('Ctrl Pts',(-19.9425721439745,31.3268860250252,124.821852782534)) ;
#68229=CARTESIAN_POINT('Ctrl Pts',(-19.8359226633174,31.1468969446624,124.539840740485)) ;
#68230=CARTESIAN_POINT('Ctrl Pts',(-19.6932575438715,31.3367426664803,124.89218888602)) ;
#68231=CARTESIAN_POINT('Ctrl Pts',(-19.6364695236485,31.1567535861175,124.596111832383)) ;
#68232=CARTESIAN_POINT('Ctrl Pts',(-19.4322556852193,31.3467280419864,124.919201640466)) ;
#68233=CARTESIAN_POINT('Ctrl Pts',(-19.4276731793723,31.1667389616235,124.617725775355)) ;
#68234=CARTESIAN_POINT('Ctrl Pts',(-19.0841345592013,31.3600120734468,124.893999424143)) ;
#68235=CARTESIAN_POINT('Ctrl Pts',(-19.1491518620383,31.180022993084,124.597557799836)) ;
#68236=CARTESIAN_POINT('Ctrl Pts',(-18.6686831095259,31.3765308653172,124.751522351196)) ;
#68237=CARTESIAN_POINT('Ctrl Pts',(-18.8168267270378,31.1965417849543,124.483599784169)) ;
#68238=CARTESIAN_POINT('Ctrl Pts',(-18.3221176258635,31.3933165823238,124.470780414967)) ;
#68239=CARTESIAN_POINT('Ctrl Pts',(-18.5395236640967,31.2133275019609,124.258964588696)) ;
#68240=CARTESIAN_POINT('Ctrl Pts',(-18.1195171640873,31.4064297308328,124.19192546978)) ;
#68241=CARTESIAN_POINT('Ctrl Pts',(-18.3774781924197,31.2264406504699,124.035919165873)) ;
#68242=CARTESIAN_POINT('Ctrl Pts',(-18.0029767278721,31.416465279913,123.955390640417)) ;
#68243=CARTESIAN_POINT('Ctrl Pts',(-18.2842367998029,31.2364761995501,123.846683979849)) ;
#68244=CARTESIAN_POINT('Ctrl Pts',(-17.930131161295,31.4264813360924,123.702427282653)) ;
#68245=CARTESIAN_POINT('Ctrl Pts',(-18.2259601153952,31.2464922557295,123.644318871564)) ;
#68246=CARTESIAN_POINT('Ctrl Pts',(-17.8927981854828,31.4396593719584,123.358188928687)) ;
#68247=CARTESIAN_POINT('Ctrl Pts',(-18.1960923899022,31.2596702915955,123.368912638922)) ;
#68248=CARTESIAN_POINT('Ctrl Pts',(-17.9589427761027,31.4562612491455,122.921846253614)) ;
#68249=CARTESIAN_POINT('Ctrl Pts',(-18.2490034305915,31.2762721687826,123.019854359994)) ;
#68250=CARTESIAN_POINT('Ctrl Pts',(-18.2153452936868,31.4763243937614,122.454312103361)) ;
#68251=CARTESIAN_POINT('Ctrl Pts',(-18.4541225899952,31.2963353133985,122.645820297505)) ;
#68252=CARTESIAN_POINT('Ctrl Pts',(-18.6105119795525,31.4961252838451,122.106643007625)) ;
#68253=CARTESIAN_POINT('Ctrl Pts',(-18.7702543020853,31.3161362034822,122.36768303858)) ;
#68254=CARTESIAN_POINT('Ctrl Pts',(-19.1034924936999,31.5160684091238,121.912133008607)) ;
#68255=CARTESIAN_POINT('Ctrl Pts',(-19.164637971874,31.3360793287609,122.212071605184)) ;
#68256=CARTESIAN_POINT('Ctrl Pts',(-19.6321465341764,31.5359664542434,121.89791137193)) ;
#68257=CARTESIAN_POINT('Ctrl Pts',(-19.5875618065476,31.3559773738805,122.200691277358)) ;
#68258=CARTESIAN_POINT('Ctrl Pts',(-20.1341066883384,31.5558522138702,122.063616102464)) ;
#68259=CARTESIAN_POINT('Ctrl Pts',(-19.9891315918773,31.3758631335073,122.333252851735)) ;
#68260=CARTESIAN_POINT('Ctrl Pts',(-20.5525283110554,31.57591738905,122.394200252169)) ;
#68261=CARTESIAN_POINT('Ctrl Pts',(-20.3238701259959,31.3959283086872,122.597717694145)) ;
#68262=CARTESIAN_POINT('Ctrl Pts',(-20.8296000415882,31.5957440321528,122.84254361497)) ;
#68263=CARTESIAN_POINT('Ctrl Pts',(-20.5455305086285,31.41575495179,122.95639217086)) ;
#68264=CARTESIAN_POINT('Ctrl Pts',(-20.9388687495492,31.6156527416012,123.360136077141)) ;
#68265=CARTESIAN_POINT('Ctrl Pts',(-20.6329476561718,31.4356636612383,123.370466593898)) ;
#68266=CARTESIAN_POINT('Ctrl Pts',(-20.8648791195812,31.635604578633,123.885385533411)) ;
#68267=CARTESIAN_POINT('Ctrl Pts',(-20.573757693884,31.4556154982701,123.790666808917)) ;
#68268=CARTESIAN_POINT('Ctrl Pts',(-20.6147262487971,31.6556130533361,124.354604940983)) ;
#68269=CARTESIAN_POINT('Ctrl Pts',(-20.3736372170781,31.4756239729733,124.166043186308)) ;
#68270=CARTESIAN_POINT('Ctrl Pts',(-20.2239265792252,31.6754145120976,124.70712499995)) ;
#68271=CARTESIAN_POINT('Ctrl Pts',(-20.0609969972757,31.4954254317348,124.448061814946)) ;
#68272=CARTESIAN_POINT('Ctrl Pts',(-19.7329944592127,31.6953714003336,124.907950846951)) ;
#68273=CARTESIAN_POINT('Ctrl Pts',(-19.6682511534378,31.5153823199707,124.608723469387)) ;
#68274=CARTESIAN_POINT('Ctrl Pts',(-19.2022559885623,31.7153552377477,124.928017723692)) ;
#68275=CARTESIAN_POINT('Ctrl Pts',(-19.2436602612597,31.5353661573848,124.624778160052)) ;
#68276=CARTESIAN_POINT('Ctrl Pts',(-18.7005580952729,31.7351636769686,124.768181953029)) ;
#68277=CARTESIAN_POINT('Ctrl Pts',(-18.8422995577168,31.5551745966057,124.496909315192)) ;
#68278=CARTESIAN_POINT('Ctrl Pts',(-18.2796327533169,31.7551493863488,124.444432947283)) ;
#68279=CARTESIAN_POINT('Ctrl Pts',(-18.505559042595,31.5751603059859,124.237909991823)) ;
#68280=CARTESIAN_POINT('Ctrl Pts',(-17.9957625956122,31.7750189093641,123.998861683797)) ;
#68281=CARTESIAN_POINT('Ctrl Pts',(-18.2784622930544,31.5950298290012,123.881451524151)) ;
#68282=CARTESIAN_POINT('Ctrl Pts',(-17.8804111930879,31.7950396484813,123.479601508631)) ;
#68283=CARTESIAN_POINT('Ctrl Pts',(-18.1861815644187,31.6150505681184,123.466043484708)) ;
#68284=CARTESIAN_POINT('Ctrl Pts',(-17.947813732566,31.8148437134583,122.957375358431)) ;
#68285=CARTESIAN_POINT('Ctrl Pts',(-18.240104726759,31.6348546330954,123.048260409413)) ;
#68286=CARTESIAN_POINT('Ctrl Pts',(-18.1922019497661,31.834905677189,122.483631625261)) ;
#68287=CARTESIAN_POINT('Ctrl Pts',(-18.4356159960294,31.6549165968261,122.669266566499)) ;
#68288=CARTESIAN_POINT('Ctrl Pts',(-18.579670503548,31.8547388574775,122.126047237428)) ;
#68289=CARTESIAN_POINT('Ctrl Pts',(-18.7455928985157,31.6747497771146,122.383198612062)) ;
#68290=CARTESIAN_POINT('Ctrl Pts',(-19.0672415407129,31.8746580548036,121.919977102834)) ;
#68291=CARTESIAN_POINT('Ctrl Pts',(-19.1356512341748,31.6946689744407,122.218343904972)) ;
#68292=CARTESIAN_POINT('Ctrl Pts',(-19.596473798273,31.8945960799169,121.892968380712)) ;
#68293=CARTESIAN_POINT('Ctrl Pts',(-19.559037724007,31.714606999554,122.196738778409)) ;
#68294=CARTESIAN_POINT('Ctrl Pts',(-20.1018977424829,31.914474125973,122.047010861552)) ;
#68295=CARTESIAN_POINT('Ctrl Pts',(-19.9633772292207,31.7344850456101,122.319975266152)) ;
#68296=CARTESIAN_POINT('Ctrl Pts',(-20.5266155989396,31.934458860261,122.365876034326)) ;
#68297=CARTESIAN_POINT('Ctrl Pts',(-20.3031501256687,31.7544697798982,122.575069435507)) ;
#68298=CARTESIAN_POINT('Ctrl Pts',(-20.8161540516341,31.9543696769395,122.809022005469)) ;
#68299=CARTESIAN_POINT('Ctrl Pts',(-20.5347790794781,31.7743805965766,122.92958819007)) ;
#68300=CARTESIAN_POINT('Ctrl Pts',(-20.9372264313366,31.9743686524582,123.326459903439)) ;
#68301=CARTESIAN_POINT('Ctrl Pts',(-20.6316344224308,31.7943795720954,123.343539156427)) ;
#68302=CARTESIAN_POINT('Ctrl Pts',(-20.8757007542274,31.9941735731034,123.849340834267)) ;
#68303=CARTESIAN_POINT('Ctrl Pts',(-20.5824107852335,31.8141844927406,123.761844941543)) ;
#68304=CARTESIAN_POINT('Ctrl Pts',(-20.6381061492539,32.0141575333947,124.324236585198)) ;
#68305=CARTESIAN_POINT('Ctrl Pts',(-20.3923321320177,31.8341684530318,124.141760152678)) ;
#68306=CARTESIAN_POINT('Ctrl Pts',(-20.254277484515,32.0340437371186,124.687750970673)) ;
#68307=CARTESIAN_POINT('Ctrl Pts',(-20.085266409861,31.8540546567557,124.432569686706)) ;
#68308=CARTESIAN_POINT('Ctrl Pts',(-19.7682819396191,32.0539929154418,124.89962239012)) ;
#68309=CARTESIAN_POINT('Ctrl Pts',(-19.696468384716,31.8740038350789,124.60206379762)) ;
#68310=CARTESIAN_POINT('Ctrl Pts',(-19.2403770539516,32.0738947146813,124.932732853793)) ;
#68311=CARTESIAN_POINT('Ctrl Pts',(-19.2741434998259,31.8939056343185,124.628548078608)) ;
#68312=CARTESIAN_POINT('Ctrl Pts',(-18.7330993587673,32.0937733197337,124.784941725984)) ;
#68313=CARTESIAN_POINT('Ctrl Pts',(-18.868322906955,31.9137842393708,124.510313181707)) ;
#68314=CARTESIAN_POINT('Ctrl Pts',(-18.3035498467669,32.1138056794594,124.470304693559)) ;
#68315=CARTESIAN_POINT('Ctrl Pts',(-18.5246822315973,31.9338165990965,124.258593399843)) ;
#68316=CARTESIAN_POINT('Ctrl Pts',(-18.0587930611329,32.1303874054155,124.103782576889)) ;
#68317=CARTESIAN_POINT('Ctrl Pts',(-18.3288903810443,31.9503983250526,123.965395758089)) ;
#68318=CARTESIAN_POINT('Ctrl Pts',(-17.9464384610694,32.1435815757134,123.775785395635)) ;
#68319=CARTESIAN_POINT('Ctrl Pts',(-18.2389994529127,31.9635924953505,123.702969740174)) ;
#68320=CARTESIAN_POINT('Ctrl Pts',(-17.8916962164165,32.1568937538066,123.430264324837)) ;
#68321=CARTESIAN_POINT('Ctrl Pts',(-18.1952099799321,31.9769046734437,123.426608864667)) ;
#68322=CARTESIAN_POINT('Ctrl Pts',(-17.9374894753685,32.1734599333999,122.99232521224)) ;
#68323=CARTESIAN_POINT('Ctrl Pts',(-18.2318514252023,31.9934708530371,123.076188915836)) ;
#68324=CARTESIAN_POINT('Ctrl Pts',(-18.1302718088824,32.1900881282601,122.594703559392)) ;
#68325=CARTESIAN_POINT('Ctrl Pts',(-18.3860665483606,32.0100990478972,122.758138239794)) ;
#68326=CARTESIAN_POINT('Ctrl Pts',(-18.3588141057148,32.2033767099699,122.330591540781)) ;
#68327=CARTESIAN_POINT('Ctrl Pts',(-18.5689151874287,32.023387629607,122.546823962737)) ;
#68328=CARTESIAN_POINT('Ctrl Pts',(-18.5618539277949,32.2133449580735,122.165112713871)) ;
#68329=CARTESIAN_POINT('Ctrl Pts',(-18.7313457221629,32.0333558777106,122.414447852175)) ;
#68330=CARTESIAN_POINT('Ctrl Pts',(-18.7891790717996,32.2232597143296,122.037790376024)) ;
#68331=CARTESIAN_POINT('Ctrl Pts',(-18.9132084602232,32.0432706339667,122.312590559703)) ;
#68332=CARTESIAN_POINT('Ctrl Pts',(-19.037513591275,32.2332728649808,121.95074327932)) ;
#68333=CARTESIAN_POINT('Ctrl Pts',(-19.1118736703297,32.0532837846179,122.242954838167)) ;
#68334=CARTESIAN_POINT('Ctrl Pts',(-19.2972230251791,32.2432855721828,121.908553873528)) ;
#68335=CARTESIAN_POINT('Ctrl Pts',(-19.3196523089538,32.0632964918199,122.209207408094)) ;
#68336=CARTESIAN_POINT('Ctrl Pts',(-19.6446403660395,32.2565048608741,121.9125795524)) ;
#68337=CARTESIAN_POINT('Ctrl Pts',(-19.5975327596128,32.0765157805112,122.212420869537)) ;
#68338=CARTESIAN_POINT('Ctrl Pts',(-20.0699198327109,32.2731235418722,122.031411460383)) ;
#68339=CARTESIAN_POINT('Ctrl Pts',(-19.937823277613,32.0931344615093,122.307507212326)) ;
#68340=CARTESIAN_POINT('Ctrl Pts',(-20.4284615240151,32.2896884496456,122.28707638829)) ;
#68341=CARTESIAN_POINT('Ctrl Pts',(-20.224607600475,32.1096993692827,122.512015776509)) ;
#68342=CARTESIAN_POINT('Ctrl Pts',(-20.6522321703216,32.3030869212564,122.55890721292)) ;
#68343=CARTESIAN_POINT('Ctrl Pts',(-20.4036500863331,32.1230978408936,122.729503326657)) ;
#68344=CARTESIAN_POINT('Ctrl Pts',(-20.7796679108865,32.3129281767434,122.783972393412)) ;
#68345=CARTESIAN_POINT('Ctrl Pts',(-20.5055910403937,32.1329390963805,122.909552376083)) ;
#68346=CARTESIAN_POINT('Ctrl Pts',(-20.8678841148157,32.3229144923316,123.031085830974)) ;
#68347=CARTESIAN_POINT('Ctrl Pts',(-20.576163376053,32.1429254119687,123.107244959995)) ;
#68348=CARTESIAN_POINT('Ctrl Pts',(-20.9117732133019,32.332851099918,123.288538866815)) ;
#68349=CARTESIAN_POINT('Ctrl Pts',(-20.6112720124456,32.1528620195551,123.313207406856)) ;
#68350=CARTESIAN_POINT('Ctrl Pts',(-20.910145815352,32.3429009672863,123.552606824038)) ;
#68351=CARTESIAN_POINT('Ctrl Pts',(-20.6099679432151,32.1629118869234,123.524461792942)) ;
#68352=CARTESIAN_POINT('Ctrl Pts',(-20.8638163142715,32.3527514619611,123.807307622436)) ;
#68353=CARTESIAN_POINT('Ctrl Pts',(-20.5729021084178,32.1727623815982,123.72822191254)) ;
#68354=CARTESIAN_POINT('Ctrl Pts',(-20.773519983493,32.3627232623556,124.053271401024)) ;
#68355=CARTESIAN_POINT('Ctrl Pts',(-20.5006629717372,32.1827341819927,123.924992078725)) ;
#68356=CARTESIAN_POINT('Ctrl Pts',(-20.6415042015941,32.3727192293814,124.280422776241)) ;
#68357=CARTESIAN_POINT('Ctrl Pts',(-20.3950484362192,32.1927301490186,124.106711993813)) ;
#68358=CARTESIAN_POINT('Ctrl Pts',(-20.4711197706811,32.3827566887626,124.481749462152)) ;
#68359=CARTESIAN_POINT('Ctrl Pts',(-20.2587391854302,32.2027676083997,124.267771863989)) ;
#68360=CARTESIAN_POINT('Ctrl Pts',(-20.2726207381904,32.3925973896634,124.6475312724)) ;
#68361=CARTESIAN_POINT('Ctrl Pts',(-20.0999386785007,32.2126083093005,124.400395461972)) ;
#68362=CARTESIAN_POINT('Ctrl Pts',(-20.0438481628859,32.4026454109307,124.779365277945)) ;
#68363=CARTESIAN_POINT('Ctrl Pts',(-19.9169195251314,32.2226563305678,124.50586072606)) ;
#68364=CARTESIAN_POINT('Ctrl Pts',(-19.7979892008617,32.4125928040134,124.868183348147)) ;
#68365=CARTESIAN_POINT('Ctrl Pts',(-19.7202316993048,32.2326037236505,124.576913031386)) ;
#68366=CARTESIAN_POINT('Ctrl Pts',(-19.5415342218403,32.4225029500598,124.913581797367)) ;
#68367=CARTESIAN_POINT('Ctrl Pts',(-19.515067529213,32.2425138696969,124.613229582587)) ;
#68368=CARTESIAN_POINT('Ctrl Pts',(-19.277223918375,32.4325618639094,124.913465271175)) ;
#68369=CARTESIAN_POINT('Ctrl Pts',(-19.3036192607228,32.2525727835465,124.613134137926)) ;
#68370=CARTESIAN_POINT('Ctrl Pts',(-19.022469311543,32.4424026341987,124.868802452506)) ;
#68371=CARTESIAN_POINT('Ctrl Pts',(-19.099816280715,32.2624135538358,124.577401773527)) ;
#68372=CARTESIAN_POINT('Ctrl Pts',(-18.7738114256327,32.4524655037773,124.778908029314)) ;
#68373=CARTESIAN_POINT('Ctrl Pts',(-18.9008906793119,32.2724764234145,124.505484170492)) ;
#68374=CARTESIAN_POINT('Ctrl Pts',(-18.5484324346786,32.4623598269078,124.649195864268)) ;
#68375=CARTESIAN_POINT('Ctrl Pts',(-18.7205888114285,32.2823707465449,124.401712667753)) ;
#68376=CARTESIAN_POINT('Ctrl Pts',(-18.3476349380033,32.4723016340023,124.482101731582)) ;
#68377=CARTESIAN_POINT('Ctrl Pts',(-18.5599523479521,32.2923125536394,124.268035850005)) ;
#68378=CARTESIAN_POINT('Ctrl Pts',(-18.1777508202333,32.4823041449576,124.281474853431)) ;
#68379=CARTESIAN_POINT('Ctrl Pts',(-18.4240467225334,32.3023150645948,124.10753302208)) ;
#68380=CARTESIAN_POINT('Ctrl Pts',(-18.0452392633268,32.492338865776,124.053503454134)) ;
#68381=CARTESIAN_POINT('Ctrl Pts',(-18.3180393459561,32.3123497854131,123.925154800795)) ;
#68382=CARTESIAN_POINT('Ctrl Pts',(-17.9556292696089,32.5021840432817,123.810780412352)) ;
#68383=CARTESIAN_POINT('Ctrl Pts',(-18.24635350555,32.3221949629189,123.73097605505)) ;
#68384=CARTESIAN_POINT('Ctrl Pts',(-17.9083727783839,32.5121688036828,123.552719582534)) ;
#68385=CARTESIAN_POINT('Ctrl Pts',(-18.2085503837353,32.3321797233199,123.524527146658)) ;
#68386=CARTESIAN_POINT('Ctrl Pts',(-17.9065240318847,32.5221077099992,123.291502653985)) ;
#68387=CARTESIAN_POINT('Ctrl Pts',(-18.2070734512826,32.3421186296363,123.315553837412)) ;
#68388=CARTESIAN_POINT('Ctrl Pts',(-17.9505907657664,32.5321499376349,123.031335993592)) ;
#68389=CARTESIAN_POINT('Ctrl Pts',(-18.242328891931,32.3521608572721,123.107420816645)) ;
#68390=CARTESIAN_POINT('Ctrl Pts',(-18.0376192936705,32.5420351492193,122.786543593569)) ;
#68391=CARTESIAN_POINT('Ctrl Pts',(-18.3119535058972,32.3620460688564,122.911587983726)) ;
#68392=CARTESIAN_POINT('Ctrl Pts',(-18.1669767556182,32.5520340794212,122.557873550048)) ;
#68393=CARTESIAN_POINT('Ctrl Pts',(-18.4154411876375,32.3720449990584,122.728653018332)) ;
#68394=CARTESIAN_POINT('Ctrl Pts',(-18.3326104946629,32.5619515023317,122.356600741746)) ;
#68395=CARTESIAN_POINT('Ctrl Pts',(-18.5479494908398,32.3819624219688,122.567636304059)) ;
#68396=CARTESIAN_POINT('Ctrl Pts',(-18.5332526173871,32.5719994344104,122.185007966984)) ;
#68397=CARTESIAN_POINT('Ctrl Pts',(-18.7084645480787,32.3920103540475,122.430363551794)) ;
#68398=CARTESIAN_POINT('Ctrl Pts',(-18.7567232187338,32.5818768102198,122.052875232647)) ;
#68399=CARTESIAN_POINT('Ctrl Pts',(-18.8872415842206,32.4018877298569,122.324659316094)) ;
#68400=CARTESIAN_POINT('Ctrl Pts',(-19.0039525695959,32.5919307033877,121.95982536141)) ;
#68401=CARTESIAN_POINT('Ctrl Pts',(-19.0850258485824,32.4119416230248,122.250221203348)) ;
#68402=CARTESIAN_POINT('Ctrl Pts',(-19.2595182815849,32.601824326641,121.911755678648)) ;
#68403=CARTESIAN_POINT('Ctrl Pts',(-19.2894783105699,32.4218352462781,122.211767438031)) ;
#68404=CARTESIAN_POINT('Ctrl Pts',(-19.5238926627054,32.611886920264,121.908700188409)) ;
#68405=CARTESIAN_POINT('Ctrl Pts',(-19.5009779851935,32.4318978399011,122.209324968628)) ;
#68406=CARTESIAN_POINT('Ctrl Pts',(-19.7791709674073,32.6217294942531,121.950535647314)) ;
#68407=CARTESIAN_POINT('Ctrl Pts',(-19.7051996362344,32.4417404138902,122.242795101324)) ;
#68408=CARTESIAN_POINT('Ctrl Pts',(-20.0271280441419,32.631720251136,122.036735366636)) ;
#68409=CARTESIAN_POINT('Ctrl Pts',(-19.9035645706121,32.4517311707731,122.311756541242)) ;
#68410=CARTESIAN_POINT('Ctrl Pts',(-20.2549311093635,32.6416483128939,122.163938821337)) ;
#68411=CARTESIAN_POINT('Ctrl Pts',(-20.0858057967329,32.4616592325311,122.413520699274)) ;
#68412=CARTESIAN_POINT('Ctrl Pts',(-20.4586943445291,32.6516362887831,122.329402962598)) ;
#68413=CARTESIAN_POINT('Ctrl Pts',(-20.2488151736051,32.4716472084202,122.545893272239)) ;
#68414=CARTESIAN_POINT('Ctrl Pts',(-20.6311078851739,32.6616719531395,122.528955452347)) ;
#68415=CARTESIAN_POINT('Ctrl Pts',(-20.3867446776176,32.4816828727767,122.705536503265)) ;
#68416=CARTESIAN_POINT('Ctrl Pts',(-20.76419350534,32.6715278915592,122.751167847475)) ;
#68417=CARTESIAN_POINT('Ctrl Pts',(-20.4932112993434,32.4915388111963,122.88330668774)) ;
#68418=CARTESIAN_POINT('Ctrl Pts',(-20.8583709770248,32.6815233829561,122.99634558384)) ;
#68419=CARTESIAN_POINT('Ctrl Pts',(-20.5685516696912,32.5015343025932,123.079449363677)) ;
#68420=CARTESIAN_POINT('Ctrl Pts',(-20.9082019158921,32.6914331879096,123.251966021349)) ;
#68421=CARTESIAN_POINT('Ctrl Pts',(-20.6084146932958,32.5114441075467,123.283945511149)) ;
#68422=CARTESIAN_POINT('Ctrl Pts',(-20.913367466307,32.7014454101763,123.515032024856)) ;
#68423=CARTESIAN_POINT('Ctrl Pts',(-20.6125455536325,32.5214563298134,123.494398306009)) ;
#68424=CARTESIAN_POINT('Ctrl Pts',(-20.8722060909322,32.7114732908691,123.775321815842)) ;
#68425=CARTESIAN_POINT('Ctrl Pts',(-20.5796147887184,32.5314842105063,123.702629927723)) ;
#68426=CARTESIAN_POINT('Ctrl Pts',(-20.7883600167789,32.7213296868517,124.02038977865)) ;
#68427=CARTESIAN_POINT('Ctrl Pts',(-20.5125366813953,32.5413406064889,123.898683026209)) ;
#68428=CARTESIAN_POINT('Ctrl Pts',(-20.6615779007813,32.7313544840317,124.25132140461)) ;
#68429=CARTESIAN_POINT('Ctrl Pts',(-20.4111096709629,32.5513654036688,124.083427628986)) ;
#68430=CARTESIAN_POINT('Ctrl Pts',(-20.4960157375153,32.7413854140155,124.456454889738)) ;
#68431=CARTESIAN_POINT('Ctrl Pts',(-20.2786586468199,32.5613963336526,124.247533447329)) ;
#68432=CARTESIAN_POINT('Ctrl Pts',(-20.3013621684409,32.7512300165242,124.626844922445)) ;
#68433=CARTESIAN_POINT('Ctrl Pts',(-20.1229354628895,32.5712409361613,124.38384373688)) ;
#68434=CARTESIAN_POINT('Ctrl Pts',(-20.0771483650704,32.7612208677483,124.763458712167)) ;
#68435=CARTESIAN_POINT('Ctrl Pts',(-19.9435638346434,32.5812317873854,124.493133506793)) ;
#68436=CARTESIAN_POINT('Ctrl Pts',(-19.8312628601083,32.7712587007595,124.858962378708)) ;
#68437=CARTESIAN_POINT('Ctrl Pts',(-19.7468547876405,32.5912696203966,124.569535079804)) ;
#68438=CARTESIAN_POINT('Ctrl Pts',(-19.5775920832475,32.7811030892249,124.909777937782)) ;
#68439=CARTESIAN_POINT('Ctrl Pts',(-19.5439188102841,32.6011140088621,124.610185961714)) ;
#68440=CARTESIAN_POINT('Ctrl Pts',(-19.3153197757331,32.7910878935945,124.916379101424)) ;
#68441=CARTESIAN_POINT('Ctrl Pts',(-19.3341011312526,32.6110988132316,124.615465586228)) ;
#68442=CARTESIAN_POINT('Ctrl Pts',(-19.0569748481772,32.8010274130773,124.877619388893)) ;
#68443=CARTESIAN_POINT('Ctrl Pts',(-19.1274258094831,32.6210383327145,124.584456619583)) ;
#68444=CARTESIAN_POINT('Ctrl Pts',(-18.8068609697535,32.8110671440787,124.793713447214)) ;
#68445=CARTESIAN_POINT('Ctrl Pts',(-18.9273350056697,32.6310780637158,124.517330604952)) ;
#68446=CARTESIAN_POINT('Ctrl Pts',(-18.5785199696836,32.820955272325,124.669655218426)) ;
#68447=CARTESIAN_POINT('Ctrl Pts',(-18.7446634574821,32.6409661919621,124.418083265181)) ;
#68448=CARTESIAN_POINT('Ctrl Pts',(-18.3728153330768,32.8309449975335,124.506569798915)) ;
#68449=CARTESIAN_POINT('Ctrl Pts',(-18.5801006004135,32.6509559171706,124.287614130099)) ;
#68450=CARTESIAN_POINT('Ctrl Pts',(-18.1992468678326,32.840902762235,124.310742518053)) ;
#68451=CARTESIAN_POINT('Ctrl Pts',(-18.4412469568537,32.6609136818721,124.130951769751)) ;
#68452=CARTESIAN_POINT('Ctrl Pts',(-18.0625524288157,32.850805103647,124.089302873787)) ;
#68453=CARTESIAN_POINT('Ctrl Pts',(-18.3318926747522,32.6708160232841,123.95380009295)) ;
#68454=CARTESIAN_POINT('Ctrl Pts',(-17.9650377613778,32.8608492993534,123.844039624706)) ;
#68455=CARTESIAN_POINT('Ctrl Pts',(-18.2538818733743,32.6808602189905,123.757588954974)) ;
#68456=CARTESIAN_POINT('Ctrl Pts',(-17.9122844842802,32.8707567001127,123.58906943826)) ;
#68457=CARTESIAN_POINT('Ctrl Pts',(-18.2116804247751,32.6907676197498,123.553613231978)) ;
#68458=CARTESIAN_POINT('Ctrl Pts',(-17.9040614841339,32.880767299987,123.326126151249)) ;
#68459=CARTESIAN_POINT('Ctrl Pts',(-18.2051029793148,32.7007782196241,123.34325861009)) ;
#68460=CARTESIAN_POINT('Ctrl Pts',(-17.9421976273555,32.8907975958992,123.065306227518)) ;
#68461=CARTESIAN_POINT('Ctrl Pts',(-18.2356129698765,32.7108085155363,123.134602745316)) ;
#68462=CARTESIAN_POINT('Ctrl Pts',(-18.0232436735507,32.9006523755489,122.819357208247)) ;
#68463=CARTESIAN_POINT('Ctrl Pts',(-18.3004504322419,32.720663295186,122.937844802407)) ;
#68464=CARTESIAN_POINT('Ctrl Pts',(-18.1463463293519,32.9106097037664,122.588444800357)) ;
#68465=CARTESIAN_POINT('Ctrl Pts',(-18.3989330865564,32.7306206234035,122.753115585193)) ;
#68466=CARTESIAN_POINT('Ctrl Pts',(-18.3093474042476,32.9206487366733,122.381033273986)) ;
#68467=CARTESIAN_POINT('Ctrl Pts',(-18.5293347464535,32.7406596563104,122.587186824327)) ;
#68468=CARTESIAN_POINT('Ctrl Pts',(-18.5023603004912,32.9305218485626,122.207583253798)) ;
#68469=CARTESIAN_POINT('Ctrl Pts',(-18.6837449255098,32.7505327681997,122.448428002608)) ;
#68470=CARTESIAN_POINT('Ctrl Pts',(-18.7269817759468,32.9405951335897,122.067617063673)) ;
#68471=CARTESIAN_POINT('Ctrl Pts',(-18.8634428286131,32.7606060532268,122.336455563458)) ;
#68472=CARTESIAN_POINT('Ctrl Pts',(-18.9663055363985,32.9504154533265,121.970905134139)) ;
#68473=CARTESIAN_POINT('Ctrl Pts',(-19.0549009577353,32.7704263729636,122.259087166004)) ;
#68474=CARTESIAN_POINT('Ctrl Pts',(-19.2252558871534,32.9604941187049,121.915591458617)) ;
#68475=CARTESIAN_POINT('Ctrl Pts',(-19.262061748827,32.780505038342,122.214836808385)) ;
#68476=CARTESIAN_POINT('Ctrl Pts',(-19.4840372151867,32.9703457091887,121.906199287805)) ;
#68477=CARTESIAN_POINT('Ctrl Pts',(-19.4690857796967,32.7903566288258,122.207323762619)) ;
#68478=CARTESIAN_POINT('Ctrl Pts',(-19.7462073716882,32.9804188595076,121.942441422299)) ;
#68479=CARTESIAN_POINT('Ctrl Pts',(-19.6788221704482,32.8004297791447,122.236318111422)) ;
#68480=CARTESIAN_POINT('Ctrl Pts',(-19.9923907933803,32.9902612394826,122.021850824201)) ;
#68481=CARTESIAN_POINT('Ctrl Pts',(-19.8757676411912,32.8102721591198,122.299845862724)) ;
#68482=CARTESIAN_POINT('Ctrl Pts',(-20.2246277641436,33.0002422157257,122.143718242006)) ;
#68483=CARTESIAN_POINT('Ctrl Pts',(-20.0615568191512,32.8202531353628,122.397340033153)) ;
#68484=CARTESIAN_POINT('Ctrl Pts',(-20.4326666594073,33.010258544081,122.304997705767)) ;
#68485=CARTESIAN_POINT('Ctrl Pts',(-20.2279876169795,32.8302694637181,122.52636399411)) ;
#68486=CARTESIAN_POINT('Ctrl Pts',(-20.6076780088902,33.0201563410721,122.497403957948)) ;
#68487=CARTESIAN_POINT('Ctrl Pts',(-20.3679958534134,32.8401672607093,122.680288693608)) ;
#68488=CARTESIAN_POINT('Ctrl Pts',(-20.7486295700232,33.0301688978042,122.719608055138)) ;
#68489=CARTESIAN_POINT('Ctrl Pts',(-20.4807568301996,32.8501798174413,122.858052122149)) ;
#68490=CARTESIAN_POINT('Ctrl Pts',(-20.8484637130917,33.0402009326507,122.96359161389)) ;
#68491=CARTESIAN_POINT('Ctrl Pts',(-20.5606237531606,32.8602118522878,123.053239243088)) ;
#68492=CARTESIAN_POINT('Ctrl Pts',(-20.9039796443904,33.0500403334661,123.216152649294)) ;
#68493=CARTESIAN_POINT('Ctrl Pts',(-20.6050359484339,32.8700512531033,123.255286987946)) ;
#68494=CARTESIAN_POINT('Ctrl Pts',(-20.9152463774755,33.0601061191177,123.480399984258)) ;
#68495=CARTESIAN_POINT('Ctrl Pts',(-20.6140490933859,32.8801170387548,123.466685170754)) ;
#68496=CARTESIAN_POINT('Ctrl Pts',(-20.8809372575507,33.0699965742323,123.738064421165)) ;
#68497=CARTESIAN_POINT('Ctrl Pts',(-20.5866016261539,32.8900074938694,123.672815854496)) ;
#68498=CARTESIAN_POINT('Ctrl Pts',(-20.8021533889854,33.0799886928681,123.98853537261)) ;
#68499=CARTESIAN_POINT('Ctrl Pts',(-20.523574446852,32.8999996125052,123.873192408795)) ;
#68500=CARTESIAN_POINT('Ctrl Pts',(-20.6812106073249,33.0899515196311,124.220732031348)) ;
#68501=CARTESIAN_POINT('Ctrl Pts',(-20.4268202076342,32.9099624392683,124.058949317243)) ;
#68502=CARTESIAN_POINT('Ctrl Pts',(-20.5232306933288,33.099855802904,124.427605321835)) ;
#68503=CARTESIAN_POINT('Ctrl Pts',(-20.3004367035077,32.9198667225411,124.22444733005)) ;
#68504=CARTESIAN_POINT('Ctrl Pts',(-20.3285971107455,33.1099162368511,124.606480559927)) ;
#68505=CARTESIAN_POINT('Ctrl Pts',(-20.1447295646736,32.9299271564882,124.36754764172)) ;
#68506=CARTESIAN_POINT('Ctrl Pts',(-20.1108525131507,33.1197567895243,124.746047511506)) ;
#68507=CARTESIAN_POINT('Ctrl Pts',(-19.970534871693,32.9397677091614,124.479200559667)) ;
#68508=CARTESIAN_POINT('Ctrl Pts',(-19.8669950901314,33.12981900947,124.84821784105)) ;
#68509=CARTESIAN_POINT('Ctrl Pts',(-19.7754486895611,32.9498299291071,124.560937006756)) ;
#68510=CARTESIAN_POINT('Ctrl Pts',(-19.6132318493154,33.1397161487486,124.905283007203)) ;
#68511=CARTESIAN_POINT('Ctrl Pts',(-19.5724388798712,32.9597270683857,124.606588967545)) ;
#68512=CARTESIAN_POINT('Ctrl Pts',(-19.3525812289575,33.1496473408836,124.918328736674)) ;
#68513=CARTESIAN_POINT('Ctrl Pts',(-19.3639189712111,32.9696582605208,124.617025749215)) ;
#68514=CARTESIAN_POINT('Ctrl Pts',(-19.090770522027,33.1596894955287,124.885264797401)) ;
#68515=CARTESIAN_POINT('Ctrl Pts',(-19.1544702195643,32.9797004151658,124.590574725584)) ;
#68516=CARTESIAN_POINT('Ctrl Pts',(-18.842487870914,33.169576256548,124.808646986439)) ;
#68517=CARTESIAN_POINT('Ctrl Pts',(-18.9558448766533,32.9895871761851,124.529280933374)) ;
#68518=CARTESIAN_POINT('Ctrl Pts',(-18.6085457635101,33.1795755582652,124.689058201042)) ;
#68519=CARTESIAN_POINT('Ctrl Pts',(-18.7686911704573,32.9995864779024,124.433610222531)) ;
#68520=CARTESIAN_POINT('Ctrl Pts',(-18.4004044124469,33.189496356432,124.532007686267)) ;
#68521=CARTESIAN_POINT('Ctrl Pts',(-18.6021783869313,33.0095072760691,124.307970451747)) ;
#68522=CARTESIAN_POINT('Ctrl Pts',(-18.2206897370185,33.1995304100287,124.339091714962)) ;
#68523=CARTESIAN_POINT('Ctrl Pts',(-18.4584063193687,33.0195413296658,124.153637825087)) ;
#68524=CARTESIAN_POINT('Ctrl Pts',(-18.0786177880743,33.2094535275951,124.120374761366)) ;
#68525=CARTESIAN_POINT('Ctrl Pts',(-18.344748777028,33.0294644472322,123.978664981646)) ;
#68526=CARTESIAN_POINT('Ctrl Pts',(-17.9753934550452,33.2195096510942,123.87713368977)) ;
#68527=CARTESIAN_POINT('Ctrl Pts',(-18.2621688831962,33.0395205707314,123.784072046529)) ;
#68528=CARTESIAN_POINT('Ctrl Pts',(-17.9170984303965,33.2293550927491,123.625046988953)) ;
#68529=CARTESIAN_POINT('Ctrl Pts',(-18.2155327344032,33.0493660123862,123.582403874291)) ;
#68530=CARTESIAN_POINT('Ctrl Pts',(-17.9024396209619,33.2393173938732,123.363675275733)) ;
#68531=CARTESIAN_POINT('Ctrl Pts',(-18.2038050999464,33.0593283135103,123.373306898927)) ;
#68532=CARTESIAN_POINT('Ctrl Pts',(-17.9339408232565,33.2493458731483,123.102009100134)) ;
#68533=CARTESIAN_POINT('Ctrl Pts',(-18.2290055541262,33.0693567927855,123.163973819942)) ;
#68534=CARTESIAN_POINT('Ctrl Pts',(-18.009402919707,33.259256226658,122.852760854094)) ;
#68535=CARTESIAN_POINT('Ctrl Pts',(-18.2893745088673,33.0792671462951,122.964575736527)) ;
#68536=CARTESIAN_POINT('Ctrl Pts',(-18.1266871223674,33.2691910988352,122.61950036567)) ;
#68537=CARTESIAN_POINT('Ctrl Pts',(-18.3832009980876,33.0892020184723,122.777967498192)) ;
#68538=CARTESIAN_POINT('Ctrl Pts',(-18.2845465433898,33.2792322364209,122.40806845954)) ;
#68539=CARTESIAN_POINT('Ctrl Pts',(-18.5094881032574,33.099243156058,122.608821464249)) ;
#68540=CARTESIAN_POINT('Ctrl Pts',(-18.4736647676083,33.2891193856355,122.229881635933)) ;
#68541=CARTESIAN_POINT('Ctrl Pts',(-18.6607816011752,33.1091303052726,122.466272069737)) ;
#68542=CARTESIAN_POINT('Ctrl Pts',(-18.6928889148738,33.2991116203865,122.085373784708)) ;
#68543=CARTESIAN_POINT('Ctrl Pts',(-18.8361603422665,33.1191225400237,122.350665209582)) ;
#68544=CARTESIAN_POINT('Ctrl Pts',(-18.9328841091275,33.3090603259495,121.981637584403)) ;
#68545=CARTESIAN_POINT('Ctrl Pts',(-19.0281557898517,33.1290712455866,122.267675703838)) ;
#68546=CARTESIAN_POINT('Ctrl Pts',(-19.1868031331839,33.3189963943732,121.920862306553)) ;
#68547=CARTESIAN_POINT('Ctrl Pts',(-19.2312903095408,33.1390073140103,122.219054752622)) ;
#68548=CARTESIAN_POINT('Ctrl Pts',(-19.4487454010854,33.328982078589,121.90471788781)) ;
#68549=CARTESIAN_POINT('Ctrl Pts',(-19.4408438645719,33.1489929982261,122.20613828772)) ;
#68550=CARTESIAN_POINT('Ctrl Pts',(-19.7108540776556,33.3390225051576,121.934873930191)) ;
#68551=CARTESIAN_POINT('Ctrl Pts',(-19.6505310372627,33.1590334247948,122.230262297346)) ;
#68552=CARTESIAN_POINT('Ctrl Pts',(-19.9588162424853,33.3488616186214,122.008165761205)) ;
#68553=CARTESIAN_POINT('Ctrl Pts',(-19.8488999925423,33.1688725382585,122.288894547529)) ;
#68554=CARTESIAN_POINT('Ctrl Pts',(-20.1950323307625,33.3588913527972,122.125097981869)) ;
#68555=CARTESIAN_POINT('Ctrl Pts',(-20.0378734209598,33.1789022724343,122.38243939003)) ;
#68556=CARTESIAN_POINT('Ctrl Pts',(-20.406784218548,33.3689134523031,122.281698617158)) ;
#68557=CARTESIAN_POINT('Ctrl Pts',(-20.2072754977896,33.1889243719402,122.507719170111)) ;
#68558=CARTESIAN_POINT('Ctrl Pts',(-20.5858350552601,33.3787818921965,122.469326974363)) ;
#68559=CARTESIAN_POINT('Ctrl Pts',(-20.350516319059,33.1987928118337,122.657820459907)) ;
#68560=CARTESIAN_POINT('Ctrl Pts',(-20.732476955186,33.3888507568821,122.68954538537)) ;
#68561=CARTESIAN_POINT('Ctrl Pts',(-20.4678308998726,33.2088616765193,122.833994843785)) ;
#68562=CARTESIAN_POINT('Ctrl Pts',(-20.8362904559934,33.3986934299808,122.926463443138)) ;
#68563=CARTESIAN_POINT('Ctrl Pts',(-20.5508822680002,33.2187043496179,123.023527908559)) ;
#68564=CARTESIAN_POINT('Ctrl Pts',(-20.8990494415645,33.4086540641432,123.180578146984)) ;
#68565=CARTESIAN_POINT('Ctrl Pts',(-20.6010906294462,33.2286649837803,123.226819047015)) ;
#68566=CARTESIAN_POINT('Ctrl Pts',(-20.916351249052,33.4186919798213,123.443786581483)) ;
#68567=CARTESIAN_POINT('Ctrl Pts',(-20.6149332528463,33.2387028994585,123.43738582393)) ;
#68568=CARTESIAN_POINT('Ctrl Pts',(-20.8886281343362,33.4285662546808,123.701819630219)) ;
#68569=CARTESIAN_POINT('Ctrl Pts',(-20.592756117805,33.2485771743179,123.643811594593)) ;
#68570=CARTESIAN_POINT('Ctrl Pts',(-20.8151004364326,33.4386360050559,123.95598455471)) ;
#68571=CARTESIAN_POINT('Ctrl Pts',(-20.5339351068565,33.258646924693,123.84714415652)) ;
#68572=CARTESIAN_POINT('Ctrl Pts',(-20.7013946872375,33.4484693004304,124.188056231771)) ;
#68573=CARTESIAN_POINT('Ctrl Pts',(-20.442972128081,33.2684802200675,124.03280115278)) ;
#68574=CARTESIAN_POINT('Ctrl Pts',(-20.5466931297227,33.45849959791,124.401459336272)) ;
#68575=CARTESIAN_POINT('Ctrl Pts',(-20.3192120229929,33.2785105175472,124.20352454908)) ;
#68576=CARTESIAN_POINT('Ctrl Pts',(-20.3567007162318,33.4685316843515,124.58424663072)) ;
#68577=CARTESIAN_POINT('Ctrl Pts',(-20.1672189437675,33.2885426039886,124.34975536662)) ;
#68578=CARTESIAN_POINT('Ctrl Pts',(-20.1426457143214,33.4783596128404,124.728735741513)) ;
#68579=CARTESIAN_POINT('Ctrl Pts',(-19.9959765796565,33.2983705324775,124.465347258471)) ;
#68580=CARTESIAN_POINT('Ctrl Pts',(-19.9029989792466,33.4883556539512,124.836308043002)) ;
#68581=CARTESIAN_POINT('Ctrl Pts',(-19.8042599394586,33.3083665735883,124.551406472735)) ;
#68582=CARTESIAN_POINT('Ctrl Pts',(-19.6474220237301,33.4983814660524,124.900335793291)) ;
#68583=CARTESIAN_POINT('Ctrl Pts',(-19.5997986983396,33.3183923856895,124.602630093288)) ;
#68584=CARTESIAN_POINT('Ctrl Pts',(-19.3882695560054,33.5082687009472,124.919091810044)) ;
#68585=CARTESIAN_POINT('Ctrl Pts',(-19.3924774972755,33.3282796205843,124.617636375343)) ;
#68586=CARTESIAN_POINT('Ctrl Pts',(-19.1274334857693,33.5182455671582,124.892759807624)) ;
#68587=CARTESIAN_POINT('Ctrl Pts',(-19.1838086836,33.3382564867954,124.596572391666)) ;
#68588=CARTESIAN_POINT('Ctrl Pts',(-18.8746590268341,33.52823851103,124.821451907867)) ;
#68589=CARTESIAN_POINT('Ctrl Pts',(-18.9815887977188,33.3482494306672,124.539527654376)) ;
#68590=CARTESIAN_POINT('Ctrl Pts',(-18.6372374521722,33.5382764337014,124.706546424498)) ;
#68591=CARTESIAN_POINT('Ctrl Pts',(-18.7916507985739,33.3582873533385,124.447604630339)) ;
#68592=CARTESIAN_POINT('Ctrl Pts',(-18.4271493677989,33.5481248979631,124.555368999614)) ;
#68593=CARTESIAN_POINT('Ctrl Pts',(-18.6235800486874,33.3681358176002,124.326664485506)) ;
#68594=CARTESIAN_POINT('Ctrl Pts',(-18.2435773439465,33.5581167647071,124.367679767415)) ;
#68595=CARTESIAN_POINT('Ctrl Pts',(-18.4767213025052,33.3781276843442,124.176514389402)) ;
#68596=CARTESIAN_POINT('Ctrl Pts',(-18.096319636919,33.5680344967483,124.152599028164)) ;
#68597=CARTESIAN_POINT('Ctrl Pts',(-18.3589139685211,33.3880454163854,124.004451152358)) ;
#68598=CARTESIAN_POINT('Ctrl Pts',(-17.9874040348388,33.5780626816436,123.912652984584)) ;
#68599=CARTESIAN_POINT('Ctrl Pts',(-18.271779888472,33.3980736012807,123.812495012593)) ;
#68600=CARTESIAN_POINT('Ctrl Pts',(-17.9226291155959,33.5879478396924,123.661079753393)) ;
#68601=CARTESIAN_POINT('Ctrl Pts',(-18.2199583955529,33.4079587593295,123.611237435979)) ;
#68602=CARTESIAN_POINT('Ctrl Pts',(-17.9016709287819,33.5979372002341,123.399402541443)) ;
#68603=CARTESIAN_POINT('Ctrl Pts',(-18.2031899993243,33.4179481198712,123.401895940217)) ;
#68604=CARTESIAN_POINT('Ctrl Pts',(-17.9271501704679,33.6079783571685,123.1367648659)) ;
#68605=CARTESIAN_POINT('Ctrl Pts',(-18.2235716341578,33.4279892768056,123.191785556007)) ;
#68606=CARTESIAN_POINT('Ctrl Pts',(-17.9959631146861,33.6178109406236,122.887710030823)) ;
#68607=CARTESIAN_POINT('Ctrl Pts',(-18.2786200105537,33.4378218602607,122.992541933455)) ;
#68608=CARTESIAN_POINT('Ctrl Pts',(-18.1081263093149,33.6278051605856,122.650231330554)) ;
#68609=CARTESIAN_POINT('Ctrl Pts',(-18.3683487586546,33.4478160802227,122.802558226559)) ;
#68610=CARTESIAN_POINT('Ctrl Pts',(-18.2607792875272,33.6378332623729,122.435411305488)) ;
#68611=CARTESIAN_POINT('Ctrl Pts',(-18.4904696240239,33.45784418201,122.630701109372)) ;
#68612=CARTESIAN_POINT('Ctrl Pts',(-18.4453797141511,33.647713206996,122.252832221367)) ;
#68613=CARTESIAN_POINT('Ctrl Pts',(-18.6381482311407,33.4677241266331,122.484636845497)) ;
#68614=CARTESIAN_POINT('Ctrl Pts',(-18.6610157891126,33.657703533553,122.10310705135)) ;
#68615=CARTESIAN_POINT('Ctrl Pts',(-18.8106558663145,33.4777144531901,122.364855145268)) ;
#68616=CARTESIAN_POINT('Ctrl Pts',(-18.8982140305105,33.6676444652073,121.993631136502)) ;
#68617=CARTESIAN_POINT('Ctrl Pts',(-19.0004133768427,33.4876553848444,122.277272732784)) ;
#68618=CARTESIAN_POINT('Ctrl Pts',(-19.1519080089799,33.6776315837102,121.92632833614)) ;
#68619=CARTESIAN_POINT('Ctrl Pts',(-19.2033679299254,33.4976425033473,122.223428561246)) ;
#68620=CARTESIAN_POINT('Ctrl Pts',(-19.4146423301779,33.6876649166074,121.904411969349)) ;
#68621=CARTESIAN_POINT('Ctrl Pts',(-19.4135552411739,33.5076758362445,122.20589349727)) ;
#68622=CARTESIAN_POINT('Ctrl Pts',(-19.6729091690056,33.6975310210521,121.927545767156)) ;
#68623=CARTESIAN_POINT('Ctrl Pts',(-19.6201683942856,33.5175419406893,122.224398461816)) ;
#68624=CARTESIAN_POINT('Ctrl Pts',(-19.9282681240009,33.7075971349325,121.996466980296)) ;
#68625=CARTESIAN_POINT('Ctrl Pts',(-19.8244562056054,33.5276080545696,122.279533486686)) ;
#68626=CARTESIAN_POINT('Ctrl Pts',(-20.1628320829574,33.7174531467009,122.10634520991)) ;
#68627=CARTESIAN_POINT('Ctrl Pts',(-20.0121077897334,33.537464066338,122.367434006079)) ;
#68628=CARTESIAN_POINT('Ctrl Pts',(-20.3781604555604,33.7274478503322,122.256728476995)) ;
#68629=CARTESIAN_POINT('Ctrl Pts',(-20.184371642184,33.5474587699693,122.487738827655)) ;
#68630=CARTESIAN_POINT('Ctrl Pts',(-20.5643974693118,33.7374791860571,122.443302838799)) ;
#68631=CARTESIAN_POINT('Ctrl Pts',(-20.3333627176559,33.5574901056942,122.636996853287)) ;
#68632=CARTESIAN_POINT('Ctrl Pts',(-20.713269761922,33.7473457112607,122.655597325724)) ;
#68633=CARTESIAN_POINT('Ctrl Pts',(-20.4524620449125,33.5673566308979,122.806830892729)) ;
#68634=CARTESIAN_POINT('Ctrl Pts',(-20.8247303532555,33.7573331393065,122.893178808627)) ;
#68635=CARTESIAN_POINT('Ctrl Pts',(-20.5416324255552,33.5773440589437,122.99689507574)) ;
#68636=CARTESIAN_POINT('Ctrl Pts',(-20.8931087336896,33.767278068993,123.145457142139)) ;
#68637=CARTESIAN_POINT('Ctrl Pts',(-20.5963371660383,33.5872889886301,123.198716996963)) ;
#68638=CARTESIAN_POINT('Ctrl Pts',(-20.9167263518425,33.7773229871015,123.408343079754)) ;
#68639=CARTESIAN_POINT('Ctrl Pts',(-20.6152334042726,33.5973339067386,123.409025569641)) ;
#68640=CARTESIAN_POINT('Ctrl Pts',(-20.8949748056446,33.7871849567154,123.666612207482)) ;
#68641=CARTESIAN_POINT('Ctrl Pts',(-20.5978343558141,33.6071958763525,123.61564071411)) ;
#68642=CARTESIAN_POINT('Ctrl Pts',(-20.8283422293108,33.7971770247366,123.920571241178)) ;
#68643=CARTESIAN_POINT('Ctrl Pts',(-20.5445304472365,33.6171879443737,123.818808427627)) ;
#68644=CARTESIAN_POINT('Ctrl Pts',(-20.7192376865205,33.8071079501112,124.157662672187)) ;
#68645=CARTESIAN_POINT('Ctrl Pts',(-20.4572488862588,33.6271188697483,124.008482329076)) ;
#68646=CARTESIAN_POINT('Ctrl Pts',(-20.5707091129721,33.8170585783346,124.372854625881)) ;
#68647=CARTESIAN_POINT('Ctrl Pts',(-20.3384279325118,33.6370694979717,124.180637052448)) ;
#68648=CARTESIAN_POINT('Ctrl Pts',(-20.3862313186414,33.8270588173937,124.560056609312)) ;
#68649=CARTESIAN_POINT('Ctrl Pts',(-20.1908473210986,33.6470697370308,124.330400159823)) ;
#68650=CARTESIAN_POINT('Ctrl Pts',(-20.1712584195521,33.8370872727629,124.71248063517)) ;
#68651=CARTESIAN_POINT('Ctrl Pts',(-20.0188703330059,33.6570981924,124.45234117015)) ;
#68652=CARTESIAN_POINT('Ctrl Pts',(-19.9370901885251,33.8469533073462,124.823799494521)) ;
#68653=CARTESIAN_POINT('Ctrl Pts',(-19.8315368156364,33.6669642269833,124.541398163761)) ;
#68654=CARTESIAN_POINT('Ctrl Pts',(-19.6841021964421,33.8569456290936,124.894057284954)) ;
#68655=CARTESIAN_POINT('Ctrl Pts',(-19.6291473694453,33.6769565487307,124.597606616661)) ;
#68656=CARTESIAN_POINT('Ctrl Pts',(-19.424287490384,33.8668779187706,124.9192160717)) ;
#68657=CARTESIAN_POINT('Ctrl Pts',(-19.4212948596349,33.6868888384077,124.617735604572)) ;
#68658=CARTESIAN_POINT('Ctrl Pts',(-19.1622401128872,33.8768795637414,124.898995670993)) ;
#68659=CARTESIAN_POINT('Ctrl Pts',(-19.2116608120875,33.6968904833785,124.60156252601)) ;
#68660=CARTESIAN_POINT('Ctrl Pts',(-18.823429392135,33.8901921971574,124.811777112252)) ;
#68661=CARTESIAN_POINT('Ctrl Pts',(-18.9405918138416,33.7102031167945,124.531785666973)) ;
#68662=CARTESIAN_POINT('Ctrl Pts',(-18.5168908225473,33.903423946539,124.639429121269)) ;
#68663=CARTESIAN_POINT('Ctrl Pts',(-18.6953483850143,33.7234348661761,124.393891756695)) ;
#68664=CARTESIAN_POINT('Ctrl Pts',(-18.266416953034,33.916747211356,124.394788919274)) ;
#68665=CARTESIAN_POINT('Ctrl Pts',(-18.4950002778242,33.7367581309931,124.198208384198)) ;
#68666=CARTESIAN_POINT('Ctrl Pts',(-18.1147393757088,33.9266229175737,124.184190734435)) ;
#68667=CARTESIAN_POINT('Ctrl Pts',(-18.3736497561591,33.7466338372108,124.029725816734)) ;
#68668=CARTESIAN_POINT('Ctrl Pts',(-18.0003398463956,33.9366125086737,123.947943873737)) ;
#68669=CARTESIAN_POINT('Ctrl Pts',(-18.2821299057794,33.7566234283109,123.840730774139)) ;
#68670=CARTESIAN_POINT('Ctrl Pts',(-17.9289645288639,33.9465396051291,123.69699206503)) ;
#68671=CARTESIAN_POINT('Ctrl Pts',(-18.2250270203462,33.7665505247663,123.639969543988)) ;
#68672=CARTESIAN_POINT('Ctrl Pts',(-17.9019571311773,33.9565647536337,123.434953214904)) ;
#68673=CARTESIAN_POINT('Ctrl Pts',(-18.2034190100901,33.7765756732709,123.430338874046)) ;
#68674=CARTESIAN_POINT('Ctrl Pts',(-17.920456867938,33.9664604077804,123.175542057052)) ;
#68675=CARTESIAN_POINT('Ctrl Pts',(-18.2182165454262,33.7864713274175,123.222809688118)) ;
#68676=CARTESIAN_POINT('Ctrl Pts',(-17.9840343132116,33.9764639421586,122.920489516577)) ;
#68677=CARTESIAN_POINT('Ctrl Pts',(-18.2690763509193,33.7964748617957,123.018767172028)) ;
#68678=CARTESIAN_POINT('Ctrl Pts',(-18.0907856147797,33.9864490805987,122.680743142477)) ;
#68679=CARTESIAN_POINT('Ctrl Pts',(-18.3544753559251,33.8064600002358,122.826969197833)) ;
#68680=CARTESIAN_POINT('Ctrl Pts',(-18.2384789185145,33.996485005194,122.462260358717)) ;
#68681=CARTESIAN_POINT('Ctrl Pts',(-18.4726280899805,33.8164959248312,122.652181813698)) ;
#68682=CARTESIAN_POINT('Ctrl Pts',(-18.4182776203018,34.0063362806217,122.276005602402)) ;
#68683=CARTESIAN_POINT('Ctrl Pts',(-18.6164655966101,33.8263472002588,122.503176330571)) ;
#68684=CARTESIAN_POINT('Ctrl Pts',(-18.6302489538193,34.0163285417831,122.121008187001)) ;
#68685=CARTESIAN_POINT('Ctrl Pts',(-18.7860413729788,33.8363394614202,122.379176658812)) ;
#68686=CARTESIAN_POINT('Ctrl Pts',(-18.8673098715377,34.0263684258007,122.00522798075)) ;
#68687=CARTESIAN_POINT('Ctrl Pts',(-18.9756890388998,33.8463793454378,122.2865505691)) ;
#68688=CARTESIAN_POINT('Ctrl Pts',(-19.1155543481873,34.0362032003031,121.933213929773)) ;
#68689=CARTESIAN_POINT('Ctrl Pts',(-19.1742842270233,33.8562141199402,122.228937167852)) ;
#68690=CARTESIAN_POINT('Ctrl Pts',(-19.3787606441446,34.0462795813234,121.904625237353)) ;
#68691=CARTESIAN_POINT('Ctrl Pts',(-19.3848492266586,33.8662905009605,122.20606409206)) ;
#68692=CARTESIAN_POINT('Ctrl Pts',(-19.636979964933,34.056125854474,121.921704730838)) ;
#68693=CARTESIAN_POINT('Ctrl Pts',(-19.591423616235,33.8761367741112,122.219725605663)) ;
#68694=CARTESIAN_POINT('Ctrl Pts',(-19.9782262367002,34.0694903757593,122.004738916925)) ;
#68695=CARTESIAN_POINT('Ctrl Pts',(-19.8644290060011,33.8895012953964,122.286150073343)) ;
#68696=CARTESIAN_POINT('Ctrl Pts',(-20.2860725515586,34.0826966201937,122.173341752895)) ;
#68697=CARTESIAN_POINT('Ctrl Pts',(-20.1107333615667,33.9027075398308,122.421054696917)) ;
#68698=CARTESIAN_POINT('Ctrl Pts',(-20.5388137926812,34.0959615748709,122.413398914322)) ;
#68699=CARTESIAN_POINT('Ctrl Pts',(-20.3128900569695,33.9159724945081,122.613069455434)) ;
#68700=CARTESIAN_POINT('Ctrl Pts',(-20.6954462284396,34.1059938554226,122.625471146507)) ;
#68701=CARTESIAN_POINT('Ctrl Pts',(-20.4382052101993,33.9260047750597,122.782731831385)) ;
#68702=CARTESIAN_POINT('Ctrl Pts',(-20.8114438350329,34.1159025889405,122.858591933872)) ;
#68703=CARTESIAN_POINT('Ctrl Pts',(-20.5310032327312,33.9359135085776,122.969226073235)) ;
#68704=CARTESIAN_POINT('Ctrl Pts',(-20.8860726329882,34.125840139808,123.108858926557)) ;
#68705=CARTESIAN_POINT('Ctrl Pts',(-20.5907085395253,33.9458510594451,123.169440598116)) ;
#68706=CARTESIAN_POINT('Ctrl Pts',(-20.9161696354576,34.1358699874019,123.370684085346)) ;
#68707=CARTESIAN_POINT('Ctrl Pts',(-20.6147885800743,33.9558809070391,123.37889723275)) ;
#68708=CARTESIAN_POINT('Ctrl Pts',(-20.8957675550664,34.1491051273224,123.717974610671)) ;
#68709=CARTESIAN_POINT('Ctrl Pts',(-20.5984660541345,33.9691160469595,123.656745092967)) ;
#68710=CARTESIAN_POINT('Ctrl Pts',(-20.7562726268257,34.1657735916935,124.138314956001)) ;
#68711=CARTESIAN_POINT('Ctrl Pts',(-20.4868736501461,33.9857845113307,123.993003032338)) ;
#68712=CARTESIAN_POINT('Ctrl Pts',(-20.4290861791078,34.1856446035674,124.553127465598)) ;
#68713=CARTESIAN_POINT('Ctrl Pts',(-20.2251415375173,34.0056555232046,124.32485414861)) ;
#68714=CARTESIAN_POINT('Ctrl Pts',(-20.0516612997823,34.2023516879504,124.786832185012)) ;
#68715=CARTESIAN_POINT('Ctrl Pts',(-19.9231542599151,34.0223626075875,124.511841034845)) ;
#68716=CARTESIAN_POINT('Ctrl Pts',(-19.7200431655426,34.215528969261,124.88675620924)) ;
#68717=CARTESIAN_POINT('Ctrl Pts',(-19.6579040689418,34.0355398888981,124.591763773494)) ;
#68718=CARTESIAN_POINT('Ctrl Pts',(-19.3739840223207,34.2287964297751,124.92908813568)) ;
#68719=CARTESIAN_POINT('Ctrl Pts',(-19.3810402452549,34.0488073494122,124.625633782971)) ;
#68720=CARTESIAN_POINT('Ctrl Pts',(-18.936720024018,34.2454103204623,124.86755517988)) ;
#68721=CARTESIAN_POINT('Ctrl Pts',(-19.0312400607427,34.0654212400994,124.576410349906)) ;
#68722=CARTESIAN_POINT('Ctrl Pts',(-18.4683529488932,34.2653591198897,124.618947214226)) ;
#68723=CARTESIAN_POINT('Ctrl Pts',(-18.6565409486287,34.0853700395268,124.377526283527)) ;
#68724=CARTESIAN_POINT('Ctrl Pts',(-18.1135823385577,34.2852802314206,124.226010700003)) ;
#68725=CARTESIAN_POINT('Ctrl Pts',(-18.3727229363681,34.1052911510577,124.063178594994)) ;
#68726=CARTESIAN_POINT('Ctrl Pts',(-17.9136663305497,34.3051466795934,123.737213595555)) ;
#68727=CARTESIAN_POINT('Ctrl Pts',(-18.2127872251194,34.1251575992306,123.672140797996)) ;
#68728=CARTESIAN_POINT('Ctrl Pts',(-17.8927069831386,34.3251730262106,123.205416904764)) ;
#68729=CARTESIAN_POINT('Ctrl Pts',(-18.1960174659992,34.1451839458477,123.246703802556)) ;
#68730=CARTESIAN_POINT('Ctrl Pts',(-18.0532950837359,34.3450350706001,122.702439446676)) ;
#68731=CARTESIAN_POINT('Ctrl Pts',(-18.3244861394055,34.1650459902372,122.844319988715)) ;
#68732=CARTESIAN_POINT('Ctrl Pts',(-18.3764719974847,34.3649803732812,122.282323158732)) ;
#68733=CARTESIAN_POINT('Ctrl Pts',(-18.5830265759983,34.1849912929184,122.50822539218)) ;
#68734=CARTESIAN_POINT('Ctrl Pts',(-18.8226102498659,34.3848756803401,121.998446004947)) ;
#68735=CARTESIAN_POINT('Ctrl Pts',(-18.9399371661432,34.2048865999772,122.281121677154)) ;
#68736=CARTESIAN_POINT('Ctrl Pts',(-19.3385786404572,34.4047689505077,121.882935209767)) ;
#68737=CARTESIAN_POINT('Ctrl Pts',(-19.3527127879478,34.2247798701449,122.188711677315)) ;
#68738=CARTESIAN_POINT('Ctrl Pts',(-19.864843872694,34.4247345431882,121.950781567567)) ;
#68739=CARTESIAN_POINT('Ctrl Pts',(-19.773725507496,34.2447454628253,122.242987830082)) ;
#68740=CARTESIAN_POINT('Ctrl Pts',(-20.3344600160615,34.444609866873,122.192739799094)) ;
#68741=CARTESIAN_POINT('Ctrl Pts',(-20.149420050782,34.2646207865101,122.436554544585)) ;
#68742=CARTESIAN_POINT('Ctrl Pts',(-20.6955112754201,34.464584929448,122.582004291072)) ;
#68743=CARTESIAN_POINT('Ctrl Pts',(-20.4382613889304,34.2845958490851,122.74796620737)) ;
#68744=CARTESIAN_POINT('Ctrl Pts',(-20.9010681970121,34.4845373390791,123.070845431308)) ;
#68745=CARTESIAN_POINT('Ctrl Pts',(-20.6027074986626,34.3045482587162,123.139039529433)) ;
#68746=CARTESIAN_POINT('Ctrl Pts',(-20.9283379623324,34.5043733933152,123.597346656962)) ;
#68747=CARTESIAN_POINT('Ctrl Pts',(-20.6245230859658,34.3243843129523,123.560242643287)) ;
#68748=CARTESIAN_POINT('Ctrl Pts',(-20.7737648833637,34.5243513047327,124.105329355223)) ;
#68749=CARTESIAN_POINT('Ctrl Pts',(-20.5008637718727,34.3443622243698,123.966628801619)) ;
#68750=CARTESIAN_POINT('Ctrl Pts',(-20.4555977349369,34.5442693542362,124.528394482397)) ;
#68751=CARTESIAN_POINT('Ctrl Pts',(-20.2463288803223,34.3642802738733,124.305081255519)) ;
#68752=CARTESIAN_POINT('Ctrl Pts',(-20.0139097341758,34.5641374980043,124.818008765311)) ;
#68753=CARTESIAN_POINT('Ctrl Pts',(-19.8929765031619,34.3841484176414,124.536772192443)) ;
#68754=CARTESIAN_POINT('Ctrl Pts',(-19.4952245290992,34.5841883545916,124.939780508264)) ;
#68755=CARTESIAN_POINT('Ctrl Pts',(-19.4780285056584,34.4041992742287,124.634188162972)) ;
#68756=CARTESIAN_POINT('Ctrl Pts',(-18.9729159061863,34.6039687910475,124.878612004196)) ;
#68757=CARTESIAN_POINT('Ctrl Pts',(-19.0601796451305,34.4239797106846,124.585251399659)) ;
#68758=CARTESIAN_POINT('Ctrl Pts',(-18.496759486199,34.6239988467253,124.640786108479)) ;
#68759=CARTESIAN_POINT('Ctrl Pts',(-18.6792557743103,34.4440097663624,124.394988854983)) ;
#68760=CARTESIAN_POINT('Ctrl Pts',(-18.1335792137849,34.6438799519001,124.256847057463)) ;
#68761=CARTESIAN_POINT('Ctrl Pts',(-18.3887122909116,34.4638908715372,124.087835457315)) ;
#68762=CARTESIAN_POINT('Ctrl Pts',(-17.9219139096296,34.6637604142679,123.772762991353)) ;
#68763=CARTESIAN_POINT('Ctrl Pts',(-18.2193820937176,34.483771333905,123.700566231009)) ;
#68764=CARTESIAN_POINT('Ctrl Pts',(-17.8881094855176,34.6837455614122,123.242649910961)) ;
#68765=CARTESIAN_POINT('Ctrl Pts',(-18.1923412744921,34.5037564810494,123.276475501805)) ;
#68766=CARTESIAN_POINT('Ctrl Pts',(-18.0366497415648,34.7036361399486,122.735276316463)) ;
#68767=CARTESIAN_POINT('Ctrl Pts',(-18.3111764212583,34.5236470595857,122.87057664201)) ;
#68768=CARTESIAN_POINT('Ctrl Pts',(-18.3487015779653,34.723530159823,122.308436690887)) ;
#68769=CARTESIAN_POINT('Ctrl Pts',(-18.5608208835814,34.5435410794601,122.529106268789)) ;
#68770=CARTESIAN_POINT('Ctrl Pts',(-18.7881430602527,34.7434516045494,122.013226846896)) ;
#68771=CARTESIAN_POINT('Ctrl Pts',(-18.9123763432651,34.5634625241865,122.292940896369)) ;
#68772=CARTESIAN_POINT('Ctrl Pts',(-19.3013427498124,34.7633497426048,121.884875817397)) ;
#68773=CARTESIAN_POINT('Ctrl Pts',(-19.3229374638322,34.583360662242,122.190263485441)) ;
#68774=CARTESIAN_POINT('Ctrl Pts',(-19.8317538659919,34.7834204978209,121.940822959894)) ;
#68775=CARTESIAN_POINT('Ctrl Pts',(-19.7472655742941,34.603431417458,122.235024637541)) ;
#68776=CARTESIAN_POINT('Ctrl Pts',(-20.3047188071783,34.8032060478722,122.170959918835)) ;
#68777=CARTESIAN_POINT('Ctrl Pts',(-20.1256368670043,34.6232169675093,122.419137989732)) ;
#68778=CARTESIAN_POINT('Ctrl Pts',(-20.6751904640124,34.8231891227495,122.55139832022)) ;
#68779=CARTESIAN_POINT('Ctrl Pts',(-20.4220114541107,34.6432000423866,122.72349136495)) ;
#68780=CARTESIAN_POINT('Ctrl Pts',(-20.8920819873269,34.8430982053954,123.034062768714)) ;
#68781=CARTESIAN_POINT('Ctrl Pts',(-20.5955208682009,34.6631091250326,123.109625335908)) ;
#68782=CARTESIAN_POINT('Ctrl Pts',(-20.9326680570592,34.8629567645182,123.560377307948)) ;
#68783=CARTESIAN_POINT('Ctrl Pts',(-20.6279870568241,34.6829676841553,123.53067592304)) ;
#68784=CARTESIAN_POINT('Ctrl Pts',(-20.7893451366516,34.8830002083569,124.073345382285)) ;
#68785=CARTESIAN_POINT('Ctrl Pts',(-20.5133192229244,34.703011127994,123.941055778839)) ;
#68786=CARTESIAN_POINT('Ctrl Pts',(-20.5344079580577,34.8995002730861,124.43033347796)) ;
#68787=CARTESIAN_POINT('Ctrl Pts',(-20.309383562949,34.7195111927232,124.226623694968)) ;
#68788=CARTESIAN_POINT('Ctrl Pts',(-20.2630356079764,34.912890012935,124.654232063007)) ;
#68789=CARTESIAN_POINT('Ctrl Pts',(-20.0922687245513,34.7329009325721,124.405758721467)) ;
#68790=CARTESIAN_POINT('Ctrl Pts',(-20.0376601532639,34.9227469141434,124.781982024209)) ;
#68791=CARTESIAN_POINT('Ctrl Pts',(-19.911970256192,34.7427578337805,124.507953327853)) ;
#68792=CARTESIAN_POINT('Ctrl Pts',(-19.7904462531825,34.9327384399899,124.870322609915)) ;
#68793=CARTESIAN_POINT('Ctrl Pts',(-19.7141969621559,34.752749359627,124.578624529211)) ;
#68794=CARTESIAN_POINT('Ctrl Pts',(-19.5333148830126,34.9426631204409,124.914209741491)) ;
#68795=CARTESIAN_POINT('Ctrl Pts',(-19.5084940323309,34.762674040078,124.613732529277)) ;
#68796=CARTESIAN_POINT('Ctrl Pts',(-19.2702905171994,34.9526737104853,124.912873328828)) ;
#68797=CARTESIAN_POINT('Ctrl Pts',(-19.2980655576572,34.7726846301224,124.61265864524)) ;
#68798=CARTESIAN_POINT('Ctrl Pts',(-18.9272936377873,34.9659329711889,124.851006430555)) ;
#68799=CARTESIAN_POINT('Ctrl Pts',(-19.0237133047444,34.7859438908261,124.563175229187)) ;
#68800=CARTESIAN_POINT('Ctrl Pts',(-18.606436005865,34.9792840463392,124.69972105366)) ;
#68801=CARTESIAN_POINT('Ctrl Pts',(-18.7669990812473,34.7992949659763,124.442141522519)) ;
#68802=CARTESIAN_POINT('Ctrl Pts',(-18.3413122765646,34.992490355574,124.475665673841)) ;
#68803=CARTESIAN_POINT('Ctrl Pts',(-18.5548921869106,34.8125012752111,124.262885113938)) ;
#68804=CARTESIAN_POINT('Ctrl Pts',(-18.1729444100433,35.0024771891643,124.274406568228)) ;
#68805=CARTESIAN_POINT('Ctrl Pts',(-18.4202016064083,34.8224881088014,124.101878384377)) ;
#68806=CARTESIAN_POINT('Ctrl Pts',(-18.0423683362087,35.0124299166604,124.047733829672)) ;
#68807=CARTESIAN_POINT('Ctrl Pts',(-18.3157421784876,34.8324408362975,123.920538559733)) ;
#68808=CARTESIAN_POINT('Ctrl Pts',(-17.9525123755645,35.022478013502,123.799470169266)) ;
#68809=CARTESIAN_POINT('Ctrl Pts',(-18.2438596889398,34.8424889331391,123.721927081998)) ;
#68810=CARTESIAN_POINT('Ctrl Pts',(-17.9077516294115,35.0323194703738,123.544724476242)) ;
#68811=CARTESIAN_POINT('Ctrl Pts',(-18.208053265257,34.8523303900109,123.518130066413)) ;
#68812=CARTESIAN_POINT('Ctrl Pts',(-17.9073445683786,35.0423057372873,123.282339109367)) ;
#68813=CARTESIAN_POINT('Ctrl Pts',(-18.2077298902901,34.8623166569244,123.308221845002)) ;
#68814=CARTESIAN_POINT('Ctrl Pts',(-17.9521637827218,35.0522423381877,123.025046666914)) ;
#68815=CARTESIAN_POINT('Ctrl Pts',(-18.2435874714704,34.8722532578248,123.10238833231)) ;
#68816=CARTESIAN_POINT('Ctrl Pts',(-18.0420906679866,35.0622922809748,122.776754559742)) ;
#68817=CARTESIAN_POINT('Ctrl Pts',(-18.3155310899466,34.8823032006119,122.903755461618)) ;
#68818=CARTESIAN_POINT('Ctrl Pts',(-18.1709996406622,35.0721424806605,122.552262724124)) ;
#68819=CARTESIAN_POINT('Ctrl Pts',(-18.4186601790438,34.8921534002976,122.724163199285)) ;
#68820=CARTESIAN_POINT('Ctrl Pts',(-18.3384352196694,35.0821153855926,122.350682137594)) ;
#68821=CARTESIAN_POINT('Ctrl Pts',(-18.5526103127129,34.9021263052297,122.562900239816)) ;
#68822=CARTESIAN_POINT('Ctrl Pts',(-18.5389407429953,35.0921137600722,122.180827804113)) ;
#68823=CARTESIAN_POINT('Ctrl Pts',(-18.7130161369838,34.9121246797094,122.427018525397)) ;
#68824=CARTESIAN_POINT('Ctrl Pts',(-18.7664484679922,35.1021339339422,122.048263316574)) ;
#68825=CARTESIAN_POINT('Ctrl Pts',(-18.8950234142683,34.9221448535794,122.320968904354)) ;
#68826=CARTESIAN_POINT('Ctrl Pts',(-19.0105165623716,35.1120349778842,121.958081319082)) ;
#68827=CARTESIAN_POINT('Ctrl Pts',(-19.0902785364057,34.9320458975213,122.24882546228)) ;
#68828=CARTESIAN_POINT('Ctrl Pts',(-19.2687227454526,35.1220237816085,121.910830619248)) ;
#68829=CARTESIAN_POINT('Ctrl Pts',(-19.2968438044793,34.9420347012456,122.211027113215)) ;
#68830=CARTESIAN_POINT('Ctrl Pts',(-19.5305882706686,35.1319892484403,121.909321300949)) ;
#68831=CARTESIAN_POINT('Ctrl Pts',(-19.5063361388599,34.9520001680775,122.209821901071)) ;
#68832=CARTESIAN_POINT('Ctrl Pts',(-19.7872767838356,35.1418928107133,121.952415553993)) ;
#68833=CARTESIAN_POINT('Ctrl Pts',(-19.7116863821234,34.9619037303504,122.244299447509)) ;
#68834=CARTESIAN_POINT('Ctrl Pts',(-20.0363461469721,35.1519534885913,122.040990349835)) ;
#68835=CARTESIAN_POINT('Ctrl Pts',(-19.9109411536517,34.9719644082284,122.315161388044)) ;
#68836=CARTESIAN_POINT('Ctrl Pts',(-20.2614426416287,35.1617937865408,122.168353377903)) ;
#68837=CARTESIAN_POINT('Ctrl Pts',(-20.0910169782063,34.9818047061779,122.417053562184)) ;
#68838=CARTESIAN_POINT('Ctrl Pts',(-20.4656690482286,35.1718567814502,122.33629520841)) ;
#68839=CARTESIAN_POINT('Ctrl Pts',(-20.2543967460004,34.9918677010873,122.551408735198)) ;
#68840=CARTESIAN_POINT('Ctrl Pts',(-20.6346269466373,35.1817510755973,122.533966500745)) ;
#68841=CARTESIAN_POINT('Ctrl Pts',(-20.389561223534,35.0017619952345,122.709546994155)) ;
#68842=CARTESIAN_POINT('Ctrl Pts',(-20.7679099510609,35.1916928732942,122.758634465352)) ;
#68843=CARTESIAN_POINT('Ctrl Pts',(-20.4961856757514,35.0117037929313,122.889282276775)) ;
#68844=CARTESIAN_POINT('Ctrl Pts',(-20.8608365588192,35.2016954508233,123.004554830575)) ;
#68845=CARTESIAN_POINT('Ctrl Pts',(-20.5705249456458,35.0217063704604,123.086019259422)) ;
#68846=CARTESIAN_POINT('Ctrl Pts',(-20.9093992123313,35.2117299147444,123.263726218813)) ;
#68847=CARTESIAN_POINT('Ctrl Pts',(-20.6093729389667,35.0317408343815,123.293356782246)) ;
#68848=CARTESIAN_POINT('Ctrl Pts',(-20.912575954229,35.2215760532655,123.522461220006)) ;
#68849=CARTESIAN_POINT('Ctrl Pts',(-20.6119121959131,35.0415869729026,123.500344358)) ;
#68850=CARTESIAN_POINT('Ctrl Pts',(-20.8707879748683,35.2315572265025,123.781384610257)) ;
#68851=CARTESIAN_POINT('Ctrl Pts',(-20.5784797854132,35.0515681461396,123.707482601004)) ;
#68852=CARTESIAN_POINT('Ctrl Pts',(-20.7848581741263,35.2415095204597,124.028409346698)) ;
#68853=CARTESIAN_POINT('Ctrl Pts',(-20.5097340530019,35.0615204400968,123.905101502577)) ;
#68854=CARTESIAN_POINT('Ctrl Pts',(-20.6570382603351,35.2515083155943,124.258005618651)) ;
#68855=CARTESIAN_POINT('Ctrl Pts',(-20.4074763796465,35.0715192352314,124.088777453895)) ;
#68856=CARTESIAN_POINT('Ctrl Pts',(-20.4902556612724,35.2615474238551,124.462394870675)) ;
#68857=CARTESIAN_POINT('Ctrl Pts',(-20.2740486420064,35.0815583434922,124.252287564926)) ;
#68858=CARTESIAN_POINT('Ctrl Pts',(-20.2951179160963,35.2713723652943,124.631484396849)) ;
#68859=CARTESIAN_POINT('Ctrl Pts',(-20.117937581225,35.0913832849314,124.387557244038)) ;
#68860=CARTESIAN_POINT('Ctrl Pts',(-20.0686559821828,35.2814270523687,124.767580615175)) ;
#68861=CARTESIAN_POINT('Ctrl Pts',(-19.9367669380912,35.1014379720058,124.496432562579)) ;
#68862=CARTESIAN_POINT('Ctrl Pts',(-19.8245654449264,35.2913698573088,124.860825828368)) ;
#68863=CARTESIAN_POINT('Ctrl Pts',(-19.74149402968,35.1113807769459,124.571026731217)) ;
#68864=CARTESIAN_POINT('Ctrl Pts',(-19.5691531625667,35.3012736433053,124.910862029586)) ;
#68865=CARTESIAN_POINT('Ctrl Pts',(-19.5371642509211,35.1212845629424,124.61105371151)) ;
#68866=CARTESIAN_POINT('Ctrl Pts',(-19.3052006854437,35.3113204598701,124.915700617854)) ;
#68867=CARTESIAN_POINT('Ctrl Pts',(-19.3260021502799,35.1313313795072,124.614922626619)) ;
#68868=CARTESIAN_POINT('Ctrl Pts',(-19.0482438728121,35.3212159793488,124.875474923149)) ;
#68869=CARTESIAN_POINT('Ctrl Pts',(-19.1204374586696,35.1412268989859,124.582740243431)) ;
#68870=CARTESIAN_POINT('Ctrl Pts',(-18.7981091918514,35.3312780646732,124.789853312718)) ;
#68871=CARTESIAN_POINT('Ctrl Pts',(-18.9203301991824,35.1512889843104,124.514241085553)) ;
#68872=CARTESIAN_POINT('Ctrl Pts',(-18.571557569673,35.3411207756312,124.664983089902)) ;
#68873=CARTESIAN_POINT('Ctrl Pts',(-18.7390904274587,35.1611316952683,124.4143435761)) ;
#68874=CARTESIAN_POINT('Ctrl Pts',(-18.3667589020139,35.3511114929372,124.500756432804)) ;
#68875=CARTESIAN_POINT('Ctrl Pts',(-18.5752527356648,35.1711224125743,124.282960925271)) ;
#68876=CARTESIAN_POINT('Ctrl Pts',(-18.1946758847601,35.3610395760338,124.304637787655)) ;
#68877=CARTESIAN_POINT('Ctrl Pts',(-18.4375879438694,35.1810504956709,124.126065105729)) ;
#68878=CARTESIAN_POINT('Ctrl Pts',(-18.0580530664321,35.3710275061455,124.080513754998)) ;
#68879=CARTESIAN_POINT('Ctrl Pts',(-18.3282912523427,35.1910384257827,123.946765097769)) ;
#68880=CARTESIAN_POINT('Ctrl Pts',(-17.9623826480587,35.3810633322728,123.83475626619)) ;
#68881=CARTESIAN_POINT('Ctrl Pts',(-18.2517565843422,35.20107425191,123.750158383688)) ;
#68882=CARTESIAN_POINT('Ctrl Pts',(-17.9113535514333,35.3909186693864,123.580830234499)) ;
#68883=CARTESIAN_POINT('Ctrl Pts',(-18.2109351630595,35.2109295890236,123.547017932825)) ;
#68884=CARTESIAN_POINT('Ctrl Pts',(-17.9046862415223,35.4009164042366,123.318213209581)) ;
#68885=CARTESIAN_POINT('Ctrl Pts',(-18.205602992744,35.2209273238737,123.336924392206)) ;
#68886=CARTESIAN_POINT('Ctrl Pts',(-17.9432873405184,35.4108243082211,123.060708970242)) ;
#68887=CARTESIAN_POINT('Ctrl Pts',(-18.2364854316828,35.2308352278582,123.130921769729)) ;
#68888=CARTESIAN_POINT('Ctrl Pts',(-18.0264553068263,35.4208353827695,122.811112169827)) ;
#68889=CARTESIAN_POINT('Ctrl Pts',(-18.3030212907696,35.2408463024066,122.931244865584)) ;
#68890=CARTESIAN_POINT('Ctrl Pts',(-18.1523789389796,35.4308632383051,122.579621476818)) ;
#68891=CARTESIAN_POINT('Ctrl Pts',(-18.403761694324,35.2508741579423,122.746053067434)) ;
#68892=CARTESIAN_POINT('Ctrl Pts',(-18.3134289650525,35.4407208322104,122.376725539727)) ;
#68893=CARTESIAN_POINT('Ctrl Pts',(-18.5326024658146,35.2607317518475,122.583737933796)) ;
#68894=CARTESIAN_POINT('Ctrl Pts',(-18.5102358433116,35.4507475190485,122.201520587918)) ;
#68895=CARTESIAN_POINT('Ctrl Pts',(-18.6900489765213,35.2707584386856,122.443575071446)) ;
#68896=CARTESIAN_POINT('Ctrl Pts',(-18.7348673255698,35.4607761882022,122.063678979707)) ;
#68897=CARTESIAN_POINT('Ctrl Pts',(-18.8697550564223,35.2807871078393,122.333303131403)) ;
#68898=CARTESIAN_POINT('Ctrl Pts',(-18.9753389392073,35.4706213964836,121.968264330612)) ;
#68899=CARTESIAN_POINT('Ctrl Pts',(-19.0621320757983,35.2906323161207,122.256973158654)) ;
#68900=CARTESIAN_POINT('Ctrl Pts',(-19.232344395239,35.4806120854467,121.914585662056)) ;
#68901=CARTESIAN_POINT('Ctrl Pts',(-19.2677365699942,35.3006230050839,122.214031608862)) ;
#68902=CARTESIAN_POINT('Ctrl Pts',(-19.4960145845419,35.490649961729,121.906896220203)) ;
#68903=CARTESIAN_POINT('Ctrl Pts',(-19.4786728720695,35.3106608813661,122.207881552385)) ;
#68904=CARTESIAN_POINT('Ctrl Pts',(-19.7520613231325,35.5004943393712,121.943923950967)) ;
#68905=CARTESIAN_POINT('Ctrl Pts',(-19.6835091319941,35.3205052590084,122.237504996433)) ;
#68906=CARTESIAN_POINT('Ctrl Pts',(-20.0014137029836,35.5104791437627,122.025494346825)) ;
#68907=CARTESIAN_POINT('Ctrl Pts',(-19.8829904412346,35.3304900633998,122.302762488264)) ;
#68908=CARTESIAN_POINT('Ctrl Pts',(-20.2318815338735,35.5204186739812,122.148494733348)) ;
#68909=CARTESIAN_POINT('Ctrl Pts',(-20.0673637209045,35.3404295936183,122.401163717447)) ;
#68910=CARTESIAN_POINT('Ctrl Pts',(-20.4394809697131,35.5304583620181,122.311280393352)) ;
#68911=CARTESIAN_POINT('Ctrl Pts',(-20.2334425657068,35.3504692816552,122.53139333392)) ;
#68912=CARTESIAN_POINT('Ctrl Pts',(-20.6131244207075,35.5403466513864,122.504619288811)) ;
#68913=CARTESIAN_POINT('Ctrl Pts',(-20.3723558935254,35.3603575710235,122.686064744329)) ;
#68914=CARTESIAN_POINT('Ctrl Pts',(-20.7523694041922,35.5503357750712,122.72713725888)) ;
#68915=CARTESIAN_POINT('Ctrl Pts',(-20.4837508097204,35.3703466947083,122.864079588493)) ;
#68916=CARTESIAN_POINT('Ctrl Pts',(-20.8503882560538,35.5602957847458,122.969824688647)) ;
#68917=CARTESIAN_POINT('Ctrl Pts',(-20.5621646481119,35.3803067043829,123.058229659203)) ;
#68918=CARTESIAN_POINT('Ctrl Pts',(-20.9050630989688,35.57019621445,123.224196430447)) ;
#68919=CARTESIAN_POINT('Ctrl Pts',(-20.6059033396929,35.3902071340872,123.261726591413)) ;
#68920=CARTESIAN_POINT('Ctrl Pts',(-20.9148664709882,35.5802392958568,123.487924566708)) ;
#68921=CARTESIAN_POINT('Ctrl Pts',(-20.6137449783066,35.4002502154939,123.472709296187)) ;
#68922=CARTESIAN_POINT('Ctrl Pts',(-20.8792189654738,35.5901466897644,123.74584291802)) ;
#68923=CARTESIAN_POINT('Ctrl Pts',(-20.5852260111583,35.4101576094016,123.679043182914)) ;
#68924=CARTESIAN_POINT('Ctrl Pts',(-20.7989552795368,35.6001584207536,123.996400804876)) ;
#68925=CARTESIAN_POINT('Ctrl Pts',(-20.5210141652758,35.4201693403907,123.879489165425)) ;
#68926=CARTESIAN_POINT('Ctrl Pts',(-20.6756899073301,35.6101906384684,124.229454654533)) ;
#68927=CARTESIAN_POINT('Ctrl Pts',(-20.4224008782605,35.4302015581055,124.065931815006)) ;
#68928=CARTESIAN_POINT('Ctrl Pts',(-20.5170202759795,35.6200431477146,124.434034154075)) ;
#68929=CARTESIAN_POINT('Ctrl Pts',(-20.2954650100176,35.4400540673517,124.229594006282)) ;
#68930=CARTESIAN_POINT('Ctrl Pts',(-20.3237177193579,35.6300010842576,124.610433802406)) ;
#68931=CARTESIAN_POINT('Ctrl Pts',(-20.1408227029007,35.4500120038947,124.370712879431)) ;
#68932=CARTESIAN_POINT('Ctrl Pts',(-20.1006943914862,35.6400399542659,124.751315017522)) ;
#68933=CARTESIAN_POINT('Ctrl Pts',(-19.9624034408403,35.460050873903,124.483417150071)) ;
#68934=CARTESIAN_POINT('Ctrl Pts',(-19.8607559657353,35.6499131094241,124.850152762012)) ;
#68935=CARTESIAN_POINT('Ctrl Pts',(-19.7704532300316,35.4699240290612,124.562486266306)) ;
#68936=CARTESIAN_POINT('Ctrl Pts',(-19.6022411196816,35.6599863842738,124.906856510779)) ;
#68937=CARTESIAN_POINT('Ctrl Pts',(-19.5636408438425,35.4799973039109,124.607848540031)) ;
#68938=CARTESIAN_POINT('Ctrl Pts',(-19.3443505908473,35.6698067014512,124.917880380727)) ;
#68939=CARTESIAN_POINT('Ctrl Pts',(-19.3573296329594,35.4898176210883,124.616666850261)) ;
#68940=CARTESIAN_POINT('Ctrl Pts',(-19.0818227174019,35.6798853872447,124.883323751729)) ;
#68941=CARTESIAN_POINT('Ctrl Pts',(-19.147307048226,35.4998963068818,124.589020826947)) ;
#68942=CARTESIAN_POINT('Ctrl Pts',(-18.8348266453424,35.6897368986278,124.805553629414)) ;
#68943=CARTESIAN_POINT('Ctrl Pts',(-18.9497113939592,35.5097478182649,124.526804423587)) ;
#68944=CARTESIAN_POINT('Ctrl Pts',(-18.5999081950905,35.6998103449344,124.683638544709)) ;
#68945=CARTESIAN_POINT('Ctrl Pts',(-18.7617765978972,35.5198212645716,124.429271661873)) ;
#68946=CARTESIAN_POINT('Ctrl Pts',(-18.3945197612094,35.7096516200591,124.526430434708)) ;
#68947=CARTESIAN_POINT('Ctrl Pts',(-18.5974671222276,35.5296625396963,124.303505384468)) ;
#68948=CARTESIAN_POINT('Ctrl Pts',(-18.2164254320828,35.7196367197159,124.333759479541)) ;
#68949=CARTESIAN_POINT('Ctrl Pts',(-18.4549921099954,35.539647639353,124.149368519473)) ;
#68950=CARTESIAN_POINT('Ctrl Pts',(-18.0744564633631,35.7296441958502,124.112362113073)) ;
#68951=CARTESIAN_POINT('Ctrl Pts',(-18.3414173794509,35.5496551154873,123.972250409102)) ;
#68952=CARTESIAN_POINT('Ctrl Pts',(-17.9737377684653,35.7395667835592,123.871857563518)) ;
#68953=CARTESIAN_POINT('Ctrl Pts',(-18.2608430645821,35.5595777031963,123.779847173338)) ;
#68954=CARTESIAN_POINT('Ctrl Pts',(-17.915514233427,35.7495533878325,123.61593526692)) ;
#68955=CARTESIAN_POINT('Ctrl Pts',(-18.2142645957526,35.5695643074696,123.575109448264)) ;
#68956=CARTESIAN_POINT('Ctrl Pts',(-17.9030386020177,35.7595935161666,123.352407710946)) ;
#68957=CARTESIAN_POINT('Ctrl Pts',(-18.2042845372192,35.5796044358037,123.364287232758)) ;
#68958=CARTESIAN_POINT('Ctrl Pts',(-17.9352873093838,35.7694329507,123.095829361004)) ;
#68959=CARTESIAN_POINT('Ctrl Pts',(-18.2300836623065,35.5894438703371,123.159025769629)) ;
#68960=CARTESIAN_POINT('Ctrl Pts',(-18.0131110083021,35.779497005191,122.843100123072)) ;
#68961=CARTESIAN_POINT('Ctrl Pts',(-18.2923429533616,35.5995079248281,122.956842160068)) ;
#68962=CARTESIAN_POINT('Ctrl Pts',(-18.1316925352344,35.7893879244282,122.611771524711)) ;
#68963=CARTESIAN_POINT('Ctrl Pts',(-18.3872080467958,35.6093988440653,122.771780155463)) ;
#68964=CARTESIAN_POINT('Ctrl Pts',(-18.2897713917017,35.7993799177342,122.402124132987)) ;
#68965=CARTESIAN_POINT('Ctrl Pts',(-18.5136711422251,35.6193908373713,122.604062465028)) ;
#68966=CARTESIAN_POINT('Ctrl Pts',(-18.4814613118421,35.8093427816935,122.223804692162)) ;
#68967=CARTESIAN_POINT('Ctrl Pts',(-18.6670229513666,35.6293537013306,122.461407311499)) ;
#68968=CARTESIAN_POINT('Ctrl Pts',(-18.6995746479886,35.8192470415113,122.081746101379)) ;
#68969=CARTESIAN_POINT('Ctrl Pts',(-18.8415130103748,35.6392579611484,122.347760879673)) ;
#68970=CARTESIAN_POINT('Ctrl Pts',(-18.9428567780933,35.8293075320827,121.978340523878)) ;
#68971=CARTESIAN_POINT('Ctrl Pts',(-19.0361390123414,35.6493184517198,122.265036395034)) ;
#68972=CARTESIAN_POINT('Ctrl Pts',(-19.1947540652062,35.8391478817137,121.919707183759)) ;
#68973=CARTESIAN_POINT('Ctrl Pts',(-19.2376556973774,35.6591588013508,122.218129998438)) ;
#68974=CARTESIAN_POINT('Ctrl Pts',(-19.4587582959314,35.8492108572037,121.905070980687)) ;
#68975=CARTESIAN_POINT('Ctrl Pts',(-19.448859376931,35.6692217768408,122.206420948279)) ;
#68976=CARTESIAN_POINT('Ctrl Pts',(-19.716930430725,35.8591051773471,121.936190237955)) ;
#68977=CARTESIAN_POINT('Ctrl Pts',(-19.6553962747645,35.6791160969842,122.231316240817)) ;
#68978=CARTESIAN_POINT('Ctrl Pts',(-19.9671129941824,35.8690468904787,122.011332156098)) ;
#68979=CARTESIAN_POINT('Ctrl Pts',(-19.8555418925478,35.6890578101158,122.291429441969)) ;
#68980=CARTESIAN_POINT('Ctrl Pts',(-20.2020024297301,35.8790497802728,122.129427167199)) ;
#68981=CARTESIAN_POINT('Ctrl Pts',(-20.0434534559638,35.69906069991,122.385905206129)) ;
#68982=CARTESIAN_POINT('Ctrl Pts',(-20.4132559197395,35.8890896374333,122.28744132461)) ;
#68983=CARTESIAN_POINT('Ctrl Pts',(-20.2124564260292,35.7091005570704,122.512316537818)) ;
#68984=CARTESIAN_POINT('Ctrl Pts',(-20.5904446049363,35.8989138182709,122.475235422024)) ;
#68985=CARTESIAN_POINT('Ctrl Pts',(-20.3542066813593,35.7189247379081,122.662550716544)) ;
#68986=CARTESIAN_POINT('Ctrl Pts',(-20.7359772784035,35.9089707917741,122.695816923843)) ;
#68987=CARTESIAN_POINT('Ctrl Pts',(-20.4706332561571,35.7289817114113,122.839015952767)) ;
#68988=CARTESIAN_POINT('Ctrl Pts',(-20.8393638309279,35.9188989159612,122.935375322683)) ;
#68989=CARTESIAN_POINT('Ctrl Pts',(-20.5533424999389,35.7389098355983,123.030662030176)) ;
#68990=CARTESIAN_POINT('Ctrl Pts',(-20.9004170383969,35.9288526110346,123.189725205683)) ;
#68991=CARTESIAN_POINT('Ctrl Pts',(-20.602185386523,35.7488635306717,123.234141416124)) ;
#68992=CARTESIAN_POINT('Ctrl Pts',(-20.9161514803797,35.9388988046099,123.453256665995)) ;
#68993=CARTESIAN_POINT('Ctrl Pts',(-20.6147732911417,35.758909724247,123.444966757205)) ;
#68994=CARTESIAN_POINT('Ctrl Pts',(-20.8867329496708,35.9487469069698,123.710376268567)) ;
#68995=CARTESIAN_POINT('Ctrl Pts',(-20.5912389928801,35.7687578266069,123.650661374287)) ;
#68996=CARTESIAN_POINT('Ctrl Pts',(-20.813048468652,35.9587084951974,123.961560575043)) ;
#68997=CARTESIAN_POINT('Ctrl Pts',(-20.5322920915651,35.7787194148345,123.851608640381)) ;
#68998=CARTESIAN_POINT('Ctrl Pts',(-20.6957786698797,35.9687371653537,124.19759210035)) ;
#68999=CARTESIAN_POINT('Ctrl Pts',(-20.4384766850489,35.7887480849908,124.04043416191)) ;
#69000=CARTESIAN_POINT('Ctrl Pts',(-20.5412377893036,35.9786474682354,124.407201312219)) ;
#69001=CARTESIAN_POINT('Ctrl Pts',(-20.3148448330596,35.7986583878725,124.208121289199)) ;
#69002=CARTESIAN_POINT('Ctrl Pts',(-20.3526398125085,35.9885823520433,124.587747365873)) ;
#69003=CARTESIAN_POINT('Ctrl Pts',(-20.1639673252218,35.8085932716804,124.352558280755)) ;
#69004=CARTESIAN_POINT('Ctrl Pts',(-20.1331135059456,35.9986234937339,124.734141809642)) ;
#69005=CARTESIAN_POINT('Ctrl Pts',(-19.9883465163358,35.8186344133711,124.469674459931)) ;
#69006=CARTESIAN_POINT('Ctrl Pts',(-19.8952608881985,36.0085106148979,124.838745840386)) ;
#69007=CARTESIAN_POINT('Ctrl Pts',(-19.7980654626942,35.828521534535,124.553357985807)) ;
#69008=CARTESIAN_POINT('Ctrl Pts',(-19.6403085962477,36.0185029577464,124.901535971408)) ;
#69009=CARTESIAN_POINT('Ctrl Pts',(-19.5941039789621,35.8385138773836,124.603590829665)) ;
#69010=CARTESIAN_POINT('Ctrl Pts',(-19.3794454821469,36.0284512589704,124.918954868183)) ;
#69011=CARTESIAN_POINT('Ctrl Pts',(-19.3854139711554,35.8484621786075,124.617526697189)) ;
#69012=CARTESIAN_POINT('Ctrl Pts',(-19.1197882532334,36.0383888366525,124.8912260194)) ;
#69013=CARTESIAN_POINT('Ctrl Pts',(-19.1776886066464,35.8583997562896,124.595344542413)) ;
#69014=CARTESIAN_POINT('Ctrl Pts',(-18.8675463523897,36.0483754111031,124.818724120264)) ;
#69015=CARTESIAN_POINT('Ctrl Pts',(-18.9758950062236,35.8683863307402,124.537343974835)) ;
#69016=CARTESIAN_POINT('Ctrl Pts',(-18.6308789216368,36.0584042210115,124.702775017872)) ;
#69017=CARTESIAN_POINT('Ctrl Pts',(-18.7865606156517,35.8784151406487,124.444585433762)) ;
#69018=CARTESIAN_POINT('Ctrl Pts',(-18.4209855121877,36.0682825423183,124.550028242115)) ;
#69019=CARTESIAN_POINT('Ctrl Pts',(-18.6186460335251,35.8882934619554,124.322389261554)) ;
#69020=CARTESIAN_POINT('Ctrl Pts',(-18.2382837456184,36.0782741896657,124.361434085726)) ;
#69021=CARTESIAN_POINT('Ctrl Pts',(-18.4724839618908,35.8982851093029,124.17151478619)) ;
#69022=CARTESIAN_POINT('Ctrl Pts',(-18.0909304837619,36.0883087131035,124.142763989122)) ;
#69023=CARTESIAN_POINT('Ctrl Pts',(-18.3546005264068,35.9083196327406,123.996579163665)) ;
#69024=CARTESIAN_POINT('Ctrl Pts',(-17.9851026047473,36.0981720699821,123.906123266323)) ;
#69025=CARTESIAN_POINT('Ctrl Pts',(-18.2699376258738,35.9181829896192,123.807267861114)) ;
#69026=CARTESIAN_POINT('Ctrl Pts',(-17.9206102595099,36.1082422966624,123.649496524002)) ;
#69027=CARTESIAN_POINT('Ctrl Pts',(-18.2183426310434,35.9282532162995,123.601966434206)) ;
#69028=CARTESIAN_POINT('Ctrl Pts',(-17.9020958099089,36.1180846047971,123.391502808904)) ;
#69029=CARTESIAN_POINT('Ctrl Pts',(-18.2035300751442,35.9380955244342,123.39557257472)) ;
#69030=CARTESIAN_POINT('Ctrl Pts',(-17.9280157514707,36.1280453368205,123.131037798645)) ;
#69031=CARTESIAN_POINT('Ctrl Pts',(-18.2242647137395,35.9480562564576,123.187200762251)) ;
#69032=CARTESIAN_POINT('Ctrl Pts',(-17.999816726095,36.1380832260186,122.877221984986)) ;
#69033=CARTESIAN_POINT('Ctrl Pts',(-18.2817043938246,35.9580941456557,122.984147689638)) ;
#69034=CARTESIAN_POINT('Ctrl Pts',(-18.1123123668843,36.1479575089374,122.643353698666)) ;
#69035=CARTESIAN_POINT('Ctrl Pts',(-18.3716994042814,35.9679684285746,122.797053236207)) ;
#69036=CARTESIAN_POINT('Ctrl Pts',(-18.2666755578384,36.1580272535549,122.428462610188)) ;
#69037=CARTESIAN_POINT('Ctrl Pts',(-18.4951890841048,35.978038173192,122.625139394901)) ;
#69038=CARTESIAN_POINT('Ctrl Pts',(-18.4515040641022,36.1678605639005,122.247839904849)) ;
#69039=CARTESIAN_POINT('Ctrl Pts',(-18.6430502466827,35.9878714835377,122.480641013743)) ;
#69040=CARTESIAN_POINT('Ctrl Pts',(-18.6687131962433,36.1778908072532,122.098528505516)) ;
#69041=CARTESIAN_POINT('Ctrl Pts',(-18.8168167817684,35.9979017268903,122.361190651918)) ;
#69042=CARTESIAN_POINT('Ctrl Pts',(-18.9089342117129,36.1879230952316,121.98989079608)) ;
#69043=CARTESIAN_POINT('Ctrl Pts',(-19.0089931242432,36.0079340148687,122.274279275505)) ;
#69044=CARTESIAN_POINT('Ctrl Pts',(-19.1589917224903,36.1977502716997,121.925355327248)) ;
#69045=CARTESIAN_POINT('Ctrl Pts',(-19.2090377774814,36.0177611913368,122.222649778263)) ;
#69046=CARTESIAN_POINT('Ctrl Pts',(-19.4210472098018,36.2077556545666,121.904313326992)) ;
#69047=CARTESIAN_POINT('Ctrl Pts',(-19.4186819756106,36.0277665742037,122.205814653997)) ;
#69048=CARTESIAN_POINT('Ctrl Pts',(-19.6822546897857,36.2177382935593,121.929130110005)) ;
#69049=CARTESIAN_POINT('Ctrl Pts',(-19.6276479311042,36.0377492131964,122.225666559862)) ;
#69050=CARTESIAN_POINT('Ctrl Pts',(-19.9365810271852,36.2277823606959,121.999644910744)) ;
#69051=CARTESIAN_POINT('Ctrl Pts',(-19.8311095076827,36.047793280333,122.282077034315)) ;
#69052=CARTESIAN_POINT('Ctrl Pts',(-20.1697398906336,36.2376035794999,122.110337795579)) ;
#69053=CARTESIAN_POINT('Ctrl Pts',(-20.0176363566891,36.057614499137,122.370629526365)) ;
#69054=CARTESIAN_POINT('Ctrl Pts',(-20.3851350977547,36.247640418438,122.262557053081)) ;
#69055=CARTESIAN_POINT('Ctrl Pts',(-20.1899535516625,36.0676513380751,122.492403621598)) ;
#69056=CARTESIAN_POINT('Ctrl Pts',(-20.5700735002195,36.2576648305357,122.450169309994)) ;
#69057=CARTESIAN_POINT('Ctrl Pts',(-20.3379053729967,36.0776757501728,122.64249237106)) ;
#69058=CARTESIAN_POINT('Ctrl Pts',(-20.7175254012894,36.267516914941,122.662985785925)) ;
#69059=CARTESIAN_POINT('Ctrl Pts',(-20.4558677751605,36.0875278345781,122.812743960038)) ;
#69060=CARTESIAN_POINT('Ctrl Pts',(-20.827658912847,36.2775078116842,122.901285416374)) ;
#69061=CARTESIAN_POINT('Ctrl Pts',(-20.5439760743343,36.0975187313213,123.003382825012)) ;
#69062=CARTESIAN_POINT('Ctrl Pts',(-20.894433698142,36.2874258035851,123.153253367672)) ;
#69063=CARTESIAN_POINT('Ctrl Pts',(-20.597397457909,36.1074367232222,123.204956301286)) ;
#69064=CARTESIAN_POINT('Ctrl Pts',(-20.9167470714456,36.2974539190421,123.415814568147)) ;
#69065=CARTESIAN_POINT('Ctrl Pts',(-20.6152498951296,36.1174648386792,123.415005141595)) ;
#69066=CARTESIAN_POINT('Ctrl Pts',(-20.8935762347595,36.3073390949842,123.674557784478)) ;
#69067=CARTESIAN_POINT('Ctrl Pts',(-20.5967150310461,36.1273500146213,123.621999285867)) ;
#69068=CARTESIAN_POINT('Ctrl Pts',(-20.8257335492576,36.3173284533911,123.928155184694)) ;
#69069=CARTESIAN_POINT('Ctrl Pts',(-20.5424427145472,36.1373393730282,123.824877566207)) ;
#69070=CARTESIAN_POINT('Ctrl Pts',(-20.7138111338408,36.3273696009714,124.167113009814)) ;
#69071=CARTESIAN_POINT('Ctrl Pts',(-20.4529063575782,36.1473805206085,124.016044644643)) ;
#69072=CARTESIAN_POINT('Ctrl Pts',(-20.5656005075822,36.3372022239778,124.378768633685)) ;
#69073=CARTESIAN_POINT('Ctrl Pts',(-20.334339803994,36.157213143615,124.185369574841)) ;
#69074=CARTESIAN_POINT('Ctrl Pts',(-20.3804184420739,36.3471962950886,124.564996698335)) ;
#69075=CARTESIAN_POINT('Ctrl Pts',(-20.1861956033881,36.1672072147257,124.334353335145)) ;
#69076=CARTESIAN_POINT('Ctrl Pts',(-20.1646550508293,36.3572249527295,124.716351716207)) ;
#69077=CARTESIAN_POINT('Ctrl Pts',(-20.013585958757,36.1772358723666,124.455438891468)) ;
#69078=CARTESIAN_POINT('Ctrl Pts',(-19.9294697798766,36.3671092789223,124.82658534845)) ;
#69079=CARTESIAN_POINT('Ctrl Pts',(-19.8254390212486,36.1871201985594,124.543627316612)) ;
#69080=CARTESIAN_POINT('Ctrl Pts',(-19.6767994745705,36.3770750224129,124.895495364823)) ;
#69081=CARTESIAN_POINT('Ctrl Pts',(-19.6233034862338,36.19708594205,124.598757213134)) ;
#69082=CARTESIAN_POINT('Ctrl Pts',(-19.4143489319624,36.3871034015441,124.91925636217)) ;
#69083=CARTESIAN_POINT('Ctrl Pts',(-19.4133432160735,36.2071143211812,124.617767958243)) ;
#69084=CARTESIAN_POINT('Ctrl Pts',(-19.1550206095445,36.397004247751,124.897758003346)) ;
#69085=CARTESIAN_POINT('Ctrl Pts',(-19.2058807986506,36.2170151673881,124.600571300824)) ;
#69086=CARTESIAN_POINT('Ctrl Pts',(-18.8994442732755,36.4070629051681,124.830453416065)) ;
#69087=CARTESIAN_POINT('Ctrl Pts',(-19.0014191286445,36.2270738248052,124.546729537339)) ;
#69088=CARTESIAN_POINT('Ctrl Pts',(-18.6640416210879,36.41692046795,124.722218749263)) ;
#69089=CARTESIAN_POINT('Ctrl Pts',(-18.8130966335472,36.2369313875871,124.460143863879)) ;
#69090=CARTESIAN_POINT('Ctrl Pts',(-18.4464240794683,36.4269888705032,124.571792635111)) ;
#69091=CARTESIAN_POINT('Ctrl Pts',(-18.6390013333269,36.2469997901403,124.339804589422)) ;
#69092=CARTESIAN_POINT('Ctrl Pts',(-18.2621870024575,36.4368442692428,124.389737932051)) ;
#69093=CARTESIAN_POINT('Ctrl Pts',(-18.4916105893428,36.2568551888799,124.194162632583)) ;
#69094=CARTESIAN_POINT('Ctrl Pts',(-18.1096139658518,36.4468391363167,124.175952224907)) ;
#69095=CARTESIAN_POINT('Ctrl Pts',(-18.3695504720034,36.2668500559538,124.023135369185)) ;
#69096=CARTESIAN_POINT('Ctrl Pts',(-17.9965739248701,36.4568704313002,123.937801266144)) ;
#69097=CARTESIAN_POINT('Ctrl Pts',(-18.2791165693549,36.2768813509373,123.832615491336)) ;
#69098=CARTESIAN_POINT('Ctrl Pts',(-17.9273507223424,36.4667369560267,123.68792118455)) ;
#69099=CARTESIAN_POINT('Ctrl Pts',(-18.2237360813941,36.2867478756638,123.632712386933)) ;
#69100=CARTESIAN_POINT('Ctrl Pts',(-17.9018470654154,36.4767244267224,123.426734881173)) ;
#69101=CARTESIAN_POINT('Ctrl Pts',(-18.2033310225224,36.2967353463596,123.423763651116)) ;
#69102=CARTESIAN_POINT('Ctrl Pts',(-17.9218551058738,36.4866691862863,123.166123729046)) ;
#69103=CARTESIAN_POINT('Ctrl Pts',(-18.2193352864995,36.3066801059234,123.215274750521)) ;
#69104=CARTESIAN_POINT('Ctrl Pts',(-17.9876098911621,36.4967147422351,122.910487765929)) ;
#69105=CARTESIAN_POINT('Ctrl Pts',(-18.2719370358106,36.3167256618723,123.010765429301)) ;
#69106=CARTESIAN_POINT('Ctrl Pts',(-18.0945065089563,36.5065743306102,122.674433491217)) ;
#69107=CARTESIAN_POINT('Ctrl Pts',(-18.3574522130804,36.3265852502474,122.821921426848)) ;
#69108=CARTESIAN_POINT('Ctrl Pts',(-18.2424940102238,36.5165752857463,122.457296954355)) ;
#69109=CARTESIAN_POINT('Ctrl Pts',(-18.4758403558108,36.3365862053834,122.648211013651)) ;
#69110=CARTESIAN_POINT('Ctrl Pts',(-18.4240741922966,36.5264795130239,122.270772500049)) ;
#69111=CARTESIAN_POINT('Ctrl Pts',(-18.6211027732019,36.346490432661,122.498990059894)) ;
#69112=CARTESIAN_POINT('Ctrl Pts',(-18.6381179777294,36.536521589919,122.116476705951)) ;
#69113=CARTESIAN_POINT('Ctrl Pts',(-18.7923365002083,36.3565325095561,122.375551632485)) ;
#69114=CARTESIAN_POINT('Ctrl Pts',(-18.8725385168482,36.5464292026052,122.003075302597)) ;
#69115=CARTESIAN_POINT('Ctrl Pts',(-18.979871801407,36.3664401222423,122.284828592145)) ;
#69116=CARTESIAN_POINT('Ctrl Pts',(-19.1267156102874,36.5564837332209,121.931052177972)) ;
#69117=CARTESIAN_POINT('Ctrl Pts',(-19.1832128661274,36.376494652858,122.227207955336)) ;
#69118=CARTESIAN_POINT('Ctrl Pts',(-19.3845283469667,36.5663445197698,121.904614760594)) ;
#69119=CARTESIAN_POINT('Ctrl Pts',(-19.3894626144026,36.3863554394069,122.206055828326)) ;
#69120=CARTESIAN_POINT('Ctrl Pts',(-19.646459660601,36.5763382748409,121.923105823683)) ;
#69121=CARTESIAN_POINT('Ctrl Pts',(-19.5990077631151,36.396349194478,122.220846431411)) ;
#69122=CARTESIAN_POINT('Ctrl Pts',(-19.8995693751158,36.5862636350808,121.986256533974)) ;
#69123=CARTESIAN_POINT('Ctrl Pts',(-19.8014959764349,36.406274554718,122.271364795615)) ;
#69124=CARTESIAN_POINT('Ctrl Pts',(-20.1402663825485,36.5962915644761,122.093453651258)) ;
#69125=CARTESIAN_POINT('Ctrl Pts',(-19.9940544515842,36.4163024841132,122.357120413461)) ;
#69126=CARTESIAN_POINT('Ctrl Pts',(-20.3558196617263,36.6061778312754,122.23855197328)) ;
#69127=CARTESIAN_POINT('Ctrl Pts',(-20.1664982539507,36.4261887509125,122.473197150911)) ;
#69128=CARTESIAN_POINT('Ctrl Pts',(-20.5456928031172,36.6162096001737,122.421371062193)) ;
#69129=CARTESIAN_POINT('Ctrl Pts',(-20.3183982921077,36.4362205198108,122.619450762827)) ;
#69130=CARTESIAN_POINT('Ctrl Pts',(-20.6988722845905,36.6260911960173,122.631115950227)) ;
#69131=CARTESIAN_POINT('Ctrl Pts',(-20.4409436684768,36.4461021156544,122.787245289088)) ;
#69132=CARTESIAN_POINT('Ctrl Pts',(-20.815415738362,36.6361530814852,122.868418182703)) ;
#69133=CARTESIAN_POINT('Ctrl Pts',(-20.5341804158425,36.4561640011224,122.97708607685)) ;
#69134=CARTESIAN_POINT('Ctrl Pts',(-20.8875930298801,36.6460105155041,123.11723735423)) ;
#69135=CARTESIAN_POINT('Ctrl Pts',(-20.5919244479909,36.4660214351412,123.176140562993)) ;
#69136=CARTESIAN_POINT('Ctrl Pts',(-20.9163988743177,36.6560037585461,123.37823043788)) ;
#69137=CARTESIAN_POINT('Ctrl Pts',(-20.6149712081136,36.4760146781832,123.384935555596)) ;
#69138=CARTESIAN_POINT('Ctrl Pts',(-20.8995719078508,36.6659345194324,123.638673612031)) ;
#69139=CARTESIAN_POINT('Ctrl Pts',(-20.6015124065235,36.4859454390695,123.593287223642)) ;
#69140=CARTESIAN_POINT('Ctrl Pts',(-20.8168446966216,36.6792835116296,123.979609103864)) ;
#69141=CARTESIAN_POINT('Ctrl Pts',(-20.535330876497,36.4992944312667,123.866051291918)) ;
#69142=CARTESIAN_POINT('Ctrl Pts',(-20.6476556408436,36.692551884446,124.288994177467)) ;
#69143=CARTESIAN_POINT('Ctrl Pts',(-20.3999608846557,36.5125628040832,124.113578703363)) ;
#69144=CARTESIAN_POINT('Ctrl Pts',(-20.4070652076398,36.7058348258304,124.541941671544)) ;
#69145=CARTESIAN_POINT('Ctrl Pts',(-20.2075187930554,36.5258457454675,124.31590241707)) ;
#69146=CARTESIAN_POINT('Ctrl Pts',(-20.1946380684897,36.7158776116726,124.698516250031)) ;
#69147=CARTESIAN_POINT('Ctrl Pts',(-20.0375727496872,36.5358885313097,124.441171067068)) ;
#69148=CARTESIAN_POINT('Ctrl Pts',(-19.9628921814832,36.7257275542247,124.813842499232)) ;
#69149=CARTESIAN_POINT('Ctrl Pts',(-19.8521787603597,36.5457384738618,124.53343231864)) ;
#69150=CARTESIAN_POINT('Ctrl Pts',(-19.7111366687982,36.7357247871437,124.888900023742)) ;
#69151=CARTESIAN_POINT('Ctrl Pts',(-19.6507730800588,36.5557357067808,124.593480421543)) ;
#69152=CARTESIAN_POINT('Ctrl Pts',(-19.4496388355441,36.7457396824782,124.918754107173)) ;
#69153=CARTESIAN_POINT('Ctrl Pts',(-19.4415808798337,36.5657506021153,124.617367625246)) ;
#69154=CARTESIAN_POINT('Ctrl Pts',(-19.1023419164485,36.7589793591164,124.897941856105)) ;
#69155=CARTESIAN_POINT('Ctrl Pts',(-19.163714991499,36.5789902787535,124.600711280948)) ;
#69156=CARTESIAN_POINT('Ctrl Pts',(-18.6847931249913,36.7755265835217,124.759912521952)) ;
#69157=CARTESIAN_POINT('Ctrl Pts',(-18.8297169408902,36.5955375031589,124.490312244877)) ;
#69158=CARTESIAN_POINT('Ctrl Pts',(-18.3371603330514,36.7921740206528,124.486198909286)) ;
#69159=CARTESIAN_POINT('Ctrl Pts',(-18.5515569759396,36.6121849402899,124.27129948126)) ;
#69160=CARTESIAN_POINT('Ctrl Pts',(-18.1282776888068,36.805463518131,124.206288377136)) ;
#69161=CARTESIAN_POINT('Ctrl Pts',(-18.3844875071243,36.6254744377682,124.047410080626)) ;
#69162=CARTESIAN_POINT('Ctrl Pts',(-18.0108710102114,36.8153369259534,123.974907927257)) ;
#69163=CARTESIAN_POINT('Ctrl Pts',(-18.2905523869042,36.6353478455905,123.86229865506)) ;
#69164=CARTESIAN_POINT('Ctrl Pts',(-17.9340138084422,36.8253893035461,123.722181735766)) ;
#69165=CARTESIAN_POINT('Ctrl Pts',(-18.2290667220401,36.6454002231832,123.660120782758)) ;
#69166=CARTESIAN_POINT('Ctrl Pts',(-17.9027830695279,36.835292957087,123.463785283055)) ;
#69167=CARTESIAN_POINT('Ctrl Pts',(-18.2040801107792,36.6553038767241,123.453402008484)) ;
#69168=CARTESIAN_POINT('Ctrl Pts',(-17.9163185741068,36.8452372260823,123.20284412538)) ;
#69169=CARTESIAN_POINT('Ctrl Pts',(-18.2149045717325,36.6652481457194,123.244652494399)) ;
#69170=CARTESIAN_POINT('Ctrl Pts',(-17.9947816309639,36.858568234415,122.86134409118)) ;
#69171=CARTESIAN_POINT('Ctrl Pts',(-18.2776833949051,36.6785791540521,122.971434015951)) ;
#69172=CARTESIAN_POINT('Ctrl Pts',(-18.2021201495934,36.8751898149393,122.471324046481)) ;
#69173=CARTESIAN_POINT('Ctrl Pts',(-18.4435276248863,36.6952007345764,122.65944458022)) ;
#69174=CARTESIAN_POINT('Ctrl Pts',(-18.5280140338344,36.8917324856377,122.176159129624)) ;
#69175=CARTESIAN_POINT('Ctrl Pts',(-18.7042903718315,36.7117434052748,122.423272175924)) ;
#69176=CARTESIAN_POINT('Ctrl Pts',(-18.8400831149496,36.9050816452006,122.015936356967)) ;
#69177=CARTESIAN_POINT('Ctrl Pts',(-18.9539021452591,36.7250925648377,122.295120890868)) ;
#69178=CARTESIAN_POINT('Ctrl Pts',(-19.1721122727388,36.9183097953601,121.912858361427)) ;
#69179=CARTESIAN_POINT('Ctrl Pts',(-19.2195445013812,36.7383207149972,122.212649893044)) ;
#69180=CARTESIAN_POINT('Ctrl Pts',(-19.6137036972869,36.9349404724976,121.895030598863)) ;
#69181=CARTESIAN_POINT('Ctrl Pts',(-19.5728023332913,36.7549513921347,122.198387296976)) ;
#69182=CARTESIAN_POINT('Ctrl Pts',(-20.1178689307979,36.9548434117857,122.055389405996)) ;
#69183=CARTESIAN_POINT('Ctrl Pts',(-19.9761410205625,36.7748543314228,122.326670629609)) ;
#69184=CARTESIAN_POINT('Ctrl Pts',(-20.5372508618261,36.974746278389,122.377628584719)) ;
#69185=CARTESIAN_POINT('Ctrl Pts',(-20.3116476493232,36.7947571980261,122.584460225814)) ;
#69186=CARTESIAN_POINT('Ctrl Pts',(-20.8224429652518,36.9946594434938,122.823616943194)) ;
#69187=CARTESIAN_POINT('Ctrl Pts',(-20.5398042577158,36.8146703631309,122.941249965246)) ;
#69188=CARTESIAN_POINT('Ctrl Pts',(-20.9381837029395,37.0146952726351,123.343330198138)) ;
#69189=CARTESIAN_POINT('Ctrl Pts',(-20.6323994047383,36.8347061922723,123.357019653058)) ;
#69190=CARTESIAN_POINT('Ctrl Pts',(-20.870660430698,37.0345138475132,123.865857791706)) ;
#69191=CARTESIAN_POINT('Ctrl Pts',(-20.5783831490658,36.8545247671503,123.775043510851)) ;
#69192=CARTESIAN_POINT('Ctrl Pts',(-20.6279168053025,37.0544841485552,124.337676429547)) ;
#69193=CARTESIAN_POINT('Ctrl Pts',(-20.3841900155139,36.8744950681923,124.152499694084)) ;
#69194=CARTESIAN_POINT('Ctrl Pts',(-20.2401177850533,37.0743756809197,124.697290350133)) ;
#69195=CARTESIAN_POINT('Ctrl Pts',(-20.0739513811675,36.8943866005569,124.440192902116)) ;
#69196=CARTESIAN_POINT('Ctrl Pts',(-19.7497910668488,37.0943987787363,124.90385539926)) ;
#69197=CARTESIAN_POINT('Ctrl Pts',(-19.6816909775682,36.9144096983734,124.60544662509)) ;
#69198=CARTESIAN_POINT('Ctrl Pts',(-19.2242516782472,37.1141955316562,124.930779156354)) ;
#69199=CARTESIAN_POINT('Ctrl Pts',(-19.2612574376801,36.9342064512933,124.626987358956)) ;
#69200=CARTESIAN_POINT('Ctrl Pts',(-18.7165851062784,37.134156620145,124.77686253658)) ;
#69201=CARTESIAN_POINT('Ctrl Pts',(-18.8551234525687,36.9541675397821,124.503854730213)) ;
#69202=CARTESIAN_POINT('Ctrl Pts',(-18.2921431805836,37.1541348890772,124.457730120068)) ;
#69203=CARTESIAN_POINT('Ctrl Pts',(-18.5155690830116,36.9741458087143,124.24854960687)) ;
#69204=CARTESIAN_POINT('Ctrl Pts',(-18.0037890981737,37.1739549038682,124.016935959716)) ;
#69205=CARTESIAN_POINT('Ctrl Pts',(-18.2848840606162,36.9939658235053,123.89591275192)) ;
#69206=CARTESIAN_POINT('Ctrl Pts',(-17.8810922820256,37.19389331312,123.50137832524)) ;
#69207=CARTESIAN_POINT('Ctrl Pts',(-18.1867266714987,37.0139042327571,123.483465809288)) ;
#69208=CARTESIAN_POINT('Ctrl Pts',(-17.9432206011059,37.2139404305124,122.97212475137)) ;
#69209=CARTESIAN_POINT('Ctrl Pts',(-18.2364291043745,37.0339513501496,123.06006363056)) ;
#69210=CARTESIAN_POINT('Ctrl Pts',(-18.1799938362226,37.2337866763463,122.500836491877)) ;
#69211=CARTESIAN_POINT('Ctrl Pts',(-18.4258485917207,37.0537975959834,122.683031144881)) ;
#69212=CARTESIAN_POINT('Ctrl Pts',(-18.5620635941251,37.2536356448583,122.137020325925)) ;
#69213=CARTESIAN_POINT('Ctrl Pts',(-18.7315064596815,37.0736465644954,122.391977845995)) ;
#69214=CARTESIAN_POINT('Ctrl Pts',(-19.0504528465872,37.2736859471696,121.923931865139)) ;
#69215=CARTESIAN_POINT('Ctrl Pts',(-19.1222177233639,37.0936968668067,122.221508236812)) ;
#69216=CARTESIAN_POINT('Ctrl Pts',(-19.5767155011093,37.2935208696008,121.890757346003)) ;
#69217=CARTESIAN_POINT('Ctrl Pts',(-19.5432297263916,37.113531789238,122.194969649968)) ;
#69218=CARTESIAN_POINT('Ctrl Pts',(-20.08511494409,37.3134512708267,122.038788804448)) ;
#69219=CARTESIAN_POINT('Ctrl Pts',(-19.9499495172448,37.1334621904638,122.313396725135)) ;
#69220=CARTESIAN_POINT('Ctrl Pts',(-20.5122328950149,37.3333362161856,122.35040788788)) ;
#69221=CARTESIAN_POINT('Ctrl Pts',(-20.2916434333738,37.1533471358227,122.562694298399)) ;
#69222=CARTESIAN_POINT('Ctrl Pts',(-20.8092661802658,37.353408824337,122.793446550335)) ;
#69223=CARTESIAN_POINT('Ctrl Pts',(-20.5292680326244,37.1734197439741,122.917125764005)) ;
#69224=CARTESIAN_POINT('Ctrl Pts',(-20.9356180404718,37.3732001406651,123.304147384377)) ;
#69225=CARTESIAN_POINT('Ctrl Pts',(-20.6303478832511,37.1932110603022,123.325688757585)) ;
#69226=CARTESIAN_POINT('Ctrl Pts',(-20.8812658706226,37.3931649304323,123.8319433124)) ;
#69227=CARTESIAN_POINT('Ctrl Pts',(-20.5868633031295,37.2131758500695,123.747925458238)) ;
#69228=CARTESIAN_POINT('Ctrl Pts',(-20.6486375255731,37.4131478861826,124.309410738548)) ;
#69229=CARTESIAN_POINT('Ctrl Pts',(-20.4007582836289,37.2331588058198,124.129898402551)) ;
#69230=CARTESIAN_POINT('Ctrl Pts',(-20.2710983170399,37.4329564081588,124.676413569009)) ;
#69231=CARTESIAN_POINT('Ctrl Pts',(-20.0987238439308,37.2529673277959,124.423499492388)) ;
#69232=CARTESIAN_POINT('Ctrl Pts',(-19.7870846025984,37.4529419828946,124.894968051368)) ;
#69233=CARTESIAN_POINT('Ctrl Pts',(-19.7115114515686,37.2729529025317,124.598340127017)) ;
#69234=CARTESIAN_POINT('Ctrl Pts',(-19.2600251516879,37.472824622963,124.934935958172)) ;
#69235=CARTESIAN_POINT('Ctrl Pts',(-19.2898629599609,37.2928355426001,124.630311187914)) ;
#69236=CARTESIAN_POINT('Ctrl Pts',(-18.7492134555832,37.4927799350949,124.792594096249)) ;
#69237=CARTESIAN_POINT('Ctrl Pts',(-18.8812143169606,37.312790854732,124.516434239319)) ;
#69238=CARTESIAN_POINT('Ctrl Pts',(-18.319033254551,37.5126542917027,124.485894779788)) ;
#69239=CARTESIAN_POINT('Ctrl Pts',(-18.5370718339478,37.3326652113398,124.27107140888)) ;
#69240=CARTESIAN_POINT('Ctrl Pts',(-18.0175106060064,37.5326364985638,124.048765115388)) ;
#69241=CARTESIAN_POINT('Ctrl Pts',(-18.2958567266438,37.3526474182009,123.921365577981)) ;
#69242=CARTESIAN_POINT('Ctrl Pts',(-17.8838308617942,37.5525675765137,123.536059048149)) ;
#69243=CARTESIAN_POINT('Ctrl Pts',(-18.1889170443655,37.3725784961509,123.5111991052)) ;
#69244=CARTESIAN_POINT('Ctrl Pts',(-17.9330320754365,37.5724945513687,123.008830582015)) ;
#69245=CARTESIAN_POINT('Ctrl Pts',(-18.2282802580598,37.3925054710058,123.089417886411)) ;
#69246=CARTESIAN_POINT('Ctrl Pts',(-18.157254622848,37.5923270103176,122.531709623646)) ;
#69247=CARTESIAN_POINT('Ctrl Pts',(-18.4076687041876,37.4123379299547,122.707716901662)) ;
#69248=CARTESIAN_POINT('Ctrl Pts',(-18.4706659458096,37.6089846944928,122.219158784054)) ;
#69249=CARTESIAN_POINT('Ctrl Pts',(-18.658380296989,37.4289956141299,122.457695891381)) ;
#69250=CARTESIAN_POINT('Ctrl Pts',(-18.7724796762074,37.6222339183999,122.045392670349)) ;
#69251=CARTESIAN_POINT('Ctrl Pts',(-18.8998510804845,37.442244838037,122.318670265349)) ;
#69252=CARTESIAN_POINT('Ctrl Pts',(-19.0206690089167,37.6322829398511,121.955269929733)) ;
#69253=CARTESIAN_POINT('Ctrl Pts',(-19.0983967704762,37.4522938594882,122.246576695617)) ;
#69254=CARTESIAN_POINT('Ctrl Pts',(-19.2758657649021,37.6421429480816,121.910397904174)) ;
#69255=CARTESIAN_POINT('Ctrl Pts',(-19.3025665790804,37.4621538677187,122.210682152963)) ;
#69256=CARTESIAN_POINT('Ctrl Pts',(-19.6249794284296,37.6554264613062,121.909413584284)) ;
#69257=CARTESIAN_POINT('Ctrl Pts',(-19.5818035064809,37.4754373809433,122.20988869481)) ;
#69258=CARTESIAN_POINT('Ctrl Pts',(-20.0524638778648,37.672072380307,122.023188295616)) ;
#69259=CARTESIAN_POINT('Ctrl Pts',(-19.9238581002366,37.4920832999442,122.300927565958)) ;
#69260=CARTESIAN_POINT('Ctrl Pts',(-20.413880776944,37.6886263581231,122.274169668414)) ;
#69261=CARTESIAN_POINT('Ctrl Pts',(-20.2129442060005,37.5086372777602,122.501691816295)) ;
#69262=CARTESIAN_POINT('Ctrl Pts',(-20.6406243713132,37.7019860870947,122.542201540504)) ;
#69263=CARTESIAN_POINT('Ctrl Pts',(-20.3943637147157,37.5219970067318,122.716138256514)) ;
#69264=CARTESIAN_POINT('Ctrl Pts',(-20.771703979078,37.7118791388914,122.766737576687)) ;
#69265=CARTESIAN_POINT('Ctrl Pts',(-20.4992200975137,37.5318900585285,122.895764440336)) ;
#69266=CARTESIAN_POINT('Ctrl Pts',(-20.8630031282262,37.7218691041725,123.012844193469)) ;
#69267=CARTESIAN_POINT('Ctrl Pts',(-20.5722587448008,37.5418800238096,123.092651501254)) ;
#69268=CARTESIAN_POINT('Ctrl Pts',(-20.9101691765086,37.7318209850333,123.270122215449)) ;
#69269=CARTESIAN_POINT('Ctrl Pts',(-20.609988980369,37.5518319046704,123.298474032624)) ;
#69270=CARTESIAN_POINT('Ctrl Pts',(-20.9117400295103,37.7418693367251,123.534149528085)) ;
#69271=CARTESIAN_POINT('Ctrl Pts',(-20.6112435209441,37.5618802563622,123.509695891286)) ;
#69272=CARTESIAN_POINT('Ctrl Pts',(-20.8686496157947,37.7517106208313,123.789179451331)) ;
#69273=CARTESIAN_POINT('Ctrl Pts',(-20.576768936994,37.5717215404684,123.713719468987)) ;
#69274=CARTESIAN_POINT('Ctrl Pts',(-20.7811945958756,37.761697323957,124.0365703206)) ;
#69275=CARTESIAN_POINT('Ctrl Pts',(-20.5068028158722,37.5817082435941,123.911631353683)) ;
#69276=CARTESIAN_POINT('Ctrl Pts',(-20.6528738763807,37.7716323527744,124.263999794878)) ;
#69277=CARTESIAN_POINT('Ctrl Pts',(-20.4041443030014,37.5916432724115,124.093573772257)) ;
#69278=CARTESIAN_POINT('Ctrl Pts',(-20.4848851322175,37.7816881476813,124.467934944113)) ;
#69279=CARTESIAN_POINT('Ctrl Pts',(-20.2697515895762,37.6016990673184,124.256720420404)) ;
#69280=CARTESIAN_POINT('Ctrl Pts',(-20.2887835292672,37.7915165109706,124.636074676787)) ;
#69281=CARTESIAN_POINT('Ctrl Pts',(-20.1128689225267,37.6115274306077,124.391230423038)) ;
#69282=CARTESIAN_POINT('Ctrl Pts',(-20.0614584855971,37.8015774808685,124.771009318032)) ;
#69283=CARTESIAN_POINT('Ctrl Pts',(-19.931007771351,37.6215884005056,124.49917617883)) ;
#69284=CARTESIAN_POINT('Ctrl Pts',(-19.8176275658583,37.8114917597583,124.862882128275)) ;
#69285=CARTESIAN_POINT('Ctrl Pts',(-19.735942339562,37.6315026793954,124.572672280903)) ;
#69286=CARTESIAN_POINT('Ctrl Pts',(-19.5592226441299,37.8215007542265,124.911986102219)) ;
#69287=CARTESIAN_POINT('Ctrl Pts',(-19.5292180435957,37.6415116738637,124.611953245993)) ;
#69288=CARTESIAN_POINT('Ctrl Pts',(-19.2956698137528,37.8315305887903,124.914944725245)) ;
#69289=CARTESIAN_POINT('Ctrl Pts',(-19.3183757846655,37.6515415084274,124.614317886194)) ;
#69290=CARTESIAN_POINT('Ctrl Pts',(-19.0399553923332,37.8413888188625,124.873312424771)) ;
#69291=CARTESIAN_POINT('Ctrl Pts',(-19.113804794043,37.6613997384997,124.581009863178)) ;
#69292=CARTESIAN_POINT('Ctrl Pts',(-18.7918216048471,37.8513875246049,124.787014243601)) ;
#69293=CARTESIAN_POINT('Ctrl Pts',(-18.915298566103,37.6713984442421,124.511969231989)) ;
#69294=CARTESIAN_POINT('Ctrl Pts',(-18.5645984860679,37.8612821805237,124.660501733372)) ;
#69295=CARTESIAN_POINT('Ctrl Pts',(-18.7335213311777,37.6812931001609,124.410757393858)) ;
#69296=CARTESIAN_POINT('Ctrl Pts',(-18.3594834848053,37.8713452449077,124.493660346681)) ;
#69297=CARTESIAN_POINT('Ctrl Pts',(-18.5694307097895,37.6913561645448,124.277282542542)) ;
#69298=CARTESIAN_POINT('Ctrl Pts',(-18.1900212161876,37.8811849031876,124.298298757576)) ;
#69299=CARTESIAN_POINT('Ctrl Pts',(-18.4338627738789,37.7011958228247,124.120992079632)) ;
#69300=CARTESIAN_POINT('Ctrl Pts',(-18.0537869453756,37.8912480702694,124.071683477115)) ;
#69301=CARTESIAN_POINT('Ctrl Pts',(-18.3248772081804,37.7112589899066,123.939698699603)) ;
#69302=CARTESIAN_POINT('Ctrl Pts',(-17.9607436771395,37.9011423153965,123.828859729569)) ;
#69303=CARTESIAN_POINT('Ctrl Pts',(-18.2504447386895,37.7211532350337,123.745439163456)) ;
#69304=CARTESIAN_POINT('Ctrl Pts',(-17.9103527062584,37.9110841370011,123.572537760102)) ;
#69305=CARTESIAN_POINT('Ctrl Pts',(-18.2101341056503,37.7310950566383,123.540381382668)) ;
#69306=CARTESIAN_POINT('Ctrl Pts',(-17.9051034699468,37.9210866679192,123.309699103469)) ;
#69307=CARTESIAN_POINT('Ctrl Pts',(-18.2059368477175,37.7410975875563,123.330110481641)) ;
#69308=CARTESIAN_POINT('Ctrl Pts',(-17.946097783474,37.9311212943767,123.049219622139)) ;
#69309=CARTESIAN_POINT('Ctrl Pts',(-18.238734443196,37.7511322140138,123.121727220956)) ;
#69310=CARTESIAN_POINT('Ctrl Pts',(-18.0297012300919,37.9409668293631,122.804359246479)) ;
#69311=CARTESIAN_POINT('Ctrl Pts',(-18.3056190713924,37.7609777490003,122.925840036189)) ;
#69312=CARTESIAN_POINT('Ctrl Pts',(-18.1557855280744,37.9509502542022,122.574313582137)) ;
#69313=CARTESIAN_POINT('Ctrl Pts',(-18.4064882631411,37.7709611738393,122.741804625682)) ;
#69314=CARTESIAN_POINT('Ctrl Pts',(-18.3194140988036,37.9609006445672,122.370342409505)) ;
#69315=CARTESIAN_POINT('Ctrl Pts',(-18.5373926050169,37.7809115642044,122.578629156935)) ;
#69316=CARTESIAN_POINT('Ctrl Pts',(-18.5166838775539,37.9708982848643,122.196785487703)) ;
#69317=CARTESIAN_POINT('Ctrl Pts',(-18.6952097128482,37.7909092045014,122.439785207195)) ;
#69318=CARTESIAN_POINT('Ctrl Pts',(-18.7422660732146,37.9809373654275,122.060023983283)) ;
#69319=CARTESIAN_POINT('Ctrl Pts',(-18.8756765999443,37.8009482850646,122.330377774988)) ;
#69320=CARTESIAN_POINT('Ctrl Pts',(-18.9827700674646,37.9907635161966,121.965984935098)) ;
#69321=CARTESIAN_POINT('Ctrl Pts',(-19.068079960445,37.8107744358337,122.255148655797)) ;
#69322=CARTESIAN_POINT('Ctrl Pts',(-19.2417735141306,38.0008200911257,121.913534414804)) ;
#69323=CARTESIAN_POINT('Ctrl Pts',(-19.2752831961908,37.8208310107629,122.213190167423)) ;
#69324=CARTESIAN_POINT('Ctrl Pts',(-19.5029368385389,38.010760630506,121.907384733562)) ;
#69325=CARTESIAN_POINT('Ctrl Pts',(-19.4842136365279,37.8307715501431,122.20827246862)) ;
#69326=CARTESIAN_POINT('Ctrl Pts',(-19.7603796758828,38.0206650234824,121.94572645087)) ;
#69327=CARTESIAN_POINT('Ctrl Pts',(-19.6901671990176,37.8406759431195,122.238947693233)) ;
#69328=CARTESIAN_POINT('Ctrl Pts',(-20.0107210558662,38.0307116776873,122.029521129623)) ;
#69329=CARTESIAN_POINT('Ctrl Pts',(-19.8904397605092,37.8507225973244,122.305985318718)) ;
#69330=CARTESIAN_POINT('Ctrl Pts',(-20.2393912303446,38.0406072396257,122.153437722029)) ;
#69331=CARTESIAN_POINT('Ctrl Pts',(-20.0733745736591,37.8606181592628,122.405120060761)) ;
#69332=CARTESIAN_POINT('Ctrl Pts',(-20.4464358604614,38.0506693174713,122.317848314889)) ;
#69333=CARTESIAN_POINT('Ctrl Pts',(-20.2390091946635,37.8706802371084,122.536650134307)) ;
#69334=CARTESIAN_POINT('Ctrl Pts',(-20.6181207395519,38.060512015885,122.511348876402)) ;
#69335=CARTESIAN_POINT('Ctrl Pts',(-20.3763552143861,37.8805229355222,122.691451327068)) ;
#69336=CARTESIAN_POINT('Ctrl Pts',(-20.7561325943481,38.0705027908465,122.734655821582)) ;
#69337=CARTESIAN_POINT('Ctrl Pts',(-20.4867630838622,37.8905137104836,122.870097716257)) ;
#69338=CARTESIAN_POINT('Ctrl Pts',(-20.8526444302202,38.0804306558656,122.977057792993)) ;
#69339=CARTESIAN_POINT('Ctrl Pts',(-20.5639707221755,37.9004415755027,123.064019601063)) ;
#69340=CARTESIAN_POINT('Ctrl Pts',(-20.9063538531691,38.0904194006318,123.234003272381)) ;
#69341=CARTESIAN_POINT('Ctrl Pts',(-20.6069365241512,37.9104303202689,123.269576200659)) ;
#69342=CARTESIAN_POINT('Ctrl Pts',(-20.9142822162603,38.1004521862187,123.497539173054)) ;
#69343=CARTESIAN_POINT('Ctrl Pts',(-20.6132774084487,37.9204631058559,123.480405034982)) ;
#69344=CARTESIAN_POINT('Ctrl Pts',(-20.8772223147212,38.1103188708394,123.754154223928)) ;
#69345=CARTESIAN_POINT('Ctrl Pts',(-20.5836278397377,37.9303297904765,123.685696137519)) ;
#69346=CARTESIAN_POINT('Ctrl Pts',(-20.7960987290107,38.1202807630025,124.00306041153)) ;
#69347=CARTESIAN_POINT('Ctrl Pts',(-20.5187275050565,37.9402916826396,123.884820316478)) ;
#69348=CARTESIAN_POINT('Ctrl Pts',(-20.6717436692743,38.1303142399151,124.235550043403)) ;
#69349=CARTESIAN_POINT('Ctrl Pts',(-20.4192419168591,37.9503251595522,124.070811279402)) ;
#69350=CARTESIAN_POINT('Ctrl Pts',(-20.5116269403932,38.1401985811634,124.440122137364)) ;
#69351=CARTESIAN_POINT('Ctrl Pts',(-20.291147641117,37.9602095008005,124.2344674478)) ;
#69352=CARTESIAN_POINT('Ctrl Pts',(-20.3149827227567,38.1502615232845,124.616881340023)) ;
#69353=CARTESIAN_POINT('Ctrl Pts',(-20.1338310207247,37.9702724429217,124.37587373082)) ;
#69354=CARTESIAN_POINT('Ctrl Pts',(-20.0953938752767,38.1601119249041,124.75399118927)) ;
#69355=CARTESIAN_POINT('Ctrl Pts',(-19.9581597997883,37.9801228445412,124.48555979968)) ;
#69356=CARTESIAN_POINT('Ctrl Pts',(-19.8513087068426,38.1701388136938,124.853234002042)) ;
#69357=CARTESIAN_POINT('Ctrl Pts',(-19.7628910767466,37.9901497333309,124.564952686841)) ;
#69358=CARTESIAN_POINT('Ctrl Pts',(-19.593491376287,38.18016742865,124.907926696643)) ;
#69359=CARTESIAN_POINT('Ctrl Pts',(-19.5566368221853,38.0001783482871,124.60870527169)) ;
#69360=CARTESIAN_POINT('Ctrl Pts',(-19.3349545228551,38.19001265177,124.917345289566)) ;
#69361=CARTESIAN_POINT('Ctrl Pts',(-19.3498081794795,38.0100235714072,124.616238591865)) ;
#69362=CARTESIAN_POINT('Ctrl Pts',(-19.0748065717966,38.200003335576,124.88189910921)) ;
#69363=CARTESIAN_POINT('Ctrl Pts',(-19.1416901604654,38.0200142552131,124.587880298934)) ;
#69364=CARTESIAN_POINT('Ctrl Pts',(-18.8237728136893,38.2100412176484,124.80088615643)) ;
#69365=CARTESIAN_POINT('Ctrl Pts',(-18.9408635131046,38.0300521372856,124.52306847567)) ;
#69366=CARTESIAN_POINT('Ctrl Pts',(-18.5948907896328,38.2198855772873,124.680287851483)) ;
#69367=CARTESIAN_POINT('Ctrl Pts',(-18.7577593811284,38.0398964969244,124.426589023562)) ;
#69368=CARTESIAN_POINT('Ctrl Pts',(-18.3872272286847,38.229870447902,124.519955106578)) ;
#69369=CARTESIAN_POINT('Ctrl Pts',(-18.5916294861403,38.0498813675391,124.298321919019)) ;
#69370=CARTESIAN_POINT('Ctrl Pts',(-18.2112252563883,38.2398097312307,124.326911572828)) ;
#69371=CARTESIAN_POINT('Ctrl Pts',(-18.4508291441772,38.0598206508678,124.143886556018)) ;
#69372=CARTESIAN_POINT('Ctrl Pts',(-18.0700954992362,38.2498503406038,124.104002776353)) ;
#69373=CARTESIAN_POINT('Ctrl Pts',(-18.3379263671355,38.0698612602409,123.9655587244)) ;
#69374=CARTESIAN_POINT('Ctrl Pts',(-17.9711690914586,38.259735191517,123.863780801288)) ;
#69375=CARTESIAN_POINT('Ctrl Pts',(-18.2587866856612,38.0797461111542,123.773381363225)) ;
#69376=CARTESIAN_POINT('Ctrl Pts',(-17.9145022539865,38.2697371476858,123.607161518794)) ;
#69377=CARTESIAN_POINT('Ctrl Pts',(-18.2134543961033,38.089748067323,123.568085793676)) ;
#69378=CARTESIAN_POINT('Ctrl Pts',(-17.9031351939843,38.2796557444063,123.34671741945)) ;
#69379=CARTESIAN_POINT('Ctrl Pts',(-18.2043619071338,38.0996666640434,123.359731038019)) ;
#69380=CARTESIAN_POINT('Ctrl Pts',(-17.9376431227796,38.2897025664821,123.084999919376)) ;
#69381=CARTESIAN_POINT('Ctrl Pts',(-18.2319694141101,38.1097134861192,123.150357019419)) ;
#69382=CARTESIAN_POINT('Ctrl Pts',(-18.0154975116536,38.2995768475948,122.837421943665)) ;
#69383=CARTESIAN_POINT('Ctrl Pts',(-18.2942537162335,38.1195877672319,122.95229576589)) ;
#69384=CARTESIAN_POINT('Ctrl Pts',(-18.1371535108144,38.3096310476394,122.602934129142)) ;
#69385=CARTESIAN_POINT('Ctrl Pts',(-18.391579553754,38.1296419672765,122.764705818433)) ;
#69386=CARTESIAN_POINT('Ctrl Pts',(-18.2951140075871,38.3195264772746,122.396304412918)) ;
#69387=CARTESIAN_POINT('Ctrl Pts',(-18.5179483256354,38.1395373969118,122.599403261707)) ;
#69388=CARTESIAN_POINT('Ctrl Pts',(-18.489664634007,38.329588105592,122.217293421697)) ;
#69389=CARTESIAN_POINT('Ctrl Pts',(-18.6735897116982,38.1495990252291,122.456195042217)) ;
#69390=CARTESIAN_POINT('Ctrl Pts',(-18.7075571482892,38.3394327344219,122.077804596519)) ;
#69391=CARTESIAN_POINT('Ctrl Pts',(-18.8479033795345,38.159443654059,122.344605407475)) ;
#69392=CARTESIAN_POINT('Ctrl Pts',(-18.9487829946581,38.3493927820275,121.976237815657)) ;
#69393=CARTESIAN_POINT('Ctrl Pts',(-19.0408840272685,38.1694037016646,122.26335285546)) ;
#69394=CARTESIAN_POINT('Ctrl Pts',(-19.2060908983608,38.3594310882016,121.918149353435)) ;
#69395=CARTESIAN_POINT('Ctrl Pts',(-19.2467306787397,38.1794420078387,122.216882950581)) ;
#69396=CARTESIAN_POINT('Ctrl Pts',(-19.4652741750424,38.3693043876342,121.905324657195)) ;
#69397=CARTESIAN_POINT('Ctrl Pts',(-19.4540764400432,38.1893153072714,122.206624032452)) ;
#69398=CARTESIAN_POINT('Ctrl Pts',(-19.7278563927704,38.3793776492205,121.938426707961)) ;
#69399=CARTESIAN_POINT('Ctrl Pts',(-19.6641424513348,38.1993885688576,122.233106527423)) ;
#69400=CARTESIAN_POINT('Ctrl Pts',(-19.9745595742938,38.3891978751772,122.014360134831)) ;
#69401=CARTESIAN_POINT('Ctrl Pts',(-19.8615035911148,38.2092087948143,122.293853602793)) ;
#69402=CARTESIAN_POINT('Ctrl Pts',(-20.2103785146625,38.3992769391167,122.134809378916)) ;
#69403=CARTESIAN_POINT('Ctrl Pts',(-20.0501587726125,38.2192878587538,122.390213775036)) ;
#69404=CARTESIAN_POINT('Ctrl Pts',(-20.4170842341087,38.4091270291365,122.29073495999)) ;
#69405=CARTESIAN_POINT('Ctrl Pts',(-20.2155221090438,38.2291379487737,122.514954115043)) ;
#69406=CARTESIAN_POINT('Ctrl Pts',(-20.5976790049717,38.4192057827503,122.484385049267)) ;
#69407=CARTESIAN_POINT('Ctrl Pts',(-20.359997738072,38.2392167023874,122.669874889421)) ;
#69408=CARTESIAN_POINT('Ctrl Pts',(-20.7384592821363,38.4290272500098,122.700777392782)) ;
#69409=CARTESIAN_POINT('Ctrl Pts',(-20.4726207917741,38.2490381696469,122.842988001983)) ;
#69410=CARTESIAN_POINT('Ctrl Pts',(-20.8423676549778,38.4390928483674,122.943961403778)) ;
#69411=CARTESIAN_POINT('Ctrl Pts',(-20.5557471819317,38.2591037680045,123.037535670951)) ;
#69412=CARTESIAN_POINT('Ctrl Pts',(-20.9014598751906,38.4489955041421,123.197461404665)) ;
#69413=CARTESIAN_POINT('Ctrl Pts',(-20.6030203204311,38.2690064237792,123.240335071546)) ;
#69414=CARTESIAN_POINT('Ctrl Pts',(-20.9159258761711,38.4590463299717,123.461136272486)) ;
#69415=CARTESIAN_POINT('Ctrl Pts',(-20.6145926705631,38.2790572496089,123.451275207691)) ;
#69416=CARTESIAN_POINT('Ctrl Pts',(-20.8851806308957,38.4689205343106,123.718849938155)) ;
#69417=CARTESIAN_POINT('Ctrl Pts',(-20.5899961850183,38.2889314539477,123.657445168674)) ;
#69418=CARTESIAN_POINT('Ctrl Pts',(-20.808697747039,38.4789929843497,123.972194060034)) ;
#69419=CARTESIAN_POINT('Ctrl Pts',(-20.5288093967578,38.2990039039868,123.860120677196)) ;
#69420=CARTESIAN_POINT('Ctrl Pts',(-20.6924452330028,38.4888220011232,124.202906653744)) ;
#69421=CARTESIAN_POINT('Ctrl Pts',(-20.4358076437675,38.3088329207603,124.044689498754)) ;
#69422=CARTESIAN_POINT('Ctrl Pts',(-20.5345088117265,38.498888847038,124.415079071641)) ;
#69423=CARTESIAN_POINT('Ctrl Pts',(-20.3094581203434,38.3188997666751,124.214427542869)) ;
#69424=CARTESIAN_POINT('Ctrl Pts',(-20.3453362910282,38.5087790183398,124.593350718177)) ;
#69425=CARTESIAN_POINT('Ctrl Pts',(-20.1581205171573,38.3287899379769,124.35704407548)) ;
#69426=CARTESIAN_POINT('Ctrl Pts',(-20.1262004053155,38.5187712119636,124.737995435515)) ;
#69427=CARTESIAN_POINT('Ctrl Pts',(-19.9828118735316,38.3387821316008,124.472759636862)) ;
#69428=CARTESIAN_POINT('Ctrl Pts',(-19.8858793197356,38.5287340225871,124.841862120209)) ;
#69429=CARTESIAN_POINT('Ctrl Pts',(-19.7905552583215,38.3487449422242,124.55585265074)) ;
#69430=CARTESIAN_POINT('Ctrl Pts',(-19.6327966736522,38.5386382954305,124.9027167446)) ;
#69431=CARTESIAN_POINT('Ctrl Pts',(-19.5880898637253,38.3586492150676,124.604536139099)) ;
#69432=CARTESIAN_POINT('Ctrl Pts',(-19.3689353661875,38.5486987872351,124.918722771456)) ;
#69433=CARTESIAN_POINT('Ctrl Pts',(-19.3770005294909,38.3687097068723,124.617340882227)) ;
#69434=CARTESIAN_POINT('Ctrl Pts',(-19.1119433120646,38.5585391189074,124.8896559552)) ;
#69435=CARTESIAN_POINT('Ctrl Pts',(-19.1714080569819,38.3785500385446,124.594087552618)) ;
#69436=CARTESIAN_POINT('Ctrl Pts',(-18.858267179598,38.5686021649992,124.815076395297)) ;
#69437=CARTESIAN_POINT('Ctrl Pts',(-18.9684668438895,38.3886130846363,124.534423889178)) ;
#69438=CARTESIAN_POINT('Ctrl Pts',(-18.6254129262552,38.5784962206943,124.699336919331)) ;
#69439=CARTESIAN_POINT('Ctrl Pts',(-18.782184165847,38.3985071403314,124.441832684119)) ;
#69440=CARTESIAN_POINT('Ctrl Pts',(-18.4147842988255,38.5884389210173,124.544774213898)) ;
#69441=CARTESIAN_POINT('Ctrl Pts',(-18.6136815630311,38.4084498406544,124.318182986908)) ;
#69442=CARTESIAN_POINT('Ctrl Pts',(-18.2329705623296,38.5984446619449,124.354785151136)) ;
#69443=CARTESIAN_POINT('Ctrl Pts',(-18.4682304676226,38.418455581582,124.166191932299)) ;
#69444=CARTESIAN_POINT('Ctrl Pts',(-18.086951476104,38.6084655724604,124.135644682199)) ;
#69445=CARTESIAN_POINT('Ctrl Pts',(-18.3514150709044,38.4284764920975,123.990879603999)) ;
#69446=CARTESIAN_POINT('Ctrl Pts',(-17.9822934308915,38.6183563079104,123.897719206915)) ;
#69447=CARTESIAN_POINT('Ctrl Pts',(-18.2676887771091,38.4383672275475,123.800540072914)) ;
#69448=CARTESIAN_POINT('Ctrl Pts',(-17.9195346698227,38.6283478486392,123.642773296593)) ;
#69449=CARTESIAN_POINT('Ctrl Pts',(-18.2174815116301,38.4483587682763,123.596583584727)) ;
#69450=CARTESIAN_POINT('Ctrl Pts',(-17.9021467020347,38.6382957090609,123.381934725884)) ;
#69451=CARTESIAN_POINT('Ctrl Pts',(-18.2035708827029,38.458306628698,123.387913220143)) ;
#69452=CARTESIAN_POINT('Ctrl Pts',(-17.9297985346469,38.6482423782472,123.121998548221)) ;
#69453=CARTESIAN_POINT('Ctrl Pts',(-18.225691882754,38.4682532978843,123.179964691049)) ;
#69454=CARTESIAN_POINT('Ctrl Pts',(-18.0031723206151,38.6582904543828,122.868354913034)) ;
#69455=CARTESIAN_POINT('Ctrl Pts',(-18.2843906358415,38.4783013740199,122.977049494518)) ;
#69456=CARTESIAN_POINT('Ctrl Pts',(-18.1169630845849,38.6681380523884,122.635927730738)) ;
#69457=CARTESIAN_POINT('Ctrl Pts',(-18.3754223953298,38.4881489720256,122.791108578199)) ;
#69458=CARTESIAN_POINT('Ctrl Pts',(-18.2704754939803,38.6780997754729,122.423894509235)) ;
#69459=CARTESIAN_POINT('Ctrl Pts',(-18.498231618631,38.49811069511,122.621481940386)) ;
#69460=CARTESIAN_POINT('Ctrl Pts',(-18.459987920288,38.6881284105559,122.240733703719)) ;
#69461=CARTESIAN_POINT('Ctrl Pts',(-18.6498412530283,38.508139330193,122.474952867454)) ;
#69462=CARTESIAN_POINT('Ctrl Pts',(-18.6757765964958,38.6980387188739,122.094945578105)) ;
#69463=CARTESIAN_POINT('Ctrl Pts',(-18.822471309607,38.5180496385111,122.358322309801)) ;
#69464=CARTESIAN_POINT('Ctrl Pts',(-18.9139298646634,38.7079736160098,121.987944654687)) ;
#69465=CARTESIAN_POINT('Ctrl Pts',(-19.0129931507068,38.5279845356469,122.272721138619)) ;
#69466=CARTESIAN_POINT('Ctrl Pts',(-19.1697940908906,38.7180146989524,121.92347677505)) ;
#69467=CARTESIAN_POINT('Ctrl Pts',(-19.2176845178362,38.5380256185895,122.221146167551)) ;
#69468=CARTESIAN_POINT('Ctrl Pts',(-19.4289447281885,38.7279020417806,121.904527054462)) ;
#69469=CARTESIAN_POINT('Ctrl Pts',(-19.4250041481742,38.5479129614178,122.20598575918)) ;
#69470=CARTESIAN_POINT('Ctrl Pts',(-19.6901903067169,38.73789355672,121.930687744959)) ;
#69471=CARTESIAN_POINT('Ctrl Pts',(-19.634000528053,38.5579044763571,122.226913496927)) ;
#69472=CARTESIAN_POINT('Ctrl Pts',(-19.9419001392369,38.7478449479164,122.001637581168)) ;
#69473=CARTESIAN_POINT('Ctrl Pts',(-19.8353681920912,38.5678558675536,122.283672501495)) ;
#69474=CARTESIAN_POINT('Ctrl Pts',(-20.1772104092053,38.7577774812491,122.114589337141)) ;
#69475=CARTESIAN_POINT('Ctrl Pts',(-20.0236163134936,38.5777884008862,122.374032878613)) ;
#69476=CARTESIAN_POINT('Ctrl Pts',(-20.3907677132585,38.7677746391485,122.267583026891)) ;
#69477=CARTESIAN_POINT('Ctrl Pts',(-20.1944625857522,38.5877855587856,122.496427023054)) ;
#69478=CARTESIAN_POINT('Ctrl Pts',(-20.5743995160923,38.777759649312,122.455072551218)) ;
#69479=CARTESIAN_POINT('Ctrl Pts',(-20.3413685642757,38.5977705689491,122.646417859673)) ;
#69480=CARTESIAN_POINT('Ctrl Pts',(-20.7231828307075,38.7878024758818,122.673007430821)) ;
#69481=CARTESIAN_POINT('Ctrl Pts',(-20.4603959891244,38.6078133955189,122.82076541107)) ;
#69482=CARTESIAN_POINT('Ctrl Pts',(-20.8301369986688,38.7976327101868,122.908200598567)) ;
#69483=CARTESIAN_POINT('Ctrl Pts',(-20.5459597363222,38.6176436298239,123.008918492089)) ;
#69484=CARTESIAN_POINT('Ctrl Pts',(-20.8963322764258,38.8077087354214,123.164523836751)) ;
#69485=CARTESIAN_POINT('Ctrl Pts',(-20.5989170207742,38.6277196550586,123.213977164575)) ;
#69486=CARTESIAN_POINT('Ctrl Pts',(-20.9166999184839,38.8175609719123,123.422684680524)) ;
#69487=CARTESIAN_POINT('Ctrl Pts',(-20.6152120890159,38.6375718915494,123.420504774744)) ;
#69488=CARTESIAN_POINT('Ctrl Pts',(-20.8916094132905,38.8276341783464,123.686162896882)) ;
#69489=CARTESIAN_POINT('Ctrl Pts',(-20.5951407373615,38.6476450979836,123.631287770219)) ;
#69490=CARTESIAN_POINT('Ctrl Pts',(-20.8226867659829,38.8374756878536,123.935453060471)) ;
#69491=CARTESIAN_POINT('Ctrl Pts',(-20.5400039281525,38.6574866074907,123.830719181644)) ;
#69492=CARTESIAN_POINT('Ctrl Pts',(-20.711078874135,38.8474366346334,124.172221368131)) ;
#69493=CARTESIAN_POINT('Ctrl Pts',(-20.4507189196892,38.6674475542705,124.020134084588)) ;
#69494=CARTESIAN_POINT('Ctrl Pts',(-20.558458951886,38.8574744634334,124.387360046542)) ;
#69495=CARTESIAN_POINT('Ctrl Pts',(-20.3286238767375,38.6774853830706,124.192245792429)) ;
#69496=CARTESIAN_POINT('Ctrl Pts',(-20.3741695323438,38.8673487731879,124.570081720976)) ;
#69497=CARTESIAN_POINT('Ctrl Pts',(-20.1811938154597,38.687359692825,124.338423469398)) ;
#69498=CARTESIAN_POINT('Ctrl Pts',(-20.1567812055592,38.8774184708611,124.72090620419)) ;
#69499=CARTESIAN_POINT('Ctrl Pts',(-20.0072836517336,38.6974293904982,124.459084262676)) ;
#69500=CARTESIAN_POINT('Ctrl Pts',(-19.9221504638818,38.8872519421485,124.82924108008)) ;
#69501=CARTESIAN_POINT('Ctrl Pts',(-19.8195805334962,38.7072628617856,124.545752917569)) ;
#69502=CARTESIAN_POINT('Ctrl Pts',(-19.6675077755331,38.8972815886784,124.897233739368)) ;
#69503=CARTESIAN_POINT('Ctrl Pts',(-19.615866693082,38.7172925083155,124.600148473551)) ;
#69504=CARTESIAN_POINT('Ctrl Pts',(-19.4047212779265,38.9073161030058,124.919189865937)) ;
#69505=CARTESIAN_POINT('Ctrl Pts',(-19.4056375333307,38.7273270226429,124.61771467157)) ;
#69506=CARTESIAN_POINT('Ctrl Pts',(-19.1475370275011,38.9171413884767,124.896304082123)) ;
#69507=CARTESIAN_POINT('Ctrl Pts',(-19.1998910344568,38.7371523081138,124.599407555355)) ;
#69508=CARTESIAN_POINT('Ctrl Pts',(-18.8935792031542,38.9271456300252,124.828433457309)) ;
#69509=CARTESIAN_POINT('Ctrl Pts',(-18.9967244455218,38.7471565496623,124.545112555679)) ;
#69510=CARTESIAN_POINT('Ctrl Pts',(-18.6557514840931,38.9371282751043,124.717603510386)) ;
#69511=CARTESIAN_POINT('Ctrl Pts',(-18.8064617880754,38.7571391947414,124.456450040447)) ;
#69512=CARTESIAN_POINT('Ctrl Pts',(-18.439669749991,38.9471734721958,124.566019704998)) ;
#69513=CARTESIAN_POINT('Ctrl Pts',(-18.633595466131,38.7671843918329,124.335184114137)) ;
#69514=CARTESIAN_POINT('Ctrl Pts',(-18.2569780632649,38.9569965879559,124.383630345431)) ;
#69515=CARTESIAN_POINT('Ctrl Pts',(-18.4874417365958,38.7770075075931,124.189274418743)) ;
#69516=CARTESIAN_POINT('Ctrl Pts',(-18.1050023548241,38.9670311997562,124.168134092341)) ;
#69517=CARTESIAN_POINT('Ctrl Pts',(-18.3658597612924,38.7870421193933,124.016878306509)) ;
#69518=CARTESIAN_POINT('Ctrl Pts',(-17.9935211048472,38.9770562085294,123.929428614842)) ;
#69519=CARTESIAN_POINT('Ctrl Pts',(-18.2766733718385,38.7970671281665,123.825914551769)) ;
#69520=CARTESIAN_POINT('Ctrl Pts',(-17.9258146375031,38.9869081333709,123.679534933401)) ;
#69521=CARTESIAN_POINT('Ctrl Pts',(-18.2225068346885,38.8069190530081,123.62600081153)) ;
#69522=CARTESIAN_POINT('Ctrl Pts',(-17.9017999976252,38.9968990716936,123.418116000194)) ;
#69523=CARTESIAN_POINT('Ctrl Pts',(-18.2032934378327,38.8169099913308,123.416865957209)) ;
#69524=CARTESIAN_POINT('Ctrl Pts',(-17.9232192572526,39.0068170568401,123.158331775182)) ;
#69525=CARTESIAN_POINT('Ctrl Pts',(-18.2204270837738,38.8268279764772,123.209038890302)) ;
#69526=CARTESIAN_POINT('Ctrl Pts',(-17.9900801459671,39.0168451577356,122.903447812489)) ;
#69527=CARTESIAN_POINT('Ctrl Pts',(-18.2739141162152,38.8368560773727,123.005131251338)) ;
#69528=CARTESIAN_POINT('Ctrl Pts',(-18.0985256645866,39.0267303986782,122.66738650819)) ;
#69529=CARTESIAN_POINT('Ctrl Pts',(-18.3606686866534,38.8467413183153,122.816282007666)) ;
#69530=CARTESIAN_POINT('Ctrl Pts',(-18.2473354546933,39.0367195116448,122.451127866607)) ;
#69531=CARTESIAN_POINT('Ctrl Pts',(-18.4797149123304,38.8567304312819,122.643274141846)) ;
#69532=CARTESIAN_POINT('Ctrl Pts',(-18.4328121554963,39.0467615759856,122.263416874408)) ;
#69533=CARTESIAN_POINT('Ctrl Pts',(-18.628095065177,38.8667724956227,122.49310404951)) ;
#69534=CARTESIAN_POINT('Ctrl Pts',(-18.6432316642718,39.0565907773901,122.113588566168)) ;
#69535=CARTESIAN_POINT('Ctrl Pts',(-18.7964289710917,38.8766016970272,122.373240345266)) ;
#69536=CARTESIAN_POINT('Ctrl Pts',(-18.8804006960058,39.0665976181483,122.000064282247)) ;
#69537=CARTESIAN_POINT('Ctrl Pts',(-18.986163304992,38.8866085377854,122.282419197407)) ;
#69538=CARTESIAN_POINT('Ctrl Pts',(-19.1333031196278,39.0765851423402,121.929712194851)) ;
#69539=CARTESIAN_POINT('Ctrl Pts',(-19.1884846090727,38.8965960619773,122.226135721828)) ;
#69540=CARTESIAN_POINT('Ctrl Pts',(-19.3956318554856,39.0866147881488,121.90442252384)) ;
#69541=CARTESIAN_POINT('Ctrl Pts',(-19.3983474399373,38.9066257077859,122.205902107864)) ;
#69542=CARTESIAN_POINT('Ctrl Pts',(-19.6543650766534,39.0964888188876,121.924438378725)) ;
#69543=CARTESIAN_POINT('Ctrl Pts',(-19.6053336278132,38.9164997385247,122.221912828069)) ;
#69544=CARTESIAN_POINT('Ctrl Pts',(-19.9088952559089,39.1064881417517,121.989562946881)) ;
#69545=CARTESIAN_POINT('Ctrl Pts',(-19.8089581746776,38.9264990613888,122.274010548606)) ;
#69546=CARTESIAN_POINT('Ctrl Pts',(-20.1463184204116,39.1163989773273,122.096736593804)) ;
#69547=CARTESIAN_POINT('Ctrl Pts',(-19.9988971842688,38.9364098969644,122.359747484487)) ;
#69548=CARTESIAN_POINT('Ctrl Pts',(-20.3645137350782,39.1264532253013,122.245659936878)) ;
#69549=CARTESIAN_POINT('Ctrl Pts',(-20.1734546335938,38.9464641449384,122.47888456104)) ;
#69550=CARTESIAN_POINT('Ctrl Pts',(-20.5501363523251,39.136311969564,122.426460600573)) ;
#69551=CARTESIAN_POINT('Ctrl Pts',(-20.3219537705766,38.9563228892011,122.623523276543)) ;
#69552=CARTESIAN_POINT('Ctrl Pts',(-20.7048400636721,39.146380055637,122.641049209758)) ;
#69553=CARTESIAN_POINT('Ctrl Pts',(-20.445718474219,38.9663909752741,122.795193064183)) ;
#69554=CARTESIAN_POINT('Ctrl Pts',(-20.8175117263284,39.1562355388165,122.87427274074)) ;
#69555=CARTESIAN_POINT('Ctrl Pts',(-20.5358574288074,38.9762464584537,122.981770549878)) ;
#69556=CARTESIAN_POINT('Ctrl Pts',(-20.889721867706,39.1662303846107,123.126796707764)) ;
#69557=CARTESIAN_POINT('Ctrl Pts',(-20.5936275684775,38.9862413042478,123.183789061337)) ;
#69558=CARTESIAN_POINT('Ctrl Pts',(-20.9165245762999,39.1762616802733,123.389047651322)) ;
#69559=CARTESIAN_POINT('Ctrl Pts',(-20.6150717949923,38.9962725999104,123.393589604221)) ;
#69560=CARTESIAN_POINT('Ctrl Pts',(-20.8981112102425,39.1861282235631,123.647684462324)) ;
#69561=CARTESIAN_POINT('Ctrl Pts',(-20.6003432386068,39.0061391432003,123.600498792257)) ;
#69562=CARTESIAN_POINT('Ctrl Pts',(-20.8347179859735,39.1961156193265,123.902339731277)) ;
#69563=CARTESIAN_POINT('Ctrl Pts',(-20.5496307722175,39.0161265389636,123.804223432309)) ;
#69564=CARTESIAN_POINT('Ctrl Pts',(-20.728622932385,39.2060606600565,124.14122345198)) ;
#69565=CARTESIAN_POINT('Ctrl Pts',(-20.4647567795798,39.0260715796936,123.9953311149)) ;
#69566=CARTESIAN_POINT('Ctrl Pts',(-20.5811155220166,39.2161051662732,124.360088757602)) ;
#69567=CARTESIAN_POINT('Ctrl Pts',(-20.3467526264366,39.0361160859103,124.170424573902)) ;
#69568=CARTESIAN_POINT('Ctrl Pts',(-20.4012820501656,39.2259686724105,124.546795194446)) ;
#69569=CARTESIAN_POINT('Ctrl Pts',(-20.2028876468785,39.0459795920477,124.319790982306)) ;
#69570=CARTESIAN_POINT('Ctrl Pts',(-20.1893406639608,39.2359615332466,124.701780528445)) ;
#69571=CARTESIAN_POINT('Ctrl Pts',(-20.033335900681,39.0559724528837,124.443780983451)) ;
#69572=CARTESIAN_POINT('Ctrl Pts',(-19.9552664329016,39.2458877269655,124.816982053056)) ;
#69573=CARTESIAN_POINT('Ctrl Pts',(-19.8460776484438,39.0658986466027,124.535944103352)) ;
#69574=CARTESIAN_POINT('Ctrl Pts',(-19.7024842949339,39.2559066529981,124.890499840195)) ;
#69575=CARTESIAN_POINT('Ctrl Pts',(-19.643852594965,39.0759175726352,124.594760445571)) ;
#69576=CARTESIAN_POINT('Ctrl Pts',(-19.4434484431289,39.2658216523657,124.918965884066)) ;
#69577=CARTESIAN_POINT('Ctrl Pts',(-19.4366243284276,39.0858325720028,124.61753546939)) ;
#69578=CARTESIAN_POINT('Ctrl Pts',(-19.1798154010535,39.275876423923,124.901733325748)) ;
#69579=CARTESIAN_POINT('Ctrl Pts',(-19.2257177564351,39.0958873435601,124.603751640336)) ;
#69580=CARTESIAN_POINT('Ctrl Pts',(-18.9280744033614,39.2857353862206,124.840355827184)) ;
#69581=CARTESIAN_POINT('Ctrl Pts',(-19.0243246392442,39.1057463058577,124.55465185544)) ;
#69582=CARTESIAN_POINT('Ctrl Pts',(-18.6874294683808,39.2957296300584,124.735252472311)) ;
#69583=CARTESIAN_POINT('Ctrl Pts',(-18.8318078469648,39.1157405496955,124.470571256637)) ;
#69584=CARTESIAN_POINT('Ctrl Pts',(-18.4700628513266,39.3056548594826,124.591021419432)) ;
#69585=CARTESIAN_POINT('Ctrl Pts',(-18.6579133993353,39.1256657791198,124.355188343277)) ;
#69586=CARTESIAN_POINT('Ctrl Pts',(-18.2791321697973,39.3156828233741,124.409439034504)) ;
#69587=CARTESIAN_POINT('Ctrl Pts',(-18.5051673400138,39.1356937430112,124.209924100878)) ;
#69588=CARTESIAN_POINT('Ctrl Pts',(-18.1245827427517,39.3255690830045,124.200558385393)) ;
#69589=CARTESIAN_POINT('Ctrl Pts',(-18.381526045183,39.1455800026416,124.042820995344)) ;
#69590=CARTESIAN_POINT('Ctrl Pts',(-18.0068578913663,39.3356008460823,123.964729079241)) ;
#69591=CARTESIAN_POINT('Ctrl Pts',(-18.2873441695228,39.1556117657195,123.854158607123)) ;
#69592=CARTESIAN_POINT('Ctrl Pts',(-17.9327236697777,39.3454824723765,123.715808953631)) ;
#69593=CARTESIAN_POINT('Ctrl Pts',(-18.2280346488682,39.1654933920136,123.65502319765)) ;
#69594=CARTESIAN_POINT('Ctrl Pts',(-17.9023337792867,39.3555442418626,123.453187507275)) ;
#69595=CARTESIAN_POINT('Ctrl Pts',(-18.2037205033373,39.1755551614998,123.444926368231)) ;
#69596=CARTESIAN_POINT('Ctrl Pts',(-17.9176154685571,39.3654021093581,123.194552719115)) ;
#69597=CARTESIAN_POINT('Ctrl Pts',(-18.2159436064791,39.1854130289952,123.238018412343)) ;
#69598=CARTESIAN_POINT('Ctrl Pts',(-17.9778056084377,39.3753937344755,122.939007178567)) ;
#69599=CARTESIAN_POINT('Ctrl Pts',(-18.2640935243759,39.1954046541126,123.033581500678)) ;
#69600=CARTESIAN_POINT('Ctrl Pts',(-18.0809465923163,39.3853305335837,122.699093789421)) ;
#69601=CARTESIAN_POINT('Ctrl Pts',(-18.3466042525769,39.2053414532208,122.841649902938)) ;
#69602=CARTESIAN_POINT('Ctrl Pts',(-18.2246316582653,39.3953213631411,122.479348914402)) ;
#69603=CARTESIAN_POINT('Ctrl Pts',(-18.4615504185501,39.2153322827782,122.66585281308)) ;
#69604=CARTESIAN_POINT('Ctrl Pts',(-18.4050975254076,39.4053445988542,122.287476075996)) ;
#69605=CARTESIAN_POINT('Ctrl Pts',(-18.6059214265816,39.2253555184914,122.512353066652)) ;
#69606=CARTESIAN_POINT('Ctrl Pts',(-18.6133254066964,39.4152409468834,122.131679228761)) ;
#69607=CARTESIAN_POINT('Ctrl Pts',(-18.7725024389883,39.2352518665205,122.387713758651)) ;
#69608=CARTESIAN_POINT('Ctrl Pts',(-18.8473919143103,39.4252305093859,122.012791074316)) ;
#69609=CARTESIAN_POINT('Ctrl Pts',(-18.9597546642961,39.245241429023,122.292601282324)) ;
#69610=CARTESIAN_POINT('Ctrl Pts',(-19.0999512728563,39.4352708170704,121.936479082214)) ;
#69611=CARTESIAN_POINT('Ctrl Pts',(-19.1618012471887,39.2552817367076,122.231549573829)) ;
#69612=CARTESIAN_POINT('Ctrl Pts',(-19.3567329848095,39.4451131204176,121.905300141157)) ;
#69613=CARTESIAN_POINT('Ctrl Pts',(-19.3672271092616,39.2651240400548,122.206604238954)) ;
#69614=CARTESIAN_POINT('Ctrl Pts',(-19.6197445019835,39.4551368286967,121.919081532484)) ;
#69615=CARTESIAN_POINT('Ctrl Pts',(-19.5776343212279,39.2751477483338,122.217627049978)) ;
#69616=CARTESIAN_POINT('Ctrl Pts',(-19.9583923044283,39.4683590061644,121.997113385212)) ;
#69617=CARTESIAN_POINT('Ctrl Pts',(-19.8485635151233,39.2883699258015,122.280050331721)) ;
#69618=CARTESIAN_POINT('Ctrl Pts',(-20.2706261181306,39.4816515912237,122.162206025503)) ;
#69619=CARTESIAN_POINT('Ctrl Pts',(-20.0983757918957,39.3016625108608,122.412145538287)) ;
#69620=CARTESIAN_POINT('Ctrl Pts',(-20.5265366200315,39.4949364471453,122.399782063078)) ;
#69621=CARTESIAN_POINT('Ctrl Pts',(-20.3030677424335,39.3149473667824,122.602175696939)) ;
#69622=CARTESIAN_POINT('Ctrl Pts',(-20.6848475062148,39.5049086743181,122.608570519109)) ;
#69623=CARTESIAN_POINT('Ctrl Pts',(-20.4297258566199,39.3249195939552,122.769211054602)) ;
#69624=CARTESIAN_POINT('Ctrl Pts',(-20.8041722375231,39.5148172907571,122.840044926829)) ;
#69625=CARTESIAN_POINT('Ctrl Pts',(-20.5251856336139,39.3348282103942,122.954388023249)) ;
#69626=CARTESIAN_POINT('Ctrl Pts',(-20.8825021974907,39.5248704961408,123.09232602936)) ;
#69627=CARTESIAN_POINT('Ctrl Pts',(-20.5878516382789,39.3448814157779,123.156213664846)) ;
#69628=CARTESIAN_POINT('Ctrl Pts',(-20.9153854640603,39.5347356299011,123.349500706136)) ;
#69629=CARTESIAN_POINT('Ctrl Pts',(-20.6141617865867,39.3547465495382,123.361949101435)) ;
#69630=CARTESIAN_POINT('Ctrl Pts',(-20.8994475638338,39.5480746875274,123.699654940672)) ;
#69631=CARTESIAN_POINT('Ctrl Pts',(-20.6014062025632,39.3680856071645,123.642094456117)) ;
#69632=CARTESIAN_POINT('Ctrl Pts',(-20.7662626209752,39.5646438748606,124.119481950554)) ;
#69633=CARTESIAN_POINT('Ctrl Pts',(-20.4948802699597,39.3846547944977,123.977922342078)) ;
#69634=CARTESIAN_POINT('Ctrl Pts',(-20.4969232972869,39.5812890147116,124.470352991445)) ;
#69635=CARTESIAN_POINT('Ctrl Pts',(-20.2793689415074,39.4012999343487,124.258669314264)) ;
#69636=CARTESIAN_POINT('Ctrl Pts',(-20.2201055636797,39.594561317185,124.682635504472)) ;
#69637=CARTESIAN_POINT('Ctrl Pts',(-20.0579520034563,39.4145722368221,124.428460073727)) ;
#69638=CARTESIAN_POINT('Ctrl Pts',(-19.9875926506158,39.6045422806326,124.803956293346)) ;
#69639=CARTESIAN_POINT('Ctrl Pts',(-19.8719346104858,39.4245532002698,124.525525821103)) ;
#69640=CARTESIAN_POINT('Ctrl Pts',(-19.7385233068285,39.6144841127019,124.882919421765)) ;
#69641=CARTESIAN_POINT('Ctrl Pts',(-19.6726839339702,39.4344950323391,124.588696443466)) ;
#69642=CARTESIAN_POINT('Ctrl Pts',(-19.3916274184842,39.6278036819174,124.929289096296)) ;
#69643=CARTESIAN_POINT('Ctrl Pts',(-19.3951539287029,39.4478146015545,124.625793702536)) ;
#69644=CARTESIAN_POINT('Ctrl Pts',(-18.9557155359981,39.6443338368501,124.873608604834)) ;
#69645=CARTESIAN_POINT('Ctrl Pts',(-19.0464382212822,39.4643447564872,124.581253473117)) ;
#69646=CARTESIAN_POINT('Ctrl Pts',(-18.4827841914937,39.6643555623422,124.629948165702)) ;
#69647=CARTESIAN_POINT('Ctrl Pts',(-18.6680869357579,39.4843664819793,124.386327764593)) ;
#69648=CARTESIAN_POINT('Ctrl Pts',(-18.1247857375982,39.684166958949,124.243642886315)) ;
#69649=CARTESIAN_POINT('Ctrl Pts',(-18.3816862675463,39.5041778785861,124.077284936914)) ;
#69650=CARTESIAN_POINT('Ctrl Pts',(-17.9175888921553,39.7041522076579,123.754678947954)) ;
#69651=CARTESIAN_POINT('Ctrl Pts',(-18.2159257535573,39.524163127295,123.686114759911)) ;
#69652=CARTESIAN_POINT('Ctrl Pts',(-17.8901646194333,39.7240462702938,123.226554358752)) ;
#69653=CARTESIAN_POINT('Ctrl Pts',(-18.1939835441653,39.5440571899309,123.263614485181)) ;
#69654=CARTESIAN_POINT('Ctrl Pts',(-18.0441177194512,39.7439779494674,122.719677099901)) ;
#69655=CARTESIAN_POINT('Ctrl Pts',(-18.3171437873971,39.5639888691045,122.858111428602)) ;
#69656=CARTESIAN_POINT('Ctrl Pts',(-18.3626008286604,39.7639420039394,122.295272619757)) ;
#69657=CARTESIAN_POINT('Ctrl Pts',(-18.5719284738746,39.5839529235765,122.518586147516)) ;
#69658=CARTESIAN_POINT('Ctrl Pts',(-18.8047431638309,39.7838229057023,122.005888410444)) ;
#69659=CARTESIAN_POINT('Ctrl Pts',(-18.9256420531025,39.6038338253394,122.287076349787)) ;
#69660=CARTESIAN_POINT('Ctrl Pts',(-19.3204270314315,39.8037615673107,121.883932996576)) ;
#69661=CARTESIAN_POINT('Ctrl Pts',(-19.3381893000524,39.6237724869478,122.189510074961)) ;
#69662=CARTESIAN_POINT('Ctrl Pts',(-19.8456885699466,39.823658092566,121.945064977875)) ;
#69663=CARTESIAN_POINT('Ctrl Pts',(-19.7583997745947,39.6436690122031,122.238414117191)) ;
#69664=CARTESIAN_POINT('Ctrl Pts',(-20.3189371293568,39.8435531310203,122.180988955681)) ;
#69665=CARTESIAN_POINT('Ctrl Pts',(-20.1370001890922,39.6635640506575,122.427152812222)) ;
#69666=CARTESIAN_POINT('Ctrl Pts',(-20.684435302286,39.8635169543264,122.565581974928)) ;
#69667=CARTESIAN_POINT('Ctrl Pts',(-20.4293997300506,39.6835278739635,122.734826840731)) ;
#69668=CARTESIAN_POINT('Ctrl Pts',(-20.8961892011034,39.8833910784555,123.049543285432)) ;
#69669=CARTESIAN_POINT('Ctrl Pts',(-20.5988040313383,39.7034019980926,123.121997016737)) ;
#69670=CARTESIAN_POINT('Ctrl Pts',(-20.9307446999035,39.9033661541827,123.579345858903)) ;
#69671=CARTESIAN_POINT('Ctrl Pts',(-20.6264486432097,39.7233770738199,123.54583933781)) ;
#69672=CARTESIAN_POINT('Ctrl Pts',(-20.7818723368726,39.9233197235393,124.088346140046)) ;
#69673=CARTESIAN_POINT('Ctrl Pts',(-20.5073509383854,39.7433306431764,123.953040241885)) ;
#69674=CARTESIAN_POINT('Ctrl Pts',(-20.4708597448831,39.9431576337272,124.514109737929)) ;
#69675=CARTESIAN_POINT('Ctrl Pts',(-20.2585393443571,39.7631685533643,124.293652633685)) ;
#69676=CARTESIAN_POINT('Ctrl Pts',(-20.0304987770853,39.9631334622981,124.810695893572)) ;
#69677=CARTESIAN_POINT('Ctrl Pts',(-19.9062499102217,39.7831443819352,124.53092102101)) ;
#69678=CARTESIAN_POINT('Ctrl Pts',(-19.5167467254977,39.9830515070084,124.938262136295)) ;
#69679=CARTESIAN_POINT('Ctrl Pts',(-19.4952471367361,39.8030624266455,124.632973548658)) ;
#69680=CARTESIAN_POINT('Ctrl Pts',(-18.9912829799873,40.002921752796,124.884310017349)) ;
#69681=CARTESIAN_POINT('Ctrl Pts',(-19.0748749155325,39.8229326724332,124.589810226705)) ;
#69682=CARTESIAN_POINT('Ctrl Pts',(-18.512059067701,40.0229707558956,124.651607827821)) ;
#69683=CARTESIAN_POINT('Ctrl Pts',(-18.691496813196,39.8429816755327,124.403647475634)) ;
#69684=CARTESIAN_POINT('Ctrl Pts',(-18.1453823899898,40.0427499971364,124.274685535331)) ;
#69685=CARTESIAN_POINT('Ctrl Pts',(-18.3981551846587,39.8627609167736,124.10210688277)) ;
#69686=CARTESIAN_POINT('Ctrl Pts',(-17.9259795061986,40.0627800608453,123.789764142162)) ;
#69687=CARTESIAN_POINT('Ctrl Pts',(-18.2226350126772,39.8827909804824,123.714169148054)) ;
#69688=CARTESIAN_POINT('Ctrl Pts',(-17.8863640755832,40.0826623457473,123.26273048994)) ;
#69689=CARTESIAN_POINT('Ctrl Pts',(-18.1909445989057,39.9026732653844,123.292541016045)) ;
#69690=CARTESIAN_POINT('Ctrl Pts',(-18.0275270007879,40.1025446466403,122.753544083108)) ;
#69691=CARTESIAN_POINT('Ctrl Pts',(-18.3038777717334,39.9225555662774,122.885191650426)) ;
#69692=CARTESIAN_POINT('Ctrl Pts',(-18.3357032518353,40.1225277562586,122.320964219485)) ;
#69693=CARTESIAN_POINT('Ctrl Pts',(-18.5504210502982,39.9425386758957,122.539129268786)) ;
#69694=CARTESIAN_POINT('Ctrl Pts',(-18.7710249752049,40.1424181516365,122.020953450762)) ;
#69695=CARTESIAN_POINT('Ctrl Pts',(-18.8986807002394,39.9624290712736,122.299122526392)) ;
#69696=CARTESIAN_POINT('Ctrl Pts',(-19.2824556627369,40.1623149416708,121.886718883341)) ;
#69697=CARTESIAN_POINT('Ctrl Pts',(-19.3078267411535,39.9823258613079,122.191737773976)) ;
#69698=CARTESIAN_POINT('Ctrl Pts',(-19.809682792952,40.1822319956124,121.93454660401)) ;
#69699=CARTESIAN_POINT('Ctrl Pts',(-19.7296086094093,40.0022429152495,122.230003389753)) ;
#69700=CARTESIAN_POINT('Ctrl Pts',(-20.290985297749,40.2022355438159,122.160572440253)) ;
#69701=CARTESIAN_POINT('Ctrl Pts',(-20.1146490294153,40.022246463453,122.410827178833)) ;
#69702=CARTESIAN_POINT('Ctrl Pts',(-20.6644175476188,40.2221738374685,122.536530476513)) ;
#69703=CARTESIAN_POINT('Ctrl Pts',(-20.4133927604481,40.0421847571056,122.711596130847)) ;
#69704=CARTESIAN_POINT('Ctrl Pts',(-20.8870164933769,40.2419953249014,123.014022848812)) ;
#69705=CARTESIAN_POINT('Ctrl Pts',(-20.591468541711,40.0620062445386,123.093592852938)) ;
#69706=CARTESIAN_POINT('Ctrl Pts',(-20.9342078753314,40.2619737178923,123.54285440319)) ;
#69707=CARTESIAN_POINT('Ctrl Pts',(-20.629219041352,40.0819846375294,123.51665686398)) ;
#69708=CARTESIAN_POINT('Ctrl Pts',(-20.798306014332,40.281872099506,124.054044528013)) ;
#69709=CARTESIAN_POINT('Ctrl Pts',(-20.5204887803847,40.1018830191431,123.925614389338)) ;
#69710=CARTESIAN_POINT('Ctrl Pts',(-20.5470819880528,40.2984550302359,124.416062159147)) ;
#69711=CARTESIAN_POINT('Ctrl Pts',(-20.319521718774,40.118465949873,124.215207873857)) ;
#69712=CARTESIAN_POINT('Ctrl Pts',(-20.281028441282,40.3117292658247,124.641768863592)) ;
#69713=CARTESIAN_POINT('Ctrl Pts',(-20.1066630077281,40.1317401854619,124.39578795603)) ;
#69714=CARTESIAN_POINT('Ctrl Pts',(-20.0530654837522,40.3217756832809,124.774877815114)) ;
#69715=CARTESIAN_POINT('Ctrl Pts',(-19.9242972790721,40.1417866029181,124.50226984556)) ;
#69716=CARTESIAN_POINT('Ctrl Pts',(-19.810464403995,40.3316209085002,124.864833820521)) ;
#69717=CARTESIAN_POINT('Ctrl Pts',(-19.7302036734289,40.1516318281373,124.574233889448)) ;
#69718=CARTESIAN_POINT('Ctrl Pts',(-19.4658929191224,40.3449558795396,124.928504806225)) ;
#69719=CARTESIAN_POINT('Ctrl Pts',(-19.4546005727731,40.1649667991767,124.625166764035)) ;
#69720=CARTESIAN_POINT('Ctrl Pts',(-19.0264390688312,40.3615387363322,124.893652813554)) ;
#69721=CARTESIAN_POINT('Ctrl Pts',(-19.1029686872478,40.1815496559694,124.597278988789)) ;
#69722=CARTESIAN_POINT('Ctrl Pts',(-18.6239205040509,40.3781817386816,124.71045606654)) ;
#69723=CARTESIAN_POINT('Ctrl Pts',(-18.7810022090588,40.1981926583188,124.450732338554)) ;
#69724=CARTESIAN_POINT('Ctrl Pts',(-18.3550031410799,40.3914254697133,124.489405088402)) ;
#69725=CARTESIAN_POINT('Ctrl Pts',(-18.5658419708258,40.2114363893504,124.273876441203)) ;
#69726=CARTESIAN_POINT('Ctrl Pts',(-18.1831556506858,40.4014798643879,124.288773158582)) ;
#69727=CARTESIAN_POINT('Ctrl Pts',(-18.4283713813035,40.221490784025,124.113372135424)) ;
#69728=CARTESIAN_POINT('Ctrl Pts',(-18.0512693189918,40.4113209257765,124.066262657595)) ;
#69729=CARTESIAN_POINT('Ctrl Pts',(-18.3228626055422,40.2313318454136,123.935361746005)) ;
#69730=CARTESIAN_POINT('Ctrl Pts',(-17.9577246777451,40.421387150133,123.818872622899)) ;
#69731=CARTESIAN_POINT('Ctrl Pts',(-18.2480294373586,40.2413980697701,123.737449245068)) ;
#69732=CARTESIAN_POINT('Ctrl Pts',(-17.9095230457467,40.4312677630526,123.563691114021)) ;
#69733=CARTESIAN_POINT('Ctrl Pts',(-18.2094701905773,40.2512786826897,123.533303479069)) ;
#69734=CARTESIAN_POINT('Ctrl Pts',(-17.9058281378729,40.4412610562122,123.30114626875)) ;
#69735=CARTESIAN_POINT('Ctrl Pts',(-18.2065165443278,40.2612719758493,123.323267634952)) ;
#69736=CARTESIAN_POINT('Ctrl Pts',(-17.9475138799179,40.4512120644359,123.042941598617)) ;
#69737=CARTESIAN_POINT('Ctrl Pts',(-18.2398673462306,40.271222984073,123.116704268342)) ;
#69738=CARTESIAN_POINT('Ctrl Pts',(-18.0344070397604,40.4612605787978,122.793614478542)) ;
#69739=CARTESIAN_POINT('Ctrl Pts',(-18.3093839709595,40.281271498435,122.917243386907)) ;
#69740=CARTESIAN_POINT('Ctrl Pts',(-18.1603863836437,40.4711020848605,122.567719550063)) ;
#69741=CARTESIAN_POINT('Ctrl Pts',(-18.4101694281105,40.2911130044976,122.736528509964)) ;
#69742=CARTESIAN_POINT('Ctrl Pts',(-18.3255788630243,40.4810877374902,122.36388078949)) ;
#69743=CARTESIAN_POINT('Ctrl Pts',(-18.5423251289196,40.3010986571273,122.573458977904)) ;
#69744=CARTESIAN_POINT('Ctrl Pts',(-18.5227257140879,40.4910267463351,122.192496536557)) ;
#69745=CARTESIAN_POINT('Ctrl Pts',(-18.7000440471516,40.3110376659722,122.436353315188)) ;
#69746=CARTESIAN_POINT('Ctrl Pts',(-18.7489120153398,40.5010676716281,122.056659651422)) ;
#69747=CARTESIAN_POINT('Ctrl Pts',(-18.8809942079959,40.3210785912652,122.327685771661)) ;
#69748=CARTESIAN_POINT('Ctrl Pts',(-18.9915421154482,40.510957993383,121.963416273453)) ;
#69749=CARTESIAN_POINT('Ctrl Pts',(-19.0750990226228,40.3309689130201,122.253093205079)) ;
#69750=CARTESIAN_POINT('Ctrl Pts',(-19.249284101431,40.5209539667164,121.912814957505)) ;
#69751=CARTESIAN_POINT('Ctrl Pts',(-19.2812929812387,40.3409648863536,122.212614377811)) ;
#69752=CARTESIAN_POINT('Ctrl Pts',(-19.5102329048635,40.5308853662985,121.907746825893)) ;
#69753=CARTESIAN_POINT('Ctrl Pts',(-19.4900519685887,40.3508962859356,122.208562125718)) ;
#69754=CARTESIAN_POINT('Ctrl Pts',(-19.7700821945994,40.5408909067755,121.947997275359)) ;
#69755=CARTESIAN_POINT('Ctrl Pts',(-19.697930995272,40.3609018264127,122.240764692487)) ;
#69756=CARTESIAN_POINT('Ctrl Pts',(-20.0195011590798,40.5509238907068,122.033437044935)) ;
#69757=CARTESIAN_POINT('Ctrl Pts',(-19.8974654062638,40.370934810344,122.30911863456)) ;
#69758=CARTESIAN_POINT('Ctrl Pts',(-20.2464637604241,40.5607795215337,122.158246335581)) ;
#69759=CARTESIAN_POINT('Ctrl Pts',(-20.0790342417892,40.3807904411708,122.408967940428)) ;
#69760=CARTESIAN_POINT('Ctrl Pts',(-20.4514141919689,40.5707789237268,122.322629146748)) ;
#69761=CARTESIAN_POINT('Ctrl Pts',(-20.2429931328991,40.390789843364,122.540475886912)) ;
#69762=CARTESIAN_POINT('Ctrl Pts',(-20.623177160939,40.5806733930879,122.517901168788)) ;
#69763=CARTESIAN_POINT('Ctrl Pts',(-20.3804017081287,40.400684312725,122.696694807102)) ;
#69764=CARTESIAN_POINT('Ctrl Pts',(-20.7606139057598,40.5907365072521,122.743776897285)) ;
#69765=CARTESIAN_POINT('Ctrl Pts',(-20.4903492208581,40.4107474268893,122.87739656958)) ;
#69766=CARTESIAN_POINT('Ctrl Pts',(-20.8549063786372,40.6005761529685,122.984593090461)) ;
#69767=CARTESIAN_POINT('Ctrl Pts',(-20.5657810296931,40.4205870726056,123.070050018048)) ;
#69768=CARTESIAN_POINT('Ctrl Pts',(-20.9074265587478,40.6106393205242,123.243737629738)) ;
#69769=CARTESIAN_POINT('Ctrl Pts',(-20.6077950427695,40.4306502401614,123.277366118892)) ;
#69770=CARTESIAN_POINT('Ctrl Pts',(-20.9138213840196,40.6205335763191,123.50369845043)) ;
#69771=CARTESIAN_POINT('Ctrl Pts',(-20.6129087015084,40.4405444959563,123.48533456448)) ;
#69772=CARTESIAN_POINT('Ctrl Pts',(-20.8755072031584,40.6304753547788,123.762100783259)) ;
#69773=CARTESIAN_POINT('Ctrl Pts',(-20.5822552681282,40.4504862744159,123.692055906574)) ;
#69774=CARTESIAN_POINT('Ctrl Pts',(-20.7924699762297,40.640478047609,124.011537115954)) ;
#69775=CARTESIAN_POINT('Ctrl Pts',(-20.5158234865121,40.4604889672461,123.891604236471)) ;
#69776=CARTESIAN_POINT('Ctrl Pts',(-20.6666615752292,40.6505120695628,124.243257679907)) ;
#69777=CARTESIAN_POINT('Ctrl Pts',(-20.4151748534295,40.4705229891999,124.076979664182)) ;
#69778=CARTESIAN_POINT('Ctrl Pts',(-20.5058740591058,40.6603598606518,124.446047890609)) ;
#69779=CARTESIAN_POINT('Ctrl Pts',(-20.2865434507489,40.480370780289,124.239210154722)) ;
#69780=CARTESIAN_POINT('Ctrl Pts',(-20.3100969713907,40.6703413852009,124.620584309683)) ;
#69781=CARTESIAN_POINT('Ctrl Pts',(-20.1299205038193,40.490352304838,124.378837647099)) ;
#69782=CARTESIAN_POINT('Ctrl Pts',(-20.0876630799493,40.6802906086918,124.75801282759)) ;
#69783=CARTESIAN_POINT('Ctrl Pts',(-19.9519724829499,40.5003015283289,124.488778579875)) ;
#69784=CARTESIAN_POINT('Ctrl Pts',(-19.8436735816779,40.6902882649084,124.85551512015)) ;
#69785=CARTESIAN_POINT('Ctrl Pts',(-19.7567802051122,40.5102991845455,124.566778487717)) ;
#69786=CARTESIAN_POINT('Ctrl Pts',(-19.5853011891557,40.7003284779634,124.908895920478)) ;
#69787=CARTESIAN_POINT('Ctrl Pts',(-19.5500818185997,40.5203393976006,124.609481080196)) ;
#69788=CARTESIAN_POINT('Ctrl Pts',(-19.3271425182227,40.7101565252397,124.917006738006)) ;
#69789=CARTESIAN_POINT('Ctrl Pts',(-19.3435554357432,40.5301674448768,124.615967681454)) ;
#69790=CARTESIAN_POINT('Ctrl Pts',(-19.0655819825205,40.7202108722721,124.87973320103)) ;
#69791=CARTESIAN_POINT('Ctrl Pts',(-19.1343072015728,40.5402217919092,124.58614687555)) ;
#69792=CARTESIAN_POINT('Ctrl Pts',(-18.8174100404169,40.7301520086006,124.798108890604)) ;
#69793=CARTESIAN_POINT('Ctrl Pts',(-18.9357705393896,40.5501629282377,124.520845572302)) ;
#69794=CARTESIAN_POINT('Ctrl Pts',(-18.5876566119404,40.7400562416803,124.675804537039)) ;
#69795=CARTESIAN_POINT('Ctrl Pts',(-18.7519690826901,40.5600671613174,124.423000582265)) ;
#69796=CARTESIAN_POINT('Ctrl Pts',(-18.3798041844874,40.7501029385239,124.513046489696)) ;
#69797=CARTESIAN_POINT('Ctrl Pts',(-18.5856882820567,40.5701138581611,124.292792552084)) ;
#69798=CARTESIAN_POINT('Ctrl Pts',(-18.2058043531865,40.7599984898042,124.319735002295)) ;
#69799=CARTESIAN_POINT('Ctrl Pts',(-18.4464901583571,40.5800094094413,124.138142422738)) ;
#69800=CARTESIAN_POINT('Ctrl Pts',(-18.0657367626924,40.7700605676437,124.095504335531)) ;
#69801=CARTESIAN_POINT('Ctrl Pts',(-18.3344376418936,40.5900714872808,123.958756744868)) ;
#69802=CARTESIAN_POINT('Ctrl Pts',(-17.9687267603788,40.7799032767398,123.855697491767)) ;
#69803=CARTESIAN_POINT('Ctrl Pts',(-18.2568316638286,40.5999141963769,123.766911199684)) ;
#69804=CARTESIAN_POINT('Ctrl Pts',(-17.9134237543617,40.7898940089782,123.599076400319)) ;
#69805=CARTESIAN_POINT('Ctrl Pts',(-18.2125910590899,40.6099049286153,123.561614081908)) ;
#69806=CARTESIAN_POINT('Ctrl Pts',(-17.9036209757213,40.799822034207,123.33834843595)) ;
#69807=CARTESIAN_POINT('Ctrl Pts',(-18.2047506639829,40.6198329538441,123.353032033196)) ;
#69808=CARTESIAN_POINT('Ctrl Pts',(-17.9390103972283,40.8098101808575,123.07826099235)) ;
#69809=CARTESIAN_POINT('Ctrl Pts',(-18.2330639096619,40.6298211004947,123.144962455833)) ;
#69810=CARTESIAN_POINT('Ctrl Pts',(-18.0197805146774,40.8198451986975,122.827221506658)) ;
#69811=CARTESIAN_POINT('Ctrl Pts',(-18.2976817439703,40.6398561183346,122.944131364963)) ;
#69812=CARTESIAN_POINT('Ctrl Pts',(-18.1405769536225,40.8297099958027,122.597859805826)) ;
#69813=CARTESIAN_POINT('Ctrl Pts',(-18.394320133305,40.6497209154398,122.76064343955)) ;
#69814=CARTESIAN_POINT('Ctrl Pts',(-18.3003100262152,40.8396707281588,122.390481778754)) ;
#69815=CARTESIAN_POINT('Ctrl Pts',(-18.5221077146717,40.6596816477959,122.594742235113)) ;
#69816=CARTESIAN_POINT('Ctrl Pts',(-18.4953203364736,40.8497041905558,122.213037685501)) ;
#69817=CARTESIAN_POINT('Ctrl Pts',(-18.6781171657498,40.6697151101929,122.452788175949)) ;
#69818=CARTESIAN_POINT('Ctrl Pts',(-18.7146955767961,40.8595897247672,122.073836456238)) ;
#69819=CARTESIAN_POINT('Ctrl Pts',(-18.8536176951084,40.6796006444043,122.341428911214)) ;
#69820=CARTESIAN_POINT('Ctrl Pts',(-18.9592101605245,40.8696545654472,121.973078301155)) ;
#69821=CARTESIAN_POINT('Ctrl Pts',(-19.0492301753213,40.6896654850843,122.260823821511)) ;
#69822=CARTESIAN_POINT('Ctrl Pts',(-19.2119712899475,40.8795026971761,121.917403865115)) ;
#69823=CARTESIAN_POINT('Ctrl Pts',(-19.2514386073647,40.6995136168132,122.216286026283)) ;
#69824=CARTESIAN_POINT('Ctrl Pts',(-19.4752106016322,40.8895301941662,121.905583046178)) ;
#69825=CARTESIAN_POINT('Ctrl Pts',(-19.4620301548535,40.7095411138033,122.206830852572)) ;
#69826=CARTESIAN_POINT('Ctrl Pts',(-19.7364587404572,40.8995586462113,121.940346685251)) ;
#69827=CARTESIAN_POINT('Ctrl Pts',(-19.6710285077072,40.7195695658484,122.234643374607)) ;
#69828=CARTESIAN_POINT('Ctrl Pts',(-19.9832352577145,40.9094039127754,122.018011497405)) ;
#69829=CARTESIAN_POINT('Ctrl Pts',(-19.8684484097077,40.7294148324125,122.296776407657)) ;
#69830=CARTESIAN_POINT('Ctrl Pts',(-20.2165109099258,40.9193945857163,122.138492853158)) ;
#69831=CARTESIAN_POINT('Ctrl Pts',(-20.0550681579274,40.7394055053534,122.393162648683)) ;
#69832=CARTESIAN_POINT('Ctrl Pts',(-20.4259458604295,40.9294324678048,122.29886132802)) ;
#69833=CARTESIAN_POINT('Ctrl Pts',(-20.2226152908657,40.7494433874419,122.521458685121)) ;
#69834=CARTESIAN_POINT('Ctrl Pts',(-20.6012563123727,40.9392768382444,122.489117146691)) ;
#69835=CARTESIAN_POINT('Ctrl Pts',(-20.3628619804321,40.7592877578816,122.67366360375)) ;
#69836=CARTESIAN_POINT('Ctrl Pts',(-20.7432721400069,40.9492616656398,122.709711313099)) ;
#69837=CARTESIAN_POINT('Ctrl Pts',(-20.4764734396498,40.7692725852769,122.850139473825)) ;
#69838=CARTESIAN_POINT('Ctrl Pts',(-20.844502824681,40.9592011110451,122.950536538216)) ;
#69839=CARTESIAN_POINT('Ctrl Pts',(-20.5574566433733,40.7792120306822,123.042799745308)) ;
#69840=CARTESIAN_POINT('Ctrl Pts',(-20.9028785373405,40.969241115331,123.20781127082)) ;
#69841=CARTESIAN_POINT('Ctrl Pts',(-20.6041559783071,40.7892520349681,123.24861993569)) ;
#69842=CARTESIAN_POINT('Ctrl Pts',(-20.9156810985871,40.9791282245166,123.46734861019)) ;
#69843=CARTESIAN_POINT('Ctrl Pts',(-20.6143967389084,40.7991391441538,123.456249117252)) ;
#69844=CARTESIAN_POINT('Ctrl Pts',(-20.8831859202662,40.9891282844191,123.728082234662)) ;
#69845=CARTESIAN_POINT('Ctrl Pts',(-20.5883994360712,40.8091392040562,123.664835757104)) ;
#69846=CARTESIAN_POINT('Ctrl Pts',(-20.8067389220528,40.9990457003338,123.977282854265)) ;
#69847=CARTESIAN_POINT('Ctrl Pts',(-20.5272409208135,40.8190566199709,123.864195371173)) ;
#69848=CARTESIAN_POINT('Ctrl Pts',(-20.6866067690655,41.0090925150746,124.212346711425)) ;
#69849=CARTESIAN_POINT('Ctrl Pts',(-20.4311340955001,40.8291034347117,124.052246084703)) ;
#69850=CARTESIAN_POINT('Ctrl Pts',(-20.5303634279957,41.0189679922713,124.419613620439)) ;
#69851=CARTESIAN_POINT('Ctrl Pts',(-20.3061390542249,40.8389789119084,124.218058285258)) ;
#69852=CARTESIAN_POINT('Ctrl Pts',(-20.3371972791705,41.0290240879925,124.599886515678)) ;
#69853=CARTESIAN_POINT('Ctrl Pts',(-20.1516052586008,40.8490350076296,124.362275967077)) ;
#69854=CARTESIAN_POINT('Ctrl Pts',(-20.1192272911797,41.0389172500076,124.741681401867)) ;
#69855=CARTESIAN_POINT('Ctrl Pts',(-19.9772293226388,40.8589281696447,124.475710604766)) ;
#69856=CARTESIAN_POINT('Ctrl Pts',(-19.8759671921668,41.0489794860302,124.845254462117)) ;
#69857=CARTESIAN_POINT('Ctrl Pts',(-19.7826206014674,40.8689904056673,124.558568216301)) ;
#69858=CARTESIAN_POINT('Ctrl Pts',(-19.6239559484601,41.0588239516591,124.903758180381)) ;
#69859=CARTESIAN_POINT('Ctrl Pts',(-19.5810124074109,40.8788348712962,124.605369962764)) ;
#69860=CARTESIAN_POINT('Ctrl Pts',(-19.3626471098562,41.0687840443633,124.918720690763)) ;
#69861=CARTESIAN_POINT('Ctrl Pts',(-19.3719656563023,40.8887949640004,124.61733915855)) ;
#69862=CARTESIAN_POINT('Ctrl Pts',(-19.1007386053563,41.0788223333443,124.887329010187)) ;
#69863=CARTESIAN_POINT('Ctrl Pts',(-19.16243883266,40.8988332529814,124.592224889164)) ;
#69864=CARTESIAN_POINT('Ctrl Pts',(-18.8522137572535,41.0886956564505,124.812656518733)) ;
#69865=CARTESIAN_POINT('Ctrl Pts',(-18.9636200453775,40.9087065760876,124.532486393259)) ;
#69866=CARTESIAN_POINT('Ctrl Pts',(-18.6158596069558,41.0987688405356,124.693571352366)) ;
#69867=CARTESIAN_POINT('Ctrl Pts',(-18.7745367877756,40.9187797601727,124.437217376295)) ;
#69868=CARTESIAN_POINT('Ctrl Pts',(-18.4088042083935,41.1085893528235,124.539431437794)) ;
#69869=CARTESIAN_POINT('Ctrl Pts',(-18.6088939047249,40.9286002724607,124.313905598339)) ;
#69870=CARTESIAN_POINT('Ctrl Pts',(-18.2269108302998,41.1186673489393,124.347022071441)) ;
#69871=CARTESIAN_POINT('Ctrl Pts',(-18.4633794360143,40.9386782685765,124.159977371275)) ;
#69872=CARTESIAN_POINT('Ctrl Pts',(-18.0843084263497,41.1285214239226,124.130796993338)) ;
#69873=CARTESIAN_POINT('Ctrl Pts',(-18.349298634213,40.9485323435597,123.986997811558)) ;
#69874=CARTESIAN_POINT('Ctrl Pts',(-17.9790049811939,41.1385853055063,123.888252695276)) ;
#69875=CARTESIAN_POINT('Ctrl Pts',(-18.2650563069979,40.9585962251434,123.792961884212)) ;
#69876=CARTESIAN_POINT('Ctrl Pts',(-17.9185435301409,41.14846873148,123.63561553845)) ;
#69877=CARTESIAN_POINT('Ctrl Pts',(-18.2166879295781,40.9684796511172,123.590852855347)) ;
#69878=CARTESIAN_POINT('Ctrl Pts',(-17.9022681371798,41.1584693354011,123.37336067713)) ;
#69879=CARTESIAN_POINT('Ctrl Pts',(-18.2036681214858,40.9784802550382,123.381049048255)) ;
#69880=CARTESIAN_POINT('Ctrl Pts',(-17.931383888056,41.168389119739,123.114261971927)) ;
#69881=CARTESIAN_POINT('Ctrl Pts',(-18.2269611056014,40.9884000393761,123.17377075239)) ;
#69882=CARTESIAN_POINT('Ctrl Pts',(-18.0060263785442,41.1784364700958,122.861044240447)) ;
#69883=CARTESIAN_POINT('Ctrl Pts',(-18.2866756080612,40.998447389733,122.971196520026)) ;
#69884=CARTESIAN_POINT('Ctrl Pts',(-18.1212813811983,41.1883138123301,122.62841137183)) ;
#69885=CARTESIAN_POINT('Ctrl Pts',(-18.3788795564563,41.0083247319672,122.785091229606)) ;
#69886=CARTESIAN_POINT('Ctrl Pts',(-18.2781294851284,41.1983836934047,122.415344458296)) ;
#69887=CARTESIAN_POINT('Ctrl Pts',(-18.504358563971,41.0183946130419,122.614637662932)) ;
#69888=CARTESIAN_POINT('Ctrl Pts',(-18.4649093676713,41.2082133986064,122.236837854703)) ;
#69889=CARTESIAN_POINT('Ctrl Pts',(-18.6537818070225,41.0282243182436,122.471833474203)) ;
#69890=CARTESIAN_POINT('Ctrl Pts',(-18.684754038693,41.2182800597728,122.089775689271)) ;
#69891=CARTESIAN_POINT('Ctrl Pts',(-18.829657944727,41.03829097941,122.354183767872)) ;
#69892=CARTESIAN_POINT('Ctrl Pts',(-18.922687539533,41.2281702816401,121.985108837478)) ;
#69893=CARTESIAN_POINT('Ctrl Pts',(-19.0200040932344,41.0481812012773,122.270450887395)) ;
#69894=CARTESIAN_POINT('Ctrl Pts',(-19.1775992382533,41.2381624577503,121.922160157756)) ;
#69895=CARTESIAN_POINT('Ctrl Pts',(-19.223933319871,41.0581733773874,122.22009212209)) ;
#69896=CARTESIAN_POINT('Ctrl Pts',(-19.4388247420797,41.2481252878629,121.904728591906)) ;
#69897=CARTESIAN_POINT('Ctrl Pts',(-19.4329133725897,41.0681362075001,122.206147099364)) ;
#69898=CARTESIAN_POINT('Ctrl Pts',(-19.6976771545585,41.2580295002633,121.932097935364)) ;
#69899=CARTESIAN_POINT('Ctrl Pts',(-19.6399945510564,41.0780404199004,122.228042530922)) ;
#69900=CARTESIAN_POINT('Ctrl Pts',(-19.9516776747255,41.2680902143511,122.005343143406)) ;
#69901=CARTESIAN_POINT('Ctrl Pts',(-19.8431952134582,41.0881011339882,122.286638869231)) ;
#69902=CARTESIAN_POINT('Ctrl Pts',(-20.1841049252899,41.2779297173339,122.118737500505)) ;
#69903=CARTESIAN_POINT('Ctrl Pts',(-20.0291359487438,41.097940636971,122.377353840953)) ;
#69904=CARTESIAN_POINT('Ctrl Pts',(-20.3982213435744,41.2879958559003,122.273999666852)) ;
#69905=CARTESIAN_POINT('Ctrl Pts',(-20.2004293795964,41.1080067755374,122.501563713022)) ;
#69906=CARTESIAN_POINT('Ctrl Pts',(-20.5787589735412,41.2978783703863,122.460739928102)) ;
#69907=CARTESIAN_POINT('Ctrl Pts',(-20.3448588816564,41.1178892900235,122.650955244937)) ;
#69908=CARTESIAN_POINT('Ctrl Pts',(-20.7261276816334,41.3078706697419,122.678026456324)) ;
#69909=CARTESIAN_POINT('Ctrl Pts',(-20.4627538900193,41.127881589379,122.82478422743)) ;
#69910=CARTESIAN_POINT('Ctrl Pts',(-20.8332007283246,41.3178237366953,122.916705335846)) ;
#69911=CARTESIAN_POINT('Ctrl Pts',(-20.5484123254759,41.1378346563324,123.01572688204)) ;
#69912=CARTESIAN_POINT('Ctrl Pts',(-20.8976084793145,41.3278584449005,123.172399737523)) ;
#69913=CARTESIAN_POINT('Ctrl Pts',(-20.5999387072137,41.1478693645376,123.220282482398)) ;
#69914=CARTESIAN_POINT('Ctrl Pts',(-20.9165553817096,41.3377466658047,123.431576287923)) ;
#69915=CARTESIAN_POINT('Ctrl Pts',(-20.6150963672015,41.1577575854418,123.427622853528)) ;
#69916=CARTESIAN_POINT('Ctrl Pts',(-20.8903621464779,41.3477410888351,123.692895458737)) ;
#69917=CARTESIAN_POINT('Ctrl Pts',(-20.5941421044658,41.1677520084722,123.636678055488)) ;
#69918=CARTESIAN_POINT('Ctrl Pts',(-20.8194388311831,41.3576864282813,123.944442205965)) ;
#69919=CARTESIAN_POINT('Ctrl Pts',(-20.5374038559839,41.1776973479184,123.837915073439)) ;
#69920=CARTESIAN_POINT('Ctrl Pts',(-20.7063724848582,41.3676337728926,124.180145089931)) ;
#69921=CARTESIAN_POINT('Ctrl Pts',(-20.446951356585,41.1876446925297,124.026477147799)) ;
#69922=CARTESIAN_POINT('Ctrl Pts',(-20.5523289698857,41.3776816683036,124.394591659)) ;
#69923=CARTESIAN_POINT('Ctrl Pts',(-20.3237167077923,41.1976925879407,124.198034766973)) ;
#69924=CARTESIAN_POINT('Ctrl Pts',(-20.3673015896202,41.387529313783,124.575522794134)) ;
#69925=CARTESIAN_POINT('Ctrl Pts',(-20.1756958838239,41.2075402334201,124.342779178533)) ;
#69926=CARTESIAN_POINT('Ctrl Pts',(-20.1516704586702,41.397491027697,124.723938642442)) ;
#69927=CARTESIAN_POINT('Ctrl Pts',(-20.0031916223503,41.2175019473341,124.461512149995)) ;
#69928=CARTESIAN_POINT('Ctrl Pts',(-19.911780850099,41.4075196519879,124.833098044345)) ;
#69929=CARTESIAN_POINT('Ctrl Pts',(-19.8112800810594,41.227530571625,124.548840178017)) ;
#69930=CARTESIAN_POINT('Ctrl Pts',(-19.6596394073023,41.4174300126446,124.898243770015)) ;
#69931=CARTESIAN_POINT('Ctrl Pts',(-19.6095677408918,41.2374409322817,124.600957108251)) ;
#69932=CARTESIAN_POINT('Ctrl Pts',(-19.3994113076568,41.4273647112179,124.91935848404)) ;
#69933=CARTESIAN_POINT('Ctrl Pts',(-19.4013858458597,41.247375630855,124.617849546606)) ;
#69934=CARTESIAN_POINT('Ctrl Pts',(-19.1367143515178,41.4374065360721,124.894447395017)) ;
#69935=CARTESIAN_POINT('Ctrl Pts',(-19.1912280682996,41.2574174557092,124.597921306122)) ;
#69936=CARTESIAN_POINT('Ctrl Pts',(-18.8862194476765,41.4472911098165,124.825610729058)) ;
#69937=CARTESIAN_POINT('Ctrl Pts',(-18.9908327711166,41.2673020294536,124.542852873517)) ;
#69938=CARTESIAN_POINT('Ctrl Pts',(-18.6486170762246,41.4572929591797,124.713315149718)) ;
#69939=CARTESIAN_POINT('Ctrl Pts',(-18.8007506471708,41.2773038788168,124.45301716696)) ;
#69940=CARTESIAN_POINT('Ctrl Pts',(-18.4357242323319,41.4672122607537,124.562839022651)) ;
#69941=CARTESIAN_POINT('Ctrl Pts',(-18.6304363934291,41.2872231803909,124.332637291821)) ;
#69942=CARTESIAN_POINT('Ctrl Pts',(-18.2499195837942,41.477256369099,124.375398346987)) ;
#69943=CARTESIAN_POINT('Ctrl Pts',(-18.4817919703577,41.2972672887361,124.182685211504)) ;
#69944=CARTESIAN_POINT('Ctrl Pts',(-18.1017911287502,41.4871407925413,124.162007655832)) ;
#69945=CARTESIAN_POINT('Ctrl Pts',(-18.3632889812558,41.3071517121784,124.011973815533)) ;
#69946=CARTESIAN_POINT('Ctrl Pts',(-17.9909819762134,41.4971571544507,123.923238127084)) ;
#69947=CARTESIAN_POINT('Ctrl Pts',(-18.27464077142,41.3171680740879,123.820958606205)) ;
#69948=CARTESIAN_POINT('Ctrl Pts',(-17.9238542028585,41.5071938099561,123.66818572458)) ;
#69949=CARTESIAN_POINT('Ctrl Pts',(-18.2209377383296,41.3272047295932,123.616916796119)) ;
#69950=CARTESIAN_POINT('Ctrl Pts',(-17.9017753134138,41.5170239401454,123.410773438911)) ;
#69951=CARTESIAN_POINT('Ctrl Pts',(-18.2032737428897,41.3370348597826,123.410988188349)) ;
#69952=CARTESIAN_POINT('Ctrl Pts',(-17.9252038428856,41.5270999932353,123.147075094843)) ;
#69953=CARTESIAN_POINT('Ctrl Pts',(-18.2220155951886,41.3471109128724,123.2000290831)) ;
#69954=CARTESIAN_POINT('Ctrl Pts',(-17.9924242809587,41.5369522224211,122.896990000681)) ;
#69955=CARTESIAN_POINT('Ctrl Pts',(-18.2757906890744,41.3569631420582,122.999961690913)) ;
#69956=CARTESIAN_POINT('Ctrl Pts',(-18.1042623444851,41.5470254302204,122.657109249406)) ;
#69957=CARTESIAN_POINT('Ctrl Pts',(-18.3652602896576,41.3670363498575,122.808056339764)) ;
#69958=CARTESIAN_POINT('Ctrl Pts',(-18.2526543868681,41.5568669415718,122.445270485562)) ;
#69959=CARTESIAN_POINT('Ctrl Pts',(-18.4839724495599,41.3768778612089,122.638585568541)) ;
#69960=CARTESIAN_POINT('Ctrl Pts',(-18.4370777102109,41.5668278796093,122.259519138152)) ;
#69961=CARTESIAN_POINT('Ctrl Pts',(-18.6315099644499,41.3868387992465,122.489983811783)) ;
#69962=CARTESIAN_POINT('Ctrl Pts',(-18.6529080737898,41.5768657415343,122.107878162832)) ;
#69963=CARTESIAN_POINT('Ctrl Pts',(-18.804173668292,41.3968766611714,122.368670011063)) ;
#69964=CARTESIAN_POINT('Ctrl Pts',(-18.8877262423687,41.5867399275314,121.997383365689)) ;
#69965=CARTESIAN_POINT('Ctrl Pts',(-18.9920269264179,41.4067508471685,122.280273361693)) ;
#69966=CARTESIAN_POINT('Ctrl Pts',(-19.1430711045837,41.5968100871093,121.928030886543)) ;
#69967=CARTESIAN_POINT('Ctrl Pts',(-19.1963027525332,41.4168210067464,122.22479007538)) ;
#69968=CARTESIAN_POINT('Ctrl Pts',(-19.4003882644743,41.6066418345351,121.904466477439)) ;
#69969=CARTESIAN_POINT('Ctrl Pts',(-19.4021553376179,41.4266527541722,122.205937341054)) ;
#69970=CARTESIAN_POINT('Ctrl Pts',(-19.6632563157754,41.6166779146064,121.925697979521)) ;
#69971=CARTESIAN_POINT('Ctrl Pts',(-19.6124499841248,41.4366888342435,122.222921102434)) ;
#69972=CARTESIAN_POINT('Ctrl Pts',(-19.9178188413347,41.6266949614589,121.992773118902)) ;
#69973=CARTESIAN_POINT('Ctrl Pts',(-19.8161003293912,41.446705881096,122.276579942071)) ;
#69974=CARTESIAN_POINT('Ctrl Pts',(-20.1538480381938,41.6365772196255,122.10109797781)) ;
#69975=CARTESIAN_POINT('Ctrl Pts',(-20.0049236160898,41.4565881392626,122.363238243392)) ;
#69976=CARTESIAN_POINT('Ctrl Pts',(-20.3699075386073,41.6465649024218,122.250068895617)) ;
#69977=CARTESIAN_POINT('Ctrl Pts',(-20.1777719215884,41.466575822059,122.482413671685)) ;
#69978=CARTESIAN_POINT('Ctrl Pts',(-20.556247785553,41.6565115591386,122.433432011487)) ;
#69979=CARTESIAN_POINT('Ctrl Pts',(-20.3268449195173,41.4765224787757,122.629102830338)) ;
#69980=CARTESIAN_POINT('Ctrl Pts',(-20.7093408277522,41.6665686172188,122.648828544842)) ;
#69981=CARTESIAN_POINT('Ctrl Pts',(-20.4493206451329,41.4865795368559,122.801419352681)) ;
#69982=CARTESIAN_POINT('Ctrl Pts',(-20.8203574276063,41.6763867967682,122.881750559428)) ;
#69983=CARTESIAN_POINT('Ctrl Pts',(-20.5381348730655,41.4963977164053,122.987755393131)) ;
#69984=CARTESIAN_POINT('Ctrl Pts',(-20.8914554133569,41.6864227312072,123.135713115928)) ;
#69985=CARTESIAN_POINT('Ctrl Pts',(-20.5950148896598,41.5064336508443,123.190925073507)) ;
#69986=CARTESIAN_POINT('Ctrl Pts',(-20.9165972820437,41.6964473856362,123.397957733958)) ;
#69987=CARTESIAN_POINT('Ctrl Pts',(-20.6151299031663,41.5164583052733,123.400720641268)) ;
#69988=CARTESIAN_POINT('Ctrl Pts',(-20.8967522553727,41.7062994052157,123.656101312759)) ;
#69989=CARTESIAN_POINT('Ctrl Pts',(-20.5992555699789,41.5263103248528,123.607234825418)) ;
#69990=CARTESIAN_POINT('Ctrl Pts',(-20.8318758704315,41.7162903189306,123.910477841226)) ;
#69991=CARTESIAN_POINT('Ctrl Pts',(-20.5473561475517,41.5363012385678,123.810736336764)) ;
#69992=CARTESIAN_POINT('Ctrl Pts',(-20.7247343585358,41.7262083077702,124.148106422392)) ;
#69993=CARTESIAN_POINT('Ctrl Pts',(-20.4616447029852,41.5462192274073,124.000839496386)) ;
#69994=CARTESIAN_POINT('Ctrl Pts',(-20.5764123274112,41.736236418501,124.365906529172)) ;
#69995=CARTESIAN_POINT('Ctrl Pts',(-20.3429885028579,41.5562473381381,124.175080585433)) ;
#69996=CARTESIAN_POINT('Ctrl Pts',(-20.395206571467,41.7461216164094,124.552049981452)) ;
#69997=CARTESIAN_POINT('Ctrl Pts',(-20.1980255691353,41.5661325360465,124.323996153329)) ;
#69998=CARTESIAN_POINT('Ctrl Pts',(-20.1825881915492,41.7561108916774,124.706022484706)) ;
#69999=CARTESIAN_POINT('Ctrl Pts',(-20.0279320600952,41.5761218113145,124.447175591284)) ;
#70000=CARTESIAN_POINT('Ctrl Pts',(-19.944994054816,41.7661523498469,124.820818389465)) ;
#70001=CARTESIAN_POINT('Ctrl Pts',(-19.837857454139,41.586163269484,124.539013942928)) ;
#70002=CARTESIAN_POINT('Ctrl Pts',(-19.6965012965203,41.7759838136352,124.891575936423)) ;
#70003=CARTESIAN_POINT('Ctrl Pts',(-19.6390644965111,41.5959947332723,124.595621546985)) ;
#70004=CARTESIAN_POINT('Ctrl Pts',(-19.4350641759092,41.7859887459391,124.919157369809)) ;
#70005=CARTESIAN_POINT('Ctrl Pts',(-19.4299150640357,41.6059996655762,124.61768861319)) ;
#70006=CARTESIAN_POINT('Ctrl Pts',(-19.1732294916453,41.7959751098338,124.900811143185)) ;
#70007=CARTESIAN_POINT('Ctrl Pts',(-19.2204473105258,41.615986029471,124.603013545684)) ;
#70008=CARTESIAN_POINT('Ctrl Pts',(-18.9175714408772,41.8060047387197,124.836821562451)) ;
#70009=CARTESIAN_POINT('Ctrl Pts',(-19.0159203902611,41.6260156583568,124.551823702806)) ;
#70010=CARTESIAN_POINT('Ctrl Pts',(-18.6804315219461,41.8158799608281,124.731353527358)) ;
#70011=CARTESIAN_POINT('Ctrl Pts',(-18.8262081643028,41.6358908804652,124.467451255553)) ;
#70012=CARTESIAN_POINT('Ctrl Pts',(-18.4623421036418,41.8258811732252,124.584757637499)) ;
#70013=CARTESIAN_POINT('Ctrl Pts',(-18.6517356019732,41.6458920928623,124.350176231393)) ;
#70014=CARTESIAN_POINT('Ctrl Pts',(-18.2745387790295,41.8357897524607,124.404326737909)) ;
#70015=CARTESIAN_POINT('Ctrl Pts',(-18.5014918287593,41.6558006720979,124.205833218676)) ;
#70016=CARTESIAN_POINT('Ctrl Pts',(-18.1187665880947,41.8458446050167,124.190948411598)) ;
#70017=CARTESIAN_POINT('Ctrl Pts',(-18.3768724125768,41.6658555246539,124.035131662587)) ;
#70018=CARTESIAN_POINT('Ctrl Pts',(-18.0043751834666,41.8557031872915,123.958446111396)) ;
#70019=CARTESIAN_POINT('Ctrl Pts',(-18.2853576981926,41.6757141069286,123.849131183936)) ;
#70020=CARTESIAN_POINT('Ctrl Pts',(-17.93042449407,41.8657713167342,123.70445148532)) ;
#70021=CARTESIAN_POINT('Ctrl Pts',(-18.2261951440607,41.6857822363713,123.645935938738)) ;
#70022=CARTESIAN_POINT('Ctrl Pts',(-17.9023200741687,41.8756267884233,123.446967189866)) ;
#70023=CARTESIAN_POINT('Ctrl Pts',(-18.2037096291495,41.6956377080604,123.439949220456)) ;
#70024=CARTESIAN_POINT('Ctrl Pts',(-17.9188032302922,41.8856216368096,123.184839420313)) ;
#70025=CARTESIAN_POINT('Ctrl Pts',(-18.2168940227441,41.7056325564467,123.23024695042)) ;
#70026=CARTESIAN_POINT('Ctrl Pts',(-17.9813304619599,41.895652933594,122.928744998837)) ;
#70027=CARTESIAN_POINT('Ctrl Pts',(-18.2669137962854,41.7156638532311,123.025370923546)) ;
#70028=CARTESIAN_POINT('Ctrl Pts',(-18.0852555186611,41.9055194698041,122.691192079478)) ;
#70029=CARTESIAN_POINT('Ctrl Pts',(-18.3500517412046,41.7255303894412,122.835328118647)) ;
#70030=CARTESIAN_POINT('Ctrl Pts',(-18.2302333322929,41.9155068927649,122.472444933182)) ;
#70031=CARTESIAN_POINT('Ctrl Pts',(-18.4660321429773,41.7355178124021,122.66032929391)) ;
#70032=CARTESIAN_POINT('Ctrl Pts',(-18.4101690101242,41.9254518317847,122.282861709824)) ;
#70033=CARTESIAN_POINT('Ctrl Pts',(-18.6099789904463,41.7454627514218,122.508661363733)) ;
#70034=CARTESIAN_POINT('Ctrl Pts',(-18.6224325374237,41.9354967176447,122.125972345834)) ;
#70035=CARTESIAN_POINT('Ctrl Pts',(-18.7797885429512,41.7555076372818,122.38314813357)) ;
#70036=CARTESIAN_POINT('Ctrl Pts',(-18.8545248231622,41.9453652527309,122.010250360349)) ;
#70037=CARTESIAN_POINT('Ctrl Pts',(-18.9654611095548,41.7653761723681,122.290568757108)) ;
#70038=CARTESIAN_POINT('Ctrl Pts',(-19.1054113849967,41.9553311207376,121.935164518734)) ;
#70039=CARTESIAN_POINT('Ctrl Pts',(-19.1661696157605,41.7753420403747,122.230497995113)) ;
#70040=CARTESIAN_POINT('Ctrl Pts',(-19.3670697024523,41.9653537681901,121.904899528248)) ;
#70041=CARTESIAN_POINT('Ctrl Pts',(-19.3754959860251,41.7853646878272,122.206283828786)) ;
#70042=CARTESIAN_POINT('Ctrl Pts',(-19.6273839317657,41.9752774071977,121.920298317369)) ;
#70043=CARTESIAN_POINT('Ctrl Pts',(-19.583747310097,41.7952883268348,122.218600653541)) ;
#70044=CARTESIAN_POINT('Ctrl Pts',(-19.8817304496807,41.9852201322034,121.980174899417)) ;
#70045=CARTESIAN_POINT('Ctrl Pts',(-19.7872249056599,41.8052310518406,122.266499716191)) ;
#70046=CARTESIAN_POINT('Ctrl Pts',(-20.1241484576752,41.9952657382553,122.084651122132)) ;
#70047=CARTESIAN_POINT('Ctrl Pts',(-19.9811601739826,41.8152766578924,122.350078652144)) ;
#70048=CARTESIAN_POINT('Ctrl Pts',(-20.3408862916986,42.0051271607764,122.22675611249)) ;
#70049=CARTESIAN_POINT('Ctrl Pts',(-20.1545514860313,41.8251380804135,122.463760663456)) ;
#70050=CARTESIAN_POINT('Ctrl Pts',(-20.5324507967766,42.0151207292256,122.406346888385)) ;
#70051=CARTESIAN_POINT('Ctrl Pts',(-20.3078045818973,41.8351316488627,122.607431606924)) ;
#70052=CARTESIAN_POINT('Ctrl Pts',(-20.6890036597013,42.0250461999809,122.615019061482)) ;
#70053=CARTESIAN_POINT('Ctrl Pts',(-20.4330486091548,41.845057119618,122.774367895725)) ;
#70054=CARTESIAN_POINT('Ctrl Pts',(-20.808139363818,42.0350738739368,122.850031069966)) ;
#70055=CARTESIAN_POINT('Ctrl Pts',(-20.528359143158,41.8550847935739,122.962376508046)) ;
#70056=CARTESIAN_POINT('Ctrl Pts',(-20.8838479741626,42.0449610519785,123.098617303755)) ;
#70057=CARTESIAN_POINT('Ctrl Pts',(-20.5889282071218,41.8649719716156,123.161244495286)) ;
#70058=CARTESIAN_POINT('Ctrl Pts',(-20.9158670631571,42.0549894313466,123.360164459768)) ;
#70059=CARTESIAN_POINT('Ctrl Pts',(-20.6145455234739,41.8750003509838,123.370482841574)) ;
#70060=CARTESIAN_POINT('Ctrl Pts',(-20.9023097751863,42.0648836740681,123.619854631483)) ;
#70061=CARTESIAN_POINT('Ctrl Pts',(-20.6037026459315,41.8848945937052,123.578231501373)) ;
#70062=CARTESIAN_POINT('Ctrl Pts',(-20.8237470249053,42.078236590719,123.961816174747)) ;
#70063=CARTESIAN_POINT('Ctrl Pts',(-20.540851905552,41.8982475103561,123.851818955548)) ;
#70064=CARTESIAN_POINT('Ctrl Pts',(-20.6595997814835,42.0914391084657,124.272009590654)) ;
#70065=CARTESIAN_POINT('Ctrl Pts',(-20.4095171791971,41.9114500281029,124.099990022592)) ;
#70066=CARTESIAN_POINT('Ctrl Pts',(-20.4209837962718,42.1047950137467,124.529355053645)) ;
#70067=CARTESIAN_POINT('Ctrl Pts',(-20.2186534466242,41.9248059333838,124.305833005313)) ;
#70068=CARTESIAN_POINT('Ctrl Pts',(-20.2138409514704,42.1146916623845,124.686668820964)) ;
#70069=CARTESIAN_POINT('Ctrl Pts',(-20.0529350989336,41.9347025820217,124.431692934571)) ;
#70070=CARTESIAN_POINT('Ctrl Pts',(-19.9790784982733,42.124739800437,124.807498749042)) ;
#70071=CARTESIAN_POINT('Ctrl Pts',(-19.8651277057987,41.9447507200741,124.528356915192)) ;
#70072=CARTESIAN_POINT('Ctrl Pts',(-19.7308134332186,42.1346307606148,124.884508092935)) ;
#70073=CARTESIAN_POINT('Ctrl Pts',(-19.6665158148451,41.9546416802519,124.589967046328)) ;
#70074=CARTESIAN_POINT('Ctrl Pts',(-19.4703782998092,42.1446235964915,124.918232356421)) ;
#70075=CARTESIAN_POINT('Ctrl Pts',(-19.4581682824578,41.9646345161287,124.616948547809)) ;
#70076=CARTESIAN_POINT('Ctrl Pts',(-19.2068788945409,42.1546626914931,124.905562765929)) ;
#70077=CARTESIAN_POINT('Ctrl Pts',(-19.2473681313206,41.9746736111302,124.606814984764)) ;
#70078=CARTESIAN_POINT('Ctrl Pts',(-18.9545800921988,42.1645000473443,124.849083179674)) ;
#70079=CARTESIAN_POINT('Ctrl Pts',(-19.0455306742898,41.9845109669814,124.56163402756)) ;
#70080=CARTESIAN_POINT('Ctrl Pts',(-18.629663451881,42.177892995275,124.713940021359)) ;
#70081=CARTESIAN_POINT('Ctrl Pts',(-18.7855850543186,41.9979039149121,124.453519158685)) ;
#70082=CARTESIAN_POINT('Ctrl Pts',(-18.3520925365356,42.1910596717019,124.500678451702)) ;
#70083=CARTESIAN_POINT('Ctrl Pts',(-18.5635083043611,42.0110705913391,124.282885722299)) ;
#70084=CARTESIAN_POINT('Ctrl Pts',(-18.1378563760038,42.2044444531087,124.221781306289)) ;
#70085=CARTESIAN_POINT('Ctrl Pts',(-18.3921499280378,42.0244553727458,124.059804293663)) ;
#70086=CARTESIAN_POINT('Ctrl Pts',(-18.0179616237773,42.2143062357526,123.991978653527)) ;
#70087=CARTESIAN_POINT('Ctrl Pts',(-18.2962255485433,42.0343171553897,123.875955881791)) ;
#70088=CARTESIAN_POINT('Ctrl Pts',(-17.9383202716689,42.2243053837056,123.741625973935)) ;
#70089=CARTESIAN_POINT('Ctrl Pts',(-18.2325120682241,42.0443163033428,123.675676550641)) ;
#70090=CARTESIAN_POINT('Ctrl Pts',(-17.9034419632737,42.2342081763227,123.483683307464)) ;
#70091=CARTESIAN_POINT('Ctrl Pts',(-18.2046075051605,42.0542190959598,123.469320792753)) ;
#70092=CARTESIAN_POINT('Ctrl Pts',(-17.9141036164672,42.2442577562136,123.21987047093)) ;
#70093=CARTESIAN_POINT('Ctrl Pts',(-18.2131325074826,42.0642686758508,123.258274986974)) ;
#70094=CARTESIAN_POINT('Ctrl Pts',(-17.9873542558445,42.2574448300231,122.881031053165)) ;
#70095=CARTESIAN_POINT('Ctrl Pts',(-18.2717422460334,42.0774557496602,122.987181397706)) ;
#70096=CARTESIAN_POINT('Ctrl Pts',(-18.1910268972478,42.2741976199943,122.48527825742)) ;
#70097=CARTESIAN_POINT('Ctrl Pts',(-18.4346521928802,42.0942085396314,122.670610268033)) ;
#70098=CARTESIAN_POINT('Ctrl Pts',(-18.5127023287359,42.290686272089,122.187393477367)) ;
#70099=CARTESIAN_POINT('Ctrl Pts',(-18.6920409981402,42.1106971917261,122.432258549758)) ;
#70100=CARTESIAN_POINT('Ctrl Pts',(-18.8227825349679,42.3040430982724,122.023091316242)) ;
#70101=CARTESIAN_POINT('Ctrl Pts',(-18.9400618893494,42.1240540179095,122.300845856215)) ;
#70102=CARTESIAN_POINT('Ctrl Pts',(-19.0702507619016,42.3139394831503,121.942948929694)) ;
#70103=CARTESIAN_POINT('Ctrl Pts',(-19.1380453748036,42.1339504027875,122.236723914257)) ;
#70104=CARTESIAN_POINT('Ctrl Pts',(-19.3305991665012,42.3239459976708,121.906474651851)) ;
#70105=CARTESIAN_POINT('Ctrl Pts',(-19.3463190360728,42.1439569173079,122.2075435789)) ;
#70106=CARTESIAN_POINT('Ctrl Pts',(-19.6771578660426,42.3371361211872,121.917859655171)) ;
#70107=CARTESIAN_POINT('Ctrl Pts',(-19.623580039702,42.1571470408243,122.216652401464)) ;
#70108=CARTESIAN_POINT('Ctrl Pts',(-20.1032957575407,42.3539026823368,122.047670197675)) ;
#70109=CARTESIAN_POINT('Ctrl Pts',(-19.9644762057803,42.1739136019739,122.320493865006)) ;
#70110=CARTESIAN_POINT('Ctrl Pts',(-20.5238873611168,42.3736871710448,122.363526341007)) ;
#70111=CARTESIAN_POINT('Ctrl Pts',(-20.3009572541404,42.1936980906819,122.573177890101)) ;
#70112=CARTESIAN_POINT('Ctrl Pts',(-20.8150059840566,42.3936326186413,122.806396279347)) ;
#70113=CARTESIAN_POINT('Ctrl Pts',(-20.5338537200683,42.2136435382784,122.927472140951)) ;
#70114=CARTESIAN_POINT('Ctrl Pts',(-20.9368565339894,42.4135442807972,123.32140844695)) ;
#70115=CARTESIAN_POINT('Ctrl Pts',(-20.6313376522247,42.2335552004343,123.33948182386)) ;
#70116=CARTESIAN_POINT('Ctrl Pts',(-20.8768601174002,42.4334364728161,123.846776921239)) ;
#70117=CARTESIAN_POINT('Ctrl Pts',(-20.583342978862,42.2534473924532,123.759777675271)) ;
#70118=CARTESIAN_POINT('Ctrl Pts',(-20.6387749464663,42.4534776033707,124.323184054214)) ;
#70119=CARTESIAN_POINT('Ctrl Pts',(-20.3928775130821,42.2734885230078,124.140904294275)) ;
#70120=CARTESIAN_POINT('Ctrl Pts',(-20.2567515623942,42.4732959379863,124.686015098705)) ;
#70121=CARTESIAN_POINT('Ctrl Pts',(-20.087259484934,42.2933068576234,124.431172000379)) ;
#70122=CARTESIAN_POINT('Ctrl Pts',(-19.7707111217134,42.4932685032059,124.899002007876)) ;
#70123=CARTESIAN_POINT('Ctrl Pts',(-19.6984277079127,42.313279422843,124.601563631414)) ;
#70124=CARTESIAN_POINT('Ctrl Pts',(-19.2430064355605,42.5131577193775,124.933361056965)) ;
#70125=CARTESIAN_POINT('Ctrl Pts',(-19.2762631018856,42.3331686390146,124.629052843148)) ;
#70126=CARTESIAN_POINT('Ctrl Pts',(-18.7322443545962,42.5331812937002,124.784326245752)) ;
#70127=CARTESIAN_POINT('Ctrl Pts',(-18.8676531273989,42.3531922133373,124.509826918718)) ;
#70128=CARTESIAN_POINT('Ctrl Pts',(-18.3074466869106,42.5529784567885,124.473672881631)) ;
#70129=CARTESIAN_POINT('Ctrl Pts',(-18.5278123342791,42.3729893764256,124.261304267751)) ;
#70130=CARTESIAN_POINT('Ctrl Pts',(-18.0107152101051,42.5729439506122,124.03387590139)) ;
#70131=CARTESIAN_POINT('Ctrl Pts',(-18.2904261458476,42.3929548702494,123.909466818997)) ;
#70132=CARTESIAN_POINT('Ctrl Pts',(-17.8825244705871,42.5928976583536,123.51911914368)) ;
#70133=CARTESIAN_POINT('Ctrl Pts',(-18.1878724815504,42.4129085779908,123.497661231514)) ;
#70134=CARTESIAN_POINT('Ctrl Pts',(-17.9375074674537,42.6128050350802,122.992998485349)) ;
#70135=CARTESIAN_POINT('Ctrl Pts',(-18.2318581752466,42.4328159547174,123.076763483073)) ;
#70136=CARTESIAN_POINT('Ctrl Pts',(-18.1669062692067,42.6326572466288,122.517738273591)) ;
#70137=CARTESIAN_POINT('Ctrl Pts',(-18.4153780968803,42.4526681662659,122.696553635092)) ;
#70138=CARTESIAN_POINT('Ctrl Pts',(-18.5491943143349,42.6527296335745,122.145651577482)) ;
#70139=CARTESIAN_POINT('Ctrl Pts',(-18.721207849793,42.4727405532116,122.398884952664)) ;
#70140=CARTESIAN_POINT('Ctrl Pts',(-19.0301333322148,42.6725675032148,121.929544757103)) ;
#70141=CARTESIAN_POINT('Ctrl Pts',(-19.1059609684924,42.4925784228519,122.225998529547)) ;
#70142=CARTESIAN_POINT('Ctrl Pts',(-19.5561067931665,42.6924181577679,121.88822002276)) ;
#70143=CARTESIAN_POINT('Ctrl Pts',(-19.5267415619836,42.5124290774051,122.19293977911)) ;
#70144=CARTESIAN_POINT('Ctrl Pts',(-20.0695211678143,42.7124700921084,122.031029897398)) ;
#70145=CARTESIAN_POINT('Ctrl Pts',(-19.9374722246251,42.5324810117455,122.307188485913)) ;
#70146=CARTESIAN_POINT('Ctrl Pts',(-20.4987389792293,42.7323032796744,122.33724488066)) ;
#70147=CARTESIAN_POINT('Ctrl Pts',(-20.2808472827428,42.5523141993116,122.552162457419)) ;
#70148=CARTESIAN_POINT('Ctrl Pts',(-20.7998323714999,42.7522324919051,122.772792578482)) ;
#70149=CARTESIAN_POINT('Ctrl Pts',(-20.5217209763658,42.5722434115422,122.900602245168)) ;
#70150=CARTESIAN_POINT('Ctrl Pts',(-20.9346324231233,42.7721174571195,123.284031475315)) ;
#70151=CARTESIAN_POINT('Ctrl Pts',(-20.6295592175581,42.5921283767566,123.309594871732)) ;
#70152=CARTESIAN_POINT('Ctrl Pts',(-20.8856369561692,42.7921911982641,123.815196128951)) ;
#70153=CARTESIAN_POINT('Ctrl Pts',(-20.5903609317186,42.6122021179012,123.734525730611)) ;
#70154=CARTESIAN_POINT('Ctrl Pts',(-20.6614795251124,42.8119843800445,124.291210805294)) ;
#70155=CARTESIAN_POINT('Ctrl Pts',(-20.4110322484531,42.6319952996816,124.115338243655)) ;
#70156=CARTESIAN_POINT('Ctrl Pts',(-20.2863715695943,42.8319470880472,124.666388958395)) ;
#70157=CARTESIAN_POINT('Ctrl Pts',(-20.1109437039454,42.6519580076843,124.415478939255)) ;
#70158=CARTESIAN_POINT('Ctrl Pts',(-19.8046741907438,42.8519300397896,124.890126754003)) ;
#70159=CARTESIAN_POINT('Ctrl Pts',(-19.7255846106919,42.6719409594268,124.594466924686)) ;
#70160=CARTESIAN_POINT('Ctrl Pts',(-19.2801592562473,42.8717406595618,124.936699673532)) ;
#70161=CARTESIAN_POINT('Ctrl Pts',(-19.3059710215937,42.6917515791989,124.631722408354)) ;
#70162=CARTESIAN_POINT('Ctrl Pts',(-18.7667862152892,42.8917243755947,124.800954951219)) ;
#70163=CARTESIAN_POINT('Ctrl Pts',(-18.8952733417193,42.7117352952318,124.523123451149)) ;
#70164=CARTESIAN_POINT('Ctrl Pts',(-18.3326279856665,42.911605839492,124.499507379797)) ;
#70165=CARTESIAN_POINT('Ctrl Pts',(-18.5479481189047,42.7316167591292,124.281962249473)) ;
#70166=CARTESIAN_POINT('Ctrl Pts',(-18.0260984755986,42.9315611693364,124.066807185146)) ;
#70167=CARTESIAN_POINT('Ctrl Pts',(-18.3027271574083,42.7515720889735,123.935799951114)) ;
#70168=CARTESIAN_POINT('Ctrl Pts',(-17.8857662260403,42.9514366301419,123.557444062347)) ;
#70169=CARTESIAN_POINT('Ctrl Pts',(-18.1904651245614,42.771447549779,123.528307551792)) ;
#70170=CARTESIAN_POINT('Ctrl Pts',(-17.9275815086194,42.9714209501934,123.027999899649)) ;
#70171=CARTESIAN_POINT('Ctrl Pts',(-18.2239197641623,42.7914318698305,123.104753757388)) ;
#70172=CARTESIAN_POINT('Ctrl Pts',(-18.1472767537667,42.991348982983,122.545930346273)) ;
#70173=CARTESIAN_POINT('Ctrl Pts',(-18.3996848299053,42.8113599026202,122.719094732473)) ;
#70174=CARTESIAN_POINT('Ctrl Pts',(-18.4563016259536,43.0079577449228,122.230836526374)) ;
#70175=CARTESIAN_POINT('Ctrl Pts',(-18.6468908763838,42.82796866456,122.467036542162)) ;
#70176=CARTESIAN_POINT('Ctrl Pts',(-18.7544287787532,43.0211453836129,122.054087877132)) ;
#70177=CARTESIAN_POINT('Ctrl Pts',(-18.8854094489693,42.84115630325,122.325626725663)) ;
#70178=CARTESIAN_POINT('Ctrl Pts',(-18.9997521034799,43.031131817973,121.960916807132)) ;
#70179=CARTESIAN_POINT('Ctrl Pts',(-19.0816631635093,42.8511427376102,122.251094035391)) ;
#70180=CARTESIAN_POINT('Ctrl Pts',(-19.2581944108813,43.0411411919324,121.911902702877)) ;
#70181=CARTESIAN_POINT('Ctrl Pts',(-19.2884287994832,42.8611521115695,122.211885725831)) ;
#70182=CARTESIAN_POINT('Ctrl Pts',(-19.6074202778413,43.0544312254977,121.907165841963)) ;
#70183=CARTESIAN_POINT('Ctrl Pts',(-19.5677560175321,42.8744421451348,122.208091120847)) ;
#70184=CARTESIAN_POINT('Ctrl Pts',(-20.0350687767284,43.0710252131601,122.015093622791)) ;
#70185=CARTESIAN_POINT('Ctrl Pts',(-19.9099409302065,42.8910361327973,122.294450399826)) ;
#70186=CARTESIAN_POINT('Ctrl Pts',(-20.4010277793674,43.0876574684357,122.26302842487)) ;
#70187=CARTESIAN_POINT('Ctrl Pts',(-20.2026637544341,42.9076683880728,122.492780756029)) ;
#70188=CARTESIAN_POINT('Ctrl Pts',(-20.6289019817072,43.1008998521035,122.526052209373)) ;
#70189=CARTESIAN_POINT('Ctrl Pts',(-20.3849854274242,42.9209107717406,122.70321807601)) ;
#70190=CARTESIAN_POINT('Ctrl Pts',(-20.7634137015571,43.1108140603309,122.749188831555)) ;
#70191=CARTESIAN_POINT('Ctrl Pts',(-20.49258810908,42.9308249799681,122.881725181544)) ;
#70192=CARTESIAN_POINT('Ctrl Pts',(-20.8581936477321,43.1208706996026,122.995865179697)) ;
#70193=CARTESIAN_POINT('Ctrl Pts',(-20.5684111153363,42.9408816192397,123.079068425544)) ;
#70194=CARTESIAN_POINT('Ctrl Pts',(-20.9079570487934,43.1307165060227,123.249794573028)) ;
#70195=CARTESIAN_POINT('Ctrl Pts',(-20.6082199684139,42.9507274256599,123.282209957339)) ;
#70196=CARTESIAN_POINT('Ctrl Pts',(-20.9134264774939,43.1407615056559,123.513697714177)) ;
#70197=CARTESIAN_POINT('Ctrl Pts',(-20.6125910612325,42.960772425293,123.493341293603)) ;
#70198=CARTESIAN_POINT('Ctrl Pts',(-20.8594473356749,43.1540425280286,123.858497845333)) ;
#70199=CARTESIAN_POINT('Ctrl Pts',(-20.569416250521,42.9740534476658,123.769136972112)) ;
#70200=CARTESIAN_POINT('Ctrl Pts',(-20.718508196259,43.1672399745533,124.17971260659)) ;
#70201=CARTESIAN_POINT('Ctrl Pts',(-20.4566616453272,42.9872508941904,124.026134275498)) ;
#70202=CARTESIAN_POINT('Ctrl Pts',(-20.4978485962577,43.1806542723603,124.454637161235)) ;
#70203=CARTESIAN_POINT('Ctrl Pts',(-20.2801208442663,43.0006651919974,124.246084216616)) ;
#70204=CARTESIAN_POINT('Ctrl Pts',(-20.3035425807458,43.190493337763,124.625241624044)) ;
#70205=CARTESIAN_POINT('Ctrl Pts',(-20.124676701218,43.0105042574002,124.382563655871)) ;
#70206=CARTESIAN_POINT('Ctrl Pts',(-20.0797235876443,43.2004765440407,124.762051652017)) ;
#70207=CARTESIAN_POINT('Ctrl Pts',(-19.9456197990869,43.0204874636778,124.492010372349)) ;
#70208=CARTESIAN_POINT('Ctrl Pts',(-19.8362597616934,43.2104277789535,124.8575472145)) ;
#70209=CARTESIAN_POINT('Ctrl Pts',(-19.7508481203091,43.0304386985906,124.568404524437)) ;
#70210=CARTESIAN_POINT('Ctrl Pts',(-19.5786965198764,43.2204287786551,124.909888505183)) ;
#70211=CARTESIAN_POINT('Ctrl Pts',(-19.544797096,43.0404396982923,124.610275379233)) ;
#70212=CARTESIAN_POINT('Ctrl Pts',(-19.3151648430061,43.2304601244425,124.916319914135)) ;
#70213=CARTESIAN_POINT('Ctrl Pts',(-19.3339717561267,43.0504710440796,124.615418233467)) ;
#70214=CARTESIAN_POINT('Ctrl Pts',(-19.0590709276985,43.2403138891475,124.877945266862)) ;
#70215=CARTESIAN_POINT('Ctrl Pts',(-19.1290970496758,43.0603248087846,124.584716300181)) ;
#70216=CARTESIAN_POINT('Ctrl Pts',(-18.8104522663154,43.2502845428158,124.79531472401)) ;
#70217=CARTESIAN_POINT('Ctrl Pts',(-18.9302029191281,43.0702954624529,124.518609759504)) ;
#70218=CARTESIAN_POINT('Ctrl Pts',(-18.5792880259183,43.260281786473,124.670397983482)) ;
#70219=CARTESIAN_POINT('Ctrl Pts',(-18.7452726496911,43.0802927061101,124.418674422827)) ;
#70220=CARTESIAN_POINT('Ctrl Pts',(-18.3728375783555,43.2703152424172,124.506422572522)) ;
#70221=CARTESIAN_POINT('Ctrl Pts',(-18.5801137193159,43.0903261620543,124.287492345244)) ;
#70222=CARTESIAN_POINT('Ctrl Pts',(-18.2007504134058,43.2801707467176,124.31283503278)) ;
#70223=CARTESIAN_POINT('Ctrl Pts',(-18.4424457883443,43.1001816663547,124.132620965001)) ;
#70224=CARTESIAN_POINT('Ctrl Pts',(-18.0626456729148,43.2901701830037,124.089333194053)) ;
#70225=CARTESIAN_POINT('Ctrl Pts',(-18.3319639343597,43.1101811026408,123.953818381161)) ;
#70226=CARTESIAN_POINT('Ctrl Pts',(-17.9661552350075,43.3000646425196,123.847830753989)) ;
#70227=CARTESIAN_POINT('Ctrl Pts',(-18.2547737161696,43.1200755621567,123.760615804186)) ;
#70228=CARTESIAN_POINT('Ctrl Pts',(-17.9122545173091,43.3101277619712,123.588980661551)) ;
#70229=CARTESIAN_POINT('Ctrl Pts',(-18.2116553113845,43.1301386816084,123.55353524895)) ;
#70230=CARTESIAN_POINT('Ctrl Pts',(-17.9040100749574,43.3199673963832,123.330493713353)) ;
#70231=CARTESIAN_POINT('Ctrl Pts',(-18.2050619671359,43.1399783160204,123.346745951152)) ;
#70232=CARTESIAN_POINT('Ctrl Pts',(-17.9412644855324,43.330030603869,123.068717754911)) ;
#70233=CARTESIAN_POINT('Ctrl Pts',(-18.2348676608804,43.1500415235061,123.137325455349)) ;
#70234=CARTESIAN_POINT('Ctrl Pts',(-18.0222521551209,43.3399247112482,122.821614169064)) ;
#70235=CARTESIAN_POINT('Ctrl Pts',(-18.2996598001454,43.1599356308853,122.939643522461)) ;
#70236=CARTESIAN_POINT('Ctrl Pts',(-18.1448649357578,43.3498670434406,122.590937416187)) ;
#70237=CARTESIAN_POINT('Ctrl Pts',(-18.3977518184139,43.1698779630777,122.755103312914)) ;
#70238=CARTESIAN_POINT('Ctrl Pts',(-18.3065565946206,43.3598676697556,122.383706851709)) ;
#70239=CARTESIAN_POINT('Ctrl Pts',(-18.5271067799686,43.1798785893927,122.589320225833)) ;
#70240=CARTESIAN_POINT('Ctrl Pts',(-18.5028573530525,43.3699094040375,122.207385535582)) ;
#70241=CARTESIAN_POINT('Ctrl Pts',(-18.6841488602168,43.1899203236746,122.448264772866)) ;
#70242=CARTESIAN_POINT('Ctrl Pts',(-18.7217003533941,43.3797348299866,122.070323331608)) ;
#70243=CARTESIAN_POINT('Ctrl Pts',(-18.8592239561885,43.1997457496237,122.338617074552)) ;
#70244=CARTESIAN_POINT('Ctrl Pts',(-18.9664691272905,43.3897916565143,121.970708884775)) ;
#70245=CARTESIAN_POINT('Ctrl Pts',(-19.0550398228914,43.2098025761514,122.258927422049)) ;
#70246=CARTESIAN_POINT('Ctrl Pts',(-19.2216018609428,43.3997190896358,121.916174470016)) ;
#70247=CARTESIAN_POINT('Ctrl Pts',(-19.2591461961739,43.219730009273,122.215302017841)) ;
#70248=CARTESIAN_POINT('Ctrl Pts',(-19.4828888562582,43.4096690820421,121.905998966867)) ;
#70249=CARTESIAN_POINT('Ctrl Pts',(-19.4681756430009,43.2296800016792,122.207163663939)) ;
#70250=CARTESIAN_POINT('Ctrl Pts',(-19.7446216548047,43.4197242831161,121.942178613796)) ;
#70251=CARTESIAN_POINT('Ctrl Pts',(-19.6775616803327,43.2397352027532,122.236109468103)) ;
#70252=CARTESIAN_POINT('Ctrl Pts',(-19.9904509322207,43.4295465571684,122.02094445218)) ;
#70253=CARTESIAN_POINT('Ctrl Pts',(-19.8742238828704,43.2495574768055,122.299123887706)) ;
#70254=CARTESIAN_POINT('Ctrl Pts',(-20.2244870380784,43.4396024511276,122.143621831466)) ;
#70255=CARTESIAN_POINT('Ctrl Pts',(-20.0614519256092,43.2596133707647,122.397267588395)) ;
#70256=CARTESIAN_POINT('Ctrl Pts',(-20.4310096168158,43.4495431729727,122.303608199071)) ;
#70257=CARTESIAN_POINT('Ctrl Pts',(-20.2266685268885,43.2695540926099,122.525258131967)) ;
#70258=CARTESIAN_POINT('Ctrl Pts',(-20.6065731184016,43.4594475170593,122.495763120482)) ;
#70259=CARTESIAN_POINT('Ctrl Pts',(-20.3671176119606,43.2794584366965,122.678983058845)) ;
#70260=CARTESIAN_POINT('Ctrl Pts',(-20.7479541652507,43.4694941843588,122.718707024721)) ;
#70261=CARTESIAN_POINT('Ctrl Pts',(-20.4802208409037,43.2895051039959,122.857339300646)) ;
#70262=CARTESIAN_POINT('Ctrl Pts',(-20.8472092355886,43.4793897428087,122.95911028977)) ;
#70263=CARTESIAN_POINT('Ctrl Pts',(-20.5596229418343,43.2994006624459,123.049662215042)) ;
#70264=CARTESIAN_POINT('Ctrl Pts',(-20.904139618028,43.4894518215134,123.217291078424)) ;
#70265=CARTESIAN_POINT('Ctrl Pts',(-20.6051653985535,43.3094627411505,123.256207403565)) ;
#70266=CARTESIAN_POINT('Ctrl Pts',(-20.9152824166523,43.4992945199792,123.475736104278)) ;
#70267=CARTESIAN_POINT('Ctrl Pts',(-20.6140777067984,43.3193054396163,123.462962813021)) ;
#70268=CARTESIAN_POINT('Ctrl Pts',(-20.8814961280243,43.5092852938737,123.736067222342)) ;
#70269=CARTESIAN_POINT('Ctrl Pts',(-20.5870468982505,43.3292962135108,123.671227335157)) ;
#70270=CARTESIAN_POINT('Ctrl Pts',(-20.8034587033046,43.5192131631086,123.985028739388)) ;
#70271=CARTESIAN_POINT('Ctrl Pts',(-20.5246153423973,43.3392240827457,123.870395633847)) ;
#70272=CARTESIAN_POINT('Ctrl Pts',(-20.6830540646815,43.5292018920784,124.218293703487)) ;
#70273=CARTESIAN_POINT('Ctrl Pts',(-20.4282901545074,43.3492128117156,124.057006673629)) ;
#70274=CARTESIAN_POINT('Ctrl Pts',(-20.5227971110946,43.5392412940622,124.427851205494)) ;
#70275=CARTESIAN_POINT('Ctrl Pts',(-20.3000830928166,43.3592522136993,124.224651637506)) ;
#70276=CARTESIAN_POINT('Ctrl Pts',(-20.3327674227349,43.549081461799,124.603250592089)) ;
#70277=CARTESIAN_POINT('Ctrl Pts',(-20.1480587518174,43.3690923814361,124.36496932946)) ;
#70278=CARTESIAN_POINT('Ctrl Pts',(-20.1108004287422,43.5591296721735,124.746255706704)) ;
#70279=CARTESIAN_POINT('Ctrl Pts',(-19.9704841479097,43.3791405918106,124.479372086508)) ;
#70280=CARTESIAN_POINT('Ctrl Pts',(-19.8696476488821,43.5690768424612,124.84714360705)) ;
#70281=CARTESIAN_POINT('Ctrl Pts',(-19.7775615548716,43.3890877620984,124.560080670385)) ;
#70282=CARTESIAN_POINT('Ctrl Pts',(-19.6157403076391,43.5789876907163,124.905179129313)) ;
#70283=CARTESIAN_POINT('Ctrl Pts',(-19.5744358437637,43.3989986103534,124.606507405916)) ;
#70284=CARTESIAN_POINT('Ctrl Pts',(-19.3518069355752,43.5890440183941,124.91818859538)) ;
#70285=CARTESIAN_POINT('Ctrl Pts',(-19.3632888855343,43.4090549380312,124.616913341816)) ;
#70286=CARTESIAN_POINT('Ctrl Pts',(-19.0949363387433,43.5988944311626,124.886068138014)) ;
#70287=CARTESIAN_POINT('Ctrl Pts',(-19.1577934324893,43.4189053507997,124.591215484819)) ;
#70288=CARTESIAN_POINT('Ctrl Pts',(-18.8429401699179,43.6089213169963,124.809086046414)) ;
#70289=CARTESIAN_POINT('Ctrl Pts',(-18.9561969026727,43.4289322366334,124.529628381766)) ;
#70290=CARTESIAN_POINT('Ctrl Pts',(-18.608395133658,43.6189499326271,124.688881455388)) ;
#70291=CARTESIAN_POINT('Ctrl Pts',(-18.7685615614303,43.4389608522643,124.433463244299)) ;
#70292=CARTESIAN_POINT('Ctrl Pts',(-18.4018522456686,43.6287951560046,124.53309241998)) ;
#70293=CARTESIAN_POINT('Ctrl Pts',(-18.6033288833992,43.4488060756417,124.308831339944)) ;
#70294=CARTESIAN_POINT('Ctrl Pts',(-18.2223621198309,43.6387858381062,124.34147662207)) ;
#70295=CARTESIAN_POINT('Ctrl Pts',(-18.4597378987131,43.4587967577433,124.15553787085)) ;
#70296=CARTESIAN_POINT('Ctrl Pts',(-18.0786893213183,43.6488237267386,124.120254417819)) ;
#70297=CARTESIAN_POINT('Ctrl Pts',(-18.344800860244,43.4688346463758,123.97855920037)) ;
#70298=CARTESIAN_POINT('Ctrl Pts',(-17.977176387725,43.6586680618418,123.882292776737)) ;
#70299=CARTESIAN_POINT('Ctrl Pts',(-18.2635921771929,43.4786789814789,123.788190198657)) ;
#70300=CARTESIAN_POINT('Ctrl Pts',(-17.917193628408,43.6686530240393,123.626883148383)) ;
#70301=CARTESIAN_POINT('Ctrl Pts',(-18.2156072828888,43.4886639436764,123.583862392775)) ;
#70302=CARTESIAN_POINT('Ctrl Pts',(-17.9024116244684,43.6785919655727,123.366078461576)) ;
#70303=CARTESIAN_POINT('Ctrl Pts',(-18.2037829771252,43.4986028852098,123.375219006614)) ;
#70304=CARTESIAN_POINT('Ctrl Pts',(-17.9335320666697,43.6886338505441,123.104055220491)) ;
#70305=CARTESIAN_POINT('Ctrl Pts',(-18.2286806289882,43.5086447701812,123.165600448032)) ;
#70306=CARTESIAN_POINT('Ctrl Pts',(-18.008352723709,43.6985203984524,122.855226846736)) ;
#70307=CARTESIAN_POINT('Ctrl Pts',(-18.2885381427592,43.5185313180895,122.966538824401)) ;
#70308=CARTESIAN_POINT('Ctrl Pts',(-18.1261385188554,43.7085143239524,122.620528575572)) ;
#70309=CARTESIAN_POINT('Ctrl Pts',(-18.3827677656657,43.5285252435895,122.778780862316)) ;
#70310=CARTESIAN_POINT('Ctrl Pts',(-18.2819245676956,43.7184504150789,122.410933846051)) ;
#70311=CARTESIAN_POINT('Ctrl Pts',(-18.5073972462572,43.538461334716,122.61110613432)) ;
#70312=CARTESIAN_POINT('Ctrl Pts',(-18.4734970875813,43.7284796840588,122.229979319978)) ;
#70313=CARTESIAN_POINT('Ctrl Pts',(-18.6606561040544,43.5484906036959,122.466343315554)) ;
#70314=CARTESIAN_POINT('Ctrl Pts',(-18.6902358432055,43.7383620666181,122.086843147979)) ;
#70315=CARTESIAN_POINT('Ctrl Pts',(-18.8340470312142,43.5583729862552,122.351835729643)) ;
#70316=CARTESIAN_POINT('Ctrl Pts',(-18.9325293093004,43.748414583706,121.981687073779)) ;
#70317=CARTESIAN_POINT('Ctrl Pts',(-19.0278824125168,43.5684255033431,122.267711767066)) ;
#70318=CARTESIAN_POINT('Ctrl Pts',(-19.1854080916355,43.7583087045299,121.921017634688)) ;
#70319=CARTESIAN_POINT('Ctrl Pts',(-19.2301849629632,43.578319624167,122.219177394001)) ;
#70320=CARTESIAN_POINT('Ctrl Pts',(-19.4492993318414,43.7683706839503,121.904850471576)) ;
#70321=CARTESIAN_POINT('Ctrl Pts',(-19.4412982796223,43.5883816035874,122.2062446672)) ;
#70322=CARTESIAN_POINT('Ctrl Pts',(-19.7063573702631,43.7782152171792,121.934076663056)) ;
#70323=CARTESIAN_POINT('Ctrl Pts',(-19.6469435446541,43.5982261368164,122.22962650948)) ;
#70324=CARTESIAN_POINT('Ctrl Pts',(-19.9576002327423,43.7881752960855,122.007446102476)) ;
#70325=CARTESIAN_POINT('Ctrl Pts',(-19.8479372613017,43.6081862157226,122.288322719679)) ;
#70326=CARTESIAN_POINT('Ctrl Pts',(-20.1938925036668,43.7982135726581,122.124695495129)) ;
#70327=CARTESIAN_POINT('Ctrl Pts',(-20.0369707873508,43.6182244922952,122.382123111982)) ;
#70328=CARTESIAN_POINT('Ctrl Pts',(-20.403085266942,43.8080869591959,122.278251260109)) ;
#70329=CARTESIAN_POINT('Ctrl Pts',(-20.2043238013652,43.6280978788331,122.504967832787)) ;
#70330=CARTESIAN_POINT('Ctrl Pts',(-20.5859442921562,43.818159901963,122.469575837394)) ;
#70331=CARTESIAN_POINT('Ctrl Pts',(-20.3506106669078,43.6381708216001,122.65802830527)) ;
#70332=CARTESIAN_POINT('Ctrl Pts',(-20.7294563688574,43.8279813160913,122.684155238316)) ;
#70333=CARTESIAN_POINT('Ctrl Pts',(-20.4654190257997,43.6479922357285,122.829691205274)) ;
#70334=CARTESIAN_POINT('Ctrl Pts',(-20.8364643232835,43.8380559461636,122.926263897482)) ;
#70335=CARTESIAN_POINT('Ctrl Pts',(-20.5510249269012,43.6580668658008,123.023378728422)) ;
#70336=CARTESIAN_POINT('Ctrl Pts',(-20.8984148212984,43.8479225834805,123.178073112069)) ;
#70337=CARTESIAN_POINT('Ctrl Pts',(-20.6005844237704,43.6679335031176,123.224825316576)) ;
#70338=CARTESIAN_POINT('Ctrl Pts',(-20.9166483132866,43.8579461288523,123.440837266538)) ;
#70339=CARTESIAN_POINT('Ctrl Pts',(-20.6151706983292,43.6779570484894,123.435036712492)) ;
#70340=CARTESIAN_POINT('Ctrl Pts',(-20.8883395523817,43.8679718803695,123.702794177763)) ;
#70341=CARTESIAN_POINT('Ctrl Pts',(-20.5925230028488,43.6879828000066,123.644602236926)) ;
#70342=CARTESIAN_POINT('Ctrl Pts',(-20.8166599479504,43.8778254673789,123.951603594725)) ;
#70343=CARTESIAN_POINT('Ctrl Pts',(-20.5351790633335,43.697836387016,123.843648589782)) ;
#70344=CARTESIAN_POINT('Ctrl Pts',(-20.702060923653,43.8878024276068,124.187422142841)) ;
#70345=CARTESIAN_POINT('Ctrl Pts',(-20.4434995981191,43.7078133472439,124.032303014082)) ;
#70346=CARTESIAN_POINT('Ctrl Pts',(-20.5472263847729,43.8978235706353,124.400424003541)) ;
#70347=CARTESIAN_POINT('Ctrl Pts',(-20.3196315437923,43.7178344902724,124.202704210316)) ;
#70348=CARTESIAN_POINT('Ctrl Pts',(-20.3607073265626,43.9077061766552,124.581187205771)) ;
#70349=CARTESIAN_POINT('Ctrl Pts',(-20.1704166645511,43.7277170962923,124.34731388807)) ;
#70350=CARTESIAN_POINT('Ctrl Pts',(-20.141598516524,43.9177746472879,124.729426223139)) ;
#70351=CARTESIAN_POINT('Ctrl Pts',(-19.9951291156329,43.737785566925,124.465904948293)) ;
#70352=CARTESIAN_POINT('Ctrl Pts',(-19.9058383854937,43.9276047304716,124.835123522503)) ;
#70353=CARTESIAN_POINT('Ctrl Pts',(-19.8065220003896,43.7476156501087,124.550461981873)) ;
#70354=CARTESIAN_POINT('Ctrl Pts',(-19.6494502413749,43.937671290152,124.900110672069)) ;
#70355=CARTESIAN_POINT('Ctrl Pts',(-19.6014111164167,43.7576822097891,124.602451541965)) ;
#70356=CARTESIAN_POINT('Ctrl Pts',(-19.3902067493444,43.9475615399812,124.919096378298)) ;
#70357=CARTESIAN_POINT('Ctrl Pts',(-19.3940171383949,43.7675724596183,124.617639759188)) ;
#70358=CARTESIAN_POINT('Ctrl Pts',(-19.1289291993489,43.95755370573,124.893086593962)) ;
#70359=CARTESIAN_POINT('Ctrl Pts',(-19.1849952828708,43.7775646253671,124.59683180778)) ;
#70360=CARTESIAN_POINT('Ctrl Pts',(-18.8769378575391,43.9675165493261,124.822071866951)) ;
#70361=CARTESIAN_POINT('Ctrl Pts',(-18.9834026165215,43.7875274689632,124.54001992677)) ;
#70362=CARTESIAN_POINT('Ctrl Pts',(-18.6421796236828,43.9774207181539,124.709636238937)) ;
#70363=CARTESIAN_POINT('Ctrl Pts',(-18.7955967231379,43.797431637791,124.450071716623)) ;
#70364=CARTESIAN_POINT('Ctrl Pts',(-18.4273472596352,43.9874815930482,124.555590382771)) ;
#70365=CARTESIAN_POINT('Ctrl Pts',(-18.6237306573745,43.8074925126853,124.32683478731)) ;
#70366=CARTESIAN_POINT('Ctrl Pts',(-18.2462912417937,43.9973204963776,124.370950929424)) ;
#70367=CARTESIAN_POINT('Ctrl Pts',(-18.4788866747654,43.8173314160147,124.179124065439)) ;
#70368=CARTESIAN_POINT('Ctrl Pts',(-18.096473040413,44.0073888727515,124.152920066805)) ;
#70369=CARTESIAN_POINT('Ctrl Pts',(-18.3590318811178,43.8273997923886,124.004699145389)) ;
#70370=CARTESIAN_POINT('Ctrl Pts',(-17.9888795242822,44.0172694893841,123.916566377132)) ;
#70371=CARTESIAN_POINT('Ctrl Pts',(-18.2729574087279,43.8372804090212,123.815617033052)) ;
#70372=CARTESIAN_POINT('Ctrl Pts',(-17.9227396809683,44.0272606496131,123.662515814642)) ;
#70373=CARTESIAN_POINT('Ctrl Pts',(-18.2200454142358,43.8472715692502,123.612376795175)) ;
#70374=CARTESIAN_POINT('Ctrl Pts',(-17.9017478866056,44.0372137230452,123.40176367561)) ;
#70375=CARTESIAN_POINT('Ctrl Pts',(-18.2032518302433,43.8572246426823,123.403775507638)) ;
#70376=CARTESIAN_POINT('Ctrl Pts',(-17.9266347799871,44.0472495586578,123.139231148737)) ;
#70377=CARTESIAN_POINT('Ctrl Pts',(-18.2231612008556,43.867260478295,123.193749351306)) ;
#70378=CARTESIAN_POINT('Ctrl Pts',(-17.9955495886584,44.057139685388,122.888614558069)) ;
#70379=CARTESIAN_POINT('Ctrl Pts',(-18.2782926266805,43.8771506050251,122.993256851643)) ;
#70380=CARTESIAN_POINT('Ctrl Pts',(-18.1076878440328,44.0671318671573,122.651194666647)) ;
#70381=CARTESIAN_POINT('Ctrl Pts',(-18.3680028793089,43.8871427867944,122.803320956342)) ;
#70382=CARTESIAN_POINT('Ctrl Pts',(-18.2587247866769,44.0770778071318,122.437883820146)) ;
#70383=CARTESIAN_POINT('Ctrl Pts',(-18.4888319257956,43.8970887267689,122.632672501952)) ;
#70384=CARTESIAN_POINT('Ctrl Pts',(-18.4441648499972,44.0870249908912,122.253628827194)) ;
#70385=CARTESIAN_POINT('Ctrl Pts',(-18.6371833541905,43.9070359105284,122.485268533601)) ;
#70386=CARTESIAN_POINT('Ctrl Pts',(-18.6611045195494,44.0970729291816,122.103115117568)) ;
#70387=CARTESIAN_POINT('Ctrl Pts',(-18.8107350578741,43.9170838488187,122.364857168353)) ;
#70388=CARTESIAN_POINT('Ctrl Pts',(-18.8960216519544,44.1069205639951,121.9945561486)) ;
#70389=CARTESIAN_POINT('Ctrl Pts',(-18.9986675796601,43.9269314836323,122.278010099489)) ;
#70390=CARTESIAN_POINT('Ctrl Pts',(-19.1488932353645,44.1168822776931,121.926880369107)) ;
#70391=CARTESIAN_POINT('Ctrl Pts',(-19.200964338225,43.9368931973302,122.223868984643)) ;
#70392=CARTESIAN_POINT('Ctrl Pts',(-19.4114837782062,44.1269109135143,121.904316948058)) ;
#70393=CARTESIAN_POINT('Ctrl Pts',(-19.4110368048726,43.9469218331514,122.205817721799)) ;
#70394=CARTESIAN_POINT('Ctrl Pts',(-19.6708855677709,44.136821228266,121.927328148373)) ;
#70395=CARTESIAN_POINT('Ctrl Pts',(-19.6185575864657,43.9568321479032,122.224226080018)) ;
#70396=CARTESIAN_POINT('Ctrl Pts',(-19.923172854028,44.1467560989287,121.994541369525)) ;
#70397=CARTESIAN_POINT('Ctrl Pts',(-19.8203870878445,43.9667670185658,122.277995832626)) ;
#70398=CARTESIAN_POINT('Ctrl Pts',(-20.1623656622643,44.1567972813305,122.105936279633)) ;
#70399=CARTESIAN_POINT('Ctrl Pts',(-20.011741745876,43.9768082009676,122.367111237361)) ;
#70400=CARTESIAN_POINT('Ctrl Pts',(-20.3754115587803,44.1666842527952,122.254696080828)) ;
#70401=CARTESIAN_POINT('Ctrl Pts',(-20.1821781748641,43.9866951724323,122.486118021261)) ;
#70402=CARTESIAN_POINT('Ctrl Pts',(-20.5616797006254,44.1766836850578,122.439998156239)) ;
#70403=CARTESIAN_POINT('Ctrl Pts',(-20.3311931547893,43.9966946046949,122.634359041277)) ;
#70404=CARTESIAN_POINT('Ctrl Pts',(-20.7119248209942,44.1866037503144,122.653074790023)) ;
#70405=CARTESIAN_POINT('Ctrl Pts',(-20.4513895765128,44.0066146699516,122.804819385592)) ;
#70406=CARTESIAN_POINT('Ctrl Pts',(-20.8242248480084,44.1966406028986,122.89171516179)) ;
#70407=CARTESIAN_POINT('Ctrl Pts',(-20.5412304078257,44.0166515225357,122.995731440884)) ;
#70408=CARTESIAN_POINT('Ctrl Pts',(-20.8925256088344,44.2065532622386,123.143101297578)) ;
#70409=CARTESIAN_POINT('Ctrl Pts',(-20.5958716458054,44.0265641818757,123.19683949956)) ;
#70410=CARTESIAN_POINT('Ctrl Pts',(-20.9168966357386,44.2165444741535,123.404542148438)) ;
#70411=CARTESIAN_POINT('Ctrl Pts',(-20.6153694127085,44.0365553937906,123.405991922717)) ;
#70412=CARTESIAN_POINT('Ctrl Pts',(-20.8948063197256,44.2265861155566,123.667478543077)) ;
#70413=CARTESIAN_POINT('Ctrl Pts',(-20.597697972569,44.0465970351937,123.616341249776)) ;
#70414=CARTESIAN_POINT('Ctrl Pts',(-20.8294398407361,44.2364149097636,123.917397995982)) ;
#70415=CARTESIAN_POINT('Ctrl Pts',(-20.5454060288172,44.0564258294008,123.816275945776)) ;
#70416=CARTESIAN_POINT('Ctrl Pts',(-20.7190966284838,44.2464913208849,124.158051348321)) ;
#70417=CARTESIAN_POINT('Ctrl Pts',(-20.45713223089,44.066502240522,124.008799361129)) ;
#70418=CARTESIAN_POINT('Ctrl Pts',(-20.5720419186679,44.2563434539274,124.371206621261)) ;
#70419=CARTESIAN_POINT('Ctrl Pts',(-20.3394898756421,44.0763543735645,124.179323355511)) ;
#70420=CARTESIAN_POINT('Ctrl Pts',(-20.3863598082827,44.2664166882687,124.559814357932)) ;
#70421=CARTESIAN_POINT('Ctrl Pts',(-20.1909447374728,44.0864276079058,124.330210536534)) ;
#70422=CARTESIAN_POINT('Ctrl Pts',(-20.1756188492781,44.2762581895953,124.709761183194)) ;
#70423=CARTESIAN_POINT('Ctrl Pts',(-20.0223534395185,44.0962691092324,124.450168264063)) ;
#70424=CARTESIAN_POINT('Ctrl Pts',(-19.9396571120249,44.2862191411901,124.823064731638)) ;
#70425=CARTESIAN_POINT('Ctrl Pts',(-19.833584900295,44.1062300608272,124.540812125368)) ;
#70426=CARTESIAN_POINT('Ctrl Pts',(-19.6855192485354,44.2962569589108,124.893713217866)) ;
#70427=CARTESIAN_POINT('Ctrl Pts',(-19.630274821082,44.1162678785479,124.597332072431)) ;
#70428=CARTESIAN_POINT('Ctrl Pts',(-19.4272568805915,44.3061313081678,124.919231077549)) ;
#70429=CARTESIAN_POINT('Ctrl Pts',(-19.4236658581151,44.1261422278049,124.617747552398)) ;
#70430=CARTESIAN_POINT('Ctrl Pts',(-19.1634421663118,44.31620085891,124.899117334135)) ;
#70431=CARTESIAN_POINT('Ctrl Pts',(-19.2126137105638,44.1362117785471,124.601657806731)) ;
#70432=CARTESIAN_POINT('Ctrl Pts',(-18.9130262792897,44.3260348784186,124.835165719918)) ;
#70433=CARTESIAN_POINT('Ctrl Pts',(-19.0122816736547,44.1460457980557,124.55049803559)) ;
#70434=CARTESIAN_POINT('Ctrl Pts',(-18.6724761256092,44.3360690329981,124.727189304434)) ;
#70435=CARTESIAN_POINT('Ctrl Pts',(-18.8198408751358,44.1560799526353,124.464118191425)) ;
#70436=CARTESIAN_POINT('Ctrl Pts',(-18.4550666358706,44.3460849588206,124.578799029693)) ;
#70437=CARTESIAN_POINT('Ctrl Pts',(-18.6459125515534,44.1660958784577,124.345407061156)) ;
#70438=CARTESIAN_POINT('Ctrl Pts',(-18.2689206934433,44.3559672140149,124.397708730824)) ;
#70439=CARTESIAN_POINT('Ctrl Pts',(-18.4969953334488,44.175978133652,124.200536340073)) ;
#70440=CARTESIAN_POINT('Ctrl Pts',(-18.1151639542311,44.3659560205258,124.184994122571)) ;
#70441=CARTESIAN_POINT('Ctrl Pts',(-18.3739888404937,44.1859669401629,124.030365648299)) ;
#70442=CARTESIAN_POINT('Ctrl Pts',(-18.0009287364672,44.3759045877885,123.949788452977)) ;
#70443=CARTESIAN_POINT('Ctrl Pts',(-18.2825994652639,44.1959155074256,123.842202101952)) ;
#70444=CARTESIAN_POINT('Ctrl Pts',(-17.9287930124207,44.3859593930905,123.695625807384)) ;
#70445=CARTESIAN_POINT('Ctrl Pts',(-18.2248894332105,44.2059703127276,123.638872216548)) ;
#70446=CARTESIAN_POINT('Ctrl Pts',(-17.9021400804517,44.3957781763541,123.438965134921)) ;
#70447=CARTESIAN_POINT('Ctrl Pts',(-18.2035656682634,44.2157890959912,123.433544841874)) ;
#70448=CARTESIAN_POINT('Ctrl Pts',(-17.9201546965115,44.4058139487147,123.175857889878)) ;
#70449=CARTESIAN_POINT('Ctrl Pts',(-18.2179757049312,44.2258248683518,123.223058844661)) ;
#70450=CARTESIAN_POINT('Ctrl Pts',(-17.9842443392215,44.4158386477433,122.920324456169)) ;
#70451=CARTESIAN_POINT('Ctrl Pts',(-18.2692459457446,44.2358495673804,123.018631708746)) ;
#70452=CARTESIAN_POINT('Ctrl Pts',(-18.0893534627256,44.4256906510024,122.683715321304)) ;
#70453=CARTESIAN_POINT('Ctrl Pts',(-18.3533314265156,44.2457015706395,122.8293444755)) ;
#70454=CARTESIAN_POINT('Ctrl Pts',(-18.2356357013134,44.4356815853996,122.46572907487)) ;
#70455=CARTESIAN_POINT('Ctrl Pts',(-18.4703557257671,44.2556925050367,122.654954642238)) ;
#70456=CARTESIAN_POINT('Ctrl Pts',(-18.41613673709,44.4455995078307,122.277671975149)) ;
#70457=CARTESIAN_POINT('Ctrl Pts',(-18.6147549895924,44.2656104274678,122.504508093951)) ;
#70458=CARTESIAN_POINT('Ctrl Pts',(-18.6288136047377,44.455627863513,122.122084840499)) ;
#70459=CARTESIAN_POINT('Ctrl Pts',(-18.7848954782,44.2756387831502,122.380036963716)) ;
#70460=CARTESIAN_POINT('Ctrl Pts',(-18.8618504936233,44.4655121480236,122.007331995514)) ;
#70461=CARTESIAN_POINT('Ctrl Pts',(-18.9713236802826,44.2855230676607,122.288233368328)) ;
#70462=CARTESIAN_POINT('Ctrl Pts',(-19.1138322342733,44.4755048319315,121.933421901147)) ;
#70463=CARTESIAN_POINT('Ctrl Pts',(-19.1729084429983,44.2955157515686,122.229103542104)) ;
#70464=CARTESIAN_POINT('Ctrl Pts',(-19.3758137501504,44.4855335689392,121.904740742867)) ;
#70465=CARTESIAN_POINT('Ctrl Pts',(-19.3824934791347,44.3055444885763,122.206156839405)) ;
#70466=CARTESIAN_POINT('Ctrl Pts',(-19.6350667634332,44.4954189655681,121.921395206069)) ;
#70467=CARTESIAN_POINT('Ctrl Pts',(-19.5898954555801,44.3154298852052,122.219478539478)) ;
#70468=CARTESIAN_POINT('Ctrl Pts',(-19.8901602887943,44.505406850982,121.983076127047)) ;
#70469=CARTESIAN_POINT('Ctrl Pts',(-19.7939705951904,44.3254177706191,122.268821404401)) ;
#70470=CARTESIAN_POINT('Ctrl Pts',(-20.1298803582596,44.5153575536426,122.087637628189)) ;
#70471=CARTESIAN_POINT('Ctrl Pts',(-19.9857471730679,44.3353684732797,122.35246874884)) ;
#70472=CARTESIAN_POINT('Ctrl Pts',(-20.3496330623717,44.52539787174,122.233619868658)) ;
#70473=CARTESIAN_POINT('Ctrl Pts',(-20.1615504313535,44.3454087913771,122.469252999656)) ;
#70474=CARTESIAN_POINT('Ctrl Pts',(-20.5377640234238,44.5352724370732,122.412390214829)) ;
#70475=CARTESIAN_POINT('Ctrl Pts',(-20.3120561285973,44.3552833567104,122.612267503124)) ;
#70476=CARTESIAN_POINT('Ctrl Pts',(-20.6941762400211,44.5452720971343,122.62349750357)) ;
#70477=CARTESIAN_POINT('Ctrl Pts',(-20.4371874373751,44.3652830167714,122.781152089198)) ;
#70478=CARTESIAN_POINT('Ctrl Pts',(-20.8107568463258,44.555181092302,122.856392682696)) ;
#70479=CARTESIAN_POINT('Ctrl Pts',(-20.5304535425006,44.3751920119392,122.967466996356)) ;
#70480=CARTESIAN_POINT('Ctrl Pts',(-20.8861166779856,44.5652358334653,123.109601455861)) ;
#70481=CARTESIAN_POINT('Ctrl Pts',(-20.5907433453259,44.3852467531024,123.170033530578)) ;
#70482=CARTESIAN_POINT('Ctrl Pts',(-20.9160838152059,44.5750944453791,123.36698258296)) ;
#70483=CARTESIAN_POINT('Ctrl Pts',(-20.6147190097219,44.3951053650162,123.375937681712)) ;
#70484=CARTESIAN_POINT('Ctrl Pts',(-20.9007482951995,44.5851625676584,123.631078613714)) ;
#70485=CARTESIAN_POINT('Ctrl Pts',(-20.6024526333435,44.4051734872955,123.587214747284)) ;
#70486=CARTESIAN_POINT('Ctrl Pts',(-20.8410433869187,44.5950180383616,123.883116987979)) ;
#70487=CARTESIAN_POINT('Ctrl Pts',(-20.5546908119095,44.4150289579987,123.788845432467)) ;
#70488=CARTESIAN_POINT('Ctrl Pts',(-20.737768269546,44.605012897855,124.124606144448)) ;
#70489=CARTESIAN_POINT('Ctrl Pts',(-20.4720727081621,44.4250238174921,123.982037522316)) ;
#70490=CARTESIAN_POINT('Ctrl Pts',(-20.5931261612872,44.6150441511969,124.344997164701)) ;
#70491=CARTESIAN_POINT('Ctrl Pts',(-20.3563607533755,44.435055070834,124.158351473366)) ;
#70492=CARTESIAN_POINT('Ctrl Pts',(-20.4156755541826,44.62491085007,124.534060702266)) ;
#70493=CARTESIAN_POINT('Ctrl Pts',(-20.2144020898501,44.4449217697071,124.309603448869)) ;
#70494=CARTESIAN_POINT('Ctrl Pts',(-20.2058546846897,44.6348976658212,124.691655677439)) ;
#70495=CARTESIAN_POINT('Ctrl Pts',(-20.0465467658949,44.4549085854583,124.435681091647)) ;
#70496=CARTESIAN_POINT('Ctrl Pts',(-19.9727822075021,44.6448448710167,124.810089850081)) ;
#70497=CARTESIAN_POINT('Ctrl Pts',(-19.8600899289393,44.4648557906538,124.530430271056)) ;
#70498=CARTESIAN_POINT('Ctrl Pts',(-19.7202958616412,44.6548878591429,124.886862052342)) ;
#70499=CARTESIAN_POINT('Ctrl Pts',(-19.6581014661053,44.4748987787801,124.591850096019)) ;
#70500=CARTESIAN_POINT('Ctrl Pts',(-19.4628869098935,44.6647552137644,124.91822843966)) ;
#70501=CARTESIAN_POINT('Ctrl Pts',(-19.4521748954927,44.4847661334015,124.616945312954)) ;
#70502=CARTESIAN_POINT('Ctrl Pts',(-19.201339436511,44.6747211070625,124.904992081208)) ;
#70503=CARTESIAN_POINT('Ctrl Pts',(-19.242936917876,44.4947320266996,124.606358443205)) ;
#70504=CARTESIAN_POINT('Ctrl Pts',(-18.9446146117008,44.6847448844386,124.845931776589)) ;
#70505=CARTESIAN_POINT('Ctrl Pts',(-19.0375565977731,44.5047558040757,124.559112343262)) ;
#70506=CARTESIAN_POINT('Ctrl Pts',(-18.7044247703961,44.6946704323703,124.744265398415)) ;
#70507=CARTESIAN_POINT('Ctrl Pts',(-18.8454040419128,44.5146813520074,124.477781340274)) ;
#70508=CARTESIAN_POINT('Ctrl Pts',(-18.4848477732278,44.7046109087913,124.602728279973)) ;
#70509=CARTESIAN_POINT('Ctrl Pts',(-18.6697413477393,44.5246218284284,124.364553593259)) ;
#70510=CARTESIAN_POINT('Ctrl Pts',(-18.2913709521149,44.7146571184542,124.423127645142)) ;
#70511=CARTESIAN_POINT('Ctrl Pts',(-18.5149583948213,44.5346680380913,124.220874721725)) ;
#70512=CARTESIAN_POINT('Ctrl Pts',(-18.1347068986328,44.724518375116,124.216672914137)) ;
#70513=CARTESIAN_POINT('Ctrl Pts',(-18.3896255050784,44.5445292947531,124.055712452699)) ;
#70514=CARTESIAN_POINT('Ctrl Pts',(-18.0143070451238,44.7345120033913,123.983318570089)) ;
#70515=CARTESIAN_POINT('Ctrl Pts',(-18.2933036525415,44.5545229230284,123.869030062897)) ;
#70516=CARTESIAN_POINT('Ctrl Pts',(-17.936633762989,44.7444374007015,123.734282199344)) ;
#70517=CARTESIAN_POINT('Ctrl Pts',(-18.2311629143838,44.5644483203386,123.669801734943)) ;
#70518=CARTESIAN_POINT('Ctrl Pts',(-17.9030399617659,44.7544653086117,123.472943722699)) ;
#70519=CARTESIAN_POINT('Ctrl Pts',(-18.2042856479589,44.5744762282489,123.46073129079)) ;
#70520=CARTESIAN_POINT('Ctrl Pts',(-17.9148956263581,44.7643516242809,123.213374011942)) ;
#70521=CARTESIAN_POINT('Ctrl Pts',(-18.2137679274287,44.584362543918,123.253075513145)) ;
#70522=CARTESIAN_POINT('Ctrl Pts',(-17.9723197114155,44.7743832191847,122.95612772885)) ;
#70523=CARTESIAN_POINT('Ctrl Pts',(-18.2597049813133,44.5943941388218,123.047278048275)) ;
#70524=CARTESIAN_POINT('Ctrl Pts',(-18.0718425713874,44.7842654621364,122.716214046185)) ;
#70525=CARTESIAN_POINT('Ctrl Pts',(-18.3393211701474,44.6042763817735,122.855346286345)) ;
#70526=CARTESIAN_POINT('Ctrl Pts',(-18.2138824565932,44.7943249331663,122.493298818431)) ;
#70527=CARTESIAN_POINT('Ctrl Pts',(-18.452951139445,44.6143358528034,122.677012948951)) ;
#70528=CARTESIAN_POINT('Ctrl Pts',(-18.3890982744024,44.8041913778294,122.302163339125)) ;
#70529=CARTESIAN_POINT('Ctrl Pts',(-18.5931221262605,44.6242022974665,122.524103052415)) ;
#70530=CARTESIAN_POINT('Ctrl Pts',(-18.5963979569655,44.8141575022781,122.142117824611)) ;
#70531=CARTESIAN_POINT('Ctrl Pts',(-18.7589604790486,44.6341684219152,122.396064874445)) ;
#70532=CARTESIAN_POINT('Ctrl Pts',(-18.8300300927451,44.8241877456692,122.020087986119)) ;
#70533=CARTESIAN_POINT('Ctrl Pts',(-18.9458651244295,44.6441986653064,122.298439056251)) ;
#70534=CARTESIAN_POINT('Ctrl Pts',(-19.0777784031114,44.8340807806223,121.941205272921)) ;
#70535=CARTESIAN_POINT('Ctrl Pts',(-19.1440629425059,44.6540917002594,122.235330716498)) ;
#70536=CARTESIAN_POINT('Ctrl Pts',(-19.3395157430304,44.8441316948591,121.905920090679)) ;
#70537=CARTESIAN_POINT('Ctrl Pts',(-19.3534531408236,44.6641426144963,122.207100459181)) ;
#70538=CARTESIAN_POINT('Ctrl Pts',(-19.5992088007417,44.8540215210837,121.916417743617)) ;
#70539=CARTESIAN_POINT('Ctrl Pts',(-19.561205041554,44.6740324407208,122.215496012711)) ;
#70540=CARTESIAN_POINT('Ctrl Pts',(-19.9417558495349,44.8673563361306,121.990481112151)) ;
#70541=CARTESIAN_POINT('Ctrl Pts',(-19.8352567550235,44.6873672557678,122.274745507017)) ;
#70542=CARTESIAN_POINT('Ctrl Pts',(-20.2554040575952,44.8806334273021,122.152088557895)) ;
#70543=CARTESIAN_POINT('Ctrl Pts',(-20.0861971038527,44.7006443469392,122.404050615546)) ;
#70544=CARTESIAN_POINT('Ctrl Pts',(-20.5136611155883,44.8938817159004,122.385626670228)) ;
#70545=CARTESIAN_POINT('Ctrl Pts',(-20.2927670421858,44.7138926355375,122.590851388565)) ;
#70546=CARTESIAN_POINT('Ctrl Pts',(-20.6757307463464,44.9039365573945,122.59426491759)) ;
#70547=CARTESIAN_POINT('Ctrl Pts',(-20.4224319383683,44.7239474770316,122.757766151545)) ;
#70548=CARTESIAN_POINT('Ctrl Pts',(-20.7967932245961,44.913767546702,122.822543238522)) ;
#70549=CARTESIAN_POINT('Ctrl Pts',(-20.5192820748052,44.7337784663392,122.940386237297)) ;
#70550=CARTESIAN_POINT('Ctrl Pts',(-20.8785256178797,44.9238441110252,123.074368365477)) ;
#70551=CARTESIAN_POINT('Ctrl Pts',(-20.5846700573935,44.7438550306624,123.141847246608)) ;
#70552=CARTESIAN_POINT('Ctrl Pts',(-20.9144646604309,44.9336934361592,123.330718388823)) ;
#70553=CARTESIAN_POINT('Ctrl Pts',(-20.6134249986564,44.7537043557963,123.346922032747)) ;
#70554=CARTESIAN_POINT('Ctrl Pts',(-20.9029627808752,44.9470414357965,123.681317025944)) ;
#70555=CARTESIAN_POINT('Ctrl Pts',(-20.60421795921,44.7670523554336,123.627426785072)) ;
#70556=CARTESIAN_POINT('Ctrl Pts',(-20.7745082951822,44.963626195333,124.10295325502)) ;
#70557=CARTESIAN_POINT('Ctrl Pts',(-20.5014772079403,44.7836371149701,123.964697051323)) ;
#70558=CARTESIAN_POINT('Ctrl Pts',(-20.5110259009966,44.9801947466811,124.455768261803)) ;
#70559=CARTESIAN_POINT('Ctrl Pts',(-20.2906509869384,44.8002056663183,124.247002496847)) ;
#70560=CARTESIAN_POINT('Ctrl Pts',(-20.2351348038895,44.9935545715001,124.672943272086)) ;
#70561=CARTESIAN_POINT('Ctrl Pts',(-20.0699761236227,44.8135654911373,124.420705379304)) ;
#70562=CARTESIAN_POINT('Ctrl Pts',(-20.0058393288218,45.0034599803308,124.796167835363)) ;
#70563=CARTESIAN_POINT('Ctrl Pts',(-19.8865323249825,44.8234708999679,124.519294746871)) ;
#70564=CARTESIAN_POINT('Ctrl Pts',(-19.757418400852,45.0134200069148,124.878510971796)) ;
#70565=CARTESIAN_POINT('Ctrl Pts',(-19.6878011258136,44.833430926552,124.585169321105)) ;
#70566=CARTESIAN_POINT('Ctrl Pts',(-19.4127381950797,45.0266775911001,124.929494089017)) ;
#70567=CARTESIAN_POINT('Ctrl Pts',(-19.4120406279165,44.8466885107373,124.62595768779)) ;
#70568=CARTESIAN_POINT('Ctrl Pts',(-18.9730728854828,45.0433288025948,124.878933487773)) ;
#70569=CARTESIAN_POINT('Ctrl Pts',(-19.0603260702002,44.8633397222319,124.585513496632)) ;
#70570=CARTESIAN_POINT('Ctrl Pts',(-18.4995381186548,45.0632470167051,124.642306903848)) ;
#70571=CARTESIAN_POINT('Ctrl Pts',(-18.6814904260909,44.8832579363422,124.396215029442)) ;
#70572=CARTESIAN_POINT('Ctrl Pts',(-18.1350210819867,45.0831247799259,124.259778759138)) ;
#70573=CARTESIAN_POINT('Ctrl Pts',(-18.3898754178223,44.9031356995631,124.090194473814)) ;
#70574=CARTESIAN_POINT('Ctrl Pts',(-17.9219902774577,45.1031374477131,123.772503946077)) ;
#70575=CARTESIAN_POINT('Ctrl Pts',(-18.219447255777,44.9231483673502,123.700376068826)) ;
#70576=CARTESIAN_POINT('Ctrl Pts',(-17.8878614143457,45.1229499703797,123.246927329174)) ;
#70577=CARTESIAN_POINT('Ctrl Pts',(-18.1921410117766,44.9429608900168,123.279913768998)) ;
#70578=CARTESIAN_POINT('Ctrl Pts',(-18.0355408684965,45.1429332703796,122.736855760796)) ;
#70579=CARTESIAN_POINT('Ctrl Pts',(-18.3102818169754,44.9629441900167,122.8718555916)) ;
#70580=CARTESIAN_POINT('Ctrl Pts',(-18.3474404946756,45.1628275474809,122.309788228837)) ;
#70581=CARTESIAN_POINT('Ctrl Pts',(-18.5597996758674,44.982838467118,122.530199273158)) ;
#70582=CARTESIAN_POINT('Ctrl Pts',(-18.786662149823,45.1827603092387,122.0135853007)) ;
#70583=CARTESIAN_POINT('Ctrl Pts',(-18.9111760676998,45.0027712288758,122.293234567284)) ;
#70584=CARTESIAN_POINT('Ctrl Pts',(-19.3015601046736,45.2027263150034,121.885187082688)) ;
#70585=CARTESIAN_POINT('Ctrl Pts',(-19.3230941010408,45.0227372346405,122.190513534484)) ;
#70586=CARTESIAN_POINT('Ctrl Pts',(-19.8271247057948,45.2226048471683,121.939586650986)) ;
#70587=CARTESIAN_POINT('Ctrl Pts',(-19.7435470906285,45.0426157668054,122.234031125667)) ;
#70588=CARTESIAN_POINT('Ctrl Pts',(-20.3041812489775,45.2425445138286,122.170281678288)) ;
#70589=CARTESIAN_POINT('Ctrl Pts',(-20.125193674908,45.0625554334657,122.418585724291)) ;
#70590=CARTESIAN_POINT('Ctrl Pts',(-20.673234757221,45.262439388474,122.549040856896)) ;
#70591=CARTESIAN_POINT('Ctrl Pts',(-20.4204384003569,45.0824503081111,122.721592696201)) ;
#70592=CARTESIAN_POINT('Ctrl Pts',(-20.8914226002841,45.2823465277673,123.03092366853)) ;
#70593=CARTESIAN_POINT('Ctrl Pts',(-20.5949902713448,45.1023574474044,123.107099401626)) ;
#70594=CARTESIAN_POINT('Ctrl Pts',(-20.933006994823,45.3022570758458,123.558648564266)) ;
#70595=CARTESIAN_POINT('Ctrl Pts',(-20.6282585345272,45.1222679954829,123.529280226432)) ;
#70596=CARTESIAN_POINT('Ctrl Pts',(-20.7897928711044,45.322325661203,124.072332126759)) ;
#70597=CARTESIAN_POINT('Ctrl Pts',(-20.513688465567,45.1423365808401,123.940226547894)) ;
#70598=CARTESIAN_POINT('Ctrl Pts',(-20.4845776581537,45.3421074585177,124.500648372566)) ;
#70599=CARTESIAN_POINT('Ctrl Pts',(-20.269515271003,45.1621183781549,124.282882031287)) ;
#70600=CARTESIAN_POINT('Ctrl Pts',(-20.0473359397164,45.3621150054623,124.802932073758)) ;
#70601=CARTESIAN_POINT('Ctrl Pts',(-19.9197218860292,45.1821259250994,124.524709061024)) ;
#70602=CARTESIAN_POINT('Ctrl Pts',(-19.5376317009415,45.3819367437651,124.936721152217)) ;
#70603=CARTESIAN_POINT('Ctrl Pts',(-19.5119562871531,45.2019476634022,124.631740691942)) ;
#70604=CARTESIAN_POINT('Ctrl Pts',(-19.0088087615849,45.4019167636693,124.889143040385)) ;
#70605=CARTESIAN_POINT('Ctrl Pts',(-19.0888977818351,45.2219276833064,124.593677332525)) ;
#70606=CARTESIAN_POINT('Ctrl Pts',(-18.5296775435496,45.4218342149315,124.664000015216)) ;
#70607=CARTESIAN_POINT('Ctrl Pts',(-18.7055922193586,45.2418451345686,124.413561830565)) ;
#70608=CARTESIAN_POINT('Ctrl Pts',(-18.1560490205525,45.4417091361042,124.2905332235)) ;
#70609=CARTESIAN_POINT('Ctrl Pts',(-18.4066894730446,45.2617200557413,124.114786420847)) ;
#70610=CARTESIAN_POINT('Ctrl Pts',(-17.9309504550834,45.461733504655,123.80830220994)) ;
#70611=CARTESIAN_POINT('Ctrl Pts',(-18.2266120673935,45.2817444242922,123.729001254374)) ;
#70612=CARTESIAN_POINT('Ctrl Pts',(-17.8844372685422,45.4816001890285,123.282245957211)) ;
#70613=CARTESIAN_POINT('Ctrl Pts',(-18.1894029640175,45.3016111086656,123.308154786778)) ;
#70614=CARTESIAN_POINT('Ctrl Pts',(-18.0199005695342,45.5015440108747,122.769835234287)) ;
#70615=CARTESIAN_POINT('Ctrl Pts',(-18.2977757249971,45.3215549305118,122.898226217715)) ;
#70616=CARTESIAN_POINT('Ctrl Pts',(-18.3217175474885,45.5214513801262,122.335254029468)) ;
#70617=CARTESIAN_POINT('Ctrl Pts',(-18.5392315505227,45.3414622997634,122.550561763219)) ;
#70618=CARTESIAN_POINT('Ctrl Pts',(-18.7524316861596,45.5413260778729,122.029454998175)) ;
#70619=CARTESIAN_POINT('Ctrl Pts',(-18.8838052127124,45.3613369975101,122.305924073514)) ;
#70620=CARTESIAN_POINT('Ctrl Pts',(-19.2643939100382,45.5613080203947,121.888099189238)) ;
#70621=CARTESIAN_POINT('Ctrl Pts',(-19.2933758171969,45.3813189400318,122.192842065019)) ;
#70622=CARTESIAN_POINT('Ctrl Pts',(-19.7916381676523,45.5812106873055,121.930204794695)) ;
#70623=CARTESIAN_POINT('Ctrl Pts',(-19.7151717616758,45.4012216069426,122.226529377587)) ;
#70624=CARTESIAN_POINT('Ctrl Pts',(-20.2724895989063,45.6010660448442,122.147814462636)) ;
#70625=CARTESIAN_POINT('Ctrl Pts',(-20.0998523930469,45.4210769644813,122.400620504394)) ;
#70626=CARTESIAN_POINT('Ctrl Pts',(-20.6536580199716,45.6211300835602,122.520640262332)) ;
#70627=CARTESIAN_POINT('Ctrl Pts',(-20.4047844905581,45.4411410031973,122.698883170157)) ;
#70628=CARTESIAN_POINT('Ctrl Pts',(-20.8822424651067,45.6409852632853,122.996499598304)) ;
#70629=CARTESIAN_POINT('Ctrl Pts',(-20.5876495721056,45.4609961829224,123.07957274604)) ;
#70630=CARTESIAN_POINT('Ctrl Pts',(-20.9354305273725,45.6609653679497,123.524661889087)) ;
#70631=CARTESIAN_POINT('Ctrl Pts',(-20.6301960379111,45.4809762875868,123.502103333297)) ;
#70632=CARTESIAN_POINT('Ctrl Pts',(-20.8068347567717,45.6807744731195,124.035365380666)) ;
#70633=CARTESIAN_POINT('Ctrl Pts',(-20.5273174457036,45.5007853927566,123.910665095287)) ;
#70634=CARTESIAN_POINT('Ctrl Pts',(-20.5095739145416,45.7007670934602,124.475605981024)) ;
#70635=CARTESIAN_POINT('Ctrl Pts',(-20.2894986134957,45.5207780130973,124.262859246648)) ;
#70636=CARTESIAN_POINT('Ctrl Pts',(-20.1539637829234,45.7173065759643,124.734247767366)) ;
#70637=CARTESIAN_POINT('Ctrl Pts',(-20.005029677627,45.5373174956014,124.469758245705)) ;
#70638=CARTESIAN_POINT('Ctrl Pts',(-19.826276696828,45.7306708940285,124.860455779892)) ;
#70639=CARTESIAN_POINT('Ctrl Pts',(-19.7428532302614,45.5506818136656,124.570733098296)) ;
#70640=CARTESIAN_POINT('Ctrl Pts',(-19.4853999049105,45.74388849653,124.927543476285)) ;
#70641=CARTESIAN_POINT('Ctrl Pts',(-19.4702042800056,45.5638994161671,124.624395485871)) ;
#70642=CARTESIAN_POINT('Ctrl Pts',(-19.0437646821752,45.7605460908078,124.897999792884)) ;
#70643=CARTESIAN_POINT('Ctrl Pts',(-19.1168393059101,45.5805570104449,124.60076273691)) ;
#70644=CARTESIAN_POINT('Ctrl Pts',(-18.5604443553513,45.7804117928495,124.685196121248)) ;
#70645=CARTESIAN_POINT('Ctrl Pts',(-18.7301974465919,45.6004227124867,124.430507595726)) ;
#70646=CARTESIAN_POINT('Ctrl Pts',(-18.240630590451,45.7970415195396,124.380241225691)) ;
#70647=CARTESIAN_POINT('Ctrl Pts',(-18.4743626408579,45.6170524391767,124.186562638723)) ;
#70648=CARTESIAN_POINT('Ctrl Pts',(-18.0589348454478,45.8103306346774,124.081934291346)) ;
#70649=CARTESIAN_POINT('Ctrl Pts',(-18.3289929495072,45.6303415543145,123.947896101221)) ;
#70650=CARTESIAN_POINT('Ctrl Pts',(-17.9633418369383,45.8202949816545,123.838171148512)) ;
#70651=CARTESIAN_POINT('Ctrl Pts',(-18.2525232679131,45.6403059012916,123.752891352259)) ;
#70652=CARTESIAN_POINT('Ctrl Pts',(-17.9115389081574,45.830223349656,123.582470100099)) ;
#70653=CARTESIAN_POINT('Ctrl Pts',(-18.2110838276306,45.6502342692931,123.548318177483)) ;
#70654=CARTESIAN_POINT('Ctrl Pts',(-17.9020047414413,45.8435067827447,123.233481404821)) ;
#70655=CARTESIAN_POINT('Ctrl Pts',(-18.2034517092472,45.6635177023819,123.269181304791)) ;
#70656=CARTESIAN_POINT('Ctrl Pts',(-18.0050894429486,45.8601588604851,122.80309786385)) ;
#70657=CARTESIAN_POINT('Ctrl Pts',(-18.2859374204291,45.6801697801222,122.924806771228)) ;
#70658=CARTESIAN_POINT('Ctrl Pts',(-18.2472042450846,45.8767102297859,122.435821289861)) ;
#70659=CARTESIAN_POINT('Ctrl Pts',(-18.4796083339964,45.696721149423,122.631034810004)) ;
#70660=CARTESIAN_POINT('Ctrl Pts',(-18.5078328375495,45.8899976579349,122.203411111269)) ;
#70661=CARTESIAN_POINT('Ctrl Pts',(-18.6881326846269,45.710008577572,122.445080306261)) ;
#70662=CARTESIAN_POINT('Ctrl Pts',(-18.7324749007102,45.900042197635,122.064839904029)) ;
#70663=CARTESIAN_POINT('Ctrl Pts',(-18.8678435288482,45.7200531172721,122.334231042964)) ;
#70664=CARTESIAN_POINT('Ctrl Pts',(-18.9727512214166,45.9098850394588,121.969029204104)) ;
#70665=CARTESIAN_POINT('Ctrl Pts',(-19.0600665012445,45.7298959590959,122.257583020281)) ;
#70666=CARTESIAN_POINT('Ctrl Pts',(-19.2294892302823,45.9198693237057,121.91505230479)) ;
#70667=CARTESIAN_POINT('Ctrl Pts',(-19.2654570275077,45.7398802433429,122.214404142504)) ;
#70668=CARTESIAN_POINT('Ctrl Pts',(-19.4908293876516,45.9298189691049,121.906556619496)) ;
#70669=CARTESIAN_POINT('Ctrl Pts',(-19.4745292486748,45.749829888742,122.207609741249)) ;
#70670=CARTESIAN_POINT('Ctrl Pts',(-19.7510268140243,45.9398187307933,121.943434488528)) ;
#70671=CARTESIAN_POINT('Ctrl Pts',(-19.6826867913636,45.7598296504304,122.23711429284)) ;
#70672=CARTESIAN_POINT('Ctrl Pts',(-20.0015055166855,45.9498500767522,122.02559641534)) ;
#70673=CARTESIAN_POINT('Ctrl Pts',(-19.8830690113146,45.7698609963893,122.302845959369)) ;
#70674=CARTESIAN_POINT('Ctrl Pts',(-20.230012990869,45.9597050312293,122.147483174595)) ;
#70675=CARTESIAN_POINT('Ctrl Pts',(-20.0658738423898,45.7797159508665,122.400357316511)) ;
#70676=CARTESIAN_POINT('Ctrl Pts',(-20.4366698390954,45.9696775692299,122.308599139529)) ;
#70677=CARTESIAN_POINT('Ctrl Pts',(-20.2311978645646,45.789688488867,122.529251805209)) ;
#70678=CARTESIAN_POINT('Ctrl Pts',(-20.6126387229705,45.9796725629648,122.503651259972)) ;
#70679=CARTESIAN_POINT('Ctrl Pts',(-20.3719712626983,45.7996834826019,122.685294957718)) ;
#70680=CARTESIAN_POINT('Ctrl Pts',(-20.7523044634586,45.9897066217589,122.727282847818)) ;
#70681=CARTESIAN_POINT('Ctrl Pts',(-20.4837019244027,45.809717541396,122.86420139806)) ;
#70682=CARTESIAN_POINT('Ctrl Pts',(-20.8496612407523,45.9995619645819,122.967303410869)) ;
#70683=CARTESIAN_POINT('Ctrl Pts',(-20.5615851977692,45.819572884219,123.056218516308)) ;
#70684=CARTESIAN_POINT('Ctrl Pts',(-20.9049869101856,46.0095614439275,123.224140951696)) ;
#70685=CARTESIAN_POINT('Ctrl Pts',(-20.6058435342198,45.8295723635646,123.261688948786)) ;
#70686=CARTESIAN_POINT('Ctrl Pts',(-20.9150723248034,46.0194558926828,123.484010185289)) ;
#70687=CARTESIAN_POINT('Ctrl Pts',(-20.6139096475916,45.8394668123199,123.469584210841)) ;
#70688=CARTESIAN_POINT('Ctrl Pts',(-20.8792184641045,46.0295190121173,123.745970407933)) ;
#70689=CARTESIAN_POINT('Ctrl Pts',(-20.5852243537012,45.8495299317544,123.67915211632)) ;
#70690=CARTESIAN_POINT('Ctrl Pts',(-20.8004631964166,46.0393586573585,123.992305910844)) ;
#70691=CARTESIAN_POINT('Ctrl Pts',(-20.5222181446683,45.8593695769957,123.876219533294)) ;
#70692=CARTESIAN_POINT('Ctrl Pts',(-20.6777341782391,46.0494218215446,124.226510235197)) ;
#70693=CARTESIAN_POINT('Ctrl Pts',(-20.4240329804487,45.8694327411817,124.063582012675)) ;
#70694=CARTESIAN_POINT('Ctrl Pts',(-20.5187010120317,46.0593160912934,124.432251752361)) ;
#70695=CARTESIAN_POINT('Ctrl Pts',(-20.2968048726953,45.8793270109305,124.228173673899)) ;
#70696=CARTESIAN_POINT('Ctrl Pts',(-20.3259612493778,46.0692578173072,124.608573010416)) ;
#70697=CARTESIAN_POINT('Ctrl Pts',(-20.1426117715884,45.8892687369444,124.369228956089)) ;
#70698=CARTESIAN_POINT('Ctrl Pts',(-20.1041752620859,46.0792607059666,124.749748717296)) ;
#70699=CARTESIAN_POINT('Ctrl Pts',(-19.965181898146,45.8992716256037,124.48216768824)) ;
#70700=CARTESIAN_POINT('Ctrl Pts',(-19.8602243413917,46.0893005547606,124.850170623594)) ;
#70701=CARTESIAN_POINT('Ctrl Pts',(-19.770020308728,45.9093114743977,124.562503212813)) ;
#70702=CARTESIAN_POINT('Ctrl Pts',(-19.6081586045614,46.0991247702215,124.906078173757)) ;
#70703=CARTESIAN_POINT('Ctrl Pts',(-19.5683677549541,45.9191356898586,124.607227074532)) ;
#70704=CARTESIAN_POINT('Ctrl Pts',(-19.3441646598656,46.109181613715,124.918003343611)) ;
#70705=CARTESIAN_POINT('Ctrl Pts',(-19.3571724382085,45.9291925333521,124.616765131644)) ;
#70706=CARTESIAN_POINT('Ctrl Pts',(-19.0854647176779,46.119110223111,124.883999596897)) ;
#70707=CARTESIAN_POINT('Ctrl Pts',(-19.150213020904,45.9391211427481,124.589560066791)) ;
#70708=CARTESIAN_POINT('Ctrl Pts',(-18.8357963857665,46.1290621071489,124.806111234111)) ;
#70709=CARTESIAN_POINT('Ctrl Pts',(-18.9504791821078,45.949073026786,124.527247495769)) ;
#70710=CARTESIAN_POINT('Ctrl Pts',(-18.6013290923237,46.1391150599565,124.684426223968)) ;
#70711=CARTESIAN_POINT('Ctrl Pts',(-18.7629062354974,45.9591259795936,124.429897589284)) ;
#70712=CARTESIAN_POINT('Ctrl Pts',(-18.3960311454174,46.1489379364227,124.527912441961)) ;
#70713=CARTESIAN_POINT('Ctrl Pts',(-18.5986696124886,45.9689488560598,124.304685323724)) ;
#70714=CARTESIAN_POINT('Ctrl Pts',(-18.2165638688177,46.1589936689928,124.333973843009)) ;
#70715=CARTESIAN_POINT('Ctrl Pts',(-18.455097186173,45.9790045886299,124.149533032839)) ;
#70716=CARTESIAN_POINT('Ctrl Pts',(-18.0755063145666,46.1689344339805,124.114086515428)) ;
#70717=CARTESIAN_POINT('Ctrl Pts',(-18.3422530053555,45.9889453536176,123.973622294175)) ;
#70718=CARTESIAN_POINT('Ctrl Pts',(-17.9743911402895,46.1788387668861,123.874249737998)) ;
#70719=CARTESIAN_POINT('Ctrl Pts',(-18.2613628144267,45.9988496865232,123.781752514046)) ;
#70720=CARTESIAN_POINT('Ctrl Pts',(-17.9157922099519,46.1888854357668,123.616841983496)) ;
#70721=CARTESIAN_POINT('Ctrl Pts',(-18.2144855602764,46.0088963554039,123.575825794976)) ;
#70722=CARTESIAN_POINT('Ctrl Pts',(-17.9027335515217,46.1987809990726,123.357082770937)) ;
#70723=CARTESIAN_POINT('Ctrl Pts',(-18.2040405772589,46.0187919187097,123.368018794538)) ;
#70724=CARTESIAN_POINT('Ctrl Pts',(-17.9355083348723,46.2088430567729,123.094739738878)) ;
#70725=CARTESIAN_POINT('Ctrl Pts',(-18.2302623332334,46.02885397641,123.158144462417)) ;
#70726=CARTESIAN_POINT('Ctrl Pts',(-18.0115191596736,46.2186858344004,122.847471415839)) ;
#70727=CARTESIAN_POINT('Ctrl Pts',(-18.2910726074192,46.0386967540375,122.960331026345)) ;
#70728=CARTESIAN_POINT('Ctrl Pts',(-18.1304936326855,46.2286763126523,122.613475678947)) ;
#70729=CARTESIAN_POINT('Ctrl Pts',(-18.3862537375702,46.0486872322894,122.773135382181)) ;
#70730=CARTESIAN_POINT('Ctrl Pts',(-18.2873793152529,46.2386052852958,122.404966075839)) ;
#70731=CARTESIAN_POINT('Ctrl Pts',(-18.5117634954812,46.0586162049329,122.60632910476)) ;
#70732=CARTESIAN_POINT('Ctrl Pts',(-18.4789900283898,46.2485964221754,122.225460708948)) ;
#70733=CARTESIAN_POINT('Ctrl Pts',(-18.6650531643566,46.0686073418125,122.462726177038)) ;
#70734=CARTESIAN_POINT('Ctrl Pts',(-18.6997158872876,46.2586185396643,122.081771774985)) ;
#70735=CARTESIAN_POINT('Ctrl Pts',(-18.8416348469598,46.0786294593014,122.347776532043)) ;
#70736=CARTESIAN_POINT('Ctrl Pts',(-18.9390004515799,46.2685190500665,121.97961691748)) ;
#70737=CARTESIAN_POINT('Ctrl Pts',(-19.0330627062083,46.0885299697036,122.266054470778)) ;
#70738=CARTESIAN_POINT('Ctrl Pts',(-19.1945546489749,46.2785080428126,121.919635191703)) ;
#70739=CARTESIAN_POINT('Ctrl Pts',(-19.2375063079573,46.0985189624497,122.218070771051)) ;
#70740=CARTESIAN_POINT('Ctrl Pts',(-19.4560195398829,46.2884732868632,121.905154403475)) ;
#70741=CARTESIAN_POINT('Ctrl Pts',(-19.4466780569291,46.1084842065003,122.206487877725)) ;
#70742=CARTESIAN_POINT('Ctrl Pts',(-19.7145391120576,46.2983775513764,121.93549611882)) ;
#70743=CARTESIAN_POINT('Ctrl Pts',(-19.653492980395,46.1183884710135,122.230762786779)) ;
#70744=CARTESIAN_POINT('Ctrl Pts',(-19.9676465193919,46.3084356430746,122.011573715253)) ;
#70745=CARTESIAN_POINT('Ctrl Pts',(-19.8559786088564,46.1284465627118,122.291626492136)) ;
#70746=CARTESIAN_POINT('Ctrl Pts',(-20.1989353902242,46.318285583503,122.127826794879)) ;
#70747=CARTESIAN_POINT('Ctrl Pts',(-20.0410082397393,46.1382965031402,122.384630018431)) ;
#70748=CARTESIAN_POINT('Ctrl Pts',(-20.4106296400589,46.3283125946766,122.284718430549)) ;
#70749=CARTESIAN_POINT('Ctrl Pts',(-20.2103627795123,46.1483235143137,122.510144538498)) ;
#70750=CARTESIAN_POINT('Ctrl Pts',(-20.5914073282754,46.3383411812886,122.476498822217)) ;
#70751=CARTESIAN_POINT('Ctrl Pts',(-20.3549837916193,46.1583521009257,122.663570001819)) ;
#70752=CARTESIAN_POINT('Ctrl Pts',(-20.7338884447941,46.3481863954013,122.692436981991)) ;
#70753=CARTESIAN_POINT('Ctrl Pts',(-20.4689669204349,46.1681973150384,122.836320620193)) ;
#70754=CARTESIAN_POINT('Ctrl Pts',(-20.838883297733,46.3581771435809,122.933081577216)) ;
#70755=CARTESIAN_POINT('Ctrl Pts',(-20.5529614728706,46.178188063218,123.028836705902)) ;
#70756=CARTESIAN_POINT('Ctrl Pts',(-20.9002222159883,46.3682147771664,123.1896289369)) ;
#70757=CARTESIAN_POINT('Ctrl Pts',(-20.6020311735636,46.1882256968035,123.234075045714)) ;
#70758=CARTESIAN_POINT('Ctrl Pts',(-20.9162101455242,46.3780600663792,123.447862222641)) ;
#70759=CARTESIAN_POINT('Ctrl Pts',(-20.614820050469,46.1980709860163,123.440660827507)) ;
#70760=CARTESIAN_POINT('Ctrl Pts',(-20.8872976540046,46.3880414671851,123.708544539136)) ;
#70761=CARTESIAN_POINT('Ctrl Pts',(-20.5916887966278,46.2080523868222,123.649206325939)) ;
#70762=CARTESIAN_POINT('Ctrl Pts',(-20.8137082785738,46.397993700175,123.959520057968)) ;
#70763=CARTESIAN_POINT('Ctrl Pts',(-20.5328161531047,46.2180046198121,123.849986010889)) ;
#70764=CARTESIAN_POINT('Ctrl Pts',(-20.6974169783614,46.4079925116317,124.195165716517)) ;
#70765=CARTESIAN_POINT('Ctrl Pts',(-20.4397820581274,46.2280034312688,124.038501896986)) ;
#70766=CARTESIAN_POINT('Ctrl Pts',(-20.5409623495954,46.4180316155623,124.407564420263)) ;
#70767=CARTESIAN_POINT('Ctrl Pts',(-20.3146171987756,46.2380425351995,124.208420165923)) ;
#70768=CARTESIAN_POINT('Ctrl Pts',(-20.3544390959673,46.4278565579816,124.586111387913)) ;
#70769=CARTESIAN_POINT('Ctrl Pts',(-20.1653985485672,46.2478674776188,124.351256099726)) ;
#70770=CARTESIAN_POINT('Ctrl Pts',(-20.134995919871,46.4379112454576,124.733256870576)) ;
#70771=CARTESIAN_POINT('Ctrl Pts',(-19.9898432095306,46.2579221650947,124.468971664984)) ;
#70772=CARTESIAN_POINT('Ctrl Pts',(-19.8958234362632,46.4478540478144,124.838477290274)) ;
#70773=CARTESIAN_POINT('Ctrl Pts',(-19.7985051353793,46.2678649674515,124.553146698639)) ;
#70774=CARTESIAN_POINT('Ctrl Pts',(-19.6432030628621,46.4577578437542,124.901101950844)) ;
#70775=CARTESIAN_POINT('Ctrl Pts',(-19.5964092448346,46.2777687633913,124.603245250316)) ;
#70776=CARTESIAN_POINT('Ctrl Pts',(-19.3798141419767,46.4678046231292,124.919009575157)) ;
#70777=CARTESIAN_POINT('Ctrl Pts',(-19.3856978663707,46.2878155427663,124.61757028202)) ;
#70778=CARTESIAN_POINT('Ctrl Pts',(-19.1211811679258,46.4777002814238,124.891553789188)) ;
#70779=CARTESIAN_POINT('Ctrl Pts',(-19.1787923210989,46.2977112010609,124.595604707242)) ;
#70780=CARTESIAN_POINT('Ctrl Pts',(-18.8671103311317,46.4877618486744,124.818449852984)) ;
#70781=CARTESIAN_POINT('Ctrl Pts',(-18.9755356841084,46.3077727683115,124.537120502504)) ;
#70782=CARTESIAN_POINT('Ctrl Pts',(-18.6346615958398,46.4976064931117,124.704865605345)) ;
#70783=CARTESIAN_POINT('Ctrl Pts',(-18.7895780913401,46.3176174127489,124.446252657151)) ;
#70784=CARTESIAN_POINT('Ctrl Pts',(-18.4224718070244,46.5075665393544,124.551629282646)) ;
#70785=CARTESIAN_POINT('Ctrl Pts',(-18.6198270211866,46.3275774589915,124.32366317014)) ;
#70786=CARTESIAN_POINT('Ctrl Pts',(-18.2390573894743,46.5176048353728,124.362048863107)) ;
#70787=CARTESIAN_POINT('Ctrl Pts',(-18.4730960549805,46.3376157550099,124.171998104319)) ;
#70788=CARTESIAN_POINT('Ctrl Pts',(-18.0933321835797,46.5274781767911,124.147328823137)) ;
#70789=CARTESIAN_POINT('Ctrl Pts',(-18.3565170542774,46.3474890964282,124.00022237033)) ;
#70790=CARTESIAN_POINT('Ctrl Pts',(-17.9850644966569,46.5375512805904,123.905828159884)) ;
#70791=CARTESIAN_POINT('Ctrl Pts',(-18.2699035102688,46.3575622002275,123.80702119456)) ;
#70792=CARTESIAN_POINT('Ctrl Pts',(-17.9216561766812,46.5473720957093,123.655604769692)) ;
#70793=CARTESIAN_POINT('Ctrl Pts',(-18.219177873809,46.3673830153464,123.606843503252)) ;
#70794=CARTESIAN_POINT('Ctrl Pts',(-17.9018683250634,46.5574489607873,123.391584873684)) ;
#70795=CARTESIAN_POINT('Ctrl Pts',(-18.2033482278461,46.3774598804244,123.395627180007)) ;
#70796=CARTESIAN_POINT('Ctrl Pts',(-17.9277757499098,46.5673137004426,123.133615388447)) ;
#70797=CARTESIAN_POINT('Ctrl Pts',(-18.2240747548872,46.3873246200797,123.189252631798)) ;
#70798=CARTESIAN_POINT('Ctrl Pts',(-17.9985297244048,46.5773361036839,122.879929630516)) ;
#70799=CARTESIAN_POINT('Ctrl Pts',(-18.2806784477161,46.397347023321,122.98630413088)) ;
#70800=CARTESIAN_POINT('Ctrl Pts',(-18.1129004945136,46.5873618279724,122.642565399525)) ;
#70801=CARTESIAN_POINT('Ctrl Pts',(-18.3721757093272,46.4073727476095,122.796412980426)) ;
#70802=CARTESIAN_POINT('Ctrl Pts',(-18.2637366876288,46.5972166109937,122.432070963929)) ;
#70803=CARTESIAN_POINT('Ctrl Pts',(-18.4928445100312,46.4172275306308,122.628018630033)) ;
#70804=CARTESIAN_POINT('Ctrl Pts',(-18.4506972916997,46.607195454717,122.248181197861)) ;
#70805=CARTESIAN_POINT('Ctrl Pts',(-18.6424130861803,46.4272063743541,122.48090728997)) ;
#70806=CARTESIAN_POINT('Ctrl Pts',(-18.6678559884878,46.6172143469536,122.099336220667)) ;
#70807=CARTESIAN_POINT('Ctrl Pts',(-18.8161403445689,46.4372252665907,122.361831725201)) ;
#70808=CARTESIAN_POINT('Ctrl Pts',(-18.9041339832422,46.6270975559946,121.991423381431)) ;
#70809=CARTESIAN_POINT('Ctrl Pts',(-19.0051620983221,46.4471084756317,122.275502163927)) ;
#70810=CARTESIAN_POINT('Ctrl Pts',(-19.1602204279234,46.6371658653348,121.925081449906)) ;
#70811=CARTESIAN_POINT('Ctrl Pts',(-19.2100316746212,46.4571767849719,122.222428931168)) ;
#70812=CARTESIAN_POINT('Ctrl Pts',(-19.4177614318243,46.6469959906675,121.904397063364)) ;
#70813=CARTESIAN_POINT('Ctrl Pts',(-19.4160632754822,46.4670069103046,122.205881850108)) ;
#70814=CARTESIAN_POINT('Ctrl Pts',(-19.6811124793488,46.6570625430445,121.928980404509)) ;
#70815=CARTESIAN_POINT('Ctrl Pts',(-19.6267444075026,46.4770734626816,122.22554879681)) ;
#70816=CARTESIAN_POINT('Ctrl Pts',(-19.93175625164,46.6669527799382,121.997866497326)) ;
#70817=CARTESIAN_POINT('Ctrl Pts',(-19.8272585403738,46.4869636995753,122.280657725669)) ;
#70818=CARTESIAN_POINT('Ctrl Pts',(-20.1692553844016,46.6769450047322,122.109835361796)) ;
#70819=CARTESIAN_POINT('Ctrl Pts',(-20.0172576312731,46.4969559243693,122.370232872609)) ;
#70820=CARTESIAN_POINT('Ctrl Pts',(-20.3829389131417,46.6869076250832,122.261097188161)) ;
#70821=CARTESIAN_POINT('Ctrl Pts',(-20.1882040373504,46.5069185447203,122.491242289893)) ;
#70822=CARTESIAN_POINT('Ctrl Pts',(-20.5665204839457,46.6968126278463,122.445649602459)) ;
#70823=CARTESIAN_POINT('Ctrl Pts',(-20.3350687382439,46.5168235474834,122.638883718221)) ;
#70824=CARTESIAN_POINT('Ctrl Pts',(-20.7173901651887,46.7068703902444,122.662639131591)) ;
#70825=CARTESIAN_POINT('Ctrl Pts',(-20.4557645655042,46.5268813098816,122.812475613443)) ;
#70826=CARTESIAN_POINT('Ctrl Pts',(-20.8262181894773,46.7167209096232,122.89753556539)) ;
#70827=CARTESIAN_POINT('Ctrl Pts',(-20.5428264841465,46.5367318292604,123.000391752439)) ;
#70828=CARTESIAN_POINT('Ctrl Pts',(-20.8943773618054,46.7267524866214,123.15217347503)) ;
#70829=CARTESIAN_POINT('Ctrl Pts',(-20.5973539588229,46.5467634062585,123.204102140928)) ;
#70830=CARTESIAN_POINT('Ctrl Pts',(-20.9167369790523,46.7367622217263,123.414295804395)) ;
#70831=CARTESIAN_POINT('Ctrl Pts',(-20.6152416326084,46.5567731413635,123.413799972381)) ;
#70832=CARTESIAN_POINT('Ctrl Pts',(-20.8937123153054,46.7466717983526,123.673666920638)) ;
#70833=CARTESIAN_POINT('Ctrl Pts',(-20.596822009193,46.5666827179897,123.621296152954)) ;
#70834=CARTESIAN_POINT('Ctrl Pts',(-20.8265171674148,46.7565991842093,123.925758286608)) ;
#70835=CARTESIAN_POINT('Ctrl Pts',(-20.5430662495124,46.5766101038464,123.822968723922)) ;
#70836=CARTESIAN_POINT('Ctrl Pts',(-20.7150850922258,46.7666441186995,124.165042883978)) ;
#70837=CARTESIAN_POINT('Ctrl Pts',(-20.4539206594605,46.5866550383367,124.014396623228)) ;
#70838=CARTESIAN_POINT('Ctrl Pts',(-20.566303423748,46.7765300508875,124.378031588581)) ;
#70839=CARTESIAN_POINT('Ctrl Pts',(-20.3348959856929,46.5965409705246,124.184786987194)) ;
#70840=CARTESIAN_POINT('Ctrl Pts',(-20.3811494336437,46.7865233568405,124.56424680321)) ;
#70841=CARTESIAN_POINT('Ctrl Pts',(-20.1867731294926,46.6065342764777,124.333759263123)) ;
#70842=CARTESIAN_POINT('Ctrl Pts',(-20.167426750717,46.7964689946224,124.714688252167)) ;
#70843=CARTESIAN_POINT('Ctrl Pts',(-20.0157955364757,46.6164799142595,124.454112381368)) ;
#70844=CARTESIAN_POINT('Ctrl Pts',(-19.9310071201226,46.8064162629683,124.826243396208)) ;
#70845=CARTESIAN_POINT('Ctrl Pts',(-19.8266604269535,46.6264271826054,124.543356680596)) ;
#70846=CARTESIAN_POINT('Ctrl Pts',(-19.6762006528589,46.8164641651054,124.895457669008)) ;
#70847=CARTESIAN_POINT('Ctrl Pts',(-19.6228151502625,46.6364750847425,124.598728484168)) ;
#70848=CARTESIAN_POINT('Ctrl Pts',(-19.4184961828357,46.8263118599456,124.91911890289)) ;
#70849=CARTESIAN_POINT('Ctrl Pts',(-19.4166527254704,46.6463227795827,124.617657767164)) ;
#70850=CARTESIAN_POINT('Ctrl Pts',(-19.1575612607115,46.83627336969,124.898251094209)) ;
#70851=CARTESIAN_POINT('Ctrl Pts',(-19.2079051028574,46.6562842893271,124.600964154411)) ;
#70852=CARTESIAN_POINT('Ctrl Pts',(-18.902556312997,46.8463027612989,124.831598304346)) ;
#70853=CARTESIAN_POINT('Ctrl Pts',(-19.0039009355955,46.666313680936,124.54764240293)) ;
#70854=CARTESIAN_POINT('Ctrl Pts',(-18.6658571373904,46.8562102568536,124.723148671996)) ;
#70855=CARTESIAN_POINT('Ctrl Pts',(-18.8145420155273,46.6762211764908,124.460883498429)) ;
#70856=CARTESIAN_POINT('Ctrl Pts',(-18.4504873824993,46.8661556485166,124.575124657286)) ;
#70857=CARTESIAN_POINT('Ctrl Pts',(-18.6422462094197,46.6861665681538,124.342465111585)) ;
#70858=CARTESIAN_POINT('Ctrl Pts',(-18.262882041295,46.876157566114,124.390984128)) ;
#70859=CARTESIAN_POINT('Ctrl Pts',(-18.4921615041804,46.6961684857511,124.195153273134)) ;
#70860=CARTESIAN_POINT('Ctrl Pts',(-18.1099479381027,46.8861976336662,124.176016249327)) ;
#70861=CARTESIAN_POINT('Ctrl Pts',(-18.3698136515618,46.7062085533033,124.023179206255)) ;
#70862=CARTESIAN_POINT('Ctrl Pts',(-17.998547175216,46.896021945106,123.943090129844)) ;
#70863=CARTESIAN_POINT('Ctrl Pts',(-18.280692897445,46.7160328647431,123.836839731432)) ;
#70864=CARTESIAN_POINT('Ctrl Pts',(-17.9273097685191,46.9060781862621,123.688632681324)) ;
#70865=CARTESIAN_POINT('Ctrl Pts',(-18.2237021026595,46.7260891058992,123.633273756565)) ;
#70866=CARTESIAN_POINT('Ctrl Pts',(-17.9019600484687,46.9160091079977,123.4288626675)) ;
#70867=CARTESIAN_POINT('Ctrl Pts',(-18.2034216287563,46.7360200276349,123.425458357104)) ;
#70868=CARTESIAN_POINT('Ctrl Pts',(-17.9215882488076,46.925952344074,123.168336310537)) ;
#70869=CARTESIAN_POINT('Ctrl Pts',(-18.2191232721713,46.7459632637111,123.217037686628)) ;
#70870=CARTESIAN_POINT('Ctrl Pts',(-17.9861745623724,46.9359336280864,122.914073624315)) ;
#70871=CARTESIAN_POINT('Ctrl Pts',(-18.2707913566683,46.7559445477236,123.01362751071)) ;
#70872=CARTESIAN_POINT('Ctrl Pts',(-18.0949933336756,46.9459779297121,122.673631325158)) ;
#70873=CARTESIAN_POINT('Ctrl Pts',(-18.3578456757999,46.7659888493492,122.821273187654)) ;
#70874=CARTESIAN_POINT('Ctrl Pts',(-18.2402478329783,46.9558060109315,122.460027367171)) ;
#70875=CARTESIAN_POINT('Ctrl Pts',(-18.474047818082,46.7758169305687,122.650390426094)) ;
#70876=CARTESIAN_POINT('Ctrl Pts',(-18.4247793331419,46.9658826137807,122.270186990604)) ;
#70877=CARTESIAN_POINT('Ctrl Pts',(-18.6216725361831,46.7858935334178,122.498517174402)) ;
#70878=CARTESIAN_POINT('Ctrl Pts',(-18.6347009617729,46.9757346928992,122.118553078034)) ;
#70879=CARTESIAN_POINT('Ctrl Pts',(-18.789608433041,46.7957456125364,122.377209782781)) ;
#70880=CARTESIAN_POINT('Ctrl Pts',(-18.8728048873028,46.9858079512082,122.002979006205)) ;
#70881=CARTESIAN_POINT('Ctrl Pts',(-18.9800913870549,46.8058188708453,122.28474940667)) ;
#70882=CARTESIAN_POINT('Ctrl Pts',(-19.1215801045156,46.9956494105884,121.93222329205)) ;
#70883=CARTESIAN_POINT('Ctrl Pts',(-19.1791102655951,46.8156603302256,122.228144091495)) ;
#70884=CARTESIAN_POINT('Ctrl Pts',(-19.381859343394,47.0056105060008,121.904442012515)) ;
#70885=CARTESIAN_POINT('Ctrl Pts',(-19.3873331982892,46.8256214256379,122.205917820199)) ;
#70886=CARTESIAN_POINT('Ctrl Pts',(-19.6449738782894,47.0156477903975,121.922928491226)) ;
#70887=CARTESIAN_POINT('Ctrl Pts',(-19.5978250114014,46.8356587100347,122.220705838776)) ;
#70888=CARTESIAN_POINT('Ctrl Pts',(-19.8969217299239,47.0255241291328,121.985363214302)) ;
#70889=CARTESIAN_POINT('Ctrl Pts',(-19.7993828256105,46.8455350487699,122.270652190592)) ;
#70890=CARTESIAN_POINT('Ctrl Pts',(-20.1386279884017,47.0355862552861,122.092504779786)) ;
#70891=CARTESIAN_POINT('Ctrl Pts',(-19.9927485620531,46.8555971749232,122.356364359904)) ;
#70892=CARTESIAN_POINT('Ctrl Pts',(-20.3539188130597,47.0454544292626,122.237128270037)) ;
#70893=CARTESIAN_POINT('Ctrl Pts',(-20.1649812567676,46.8654653488997,122.472061612692)) ;
#70894=CARTESIAN_POINT('Ctrl Pts',(-20.5437493740665,47.0554599777664,122.419010050859)) ;
#70895=CARTESIAN_POINT('Ctrl Pts',(-20.3168466298338,46.8754708974035,122.617565974457)) ;
#70896=CARTESIAN_POINT('Ctrl Pts',(-20.6987362985448,47.065442609662,122.630724270001)) ;
#70897=CARTESIAN_POINT('Ctrl Pts',(-20.440837183443,46.8854535292991,122.786936385641)) ;
#70898=CARTESIAN_POINT('Ctrl Pts',(-20.8150425909332,47.0754865520838,122.867637130232)) ;
#70899=CARTESIAN_POINT('Ctrl Pts',(-20.5338834673555,46.8954974717209,122.976466203145)) ;
#70900=CARTESIAN_POINT('Ctrl Pts',(-20.8872078791894,47.0853147001109,123.115624213289)) ;
#70901=CARTESIAN_POINT('Ctrl Pts',(-20.5916167561873,46.9053256197481,123.174854489363)) ;
#70902=CARTESIAN_POINT('Ctrl Pts',(-20.9165166534759,47.0953045674853,123.37650718992)) ;
#70903=CARTESIAN_POINT('Ctrl Pts',(-20.6150653220902,46.9153154871225,123.383560557976)) ;
#70904=CARTESIAN_POINT('Ctrl Pts',(-20.8993091493922,47.1053483064408,123.639884268201)) ;
#70905=CARTESIAN_POINT('Ctrl Pts',(-20.6013007427833,46.925359226078,123.594262430873)) ;
#70906=CARTESIAN_POINT('Ctrl Pts',(-20.8385403650369,47.1151700549788,123.890732974447)) ;
#70907=CARTESIAN_POINT('Ctrl Pts',(-20.5526874481851,46.9351809746159,123.794940790409)) ;
#70908=CARTESIAN_POINT('Ctrl Pts',(-20.7334869965978,47.1252050325885,124.132613019297)) ;
#70909=CARTESIAN_POINT('Ctrl Pts',(-20.4686462451259,46.9452159522256,123.988445566052)) ;
#70910=CARTESIAN_POINT('Ctrl Pts',(-20.5875612969449,47.1352299453462,124.351957946675)) ;
#70911=CARTESIAN_POINT('Ctrl Pts',(-20.3519069440029,46.9552408649833,124.163922368766)) ;
#70912=CARTESIAN_POINT('Ctrl Pts',(-20.4093144805832,47.14508188844,124.539733165987)) ;
#70913=CARTESIAN_POINT('Ctrl Pts',(-20.209311228941,46.9650928080772,124.314143082127)) ;
#70914=CARTESIAN_POINT('Ctrl Pts',(-20.1985036701278,47.1550728497691,124.69617951058)) ;
#70915=CARTESIAN_POINT('Ctrl Pts',(-20.0406637063053,46.9750837694063,124.439301445059)) ;
#70916=CARTESIAN_POINT('Ctrl Pts',(-19.9654674976531,47.1649907246376,124.812968953075)) ;
#70917=CARTESIAN_POINT('Ctrl Pts',(-19.8542359521288,46.9850016442747,124.532734341221)) ;
#70918=CARTESIAN_POINT('Ctrl Pts',(-19.71297510293,47.1750192436388,124.88839013585)) ;
#70919=CARTESIAN_POINT('Ctrl Pts',(-19.652242507693,46.9950301632759,124.593072964507)) ;
#70920=CARTESIAN_POINT('Ctrl Pts',(-19.4549854354218,47.1849029224366,124.918522015687)) ;
#70921=CARTESIAN_POINT('Ctrl Pts',(-19.4458515655707,47.0049138420738,124.617180149726)) ;
#70922=CARTESIAN_POINT('Ctrl Pts',(-19.1927415406444,47.1948978658764,124.903808702217)) ;
#70923=CARTESIAN_POINT('Ctrl Pts',(-19.2360564571309,47.0149087855135,124.605411359916)) ;
#70924=CARTESIAN_POINT('Ctrl Pts',(-18.9363215273581,47.2049247196988,124.843152452533)) ;
#70925=CARTESIAN_POINT('Ctrl Pts',(-19.0309200183396,47.0249356393359,124.55688809248)) ;
#70926=CARTESIAN_POINT('Ctrl Pts',(-18.6976217950589,47.2148088840377,124.740702605869)) ;
#70927=CARTESIAN_POINT('Ctrl Pts',(-18.8399600159307,47.0348198036749,124.47493012311)) ;
#70928=CARTESIAN_POINT('Ctrl Pts',(-18.4778918251213,47.2247969820801,124.597178175501)) ;
#70929=CARTESIAN_POINT('Ctrl Pts',(-18.6641751118157,47.0448079017172,124.360112235116)) ;
#70930=CARTESIAN_POINT('Ctrl Pts',(-18.2869868870465,47.2347480885372,124.418412493407)) ;
#70931=CARTESIAN_POINT('Ctrl Pts',(-18.511450049831,47.0547590081743,124.2171012666)) ;
#70932=CARTESIAN_POINT('Ctrl Pts',(-18.1286864683151,47.2447931397053,124.207190353518)) ;
#70933=CARTESIAN_POINT('Ctrl Pts',(-18.3848081587268,47.0648040593424,124.048124631986)) ;
#70934=CARTESIAN_POINT('Ctrl Pts',(-18.0115053675036,47.2546549000636,123.976037450219)) ;
#70935=CARTESIAN_POINT('Ctrl Pts',(-18.2910618397786,47.0746658197007,123.863203703224)) ;
#70936=CARTESIAN_POINT('Ctrl Pts',(-17.9346962187188,47.264617716894,123.725744078448)) ;
#70937=CARTESIAN_POINT('Ctrl Pts',(-18.2296126464617,47.0846286365312,123.662969789116)) ;
#70938=CARTESIAN_POINT('Ctrl Pts',(-17.9027315659369,47.2746523981748,123.463999492697)) ;
#70939=CARTESIAN_POINT('Ctrl Pts',(-18.2040389739103,47.0946633178119,123.453574331988)) ;
#70940=CARTESIAN_POINT('Ctrl Pts',(-17.9160504867167,47.2845374279556,123.204536864795)) ;
#70941=CARTESIAN_POINT('Ctrl Pts',(-18.214692073012,47.1045483475927,123.246004576489)) ;
#70942=CARTESIAN_POINT('Ctrl Pts',(-17.9753215326006,47.2946030213536,122.946793722897)) ;
#70943=CARTESIAN_POINT('Ctrl Pts',(-18.2621069751575,47.1146139409907,123.039809496486)) ;
#70944=CARTESIAN_POINT('Ctrl Pts',(-18.0759175402315,47.3044421897151,122.708557598471)) ;
#70945=CARTESIAN_POINT('Ctrl Pts',(-18.3425816822834,47.1244531093522,122.84922032325)) ;
#70946=CARTESIAN_POINT('Ctrl Pts',(-18.2191949884316,47.3145047874566,122.486339905974)) ;
#70947=CARTESIAN_POINT('Ctrl Pts',(-18.4572019469866,47.1345157070937,122.671444952012)) ;
#70948=CARTESIAN_POINT('Ctrl Pts',(-18.396159615514,47.3244017998635,122.295722821703)) ;
#70949=CARTESIAN_POINT('Ctrl Pts',(-18.5987718917569,47.1444127195006,122.518950162102)) ;
#70950=CARTESIAN_POINT('Ctrl Pts',(-18.6037098264549,47.3343331216891,122.137504758704)) ;
#70951=CARTESIAN_POINT('Ctrl Pts',(-18.7648105710639,47.1543440413262,122.392374154288)) ;
#70952=CARTESIAN_POINT('Ctrl Pts',(-18.8382907890392,47.3443748844436,122.016648795488)) ;
#70953=CARTESIAN_POINT('Ctrl Pts',(-18.9524743954627,47.1643858040807,122.295687495838)) ;
#70954=CARTESIAN_POINT('Ctrl Pts',(-19.0864023365642,47.3542630833343,121.939374027969)) ;
#70955=CARTESIAN_POINT('Ctrl Pts',(-19.1509626756622,47.1742740029714,122.233865749171)) ;
#70956=CARTESIAN_POINT('Ctrl Pts',(-19.3468297085847,47.3642570219342,121.905591956175)) ;
#70957=CARTESIAN_POINT('Ctrl Pts',(-19.3593042135663,47.1842679415713,122.206837953697)) ;
#70958=CARTESIAN_POINT('Ctrl Pts',(-19.6078094898697,47.374197842971,121.917497147633)) ;
#70959=CARTESIAN_POINT('Ctrl Pts',(-19.568087947677,47.1942087626082,122.216359938901)) ;
#70960=CARTESIAN_POINT('Ctrl Pts',(-19.8632760200849,47.3841572252593,121.974310927408)) ;
#70961=CARTESIAN_POINT('Ctrl Pts',(-19.772461509312,47.2041681448964,122.261808795976)) ;
#70962=CARTESIAN_POINT('Ctrl Pts',(-20.1060266518377,47.3941549849116,122.074874782439)) ;
#70963=CARTESIAN_POINT('Ctrl Pts',(-19.966662791665,47.2141659045487,122.342257824521)) ;
#70964=CARTESIAN_POINT('Ctrl Pts',(-20.3282563986287,47.4041911211139,122.216891398893)) ;
#70965=CARTESIAN_POINT('Ctrl Pts',(-20.1444477453573,47.224202040751,122.455869277174)) ;
#70966=CARTESIAN_POINT('Ctrl Pts',(-20.5190751999569,47.4140419186048,122.391820347718)) ;
#70967=CARTESIAN_POINT('Ctrl Pts',(-20.2971040399441,47.2340528382419,122.595810607946)) ;
#70968=CARTESIAN_POINT('Ctrl Pts',(-20.6789956607079,47.4240027836811,122.599038839022)) ;
#70969=CARTESIAN_POINT('Ctrl Pts',(-20.4250421187195,47.2440137033182,122.76158395382)) ;
#70970=CARTESIAN_POINT('Ctrl Pts',(-20.8010651623618,47.4340316513115,122.832629226849)) ;
#70971=CARTESIAN_POINT('Ctrl Pts',(-20.5226996700031,47.2540425709486,122.948455205887)) ;
#70972=CARTESIAN_POINT('Ctrl Pts',(-20.8798481803655,47.4439418874479,123.080846336945)) ;
#70973=CARTESIAN_POINT('Ctrl Pts',(-20.5857281550626,47.263952807085,123.147028060503)) ;
#70974=CARTESIAN_POINT('Ctrl Pts',(-20.9151022554273,47.4538768407624,123.339542816455)) ;
#70975=CARTESIAN_POINT('Ctrl Pts',(-20.6139336294218,47.2738877603996,123.353984836361)) ;
#70976=CARTESIAN_POINT('Ctrl Pts',(-20.9045535939109,47.463917771172,123.603190649991)) ;
#70977=CARTESIAN_POINT('Ctrl Pts',(-20.605496940888,47.2839286908091,123.564903155438)) ;
#70978=CARTESIAN_POINT('Ctrl Pts',(-20.849402115707,47.4738056679536,123.857124325427)) ;
#70979=CARTESIAN_POINT('Ctrl Pts',(-20.5613779800688,47.2938165875907,123.768050447587)) ;
#70980=CARTESIAN_POINT('Ctrl Pts',(-20.750444918412,47.4837951196123,124.1002641636)) ;
#70981=CARTESIAN_POINT('Ctrl Pts',(-20.4822143310711,47.3038060392494,123.962563117497)) ;
#70982=CARTESIAN_POINT('Ctrl Pts',(-20.6110220669267,47.4937542099777,124.321740017003)) ;
#70983=CARTESIAN_POINT('Ctrl Pts',(-20.3706779971095,47.3137651296148,124.13974493574)) ;
#70984=CARTESIAN_POINT('Ctrl Pts',(-20.4368281965108,47.503651522284,124.514904688104)) ;
#70985=CARTESIAN_POINT('Ctrl Pts',(-20.2313246021344,47.3236624419211,124.294278151825)) ;
#70986=CARTESIAN_POINT('Ctrl Pts',(-20.2283967744204,47.5137079481842,124.677338457595)) ;
#70987=CARTESIAN_POINT('Ctrl Pts',(-20.064580902708,47.3337188678213,124.424226901582)) ;
#70988=CARTESIAN_POINT('Ctrl Pts',(-19.9992773799533,47.523577950774,124.798958001509)) ;
#70989=CARTESIAN_POINT('Ctrl Pts',(-19.8812864635495,47.3435888704111,124.521524526354)) ;
#70990=CARTESIAN_POINT('Ctrl Pts',(-19.7493845402161,47.5335818839512,124.880515352736)) ;
#70991=CARTESIAN_POINT('Ctrl Pts',(-19.6813728797849,47.3535928035883,124.586772510695)) ;
#70992=CARTESIAN_POINT('Ctrl Pts',(-19.4894723640348,47.5435691444151,124.917254732859)) ;
#70993=CARTESIAN_POINT('Ctrl Pts',(-19.4734436940258,47.3635800640522,124.616166289918)) ;
#70994=CARTESIAN_POINT('Ctrl Pts',(-19.2261503135035,47.5535961960008,124.908119289949)) ;
#70995=CARTESIAN_POINT('Ctrl Pts',(-19.2627853251842,47.3736071156379,124.608859963816)) ;
#70996=CARTESIAN_POINT('Ctrl Pts',(-18.9718149570964,47.5634872858269,124.854385043497)) ;
#70997=CARTESIAN_POINT('Ctrl Pts',(-19.0593192486441,47.383498205464,124.565875589659)) ;
#70998=CARTESIAN_POINT('Ctrl Pts',(-18.6475331408761,47.576785040608,124.724300286802)) ;
#70999=CARTESIAN_POINT('Ctrl Pts',(-18.7998792298712,47.3967959602451,124.461806395647)) ;
#71000=CARTESIAN_POINT('Ctrl Pts',(-18.3663382799237,47.5899831002161,124.51451143139)) ;
#71001=CARTESIAN_POINT('Ctrl Pts',(-18.5749054443382,47.4099940198532,124.29395298759)) ;
#71002=CARTESIAN_POINT('Ctrl Pts',(-18.1483991888473,47.6033798407853,124.238054641967)) ;
#71003=CARTESIAN_POINT('Ctrl Pts',(-18.4005844644017,47.4233907604224,124.072822927662)) ;
#71004=CARTESIAN_POINT('Ctrl Pts',(-18.025347143704,47.6132507528587,124.009644853001)) ;
#71005=CARTESIAN_POINT('Ctrl Pts',(-18.3021342785884,47.4332616724959,123.890089214301)) ;
#71006=CARTESIAN_POINT('Ctrl Pts',(-17.9421929511721,47.6233243146269,123.758382877817)) ;
#71007=CARTESIAN_POINT('Ctrl Pts',(-18.2356106624253,47.443335234264,123.689082422527)) ;
#71008=CARTESIAN_POINT('Ctrl Pts',(-17.9045616883877,47.6331457272152,123.502983370987)) ;
#71009=CARTESIAN_POINT('Ctrl Pts',(-18.2055029686415,47.4531566468523,123.484761871704)) ;
#71010=CARTESIAN_POINT('Ctrl Pts',(-17.911781843042,47.6432197444462,123.238412336144)) ;
#71011=CARTESIAN_POINT('Ctrl Pts',(-18.2112771669349,47.4632306640834,123.273106890456)) ;
#71012=CARTESIAN_POINT('Ctrl Pts',(-17.9808569614933,47.6563785314108,122.899509564629)) ;
#71013=CARTESIAN_POINT('Ctrl Pts',(-18.2665340443339,47.4763894510479,123.001975913631)) ;
#71014=CARTESIAN_POINT('Ctrl Pts',(-18.1386436633673,47.669744634505,122.581350825213)) ;
#71015=CARTESIAN_POINT('Ctrl Pts',(-18.3927847615618,47.4897555541421,122.74742093734)) ;
#71016=CARTESIAN_POINT('Ctrl Pts',(-18.370652315842,47.683058569394,122.319320691079)) ;
#71017=CARTESIAN_POINT('Ctrl Pts',(-18.5783616726508,47.5030694890312,122.537834646464)) ;
#71018=CARTESIAN_POINT('Ctrl Pts',(-18.5739282398627,47.6929586088415,122.157012936139)) ;
#71019=CARTESIAN_POINT('Ctrl Pts',(-18.7409870352096,47.5129695284786,122.407978673393)) ;
#71020=CARTESIAN_POINT('Ctrl Pts',(-18.8036181717246,47.702923011976,122.031241515346)) ;
#71021=CARTESIAN_POINT('Ctrl Pts',(-18.9247363827808,47.5229339316132,122.307361838149)) ;
#71022=CARTESIAN_POINT('Ctrl Pts',(-19.0533535758895,47.7129529790972,121.946938831321)) ;
#71023=CARTESIAN_POINT('Ctrl Pts',(-19.1245251698578,47.5329638987343,122.239917409977)) ;
#71024=CARTESIAN_POINT('Ctrl Pts',(-19.3105838879911,47.7228552557062,121.907675661922)) ;
#71025=CARTESIAN_POINT('Ctrl Pts',(-19.3303061564412,47.5428661753434,122.208504383687)) ;
#71026=CARTESIAN_POINT('Ctrl Pts',(-19.6591650885652,47.7361211848754,121.914819682812)) ;
#71027=CARTESIAN_POINT('Ctrl Pts',(-19.609187461542,47.5561321045125,122.214219997551)) ;
#71028=CARTESIAN_POINT('Ctrl Pts',(-20.0833550247634,47.7527427159818,122.037930509702)) ;
#71029=CARTESIAN_POINT('Ctrl Pts',(-19.9485240134624,47.5727536356189,122.312705495618)) ;
#71030=CARTESIAN_POINT('Ctrl Pts',(-20.510453729545,47.7726175446265,122.348898697034)) ;
#71031=CARTESIAN_POINT('Ctrl Pts',(-20.2902038142842,47.5926284642636,122.561462978366)) ;
#71032=CARTESIAN_POINT('Ctrl Pts',(-20.7582479358267,47.7892907527283,122.71623189636)) ;
#71033=CARTESIAN_POINT('Ctrl Pts',(-20.4884640703777,47.6093016723655,122.855376229388)) ;
#71034=CARTESIAN_POINT('Ctrl Pts',(-20.8714295868913,47.8025418777096,123.04557591284)) ;
#71035=CARTESIAN_POINT('Ctrl Pts',(-20.5789911114765,47.6225527973467,123.118807090608)) ;
#71036=CARTESIAN_POINT('Ctrl Pts',(-20.9269298434521,47.8157841965304,123.389178316211)) ;
#71037=CARTESIAN_POINT('Ctrl Pts',(-20.6233964746189,47.6357951161676,123.393706836067)) ;
#71038=CARTESIAN_POINT('Ctrl Pts',(-20.881145520325,47.8325174368699,123.831476120658)) ;
#71039=CARTESIAN_POINT('Ctrl Pts',(-20.5867718080052,47.652528356507,123.747531615695)) ;
#71040=CARTESIAN_POINT('Ctrl Pts',(-20.6511822086368,47.8523465850579,124.305796219641)) ;
#71041=CARTESIAN_POINT('Ctrl Pts',(-20.4028036328943,47.672357504695,124.126994379831)) ;
#71042=CARTESIAN_POINT('Ctrl Pts',(-20.2723934902227,47.8722712801585,124.675711001554)) ;
#71043=CARTESIAN_POINT('Ctrl Pts',(-20.0997742015209,47.6922821997956,124.422927479501)) ;
#71044=CARTESIAN_POINT('Ctrl Pts',(-19.7899432576281,47.8921945087419,124.89417687357)) ;
#71045=CARTESIAN_POINT('Ctrl Pts',(-19.7138146109579,47.7122054283791,124.597703165401)) ;
#71046=CARTESIAN_POINT('Ctrl Pts',(-19.2619554888101,47.912121647868,124.935052545408)) ;
#71047=CARTESIAN_POINT('Ctrl Pts',(-19.2914239665457,47.7321325675052,124.630406187641)) ;
#71048=CARTESIAN_POINT('Ctrl Pts',(-18.7527354696576,47.9319981104837,124.794293876189)) ;
#71049=CARTESIAN_POINT('Ctrl Pts',(-18.8840463051201,47.7520090301208,124.51780103702)) ;
#71050=CARTESIAN_POINT('Ctrl Pts',(-18.3198015893089,47.951975339089,124.486914551041)) ;
#71051=CARTESIAN_POINT('Ctrl Pts',(-18.5376979391742,47.7719862587261,124.271898997653)) ;
#71052=CARTESIAN_POINT('Ctrl Pts',(-18.0187050938315,47.9719101970627,124.050892286809)) ;
#71053=CARTESIAN_POINT('Ctrl Pts',(-18.2968188352507,47.7919211166998,123.923081749406)) ;
#71054=CARTESIAN_POINT('Ctrl Pts',(-17.8842318765923,47.9918066459935,123.539502996666)) ;
#71055=CARTESIAN_POINT('Ctrl Pts',(-18.1892385060343,47.8118175656306,123.51396964369)) ;
#71056=CARTESIAN_POINT('Ctrl Pts',(-17.9318165298211,48.0117279300601,123.012148120241)) ;
#71057=CARTESIAN_POINT('Ctrl Pts',(-18.227305199235,47.8317388496972,123.092084787911)) ;
#71058=CARTESIAN_POINT('Ctrl Pts',(-18.1570558911766,48.0316845797311,122.53190203543)) ;
#71059=CARTESIAN_POINT('Ctrl Pts',(-18.4074959798686,47.8516954993682,122.7078870895)) ;
#71060=CARTESIAN_POINT('Ctrl Pts',(-18.5309774065162,48.0515618728427,122.158784664484)) ;
#71061=CARTESIAN_POINT('Ctrl Pts',(-18.7066337296029,47.8715727924798,122.409391583344)) ;
#71062=CARTESIAN_POINT('Ctrl Pts',(-19.0095199143223,48.0714483450711,121.934235959805)) ;
#71063=CARTESIAN_POINT('Ctrl Pts',(-19.0894691453368,47.8914592647082,122.229752104761)) ;
#71064=CARTESIAN_POINT('Ctrl Pts',(-19.540633493891,48.0915099109951,121.886851609452)) ;
#71065=CARTESIAN_POINT('Ctrl Pts',(-19.5143591422602,47.9115208306322,122.191844655207)) ;
#71066=CARTESIAN_POINT('Ctrl Pts',(-20.0501821768271,48.1113503185359,122.022521216227)) ;
#71067=CARTESIAN_POINT('Ctrl Pts',(-19.9220001526352,47.931361238173,122.300380806211)) ;
#71068=CARTESIAN_POINT('Ctrl Pts',(-20.4843799802069,48.1312016425088,122.322303458234)) ;
#71069=CARTESIAN_POINT('Ctrl Pts',(-20.2693591621974,47.9512125621459,122.540208559723)) ;
#71070=CARTESIAN_POINT('Ctrl Pts',(-20.7926161664346,48.1512549124602,122.757030819445)) ;
#71071=CARTESIAN_POINT('Ctrl Pts',(-20.5159469547042,47.9712658320974,122.887990515959)) ;
#71072=CARTESIAN_POINT('Ctrl Pts',(-20.93252583496,48.1710755698436,123.265061844735)) ;
#71073=CARTESIAN_POINT('Ctrl Pts',(-20.627874051427,47.9910864894807,123.294417505765)) ;
#71074=CARTESIAN_POINT('Ctrl Pts',(-20.8912365983079,48.1910469911741,123.794086280571)) ;
#71075=CARTESIAN_POINT('Ctrl Pts',(-20.5948408958009,48.0110579108112,123.717637230084)) ;
#71076=CARTESIAN_POINT('Ctrl Pts',(-20.6727225902505,48.2109404835378,124.275764014104)) ;
#71077=CARTESIAN_POINT('Ctrl Pts',(-20.4200275548019,48.0309514031749,124.102979505904)) ;
#71078=CARTESIAN_POINT('Ctrl Pts',(-20.3004819424767,48.2309645697788,124.655976968053)) ;
#71079=CARTESIAN_POINT('Ctrl Pts',(-20.1222337727236,48.050975489416,124.407148369197)) ;
#71080=CARTESIAN_POINT('Ctrl Pts',(-19.8260643109497,48.2507694488917,124.884148701362)) ;
#71081=CARTESIAN_POINT('Ctrl Pts',(-19.7426971430051,48.0707803685288,124.589684526452)) ;
#71082=CARTESIAN_POINT('Ctrl Pts',(-19.298401689414,48.2707284645896,124.938563164576)) ;
#71083=CARTESIAN_POINT('Ctrl Pts',(-19.3205664831375,48.0907393842267,124.633213331361)) ;
#71084=CARTESIAN_POINT('Ctrl Pts',(-18.7834401752579,48.2907144882186,124.808270536172)) ;
#71085=CARTESIAN_POINT('Ctrl Pts',(-18.9085977754014,48.1107254078558,124.528976723537)) ;
#71086=CARTESIAN_POINT('Ctrl Pts',(-18.3471324483424,48.3105229839791,124.513544556307)) ;
#71087=CARTESIAN_POINT('Ctrl Pts',(-18.5595521151312,48.1305339036163,124.29319269375)) ;
#71088=CARTESIAN_POINT('Ctrl Pts',(-18.0344280932835,48.3305056230847,124.084394876722)) ;
#71089=CARTESIAN_POINT('Ctrl Pts',(-18.3093912303342,48.1505165427219,123.949870956698)) ;
#71090=CARTESIAN_POINT('Ctrl Pts',(-17.8877491679608,48.3503870708787,123.576606049549)) ;
#71091=CARTESIAN_POINT('Ctrl Pts',(-18.1920510956395,48.1703979905159,123.543638317555)) ;
#71092=CARTESIAN_POINT('Ctrl Pts',(-17.9228534217252,48.3703435376163,123.047472668677)) ;
#71093=CARTESIAN_POINT('Ctrl Pts',(-18.2201380308155,48.1903544572534,123.120331605847)) ;
#71094=CARTESIAN_POINT('Ctrl Pts',(-18.1353200268485,48.3902209345718,122.563676201082)) ;
#71095=CARTESIAN_POINT('Ctrl Pts',(-18.3901149639764,48.210231854209,122.733295384716)) ;
#71096=CARTESIAN_POINT('Ctrl Pts',(-18.5017348375152,48.4102028807471,122.179310317759)) ;
#71097=CARTESIAN_POINT('Ctrl Pts',(-18.6832494823206,48.2302138003843,122.425805199473)) ;
#71098=CARTESIAN_POINT('Ctrl Pts',(-18.9763255338847,48.4301319797839,121.943845821942)) ;
#71099=CARTESIAN_POINT('Ctrl Pts',(-19.0629244628759,48.250142899421,122.237437292873)) ;
#71100=CARTESIAN_POINT('Ctrl Pts',(-19.5025485758174,48.4500606029965,121.8844085627)) ;
#71101=CARTESIAN_POINT('Ctrl Pts',(-19.4839018350502,48.2700715226336,122.189890020095)) ;
#71102=CARTESIAN_POINT('Ctrl Pts',(-20.0154041734413,48.4698949271029,122.006602474331)) ;
#71103=CARTESIAN_POINT('Ctrl Pts',(-19.8941925598735,48.28990584674,122.287654399379)) ;
#71104=CARTESIAN_POINT('Ctrl Pts',(-20.3852740340378,48.4865472144863,122.249514009236)) ;
#71105=CARTESIAN_POINT('Ctrl Pts',(-20.1900656488884,48.3065581341234,122.481970779686)) ;
#71106=CARTESIAN_POINT('Ctrl Pts',(-20.6170557319961,48.4998077155085,122.509808729621)) ;
#71107=CARTESIAN_POINT('Ctrl Pts',(-20.3755074720273,48.3198186351457,122.690222602484)) ;
#71108=CARTESIAN_POINT('Ctrl Pts',(-20.7555225669231,48.5098091927098,122.73319887295)) ;
#71109=CARTESIAN_POINT('Ctrl Pts',(-20.4862754159992,48.3298201123469,122.868932815288)) ;
#71110=CARTESIAN_POINT('Ctrl Pts',(-20.8529891978789,48.5198412135693,122.978158629166)) ;
#71111=CARTESIAN_POINT('Ctrl Pts',(-20.5642475521182,48.3398521332064,123.064902698722)) ;
#71112=CARTESIAN_POINT('Ctrl Pts',(-20.9058519382839,48.5297047572949,123.231906669117)) ;
#71113=CARTESIAN_POINT('Ctrl Pts',(-20.6065360580068,48.349715676932,123.267899228391)) ;
#71114=CARTESIAN_POINT('Ctrl Pts',(-20.9146324101858,48.539673470965,123.493731289981)) ;
#71115=CARTESIAN_POINT('Ctrl Pts',(-20.613556026208,48.3596843906021,123.477368180223)) ;
#71116=CARTESIAN_POINT('Ctrl Pts',(-20.8648547231583,48.5530192183687,123.840870176946)) ;
#71117=CARTESIAN_POINT('Ctrl Pts',(-20.5737423451447,48.3730301380058,123.755033409764)) ;
#71118=CARTESIAN_POINT('Ctrl Pts',(-20.7281894338226,48.5661697734414,124.16259745941)) ;
#71119=CARTESIAN_POINT('Ctrl Pts',(-20.4644056241511,48.3861806930785,124.012444016206)) ;
#71120=CARTESIAN_POINT('Ctrl Pts',(-20.5118249048892,48.5795551539912,124.439903596676)) ;
#71121=CARTESIAN_POINT('Ctrl Pts',(-20.2913023607941,48.3995660736284,124.234297052958)) ;
#71122=CARTESIAN_POINT('Ctrl Pts',(-20.3188115906214,48.5894430899841,124.613917552832)) ;
#71123=CARTESIAN_POINT('Ctrl Pts',(-20.1368920377986,48.4094540096212,124.373504600187)) ;
#71124=CARTESIAN_POINT('Ctrl Pts',(-20.0965059871697,48.5994342797967,124.753554193822)) ;
#71125=CARTESIAN_POINT('Ctrl Pts',(-19.9590458940921,48.4194451994339,124.485212524752)) ;
#71126=CARTESIAN_POINT('Ctrl Pts',(-19.8542566549361,48.609386378335,124.852215716831)) ;
#71127=CARTESIAN_POINT('Ctrl Pts',(-19.7652457303651,48.4293972979721,124.5641395104)) ;
#71128=CARTESIAN_POINT('Ctrl Pts',(-19.5961577410576,48.6194326347855,124.907656726796)) ;
#71129=CARTESIAN_POINT('Ctrl Pts',(-19.5587661686804,48.4394435544226,124.608490145194)) ;
#71130=CARTESIAN_POINT('Ctrl Pts',(-19.337504837007,48.6292820821796,124.917439257159)) ;
#71131=CARTESIAN_POINT('Ctrl Pts',(-19.3518437348216,48.4492930018168,124.616313910644)) ;
#71132=CARTESIAN_POINT('Ctrl Pts',(-19.078037022272,48.6392447346748,124.882575057759)) ;
#71133=CARTESIAN_POINT('Ctrl Pts',(-19.1442698490704,48.4592556543119,124.588420320008)) ;
#71134=CARTESIAN_POINT('Ctrl Pts',(-18.8271502999389,48.6492678203169,124.802367820736)) ;
#71135=CARTESIAN_POINT('Ctrl Pts',(-18.9435612086211,48.469278739954,124.524252395797)) ;
#71136=CARTESIAN_POINT('Ctrl Pts',(-18.5961153422512,48.6591929360738,124.681264951306)) ;
#71137=CARTESIAN_POINT('Ctrl Pts',(-18.7587343441336,48.479203855711,124.427368128863)) ;
#71138=CARTESIAN_POINT('Ctrl Pts',(-18.3870750955819,48.6692454144736,124.519790373217)) ;
#71139=CARTESIAN_POINT('Ctrl Pts',(-18.5915035653785,48.4892563341108,124.298186706336)) ;
#71140=CARTESIAN_POINT('Ctrl Pts',(-18.2126444694148,48.6790969131764,124.328462267053)) ;
#71141=CARTESIAN_POINT('Ctrl Pts',(-18.4519607973613,48.4991078328135,124.14512276976)) ;
#71142=CARTESIAN_POINT('Ctrl Pts',(-18.0718445075732,48.6890686523789,124.107495060904)) ;
#71143=CARTESIAN_POINT('Ctrl Pts',(-18.339322775097,48.509079572016,123.968347874547)) ;
#71144=CARTESIAN_POINT('Ctrl Pts',(-17.9713155069276,48.6990638601446,123.86478462589)) ;
#71145=CARTESIAN_POINT('Ctrl Pts',(-18.2589016723393,48.5190747797817,123.774178726449)) ;
#71146=CARTESIAN_POINT('Ctrl Pts',(-17.9145635742469,48.7090978616136,123.607305099869)) ;
#71147=CARTESIAN_POINT('Ctrl Pts',(-18.213502337176,48.5291087812508,123.568194649321)) ;
#71148=CARTESIAN_POINT('Ctrl Pts',(-17.9031654069168,48.718953219706,123.348541528174)) ;
#71149=CARTESIAN_POINT('Ctrl Pts',(-18.2043860513762,48.5389641393431,123.361183881843)) ;
#71150=CARTESIAN_POINT('Ctrl Pts',(-17.937003026666,48.7289526952993,123.088000944887)) ;
#71151=CARTESIAN_POINT('Ctrl Pts',(-18.231458353244,48.5489636149364,123.152751774568)) ;
#71152=CARTESIAN_POINT('Ctrl Pts',(-18.0144858731634,48.7388471437944,122.839746756377)) ;
#71153=CARTESIAN_POINT('Ctrl Pts',(-18.29344667902,48.5588580634315,122.954149283923)) ;
#71154=CARTESIAN_POINT('Ctrl Pts',(-18.1359580112243,48.7489102680221,122.604899456879)) ;
#71155=CARTESIAN_POINT('Ctrl Pts',(-18.3906263763058,48.5689211876593,122.766272439426)) ;
#71156=CARTESIAN_POINT('Ctrl Pts',(-18.2926260056632,48.7587498943507,122.399136493447)) ;
#71157=CARTESIAN_POINT('Ctrl Pts',(-18.5159623218924,48.5787608139879,122.601663664949)) ;
#71158=CARTESIAN_POINT('Ctrl Pts',(-18.4866726839865,48.7688131293937,122.219522458127)) ;
#71159=CARTESIAN_POINT('Ctrl Pts',(-18.6712011734618,48.5888240490308,122.457974012859)) ;
#71160=CARTESIAN_POINT('Ctrl Pts',(-18.7053931823134,48.7787071346277,122.078888414331)) ;
#71161=CARTESIAN_POINT('Ctrl Pts',(-18.8461785372344,48.5987180542649,122.345468767959)) ;
#71162=CARTESIAN_POINT('Ctrl Pts',(-18.9460602718396,48.7886498478435,121.977234200229)) ;
#71163=CARTESIAN_POINT('Ctrl Pts',(-19.038712845065,48.6086607674806,122.264147453385)) ;
#71164=CARTESIAN_POINT('Ctrl Pts',(-19.2023805082056,48.7986555876417,121.918479266341)) ;
#71165=CARTESIAN_POINT('Ctrl Pts',(-19.2437694535632,48.6186665072788,122.217145598752)) ;
#71166=CARTESIAN_POINT('Ctrl Pts',(-19.4653884139487,48.8086764897881,121.905400360003)) ;
#71167=CARTESIAN_POINT('Ctrl Pts',(-19.4541758671944,48.6286874094252,122.206684634383)) ;
#71168=CARTESIAN_POINT('Ctrl Pts',(-19.7233301714243,48.818567259837,121.937466358609)) ;
#71169=CARTESIAN_POINT('Ctrl Pts',(-19.660528678975,48.6385781794741,122.232339509988)) ;
#71170=CARTESIAN_POINT('Ctrl Pts',(-19.9744129235702,48.8285586706167,122.014229612701)) ;
#71171=CARTESIAN_POINT('Ctrl Pts',(-19.8613941678022,48.6485695902538,122.29375209031)) ;
#71172=CARTESIAN_POINT('Ctrl Pts',(-20.2073088426993,48.8385070162812,122.13298779378)) ;
#71173=CARTESIAN_POINT('Ctrl Pts',(-20.0477097505346,48.6585179359183,122.388760413796)) ;
#71174=CARTESIAN_POINT('Ctrl Pts',(-20.4163278633967,48.8484518743424,122.289901832939)) ;
#71175=CARTESIAN_POINT('Ctrl Pts',(-20.2149235466463,48.6684627939795,122.514293137704)) ;
#71176=CARTESIAN_POINT('Ctrl Pts',(-20.5965846062851,48.8585067097353,122.483065165235)) ;
#71177=CARTESIAN_POINT('Ctrl Pts',(-20.3591274717753,48.6785176293724,122.66882529591)) ;
#71178=CARTESIAN_POINT('Ctrl Pts',(-20.7376368968491,48.8683290818368,122.699266149593)) ;
#71179=CARTESIAN_POINT('Ctrl Pts',(-20.4719672538664,48.6883400014739,122.841786671009)) ;
#71180=CARTESIAN_POINT('Ctrl Pts',(-20.8418372689003,48.8783849492805,122.942091527948)) ;
#71181=CARTESIAN_POINT('Ctrl Pts',(-20.555325764693,48.6983958689176,123.036047837099)) ;
#71182=CARTESIAN_POINT('Ctrl Pts',(-20.9011534756052,48.8883256791384,123.196510502706)) ;
#71183=CARTESIAN_POINT('Ctrl Pts',(-20.6027766814318,48.7083365987755,123.239583219455)) ;
#71184=CARTESIAN_POINT('Ctrl Pts',(-20.9161549876618,48.8982300176895,123.456358415646)) ;
#71185=CARTESIAN_POINT('Ctrl Pts',(-20.6147759351108,48.7182409373267,123.447461235112)) ;
#71186=CARTESIAN_POINT('Ctrl Pts',(-20.8852105592629,48.908276699118,123.718532273713)) ;
#71187=CARTESIAN_POINT('Ctrl Pts',(-20.5900184387417,48.7282876187551,123.657200174612)) ;
#71188=CARTESIAN_POINT('Ctrl Pts',(-20.810567540589,48.9181722065873,123.967677397249)) ;
#71189=CARTESIAN_POINT('Ctrl Pts',(-20.530302315986,48.7381831262244,123.856515274534)) ;
#71190=CARTESIAN_POINT('Ctrl Pts',(-20.6918640066937,48.9282344750859,124.203918318717)) ;
#71191=CARTESIAN_POINT('Ctrl Pts',(-20.4353377019454,48.748245394723,124.045507277748)) ;
#71192=CARTESIAN_POINT('Ctrl Pts',(-20.5374874732684,48.9380764653565,124.4114706526)) ;
#71193=CARTESIAN_POINT('Ctrl Pts',(-20.3118353640093,48.7580873849936,124.211547452761)) ;
#71194=CARTESIAN_POINT('Ctrl Pts',(-20.346982966348,48.9480698822375,124.59217583248)) ;
#71195=CARTESIAN_POINT('Ctrl Pts',(-20.1594306094742,48.7680808018746,124.356110185967)) ;
#71196=CARTESIAN_POINT('Ctrl Pts',(-20.1294622771985,48.9579943700896,124.736115686117)) ;
#71197=CARTESIAN_POINT('Ctrl Pts',(-19.9854133980772,48.7780052897268,124.471260339818)) ;
#71198=CARTESIAN_POINT('Ctrl Pts',(-19.8885974147487,48.9679940039981,124.841121711921)) ;
#71199=CARTESIAN_POINT('Ctrl Pts',(-19.7927208876813,48.7880049236352,124.555263504968)) ;
#71200=CARTESIAN_POINT('Ctrl Pts',(-19.6334469697658,48.9779801142549,124.9026502756)) ;
#71201=CARTESIAN_POINT('Ctrl Pts',(-19.5886002554755,48.797991033892,124.604484611095)) ;
#71202=CARTESIAN_POINT('Ctrl Pts',(-19.3702291570135,48.988016065442,124.918743054803)) ;
#71203=CARTESIAN_POINT('Ctrl Pts',(-19.3780258273931,48.8080269850791,124.617357030523)) ;
#71204=CARTESIAN_POINT('Ctrl Pts',(-19.1128025382839,48.9978727037768,124.889803469788)) ;
#71205=CARTESIAN_POINT('Ctrl Pts',(-19.1720854580198,48.8178836234139,124.594203711341)) ;
#71206=CARTESIAN_POINT('Ctrl Pts',(-18.8606911455665,49.0078716638548,124.815911669425)) ;
#71207=CARTESIAN_POINT('Ctrl Pts',(-18.9703969207896,48.8278825834919,124.535088685264)) ;
#71208=CARTESIAN_POINT('Ctrl Pts',(-18.6274774420179,49.0177668941686,124.700789980476)) ;
#71209=CARTESIAN_POINT('Ctrl Pts',(-18.7838272068471,48.8377778138057,124.442990132716)) ;
#71210=CARTESIAN_POINT('Ctrl Pts',(-18.4143731818113,49.0278274066372,124.544376734575)) ;
#71211=CARTESIAN_POINT('Ctrl Pts',(-18.6133446125383,48.8478383262744,124.317858101007)) ;
#71212=CARTESIAN_POINT('Ctrl Pts',(-18.2353571530203,49.0376766981834,124.357410469631)) ;
#71213=CARTESIAN_POINT('Ctrl Pts',(-18.4701335294732,48.8576876178205,124.168284578467)) ;
#71214=CARTESIAN_POINT('Ctrl Pts',(-18.0883869155088,49.0477038841156,124.13870846236)) ;
#71215=CARTESIAN_POINT('Ctrl Pts',(-18.3525585546623,48.8677148037527,123.993322118891)) ;
#71216=CARTESIAN_POINT('Ctrl Pts',(-17.9822338382996,49.0577324205749,123.89747926818)) ;
#71217=CARTESIAN_POINT('Ctrl Pts',(-18.2676375508408,48.8777433402121,123.800338060987)) ;
#71218=CARTESIAN_POINT('Ctrl Pts',(-17.9202532459207,49.0675776605399,123.646304603655)) ;
#71219=CARTESIAN_POINT('Ctrl Pts',(-18.2180547698184,48.887588580177,123.599398834632)) ;
#71220=CARTESIAN_POINT('Ctrl Pts',(-17.9018658552473,49.0775683554631,123.384397836007)) ;
#71221=CARTESIAN_POINT('Ctrl Pts',(-18.2033462475352,48.8975792751002,123.389873479783)) ;
#71222=CARTESIAN_POINT('Ctrl Pts',(-17.9299430170255,49.0876061762217,123.122114050778)) ;
#71223=CARTESIAN_POINT('Ctrl Pts',(-18.2258094796159,48.9076170958588,123.180046505559)) ;
#71224=CARTESIAN_POINT('Ctrl Pts',(-18.0013047262961,49.0974507699987,122.873439403411)) ;
#71225=CARTESIAN_POINT('Ctrl Pts',(-18.2828999451431,48.9174616896358,122.981108076686)) ;
#71226=CARTESIAN_POINT('Ctrl Pts',(-18.1158511804771,49.1074347653747,122.637421711162)) ;
#71227=CARTESIAN_POINT('Ctrl Pts',(-18.3745381797035,48.9274456850118,122.792294678741)) ;
#71228=CARTESIAN_POINT('Ctrl Pts',(-18.2691440175312,49.1173838139361,122.425609469171)) ;
#71229=CARTESIAN_POINT('Ctrl Pts',(-18.4971732750292,48.9373947335732,122.622845958059)) ;
#71230=CARTESIAN_POINT('Ctrl Pts',(-18.4576938725769,49.1273862529106,122.242453382412)) ;
#71231=CARTESIAN_POINT('Ctrl Pts',(-18.6480139645982,48.9473971725478,122.476322036241)) ;
#71232=CARTESIAN_POINT('Ctrl Pts',(-18.6757844901155,49.137407494207,122.094840814009)) ;
#71233=CARTESIAN_POINT('Ctrl Pts',(-18.8224872183678,48.9574184138441,122.358233056651)) ;
#71234=CARTESIAN_POINT('Ctrl Pts',(-18.912980073684,49.1473001726465,121.988431832938)) ;
#71235=CARTESIAN_POINT('Ctrl Pts',(-19.0122435443815,48.9673110922836,122.273107306657)) ;
#71236=CARTESIAN_POINT('Ctrl Pts',(-19.1674232251513,49.1572902265941,121.923790931797)) ;
#71237=CARTESIAN_POINT('Ctrl Pts',(-19.2157981795932,48.9773011462313,122.221395753359)) ;
#71238=CARTESIAN_POINT('Ctrl Pts',(-19.4284019621495,49.1672485877426,121.904559887262)) ;
#71239=CARTESIAN_POINT('Ctrl Pts',(-19.4245809128314,48.9872595073797,122.206012139739)) ;
#71240=CARTESIAN_POINT('Ctrl Pts',(-19.6873094646854,49.1771482146274,121.930145178779)) ;
#71241=CARTESIAN_POINT('Ctrl Pts',(-19.6317061102632,48.9971591342646,122.226481354379)) ;
#71242=CARTESIAN_POINT('Ctrl Pts',(-19.941526102593,49.1871961114308,122.001425268329)) ;
#71243=CARTESIAN_POINT('Ctrl Pts',(-19.8350792979722,49.0072070310679,122.283506510641)) ;
#71244=CARTESIAN_POINT('Ctrl Pts',(-20.1760417540059,49.1970914690668,122.113872563223)) ;
#71245=CARTESIAN_POINT('Ctrl Pts',(-20.022690714718,49.0171023887039,122.373464959482)) ;
#71246=CARTESIAN_POINT('Ctrl Pts',(-20.3909878097268,49.2071531215235,122.267804384145)) ;
#71247=CARTESIAN_POINT('Ctrl Pts',(-20.1946471758079,49.0271640411606,122.496611400077)) ;
#71248=CARTESIAN_POINT('Ctrl Pts',(-20.5720068053571,49.2169977257954,122.452644101985)) ;
#71249=CARTESIAN_POINT('Ctrl Pts',(-20.3394609075565,49.0370086454325,122.644483128646)) ;
#71250=CARTESIAN_POINT('Ctrl Pts',(-20.7206623097227,49.2269578474934,122.668068984939)) ;
#71251=CARTESIAN_POINT('Ctrl Pts',(-20.4583844503407,49.0469687671305,122.816823184735)) ;
#71252=CARTESIAN_POINT('Ctrl Pts',(-20.8300406886576,49.2369958818559,122.90810181371)) ;
#71253=CARTESIAN_POINT('Ctrl Pts',(-20.5458863746886,49.0570068014931,123.008849944546)) ;
#71254=CARTESIAN_POINT('Ctrl Pts',(-20.895474107219,49.2468701944424,123.15923667191)) ;
#71255=CARTESIAN_POINT('Ctrl Pts',(-20.5982321097899,49.0668811140795,123.209757165169)) ;
#71256=CARTESIAN_POINT('Ctrl Pts',(-20.9167021696326,49.2569396752251,123.422962968094)) ;
#71257=CARTESIAN_POINT('Ctrl Pts',(-20.6152137829838,49.0769505948622,123.420738590608)) ;
#71258=CARTESIAN_POINT('Ctrl Pts',(-20.8925309748415,49.2667740112422,123.680288852952)) ;
#71259=CARTESIAN_POINT('Ctrl Pts',(-20.5958761715019,49.0867849308793,123.626598057855)) ;
#71260=CARTESIAN_POINT('Ctrl Pts',(-20.8233682239885,49.2768069689704,123.934702843844)) ;
#71261=CARTESIAN_POINT('Ctrl Pts',(-20.5405453724813,49.0968178886076,123.830129187291)) ;
#71262=CARTESIAN_POINT('Ctrl Pts',(-20.7105597644519,49.2868273675456,124.172644633411)) ;
#71263=CARTESIAN_POINT('Ctrl Pts',(-20.4502978908563,49.1068382871827,124.020482314942)) ;
#71264=CARTESIAN_POINT('Ctrl Pts',(-20.5610300420917,49.2966929413168,124.38445939655)) ;
#71265=CARTESIAN_POINT('Ctrl Pts',(-20.3306741735145,49.116703860954,124.189932981708)) ;
#71266=CARTESIAN_POINT('Ctrl Pts',(-20.3732384290242,49.3067618159729,124.570826297004)) ;
#71267=CARTESIAN_POINT('Ctrl Pts',(-20.1804402169388,49.12677273561,124.33902629884)) ;
#71268=CARTESIAN_POINT('Ctrl Pts',(-20.1607506292362,49.3166072468784,124.718462326025)) ;
#71269=CARTESIAN_POINT('Ctrl Pts',(-20.0104505595802,49.1366181665155,124.457133981811)) ;
#71270=CARTESIAN_POINT('Ctrl Pts',(-19.9230300882037,49.3265868717491,124.829197136237)) ;
#71271=CARTESIAN_POINT('Ctrl Pts',(-19.820274187598,49.1465977913862,124.545721370372)) ;
#71272=CARTESIAN_POINT('Ctrl Pts',(-19.6685730451368,49.3366055546632,124.896756529863)) ;
#71273=CARTESIAN_POINT('Ctrl Pts',(-19.6167084117739,49.1566164743003,124.599768387045)) ;
#71274=CARTESIAN_POINT('Ctrl Pts',(-19.4098038796016,49.346488819847,124.919356964503)) ;
#71275=CARTESIAN_POINT('Ctrl Pts',(-19.4096939213468,49.1664997394842,124.617848281741)) ;
#71276=CARTESIAN_POINT('Ctrl Pts',(-19.1462832607712,49.3565571139384,124.89615090551)) ;
#71277=CARTESIAN_POINT('Ctrl Pts',(-19.1988771347697,49.1765680335755,124.599282999011)) ;
#71278=CARTESIAN_POINT('Ctrl Pts',(-18.8966752356581,49.3663872441237,124.829435060277)) ;
#71279=CARTESIAN_POINT('Ctrl Pts',(-18.999191990857,49.1863981637609,124.545910321874)) ;
#71280=CARTESIAN_POINT('Ctrl Pts',(-18.656744831752,49.3764537923389,124.718117896912)) ;
#71281=CARTESIAN_POINT('Ctrl Pts',(-18.8072474823496,49.196464711976,124.456856234754)) ;
#71282=CARTESIAN_POINT('Ctrl Pts',(-18.4436181844938,49.3863440410275,124.569306863408)) ;
#71283=CARTESIAN_POINT('Ctrl Pts',(-18.6367470167291,49.2063549606646,124.337807652728)) ;
#71284=CARTESIAN_POINT('Ctrl Pts',(-18.2572992166369,49.3963362228035,124.384299698902)) ;
#71285=CARTESIAN_POINT('Ctrl Pts',(-18.4876920638657,49.2163471424406,124.189801941018)) ;
#71286=CARTESIAN_POINT('Ctrl Pts',(-18.1065741069592,49.4062990034313,124.170232758712)) ;
#71287=CARTESIAN_POINT('Ctrl Pts',(-18.3671123543255,49.2263099230684,124.018548569717)) ;
#71288=CARTESIAN_POINT('Ctrl Pts',(-17.9953598077173,49.4162034081051,123.934891647468)) ;
#71289=CARTESIAN_POINT('Ctrl Pts',(-18.2781412702089,49.2362143277422,123.830276340777)) ;
#71290=CARTESIAN_POINT('Ctrl Pts',(-17.9258209627765,49.4262634025841,123.679859999836)) ;
#71291=CARTESIAN_POINT('Ctrl Pts',(-18.2225102077793,49.2462743222212,123.626250739129)) ;
#71292=CARTESIAN_POINT('Ctrl Pts',(-17.9019035489539,49.4361120245539,123.422136143483)) ;
#71293=CARTESIAN_POINT('Ctrl Pts',(-18.2033764111946,49.256122944191,123.42007277146)) ;
#71294=CARTESIAN_POINT('Ctrl Pts',(-17.9228967151139,49.4461424639657,123.159399391363)) ;
#71295=CARTESIAN_POINT('Ctrl Pts',(-18.2201708355214,49.2661533836029,123.209883266575)) ;
#71296=CARTESIAN_POINT('Ctrl Pts',(-17.9895783325629,49.4561521796005,122.90491683128)) ;
#71297=CARTESIAN_POINT('Ctrl Pts',(-18.2735161375883,49.2761630992376,123.006297255522)) ;
#71298=CARTESIAN_POINT('Ctrl Pts',(-18.0980952655541,49.4660629322931,122.668183285469)) ;
#71299=CARTESIAN_POINT('Ctrl Pts',(-18.3603293441848,49.2860738519302,122.816911054056)) ;
#71300=CARTESIAN_POINT('Ctrl Pts',(-18.245826326081,49.4759922052395,122.453085432562)) ;
#71301=CARTESIAN_POINT('Ctrl Pts',(-18.4785136798849,49.2960031248766,122.644833143533)) ;
#71302=CARTESIAN_POINT('Ctrl Pts',(-18.4308927790873,49.4860348966322,122.264952869192)) ;
#71303=CARTESIAN_POINT('Ctrl Pts',(-18.6265668504671,49.3060458162693,122.494326860631)) ;
#71304=CARTESIAN_POINT('Ctrl Pts',(-18.6423948660931,49.4959214298497,122.114039679069)) ;
#71305=CARTESIAN_POINT('Ctrl Pts',(-18.7957676964125,49.3159323494868,122.373596652419)) ;
#71306=CARTESIAN_POINT('Ctrl Pts',(-18.8791977037883,49.5059145747817,122.000547015104)) ;
#71307=CARTESIAN_POINT('Ctrl Pts',(-18.9852096849577,49.3259254944189,122.282802310595)) ;
#71308=CARTESIAN_POINT('Ctrl Pts',(-19.1309496466814,49.5158602556182,121.930322869947)) ;
#71309=CARTESIAN_POINT('Ctrl Pts',(-19.1866107041673,49.3358711752553,122.226622847818)) ;
#71310=CARTESIAN_POINT('Ctrl Pts',(-19.3910719340289,49.5258075127667,121.904340399635)) ;
#71311=CARTESIAN_POINT('Ctrl Pts',(-19.3947080350026,49.3458184324039,122.205836499033)) ;
#71312=CARTESIAN_POINT('Ctrl Pts',(-19.6543477211243,49.5358554166387,121.924410607122)) ;
#71313=CARTESIAN_POINT('Ctrl Pts',(-19.605328890607,49.3558663362759,122.221892336368)) ;
#71314=CARTESIAN_POINT('Ctrl Pts',(-19.9051063909627,49.5457031157367,121.988376325681)) ;
#71315=CARTESIAN_POINT('Ctrl Pts',(-19.8059348407056,49.3657140353738,122.273064246999)) ;
#71316=CARTESIAN_POINT('Ctrl Pts',(-20.1440032593785,49.5556646067154,122.095383178499)) ;
#71317=CARTESIAN_POINT('Ctrl Pts',(-19.9970522508123,49.3756755263525,122.358669026334)) ;
#71318=CARTESIAN_POINT('Ctrl Pts',(-20.3619888762732,49.5656940691293,122.243550726972)) ;
#71319=CARTESIAN_POINT('Ctrl Pts',(-20.1714411021644,49.3857049887665,122.47720268182)) ;
#71320=CARTESIAN_POINT('Ctrl Pts',(-20.5487252565727,49.5756013002292,122.424969613015)) ;
#71321=CARTESIAN_POINT('Ctrl Pts',(-20.3208300784889,49.3956122198664,122.622336896963)) ;
#71322=CARTESIAN_POINT('Ctrl Pts',(-20.7021484057419,49.5855476789066,122.636565942067)) ;
#71323=CARTESIAN_POINT('Ctrl Pts',(-20.4435688760117,49.4055585985438,122.791613175442)) ;
#71324=CARTESIAN_POINT('Ctrl Pts',(-20.817273052069,49.5955524477155,122.872960551607)) ;
#71325=CARTESIAN_POINT('Ctrl Pts',(-20.5356691966512,49.4155633673526,122.980728486746)) ;
#71326=CARTESIAN_POINT('Ctrl Pts',(-20.8894241945035,49.6055735687357,123.126222955828)) ;
#71327=CARTESIAN_POINT('Ctrl Pts',(-20.5933907246933,49.4255844883728,123.183338265928)) ;
#71328=CARTESIAN_POINT('Ctrl Pts',(-20.9164510303163,49.6154644345883,123.384745011977)) ;
#71329=CARTESIAN_POINT('Ctrl Pts',(-20.6150128120107,49.4354753542255,123.390155041313)) ;
#71330=CARTESIAN_POINT('Ctrl Pts',(-20.8983831554368,49.6254552433476,123.64665553533)) ;
#71331=CARTESIAN_POINT('Ctrl Pts',(-20.6005593184925,49.4454661629847,123.599683344797)) ;
#71332=CARTESIAN_POINT('Ctrl Pts',(-20.8353127628865,49.6354059015279,123.900441641724)) ;
#71333=CARTESIAN_POINT('Ctrl Pts',(-20.550103868979,49.4554168211651,123.802711999998)) ;
#71334=CARTESIAN_POINT('Ctrl Pts',(-20.7296226128942,49.64534211117,124.139186358957)) ;
#71335=CARTESIAN_POINT('Ctrl Pts',(-20.4655527511557,49.4653530308072,123.993707659371)) ;
#71336=CARTESIAN_POINT('Ctrl Pts',(-20.5836489640743,49.6553252778949,124.357211327668)) ;
#71337=CARTESIAN_POINT('Ctrl Pts',(-20.3487747338897,49.475336197532,124.168127991278)) ;
#71338=CARTESIAN_POINT('Ctrl Pts',(-20.4006247563479,49.6653690751052,124.547345114736)) ;
#71339=CARTESIAN_POINT('Ctrl Pts',(-20.2023558633861,49.4853799947423,124.320235708206)) ;
#71340=CARTESIAN_POINT('Ctrl Pts',(-20.1922492122206,49.6751972912734,124.70000920038)) ;
#71341=CARTESIAN_POINT('Ctrl Pts',(-20.0356569367093,49.4952082109106,124.442367083583)) ;
#71342=CARTESIAN_POINT('Ctrl Pts',(-19.9548171286621,49.6852738587427,124.817128808093)) ;
#71343=CARTESIAN_POINT('Ctrl Pts',(-19.84571140594,49.5052847783798,124.536063826559)) ;
#71344=CARTESIAN_POINT('Ctrl Pts',(-19.706248503042,49.6951259444321,124.889748332412)) ;
#71345=CARTESIAN_POINT('Ctrl Pts',(-19.646857742828,49.5151368640692,124.594160163181)) ;
#71346=CARTESIAN_POINT('Ctrl Pts',(-19.4431934347657,49.7051992118375,124.918954084388)) ;
#71347=CARTESIAN_POINT('Ctrl Pts',(-19.436413489415,49.5252101314746,124.617525881266)) ;
#71348=CARTESIAN_POINT('Ctrl Pts',(-19.1850858539182,49.7150406282611,124.902355961624)) ;
#71349=CARTESIAN_POINT('Ctrl Pts',(-19.2299283962633,49.5350515478982,124.604248517549)) ;
#71350=CARTESIAN_POINT('Ctrl Pts',(-18.93051882681,49.7250018864038,124.841407931651)) ;
#71351=CARTESIAN_POINT('Ctrl Pts',(-19.0262747888918,49.545012806041,124.555491422723)) ;
#71352=CARTESIAN_POINT('Ctrl Pts',(-18.6887821551517,49.7350385628358,124.735926054212)) ;
#71353=CARTESIAN_POINT('Ctrl Pts',(-18.8328848873509,49.5550494824729,124.471106955947)) ;
#71354=CARTESIAN_POINT('Ctrl Pts',(-18.472223638631,49.7449171706996,124.592716974689)) ;
#71355=CARTESIAN_POINT('Ctrl Pts',(-18.6596380365307,49.5649280903367,124.356541193233)) ;
#71356=CARTESIAN_POINT('Ctrl Pts',(-18.2803615486336,49.7549773993384,124.410883615209)) ;
#71357=CARTESIAN_POINT('Ctrl Pts',(-18.5061473145343,49.5749883189755,124.211075281749)) ;
#71358=CARTESIAN_POINT('Ctrl Pts',(-18.1259078276829,49.7648443834992,124.2025693445)) ;
#71359=CARTESIAN_POINT('Ctrl Pts',(-18.3825837898089,49.5848553031363,124.044425304176)) ;
#71360=CARTESIAN_POINT('Ctrl Pts',(-18.007919160607,49.7748499497519,123.967632043592)) ;
#71361=CARTESIAN_POINT('Ctrl Pts',(-18.2881916293145,49.594860869389,123.856476155528)) ;
#71362=CARTESIAN_POINT('Ctrl Pts',(-17.9327202356782,49.7848337381665,123.716228002346)) ;
#71363=CARTESIAN_POINT('Ctrl Pts',(-18.2280312110072,49.6048446578036,123.655353491718)) ;
#71364=CARTESIAN_POINT('Ctrl Pts',(-17.9024202751919,49.7948795949691,123.453999545748)) ;
#71365=CARTESIAN_POINT('Ctrl Pts',(-18.2037899069106,49.6148905146063,123.445570751579)) ;
#71366=CARTESIAN_POINT('Ctrl Pts',(-17.9174338428605,49.8047054721851,123.196221483282)) ;
#71367=CARTESIAN_POINT('Ctrl Pts',(-18.2157993021619,49.6247163918222,123.23934924798)) ;
#71368=CARTESIAN_POINT('Ctrl Pts',(-17.9771398351836,49.8146959480264,122.940561425494)) ;
#71369=CARTESIAN_POINT('Ctrl Pts',(-18.2635625340082,49.6347068676635,123.034820978752)) ;
#71370=CARTESIAN_POINT('Ctrl Pts',(-18.0815158765867,49.8247395239252,122.698141841169)) ;
#71371=CARTESIAN_POINT('Ctrl Pts',(-18.3470620957204,49.6447504435623,122.840884636504)) ;
#71372=CARTESIAN_POINT('Ctrl Pts',(-18.2227460406671,49.8345613162232,122.482103844544)) ;
#71373=CARTESIAN_POINT('Ctrl Pts',(-18.4600443913908,49.6545722358604,122.668054229687)) ;
#71374=CARTESIAN_POINT('Ctrl Pts',(-18.4027042307795,49.8445962818491,122.289342033901)) ;
#71375=CARTESIAN_POINT('Ctrl Pts',(-18.6040097854602,49.6646072014862,122.513843584762)) ;
#71376=CARTESIAN_POINT('Ctrl Pts',(-18.6136336981396,49.8546211987822,122.131496311253)) ;
#71377=CARTESIAN_POINT('Ctrl Pts',(-18.772752461505,49.6746321184193,122.38756577421)) ;
#71378=CARTESIAN_POINT('Ctrl Pts',(-18.844452425863,49.8644731371583,122.014217927815)) ;
#71379=CARTESIAN_POINT('Ctrl Pts',(-18.9574059859319,49.6844840567954,122.293741978756)) ;
#71380=CARTESIAN_POINT('Ctrl Pts',(-19.0954698169911,49.8744641131831,121.937362207403)) ;
#71381=CARTESIAN_POINT('Ctrl Pts',(-19.1582192690863,49.6944750328202,122.232255812791)) ;
#71382=CARTESIAN_POINT('Ctrl Pts',(-19.3541562238253,49.8843819339867,121.905312031361)) ;
#71383=CARTESIAN_POINT('Ctrl Pts',(-19.3651677277275,49.7043928536238,122.206614010283)) ;
#71384=CARTESIAN_POINT('Ctrl Pts',(-19.6173285205986,49.8944106545513,121.918768394832)) ;
#71385=CARTESIAN_POINT('Ctrl Pts',(-19.5757056845183,49.7144215741884,122.217377365489)) ;
#71386=CARTESIAN_POINT('Ctrl Pts',(-19.8705237928236,49.9042935811605,121.976696588945)) ;
#71387=CARTESIAN_POINT('Ctrl Pts',(-19.7782617108459,49.7243045007976,122.263718061929)) ;
#71388=CARTESIAN_POINT('Ctrl Pts',(-20.1128653758692,49.91429786628,122.078541501099)) ;
#71389=CARTESIAN_POINT('Ctrl Pts',(-19.9721356237173,49.7343087859171,122.345192269613)) ;
#71390=CARTESIAN_POINT('Ctrl Pts',(-20.3334334359267,49.9242815474878,122.22068996082)) ;
#71391=CARTESIAN_POINT('Ctrl Pts',(-20.1485909406997,49.7442924671249,122.458909422584)) ;
#71392=CARTESIAN_POINT('Ctrl Pts',(-20.5268216963565,49.9343225462177,122.400179102875)) ;
#71393=CARTESIAN_POINT('Ctrl Pts',(-20.3033028181441,49.7543334658549,122.602499480691)) ;
#71394=CARTESIAN_POINT('Ctrl Pts',(-20.683102613612,49.9441549910849,122.605949735523)) ;
#71395=CARTESIAN_POINT('Ctrl Pts',(-20.4283285548429,49.764165910722,122.767114266815)) ;
#71396=CARTESIAN_POINT('Ctrl Pts',(-20.8039177883312,49.9541499895152,122.839164524174)) ;
#71397=CARTESIAN_POINT('Ctrl Pts',(-20.5249823843959,49.7741609091523,122.953685109195)) ;
#71398=CARTESIAN_POINT('Ctrl Pts',(-20.8821585762413,49.9641815382648,123.090919199762)) ;
#71399=CARTESIAN_POINT('Ctrl Pts',(-20.5875768107398,49.7841924579019,123.155088321944)) ;
#71400=CARTESIAN_POINT('Ctrl Pts',(-20.9152659613685,49.9740469165703,123.348034537658)) ;
#71401=CARTESIAN_POINT('Ctrl Pts',(-20.6140645490356,49.7940578362074,123.3607797692)) ;
#71402=CARTESIAN_POINT('Ctrl Pts',(-20.9038469302478,49.9840087640306,123.609580354995)) ;
#71403=CARTESIAN_POINT('Ctrl Pts',(-20.6049313502839,49.8040196836677,123.57001630993)) ;
#71404=CARTESIAN_POINT('Ctrl Pts',(-20.8463577366402,49.9940437048448,123.8669305923)) ;
#71405=CARTESIAN_POINT('Ctrl Pts',(-20.5589419045982,49.814054624482,123.77589695398)) ;
#71406=CARTESIAN_POINT('Ctrl Pts',(-20.7469555508652,50.003928665862,124.106966043971)) ;
#71407=CARTESIAN_POINT('Ctrl Pts',(-20.4794221918956,49.8239395854991,123.967925670353)) ;
#71408=CARTESIAN_POINT('Ctrl Pts',(-20.6048292012254,50.0139942747808,124.330001338928)) ;
#71409=CARTESIAN_POINT('Ctrl Pts',(-20.3657227455692,49.8340051944179,124.146355087729)) ;
#71410=CARTESIAN_POINT('Ctrl Pts',(-20.4302906277304,50.0238334498225,124.520821628096)) ;
#71411=CARTESIAN_POINT('Ctrl Pts',(-20.2260937730439,49.8438443694597,124.299012279554)) ;
#71412=CARTESIAN_POINT('Ctrl Pts',(-20.2208961768224,50.0338960053224,124.682260919657)) ;
#71413=CARTESIAN_POINT('Ctrl Pts',(-20.0585794010133,49.8539069249596,124.42816542681)) ;
#71414=CARTESIAN_POINT('Ctrl Pts',(-19.990330202873,50.0437931800154,124.802645968509)) ;
#71415=CARTESIAN_POINT('Ctrl Pts',(-19.8741279016726,49.8638040996525,124.524475111746)) ;
#71416=CARTESIAN_POINT('Ctrl Pts',(-19.7418079589796,50.0537238949387,124.882264366511)) ;
#71417=CARTESIAN_POINT('Ctrl Pts',(-19.6753109887391,49.8737348145758,124.588171796186)) ;
#71418=CARTESIAN_POINT('Ctrl Pts',(-19.4802461248259,50.0637679230163,124.91762289268)) ;
#71419=CARTESIAN_POINT('Ctrl Pts',(-19.4660617807019,49.8837788426534,124.616460713011)) ;
#71420=CARTESIAN_POINT('Ctrl Pts',(-19.2206304688887,50.0736541248696,124.907397165842)) ;
#71421=CARTESIAN_POINT('Ctrl Pts',(-19.2583695113846,49.8936650445067,124.608282273323)) ;
#71422=CARTESIAN_POINT('Ctrl Pts',(-18.9639476699514,50.0836472913365,124.852050273482)) ;
#71423=CARTESIAN_POINT('Ctrl Pts',(-19.0530228963227,49.9036582109736,124.564006892753)) ;
#71424=CARTESIAN_POINT('Ctrl Pts',(-18.7219951492464,50.0935867623236,124.753556604735)) ;
#71425=CARTESIAN_POINT('Ctrl Pts',(-18.8594602370748,49.9135976819608,124.485214036914)) ;
#71426=CARTESIAN_POINT('Ctrl Pts',(-18.4991286839628,50.1036032766778,124.613546547454)) ;
#71427=CARTESIAN_POINT('Ctrl Pts',(-18.6811659438584,49.9236141963149,124.37320785353)) ;
#71428=CARTESIAN_POINT('Ctrl Pts',(-18.305447857855,50.1135333031546,124.438612238836)) ;
#71429=CARTESIAN_POINT('Ctrl Pts',(-18.5262199636435,49.9335442227918,124.233262162402)) ;
#71430=CARTESIAN_POINT('Ctrl Pts',(-18.1432330982203,50.1235858386641,124.23014085339)) ;
#71431=CARTESIAN_POINT('Ctrl Pts',(-18.396446423529,49.9435967583012,124.066486379902)) ;
#71432=CARTESIAN_POINT('Ctrl Pts',(-18.0220679537995,50.1334322418838,124.001499451881)) ;
#71433=CARTESIAN_POINT('Ctrl Pts',(-18.2995125219658,49.9534431615209,123.883574567668)) ;
#71434=CARTESIAN_POINT('Ctrl Pts',(-17.9407108291128,50.1433942847378,123.752685556883)) ;
#71435=CARTESIAN_POINT('Ctrl Pts',(-18.2344247243619,49.963405204375,123.684524241367)) ;
#71436=CARTESIAN_POINT('Ctrl Pts',(-17.903879790198,50.1534228355285,123.491714650898)) ;
#71437=CARTESIAN_POINT('Ctrl Pts',(-18.2049577020538,49.9734337551656,123.475747861428)) ;
#71438=CARTESIAN_POINT('Ctrl Pts',(-17.9127260347505,50.1633331612461,123.23144379837)) ;
#71439=CARTESIAN_POINT('Ctrl Pts',(-18.212032467387,49.9833440808833,123.267531271564)) ;
#71440=CARTESIAN_POINT('Ctrl Pts',(-17.9660995838745,50.1732680730757,122.975870378448)) ;
#71441=CARTESIAN_POINT('Ctrl Pts',(-18.2547290835788,49.9932789927128,123.063072178671)) ;
#71442=CARTESIAN_POINT('Ctrl Pts',(-18.0642927488552,50.1833090798438,122.730962183356)) ;
#71443=CARTESIAN_POINT('Ctrl Pts',(-18.3332815219319,50.0033199994809,122.867144823383)) ;
#71444=CARTESIAN_POINT('Ctrl Pts',(-18.201255664043,50.193196712676,122.510138724716)) ;
#71445=CARTESIAN_POINT('Ctrl Pts',(-18.4428498771025,50.0132076323131,122.690484981077)) ;
#71446=CARTESIAN_POINT('Ctrl Pts',(-18.3759163267486,50.203187143774,122.314146410369)) ;
#71447=CARTESIAN_POINT('Ctrl Pts',(-18.5825766919906,50.0231980634112,122.533689671197)) ;
#71448=CARTESIAN_POINT('Ctrl Pts',(-18.5813368510253,50.2131425803313,122.152125343484)) ;
#71449=CARTESIAN_POINT('Ctrl Pts',(-18.7469116404268,50.0331534999684,122.404071093068)) ;
#71450=CARTESIAN_POINT('Ctrl Pts',(-18.8104932141694,50.2230535284306,122.028377092564)) ;
#71451=CARTESIAN_POINT('Ctrl Pts',(-18.9302356832612,50.0430644480677,122.305070539431)) ;
#71452=CARTESIAN_POINT('Ctrl Pts',(-19.0601191774314,50.2330656045283,121.945157820195)) ;
#71453=CARTESIAN_POINT('Ctrl Pts',(-19.1299354530242,50.0530765241654,122.238492965492)) ;
#71454=CARTESIAN_POINT('Ctrl Pts',(-19.3208286510922,50.2430929266033,121.907019503274)) ;
#71455=CARTESIAN_POINT('Ctrl Pts',(-19.3385035281413,50.0631038462404,122.207980229758)) ;
#71456=CARTESIAN_POINT('Ctrl Pts',(-19.5798646279409,50.2529517015574,121.913948569486)) ;
#71457=CARTESIAN_POINT('Ctrl Pts',(-19.5457290400626,50.0729626211945,122.213520711451)) ;
#71458=CARTESIAN_POINT('Ctrl Pts',(-19.9254133373517,50.2663778943698,121.984759551957)) ;
#71459=CARTESIAN_POINT('Ctrl Pts',(-19.8221850711281,50.086388814007,122.270169142813)) ;
#71460=CARTESIAN_POINT('Ctrl Pts',(-20.2369013110527,50.2794619101513,122.13968280904)) ;
#71461=CARTESIAN_POINT('Ctrl Pts',(-20.0713939474092,50.0994728297884,122.394125151919)) ;
#71462=CARTESIAN_POINT('Ctrl Pts',(-20.5024950621529,50.2929353589065,122.373723117195)) ;
#71463=CARTESIAN_POINT('Ctrl Pts',(-20.2838339357162,50.1129462785436,122.581328603426)) ;
#71464=CARTESIAN_POINT('Ctrl Pts',(-20.6634968410946,50.3027683167123,122.575877232274)) ;
#71465=CARTESIAN_POINT('Ctrl Pts',(-20.4126446009124,50.1227792363495,122.743055923512)) ;
#71466=CARTESIAN_POINT('Ctrl Pts',(-20.7895391335986,50.312731590163,122.805346777483)) ;
#71467=CARTESIAN_POINT('Ctrl Pts',(-20.5134783878091,50.1327425098001,122.926629108663)) ;
#71468=CARTESIAN_POINT('Ctrl Pts',(-20.8739118055342,50.322768663981,123.05524832364)) ;
#71469=CARTESIAN_POINT('Ctrl Pts',(-20.5809791128739,50.1427795836181,123.126549935224)) ;
#71470=CARTESIAN_POINT('Ctrl Pts',(-20.9134611751376,50.3326436669926,123.311752830501)) ;
#71471=CARTESIAN_POINT('Ctrl Pts',(-20.6126206731099,50.1526545866297,123.331753172435)) ;
#71472=CARTESIAN_POINT('Ctrl Pts',(-20.9077542261225,50.3427113466188,123.576222416539)) ;
#71473=CARTESIAN_POINT('Ctrl Pts',(-20.6080572696327,50.1627222662559,123.543329200487)) ;
#71474=CARTESIAN_POINT('Ctrl Pts',(-20.857508009601,50.3525521968365,123.829932935511)) ;
#71475=CARTESIAN_POINT('Ctrl Pts',(-20.5678626302659,50.1725631164736,123.746296581769)) ;
#71476=CARTESIAN_POINT('Ctrl Pts',(-20.7314548291478,50.3658883953125,124.156910684336)) ;
#71477=CARTESIAN_POINT('Ctrl Pts',(-20.4670213805127,50.1858993149496,124.00788851066)) ;
#71478=CARTESIAN_POINT('Ctrl Pts',(-20.524653068368,50.3791059191269,124.440925618285)) ;
#71479=CARTESIAN_POINT('Ctrl Pts',(-20.3015547453208,50.199116838764,124.235123745287)) ;
#71480=CARTESIAN_POINT('Ctrl Pts',(-20.252395006723,50.3924408456182,124.66151880778)) ;
#71481=CARTESIAN_POINT('Ctrl Pts',(-20.0837839668042,50.2124517652553,124.411566257854)) ;
#71482=CARTESIAN_POINT('Ctrl Pts',(-20.0229851842833,50.4024239462128,124.788869046757)) ;
#71483=CARTESIAN_POINT('Ctrl Pts',(-19.9002502106648,50.2224348658499,124.513455083149)) ;
#71484=CARTESIAN_POINT('Ctrl Pts',(-19.7733522297728,50.4124687221124,124.874590001612)) ;
#71485=CARTESIAN_POINT('Ctrl Pts',(-19.7005468471622,50.2324796417495,124.582032094973)) ;
#71486=CARTESIAN_POINT('Ctrl Pts',(-19.5185568926512,50.4222866452983,124.915250650633)) ;
#71487=CARTESIAN_POINT('Ctrl Pts',(-19.4967086995116,50.2422975649354,124.614562632195)) ;
#71488=CARTESIAN_POINT('Ctrl Pts',(-19.2545052235582,50.4323359592536,124.911493375565)) ;
#71489=CARTESIAN_POINT('Ctrl Pts',(-19.2854717860523,50.2523468788908,124.611560855551)) ;
#71490=CARTESIAN_POINT('Ctrl Pts',(-18.9112636456039,50.4456396998762,124.845209773811)) ;
#71491=CARTESIAN_POINT('Ctrl Pts',(-19.0108574254215,50.2656506195133,124.558525723013)) ;
#71492=CARTESIAN_POINT('Ctrl Pts',(-18.5163636183236,50.4621298953529,124.654888417403)) ;
#71493=CARTESIAN_POINT('Ctrl Pts',(-18.6949672451094,50.28214081499,124.406294866323)) ;
#71494=CARTESIAN_POINT('Ctrl Pts',(-18.2061311342259,50.4788490602775,124.336917792434)) ;
#71495=CARTESIAN_POINT('Ctrl Pts',(-18.4467378517919,50.2988599799146,124.151872297986)) ;
#71496=CARTESIAN_POINT('Ctrl Pts',(-18.0368827272804,50.4920100539476,124.035219084609)) ;
#71497=CARTESIAN_POINT('Ctrl Pts',(-18.311368220634,50.3120209735847,123.910554390484)) ;
#71498=CARTESIAN_POINT('Ctrl Pts',(-17.9492027072533,50.5020062760529,123.787616040863)) ;
#71499=CARTESIAN_POINT('Ctrl Pts',(-18.2412163833771,50.32201719569,123.712463854449)) ;
#71500=CARTESIAN_POINT('Ctrl Pts',(-17.9063100733637,50.5120301155866,123.527712476807)) ;
#71501=CARTESIAN_POINT('Ctrl Pts',(-18.2069016114084,50.3320410352238,123.504545668271)) ;
#71502=CARTESIAN_POINT('Ctrl Pts',(-17.9093431973629,50.5252234375799,123.180991999699)) ;
#71503=CARTESIAN_POINT('Ctrl Pts',(-18.2093282776367,50.345234357217,123.227157652856)) ;
#71504=CARTESIAN_POINT('Ctrl Pts',(-18.027118283777,50.5418826093572,122.754212984447)) ;
#71505=CARTESIAN_POINT('Ctrl Pts',(-18.3035426189576,50.3618935289943,122.885745424795)) ;
#71506=CARTESIAN_POINT('Ctrl Pts',(-18.333937561739,50.5617927848429,122.323039035125)) ;
#71507=CARTESIAN_POINT('Ctrl Pts',(-18.5489966706976,50.38180370448,122.540800132755)) ;
#71508=CARTESIAN_POINT('Ctrl Pts',(-18.7684393921744,50.5816827726873,122.021820822919)) ;
#71509=CARTESIAN_POINT('Ctrl Pts',(-18.8965968570353,50.4016936923244,122.299823770032)) ;
#71510=CARTESIAN_POINT('Ctrl Pts',(-19.2825937715403,50.6016882207021,121.886677539595)) ;
#71511=CARTESIAN_POINT('Ctrl Pts',(-19.307919625913,50.4216991403392,122.191706067227)) ;
#71512=CARTESIAN_POINT('Ctrl Pts',(-19.8078113963263,50.6215246147294,121.934169205366)) ;
#71513=CARTESIAN_POINT('Ctrl Pts',(-19.7280952319297,50.4415355343665,122.229696987763)) ;
#71514=CARTESIAN_POINT('Ctrl Pts',(-20.2892513212485,50.6415324086261,122.159662815759)) ;
#71515=CARTESIAN_POINT('Ctrl Pts',(-20.1132481557937,50.4615433282632,122.410089630547)) ;
#71516=CARTESIAN_POINT('Ctrl Pts',(-20.6617398847741,50.66135904492,122.532541564671)) ;
#71517=CARTESIAN_POINT('Ctrl Pts',(-20.4112416638867,50.4813699645572,122.708392168977)) ;
#71518=CARTESIAN_POINT('Ctrl Pts',(-20.8871620269531,50.6813379878739,123.013304098428)) ;
#71519=CARTESIAN_POINT('Ctrl Pts',(-20.5915810553221,50.501348907511,123.093001677507)) ;
#71520=CARTESIAN_POINT('Ctrl Pts',(-20.9339369378857,50.701269789743,123.540918150504)) ;
#71521=CARTESIAN_POINT('Ctrl Pts',(-20.6290028531258,50.5212807093801,123.515093416669)) ;
#71522=CARTESIAN_POINT('Ctrl Pts',(-20.8002489892957,50.7210940902405,124.050742162796)) ;
#71523=CARTESIAN_POINT('Ctrl Pts',(-20.5220534268662,50.5411050098776,123.922954725086)) ;
#71524=CARTESIAN_POINT('Ctrl Pts',(-20.4959470937685,50.7411900915803,124.489434446394)) ;
#71525=CARTESIAN_POINT('Ctrl Pts',(-20.2786119963971,50.5612010112175,124.273908331322)) ;
#71526=CARTESIAN_POINT('Ctrl Pts',(-20.0674250455001,50.7609485076843,124.793529199864)) ;
#71527=CARTESIAN_POINT('Ctrl Pts',(-19.9357982255067,50.5809594273214,124.517186790158)) ;
#71528=CARTESIAN_POINT('Ctrl Pts',(-19.5529196248031,50.7810422005684,124.935512899744)) ;
#71529=CARTESIAN_POINT('Ctrl Pts',(-19.524171586782,50.6010531202055,124.630773511285)) ;
#71530=CARTESIAN_POINT('Ctrl Pts',(-19.2053312341041,50.7941531664751,124.907880339345)) ;
#71531=CARTESIAN_POINT('Ctrl Pts',(-19.2461441930599,50.6141640861122,124.608669210494)) ;
#71532=CARTESIAN_POINT('Ctrl Pts',(-19.035117438896,50.8008665412629,124.864312062334)) ;
#71533=CARTESIAN_POINT('Ctrl Pts',(-19.1099467513572,50.6208774609001,124.573813086965)) ;
#71534=CARTESIAN_POINT('',(-20.6544117723369,12.0237783230283,123.301689203239)) ;
#71535=CARTESIAN_POINT('Ctrl Pts',(-20.6544115797749,12.0237782093581,123.301688455234)) ;
#71536=CARTESIAN_POINT('Ctrl Pts',(-20.6751132995434,12.0362928130092,123.293550512105)) ;
#71537=CARTESIAN_POINT('Ctrl Pts',(-20.6957063040839,12.0487910861619,123.284611049605)) ;
#71538=CARTESIAN_POINT('Ctrl Pts',(-20.7158767772876,12.0611019792037,123.274999238965)) ;
#71539=CARTESIAN_POINT('Ctrl Pts',(-20.7358112078758,12.0732688054522,123.26549990942)) ;
#71540=CARTESIAN_POINT('Ctrl Pts',(-20.7553325868204,12.0852526121581,123.255343873335)) ;
#71541=CARTESIAN_POINT('Ctrl Pts',(-20.774148982094,12.0968882682071,123.24470604279)) ;
#71542=CARTESIAN_POINT('Ctrl Pts',(-20.7790756776112,12.0999348312529,123.24192074033)) ;
#71543=CARTESIAN_POINT('Ctrl Pts',(-20.7839541174359,12.102957526743,123.239102676279)) ;
#71544=CARTESIAN_POINT('Ctrl Pts',(-20.788779231699,12.1059533903454,123.236255555915)) ;
#71545=CARTESIAN_POINT('Ctrl Pts',(-20.808608031553,12.1182648873431,123.224555319035)) ;
#71546=CARTESIAN_POINT('Ctrl Pts',(-20.8282355576711,12.1305576883349,123.211948910434)) ;
#71547=CARTESIAN_POINT('Ctrl Pts',(-20.8472694739559,12.1426194691851,123.198544107178)) ;
#71548=CARTESIAN_POINT('Ctrl Pts',(-20.8615954260223,12.1516978160533,123.188454929207)) ;
#71549=CARTESIAN_POINT('Ctrl Pts',(-20.8755851620327,12.1606452915608,123.177914421792)) ;
#71550=CARTESIAN_POINT('Ctrl Pts',(-20.8890752031254,12.1693713464509,123.166987767337)) ;
#71551=CARTESIAN_POINT('',(-18.3268339991922,12.1788250889762,124.036972600407)) ;
#71552=CARTESIAN_POINT('Ctrl Pts',(-18.1733332732719,12.2002112739617,123.598774336477)) ;
#71553=CARTESIAN_POINT('Ctrl Pts',(-18.1437739434563,12.2192124780422,123.626890688012)) ;
#71554=CARTESIAN_POINT('Ctrl Pts',(-18.1155519840929,12.2380735843825,123.659034167815)) ;
#71555=CARTESIAN_POINT('Ctrl Pts',(-18.0788950768115,12.264782265653,123.716747867416)) ;
#71556=CARTESIAN_POINT('Ctrl Pts',(-18.0663998540908,12.2745789428676,123.741420731664)) ;
#71557=CARTESIAN_POINT('Ctrl Pts',(-18.0527323281464,12.2874752510621,123.784178421799)) ;
#71558=CARTESIAN_POINT('Ctrl Pts',(-18.049031605284,12.2917819347337,123.8016488575)) ;
#71559=CARTESIAN_POINT('Ctrl Pts',(-18.0469608922576,12.2970228146757,123.831943690158)) ;
#71560=CARTESIAN_POINT('Ctrl Pts',(-18.0473135809881,12.2985681111668,123.844453983307)) ;
#71561=CARTESIAN_POINT('Ctrl Pts',(-18.0497385762831,12.2996578525868,123.861380043343)) ;
#71562=CARTESIAN_POINT('Ctrl Pts',(-18.0505576652496,12.2998485070101,123.865811638863)) ;
#71563=CARTESIAN_POINT('Ctrl Pts',(-18.0527703707483,12.3000477727242,123.875497560335)) ;
#71564=CARTESIAN_POINT('Ctrl Pts',(-18.0542408074423,12.300011368751,123.880712238468)) ;
#71565=CARTESIAN_POINT('Ctrl Pts',(-18.0561492734575,12.2998090598907,123.886360179938)) ;
#71566=CARTESIAN_POINT('Ctrl Pts',(-18.0563249547583,12.2997892478978,123.886871506831)) ;
#71567=CARTESIAN_POINT('Ctrl Pts',(-18.0565108989679,12.2997670567988,123.887403881291)) ;
#71568=CARTESIAN_POINT('Ctrl Pts',(-18.0565185857082,12.2997661372984,123.887425873618)) ;
#71569=CARTESIAN_POINT('Ctrl Pts',(-18.0565331994726,12.2997643851054,123.887467655272)) ;
#71570=CARTESIAN_POINT('Ctrl Pts',(-18.0565401250457,12.2997635529941,123.887487443392)) ;
#71571=CARTESIAN_POINT('Ctrl Pts',(-18.0565502565831,12.2997623331508,123.887516373468)) ;
#71572=CARTESIAN_POINT('Ctrl Pts',(-18.0565534594976,12.2997619471482,123.887525516553)) ;
#71573=CARTESIAN_POINT('Ctrl Pts',(-18.0565590575015,12.2997612718528,123.887541492028)) ;
#71574=CARTESIAN_POINT('Ctrl Pts',(-18.0565614522309,12.2997609827666,123.88754832457)) ;
#71575=CARTESIAN_POINT('Ctrl Pts',(-18.0565663690132,12.2997603888004,123.887562349868)) ;
#71576=CARTESIAN_POINT('Ctrl Pts',(-18.0565688910754,12.2997600838969,123.887569542489)) ;
#71577=CARTESIAN_POINT('Ctrl Pts',(-18.0565752815213,12.2997593107477,123.887587763097)) ;
#71578=CARTESIAN_POINT('Ctrl Pts',(-18.0565791506111,12.2997588421077,123.887598790867)) ;
#71579=CARTESIAN_POINT('Ctrl Pts',(-18.0565942212527,12.2997570145979,123.887641730451)) ;
#71580=CARTESIAN_POINT('Ctrl Pts',(-18.0566054316885,12.2997556506893,123.887673638972)) ;
#71581=CARTESIAN_POINT('Ctrl Pts',(-18.0590015798815,12.2994631655,123.894486919769)) ;
#71582=CARTESIAN_POINT('Ctrl Pts',(-18.061830203414,12.298915038444,123.901065001398)) ;
#71583=CARTESIAN_POINT('Ctrl Pts',(-18.0701064049968,12.2968881910932,123.917270600894)) ;
#71584=CARTESIAN_POINT('Ctrl Pts',(-18.0760644154365,12.2950839853311,123.926456828537)) ;
#71585=CARTESIAN_POINT('Ctrl Pts',(-18.0926654304272,12.2894248879463,123.947565980743)) ;
#71586=CARTESIAN_POINT('Ctrl Pts',(-18.1040515527384,12.285054139982,123.958571881896)) ;
#71587=CARTESIAN_POINT('Ctrl Pts',(-18.1349180947271,12.2723955189041,123.982828648664)) ;
#71588=CARTESIAN_POINT('Ctrl Pts',(-18.155694410254,12.26318030131,123.994378655851)) ;
#71589=CARTESIAN_POINT('Ctrl Pts',(-18.2194310980166,12.2336621656688,124.021802848732)) ;
#71590=CARTESIAN_POINT('Ctrl Pts',(-18.2704827038226,12.2083681409552,124.033080779891)) ;
#71591=CARTESIAN_POINT('Ctrl Pts',(-18.3268339991922,12.1788250889762,124.036972600407)) ;
#71592=CARTESIAN_POINT('Ctrl Pts',(-18.3268329934248,12.1788261493768,124.036974575079)) ;
#71593=CARTESIAN_POINT('Ctrl Pts',(-18.3309561086821,12.1784521366068,124.044113579922)) ;
#71594=CARTESIAN_POINT('Ctrl Pts',(-18.335149729096,12.1780774444603,124.051211586361)) ;
#71595=CARTESIAN_POINT('Ctrl Pts',(-18.3423169557771,12.1774461337977,124.063073113184)) ;
#71596=CARTESIAN_POINT('Ctrl Pts',(-18.3452530035821,12.1771899809839,124.06785902791)) ;
#71597=CARTESIAN_POINT('Ctrl Pts',(-18.3498365787837,12.1767937826142,124.075218787483)) ;
#71598=CARTESIAN_POINT('Ctrl Pts',(-18.3514614724111,12.1766540296321,124.077806653189)) ;
#71599=CARTESIAN_POINT('Ctrl Pts',(-18.3547371233891,12.1763736859824,124.082981345011)) ;
#71600=CARTESIAN_POINT('Ctrl Pts',(-18.3563879496659,12.1762330952556,124.085568102145)) ;
#71601=CARTESIAN_POINT('Ctrl Pts',(-18.359959596429,12.1759303975391,124.091119499098)) ;
#71602=CARTESIAN_POINT('Ctrl Pts',(-18.3618834914386,12.175768251981,124.094082126548)) ;
#71603=CARTESIAN_POINT('Ctrl Pts',(-18.3670623375374,12.1753341801676,124.101983558783)) ;
#71604=CARTESIAN_POINT('Ctrl Pts',(-18.3703398205182,12.175061972512,124.106907469637)) ;
#71605=CARTESIAN_POINT('Ctrl Pts',(-18.3847847100382,12.1738731097679,124.128278263932)) ;
#71606=CARTESIAN_POINT('Ctrl Pts',(-18.3963085270288,12.1729521993781,124.144480537417)) ;
#71607=CARTESIAN_POINT('Ctrl Pts',(-18.4232925461838,12.1708620966218,124.18056531699)) ;
#71608=CARTESIAN_POINT('Ctrl Pts',(-18.4389773134463,12.1696945627848,124.200269661361)) ;
#71609=CARTESIAN_POINT('Ctrl Pts',(-18.4678172941385,12.1676312235368,124.23433555177)) ;
#71610=CARTESIAN_POINT('Ctrl Pts',(-18.4807330953577,12.1667338677983,124.248888783628)) ;
#71611=CARTESIAN_POINT('Ctrl Pts',(-18.4982848415437,12.1655482404027,124.267759375193)) ;
#71612=CARTESIAN_POINT('Ctrl Pts',(-18.5026213166717,12.1652579317476,124.272351409021)) ;
#71613=CARTESIAN_POINT('Ctrl Pts',(-18.5107463421741,12.1647187963383,124.280825666637)) ;
#71614=CARTESIAN_POINT('Ctrl Pts',(-18.5145257195718,12.1644699057803,124.284716476236)) ;
#71615=CARTESIAN_POINT('Ctrl Pts',(-18.5222714957369,12.1639636048236,124.292587469649)) ;
#71616=CARTESIAN_POINT('Ctrl Pts',(-18.526239649542,12.1637062151148,124.296565757538)) ;
#71617=CARTESIAN_POINT('Ctrl Pts',(-18.5354269798619,12.1631147968241,124.305653171346)) ;
#71618=CARTESIAN_POINT('Ctrl Pts',(-18.5406643862709,12.1627809370258,124.310743587654)) ;
#71619=CARTESIAN_POINT('Ctrl Pts',(-18.5568490594105,12.1617591296451,124.326200513915)) ;
#71620=CARTESIAN_POINT('Ctrl Pts',(-18.5679395411594,12.1610726680707,124.336415145548)) ;
#71621=CARTESIAN_POINT('Ctrl Pts',(-18.5833701166089,12.160135177217,124.350119548717)) ;
#71622=CARTESIAN_POINT('Ctrl Pts',(-18.5875526761695,12.1598827561002,124.353784584154)) ;
#71623=CARTESIAN_POINT('Ctrl Pts',(-18.5987779267441,12.1592095596942,124.363489231507)) ;
#71624=CARTESIAN_POINT('Ctrl Pts',(-18.605863636986,12.1587890311453,124.369478554744)) ;
#71625=CARTESIAN_POINT('Ctrl Pts',(-18.6339450219884,12.1571381352803,124.392683823556)) ;
#71626=CARTESIAN_POINT('Ctrl Pts',(-18.6554325503652,12.1559086064401,124.409292637778)) ;
#71627=CARTESIAN_POINT('Ctrl Pts',(-18.6866563009285,12.1541580311278,124.431841495251)) ;
#71628=CARTESIAN_POINT('Ctrl Pts',(-18.6959590741923,12.1536408492618,124.438368536798)) ;
#71629=CARTESIAN_POINT('Ctrl Pts',(-18.7110045839349,12.1528107345973,124.448621541144)) ;
#71630=CARTESIAN_POINT('Ctrl Pts',(-18.7166911876344,12.1524984057569,124.452428763065)) ;
#71631=CARTESIAN_POINT('Ctrl Pts',(-18.7276119130962,12.1519011693592,124.459611096525)) ;
#71632=CARTESIAN_POINT('Ctrl Pts',(-18.7328405599809,12.1516163314452,124.462994165875)) ;
#71633=CARTESIAN_POINT('Ctrl Pts',(-18.7416520111582,12.1511380934684,124.468602434594)) ;
#71634=CARTESIAN_POINT('Ctrl Pts',(-18.745221195541,12.150944861499,124.470848832909)) ;
#71635=CARTESIAN_POINT('Ctrl Pts',(-18.7531205419484,12.150518239497,124.475764944144)) ;
#71636=CARTESIAN_POINT('Ctrl Pts',(-18.7574557686962,12.1502847897276,124.478426371889)) ;
#71637=CARTESIAN_POINT('Ctrl Pts',(-18.769540168913,12.1496358997812,124.485743884565)) ;
#71638=CARTESIAN_POINT('Ctrl Pts',(-18.7773237713421,12.1492200402206,124.490342467398)) ;
#71639=CARTESIAN_POINT('Ctrl Pts',(-18.8214619475145,12.1468732364854,124.515777614443)) ;
#71640=CARTESIAN_POINT('Ctrl Pts',(-18.8587960674524,12.1449299126189,124.53486009634)) ;
#71641=CARTESIAN_POINT('Ctrl Pts',(-18.9139729955992,12.1421242821054,124.559648928632)) ;
#71642=CARTESIAN_POINT('Ctrl Pts',(-18.9310965056275,12.1412627503848,124.566887306796)) ;
#71643=CARTESIAN_POINT('Ctrl Pts',(-18.9564533001242,12.1400023439097,124.576945490497)) ;
#71644=CARTESIAN_POINT('Ctrl Pts',(-18.9645646880267,12.1396013872073,124.580065504982)) ;
#71645=CARTESIAN_POINT('Ctrl Pts',(-18.9791159272324,12.1388860855064,124.585489072915)) ;
#71646=CARTESIAN_POINT('Ctrl Pts',(-18.9855433853753,12.1385715029736,124.587824837599)) ;
#71647=CARTESIAN_POINT('Ctrl Pts',(-18.995936113443,12.1380650310906,124.591505333423)) ;
#71648=CARTESIAN_POINT('Ctrl Pts',(-18.9998895246317,12.1378728744833,124.592883087366)) ;
#71649=CARTESIAN_POINT('Ctrl Pts',(-19.0076657347591,12.1374958891479,124.595549341794)) ;
#71650=CARTESIAN_POINT('Ctrl Pts',(-19.0114879973792,12.1373110507774,124.596839249442)) ;
#71651=CARTESIAN_POINT('Ctrl Pts',(-19.0203630306894,12.1368829207235,124.599786549263)) ;
#71652=CARTESIAN_POINT('Ctrl Pts',(-19.0254202715219,12.1366397478072,124.601430248465)) ;
#71653=CARTESIAN_POINT('Ctrl Pts',(-19.0407068717453,12.1359070071212,124.606291055064)) ;
#71654=CARTESIAN_POINT('Ctrl Pts',(-19.0509673168084,12.1354182904964,124.609408861383)) ;
#71655=CARTESIAN_POINT('Ctrl Pts',(-19.0983481678484,12.1331745141152,124.62314289154)) ;
#71656=CARTESIAN_POINT('Ctrl Pts',(-19.135907308955,12.1314352924154,124.63216766381)) ;
#71657=CARTESIAN_POINT('Ctrl Pts',(-19.185832039001,12.12913802557,124.641742810519)) ;
#71658=CARTESIAN_POINT('Ctrl Pts',(-19.1978732237918,12.1285845297001,124.643869541303)) ;
#71659=CARTESIAN_POINT('Ctrl Pts',(-19.2155834909889,12.1277695243768,124.646730277972)) ;
#71660=CARTESIAN_POINT('Ctrl Pts',(-19.2212295206173,12.1275095723486,124.64760260689)) ;
#71661=CARTESIAN_POINT('Ctrl Pts',(-19.2303371967085,12.1270899040682,124.648945909585)) ;
#71662=CARTESIAN_POINT('Ctrl Pts',(-19.2337951920354,12.1269304872354,124.649441131769)) ;
#71663=CARTESIAN_POINT('Ctrl Pts',(-19.2404037493357,12.1266256527697,124.650359294679)) ;
#71664=CARTESIAN_POINT('Ctrl Pts',(-19.243553938108,12.1264802680291,124.650784725532)) ;
#71665=CARTESIAN_POINT('Ctrl Pts',(-19.2491898898548,12.1262200146339,124.651523977672)) ;
#71666=CARTESIAN_POINT('Ctrl Pts',(-19.2516750402328,12.1261052056308,124.651842350628)) ;
#71667=CARTESIAN_POINT('Ctrl Pts',(-19.2567554186499,12.1258703922224,124.652477679522)) ;
#71668=CARTESIAN_POINT('Ctrl Pts',(-19.259350716869,12.1257503797777,124.652793969034)) ;
#71669=CARTESIAN_POINT('Ctrl Pts',(-19.2666646898003,12.1254119951527,124.653662045682)) ;
#71670=CARTESIAN_POINT('Ctrl Pts',(-19.2713855323837,12.1251933830539,124.654195075941)) ;
#71671=CARTESIAN_POINT('Ctrl Pts',(-19.2980125716004,12.123959212496,124.657047898168)) ;
#71672=CARTESIAN_POINT('Ctrl Pts',(-19.3199737148664,12.1229365148661,124.65881517204)) ;
#71673=CARTESIAN_POINT('Ctrl Pts',(-19.3583755690349,12.1211461929445,124.66088580607)) ;
#71674=CARTESIAN_POINT('Ctrl Pts',(-19.3747972379329,12.1203803250949,124.661446876312)) ;
#71675=CARTESIAN_POINT('Ctrl Pts',(-19.4025984884849,12.1190879848973,124.661848301862)) ;
#71676=CARTESIAN_POINT('Ctrl Pts',(-19.4139735268802,12.1185603883619,124.661857277545)) ;
#71677=CARTESIAN_POINT('Ctrl Pts',(-19.4308582588047,12.1177796885816,124.661640122708)) ;
#71678=CARTESIAN_POINT('Ctrl Pts',(-19.4363688273304,12.1175252776935,124.661532795761)) ;
#71679=CARTESIAN_POINT('Ctrl Pts',(-19.4463925817608,12.1170632365372,124.661271236795)) ;
#71680=CARTESIAN_POINT('Ctrl Pts',(-19.4509059776786,12.1168554636031,124.661128987644)) ;
#71681=CARTESIAN_POINT('Ctrl Pts',(-19.4581089955715,12.1165243081718,124.660862892255)) ;
#71682=CARTESIAN_POINT('Ctrl Pts',(-19.4607991489641,12.1164007259829,124.660754807863)) ;
#71683=CARTESIAN_POINT('Ctrl Pts',(-19.4660166369468,12.1161612255412,124.660528294707)) ;
#71684=CARTESIAN_POINT('Ctrl Pts',(-19.4685440016305,12.1160452947918,124.660410882346)) ;
#71685=CARTESIAN_POINT('Ctrl Pts',(-19.4744209069952,12.1157759099962,124.660119978235)) ;
#71686=CARTESIAN_POINT('Ctrl Pts',(-19.4777701431751,12.1156225319265,124.659940676791)) ;
#71687=CARTESIAN_POINT('Ctrl Pts',(-19.4879808771949,12.1151553471206,124.659352821464)) ;
#71688=CARTESIAN_POINT('Ctrl Pts',(-19.4948397796812,12.1148420982047,124.658901149022)) ;
#71689=CARTESIAN_POINT('Ctrl Pts',(-19.5395975418219,12.1128010645601,124.655582770018)) ;
#71690=CARTESIAN_POINT('Ctrl Pts',(-19.5773517629285,12.1110970236261,124.651045488828)) ;
#71691=CARTESIAN_POINT('Ctrl Pts',(-19.6243814208216,12.1089411400518,124.643204471514)) ;
#71692=CARTESIAN_POINT('Ctrl Pts',(-19.6339031091612,12.1085028465813,124.641503156803)) ;
#71693=CARTESIAN_POINT('Ctrl Pts',(-19.6482180187781,12.1078404098274,124.638773587489)) ;
#71694=CARTESIAN_POINT('Ctrl Pts',(-19.6530265275211,12.1076172964537,124.637827360772)) ;
#71695=CARTESIAN_POINT('Ctrl Pts',(-19.6609096731925,12.1072504731384,124.636227891222)) ;
#71696=CARTESIAN_POINT('Ctrl Pts',(-19.6639876373078,12.1071069848894,124.635591283902)) ;
#71697=CARTESIAN_POINT('Ctrl Pts',(-19.6696692547856,12.1068416198828,124.634393806143)) ;
#71698=CARTESIAN_POINT('Ctrl Pts',(-19.6722735808662,12.1067197881108,124.633836210074)) ;
#71699=CARTESIAN_POINT('Ctrl Pts',(-19.6772531681451,12.1064864619113,124.632753405863)) ;
#71700=CARTESIAN_POINT('Ctrl Pts',(-19.679628717628,12.1063749867977,124.632229578891)) ;
#71701=CARTESIAN_POINT('Ctrl Pts',(-19.684523120746,12.1061449682624,124.631135333513)) ;
#71702=CARTESIAN_POINT('Ctrl Pts',(-19.6870417652005,12.1060264134561,124.630564036756)) ;
#71703=CARTESIAN_POINT('Ctrl Pts',(-19.6942618608993,12.1056860159488,124.628902779674)) ;
#71704=CARTESIAN_POINT('Ctrl Pts',(-19.698958780763,12.1054639154586,124.627793394794)) ;
#71705=CARTESIAN_POINT('Ctrl Pts',(-19.7311424377226,12.103937583566,124.619994749598)) ;
#71706=CARTESIAN_POINT('Ctrl Pts',(-19.7584012552096,12.1026208615476,124.612401345337)) ;
#71707=CARTESIAN_POINT('Ctrl Pts',(-19.8078142985598,12.100211998718,124.596811287358)) ;
#71708=CARTESIAN_POINT('Ctrl Pts',(-19.830046894039,12.0991213656254,124.589100324975)) ;
#71709=CARTESIAN_POINT('Ctrl Pts',(-19.8577117655564,12.0977581546964,124.578621401988)) ;
#71710=CARTESIAN_POINT('Ctrl Pts',(-19.863359027879,12.0974795315819,124.576435272909)) ;
#71711=CARTESIAN_POINT('Ctrl Pts',(-19.872219293051,12.0970418066097,124.572931105043)) ;
#71712=CARTESIAN_POINT('Ctrl Pts',(-19.8754430554125,12.0968824207354,124.571640571314)) ;
#71713=CARTESIAN_POINT('Ctrl Pts',(-19.8819030589345,12.0965627736227,124.569023223501)) ;
#71714=CARTESIAN_POINT('Ctrl Pts',(-19.885139192205,12.0964025158514,124.567696226204)) ;
#71715=CARTESIAN_POINT('Ctrl Pts',(-19.8883899053704,12.0962413949055,124.56634728485)) ;
#71716=CARTESIAN_POINT('Ctrl Pts',(-19.8884100912478,12.096240394391,124.56633890774)) ;
#71717=CARTESIAN_POINT('Ctrl Pts',(-19.8884505059743,12.0962383912212,124.566322134444)) ;
#71718=CARTESIAN_POINT('Ctrl Pts',(-19.8884707355008,12.0962373885322,124.566313737975)) ;
#71719=CARTESIAN_POINT('Ctrl Pts',(-19.8885112400915,12.0962353808862,124.566296924886)) ;
#71720=CARTESIAN_POINT('Ctrl Pts',(-19.8885315141901,12.0962343759769,124.566288508666)) ;
#71721=CARTESIAN_POINT('Ctrl Pts',(-19.8885721091959,12.096232363827,124.56627165554)) ;
#71722=CARTESIAN_POINT('Ctrl Pts',(-19.8885924305321,12.0962313565652,124.566263218454)) ;
#71723=CARTESIAN_POINT('Ctrl Pts',(-19.8886331225267,12.0962293395857,124.566246322543)) ;
#71724=CARTESIAN_POINT('Ctrl Pts',(-19.8886534916079,12.0962283299461,124.566237864371)) ;
#71725=CARTESIAN_POINT('Ctrl Pts',(-19.8886942795243,12.0962263081895,124.566220926102)) ;
#71726=CARTESIAN_POINT('Ctrl Pts',(-19.8887146995792,12.0962252960121,124.566212445494)) ;
#71727=CARTESIAN_POINT('Ctrl Pts',(-19.8887555907354,12.0962232691156,124.566195461807)) ;
#71728=CARTESIAN_POINT('Ctrl Pts',(-19.8887760621694,12.0962222543801,124.566186958586)) ;
#71729=CARTESIAN_POINT('Ctrl Pts',(-19.8888170578738,12.0962202222786,124.566169928919)) ;
#71730=CARTESIAN_POINT('Ctrl Pts',(-19.8888375826562,12.0962192048873,124.566161402256)) ;
#71731=CARTESIAN_POINT('Ctrl Pts',(-19.8888786872779,12.0962171673641,124.566144324774)) ;
#71732=CARTESIAN_POINT('Ctrl Pts',(-19.8888992666296,12.0962161472564,124.566135774153)) ;
#71733=CARTESIAN_POINT('Ctrl Pts',(-19.8889404823842,12.0962141042014,124.566118647913)) ;
#71734=CARTESIAN_POINT('Ctrl Pts',(-19.8889611182149,12.0962130812825,124.566110072529)) ;
#71735=CARTESIAN_POINT('Ctrl Pts',(-19.8890024476845,12.0962110325677,124.566092896439)) ;
#71736=CARTESIAN_POINT('Ctrl Pts',(-19.8890231420417,12.096210006736,124.566084295431)) ;
#71737=CARTESIAN_POINT('Ctrl Pts',(-19.8890645907982,12.0962079520848,124.566067067152)) ;
#71738=CARTESIAN_POINT('Ctrl Pts',(-19.8890853443253,12.0962069233084,124.56605844024)) ;
#71739=CARTESIAN_POINT('Ctrl Pts',(-19.8891269129884,12.0962048626899,124.566041159492)) ;
#71740=CARTESIAN_POINT('Ctrl Pts',(-19.8891477280691,12.0962038308505,124.566032505674)) ;
#71741=CARTESIAN_POINT('Ctrl Pts',(-19.8891894207076,12.0962017640628,124.566015170742)) ;
#71742=CARTESIAN_POINT('Ctrl Pts',(-19.8892102988711,12.0962007290844,124.566006489371)) ;
#71743=CARTESIAN_POINT('Ctrl Pts',(-19.889252119754,12.0961986559157,124.565989098456)) ;
#71744=CARTESIAN_POINT('Ctrl Pts',(-19.8892730620161,12.0961976177479,124.565980389097)) ;
#71745=CARTESIAN_POINT('Ctrl Pts',(-19.8893150125022,12.0961955381305,124.565962941608)) ;
#71746=CARTESIAN_POINT('Ctrl Pts',(-19.8893360210389,12.0961944966653,124.565954203344)) ;
#71747=CARTESIAN_POINT('Ctrl Pts',(-19.8893781051252,12.0961924104008,124.565936697595)) ;
#71748=CARTESIAN_POINT('Ctrl Pts',(-19.8893991813962,12.0961913655658,124.565927929805)) ;
#71749=CARTESIAN_POINT('Ctrl Pts',(-19.8894414030598,12.0961892724569,124.565910364114)) ;
#71750=CARTESIAN_POINT('Ctrl Pts',(-19.8894625481686,12.0961882241971,124.565901566326)) ;
#71751=CARTESIAN_POINT('Ctrl Pts',(-19.8895049100727,12.0961861241116,124.565883939559)) ;
#71752=CARTESIAN_POINT('Ctrl Pts',(-19.8895261255919,12.096185072349,124.565875111105)) ;
#71753=CARTESIAN_POINT('Ctrl Pts',(-19.8895686279618,12.0961829652752,124.56585742314)) ;
#71754=CARTESIAN_POINT('Ctrl Pts',(-19.8895899168957,12.0961819098608,124.565848562757)) ;
#71755=CARTESIAN_POINT('Ctrl Pts',(-19.8896325689494,12.0961797953417,124.565830809729)) ;
#71756=CARTESIAN_POINT('Ctrl Pts',(-19.8896539305731,12.0961787363111,124.565821917703)) ;
#71757=CARTESIAN_POINT('Ctrl Pts',(-19.8896967300142,12.0961766144602,124.56580410054)) ;
#71758=CARTESIAN_POINT('Ctrl Pts',(-19.8897181674514,12.0961755516586,124.565795175556)) ;
#71759=CARTESIAN_POINT('Ctrl Pts',(-19.8897611191027,12.0961734222365,124.56577729222)) ;
#71760=CARTESIAN_POINT('Ctrl Pts',(-19.8897826338468,12.0961723555896,124.565768333642)) ;
#71761=CARTESIAN_POINT('Ctrl Pts',(-19.8898257416592,12.0961702184002,124.565750382458)) ;
#71762=CARTESIAN_POINT('Ctrl Pts',(-19.8898473348348,12.0961691478522,124.565741389802)) ;
#71763=CARTESIAN_POINT('Ctrl Pts',(-19.8898906012064,12.0961670027762,124.565723369739)) ;
#71764=CARTESIAN_POINT('Ctrl Pts',(-19.8899122745324,12.0961659282417,124.565714342273)) ;
#71765=CARTESIAN_POINT('Ctrl Pts',(-19.8899557030499,12.096163775101,124.565696251807)) ;
#71766=CARTESIAN_POINT('Ctrl Pts',(-19.8899774579468,12.0961626965094,124.565687188923)) ;
#71767=CARTESIAN_POINT('Ctrl Pts',(-19.8900132216144,12.0961609233627,124.565672288932)) ;
#71768=CARTESIAN_POINT('Ctrl Pts',(-19.8900272315851,12.0961602287519,124.565666451747)) ;
#71769=CARTESIAN_POINT('Ctrl Pts',(-19.8900553823775,12.0961588330374,124.565654722257)) ;
#71770=CARTESIAN_POINT('Ctrl Pts',(-19.8900695230093,12.096158131943,124.565648830025)) ;
#71771=CARTESIAN_POINT('Ctrl Pts',(-19.8900979393219,12.096156723053,124.565636988675)) ;
#71772=CARTESIAN_POINT('Ctrl Pts',(-19.890112213525,12.0961560153306,124.565631040167)) ;
#71773=CARTESIAN_POINT('Ctrl Pts',(-19.8901408985717,12.0961545931055,124.565619085583)) ;
#71774=CARTESIAN_POINT('Ctrl Pts',(-19.8901553106431,12.0961538785419,124.56561307899)) ;
#71775=CARTESIAN_POINT('Ctrl Pts',(-19.8901842732507,12.0961524425436,124.565601007459)) ;
#71776=CARTESIAN_POINT('Ctrl Pts',(-19.8901988254819,12.096151721025,124.565594941808)) ;
#71777=CARTESIAN_POINT('Ctrl Pts',(-19.8902280740247,12.0961502708381,124.5655827498)) ;
#71778=CARTESIAN_POINT('Ctrl Pts',(-19.890242768038,12.0961495422838,124.565576624395)) ;
#71779=CARTESIAN_POINT('Ctrl Pts',(-19.8902723027371,12.0961480778969,124.565564311781)) ;
#71780=CARTESIAN_POINT('Ctrl Pts',(-19.8902871439326,12.0961473420391,124.565558124353)) ;
#71781=CARTESIAN_POINT('Ctrl Pts',(-19.8903169751637,12.0961458629374,124.565545686767)) ;
#71782=CARTESIAN_POINT('Ctrl Pts',(-19.890331965887,12.0961451196595,124.565539436317)) ;
#71783=CARTESIAN_POINT('Ctrl Pts',(-19.8903621001897,12.0961436255185,124.565526870992)) ;
#71784=CARTESIAN_POINT('Ctrl Pts',(-19.8903772432713,12.0961428746801,124.565520556319)) ;
#71785=CARTESIAN_POINT('Ctrl Pts',(-19.8904076862415,12.0961413652218,124.56550786088)) ;
#71786=CARTESIAN_POINT('Ctrl Pts',(-19.8904229853098,12.0961406066427,124.565501480449)) ;
#71787=CARTESIAN_POINT('Ctrl Pts',(-19.8904537435082,12.0961390815415,124.565488652116)) ;
#71788=CARTESIAN_POINT('Ctrl Pts',(-19.8904692022185,12.0961383150403,124.565482204381)) ;
#71789=CARTESIAN_POINT('Ctrl Pts',(-19.8905002824576,12.096136773958,124.565469240268)) ;
#71790=CARTESIAN_POINT('Ctrl Pts',(-19.8905159044465,12.0961359993541,124.565462723689)) ;
#71791=CARTESIAN_POINT('Ctrl Pts',(-19.8905473146054,12.0961344418996,124.565449620462)) ;
#71792=CARTESIAN_POINT('Ctrl Pts',(-19.8905631030922,12.0961336590332,124.565443033674)) ;
#71793=CARTESIAN_POINT('Ctrl Pts',(-19.8905948499206,12.0961320848713,124.56542978847)) ;
#71794=CARTESIAN_POINT('Ctrl Pts',(-19.8906108085725,12.0961312935604,124.565423129917)) ;
#71795=CARTESIAN_POINT('Ctrl Pts',(-19.8906428998161,12.0961297023067,124.565409739454)) ;
#71796=CARTESIAN_POINT('Ctrl Pts',(-19.8906590321436,12.0961289023769,124.565403007647)) ;
#71797=CARTESIAN_POINT('Ctrl Pts',(-19.8906914750132,12.0961272936733,124.565389468866)) ;
#71798=CARTESIAN_POINT('Ctrl Pts',(-19.8907077848372,12.096126484935,124.565382662184)) ;
#71799=CARTESIAN_POINT('Ctrl Pts',(-19.8907405852627,12.096124858487,124.565368972558)) ;
#71800=CARTESIAN_POINT('Ctrl Pts',(-19.8907570772909,12.0961240407065,124.565362089009)) ;
#71801=CARTESIAN_POINT('Ctrl Pts',(-19.8907902471995,12.0961223959221,124.565348243504)) ;
#71802=CARTESIAN_POINT('Ctrl Pts',(-19.8908069237545,12.0961215689839,124.565341282092)) ;
#71803=CARTESIAN_POINT('Ctrl Pts',(-19.8908404664989,12.0961199056965,124.565327279253)) ;
#71804=CARTESIAN_POINT('Ctrl Pts',(-19.8908573330806,12.0961190693277,124.565320237652)) ;
#71805=CARTESIAN_POINT('Ctrl Pts',(-19.8908912602615,12.0961173869614,124.565306072578)) ;
#71806=CARTESIAN_POINT('Ctrl Pts',(-19.8909083199804,12.0961165410075,124.565298949461)) ;
#71807=CARTESIAN_POINT('Ctrl Pts',(-19.8909426362466,12.0961148393312,124.56528462015)) ;
#71808=CARTESIAN_POINT('Ctrl Pts',(-19.8909598946158,12.0961139835185,124.565277413184)) ;
#71809=CARTESIAN_POINT('Ctrl Pts',(-19.8909946128312,12.0961122618939,124.565262914202)) ;
#71810=CARTESIAN_POINT('Ctrl Pts',(-19.8910120725937,12.096111396086,124.565255622211)) ;
#71811=CARTESIAN_POINT('Ctrl Pts',(-19.8932200461518,12.0960019048985,124.564333413046)) ;
#71812=CARTESIAN_POINT('Ctrl Pts',(-19.8954079518662,12.095893342643,124.563412256993)) ;
#71813=CARTESIAN_POINT('Ctrl Pts',(-19.9018327066309,12.0955743452035,124.560685722707)) ;
#71814=CARTESIAN_POINT('Ctrl Pts',(-19.9060622234605,12.095364080751,124.558863153119)) ;
#71815=CARTESIAN_POINT('Ctrl Pts',(-19.9172083501097,12.0948091825736,124.553986887343)) ;
#71816=CARTESIAN_POINT('Ctrl Pts',(-19.9241075017011,12.0944649162962,124.55089373742)) ;
#71817=CARTESIAN_POINT('Ctrl Pts',(-19.947189550004,12.0933098005277,124.540292637351)) ;
#71818=CARTESIAN_POINT('Ctrl Pts',(-19.9632397016889,12.0925011604031,124.532500894411)) ;
#71819=CARTESIAN_POINT('Ctrl Pts',(-19.9997021501647,12.0906432498922,124.513824984359)) ;
#71820=CARTESIAN_POINT('Ctrl Pts',(-20.0199899485757,12.0895932315963,124.502712505895)) ;
#71821=CARTESIAN_POINT('Ctrl Pts',(-20.0451574487418,12.0882630667123,124.488004994032)) ;
#71822=CARTESIAN_POINT('Ctrl Pts',(-20.0503351268551,12.0879879339241,124.484928824601)) ;
#71823=CARTESIAN_POINT('Ctrl Pts',(-20.0592641580973,12.087510822128,124.479536211108)) ;
#71824=CARTESIAN_POINT('Ctrl Pts',(-20.0630258648687,12.0873090005106,124.47723711304)) ;
#71825=CARTESIAN_POINT('Ctrl Pts',(-20.0707724660396,12.0868916700692,124.472446034137)) ;
#71826=CARTESIAN_POINT('Ctrl Pts',(-20.0747556264624,12.0866761410594,124.469951382956)) ;
#71827=CARTESIAN_POINT('Ctrl Pts',(-20.0829831587476,12.0862289818328,124.464733651904)) ;
#71828=CARTESIAN_POINT('Ctrl Pts',(-20.0872253118421,12.0859973280671,124.462007232492)) ;
#71829=CARTESIAN_POINT('Ctrl Pts',(-20.0977563432511,12.0854195367764,124.455148569015)) ;
#71830=CARTESIAN_POINT('Ctrl Pts',(-20.1040246172856,12.0850731844949,124.450985070618)) ;
#71831=CARTESIAN_POINT('Ctrl Pts',(-20.1253685275516,12.083885700615,124.436528624841)) ;
#71832=CARTESIAN_POINT('Ctrl Pts',(-20.1402560706855,12.0830432374429,124.425962206619)) ;
#71833=CARTESIAN_POINT('Ctrl Pts',(-20.1608000932679,12.0818640137746,124.410693635432)) ;
#71834=CARTESIAN_POINT('Ctrl Pts',(-20.1666546517558,12.0815260381859,124.406261847004)) ;
#71835=CARTESIAN_POINT('Ctrl Pts',(-20.1766176495245,12.0809479577298,124.398581028828)) ;
#71836=CARTESIAN_POINT('Ctrl Pts',(-20.1807453202545,12.0807075591967,124.395357304067)) ;
#71837=CARTESIAN_POINT('Ctrl Pts',(-20.1890187257961,12.0802237303642,124.388811619601)) ;
#71838=CARTESIAN_POINT('Ctrl Pts',(-20.1931637870648,12.0799803109458,124.385488982202)) ;
#71839=CARTESIAN_POINT('Ctrl Pts',(-20.1980454916039,12.0796923303333,124.381524480264)) ;
#71840=CARTESIAN_POINT('Ctrl Pts',(-20.1988027142953,12.0796476230646,124.380908055126)) ;
#71841=CARTESIAN_POINT('Ctrl Pts',(-20.2005462007064,12.0795445984949,124.379485351754)) ;
#71842=CARTESIAN_POINT('Ctrl Pts',(-20.2015319558203,12.0794862846559,124.378678451714)) ;
#71843=CARTESIAN_POINT('Ctrl Pts',(-20.2033067724417,12.0793811744691,124.377221120535)) ;
#71844=CARTESIAN_POINT('Ctrl Pts',(-20.2040962724662,12.0793343755022,124.376571225431)) ;
#71845=CARTESIAN_POINT('Ctrl Pts',(-20.2070796773395,12.0791573668663,124.374109219249)) ;
#71846=CARTESIAN_POINT('Ctrl Pts',(-20.2092681907218,12.0790271876121,124.372290586679)) ;
#71847=CARTESIAN_POINT('Ctrl Pts',(-20.2227467037841,12.0782233181007,124.361012050794)) ;
#71848=CARTESIAN_POINT('Ctrl Pts',(-20.2338749828313,12.0775503409761,124.351360674119)) ;
#71849=CARTESIAN_POINT('Ctrl Pts',(-20.2557121074218,12.0762081999463,124.331734804513)) ;
#71850=CARTESIAN_POINT('Ctrl Pts',(-20.2664215418767,12.075539144723,124.321764438779)) ;
#71851=CARTESIAN_POINT('Ctrl Pts',(-20.279945206364,12.0746787217884,124.308723421208)) ;
#71852=CARTESIAN_POINT('Ctrl Pts',(-20.2829225436843,12.0744883010146,124.305823546296)) ;
#71853=CARTESIAN_POINT('Ctrl Pts',(-20.2911382071323,12.0739600312075,124.297741397543)) ;
#71854=CARTESIAN_POINT('Ctrl Pts',(-20.296345248864,12.0736220001745,124.292527580215)) ;
#71855=CARTESIAN_POINT('Ctrl Pts',(-20.3085062999761,12.0728246403682,124.280133436177)) ;
#71856=CARTESIAN_POINT('Ctrl Pts',(-20.3154208739859,12.0723650571799,124.272915146482)) ;
#71857=CARTESIAN_POINT('Ctrl Pts',(-20.3298226096132,12.0713941369018,124.257515249955)) ;
#71858=CARTESIAN_POINT('Ctrl Pts',(-20.337288955113,12.070882556332,124.249315376395)) ;
#71859=CARTESIAN_POINT('Ctrl Pts',(-20.3604436677817,12.0692712293282,124.223195965355)) ;
#71860=CARTESIAN_POINT('Ctrl Pts',(-20.3757297246262,12.0681712569354,124.20492667103)) ;
#71861=CARTESIAN_POINT('Ctrl Pts',(-20.3937476135386,12.0668338044131,124.182097412825)) ;
#71862=CARTESIAN_POINT('Ctrl Pts',(-20.3969844870212,12.0665918185485,124.177942456214)) ;
#71863=CARTESIAN_POINT('Ctrl Pts',(-20.4028076011051,12.0661533702789,124.170369472117)) ;
#71864=CARTESIAN_POINT('Ctrl Pts',(-20.4054027039292,12.0659568257136,124.166958366656)) ;
#71865=CARTESIAN_POINT('Ctrl Pts',(-20.4104438072535,12.0655727692254,124.160260935774)) ;
#71866=CARTESIAN_POINT('Ctrl Pts',(-20.412891297502,12.0653852443372,124.156975799786)) ;
#71867=CARTESIAN_POINT('Ctrl Pts',(-20.4153869236975,12.0651929285345,124.153591453652)) ;
#71868=CARTESIAN_POINT('Ctrl Pts',(-20.4154512373072,12.0651879716971,124.153504213507)) ;
#71869=CARTESIAN_POINT('Ctrl Pts',(-20.4155837796079,12.065177754714,124.153324373518)) ;
#71870=CARTESIAN_POINT('Ctrl Pts',(-20.4156520067771,12.06517249459,124.153231772741)) ;
#71871=CARTESIAN_POINT('Ctrl Pts',(-20.4157927131427,12.0651616447619,124.15304074495)) ;
#71872=CARTESIAN_POINT('Ctrl Pts',(-20.4158651907121,12.0651560550728,124.152942316683)) ;
#71873=CARTESIAN_POINT('Ctrl Pts',(-20.41601476633,12.0651445173581,124.152739122883)) ;
#71874=CARTESIAN_POINT('Ctrl Pts',(-20.4160918624688,12.0651385693522,124.15263435594)) ;
#71875=CARTESIAN_POINT('Ctrl Pts',(-20.41625107805,12.065126283532,124.152417925061)) ;
#71876=CARTESIAN_POINT('Ctrl Pts',(-20.4163331952535,12.0651199457425,124.152306259526)) ;
#71877=CARTESIAN_POINT('Ctrl Pts',(-20.4165028930751,12.0651068459312,124.152075418696)) ;
#71878=CARTESIAN_POINT('Ctrl Pts',(-20.4165904711245,12.0651000839356,124.151956241505)) ;
#71879=CARTESIAN_POINT('Ctrl Pts',(-20.4167715711197,12.0650860980831,124.151709706921)) ;
#71880=CARTESIAN_POINT('Ctrl Pts',(-20.4168650901363,12.0650788742523,124.151582347246)) ;
#71881=CARTESIAN_POINT('Ctrl Pts',(-20.4170585962738,12.0650639236198,124.151318714486)) ;
#71882=CARTESIAN_POINT('Ctrl Pts',(-20.4171585798546,12.0650561968585,124.151182438921)) ;
#71883=CARTESIAN_POINT('Ctrl Pts',(-20.4173655861165,12.0650401955187,124.150900173625)) ;
#71884=CARTESIAN_POINT('Ctrl Pts',(-20.4174726047053,12.0650319209845,124.150754180954)) ;
#71885=CARTESIAN_POINT('Ctrl Pts',(-20.4176943019083,12.0650147752497,124.150451608138)) ;
#71886=CARTESIAN_POINT('Ctrl Pts',(-20.4178089758365,12.0650059040936,124.150295024435)) ;
#71887=CARTESIAN_POINT('Ctrl Pts',(-20.4180466577821,12.0649875119879,124.149970318471)) ;
#71888=CARTESIAN_POINT('Ctrl Pts',(-20.4181696602443,12.0649779910963,124.149802192162)) ;
#71889=CARTESIAN_POINT('Ctrl Pts',(-20.4184247291509,12.0649582418742,124.14945336746)) ;
#71890=CARTESIAN_POINT('Ctrl Pts',(-20.4185567891168,12.0649480136099,124.14927266431)) ;
#71891=CARTESIAN_POINT('Ctrl Pts',(-20.4188307611062,12.0649267872597,124.148897565596)) ;
#71892=CARTESIAN_POINT('Ctrl Pts',(-20.418972665493,12.0649157892556,124.148703164546)) ;
#71893=CARTESIAN_POINT('Ctrl Pts',(-20.422192437283,12.0646661618952,124.144289581556)) ;
#71894=CARTESIAN_POINT('Ctrl Pts',(-20.4252438958259,12.0644278074472,124.140051183426)) ;
#71895=CARTESIAN_POINT('Ctrl Pts',(-20.4331073680391,12.0638088571386,124.128983395644)) ;
#71896=CARTESIAN_POINT('Ctrl Pts',(-20.4378776439048,12.0634286941462,124.122124657684)) ;
#71897=CARTESIAN_POINT('Ctrl Pts',(-20.4528336824315,12.062221153675,124.100154114118)) ;
#71898=CARTESIAN_POINT('Ctrl Pts',(-20.4627578372336,12.0613965442986,124.084867254394)) ;
#71899=CARTESIAN_POINT('Ctrl Pts',(-20.4727813146158,12.0605343833122,124.068662240816)) ;
#71900=CARTESIAN_POINT('Ctrl Pts',(-20.4732176477929,12.0604967910872,124.067955243916)) ;
#71901=CARTESIAN_POINT('Ctrl Pts',(-20.4738579534048,12.0604415344476,124.066915429489)) ;
#71902=CARTESIAN_POINT('Ctrl Pts',(-20.47406247534,12.0604238710399,124.066582950534)) ;
#71903=CARTESIAN_POINT('Ctrl Pts',(-20.4843179391799,12.0595374725998,124.049893750197)) ;
#71904=CARTESIAN_POINT('Ctrl Pts',(-20.4939908272755,12.0586677426322,124.033307837398)) ;
#71905=CARTESIAN_POINT('Ctrl Pts',(-20.5059948635859,12.0575370041652,124.011590177861)) ;
#71906=CARTESIAN_POINT('Ctrl Pts',(-20.5086787182254,12.0572806733436,124.00665630531)) ;
#71907=CARTESIAN_POINT('Ctrl Pts',(-20.512853324228,12.056876255664,123.998857135199)) ;
#71908=CARTESIAN_POINT('Ctrl Pts',(-20.5143663828104,12.0567284643461,123.996003853889)) ;
#71909=CARTESIAN_POINT('Ctrl Pts',(-20.517005735188,12.0564685004419,123.990979693407)) ;
#71910=CARTESIAN_POINT('Ctrl Pts',(-20.5181367485304,12.05635639112,123.988811310969)) ;
#71911=CARTESIAN_POINT('Ctrl Pts',(-20.5205349422282,12.0561171488925,123.984180392362)) ;
#71912=CARTESIAN_POINT('Ctrl Pts',(-20.521800316381,12.0559899929009,123.98171693723)) ;
#71913=CARTESIAN_POINT('Ctrl Pts',(-20.5246253246488,12.0557040202269,123.976171891689)) ;
#71914=CARTESIAN_POINT('Ctrl Pts',(-20.5261803932535,12.0555451455551,123.973088004535)) ;
#71915=CARTESIAN_POINT('Ctrl Pts',(-20.5301083198074,12.0551401077827,123.965217488337)) ;
#71916=CARTESIAN_POINT('Ctrl Pts',(-20.5324633030709,12.0548937254411,123.96042203006)) ;
#71917=CARTESIAN_POINT('Ctrl Pts',(-20.5394434255522,12.054152739411,123.945975039241)) ;
#71918=CARTESIAN_POINT('Ctrl Pts',(-20.5439754046794,12.0536571107952,123.936279101889)) ;
#71919=CARTESIAN_POINT('Ctrl Pts',(-20.5620006759575,12.0516265810683,123.896387329024)) ;
#71920=CARTESIAN_POINT('Ctrl Pts',(-20.5744178530992,12.0500879661591,123.865719170608)) ;
#71921=CARTESIAN_POINT('Ctrl Pts',(-20.5880790005414,12.0482251157667,123.827708763827)) ;
#71922=CARTESIAN_POINT('Ctrl Pts',(-20.5904932724967,12.0478882184446,123.820801409786)) ;
#71923=CARTESIAN_POINT('Ctrl Pts',(-20.5942155879645,12.0473563127395,123.809843716294)) ;
#71924=CARTESIAN_POINT('Ctrl Pts',(-20.5955638247531,12.0471609157256,123.805807230995)) ;
#71925=CARTESIAN_POINT('Ctrl Pts',(-20.59804666127,12.0467958645489,123.798245575422)) ;
#71926=CARTESIAN_POINT('Ctrl Pts',(-20.5991862591325,12.0466261635597,123.794722098284)) ;
#71927=CARTESIAN_POINT('Ctrl Pts',(-20.6016697257812,12.0462515135264,123.786925406358)) ;
#71928=CARTESIAN_POINT('Ctrl Pts',(-20.6030063164397,12.0460466360809,123.782649924706)) ;
#71929=CARTESIAN_POINT('Ctrl Pts',(-20.6071630785038,12.0453989591058,123.769097916851)) ;
#71930=CARTESIAN_POINT('Ctrl Pts',(-20.6098983232399,12.0449569452473,123.759795696497)) ;
#71931=CARTESIAN_POINT('Ctrl Pts',(-20.6165612161888,12.0438375928716,123.736121732893)) ;
#71932=CARTESIAN_POINT('Ctrl Pts',(-20.6203406615935,12.0431613709553,123.721709865636)) ;
#71933=CARTESIAN_POINT('Ctrl Pts',(-20.6297784283664,12.0413493131084,123.682907377856)) ;
#71934=CARTESIAN_POINT('Ctrl Pts',(-20.6349630441291,12.0402131776064,123.658408815265)) ;
#71935=CARTESIAN_POINT('Ctrl Pts',(-20.6406211340074,12.0387595178698,123.627050353775)) ;
#71936=CARTESIAN_POINT('Ctrl Pts',(-20.6417786739652,12.0384476006976,123.620319807053)) ;
#71937=CARTESIAN_POINT('Ctrl Pts',(-20.6436637759499,12.0379135113278,123.608794173082)) ;
#71938=CARTESIAN_POINT('Ctrl Pts',(-20.6444186943254,12.0376915400198,123.604003711717)) ;
#71939=CARTESIAN_POINT('Ctrl Pts',(-20.6458999344702,12.037238901197,123.594234885875)) ;
#71940=CARTESIAN_POINT('Ctrl Pts',(-20.6466241161967,12.0370082231259,123.589256286303)) ;
#71941=CARTESIAN_POINT('Ctrl Pts',(-20.6480658827345,12.0365286695965,123.578906160684)) ;
#71942=CARTESIAN_POINT('Ctrl Pts',(-20.6487786317843,12.0362797683314,123.573534066836)) ;
#71943=CARTESIAN_POINT('Ctrl Pts',(-20.650463700079,12.035660496697,123.560167347254)) ;
#71944=CARTESIAN_POINT('Ctrl Pts',(-20.6513937331328,12.0352899070978,123.552167646638)) ;
#71945=CARTESIAN_POINT('Ctrl Pts',(-20.6544396878819,12.0339650937015,123.523560307749)) ;
#71946=CARTESIAN_POINT('Ctrl Pts',(-20.6561205682173,12.0330093666764,123.502909777888)) ;
#71947=CARTESIAN_POINT('Ctrl Pts',(-20.6576438143366,12.0317651851348,123.475911306821)) ;
#71948=CARTESIAN_POINT('Ctrl Pts',(-20.657952198977,12.0314744462619,123.469592960766)) ;
#71949=CARTESIAN_POINT('Ctrl Pts',(-20.6584354889974,12.0309355557161,123.457863030485)) ;
#71950=CARTESIAN_POINT('Ctrl Pts',(-20.6586232206058,12.0306872812204,123.452452151454)) ;
#71951=CARTESIAN_POINT('Ctrl Pts',(-20.659418912749,12.0293933844223,123.424227986118)) ;
#71952=CARTESIAN_POINT('Ctrl Pts',(-20.6594371880276,12.028350724203,123.40140236518)) ;
#71953=CARTESIAN_POINT('Ctrl Pts',(-20.6584226153015,12.0266050694688,123.363245728406)) ;
#71954=CARTESIAN_POINT('Ctrl Pts',(-20.657732078491,12.0259028403014,123.347911293571)) ;
#71955=CARTESIAN_POINT('Ctrl Pts',(-20.6564251327272,12.0249580295856,123.327330883274)) ;
#71956=CARTESIAN_POINT('Ctrl Pts',(-20.656057636337,12.024716329629,123.322070441065)) ;
#71957=CARTESIAN_POINT('Ctrl Pts',(-20.6552721826119,12.024242401614,123.311765619155)) ;
#71958=CARTESIAN_POINT('Ctrl Pts',(-20.6548576526987,12.0240106250304,123.306730645549)) ;
#71959=CARTESIAN_POINT('Ctrl Pts',(-20.6544117326069,12.0237782986488,123.30168882934)) ;
#71960=CARTESIAN_POINT('Origin',(-19.4092722359532,16.5113612779716,123.411814366564)) ;
#71961=CARTESIAN_POINT('',(-20.5919049252751,11.7,123.006993514553)) ;
#71962=CARTESIAN_POINT('',(-20.5919021064381,16.5113612779716,123.006985279772)) ;
#71963=CARTESIAN_POINT('Ctrl Pts',(-20.6544117668603,12.0237783015714,123.301689216628)) ;
#71964=CARTESIAN_POINT('Ctrl Pts',(-20.6544694561418,12.0157819840134,123.302341485478)) ;
#71965=CARTESIAN_POINT('Ctrl Pts',(-20.6544970374151,12.0078383226351,123.302657626506)) ;
#71966=CARTESIAN_POINT('Ctrl Pts',(-20.6544970374151,11.9621695797156,123.302657626506)) ;
#71967=CARTESIAN_POINT('Ctrl Pts',(-20.6538866180435,11.9219235159018,123.294843389787)) ;
#71968=CARTESIAN_POINT('Ctrl Pts',(-20.6505510417636,11.8480564696761,123.263577766805)) ;
#71969=CARTESIAN_POINT('Ctrl Pts',(-20.6477244677879,11.8144220247008,123.24016910469)) ;
#71970=CARTESIAN_POINT('Ctrl Pts',(-20.6391780918807,11.761317155029,123.186964545377)) ;
#71971=CARTESIAN_POINT('Ctrl Pts',(-20.6328682032119,11.7382522587826,123.15357258444)) ;
#71972=CARTESIAN_POINT('Ctrl Pts',(-20.6154021887202,11.7075896772133,123.081471444624)) ;
#71973=CARTESIAN_POINT('Ctrl Pts',(-20.6041551258135,11.7,123.042780919119)) ;
#71974=CARTESIAN_POINT('Ctrl Pts',(-20.5919049252751,11.7,123.006993514553)) ;
#71975=CARTESIAN_POINT('Ctrl Pts',(-18.3268334740834,12.1788217328616,124.036975407319)) ;
#71976=CARTESIAN_POINT('Ctrl Pts',(-18.3340422145277,12.1597692257128,124.049457023371)) ;
#71977=CARTESIAN_POINT('Ctrl Pts',(-18.3403342428411,12.139044727822,124.059859793497)) ;
#71978=CARTESIAN_POINT('Ctrl Pts',(-18.3453503566598,12.1170531743812,124.067992874926)) ;
#71979=CARTESIAN_POINT('',(-18.2266508223232,11.7,123.81666815758)) ;
#71980=CARTESIAN_POINT('Ctrl Pts',(-18.3583806245238,12.,124.088665030377)) ;
#71981=CARTESIAN_POINT('Ctrl Pts',(-18.3583806245238,11.9621695797156,124.088665030377)) ;
#71982=CARTESIAN_POINT('Ctrl Pts',(-18.3540742080748,11.9219235159018,124.082116008719)) ;
#71983=CARTESIAN_POINT('Ctrl Pts',(-18.3375495990129,11.8480564696761,124.055365260225)) ;
#71984=CARTESIAN_POINT('Ctrl Pts',(-18.3254377303918,11.8144220247008,124.035135143544)) ;
#71985=CARTESIAN_POINT('Ctrl Pts',(-18.2995859960063,11.761317155029,123.987854560826)) ;
#71986=CARTESIAN_POINT('Ctrl Pts',(-18.2841086594605,11.7382522587826,123.957600803974)) ;
#71987=CARTESIAN_POINT('Ctrl Pts',(-18.2537250256192,11.7075896772133,123.889921628303)) ;
#71988=CARTESIAN_POINT('Ctrl Pts',(-18.2389020196221,11.7,123.852455220934)) ;
#71989=CARTESIAN_POINT('Ctrl Pts',(-18.2266508223232,11.7,123.81666815758)) ;
#71990=CARTESIAN_POINT('Ctrl Pts',(-18.2266508223232,11.7,123.81666815758)) ;
#71991=CARTESIAN_POINT('Ctrl Pts',(-18.2143996574381,11.7,123.78088118891)) ;
#71992=CARTESIAN_POINT('Ctrl Pts',(-18.2031515402731,11.7075896412593,123.742191073382)) ;
#71993=CARTESIAN_POINT('Ctrl Pts',(-18.1856835511285,11.7382521626639,123.670090636116)) ;
#71994=CARTESIAN_POINT('Ctrl Pts',(-18.1793727421956,11.7613170365764,123.636698971197)) ;
#71995=CARTESIAN_POINT('Ctrl Pts',(-18.1708248842569,11.8144219229966,123.583494827023)) ;
#71996=CARTESIAN_POINT('Ctrl Pts',(-18.1679976569785,11.8480564142548,123.560086346945)) ;
#71997=CARTESIAN_POINT('Ctrl Pts',(-18.1646612055237,11.9219235188396,123.528820989278)) ;
#71998=CARTESIAN_POINT('Ctrl Pts',(-18.1640505668151,11.9621695923928,123.521006833268)) ;
#71999=CARTESIAN_POINT('Ctrl Pts',(-18.1640505668151,12.,123.521006833268)) ;
#72000=CARTESIAN_POINT('Ctrl Pts',(-20.5919021064174,11.7000000001262,123.006985279712)) ;
#72001=CARTESIAN_POINT('Ctrl Pts',(-20.579651689103,11.7000010975739,122.971198055147)) ;
#72002=CARTESIAN_POINT('Ctrl Pts',(-20.5648328354892,11.7075896412593,122.933739475197)) ;
#72003=CARTESIAN_POINT('Ctrl Pts',(-20.5344511925933,11.7382521626639,122.86605964457)) ;
#72004=CARTESIAN_POINT('Ctrl Pts',(-20.5189747646632,11.7613170365764,122.835805557673)) ;
#72005=CARTESIAN_POINT('Ctrl Pts',(-20.4931244558125,11.8144219229966,122.788524394775)) ;
#72006=CARTESIAN_POINT('Ctrl Pts',(-20.4810132149992,11.8480564142548,122.76829402158)) ;
#72007=CARTESIAN_POINT('Ctrl Pts',(-20.4644894601081,11.9219235188396,122.741542946412)) ;
#72008=CARTESIAN_POINT('Ctrl Pts',(-20.4601832664426,11.9621695923928,122.734993854115)) ;
#72009=CARTESIAN_POINT('Ctrl Pts',(-20.4601832664426,12.,122.734993854115)) ;
#72010=CARTESIAN_POINT('Ctrl Pts',(-17.9901976316281,-10.0000000000559,
123.897592500191)) ;
#72011=CARTESIAN_POINT('Ctrl Pts',(-18.2740109056134,-9.82001091963712,
123.800437437226)) ;
#72012=CARTESIAN_POINT('Ctrl Pts',(-18.0463587734038,-10.006626850874,124.061733136848)) ;
#72013=CARTESIAN_POINT('Ctrl Pts',(-18.318952820002,-9.82663777045524,123.931772257896)) ;
#72014=CARTESIAN_POINT('Ctrl Pts',(-18.215820208241,-10.019857477355,124.369865791256)) ;
#72015=CARTESIAN_POINT('Ctrl Pts',(-18.4544999964107,-9.83986839693625,
124.178242269465)) ;
#72016=CARTESIAN_POINT('Ctrl Pts',(-18.6148367044591,-10.0398330986136,
124.720100586831)) ;
#72017=CARTESIAN_POINT('Ctrl Pts',(-18.7737259547846,-9.85984401819488,
124.458448709452)) ;
#72018=CARTESIAN_POINT('Ctrl Pts',(-19.1081207670021,-10.0597504335156,
124.912141899957)) ;
#72019=CARTESIAN_POINT('Ctrl Pts',(-19.1683517739458,-9.87976135309682,
124.612076728176)) ;
#72020=CARTESIAN_POINT('Ctrl Pts',(-19.6362061149481,-10.0796237102316,
124.925498515574)) ;
#72021=CARTESIAN_POINT('Ctrl Pts',(-19.5908222086086,-9.89963462981282,
124.622761886445)) ;
#72022=CARTESIAN_POINT('Ctrl Pts',(-20.1407529320643,-10.0996482003955,
124.756244590418)) ;
#72023=CARTESIAN_POINT('Ctrl Pts',(-19.994458721673,-9.91965911997678,124.487357109044)) ;
#72024=CARTESIAN_POINT('Ctrl Pts',(-20.5540202996666,-10.1195160415463,
124.427406225496)) ;
#72025=CARTESIAN_POINT('Ctrl Pts',(-20.3250727353524,-9.9395269611275,124.224284451464)) ;
#72026=CARTESIAN_POINT('Ctrl Pts',(-20.8319818408465,-10.1394616924258,
123.976064807466)) ;
#72027=CARTESIAN_POINT('Ctrl Pts',(-20.547440485577,-9.95947261200706,123.863209762279)) ;
#72028=CARTESIAN_POINT('Ctrl Pts',(-20.9388342401899,-10.1593670930428,
123.457915382838)) ;
#72029=CARTESIAN_POINT('Ctrl Pts',(-20.6329204948871,-9.97937801262402,
123.448688955287)) ;
#72030=CARTESIAN_POINT('Ctrl Pts',(-20.8636098403204,-10.1792413208591,
122.935072644698)) ;
#72031=CARTESIAN_POINT('Ctrl Pts',(-20.5727382379585,-9.99925224044038,
123.03041411648)) ;
#72032=CARTESIAN_POINT('Ctrl Pts',(-20.6131115834828,-10.1992271117367,
122.466642059168)) ;
#72033=CARTESIAN_POINT('Ctrl Pts',(-20.3723371633396,-10.019238031318,122.655670872381)) ;
#72034=CARTESIAN_POINT('Ctrl Pts',(-20.2194466572393,-10.2191213543965,
122.113692749269)) ;
#72035=CARTESIAN_POINT('Ctrl Pts',(-20.0574027588299,-10.0391322739778,
122.373312971228)) ;
#72036=CARTESIAN_POINT('Ctrl Pts',(-19.7297807740129,-10.2390000704686,
121.915093775285)) ;
#72037=CARTESIAN_POINT('Ctrl Pts',(-19.6656681100072,-10.0590109900498,
122.21443654672)) ;
#72038=CARTESIAN_POINT('Ctrl Pts',(-19.1975679684638,-10.2590395203132,
121.895998337722)) ;
#72039=CARTESIAN_POINT('Ctrl Pts',(-19.2398980466007,-10.0790504398944,
122.199163431724)) ;
#72040=CARTESIAN_POINT('Ctrl Pts',(-18.6950312339479,-10.278902681851,122.058270950154)) ;
#72041=CARTESIAN_POINT('Ctrl Pts',(-18.837868920824,-10.0989136014323,122.328984924085)) ;
#72042=CARTESIAN_POINT('Ctrl Pts',(-18.2756669291074,-10.2988820498653,
122.383749835499)) ;
#72043=CARTESIAN_POINT('Ctrl Pts',(-18.5023795133954,-10.1188929694465,
122.589370885141)) ;
#72044=CARTESIAN_POINT('Ctrl Pts',(-17.9943038604906,-10.3186926303881,
122.828930487525)) ;
#72045=CARTESIAN_POINT('Ctrl Pts',(-18.2772917344201,-10.1387035499693,
122.945518187819)) ;
#72046=CARTESIAN_POINT('Ctrl Pts',(-17.8800540060949,-10.3386735586737,
123.347451469639)) ;
#72047=CARTESIAN_POINT('Ctrl Pts',(-18.1858955346146,-10.1586844782549,
123.360335798021)) ;
#72048=CARTESIAN_POINT('Ctrl Pts',(-17.9496636135844,-10.3585662305431,
123.871624239551)) ;
#72049=CARTESIAN_POINT('Ctrl Pts',(-18.2415877728661,-10.1785771501243,
123.779674103343)) ;
#72050=CARTESIAN_POINT('Ctrl Pts',(-18.1935384904097,-10.3784925608302,
124.341742095298)) ;
#72051=CARTESIAN_POINT('Ctrl Pts',(-18.4366892418074,-10.1985034804115,
124.155765909524)) ;
#72052=CARTESIAN_POINT('Ctrl Pts',(-18.5843830565522,-10.3984631149225,
124.700856014359)) ;
#72053=CARTESIAN_POINT('Ctrl Pts',(-18.7493759717748,-10.2184740345037,
124.44305681766)) ;
#72054=CARTESIAN_POINT('Ctrl Pts',(-18.9897866675732,-10.4149949540101,
124.87030674843)) ;
#72055=CARTESIAN_POINT('Ctrl Pts',(-19.0736749228579,-10.2350058735914,
124.578605598989)) ;
#72056=CARTESIAN_POINT('Ctrl Pts',(-19.3371420473562,-10.4283346928377,
124.91771178987)) ;
#72057=CARTESIAN_POINT('Ctrl Pts',(-19.3515822796175,-10.2483456124189,
124.6165344309)) ;
#72058=CARTESIAN_POINT('Ctrl Pts',(-19.600556266745,-10.4383669350563,124.907063768875)) ;
#72059=CARTESIAN_POINT('Ctrl Pts',(-19.5623087731277,-10.2583778546375,
124.608012505296)) ;
#72060=CARTESIAN_POINT('Ctrl Pts',(-19.8537397871011,-10.4482246356997,
124.852203726836)) ;
#72061=CARTESIAN_POINT('Ctrl Pts',(-19.7648571225557,-10.268235555281,124.564122220758)) ;
#72062=CARTESIAN_POINT('Ctrl Pts',(-20.0969735540212,-10.458216500339,124.753332920167)) ;
#72063=CARTESIAN_POINT('Ctrl Pts',(-19.9594412734619,-10.2782274199202,
124.485025314983)) ;
#72064=CARTESIAN_POINT('Ctrl Pts',(-20.3177787346959,-10.4681390500991,
124.61465218344)) ;
#72065=CARTESIAN_POINT('Ctrl Pts',(-20.1360907041886,-10.2881499696804,
124.374071880139)) ;
#72066=CARTESIAN_POINT('Ctrl Pts',(-20.5771970982088,-10.4814168235926,
124.381203458951)) ;
#72067=CARTESIAN_POINT('Ctrl Pts',(-20.3435922192053,-10.3014277431738,
124.18734533642)) ;
#72068=CARTESIAN_POINT('Ctrl Pts',(-20.7701003709019,-10.4947641625332,
124.083584310499)) ;
#72069=CARTESIAN_POINT('Ctrl Pts',(-20.4979358992389,-10.3147750821144,
123.949230612993)) ;
#72070=CARTESIAN_POINT('Ctrl Pts',(-20.8774553694635,-10.5079713943264,
123.753475217075)) ;
#72071=CARTESIAN_POINT('Ctrl Pts',(-20.5838202404129,-10.3279823139076,
123.685128879657)) ;
#72072=CARTESIAN_POINT('Ctrl Pts',(-20.914528239215,-10.5179585104161,123.493699384281)) ;
#72073=CARTESIAN_POINT('Ctrl Pts',(-20.6134756829108,-10.3379694299973,
123.477310647391)) ;
#72074=CARTESIAN_POINT('Ctrl Pts',(-20.9061303770652,-10.5279094159958,
123.232285620256)) ;
#72075=CARTESIAN_POINT('Ctrl Pts',(-20.6067552793287,-10.3479203355771,
123.268178977505)) ;
#72076=CARTESIAN_POINT('Ctrl Pts',(-20.8516285273061,-10.5379645180033,
122.97376743032)) ;
#72077=CARTESIAN_POINT('Ctrl Pts',(-20.5631517097427,-10.3579754375845,
123.061365248372)) ;
#72078=CARTESIAN_POINT('Ctrl Pts',(-20.7557521455566,-10.5477861913244,
122.73410076229)) ;
#72079=CARTESIAN_POINT('Ctrl Pts',(-20.4864480022253,-10.3677971109056,
122.869632334128)) ;
#72080=CARTESIAN_POINT('Ctrl Pts',(-20.6168357131279,-10.5578446623993,
122.509252277658)) ;
#72081=CARTESIAN_POINT('Ctrl Pts',(-20.3753148734437,-10.3778555819805,
122.689756047917)) ;
#72082=CARTESIAN_POINT('Ctrl Pts',(-20.443040351458,-10.5677692735758,122.314768071388)) ;
#72083=CARTESIAN_POINT('Ctrl Pts',(-20.2362698376991,-10.387780193157,122.534165626482)) ;
#72084=CARTESIAN_POINT('Ctrl Pts',(-20.1694406713465,-10.5810466124762,
122.098190251823)) ;
#72085=CARTESIAN_POINT('Ctrl Pts',(-20.0174235370575,-10.4010575320574,
122.360928563111)) ;
#72086=CARTESIAN_POINT('Ctrl Pts',(-19.8449850135089,-10.5943454917138,
121.958111265245)) ;
#72087=CARTESIAN_POINT('Ctrl Pts',(-19.7578454755217,-10.414356411295,122.248851541412)) ;
#72088=CARTESIAN_POINT('Ctrl Pts',(-19.5008057716398,-10.6075843638845,
121.907157355555)) ;
#72089=CARTESIAN_POINT('Ctrl Pts',(-19.4824812721784,-10.4275952834657,
122.208088431707)) ;
#72090=CARTESIAN_POINT('Ctrl Pts',(-19.2379220825766,-10.6175909820211,
121.913944971311)) ;
#72091=CARTESIAN_POINT('Ctrl Pts',(-19.2721785612158,-10.4376019016023,
122.213521362329)) ;
#72092=CARTESIAN_POINT('Ctrl Pts',(-18.9796997397217,-10.6276219270826,
121.966900411334)) ;
#72093=CARTESIAN_POINT('Ctrl Pts',(-19.0656000663898,-10.4476328466638,
122.255887759951)) ;
#72094=CARTESIAN_POINT('Ctrl Pts',(-18.7386663423007,-10.6374781004344,
122.061762842518)) ;
#72095=CARTESIAN_POINT('Ctrl Pts',(-18.8727746408769,-10.4574890200157,
122.33177976469)) ;
#72096=CARTESIAN_POINT('Ctrl Pts',(-18.5144394578207,-10.6474773713973,
122.198683103342)) ;
#72097=CARTESIAN_POINT('Ctrl Pts',(-18.6933942799492,-10.4674882909785,
122.44131783091)) ;
#72098=CARTESIAN_POINT('Ctrl Pts',(-18.319187379609,-10.6573718231546,122.370468477367)) ;
#72099=CARTESIAN_POINT('Ctrl Pts',(-18.5371942578644,-10.4773827427359,
122.578747654411)) ;
#72100=CARTESIAN_POINT('Ctrl Pts',(-18.1540827676739,-10.667435138964,122.576990252215)) ;
#72101=CARTESIAN_POINT('Ctrl Pts',(-18.4051122800728,-10.4874460585452,
122.743966484082)) ;
#72102=CARTESIAN_POINT('Ctrl Pts',(-18.0298636946178,-10.6772739957036,
122.803803190582)) ;
#72103=CARTESIAN_POINT('Ctrl Pts',(-18.3057391118683,-10.4972849152848,
122.925417599334)) ;
#72104=CARTESIAN_POINT('Ctrl Pts',(-17.9447485717296,-10.6873401175212,
123.054218033079)) ;
#72105=CARTESIAN_POINT('Ctrl Pts',(-18.2376490673584,-10.5073510371024,
123.125750218179)) ;
#72106=CARTESIAN_POINT('Ctrl Pts',(-17.9052474070553,-10.6972233452454,
123.310952604461)) ;
#72107=CARTESIAN_POINT('Ctrl Pts',(-18.2060503446323,-10.5172342648267,
123.331137917859)) ;
#72108=CARTESIAN_POINT('Ctrl Pts',(-17.9104088182972,-10.7072128065242,
123.573388107822)) ;
#72109=CARTESIAN_POINT('Ctrl Pts',(-18.2101816191011,-10.5272237261055,
123.541086174157)) ;
#72110=CARTESIAN_POINT('Ctrl Pts',(-17.9610292609966,-10.7171765169507,
123.830297050008)) ;
#72111=CARTESIAN_POINT('Ctrl Pts',(-18.2506800579227,-10.5371874365319,
123.746612765702)) ;
#72112=CARTESIAN_POINT('Ctrl Pts',(-18.055529675123,-10.7271715196816,124.07538741282)) ;
#72113=CARTESIAN_POINT('Ctrl Pts',(-18.3262823460712,-10.5471824392628,
123.942684211435)) ;
#72114=CARTESIAN_POINT('Ctrl Pts',(-18.1920485022638,-10.7372078506919,
124.301034603995)) ;
#72115=CARTESIAN_POINT('Ctrl Pts',(-18.4354992728269,-10.5572187702731,
124.12320085702)) ;
#72116=CARTESIAN_POINT('Ctrl Pts',(-18.3620830673666,-10.7470540800342,
124.496092551294)) ;
#72117=CARTESIAN_POINT('Ctrl Pts',(-18.5715282310147,-10.5670649996154,
124.279245472498)) ;
#72118=CARTESIAN_POINT('Ctrl Pts',(-18.5658978745398,-10.7570395783094,
124.661307440014)) ;
#72119=CARTESIAN_POINT('Ctrl Pts',(-18.7345812884953,-10.5770504978907,
124.411415684018)) ;
#72120=CARTESIAN_POINT('Ctrl Pts',(-18.7941275674309,-10.7669744812924,
124.788187738313)) ;
#72121=CARTESIAN_POINT('Ctrl Pts',(-18.9171658133098,-10.5869854008736,
124.51291799715)) ;
#72122=CARTESIAN_POINT('Ctrl Pts',(-19.0439620659732,-10.7770319843876,
124.87431287249)) ;
#72123=CARTESIAN_POINT('Ctrl Pts',(-19.1170341816332,-10.5970429039689,
124.58181616074)) ;
#72124=CARTESIAN_POINT('Ctrl Pts',(-19.2988377714731,-10.7868536407581,
124.915180256281)) ;
#72125=CARTESIAN_POINT('Ctrl Pts',(-19.3209344474807,-10.6068645603394,
124.614507954235)) ;
#72126=CARTESIAN_POINT('Ctrl Pts',(-19.5630543230719,-10.7969097034233,
124.911570311864)) ;
#72127=CARTESIAN_POINT('Ctrl Pts',(-19.5323077507347,-10.6169206230045,
124.611618015563)) ;
#72128=CARTESIAN_POINT('Ctrl Pts',(-19.8195954463674,-10.8068503681265,
124.862237558384)) ;
#72129=CARTESIAN_POINT('Ctrl Pts',(-19.7375400007717,-10.6268612877077,
124.572149858921)) ;
#72130=CARTESIAN_POINT('Ctrl Pts',(-20.0630665620779,-10.816754772075,124.770214821725)) ;
#72131=CARTESIAN_POINT('Ctrl Pts',(-19.9323158100592,-10.6367656916563,
124.498530010754)) ;
#72132=CARTESIAN_POINT('Ctrl Pts',(-20.2899670416391,-10.8268012570685,
124.635280761844)) ;
#72133=CARTESIAN_POINT('Ctrl Pts',(-20.1138352645202,-10.6468121766498,
124.390581038644)) ;
#72134=CARTESIAN_POINT('Ctrl Pts',(-20.4871895042014,-10.8366974848803,
124.465706330273)) ;
#72135=CARTESIAN_POINT('Ctrl Pts',(-20.2716116273665,-10.6567084044615,
124.254920337405)) ;
#72136=CARTESIAN_POINT('Ctrl Pts',(-20.6546848716755,-10.8467570684437,
124.261221540579)) ;
#72137=CARTESIAN_POINT('Ctrl Pts',(-20.4056065232405,-10.666767988025,124.091331180759)) ;
#72138=CARTESIAN_POINT('Ctrl Pts',(-20.7815048415896,-10.8566090781126,
124.035494716852)) ;
#72139=CARTESIAN_POINT('Ctrl Pts',(-20.5070605035221,-10.6766199976938,
123.910749362364)) ;
#72140=CARTESIAN_POINT('Ctrl Pts',(-20.8689878383844,-10.8665716095522,
123.788751735719)) ;
#72141=CARTESIAN_POINT('Ctrl Pts',(-20.5770451355397,-10.6865825291334,
123.713354624159)) ;
#72142=CARTESIAN_POINT('Ctrl Pts',(-20.9122007989983,-10.8766031577915,
123.528690516738)) ;
#72143=CARTESIAN_POINT('Ctrl Pts',(-20.6116136920761,-10.6966140773728,
123.505305293071)) ;
#72144=CARTESIAN_POINT('Ctrl Pts',(-20.9098873496379,-10.8864945690046,
123.268764662033)) ;
#72145=CARTESIAN_POINT('Ctrl Pts',(-20.6097611319996,-10.7065054885858,
123.297365172637)) ;
#72146=CARTESIAN_POINT('Ctrl Pts',(-20.8623452480794,-10.8965108227126,
123.009867420376)) ;
#72147=CARTESIAN_POINT('Ctrl Pts',(-20.5717257539026,-10.7165217422938,
123.090247714627)) ;
#72148=CARTESIAN_POINT('Ctrl Pts',(-20.7699148714446,-10.9065409255573,
122.763029266293)) ;
#72149=CARTESIAN_POINT('Ctrl Pts',(-20.4977797294624,-10.7265518451385,
122.89277779572)) ;
#72150=CARTESIAN_POINT('Ctrl Pts',(-20.6387642262215,-10.916397374511,122.53965056504)) ;
#72151=CARTESIAN_POINT('Ctrl Pts',(-20.3928580826567,-10.7364082940922,
122.714076343171)) ;
#72152=CARTESIAN_POINT('Ctrl Pts',(-20.4686808694509,-10.9263963852833,
122.339414946331)) ;
#72153=CARTESIAN_POINT('Ctrl Pts',(-20.2567901831118,-10.7464073048645,
122.553889022845)) ;
#72154=CARTESIAN_POINT('Ctrl Pts',(-20.2686322562865,-10.9362916022013,
122.173218025973)) ;
#72155=CARTESIAN_POINT('Ctrl Pts',(-20.0967507033617,-10.7563025217825,
122.420933115589)) ;
#72156=CARTESIAN_POINT('Ctrl Pts',(-20.0390441622035,-10.9463521175586,
122.042191046902)) ;
#72157=CARTESIAN_POINT('Ctrl Pts',(-19.9130792483847,-10.7663630371399,
122.316112859812)) ;
#72158=CARTESIAN_POINT('Ctrl Pts',(-19.7954165502378,-10.9562014109456,
121.954734482414)) ;
#72159=CARTESIAN_POINT('Ctrl Pts',(-19.7181774003615,-10.7762123305269,
122.246149405366)) ;
#72160=CARTESIAN_POINT('Ctrl Pts',(-19.5358374377784,-10.9662285866257,
121.909463378903)) ;
#72161=CARTESIAN_POINT('Ctrl Pts',(-19.5105138249597,-10.7862395062069,
122.209933979971)) ;
#72162=CARTESIAN_POINT('Ctrl Pts',(-19.2722869357708,-10.9762571622528,
121.910644966018)) ;
#72163=CARTESIAN_POINT('Ctrl Pts',(-19.2996733747243,-10.7962680818341,
122.210880867466)) ;
#72164=CARTESIAN_POINT('Ctrl Pts',(-19.0176264126099,-10.9861022557987,
121.956219772802)) ;
#72165=CARTESIAN_POINT('Ctrl Pts',(-19.0959461067893,-10.80611317538,122.247342053206)) ;
#72166=CARTESIAN_POINT('Ctrl Pts',(-18.7708903038196,-10.9960934972305,
122.045998590388)) ;
#72167=CARTESIAN_POINT('Ctrl Pts',(-18.8985578386737,-10.8161044168118,
122.319166355093)) ;
#72168=CARTESIAN_POINT('Ctrl Pts',(-18.542748292224,-11.0061292783738,122.178316885935)) ;
#72169=CARTESIAN_POINT('Ctrl Pts',(-18.7160448934344,-10.826140197955,122.425022334904)) ;
#72170=CARTESIAN_POINT('Ctrl Pts',(-18.344525155925,-11.0159814841035,122.344856285558)) ;
#72171=CARTESIAN_POINT('Ctrl Pts',(-18.5574679962225,-10.8359924036847,
122.558254360555)) ;
#72172=CARTESIAN_POINT('Ctrl Pts',(-18.175788051193,-11.0259435782205,122.545009574779)) ;
#72173=CARTESIAN_POINT('Ctrl Pts',(-18.422479486084,-10.8459544978017,122.718377561325)) ;
#72174=CARTESIAN_POINT('Ctrl Pts',(-18.0438458205834,-11.0359661390476,
122.77296014226)) ;
#72175=CARTESIAN_POINT('Ctrl Pts',(-18.3169268399301,-10.8559770586288,
122.900738711909)) ;
#72176=CARTESIAN_POINT('Ctrl Pts',(-17.9540915965204,-11.0458939106991,
123.017952668902)) ;
#72177=CARTESIAN_POINT('Ctrl Pts',(-18.245124831637,-10.8659048302804,123.096732704545)) ;
#72178=CARTESIAN_POINT('Ctrl Pts',(-17.9077456059783,-11.055936294824,123.27773445602)) ;
#72179=CARTESIAN_POINT('Ctrl Pts',(-18.2080492829974,-10.8759472144052,
123.304558492291)) ;
#72180=CARTESIAN_POINT('Ctrl Pts',(-17.9071113955482,-11.0658255188946,
123.537627775345)) ;
#72181=CARTESIAN_POINT('Ctrl Pts',(-18.2075431810581,-10.8858364384758,
123.512472408022)) ;
#72182=CARTESIAN_POINT('Ctrl Pts',(-17.9515732677146,-11.0758147670619,
123.796333212576)) ;
#72183=CARTESIAN_POINT('Ctrl Pts',(-18.2431137880875,-10.8958256866432,
123.719436394321)) ;
#72184=CARTESIAN_POINT('Ctrl Pts',(-18.0401957306553,-11.0857733441039,
124.042564530885)) ;
#72185=CARTESIAN_POINT('Ctrl Pts',(-18.3140127714057,-10.9057842636851,
123.916420715581)) ;
#72186=CARTESIAN_POINT('Ctrl Pts',(-18.1689090611489,-11.0956729131951,
124.26866068517)) ;
#72187=CARTESIAN_POINT('Ctrl Pts',(-18.4169840046767,-10.9156838327764,
124.097296505228)) ;
#72188=CARTESIAN_POINT('Ctrl Pts',(-18.3374567294345,-11.1057208252791,
124.471882073848)) ;
#72189=CARTESIAN_POINT('Ctrl Pts',(-18.5518230802635,-10.9257317448604,
124.259873062704)) ;
#72190=CARTESIAN_POINT('Ctrl Pts',(-18.5355938113499,-11.1156161795864,
124.640356432231)) ;
#72191=CARTESIAN_POINT('Ctrl Pts',(-18.7103328563198,-10.9356270991676,
124.394651291218)) ;
#72192=CARTESIAN_POINT('Ctrl Pts',(-18.7636640135748,-11.1256778300776,
124.77407551391)) ;
#72193=CARTESIAN_POINT('Ctrl Pts',(-18.8927897608012,-10.9456887496588,
124.50162580593)) ;
#72194=CARTESIAN_POINT('Ctrl Pts',(-19.0061643664109,-11.13552244554,124.864226909318)) ;
#72195=CARTESIAN_POINT('Ctrl Pts',(-19.0867894053353,-10.9555333651213,
124.573745602818)) ;
#72196=CARTESIAN_POINT('Ctrl Pts',(-19.263434682644,-11.1454825244414,124.912371167805)) ;
#72197=CARTESIAN_POINT('Ctrl Pts',(-19.2926054448866,-10.9654934440227,
124.612260162443)) ;
#72198=CARTESIAN_POINT('Ctrl Pts',(-19.5272078042054,-11.1555207187998,
124.914621442869)) ;
#72199=CARTESIAN_POINT('Ctrl Pts',(-19.5036240790433,-10.9755316383811,
124.614059468937)) ;
#72200=CARTESIAN_POINT('Ctrl Pts',(-19.7832249578814,-11.1653944341994,
124.872221302239)) ;
#72201=CARTESIAN_POINT('Ctrl Pts',(-19.7084367869545,-10.9854053537807,
124.580138714143)) ;
#72202=CARTESIAN_POINT('Ctrl Pts',(-20.0328232712433,-11.1754661437337,
124.784280775652)) ;
#72203=CARTESIAN_POINT('Ctrl Pts',(-19.9081154761896,-10.9954770633149,
124.509785425241)) ;
#72204=CARTESIAN_POINT('Ctrl Pts',(-20.2580073160993,-11.1852985841862,
124.657525797666)) ;
#72205=CARTESIAN_POINT('Ctrl Pts',(-20.0882613121544,-11.0053095037674,
124.408381348776)) ;
#72206=CARTESIAN_POINT('Ctrl Pts',(-20.4622563154496,-11.1953304051116,
124.490859965115)) ;
#72207=CARTESIAN_POINT('Ctrl Pts',(-20.2516602105671,-11.0153413246928,
124.275048161913)) ;
#72208=CARTESIAN_POINT('Ctrl Pts',(-20.6337047073231,-11.2053507749972,
124.29099219891)) ;
#72209=CARTESIAN_POINT('Ctrl Pts',(-20.388818355727,-11.0253616945784,124.115153420591)) ;
#72210=CARTESIAN_POINT('Ctrl Pts',(-20.7663802889298,-11.2152175461309,
124.068198059757)) ;
#72211=CARTESIAN_POINT('Ctrl Pts',(-20.4949578009106,-11.0352284657122,
123.936918629634)) ;
#72212=CARTESIAN_POINT('Ctrl Pts',(-20.8602333251002,-11.2252883173203,
123.820777914733)) ;
#72213=CARTESIAN_POINT('Ctrl Pts',(-20.5700397729981,-11.0452992369015,
123.738981987884)) ;
#72214=CARTESIAN_POINT('Ctrl Pts',(-20.9086197172396,-11.2351314778419,
123.566660443402)) ;
#72215=CARTESIAN_POINT('Ctrl Pts',(-20.608748082228,-11.0551423974231,123.535689006923)) ;
#72216=CARTESIAN_POINT('Ctrl Pts',(-20.9130575838385,-11.2451117110283,
123.3044363292)) ;
#72217=CARTESIAN_POINT('Ctrl Pts',(-20.6122979803846,-11.0651226306096,
123.325909958137)) ;
#72218=CARTESIAN_POINT('Ctrl Pts',(-20.8712385789228,-11.2551302310635,
123.044509679232)) ;
#72219=CARTESIAN_POINT('Ctrl Pts',(-20.5788422638188,-11.0751411506447,
123.117968711757)) ;
#72220=CARTESIAN_POINT('Ctrl Pts',(-20.7865977119189,-11.2650135394472,
122.798931493941)) ;
#72221=CARTESIAN_POINT('Ctrl Pts',(-20.5111294989851,-11.0850244590284,
122.921507117009)) ;
#72222=CARTESIAN_POINT('Ctrl Pts',(-20.6581795185129,-11.275081823618,122.567651782583)) ;
#72223=CARTESIAN_POINT('Ctrl Pts',(-20.4083944277967,-11.0950927431992,
122.736483258853)) ;
#72224=CARTESIAN_POINT('Ctrl Pts',(-20.4956768374631,-11.2849119502856,
122.366783576228)) ;
#72225=CARTESIAN_POINT('Ctrl Pts',(-20.278392801361,-11.1049228698669,122.575789859925)) ;
#72226=CARTESIAN_POINT('Ctrl Pts',(-20.2963683002657,-11.2949785224922,
122.192903170053)) ;
#72227=CARTESIAN_POINT('Ctrl Pts',(-20.1189455705143,-11.1149894420734,
122.436685510706)) ;
#72228=CARTESIAN_POINT('Ctrl Pts',(-20.0737183941144,-11.3048686787329,
122.058761956698)) ;
#72229=CARTESIAN_POINT('Ctrl Pts',(-19.9408262162374,-11.1248795983141,
122.329373218762)) ;
#72230=CARTESIAN_POINT('Ctrl Pts',(-19.8289002832295,-11.3148612063093,
121.963839656231)) ;
#72231=CARTESIAN_POINT('Ctrl Pts',(-19.7449718346838,-11.1348721258905,
122.253435573056)) ;
#72232=CARTESIAN_POINT('Ctrl Pts',(-19.5720596013039,-11.3248226961836,
121.913243324942)) ;
#72233=CARTESIAN_POINT('Ctrl Pts',(-19.53949961243,-11.1448336157648,122.212958778088)) ;
#72234=CARTESIAN_POINT('Ctrl Pts',(-19.3117087063704,-11.3347319180708,
121.907440658288)) ;
#72235=CARTESIAN_POINT('Ctrl Pts',(-19.3312196283681,-11.154742837652,122.208316707602)) ;
#72236=CARTESIAN_POINT('Ctrl Pts',(-19.0507261790617,-11.3447804978811,
121.947576761834)) ;
#72237=CARTESIAN_POINT('Ctrl Pts',(-19.1224334112309,-11.1647914174624,
122.240425692634)) ;
#72238=CARTESIAN_POINT('Ctrl Pts',(-18.804739750581,-11.3546634723512,122.030941792097)) ;
#72239=CARTESIAN_POINT('Ctrl Pts',(-18.9256451263576,-11.1746743919324,
122.307117480373)) ;
#72240=CARTESIAN_POINT('Ctrl Pts',(-18.5741327464294,-11.3646583834939,
122.156656021999)) ;
#72241=CARTESIAN_POINT('Ctrl Pts',(-18.7411596022947,-11.1846693030751,
122.407688711713)) ;
#72242=CARTESIAN_POINT('Ctrl Pts',(-18.3685394795341,-11.3746787700675,
122.321218804794)) ;
#72243=CARTESIAN_POINT('Ctrl Pts',(-18.5766849675727,-11.1946896896487,
122.539338955783)) ;
#72244=CARTESIAN_POINT('Ctrl Pts',(-18.1964679002399,-11.3845888739245,
122.516679816492)) ;
#72245=CARTESIAN_POINT('Ctrl Pts',(-18.4390281618024,-11.2045997935058,
122.69570718939)) ;
#72246=CARTESIAN_POINT('Ctrl Pts',(-18.0601098923841,-11.3945165861344,
122.739110167185)) ;
#72247=CARTESIAN_POINT('Ctrl Pts',(-18.3299418822673,-11.2145275057157,
122.873650852243)) ;
#72248=CARTESIAN_POINT('Ctrl Pts',(-17.9635464110785,-11.4045596959017,
122.984721718115)) ;
#72249=CARTESIAN_POINT('Ctrl Pts',(-18.2526908895868,-11.2245706154829,
123.070140194401)) ;
#72250=CARTESIAN_POINT('Ctrl Pts',(-17.9117458664218,-11.4144461163572,
123.239325516357)) ;
#72251=CARTESIAN_POINT('Ctrl Pts',(-18.2112504325607,-11.2344570359385,
123.273822340803)) ;
#72252=CARTESIAN_POINT('Ctrl Pts',(-17.9044206321702,-11.4244392939629,
123.501819128655)) ;
#72253=CARTESIAN_POINT('Ctrl Pts',(-18.2053899382535,-11.2444502135441,
123.483817059054)) ;
#72254=CARTESIAN_POINT('Ctrl Pts',(-17.9427031377014,-11.4343849568668,
123.760362733603)) ;
#72255=CARTESIAN_POINT('Ctrl Pts',(-18.2360155909013,-11.254395876448,123.690651513861)) ;
#72256=CARTESIAN_POINT('Ctrl Pts',(-18.0248064636778,-11.444332253072,124.008552115049)) ;
#72257=CARTESIAN_POINT('Ctrl Pts',(-18.3016977085877,-11.2643431726532,
123.889202714741)) ;
#72258=CARTESIAN_POINT('Ctrl Pts',(-18.1502567639507,-11.4543800186499,
124.240883955194)) ;
#72259=CARTESIAN_POINT('Ctrl Pts',(-18.402057739547,-11.2743909382311,124.075068526834)) ;
#72260=CARTESIAN_POINT('Ctrl Pts',(-18.3107289743718,-11.4642282318675,
124.443923603777)) ;
#72261=CARTESIAN_POINT('Ctrl Pts',(-18.5304345036023,-11.2842391514487,
124.237499615883)) ;
#72262=CARTESIAN_POINT('Ctrl Pts',(-18.505629079582,-11.4741878046616,124.618608196074)) ;
#72263=CARTESIAN_POINT('Ctrl Pts',(-18.6863538979281,-11.2941987242428,
124.377247496808)) ;
#72264=CARTESIAN_POINT('Ctrl Pts',(-18.7298566496117,-11.4842244256941,
124.7574702214)) ;
#72265=CARTESIAN_POINT('Ctrl Pts',(-18.8657357990191,-11.3042353452753,
124.488337605862)) ;
#72266=CARTESIAN_POINT('Ctrl Pts',(-18.9708633136345,-11.4941049405044,
124.854157638522)) ;
#72267=CARTESIAN_POINT('Ctrl Pts',(-19.0585400766373,-11.3141158600857,
124.565687764043)) ;
#72268=CARTESIAN_POINT('Ctrl Pts',(-19.2293390121341,-11.5041575918115,
124.908543575082)) ;
#72269=CARTESIAN_POINT('Ctrl Pts',(-19.265320722865,-11.3241685113927,124.609197170298)) ;
#72270=CARTESIAN_POINT('Ctrl Pts',(-19.4892814881004,-11.5140529900915,
124.917196362608)) ;
#72271=CARTESIAN_POINT('Ctrl Pts',(-19.4732739141341,-11.3340639096727,
124.61612002099)) ;
#72272=CARTESIAN_POINT('Ctrl Pts',(-19.7507413265395,-11.5241031117976,
124.880139860479)) ;
#72273=CARTESIAN_POINT('Ctrl Pts',(-19.6824420883012,-11.3441140313788,
124.586475461409)) ;
#72274=CARTESIAN_POINT('Ctrl Pts',(-19.9977235239071,-11.5339873913395,
124.799620909401)) ;
#72275=CARTESIAN_POINT('Ctrl Pts',(-19.8800272541223,-11.3539983109207,
124.522061213482)) ;
#72276=CARTESIAN_POINT('Ctrl Pts',(-20.2297217101935,-11.5439821726314,
124.676533838813)) ;
#72277=CARTESIAN_POINT('Ctrl Pts',(-20.0656260392352,-11.3639930922127,
124.423592342302)) ;
#72278=CARTESIAN_POINT('Ctrl Pts',(-20.4358226950953,-11.5539300178182,
124.51568737912)) ;
#72279=CARTESIAN_POINT('Ctrl Pts',(-20.2305069652934,-11.3739409373994,
124.294916057216)) ;
#72280=CARTESIAN_POINT('Ctrl Pts',(-20.6109276227869,-11.5638669812056,
124.321995034951)) ;
#72281=CARTESIAN_POINT('Ctrl Pts',(-20.37059121164,-11.3838779007868,124.139963144074)) ;
#72282=CARTESIAN_POINT('Ctrl Pts',(-20.7506923360164,-11.5738499459428,
124.099943607962)) ;
#72283=CARTESIAN_POINT('Ctrl Pts',(-20.482403674932,-11.3938608655241,123.962322680992)) ;
#72284=CARTESIAN_POINT('Ctrl Pts',(-20.849910076086,-11.5838937973584,123.855392878885)) ;
#72285=CARTESIAN_POINT('Ctrl Pts',(-20.561778696542,-11.4039047169397,123.766682270914)) ;
#72286=CARTESIAN_POINT('Ctrl Pts',(-20.9045834154324,-11.5937219986932,
123.602930177821)) ;
#72287=CARTESIAN_POINT('Ctrl Pts',(-20.6055180794411,-11.4137329182744,
123.5647134447)) ;
#72288=CARTESIAN_POINT('Ctrl Pts',(-20.9149654650687,-11.6037985712912,
123.338386769832)) ;
#72289=CARTESIAN_POINT('Ctrl Pts',(-20.6138247398722,-11.4238094908725,
123.353078412637)) ;
#72290=CARTESIAN_POINT('Ctrl Pts',(-20.8801663078721,-11.6136506512988,
123.081776137411)) ;
#72291=CARTESIAN_POINT('Ctrl Pts',(-20.5859865727851,-11.43366157088,123.147790745259)) ;
#72292=CARTESIAN_POINT('Ctrl Pts',(-20.7998144513112,-11.6237239363029,
122.82959680017)) ;
#72293=CARTESIAN_POINT('Ctrl Pts',(-20.5217060262302,-11.4437348558841,
122.946046639568)) ;
#72294=CARTESIAN_POINT('Ctrl Pts',(-20.6796373591694,-11.6335652880134,
122.600571403719)) ;
#72295=CARTESIAN_POINT('Ctrl Pts',(-20.4255657854105,-11.4535762075946,
122.762826748449)) ;
#72296=CARTESIAN_POINT('Ctrl Pts',(-20.5203770952536,-11.6435267874099,
122.392832222546)) ;
#72297=CARTESIAN_POINT('Ctrl Pts',(-20.2981587895807,-11.4635377069911,
122.59663487523)) ;
#72298=CARTESIAN_POINT('Ctrl Pts',(-20.3256964581536,-11.6535625635399,
122.214906329216)) ;
#72299=CARTESIAN_POINT('Ctrl Pts',(-20.1424150134632,-11.4735734831211,
122.454293226116)) ;
#72300=CARTESIAN_POINT('Ctrl Pts',(-20.1065035193334,-11.6634509901774,
122.075338994237)) ;
#72301=CARTESIAN_POINT('Ctrl Pts',(-19.9670619537043,-11.4834619097587,
122.34263870474)) ;
#72302=CARTESIAN_POINT('Ctrl Pts',(-19.863504629617,-11.6734663122523,121.97420927489)) ;
#72303=CARTESIAN_POINT('Ctrl Pts',(-19.7726633636097,-11.4934772318336,
122.261733686333)) ;
#72304=CARTESIAN_POINT('Ctrl Pts',(-19.6061275734834,-11.6834966611526,
121.917323321507)) ;
#72305=CARTESIAN_POINT('Ctrl Pts',(-19.5667619143694,-11.5035075807338,
122.216223718493)) ;
#72306=CARTESIAN_POINT('Ctrl Pts',(-19.3477206075202,-11.6933400367592,
121.905682077729)) ;
#72307=CARTESIAN_POINT('Ctrl Pts',(-19.3600373704475,-11.5133509563405,
122.206909440148)) ;
#72308=CARTESIAN_POINT('Ctrl Pts',(-19.0862848802526,-11.7033694736564,
121.939135039811)) ;
#72309=CARTESIAN_POINT('Ctrl Pts',(-19.1508885485966,-11.5233803932376,
122.233670378294)) ;
#72310=CARTESIAN_POINT('Ctrl Pts',(-18.8347782583874,-11.7134013515893,
122.018183059093)) ;
#72311=CARTESIAN_POINT('Ctrl Pts',(-18.9496827948867,-11.5334122711706,
122.296907572202)) ;
#72312=CARTESIAN_POINT('Ctrl Pts',(-18.605313347461,-11.7232309746948,122.136772150878)) ;
#72313=CARTESIAN_POINT('Ctrl Pts',(-18.7661111198526,-11.543241894276,122.391777125529)) ;
#72314=CARTESIAN_POINT('Ctrl Pts',(-18.3960907644608,-11.7332204458479,
122.295336373502)) ;
#72315=CARTESIAN_POINT('Ctrl Pts',(-18.5987322188273,-11.5532313654291,
122.518627168111)) ;
#72316=CARTESIAN_POINT('Ctrl Pts',(-18.2171052462607,-11.7432642946103,
122.489315907986)) ;
#72317=CARTESIAN_POINT('Ctrl Pts',(-18.4555426693397,-11.5632752141915,
122.673809908671)) ;
#72318=CARTESIAN_POINT('Ctrl Pts',(-18.0772224087979,-11.753086000142,122.706227559869)) ;
#72319=CARTESIAN_POINT('Ctrl Pts',(-18.3436356441143,-11.5730969197232,
122.847337557249)) ;
#72320=CARTESIAN_POINT('Ctrl Pts',(-17.9743582755339,-11.7631210399698,
122.949047320003)) ;
#72321=CARTESIAN_POINT('Ctrl Pts',(-18.2613427735164,-11.583131959551,123.041592794472)) ;
#72322=CARTESIAN_POINT('Ctrl Pts',(-17.9159869175349,-11.7731457468612,
123.20594742871)) ;
#72323=CARTESIAN_POINT('Ctrl Pts',(-18.2146441954026,-11.5931566664425,
123.247112562016)) ;
#72324=CARTESIAN_POINT('Ctrl Pts',(-17.9027824759829,-11.782998451202,123.464529062488)) ;
#72325=CARTESIAN_POINT('Ctrl Pts',(-18.2040790568452,-11.6030093707832,
123.453976982937)) ;
#72326=CARTESIAN_POINT('Ctrl Pts',(-17.9346582754265,-11.7929865734097,
123.725044751909)) ;
#72327=CARTESIAN_POINT('Ctrl Pts',(-18.2295779793896,-11.6129974929909,
123.662389596345)) ;
#72328=CARTESIAN_POINT('Ctrl Pts',(-18.0108208429798,-11.802915043517,123.97459768502)) ;
#72329=CARTESIAN_POINT('Ctrl Pts',(-18.290506276576,-11.6229259630982,123.862032045727)) ;
#72330=CARTESIAN_POINT('Ctrl Pts',(-18.1294925171115,-11.8129040206842,
124.208755459199)) ;
#72331=CARTESIAN_POINT('Ctrl Pts',(-18.3854419582014,-11.6329149402654,
124.049358946099)) ;
#72332=CARTESIAN_POINT('Ctrl Pts',(-18.2881378410589,-11.8229418279639,
124.419490767669)) ;
#72333=CARTESIAN_POINT('Ctrl Pts',(-18.5123568914905,-11.6429527475451,
124.217948275703)) ;
#72334=CARTESIAN_POINT('Ctrl Pts',(-18.4770035096393,-11.8327881288271,
124.596360779288)) ;
#72335=CARTESIAN_POINT('Ctrl Pts',(-18.6634476664908,-11.6527990484084,
124.359445074232)) ;
#72336=CARTESIAN_POINT('Ctrl Pts',(-18.6973386410896,-11.8428138722065,
124.740820127124)) ;
#72337=CARTESIAN_POINT('Ctrl Pts',(-18.8397147708248,-11.6628247917877,
124.47501413786)) ;
#72338=CARTESIAN_POINT('Ctrl Pts',(-18.9398076656902,-11.8528447386455,
124.84425093062)) ;
#72339=CARTESIAN_POINT('Ctrl Pts',(-19.0336893273778,-11.6728556582267,
124.557760414888)) ;
#72340=CARTESIAN_POINT('Ctrl Pts',(-19.1914647637009,-11.8626820974443,
124.903358127401)) ;
#72341=CARTESIAN_POINT('Ctrl Pts',(-19.2350138511474,-11.6826930170255,
124.605047798239)) ;
#72342=CARTESIAN_POINT('Ctrl Pts',(-19.4535879451871,-11.872674058378,124.918802859936)) ;
#72343=CARTESIAN_POINT('Ctrl Pts',(-19.4447121787566,-11.6926849779593,
124.617405527106)) ;
#72344=CARTESIAN_POINT('Ctrl Pts',(-19.7154151681475,-11.8827064209346,
124.887849956771)) ;
#72345=CARTESIAN_POINT('Ctrl Pts',(-19.6541742063547,-11.7027173405158,
124.592645060716)) ;
#72346=CARTESIAN_POINT('Ctrl Pts',(-19.963751398213,-11.892571581509,124.813477415183)) ;
#72347=CARTESIAN_POINT('Ctrl Pts',(-19.8528431830511,-11.7125825010902,
124.533149033972)) ;
#72348=CARTESIAN_POINT('Ctrl Pts',(-20.1980246865073,-11.9025334860867,
124.696630723428)) ;
#72349=CARTESIAN_POINT('Ctrl Pts',(-20.0402625347496,-11.7225444056679,
124.439673577518)) ;
#72350=CARTESIAN_POINT('Ctrl Pts',(-20.4097188088808,-11.9125684161624,
124.539405883201)) ;
#72351=CARTESIAN_POINT('Ctrl Pts',(-20.2096190243359,-11.7325793357437,
124.313895264542)) ;
#72352=CARTESIAN_POINT('Ctrl Pts',(-20.5885436051697,-11.922453363016,124.350939834782)) ;
#72353=CARTESIAN_POINT('Ctrl Pts',(-20.3526800140608,-11.7424642825973,
124.163124141174)) ;
#72354=CARTESIAN_POINT('Ctrl Pts',(-20.7344544462776,-11.9325190393275,
124.13036082964)) ;
#72355=CARTESIAN_POINT('Ctrl Pts',(-20.4694104306545,-11.7525299589087,
123.986661948345)) ;
#72356=CARTESIAN_POINT('Ctrl Pts',(-20.8377538536608,-11.9423579589624,
123.89328858745)) ;
#72357=CARTESIAN_POINT('Ctrl Pts',(-20.5520516016734,-11.7623688785436,
123.797005487303)) ;
#72358=CARTESIAN_POINT('Ctrl Pts',(-20.9000168314442,-11.9524214686968,
123.636302931603)) ;
#72359=CARTESIAN_POINT('Ctrl Pts',(-20.6018640323336,-11.7724323882781,
123.591417349548)) ;
#72360=CARTESIAN_POINT('Ctrl Pts',(-20.9162207082288,-11.9623150818586,
123.376783859033)) ;
#72361=CARTESIAN_POINT('Ctrl Pts',(-20.6148291614224,-11.7823260014398,
123.383802596767)) ;
#72362=CARTESIAN_POINT('Ctrl Pts',(-20.887664564412,-11.972259088672,123.117066234083)) ;
#72363=CARTESIAN_POINT('Ctrl Pts',(-20.5919863882844,-11.7922700082532,
123.176028481019)) ;
#72364=CARTESIAN_POINT('Ctrl Pts',(-20.8141243156859,-11.9822600430263,
122.864708641766)) ;
#72365=CARTESIAN_POINT('Ctrl Pts',(-20.5331562591136,-11.8022709626075,
122.974141872013)) ;
#72366=CARTESIAN_POINT('Ctrl Pts',(-20.697050499779,-11.9922988007186,122.628327620954)) ;
#72367=CARTESIAN_POINT('Ctrl Pts',(-20.4394990793776,-11.8123097202998,
122.78503611631)) ;
#72368=CARTESIAN_POINT('Ctrl Pts',(-20.5444825752597,-12.0021229848886,
122.420035360942)) ;
#72369=CARTESIAN_POINT('Ctrl Pts',(-20.3174467467038,-11.8221339044698,
122.618401417283)) ;
#72370=CARTESIAN_POINT('Ctrl Pts',(-20.3539293396122,-12.012181050488,122.236896566253)) ;
#72371=CARTESIAN_POINT('Ctrl Pts',(-20.1650056265507,-11.8321919700692,
122.471888771544)) ;
#72372=CARTESIAN_POINT('Ctrl Pts',(-20.1370409747598,-12.0221110972627,
122.09176436793)) ;
#72373=CARTESIAN_POINT('Ctrl Pts',(-19.9914963147766,-11.8421220168439,
122.355781349936)) ;
#72374=CARTESIAN_POINT('Ctrl Pts',(-19.8980237231971,-12.0320625395998,
121.98564356461)) ;
#72375=CARTESIAN_POINT('Ctrl Pts',(-19.8002835442428,-11.8520734591811,
122.270882756195)) ;
#72376=CARTESIAN_POINT('Ctrl Pts',(-19.6416983085851,-12.0421093367791,
121.922384338885)) ;
#72377=CARTESIAN_POINT('Ctrl Pts',(-19.5952237285874,-11.8621202563603,
122.220273262082)) ;
#72378=CARTESIAN_POINT('Ctrl Pts',(-19.3835093232659,-12.0519572774592,
121.904703348249)) ;
#72379=CARTESIAN_POINT('Ctrl Pts',(-19.3886730067727,-11.8719681970404,
122.206126303218)) ;
#72380=CARTESIAN_POINT('Ctrl Pts',(-19.1231275997135,-12.0619189088018,
121.931627958195)) ;
#72381=CARTESIAN_POINT('Ctrl Pts',(-19.1803674964563,-11.881929828383,122.227663754114)) ;
#72382=CARTESIAN_POINT('Ctrl Pts',(-18.869747044229,-12.0719475681777,122.00416367076)) ;
#72383=CARTESIAN_POINT('Ctrl Pts',(-18.9776624753786,-11.8919584877589,
122.28569018209)) ;
#72384=CARTESIAN_POINT('Ctrl Pts',(-18.6355935849855,-12.0818578710659,
122.118142693062)) ;
#72385=CARTESIAN_POINT('Ctrl Pts',(-18.7903388847647,-11.9018687906471,
122.376871325098)) ;
#72386=CARTESIAN_POINT('Ctrl Pts',(-18.4238474019215,-12.0917927656281,
122.270883952983)) ;
#72387=CARTESIAN_POINT('Ctrl Pts',(-18.6209407077585,-11.9118036852093,
122.49906244756)) ;
#72388=CARTESIAN_POINT('Ctrl Pts',(-18.2400799717169,-12.101833864295,122.46023114314)) ;
#72389=CARTESIAN_POINT('Ctrl Pts',(-18.4739251815215,-11.9218447838762,
122.650538612055)) ;
#72390=CARTESIAN_POINT('Ctrl Pts',(-18.0940875092482,-12.1117211467993,
122.675182672161)) ;
#72391=CARTESIAN_POINT('Ctrl Pts',(-18.3571294254557,-11.9317320663806,
122.822498468009)) ;
#72392=CARTESIAN_POINT('Ctrl Pts',(-17.9861176822328,-12.1217128873099,
122.914511116788)) ;
#72393=CARTESIAN_POINT('Ctrl Pts',(-18.2707515313325,-11.9417238068911,
123.013960245955)) ;
#72394=CARTESIAN_POINT('Ctrl Pts',(-17.9216897295086,-12.1316634365453,
123.167952928715)) ;
#72395=CARTESIAN_POINT('Ctrl Pts',(-18.2192070041483,-11.9516743561265,
123.216713069332)) ;
#72396=CARTESIAN_POINT('Ctrl Pts',(-17.9018892647571,-12.1415991141801,
123.428284203219)) ;
#72397=CARTESIAN_POINT('Ctrl Pts',(-18.203364387403,-11.9616100337613,123.424977867107)) ;
#72398=CARTESIAN_POINT('Ctrl Pts',(-17.9274444397156,-12.1515845319728,
123.689463440896)) ;
#72399=CARTESIAN_POINT('Ctrl Pts',(-18.2238062820509,-11.9715954515541,
123.633921427947)) ;
#72400=CARTESIAN_POINT('Ctrl Pts',(-17.9985764204831,-12.1616133248434,
123.94322681677)) ;
#72401=CARTESIAN_POINT('Ctrl Pts',(-18.2807096769127,-11.9816242444246,
123.836932670854)) ;
#72402=CARTESIAN_POINT('Ctrl Pts',(-18.1107411249802,-12.1714928360713,
124.177366527425)) ;
#72403=CARTESIAN_POINT('Ctrl Pts',(-18.3704394042732,-11.9915037556526,
124.024245403531)) ;
#72404=CARTESIAN_POINT('Ctrl Pts',(-18.2631174664648,-12.1814863727443,
124.391272663534)) ;
#72405=CARTESIAN_POINT('Ctrl Pts',(-18.4923386313118,-12.0014972923255,
124.195371583237)) ;
#72406=CARTESIAN_POINT('Ctrl Pts',(-18.4514152852982,-12.1915186410081,
124.575779592077)) ;
#72407=CARTESIAN_POINT('Ctrl Pts',(-18.6429752478029,-12.0115295605894,
124.342978676221)) ;
#72408=CARTESIAN_POINT('Ctrl Pts',(-18.6649582254525,-12.201382603014,124.722768521375)) ;
#72409=CARTESIAN_POINT('Ctrl Pts',(-18.813808386405,-12.0213935225952,124.460571699597)) ;
#72410=CARTESIAN_POINT('Ctrl Pts',(-18.9056381213236,-12.2114526643589,
124.83271375166)) ;
#72411=CARTESIAN_POINT('Ctrl Pts',(-19.0063512619196,-12.0314635839401,
124.548529868389)) ;
#72412=CARTESIAN_POINT('Ctrl Pts',(-19.1560012005584,-12.2212950287076,
124.897694900667)) ;
#72413=CARTESIAN_POINT('Ctrl Pts',(-19.2066412928752,-12.0413059482889,
124.600516988053)) ;
#72414=CARTESIAN_POINT('Ctrl Pts',(-19.4168488001021,-12.2312557012101,
124.919426126798)) ;
#72415=CARTESIAN_POINT('Ctrl Pts',(-19.4153192326186,-12.0512666207913,
124.617904150398)) ;
#72416=CARTESIAN_POINT('Ctrl Pts',(-19.6794781670502,-12.2412937722779,
124.894826056508)) ;
#72417=CARTESIAN_POINT('Ctrl Pts',(-19.6254228033852,-12.0613046918591,
124.598226319022)) ;
#72418=CARTESIAN_POINT('Ctrl Pts',(-19.9298584470628,-12.2511673872383,
124.826609084819)) ;
#72419=CARTESIAN_POINT('Ctrl Pts',(-19.82572781557,-12.0711783068196,124.543654773306)) ;
#72420=CARTESIAN_POINT('Ctrl Pts',(-20.1692027686012,-12.2612396218196,
124.713703674944)) ;
#72421=CARTESIAN_POINT('Ctrl Pts',(-20.0172039403952,-12.0812505414008,
124.45333259084)) ;
#72422=CARTESIAN_POINT('Ctrl Pts',(-20.3802336085162,-12.2710636402683,
124.564901741631)) ;
#72423=CARTESIAN_POINT('Ctrl Pts',(-20.1860304834579,-12.0910745598496,
124.334292311524)) ;
#72424=CARTESIAN_POINT('Ctrl Pts',(-20.5668505339753,-12.2811285612444,
124.37754684746)) ;
#72425=CARTESIAN_POINT('Ctrl Pts',(-20.3353241585353,-12.1011394808256,
124.184411132778)) ;
#72426=CARTESIAN_POINT('Ctrl Pts',(-20.7654710389229,-12.2943388595391,
124.09273138074)) ;
#72427=CARTESIAN_POINT('Ctrl Pts',(-20.4942292379436,-12.1143497791204,
123.9565547192)) ;
#72428=CARTESIAN_POINT('Ctrl Pts',(-20.8864681735863,-12.3076543062711,
123.760293059353)) ;
#72429=CARTESIAN_POINT('Ctrl Pts',(-20.5910323501045,-12.1276652258523,
123.690569694297)) ;
#72430=CARTESIAN_POINT('Ctrl Pts',(-20.9168412403421,-12.3209445515383,
123.412248798329)) ;
#72431=CARTESIAN_POINT('Ctrl Pts',(-20.6153241110925,-12.1409554711196,
123.412181858016)) ;
#72432=CARTESIAN_POINT('Ctrl Pts',(-20.8936136565225,-12.3309953011455,
123.149204261567)) ;
#72433=CARTESIAN_POINT('Ctrl Pts',(-20.5967459980804,-12.1510062207267,
123.20173670269)) ;
#72434=CARTESIAN_POINT('Ctrl Pts',(-20.8271599101353,-12.3408079081277,
122.900008574074)) ;
#72435=CARTESIAN_POINT('Ctrl Pts',(-20.5435845615401,-12.160818827709,123.002381693859)) ;
#72436=CARTESIAN_POINT('Ctrl Pts',(-20.7159339873303,-12.350879006122,122.659895486388)) ;
#72437=CARTESIAN_POINT('Ctrl Pts',(-20.4546048866285,-12.1708899257032,
122.810289464688)) ;
#72438=CARTESIAN_POINT('Ctrl Pts',(-20.567182547186,-12.3607685788968,122.446765213272)) ;
#72439=CARTESIAN_POINT('Ctrl Pts',(-20.3356088789073,-12.1807794984781,
122.639785845869)) ;
#72440=CARTESIAN_POINT('Ctrl Pts',(-20.3217335958412,-12.3740386857001,
122.1990367701)) ;
#72441=CARTESIAN_POINT('Ctrl Pts',(-20.1392327070889,-12.1940496052814,
122.441591581826)) ;
#72442=CARTESIAN_POINT('Ctrl Pts',(-19.9402799223617,-12.3906553726226,
121.976489963094)) ;
#72443=CARTESIAN_POINT('Ctrl Pts',(-19.8341061887492,-12.2106662922039,
122.263562894215)) ;
#72444=CARTESIAN_POINT('Ctrl Pts',(-19.5069560654144,-12.4072294159389,
121.897341845793)) ;
#72445=CARTESIAN_POINT('Ctrl Pts',(-19.4873858330109,-12.2272403355201,
122.200234744545)) ;
#72446=CARTESIAN_POINT('Ctrl Pts',(-19.1586250795986,-12.4205259833707,
121.925240968609)) ;
#72447=CARTESIAN_POINT('Ctrl Pts',(-19.2087707820573,-12.2405369029519,
122.222555129474)) ;
#72448=CARTESIAN_POINT('Ctrl Pts',(-18.903549791528,-12.4305560469481,121.991664800818)) ;
#72449=CARTESIAN_POINT('Ctrl Pts',(-19.0046999503751,-12.2505669665293,
122.275692101065)) ;
#72450=CARTESIAN_POINT('Ctrl Pts',(-18.6671468528591,-12.4404499387973,
122.099840645891)) ;
#72451=CARTESIAN_POINT('Ctrl Pts',(-18.8155801630729,-12.2604608583786,
122.362230133135)) ;
#72452=CARTESIAN_POINT('Ctrl Pts',(-18.3796682060552,-12.4537026945829,
122.296549637397)) ;
#72453=CARTESIAN_POINT('Ctrl Pts',(-18.5855889437377,-12.2737136141641,
122.519603145883)) ;
#72454=CARTESIAN_POINT('Ctrl Pts',(-18.0908280312836,-12.4704307995753,
122.63446210067)) ;
#72455=CARTESIAN_POINT('Ctrl Pts',(-18.3545219823308,-12.2904417191566,
122.789922698833)) ;
#72456=CARTESIAN_POINT('Ctrl Pts',(-17.9056069776855,-12.4902616360538,
123.128014485506)) ;
#72457=CARTESIAN_POINT('Ctrl Pts',(-18.2063394436304,-12.3102725556351,
123.184767136768)) ;
#72458=CARTESIAN_POINT('Ctrl Pts',(-17.8986058473091,-12.5101870279439,
123.657435239685)) ;
#72459=CARTESIAN_POINT('Ctrl Pts',(-18.2007363231524,-12.3301979475252,
123.608303576448)) ;
#72460=CARTESIAN_POINT('Ctrl Pts',(-18.0728134811667,-12.530112241296,124.157630024476)) ;
#72461=CARTESIAN_POINT('Ctrl Pts',(-18.3400999156776,-12.3501231608772,
124.00846101179)) ;
#72462=CARTESIAN_POINT('Ctrl Pts',(-18.407056128328,-12.5500372547811,124.568319257419)) ;
#72463=CARTESIAN_POINT('Ctrl Pts',(-18.6074925126866,-12.3700481743623,
124.337014427016)) ;
#72464=CARTESIAN_POINT('Ctrl Pts',(-18.8599799730915,-12.5699137264811,
124.840308097054)) ;
#72465=CARTESIAN_POINT('Ctrl Pts',(-18.9698314340081,-12.3899246460623,
124.554607919997)) ;
#72466=CARTESIAN_POINT('Ctrl Pts',(-19.3811313633276,-12.5898930443899,
124.94215813979)) ;
#72467=CARTESIAN_POINT('Ctrl Pts',(-19.3867523851537,-12.4099039639712,
124.636089848104)) ;
#72468=CARTESIAN_POINT('Ctrl Pts',(-19.904526260355,-12.6098260479659,124.859844414559)) ;
#72469=CARTESIAN_POINT('Ctrl Pts',(-19.8054692095567,-12.4298369675472,
124.570240637955)) ;
#72470=CARTESIAN_POINT('Ctrl Pts',(-20.3677432424787,-12.6297213179936,
124.604878989374)) ;
#72471=CARTESIAN_POINT('Ctrl Pts',(-20.1760444928505,-12.4497322375749,
124.366269105617)) ;
#72472=CARTESIAN_POINT('Ctrl Pts',(-20.7170498596776,-12.6496426558995,
124.206944794336)) ;
#72473=CARTESIAN_POINT('Ctrl Pts',(-20.4554911883008,-12.4696535754807,
124.047921837557)) ;
#72474=CARTESIAN_POINT('Ctrl Pts',(-20.9098403566524,-12.6696002791656,
123.71275120436)) ;
#72475=CARTESIAN_POINT('Ctrl Pts',(-20.6097246738742,-12.4896111987469,
123.652566906432)) ;
#72476=CARTESIAN_POINT('Ctrl Pts',(-20.922485985097,-12.6894801111229,123.184612097155)) ;
#72477=CARTESIAN_POINT('Ctrl Pts',(-20.6198419805455,-12.5094910307041,
123.230054122359)) ;
#72478=CARTESIAN_POINT('Ctrl Pts',(-20.7554545445887,-12.7093619624198,
122.683172172791)) ;
#72479=CARTESIAN_POINT('Ctrl Pts',(-20.4862161995466,-12.529372882001,122.828900805559)) ;
#72480=CARTESIAN_POINT('Ctrl Pts',(-20.4235254244921,-12.7294329795236,
122.265649140975)) ;
#72481=CARTESIAN_POINT('Ctrl Pts',(-20.2206735911977,-12.5494438991048,
122.494883034392)) ;
#72482=CARTESIAN_POINT('Ctrl Pts',(-19.9749237655552,-12.7492402032767,
121.989968961394)) ;
#72483=CARTESIAN_POINT('Ctrl Pts',(-19.8617900839095,-12.5692511228579,
122.274337697005)) ;
#72484=CARTESIAN_POINT('Ctrl Pts',(-19.4550399386811,-12.7692213388454,
121.881799009458)) ;
#72485=CARTESIAN_POINT('Ctrl Pts',(-19.4458826423283,-12.5892322584267,
122.18780260183)) ;
#72486=CARTESIAN_POINT('Ctrl Pts',(-18.9310095255379,-12.7891488321847,
121.958350587215)) ;
#72487=CARTESIAN_POINT('Ctrl Pts',(-19.0266575304228,-12.6091597517659,
122.24904461452)) ;
#72488=CARTESIAN_POINT('Ctrl Pts',(-18.4660378435097,-12.8089694935425,
122.206286369138)) ;
#72489=CARTESIAN_POINT('Ctrl Pts',(-18.6546792788745,-12.6289804131237,
122.447395528075)) ;
#72490=CARTESIAN_POINT('Ctrl Pts',(-18.1095237057662,-12.8290666827643,
122.603786127355)) ;
#72491=CARTESIAN_POINT('Ctrl Pts',(-18.3694696834846,-12.6490776023455,
122.765395547961)) ;
#72492=CARTESIAN_POINT('Ctrl Pts',(-17.9128685241176,-12.8488303617726,
123.091145395857)) ;
#72493=CARTESIAN_POINT('Ctrl Pts',(-18.212146236786,-12.6688412813539,123.155285756016)) ;
#72494=CARTESIAN_POINT('Ctrl Pts',(-17.8934532249177,-12.8688876404457,
123.623648070247)) ;
#72495=CARTESIAN_POINT('Ctrl Pts',(-18.1966161448372,-12.6888985600269,
123.581287459871)) ;
#72496=CARTESIAN_POINT('Ctrl Pts',(-18.0551868057906,-12.8886830641931,
124.124451004265)) ;
#72497=CARTESIAN_POINT('Ctrl Pts',(-18.3260055893083,-12.7086939837743,
123.981930874229)) ;
#72498=CARTESIAN_POINT('Ctrl Pts',(-18.379428806349,-12.9086467089207,124.544379679897)) ;
#72499=CARTESIAN_POINT('Ctrl Pts',(-18.5854015952883,-12.7286576285019,
124.317872293328)) ;
#72500=CARTESIAN_POINT('Ctrl Pts',(-18.8287006511191,-12.9286302001948,
124.827680379783)) ;
#72501=CARTESIAN_POINT('Ctrl Pts',(-18.9448205353017,-12.748641119776,124.544510768176)) ;
#72502=CARTESIAN_POINT('Ctrl Pts',(-19.342918686626,-12.9484376953441,124.940731620075)) ;
#72503=CARTESIAN_POINT('Ctrl Pts',(-19.3561969576373,-12.7684486149253,
124.634949144309)) ;
#72504=CARTESIAN_POINT('Ctrl Pts',(-19.8693844497471,-12.9684202860642,
124.871533418485)) ;
#72505=CARTESIAN_POINT('Ctrl Pts',(-19.7773692207012,-12.7884312056454,
124.579587326227)) ;
#72506=CARTESIAN_POINT('Ctrl Pts',(-20.3384447755248,-12.9883029400554,
124.627871581424)) ;
#72507=CARTESIAN_POINT('Ctrl Pts',(-20.1526165530644,-12.8083138596367,
124.384654591439)) ;
#72508=CARTESIAN_POINT('Ctrl Pts',(-20.6976976848922,-13.0082611849185,
124.237731507695)) ;
#72509=CARTESIAN_POINT('Ctrl Pts',(-20.4400164509615,-12.8282721044997,
124.072539967842)) ;
#72510=CARTESIAN_POINT('Ctrl Pts',(-20.9017768870184,-13.0281367719601,
123.750397269465)) ;
#72511=CARTESIAN_POINT('Ctrl Pts',(-20.6032766081325,-12.8481476915413,
123.682670590867)) ;
#72512=CARTESIAN_POINT('Ctrl Pts',(-20.9278087944924,-13.0481176600953,
123.220011471914)) ;
#72513=CARTESIAN_POINT('Ctrl Pts',(-20.6240984650254,-12.8681285796766,
123.258361753543)) ;
#72514=CARTESIAN_POINT('Ctrl Pts',(-20.7712144054665,-13.0680528012063,
122.713763278184)) ;
#72515=CARTESIAN_POINT('Ctrl Pts',(-20.4988186174616,-12.8880637207876,
122.853363994619)) ;
#72516=CARTESIAN_POINT('Ctrl Pts',(-20.4520106816662,-13.0879648192174,
122.291696114203)) ;
#72517=CARTESIAN_POINT('Ctrl Pts',(-20.2434545045575,-12.9079757387987,
122.515712746724)) ;
#72518=CARTESIAN_POINT('Ctrl Pts',(-20.0087285877689,-13.107853037461,122.003722192622)) ;
#72519=CARTESIAN_POINT('Ctrl Pts',(-19.8888179313836,-12.9278639570422,
122.285335578687)) ;
#72520=CARTESIAN_POINT('Ctrl Pts',(-19.5791090604669,-13.1244513413079,
121.903703056127)) ;
#72521=CARTESIAN_POINT('Ctrl Pts',(-19.5451473403849,-12.9444622608891,
122.20532771232)) ;
#72522=CARTESIAN_POINT('Ctrl Pts',(-19.2304680801344,-13.1377239312107,
121.914976366531)) ;
#72523=CARTESIAN_POINT('Ctrl Pts',(-19.2662110826215,-12.957734850792,122.214345972793)) ;
#72524=CARTESIAN_POINT('Ctrl Pts',(-18.9730360739055,-13.1477313461616,
121.968723010313)) ;
#72525=CARTESIAN_POINT('Ctrl Pts',(-19.0602727214037,-12.9677422657428,
122.25734421058)) ;
#72526=CARTESIAN_POINT('Ctrl Pts',(-18.728923774741,-13.1577386928942,122.066570256233)) ;
#72527=CARTESIAN_POINT('Ctrl Pts',(-18.8649743141328,-12.9777496124754,
122.335631001214)) ;
#72528=CARTESIAN_POINT('Ctrl Pts',(-18.4326373531088,-13.1710050526958,
122.250316913769)) ;
#72529=CARTESIAN_POINT('Ctrl Pts',(-18.6279877739114,-12.991015972277,122.482594753417)) ;
#72530=CARTESIAN_POINT('Ctrl Pts',(-18.1316373287042,-13.1875197103187,
122.569692622232)) ;
#72531=CARTESIAN_POINT('Ctrl Pts',(-18.3871406493088,-13.0075306299,122.738147077933)) ;
#72532=CARTESIAN_POINT('Ctrl Pts',(-17.9558681006143,-13.2041171435614,
122.974265631464)) ;
#72533=CARTESIAN_POINT('Ctrl Pts',(-18.2465546550527,-13.0241280631426,
123.061762709622)) ;
#72534=CARTESIAN_POINT('Ctrl Pts',(-17.9045373895887,-13.2174651407064,
123.321302564887)) ;
#72535=CARTESIAN_POINT('Ctrl Pts',(-18.20548016203,-13.0374760602876,123.339423056025)) ;
#72536=CARTESIAN_POINT('Ctrl Pts',(-17.9113737957026,-13.227360895058,123.581262925392)) ;
#72537=CARTESIAN_POINT('Ctrl Pts',(-18.2109541050246,-13.0473718146392,
123.547385244145)) ;
#72538=CARTESIAN_POINT('Ctrl Pts',(-17.9634088820115,-13.2373488489893,
123.838506352565)) ;
#72539=CARTESIAN_POINT('Ctrl Pts',(-18.2525836755494,-13.0573597685706,
123.753181135679)) ;
#72540=CARTESIAN_POINT('Ctrl Pts',(-18.0589349738846,-13.2473060726941,
124.082144873692)) ;
#72541=CARTESIAN_POINT('Ctrl Pts',(-18.3290068212281,-13.0673169922753,
123.948090676495)) ;
#72542=CARTESIAN_POINT('Ctrl Pts',(-18.1964661585353,-13.2573416192507,
124.307146372521)) ;
#72543=CARTESIAN_POINT('Ctrl Pts',(-18.4390335973166,-13.077352538832,124.128090758229)) ;
#72544=CARTESIAN_POINT('Ctrl Pts',(-18.368270053298,-13.2672287305268,124.502082982774)) ;
#72545=CARTESIAN_POINT('Ctrl Pts',(-18.576478424902,-13.0872396501081,124.284038539208)) ;
#72546=CARTESIAN_POINT('Ctrl Pts',(-18.5731686000291,-13.2772201356277,
124.66624633591)) ;
#72547=CARTESIAN_POINT('Ctrl Pts',(-18.7403986257916,-13.0972310552089,
124.415367430382)) ;
#72548=CARTESIAN_POINT('Ctrl Pts',(-18.8024527486547,-13.2871657568424,
124.791696662214)) ;
#72549=CARTESIAN_POINT('Ctrl Pts',(-18.9238269941468,-13.1071766764237,
124.515725689855)) ;
#72550=CARTESIAN_POINT('Ctrl Pts',(-19.0499707909239,-13.2971150051108,
124.875968223261)) ;
#72551=CARTESIAN_POINT('Ctrl Pts',(-19.1218420945713,-13.117125924692,124.58314078008)) ;
#72552=CARTESIAN_POINT('Ctrl Pts',(-19.3109074952324,-13.3071615002794,
124.916064204563)) ;
#72553=CARTESIAN_POINT('Ctrl Pts',(-19.3305917563602,-13.1271724198607,
124.615215324585)) ;
#72554=CARTESIAN_POINT('Ctrl Pts',(-19.5697458477352,-13.3170128430709,
124.910614060222)) ;
#72555=CARTESIAN_POINT('Ctrl Pts',(-19.5376622956873,-13.1370237626522,
124.610852953311)) ;
#72556=CARTESIAN_POINT('Ctrl Pts',(-19.8268961278623,-13.3269846231983,
124.86034740177)) ;
#72557=CARTESIAN_POINT('Ctrl Pts',(-19.7433819968767,-13.1469955427795,
124.570637436565)) ;
#72558=CARTESIAN_POINT('Ctrl Pts',(-20.0720441859134,-13.336979823176,124.76592134673)) ;
#72559=CARTESIAN_POINT('Ctrl Pts',(-19.9394995773028,-13.1569907427572,
124.495094521128)) ;
#72560=CARTESIAN_POINT('Ctrl Pts',(-20.2977248332658,-13.347013814872,124.629595035423)) ;
#72561=CARTESIAN_POINT('Ctrl Pts',(-20.1200429020722,-13.1670247344533,
124.386031555564)) ;
#72562=CARTESIAN_POINT('Ctrl Pts',(-20.4930785404937,-13.3568692198445,
124.459519571189)) ;
#72563=CARTESIAN_POINT('Ctrl Pts',(-20.2763242533844,-13.1768801394258,
124.2499696171)) ;
#72564=CARTESIAN_POINT('Ctrl Pts',(-20.6585461152762,-13.3668685176903,
124.255447402395)) ;
#72565=CARTESIAN_POINT('Ctrl Pts',(-20.4086965325383,-13.1868794372715,
124.086710531574)) ;
#72566=CARTESIAN_POINT('Ctrl Pts',(-20.7850259764522,-13.3767636302955,
124.028196369729)) ;
#72567=CARTESIAN_POINT('Ctrl Pts',(-20.509878386038,-13.1967745498767,123.904908812571)) ;
#72568=CARTESIAN_POINT('Ctrl Pts',(-20.8714967333463,-13.3868242758305,
123.778389961142)) ;
#72569=CARTESIAN_POINT('Ctrl Pts',(-20.5790529024792,-13.2068351954117,
123.705062936695)) ;
#72570=CARTESIAN_POINT('Ctrl Pts',(-20.9125557495548,-13.3966731528197,
123.522828864948)) ;
#72571=CARTESIAN_POINT('Ctrl Pts',(-20.6118978858686,-13.2166840724009,
123.500614018673)) ;
#72572=CARTESIAN_POINT('Ctrl Pts',(-20.9092102412474,-13.4067018639133,
123.259309807955)) ;
#72573=CARTESIAN_POINT('Ctrl Pts',(-20.60921931471,-13.2267127834945,123.289798833326)) ;
#72574=CARTESIAN_POINT('Ctrl Pts',(-20.8594509751279,-13.4167312651694,
123.000482346254)) ;
#72575=CARTESIAN_POINT('Ctrl Pts',(-20.5694097280133,-13.2367421847506,
123.082737285215)) ;
#72576=CARTESIAN_POINT('Ctrl Pts',(-20.7678172836453,-13.4265714569654,
122.758667592134)) ;
#72577=CARTESIAN_POINT('Ctrl Pts',(-20.4961008807738,-13.2465823765466,
122.889286615854)) ;
#72578=CARTESIAN_POINT('Ctrl Pts',(-20.6338292437807,-13.4365748861584,
122.532528062979)) ;
#72579=CARTESIAN_POINT('Ctrl Pts',(-20.3889086516706,-13.2565858057396,
122.708376145626)) ;
#72580=CARTESIAN_POINT('Ctrl Pts',(-20.4628072718296,-13.4465603986246,
122.333446821081)) ;
#72581=CARTESIAN_POINT('Ctrl Pts',(-20.2520895182278,-13.2665713182058,
122.549112622993)) ;
#72582=CARTESIAN_POINT('Ctrl Pts',(-20.2585721952877,-13.4566014950085,
122.166409914503)) ;
#72583=CARTESIAN_POINT('Ctrl Pts',(-20.0887000684384,-13.2766124145898,
122.415484760473)) ;
#72584=CARTESIAN_POINT('Ctrl Pts',(-20.0331061121513,-13.4664446909596,
122.039577187864)) ;
#72585=CARTESIAN_POINT('Ctrl Pts',(-19.9083265551085,-13.2864556105408,
122.314020659262)) ;
#72586=CARTESIAN_POINT('Ctrl Pts',(-19.7857320971706,-13.476431002014,121.952101012355)) ;
#72587=CARTESIAN_POINT('Ctrl Pts',(-19.7104267699532,-13.2964419215952,
122.2440417256)) ;
#72588=CARTESIAN_POINT('Ctrl Pts',(-19.5282010411942,-13.4863656872717,
121.908939846923)) ;
#72589=CARTESIAN_POINT('Ctrl Pts',(-19.5044018436985,-13.3063766068529,
122.209514865674)) ;
#72590=CARTESIAN_POINT('Ctrl Pts',(-19.2639488168524,-13.4964232484887,
121.911409438733)) ;
#72591=CARTESIAN_POINT('Ctrl Pts',(-19.2929999897462,-13.31643416807,122.211492628297)) ;
#72592=CARTESIAN_POINT('Ctrl Pts',(-19.010096667528,-13.5062448900973,121.958214888059)) ;
#72593=CARTESIAN_POINT('Ctrl Pts',(-19.0899192590891,-13.3262558096786,
122.248938879444)) ;
#72594=CARTESIAN_POINT('Ctrl Pts',(-18.7623301681883,-13.5163009536883,
122.050058119872)) ;
#72595=CARTESIAN_POINT('Ctrl Pts',(-18.8917066650352,-13.3363118732695,
122.322415354375)) ;
#72596=CARTESIAN_POINT('Ctrl Pts',(-18.5371012425421,-13.5262416294501,
122.182417857211)) ;
#72597=CARTESIAN_POINT('Ctrl Pts',(-18.7115247897244,-13.3462525490313,
122.428304768289)) ;
#72598=CARTESIAN_POINT('Ctrl Pts',(-18.3384782455445,-13.5361459882384,
122.350628473845)) ;
#72599=CARTESIAN_POINT('Ctrl Pts',(-18.5526279681694,-13.3561569078197,
122.562874462125)) ;
#72600=CARTESIAN_POINT('Ctrl Pts',(-18.1698329825616,-13.5461926428142,
122.553733855512)) ;
#72601=CARTESIAN_POINT('Ctrl Pts',(-18.4177132105659,-13.3662035623955,
122.725360081205)) ;
#72602=CARTESIAN_POINT('Ctrl Pts',(-18.0407519035807,-13.5560882374571,
122.779526388137)) ;
#72603=CARTESIAN_POINT('Ctrl Pts',(-18.314450248629,-13.3760991570383,122.905994658498)) ;
#72604=CARTESIAN_POINT('Ctrl Pts',(-17.9513576420596,-13.5661501841139,
123.028342279831)) ;
#72605=CARTESIAN_POINT('Ctrl Pts',(-18.2429366010411,-13.3861611036952,
123.105048152778)) ;
#72606=CARTESIAN_POINT('Ctrl Pts',(-17.9074152112643,-13.5759998080461,
123.283436990163)) ;
#72607=CARTESIAN_POINT('Ctrl Pts',(-18.2077846559609,-13.3960107276274,
123.30912358981)) ;
#72608=CARTESIAN_POINT('Ctrl Pts',(-17.9075794489119,-13.5859630470759,
123.545245160126)) ;
#72609=CARTESIAN_POINT('Ctrl Pts',(-18.2079178311045,-13.4059739666572,
123.518569875125)) ;
#72610=CARTESIAN_POINT('Ctrl Pts',(-17.953843845115,-13.5959876218518,123.804601716879)) ;
#72611=CARTESIAN_POINT('Ctrl Pts',(-18.2449311618866,-13.415998541433,123.726054822038)) ;
#72612=CARTESIAN_POINT('Ctrl Pts',(-18.0433151853354,-13.6059061845395,
124.049406829339)) ;
#72613=CARTESIAN_POINT('Ctrl Pts',(-18.3165097898856,-13.4259171041207,
123.921897880132)) ;
#72614=CARTESIAN_POINT('Ctrl Pts',(-18.1745142882444,-13.6158983712635,
124.276882942857)) ;
#72615=CARTESIAN_POINT('Ctrl Pts',(-18.4214705117975,-13.4359092908447,
124.103877785203)) ;
#72616=CARTESIAN_POINT('Ctrl Pts',(-18.3442843563145,-13.6259331698477,
124.478655912782)) ;
#72617=CARTESIAN_POINT('Ctrl Pts',(-18.5572880000568,-13.4459440894289,
124.265295042287)) ;
#72618=CARTESIAN_POINT('Ctrl Pts',(-18.542628717793,-13.6357883605213,124.645217964086)) ;
#72619=CARTESIAN_POINT('Ctrl Pts',(-18.7159640464026,-13.4557992801026,
124.398542876088)) ;
#72620=CARTESIAN_POINT('Ctrl Pts',(-18.7699291705577,-13.6457877086743,
124.776978497938)) ;
#72621=CARTESIAN_POINT('Ctrl Pts',(-18.8978051604027,-13.4657986282556,
124.503949791851)) ;
#72622=CARTESIAN_POINT('Ctrl Pts',(-19.0140681533334,-13.6556828343495,
124.86662328355)) ;
#72623=CARTESIAN_POINT('Ctrl Pts',(-19.0931163563245,-13.4756937539307,
124.57566388753)) ;
#72624=CARTESIAN_POINT('Ctrl Pts',(-19.2742712713138,-13.6657433772976,
124.913241818075)) ;
#72625=CARTESIAN_POINT('Ctrl Pts',(-19.3012793296211,-13.4857542968788,
124.612957136434)) ;
#72626=CARTESIAN_POINT('Ctrl Pts',(-19.5331191648045,-13.6755926515645,
124.914103544995)) ;
#72627=CARTESIAN_POINT('Ctrl Pts',(-19.5083568152058,-13.4956035711457,
124.613644905364)) ;
#72628=CARTESIAN_POINT('Ctrl Pts',(-19.7928781485179,-13.6856198761344,
124.869872597729)) ;
#72629=CARTESIAN_POINT('Ctrl Pts',(-19.7161637833577,-13.5056307957156,
124.578258678487)) ;
#72630=CARTESIAN_POINT('Ctrl Pts',(-20.0408282969086,-13.6956482753222,
124.780544744238)) ;
#72631=CARTESIAN_POINT('Ctrl Pts',(-19.9145234061736,-13.5156591949034,
124.506794855646)) ;
#72632=CARTESIAN_POINT('Ctrl Pts',(-20.2655486147192,-13.7054940257356,
124.652339842783)) ;
#72633=CARTESIAN_POINT('Ctrl Pts',(-20.0942981282645,-13.5255049453169,
124.404230053982)) ;
#72634=CARTESIAN_POINT('Ctrl Pts',(-20.4679785319136,-13.7154828161364,
124.485209945388)) ;
#72635=CARTESIAN_POINT('Ctrl Pts',(-20.2562410584806,-13.5354937357177,
124.270525177274)) ;
#72636=CARTESIAN_POINT('Ctrl Pts',(-20.6387470355723,-13.7255277445361,
124.283933112309)) ;
#72637=CARTESIAN_POINT('Ctrl Pts',(-20.3928547958644,-13.5455386641174,
124.109502630356)) ;
#72638=CARTESIAN_POINT('Ctrl Pts',(-20.7695822851755,-13.7353522293251,
124.061344007619)) ;
#72639=CARTESIAN_POINT('Ctrl Pts',(-20.4975212694255,-13.5553631489063,
123.931431547031)) ;
#72640=CARTESIAN_POINT('Ctrl Pts',(-20.8622650302476,-13.7454096268663,
123.813853115584)) ;
#72641=CARTESIAN_POINT('Ctrl Pts',(-20.5716663117887,-13.5654205464475,
123.733438175729)) ;
#72642=CARTESIAN_POINT('Ctrl Pts',(-20.9096073545619,-13.7553357184525,
123.557318498513)) ;
#72643=CARTESIAN_POINT('Ctrl Pts',(-20.6095387227254,-13.5753466380337,
123.528210720789)) ;
#72644=CARTESIAN_POINT('Ctrl Pts',(-20.9123708211663,-13.765290503597,123.295734355716)) ;
#72645=CARTESIAN_POINT('Ctrl Pts',(-20.6117482517937,-13.5853014231783,
123.318943754624)) ;
#72646=CARTESIAN_POINT('Ctrl Pts',(-20.8690285857303,-13.7753278732547,
123.035549479077)) ;
#72647=CARTESIAN_POINT('Ctrl Pts',(-20.5770731610732,-13.5953387928359,
123.110795969221)) ;
#72648=CARTESIAN_POINT('Ctrl Pts',(-20.7826546062724,-13.7852166833763,
122.790448432896)) ;
#72649=CARTESIAN_POINT('Ctrl Pts',(-20.5079730348007,-13.6052276029575,
122.914716243319)) ;
#72650=CARTESIAN_POINT('Ctrl Pts',(-20.6541544833678,-13.7952060424273,
122.561546360063)) ;
#72651=CARTESIAN_POINT('Ctrl Pts',(-20.4051720120301,-13.6152169620086,
122.731595301545)) ;
#72652=CARTESIAN_POINT('Ctrl Pts',(-20.4882245282182,-13.8051645898834,
122.359184923962)) ;
#72653=CARTESIAN_POINT('Ctrl Pts',(-20.2724273390847,-13.6251755094647,
122.569707182105)) ;
#72654=CARTESIAN_POINT('Ctrl Pts',(-20.2912542116433,-13.8150641664345,
122.189215690087)) ;
#72655=CARTESIAN_POINT('Ctrl Pts',(-20.1148509292206,-13.6350750860157,
122.433733053993)) ;
#72656=CARTESIAN_POINT('Ctrl Pts',(-20.0644048945388,-13.8251120782652,
122.054135819841)) ;
#72657=CARTESIAN_POINT('Ctrl Pts',(-19.9333707741338,-13.6451229978464,
122.325669994257)) ;
#72658=CARTESIAN_POINT('Ctrl Pts',(-19.8213040212545,-13.8350074261257,
121.961702812334)) ;
#72659=CARTESIAN_POINT('Ctrl Pts',(-19.7388903925254,-13.655018345707,122.251724810852)) ;
#72660=CARTESIAN_POINT('Ctrl Pts',(-19.5616299166023,-13.8450691026569,
121.912040392366)) ;
#72661=CARTESIAN_POINT('Ctrl Pts',(-19.5311506601532,-13.6650800222382,
122.211995830886)) ;
#72662=CARTESIAN_POINT('Ctrl Pts',(-19.3029437659874,-13.8549136204061,
121.908260248707)) ;
#72663=CARTESIAN_POINT('Ctrl Pts',(-19.3242027824673,-13.6749245399873,
122.208972745531)) ;
#72664=CARTESIAN_POINT('Ctrl Pts',(-19.0443926106545,-13.8648740641208,
121.949016797518)) ;
#72665=CARTESIAN_POINT('Ctrl Pts',(-19.1173623421421,-13.6848849837021,
122.241578712485)) ;
#72666=CARTESIAN_POINT('Ctrl Pts',(-18.7951065532915,-13.8749108969391,
122.035163624188)) ;
#72667=CARTESIAN_POINT('Ctrl Pts',(-18.9179336758563,-13.6949218165203,
122.310497076572)) ;
#72668=CARTESIAN_POINT('Ctrl Pts',(-18.5679607592285,-13.8847896936859,
122.160911880391)) ;
#72669=CARTESIAN_POINT('Ctrl Pts',(-18.7362182015604,-13.7048006132671,
122.411095961693)) ;
#72670=CARTESIAN_POINT('Ctrl Pts',(-18.3623992980215,-13.8948490098142,
122.327074678638)) ;
#72671=CARTESIAN_POINT('Ctrl Pts',(-18.5717693261378,-13.7148599293955,
122.544026976484)) ;
#72672=CARTESIAN_POINT('Ctrl Pts',(-18.1920392190739,-13.9047194565674,
122.522692233417)) ;
#72673=CARTESIAN_POINT('Ctrl Pts',(-18.4354824658003,-13.7247303761487,
122.700520842774)) ;
#72674=CARTESIAN_POINT('Ctrl Pts',(-18.0559754686605,-13.9147120948255,
122.747289602254)) ;
#72675=CARTESIAN_POINT('Ctrl Pts',(-18.3266320713964,-13.7347230144067,
122.880198925302)) ;
#72676=CARTESIAN_POINT('Ctrl Pts',(-17.9611352242736,-13.9247441103734,
122.99326074619)) ;
#72677=CARTESIAN_POINT('Ctrl Pts',(-18.2507605487093,-13.7447550299547,
123.076976202334)) ;
#72678=CARTESIAN_POINT('Ctrl Pts',(-17.9107237977274,-13.93460996668,123.247603809018)) ;
#72679=CARTESIAN_POINT('Ctrl Pts',(-18.210432205314,-13.7546208862612,123.280449806178)) ;
#72680=CARTESIAN_POINT('Ctrl Pts',(-17.905103874463,-13.9446792561491,123.512124786774)) ;
#72681=CARTESIAN_POINT('Ctrl Pts',(-18.2059368701527,-13.7646901757304,
123.492066934925)) ;
#72682=CARTESIAN_POINT('Ctrl Pts',(-17.9445700337425,-13.9545228137004,
123.767790797014)) ;
#72683=CARTESIAN_POINT('Ctrl Pts',(-18.2375102230327,-13.7745337332817,
123.696598534101)) ;
#72684=CARTESIAN_POINT('Ctrl Pts',(-18.0281629109246,-13.9645029404882,
124.016370584135)) ;
#72685=CARTESIAN_POINT('Ctrl Pts',(-18.3043848156925,-13.7845138600695,
123.895462003248)) ;
#72686=CARTESIAN_POINT('Ctrl Pts',(-18.1545752562792,-13.9745214890882,
124.247305606064)) ;
#72687=CARTESIAN_POINT('Ctrl Pts',(-18.4055151504625,-13.7945324086694,
124.080209779767)) ;
#72688=CARTESIAN_POINT('Ctrl Pts',(-18.316536321276,-13.9844047896114,124.450385028018)) ;
#72689=CARTESIAN_POINT('Ctrl Pts',(-18.535083750399,-13.8044157091926,124.242672395031)) ;
#72690=CARTESIAN_POINT('Ctrl Pts',(-18.5149631926706,-13.9944730766595,
124.62533735748)) ;
#72691=CARTESIAN_POINT('Ctrl Pts',(-18.6938257640231,-13.8144839962408,
124.382634169633)) ;
#72692=CARTESIAN_POINT('Ctrl Pts',(-18.7353286473333,-14.0043031996781,
124.760223493751)) ;
#72693=CARTESIAN_POINT('Ctrl Pts',(-18.8701172488312,-13.8243141192594,
124.49054215336)) ;
#72694=CARTESIAN_POINT('Ctrl Pts',(-18.9813430292537,-14.0143697836035,
124.857357794723)) ;
#72695=CARTESIAN_POINT('Ctrl Pts',(-19.0669291407156,-13.8343807031847,
124.568249482507)) ;
#72696=CARTESIAN_POINT('Ctrl Pts',(-19.2360505050049,-14.0242598966179,
124.909235187394)) ;
#72697=CARTESIAN_POINT('Ctrl Pts',(-19.2706943553894,-13.8442708161992,
124.60975094901)) ;
#72698=CARTESIAN_POINT('Ctrl Pts',(-19.4985188781197,-14.0342525853805,
124.916724579576)) ;
#72699=CARTESIAN_POINT('Ctrl Pts',(-19.4806688914999,-13.8542635049618,
124.615742311681)) ;
#72700=CARTESIAN_POINT('Ctrl Pts',(-19.7574815058641,-14.0442134737363,
124.878462065185)) ;
#72701=CARTESIAN_POINT('Ctrl Pts',(-19.6878385846522,-13.8642243933176,
124.585132166976)) ;
#72702=CARTESIAN_POINT('Ctrl Pts',(-20.0049101277861,-14.0541314186163,
124.796606975599)) ;
#72703=CARTESIAN_POINT('Ctrl Pts',(-19.8857808233358,-13.8741423381976,
124.519648232361)) ;
#72704=CARTESIAN_POINT('Ctrl Pts',(-20.2366270329028,-14.0641391717125,
124.672163407171)) ;
#72705=CARTESIAN_POINT('Ctrl Pts',(-20.0711543039772,-13.8841500912938,
124.420093397815)) ;
#72706=CARTESIAN_POINT('Ctrl Pts',(-20.4433359396019,-14.0741702656716,
124.508602153835)) ;
#72707=CARTESIAN_POINT('Ctrl Pts',(-20.2365214217928,-13.8941811852529,
124.289244226254)) ;
#72708=CARTESIAN_POINT('Ctrl Pts',(-20.6157637308893,-14.0840182336996,
124.315591986934)) ;
#72709=CARTESIAN_POINT('Ctrl Pts',(-20.3744629095565,-13.9040291532808,
124.134836941808)) ;
#72710=CARTESIAN_POINT('Ctrl Pts',(-20.7551952257983,-14.0940801898254,
124.090948557005)) ;
#72711=CARTESIAN_POINT('Ctrl Pts',(-20.4860083127366,-13.9140911094067,
123.955121992217)) ;
#72712=CARTESIAN_POINT('Ctrl Pts',(-20.8516795937115,-14.1039774014266,
123.849406694899)) ;
#72713=CARTESIAN_POINT('Ctrl Pts',(-20.5631955167448,-13.9239883210078,
123.761889246969)) ;
#72714=CARTESIAN_POINT('Ctrl Pts',(-20.905779742348,-14.1139085680912,123.594099508429)) ;
#72715=CARTESIAN_POINT('Ctrl Pts',(-20.6064757368551,-13.9339194876725,
123.557644109238)) ;
#72716=CARTESIAN_POINT('Ctrl Pts',(-20.9145419979697,-14.1239507522954,
123.330350913862)) ;
#72717=CARTESIAN_POINT('Ctrl Pts',(-20.6134856993466,-13.9439616718766,
123.346645072015)) ;
#72718=CARTESIAN_POINT('Ctrl Pts',(-20.8781348522192,-14.1338374205485,
123.073090399085)) ;
#72719=CARTESIAN_POINT('Ctrl Pts',(-20.5843603024591,-13.9538483401298,
123.140837492851)) ;
#72720=CARTESIAN_POINT('Ctrl Pts',(-20.7971713176932,-14.1438305325268,
122.823288399599)) ;
#72721=CARTESIAN_POINT('Ctrl Pts',(-20.5195898212087,-13.963841452108,122.940995952471)) ;
#72722=CARTESIAN_POINT('Ctrl Pts',(-20.6745548236783,-14.1537762101426,
122.5924733342)) ;
#72723=CARTESIAN_POINT('Ctrl Pts',(-20.4214971012033,-13.9737871297239,
122.756344186729)) ;
#72724=CARTESIAN_POINT('Ctrl Pts',(-20.514110475055,-14.1637235131276,122.386083823483)) ;
#72725=CARTESIAN_POINT('Ctrl Pts',(-20.2931422359031,-13.9837344327088,
122.591232683106)) ;
#72726=CARTESIAN_POINT('Ctrl Pts',(-20.318129265181,-14.1737712368743,122.209146648003)) ;
#72727=CARTESIAN_POINT('Ctrl Pts',(-20.1363573513922,-13.9937821564556,
122.449682552309)) ;
#72728=CARTESIAN_POINT('Ctrl Pts',(-20.0989460634278,-14.1836196106369,
122.071534647431)) ;
#72729=CARTESIAN_POINT('Ctrl Pts',(-19.961011947168,-14.0036305302181,122.339593209163)) ;
#72730=CARTESIAN_POINT('Ctrl Pts',(-19.8568324061837,-14.1935785830826,
121.972166958838)) ;
#72731=CARTESIAN_POINT('Ctrl Pts',(-19.767321602057,-14.0135895026638,122.260098632269)) ;
#72732=CARTESIAN_POINT('Ctrl Pts',(-19.5989991593739,-14.2036174449637,
121.916368996526)) ;
#72733=CARTESIAN_POINT('Ctrl Pts',(-19.5610549871586,-14.023628364545,122.215459749838)) ;
#72734=CARTESIAN_POINT('Ctrl Pts',(-19.3395819370227,-14.2134960491355,
121.905934350628)) ;
#72735=CARTESIAN_POINT('Ctrl Pts',(-19.3535221269257,-14.0335069687168,
122.207111469005)) ;
#72736=CARTESIAN_POINT('Ctrl Pts',(-19.077837641455,-14.2235475903388,121.94118979378)) ;
#72737=CARTESIAN_POINT('Ctrl Pts',(-19.1441263879232,-14.0435585099201,
122.235315233814)) ;
#72738=CARTESIAN_POINT('Ctrl Pts',(-18.8299973984086,-14.2334429883192,
122.020057862205)) ;
#72739=CARTESIAN_POINT('Ctrl Pts',(-18.9458547296678,-14.0534539079004,
122.298408839437)) ;
#72740=CARTESIAN_POINT('Ctrl Pts',(-18.5959941771807,-14.2434942208645,
122.142497342956)) ;
#72741=CARTESIAN_POINT('Ctrl Pts',(-18.7586516520923,-14.0635051404457,
122.396359920337)) ;
#72742=CARTESIAN_POINT('Ctrl Pts',(-18.3901717061781,-14.2533804114888,
122.301075810724)) ;
#72743=CARTESIAN_POINT('Ctrl Pts',(-18.5939939275408,-14.07339133107,122.523221635957)) ;
#72744=CARTESIAN_POINT('Ctrl Pts',(-18.2128046216458,-14.2633729508045,
122.494683384624)) ;
#72745=CARTESIAN_POINT('Ctrl Pts',(-18.4520997745653,-14.0833838703858,
122.678107034334)) ;
#72746=CARTESIAN_POINT('Ctrl Pts',(-18.0724208013344,-14.2733213966993,
122.715249428743)) ;
#72747=CARTESIAN_POINT('Ctrl Pts',(-18.339792292697,-14.0933323162805,122.854559084059)) ;
#72748=CARTESIAN_POINT('Ctrl Pts',(-17.9722554346234,-14.2832581992312,
122.956378922637)) ;
#72749=CARTESIAN_POINT('Ctrl Pts',(-18.2596593906044,-14.1032691188124,
123.047461874324)) ;
#72750=CARTESIAN_POINT('Ctrl Pts',(-17.9148800449504,-14.2932412066825,
123.21240535779)) ;
#72751=CARTESIAN_POINT('Ctrl Pts',(-18.2137581989984,-14.1132521262637,
123.252282614946)) ;
#72752=CARTESIAN_POINT('Ctrl Pts',(-17.9032450353391,-14.3032850480973,
123.47605995493)) ;
#72753=CARTESIAN_POINT('Ctrl Pts',(-18.2044493516429,-14.1232959676785,
123.463206407145)) ;
#72754=CARTESIAN_POINT('Ctrl Pts',(-17.9362327115269,-14.3131132467212,
123.732259863048)) ;
#72755=CARTESIAN_POINT('Ctrl Pts',(-18.2308383754507,-14.1331241663024,
123.668165314127)) ;
#72756=CARTESIAN_POINT('Ctrl Pts',(-18.0150012318199,-14.3231898401634,
123.985018013465)) ;
#72757=CARTESIAN_POINT('Ctrl Pts',(-18.2938523322178,-14.1432007597447,
123.870372464175)) ;
#72758=CARTESIAN_POINT('Ctrl Pts',(-18.133686667507,-14.333041839505,124.215176688649)) ;
#72759=CARTESIAN_POINT('Ctrl Pts',(-18.3887993080397,-14.1530527590862,
124.054499001948)) ;
#72760=CARTESIAN_POINT('Ctrl Pts',(-18.2938233161028,-14.3431154263288,
124.425914521009)) ;
#72761=CARTESIAN_POINT('Ctrl Pts',(-18.5169079559941,-14.1631263459101,
124.223090181388)) ;
#72762=CARTESIAN_POINT('Ctrl Pts',(-18.4837016928437,-14.3529556514263,
124.601492972283)) ;
#72763=CARTESIAN_POINT('Ctrl Pts',(-18.6688091616826,-14.1729665710076,
124.363553020106)) ;
#72764=CARTESIAN_POINT('Ctrl Pts',(-18.7034169617972,-14.362921355455,124.743969337095)) ;
#72765=CARTESIAN_POINT('Ctrl Pts',(-18.844580419153,-14.1829322750362,124.47753501832)) ;
#72766=CARTESIAN_POINT('Ctrl Pts',(-18.9461903268553,-14.3729479887616,
124.846418837686)) ;
#72767=CARTESIAN_POINT('Ctrl Pts',(-19.0387986926441,-14.1929589083428,
124.559495739056)) ;
#72768=CARTESIAN_POINT('Ctrl Pts',(-19.2001264119719,-14.3828622844734,
124.9046678972)) ;
#72769=CARTESIAN_POINT('Ctrl Pts',(-19.2419467128813,-14.2028732040546,
124.60609605546)) ;
#72770=CARTESIAN_POINT('Ctrl Pts',(-19.4622585244001,-14.3928505731658,
124.918515058878)) ;
#72771=CARTESIAN_POINT('Ctrl Pts',(-19.4516521770258,-14.2128614927471,
124.617175109609)) ;
#72772=CARTESIAN_POINT('Ctrl Pts',(-19.7240472766197,-14.4028893063242,
124.886002641522)) ;
#72773=CARTESIAN_POINT('Ctrl Pts',(-19.6610834379714,-14.2229002259054,
124.591166382665)) ;
#72774=CARTESIAN_POINT('Ctrl Pts',(-19.971442278505,-14.4127326381517,124.81045280007)) ;
#72775=CARTESIAN_POINT('Ctrl Pts',(-19.8589988887457,-14.232743557733,124.530728061937)) ;
#72776=CARTESIAN_POINT('Ctrl Pts',(-20.2065561511299,-14.4227603640313,
124.691438006589)) ;
#72777=CARTESIAN_POINT('Ctrl Pts',(-20.0470906952005,-14.2427712836126,
124.435517495806)) ;
#72778=CARTESIAN_POINT('Ctrl Pts',(-20.4171057819687,-14.4327927004199,
124.532757562432)) ;
#72779=CARTESIAN_POINT('Ctrl Pts',(-20.2155312378511,-14.2528036200011,
124.308574138805)) ;
#72780=CARTESIAN_POINT('Ctrl Pts',(-20.5936350311629,-14.4426222007205,
124.344201635608)) ;
#72781=CARTESIAN_POINT('Ctrl Pts',(-20.3567549741227,-14.2626331203018,
124.15773110315)) ;
#72782=CARTESIAN_POINT('Ctrl Pts',(-20.7377126083649,-14.4526117046373,
124.124750610615)) ;
#72783=CARTESIAN_POINT('Ctrl Pts',(-20.4720182693449,-14.2726226242185,
123.982171262254)) ;
#72784=CARTESIAN_POINT('Ctrl Pts',(-20.8414417059571,-14.4626555451497,
123.882049023588)) ;
#72785=CARTESIAN_POINT('Ctrl Pts',(-20.5550029138087,-14.2826664647309,
123.788010448594)) ;
#72786=CARTESIAN_POINT('Ctrl Pts',(-20.9006480360546,-14.4724772509177,
123.630827043124)) ;
#72787=CARTESIAN_POINT('Ctrl Pts',(-20.602369249548,-14.292488170499,123.587034187836)) ;
#72788=CARTESIAN_POINT('Ctrl Pts',(-20.9162986355371,-14.4825122980501,
123.367582647656)) ;
#72789=CARTESIAN_POINT('Ctrl Pts',(-20.6148913940102,-14.3025232176314,
123.376438685901)) ;
#72790=CARTESIAN_POINT('Ctrl Pts',(-20.8853105896396,-14.492536975487,123.105964149148)) ;
#72791=CARTESIAN_POINT('Ctrl Pts',(-20.5901024698145,-14.3125478950683,
123.167143688753)) ;
#72792=CARTESIAN_POINT('Ctrl Pts',(-20.8111959912493,-14.5023897903414,
122.857876731646)) ;
#72793=CARTESIAN_POINT('Ctrl Pts',(-20.5308125817991,-14.3224007099227,
122.96867405913)) ;
#72794=CARTESIAN_POINT('Ctrl Pts',(-20.6939628549343,-14.512377499949,122.623068574737)) ;
#72795=CARTESIAN_POINT('Ctrl Pts',(-20.4370276691554,-14.3323884195303,
122.780826900379)) ;
#72796=CARTESIAN_POINT('Ctrl Pts',(-20.5386353139863,-14.5223075099431,
122.413370344801)) ;
#72797=CARTESIAN_POINT('Ctrl Pts',(-20.3127672606121,-14.3423184295243,
122.613067632083)) ;
#72798=CARTESIAN_POINT('Ctrl Pts',(-20.3483991860462,-14.5322972651622,
122.232456679558)) ;
#72799=CARTESIAN_POINT('Ctrl Pts',(-20.1605796814699,-14.3523081847435,
122.468335499922)) ;
#72800=CARTESIAN_POINT('Ctrl Pts',(-20.1286457022136,-14.5423238738451,
122.087070807821)) ;
#72801=CARTESIAN_POINT('Ctrl Pts',(-19.9847778210034,-14.3623347934264,
122.352025351931)) ;
#72802=CARTESIAN_POINT('Ctrl Pts',(-19.8905327192544,-14.552207813867,121.983318872827)) ;
#72803=CARTESIAN_POINT('Ctrl Pts',(-19.7942886798817,-14.3722187334482,
122.269022420981)) ;
#72804=CARTESIAN_POINT('Ctrl Pts',(-19.635462587823,-14.5621970414055,121.921242080252)) ;
#72805=CARTESIAN_POINT('Ctrl Pts',(-19.5902331362649,-14.3822079609867,
122.219359208042)) ;
#72806=CARTESIAN_POINT('Ctrl Pts',(-19.3720577988272,-14.5722399119292,
121.904853032936)) ;
#72807=CARTESIAN_POINT('Ctrl Pts',(-19.3795093430328,-14.3922508315104,
122.206246194466)) ;
#72808=CARTESIAN_POINT('Ctrl Pts',(-19.1152596800148,-14.5820722986846,
121.933419317755)) ;
#72809=CARTESIAN_POINT('Ctrl Pts',(-19.1740714024378,-14.4020832182658,
122.229097307701)) ;
#72810=CARTESIAN_POINT('Ctrl Pts',(-18.8630536664774,-14.5920655918562,
122.006599511794)) ;
#72811=CARTESIAN_POINT('Ctrl Pts',(-18.9723061434464,-14.4120765114374,
122.287639558264)) ;
#72812=CARTESIAN_POINT('Ctrl Pts',(-18.626700387474,-14.6020975975046,122.123410637896)) ;
#72813=CARTESIAN_POINT('Ctrl Pts',(-18.7832226648472,-14.4221085170859,
122.38108679379)) ;
#72814=CARTESIAN_POINT('Ctrl Pts',(-18.4175822404047,-14.6119628534736,
122.276618419856)) ;
#72815=CARTESIAN_POINT('Ctrl Pts',(-18.61592748227,-14.4319737730548,122.503651126042)) ;
#72816=CARTESIAN_POINT('Ctrl Pts',(-18.2359363519332,-14.6219247333811,
122.46514351394)) ;
#72817=CARTESIAN_POINT('Ctrl Pts',(-18.4706094571108,-14.4419356529623,
122.654469655171)) ;
#72818=CARTESIAN_POINT('Ctrl Pts',(-18.0890820795263,-14.631959666743,122.684159241036)) ;
#72819=CARTESIAN_POINT('Ctrl Pts',(-18.3531243943116,-14.4519705863242,
122.829681166478)) ;
#72820=CARTESIAN_POINT('Ctrl Pts',(-17.9836588830018,-14.6418446251222,
122.921611991618)) ;
#72821=CARTESIAN_POINT('Ctrl Pts',(-18.2687841767101,-14.4618555447035,
123.019642136378)) ;
#72822=CARTESIAN_POINT('Ctrl Pts',(-17.9199993003975,-14.6519102520449,
123.178306439061)) ;
#72823=CARTESIAN_POINT('Ctrl Pts',(-18.217854528994,-14.4719211716262,123.224997325049)) ;
#72824=CARTESIAN_POINT('Ctrl Pts',(-17.902016923723,-14.6617493577093,123.436284553321)) ;
#72825=CARTESIAN_POINT('Ctrl Pts',(-18.2034666313559,-14.4817602772905,
123.431379111336)) ;
#72826=CARTESIAN_POINT('Ctrl Pts',(-17.9293579839906,-14.6718121727146,
123.699271479255)) ;
#72827=CARTESIAN_POINT('Ctrl Pts',(-18.2253374197392,-14.4918230922959,
123.641768973016)) ;
#72828=CARTESIAN_POINT('Ctrl Pts',(-18.0009916818358,-14.6817083787633,
123.949301618016)) ;
#72829=CARTESIAN_POINT('Ctrl Pts',(-18.2826422983745,-14.5017192983446,
123.841793287146)) ;
#72830=CARTESIAN_POINT('Ctrl Pts',(-18.1147854787737,-14.6916492017886,
124.184415931293)) ;
#72831=CARTESIAN_POINT('Ctrl Pts',(-18.3736753208548,-14.5116601213698,
124.029885468125)) ;
#72832=CARTESIAN_POINT('Ctrl Pts',(-18.268637847317,-14.7016537847672,124.397645063543)) ;
#72833=CARTESIAN_POINT('Ctrl Pts',(-18.4967554534644,-14.5216647043485,
124.200469975829)) ;
#72834=CARTESIAN_POINT('Ctrl Pts',(-18.4576820791723,-14.711674679212,124.580965224255)) ;
#72835=CARTESIAN_POINT('Ctrl Pts',(-18.6479893550732,-14.5316855987932,
124.347127597631)) ;
#72836=CARTESIAN_POINT('Ctrl Pts',(-18.6727084409686,-14.7215665998014,
124.727050531071)) ;
#72837=CARTESIAN_POINT('Ctrl Pts',(-18.8200089755962,-14.5415775193826,
124.463997424165)) ;
#72838=CARTESIAN_POINT('Ctrl Pts',(-18.9120984381153,-14.7315600321468,
124.835009694334)) ;
#72839=CARTESIAN_POINT('Ctrl Pts',(-19.0115200042416,-14.551570951728,124.55036669427)) ;
#72840=CARTESIAN_POINT('Ctrl Pts',(-19.1654082296923,-14.7415056370466,
124.899373825314)) ;
#72841=CARTESIAN_POINT('Ctrl Pts',(-19.2141671271123,-14.5615165566279,
124.601860046211)) ;
#72842=CARTESIAN_POINT('Ctrl Pts',(-19.4260649276636,-14.7514529105282,
124.919311654111)) ;
#72843=CARTESIAN_POINT('Ctrl Pts',(-19.4226921583559,-14.5714638301094,
124.617812487927)) ;
#72844=CARTESIAN_POINT('Ctrl Pts',(-19.688803998052,-14.7615008250045,124.893135998559)) ;
#72845=CARTESIAN_POINT('Ctrl Pts',(-19.6328836382695,-14.5815117445858,
124.596874129132)) ;
#72846=CARTESIAN_POINT('Ctrl Pts',(-19.9380105597633,-14.7713484653519,
124.823369065501)) ;
#72847=CARTESIAN_POINT('Ctrl Pts',(-19.8322491726103,-14.5913593849331,
124.541062779856)) ;
#72848=CARTESIAN_POINT('Ctrl Pts',(-20.1743610166354,-14.7813101807285,
124.710840541203)) ;
#72849=CARTESIAN_POINT('Ctrl Pts',(-20.0213304109851,-14.6013211003097,
124.451042024514)) ;
#72850=CARTESIAN_POINT('Ctrl Pts',(-20.3888445239837,-14.7913388043013,
124.557674697963)) ;
#72851=CARTESIAN_POINT('Ctrl Pts',(-20.1929184772654,-14.6113497238825,
124.32851117537)) ;
#72852=CARTESIAN_POINT('Ctrl Pts',(-20.5713377847483,-14.8012491663677,
124.37189085968)) ;
#72853=CARTESIAN_POINT('Ctrl Pts',(-20.3389145561169,-14.6212600859489,
124.179885784323)) ;
#72854=CARTESIAN_POINT('Ctrl Pts',(-20.7197431782127,-14.8111838600201,
124.157087470511)) ;
#72855=CARTESIAN_POINT('Ctrl Pts',(-20.457640661641,-14.6311947796013,124.008044437838)) ;
#72856=CARTESIAN_POINT('Ctrl Pts',(-20.8295234845985,-14.821225703148,123.917131743873)) ;
#72857=CARTESIAN_POINT('Ctrl Pts',(-20.5454669287708,-14.6412366227292,
123.816080822821)) ;
#72858=CARTESIAN_POINT('Ctrl Pts',(-20.895164226046,-14.8311102087184,123.665780824493)) ;
#72859=CARTESIAN_POINT('Ctrl Pts',(-20.5979816634709,-14.6511211282996,
123.615000778527)) ;
#72860=CARTESIAN_POINT('Ctrl Pts',(-20.9167156315003,-14.8411123125036,
123.403859517349)) ;
#72861=CARTESIAN_POINT('Ctrl Pts',(-20.6152250273271,-14.6611232320848,
123.405463971272)) ;
#72862=CARTESIAN_POINT('Ctrl Pts',(-20.892871759179,-14.8510306639186,123.144264974581)) ;
#72863=CARTESIAN_POINT('Ctrl Pts',(-20.5961521920614,-14.6710415834998,
123.197788211826)) ;
#72864=CARTESIAN_POINT('Ctrl Pts',(-20.8233784417563,-14.8610783199395,
122.889574983723)) ;
#72865=CARTESIAN_POINT('Ctrl Pts',(-20.5405596778779,-14.6810892395207,
122.994035641784)) ;
#72866=CARTESIAN_POINT('Ctrl Pts',(-20.7129195792961,-14.8709495129677,
122.654803032933)) ;
#72867=CARTESIAN_POINT('Ctrl Pts',(-20.4521948362717,-14.6909604325489,
122.806217311393)) ;
#72868=CARTESIAN_POINT('Ctrl Pts',(-20.5605298604952,-14.8810152261112,
122.438669790552)) ;
#72869=CARTESIAN_POINT('Ctrl Pts',(-20.330284230218,-14.7010261456924,122.633308925959)) ;
#72870=CARTESIAN_POINT('Ctrl Pts',(-20.3770184511799,-14.8908676866838,
122.255919658945)) ;
#72871=CARTESIAN_POINT('Ctrl Pts',(-20.1834793625096,-14.7108786062651,
122.487109277975)) ;
#72872=CARTESIAN_POINT('Ctrl Pts',(-20.0875427687652,-14.9042961494064,
122.05428711409)) ;
#72873=CARTESIAN_POINT('Ctrl Pts',(-19.9518873140162,-14.7243070689876,
122.325790630287)) ;
#72874=CARTESIAN_POINT('Ctrl Pts',(-19.7606733441764,-14.9173770969235,
121.935403530438)) ;
#72875=CARTESIAN_POINT('Ctrl Pts',(-19.6903664132712,-14.7373880165047,
122.230682365548)) ;
#72876=CARTESIAN_POINT('Ctrl Pts',(-19.4080294143568,-14.930851595158,121.904239537991)) ;
#72877=CARTESIAN_POINT('Ctrl Pts',(-19.408296278235,-14.7508625147393,122.205756669958)) ;
#72878=CARTESIAN_POINT('Ctrl Pts',(-19.1506048229963,-14.9406836987675,
121.926886772549)) ;
#72879=CARTESIAN_POINT('Ctrl Pts',(-19.2023472618255,-14.7606946183488,
122.223870633588)) ;
#72880=CARTESIAN_POINT('Ctrl Pts',(-18.8974267386833,-14.9506496018942,
121.993755117911)) ;
#72881=CARTESIAN_POINT('Ctrl Pts',(-18.9998068131851,-14.7706605214754,
122.277363288063)) ;
#72882=CARTESIAN_POINT('Ctrl Pts',(-18.658349854463,-14.9606770112044,122.104643278286)) ;
#72883=CARTESIAN_POINT('Ctrl Pts',(-18.8085430338256,-14.7806879307857,
122.366073028994)) ;
#72884=CARTESIAN_POINT('Ctrl Pts',(-18.4446798400925,-14.970588042571,122.253516252919)) ;
#72885=CARTESIAN_POINT('Ctrl Pts',(-18.6376088003778,-14.7905989621522,
122.485164544284)) ;
#72886=CARTESIAN_POINT('Ctrl Pts',(-18.1971580267573,-14.983832350192,122.498300087687)) ;
#72887=CARTESIAN_POINT('Ctrl Pts',(-18.4395744217537,-14.8038432697733,
122.681015310389)) ;
#72888=CARTESIAN_POINT('Ctrl Pts',(-17.9735883959182,-15.0005328328632,
122.881645823223)) ;
#72889=CARTESIAN_POINT('Ctrl Pts',(-18.2607334713096,-14.8205437524445,
122.987646040595)) ;
#72890=CARTESIAN_POINT('Ctrl Pts',(-17.8949212634125,-15.017039662019,123.313331293307)) ;
#72891=CARTESIAN_POINT('Ctrl Pts',(-18.197786980337,-14.8370505816002,123.333061833224)) ;
#72892=CARTESIAN_POINT('Ctrl Pts',(-17.9226408362243,-15.0303502902566,
123.66198197427)) ;
#72893=CARTESIAN_POINT('Ctrl Pts',(-18.2199642568686,-14.8503612098378,
123.611928568434)) ;
#72894=CARTESIAN_POINT('Ctrl Pts',(-17.9885443791132,-15.0403428537967,
123.916213406508)) ;
#72895=CARTESIAN_POINT('Ctrl Pts',(-18.2726848749169,-14.8603537733779,
123.815325758311)) ;
#72896=CARTESIAN_POINT('Ctrl Pts',(-18.0982567044604,-15.0503729367982,
124.155839488602)) ;
#72897=CARTESIAN_POINT('Ctrl Pts',(-18.3604503472436,-14.8703838563795,
124.007021726878)) ;
#72898=CARTESIAN_POINT('Ctrl Pts',(-18.2942816287218,-15.063546540796,124.44126177794)) ;
#72899=CARTESIAN_POINT('Ctrl Pts',(-18.5172815099474,-14.8835574603772,
124.235376257215)) ;
#72900=CARTESIAN_POINT('Ctrl Pts',(-18.6299004804295,-15.0801842460274,
124.728937538232)) ;
#72901=CARTESIAN_POINT('Ctrl Pts',(-18.785763290496,-14.9001951656086,124.465502997211)) ;
#72902=CARTESIAN_POINT('Ctrl Pts',(-19.1244402676939,-15.1000660085948,
124.915683237947)) ;
#72903=CARTESIAN_POINT('Ctrl Pts',(-19.1813811513845,-14.9200769281761,
124.614910725455)) ;
#72904=CARTESIAN_POINT('Ctrl Pts',(-19.5680268436955,-15.1167623608113,
124.921075710922)) ;
#72905=CARTESIAN_POINT('Ctrl Pts',(-19.5363048231766,-14.9367732803926,
124.619219761806)) ;
#72906=CARTESIAN_POINT('Ctrl Pts',(-19.9032277012464,-15.1299193886004,
124.836006277043)) ;
#72907=CARTESIAN_POINT('Ctrl Pts',(-19.804416663056,-14.9499303081817,124.551173733196)) ;
#72908=CARTESIAN_POINT('Ctrl Pts',(-20.2240299228252,-15.1432967432439,
124.69232618413)) ;
#72909=CARTESIAN_POINT('Ctrl Pts',(-20.0610789329257,-14.9633076628252,
124.436222806107)) ;
#72910=CARTESIAN_POINT('Ctrl Pts',(-20.5648835408939,-15.1598275775027,
124.415004995523)) ;
#72911=CARTESIAN_POINT('Ctrl Pts',(-20.33374952369,-14.979838497084,124.214377150155)) ;
#72912=CARTESIAN_POINT('Ctrl Pts',(-20.8382356611217,-15.1797922672458,
123.96026126481)) ;
#72913=CARTESIAN_POINT('Ctrl Pts',(-20.5524388724161,-14.9998031868271,
123.850580630537)) ;
#72914=CARTESIAN_POINT('Ctrl Pts',(-20.9392779040773,-15.1997087606695,
123.440635012869)) ;
#72915=CARTESIAN_POINT('Ctrl Pts',(-20.6332747129782,-15.0197196802507,
123.434880576487)) ;
#72916=CARTESIAN_POINT('Ctrl Pts',(-20.8580805310066,-15.219598480019,122.918218801413)) ;
#72917=CARTESIAN_POINT('Ctrl Pts',(-20.5683198928512,-15.0396093996003,
123.016946176903)) ;
#72918=CARTESIAN_POINT('Ctrl Pts',(-20.6016712396936,-15.2396052096669,
122.452465436921)) ;
#72919=CARTESIAN_POINT('Ctrl Pts',(-20.363194945236,-15.0596161292481,122.644342199294)) ;
#72920=CARTESIAN_POINT('Ctrl Pts',(-20.2052118910456,-15.2594432633138,
122.104699832053)) ;
#72921=CARTESIAN_POINT('Ctrl Pts',(-20.0460282780659,-15.079454182895,122.366126875178)) ;
#72922=CARTESIAN_POINT('Ctrl Pts',(-19.7104197648693,-15.2794366015274,
121.91117270604)) ;
#72923=CARTESIAN_POINT('Ctrl Pts',(-19.6501953671741,-15.0994475211086,
122.211302958785)) ;
#72924=CARTESIAN_POINT('Ctrl Pts',(-19.1820210308672,-15.299319400934,121.898505004047)) ;
#72925=CARTESIAN_POINT('Ctrl Pts',(-19.2274754164287,-15.1193303205152,
122.201166461084)) ;
#72926=CARTESIAN_POINT('Ctrl Pts',(-18.6807320925473,-15.3192115818527,
122.066058969387)) ;
#72927=CARTESIAN_POINT('Ctrl Pts',(-18.8264426177306,-15.1392225014339,
122.335208221256)) ;
#72928=CARTESIAN_POINT('Ctrl Pts',(-18.2657076845976,-15.3391137603478,
122.394277865581)) ;
#72929=CARTESIAN_POINT('Ctrl Pts',(-18.494421510302,-15.159124679929,122.597782896425)) ;
#72930=CARTESIAN_POINT('Ctrl Pts',(-17.9866547280491,-15.3591510715515,
122.847707709336)) ;
#72931=CARTESIAN_POINT('Ctrl Pts',(-18.2711780423566,-15.1791619911328,
122.960525608524)) ;
#72932=CARTESIAN_POINT('Ctrl Pts',(-17.8794922156579,-15.3789635130924,
123.363506708321)) ;
#72933=CARTESIAN_POINT('Ctrl Pts',(-18.1854465971545,-15.1989744326736,
123.373166586324)) ;
#72934=CARTESIAN_POINT('Ctrl Pts',(-17.9558345969628,-15.3990287538273,
123.891058298173)) ;
#72935=CARTESIAN_POINT('Ctrl Pts',(-18.2465194339574,-15.2190396734085,
123.795207317988)) ;
#72936=CARTESIAN_POINT('Ctrl Pts',(-18.2036257716966,-15.4187859586831,
124.354317293428)) ;
#72937=CARTESIAN_POINT('Ctrl Pts',(-18.444753257949,-15.2387968782644,124.165817334642)) ;
#72938=CARTESIAN_POINT('Ctrl Pts',(-18.5991767272992,-15.4388192313288,
124.71034908512)) ;
#72939=CARTESIAN_POINT('Ctrl Pts',(-18.7611938046602,-15.2588301509101,
124.450642577608)) ;
#72940=CARTESIAN_POINT('Ctrl Pts',(-19.0875441523819,-15.4586321397826,
124.907957059545)) ;
#72941=CARTESIAN_POINT('Ctrl Pts',(-19.1518899723408,-15.2786430593639,
124.608729644721)) ;
#72942=CARTESIAN_POINT('Ctrl Pts',(-19.6183970906438,-15.4786282859101,
124.927914166539)) ;
#72943=CARTESIAN_POINT('Ctrl Pts',(-19.576572466702,-15.2986392054913,124.62469458261)) ;
#72944=CARTESIAN_POINT('Ctrl Pts',(-20.1213238856108,-15.4984900391326,
124.766723103291)) ;
#72945=CARTESIAN_POINT('Ctrl Pts',(-19.9789150179613,-15.3185009587138,
124.495740310664)) ;
#72946=CARTESIAN_POINT('Ctrl Pts',(-20.5429196526886,-15.5185585562607,
124.440174246475)) ;
#72947=CARTESIAN_POINT('Ctrl Pts',(-20.3161903555175,-15.3385694758419,
124.234500854143)) ;
#72948=CARTESIAN_POINT('Ctrl Pts',(-20.8242320696913,-15.5383894292575,
123.994315885948)) ;
#72949=CARTESIAN_POINT('Ctrl Pts',(-20.5412403549953,-15.3584003488387,
123.877812029321)) ;
#72950=CARTESIAN_POINT('Ctrl Pts',(-20.9383743236611,-15.5583113400742,
123.477399544048)) ;
#72951=CARTESIAN_POINT('Ctrl Pts',(-20.6325525210197,-15.3783222596554,
123.464277746288)) ;
#72952=CARTESIAN_POINT('Ctrl Pts',(-20.8690610708311,-15.5782407835095,
122.952175131988)) ;
#72953=CARTESIAN_POINT('Ctrl Pts',(-20.5770999180587,-15.3982517030907,
123.044097841455)) ;
#72954=CARTESIAN_POINT('Ctrl Pts',(-20.6251692263839,-15.5981504536259,
122.482655310881)) ;
#72955=CARTESIAN_POINT('Ctrl Pts',(-20.3819841289406,-15.4181613732071,
122.668482232618)) ;
#72956=CARTESIAN_POINT('Ctrl Pts',(-20.236940502455,-15.6180238108887,122.124408327006)) ;
#72957=CARTESIAN_POINT('Ctrl Pts',(-20.0713986144983,-15.43803473047,122.381885868014)) ;
#72958=CARTESIAN_POINT('Ctrl Pts',(-19.7469529682566,-15.6380153455067,
121.919076471778)) ;
#72959=CARTESIAN_POINT('Ctrl Pts',(-19.6794074858345,-15.4580262650879,
122.217622870441)) ;
#72960=CARTESIAN_POINT('Ctrl Pts',(-19.2195107524765,-15.6578809629174,
121.893213319222)) ;
#72961=CARTESIAN_POINT('Ctrl Pts',(-19.257452611772,-15.4778918824987,122.196935186946)) ;
#72962=CARTESIAN_POINT('Ctrl Pts',(-18.7119132759881,-15.6778618927456,
122.049260143558)) ;
#72963=CARTESIAN_POINT('Ctrl Pts',(-18.8513754816871,-15.4978728123269,
122.321775691797)) ;
#72964=CARTESIAN_POINT('Ctrl Pts',(-18.2892684219138,-15.6978003548287,
122.368964780191)) ;
#72965=CARTESIAN_POINT('Ctrl Pts',(-18.513261161945,-15.51781127441,122.577542114275)) ;
#72966=CARTESIAN_POINT('Ctrl Pts',(-18.0010412602358,-15.7176925480505,
122.812265657364)) ;
#72967=CARTESIAN_POINT('Ctrl Pts',(-18.2826819358055,-15.5377034676318,
122.932185207393)) ;
#72968=CARTESIAN_POINT('Ctrl Pts',(-17.8812058282244,-15.7376632630859,
123.329230583629)) ;
#72969=CARTESIAN_POINT('Ctrl Pts',(-18.1868169736697,-15.5576741826671,
123.345758094485)) ;
#72970=CARTESIAN_POINT('Ctrl Pts',(-17.9435942351176,-15.757472934752,123.852155946801)) ;
#72971=CARTESIAN_POINT('Ctrl Pts',(-18.236731360586,-15.5774838543332,123.764098868335)) ;
#72972=CARTESIAN_POINT('Ctrl Pts',(-18.182383268691,-15.7774661514431,124.326648974565)) ;
#72973=CARTESIAN_POINT('Ctrl Pts',(-18.4277666392234,-15.5974770710244,
124.143691534973)) ;
#72974=CARTESIAN_POINT('Ctrl Pts',(-18.566008687816,-15.7973170636395,124.689180060731)) ;
#72975=CARTESIAN_POINT('Ctrl Pts',(-18.7346680390251,-15.6173279832208,
124.433713872996)) ;
#72976=CARTESIAN_POINT('Ctrl Pts',(-19.0555605459816,-15.8173916699585,
124.900980308336)) ;
#72977=CARTESIAN_POINT('Ctrl Pts',(-19.126318602416,-15.6374025895398,124.603150145415)) ;
#72978=CARTESIAN_POINT('Ctrl Pts',(-19.4939341246382,-15.8339083018419,
124.927054797018)) ;
#72979=CARTESIAN_POINT('Ctrl Pts',(-19.4769939508857,-15.6539192214231,
124.62400662122)) ;
#72980=CARTESIAN_POINT('Ctrl Pts',(-19.8373421472815,-15.847247009536,124.85716735999)) ;
#72981=CARTESIAN_POINT('Ctrl Pts',(-19.7517415685983,-15.6672579291172,
124.568093350014)) ;
#72982=CARTESIAN_POINT('Ctrl Pts',(-20.0781804979538,-15.8570893838442,
124.762739875936)) ;
#72983=CARTESIAN_POINT('Ctrl Pts',(-19.9444057990373,-15.6771003034255,
124.492551480651)) ;
#72984=CARTESIAN_POINT('Ctrl Pts',(-20.3037960538785,-15.867144403827,124.625272793308)) ;
#72985=CARTESIAN_POINT('Ctrl Pts',(-20.1249049700663,-15.6871553234083,
124.38256759213)) ;
#72986=CARTESIAN_POINT('Ctrl Pts',(-20.5648469001971,-15.8803765604846,
124.395495442163)) ;
#72987=CARTESIAN_POINT('Ctrl Pts',(-20.333709310747,-15.7003874800658,124.198785755722)) ;
#72988=CARTESIAN_POINT('Ctrl Pts',(-20.8101326080118,-15.8969915278297,
124.028323713328)) ;
#72989=CARTESIAN_POINT('Ctrl Pts',(-20.5299755608498,-15.717002447411,123.904990049025)) ;
#72990=CARTESIAN_POINT('Ctrl Pts',(-20.9150857052234,-15.9135861148409,
123.59995181053)) ;
#72991=CARTESIAN_POINT('Ctrl Pts',(-20.6139164049773,-15.7335970344222,
123.562338490809)) ;
#72992=CARTESIAN_POINT('Ctrl Pts',(-20.9083137994438,-15.9268196831963,
123.252228775186)) ;
#72993=CARTESIAN_POINT('Ctrl Pts',(-20.6085033810929,-15.7468306027775,
123.28412879026)) ;
#72994=CARTESIAN_POINT('Ctrl Pts',(-20.8574915954294,-15.9368633010049,
122.993254896147)) ;
#72995=CARTESIAN_POINT('Ctrl Pts',(-20.5678420886449,-15.7568742205862,
123.076956586024)) ;
#72996=CARTESIAN_POINT('Ctrl Pts',(-20.7640240611452,-15.9467502252398,
122.75080795887)) ;
#72997=CARTESIAN_POINT('Ctrl Pts',(-20.4930658151328,-15.766761144821,122.88299771998)) ;
#72998=CARTESIAN_POINT('Ctrl Pts',(-20.6288932482248,-15.9567408796866,
122.525730668333)) ;
#72999=CARTESIAN_POINT('Ctrl Pts',(-20.3849611673798,-15.7767517992678,
122.702938858516)) ;
#73000=CARTESIAN_POINT('Ctrl Pts',(-20.4571800170239,-15.9667026381405,
122.328129169737)) ;
#73001=CARTESIAN_POINT('Ctrl Pts',(-20.2475814010665,-15.7867135577218,
122.544854090362)) ;
#73002=CARTESIAN_POINT('Ctrl Pts',(-20.184971644941,-15.9800425032078,122.107130949317)) ;
#73003=CARTESIAN_POINT('Ctrl Pts',(-20.0298503330428,-15.800053422789,122.368082503893)) ;
#73004=CARTESIAN_POINT('Ctrl Pts',(-19.8618390549688,-15.9933512861211,
121.963354375923)) ;
#73005=CARTESIAN_POINT('Ctrl Pts',(-19.7713258119905,-15.8133622057023,
122.25304504801)) ;
#73006=CARTESIAN_POINT('Ctrl Pts',(-19.5194352460045,-16.0065470435651,
121.908483591858)) ;
#73007=CARTESIAN_POINT('Ctrl Pts',(-19.4973853555819,-15.8265579631464,
122.209149363533)) ;
#73008=CARTESIAN_POINT('Ctrl Pts',(-19.2576646411424,-16.0165089272416,
121.911843868046)) ;
#73009=CARTESIAN_POINT('Ctrl Pts',(-19.2879723775728,-15.8365198468229,
122.211840251455)) ;
#73010=CARTESIAN_POINT('Ctrl Pts',(-18.998445535369,-16.0265520367563,121.96142659732)) ;
#73011=CARTESIAN_POINT('Ctrl Pts',(-19.0805966476983,-15.8465629563375,
122.251508536236)) ;
#73012=CARTESIAN_POINT('Ctrl Pts',(-18.7563398526898,-16.0364042867555,
122.053197919768)) ;
#73013=CARTESIAN_POINT('Ctrl Pts',(-18.8869132360213,-15.8564152063368,
122.324927701526)) ;
#73014=CARTESIAN_POINT('Ctrl Pts',(-18.5308557512997,-16.046375823706,122.186642824453)) ;
#73015=CARTESIAN_POINT('Ctrl Pts',(-18.7065271150843,-15.8663867432872,
122.431685506008)) ;
#73016=CARTESIAN_POINT('Ctrl Pts',(-18.3314551896141,-16.0563710891835,
122.357680218338)) ;
#73017=CARTESIAN_POINT('Ctrl Pts',(-18.5470081927436,-15.8763820087648,
122.568517085258)) ;
#73018=CARTESIAN_POINT('Ctrl Pts',(-18.1644264951237,-16.0664050620571,
122.561684900295)) ;
#73019=CARTESIAN_POINT('Ctrl Pts',(-18.4133869982469,-15.8864159816384,
122.731722236848)) ;
#73020=CARTESIAN_POINT('Ctrl Pts',(-18.0372716142788,-16.0762604768195,
122.787340539606)) ;
#73021=CARTESIAN_POINT('Ctrl Pts',(-18.3116651407134,-15.8962713964007,
122.912247684701)) ;
#73022=CARTESIAN_POINT('Ctrl Pts',(-17.9496588451068,-16.0862597543283,
123.035027131231)) ;
#73023=CARTESIAN_POINT('Ctrl Pts',(-18.2415770550694,-15.9062706739096,
123.110397634539)) ;
#73024=CARTESIAN_POINT('Ctrl Pts',(-17.9065430994012,-16.0961549384913,
123.291508010333)) ;
#73025=CARTESIAN_POINT('Ctrl Pts',(-18.2070866753849,-15.9161658580725,
123.315582497717)) ;
#73026=CARTESIAN_POINT('Ctrl Pts',(-17.9086795502078,-16.1062153181321,
123.555839709395)) ;
#73027=CARTESIAN_POINT('Ctrl Pts',(-18.2087980556812,-15.9262262377133,
123.527047864045)) ;
#73028=CARTESIAN_POINT('Ctrl Pts',(-17.9555303865302,-16.1160651871402,
123.810434776877)) ;
#73029=CARTESIAN_POINT('Ctrl Pts',(-18.246280837973,-15.9360761067214,123.730723208321)) ;
#73030=CARTESIAN_POINT('Ctrl Pts',(-18.0469625662497,-16.1260967483481,
124.057672087737)) ;
#73031=CARTESIAN_POINT('Ctrl Pts',(-18.3194286080762,-15.9461076679293,
123.928512283029)) ;
#73032=CARTESIAN_POINT('Ctrl Pts',(-18.180132940785,-16.1361071972304,124.284566442488)) ;
#73033=CARTESIAN_POINT('Ctrl Pts',(-18.4259667878995,-15.9561181168116,
124.110026615654)) ;
#73034=CARTESIAN_POINT('Ctrl Pts',(-18.3486698657814,-16.1460139366474,
124.482977937595)) ;
#73035=CARTESIAN_POINT('Ctrl Pts',(-18.560797834217,-15.9660248562286,124.26875420935)) ;
#73036=CARTESIAN_POINT('Ctrl Pts',(-18.549400664436,-16.1559519527158,124.650023534737)) ;
#73037=CARTESIAN_POINT('Ctrl Pts',(-18.7213836797502,-15.9759628722971,
124.402388898548)) ;
#73038=CARTESIAN_POINT('Ctrl Pts',(-18.7775718600951,-16.1659571991669,
124.780727182759)) ;
#73039=CARTESIAN_POINT('Ctrl Pts',(-18.9039216373305,-15.9859681187482,
124.506949936595)) ;
#73040=CARTESIAN_POINT('Ctrl Pts',(-19.0257972538553,-16.1759912602232,
124.869646857072)) ;
#73041=CARTESIAN_POINT('Ctrl Pts',(-19.1025026967416,-15.9960021798045,
124.578083637669)) ;
#73042=CARTESIAN_POINT('Ctrl Pts',(-19.2807496064562,-16.1858363412814,
124.913723831304)) ;
#73043=CARTESIAN_POINT('Ctrl Pts',(-19.3064644940587,-16.0058472608626,
124.613343042249)) ;
#73044=CARTESIAN_POINT('Ctrl Pts',(-19.543124427014,-16.1958221472349,124.913341409627)) ;
#73045=CARTESIAN_POINT('Ctrl Pts',(-19.5163642183528,-16.0158330668161,
124.61303502158)) ;
#73046=CARTESIAN_POINT('Ctrl Pts',(-19.8002495182359,-16.205756967789,124.86781116903)) ;
#73047=CARTESIAN_POINT('Ctrl Pts',(-19.7220636745429,-16.0257678873703,
124.576608849091)) ;
#73048=CARTESIAN_POINT('Ctrl Pts',(-20.0484305675954,-16.2158144929213,
124.777029790911)) ;
#73049=CARTESIAN_POINT('Ctrl Pts',(-19.9206078848616,-16.0358254125025,
124.503981752975)) ;
#73050=CARTESIAN_POINT('Ctrl Pts',(-20.2719717473582,-16.2256361435726,
124.647952173839)) ;
#73051=CARTESIAN_POINT('Ctrl Pts',(-20.0994392637093,-16.0456470631539,
124.40071820774)) ;
#73052=CARTESIAN_POINT('Ctrl Pts',(-20.4747026404971,-16.2356922070774,
124.478471590781)) ;
#73053=CARTESIAN_POINT('Ctrl Pts',(-20.2616227752683,-16.0557031266586,
124.265132163495)) ;
#73054=CARTESIAN_POINT('Ctrl Pts',(-20.6426334923553,-16.2456328741413,
124.278356285855)) ;
#73055=CARTESIAN_POINT('Ctrl Pts',(-20.395965720866,-16.0656437937226,124.105038812576)) ;
#73056=CARTESIAN_POINT('Ctrl Pts',(-20.7734945782826,-16.2555372678073,
124.053362462527)) ;
#73057=CARTESIAN_POINT('Ctrl Pts',(-20.5006527028132,-16.0755481873885,
123.925043150666)) ;
#73058=CARTESIAN_POINT('Ctrl Pts',(-20.864420115776,-16.2655837915703,123.805527276514)) ;
#73059=CARTESIAN_POINT('Ctrl Pts',(-20.5733913233788,-16.0855947111516,
123.726774248411)) ;
#73060=CARTESIAN_POINT('Ctrl Pts',(-20.9104948422774,-16.2754798745867,
123.549534920309)) ;
#73061=CARTESIAN_POINT('Ctrl Pts',(-20.6102491311177,-16.0954907941679,
123.521980487086)) ;
#73062=CARTESIAN_POINT('Ctrl Pts',(-20.9113721563936,-16.2855465738167,
123.285041710429)) ;
#73063=CARTESIAN_POINT('Ctrl Pts',(-20.6109490499967,-16.105557493398,123.310385748136)) ;
#73064=CARTESIAN_POINT('Ctrl Pts',(-20.8676796983875,-16.2953701842178,
123.030571216655)) ;
#73065=CARTESIAN_POINT('Ctrl Pts',(-20.5759933528988,-16.115381103799,123.106810427065)) ;
#73066=CARTESIAN_POINT('Ctrl Pts',(-20.7788672823149,-16.3054260443953,
122.781720920191)) ;
#73067=CARTESIAN_POINT('Ctrl Pts',(-20.5049416634882,-16.1254369639765,
122.907730678547)) ;
#73068=CARTESIAN_POINT('Ctrl Pts',(-20.6494650622141,-16.3153591907002,
122.554983567627)) ;
#73069=CARTESIAN_POINT('Ctrl Pts',(-20.4014184363261,-16.1353701102815,
122.726342029914)) ;
#73070=CARTESIAN_POINT('Ctrl Pts',(-20.4829072058007,-16.3253044464708,
122.353620794858)) ;
#73071=CARTESIAN_POINT('Ctrl Pts',(-20.2681709878727,-16.1453153660521,
122.565253212726)) ;
#73072=CARTESIAN_POINT('Ctrl Pts',(-20.2832435138197,-16.3352877449093,
122.183387066511)) ;
#73073=CARTESIAN_POINT('Ctrl Pts',(-20.1084390193321,-16.1552986644905,
122.42906766522)) ;
#73074=CARTESIAN_POINT('Ctrl Pts',(-20.0556974557649,-16.3453249250559,
122.050026596334)) ;
#73075=CARTESIAN_POINT('Ctrl Pts',(-19.9264011931984,-16.1653358446372,
122.322380816789)) ;
#73076=CARTESIAN_POINT('Ctrl Pts',(-19.8130492091126,-16.3551794777654,
121.959479734129)) ;
#73077=CARTESIAN_POINT('Ctrl Pts',(-19.7322826766303,-16.1751903973466,
122.249945218267)) ;
#73078=CARTESIAN_POINT('Ctrl Pts',(-19.5547543717507,-16.3651789962127,
121.911400782511)) ;
#73079=CARTESIAN_POINT('Ctrl Pts',(-19.5256466039838,-16.185189915794,122.211483732283)) ;
#73080=CARTESIAN_POINT('Ctrl Pts',(-19.294692522933,-16.3750740786748,121.908649507672)) ;
#73081=CARTESIAN_POINT('Ctrl Pts',(-19.3175976958741,-16.195084998256,122.209284348646)) ;
#73082=CARTESIAN_POINT('Ctrl Pts',(-19.0338948184635,-16.3851346241809,
121.951817978814)) ;
#73083=CARTESIAN_POINT('Ctrl Pts',(-19.1089596094464,-16.2051455437621,
122.243820773441)) ;
#73084=CARTESIAN_POINT('Ctrl Pts',(-18.7896903909364,-16.3949839314289,
122.03765160035)) ;
#73085=CARTESIAN_POINT('Ctrl Pts',(-18.9135973885813,-16.2149948510101,
122.312488912832)) ;
#73086=CARTESIAN_POINT('Ctrl Pts',(-18.5597221685073,-16.4050110215162,
122.166277137807)) ;
#73087=CARTESIAN_POINT('Ctrl Pts',(-18.729623508621,-16.2250219410975,122.415390653368)) ;
#73088=CARTESIAN_POINT('Ctrl Pts',(-18.355973838298,-16.4150399256532,122.33346171739)) ;
#73089=CARTESIAN_POINT('Ctrl Pts',(-18.5666258270769,-16.2350508452344,
122.549139604119)) ;
#73090=CARTESIAN_POINT('Ctrl Pts',(-18.1871403034402,-16.4248837907525,
122.529443722456)) ;
#73091=CARTESIAN_POINT('Ctrl Pts',(-18.4315607383292,-16.2448947103337,
122.705925518047)) ;
#73092=CARTESIAN_POINT('Ctrl Pts',(-18.0522973395216,-16.4348796174609,
122.754872248867)) ;
#73093=CARTESIAN_POINT('Ctrl Pts',(-18.3236876314131,-16.2548905370421,
122.886268932754)) ;
#73094=CARTESIAN_POINT('Ctrl Pts',(-17.9588203685042,-16.4449048341099,
123.001188739192)) ;
#73095=CARTESIAN_POINT('Ctrl Pts',(-18.2489074300727,-16.2649157536911,
123.083322689755)) ;
#73096=CARTESIAN_POINT('Ctrl Pts',(-17.909853990808,-16.4547946662675,123.256433493452)) ;
#73097=CARTESIAN_POINT('Ctrl Pts',(-18.2097358498301,-16.2748055858487,
123.287518087541)) ;
#73098=CARTESIAN_POINT('Ctrl Pts',(-17.9055514640211,-16.4647855223522,
123.518938743182)) ;
#73099=CARTESIAN_POINT('Ctrl Pts',(-18.2062951731,-16.2847964419335,123.497522159626)) ;
#73100=CARTESIAN_POINT('Ctrl Pts',(-17.9467544396273,-16.4747306169451,
123.777016725477)) ;
#73101=CARTESIAN_POINT('Ctrl Pts',(-18.2392588287559,-16.2947415365263,
123.70398393257)) ;
#73102=CARTESIAN_POINT('Ctrl Pts',(-18.0317409621934,-16.4846825207132,
124.024359260658)) ;
#73103=CARTESIAN_POINT('Ctrl Pts',(-18.3072491056377,-16.3046934402944,
123.901857190127)) ;
#73104=CARTESIAN_POINT('Ctrl Pts',(-18.159652183143,-16.4947189201826,124.255004194038)) ;
#73105=CARTESIAN_POINT('Ctrl Pts',(-18.4095792698802,-16.3147298397639,
124.086372598792)) ;
#73106=CARTESIAN_POINT('Ctrl Pts',(-18.3230928106585,-16.5046079902713,
124.457060170945)) ;
#73107=CARTESIAN_POINT('Ctrl Pts',(-18.5403322885734,-16.3246189098525,
124.248016015903)) ;
#73108=CARTESIAN_POINT('Ctrl Pts',(-18.5207993714394,-16.5145972796422,
124.629742950596)) ;
#73109=CARTESIAN_POINT('Ctrl Pts',(-18.6984981684148,-16.3346081992234,
124.386161255533)) ;
#73110=CARTESIAN_POINT('Ctrl Pts',(-18.7448946531259,-16.5245558458519,
124.76488924082)) ;
#73111=CARTESIAN_POINT('Ctrl Pts',(-18.8777747171326,-16.3445667654331,
124.494277080252)) ;
#73112=CARTESIAN_POINT('Ctrl Pts',(-18.987396430641,-16.5344554170687,124.859121187933)) ;
#73113=CARTESIAN_POINT('Ctrl Pts',(-19.0717758652844,-16.3544663366499,
124.569661399205)) ;
#73114=CARTESIAN_POINT('Ctrl Pts',(-19.2463751320927,-16.5445033314829,
124.910475054145)) ;
#73115=CARTESIAN_POINT('Ctrl Pts',(-19.2789592074066,-16.3645142510642,
124.610743469147)) ;
#73116=CARTESIAN_POINT('Ctrl Pts',(-19.5063926931737,-16.5543986743435,
124.91620248226)) ;
#73117=CARTESIAN_POINT('Ctrl Pts',(-19.4869725482659,-16.3744095939248,
124.615324365784)) ;
#73118=CARTESIAN_POINT('Ctrl Pts',(-19.7677103786789,-16.5644603682909,
124.876078188776)) ;
#73119=CARTESIAN_POINT('Ctrl Pts',(-19.696026799547,-16.3844712878722,124.583223879591)) ;
#73120=CARTESIAN_POINT('Ctrl Pts',(-20.0127402827486,-16.5743048213751,
124.793052261211)) ;
#73121=CARTESIAN_POINT('Ctrl Pts',(-19.8920493950965,-16.3943157409564,
124.516802517793)) ;
#73122=CARTESIAN_POINT('Ctrl Pts',(-20.2427297442012,-16.5842655063335,
124.6680922279)) ;
#73123=CARTESIAN_POINT('Ctrl Pts',(-20.0760402661694,-16.4042764259148,
124.416833962095)) ;
#73124=CARTESIAN_POINT('Ctrl Pts',(-20.4488151080384,-16.5943014388421,
124.503505578235)) ;
#73125=CARTESIAN_POINT('Ctrl Pts',(-20.2409080798894,-16.4143123584233,
124.285163870932)) ;
#73126=CARTESIAN_POINT('Ctrl Pts',(-20.6208188760599,-16.6041900545301,
124.308721850991)) ;
#73127=CARTESIAN_POINT('Ctrl Pts',(-20.3785099279013,-16.4242009741114,
124.129336942414)) ;
#73128=CARTESIAN_POINT('Ctrl Pts',(-20.7585722335936,-16.6142044636726,
124.084465548674)) ;
#73129=CARTESIAN_POINT('Ctrl Pts',(-20.4887119985352,-16.4342153832538,
123.949931533889)) ;
#73130=CARTESIAN_POINT('Ctrl Pts',(-20.8548321533235,-16.6242382726304,
123.839003471663)) ;
#73131=CARTESIAN_POINT('Ctrl Pts',(-20.5657191556869,-16.4442491922116,
123.753561447325)) ;
#73132=CARTESIAN_POINT('Ctrl Pts',(-20.9066678160013,-16.6340687268866,
123.585891332057)) ;
#73133=CARTESIAN_POINT('Ctrl Pts',(-20.6071867566373,-16.4540796464678,
123.551072756513)) ;
#73134=CARTESIAN_POINT('Ctrl Pts',(-20.9140293673925,-16.6441463944648,
123.321214560577)) ;
#73135=CARTESIAN_POINT('Ctrl Pts',(-20.6130753215692,-16.464157314046,123.33933095717)) ;
#73136=CARTESIAN_POINT('Ctrl Pts',(-20.8763072381655,-16.653998262587,123.065023312854)) ;
#73137=CARTESIAN_POINT('Ctrl Pts',(-20.5828971286681,-16.4740091821683,
123.134379095039)) ;
#73138=CARTESIAN_POINT('Ctrl Pts',(-20.7930831563035,-16.6640713001524,
122.813785638033)) ;
#73139=CARTESIAN_POINT('Ctrl Pts',(-20.5163171841745,-16.4840822197336,
122.933388811495)) ;
#73140=CARTESIAN_POINT('Ctrl Pts',(-20.6703077317906,-16.6739138535032,
122.586104119097)) ;
#73141=CARTESIAN_POINT('Ctrl Pts',(-20.4180968468373,-16.4939247730845,
122.751244883158)) ;
#73142=CARTESIAN_POINT('Ctrl Pts',(-20.5083311851296,-16.6838942489967,
122.379838432736)) ;
#73143=CARTESIAN_POINT('Ctrl Pts',(-20.288515456469,-16.5039051685779,122.586232769824)) ;
#73144=CARTESIAN_POINT('Ctrl Pts',(-20.3119093380156,-16.6939127269745,
122.204541346701)) ;
#73145=CARTESIAN_POINT('Ctrl Pts',(-20.1313776273068,-16.5139236465557,
122.445995481957)) ;
#73146=CARTESIAN_POINT('Ctrl Pts',(-20.0913143431078,-16.7037960412805,
122.067389838538)) ;
#73147=CARTESIAN_POINT('Ctrl Pts',(-19.9549021776647,-16.5238069608618,
122.336275060039)) ;
#73148=CARTESIAN_POINT('Ctrl Pts',(-19.8457714437435,-16.7138643438193,
121.968950139482)) ;
#73149=CARTESIAN_POINT('Ctrl Pts',(-19.7584674011895,-16.5338752634005,
122.25752355759)) ;
#73150=CARTESIAN_POINT('Ctrl Pts',(-19.5929691002769,-16.7236943910927,
121.91560728989)) ;
#73151=CARTESIAN_POINT('Ctrl Pts',(-19.5562266645258,-16.543705310674,122.214849855465)) ;
#73152=CARTESIAN_POINT('Ctrl Pts',(-19.3286263043333,-16.7337612625082,
121.906429428232)) ;
#73153=CARTESIAN_POINT('Ctrl Pts',(-19.3447521004645,-16.5537721820895,
122.207507801228)) ;
#73154=CARTESIAN_POINT('Ctrl Pts',(-19.0712701351288,-16.7436503013073,
121.942787563533)) ;
#73155=CARTESIAN_POINT('Ctrl Pts',(-19.1388680389634,-16.5636612208885,
122.236594472759)) ;
#73156=CARTESIAN_POINT('Ctrl Pts',(-18.8213494437406,-16.7536469994414,
122.02364571564)) ;
#73157=CARTESIAN_POINT('Ctrl Pts',(-18.9389316809213,-16.5736579190226,
122.301281090436)) ;
#73158=CARTESIAN_POINT('Ctrl Pts',(-18.5903042632467,-16.7635994251533,
122.146243992594)) ;
#73159=CARTESIAN_POINT('Ctrl Pts',(-18.7540959986369,-16.5836103447346,
122.399359670759)) ;
#73160=CARTESIAN_POINT('Ctrl Pts',(-18.3840928903676,-16.7735407273863,
122.306608387352)) ;
#73161=CARTESIAN_POINT('Ctrl Pts',(-18.5891273551198,-16.5935516469676,
122.52765094837)) ;
#73162=CARTESIAN_POINT('Ctrl Pts',(-18.2078769998156,-16.7835239664702,
122.501007316715)) ;
#73163=CARTESIAN_POINT('Ctrl Pts',(-18.4481547970743,-16.6035348860515,
122.683169946801)) ;
#73164=CARTESIAN_POINT('Ctrl Pts',(-18.067689740485,-16.7935627680388,122.724459360855)) ;
#73165=CARTESIAN_POINT('Ctrl Pts',(-18.3360050210743,-16.6135736876201,
122.861931768501)) ;
#73166=CARTESIAN_POINT('Ctrl Pts',(-17.969830608219,-16.8034108741604,122.964068373375)) ;
#73167=CARTESIAN_POINT('Ctrl Pts',(-18.2577181420015,-16.6234217937417,
123.053617920861)) ;
#73168=CARTESIAN_POINT('Ctrl Pts',(-17.9136507970271,-16.8134710697358,
123.222378870913)) ;
#73169=CARTESIAN_POINT('Ctrl Pts',(-18.2127741641893,-16.633481989317,123.260266584404)) ;
#73170=CARTESIAN_POINT('Ctrl Pts',(-17.9035805405926,-16.8233687530472,
123.482295776235)) ;
#73171=CARTESIAN_POINT('Ctrl Pts',(-18.2047179840723,-16.6433796726285,
123.468199309359)) ;
#73172=CARTESIAN_POINT('Ctrl Pts',(-17.9380616314296,-16.8332997934212,
123.740980891364)) ;
#73173=CARTESIAN_POINT('Ctrl Pts',(-18.2323025565366,-16.6533107130024,
123.675146859333)) ;
#73174=CARTESIAN_POINT('Ctrl Pts',(-18.0180896345586,-16.8433420110778,
123.992448629451)) ;
#73175=CARTESIAN_POINT('Ctrl Pts',(-18.2963248642871,-16.6633529306591,
123.876321254892)) ;
#73176=CARTESIAN_POINT('Ctrl Pts',(-18.1385099720365,-16.8532286718118,
124.222681786381)) ;
#73177=CARTESIAN_POINT('Ctrl Pts',(-18.3926605542748,-16.673239591393,124.06050710284)) ;
#73178=CARTESIAN_POINT('Ctrl Pts',(-18.2984195186838,-16.8632217804142,
124.43097259022)) ;
#73179=CARTESIAN_POINT('Ctrl Pts',(-18.5205878453715,-16.6832326999955,
124.227139806063)) ;
#73180=CARTESIAN_POINT('Ctrl Pts',(-18.4912243940238,-16.8731674790525,
124.607428923771)) ;
#73181=CARTESIAN_POINT('Ctrl Pts',(-18.6748312019824,-16.6931783986337,
124.368304761902)) ;
#73182=CARTESIAN_POINT('Ctrl Pts',(-18.711496354762,-16.8831147013235,124.748207213419)) ;
#73183=CARTESIAN_POINT('Ctrl Pts',(-18.8510481570175,-16.7031256209048,
124.480927500203)) ;
#73184=CARTESIAN_POINT('Ctrl Pts',(-18.9554062189345,-16.8931627269037,
124.849334419994)) ;
#73185=CARTESIAN_POINT('Ctrl Pts',(-19.0461761012947,-16.7131736464849,
124.561829660936)) ;
#73186=CARTESIAN_POINT('Ctrl Pts',(-19.2079801341347,-16.9030099740466,
124.905647600028)) ;
#73187=CARTESIAN_POINT('Ctrl Pts',(-19.2482340537887,-16.7230208936278,
124.606880351078)) ;
#73188=CARTESIAN_POINT('Ctrl Pts',(-19.4694948938872,-16.9129731511373,
124.918213293094)) ;
#73189=CARTESIAN_POINT('Ctrl Pts',(-19.4574454686167,-16.7329840707186,
124.616933496724)) ;
#73190=CARTESIAN_POINT('Ctrl Pts',(-19.7309060814747,-16.9230028721707,
124.884564981869)) ;
#73191=CARTESIAN_POINT('Ctrl Pts',(-19.6665745634729,-16.743013791752,124.590015342495)) ;
#73192=CARTESIAN_POINT('Ctrl Pts',(-19.9794823375519,-16.9329073397036,
124.807315147006)) ;
#73193=CARTESIAN_POINT('Ctrl Pts',(-19.8654350540059,-16.7529182592849,
124.528216247189)) ;
#73194=CARTESIAN_POINT('Ctrl Pts',(-20.2136657522084,-16.9429318255334,
124.686737651445)) ;
#73195=CARTESIAN_POINT('Ctrl Pts',(-20.0527821064406,-16.7629427451146,
124.431754771356)) ;
#73196=CARTESIAN_POINT('Ctrl Pts',(-20.4210159639658,-16.9528356606573,
124.529379524856)) ;
#73197=CARTESIAN_POINT('Ctrl Pts',(-20.2186620983548,-16.7728465802385,
124.305869231909)) ;
#73198=CARTESIAN_POINT('Ctrl Pts',(-20.6005228715883,-16.9628868513673,
124.33565635499)) ;
#73199=CARTESIAN_POINT('Ctrl Pts',(-20.3622682531827,-16.7828977709485,
124.150891007985)) ;
#73200=CARTESIAN_POINT('Ctrl Pts',(-20.7413629699218,-16.9727712940256,
124.117369250325)) ;
#73201=CARTESIAN_POINT('Ctrl Pts',(-20.4749404514896,-16.7927822136068,
123.976262404854)) ;
#73202=CARTESIAN_POINT('Ctrl Pts',(-20.8436992077545,-16.9827643018774,
123.875549411245)) ;
#73203=CARTESIAN_POINT('Ctrl Pts',(-20.5568101194757,-16.8027752214587,
123.782806994121)) ;
#73204=CARTESIAN_POINT('Ctrl Pts',(-20.9021522988049,-16.9927126215937,
123.620718922293)) ;
#73205=CARTESIAN_POINT('Ctrl Pts',(-20.6035732565573,-16.812723541175,123.578943200647)) ;
#73206=CARTESIAN_POINT('Ctrl Pts',(-20.91582621704,-17.0026494603032,123.359970070183)) ;
#73207=CARTESIAN_POINT('Ctrl Pts',(-20.6145132340894,-16.8226603798844,
123.370344673644)) ;
#73208=CARTESIAN_POINT('Ctrl Pts',(-20.8841917166136,-17.0126324492228,
123.099507780377)) ;
#73209=CARTESIAN_POINT('Ctrl Pts',(-20.5892065993372,-16.832643368804,123.161974931273)) ;
#73210=CARTESIAN_POINT('Ctrl Pts',(-20.8069010685589,-17.0226763285869,
122.847167752355)) ;
#73211=CARTESIAN_POINT('Ctrl Pts',(-20.5273748335759,-16.8426872481681,
122.960102519886)) ;
#73212=CARTESIAN_POINT('Ctrl Pts',(-20.6900614937302,-17.0325043939453,
122.616789554245)) ;
#73213=CARTESIAN_POINT('Ctrl Pts',(-20.4339045684967,-16.8525153135265,
122.775800548252)) ;
#73214=CARTESIAN_POINT('Ctrl Pts',(-20.5312178370852,-17.0425814825002,
122.404977089985)) ;
#73215=CARTESIAN_POINT('Ctrl Pts',(-20.306830239219,-16.8625924020815,122.606349695402)) ;
#73216=CARTESIAN_POINT('Ctrl Pts',(-20.3423853677135,-17.0524316346565,
122.227828485148)) ;
#73217=CARTESIAN_POINT('Ctrl Pts',(-20.1557657033809,-16.8724425542378,
122.464630732549)) ;
#73218=CARTESIAN_POINT('Ctrl Pts',(-20.1207672096657,-17.0625121151088,
122.082830799822)) ;
#73219=CARTESIAN_POINT('Ctrl Pts',(-19.9784714607027,-16.8825230346901,
122.348631493821)) ;
#73220=CARTESIAN_POINT('Ctrl Pts',(-19.8837370347765,-17.0723266128777,
121.981011738128)) ;
#73221=CARTESIAN_POINT('Ctrl Pts',(-19.7888488634291,-16.8923375324589,
122.267175689381)) ;
#73222=CARTESIAN_POINT('Ctrl Pts',(-19.6263495978727,-17.0823949088978,
121.919989507311)) ;
#73223=CARTESIAN_POINT('Ctrl Pts',(-19.5829389187349,-16.9024058284791,
122.218356659132)) ;
#73224=CARTESIAN_POINT('Ctrl Pts',(-19.3665898868757,-17.0922937413806,
121.904909547318)) ;
#73225=CARTESIAN_POINT('Ctrl Pts',(-19.3751318865944,-16.9123046609618,
122.206291541471)) ;
#73226=CARTESIAN_POINT('Ctrl Pts',(-19.1042454569166,-17.1023466213951,
121.935528536151)) ;
#73227=CARTESIAN_POINT('Ctrl Pts',(-19.1652560101051,-16.9223575409764,
122.230785548798)) ;
#73228=CARTESIAN_POINT('Ctrl Pts',(-18.8556383074816,-17.1122164368913,
122.00965239921)) ;
#73229=CARTESIAN_POINT('Ctrl Pts',(-18.9663707255866,-16.9322273564725,
122.29008319219)) ;
#73230=CARTESIAN_POINT('Ctrl Pts',(-18.618966820546,-17.1222891179741,122.128093849662)) ;
#73231=CARTESIAN_POINT('Ctrl Pts',(-18.7770327094499,-16.9423000375553,
122.384835334691)) ;
#73232=CARTESIAN_POINT('Ctrl Pts',(-18.4114058096266,-17.132121596545,122.282028735427)) ;
#73233=CARTESIAN_POINT('Ctrl Pts',(-18.6109839479363,-16.9521325161263,
122.507981587497)) ;
#73234=CARTESIAN_POINT('Ctrl Pts',(-18.2296195608036,-17.1421522305311,
122.472896223361)) ;
#73235=CARTESIAN_POINT('Ctrl Pts',(-18.4655538438899,-16.9621631501124,
122.660674621782)) ;
#73236=CARTESIAN_POINT('Ctrl Pts',(-18.0843508673433,-17.1521837877503,
122.692895741851)) ;
#73237=CARTESIAN_POINT('Ctrl Pts',(-18.3493377687508,-16.9721947073315,
122.836673575722)) ;
#73238=CARTESIAN_POINT('Ctrl Pts',(-17.9811153911421,-17.162013496622,122.92966578501)) ;
#73239=CARTESIAN_POINT('Ctrl Pts',(-18.2667484984008,-16.9820244162032,
123.026088115789)) ;
#73240=CARTESIAN_POINT('Ctrl Pts',(-17.9188078333547,-17.1720029454241,
123.184684449021)) ;
#73241=CARTESIAN_POINT('Ctrl Pts',(-18.2169009623757,-16.9920138650053,
123.230102537214)) ;
#73242=CARTESIAN_POINT('Ctrl Pts',(-17.9023020184727,-17.1820467978241,
123.448106892892)) ;
#73243=CARTESIAN_POINT('Ctrl Pts',(-18.2036948702119,-17.0020577174053,
123.440840520039)) ;
#73244=CARTESIAN_POINT('Ctrl Pts',(-17.93060345216,-17.1918685111562,123.704655127939)) ;
#73245=CARTESIAN_POINT('Ctrl Pts',(-18.2263343758186,-17.0118794307374,
123.646078286481)) ;
#73246=CARTESIAN_POINT('Ctrl Pts',(-18.0039709951869,-17.2019035161449,
123.957951976988)) ;
#73247=CARTESIAN_POINT('Ctrl Pts',(-18.2850268365724,-17.0219144357261,
123.848716309395)) ;
#73248=CARTESIAN_POINT('Ctrl Pts',(-18.1207470222398,-17.2119283545925,
124.194108297282)) ;
#73249=CARTESIAN_POINT('Ctrl Pts',(-18.3784462993163,-17.0319392741737,
124.03764205884)) ;
#73250=CARTESIAN_POINT('Ctrl Pts',(-18.273615812405,-17.2217805675477,124.403066982292)) ;
#73251=CARTESIAN_POINT('Ctrl Pts',(-18.5007395422443,-17.0417914871289,
124.204809319358)) ;
#73252=CARTESIAN_POINT('Ctrl Pts',(-18.4627330156094,-17.2317705237415,
124.585121418579)) ;
#73253=CARTESIAN_POINT('Ctrl Pts',(-18.6520320121567,-17.0517814433227,
124.350453999726)) ;
#73254=CARTESIAN_POINT('Ctrl Pts',(-18.6792511906534,-17.2416986340247,
124.730700896736)) ;
#73255=CARTESIAN_POINT('Ctrl Pts',(-18.8252452509934,-17.061709553606,124.466918770551)) ;
#73256=CARTESIAN_POINT('Ctrl Pts',(-18.9190395513251,-17.2516872341043,
124.837500135921)) ;
#73257=CARTESIAN_POINT('Ctrl Pts',(-19.0170750943207,-17.0716981536855,
124.552359735373)) ;
#73258=CARTESIAN_POINT('Ctrl Pts',(-19.1747837504995,-17.2617138260318,
124.900929840518)) ;
#73259=CARTESIAN_POINT('Ctrl Pts',(-19.2216700660752,-17.081724745613,124.603105176145)) ;
#73260=CARTESIAN_POINT('Ctrl Pts',(-19.433918408786,-17.271598954096,124.919007255926)) ;
#73261=CARTESIAN_POINT('Ctrl Pts',(-19.4289770822547,-17.0916098736772,
124.617568828664)) ;
#73262=CARTESIAN_POINT('Ctrl Pts',(-19.6951036459839,-17.2815900715695,
124.892117022708)) ;
#73263=CARTESIAN_POINT('Ctrl Pts',(-19.6379253382598,-17.1016009911507,
124.596058506662)) ;
#73264=CARTESIAN_POINT('Ctrl Pts',(-19.948740310072,-17.2916306874213,124.81939696296)) ;
#73265=CARTESIAN_POINT('Ctrl Pts',(-19.8408352281527,-17.1116416070025,
124.537884144439)) ;
#73266=CARTESIAN_POINT('Ctrl Pts',(-20.1811784262564,-17.301463678275,124.706518373468)) ;
#73267=CARTESIAN_POINT('Ctrl Pts',(-20.0267858395131,-17.1214745978562,
124.447583262725)) ;
#73268=CARTESIAN_POINT('Ctrl Pts',(-20.394335547211,-17.3114568097253,124.553138757131)) ;
#73269=CARTESIAN_POINT('Ctrl Pts',(-20.1973125961385,-17.1314677293065,
124.324881214405)) ;
#73270=CARTESIAN_POINT('Ctrl Pts',(-20.5779551583713,-17.3214888581607,
124.363950983879)) ;
#73271=CARTESIAN_POINT('Ctrl Pts',(-20.3442096485662,-17.1414997777419,
124.17353227877)) ;
#73272=CARTESIAN_POINT('Ctrl Pts',(-20.723726125488,-17.3313541047031,124.149582721449)) ;
#73273=CARTESIAN_POINT('Ctrl Pts',(-20.4608276825751,-17.1513650242843,
124.002039230348)) ;
#73274=CARTESIAN_POINT('Ctrl Pts',(-20.8317883621743,-17.3413159795299,
123.911130472927)) ;
#73275=CARTESIAN_POINT('Ctrl Pts',(-20.5472792280348,-17.1613268991111,
123.811278448521)) ;
#73276=CARTESIAN_POINT('Ctrl Pts',(-20.8968589918671,-17.3513509426412,
123.655591647124)) ;
#73277=CARTESIAN_POINT('Ctrl Pts',(-20.5993376400282,-17.1713618622224,
123.606847845879)) ;
#73278=CARTESIAN_POINT('Ctrl Pts',(-20.9167197830602,-17.3612357871036,
123.396550342785)) ;
#73279=CARTESIAN_POINT('Ctrl Pts',(-20.6152282496205,-17.1812467066848,
123.399615406321)) ;
#73280=CARTESIAN_POINT('Ctrl Pts',(-20.8907754477055,-17.3713018399443,
123.133346946216)) ;
#73281=CARTESIAN_POINT('Ctrl Pts',(-20.5944747717883,-17.1913127595256,
123.189052373295)) ;
#73282=CARTESIAN_POINT('Ctrl Pts',(-20.8213961193657,-17.3811393558533,
122.884260853047)) ;
#73283=CARTESIAN_POINT('Ctrl Pts',(-20.5389734280671,-17.2011502754345,
122.989783496606)) ;
#73284=CARTESIAN_POINT('Ctrl Pts',(-20.707493461148,-17.3912081039621,122.645486865897)) ;
#73285=CARTESIAN_POINT('Ctrl Pts',(-20.4478531284103,-17.2112190235434,
122.798763308908)) ;
#73286=CARTESIAN_POINT('Ctrl Pts',(-20.5566061674154,-17.4010886209932,
122.434129920222)) ;
#73287=CARTESIAN_POINT('Ctrl Pts',(-20.3271452112243,-17.2210995405744,
122.629676886925)) ;
#73288=CARTESIAN_POINT('Ctrl Pts',(-20.3696663137134,-17.4110798079276,
122.24982053188)) ;
#73289=CARTESIAN_POINT('Ctrl Pts',(-20.1775948836073,-17.2310907275089,
122.482227931951)) ;
#73290=CARTESIAN_POINT('Ctrl Pts',(-20.1543475644232,-17.4210328742026,
122.101259878742)) ;
#73291=CARTESIAN_POINT('Ctrl Pts',(-20.0053412412653,-17.2410437937838,
122.363377768744)) ;
#73292=CARTESIAN_POINT('Ctrl Pts',(-19.914546699615,-17.4310687117352,121.991540433693)) ;
#73293=CARTESIAN_POINT('Ctrl Pts',(-19.8135014215866,-17.2510796313164,
122.275600286841)) ;
#73294=CARTESIAN_POINT('Ctrl Pts',(-19.6630503154199,-17.4409588379466,
121.925907930573)) ;
#73295=CARTESIAN_POINT('Ctrl Pts',(-19.6123051763993,-17.2609697575279,
122.223092308256)) ;
#73296=CARTESIAN_POINT('Ctrl Pts',(-19.401369792171,-17.4509510198546,121.904306259292)) ;
#73297=CARTESIAN_POINT('Ctrl Pts',(-19.4029610196723,-17.2709619394358,
122.205808818119)) ;
#73298=CARTESIAN_POINT('Ctrl Pts',(-19.1411178680635,-17.4608969597931,
121.928446401785)) ;
#73299=CARTESIAN_POINT('Ctrl Pts',(-19.1947594651076,-17.2809078793744,
122.22511876556)) ;
#73300=CARTESIAN_POINT('Ctrl Pts',(-18.8888264116577,-17.4708441435572,
121.996908692717)) ;
#73301=CARTESIAN_POINT('Ctrl Pts',(-18.9929258788226,-17.2908550631385,
122.279886435726)) ;
#73302=CARTESIAN_POINT('Ctrl Pts',(-18.6500049664058,-17.4808920818647,
122.109521528278)) ;
#73303=CARTESIAN_POINT('Ctrl Pts',(-18.8018677870459,-17.300903001446,122.369974738324)) ;
#73304=CARTESIAN_POINT('Ctrl Pts',(-18.4385276907315,-17.490739716605,122.258681232151)) ;
#73305=CARTESIAN_POINT('Ctrl Pts',(-18.6326849625005,-17.3107506361862,
122.489300526383)) ;
#73306=CARTESIAN_POINT('Ctrl Pts',(-18.2534782916125,-17.5007014305788,
122.443832320231)) ;
#73307=CARTESIAN_POINT('Ctrl Pts',(-18.4846439297647,-17.3207123501601,
122.637419744003)) ;
#73308=CARTESIAN_POINT('Ctrl Pts',(-18.102637182743,-17.5107300653696,122.659957308394)) ;
#73309=CARTESIAN_POINT('Ctrl Pts',(-18.3639692439427,-17.3307409849509,
122.810318436287)) ;
#73310=CARTESIAN_POINT('Ctrl Pts',(-17.9928588042653,-17.5206403839668,
122.896109111967)) ;
#73311=CARTESIAN_POINT('Ctrl Pts',(-18.2761445935121,-17.340651303548,122.999238788582)) ;
#73312=CARTESIAN_POINT('Ctrl Pts',(-17.9249170447075,-17.5305752402783,
123.148201377901)) ;
#73313=CARTESIAN_POINT('Ctrl Pts',(-18.2217890416061,-17.3505861598595,
123.200911914671)) ;
#73314=CARTESIAN_POINT('Ctrl Pts',(-17.9017863180656,-17.540616476239,123.411046406639)) ;
#73315=CARTESIAN_POINT('Ctrl Pts',(-18.2032822312824,-17.3606273958202,
123.411187703811)) ;
#73316=CARTESIAN_POINT('Ctrl Pts',(-17.9240826084137,-17.550503247819,123.669927416852)) ;
#73317=CARTESIAN_POINT('Ctrl Pts',(-18.221117014871,-17.3705141674002,123.618292577988)) ;
#73318=CARTESIAN_POINT('Ctrl Pts',(-17.991434789248,-17.5605034265252,123.923904178017)) ;
#73319=CARTESIAN_POINT('Ctrl Pts',(-18.274996565428,-17.3805143461064,123.821474510317)) ;
#73320=CARTESIAN_POINT('Ctrl Pts',(-18.1007768932727,-17.5704207047348,
124.160520976259)) ;
#73321=CARTESIAN_POINT('Ctrl Pts',(-18.3624681751621,-17.390431624316,124.010768829435)) ;
#73322=CARTESIAN_POINT('Ctrl Pts',(-18.2515125585138,-17.5804679511484,
124.377250917373)) ;
#73323=CARTESIAN_POINT('Ctrl Pts',(-18.4830548228013,-17.4004788707297,
124.184154022707)) ;
#73324=CARTESIAN_POINT('Ctrl Pts',(-18.4342365121669,-17.5903418401297,
124.561534748414)) ;
#73325=CARTESIAN_POINT('Ctrl Pts',(-18.6292323540018,-17.410352759711,124.331582640151)) ;
#73326=CARTESIAN_POINT('Ctrl Pts',(-18.650076844133,-17.6004038577103,124.714221581085)) ;
#73327=CARTESIAN_POINT('Ctrl Pts',(-18.8019032612626,-17.4204147772915,
124.453733907963)) ;
#73328=CARTESIAN_POINT('Ctrl Pts',(-18.8846741124993,-17.6102749194446,
124.824958215728)) ;
#73329=CARTESIAN_POINT('Ctrl Pts',(-18.9895801047362,-17.4302858390258,
124.542325248395)) ;
#73330=CARTESIAN_POINT('Ctrl Pts',(-19.1378416764561,-17.6202689828049,
124.894832090655)) ;
#73331=CARTESIAN_POINT('Ctrl Pts',(-19.1921135246435,-17.4402799023861,
124.598226499213)) ;
#73332=CARTESIAN_POINT('Ctrl Pts',(-19.4003404043873,-17.6303011408383,
124.919197850821)) ;
#73333=CARTESIAN_POINT('Ctrl Pts',(-19.4021122156701,-17.4503120604195,
124.617721341599)) ;
#73334=CARTESIAN_POINT('Ctrl Pts',(-19.6587556166612,-17.6401650170784,
124.898540308971)) ;
#73335=CARTESIAN_POINT('Ctrl Pts',(-19.6088446217045,-17.4601759366597,
124.601197540958)) ;
#73336=CARTESIAN_POINT('Ctrl Pts',(-19.9148657636386,-17.6502355317167,
124.83200511838)) ;
#73337=CARTESIAN_POINT('Ctrl Pts',(-19.8137332138143,-17.470246451298,124.54797155282)) ;
#73338=CARTESIAN_POINT('Ctrl Pts',(-20.15009547768,-17.6600761686577,124.72452389288)) ;
#73339=CARTESIAN_POINT('Ctrl Pts',(-20.0019179240621,-17.4800870882389,
124.461988673264)) ;
#73340=CARTESIAN_POINT('Ctrl Pts',(-20.36628172174,-17.6700432974979,124.576684081939)) ;
#73341=CARTESIAN_POINT('Ctrl Pts',(-20.1748686108959,-17.4900542170791,
124.343718154926)) ;
#73342=CARTESIAN_POINT('Ctrl Pts',(-20.5542290543872,-17.6800572706224,
124.392466662708)) ;
#73343=CARTESIAN_POINT('Ctrl Pts',(-20.3252263581462,-17.5000681902037,
124.196347578167)) ;
#73344=CARTESIAN_POINT('Ctrl Pts',(-20.7574242466008,-17.6933420044857,
124.108563216876)) ;
#73345=CARTESIAN_POINT('Ctrl Pts',(-20.487792909875,-17.5133529240669,123.969217895372)) ;
#73346=CARTESIAN_POINT('Ctrl Pts',(-20.8815792328833,-17.7065672692004,
123.77977638725)) ;
#73347=CARTESIAN_POINT('Ctrl Pts',(-20.5871211385938,-17.5265781887817,
123.706157444669)) ;
#73348=CARTESIAN_POINT('Ctrl Pts',(-20.916715626838,-17.7198777917553,123.431719811704)) ;
#73349=CARTESIAN_POINT('Ctrl Pts',(-20.6152233992077,-17.5398887113366,
123.427758937628)) ;
#73350=CARTESIAN_POINT('Ctrl Pts',(-20.8970403046857,-17.7299064366575,
123.168922156218)) ;
#73351=CARTESIAN_POINT('Ctrl Pts',(-20.599487173877,-17.5499173562387,123.217511388876)) ;
#73352=CARTESIAN_POINT('Ctrl Pts',(-20.8332113375224,-17.7397874690114,
122.91722016416)) ;
#73353=CARTESIAN_POINT('Ctrl Pts',(-20.5484257925112,-17.5597983885926,
123.016151680332)) ;
#73354=CARTESIAN_POINT('Ctrl Pts',(-20.7260717927745,-17.7497684416915,
122.677813694356)) ;
#73355=CARTESIAN_POINT('Ctrl Pts',(-20.4627150058846,-17.5697793612727,
122.824624299976)) ;
#73356=CARTESIAN_POINT('Ctrl Pts',(-20.5788081877932,-17.7597495692775,
122.460780265019)) ;
#73357=CARTESIAN_POINT('Ctrl Pts',(-20.3449101987234,-17.5797604888587,
122.650998991699)) ;
#73358=CARTESIAN_POINT('Ctrl Pts',(-20.3368568947964,-17.7729927595389,
122.210535455746)) ;
#73359=CARTESIAN_POINT('Ctrl Pts',(-20.1513291199415,-17.5930036791201,
122.450788794857)) ;
#73360=CARTESIAN_POINT('Ctrl Pts',(-19.9569936985666,-17.7896607548997,
121.982786748416)) ;
#73361=CARTESIAN_POINT('Ctrl Pts',(-19.8474794990023,-17.6096716744809,
122.26860190868)) ;
#73362=CARTESIAN_POINT('Ctrl Pts',(-19.5259606159714,-17.8061812549117,
121.898720902047)) ;
#73363=CARTESIAN_POINT('Ctrl Pts',(-19.5025885463891,-17.626192174493,122.201337274905)) ;
#73364=CARTESIAN_POINT('Ctrl Pts',(-19.1769501917538,-17.8194942712277,
121.922374301819)) ;
#73365=CARTESIAN_POINT('Ctrl Pts',(-19.2234321602598,-17.639505190809,122.220261939682)) ;
#73366=CARTESIAN_POINT('Ctrl Pts',(-18.923841446365,-17.8294108294607,121.984571342108)) ;
#73367=CARTESIAN_POINT('Ctrl Pts',(-19.0209334397387,-17.649421749042,122.270017435273)) ;
#73368=CARTESIAN_POINT('Ctrl Pts',(-18.6828367950718,-17.8394384977636,
122.090994480647)) ;
#73369=CARTESIAN_POINT('Ctrl Pts',(-18.8281336451652,-17.6594494173448,
122.355152451845)) ;
#73370=CARTESIAN_POINT('Ctrl Pts',(-18.39451589716,-17.8526190875082,122.283176068352)) ;
#73371=CARTESIAN_POINT('Ctrl Pts',(-18.5974653676165,-17.6726300070895,
122.50890583314)) ;
#73372=CARTESIAN_POINT('Ctrl Pts',(-18.10101635581,-17.8693672266276,122.617564692497)) ;
#73373=CARTESIAN_POINT('Ctrl Pts',(-18.3626740164398,-17.6893781462089,
122.776403445059)) ;
#73374=CARTESIAN_POINT('Ctrl Pts',(-17.9093611844789,-17.8891619691382,
123.107788785558)) ;
#73375=CARTESIAN_POINT('Ctrl Pts',(-18.2093429356618,-17.7091728887194,
123.168586034307)) ;
#73376=CARTESIAN_POINT('Ctrl Pts',(-17.8958042830231,-17.909206361947,123.640179567823)) ;
#73377=CARTESIAN_POINT('Ctrl Pts',(-18.198495043607,-17.7292172815282,123.594497346099)) ;
#73378=CARTESIAN_POINT('Ctrl Pts',(-18.0635490482138,-17.9290455442457,
124.140228438877)) ;
#73379=CARTESIAN_POINT('Ctrl Pts',(-18.3326878464618,-17.7490564638269,
123.994538700796)) ;
#73380=CARTESIAN_POINT('Ctrl Pts',(-18.3920994919376,-17.9489708679386,
124.555410464729)) ;
#73381=CARTESIAN_POINT('Ctrl Pts',(-18.5955264281991,-17.7689817875198,
124.3266864764)) ;
#73382=CARTESIAN_POINT('Ctrl Pts',(-18.8427886963338,-17.9688945059901,
124.833584548263)) ;
#73383=CARTESIAN_POINT('Ctrl Pts',(-18.9560768416233,-17.7889054255713,
124.549228339882)) ;
#73384=CARTESIAN_POINT('Ctrl Pts',(-19.3612051307103,-17.9888193794556,
124.941403037261)) ;
#73385=CARTESIAN_POINT('Ctrl Pts',(-19.3708100925674,-17.8088302990368,
124.635485728076)) ;
#73386=CARTESIAN_POINT('Ctrl Pts',(-19.8842672961532,-18.0086979865345,
124.866686275116)) ;
#73387=CARTESIAN_POINT('Ctrl Pts',(-19.7892612316858,-17.8287089061158,
124.575714277679)) ;
#73388=CARTESIAN_POINT('Ctrl Pts',(-20.3528378763399,-18.0286754293665,
124.61697267285)) ;
#73389=CARTESIAN_POINT('Ctrl Pts',(-20.1641187657695,-17.8486863489478,
124.375944971353)) ;
#73390=CARTESIAN_POINT('Ctrl Pts',(-20.7070199752572,-18.0486072774512,
124.222957551438)) ;
#73391=CARTESIAN_POINT('Ctrl Pts',(-20.4474662649599,-17.8686181970324,
124.060733674475)) ;
#73392=CARTESIAN_POINT('Ctrl Pts',(-20.9055702119304,-18.0685025457937,
123.732901280478)) ;
#73393=CARTESIAN_POINT('Ctrl Pts',(-20.6063082810486,-17.888513465375,123.668688213802)) ;
#73394=CARTESIAN_POINT('Ctrl Pts',(-20.9255908589507,-18.0884250442059,
123.203759760793)) ;
#73395=CARTESIAN_POINT('Ctrl Pts',(-20.622325941902,-17.9084359637871,123.245374181992)) ;
#73396=CARTESIAN_POINT('Ctrl Pts',(-20.7634037511699,-18.1083845260819,
122.698638234476)) ;
#73397=CARTESIAN_POINT('Ctrl Pts',(-20.4925770626071,-17.9283954456631,
122.84127622867)) ;
#73398=CARTESIAN_POINT('Ctrl Pts',(-20.4400561873838,-18.1282622785412,
122.280931726658)) ;
#73399=CARTESIAN_POINT('Ctrl Pts',(-20.2338986900793,-17.9482731981225,
122.507109352624)) ;
#73400=CARTESIAN_POINT('Ctrl Pts',(-19.9941357017642,-18.1481440692758,
121.997211525616)) ;
#73401=CARTESIAN_POINT('Ctrl Pts',(-19.8771609449229,-17.9681549888571,
122.280132520306)) ;
#73402=CARTESIAN_POINT('Ctrl Pts',(-19.473136676443,-18.1682174081268,121.882665391147)) ;
#73403=CARTESIAN_POINT('Ctrl Pts',(-19.4603626713499,-17.988228327708,122.188495684092)) ;
#73404=CARTESIAN_POINT('Ctrl Pts',(-18.9512092801741,-18.1880218753626,
121.951729931277)) ;
#73405=CARTESIAN_POINT('Ctrl Pts',(-19.0428183076886,-18.0080327949438,
122.243747774639)) ;
#73406=CARTESIAN_POINT('Ctrl Pts',(-18.4795781027721,-18.2080052157704,
122.195819043175)) ;
#73407=CARTESIAN_POINT('Ctrl Pts',(-18.665513625463,-18.0280161353516,122.43901994105)) ;
#73408=CARTESIAN_POINT('Ctrl Pts',(-18.1213593078201,-18.2279201803684,
122.58549305673)) ;
#73409=CARTESIAN_POINT('Ctrl Pts',(-18.3789384269809,-18.0479310999496,
122.750760357878)) ;
#73410=CARTESIAN_POINT('Ctrl Pts',(-17.9166900270901,-18.2477887150847,
123.07239884694)) ;
#73411=CARTESIAN_POINT('Ctrl Pts',(-18.2152038535447,-18.067799634666,123.140286849332)) ;
#73412=CARTESIAN_POINT('Ctrl Pts',(-17.8910961295318,-18.2678410992965,
123.604588275997)) ;
#73413=CARTESIAN_POINT('Ctrl Pts',(-18.1947300898754,-18.0878520188777,
123.566037963837)) ;
#73414=CARTESIAN_POINT('Ctrl Pts',(-18.0458895721148,-18.2876150630857,
124.107054946162)) ;
#73415=CARTESIAN_POINT('Ctrl Pts',(-18.3185671783008,-18.1076259826669,
123.968012895512)) ;
#73416=CARTESIAN_POINT('Ctrl Pts',(-18.3667637787931,-18.307669442107,124.53239666569)) ;
#73417=CARTESIAN_POINT('Ctrl Pts',(-18.5752679245152,-18.1276803616883,
124.308284615384)) ;
#73418=CARTESIAN_POINT('Ctrl Pts',(-18.8082021318199,-18.3274661796803,
124.819004328832)) ;
#73419=CARTESIAN_POINT('Ctrl Pts',(-18.9284212935939,-18.1474770992615,
124.537569929665)) ;
#73420=CARTESIAN_POINT('Ctrl Pts',(-19.3247749684694,-18.3474339920317,
124.940168786591)) ;
#73421=CARTESIAN_POINT('Ctrl Pts',(-19.3416804332519,-18.167444911613,124.634498827263)) ;
#73422=CARTESIAN_POINT('Ctrl Pts',(-19.8515753100057,-18.3673929680968,
124.876958419537)) ;
#73423=CARTESIAN_POINT('Ctrl Pts',(-19.7631206608013,-18.187403887678,124.583927892231)) ;
#73424=CARTESIAN_POINT('Ctrl Pts',(-20.3237057375478,-18.3872878863742,
124.638896796403)) ;
#73425=CARTESIAN_POINT('Ctrl Pts',(-20.140824401647,-18.2072988059554,124.393475677266)) ;
#73426=CARTESIAN_POINT('Ctrl Pts',(-20.6867396805828,-18.4071841988245,
124.254454113003)) ;
#73427=CARTESIAN_POINT('Ctrl Pts',(-20.4312497270068,-18.2271951184057,
124.085918852288)) ;
#73428=CARTESIAN_POINT('Ctrl Pts',(-20.8974889910518,-18.4270921321986,
123.769075405449)) ;
#73429=CARTESIAN_POINT('Ctrl Pts',(-20.5998462757639,-18.2471030517799,
123.697614033343)) ;
#73430=CARTESIAN_POINT('Ctrl Pts',(-20.9299591275566,-18.4470420224871,
123.239880881326)) ;
#73431=CARTESIAN_POINT('Ctrl Pts',(-20.6258188645366,-18.2670529420683,
123.274257946613)) ;
#73432=CARTESIAN_POINT('Ctrl Pts',(-20.7809301919125,-18.4669192529884,
122.732978965345)) ;
#73433=CARTESIAN_POINT('Ctrl Pts',(-20.5065921666265,-18.2869301725696,
122.868736840689)) ;
#73434=CARTESIAN_POINT('Ctrl Pts',(-20.4664719535543,-18.4869019218594,
122.305004321839)) ;
#73435=CARTESIAN_POINT('Ctrl Pts',(-20.2550218602243,-18.3069128414406,
122.526359509871)) ;
#73436=CARTESIAN_POINT('Ctrl Pts',(-20.0256670326503,-18.5068348084397,
122.011010323999)) ;
#73437=CARTESIAN_POINT('Ctrl Pts',(-19.9023778434081,-18.326845728021,122.291166823134)) ;
#73438=CARTESIAN_POINT('Ctrl Pts',(-19.5117084694472,-18.5267475544577,
121.884894904179)) ;
#73439=CARTESIAN_POINT('Ctrl Pts',(-19.4912012916676,-18.3467584740389,
122.190280271835)) ;
#73440=CARTESIAN_POINT('Ctrl Pts',(-19.073811833589,-18.5433172757995,121.931691304988)) ;
#73441=CARTESIAN_POINT('Ctrl Pts',(-19.140910274212,-18.3633281953808,122.227714621675)) ;
#73442=CARTESIAN_POINT('Ctrl Pts',(-18.7476501459948,-18.5566172871045,
122.057314468822)) ;
#73443=CARTESIAN_POINT('Ctrl Pts',(-18.8799531105504,-18.3766282066857,
122.32822609425)) ;
#73444=CARTESIAN_POINT('Ctrl Pts',(-18.4486656985439,-18.5698874748544,
122.236842368707)) ;
#73445=CARTESIAN_POINT('Ctrl Pts',(-18.6408115504094,-18.3898983944356,
122.471815668889)) ;
#73446=CARTESIAN_POINT('Ctrl Pts',(-18.1413722272559,-18.5865148572198,
122.554451895043)) ;
#73447=CARTESIAN_POINT('Ctrl Pts',(-18.3949285205775,-18.406525776801,122.72595265338)) ;
#73448=CARTESIAN_POINT('Ctrl Pts',(-17.9611265355319,-18.603137146965,122.957810899834)) ;
#73449=CARTESIAN_POINT('Ctrl Pts',(-18.2507608262965,-18.4231480665462,
123.048601618741)) ;
#73450=CARTESIAN_POINT('Ctrl Pts',(-17.9059528960428,-18.6163823613595,
123.301475150402)) ;
#73451=CARTESIAN_POINT('Ctrl Pts',(-18.2066124741129,-18.4363932809408,
123.323560293853)) ;
#73452=CARTESIAN_POINT('Ctrl Pts',(-17.9091768533096,-18.6262943263202,
123.56194849763)) ;
#73453=CARTESIAN_POINT('Ctrl Pts',(-18.2091963170387,-18.4463052459014,
123.53193369723)) ;
#73454=CARTESIAN_POINT('Ctrl Pts',(-17.9585883654437,-18.6363529494846,
123.821589557135)) ;
#73455=CARTESIAN_POINT('Ctrl Pts',(-18.2487269958253,-18.4563638690659,
123.739647432984)) ;
#73456=CARTESIAN_POINT('Ctrl Pts',(-18.049960971692,-18.6461930636004,124.063536985051)) ;
#73457=CARTESIAN_POINT('Ctrl Pts',(-18.3218274009337,-18.4662039831817,
123.933204397028)) ;
#73458=CARTESIAN_POINT('Ctrl Pts',(-18.1847150492147,-18.6562588485581,
124.291112489649)) ;
#73459=CARTESIAN_POINT('Ctrl Pts',(-18.4296324649852,-18.4762697681393,
124.11526364337)) ;
#73460=CARTESIAN_POINT('Ctrl Pts',(-18.3539469882503,-18.666142166346,124.488176476343)) ;
#73461=CARTESIAN_POINT('Ctrl Pts',(-18.5650197804419,-18.4861530859272,
124.272913430482)) ;
#73462=CARTESIAN_POINT('Ctrl Pts',(-18.5565725703679,-18.6761316042045,
124.655035297665)) ;
#73463=CARTESIAN_POINT('Ctrl Pts',(-18.7271216359093,-18.4961425237858,
124.406398725453)) ;
#73464=CARTESIAN_POINT('Ctrl Pts',(-18.7845837389878,-18.6860953182573,
124.783781642354)) ;
#73465=CARTESIAN_POINT('Ctrl Pts',(-18.9095316568693,-18.5061062378385,
124.509393835218)) ;
#73466=CARTESIAN_POINT('Ctrl Pts',(-19.0321760408451,-18.6960903299165,
124.871518685356)) ;
#73467=CARTESIAN_POINT('Ctrl Pts',(-19.1076061994151,-18.5161012494978,
124.579581328801)) ;
#73468=CARTESIAN_POINT('Ctrl Pts',(-19.2923475774085,-18.7061266216107,
124.914699798587)) ;
#73469=CARTESIAN_POINT('Ctrl Pts',(-19.3157437283926,-18.526137541192,124.614123995732)) ;
#73470=CARTESIAN_POINT('Ctrl Pts',(-19.5511061455459,-18.7159729993042,
124.912522869841)) ;
#73471=CARTESIAN_POINT('Ctrl Pts',(-19.5227505956409,-18.5359839188854,
124.612380200103)) ;
#73472=CARTESIAN_POINT('Ctrl Pts',(-19.8091754394453,-18.7259579434549,
124.865290742825)) ;
#73473=CARTESIAN_POINT('Ctrl Pts',(-19.7292055595761,-18.5459688630361,
124.574592283995)) ;
#73474=CARTESIAN_POINT('Ctrl Pts',(-20.0540693302902,-18.7358949145848,
124.774521245397)) ;
#73475=CARTESIAN_POINT('Ctrl Pts',(-19.9251198339151,-18.5559058341661,
124.50197459087)) ;
#73476=CARTESIAN_POINT('Ctrl Pts',(-20.2819125649474,-18.7459446992166,
124.641024555296)) ;
#73477=CARTESIAN_POINT('Ctrl Pts',(-20.1073932380398,-18.5659556187978,
124.395175312067)) ;
#73478=CARTESIAN_POINT('Ctrl Pts',(-20.4792864442307,-18.755795161294,124.473508135912)) ;
#73479=CARTESIAN_POINT('Ctrl Pts',(-20.2652908081466,-18.5758060808753,
124.261160516284)) ;
#73480=CARTESIAN_POINT('Ctrl Pts',(-20.6471074504363,-18.7657671748145,
124.272284173906)) ;
#73481=CARTESIAN_POINT('Ctrl Pts',(-20.3995458257233,-18.5857780943957,
124.100179977328)) ;
#73482=CARTESIAN_POINT('Ctrl Pts',(-20.7777500987277,-18.7757623219339,
124.044367513395)) ;
#73483=CARTESIAN_POINT('Ctrl Pts',(-20.5040579656922,-18.5957732415151,
123.917845587999)) ;
#73484=CARTESIAN_POINT('Ctrl Pts',(-20.8668580982505,-18.78579629167,123.796222100958)) ;
#73485=CARTESIAN_POINT('Ctrl Pts',(-20.5753422305749,-18.6058072112512,
123.719328523745)) ;
#73486=CARTESIAN_POINT('Ctrl Pts',(-20.9111412971534,-18.7956518373406,
123.541018035023)) ;
#73487=CARTESIAN_POINT('Ctrl Pts',(-20.6107665482665,-18.6156627569218,
123.515165073301)) ;
#73488=CARTESIAN_POINT('Ctrl Pts',(-20.9107995972863,-18.8056505943538,
123.278303845411)) ;
#73489=CARTESIAN_POINT('Ctrl Pts',(-20.6104909554121,-18.6256615139351,
123.304993798075)) ;
#73490=CARTESIAN_POINT('Ctrl Pts',(-20.8655454312837,-18.815547729591,123.02214521666)) ;
#73491=CARTESIAN_POINT('Ctrl Pts',(-20.5742854776814,-18.6355586491722,
123.100067482626)) ;
#73492=CARTESIAN_POINT('Ctrl Pts',(-20.775165350312,-18.8256008254306,122.773930212828)) ;
#73493=CARTESIAN_POINT('Ctrl Pts',(-20.5019793282326,-18.6456117450119,
122.901496230122)) ;
#73494=CARTESIAN_POINT('Ctrl Pts',(-20.6452882014152,-18.8354843341612,
122.548985779886)) ;
#73495=CARTESIAN_POINT('Ctrl Pts',(-20.3980758193706,-18.6554952537425,
122.72154200763)) ;
#73496=CARTESIAN_POINT('Ctrl Pts',(-20.4769328739759,-18.8454792068073,
122.347392525911)) ;
#73497=CARTESIAN_POINT('Ctrl Pts',(-20.2633899435099,-18.6654901263886,
122.56026886385)) ;
#73498=CARTESIAN_POINT('Ctrl Pts',(-20.2753461931263,-18.855499168443,122.177967546798)) ;
#73499=CARTESIAN_POINT('Ctrl Pts',(-20.1021192027833,-18.6755100880243,
122.424730580812)) ;
#73500=CARTESIAN_POINT('Ctrl Pts',(-20.0501362495911,-18.8654045322428,
122.047445707161)) ;
#73501=CARTESIAN_POINT('Ctrl Pts',(-19.9219503672684,-18.6854154518241,
122.320315127144)) ;
#73502=CARTESIAN_POINT('Ctrl Pts',(-19.8050116122457,-18.8753451198504,
121.957195984755)) ;
#73503=CARTESIAN_POINT('Ctrl Pts',(-19.7258501182768,-18.6953560394316,
122.248117437871)) ;
#73504=CARTESIAN_POINT('Ctrl Pts',(-19.546310543461,-18.885347937951,121.91043255485)) ;
#73505=CARTESIAN_POINT('Ctrl Pts',(-19.5188889496675,-18.7053588575323,
122.21070880072)) ;
#73506=CARTESIAN_POINT('Ctrl Pts',(-19.2826245313338,-18.8953826496752,
121.909724812261)) ;
#73507=CARTESIAN_POINT('Ctrl Pts',(-19.307940120733,-18.7153935692564,122.21014477667)) ;
#73508=CARTESIAN_POINT('Ctrl Pts',(-19.0276297317508,-18.9052275564125,
121.953532899853)) ;
#73509=CARTESIAN_POINT('Ctrl Pts',(-19.1039450889391,-18.7252384759937,
122.245193267705)) ;
#73510=CARTESIAN_POINT('Ctrl Pts',(-18.7805173028943,-18.9152134089815,
122.041718001938)) ;
#73511=CARTESIAN_POINT('Ctrl Pts',(-18.906255967733,-18.7352243285627,122.315743268288)) ;
#73512=CARTESIAN_POINT('Ctrl Pts',(-18.5534655976855,-18.9251482173945,
122.170689853557)) ;
#73513=CARTESIAN_POINT('Ctrl Pts',(-18.7246158475465,-18.7451591369758,
122.418922408914)) ;
#73514=CARTESIAN_POINT('Ctrl Pts',(-18.3499886137343,-18.9352057444756,
122.339308389703)) ;
#73515=CARTESIAN_POINT('Ctrl Pts',(-18.5618355205911,-18.7552166640568,
122.553818905849)) ;
#73516=CARTESIAN_POINT('Ctrl Pts',(-18.1825491267015,-18.9450273994727,
122.535766487473)) ;
#73517=CARTESIAN_POINT('Ctrl Pts',(-18.4278858915271,-18.7650383190539,
122.710986228041)) ;
#73518=CARTESIAN_POINT('Ctrl Pts',(-18.0482437941304,-18.9550834436457,
122.76333018738)) ;
#73519=CARTESIAN_POINT('Ctrl Pts',(-18.3204432872126,-18.775094363227,122.893038272163)) ;
#73520=CARTESIAN_POINT('Ctrl Pts',(-17.956984649217,-18.9650241836909,123.008115620712)) ;
#73521=CARTESIAN_POINT('Ctrl Pts',(-18.2474379774065,-18.7850351032721,
123.08886708059)) ;
#73522=CARTESIAN_POINT('Ctrl Pts',(-17.9089873947582,-18.9749283047637,
123.263925149261)) ;
#73523=CARTESIAN_POINT('Ctrl Pts',(-18.2090421543443,-18.794939224345,123.293514641434)) ;
#73524=CARTESIAN_POINT('Ctrl Pts',(-17.9062567713338,-18.984975845918,123.527931134954)) ;
#73525=CARTESIAN_POINT('Ctrl Pts',(-18.2068596105166,-18.8049867654992,
123.504719530089)) ;
#73526=CARTESIAN_POINT('Ctrl Pts',(-17.9485884795038,-18.9948745975184,
123.784627499335)) ;
#73527=CARTESIAN_POINT('Ctrl Pts',(-18.2407268052107,-18.8148855170996,
123.710075859708)) ;
#73528=CARTESIAN_POINT('Ctrl Pts',(-18.0360231030446,-19.0049230764842,
124.033764662954)) ;
#73529=CARTESIAN_POINT('Ctrl Pts',(-18.3106763436582,-18.8249339960654,
123.909385048735)) ;
#73530=CARTESIAN_POINT('Ctrl Pts',(-18.1633256706867,-19.0148105735679,
124.260307326512)) ;
#73531=CARTESIAN_POINT('Ctrl Pts',(-18.4125198128121,-18.8348214931492,
124.09061779922)) ;
#73532=CARTESIAN_POINT('Ctrl Pts',(-18.3293793931131,-19.024803663866,124.463720725773)) ;
#73533=CARTESIAN_POINT('Ctrl Pts',(-18.5453641388487,-18.8448145834472,
124.253347258974)) ;
#73534=CARTESIAN_POINT('Ctrl Pts',(-18.5275042406055,-19.0347558339263,
124.634466519948)) ;
#73535=CARTESIAN_POINT('Ctrl Pts',(-18.7038650100524,-18.8547667535075,
124.389942302569)) ;
#73536=CARTESIAN_POINT('Ctrl Pts',(-18.7517438317054,-19.0446942538408,
124.768323296915)) ;
#73537=CARTESIAN_POINT('Ctrl Pts',(-18.8832572996416,-18.864705173422,124.497025999753)) ;
#73538=CARTESIAN_POINT('Ctrl Pts',(-18.9969024435073,-19.0546793839264,
124.861939962905)) ;
#73539=CARTESIAN_POINT('Ctrl Pts',(-19.079384667915,-18.8746903035076,124.571917644386)) ;
#73540=CARTESIAN_POINT('Ctrl Pts',(-19.2559540582283,-19.0647160733405,
124.911430511903)) ;
#73541=CARTESIAN_POINT('Ctrl Pts',(-19.286626370737,-18.8847269929217,124.611508315008)) ;
#73542=CARTESIAN_POINT('Ctrl Pts',(-19.5149158429189,-19.074570757333,124.915534596045)) ;
#73543=CARTESIAN_POINT('Ctrl Pts',(-19.4937950895379,-18.8945816769142,
124.614789827494)) ;
#73544=CARTESIAN_POINT('Ctrl Pts',(-19.7744035154706,-19.0845702413808,
124.874379795797)) ;
#73545=CARTESIAN_POINT('Ctrl Pts',(-19.7013848578054,-18.9045811609621,
124.581864340682)) ;
#73546=CARTESIAN_POINT('Ctrl Pts',(-20.0203843648942,-19.0944653301577,
124.789921645729)) ;
#73547=CARTESIAN_POINT('Ctrl Pts',(-19.898168451651,-18.914476249739,124.514296469915)) ;
#73548=CARTESIAN_POINT('Ctrl Pts',(-20.2516876995476,-19.1045258848039,
124.661945764437)) ;
#73549=CARTESIAN_POINT('Ctrl Pts',(-20.0832104950723,-18.9245368043851,
124.41191423788)) ;
#73550=CARTESIAN_POINT('Ctrl Pts',(-20.4530733453764,-19.1143751491768,
124.49932172969)) ;
#73551=CARTESIAN_POINT('Ctrl Pts',(-20.2443173510078,-18.934386068758,124.281814281811)) ;
#73552=CARTESIAN_POINT('Ctrl Pts',(-20.6267212720939,-19.1244024016246,
124.301134264947)) ;
#73553=CARTESIAN_POINT('Ctrl Pts',(-20.3832345959501,-18.9444133212059,
124.123263308682)) ;
#73554=CARTESIAN_POINT('Ctrl Pts',(-20.7627508778344,-19.1344306991948,
124.075408616425)) ;
#73555=CARTESIAN_POINT('Ctrl Pts',(-20.4920569238612,-18.954441618776,123.942681905956)) ;
#73556=CARTESIAN_POINT('Ctrl Pts',(-20.8562554222548,-19.1442768282008,
123.834159661691)) ;
#73557=CARTESIAN_POINT('Ctrl Pts',(-20.5668588165386,-18.964287747782,123.749683032266)) ;
#73558=CARTESIAN_POINT('Ctrl Pts',(-20.9078510941578,-19.1542707335628,
123.576649296548)) ;
#73559=CARTESIAN_POINT('Ctrl Pts',(-20.6081339643689,-18.9742816531441,
123.543674604084)) ;
#73560=CARTESIAN_POINT('Ctrl Pts',(-20.9134974108288,-19.1642948312459,
123.313280162655)) ;
#73561=CARTESIAN_POINT('Ctrl Pts',(-20.6126495326501,-18.9843057508271,
123.332979224958)) ;
#73562=CARTESIAN_POINT('Ctrl Pts',(-20.8741896283394,-19.1741846590999,
123.056370784483)) ;
#73563=CARTESIAN_POINT('Ctrl Pts',(-20.5812020083466,-18.9941955786812,
123.127452614158)) ;
#73564=CARTESIAN_POINT('Ctrl Pts',(-20.7903778747914,-19.1841766405303,
122.807538053467)) ;
#73565=CARTESIAN_POINT('Ctrl Pts',(-20.5141513809669,-19.0041875601116,
122.928386999942)) ;
#73566=CARTESIAN_POINT('Ctrl Pts',(-20.665139925764,-19.1941236452962,122.578095153236)) ;
#73567=CARTESIAN_POINT('Ctrl Pts',(-20.41396002509,-19.0141345648774,122.744833684279)) ;
#73568=CARTESIAN_POINT('Ctrl Pts',(-20.5022911488211,-19.204073296686,122.373520731225)) ;
#73569=CARTESIAN_POINT('Ctrl Pts',(-20.2836802639546,-19.0240842162672,
122.581175227014)) ;
#73570=CARTESIAN_POINT('Ctrl Pts',(-20.304546822287,-19.2141102996634,122.19898292141)) ;
#73571=CARTESIAN_POINT('Ctrl Pts',(-20.125483863784,-19.0341212192446,122.441545883708)) ;
#73572=CARTESIAN_POINT('Ctrl Pts',(-20.0829020054006,-19.2239992080984,
122.063295386289)) ;
#73573=CARTESIAN_POINT('Ctrl Pts',(-19.9481679801292,-19.0440101276797,
122.332997314253)) ;
#73574=CARTESIAN_POINT('Ctrl Pts',(-19.838797485772,-19.2339885405759,121.966751761761)) ;
#73575=CARTESIAN_POINT('Ctrl Pts',(-19.7528840990243,-19.0539994601571,
122.255763553244)) ;
#73576=CARTESIAN_POINT('Ctrl Pts',(-19.5823918613862,-19.243947096013,121.914413714457)) ;
#73577=CARTESIAN_POINT('Ctrl Pts',(-19.547759698978,-19.0639580155942,122.213894361448)) ;
#73578=CARTESIAN_POINT('Ctrl Pts',(-19.3223367513851,-19.2538466672135,
121.906790613273)) ;
#73579=CARTESIAN_POINT('Ctrl Pts',(-19.3397162836837,-19.0738575867947,
122.20779695611)) ;
#73580=CARTESIAN_POINT('Ctrl Pts',(-19.0611077173771,-19.2638945924655,
121.945087876707)) ;
#73581=CARTESIAN_POINT('Ctrl Pts',(-19.1307330399337,-19.0839055120467,
122.23843585839)) ;
#73582=CARTESIAN_POINT('Ctrl Pts',(-18.814173133089,-19.2737898919915,122.026726024973)) ;
#73583=CARTESIAN_POINT('Ctrl Pts',(-18.9331863897438,-19.0938008115727,
122.303747125533)) ;
#73584=CARTESIAN_POINT('Ctrl Pts',(-18.5813585769852,-19.2838517484394,
122.152010675361)) ;
#73585=CARTESIAN_POINT('Ctrl Pts',(-18.7469349998699,-19.1038626680207,
122.403975871039)) ;
#73586=CARTESIAN_POINT('Ctrl Pts',(-18.3782635158702,-19.2936955948561,
122.312252866395)) ;
#73587=CARTESIAN_POINT('Ctrl Pts',(-18.5844604094953,-19.1137065144373,
122.53216976341)) ;
#73588=CARTESIAN_POINT('Ctrl Pts',(-18.2033377996741,-19.3036585439841,
122.507039819568)) ;
#73589=CARTESIAN_POINT('Ctrl Pts',(-18.4445206716217,-19.1236694635654,
122.687999590902)) ;
#73590=CARTESIAN_POINT('Ctrl Pts',(-18.0642605165133,-19.3136925804121,
122.731072713043)) ;
#73591=CARTESIAN_POINT('Ctrl Pts',(-18.3332595529383,-19.1337034999934,
122.867226472839)) ;
#73592=CARTESIAN_POINT('Ctrl Pts',(-17.9673787965976,-19.3235800073702,
122.972163161429)) ;
#73593=CARTESIAN_POINT('Ctrl Pts',(-18.2557552582931,-19.1435909269514,
123.060098390728)) ;
#73594=CARTESIAN_POINT('Ctrl Pts',(-17.9126484520126,-19.3335944417065,
123.229596243484)) ;
#73595=CARTESIAN_POINT('Ctrl Pts',(-18.2119716852264,-19.1536053612878,
123.266044996015)) ;
#73596=CARTESIAN_POINT('Ctrl Pts',(-17.9040917215466,-19.3436293863415,
123.493147352363)) ;
#73597=CARTESIAN_POINT('Ctrl Pts',(-18.2051271768608,-19.1636403059227,
123.476886022838)) ;
#73598=CARTESIAN_POINT('Ctrl Pts',(-17.9399787130292,-19.3534617363725,
123.749059430695)) ;
#73599=CARTESIAN_POINT('Ctrl Pts',(-18.2338373040545,-19.1734726559537,
123.681614412356)) ;
#73600=CARTESIAN_POINT('Ctrl Pts',(-18.0216292179886,-19.3635371754897,
124.00087385618)) ;
#73601=CARTESIAN_POINT('Ctrl Pts',(-18.2991584729874,-19.183548095071,123.883066086777)) ;
#73602=CARTESIAN_POINT('Ctrl Pts',(-18.1429328956013,-19.3733896407243,
124.229675102656)) ;
#73603=CARTESIAN_POINT('Ctrl Pts',(-18.396201496122,-19.1934005603056,124.066105849519)) ;
#73604=CARTESIAN_POINT('Ctrl Pts',(-18.3054527183703,-19.3834625183012,
124.43855780688)) ;
#73605=CARTESIAN_POINT('Ctrl Pts',(-18.5262180422587,-19.2034734378824,
124.23321192103)) ;
#73606=CARTESIAN_POINT('Ctrl Pts',(-18.4973580639054,-19.3933051144937,
124.612009431565)) ;
#73607=CARTESIAN_POINT('Ctrl Pts',(-18.6797418858111,-19.2133160340749,
124.371972008953)) ;
#73608=CARTESIAN_POINT('Ctrl Pts',(-18.7190343990378,-19.403285498609,124.752157350423)) ;
#73609=CARTESIAN_POINT('Ctrl Pts',(-18.8570829522641,-19.2232964181902,
124.4840898822)) ;
#73610=CARTESIAN_POINT('Ctrl Pts',(-18.9628028394589,-19.4133039792578,
124.851593566048)) ;
#73611=CARTESIAN_POINT('Ctrl Pts',(-19.0520979082859,-19.233314898839,124.56363837805)) ;
#73612=CARTESIAN_POINT('Ctrl Pts',(-19.2165815610818,-19.4231872942581,
124.906993129044)) ;
#73613=CARTESIAN_POINT('Ctrl Pts',(-19.2551201081469,-19.2431982138394,
124.607957472016)) ;
#73614=CARTESIAN_POINT('Ctrl Pts',(-19.4809103809745,-19.4332555913486,
124.917562972761)) ;
#73615=CARTESIAN_POINT('Ctrl Pts',(-19.4665835088432,-19.2532665109298,
124.616412951815)) ;
#73616=CARTESIAN_POINT('Ctrl Pts',(-19.736986666509,-19.4430856597209,124.883208337383)) ;
#73617=CARTESIAN_POINT('Ctrl Pts',(-19.6714432710506,-19.2630965793021,
124.588929081079)) ;
#73618=CARTESIAN_POINT('Ctrl Pts',(-19.9891462344599,-19.4531524521893,
124.803370269059)) ;
#73619=CARTESIAN_POINT('Ctrl Pts',(-19.8731711567886,-19.2731633717705,
124.525058292213)) ;
#73620=CARTESIAN_POINT('Ctrl Pts',(-20.2195097660889,-19.4630417856778,
124.682973671284)) ;
#73621=CARTESIAN_POINT('Ctrl Pts',(-20.0574610978455,-19.2830527052591,
124.428741164273)) ;
#73622=CARTESIAN_POINT('Ctrl Pts',(-20.4279957456454,-19.4730439170939,
124.522983695166)) ;
#73623=CARTESIAN_POINT('Ctrl Pts',(-20.2242496883146,-19.2930548366751,
124.300749114728)) ;
#73624=CARTESIAN_POINT('Ctrl Pts',(-20.6043330328565,-19.4829677867149,
124.330784900603)) ;
#73625=CARTESIAN_POINT('Ctrl Pts',(-20.3653190116598,-19.3029787062961,
124.146990434962)) ;
#73626=CARTESIAN_POINT('Ctrl Pts',(-20.7461987471793,-19.4930113022321,
124.108267757286)) ;
#73627=CARTESIAN_POINT('Ctrl Pts',(-20.4788115505222,-19.3130222218133,
123.968976491356)) ;
#73628=CARTESIAN_POINT('Ctrl Pts',(-20.8459623354037,-19.5028935151204,
123.868447779217)) ;
#73629=CARTESIAN_POINT('Ctrl Pts',(-20.5586220080263,-19.3229044347016,
123.77712130273)) ;
#73630=CARTESIAN_POINT('Ctrl Pts',(-20.9036081810683,-19.5129615923398,
123.610275746696)) ;
#73631=CARTESIAN_POINT('Ctrl Pts',(-20.6047386771519,-19.332972511921,123.570583349477)) ;
#73632=CARTESIAN_POINT('Ctrl Pts',(-20.915515712549,-19.522800097074,123.351961006774)) ;
#73633=CARTESIAN_POINT('Ctrl Pts',(-20.6142646315837,-19.3428110166552,
123.363932740499)) ;
#73634=CARTESIAN_POINT('Ctrl Pts',(-20.8820171906125,-19.5328628655034,
123.089685129355)) ;
#73635=CARTESIAN_POINT('Ctrl Pts',(-20.5874658526555,-19.3528737850846,
123.154111733586)) ;
#73636=CARTESIAN_POINT('Ctrl Pts',(-20.8044967774728,-19.5427598587861,
122.841407511861)) ;
#73637=CARTESIAN_POINT('Ctrl Pts',(-20.5254497644867,-19.3627707783674,
122.955490404283)) ;
#73638=CARTESIAN_POINT('Ctrl Pts',(-20.6854165301344,-19.5526910864209,
122.60918260394)) ;
#73639=CARTESIAN_POINT('Ctrl Pts',(-20.4301860313907,-19.3727020060021,
122.769710887484)) ;
#73640=CARTESIAN_POINT('Ctrl Pts',(-20.5258305092585,-19.562733245063,122.39901017829)) ;
#73641=CARTESIAN_POINT('Ctrl Pts',(-20.3025172352716,-19.3827441646443,
122.601572722186)) ;
#73642=CARTESIAN_POINT('Ctrl Pts',(-20.3352897321576,-19.5726199545941,
122.222366967622)) ;
#73643=CARTESIAN_POINT('Ctrl Pts',(-20.1500853867411,-19.3926308741753,
122.460258598056)) ;
#73644=CARTESIAN_POINT('Ctrl Pts',(-20.1148863727612,-19.5826129270227,
122.079617245424)) ;
#73645=CARTESIAN_POINT('Ctrl Pts',(-19.9737630061899,-19.4026238466039,
122.346058647369)) ;
#73646=CARTESIAN_POINT('Ctrl Pts',(-19.874126422685,-19.5925591215593,121.977883229097)) ;
#73647=CARTESIAN_POINT('Ctrl Pts',(-19.7811555923769,-19.4125700411405,
122.264671358312)) ;
#73648=CARTESIAN_POINT('Ctrl Pts',(-19.6194821905601,-19.6025044964108,
121.91893843079)) ;
#73649=CARTESIAN_POINT('Ctrl Pts',(-19.5774407611386,-19.422515415992,122.217515208665)) ;
#73650=CARTESIAN_POINT('Ctrl Pts',(-19.3556280435148,-19.6125594157707,
121.905362356755)) ;
#73651=CARTESIAN_POINT('Ctrl Pts',(-19.3663572165396,-19.4325703353519,
122.206654013868)) ;
#73652=CARTESIAN_POINT('Ctrl Pts',(-19.0993869104876,-19.6223809352142,
121.936569596332)) ;
#73653=CARTESIAN_POINT('Ctrl Pts',(-19.1613655396477,-19.4423918547954,
122.231619200685)) ;
#73654=CARTESIAN_POINT('Ctrl Pts',(-18.8463008166407,-19.6324467039811,
122.01333370423)) ;
#73655=CARTESIAN_POINT('Ctrl Pts',(-18.9588962140942,-19.4524576235623,
122.29303006788)) ;
#73656=CARTESIAN_POINT('Ctrl Pts',(-18.614184741333,-19.6423486256361,122.131051371053)) ;
#73657=CARTESIAN_POINT('Ctrl Pts',(-18.7732037818426,-19.4623595452174,
122.387203418498)) ;
#73658=CARTESIAN_POINT('Ctrl Pts',(-18.4029852172984,-19.6523916844572,
122.289280682559)) ;
#73659=CARTESIAN_POINT('Ctrl Pts',(-18.604243687009,-19.4724026040384,122.513786518166)) ;
#73660=CARTESIAN_POINT('Ctrl Pts',(-18.2250106931332,-19.6622976784999,
122.479267826247)) ;
#73661=CARTESIAN_POINT('Ctrl Pts',(-18.4618641781161,-19.4823085980811,
122.665775345268)) ;
#73662=CARTESIAN_POINT('Ctrl Pts',(-18.0816334127858,-19.6722354515817,
122.697543077619)) ;
#73663=CARTESIAN_POINT('Ctrl Pts',(-18.3471620419146,-19.4922463711629,
122.840394715573)) ;
#73664=CARTESIAN_POINT('Ctrl Pts',(-17.9775290975299,-19.682275815314,122.939982086289)) ;
#73665=CARTESIAN_POINT('Ctrl Pts',(-18.2638779349782,-19.5022867348952,
123.034345802999)) ;
#73666=CARTESIAN_POINT('Ctrl Pts',(-17.9178270663796,-19.6921631590375,
123.192873036783)) ;
#73667=CARTESIAN_POINT('Ctrl Pts',(-18.2161158243129,-19.5121740786187,
123.236657594822)) ;
#73668=CARTESIAN_POINT('Ctrl Pts',(-17.9023535730021,-19.7021553896062,
123.454984271161)) ;
#73669=CARTESIAN_POINT('Ctrl Pts',(-18.2037362398585,-19.5221663091874,
123.446346372631)) ;
#73670=CARTESIAN_POINT('Ctrl Pts',(-17.9325684279104,-19.7121039173898,
123.714684335716)) ;
#73671=CARTESIAN_POINT('Ctrl Pts',(-18.2279072969856,-19.532114836971,123.654106084101)) ;
#73672=CARTESIAN_POINT('Ctrl Pts',(-18.0069653212784,-19.7220407011131,
123.964967568123)) ;
#73673=CARTESIAN_POINT('Ctrl Pts',(-18.2874238319089,-19.5420516206943,
123.854332429313)) ;
#73674=CARTESIAN_POINT('Ctrl Pts',(-18.1239596003207,-19.73202370191,124.199815869737)) ;
#73675=CARTESIAN_POINT('Ctrl Pts',(-18.3810183152476,-19.5520346214913,
124.042211309555)) ;
#73676=CARTESIAN_POINT('Ctrl Pts',(-18.2812582376319,-19.7420675887508,
124.411727571311)) ;
#73677=CARTESIAN_POINT('Ctrl Pts',(-18.5068566460487,-19.562078508332,124.21174128928)) ;
#73678=CARTESIAN_POINT('Ctrl Pts',(-18.4684715102888,-19.7518956123253,
124.58970605599)) ;
#73679=CARTESIAN_POINT('Ctrl Pts',(-18.6566257534126,-19.5719065319066,
124.3541239909)) ;
#73680=CARTESIAN_POINT('Ctrl Pts',(-18.689056614064,-19.761972860539,124.736130030158)) ;
#73681=CARTESIAN_POINT('Ctrl Pts',(-18.8330935698082,-19.5819837801202,
124.471264200358)) ;
#73682=CARTESIAN_POINT('Ctrl Pts',(-18.9262775518946,-19.7718224158442,
124.839850242378)) ;
#73683=CARTESIAN_POINT('Ctrl Pts',(-19.0228689899652,-19.5918333354255,
124.554240926399)) ;
#73684=CARTESIAN_POINT('Ctrl Pts',(-19.1837052991542,-19.781905124042,124.902304787764)) ;
#73685=CARTESIAN_POINT('Ctrl Pts',(-19.2288112851542,-19.6019160436232,
124.604205685487)) ;
#73686=CARTESIAN_POINT('Ctrl Pts',(-19.4410933758814,-19.7917177169684,
124.918904855349)) ;
#73687=CARTESIAN_POINT('Ctrl Pts',(-19.434720478767,-19.6117286365497,124.61748677879)) ;
#73688=CARTESIAN_POINT('Ctrl Pts',(-19.7040333399978,-19.8017849092264,
124.890266579445)) ;
#73689=CARTESIAN_POINT('Ctrl Pts',(-19.6450728626718,-19.6217958288076,
124.594577333264)) ;
#73690=CARTESIAN_POINT('Ctrl Pts',(-19.953852926939,-19.811683738689,124.817515981113)) ;
#73691=CARTESIAN_POINT('Ctrl Pts',(-19.8449282229179,-19.6316946582702,
124.536378184494)) ;
#73692=CARTESIAN_POINT('Ctrl Pts',(-20.1908446169336,-19.8217377298791,
124.700847328408)) ;
#73693=CARTESIAN_POINT('Ctrl Pts',(-20.0345222842642,-19.6417486494604,
124.443044266715)) ;
#73694=CARTESIAN_POINT('Ctrl Pts',(-20.4003396793583,-19.8316094546624,
124.547752149645)) ;
#73695=CARTESIAN_POINT('Ctrl Pts',(-20.2021184087781,-19.6516203742436,
124.32056963313)) ;
#73696=CARTESIAN_POINT('Ctrl Pts',(-20.5836646743315,-19.8416798967926,
124.356956666515)) ;
#73697=CARTESIAN_POINT('Ctrl Pts',(-20.3487795243232,-19.6616908163738,
124.167933928758)) ;
#73698=CARTESIAN_POINT('Ctrl Pts',(-20.7277380469085,-19.8515129752229,
124.142415105661)) ;
#73699=CARTESIAN_POINT('Ctrl Pts',(-20.4640387321514,-19.6715238948041,
123.996302256258)) ;
#73700=CARTESIAN_POINT('Ctrl Pts',(-20.8351448172692,-19.8615434487242,
123.901710971188)) ;
#73701=CARTESIAN_POINT('Ctrl Pts',(-20.5499655097051,-19.6815543683055,
123.803739479692)) ;
#73702=CARTESIAN_POINT('Ctrl Pts',(-20.8983935515043,-19.8715750480229,
123.645775745963)) ;
#73703=CARTESIAN_POINT('Ctrl Pts',(-20.6005657740463,-19.6915859676042,
123.598991547224)) ;
#73704=CARTESIAN_POINT('Ctrl Pts',(-20.9164189115972,-19.8814047490611,
123.388108112837)) ;
#73705=CARTESIAN_POINT('Ctrl Pts',(-20.6149874004344,-19.7014156686424,
123.392858551262)) ;
#73706=CARTESIAN_POINT('Ctrl Pts',(-20.8897697071989,-19.8913941871176,
123.126944309957)) ;
#73707=CARTESIAN_POINT('Ctrl Pts',(-20.5936696114577,-19.7114051066988,
123.183927490661)) ;
#73708=CARTESIAN_POINT('Ctrl Pts',(-20.8171461451354,-19.9014380903337,
122.873192498231)) ;
#73709=CARTESIAN_POINT('Ctrl Pts',(-20.5355721095239,-19.7214490099149,
122.980925533021)) ;
#73710=CARTESIAN_POINT('Ctrl Pts',(-20.7046073618449,-19.9112596111472,
122.640918152615)) ;
#73711=CARTESIAN_POINT('Ctrl Pts',(-20.4455429052235,-19.7312705307284,
122.795106281435)) ;
#73712=CARTESIAN_POINT('Ctrl Pts',(-20.5506673334874,-19.9212953353943,
122.426787436371)) ;
#73713=CARTESIAN_POINT('Ctrl Pts',(-20.3223921809841,-19.7413062549755,
122.623800668938)) ;
#73714=CARTESIAN_POINT('Ctrl Pts',(-20.361646906176,-19.9313174893268,122.243358309502)) ;
#73715=CARTESIAN_POINT('Ctrl Pts',(-20.1711768967696,-19.751328408908,122.477056260967)) ;
#73716=CARTESIAN_POINT('Ctrl Pts',(-20.147396817326,-19.9411797210841,122.097565987391)) ;
#73717=CARTESIAN_POINT('Ctrl Pts',(-19.9997783728668,-19.7611906406653,
122.360421503876)) ;
#73718=CARTESIAN_POINT('Ctrl Pts',(-19.9090443946138,-19.951138791542,121.989462309711)) ;
#73719=CARTESIAN_POINT('Ctrl Pts',(-19.8090974023785,-19.7711497111232,
122.273937084454)) ;
#73720=CARTESIAN_POINT('Ctrl Pts',(-19.6535218175542,-19.9611739639181,
121.924289992002)) ;
#73721=CARTESIAN_POINT('Ctrl Pts',(-19.6046796893941,-19.7811848834994,
122.221797596013)) ;
#73722=CARTESIAN_POINT('Ctrl Pts',(-19.3946113132466,-19.9710543490764,
121.904388967415)) ;
#73723=CARTESIAN_POINT('Ctrl Pts',(-19.397552035366,-19.7910652686577,122.205875089908)) ;
#73724=CARTESIAN_POINT('Ctrl Pts',(-19.1316102592224,-19.9811110636703,
121.930090607189)) ;
#73725=CARTESIAN_POINT('Ctrl Pts',(-19.1871508676461,-19.8011219832516,
122.226434670213)) ;
#73726=CARTESIAN_POINT('Ctrl Pts',(-18.8815248170263,-19.9909903322424,
121.999843995955)) ;
#73727=CARTESIAN_POINT('Ctrl Pts',(-18.9870826419165,-19.8110012518237,
122.282235527794)) ;
#73728=CARTESIAN_POINT('Ctrl Pts',(-18.6444106248793,-20.0009812897281,
122.112585153764)) ;
#73729=CARTESIAN_POINT('Ctrl Pts',(-18.7973905924176,-19.8209922093093,
122.372426718099)) ;
#73730=CARTESIAN_POINT('Ctrl Pts',(-18.4297462675424,-20.0110219483633,
122.266017180275)) ;
#73731=CARTESIAN_POINT('Ctrl Pts',(-18.6256580184065,-19.8310328679445,
122.495170938252)) ;
#73732=CARTESIAN_POINT('Ctrl Pts',(-18.2485010034017,-20.0208549280713,
122.450186849487)) ;
#73733=CARTESIAN_POINT('Ctrl Pts',(-18.4806610287741,-19.8408658476525,
122.642504838089)) ;
#73734=CARTESIAN_POINT('Ctrl Pts',(-18.0989811417454,-20.030848061321,122.6660694596)) ;
#73735=CARTESIAN_POINT('Ctrl Pts',(-18.361043590352,-19.8508589809022,122.815209731099)) ;
#73736=CARTESIAN_POINT('Ctrl Pts',(-17.9892812123843,-20.0408801137044,
122.905806909228)) ;
#73737=CARTESIAN_POINT('Ctrl Pts',(-18.2732819325311,-19.8608910332856,
123.006998938251)) ;
#73738=CARTESIAN_POINT('Ctrl Pts',(-17.9236747634942,-20.0507453426556,
123.156602970164)) ;
#73739=CARTESIAN_POINT('Ctrl Pts',(-18.2207950630936,-19.8707562622369,
123.207634737405)) ;
#73740=CARTESIAN_POINT('Ctrl Pts',(-17.901665291667,-20.0607072838989,123.417472522822)) ;
#73741=CARTESIAN_POINT('Ctrl Pts',(-18.2031854905323,-19.8807182034801,
123.416330009112)) ;
#73742=CARTESIAN_POINT('Ctrl Pts',(-17.9258798987478,-20.0707419989356,
123.680047914993)) ;
#73743=CARTESIAN_POINT('Ctrl Pts',(-18.2225552242478,-19.8907529185169,
123.626390529728)) ;
#73744=CARTESIAN_POINT('Ctrl Pts',(-17.9938945220798,-20.0806277692797,
123.930807070513)) ;
#73745=CARTESIAN_POINT('Ctrl Pts',(-18.2769648599555,-19.9006386888609,
123.82699794779)) ;
#73746=CARTESIAN_POINT('Ctrl Pts',(-18.1063688770827,-20.0906903666684,
124.170094182597)) ;
#73747=CARTESIAN_POINT('Ctrl Pts',(-18.3669425672961,-19.9107012862497,
124.018428597259)) ;
#73748=CARTESIAN_POINT('Ctrl Pts',(-18.2554062654067,-20.1005407785037,
124.381769206432)) ;
#73749=CARTESIAN_POINT('Ctrl Pts',(-18.4861705070814,-19.9205516980849,
124.187769342642)) ;
#73750=CARTESIAN_POINT('Ctrl Pts',(-18.4417280628566,-20.1105679477896,
124.568087270984)) ;
#73751=CARTESIAN_POINT('Ctrl Pts',(-18.635226462847,-19.9305788673709,124.336825291195)) ;
#73752=CARTESIAN_POINT('Ctrl Pts',(-18.6579883240509,-20.1205954285038,
124.718674943171)) ;
#73753=CARTESIAN_POINT('Ctrl Pts',(-18.808233509183,-19.940606348085,124.457297090605)) ;
#73754=CARTESIAN_POINT('Ctrl Pts',(-18.8924830332927,-20.1304384810831,
124.827831022271)) ;
#73755=CARTESIAN_POINT('Ctrl Pts',(-18.9958279396515,-19.9504494006643,
124.544623631068)) ;
#73756=CARTESIAN_POINT('Ctrl Pts',(-19.1460332396002,-20.1404323845217,
124.89628582595)) ;
#73757=CARTESIAN_POINT('Ctrl Pts',(-19.1986674699778,-19.9604433041029,
124.599389529279)) ;
#73758=CARTESIAN_POINT('Ctrl Pts',(-19.408537282864,-20.1504595072981,124.919271899811)) ;
#73759=CARTESIAN_POINT('Ctrl Pts',(-19.408670501884,-19.9704704268793,124.617780480819)) ;
#73760=CARTESIAN_POINT('Ctrl Pts',(-19.6674999586664,-20.1603502121901,
124.896966576187)) ;
#73761=CARTESIAN_POINT('Ctrl Pts',(-19.6158404984156,-19.9803611317714,
124.599938376062)) ;
#73762=CARTESIAN_POINT('Ctrl Pts',(-19.9213144643945,-20.1703422390405,
124.829720703275)) ;
#73763=CARTESIAN_POINT('Ctrl Pts',(-19.8188925751091,-19.9903531586217,
124.546143793371)) ;
#73764=CARTESIAN_POINT('Ctrl Pts',(-20.1584732283506,-20.180288220529,124.719860821127)) ;
#73765=CARTESIAN_POINT('Ctrl Pts',(-20.0086203263769,-20.0002991401102,
124.458257924358)) ;
#73766=CARTESIAN_POINT('Ctrl Pts',(-20.3732942471525,-20.1902353931509,
124.57089728247)) ;
#73767=CARTESIAN_POINT('Ctrl Pts',(-20.1804782620418,-20.0102463127322,
124.339088990223)) ;
#73768=CARTESIAN_POINT('Ctrl Pts',(-20.56064383046,-20.2002833344771,124.384839709402)) ;
#73769=CARTESIAN_POINT('Ctrl Pts',(-20.3303594683394,-20.0202942540583,
124.19024447105)) ;
#73770=CARTESIAN_POINT('Ctrl Pts',(-20.7099931678072,-20.2101309682848,
124.173496321027)) ;
#73771=CARTESIAN_POINT('Ctrl Pts',(-20.4498405454841,-20.0301418878661,
124.021171285439)) ;
#73772=CARTESIAN_POINT('Ctrl Pts',(-20.8223918371463,-20.2200926829699,
123.937083946807)) ;
#73773=CARTESIAN_POINT('Ctrl Pts',(-20.5397614600564,-20.0401036025511,
123.832042436741)) ;
#73774=CARTESIAN_POINT('Ctrl Pts',(-20.8921871413326,-20.2301213158484,
123.682935524395)) ;
#73775=CARTESIAN_POINT('Ctrl Pts',(-20.5955998340411,-20.0501322354297,
123.628724320913)) ;
#73776=CARTESIAN_POINT('Ctrl Pts',(-20.916586665412,-20.2400316413835,123.423658765385)) ;
#73777=CARTESIAN_POINT('Ctrl Pts',(-20.6151216495105,-20.0600425609648,
123.421303286286)) ;
#73778=CARTESIAN_POINT('Ctrl Pts',(-20.8962205047592,-20.2499664718553,
123.163371888253)) ;
#73779=CARTESIAN_POINT('Ctrl Pts',(-20.5988309868347,-20.0699773914365,
123.213073725564)) ;
#73780=CARTESIAN_POINT('Ctrl Pts',(-20.8300540057816,-20.2600078042372,
122.907927043683)) ;
#73781=CARTESIAN_POINT('Ctrl Pts',(-20.545899908751,-20.0800187238185,123.008717280529)) ;
#73782=CARTESIAN_POINT('Ctrl Pts',(-20.72224421422,-20.2699006776761,122.671362855086)) ;
#73783=CARTESIAN_POINT('Ctrl Pts',(-20.4596543888742,-20.0899115972573,
122.819465277106)) ;
#73784=CARTESIAN_POINT('Ctrl Pts',(-20.5744033926093,-20.279869843494,122.455071839391)) ;
#73785=CARTESIAN_POINT('Ctrl Pts',(-20.3413828139098,-20.0998807630752,
122.646430631496)) ;
#73786=CARTESIAN_POINT('Ctrl Pts',(-20.3898674157818,-20.2898985772105,
122.266945763592)) ;
#73787=CARTESIAN_POINT('Ctrl Pts',(-20.1937587117748,-20.1099094967917,
122.495930505573)) ;
#73788=CARTESIAN_POINT('Ctrl Pts',(-20.1081899355574,-20.3030910959816,
122.064717611269)) ;
#73789=CARTESIAN_POINT('Ctrl Pts',(-19.9684034754264,-20.1231020155629,
122.334134312511)) ;
#73790=CARTESIAN_POINT('Ctrl Pts',(-19.7762004294478,-20.3164509640243,
121.939098029962)) ;
#73791=CARTESIAN_POINT('Ctrl Pts',(-19.70278986189,-20.1364618836056,122.233638111856)) ;
#73792=CARTESIAN_POINT('Ctrl Pts',(-19.4302944299189,-20.3296763011732,
121.904585070765)) ;
#73793=CARTESIAN_POINT('Ctrl Pts',(-19.4261079855339,-20.1496872207544,
122.206033326473)) ;
#73794=CARTESIAN_POINT('Ctrl Pts',(-19.16869005573,-20.3396575270138,121.923502397356)) ;
#73795=CARTESIAN_POINT('Ctrl Pts',(-19.2168157977084,-20.1596684465951,
122.221163228254)) ;
#73796=CARTESIAN_POINT('Ctrl Pts',(-18.9130849261676,-20.3496930939967,
121.988403504239)) ;
#73797=CARTESIAN_POINT('Ctrl Pts',(-19.0123335164269,-20.1697040135779,
122.273082369404)) ;
#73798=CARTESIAN_POINT('Ctrl Pts',(-18.676515944024,-20.3595561719588,122.094373600207)) ;
#73799=CARTESIAN_POINT('Ctrl Pts',(-18.8230767411481,-20.17956709154,122.357856308508)) ;
#73800=CARTESIAN_POINT('Ctrl Pts',(-18.4574468061026,-20.3696264707599,
122.242786566427)) ;
#73801=CARTESIAN_POINT('Ctrl Pts',(-18.6478204417451,-20.1896373903411,
122.476584793139)) ;
#73802=CARTESIAN_POINT('Ctrl Pts',(-18.2717579004932,-20.3794687693277,
122.422851075658)) ;
#73803=CARTESIAN_POINT('Ctrl Pts',(-18.4992676185254,-20.1994796889089,
122.620634878705)) ;
#73804=CARTESIAN_POINT('Ctrl Pts',(-18.117558664648,-20.3894294674975,122.634360678024)) ;
#73805=CARTESIAN_POINT('Ctrl Pts',(-18.3759064506187,-20.2094403870787,
122.78984130679)) ;
#73806=CARTESIAN_POINT('Ctrl Pts',(-18.0020059071283,-20.3994675016769,
122.871483585748)) ;
#73807=CARTESIAN_POINT('Ctrl Pts',(-18.2834623026179,-20.2194784212582,
122.97953855026)) ;
#73808=CARTESIAN_POINT('Ctrl Pts',(-17.9300887192863,-20.4093412385234,
123.120824683892)) ;
#73809=CARTESIAN_POINT('Ctrl Pts',(-18.2259264014613,-20.2293521581047,
123.179011012652)) ;
#73810=CARTESIAN_POINT('Ctrl Pts',(-17.9020448473122,-20.4194130224487,
123.383973224124)) ;
#73811=CARTESIAN_POINT('Ctrl Pts',(-18.2034891482727,-20.2394239420299,
123.389529423009)) ;
#73812=CARTESIAN_POINT('Ctrl Pts',(-17.9195350318856,-20.4292451436499,
123.641783391203)) ;
#73813=CARTESIAN_POINT('Ctrl Pts',(-18.2174791482912,-20.2492560632311,
123.595778035105)) ;
#73814=CARTESIAN_POINT('Ctrl Pts',(-17.9820931575839,-20.4392781676753,
123.897898640815)) ;
#73815=CARTESIAN_POINT('Ctrl Pts',(-18.2675235858112,-20.2592890872566,
123.8006706467)) ;
#73816=CARTESIAN_POINT('Ctrl Pts',(-18.0886185613689,-20.449294047872,124.138604141892)) ;
#73817=CARTESIAN_POINT('Ctrl Pts',(-18.3527418295689,-20.2693049674532,
123.993235758513)) ;
#73818=CARTESIAN_POINT('Ctrl Pts',(-18.2329706507944,-20.4591775669661,
124.354523331937)) ;
#73819=CARTESIAN_POINT('Ctrl Pts',(-18.4682220840992,-20.2791884865474,
124.165972815499)) ;
#73820=CARTESIAN_POINT('Ctrl Pts',(-18.4143074090764,-20.4691679793298,
124.54434899159)) ;
#73821=CARTESIAN_POINT('Ctrl Pts',(-18.6132892508366,-20.2891788989111,
124.31783370646)) ;
#73822=CARTESIAN_POINT('Ctrl Pts',(-18.6951170309622,-20.4824311425333,
124.750853866848)) ;
#73823=CARTESIAN_POINT('Ctrl Pts',(-18.8379390825619,-20.3024420621145,
124.483045334698)) ;
#73824=CARTESIAN_POINT('Ctrl Pts',(-19.0235816254363,-20.4957087127844,
124.879780338538)) ;
#73825=CARTESIAN_POINT('Ctrl Pts',(-19.1007466138958,-20.3157196323657,
124.586193622694)) ;
#73826=CARTESIAN_POINT('Ctrl Pts',(-19.3717460245755,-20.5090390152911,
124.918788838363)) ;
#73827=CARTESIAN_POINT('Ctrl Pts',(-19.3792305302181,-20.3290499348723,
124.617392368579)) ;
#73828=CARTESIAN_POINT('Ctrl Pts',(-19.6313783521578,-20.5189376971075,
124.902811153658)) ;
#73829=CARTESIAN_POINT('Ctrl Pts',(-19.586946416879,-20.3389486166887,124.604614298726)) ;
#73830=CARTESIAN_POINT('Ctrl Pts',(-19.8866819313856,-20.528927212155,124.841743662591)) ;
#73831=CARTESIAN_POINT('Ctrl Pts',(-19.7911870921237,-20.3489381317363,
124.555761778186)) ;
#73832=CARTESIAN_POINT('Ctrl Pts',(-20.126518376041,-20.53887526393,124.73768939616)) ;
#73833=CARTESIAN_POINT('Ctrl Pts',(-19.9830583085483,-20.3588861835113,
124.472519572636)) ;
#73834=CARTESIAN_POINT('Ctrl Pts',(-20.3446556457817,-20.5488166672085,
124.593959706051)) ;
#73835=CARTESIAN_POINT('Ctrl Pts',(-20.1575676024382,-20.3688275867898,
124.357539619825)) ;
#73836=CARTESIAN_POINT('Ctrl Pts',(-20.5987445476816,-20.5621033319895,
124.35442785802)) ;
#73837=CARTESIAN_POINT('Ctrl Pts',(-20.3608485152388,-20.3821142515707,
124.165903776339)) ;
#73838=CARTESIAN_POINT('Ctrl Pts',(-20.8307521720985,-20.5787137536443,
123.978870507215)) ;
#73839=CARTESIAN_POINT('Ctrl Pts',(-20.5464484061325,-20.3987246732255,
123.865472812429)) ;
#73840=CARTESIAN_POINT('Ctrl Pts',(-20.9389514261438,-20.5986250158951,
123.46082131634)) ;
#73841=CARTESIAN_POINT('Ctrl Pts',(-20.6330141894971,-20.4186359354763,
123.451029346131)) ;
#73842=CARTESIAN_POINT('Ctrl Pts',(-20.8639502682869,-20.6185691450599,
122.936042849581)) ;
#73843=CARTESIAN_POINT('Ctrl Pts',(-20.5730157436839,-20.4385800646412,
123.031206971255)) ;
#73844=CARTESIAN_POINT('Ctrl Pts',(-20.6146112119338,-20.6384923076651,
122.46895137449)) ;
#73845=CARTESIAN_POINT('Ctrl Pts',(-20.373547351219,-20.4585032272464,122.657531515704)) ;
#73846=CARTESIAN_POINT('Ctrl Pts',(-20.2219924331612,-20.6583824300717,
122.114827126847)) ;
#73847=CARTESIAN_POINT('Ctrl Pts',(-20.0594536357031,-20.4783933496529,
122.374229525961)) ;
#73848=CARTESIAN_POINT('Ctrl Pts',(-19.7292685932823,-20.6783873836718,
121.915230361475)) ;
#73849=CARTESIAN_POINT('Ctrl Pts',(-19.6652757291056,-20.498398303253,122.2145494258)) ;
#73850=CARTESIAN_POINT('Ctrl Pts',(-19.2022698837566,-20.6982256406874,
121.895490958109)) ;
#73851=CARTESIAN_POINT('Ctrl Pts',(-19.2436755852947,-20.5182365602686,
122.198755216504)) ;
#73852=CARTESIAN_POINT('Ctrl Pts',(-18.696210882358,-20.7182199414739,122.057473862863)) ;
#73853=CARTESIAN_POINT('Ctrl Pts',(-18.8388276085648,-20.5382308610552,
122.328339327978)) ;
#73854=CARTESIAN_POINT('Ctrl Pts',(-18.2783285951909,-20.7381051835183,
122.38107556081)) ;
#73855=CARTESIAN_POINT('Ctrl Pts',(-18.5045195347661,-20.5581161030996,
122.587219431288)) ;
#73856=CARTESIAN_POINT('Ctrl Pts',(-17.9948546692312,-20.7579801299943,
122.826813664097)) ;
#73857=CARTESIAN_POINT('Ctrl Pts',(-18.2777383070033,-20.5779910495756,
122.943810054151)) ;
#73858=CARTESIAN_POINT('Ctrl Pts',(-17.8799919147253,-20.7780131999354,
123.346775629794)) ;
#73859=CARTESIAN_POINT('Ctrl Pts',(-18.1858465680844,-20.5980241195166,
123.359778876185)) ;
#73860=CARTESIAN_POINT('Ctrl Pts',(-17.9496011377498,-20.7979017068358,
123.870729922715)) ;
#73861=CARTESIAN_POINT('Ctrl Pts',(-18.2415323136978,-20.617912626417,123.778943688252)) ;
#73862=CARTESIAN_POINT('Ctrl Pts',(-18.1918462218339,-20.8177565666171,
124.339642131858)) ;
#73863=CARTESIAN_POINT('Ctrl Pts',(-18.4353283966454,-20.6377674861983,
124.15407531908)) ;
#73864=CARTESIAN_POINT('Ctrl Pts',(-18.5838321067755,-20.8378074004048,
124.700496054213)) ;
#73865=CARTESIAN_POINT('Ctrl Pts',(-18.7489159490425,-20.657818319986,124.442758816039)) ;
#73866=CARTESIAN_POINT('Ctrl Pts',(-19.0684642768098,-20.857573342294,124.903648311974)) ;
#73867=CARTESIAN_POINT('Ctrl Pts',(-19.1366240867067,-20.6775842618753,
124.605282256728)) ;
#73868=CARTESIAN_POINT('Ctrl Pts',(-19.5995315082767,-20.8775860737534,
124.930591112263)) ;
#73869=CARTESIAN_POINT('Ctrl Pts',(-19.5614778234741,-20.6975969933346,
124.626836366824)) ;
#73870=CARTESIAN_POINT('Ctrl Pts',(-20.1049415619747,-20.8974789086969,
124.774856355386)) ;
#73871=CARTESIAN_POINT('Ctrl Pts',(-19.9658071300402,-20.7174898282782,
124.502248164714)) ;
#73872=CARTESIAN_POINT('Ctrl Pts',(-20.5274834956849,-20.9173859320365,
124.456638371379)) ;
#73873=CARTESIAN_POINT('Ctrl Pts',(-20.3038412440261,-20.7373968516177,
124.247672563111)) ;
#73874=CARTESIAN_POINT('Ctrl Pts',(-20.8168305785184,-20.9373011969372,
124.013259477113)) ;
#73875=CARTESIAN_POINT('Ctrl Pts',(-20.5353184953281,-20.7573121165184,
123.892968103574)) ;
#73876=CARTESIAN_POINT('Ctrl Pts',(-20.9375148305264,-20.9573328890969,
123.494752291653)) ;
#73877=CARTESIAN_POINT('Ctrl Pts',(-20.6318648818766,-20.7773438086781,
123.47816249865)) ;
#73878=CARTESIAN_POINT('Ctrl Pts',(-20.8746353857485,-20.9771759356699,
122.971063764424)) ;
#73879=CARTESIAN_POINT('Ctrl Pts',(-20.5815599743237,-20.7971868552511,
123.059210077434)) ;
#73880=CARTESIAN_POINT('Ctrl Pts',(-20.6370889547926,-20.9970924835697,
122.498095047668)) ;
#73881=CARTESIAN_POINT('Ctrl Pts',(-20.3915208071778,-20.8171034031509,
122.680835172587)) ;
#73882=CARTESIAN_POINT('Ctrl Pts',(-20.2519449229786,-21.017024726561,122.134274226636)) ;
#73883=CARTESIAN_POINT('Ctrl Pts',(-20.0834038045587,-20.8370356461422,
122.389779490593)) ;
#73884=CARTESIAN_POINT('Ctrl Pts',(-19.7666424548866,-21.0369285613703,
121.923791010099)) ;
#73885=CARTESIAN_POINT('Ctrl Pts',(-19.6951601330397,-20.8569394809515,
122.221394579836)) ;
#73886=CARTESIAN_POINT('Ctrl Pts',(-19.2387517746191,-21.0568289615578,
121.890890792303)) ;
#73887=CARTESIAN_POINT('Ctrl Pts',(-19.2728466143262,-20.876839881139,122.195076908479)) ;
#73888=CARTESIAN_POINT('Ctrl Pts',(-18.7299794806425,-21.0767786379371,
122.04027094574)) ;
#73889=CARTESIAN_POINT('Ctrl Pts',(-18.8658292110054,-20.8967895575183,
122.314583763135)) ;
#73890=CARTESIAN_POINT('Ctrl Pts',(-18.3031667102184,-21.0967111621575,
122.354115893624)) ;
#73891=CARTESIAN_POINT('Ctrl Pts',(-18.5243802930808,-20.9167220817387,
122.565662292929)) ;
#73892=CARTESIAN_POINT('Ctrl Pts',(-18.0088633208664,-21.1166311711436,
122.794268679496)) ;
#73893=CARTESIAN_POINT('Ctrl Pts',(-18.2889398325272,-20.9366420907249,
122.917786669233)) ;
#73894=CARTESIAN_POINT('Ctrl Pts',(-17.8822937307216,-21.1365880773198,
123.309313272759)) ;
#73895=CARTESIAN_POINT('Ctrl Pts',(-18.1876872095001,-20.9565989969011,
123.329823376665)) ;
#73896=CARTESIAN_POINT('Ctrl Pts',(-17.9384143245851,-21.1564739168213,
123.834958994837)) ;
#73897=CARTESIAN_POINT('Ctrl Pts',(-18.2325869694415,-20.9764848364026,
123.750340253762)) ;
#73898=CARTESIAN_POINT('Ctrl Pts',(-18.1714993858974,-21.1764450889572,
124.311714842716)) ;
#73899=CARTESIAN_POINT('Ctrl Pts',(-18.4190587792687,-20.9964560085384,
124.131743525052)) ;
#73900=CARTESIAN_POINT('Ctrl Pts',(-18.5499193846683,-21.1962592859416,
124.678080172015)) ;
#73901=CARTESIAN_POINT('Ctrl Pts',(-18.7217959353721,-21.0162702055228,
124.424833857205)) ;
#73902=CARTESIAN_POINT('Ctrl Pts',(-19.0342352621691,-21.2162404719098,
124.895714964022)) ;
#73903=CARTESIAN_POINT('Ctrl Pts',(-19.1092580929924,-21.0362513914911,
124.598937764021)) ;
#73904=CARTESIAN_POINT('Ctrl Pts',(-19.4736619237812,-21.2328159772991,
124.928069751283)) ;
#73905=CARTESIAN_POINT('Ctrl Pts',(-19.4607756982869,-21.0528268968803,
124.624819424069)) ;
#73906=CARTESIAN_POINT('Ctrl Pts',(-19.8173383619341,-21.2461254251627,
124.863112509731)) ;
#73907=CARTESIAN_POINT('Ctrl Pts',(-19.7357439277155,-21.0661363447439,
124.572846691441)) ;
#73908=CARTESIAN_POINT('Ctrl Pts',(-20.1458733463393,-21.2594931229393,
124.73871434374)) ;
#73909=CARTESIAN_POINT('Ctrl Pts',(-19.998523136109,-21.0795040425205,124.473349266923)) ;
#73910=CARTESIAN_POINT('Ctrl Pts',(-20.5018728442844,-21.2759836946052,
124.483060829729)) ;
#73911=CARTESIAN_POINT('Ctrl Pts',(-20.2833722640373,-21.0959946141864,
124.268798320229)) ;
#73912=CARTESIAN_POINT('Ctrl Pts',(-20.801833760268,-21.295903966938,124.046874735379)) ;
#73913=CARTESIAN_POINT('Ctrl Pts',(-20.5233223409627,-21.1159148865192,
123.919846740881)) ;
#73914=CARTESIAN_POINT('Ctrl Pts',(-20.9126872838241,-21.312521002659,123.619326861725)) ;
#73915=CARTESIAN_POINT('Ctrl Pts',(-20.6120012338397,-21.1325319222402,
123.57783290666)) ;
#73916=CARTESIAN_POINT('Ctrl Pts',(-20.9100801365058,-21.3258118529401,
123.270041130559)) ;
#73917=CARTESIAN_POINT('Ctrl Pts',(-20.6099160373388,-21.1458227725213,
123.298380131864)) ;
#73918=CARTESIAN_POINT('Ctrl Pts',(-20.8627908877949,-21.3357808980945,
123.012396956915)) ;
#73919=CARTESIAN_POINT('Ctrl Pts',(-20.572081952972,-21.1557918176758,123.092270099761)) ;
#73920=CARTESIAN_POINT('Ctrl Pts',(-20.7725483588054,-21.3456842887281,
122.768260657571)) ;
#73921=CARTESIAN_POINT('Ctrl Pts',(-20.499885452573,-21.1656952083094,122.896960032138)) ;
#73922=CARTESIAN_POINT('Ctrl Pts',(-20.639146259406,-21.3557420748408,122.540122041368)) ;
#73923=CARTESIAN_POINT('Ctrl Pts',(-20.3931639432043,-21.1757529944221,
122.714452096665)) ;
#73924=CARTESIAN_POINT('Ctrl Pts',(-20.4717962813349,-21.3655941114906,
122.342544854359)) ;
#73925=CARTESIAN_POINT('Ctrl Pts',(-20.2592745302504,-21.1856050310718,
122.556386398767)) ;
#73926=CARTESIAN_POINT('Ctrl Pts',(-20.2020865685042,-21.3789592356338,
122.117585029571)) ;
#73927=CARTESIAN_POINT('Ctrl Pts',(-20.0435429434541,-21.198970155215,122.376446523523)) ;
#73928=CARTESIAN_POINT('Ctrl Pts',(-19.8829746643163,-21.3921852985968,
121.970083355977)) ;
#73929=CARTESIAN_POINT('Ctrl Pts',(-19.7882331633885,-21.2121962181781,
122.25842782825)) ;
#73930=CARTESIAN_POINT('Ctrl Pts',(-19.5386166648349,-21.4054889468791,
121.909867161764)) ;
#73931=CARTESIAN_POINT('Ctrl Pts',(-19.5127307955836,-21.2254998664603,
122.210256068313)) ;
#73932=CARTESIAN_POINT('Ctrl Pts',(-19.2760167649112,-21.4154804780421,
121.910107183549)) ;
#73933=CARTESIAN_POINT('Ctrl Pts',(-19.302654042271,-21.2354913976233,122.210450691306)) ;
#73934=CARTESIAN_POINT('Ctrl Pts',(-19.0163207496218,-21.4255199258414,
121.956500605388)) ;
#73935=CARTESIAN_POINT('Ctrl Pts',(-19.0948968590476,-21.2455308454226,
122.247567530299)) ;
#73936=CARTESIAN_POINT('Ctrl Pts',(-18.7732843138924,-21.4353637013552,
122.045159677544)) ;
#73937=CARTESIAN_POINT('Ctrl Pts',(-18.9004686755779,-21.2553746209365,
122.318496939825)) ;
#73938=CARTESIAN_POINT('Ctrl Pts',(-18.5458944196666,-21.4453493427429,
122.176053036264)) ;
#73939=CARTESIAN_POINT('Ctrl Pts',(-18.7185578856858,-21.2653602623241,
122.42321354917)) ;
#73940=CARTESIAN_POINT('Ctrl Pts',(-18.3455158402241,-21.4552861271047,
122.343559635679)) ;
#73941=CARTESIAN_POINT('Ctrl Pts',(-18.5582565294496,-21.2752970466859,
122.557220524187)) ;
#73942=CARTESIAN_POINT('Ctrl Pts',(-18.1755004123223,-21.465335961572,122.545621877057)) ;
#73943=CARTESIAN_POINT('Ctrl Pts',(-18.4222459430947,-21.2853468811533,
122.718871736199)) ;
#73944=CARTESIAN_POINT('Ctrl Pts',(-18.0455857951016,-21.4751864110752,
122.769542152849)) ;
#73945=CARTESIAN_POINT('Ctrl Pts',(-18.3183162510833,-21.2951973306564,
122.898009008209)) ;
#73946=CARTESIAN_POINT('Ctrl Pts',(-17.9548017336223,-21.4851584250573,
123.015333175411)) ;
#73947=CARTESIAN_POINT('Ctrl Pts',(-18.2456911442363,-21.3051693446385,
123.094642518288)) ;
#73948=CARTESIAN_POINT('Ctrl Pts',(-17.9079865988999,-21.4951535829044,
123.273832595295)) ;
#73949=CARTESIAN_POINT('Ctrl Pts',(-18.2082412561885,-21.3151645024856,
123.3014423916)) ;
#73950=CARTESIAN_POINT('Ctrl Pts',(-17.9070803717474,-21.5051875092681,
123.537489745396)) ;
#73951=CARTESIAN_POINT('Ctrl Pts',(-18.2075185318219,-21.3251984288494,
123.512368089065)) ;
#73952=CARTESIAN_POINT('Ctrl Pts',(-17.9507793757721,-21.5150432177005,
123.792798278257)) ;
#73953=CARTESIAN_POINT('Ctrl Pts',(-18.2424799133806,-21.3350541372817,
123.716614351345)) ;
#73954=CARTESIAN_POINT('Ctrl Pts',(-18.0390300007286,-21.5250413670391,
124.040230621181)) ;
#73955=CARTESIAN_POINT('Ctrl Pts',(-18.3130824917955,-21.3450522866204,
123.914559406275)) ;
#73956=CARTESIAN_POINT('Ctrl Pts',(-18.1674560177498,-21.5349407702127,
124.266510551669)) ;
#73957=CARTESIAN_POINT('Ctrl Pts',(-18.4158251303191,-21.354951689794,124.095582078707)) ;
#73958=CARTESIAN_POINT('Ctrl Pts',(-18.3356760699682,-21.5449919671012,
124.470114255053)) ;
#73959=CARTESIAN_POINT('Ctrl Pts',(-18.5504028849582,-21.3650028866824,
124.258463636638)) ;
#73960=CARTESIAN_POINT('Ctrl Pts',(-18.5333267196621,-21.554874290914,124.638598756926)) ;
#73961=CARTESIAN_POINT('Ctrl Pts',(-18.7085246479764,-21.3748852104953,
124.393249391773)) ;
#73962=CARTESIAN_POINT('Ctrl Pts',(-18.759456001813,-21.5648691865706,124.772199668069)) ;
#73963=CARTESIAN_POINT('Ctrl Pts',(-18.8894291059458,-21.3848801061519,
124.500128205226)) ;
#73964=CARTESIAN_POINT('Ctrl Pts',(-19.0061476935315,-21.5748902859531,
124.864395292347)) ;
#73965=CARTESIAN_POINT('Ctrl Pts',(-19.0867832058502,-21.3949012055344,
124.573882634977)) ;
#73966=CARTESIAN_POINT('Ctrl Pts',(-19.2621059878514,-21.5847975538152,
124.912011501675)) ;
#73967=CARTESIAN_POINT('Ctrl Pts',(-19.2915499957338,-21.4048084733965,
124.611973405595)) ;
#73968=CARTESIAN_POINT('Ctrl Pts',(-19.5232414618361,-21.5947358976405,
124.914993347276)) ;
#73969=CARTESIAN_POINT('Ctrl Pts',(-19.5004581837589,-21.4147468172218,
124.61435673395)) ;
#73970=CARTESIAN_POINT('Ctrl Pts',(-19.7826877608884,-21.604739316941,124.872466522389)) ;
#73971=CARTESIAN_POINT('Ctrl Pts',(-19.7080148132996,-21.4247502365222,
124.580333183701)) ;
#73972=CARTESIAN_POINT('Ctrl Pts',(-20.0313953526549,-21.6147738676481,
124.784868563524)) ;
#73973=CARTESIAN_POINT('Ctrl Pts',(-19.9069801784579,-21.4347847872293,
124.510252765367)) ;
#73974=CARTESIAN_POINT('Ctrl Pts',(-20.2570175361581,-21.6246188172537,
124.658232944554)) ;
#73975=CARTESIAN_POINT('Ctrl Pts',(-20.0874764875126,-21.4446297368349,
124.408942636223)) ;
#73976=CARTESIAN_POINT('Ctrl Pts',(-20.4603562192265,-21.6346046593666,
124.492418457944)) ;
#73977=CARTESIAN_POINT('Ctrl Pts',(-20.2501460171759,-21.4546155789478,
124.276289513827)) ;
#73978=CARTESIAN_POINT('Ctrl Pts',(-20.6311392302461,-21.6445394667356,
124.294885221569)) ;
#73979=CARTESIAN_POINT('Ctrl Pts',(-20.3867706983452,-21.4645503863169,
124.118261777518)) ;
#73980=CARTESIAN_POINT('Ctrl Pts',(-20.7664361278029,-21.6545970084489,
124.067883129718)) ;
#73981=CARTESIAN_POINT('Ctrl Pts',(-20.4950064705292,-21.4746079280302,
123.936658954064)) ;
#73982=CARTESIAN_POINT('Ctrl Pts',(-20.8584564949469,-21.6644186059611,
123.826712005203)) ;
#73983=CARTESIAN_POINT('Ctrl Pts',(-20.5686206343265,-21.4844295255424,
123.743721915454)) ;
#73984=CARTESIAN_POINT('Ctrl Pts',(-20.9088388979674,-21.6744748654416,
123.567314526494)) ;
#73985=CARTESIAN_POINT('Ctrl Pts',(-20.6089246277522,-21.4944857850228,
123.536203466964)) ;
#73986=CARTESIAN_POINT('Ctrl Pts',(-20.9129054422664,-21.684414801742,123.306120784311)) ;
#73987=CARTESIAN_POINT('Ctrl Pts',(-20.61217581895,-21.5044257213232,123.327248710015)) ;
#73988=CARTESIAN_POINT('Ctrl Pts',(-20.8724715626847,-21.6943219224864,
123.048933898894)) ;
#73989=CARTESIAN_POINT('Ctrl Pts',(-20.5798268670816,-21.5143328420676,
123.121499921516)) ;
#73990=CARTESIAN_POINT('Ctrl Pts',(-20.786747108785,-21.7043648284116,122.79933394968)) ;
#73991=CARTESIAN_POINT('Ctrl Pts',(-20.5112454371669,-21.5243757479929,
122.921820528242)) ;
#73992=CARTESIAN_POINT('Ctrl Pts',(-20.6607421011446,-21.7142726095109,
122.571477249556)) ;
#73993=CARTESIAN_POINT('Ctrl Pts',(-20.4104399317555,-21.5342835290921,
122.739536474708)) ;
#73994=CARTESIAN_POINT('Ctrl Pts',(-20.495754325636,-21.7242829785133,122.366574426268)) ;
#73995=CARTESIAN_POINT('Ctrl Pts',(-20.2784482779818,-21.5442938980945,
122.575615429182)) ;
#73996=CARTESIAN_POINT('Ctrl Pts',(-20.2969450012805,-21.7343138170821,
122.193488770764)) ;
#73997=CARTESIAN_POINT('Ctrl Pts',(-20.1193995041773,-21.5543247366633,
122.437148355907)) ;
#73998=CARTESIAN_POINT('Ctrl Pts',(-20.0753430040867,-21.7441666567218,
122.05956218883)) ;
#73999=CARTESIAN_POINT('Ctrl Pts',(-19.9421175002561,-21.564177576303,122.330009052223)) ;
#74000=CARTESIAN_POINT('Ctrl Pts',(-19.8307389892277,-21.7541546578867,
121.964427436331)) ;
#74001=CARTESIAN_POINT('Ctrl Pts',(-19.7464337668386,-21.574165577468,122.253902995604)) ;
#74002=CARTESIAN_POINT('Ctrl Pts',(-19.5748309877836,-21.7640834768659,
121.913501885796)) ;
#74003=CARTESIAN_POINT('Ctrl Pts',(-19.5417073934896,-21.5840943964472,
122.213164409837)) ;
#74004=CARTESIAN_POINT('Ctrl Pts',(-19.3124241042383,-21.7740711795882,
121.907308023962)) ;
#74005=CARTESIAN_POINT('Ctrl Pts',(-19.3317819920219,-21.5940820991695,
122.208211065179)) ;
#74006=CARTESIAN_POINT('Ctrl Pts',(-19.0517647367199,-21.7841071793909,
121.947395957951)) ;
#74007=CARTESIAN_POINT('Ctrl Pts',(-19.1232547049505,-21.6041180989721,
122.240283218186)) ;
#74008=CARTESIAN_POINT('Ctrl Pts',(-18.8063639186808,-21.7939620491923,
122.030208537062)) ;
#74009=CARTESIAN_POINT('Ctrl Pts',(-18.9269353053611,-21.6139729687736,
122.306534697317)) ;
#74010=CARTESIAN_POINT('Ctrl Pts',(-18.575622053571,-21.8039614796158,122.155848712775)) ;
#74011=CARTESIAN_POINT('Ctrl Pts',(-18.7423427130502,-21.6239723991971,
122.407048265854)) ;
#74012=CARTESIAN_POINT('Ctrl Pts',(-18.3721015981849,-21.8138565970811,
122.317772569595)) ;
#74013=CARTESIAN_POINT('Ctrl Pts',(-18.5795278239004,-21.6338675166624,
122.536588260672)) ;
#74014=CARTESIAN_POINT('Ctrl Pts',(-18.1969788650004,-21.8239170905981,
122.515789157029)) ;
#74015=CARTESIAN_POINT('Ctrl Pts',(-18.4394307367387,-21.6439280101794,
122.695002760507)) ;
#74016=CARTESIAN_POINT('Ctrl Pts',(-18.0616465448308,-21.8337665707993,
122.736447563601)) ;
#74017=CARTESIAN_POINT('Ctrl Pts',(-18.3311666894869,-21.6537774903805,
122.871529616356)) ;
#74018=CARTESIAN_POINT('Ctrl Pts',(-17.9643529996744,-21.8437930210631,
122.981307539536)) ;
#74019=CARTESIAN_POINT('Ctrl Pts',(-18.2533332210301,-21.6638039406443,
123.067418172796)) ;
#74020=CARTESIAN_POINT('Ctrl Pts',(-17.91173712929,-21.8538243115412,123.239620782811)) ;
#74021=CARTESIAN_POINT('Ctrl Pts',(-18.2112421016013,-21.6738352311224,
123.274069149451)) ;
#74022=CARTESIAN_POINT('Ctrl Pts',(-17.904341497502,-21.863665699193,123.498138969841)) ;
#74023=CARTESIAN_POINT('Ctrl Pts',(-18.2053271327317,-21.6836766187742,
123.480882829659)) ;
#74024=CARTESIAN_POINT('Ctrl Pts',(-17.9420552179328,-21.8736691000842,
123.758271923729)) ;
#74025=CARTESIAN_POINT('Ctrl Pts',(-18.2354994952421,-21.6936800196655,
123.688988903637)) ;
#74026=CARTESIAN_POINT('Ctrl Pts',(-18.0243333211888,-21.8836534828754,
124.007465107882)) ;
#74027=CARTESIAN_POINT('Ctrl Pts',(-18.3013232846925,-21.7036644024566,
123.888342843706)) ;
#74028=CARTESIAN_POINT('Ctrl Pts',(-18.1494974494825,-21.8936925728888,
124.239670692919)) ;
#74029=CARTESIAN_POINT('Ctrl Pts',(-18.4014559474029,-21.71370349247,124.074106700481)) ;
#74030=CARTESIAN_POINT('Ctrl Pts',(-18.30967337421,-21.9035383817979,124.442892027239)) ;
#74031=CARTESIAN_POINT('Ctrl Pts',(-18.5295972153698,-21.7235493013792,
124.236682156643)) ;
#74032=CARTESIAN_POINT('Ctrl Pts',(-18.5050211084765,-21.9135228046169,
124.618000034217)) ;
#74033=CARTESIAN_POINT('Ctrl Pts',(-18.6858761220133,-21.7335337241982,
124.376767460048)) ;
#74034=CARTESIAN_POINT('Ctrl Pts',(-18.7268105926393,-21.9234624298581,
124.756042327735)) ;
#74035=CARTESIAN_POINT('Ctrl Pts',(-18.8633080134688,-21.7434733494394,
124.487199981582)) ;
#74036=CARTESIAN_POINT('Ctrl Pts',(-18.97160932172,-21.9335021193768,124.854379340685)) ;
#74037=CARTESIAN_POINT('Ctrl Pts',(-19.0591475870826,-21.7535130389581,
124.565868438061)) ;
#74038=CARTESIAN_POINT('Ctrl Pts',(-19.2258769015524,-21.9433903077954,
124.908032136416)) ;
#74039=CARTESIAN_POINT('Ctrl Pts',(-19.2625611888641,-21.7634012273766,
124.608789286634)) ;
#74040=CARTESIAN_POINT('Ctrl Pts',(-19.4882188467812,-21.9533798337974,
124.917301153526)) ;
#74041=CARTESIAN_POINT('Ctrl Pts',(-19.4724346146083,-21.7733907533787,
124.616203339472)) ;
#74042=CARTESIAN_POINT('Ctrl Pts',(-19.7473517520532,-21.9633383351526,
124.880791790101)) ;
#74043=CARTESIAN_POINT('Ctrl Pts',(-19.679740427849,-21.7833492547339,124.586994707607)) ;
#74044=CARTESIAN_POINT('Ctrl Pts',(-19.9949571853536,-21.9732379291563,
124.800926502681)) ;
#74045=CARTESIAN_POINT('Ctrl Pts',(-19.8778237805908,-21.7932488487375,
124.523101689369)) ;
#74046=CARTESIAN_POINT('Ctrl Pts',(-20.2282969935453,-21.9832858172776,
124.677397513658)) ;
#74047=CARTESIAN_POINT('Ctrl Pts',(-20.0644952773521,-21.8032967368588,
124.424277463967)) ;
#74048=CARTESIAN_POINT('Ctrl Pts',(-20.4336615726101,-21.9931812425231,
124.517808969279)) ;
#74049=CARTESIAN_POINT('Ctrl Pts',(-20.2287857314875,-21.8131921621044,
124.296606263855)) ;
#74050=CARTESIAN_POINT('Ctrl Pts',(-20.6111028162001,-22.0032426332237,
124.321832201038)) ;
#74051=CARTESIAN_POINT('Ctrl Pts',(-20.3707381429069,-21.8232535528049,
124.139823967692)) ;
#74052=CARTESIAN_POINT('Ctrl Pts',(-20.7488672564471,-22.0130882169104,
124.102810049115)) ;
#74053=CARTESIAN_POINT('Ctrl Pts',(-20.4809482739668,-21.8330991364916,
123.964606606129)) ;
#74054=CARTESIAN_POINT('Ctrl Pts',(-20.8484784323002,-22.0230511902195,
123.860702848392)) ;
#74055=CARTESIAN_POINT('Ctrl Pts',(-20.5606363386565,-21.8430621098008,
123.770920863267)) ;
#74056=CARTESIAN_POINT('Ctrl Pts',(-20.9045567468612,-22.0330768570453,
123.603259320316)) ;
#74057=CARTESIAN_POINT('Ctrl Pts',(-20.6054981356393,-21.8530877766266,
123.564965788728)) ;
#74058=CARTESIAN_POINT('Ctrl Pts',(-20.9151055479369,-22.0429913349116,
123.342939247582)) ;
#74059=CARTESIAN_POINT('Ctrl Pts',(-20.6139362973576,-21.8630022544929,
123.356710337489)) ;
#74060=CARTESIAN_POINT('Ctrl Pts',(-20.8805485314069,-22.0529798495866,
123.082714706922)) ;
#74061=CARTESIAN_POINT('Ctrl Pts',(-20.586289982988,-21.8729907691679,123.148530979108)) ;
#74062=CARTESIAN_POINT('Ctrl Pts',(-20.8003679518877,-22.0630239605021,
122.831264561831)) ;
#74063=CARTESIAN_POINT('Ctrl Pts',(-20.5221446448977,-21.8830348800833,
122.947370978964)) ;
#74064=CARTESIAN_POINT('Ctrl Pts',(-20.6809098953826,-22.0728520980966,
122.602235481597)) ;
#74065=CARTESIAN_POINT('Ctrl Pts',(-20.4265781234052,-21.8928630176779,
122.76414910543)) ;
#74066=CARTESIAN_POINT('Ctrl Pts',(-20.5196736796147,-22.0829286661556,
122.392249516392)) ;
#74067=CARTESIAN_POINT('Ctrl Pts',(-20.2975883848863,-21.9029395857368,
122.596160459755)) ;
#74068=CARTESIAN_POINT('Ctrl Pts',(-20.3287820284441,-22.0927808280597,
122.217258955723)) ;
#74069=CARTESIAN_POINT('Ctrl Pts',(-20.1448754008448,-21.912791747641,122.456169202449)) ;
#74070=CARTESIAN_POINT('Ctrl Pts',(-20.1057172726031,-22.1028537900166,
122.074824536905)) ;
#74071=CARTESIAN_POINT('Ctrl Pts',(-19.9664229786563,-21.9228647095978,
122.342221984015)) ;
#74072=CARTESIAN_POINT('Ctrl Pts',(-19.8668228113682,-22.1126963520195,
121.97561587134)) ;
#74073=CARTESIAN_POINT('Ctrl Pts',(-19.7753082232677,-21.9327072716007,
122.262856048578)) ;
#74074=CARTESIAN_POINT('Ctrl Pts',(-19.6110214816257,-22.1226767885133,
121.917755554063)) ;
#74075=CARTESIAN_POINT('Ctrl Pts',(-19.5706673154193,-21.9426877080945,
122.216568229645)) ;
#74076=CARTESIAN_POINT('Ctrl Pts',(-19.3480335183773,-22.1326950938377,
121.905648968593)) ;
#74077=CARTESIAN_POINT('Ctrl Pts',(-19.3602769131939,-21.9527060134189,
122.206883477632)) ;
#74078=CARTESIAN_POINT('Ctrl Pts',(-19.0903400797142,-22.1425790577571,
121.938406487009)) ;
#74079=CARTESIAN_POINT('Ctrl Pts',(-19.1541230782783,-21.9625899773384,
122.233089760099)) ;
#74080=CARTESIAN_POINT('Ctrl Pts',(-18.8377600204404,-22.1526449344956,
122.016875429342)) ;
#74081=CARTESIAN_POINT('Ctrl Pts',(-18.9520588488056,-21.9726558540769,
122.295865388187)) ;
#74082=CARTESIAN_POINT('Ctrl Pts',(-18.6078114381679,-22.1624840353566,
122.135152615133)) ;
#74083=CARTESIAN_POINT('Ctrl Pts',(-18.7681011911182,-21.9824949549378,
122.390486916667)) ;
#74084=CARTESIAN_POINT('Ctrl Pts',(-18.3974600457077,-22.1725171182223,
122.294091316756)) ;
#74085=CARTESIAN_POINT('Ctrl Pts',(-18.5998201180981,-21.9925280378036,
122.517638081399)) ;
#74086=CARTESIAN_POINT('Ctrl Pts',(-18.2185627412926,-22.1825388034977,
122.487389938075)) ;
#74087=CARTESIAN_POINT('Ctrl Pts',(-18.4567025086376,-22.002549723079,122.67227724618)) ;
#74088=CARTESIAN_POINT('Ctrl Pts',(-18.0778211453225,-22.1924054985962,
122.705132096636)) ;
#74089=CARTESIAN_POINT('Ctrl Pts',(-18.3441099857594,-22.0124164181775,
122.846470267623)) ;
#74090=CARTESIAN_POINT('Ctrl Pts',(-17.9754225073383,-22.2023653883308,
122.946017980741)) ;
#74091=CARTESIAN_POINT('Ctrl Pts',(-18.2621912862455,-22.0223763079121,
123.039178659271)) ;
#74092=CARTESIAN_POINT('Ctrl Pts',(-17.9163607641115,-22.2124003761563,
123.203010659021)) ;
#74093=CARTESIAN_POINT('Ctrl Pts',(-18.2149420385229,-22.0324112957375,
123.244772955829)) ;
#74094=CARTESIAN_POINT('Ctrl Pts',(-17.9025839573901,-22.2222870802306,
123.462494584698)) ;
#74095=CARTESIAN_POINT('Ctrl Pts',(-18.2039207061201,-22.0422979998118,
123.452359223595)) ;
#74096=CARTESIAN_POINT('Ctrl Pts',(-17.9346959979923,-22.2323522244635,
123.724996117173)) ;
#74097=CARTESIAN_POINT('Ctrl Pts',(-18.2296104579225,-22.0523631440447,
123.662360751984)) ;
#74098=CARTESIAN_POINT('Ctrl Pts',(-18.009937769105,-22.242191515192,123.972415043897)) ;
#74099=CARTESIAN_POINT('Ctrl Pts',(-18.2898035447589,-22.0622024347733,
123.860294755891)) ;
#74100=CARTESIAN_POINT('Ctrl Pts',(-18.1292969690011,-22.2522540726305,
124.208342841521)) ;
#74101=CARTESIAN_POINT('Ctrl Pts',(-18.3852909705668,-22.0722649922117,
124.049037294054)) ;
#74102=CARTESIAN_POINT('Ctrl Pts',(-18.285451684864,-22.2621511238826,124.416351010889)) ;
#74103=CARTESIAN_POINT('Ctrl Pts',(-18.5102142588833,-22.0821620434638,
124.215443190149)) ;
#74104=CARTESIAN_POINT('Ctrl Pts',(-18.4753956189542,-22.2720823306308,
124.595319409297)) ;
#74105=CARTESIAN_POINT('Ctrl Pts',(-18.6621688310842,-22.0920932502121,
124.358617678543)) ;
#74106=CARTESIAN_POINT('Ctrl Pts',(-18.6961275310964,-22.2821245148496,
124.739948983668)) ;
#74107=CARTESIAN_POINT('Ctrl Pts',(-18.8387544167778,-22.1021354344309,
124.47432155666)) ;
#74108=CARTESIAN_POINT('Ctrl Pts',(-18.9348029986471,-22.2920111429606,
124.842623278205)) ;
#74109=CARTESIAN_POINT('Ctrl Pts',(-19.0296939129993,-22.1120220625418,
124.556460832634)) ;
#74110=CARTESIAN_POINT('Ctrl Pts',(-19.1902815584454,-22.302004415493,124.90335805786)) ;
#74111=CARTESIAN_POINT('Ctrl Pts',(-19.2340765313827,-22.1220153350742,
124.605048920887)) ;
#74112=CARTESIAN_POINT('Ctrl Pts',(-19.4511817330622,-22.3119494910344,
124.918648968618)) ;
#74113=CARTESIAN_POINT('Ctrl Pts',(-19.442796174619,-22.1319604106157,124.61728190834)) ;
#74114=CARTESIAN_POINT('Ctrl Pts',(-19.7109595708838,-22.3218990417627,
124.888897659264)) ;
#74115=CARTESIAN_POINT('Ctrl Pts',(-19.6506180532169,-22.141909961344,124.593481323135)) ;
#74116=CARTESIAN_POINT('Ctrl Pts',(-19.9637921602484,-22.3319383766107,
124.813587576236)) ;
#74117=CARTESIAN_POINT('Ctrl Pts',(-19.8528843512006,-22.1519492961919,
124.533233558072)) ;
#74118=CARTESIAN_POINT('Ctrl Pts',(-20.1962451731138,-22.3418245155546,
124.697521392909)) ;
#74119=CARTESIAN_POINT('Ctrl Pts',(-20.0388461770694,-22.1618354351359,
124.440381365318)) ;
#74120=CARTESIAN_POINT('Ctrl Pts',(-20.4075357060936,-22.3518226285283,
124.541405526239)) ;
#74121=CARTESIAN_POINT('Ctrl Pts',(-20.2078787966008,-22.1718335481096,
124.315489143515)) ;
#74122=CARTESIAN_POINT('Ctrl Pts',(-20.5872481935433,-22.3617423908807,
124.352530361832)) ;
#74123=CARTESIAN_POINT('Ctrl Pts',(-20.3516487449868,-22.181753310462,124.164389831893)) ;
#74124=CARTESIAN_POINT('Ctrl Pts',(-20.7332188477084,-22.3717817864934,
124.132782767691)) ;
#74125=CARTESIAN_POINT('Ctrl Pts',(-20.4684258066509,-22.1917927060747,
123.988591943343)) ;
#74126=CARTESIAN_POINT('Ctrl Pts',(-20.8373803849402,-22.3816909722817,
123.894117096674)) ;
#74127=CARTESIAN_POINT('Ctrl Pts',(-20.5517552368214,-22.2017018918629,
123.797660275818)) ;
#74128=CARTESIAN_POINT('Ctrl Pts',(-20.8993918233242,-22.3916261564392,
123.640499494835)) ;
#74129=CARTESIAN_POINT('Ctrl Pts',(-20.6013649575712,-22.2116370760204,
123.594766873805)) ;
#74130=CARTESIAN_POINT('Ctrl Pts',(-20.9163470244169,-22.4016672138251,
123.377183112357)) ;
#74131=CARTESIAN_POINT('Ctrl Pts',(-20.6149297759424,-22.2216781334063,
123.38411366101)) ;
#74132=CARTESIAN_POINT('Ctrl Pts',(-20.8879521472954,-22.4115543718584,
123.118900643928)) ;
#74133=CARTESIAN_POINT('Ctrl Pts',(-20.5922146560384,-22.2315652914396,
123.177488436444)) ;
#74134=CARTESIAN_POINT('Ctrl Pts',(-20.8147966667285,-22.4215466515343,
122.866729097608)) ;
#74135=CARTESIAN_POINT('Ctrl Pts',(-20.5336910860111,-22.2415575711155,
122.97575113261)) ;
#74136=CARTESIAN_POINT('Ctrl Pts',(-20.6993946933996,-22.4314951685793,
122.63212443824)) ;
#74137=CARTESIAN_POINT('Ctrl Pts',(-20.4413704002996,-22.2515060881606,
122.788067448919)) ;
#74138=CARTESIAN_POINT('Ctrl Pts',(-20.5455120187873,-22.4414319461497,
122.421182047668)) ;
#74139=CARTESIAN_POINT('Ctrl Pts',(-20.3182652644741,-22.261442865731,122.619313435312)) ;
#74140=CARTESIAN_POINT('Ctrl Pts',(-20.3566546113956,-22.4514149822967,
122.239043334133)) ;
#74141=CARTESIAN_POINT('Ctrl Pts',(-20.1671801441174,-22.2714259018779,
122.473601924756)) ;
#74142=CARTESIAN_POINT('Ctrl Pts',(-20.1374997937771,-22.4614587338904,
122.092007982377)) ;
#74143=CARTESIAN_POINT('Ctrl Pts',(-19.9918566291476,-22.2814696534717,
122.355972866551)) ;
#74144=CARTESIAN_POINT('Ctrl Pts',(-19.9014984820175,-22.471287263103,121.986966332281)) ;
#74145=CARTESIAN_POINT('Ctrl Pts',(-19.803057030311,-22.2912981826842,122.27193912262)) ;
#74146=CARTESIAN_POINT('Ctrl Pts',(-19.6446726698096,-22.4813626240117,
121.922812414337)) ;
#74147=CARTESIAN_POINT('Ctrl Pts',(-19.5975962939444,-22.3013735435929,
122.220614925738)) ;
#74148=CARTESIAN_POINT('Ctrl Pts',(-19.3862413607604,-22.4912192228988,
121.904531259499)) ;
#74149=CARTESIAN_POINT('Ctrl Pts',(-19.3908522878681,-22.3112301424801,
122.205989042091)) ;
#74150=CARTESIAN_POINT('Ctrl Pts',(-19.1232446772994,-22.5012822169167,
121.931678446554)) ;
#74151=CARTESIAN_POINT('Ctrl Pts',(-19.1804545703553,-22.321293136498,122.227705729695)) ;
#74152=CARTESIAN_POINT('Ctrl Pts',(-18.8735448281445,-22.5111601512062,
122.002791143802)) ;
#74153=CARTESIAN_POINT('Ctrl Pts',(-18.9806951761436,-22.3311710707875,
122.284594621574)) ;
#74154=CARTESIAN_POINT('Ctrl Pts',(-18.6369922199402,-22.5211607987643,
122.117182285991)) ;
#74155=CARTESIAN_POINT('Ctrl Pts',(-18.7914526693458,-22.3411717183456,
122.376106428338)) ;
#74156=CARTESIAN_POINT('Ctrl Pts',(-18.4254683343304,-22.5310786452023,
122.269531684406)) ;
#74157=CARTESIAN_POINT('Ctrl Pts',(-18.6222333099972,-22.3510895647836,
122.497984627214)) ;
#74158=CARTESIAN_POINT('Ctrl Pts',(-18.2412825268734,-22.541129762208,122.458791235511)) ;
#74159=CARTESIAN_POINT('Ctrl Pts',(-18.4748836852717,-22.3611406817893,
122.649391549011)) ;
#74160=CARTESIAN_POINT('Ctrl Pts',(-18.0951286475946,-22.5510004975186,
122.673148447067)) ;
#74161=CARTESIAN_POINT('Ctrl Pts',(-18.3579599995673,-22.3710114170999,
122.820875923692)) ;
#74162=CARTESIAN_POINT('Ctrl Pts',(-17.9862416101576,-22.5610712047616,
122.914310640387)) ;
#74163=CARTESIAN_POINT('Ctrl Pts',(-18.270849088114,-22.3810821243429,123.013805409563)) ;
#74164=CARTESIAN_POINT('Ctrl Pts',(-17.9222939723837,-22.5709042122135,
123.164699747297)) ;
#74165=CARTESIAN_POINT('Ctrl Pts',(-18.2196899694515,-22.3909151317947,
123.214115380671)) ;
#74166=CARTESIAN_POINT('Ctrl Pts',(-17.9016542678297,-22.5809347045157,
123.427471548307)) ;
#74167=CARTESIAN_POINT('Ctrl Pts',(-18.2031767454531,-22.400945624097,123.424332776703)) ;
#74168=CARTESIAN_POINT('Ctrl Pts',(-17.9277238840771,-22.5909662995892,
123.689813957219)) ;
#74169=CARTESIAN_POINT('Ctrl Pts',(-18.2240311522087,-22.4109772191704,
123.634206897862)) ;
#74170=CARTESIAN_POINT('Ctrl Pts',(-17.996987812227,-22.6007959987274,123.938651312462)) ;
#74171=CARTESIAN_POINT('Ctrl Pts',(-18.2794406618939,-22.4208069183087,
123.833276183553)) ;
#74172=CARTESIAN_POINT('Ctrl Pts',(-18.1095198728437,-22.610785448609,124.175829192036)) ;
#74173=CARTESIAN_POINT('Ctrl Pts',(-18.3694648327991,-22.4307963681902,
124.023019031505)) ;
#74174=CARTESIAN_POINT('Ctrl Pts',(-18.2628916856932,-22.6208293064246,
124.390633246443)) ;
#74175=CARTESIAN_POINT('Ctrl Pts',(-18.4921611832323,-22.4408402260059,
124.194863205091)) ;
#74176=CARTESIAN_POINT('Ctrl Pts',(-18.4466924342053,-22.6306509970149,
124.571839161865)) ;
#74177=CARTESIAN_POINT('Ctrl Pts',(-18.6391999895716,-22.4506619165961,
124.339828335497)) ;
#74178=CARTESIAN_POINT('Ctrl Pts',(-18.663412437741,-22.6406860875553,124.722085054517)) ;
#74179=CARTESIAN_POINT('Ctrl Pts',(-18.8125751167322,-22.4606970071365,
124.460026463756)) ;
#74180=CARTESIAN_POINT('Ctrl Pts',(-18.9029886662183,-22.650710606538,124.831675526104)) ;
#74181=CARTESIAN_POINT('Ctrl Pts',(-19.0042354735576,-22.4707215261192,
124.547700237809)) ;
#74182=CARTESIAN_POINT('Ctrl Pts',(-19.1536198777415,-22.6605704519482,
124.897332264214)) ;
#74183=CARTESIAN_POINT('Ctrl Pts',(-19.204739284053,-22.4805813715294,124.600226994176)) ;
#74184=CARTESIAN_POINT('Ctrl Pts',(-19.4144244913006,-22.6705302282638,
124.919409093061)) ;
#74185=CARTESIAN_POINT('Ctrl Pts',(-19.4133825651792,-22.4905411478451,
124.617890170222)) ;
#74186=CARTESIAN_POINT('Ctrl Pts',(-19.6768496651458,-22.6805584255785,
124.895342097737)) ;
#74187=CARTESIAN_POINT('Ctrl Pts',(-19.6233228939347,-22.5005693451597,
124.598638241263)) ;
#74188=CARTESIAN_POINT('Ctrl Pts',(-19.9281559636439,-22.6904659678688,
124.827199647071)) ;
#74189=CARTESIAN_POINT('Ctrl Pts',(-19.8243678986999,-22.51047688745,124.544126081424)) ;
#74190=CARTESIAN_POINT('Ctrl Pts',(-20.1667897462468,-22.7004986184326,
124.715157775164)) ;
#74191=CARTESIAN_POINT('Ctrl Pts',(-20.0152757027157,-22.5205095380139,
124.454494146685)) ;
#74192=CARTESIAN_POINT('Ctrl Pts',(-20.3792168210654,-22.7103825748593,
124.565679509322)) ;
#74193=CARTESIAN_POINT('Ctrl Pts',(-20.1852178909652,-22.5303934944406,
124.334913312455)) ;
#74194=CARTESIAN_POINT('Ctrl Pts',(-20.5648833310454,-22.7203722762211,
124.380082284129)) ;
#74195=CARTESIAN_POINT('Ctrl Pts',(-20.333752327996,-22.5403831958024,124.18643693813)) ;
#74196=CARTESIAN_POINT('Ctrl Pts',(-20.7158142404303,-22.7304132714972,
124.163643559997)) ;
#74197=CARTESIAN_POINT('Ctrl Pts',(-20.454498551908,-22.5504241910784,124.013286914038)) ;
#74198=CARTESIAN_POINT('Ctrl Pts',(-20.8249543880197,-22.7402461607655,
123.929430163596)) ;
#74199=CARTESIAN_POINT('Ctrl Pts',(-20.5418120172613,-22.5602570803468,
123.825917666245)) ;
#74200=CARTESIAN_POINT('Ctrl Pts',(-20.8935867560127,-22.750239319133,123.675951817859)) ;
#74201=CARTESIAN_POINT('Ctrl Pts',(-20.5967197715693,-22.5702502387142,
123.623135597207)) ;
#74202=CARTESIAN_POINT('Ctrl Pts',(-20.9167106283964,-22.7602713614851,
123.413324039136)) ;
#74203=CARTESIAN_POINT('Ctrl Pts',(-20.6152207367782,-22.5802822810663,
123.413033509542)) ;
#74204=CARTESIAN_POINT('Ctrl Pts',(-20.8945827854885,-22.7701366054435,
123.155034786076)) ;
#74205=CARTESIAN_POINT('Ctrl Pts',(-20.5975204254551,-22.5901475250248,
123.206402523635)) ;
#74206=CARTESIAN_POINT('Ctrl Pts',(-20.8280023409781,-22.7800984966895,
122.901847296209)) ;
#74207=CARTESIAN_POINT('Ctrl Pts',(-20.5442580738547,-22.6001094162708,
123.003852212977)) ;
#74208=CARTESIAN_POINT('Ctrl Pts',(-20.7172881604763,-22.790133396708,122.66252192034)) ;
#74209=CARTESIAN_POINT('Ctrl Pts',(-20.4556884995148,-22.6101443162892,
122.812391063934)) ;
#74210=CARTESIAN_POINT('Ctrl Pts',(-20.5692752425529,-22.8000184771226,
122.449004039162)) ;
#74211=CARTESIAN_POINT('Ctrl Pts',(-20.3372800779245,-22.6200293967038,
122.641575980296)) ;
#74212=CARTESIAN_POINT('Ctrl Pts',(-20.3831352081332,-22.8100836492474,
122.261135086184)) ;
#74213=CARTESIAN_POINT('Ctrl Pts',(-20.1883694027549,-22.6300945688287,
122.491279318454)) ;
#74214=CARTESIAN_POINT('Ctrl Pts',(-20.1719153766464,-22.8199308839709,
122.111588554408)) ;
#74215=CARTESIAN_POINT('Ctrl Pts',(-20.0193951546591,-22.6399418035521,
122.37164074922)) ;
#74216=CARTESIAN_POINT('Ctrl Pts',(-19.9338810020047,-22.8299616952886,
121.998385955135)) ;
#74217=CARTESIAN_POINT('Ctrl Pts',(-19.8289685381442,-22.6499726148699,
122.281076763213)) ;
#74218=CARTESIAN_POINT('Ctrl Pts',(-19.6801542546411,-22.8399713112021,
121.92888895062)) ;
#74219=CARTESIAN_POINT('Ctrl Pts',(-19.6259877257716,-22.6599822307834,
122.225477204985)) ;
#74220=CARTESIAN_POINT('Ctrl Pts',(-19.4208786354204,-22.8498820906059,
121.904493618339)) ;
#74221=CARTESIAN_POINT('Ctrl Pts',(-19.4185677565269,-22.6698930101871,
122.20595890965)) ;
#74222=CARTESIAN_POINT('Ctrl Pts',(-19.1607322268199,-22.8598113563949,
121.924877430806)) ;
#74223=CARTESIAN_POINT('Ctrl Pts',(-19.2104507120868,-22.6798222759761,
122.222263811396)) ;
#74224=CARTESIAN_POINT('Ctrl Pts',(-18.9052696005904,-22.8698540497075,
121.991077325564)) ;
#74225=CARTESIAN_POINT('Ctrl Pts',(-19.0060800555527,-22.6898649692887,
122.275221687729)) ;
#74226=CARTESIAN_POINT('Ctrl Pts',(-18.6688210508007,-22.8797405824022,
122.098781259465)) ;
#74227=CARTESIAN_POINT('Ctrl Pts',(-18.8169206428243,-22.6997515019835,
122.361382756701)) ;
#74228=CARTESIAN_POINT('Ctrl Pts',(-18.4521283292077,-22.8897337275055,
122.247107144914)) ;
#74229=CARTESIAN_POINT('Ctrl Pts',(-18.6435653091888,-22.7097446470868,
122.480041629506)) ;
#74230=CARTESIAN_POINT('Ctrl Pts',(-18.2654318575566,-22.8996794081796,
122.430014319168)) ;
#74231=CARTESIAN_POINT('Ctrl Pts',(-18.4942067535944,-22.7196903277608,
122.626365697427)) ;
#74232=CARTESIAN_POINT('Ctrl Pts',(-18.1128639587461,-22.9096266658063,
122.642292140938)) ;
#74233=CARTESIAN_POINT('Ctrl Pts',(-18.372150743422,-22.7296375853876,122.796186542585)) ;
#74234=CARTESIAN_POINT('Ctrl Pts',(-17.9986015571631,-22.9196745679278,
122.8803282538)) ;
#74235=CARTESIAN_POINT('Ctrl Pts',(-18.280738856107,-22.739685487509,122.986614497746)) ;
#74236=CARTESIAN_POINT('Ctrl Pts',(-17.9286121290648,-22.9295222735495,
123.129473138902)) ;
#74237=CARTESIAN_POINT('Ctrl Pts',(-18.2247452886835,-22.7495331931307,
123.18592950677)) ;
#74238=CARTESIAN_POINT('Ctrl Pts',(-17.9018275041775,-22.9394837401836,
123.389866644)) ;
#74239=CARTESIAN_POINT('Ctrl Pts',(-18.2033153717119,-22.7594946597648,
123.394243983057)) ;
#74240=CARTESIAN_POINT('Ctrl Pts',(-17.9211473398124,-22.9495132934518,
123.652733485391)) ;
#74241=CARTESIAN_POINT('Ctrl Pts',(-18.2187690258878,-22.769524213033,123.604537583863)) ;
#74242=CARTESIAN_POINT('Ctrl Pts',(-17.9848788716588,-22.9594201854792,
123.905158576433)) ;
#74243=CARTESIAN_POINT('Ctrl Pts',(-18.2697520510413,-22.7794311050604,
123.806478038071)) ;
#74244=CARTESIAN_POINT('Ctrl Pts',(-18.0914378077315,-22.9693678295922,
124.143845240082)) ;
#74245=CARTESIAN_POINT('Ctrl Pts',(-18.3549971072633,-22.7893787491735,
123.997428193049)) ;
#74246=CARTESIAN_POINT('Ctrl Pts',(-18.2384883381668,-22.9793678726211,
124.361682579481)) ;
#74247=CARTESIAN_POINT('Ctrl Pts',(-18.4726356373326,-22.7993787922023,
124.17169927459)) ;
#74248=CARTESIAN_POINT('Ctrl Pts',(-18.4221353270863,-22.9894066386151,
124.551044334178)) ;
#74249=CARTESIAN_POINT('Ctrl Pts',(-18.6195515901072,-22.8094175581963,
124.323190202852)) ;
#74250=CARTESIAN_POINT('Ctrl Pts',(-18.6310313254935,-22.9992317006373,
124.702816918831)) ;
#74251=CARTESIAN_POINT('Ctrl Pts',(-18.7866669492004,-22.8192426202186,
124.444610004211)) ;
#74252=CARTESIAN_POINT('Ctrl Pts',(-18.8683046803301,-23.0092862479637,
124.819034540498)) ;
#74253=CARTESIAN_POINT('Ctrl Pts',(-18.9764846127344,-22.8292971675449,
124.537586113637)) ;
#74254=CARTESIAN_POINT('Ctrl Pts',(-19.1194917233143,-23.0192294914129,
124.89104987129)) ;
#74255=CARTESIAN_POINT('Ctrl Pts',(-19.1774335457929,-22.8392404109942,
124.59520052088)) ;
#74256=CARTESIAN_POINT('Ctrl Pts',(-19.3782034066458,-23.0291316630208,
124.919048155832)) ;
#74257=CARTESIAN_POINT('Ctrl Pts',(-19.3844026140547,-22.849142582602,124.617601382244)) ;
#74258=CARTESIAN_POINT('Ctrl Pts',(-19.6417720055684,-23.039184498631,124.901274622892)) ;
#74259=CARTESIAN_POINT('Ctrl Pts',(-19.5952575647132,-22.8591954182122,
124.603384820688)) ;
#74260=CARTESIAN_POINT('Ctrl Pts',(-19.8937094830224,-23.0490575563165,
124.839234191548)) ;
#74261=CARTESIAN_POINT('Ctrl Pts',(-19.7968081119254,-22.8690684758978,
124.553754624461)) ;
#74262=CARTESIAN_POINT('Ctrl Pts',(-20.1342348698511,-23.0590528178422,
124.733693798466)) ;
#74263=CARTESIAN_POINT('Ctrl Pts',(-19.9892291535961,-22.8790637374234,
124.469324531308)) ;
#74264=CARTESIAN_POINT('Ctrl Pts',(-20.3531841876224,-23.0690781872627,
124.587158170205)) ;
#74265=CARTESIAN_POINT('Ctrl Pts',(-20.1643902941915,-22.8890891068439,
124.352097370289)) ;
#74266=CARTESIAN_POINT('Ctrl Pts',(-20.5410358789156,-23.0789680197893,
124.407538040027)) ;
#74267=CARTESIAN_POINT('Ctrl Pts',(-20.3146713621505,-22.8989789393705,
124.208404998467)) ;
#74268=CARTESIAN_POINT('Ctrl Pts',(-20.7481493171931,-23.0922659905986,
124.126127329807)) ;
#74269=CARTESIAN_POINT('Ctrl Pts',(-20.4803737638767,-22.9122769101799,
123.98326757738)) ;
#74270=CARTESIAN_POINT('Ctrl Pts',(-20.8766367896411,-23.1054643857078,
123.799667857757)) ;
#74271=CARTESIAN_POINT('Ctrl Pts',(-20.58316718686,-22.9254753052891,123.722071594726)) ;
#74272=CARTESIAN_POINT('Ctrl Pts',(-20.9162580762145,-23.1188598279873,
123.449902418925)) ;
#74273=CARTESIAN_POINT('Ctrl Pts',(-20.6148571213026,-22.9388707475686,
123.442305273441)) ;
#74274=CARTESIAN_POINT('Ctrl Pts',(-20.9004717404035,-23.1287356662262,
123.190816756854)) ;
#74275=CARTESIAN_POINT('Ctrl Pts',(-20.6022321474832,-22.9487465858075,
123.235027218103)) ;
#74276=CARTESIAN_POINT('Ctrl Pts',(-20.8389416667209,-23.138797068824,122.933714939008)) ;
#74277=CARTESIAN_POINT('Ctrl Pts',(-20.5530100608366,-22.9588079884053,
123.029348080478)) ;
#74278=CARTESIAN_POINT('Ctrl Pts',(-20.7357971607968,-23.1486621257591,
122.695832837335)) ;
#74279=CARTESIAN_POINT('Ctrl Pts',(-20.4704951899831,-22.9686730453404,
122.839039863601)) ;
#74280=CARTESIAN_POINT('Ctrl Pts',(-20.5912157870912,-23.1586742217079,
122.476050346829)) ;
#74281=CARTESIAN_POINT('Ctrl Pts',(-20.3548367390331,-22.9786851412892,
122.663215848403)) ;
#74282=CARTESIAN_POINT('Ctrl Pts',(-20.3516936594629,-23.1719515308534,
122.222286259343)) ;
#74283=CARTESIAN_POINT('Ctrl Pts',(-20.1631968596537,-22.9919624504346,
122.460187975031)) ;
#74284=CARTESIAN_POINT('Ctrl Pts',(-19.976439806796,-23.1885505563607,121.990323874567)) ;
#74285=CARTESIAN_POINT('Ctrl Pts',(-19.8630376390117,-23.0085614759419,
122.27463286839)) ;
#74286=CARTESIAN_POINT('Ctrl Pts',(-19.5445846288345,-23.2051496043937,
121.900290049197)) ;
#74287=CARTESIAN_POINT('Ctrl Pts',(-19.5174874237851,-23.025160523975,122.202591932357)) ;
#74288=CARTESIAN_POINT('Ctrl Pts',(-19.1970504323598,-23.2183930164246,
121.919316506813)) ;
#74289=CARTESIAN_POINT('Ctrl Pts',(-19.2395130687559,-23.0384039360059,
122.217815974426)) ;
#74290=CARTESIAN_POINT('Ctrl Pts',(-18.9401631490869,-23.2284304441131,
121.979134289614)) ;
#74291=CARTESIAN_POINT('Ctrl Pts',(-19.0339916375281,-23.0484413636943,
122.26566763804)) ;
#74292=CARTESIAN_POINT('Ctrl Pts',(-18.7007825062175,-23.2383347460687,
122.081317818178)) ;
#74293=CARTESIAN_POINT('Ctrl Pts',(-18.8424912391791,-23.0583456656499,
122.347410849636)) ;
#74294=CARTESIAN_POINT('Ctrl Pts',(-18.4082618728007,-23.2516015860438,
122.27103030745)) ;
#74295=CARTESIAN_POINT('Ctrl Pts',(-18.60846034993,-23.0716125056251,122.499189722715)) ;
#74296=CARTESIAN_POINT('Ctrl Pts',(-18.1123399886893,-23.2682277841338,
122.599191193704)) ;
#74297=CARTESIAN_POINT('Ctrl Pts',(-18.37173453001,-23.088238703715,122.761707661206)) ;
#74298=CARTESIAN_POINT('Ctrl Pts',(-17.9131297580703,-23.2881468995172,
123.089717711768)) ;
#74299=CARTESIAN_POINT('Ctrl Pts',(-18.2123565653371,-23.1081578190985,
123.154114524712)) ;
#74300=CARTESIAN_POINT('Ctrl Pts',(-17.8962057486873,-23.3047533226514,
123.530754190473)) ;
#74301=CARTESIAN_POINT('Ctrl Pts',(-18.1988208182487,-23.1247642422327,
123.506996945006)) ;
#74302=CARTESIAN_POINT('Ctrl Pts',(-17.9736383079811,-23.3180495431471,
123.871481315113)) ;
#74303=CARTESIAN_POINT('Ctrl Pts',(-18.260758884604,-23.1380604627284,123.779530840826)) ;
#74304=CARTESIAN_POINT('Ctrl Pts',(-18.1080876894243,-23.3313183754886,
124.193291225487)) ;
#74305=CARTESIAN_POINT('Ctrl Pts',(-18.3683238288418,-23.1513292950698,
124.03699746914)) ;
#74306=CARTESIAN_POINT('Ctrl Pts',(-18.3795904845169,-23.3480096235217,
124.544002089699)) ;
#74307=CARTESIAN_POINT('Ctrl Pts',(-18.5855160258156,-23.1680205431029,
124.317555357592)) ;
#74308=CARTESIAN_POINT('Ctrl Pts',(-18.8243580038421,-23.3678193551945,
124.825895671642)) ;
#74309=CARTESIAN_POINT('Ctrl Pts',(-18.9413318339364,-23.1878302747757,
124.543077599675)) ;
#74310=CARTESIAN_POINT('Ctrl Pts',(-19.342669247738,-23.387796962523,124.941057197764)) ;
#74311=CARTESIAN_POINT('Ctrl Pts',(-19.3559797197809,-23.2078078821043,
124.635208534349)) ;
#74312=CARTESIAN_POINT('Ctrl Pts',(-19.8676443126911,-23.4077232715809,
124.871649885316)) ;
#74313=CARTESIAN_POINT('Ctrl Pts',(-19.7759608640312,-23.2277341911621,
124.579685870567)) ;
#74314=CARTESIAN_POINT('Ctrl Pts',(-20.3358743902142,-23.4275401317456,
124.63015528066)) ;
#74315=CARTESIAN_POINT('Ctrl Pts',(-20.1505472945724,-23.2475510513268,
124.386491407269)) ;
#74316=CARTESIAN_POINT('Ctrl Pts',(-20.6978674016967,-23.4476399473396,
124.237525821814)) ;
#74317=CARTESIAN_POINT('Ctrl Pts',(-20.4401428874829,-23.2676508669208,
124.072390151263)) ;
#74318=CARTESIAN_POINT('Ctrl Pts',(-20.9010174942789,-23.4673969112221,
123.753071870138)) ;
#74319=CARTESIAN_POINT('Ctrl Pts',(-20.6026658029561,-23.2874078308034,
123.684825804928)) ;
#74320=CARTESIAN_POINT('Ctrl Pts',(-20.9280426936551,-23.4874338372916,
123.221391133702)) ;
#74321=CARTESIAN_POINT('Ctrl Pts',(-20.6242875973045,-23.3074447568728,
123.259481619139)) ;
#74322=CARTESIAN_POINT('Ctrl Pts',(-20.7724260968496,-23.5073034196731,
122.716597558735)) ;
#74323=CARTESIAN_POINT('Ctrl Pts',(-20.4997956703775,-23.3273143392544,
122.855645015619)) ;
#74324=CARTESIAN_POINT('Ctrl Pts',(-20.4545393934254,-23.5272079914263,
122.293853597021)) ;
#74325=CARTESIAN_POINT('Ctrl Pts',(-20.245486515064,-23.3472189110075,122.517448272747)) ;
#74326=CARTESIAN_POINT('Ctrl Pts',(-20.010214950493,-23.5471605936248,122.004204373884)) ;
#74327=CARTESIAN_POINT('Ctrl Pts',(-19.8900270498159,-23.367171513206,122.28572785493)) ;
#74328=CARTESIAN_POINT('Ctrl Pts',(-19.4949902616996,-23.567070084595,121.884042017119)) ;
#74329=CARTESIAN_POINT('Ctrl Pts',(-19.477846400596,-23.3870810041763,122.189596888272)) ;
#74330=CARTESIAN_POINT('Ctrl Pts',(-18.9708122647387,-23.5869214532945,
121.945279500549)) ;
#74331=CARTESIAN_POINT('Ctrl Pts',(-19.0585021151188,-23.4069323728757,
122.23858718962)) ;
#74332=CARTESIAN_POINT('Ctrl Pts',(-18.4941229339975,-23.6070016494305,
122.185035924268)) ;
#74333=CARTESIAN_POINT('Ctrl Pts',(-18.6771515404996,-23.4270125690117,
122.43039179208)) ;
#74334=CARTESIAN_POINT('Ctrl Pts',(-18.1327837984762,-23.6268025930059,
122.567847534535)) ;
#74335=CARTESIAN_POINT('Ctrl Pts',(-18.3880785930256,-23.4468135125871,
122.736642978161)) ;
#74336=CARTESIAN_POINT('Ctrl Pts',(-17.9208269263131,-23.6467865695154,
123.054772698346)) ;
#74337=CARTESIAN_POINT('Ctrl Pts',(-18.2185138580659,-23.4667974890966,
123.126183626084)) ;
#74338=CARTESIAN_POINT('Ctrl Pts',(-17.8886839109788,-23.666702532491,123.583127051777)) ;
#74339=CARTESIAN_POINT('Ctrl Pts',(-18.1928000784033,-23.4867134520722,
123.548868146991)) ;
#74340=CARTESIAN_POINT('Ctrl Pts',(-18.0370543005805,-23.6865729673129,
124.090087584565)) ;
#74341=CARTESIAN_POINT('Ctrl Pts',(-18.3114982241245,-23.5065838868942,
123.954437479053)) ;
#74342=CARTESIAN_POINT('Ctrl Pts',(-18.3529120735645,-23.706623252546,124.519105466841)) ;
#74343=CARTESIAN_POINT('Ctrl Pts',(-18.5641852225777,-23.5266341721272,
124.297650597675)) ;
#74344=CARTESIAN_POINT('Ctrl Pts',(-18.7899845412355,-23.7263972213053,
124.811340607941)) ;
#74345=CARTESIAN_POINT('Ctrl Pts',(-18.9138460145566,-23.5464081408865,
124.531438476037)) ;
#74346=CARTESIAN_POINT('Ctrl Pts',(-19.3073372095551,-23.7464536794248,
124.938934907385)) ;
#74347=CARTESIAN_POINT('Ctrl Pts',(-19.3277281762554,-23.5664645990061,
124.633511759487)) ;
#74348=CARTESIAN_POINT('Ctrl Pts',(-19.8306051755305,-23.7662485624158,
124.882843707618)) ;
#74349=CARTESIAN_POINT('Ctrl Pts',(-19.7463441186502,-23.5862594819971,
124.588636471734)) ;
#74350=CARTESIAN_POINT('Ctrl Pts',(-20.3078444225555,-23.7862152177182,
124.651011447799)) ;
#74351=CARTESIAN_POINT('Ctrl Pts',(-20.1281345081567,-23.6062261372994,
124.40316804433)) ;
#74352=CARTESIAN_POINT('Ctrl Pts',(-20.6767016462669,-23.8061741877947,
124.269621393415)) ;
#74353=CARTESIAN_POINT('Ctrl Pts',(-20.4232185854534,-23.6261851073759,
124.09805398004)) ;
#74354=CARTESIAN_POINT('Ctrl Pts',(-20.8928840688212,-23.8260702753848,
123.787054530336)) ;
#74355=CARTESIAN_POINT('Ctrl Pts',(-20.5961622166163,-23.6460811949661,
123.711998606436)) ;
#74356=CARTESIAN_POINT('Ctrl Pts',(-20.9320464015032,-23.8459684452964,
123.25969081321)) ;
#74357=CARTESIAN_POINT('Ctrl Pts',(-20.6274889756677,-23.6659793648776,
123.290106706066)) ;
#74358=CARTESIAN_POINT('Ctrl Pts',(-20.7893616369833,-23.8658742806635,
122.750190072166)) ;
#74359=CARTESIAN_POINT('Ctrl Pts',(-20.5133377383693,-23.6858852002447,
122.882506513553)) ;
#74360=CARTESIAN_POINT('Ctrl Pts',(-20.4807327589257,-23.8858242056014,
122.319088447616)) ;
#74361=CARTESIAN_POINT('Ctrl Pts',(-20.2664316366618,-23.7058351251827,
122.537627039628)) ;
#74362=CARTESIAN_POINT('Ctrl Pts',(-20.0452649316596,-23.9057033955118,
122.019778092152)) ;
#74363=CARTESIAN_POINT('Ctrl Pts',(-19.9180547884745,-23.725714315093,122.298181446568)) ;
#74364=CARTESIAN_POINT('Ctrl Pts',(-19.5313379425043,-23.9256847197924,
121.886108845962)) ;
#74365=CARTESIAN_POINT('Ctrl Pts',(-19.5069121971362,-23.7456956393736,
122.191249793125)) ;
#74366=CARTESIAN_POINT('Ctrl Pts',(-19.0038793189926,-23.9456145040007,
121.936000230765)) ;
#74367=CARTESIAN_POINT('Ctrl Pts',(-19.084945405429,-23.765625423582,122.231166579714)) ;
#74368=CARTESIAN_POINT('Ctrl Pts',(-18.5255093850122,-23.9655344933915,
122.162577000596)) ;
#74369=CARTESIAN_POINT('Ctrl Pts',(-18.70225086222,-23.7855454129728,122.412432333271)) ;
#74370=CARTESIAN_POINT('Ctrl Pts',(-18.1533588422932,-23.9853896887455,
122.536910497514)) ;
#74371=CARTESIAN_POINT('Ctrl Pts',(-18.4045331019949,-23.8054006083268,
122.711900044301)) ;
#74372=CARTESIAN_POINT('Ctrl Pts',(-17.9297252154946,-24.0054356904049,
123.020349675074)) ;
#74373=CARTESIAN_POINT('Ctrl Pts',(-18.225629991919,-23.8254466099861,123.098661705087)) ;
#74374=CARTESIAN_POINT('Ctrl Pts',(-17.8922881636494,-24.0219354376147,
123.457418896115)) ;
#74375=CARTESIAN_POINT('Ctrl Pts',(-18.1956840852011,-23.8419463571959,
123.448290621712)) ;
#74376=CARTESIAN_POINT('Ctrl Pts',(-17.9536182368234,-24.0353240420628,
123.80382318546)) ;
#74377=CARTESIAN_POINT('Ctrl Pts',(-18.2447511118131,-23.855334961644,123.725437823404)) ;
#74378=CARTESIAN_POINT('Ctrl Pts',(-18.0424306541701,-24.0451858703977,
124.047300970895)) ;
#74379=CARTESIAN_POINT('Ctrl Pts',(-18.3158010379649,-23.8651967899789,
123.920212948107)) ;
#74380=CARTESIAN_POINT('Ctrl Pts',(-18.1728224347277,-24.0551520131552,
124.274441107763)) ;
#74381=CARTESIAN_POINT('Ctrl Pts',(-18.4201247042669,-23.8751629327365,
124.101932317986)) ;
#74382=CARTESIAN_POINT('Ctrl Pts',(-18.3983154769493,-24.0685137592802,
124.543527593451)) ;
#74383=CARTESIAN_POINT('Ctrl Pts',(-18.600479724246,-23.8885246788614,124.317163946771)) ;
#74384=CARTESIAN_POINT('Ctrl Pts',(-18.7557534013745,-24.0849680882353,
124.79576607839)) ;
#74385=CARTESIAN_POINT('Ctrl Pts',(-18.8864880582342,-23.9049790078165,
124.518993913012)) ;
#74386=CARTESIAN_POINT('Ctrl Pts',(-19.1855079887592,-24.1017353332835,
124.913045707108)) ;
#74387=CARTESIAN_POINT('Ctrl Pts',(-19.2302449597953,-23.9217462528648,
124.61279458323)) ;
#74388=CARTESIAN_POINT('Ctrl Pts',(-19.5321625871977,-24.1149218985576,
124.914163508208)) ;
#74389=CARTESIAN_POINT('Ctrl Pts',(-19.5076007478974,-23.9349328181389,
124.613694249745)) ;
#74390=CARTESIAN_POINT('Ctrl Pts',(-19.7909027433504,-24.1249113573022,
124.870218955384)) ;
#74391=CARTESIAN_POINT('Ctrl Pts',(-19.7145860227272,-23.9449222768835,
124.578534711631)) ;
#74392=CARTESIAN_POINT('Ctrl Pts',(-20.0373293988203,-24.1348651297833,
124.782335916203)) ;
#74393=CARTESIAN_POINT('Ctrl Pts',(-19.9117282978741,-23.9548760493646,
124.508226619746)) ;
#74394=CARTESIAN_POINT('Ctrl Pts',(-20.2667248445259,-24.144912946316,124.651640371328)) ;
#74395=CARTESIAN_POINT('Ctrl Pts',(-20.0952430132553,-23.9649238658972,
124.403668150689)) ;
#74396=CARTESIAN_POINT('Ctrl Pts',(-20.4660081192489,-24.1547544794385,
124.486757064538)) ;
#74397=CARTESIAN_POINT('Ctrl Pts',(-20.2546683482556,-23.9747653990197,
124.27175978153)) ;
#74398=CARTESIAN_POINT('Ctrl Pts',(-20.636481553147,-24.1647407216582,124.287296273897)) ;
#74399=CARTESIAN_POINT('Ctrl Pts',(-20.3910452989074,-23.9847516412394,
124.112189719401)) ;
#74400=CARTESIAN_POINT('Ctrl Pts',(-20.7692271457761,-24.1746773450831,
124.06238042497)) ;
#74401=CARTESIAN_POINT('Ctrl Pts',(-20.497239809877,-23.9946882646643,123.932255945756)) ;
#74402=CARTESIAN_POINT('Ctrl Pts',(-20.8617993883926,-24.184727222466,123.815064619608)) ;
#74403=CARTESIAN_POINT('Ctrl Pts',(-20.5712954677108,-24.0047381420473,
123.734402552555)) ;
#74404=CARTESIAN_POINT('Ctrl Pts',(-20.9092661001648,-24.1945776612436,
123.560575071868)) ;
#74405=CARTESIAN_POINT('Ctrl Pts',(-20.6092666006814,-24.0145885808249,
123.53081059359)) ;
#74406=CARTESIAN_POINT('Ctrl Pts',(-20.9125392724031,-24.2045496752123,
123.298574461712)) ;
#74407=CARTESIAN_POINT('Ctrl Pts',(-20.6118828876205,-24.0245605947936,
123.3212101705)) ;
#74408=CARTESIAN_POINT('Ctrl Pts',(-20.8701252718286,-24.2145448438384,
123.039316830686)) ;
#74409=CARTESIAN_POINT('Ctrl Pts',(-20.5779494825875,-24.0345557634197,
123.113804490714)) ;
#74410=CARTESIAN_POINT('Ctrl Pts',(-20.78272672112,-24.2245787270997,122.790564493775)) ;
#74411=CARTESIAN_POINT('Ctrl Pts',(-20.5080285227167,-24.0445896466809,
122.914803398227)) ;
#74412=CARTESIAN_POINT('Ctrl Pts',(-20.6560814228893,-24.234434597163,122.564616215092)) ;
#74413=CARTESIAN_POINT('Ctrl Pts',(-20.4067104191487,-24.0544455167443,
122.734046035466)) ;
#74414=CARTESIAN_POINT('Ctrl Pts',(-20.4901252099173,-24.2444321430802,
122.360979293834)) ;
#74415=CARTESIAN_POINT('Ctrl Pts',(-20.2739437686294,-24.0644430626614,
122.571137967992)) ;
#74416=CARTESIAN_POINT('Ctrl Pts',(-20.2931350357888,-24.2543402699794,
122.190698398453)) ;
#74417=CARTESIAN_POINT('Ctrl Pts',(-20.1163503191905,-24.0743511895607,
122.434915056073)) ;
#74418=CARTESIAN_POINT('Ctrl Pts',(-20.0674961654785,-24.2643506415016,
122.055437128111)) ;
#74419=CARTESIAN_POINT('Ctrl Pts',(-19.9358381408742,-24.0843615610829,
122.326707954225)) ;
#74420=CARTESIAN_POINT('Ctrl Pts',(-19.8211172047511,-24.274381084249,121.961778537645)) ;
#74421=CARTESIAN_POINT('Ctrl Pts',(-19.7387341883922,-24.0943920038303,
122.251783172163)) ;
#74422=CARTESIAN_POINT('Ctrl Pts',(-19.567014787891,-24.2842290368023,121.912623318363)) ;
#74423=CARTESIAN_POINT('Ctrl Pts',(-19.5354521536671,-24.1042399563836,
122.212461213181)) ;
#74424=CARTESIAN_POINT('Ctrl Pts',(-19.3026436245722,-24.2942917058233,
121.908036630915)) ;
#74425=CARTESIAN_POINT('Ctrl Pts',(-19.3239551506336,-24.1143026254045,
122.208794046212)) ;
#74426=CARTESIAN_POINT('Ctrl Pts',(-19.0458393133489,-24.3041860812872,
121.948921771781)) ;
#74427=CARTESIAN_POINT('Ctrl Pts',(-19.1185123080235,-24.1241970008685,
122.24150428493)) ;
#74428=CARTESIAN_POINT('Ctrl Pts',(-18.7986820358378,-24.3141278796054,
122.033501629757)) ;
#74429=CARTESIAN_POINT('Ctrl Pts',(-18.9207873807656,-24.1341387991866,
122.309170130401)) ;
#74430=CARTESIAN_POINT('Ctrl Pts',(-18.568460887549,-24.3241303733327,122.160425707842)) ;
#74431=CARTESIAN_POINT('Ctrl Pts',(-18.7366115490919,-24.1441412929139,
122.410711225786)) ;
#74432=CARTESIAN_POINT('Ctrl Pts',(-18.3634159134579,-24.3341651718396,
122.32621930411)) ;
#74433=CARTESIAN_POINT('Ctrl Pts',(-18.572576923515,-24.1541760914208,122.543347798557)) ;
#74434=CARTESIAN_POINT('Ctrl Pts',(-18.1931997743441,-24.3440100558189,
122.521073096118)) ;
#74435=CARTESIAN_POINT('Ctrl Pts',(-18.4364059140593,-24.1640209754002,
122.699231890635)) ;
#74436=CARTESIAN_POINT('Ctrl Pts',(-18.0570939033418,-24.353995912637,122.74538606812)) ;
#74437=CARTESIAN_POINT('Ctrl Pts',(-18.3275230654761,-24.1740068322182,
122.878683238655)) ;
#74438=CARTESIAN_POINT('Ctrl Pts',(-17.9622837120141,-24.3639307268117,
122.988691099176)) ;
#74439=CARTESIAN_POINT('Ctrl Pts',(-18.2516769244132,-24.183941646393,123.07332776623)) ;
#74440=CARTESIAN_POINT('Ctrl Pts',(-17.9107758865764,-24.3739882265971,
123.247885387994)) ;
#74441=CARTESIAN_POINT('Ctrl Pts',(-18.2104726941361,-24.1939991461783,
123.28068369653)) ;
#74442=CARTESIAN_POINT('Ctrl Pts',(-17.9047935451196,-24.3838099850154,
123.505950068635)) ;
#74443=CARTESIAN_POINT('Ctrl Pts',(-18.2056888745737,-24.2038209045966,
123.487134859051)) ;
#74444=CARTESIAN_POINT('Ctrl Pts',(-17.9441385894984,-24.3938656427994,
123.767234420937)) ;
#74445=CARTESIAN_POINT('Ctrl Pts',(-18.2371668835213,-24.2138765623806,
123.696162133941)) ;
#74446=CARTESIAN_POINT('Ctrl Pts',(-18.0277646257666,-24.4038078249794,
124.014774122517)) ;
#74447=CARTESIAN_POINT('Ctrl Pts',(-18.3040695599417,-24.2238187445607,
123.894192987516)) ;
#74448=CARTESIAN_POINT('Ctrl Pts',(-18.1519307758805,-24.4137130336741,
124.243545142384)) ;
#74449=CARTESIAN_POINT('Ctrl Pts',(-18.4034039803286,-24.2337239532553,
124.077208506641)) ;
#74450=CARTESIAN_POINT('Ctrl Pts',(-18.3162322484319,-24.4237548246365,
124.450038000941)) ;
#74451=CARTESIAN_POINT('Ctrl Pts',(-18.5348467279855,-24.2437657442178,
124.242401635478)) ;
#74452=CARTESIAN_POINT('Ctrl Pts',(-18.5112465950809,-24.4336625991088,
124.622564118238)) ;
#74453=CARTESIAN_POINT('Ctrl Pts',(-18.6908591806819,-24.25367351869,124.380420796196)) ;
#74454=CARTESIAN_POINT('Ctrl Pts',(-18.7353216882154,-24.4436740993364,
124.760445262969)) ;
#74455=CARTESIAN_POINT('Ctrl Pts',(-18.8701201999352,-24.2636850189176,
124.490724088854)) ;
#74456=CARTESIAN_POINT('Ctrl Pts',(-18.9806475911466,-24.4537068597291,
124.857016709401)) ;
#74457=CARTESIAN_POINT('Ctrl Pts',(-19.0663816751917,-24.2737177793103,
124.567979438308)) ;
#74458=CARTESIAN_POINT('Ctrl Pts',(-19.2342398512339,-24.463557428864,124.909018469906)) ;
#74459=CARTESIAN_POINT('Ctrl Pts',(-19.2692552091276,-24.2835683484452,
124.609578862469)) ;
#74460=CARTESIAN_POINT('Ctrl Pts',(-19.4965930730574,-24.4735460383939,
124.916794312938)) ;
#74461=CARTESIAN_POINT('Ctrl Pts',(-19.4791376938432,-24.2935569579751,
124.615797717518)) ;
#74462=CARTESIAN_POINT('Ctrl Pts',(-19.7547810174252,-24.483474694418,124.879120015972)) ;
#74463=CARTESIAN_POINT('Ctrl Pts',(-19.685687402309,-24.3034856139992,124.585656541612)) ;
#74464=CARTESIAN_POINT('Ctrl Pts',(-20.0041249025527,-24.4934624405958,
124.797121058198)) ;
#74465=CARTESIAN_POINT('Ctrl Pts',(-19.8851618270809,-24.313473360177,124.520055766498)) ;
#74466=CARTESIAN_POINT('Ctrl Pts',(-20.2363287244197,-24.5034984295315,
124.672094532579)) ;
#74467=CARTESIAN_POINT('Ctrl Pts',(-20.0709240851037,-24.3235093491128,
124.42003291363)) ;
#74468=CARTESIAN_POINT('Ctrl Pts',(-20.4398532894537,-24.5133532993451,
124.511915768952)) ;
#74469=CARTESIAN_POINT('Ctrl Pts',(-20.23374208075,-24.3333642189264,124.291888988596)) ;
#74470=CARTESIAN_POINT('Ctrl Pts',(-20.6152286146968,-24.5233527405869,
124.316286380205)) ;
#74471=CARTESIAN_POINT('Ctrl Pts',(-20.3740410150847,-24.3433636601681,
124.135384433191)) ;
#74472=CARTESIAN_POINT('Ctrl Pts',(-20.7528077612701,-24.533247814767,124.095579716409)) ;
#74473=CARTESIAN_POINT('Ctrl Pts',(-20.4841026378956,-24.3532587343482,
123.958818739032)) ;
#74474=CARTESIAN_POINT('Ctrl Pts',(-20.8515452177521,-24.5433084706067,
123.850362627623)) ;
#74475=CARTESIAN_POINT('Ctrl Pts',(-20.5630911554068,-24.3633193901879,
123.762644277068)) ;
#74476=CARTESIAN_POINT('Ctrl Pts',(-20.9052114657529,-24.5531573448023,
123.597149046197)) ;
#74477=CARTESIAN_POINT('Ctrl Pts',(-20.6060224056543,-24.3731682643835,
123.560073894341)) ;
#74478=CARTESIAN_POINT('Ctrl Pts',(-20.9149218985276,-24.5631860567655,
123.333787858279)) ;
#74479=CARTESIAN_POINT('Ctrl Pts',(-20.6137892700435,-24.3831969763468,
123.349384859398)) ;
#74480=CARTESIAN_POINT('Ctrl Pts',(-20.8780431868156,-24.5732154573486,
123.072813707598)) ;
#74481=CARTESIAN_POINT('Ctrl Pts',(-20.5842846871539,-24.3932263769299,
123.140605706527)) ;
#74482=CARTESIAN_POINT('Ctrl Pts',(-20.7984988601389,-24.5830556509655,
122.826757371422)) ;
#74483=CARTESIAN_POINT('Ctrl Pts',(-20.5206480690799,-24.4030665705467,
122.943761971265)) ;
#74484=CARTESIAN_POINT('Ctrl Pts',(-20.6758759732977,-24.5930590735407,
122.594259198582)) ;
#74485=CARTESIAN_POINT('Ctrl Pts',(-20.4225485501973,-24.4130699931219,
122.757764169377)) ;
#74486=CARTESIAN_POINT('Ctrl Pts',(-20.5149236679389,-24.6030446106337,
122.386952011264)) ;
#74487=CARTESIAN_POINT('Ctrl Pts',(-20.2937856775477,-24.423055530215,122.591919429252)) ;
#74488=CARTESIAN_POINT('Ctrl Pts',(-20.3192148830305,-24.6130856151206,
122.210004149997)) ;
#74489=CARTESIAN_POINT('Ctrl Pts',(-20.1372175724213,-24.4330965347018,
122.450362171703)) ;
#74490=CARTESIAN_POINT('Ctrl Pts',(-20.1002988243439,-24.6229291540618,
122.072161974202)) ;
#74491=CARTESIAN_POINT('Ctrl Pts',(-19.9620847673465,-24.442940073643,122.340090125974)) ;
#74492=CARTESIAN_POINT('Ctrl Pts',(-19.8575938758028,-24.6329141850526,
121.972533729816)) ;
#74493=CARTESIAN_POINT('Ctrl Pts',(-19.7679204996431,-24.4529251046338,
122.260388809874)) ;
#74494=CARTESIAN_POINT('Ctrl Pts',(-19.6023947114869,-24.6428536475746,
121.916697509482)) ;
#74495=CARTESIAN_POINT('Ctrl Pts',(-19.5637613212233,-24.4628645671558,
122.215721172914)) ;
#74496=CARTESIAN_POINT('Ctrl Pts',(-19.3388001962172,-24.6528933797984,
121.905974359245)) ;
#74497=CARTESIAN_POINT('Ctrl Pts',(-19.3528855389491,-24.4729042993796,
122.207143937649)) ;
#74498=CARTESIAN_POINT('Ctrl Pts',(-19.0812413724827,-24.6627815601156,
121.940528367515)) ;
#74499=CARTESIAN_POINT('Ctrl Pts',(-19.1468393800042,-24.4827924796968,
122.23478829755)) ;
#74500=CARTESIAN_POINT('Ctrl Pts',(-18.8309303395571,-24.6727710758181,
122.019607849818)) ;
#74501=CARTESIAN_POINT('Ctrl Pts',(-18.9465910651468,-24.4927819953993,
122.298052933552)) ;
#74502=CARTESIAN_POINT('Ctrl Pts',(-18.5989667873203,-24.6827296264728,
122.140752466217)) ;
#74503=CARTESIAN_POINT('Ctrl Pts',(-18.7610210868457,-24.502740546054,122.394969531165)) ;
#74504=CARTESIAN_POINT('Ctrl Pts',(-18.3923783176622,-24.6926290335778,
122.298887165162)) ;
#74505=CARTESIAN_POINT('Ctrl Pts',(-18.5957515114888,-24.5126399531591,
122.521477699572)) ;
#74506=CARTESIAN_POINT('Ctrl Pts',(-18.2138481636783,-24.7026776199941,
122.49341457571)) ;
#74507=CARTESIAN_POINT('Ctrl Pts',(-18.4529280643294,-24.5226885395753,
122.677100488762)) ;
#74508=CARTESIAN_POINT('Ctrl Pts',(-18.0737497674952,-24.7125704389585,
122.712471449069)) ;
#74509=CARTESIAN_POINT('Ctrl Pts',(-18.3408506079003,-24.5325813585398,
122.852345913931)) ;
#74510=CARTESIAN_POINT('Ctrl Pts',(-17.9721440403663,-24.7226415564883,
122.956790585532)) ;
#74511=CARTESIAN_POINT('Ctrl Pts',(-18.2595668744231,-24.5426524760696,
123.047801904658)) ;
#74512=CARTESIAN_POINT('Ctrl Pts',(-17.9156039986773,-24.7324572504544,
123.20851484051)) ;
#74513=CARTESIAN_POINT('Ctrl Pts',(-18.214336048054,-24.5524681700357,123.249180320883)) ;
#74514=CARTESIAN_POINT('Ctrl Pts',(-17.9029486724809,-24.7425236279517,
123.472689210433)) ;
#74515=CARTESIAN_POINT('Ctrl Pts',(-18.2042126493569,-24.562534547533,123.460520152789)) ;
#74516=CARTESIAN_POINT('Ctrl Pts',(-17.9358920954066,-24.7524226140335,
123.730795685737)) ;
#74517=CARTESIAN_POINT('Ctrl Pts',(-18.2305681821553,-24.5724335336148,
123.667004510187)) ;
#74518=CARTESIAN_POINT('Ctrl Pts',(-18.0142279453785,-24.7624767940271,
123.983068491414)) ;
#74519=CARTESIAN_POINT('Ctrl Pts',(-18.2932377609771,-24.5824877136083,
123.868822703197)) ;
#74520=CARTESIAN_POINT('Ctrl Pts',(-18.1327982652651,-24.7723476069598,
124.213846997065)) ;
#74521=CARTESIAN_POINT('Ctrl Pts',(-18.3880943171351,-24.592358526541,124.053444317472)) ;
#74522=CARTESIAN_POINT('Ctrl Pts',(-18.2927953165184,-24.7824215078136,
124.42468023211)) ;
#74523=CARTESIAN_POINT('Ctrl Pts',(-18.5160928152564,-24.6024324273948,
124.222110690457)) ;
#74524=CARTESIAN_POINT('Ctrl Pts',(-18.4819523062245,-24.7922416632002,
124.600316090987)) ;
#74525=CARTESIAN_POINT('Ctrl Pts',(-18.6674179941489,-24.6122525827815,
124.36261799151)) ;
#74526=CARTESIAN_POINT('Ctrl Pts',(-18.7041959808915,-24.8023203701525,
124.744270009399)) ;
#74527=CARTESIAN_POINT('Ctrl Pts',(-18.8452136184264,-24.6223312897337,
124.477780764093)) ;
#74528=CARTESIAN_POINT('Ctrl Pts',(-18.9426453969899,-24.8121719586913,
124.845254460317)) ;
#74529=CARTESIAN_POINT('Ctrl Pts',(-19.0359724337194,-24.6321828782725,
124.558567311492)) ;
#74530=CARTESIAN_POINT('Ctrl Pts',(-19.200521069124,-24.8222450752162,124.904809172644)) ;
#74531=CARTESIAN_POINT('Ctrl Pts',(-19.2422734477073,-24.6422559947975,
124.606210577257)) ;
#74532=CARTESIAN_POINT('Ctrl Pts',(-19.4588424041195,-24.8320875923121,
124.918328324864)) ;
#74533=CARTESIAN_POINT('Ctrl Pts',(-19.4489294152064,-24.6520985118933,
124.617025231616)) ;
#74534=CARTESIAN_POINT('Ctrl Pts',(-19.719255391812,-24.8420680538661,124.887225976223)) ;
#74535=CARTESIAN_POINT('Ctrl Pts',(-19.6572595128658,-24.6620789734473,
124.592142995155)) ;
#74536=CARTESIAN_POINT('Ctrl Pts',(-19.9711242826378,-24.8520863038568,
124.810604842159)) ;
#74537=CARTESIAN_POINT('Ctrl Pts',(-19.8587544824804,-24.6720972234381,
124.530845590783)) ;
#74538=CARTESIAN_POINT('Ctrl Pts',(-20.2029896411128,-24.8619704640506,
124.693474375269)) ;
#74539=CARTESIAN_POINT('Ctrl Pts',(-20.0442458164623,-24.6819813836318,
124.437141271385)) ;
#74540=CARTESIAN_POINT('Ctrl Pts',(-20.4147243951866,-24.8720356110256,
124.535001991893)) ;
#74541=CARTESIAN_POINT('Ctrl Pts',(-20.2136336325646,-24.6920465306068,
124.310362857701)) ;
#74542=CARTESIAN_POINT('Ctrl Pts',(-20.5918496187406,-24.8818774346664,
124.346514930606)) ;
#74543=CARTESIAN_POINT('Ctrl Pts',(-20.3553327465534,-24.7018883542476,
124.159573817455)) ;
#74544=CARTESIAN_POINT('Ctrl Pts',(-20.7368372685896,-24.8919069071272,
124.126420308685)) ;
#74545=CARTESIAN_POINT('Ctrl Pts',(-20.4713227600886,-24.7119178267085,
123.983497953276)) ;
#74546=CARTESIAN_POINT('Ctrl Pts',(-20.8407071585542,-24.9019337623892,
123.884255456022)) ;
#74547=CARTESIAN_POINT('Ctrl Pts',(-20.5544183607699,-24.7219446819705,
123.789765854984)) ;
#74548=CARTESIAN_POINT('Ctrl Pts',(-20.9004509563843,-24.9117770124998,
123.632574419161)) ;
#74549=CARTESIAN_POINT('Ctrl Pts',(-20.6022129291242,-24.731787932081,123.588422099066)) ;
#74550=CARTESIAN_POINT('Ctrl Pts',(-20.9162606113356,-24.9218254520829,
123.368993380641)) ;
#74551=CARTESIAN_POINT('Ctrl Pts',(-20.614860543706,-24.7418363716642,123.377557052921)) ;
#74552=CARTESIAN_POINT('Ctrl Pts',(-20.8859488524608,-24.9317749463308,
123.10929263775)) ;
#74553=CARTESIAN_POINT('Ctrl Pts',(-20.59061096289,-24.7517858659121,123.169796946132)) ;
#74554=CARTESIAN_POINT('Ctrl Pts',(-20.8120633746021,-24.9416828020568,
122.859612422506)) ;
#74555=CARTESIAN_POINT('Ctrl Pts',(-20.531502761985,-24.7616937216381,122.970053477872)) ;
#74556=CARTESIAN_POINT('Ctrl Pts',(-20.6939388265483,-24.9517422787068,
122.623150935592)) ;
#74557=CARTESIAN_POINT('Ctrl Pts',(-20.4370029110324,-24.771753198288,122.7808840852)) ;
#74558=CARTESIAN_POINT('Ctrl Pts',(-20.540217779766,-24.9615830881155,122.415150839265)) ;
#74559=CARTESIAN_POINT('Ctrl Pts',(-20.3140267650596,-24.7815940076967,
122.614484958291)) ;
#74560=CARTESIAN_POINT('Ctrl Pts',(-20.3487716521586,-24.9716452384163,
122.232796879452)) ;
#74561=CARTESIAN_POINT('Ctrl Pts',(-20.1608697005257,-24.7916561579975,
122.46860153275)) ;
#74562=CARTESIAN_POINT('Ctrl Pts',(-20.1319979379297,-24.9815423995388,
122.089055106635)) ;
#74563=CARTESIAN_POINT('Ctrl Pts',(-19.9874513995793,-24.8015533191201,
122.353608554069)) ;
#74564=CARTESIAN_POINT('Ctrl Pts',(-19.8931048762983,-24.9914735739429,
121.98399178358)) ;
#74565=CARTESIAN_POINT('Ctrl Pts',(-19.7963375692776,-24.8114844935241,
122.269557920393)) ;
#74566=CARTESIAN_POINT('Ctrl Pts',(-19.6366938542518,-25.0015157776679,
121.921591372293)) ;
#74567=CARTESIAN_POINT('Ctrl Pts',(-19.5912086257086,-24.8215266972492,
122.219637404033)) ;
#74568=CARTESIAN_POINT('Ctrl Pts',(-19.3774193320299,-25.0114023600983,
121.904731667658)) ;
#74569=CARTESIAN_POINT('Ctrl Pts',(-19.3837898885551,-24.8314132796796,
122.206149496955)) ;
#74570=CARTESIAN_POINT('Ctrl Pts',(-19.1163451180578,-25.0213957958467,
121.933019785977)) ;
#74571=CARTESIAN_POINT('Ctrl Pts',(-19.1749306450464,-24.8414067154279,
122.228779665525)) ;
#74572=CARTESIAN_POINT('Ctrl Pts',(-18.8653899853396,-25.0313402642048,
122.005933155613)) ;
#74573=CARTESIAN_POINT('Ctrl Pts',(-18.9741669200582,-24.8513511837861,
122.287109951159)) ;
#74574=CARTESIAN_POINT('Ctrl Pts',(-18.630508190403,-25.0412920804504,122.120959221041)) ;
#74575=CARTESIAN_POINT('Ctrl Pts',(-18.7862616983895,-24.8613030000317,
122.379130236719)) ;
#74576=CARTESIAN_POINT('Ctrl Pts',(-18.417510698376,-25.0513295165649,122.276526693795)) ;
#74577=CARTESIAN_POINT('Ctrl Pts',(-18.6158633904333,-24.8713404361461,
122.503584006888)) ;
#74578=CARTESIAN_POINT('Ctrl Pts',(-18.2373294886362,-25.0612144757412,
122.463677159513)) ;
#74579=CARTESIAN_POINT('Ctrl Pts',(-18.4717187211798,-24.8812253953225,
122.653303473347)) ;
#74580=CARTESIAN_POINT('Ctrl Pts',(-18.0904935272417,-25.0712125939532,
122.681519130297)) ;
#74581=CARTESIAN_POINT('Ctrl Pts',(-18.3542496121446,-24.8912235135344,
122.82757667031)) ;
#74582=CARTESIAN_POINT('Ctrl Pts',(-17.9843474113047,-25.0811335264651,
122.919675638683)) ;
#74583=CARTESIAN_POINT('Ctrl Pts',(-18.2693324840715,-24.9011444460464,
123.018101090549)) ;
#74584=CARTESIAN_POINT('Ctrl Pts',(-17.9203421284169,-25.0911748266872,
123.17565728928)) ;
#74585=CARTESIAN_POINT('Ctrl Pts',(-18.2181276878849,-24.9111857462685,
123.222886415152)) ;
#74586=CARTESIAN_POINT('Ctrl Pts',(-17.9020926497319,-25.1010817450772,
123.435363279086)) ;
#74587=CARTESIAN_POINT('Ctrl Pts',(-18.2035276252548,-24.9210926646584,
123.430650454951)) ;
#74588=CARTESIAN_POINT('Ctrl Pts',(-17.9285484880393,-25.1110175367862,
123.695123310098)) ;
#74589=CARTESIAN_POINT('Ctrl Pts',(-18.2246915312731,-24.9310284563675,
123.638458030304)) ;
#74590=CARTESIAN_POINT('Ctrl Pts',(-18.0007127841667,-25.1210584313641,
123.948921149968)) ;
#74591=CARTESIAN_POINT('Ctrl Pts',(-18.2824223843685,-24.9410693509454,
123.841496622937)) ;
#74592=CARTESIAN_POINT('Ctrl Pts',(-18.1139247514604,-25.130945633078,124.182800630708)) ;
#74593=CARTESIAN_POINT('Ctrl Pts',(-18.3729909704001,-24.9509565526592,
124.028599762318)) ;
#74594=CARTESIAN_POINT('Ctrl Pts',(-18.2672700656085,-25.1409379008396,
124.395937506913)) ;
#74595=CARTESIAN_POINT('Ctrl Pts',(-18.4956664766225,-24.9609488204208,
124.199109598826)) ;
#74596=CARTESIAN_POINT('Ctrl Pts',(-18.4545445264255,-25.1508864218614,
124.578379945121)) ;
#74597=CARTESIAN_POINT('Ctrl Pts',(-18.6454851891911,-24.9708973414426,
124.345063807)) ;
#74598=CARTESIAN_POINT('Ctrl Pts',(-18.6701593794366,-25.1608231954391,
124.725644505592)) ;
#74599=CARTESIAN_POINT('Ctrl Pts',(-18.8179761594363,-24.9808341150203,
124.462875886773)) ;
#74600=CARTESIAN_POINT('Ctrl Pts',(-18.9090898745942,-25.1708062435801,
124.83405904649)) ;
#74601=CARTESIAN_POINT('Ctrl Pts',(-19.0091199773882,-24.9908171631614,
124.549608297516)) ;
#74602=CARTESIAN_POINT('Ctrl Pts',(-19.1648198261258,-25.1808499511902,
124.899256681816)) ;
#74603=CARTESIAN_POINT('Ctrl Pts',(-19.2137038781447,-25.0008608707714,
124.601767252083)) ;
#74604=CARTESIAN_POINT('Ctrl Pts',(-19.4223677819922,-25.1906786443434,
124.919232914467)) ;
#74605=CARTESIAN_POINT('Ctrl Pts',(-19.4197410212802,-25.0106895639247,
124.617749120168)) ;
#74606=CARTESIAN_POINT('Ctrl Pts',(-19.6858526790718,-25.2007533934729,
124.893750955918)) ;
#74607=CARTESIAN_POINT('Ctrl Pts',(-19.6305293633067,-25.0207643130542,
124.59736453674)) ;
#74608=CARTESIAN_POINT('Ctrl Pts',(-19.9356579462485,-25.2106187192684,
124.824304856652)) ;
#74609=CARTESIAN_POINT('Ctrl Pts',(-19.8303729649698,-25.0306296388497,
124.541808869368)) ;
#74610=CARTESIAN_POINT('Ctrl Pts',(-20.1735854693504,-25.2206408936254,
124.711387601667)) ;
#74611=CARTESIAN_POINT('Ctrl Pts',(-20.0207155100975,-25.0406518132067,
124.451476093775)) ;
#74612=CARTESIAN_POINT('Ctrl Pts',(-20.388022656134,-25.2306669468323,124.558270853455)) ;
#74613=CARTESIAN_POINT('Ctrl Pts',(-20.1922658914238,-25.0506778664136,
124.328983483751)) ;
#74614=CARTESIAN_POINT('Ctrl Pts',(-20.5697163879502,-25.2405206436786,
124.373799671738)) ;
#74615=CARTESIAN_POINT('Ctrl Pts',(-20.3376209782561,-25.0605315632599,
124.181408007588)) ;
#74616=CARTESIAN_POINT('Ctrl Pts',(-20.7188606914662,-25.2504800484316,
124.158719634567)) ;
#74617=CARTESIAN_POINT('Ctrl Pts',(-20.4569372775264,-25.0704909680128,
124.009344986073)) ;
#74618=CARTESIAN_POINT('Ctrl Pts',(-20.8288249196023,-25.2605182941365,
123.918954163192)) ;
#74619=CARTESIAN_POINT('Ctrl Pts',(-20.5449097751489,-25.0805292137177,
123.817532999354)) ;
#74620=CARTESIAN_POINT('Ctrl Pts',(-20.8948612314061,-25.2703924782985,
123.667978712692)) ;
#74621=CARTESIAN_POINT('Ctrl Pts',(-20.5977398529196,-25.0904033978798,
123.616753747338)) ;
#74622=CARTESIAN_POINT('Ctrl Pts',(-20.9167246662131,-25.2804622614364,
123.404296836379)) ;
#74623=CARTESIAN_POINT('Ctrl Pts',(-20.6152318948764,-25.1004731810177,
123.405808073507)) ;
#74624=CARTESIAN_POINT('Ctrl Pts',(-20.8931748951374,-25.2902955164572,
123.146942101515)) ;
#74625=CARTESIAN_POINT('Ctrl Pts',(-20.5963934691841,-25.1103064360384,
123.199925185877)) ;
#74626=CARTESIAN_POINT('Ctrl Pts',(-20.8246646035839,-25.3003259425889,
122.892421113389)) ;
#74627=CARTESIAN_POINT('Ctrl Pts',(-20.5415866267975,-25.1203368621701,
122.996307948949)) ;
#74628=CARTESIAN_POINT('Ctrl Pts',(-20.7122848539865,-25.3103575547759,
122.653938383756)) ;
#74629=CARTESIAN_POINT('Ctrl Pts',(-20.4516839742709,-25.1303684743571,
122.805521151809)) ;
#74630=CARTESIAN_POINT('Ctrl Pts',(-20.5637225648763,-25.3201872516305,
122.442640422415)) ;
#74631=CARTESIAN_POINT('Ctrl Pts',(-20.3328358819854,-25.1401981712117,
122.636482800151)) ;
#74632=CARTESIAN_POINT('Ctrl Pts',(-20.3782914259856,-25.330176693533,122.256812973028)) ;
#74633=CARTESIAN_POINT('Ctrl Pts',(-20.1844921808869,-25.1501876131142,
122.487819833207)) ;
#74634=CARTESIAN_POINT('Ctrl Pts',(-20.1618642262866,-25.3402205855486,
122.105737144938)) ;
#74635=CARTESIAN_POINT('Ctrl Pts',(-20.0113511467643,-25.1602315051299,
122.366957925949)) ;
#74636=CARTESIAN_POINT('Ctrl Pts',(-19.9280150892586,-25.3500421473179,
121.996514020468)) ;
#74637=CARTESIAN_POINT('Ctrl Pts',(-19.8242733908789,-25.1700530668991,
122.279578452109)) ;
#74638=CARTESIAN_POINT('Ctrl Pts',(-19.6734892887017,-25.3600777189421,
121.927457195614)) ;
#74639=CARTESIAN_POINT('Ctrl Pts',(-19.6206531100156,-25.1800886385233,
122.224331363423)) ;
#74640=CARTESIAN_POINT('Ctrl Pts',(-19.4109364974855,-25.3701069932239,
121.904446478654)) ;
#74641=CARTESIAN_POINT('Ctrl Pts',(-19.410610970347,-25.1901179128051,122.205921274802)) ;
#74642=CARTESIAN_POINT('Ctrl Pts',(-19.1534256983001,-25.3799408303425,
121.926236678618)) ;
#74643=CARTESIAN_POINT('Ctrl Pts',(-19.2046030736676,-25.1999517499238,
122.223351721254)) ;
#74644=CARTESIAN_POINT('Ctrl Pts',(-18.8979973838584,-25.3899932264307,
121.993564432332)) ;
#74645=CARTESIAN_POINT('Ctrl Pts',(-19.0002598327071,-25.2100041460119,
122.277212317537)) ;
#74646=CARTESIAN_POINT('Ctrl Pts',(-18.6610161340468,-25.3999299933812,
122.103265136515)) ;
#74647=CARTESIAN_POINT('Ctrl Pts',(-18.8106744978957,-25.2199409129625,
122.364971228474)) ;
#74648=CARTESIAN_POINT('Ctrl Pts',(-18.4463642083807,-25.4098642283605,
122.251846102336)) ;
#74649=CARTESIAN_POINT('Ctrl Pts',(-18.6389522789307,-25.2298751479417,
122.483834331329)) ;
#74650=CARTESIAN_POINT('Ctrl Pts',(-18.2592125480837,-25.4198879916873,
122.437210228651)) ;
#74651=CARTESIAN_POINT('Ctrl Pts',(-18.4892297234926,-25.2398989112685,
122.632124410148)) ;
#74652=CARTESIAN_POINT('Ctrl Pts',(-18.1090179640619,-25.4297743330719,
122.649196677349)) ;
#74653=CARTESIAN_POINT('Ctrl Pts',(-18.3690729553001,-25.2497852526532,
122.801712072819)) ;
#74654=CARTESIAN_POINT('Ctrl Pts',(-17.9962023975987,-25.4397633818389,
122.88622883429)) ;
#74655=CARTESIAN_POINT('Ctrl Pts',(-18.2788188754758,-25.2597743014202,
122.991336884264)) ;
#74656=CARTESIAN_POINT('Ctrl Pts',(-17.926423247948,-25.4498046025363,123.140706746053)) ;
#74657=CARTESIAN_POINT('Ctrl Pts',(-18.2229938254166,-25.2698155221175,
123.194918814878)) ;
#74658=CARTESIAN_POINT('Ctrl Pts',(-17.9019779829779,-25.4596372427142,
123.397935296117)) ;
#74659=CARTESIAN_POINT('Ctrl Pts',(-18.2034358520446,-25.2796481622954,
123.400700720434)) ;
#74660=CARTESIAN_POINT('Ctrl Pts',(-17.9221548129474,-25.4696311720221,
123.659787613419)) ;
#74661=CARTESIAN_POINT('Ctrl Pts',(-18.2195753605606,-25.2896420916034,
123.610182627543)) ;
#74662=CARTESIAN_POINT('Ctrl Pts',(-17.9882634626665,-25.4796603797027,
123.914920831984)) ;
#74663=CARTESIAN_POINT('Ctrl Pts',(-18.2724604733462,-25.2996712992839,
123.814289688043)) ;
#74664=CARTESIAN_POINT('Ctrl Pts',(-18.0956149027315,-25.4895361914068,
124.151219574851)) ;
#74665=CARTESIAN_POINT('Ctrl Pts',(-18.3583396441264,-25.309547110988,124.003328991269)) ;
#74666=CARTESIAN_POINT('Ctrl Pts',(-18.2439323543506,-25.4995354183782,
124.368086107254)) ;
#74667=CARTESIAN_POINT('Ctrl Pts',(-18.4769919264261,-25.3195463379594,
124.176823257669)) ;
#74668=CARTESIAN_POINT('Ctrl Pts',(-18.4258762774548,-25.5094448995339,
124.554446462842)) ;
#74669=CARTESIAN_POINT('Ctrl Pts',(-18.6225453691918,-25.3294558191151,
124.325912669467)) ;
#74670=CARTESIAN_POINT('Ctrl Pts',(-18.640448928703,-25.5194981298348,124.708521880039)) ;
#74671=CARTESIAN_POINT('Ctrl Pts',(-18.7942023889779,-25.339509049416,124.449174675351)) ;
#74672=CARTESIAN_POINT('Ctrl Pts',(-18.8741769469214,-25.5293687463858,
124.821053391343)) ;
#74673=CARTESIAN_POINT('Ctrl Pts',(-18.981183490012,-25.3493796659671,124.539201487123)) ;
#74674=CARTESIAN_POINT('Ctrl Pts',(-19.1275355267195,-25.5393904081179,
124.89292358676)) ;
#74675=CARTESIAN_POINT('Ctrl Pts',(-19.1838697832088,-25.3594013276991,
124.596699645032)) ;
#74676=CARTESIAN_POINT('Ctrl Pts',(-19.3896325300269,-25.549413221299,124.919115026296)) ;
#74677=CARTESIAN_POINT('Ctrl Pts',(-19.3935471728134,-25.3694241408802,
124.617654797419)) ;
#74678=CARTESIAN_POINT('Ctrl Pts',(-19.6482244565254,-25.5592803857589,
124.900141299452)) ;
#74679=CARTESIAN_POINT('Ctrl Pts',(-19.6004204014471,-25.3792913053402,
124.602477906034)) ;
#74680=CARTESIAN_POINT('Ctrl Pts',(-19.9029765855987,-25.5692738279788,
124.836321404658)) ;
#74681=CARTESIAN_POINT('Ctrl Pts',(-19.8042225357259,-25.3892847475601,
124.551424072953)) ;
#74682=CARTESIAN_POINT('Ctrl Pts',(-20.143477500317,-25.5793055015792,124.728362358355)) ;
#74683=CARTESIAN_POINT('Ctrl Pts',(-19.9966241166619,-25.3993164211604,
124.465058726285)) ;
#74684=CARTESIAN_POINT('Ctrl Pts',(-20.3582214202601,-25.5891719366922,
124.583046155719)) ;
#74685=CARTESIAN_POINT('Ctrl Pts',(-20.1684200947875,-25.4091828562734,
124.348807744366)) ;
#74686=CARTESIAN_POINT('Ctrl Pts',(-20.5470220993923,-25.5991593872253,
124.400775187898)) ;
#74687=CARTESIAN_POINT('Ctrl Pts',(-20.3194620631275,-25.4191703068065,
124.202992587349)) ;
#74688=CARTESIAN_POINT('Ctrl Pts',(-20.7008042110465,-25.6091043170532,
124.189419968469)) ;
#74689=CARTESIAN_POINT('Ctrl Pts',(-20.4424893892085,-25.4291152366345,
124.033909833955)) ;
#74690=CARTESIAN_POINT('Ctrl Pts',(-20.8165443609965,-25.6191492121083,
123.95220482888)) ;
#74691=CARTESIAN_POINT('Ctrl Pts',(-20.535083449004,-25.4391601316896,123.844138651969)) ;
#74692=CARTESIAN_POINT('Ctrl Pts',(-20.8882445302655,-25.6290112737942,
123.703135751158)) ;
#74693=CARTESIAN_POINT('Ctrl Pts',(-20.5924455729224,-25.4490221933754,
123.644884316791)) ;
#74694=CARTESIAN_POINT('Ctrl Pts',(-20.916487089586,-25.639002996581,123.442107956853)) ;
#74695=CARTESIAN_POINT('Ctrl Pts',(-20.6150418055074,-25.4590139161623,
123.436062394398)) ;
#74696=CARTESIAN_POINT('Ctrl Pts',(-20.8989852871398,-25.648935210821,123.181683998681)) ;
#74697=CARTESIAN_POINT('Ctrl Pts',(-20.6010425682798,-25.4689461304023,
123.227723257091)) ;
#74698=CARTESIAN_POINT('Ctrl Pts',(-20.8370703424322,-25.6588745293867,
122.927926047639)) ;
#74699=CARTESIAN_POINT('Ctrl Pts',(-20.5515128122733,-25.478885448968,123.024716500619)) ;
#74700=CARTESIAN_POINT('Ctrl Pts',(-20.7307098427512,-25.6689187041626,
122.686357803577)) ;
#74701=CARTESIAN_POINT('Ctrl Pts',(-20.4664264490109,-25.4889296237439,
122.831461026835)) ;
#74702=CARTESIAN_POINT('Ctrl Pts',(-20.5866715410946,-25.6787892582276,
122.470638672561)) ;
#74703=CARTESIAN_POINT('Ctrl Pts',(-20.351197775471,-25.4988001778088,122.658884659411)) ;
#74704=CARTESIAN_POINT('Ctrl Pts',(-20.4061979029377,-25.6887542405818,
122.280888722107)) ;
#74705=CARTESIAN_POINT('Ctrl Pts',(-20.2068205491805,-25.508765160163,122.507083201106)) ;
#74706=CARTESIAN_POINT('Ctrl Pts',(-20.1938959519835,-25.6987849434716,
122.124661424596)) ;
#74707=CARTESIAN_POINT('Ctrl Pts',(-20.0369803529524,-25.5187958630528,
122.382099587623)) ;
#74708=CARTESIAN_POINT('Ctrl Pts',(-19.9610841220757,-25.7086772834968,
122.008927766467)) ;
#74709=CARTESIAN_POINT('Ctrl Pts',(-19.8507319966017,-25.528688203078,122.289510701505)) ;
#74710=CARTESIAN_POINT('Ctrl Pts',(-19.7077317559473,-25.7187305166567,
121.934171888527)) ;
#74711=CARTESIAN_POINT('Ctrl Pts',(-19.6480507770561,-25.538741436238,122.229703850899)) ;
#74712=CARTESIAN_POINT('Ctrl Pts',(-19.4496748815456,-25.7286117611335,
121.90488225927)) ;
#74713=CARTESIAN_POINT('Ctrl Pts',(-19.4416056279945,-25.5486226807147,
122.206269922949)) ;
#74714=CARTESIAN_POINT('Ctrl Pts',(-19.1865495494693,-25.7386448820045,
121.920889891574)) ;
#74715=CARTESIAN_POINT('Ctrl Pts',(-19.2311052788292,-25.5586558015858,
122.219073772921)) ;
#74716=CARTESIAN_POINT('Ctrl Pts',(-18.9339340957585,-25.7485260922796,
121.981208014926)) ;
#74717=CARTESIAN_POINT('Ctrl Pts',(-19.029012442334,-25.5685370118608,122.26732607008)) ;
#74718=CARTESIAN_POINT('Ctrl Pts',(-18.6913224502275,-25.7585881680489,
122.086259918681)) ;
#74719=CARTESIAN_POINT('Ctrl Pts',(-18.8349222926242,-25.5785990876302,
122.351365495269)) ;
#74720=CARTESIAN_POINT('Ctrl Pts',(-18.4750177695865,-25.7684452264307,
122.228841554616)) ;
#74721=CARTESIAN_POINT('Ctrl Pts',(-18.6618773148377,-25.5884561460119,
122.465428920654)) ;
#74722=CARTESIAN_POINT('Ctrl Pts',(-18.2838238476574,-25.7784397817196,
122.408857735646)) ;
#74723=CARTESIAN_POINT('Ctrl Pts',(-18.5089206655225,-25.5984507013009,
122.60944020259)) ;
#74724=CARTESIAN_POINT('Ctrl Pts',(-18.1277492565297,-25.7883656692552,
122.61789787757)) ;
#74725=CARTESIAN_POINT('Ctrl Pts',(-18.3840591928632,-25.6083765888364,
122.77667098702)) ;
#74726=CARTESIAN_POINT('Ctrl Pts',(-18.0091260993102,-25.7983906892504,
122.8531052283)) ;
#74727=CARTESIAN_POINT('Ctrl Pts',(-18.2891587030672,-25.6184016088317,
122.964835791046)) ;
#74728=CARTESIAN_POINT('Ctrl Pts',(-17.9340157761672,-25.8082880663541,
123.102124235162)) ;
#74729=CARTESIAN_POINT('Ctrl Pts',(-18.2290682857916,-25.6282989859354,
123.164050416227)) ;
#74730=CARTESIAN_POINT('Ctrl Pts',(-17.9024264991697,-25.818278303435,123.362756958183)) ;
#74731=CARTESIAN_POINT('Ctrl Pts',(-18.2037946795891,-25.6382892230162,
123.372556307197)) ;
#74732=CARTESIAN_POINT('Ctrl Pts',(-17.9171433201886,-25.8283149162438,
123.626094022944)) ;
#74733=CARTESIAN_POINT('Ctrl Pts',(-18.2155658929526,-25.648325835825,123.583225962692)) ;
#74734=CARTESIAN_POINT('Ctrl Pts',(-17.9758333008646,-25.8381647996618,
123.878206838387)) ;
#74735=CARTESIAN_POINT('Ctrl Pts',(-18.2625157992265,-25.658175719243,123.784916942111)) ;
#74736=CARTESIAN_POINT('Ctrl Pts',(-18.0784917994839,-25.8481684165642,
124.120189945123)) ;
#74737=CARTESIAN_POINT('Ctrl Pts',(-18.3446404819217,-25.6681793361455,
123.978504135792)) ;
#74738=CARTESIAN_POINT('Ctrl Pts',(-18.2215613396914,-25.8581578283294,
124.340338256961)) ;
#74739=CARTESIAN_POINT('Ctrl Pts',(-18.4590946437798,-25.6781687479106,
124.154624345632)) ;
#74740=CARTESIAN_POINT('Ctrl Pts',(-18.4012825634563,-25.8681765896742,
124.532704279354)) ;
#74741=CARTESIAN_POINT('Ctrl Pts',(-18.6028685580281,-25.6881875092555,
124.308517112761)) ;
#74742=CARTESIAN_POINT('Ctrl Pts',(-18.6786331146078,-25.8813952650552,
124.741942400083)) ;
#74743=CARTESIAN_POINT('Ctrl Pts',(-18.8247543705837,-25.7014061846365,
124.475917413394)) ;
#74744=CARTESIAN_POINT('Ctrl Pts',(-19.0063037436374,-25.8947055723,124.87503799074)) ;
#74745=CARTESIAN_POINT('Ctrl Pts',(-19.0869232033359,-25.7147164918812,
124.582399636663)) ;
#74746=CARTESIAN_POINT('Ctrl Pts',(-19.3515492792996,-25.907943238526,124.918059062517)) ;
#74747=CARTESIAN_POINT('Ctrl Pts',(-19.3630728386149,-25.7279541581072,
124.616808324183)) ;
#74748=CARTESIAN_POINT('Ctrl Pts',(-19.6119358669672,-25.9178629339367,
124.905712873571)) ;
#74749=CARTESIAN_POINT('Ctrl Pts',(-19.5713918638856,-25.7378738535179,
124.606935541768)) ;
#74750=CARTESIAN_POINT('Ctrl Pts',(-19.8695568707242,-25.9279158009352,
124.847282646944)) ;
#74751=CARTESIAN_POINT('Ctrl Pts',(-19.7774862246626,-25.7479267205165,
124.560193132552)) ;
#74752=CARTESIAN_POINT('Ctrl Pts',(-20.1084811471068,-25.9377712092645,
124.747272818654)) ;
#74753=CARTESIAN_POINT('Ctrl Pts',(-19.9686281873536,-25.7577821288458,
124.480186034087)) ;
#74754=CARTESIAN_POINT('Ctrl Pts',(-20.3306652048193,-25.9478098409411,
124.605081165744)) ;
#74755=CARTESIAN_POINT('Ctrl Pts',(-20.1463738336963,-25.7678207605223,
124.366438470224)) ;
#74756=CARTESIAN_POINT('Ctrl Pts',(-20.5876341489434,-25.9611120232081,
124.368071353077)) ;
#74757=CARTESIAN_POINT('Ctrl Pts',(-20.3519625615486,-25.7811229427894,
124.176812457001)) ;
#74758=CARTESIAN_POINT('Ctrl Pts',(-20.8234715239906,-25.977657036291,123.996893725418)) ;
#74759=CARTESIAN_POINT('Ctrl Pts',(-20.5406208335467,-25.7976679558722,
123.87990862136)) ;
#74760=CARTESIAN_POINT('Ctrl Pts',(-20.9191905980385,-25.9943090523672,
123.56485434144)) ;
#74761=CARTESIAN_POINT('Ctrl Pts',(-20.6172087980807,-25.8143199719484,
123.534214776845)) ;
#74762=CARTESIAN_POINT('Ctrl Pts',(-20.9040855807163,-26.0075321432724,
123.217655815584)) ;
#74763=CARTESIAN_POINT('Ctrl Pts',(-20.6051216995438,-25.8275430628537,
123.256506511511)) ;
#74764=CARTESIAN_POINT('Ctrl Pts',(-20.8481710289806,-26.0174931028318,
122.9619384918)) ;
#74765=CARTESIAN_POINT('Ctrl Pts',(-20.5603924152172,-25.837504022413,123.051921427646)) ;
#74766=CARTESIAN_POINT('Ctrl Pts',(-20.7477672744472,-26.0275178995829,
122.718386742836)) ;
#74767=CARTESIAN_POINT('Ctrl Pts',(-20.4800725252395,-25.8475288191641,
122.857083778402)) ;
#74768=CARTESIAN_POINT('Ctrl Pts',(-20.5619333818836,-26.0407423469787,
122.42467916469)) ;
#74769=CARTESIAN_POINT('Ctrl Pts',(-20.3313987756676,-25.8607532665599,
122.622107468328)) ;
#74770=CARTESIAN_POINT('Ctrl Pts',(-20.2373134507114,-26.0573761316778,
122.124643357332)) ;
#74771=CARTESIAN_POINT('Ctrl Pts',(-20.0717139940136,-25.877387051259,122.382085646915)) ;
#74772=CARTESIAN_POINT('Ctrl Pts',(-19.7495611854101,-26.0772787984027,
121.919792632178)) ;
#74773=CARTESIAN_POINT('Ctrl Pts',(-19.6815098776299,-25.897289717984,122.218198920366)) ;
#74774=CARTESIAN_POINT('Ctrl Pts',(-19.2213622812283,-26.0971790261846,
121.89299185719)) ;
#74775=CARTESIAN_POINT('Ctrl Pts',(-19.2589510054893,-25.9171899457658,
122.196756056214)) ;
#74776=CARTESIAN_POINT('Ctrl Pts',(-18.7151476741329,-26.1170965137161,
122.047840068811)) ;
#74777=CARTESIAN_POINT('Ctrl Pts',(-18.8539776981445,-25.9371074332973,
122.320631958508)) ;
#74778=CARTESIAN_POINT('Ctrl Pts',(-18.2916834898389,-26.137026039533,122.366086543257)) ;
#74779=CARTESIAN_POINT('Ctrl Pts',(-18.5152044325254,-25.9570369591142,
122.575227523537)) ;
#74780=CARTESIAN_POINT('Ctrl Pts',(-18.0018457090741,-26.1569883074192,
122.810521280974)) ;
#74781=CARTESIAN_POINT('Ctrl Pts',(-18.283332009678,-25.9769992270005,122.930774214087)) ;
#74782=CARTESIAN_POINT('Ctrl Pts',(-17.8814876927673,-26.1768785023714,
123.325213587116)) ;
#74783=CARTESIAN_POINT('Ctrl Pts',(-18.1870431423497,-25.9968894219527,
123.342528513262)) ;
#74784=CARTESIAN_POINT('Ctrl Pts',(-17.9426863607119,-26.1967687471177,
123.850425839063)) ;
#74785=CARTESIAN_POINT('Ctrl Pts',(-18.2360005788665,-26.016779666699,123.762699536368)) ;
#74786=CARTESIAN_POINT('Ctrl Pts',(-18.1825328725628,-26.2168431196802,
124.326942241142)) ;
#74787=CARTESIAN_POINT('Ctrl Pts',(-18.4278757324527,-26.0368540392614,
124.143912810045)) ;
#74788=CARTESIAN_POINT('Ctrl Pts',(-18.5649877789948,-26.2366284970405,
124.687956672243)) ;
#74789=CARTESIAN_POINT('Ctrl Pts',(-18.7338401401723,-26.0566394166217,
124.432727122548)) ;
#74790=CARTESIAN_POINT('Ctrl Pts',(-19.0512197803055,-26.2565903711076,
124.900124064246)) ;
#74791=CARTESIAN_POINT('Ctrl Pts',(-19.1228258509435,-26.0766012906889,
124.602461970491)) ;
#74792=CARTESIAN_POINT('Ctrl Pts',(-19.5812880978493,-26.2765703465981,
124.932395779839)) ;
#74793=CARTESIAN_POINT('Ctrl Pts',(-19.5468805975335,-26.0965812661794,
124.628280541388)) ;
#74794=CARTESIAN_POINT('Ctrl Pts',(-20.0865875254808,-26.296382776476,124.784090581371)) ;
#74795=CARTESIAN_POINT('Ctrl Pts',(-19.9511225306785,-26.1163936960573,
124.50963622777)) ;
#74796=CARTESIAN_POINT('Ctrl Pts',(-20.5148410357774,-26.3163628845663,
124.470248873514)) ;
#74797=CARTESIAN_POINT('Ctrl Pts',(-20.2937255891069,-26.1363738041476,
124.258562667596)) ;
#74798=CARTESIAN_POINT('Ctrl Pts',(-20.8089496481793,-26.3362572681636,
124.030690459084)) ;
#74799=CARTESIAN_POINT('Ctrl Pts',(-20.5290131148898,-26.1562681877448,
123.906914797705)) ;
#74800=CARTESIAN_POINT('Ctrl Pts',(-20.9360216456887,-26.3561841961408,
123.516657893159)) ;
#74801=CARTESIAN_POINT('Ctrl Pts',(-20.6306703947907,-26.1761951157221,
123.495687702575)) ;
#74802=CARTESIAN_POINT('Ctrl Pts',(-20.8808211229256,-26.376079053442,122.990653192989)) ;
#74803=CARTESIAN_POINT('Ctrl Pts',(-20.5865088182755,-26.1960899730233,
123.074882896028)) ;
#74804=CARTESIAN_POINT('Ctrl Pts',(-20.6473502027379,-26.3961182470457,
122.512000068549)) ;
#74805=CARTESIAN_POINT('Ctrl Pts',(-20.3997313810415,-26.2161291666269,
122.691961220065)) ;
#74806=CARTESIAN_POINT('Ctrl Pts',(-20.2682064550008,-26.4159582149564,
122.145440895257)) ;
#74807=CARTESIAN_POINT('Ctrl Pts',(-20.0964143290626,-26.2359691345377,
122.398713470548)) ;
#74808=CARTESIAN_POINT('Ctrl Pts',(-19.7855675978604,-26.4358730319205,
121.92824336016)) ;
#74809=CARTESIAN_POINT('Ctrl Pts',(-19.7103017055272,-26.2558839515018,
122.224956789686)) ;
#74810=CARTESIAN_POINT('Ctrl Pts',(-19.2570238059644,-26.4558152773168,
121.889095738651)) ;
#74811=CARTESIAN_POINT('Ctrl Pts',(-19.2874659515853,-26.275826196898,122.193640519728)) ;
#74812=CARTESIAN_POINT('Ctrl Pts',(-18.748249738838,-26.4756873254313,122.031335489846)) ;
#74813=CARTESIAN_POINT('Ctrl Pts',(-18.8804462675257,-26.2956982450125,
122.307434864793)) ;
#74814=CARTESIAN_POINT('Ctrl Pts',(-18.3160101802947,-26.4956983903854,
122.340952921537)) ;
#74815=CARTESIAN_POINT('Ctrl Pts',(-18.5346560494726,-26.3157093099666,
122.555130681776)) ;
#74816=CARTESIAN_POINT('Ctrl Pts',(-18.0174531568,-26.515509914689,122.774978345827)) ;
#74817=CARTESIAN_POINT('Ctrl Pts',(-18.2958118673303,-26.3355208342703,
122.902353753564)) ;
#74818=CARTESIAN_POINT('Ctrl Pts',(-17.8834572829533,-26.5356051266524,
123.291778439983)) ;
#74819=CARTESIAN_POINT('Ctrl Pts',(-18.188618039186,-26.3556160462336,123.315793821141)) ;
#74820=CARTESIAN_POINT('Ctrl Pts',(-17.9332038025589,-26.5553858505722,
123.815368387759)) ;
#74821=CARTESIAN_POINT('Ctrl Pts',(-18.2284182371962,-26.3753967701534,
123.734667085211)) ;
#74822=CARTESIAN_POINT('Ctrl Pts',(-18.1597535329201,-26.575376926215,124.295760856993)) ;
#74823=CARTESIAN_POINT('Ctrl Pts',(-18.409661050836,-26.3953878457962,124.118979676145)) ;
#74824=CARTESIAN_POINT('Ctrl Pts',(-18.5350790244708,-26.595258865258,124.667951356092)) ;
#74825=CARTESIAN_POINT('Ctrl Pts',(-18.7099242517618,-26.4152697848392,
124.416730225271)) ;
#74826=CARTESIAN_POINT('Ctrl Pts',(-19.0161267181929,-26.6152114697612,
124.890949085832)) ;
#74827=CARTESIAN_POINT('Ctrl Pts',(-19.0947641449975,-26.4352223893425,
124.595125248235)) ;
#74828=CARTESIAN_POINT('Ctrl Pts',(-19.5431138580718,-26.6351103384919,
124.936289536538)) ;
#74829=CARTESIAN_POINT('Ctrl Pts',(-19.5163546351924,-26.4551212580731,
124.631394176078)) ;
#74830=CARTESIAN_POINT('Ctrl Pts',(-20.0538241489815,-26.6550037383015,
124.79978424578)) ;
#74831=CARTESIAN_POINT('Ctrl Pts',(-19.9249224379141,-26.4750146578827,
124.522185551533)) ;
#74832=CARTESIAN_POINT('Ctrl Pts',(-20.4882718450487,-26.6749128691415,
124.497507103276)) ;
#74833=CARTESIAN_POINT('Ctrl Pts',(-20.2724781151579,-26.4949237887228,
124.280362392057)) ;
#74834=CARTESIAN_POINT('Ctrl Pts',(-20.7946862217622,-26.6949449689051,
124.062171882812)) ;
#74835=CARTESIAN_POINT('Ctrl Pts',(-20.5176077611612,-26.5149558884863,
123.932084425509)) ;
#74836=CARTESIAN_POINT('Ctrl Pts',(-20.9099487232185,-26.7114770420745,
123.638071483018)) ;
#74837=CARTESIAN_POINT('Ctrl Pts',(-20.6098098769218,-26.5314879616558,
123.592826514406)) ;
#74838=CARTESIAN_POINT('Ctrl Pts',(-20.9115489478564,-26.7248123826805,
123.287684923667)) ;
#74839=CARTESIAN_POINT('Ctrl Pts',(-20.6110911397521,-26.5448233022617,
123.312495827901)) ;
#74840=CARTESIAN_POINT('Ctrl Pts',(-20.8682561092861,-26.7346549412202,
123.032650001419)) ;
#74841=CARTESIAN_POINT('Ctrl Pts',(-20.5764556671409,-26.5546658608015,
123.108474233604)) ;
#74842=CARTESIAN_POINT('Ctrl Pts',(-20.7797708303451,-26.7447068480701,
122.783795004311)) ;
#74843=CARTESIAN_POINT('Ctrl Pts',(-20.5056588060069,-26.5647177676514,
122.909381558418)) ;
#74844=CARTESIAN_POINT('Ctrl Pts',(-20.6078481494065,-26.757955362461,122.48098979156)) ;
#74845=CARTESIAN_POINT('Ctrl Pts',(-20.368152466766,-26.5779662820423,122.667181160605)) ;
#74846=CARTESIAN_POINT('Ctrl Pts',(-20.2986718810033,-26.7745545374087,
122.166348506582)) ;
#74847=CARTESIAN_POINT('Ctrl Pts',(-20.120762032831,-26.59456545699,122.415419305003)) ;
#74848=CARTESIAN_POINT('Ctrl Pts',(-19.9009478345322,-26.7911433232038,
121.976048096969)) ;
#74849=CARTESIAN_POINT('Ctrl Pts',(-19.8026233502208,-26.6111542427851,
122.263209553901)) ;
#74850=CARTESIAN_POINT('Ctrl Pts',(-19.5580496300538,-26.8044191395458,
121.911724128116)) ;
#74851=CARTESIAN_POINT('Ctrl Pts',(-19.5282751818262,-26.624430059127,122.211739560136)) ;
#74852=CARTESIAN_POINT('Ctrl Pts',(-19.2959531359135,-26.8143929903396,
121.908486612998)) ;
#74853=CARTESIAN_POINT('Ctrl Pts',(-19.3186038165586,-26.6344039099208,
122.209154538032)) ;
#74854=CARTESIAN_POINT('Ctrl Pts',(-19.035911538622,-26.824422022432,121.951317775041)) ;
#74855=CARTESIAN_POINT('Ctrl Pts',(-19.1105694160277,-26.6444329420132,
122.243420903689)) ;
#74856=CARTESIAN_POINT('Ctrl Pts',(-18.7905877642868,-26.8343121479339,
122.037189061947)) ;
#74857=CARTESIAN_POINT('Ctrl Pts',(-18.9143114743061,-26.6543230675151,
122.312120264419)) ;
#74858=CARTESIAN_POINT('Ctrl Pts',(-18.56142280297,-26.8443046262054,122.165337469994)) ;
#74859=CARTESIAN_POINT('Ctrl Pts',(-18.7309805312086,-26.6643155457866,
122.414640877474)) ;
#74860=CARTESIAN_POINT('Ctrl Pts',(-18.3586851595701,-26.8542558413028,
122.330580371104)) ;
#74861=CARTESIAN_POINT('Ctrl Pts',(-18.5687918791563,-26.674266760884,122.546836944886)) ;
#74862=CARTESIAN_POINT('Ctrl Pts',(-18.1862556412877,-26.8643043430578,
122.53053785774)) ;
#74863=CARTESIAN_POINT('Ctrl Pts',(-18.4308500085545,-26.6843152626391,
122.706804337278)) ;
#74864=CARTESIAN_POINT('Ctrl Pts',(-18.0536640723902,-26.8741456926746,
122.752611956665)) ;
#74865=CARTESIAN_POINT('Ctrl Pts',(-18.3247786705187,-26.6941566122558,
122.884464800855)) ;
#74866=CARTESIAN_POINT('Ctrl Pts',(-17.9597894558871,-26.8841319836948,
122.997630523687)) ;
#74867=CARTESIAN_POINT('Ctrl Pts',(-18.2496811140076,-26.7041429032761,
123.080480402911)) ;
#74868=CARTESIAN_POINT('Ctrl Pts',(-17.9099883260882,-26.8940685954234,
123.254005646123)) ;
#74869=CARTESIAN_POINT('Ctrl Pts',(-18.2098424357147,-26.7140795150047,
123.285580874397)) ;
#74870=CARTESIAN_POINT('Ctrl Pts',(-17.9055405281583,-26.904118470791,123.51804154586)) ;
#74871=CARTESIAN_POINT('Ctrl Pts',(-18.2062864585873,-26.7241293903722,
123.496809585011)) ;
#74872=CARTESIAN_POINT('Ctrl Pts',(-17.9459982768416,-26.9139689293264,
123.773739288623)) ;
#74873=CARTESIAN_POINT('Ctrl Pts',(-18.2386548730221,-26.7339798489077,
123.70136733283)) ;
#74874=CARTESIAN_POINT('Ctrl Pts',(-18.0306120393503,-26.9239408662792,
124.021720774569)) ;
#74875=CARTESIAN_POINT('Ctrl Pts',(-18.3063479820366,-26.7439517858604,
123.89975170688)) ;
#74876=CARTESIAN_POINT('Ctrl Pts',(-18.1573679302454,-26.9339363232113,
124.251828560774)) ;
#74877=CARTESIAN_POINT('Ctrl Pts',(-18.4077546301214,-26.7539472427925,
124.083836797404)) ;
#74878=CARTESIAN_POINT('Ctrl Pts',(-18.322964634766,-26.9439691302644,124.456964358617)) ;
#74879=CARTESIAN_POINT('Ctrl Pts',(-18.540233729948,-26.7639800498456,124.24794399399)) ;
#74880=CARTESIAN_POINT('Ctrl Pts',(-18.518031277806,-26.9538290168543,124.627530239038)) ;
#74881=CARTESIAN_POINT('Ctrl Pts',(-18.6962883826648,-26.7738399364356,
124.384394886845)) ;
#74882=CARTESIAN_POINT('Ctrl Pts',(-18.7423698226373,-26.9638180974196,
124.763794005541)) ;
#74883=CARTESIAN_POINT('Ctrl Pts',(-18.8757603004552,-26.7838290170008,
124.493403950581)) ;
#74884=CARTESIAN_POINT('Ctrl Pts',(-18.9855793301348,-26.9737495766287,
124.858494603995)) ;
#74885=CARTESIAN_POINT('Ctrl Pts',(-19.07032857135,-26.79376049621,124.569162300801)) ;
#74886=CARTESIAN_POINT('Ctrl Pts',(-19.2428644372131,-26.9837354360747,
124.910233267547)) ;
#74887=CARTESIAN_POINT('Ctrl Pts',(-19.2761570014402,-26.8037463556559,
124.610551055388)) ;
#74888=CARTESIAN_POINT('Ctrl Pts',(-19.5065740592346,-26.9937735867218,
124.91607984277)) ;
#74889=CARTESIAN_POINT('Ctrl Pts',(-19.4871247473151,-26.8137845063031,
124.615226085904)) ;
#74890=CARTESIAN_POINT('Ctrl Pts',(-19.7624778086787,-27.0036216772263,
124.877322071488)) ;
#74891=CARTESIAN_POINT('Ctrl Pts',(-19.691847097787,-26.8236325968075,124.584217745267)) ;
#74892=CARTESIAN_POINT('Ctrl Pts',(-20.0130872707403,-27.0136825857442,
124.793163184931)) ;
#74893=CARTESIAN_POINT('Ctrl Pts',(-19.892334005724,-26.8336935053255,124.51688855541)) ;
#74894=CARTESIAN_POINT('Ctrl Pts',(-20.2414042797423,-27.0235774329022,
124.668672645379)) ;
#74895=CARTESIAN_POINT('Ctrl Pts',(-20.0749863296734,-26.8435883524835,
124.417294323175)) ;
#74896=CARTESIAN_POINT('Ctrl Pts',(-20.4459889975372,-27.0335191049473,
124.506241389313)) ;
#74897=CARTESIAN_POINT('Ctrl Pts',(-20.238652605061,-26.8535300245285,124.287347771796)) ;
#74898=CARTESIAN_POINT('Ctrl Pts',(-20.620444844537,-27.0435216320727,124.3095765436)) ;
#74899=CARTESIAN_POINT('Ctrl Pts',(-20.3782156448559,-26.863532551654,124.130014531869)) ;
#74900=CARTESIAN_POINT('Ctrl Pts',(-20.7581648056357,-27.0535564232602,
124.084711962455)) ;
#74901=CARTESIAN_POINT('Ctrl Pts',(-20.4883897705064,-26.8735673428414,
123.950121722146)) ;
#74902=CARTESIAN_POINT('Ctrl Pts',(-20.8533381772439,-27.0634013031193,
123.844121950427)) ;
#74903=CARTESIAN_POINT('Ctrl Pts',(-20.5645263213738,-26.8834122227005,
123.757649351723)) ;
#74904=CARTESIAN_POINT('Ctrl Pts',(-20.906507383153,-27.0733871837378,123.587189440389)) ;
#74905=CARTESIAN_POINT('Ctrl Pts',(-20.6070596196296,-26.893398103319,123.552103047888)) ;
#74906=CARTESIAN_POINT('Ctrl Pts',(-20.9144081115239,-27.083321906831,123.326185418477)) ;
#74907=CARTESIAN_POINT('Ctrl Pts',(-20.6133781382632,-26.9033328264122,
123.343300030194)) ;
#74908=CARTESIAN_POINT('Ctrl Pts',(-20.8761775035436,-27.0933797471422,
123.064696003681)) ;
#74909=CARTESIAN_POINT('Ctrl Pts',(-20.5827915712378,-26.9133906667234,
123.134108707124)) ;
#74910=CARTESIAN_POINT('Ctrl Pts',(-20.7954566741114,-27.1032002345387,
122.819537535235)) ;
#74911=CARTESIAN_POINT('Ctrl Pts',(-20.5182131694661,-26.9232111541199,
122.937983169382)) ;
#74912=CARTESIAN_POINT('Ctrl Pts',(-20.6708300596011,-27.1132606358838,
122.586414372797)) ;
#74913=CARTESIAN_POINT('Ctrl Pts',(-20.418510079688,-26.9332715554651,122.751485490579)) ;
#74914=CARTESIAN_POINT('Ctrl Pts',(-20.5094030853838,-27.1231916014367,
122.381316698567)) ;
#74915=CARTESIAN_POINT('Ctrl Pts',(-20.2893670916496,-26.943202521018,122.587408842451)) ;
#74916=CARTESIAN_POINT('Ctrl Pts',(-20.3150919759959,-27.1331304637732,
122.206830149634)) ;
#74917=CARTESIAN_POINT('Ctrl Pts',(-20.133917119692,-26.9531413833544,122.44782126066)) ;
#74918=CARTESIAN_POINT('Ctrl Pts',(-20.0924353594026,-27.1431161946993,
122.067902692441)) ;
#74919=CARTESIAN_POINT('Ctrl Pts',(-19.9557909146957,-26.9631271142806,
122.336681000983)) ;
#74920=CARTESIAN_POINT('Ctrl Pts',(-19.8480377025448,-27.1531405801268,
121.96964338509)) ;
#74921=CARTESIAN_POINT('Ctrl Pts',(-19.7602720483066,-26.9731514997081,
122.258075383028)) ;
#74922=CARTESIAN_POINT('Ctrl Pts',(-19.5934350819515,-27.1630438644801,
121.915568323327)) ;
#74923=CARTESIAN_POINT('Ctrl Pts',(-19.5565899913194,-26.9830547840613,
122.214817300124)) ;
#74924=CARTESIAN_POINT('Ctrl Pts',(-19.3292573389853,-27.1731038690581,
121.906468774186)) ;
#74925=CARTESIAN_POINT('Ctrl Pts',(-19.3452475890792,-26.9931147886393,
122.207539583563)) ;
#74926=CARTESIAN_POINT('Ctrl Pts',(-19.0730690560333,-27.1829471381272,
121.942410468998)) ;
#74927=CARTESIAN_POINT('Ctrl Pts',(-19.1402979129544,-27.0029580577084,
122.236294726187)) ;
#74928=CARTESIAN_POINT('Ctrl Pts',(-18.8231985706341,-27.1929377037349,
122.022885562064)) ;
#74929=CARTESIAN_POINT('Ctrl Pts',(-18.9404022136018,-27.0129486233161,
122.300676481672)) ;
#74930=CARTESIAN_POINT('Ctrl Pts',(-18.5925284415129,-27.2028658355137,
122.144814464939)) ;
#74931=CARTESIAN_POINT('Ctrl Pts',(-18.7558673038755,-27.022876755095,122.398221026076)) ;
#74932=CARTESIAN_POINT('Ctrl Pts',(-18.3850125184696,-27.2128537225946,
122.305545417233)) ;
#74933=CARTESIAN_POINT('Ctrl Pts',(-18.5898557473657,-27.0328646421759,
122.526807075092)) ;
#74934=CARTESIAN_POINT('Ctrl Pts',(-18.2080550367368,-27.2228896721633,
122.501085855597)) ;
#74935=CARTESIAN_POINT('Ctrl Pts',(-18.4482910618857,-27.0429005917445,
122.683240696432)) ;
#74936=CARTESIAN_POINT('Ctrl Pts',(-18.0698877944211,-27.2327445585421,
122.720150718089)) ;
#74937=CARTESIAN_POINT('Ctrl Pts',(-18.3377591347981,-27.0527554781234,
122.858492893348)) ;
#74938=CARTESIAN_POINT('Ctrl Pts',(-17.9701127119462,-27.24274397289,122.963197940048)) ;
#74939=CARTESIAN_POINT('Ctrl Pts',(-18.2579406678591,-27.0627548924712,
123.05293121135)) ;
#74940=CARTESIAN_POINT('Ctrl Pts',(-17.9143476220501,-27.2526391380805,
123.217227543741)) ;
#74941=CARTESIAN_POINT('Ctrl Pts',(-18.2133303139703,-27.0726500576617,
123.256154668995)) ;
#74942=CARTESIAN_POINT('Ctrl Pts',(-17.9033877647494,-27.2626994567724,
123.481339637187)) ;
#74943=CARTESIAN_POINT('Ctrl Pts',(-18.2045640578609,-27.0827103763537,
123.467444605589)) ;
#74944=CARTESIAN_POINT('Ctrl Pts',(-17.9375767428716,-27.2725495885485,
123.737946697379)) ;
#74945=CARTESIAN_POINT('Ctrl Pts',(-18.2319167231407,-27.0925605081298,
123.672729209851)) ;
#74946=CARTESIAN_POINT('Ctrl Pts',(-18.016630672151,-27.2825801589988,123.989393136754)) ;
#74947=CARTESIAN_POINT('Ctrl Pts',(-18.2951613035429,-27.10259107858,123.873885960265)) ;
#74948=CARTESIAN_POINT('Ctrl Pts',(-18.1384764759908,-27.2925943096716,
124.222663794545)) ;
#74949=CARTESIAN_POINT('Ctrl Pts',(-18.3926393637792,-27.1126052292528,
124.060501732075)) ;
#74950=CARTESIAN_POINT('Ctrl Pts',(-18.2966929164061,-27.302487243217,124.428958569304)) ;
#74951=CARTESIAN_POINT('Ctrl Pts',(-18.5192133357134,-27.1224981627982,
124.225536119169)) ;
#74952=CARTESIAN_POINT('Ctrl Pts',(-18.4899718703588,-27.3124767572072,
124.606563738804)) ;
#74953=CARTESIAN_POINT('Ctrl Pts',(-18.673837373234,-27.1324876767885,124.367619065612)) ;
#74954=CARTESIAN_POINT('Ctrl Pts',(-18.7103215045475,-27.3224305278597,
124.747585098893)) ;
#74955=CARTESIAN_POINT('Ctrl Pts',(-18.8501175596139,-27.1424414474409,
124.480434760865)) ;
#74956=CARTESIAN_POINT('Ctrl Pts',(-18.9541222140614,-27.3324782965202,
124.848911596921)) ;
#74957=CARTESIAN_POINT('Ctrl Pts',(-19.0451588376447,-27.1524892161015,
124.561494652999)) ;
#74958=CARTESIAN_POINT('Ctrl Pts',(-19.2065092981339,-27.3423200229601,
124.905498198079)) ;
#74959=CARTESIAN_POINT('Ctrl Pts',(-19.2470678872194,-27.1623309425413,
124.606762343776)) ;
#74960=CARTESIAN_POINT('Ctrl Pts',(-19.4685730602029,-27.3523055397828,
124.918145049044)) ;
#74961=CARTESIAN_POINT('Ctrl Pts',(-19.456718762585,-27.172316459364,124.616878517439)) ;
#74962=CARTESIAN_POINT('Ctrl Pts',(-19.7277379052748,-27.3622448714784,
124.88533514878)) ;
#74963=CARTESIAN_POINT('Ctrl Pts',(-19.6640500453479,-27.1822557910596,
124.590629385903)) ;
#74964=CARTESIAN_POINT('Ctrl Pts',(-19.9797167083785,-27.3722846411759,
124.807206664795)) ;
#74965=CARTESIAN_POINT('Ctrl Pts',(-19.8656328181808,-27.1922955607571,
124.528125331113)) ;
#74966=CARTESIAN_POINT('Ctrl Pts',(-20.2108513393377,-27.3821728024247,
124.68843293536)) ;
#74967=CARTESIAN_POINT('Ctrl Pts',(-20.0505392887375,-27.2021837220059,
124.433105562087)) ;
#74968=CARTESIAN_POINT('Ctrl Pts',(-20.4202523049832,-27.392162356927,124.530127299202)) ;
#74969=CARTESIAN_POINT('Ctrl Pts',(-20.2180592277372,-27.2121732765083,
124.306460234651)) ;
#74970=CARTESIAN_POINT('Ctrl Pts',(-20.5982841261792,-27.4021207714507,
124.338329003552)) ;
#74971=CARTESIAN_POINT('Ctrl Pts',(-20.360483568371,-27.222131691032,124.153021035403)) ;
#74972=CARTESIAN_POINT('Ctrl Pts',(-20.7400208953104,-27.4120206842801,
124.120151747185)) ;
#74973=CARTESIAN_POINT('Ctrl Pts',(-20.473871715113,-27.2320316038613,123.9784792444)) ;
#74974=CARTESIAN_POINT('Ctrl Pts',(-20.8431437131481,-27.42206738393,123.877134998713)) ;
#74975=CARTESIAN_POINT('Ctrl Pts',(-20.5563690459131,-27.2420783035112,
123.784065268537)) ;
#74976=CARTESIAN_POINT('Ctrl Pts',(-20.9018126856144,-27.4319672442356,
123.623637353361)) ;
#74977=CARTESIAN_POINT('Ctrl Pts',(-20.6033030544183,-27.2519781638168,
123.581267614642)) ;
#74978=CARTESIAN_POINT('Ctrl Pts',(-20.9158681862784,-27.442018648441,123.359908517842)) ;
#74979=CARTESIAN_POINT('Ctrl Pts',(-20.614546450276,-27.2620295680223,123.370284295332)) ;
#74980=CARTESIAN_POINT('Ctrl Pts',(-20.8845444216374,-27.4518996853622,
123.102102763096)) ;
#74981=CARTESIAN_POINT('Ctrl Pts',(-20.5894865476393,-27.2719106049434,
123.164040624998)) ;
#74982=CARTESIAN_POINT('Ctrl Pts',(-20.8083897018566,-27.4618995175397,
122.850639705385)) ;
#74983=CARTESIAN_POINT('Ctrl Pts',(-20.5285619312095,-27.2819104371209,
122.962870552448)) ;
#74984=CARTESIAN_POINT('Ctrl Pts',(-20.6908521996754,-27.4718175205245,
122.617961007271)) ;
#74985=CARTESIAN_POINT('Ctrl Pts',(-20.43453143348,-27.2918284401058,122.776728527516)) ;
#74986=CARTESIAN_POINT('Ctrl Pts',(-20.5325862277166,-27.4818688263991,
122.406544566077)) ;
#74987=CARTESIAN_POINT('Ctrl Pts',(-20.3079178321186,-27.3018797459804,
122.607595752983)) ;
#74988=CARTESIAN_POINT('Ctrl Pts',(-20.3436360268456,-27.4917386497907,
122.228783160623)) ;
#74989=CARTESIAN_POINT('Ctrl Pts',(-20.1567577854576,-27.3117495693719,
122.465387842878)) ;
#74990=CARTESIAN_POINT('Ctrl Pts',(-20.1222882553829,-27.501812815841,122.083664260609)) ;
#74991=CARTESIAN_POINT('Ctrl Pts',(-19.9796788329855,-27.3218237354222,
122.349293214515)) ;
#74992=CARTESIAN_POINT('Ctrl Pts',(-19.8852542608769,-27.5116328999826,
121.981478175985)) ;
#74993=CARTESIAN_POINT('Ctrl Pts',(-19.7900524902871,-27.3316438195639,
122.267545514143)) ;
#74994=CARTESIAN_POINT('Ctrl Pts',(-19.6276445348862,-27.5217116267184,
121.920220233183)) ;
#74995=CARTESIAN_POINT('Ctrl Pts',(-19.5839641856869,-27.3417225462997,
122.218539730451)) ;
#74996=CARTESIAN_POINT('Ctrl Pts',(-19.3691479103159,-27.531563207368,121.904877852265)) ;
#74997=CARTESIAN_POINT('Ctrl Pts',(-19.3771679014181,-27.3515741269492,
122.206266540335)) ;
#74998=CARTESIAN_POINT('Ctrl Pts',(-19.1062132173392,-27.5416363356664,
121.935078087931)) ;
#74999=CARTESIAN_POINT('Ctrl Pts',(-19.1668198669398,-27.3616472552476,
122.230427363407)) ;
#75000=CARTESIAN_POINT('Ctrl Pts',(-18.8582685979717,-27.5514788135578,
122.008806224797)) ;
#75001=CARTESIAN_POINT('Ctrl Pts',(-18.9684654319779,-27.3714897331391,
122.289410133124)) ;
#75002=CARTESIAN_POINT('Ctrl Pts',(-18.6232876860995,-27.5614594201559,
122.125286522792)) ;
#75003=CARTESIAN_POINT('Ctrl Pts',(-18.7804810973601,-27.3814703397371,
122.382594611719)) ;
#75004=CARTESIAN_POINT('Ctrl Pts',(-18.411600270402,-27.5714771291747,122.281782687908)) ;
#75005=CARTESIAN_POINT('Ctrl Pts',(-18.6111314675826,-27.3914880487559,
122.507791959957)) ;
#75006=CARTESIAN_POINT('Ctrl Pts',(-18.2323009870083,-27.5813633082121,
122.469819398484)) ;
#75007=CARTESIAN_POINT('Ctrl Pts',(-18.4676929146779,-27.4013742277934,
122.65822097498)) ;
#75008=CARTESIAN_POINT('Ctrl Pts',(-18.085888722091,-27.5914209207844,122.689836404028)) ;
#75009=CARTESIAN_POINT('Ctrl Pts',(-18.3505632824027,-27.4114318403657,
122.834234999918)) ;
#75010=CARTESIAN_POINT('Ctrl Pts',(-17.9817726806253,-27.6012973141566,
122.92759672565)) ;
#75011=CARTESIAN_POINT('Ctrl Pts',(-18.2672711670262,-27.4213082337378,
123.024442556299)) ;
#75012=CARTESIAN_POINT('Ctrl Pts',(-17.9191542664928,-27.611292342307,123.182674524729)) ;
#75013=CARTESIAN_POINT('Ctrl Pts',(-18.2171766775005,-27.4313032618883,
123.228504708676)) ;
#75014=CARTESIAN_POINT('Ctrl Pts',(-17.9021807329036,-27.621313089153,123.445473162293)) ;
#75015=CARTESIAN_POINT('Ctrl Pts',(-18.2035981738734,-27.4413240087343,
123.4387436757)) ;
#75016=CARTESIAN_POINT('Ctrl Pts',(-17.9304488696092,-27.6312151578194,
123.704146901857)) ;
#75017=CARTESIAN_POINT('Ctrl Pts',(-18.2262128505501,-27.4512260774006,
123.645681876394)) ;
#75018=CARTESIAN_POINT('Ctrl Pts',(-18.0034825911489,-27.6412058976391,
123.956332064163)) ;
#75019=CARTESIAN_POINT('Ctrl Pts',(-18.2846399233845,-27.4612168172203,
123.847429782292)) ;
#75020=CARTESIAN_POINT('Ctrl Pts',(-18.1190427861828,-27.6511690938494,
124.191258163487)) ;
#75021=CARTESIAN_POINT('Ctrl Pts',(-18.3770881012001,-27.4711800134306,
124.035370248739)) ;
#75022=CARTESIAN_POINT('Ctrl Pts',(-18.2722240570059,-27.6610732781495,
124.401708795439)) ;
#75023=CARTESIAN_POINT('Ctrl Pts',(-18.4996327056077,-27.4810841977308,
124.203730123677)) ;
#75024=CARTESIAN_POINT('Ctrl Pts',(-18.4626903999786,-27.6711337385404,
124.585014918557)) ;
#75025=CARTESIAN_POINT('Ctrl Pts',(-18.6520060497622,-27.4911446581216,
124.350375149966)) ;
#75026=CARTESIAN_POINT('Ctrl Pts',(-18.6771667745234,-27.6809742844111,
124.729554078356)) ;
#75027=CARTESIAN_POINT('Ctrl Pts',(-18.8235861793774,-27.5009852039924,
124.466005811902)) ;
#75028=CARTESIAN_POINT('Ctrl Pts',(-18.9186090603033,-27.6910365051229,
124.837307374899)) ;
#75029=CARTESIAN_POINT('Ctrl Pts',(-19.016740247443,-27.5110474247042,124.552208638131)) ;
#75030=CARTESIAN_POINT('Ctrl Pts',(-19.1709926750381,-27.7009336481395,
124.900195583819)) ;
#75031=CARTESIAN_POINT('Ctrl Pts',(-19.2186463603094,-27.5209445677207,
124.602519015299)) ;
#75032=CARTESIAN_POINT('Ctrl Pts',(-19.4312729665499,-27.7108648245567,
124.919233320741)) ;
#75033=CARTESIAN_POINT('Ctrl Pts',(-19.4268700019089,-27.5308757441379,
124.617749388828)) ;
#75034=CARTESIAN_POINT('Ctrl Pts',(-19.6937795869066,-27.7209070383353,
124.892204557347)) ;
#75035=CARTESIAN_POINT('Ctrl Pts',(-19.636875479684,-27.5409179579165,124.59612651213)) ;
#75036=CARTESIAN_POINT('Ctrl Pts',(-19.9437421483917,-27.730793578538,124.821306255777)) ;
#75037=CARTESIAN_POINT('Ctrl Pts',(-19.836844746594,-27.5508044981193,124.539408302028)) ;
#75038=CARTESIAN_POINT('Ctrl Pts',(-20.1802824076589,-27.7407871731435,
124.707252644215)) ;
#75039=CARTESIAN_POINT('Ctrl Pts',(-20.0260769445174,-27.5607980927247,
124.448165758018)) ;
#75040=CARTESIAN_POINT('Ctrl Pts',(-20.3923713221188,-27.7507310483009,
124.554570637496)) ;
#75041=CARTESIAN_POINT('Ctrl Pts',(-20.1957478479467,-27.5707419678822,
124.326020684454)) ;
#75042=CARTESIAN_POINT('Ctrl Pts',(-20.5752568934458,-27.7606915844158,
124.36733113008)) ;
#75043=CARTESIAN_POINT('Ctrl Pts',(-20.3420563159796,-27.5807025039971,
124.176229618266)) ;
#75044=CARTESIAN_POINT('Ctrl Pts',(-20.7235437791157,-27.7706881877385,
124.150451479932)) ;
#75045=CARTESIAN_POINT('Ctrl Pts',(-20.4606861037265,-27.5906991073198,
124.002726235317)) ;
#75046=CARTESIAN_POINT('Ctrl Pts',(-20.8319614751278,-27.780721270693,123.910121632743)) ;
#75047=CARTESIAN_POINT('Ctrl Pts',(-20.5474206058342,-27.6007321902743,
123.810462391625)) ;
#75048=CARTESIAN_POINT('Ctrl Pts',(-20.8961417941219,-27.7905724393946,
123.659328927906)) ;
#75049=CARTESIAN_POINT('Ctrl Pts',(-20.5987649851893,-27.6105833589758,
123.609829391344)) ;
#75050=CARTESIAN_POINT('Ctrl Pts',(-20.9167937428993,-27.8005349300935,
123.398350225033)) ;
#75051=CARTESIAN_POINT('Ctrl Pts',(-20.6152871158748,-27.6205458496747,
123.401046845239)) ;
#75052=CARTESIAN_POINT('Ctrl Pts',(-20.8913248728569,-27.8105633585112,
123.13603219385)) ;
#75053=CARTESIAN_POINT('Ctrl Pts',(-20.5949125321571,-27.6305742780925,
123.191192291486)) ;
#75054=CARTESIAN_POINT('Ctrl Pts',(-20.8216156441421,-27.8204737258758,
122.88511292039)) ;
#75055=CARTESIAN_POINT('Ctrl Pts',(-20.5391458591745,-27.640484645457,122.990457403175)) ;
#75056=CARTESIAN_POINT('Ctrl Pts',(-20.7097290522981,-27.8304085934909,
122.649216253088)) ;
#75057=CARTESIAN_POINT('Ctrl Pts',(-20.4496374549925,-27.6504195130721,
122.801740241644)) ;
#75058=CARTESIAN_POINT('Ctrl Pts',(-20.5567753118264,-27.8404497354699,
122.434208642575)) ;
#75059=CARTESIAN_POINT('Ctrl Pts',(-20.3272749058312,-27.6604606550512,
122.629733654314)) ;
#75060=CARTESIAN_POINT('Ctrl Pts',(-20.3718067249568,-27.8503368716731,
122.251718186842)) ;
#75061=CARTESIAN_POINT('Ctrl Pts',(-20.1793011160621,-27.6703477912543,
122.483741378946)) ;
#75062=CARTESIAN_POINT('Ctrl Pts',(-20.1559638842392,-27.8603291540765,
122.102205529712)) ;
#75063=CARTESIAN_POINT('Ctrl Pts',(-20.006627433317,-27.6803400736577,122.364130687556)) ;
#75064=CARTESIAN_POINT('Ctrl Pts',(-19.9184230348572,-27.8702776820417,
121.992974547552)) ;
#75065=CARTESIAN_POINT('Ctrl Pts',(-19.816595474273,-27.6902886016229,122.276745372545)) ;
#75066=CARTESIAN_POINT('Ctrl Pts',(-19.6659531803029,-27.8802144132038,
121.926377817736)) ;
#75067=CARTESIAN_POINT('Ctrl Pts',(-19.6146203057764,-27.7002253327851,
122.223467276849)) ;
#75068=CARTESIAN_POINT('Ctrl Pts',(-19.4045120642445,-27.8901976240638,
121.904196807102)) ;
#75069=CARTESIAN_POINT('Ctrl Pts',(-19.4054676973117,-27.710208543645,122.205721541653)) ;
#75070=CARTESIAN_POINT('Ctrl Pts',(-19.1417251311508,-27.9002407232137,
121.928354401178)) ;
#75071=CARTESIAN_POINT('Ctrl Pts',(-19.1952379245654,-27.7202516427949,
122.225046799241)) ;
#75072=CARTESIAN_POINT('Ctrl Pts',(-18.8922932247539,-27.9100716874885,
121.99576525242)) ;
#75073=CARTESIAN_POINT('Ctrl Pts',(-18.9956932551907,-27.7300826070698,
122.278974240053)) ;
#75074=CARTESIAN_POINT('Ctrl Pts',(-18.6525836804563,-27.9201445398745,
122.107953193287)) ;
#75075=CARTESIAN_POINT('Ctrl Pts',(-18.8039248906843,-27.7401554594558,
122.368723808351)) ;
#75076=CARTESIAN_POINT('Ctrl Pts',(-18.4404518361737,-27.9300086675863,
122.256983728399)) ;
#75077=CARTESIAN_POINT('Ctrl Pts',(-18.6342195866533,-27.7500195871675,
122.487946889381)) ;
#75078=CARTESIAN_POINT('Ctrl Pts',(-18.2540538809993,-27.9400308697212,
122.44303741663)) ;
#75079=CARTESIAN_POINT('Ctrl Pts',(-18.4851003818533,-27.7600417893024,
122.636789047312)) ;
#75080=CARTESIAN_POINT('Ctrl Pts',(-18.1032133229572,-27.9500580626896,
122.659116134861)) ;
#75081=CARTESIAN_POINT('Ctrl Pts',(-18.3644270759834,-27.7700689822708,
122.809651490149)) ;
#75082=CARTESIAN_POINT('Ctrl Pts',(-17.9937284542524,-27.9599136566566,
122.893810711262)) ;
#75083=CARTESIAN_POINT('Ctrl Pts',(-18.2768385935525,-27.7799245762378,
122.997405800576)) ;
#75084=CARTESIAN_POINT('Ctrl Pts',(-17.9252066476934,-27.9698708285219,
123.146353412753)) ;
#75085=CARTESIAN_POINT('Ctrl Pts',(-18.2220200039114,-27.7898817481031,
123.199439298674)) ;
#75086=CARTESIAN_POINT('Ctrl Pts',(-17.901836392515,-27.9799096725203,123.409110487333)) ;
#75087=CARTESIAN_POINT('Ctrl Pts',(-18.2033226182715,-27.7999205921015,
123.409644963665)) ;
#75088=CARTESIAN_POINT('Ctrl Pts',(-17.9236207436756,-27.9897836963958,
123.667708642631)) ;
#75089=CARTESIAN_POINT('Ctrl Pts',(-18.2207487591916,-27.8097946159771,
123.616522787693)) ;
#75090=CARTESIAN_POINT('Ctrl Pts',(-17.9912807796394,-27.9998535223862,
123.923499029273)) ;
#75091=CARTESIAN_POINT('Ctrl Pts',(-18.2748756263371,-27.8198644419675,
123.821155692994)) ;
#75092=CARTESIAN_POINT('Ctrl Pts',(-18.0996170115051,-28.0096867662835,
124.158124720486)) ;
#75093=CARTESIAN_POINT('Ctrl Pts',(-18.3615429995661,-27.8296976858648,
124.008855863308)) ;
#75094=CARTESIAN_POINT('Ctrl Pts',(-18.2493713827489,-28.0197171940566,
124.375030745344)) ;
#75095=CARTESIAN_POINT('Ctrl Pts',(-18.481345335379,-27.8397281136378,124.182381569428)) ;
#75096=CARTESIAN_POINT('Ctrl Pts',(-18.4350962680319,-28.0297488108017,
124.562139179314)) ;
#75097=CARTESIAN_POINT('Ctrl Pts',(-18.6299243679393,-27.8497597303829,
124.332069278655)) ;
#75098=CARTESIAN_POINT('Ctrl Pts',(-18.6458160519493,-28.0395784877824,
124.71151934182)) ;
#75099=CARTESIAN_POINT('Ctrl Pts',(-18.798498550654,-27.8595894073637,124.451573974288)) ;
#75100=CARTESIAN_POINT('Ctrl Pts',(-18.8827549500169,-28.0495680046223,
124.824558143957)) ;
#75101=CARTESIAN_POINT('Ctrl Pts',(-18.9880488657586,-27.8695789242036,
124.542006370576)) ;
#75102=CARTESIAN_POINT('Ctrl Pts',(-19.1372585886955,-28.0596116167621,
124.894470815624)) ;
#75103=CARTESIAN_POINT('Ctrl Pts',(-19.1916515109275,-27.8796225363434,
124.597937922925)) ;
#75104=CARTESIAN_POINT('Ctrl Pts',(-19.3942099817869,-28.0694342230974,
124.919127791783)) ;
#75105=CARTESIAN_POINT('Ctrl Pts',(-19.3972114824336,-27.8894451426787,
124.617664945199)) ;
#75106=CARTESIAN_POINT('Ctrl Pts',(-19.6572218646188,-28.0794724529966,
124.898947663113)) ;
#75107=CARTESIAN_POINT('Ctrl Pts',(-19.6076212137935,-27.8994833725779,
124.601522486604)) ;
#75108=CARTESIAN_POINT('Ctrl Pts',(-19.9119170104827,-28.0894834877886,
124.832984826459)) ;
#75109=CARTESIAN_POINT('Ctrl Pts',(-19.8113776795567,-27.9094944073698,
124.548753715423)) ;
#75110=CARTESIAN_POINT('Ctrl Pts',(-20.1487320477666,-28.0993812187557,
124.725423875362)) ;
#75111=CARTESIAN_POINT('Ctrl Pts',(-20.000829845105,-27.919392138337,124.462706670356)) ;
#75112=CARTESIAN_POINT('Ctrl Pts',(-20.3654611749056,-28.1093708466062,
124.577295140872)) ;
#75113=CARTESIAN_POINT('Ctrl Pts',(-20.1742139780183,-27.9293817661874,
124.344205147162)) ;
#75114=CARTESIAN_POINT('Ctrl Pts',(-20.5524779416737,-28.1193266370522,
124.394341663495)) ;
#75115=CARTESIAN_POINT('Ctrl Pts',(-20.3238283305594,-27.9393375566334,
124.197843770989)) ;
#75116=CARTESIAN_POINT('Ctrl Pts',(-20.7048656205572,-28.1292540356142,
124.182581520331)) ;
#75117=CARTESIAN_POINT('Ctrl Pts',(-20.4457396528893,-27.9492649551955,
124.028437013102)) ;
#75118=CARTESIAN_POINT('Ctrl Pts',(-20.8192132352062,-28.1392796307241,
123.945237856625)) ;
#75119=CARTESIAN_POINT('Ctrl Pts',(-20.5372193152296,-27.9592905503054,
123.838562820331)) ;
#75120=CARTESIAN_POINT('Ctrl Pts',(-20.8897744388912,-28.1491654813937,
123.695212486586)) ;
#75121=CARTESIAN_POINT('Ctrl Pts',(-20.5936698151312,-27.9691764009749,
123.638543566476)) ;
#75122=CARTESIAN_POINT('Ctrl Pts',(-20.916742686365,-28.1591546612379,123.434089007644)) ;
#75123=CARTESIAN_POINT('Ctrl Pts',(-20.6152462522755,-27.9791655808191,
123.429645100009)) ;
#75124=CARTESIAN_POINT('Ctrl Pts',(-20.8973138530435,-28.1691958483415,
123.170934263107)) ;
#75125=CARTESIAN_POINT('Ctrl Pts',(-20.5997049495287,-27.9892067679227,
123.219121101024)) ;
#75126=CARTESIAN_POINT('Ctrl Pts',(-20.8342467262593,-28.1790284918174,
122.920361624819)) ;
#75127=CARTESIAN_POINT('Ctrl Pts',(-20.5492532207289,-27.9990394113987,
123.018663281372)) ;
#75128=CARTESIAN_POINT('Ctrl Pts',(-20.727582872687,-28.1890224415269,122.680368443605)) ;
#75129=CARTESIAN_POINT('Ctrl Pts',(-20.463923962656,-28.0090333611081,122.826668031653)) ;
#75130=CARTESIAN_POINT('Ctrl Pts',(-20.5798888067708,-28.1990515643034,
122.462081994055)) ;
#75131=CARTESIAN_POINT('Ctrl Pts',(-20.3457702502389,-28.0190624838847,
122.652037809533)) ;
#75132=CARTESIAN_POINT('Ctrl Pts',(-20.3996251641933,-28.2089276952221,
122.275347174476)) ;
#75133=CARTESIAN_POINT('Ctrl Pts',(-20.2015610992789,-28.0289386148033,
122.502648999522)) ;
#75134=CARTESIAN_POINT('Ctrl Pts',(-20.1873021799924,-28.2189257302391,
122.120642324666)) ;
#75135=CARTESIAN_POINT('Ctrl Pts',(-20.0317039475205,-28.0389366498204,
122.37888357736)) ;
#75136=CARTESIAN_POINT('Ctrl Pts',(-19.9533587455993,-28.2288396599978,
122.005916898507)) ;
#75137=CARTESIAN_POINT('Ctrl Pts',(-19.8445504140462,-28.0488505795791,
122.287101605949)) ;
#75138=CARTESIAN_POINT('Ctrl Pts',(-19.6998517914113,-28.2388828477356,
121.932573093213)) ;
#75139=CARTESIAN_POINT('Ctrl Pts',(-19.6417453532736,-28.0588937673169,
122.228424618319)) ;
#75140=CARTESIAN_POINT('Ctrl Pts',(-19.4411734358219,-28.248782689876,121.904743447145)) ;
#75141=CARTESIAN_POINT('Ctrl Pts',(-19.4348032777468,-28.0687936094572,
122.206158949824)) ;
#75142=CARTESIAN_POINT('Ctrl Pts',(-19.1791693222419,-28.258773956684,121.921854203965)) ;
#75143=CARTESIAN_POINT('Ctrl Pts',(-19.2251999469823,-28.0787848762652,
122.219845480099)) ;
#75144=CARTESIAN_POINT('Ctrl Pts',(-18.9231809982918,-28.2688060588159,
121.984895781364)) ;
#75145=CARTESIAN_POINT('Ctrl Pts',(-19.0204087941554,-28.0888169783972,
122.270276784581)) ;
#75146=CARTESIAN_POINT('Ctrl Pts',(-18.6858684267208,-28.2786729397707,
122.089356190558)) ;
#75147=CARTESIAN_POINT('Ctrl Pts',(-18.830558338332,-28.098683859352,122.353843037551)) ;
#75148=CARTESIAN_POINT('Ctrl Pts',(-18.4672132264003,-28.2886647310588,
122.234743944301)) ;
#75149=CARTESIAN_POINT('Ctrl Pts',(-18.6556330730798,-28.1086756506401,
122.470151422643)) ;
#75150=CARTESIAN_POINT('Ctrl Pts',(-18.2767129740866,-28.2986968469704,
122.416985014521)) ;
#75151=CARTESIAN_POINT('Ctrl Pts',(-18.5032314387329,-28.1187077665516,
122.615942781619)) ;
#75152=CARTESIAN_POINT('Ctrl Pts',(-18.123001634018,-28.3085631637704,122.62579831498)) ;
#75153=CARTESIAN_POINT('Ctrl Pts',(-18.380260910136,-28.1285740833517,122.782991837959)) ;
#75154=CARTESIAN_POINT('Ctrl Pts',(-18.0061033568206,-28.318550645244,122.860752752816)) ;
#75155=CARTESIAN_POINT('Ctrl Pts',(-18.2867404042396,-28.1385615648253,
122.970954341277)) ;
#75156=CARTESIAN_POINT('Ctrl Pts',(-17.9319400038303,-28.3284955696229,
123.111391293692)) ;
#75157=CARTESIAN_POINT('Ctrl Pts',(-18.2274077034628,-28.1485064892042,
123.171464381746)) ;
#75158=CARTESIAN_POINT('Ctrl Pts',(-17.9022796487735,-28.3385404555336,
123.373664123608)) ;
#75159=CARTESIAN_POINT('Ctrl Pts',(-18.2036772802856,-28.1585513751149,
123.381282418945)) ;
#75160=CARTESIAN_POINT('Ctrl Pts',(-17.9180879855161,-28.3484025592462,
123.632366059923)) ;
#75161=CARTESIAN_POINT('Ctrl Pts',(-18.2163217656105,-28.1684134788274,
123.588243760099)) ;
#75162=CARTESIAN_POINT('Ctrl Pts',(-17.9788452222252,-28.3583941230706,
123.887787950751)) ;
#75163=CARTESIAN_POINT('Ctrl Pts',(-18.2649253910361,-28.1784050426519,
123.792581709161)) ;
#75164=CARTESIAN_POINT('Ctrl Pts',(-18.0825235359367,-28.3683269311335,
124.127337211382)) ;
#75165=CARTESIAN_POINT('Ctrl Pts',(-18.3478659549648,-28.1883378507148,
123.984221828264)) ;
#75166=CARTESIAN_POINT('Ctrl Pts',(-18.2257556810704,-28.3782640333699,
124.345706898294)) ;
#75167=CARTESIAN_POINT('Ctrl Pts',(-18.4624497295589,-28.1982749529511,
124.158918686381)) ;
#75168=CARTESIAN_POINT('Ctrl Pts',(-18.4070352869931,-28.3883164796403,
124.537830699368)) ;
#75169=CARTESIAN_POINT('Ctrl Pts',(-18.6074717934068,-28.2083273992215,
124.312619238854)) ;
#75170=CARTESIAN_POINT('Ctrl Pts',(-18.61438364314,-28.3981625952219,124.692645379535)) ;
#75171=CARTESIAN_POINT('Ctrl Pts',(-18.7733489636727,-28.2181735148031,
124.436472636285)) ;
#75172=CARTESIAN_POINT('Ctrl Pts',(-18.8499799673365,-28.4082106149368,
124.811841582579)) ;
#75173=CARTESIAN_POINT('Ctrl Pts',(-18.9618249984737,-28.228221534518,124.531831597543)) ;
#75174=CARTESIAN_POINT('Ctrl Pts',(-19.100163676913,-28.4181525665657,124.887173703437)) ;
#75175=CARTESIAN_POINT('Ctrl Pts',(-19.1619712108279,-28.238163486147,124.592099400923)) ;
#75176=CARTESIAN_POINT('Ctrl Pts',(-19.3594558684225,-28.4280913475648,
124.918552242623)) ;
#75177=CARTESIAN_POINT('Ctrl Pts',(-19.3694046064628,-28.248102267146,124.61720445296)) ;
#75178=CARTESIAN_POINT('Ctrl Pts',(-19.6225169288558,-28.4381173962909,
124.904110048456)) ;
#75179=CARTESIAN_POINT('Ctrl Pts',(-19.5798535127197,-28.2581283158721,
124.60565295931)) ;
#75180=CARTESIAN_POINT('Ctrl Pts',(-19.8756354818574,-28.4480042566991,
124.845353062443)) ;
#75181=CARTESIAN_POINT('Ctrl Pts',(-19.7823488152932,-28.2680151762803,
124.55864953328)) ;
#75182=CARTESIAN_POINT('Ctrl Pts',(-20.1181752200721,-28.4580355318309,
124.742190925172)) ;
#75183=CARTESIAN_POINT('Ctrl Pts',(-19.9763812831176,-28.2780464514121,
124.476122110811)) ;
#75184=CARTESIAN_POINT('Ctrl Pts',(-20.3360779497552,-28.4679185091313,
124.600777052359)) ;
#75185=CARTESIAN_POINT('Ctrl Pts',(-20.1507052303913,-28.2879294287125,
124.362992221081)) ;
#75186=CARTESIAN_POINT('Ctrl Pts',(-20.5293776949433,-28.4779753625384,
124.42064431498)) ;
#75187=CARTESIAN_POINT('Ctrl Pts',(-20.3053443489214,-28.2979862821197,
124.218890369488)) ;
#75188=CARTESIAN_POINT('Ctrl Pts',(-20.7382563361308,-28.4911436036144,
124.144618304014)) ;
#75189=CARTESIAN_POINT('Ctrl Pts',(-20.4724604249661,-28.3111545231956,
123.998058237581)) ;
#75190=CARTESIAN_POINT('Ctrl Pts',(-20.8725696184316,-28.5045446328409,
123.814898573021)) ;
#75191=CARTESIAN_POINT('Ctrl Pts',(-20.5799131718557,-28.3245555524222,
123.734258095252)) ;
#75192=CARTESIAN_POINT('Ctrl Pts',(-20.9154664865249,-28.5177575495718,
123.47022980443)) ;
#75193=CARTESIAN_POINT('Ctrl Pts',(-20.6142236339119,-28.337768469153,123.458566993245)) ;
#75194=CARTESIAN_POINT('Ctrl Pts',(-20.903122860515,-28.527685944025,123.209668872565)) ;
#75195=CARTESIAN_POINT('Ctrl Pts',(-20.6043529645336,-28.3476968636062,
123.250109340891)) ;
#75196=CARTESIAN_POINT('Ctrl Pts',(-20.8455899284453,-28.5376674441531,
122.953713451774)) ;
#75197=CARTESIAN_POINT('Ctrl Pts',(-20.5583282472634,-28.3576783637344,
123.045346890605)) ;
#75198=CARTESIAN_POINT('Ctrl Pts',(-20.7435726950686,-28.5477079874232,
122.710393832295)) ;
#75199=CARTESIAN_POINT('Ctrl Pts',(-20.4767166760668,-28.3677189070045,
122.850689784726)) ;
#75200=CARTESIAN_POINT('Ctrl Pts',(-20.6038530330723,-28.5575573192063,
122.492510433915)) ;
#75201=CARTESIAN_POINT('Ctrl Pts',(-20.3649427782715,-28.3775682387876,
122.676381961247)) ;
#75202=CARTESIAN_POINT('Ctrl Pts',(-20.4263234254908,-28.567552723678,122.298921849218)) ;
#75203=CARTESIAN_POINT('Ctrl Pts',(-20.2229202780013,-28.3875636432592,
122.521509270193)) ;
#75204=CARTESIAN_POINT('Ctrl Pts',(-20.217150439779,-28.5775690511266,122.139134607497)) ;
#75205=CARTESIAN_POINT('Ctrl Pts',(-20.0555849188895,-28.3975799707078,
122.393679028551)) ;
#75206=CARTESIAN_POINT('Ctrl Pts',(-19.9087920778234,-28.5907927082931,
121.978832990182)) ;
#75207=CARTESIAN_POINT('Ctrl Pts',(-19.8088913174118,-28.4108036278744,
122.265428956437)) ;
#75208=CARTESIAN_POINT('Ctrl Pts',(-19.5639959876128,-28.6040869996825,
121.902007063476)) ;
#75209=CARTESIAN_POINT('Ctrl Pts',(-19.5330215630254,-28.4240979192637,
122.203967911005)) ;
#75210=CARTESIAN_POINT('Ctrl Pts',(-19.2151418343575,-28.617371350614,121.916882629561)) ;
#75211=CARTESIAN_POINT('Ctrl Pts',(-19.2539858779433,-28.4373822701952,
122.215868656955)) ;
#75212=CARTESIAN_POINT('Ctrl Pts',(-18.9592277477031,-28.6273437316758,
121.973142750663)) ;
#75213=CARTESIAN_POINT('Ctrl Pts',(-19.0492444708714,-28.447354651257,122.260874150028)) ;
#75214=CARTESIAN_POINT('Ctrl Pts',(-18.7182849243159,-28.6372521113014,
122.07194877023)) ;
#75215=CARTESIAN_POINT('Ctrl Pts',(-18.8564918768448,-28.4572630308826,
122.33991702492)) ;
#75216=CARTESIAN_POINT('Ctrl Pts',(-18.4950390577164,-28.6473061100494,
122.213201779961)) ;
#75217=CARTESIAN_POINT('Ctrl Pts',(-18.6778931410017,-28.4673170296307,
122.452918687146)) ;
#75218=CARTESIAN_POINT('Ctrl Pts',(-18.3032620687832,-28.6571683071657,
122.387567726326)) ;
#75219=CARTESIAN_POINT('Ctrl Pts',(-18.5244716495436,-28.477179226747,122.592405885585)) ;
#75220=CARTESIAN_POINT('Ctrl Pts',(-18.0882237966401,-28.6705154335399,
122.6646378721)) ;
#75221=CARTESIAN_POINT('Ctrl Pts',(-18.352430803744,-28.4905263531211,122.814082073788)) ;
#75222=CARTESIAN_POINT('Ctrl Pts',(-17.9176634711222,-28.6870523991813,
123.069772556852)) ;
#75223=CARTESIAN_POINT('Ctrl Pts',(-18.2159875992731,-28.5070633187626,
123.138150149593)) ;
#75224=CARTESIAN_POINT('Ctrl Pts',(-17.8947632868144,-28.7036870033552,
123.511208297087)) ;
#75225=CARTESIAN_POINT('Ctrl Pts',(-18.1976653221791,-28.5236979229365,
123.491362432851)) ;
#75226=CARTESIAN_POINT('Ctrl Pts',(-17.9677541225909,-28.7169767965979,
123.852806493796)) ;
#75227=CARTESIAN_POINT('Ctrl Pts',(-18.256052534024,-28.5369877161791,123.764590263567)) ;
#75228=CARTESIAN_POINT('Ctrl Pts',(-18.0656567608819,-28.7269294278573,
124.095304375475)) ;
#75229=CARTESIAN_POINT('Ctrl Pts',(-18.3343741827955,-28.5469403474385,
123.9586001496)) ;
#75230=CARTESIAN_POINT('Ctrl Pts',(-18.2039394802369,-28.736881395162,124.317317362314)) ;
#75231=CARTESIAN_POINT('Ctrl Pts',(-18.444996651739,-28.5568923147432,124.136207458359)) ;
#75232=CARTESIAN_POINT('Ctrl Pts',(-18.438736320031,-28.7502486536258,124.578542730228)) ;
#75233=CARTESIAN_POINT('Ctrl Pts',(-18.6328430825618,-28.570259573207,124.345197322045)) ;
#75234=CARTESIAN_POINT('Ctrl Pts',(-18.8064292375722,-28.7667654655749,
124.818587725971)) ;
#75235=CARTESIAN_POINT('Ctrl Pts',(-18.9269842710425,-28.5867763851562,
124.537227610055)) ;
#75236=CARTESIAN_POINT('Ctrl Pts',(-19.3245222155881,-28.7867913605813,
124.93992203315)) ;
#75237=CARTESIAN_POINT('Ctrl Pts',(-19.3414616488824,-28.6068022801626,
124.634301067543)) ;
#75238=CARTESIAN_POINT('Ctrl Pts',(-19.8475073460712,-28.8066020907114,
124.877979440218)) ;
#75239=CARTESIAN_POINT('Ctrl Pts',(-19.7598502986681,-28.6266130102927,
124.58474931514)) ;
#75240=CARTESIAN_POINT('Ctrl Pts',(-20.3222930273454,-28.8265793068413,
124.640387404722)) ;
#75241=CARTESIAN_POINT('Ctrl Pts',(-20.1396805393653,-28.6465902264226,
124.39467832848)) ;
#75242=CARTESIAN_POINT('Ctrl Pts',(-20.6858890814161,-28.8465061822366,
124.255335344377)) ;
#75243=CARTESIAN_POINT('Ctrl Pts',(-20.4305598381238,-28.6665171018178,
124.086638285115)) ;
#75244=CARTESIAN_POINT('Ctrl Pts',(-20.8967489377304,-28.8663276437128,
123.772474684053)) ;
#75245=CARTESIAN_POINT('Ctrl Pts',(-20.5992504644692,-28.6863385632941,
123.700349310091)) ;
#75246=CARTESIAN_POINT('Ctrl Pts',(-20.9302406514315,-28.8864019615222,
123.240064582402)) ;
#75247=CARTESIAN_POINT('Ctrl Pts',(-20.6260460784137,-28.7064128811034,
123.27442205142)) ;
#75248=CARTESIAN_POINT('Ctrl Pts',(-20.781174527664,-28.9062499305301,122.733886817076)) ;
#75249=CARTESIAN_POINT('Ctrl Pts',(-20.5067950359757,-28.7262608501113,
122.869477923346)) ;
#75250=CARTESIAN_POINT('Ctrl Pts',(-20.4677973260754,-28.9261969645933,
122.306404432503)) ;
#75251=CARTESIAN_POINT('Ctrl Pts',(-20.2560944036663,-28.7462078841745,
122.527490503496)) ;
#75252=CARTESIAN_POINT('Ctrl Pts',(-20.0282780333266,-28.9460929155654,
122.012300463445)) ;
#75253=CARTESIAN_POINT('Ctrl Pts',(-19.9044790239162,-28.7661038351467,
122.292205334614)) ;
#75254=CARTESIAN_POINT('Ctrl Pts',(-19.5150711784619,-28.9659883951837,
121.885006525094)) ;
#75255=CARTESIAN_POINT('Ctrl Pts',(-19.4939126765269,-28.7859993147649,
122.190368780619)) ;
#75256=CARTESIAN_POINT('Ctrl Pts',(-18.9875437561368,-28.9859445061485,
121.940541079265)) ;
#75257=CARTESIAN_POINT('Ctrl Pts',(-19.0718901729245,-28.8059554257297,
122.234795557163)) ;
#75258=CARTESIAN_POINT('Ctrl Pts',(-18.5120357100292,-29.0058490541885,
122.172247469398)) ;
#75259=CARTESIAN_POINT('Ctrl Pts',(-18.6914823057681,-28.8258599737697,
122.420160465214)) ;
#75260=CARTESIAN_POINT('Ctrl Pts',(-18.1436273509205,-29.0257231785076,
122.55092549477)) ;
#75261=CARTESIAN_POINT('Ctrl Pts',(-18.3967545360288,-28.8457340980888,
122.723104052043)) ;
#75262=CARTESIAN_POINT('Ctrl Pts',(-17.9253569900103,-29.0457777085066,
123.037111210468)) ;
#75263=CARTESIAN_POINT('Ctrl Pts',(-18.2221384159378,-28.8657886280878,
123.112051915873)) ;
#75264=CARTESIAN_POINT('Ctrl Pts',(-17.8864107135398,-29.0655852222666,
123.562230606213)) ;
#75265=CARTESIAN_POINT('Ctrl Pts',(-18.1909813694771,-28.8855961418478,
123.532149866875)) ;
#75266=CARTESIAN_POINT('Ctrl Pts',(-18.0291344864782,-29.0855685780343,
124.073742812793)) ;
#75267=CARTESIAN_POINT('Ctrl Pts',(-18.3051612924804,-28.9055794976156,
123.941359571674)) ;
#75268=CARTESIAN_POINT('Ctrl Pts',(-18.3375275326525,-29.1054868806182,
124.504029337566)) ;
#75269=CARTESIAN_POINT('Ctrl Pts',(-18.5518768788528,-28.9254978001995,
124.285589192693)) ;
#75270=CARTESIAN_POINT('Ctrl Pts',(-18.77243317676,-29.125355096064,124.803732067738)) ;
#75271=CARTESIAN_POINT('Ctrl Pts',(-18.8998033875348,-28.9453660156452,
124.525350924034)) ;
#75272=CARTESIAN_POINT('Ctrl Pts',(-19.288147951908,-29.1454054128603,124.937374691258)) ;
#75273=CARTESIAN_POINT('Ctrl Pts',(-19.3123750642973,-28.9654163324415,
124.632263609282)) ;
#75274=CARTESIAN_POINT('Ctrl Pts',(-19.8116842876808,-29.1651814747427,
124.888368150147)) ;
#75275=CARTESIAN_POINT('Ctrl Pts',(-19.7312061711631,-28.985192394324,124.59305641669)) ;
#75276=CARTESIAN_POINT('Ctrl Pts',(-20.2935470559917,-29.1852360804352,
124.661024000747)) ;
#75277=CARTESIAN_POINT('Ctrl Pts',(-20.1166950466578,-29.0052470000165,
124.411179407397)) ;
#75278=CARTESIAN_POINT('Ctrl Pts',(-20.6641709204991,-29.2050297695911,
124.28743570735)) ;
#75279=CARTESIAN_POINT('Ctrl Pts',(-20.413193887911,-29.0250406891723,124.112305976162)) ;
#75280=CARTESIAN_POINT('Ctrl Pts',(-20.8881946383036,-29.2249964611855,
123.806481690349)) ;
#75281=CARTESIAN_POINT('Ctrl Pts',(-20.592410427374,-29.0450073807667,123.727541366071)) ;
#75282=CARTESIAN_POINT('Ctrl Pts',(-20.9338249694019,-29.2449565069365,
123.277844260734)) ;
#75283=CARTESIAN_POINT('Ctrl Pts',(-20.62891209658,-29.0649674265177,123.304630928054)) ;
#75284=CARTESIAN_POINT('Ctrl Pts',(-20.7971171357436,-29.2648547670867,
122.766988876767)) ;
#75285=CARTESIAN_POINT('Ctrl Pts',(-20.5195428530867,-29.084865686668,122.895946613903)) ;
#75286=CARTESIAN_POINT('Ctrl Pts',(-20.4948597930559,-29.2847496826359,
122.333148374943)) ;
#75287=CARTESIAN_POINT('Ctrl Pts',(-20.2777339778196,-29.1047606022171,
122.548875457773)) ;
#75288=CARTESIAN_POINT('Ctrl Pts',(-20.0626359965353,-29.3046598630495,
122.027845909636)) ;
#75289=CARTESIAN_POINT('Ctrl Pts',(-19.9319525576066,-29.1246707826307,
122.304635941344)) ;
#75290=CARTESIAN_POINT('Ctrl Pts',(-19.551559332726,-29.3245956621637,121.887948224287)) ;
#75291=CARTESIAN_POINT('Ctrl Pts',(-19.5230899669336,-29.144606581745,122.19272116096)) ;
#75292=CARTESIAN_POINT('Ctrl Pts',(-19.0233846938504,-29.3445335238179,
121.930820616994)) ;
#75293=CARTESIAN_POINT('Ctrl Pts',(-19.1005502612154,-29.1645444433991,
122.227022574999)) ;
#75294=CARTESIAN_POINT('Ctrl Pts',(-18.5418309889257,-29.3644525704555,
122.150865733226)) ;
#75295=CARTESIAN_POINT('Ctrl Pts',(-18.7153085362879,-29.1844634900368,
122.403062807844)) ;
#75296=CARTESIAN_POINT('Ctrl Pts',(-18.1636813293389,-29.3844014685097,
122.522511403311)) ;
#75297=CARTESIAN_POINT('Ctrl Pts',(-18.4127914568634,-29.2044123880909,
122.700380148177)) ;
#75298=CARTESIAN_POINT('Ctrl Pts',(-17.9354075383592,-29.4043072959527,
122.999821271238)) ;
#75299=CARTESIAN_POINT('Ctrl Pts',(-18.2301756194061,-29.224318215534,123.082237846385)) ;
#75300=CARTESIAN_POINT('Ctrl Pts',(-17.8918934978953,-29.420889991318,123.438338526593)) ;
#75301=CARTESIAN_POINT('Ctrl Pts',(-18.195368494416,-29.2409009108993,123.4330280738)) ;
#75302=CARTESIAN_POINT('Ctrl Pts',(-17.9480247351245,-29.4341642050417,
123.782679410184)) ;
#75303=CARTESIAN_POINT('Ctrl Pts',(-18.2402760241612,-29.2541751246229,
123.708522277928)) ;
#75304=CARTESIAN_POINT('Ctrl Pts',(-18.035229582076,-29.444210924241,124.031850013666)) ;
#75305=CARTESIAN_POINT('Ctrl Pts',(-18.3100397891959,-29.2642218438223,
123.907851739695)) ;
#75306=CARTESIAN_POINT('Ctrl Pts',(-18.1615379686828,-29.4540549588867,
124.257627504395)) ;
#75307=CARTESIAN_POINT('Ctrl Pts',(-18.4110966944545,-29.2740658784679,
124.088481420666)) ;
#75308=CARTESIAN_POINT('Ctrl Pts',(-18.3825117400289,-29.4673893437912,
124.529570908601)) ;
#75309=CARTESIAN_POINT('Ctrl Pts',(-18.587837079466,-29.2874002633725,124.305998087073)) ;
#75310=CARTESIAN_POINT('Ctrl Pts',(-18.7397290348901,-29.483976561091,124.788022651573)) ;
#75311=CARTESIAN_POINT('Ctrl Pts',(-18.8736672821377,-29.3039874806722,
124.512799388885)) ;
#75312=CARTESIAN_POINT('Ctrl Pts',(-19.1646822605665,-29.5006097731289,
124.909710774663)) ;
#75313=CARTESIAN_POINT('Ctrl Pts',(-19.2135860980992,-29.3206206927101,
124.610126710635)) ;
#75314=CARTESIAN_POINT('Ctrl Pts',(-19.513720388534,-29.5138922154011,124.915596996218)) ;
#75315=CARTESIAN_POINT('Ctrl Pts',(-19.4928464224192,-29.3339031349823,
124.614841247233)) ;
#75316=CARTESIAN_POINT('Ctrl Pts',(-19.770872928767,-29.5237981033153,124.875254844447)) ;
#75317=CARTESIAN_POINT('Ctrl Pts',(-19.6985621395063,-29.3438090228965,
124.582563747932)) ;
#75318=CARTESIAN_POINT('Ctrl Pts',(-20.0193014854931,-29.5337865214204,
124.790472867308)) ;
#75319=CARTESIAN_POINT('Ctrl Pts',(-19.8973061999821,-29.3537974410017,
124.51473599808)) ;
#75320=CARTESIAN_POINT('Ctrl Pts',(-20.2499022752386,-29.5438099486591,
124.66315381133)) ;
#75321=CARTESIAN_POINT('Ctrl Pts',(-20.0817838661683,-29.3638208682404,
124.412880687566)) ;
#75322=CARTESIAN_POINT('Ctrl Pts',(-20.4525327560712,-29.5537143797761,
124.499823981661)) ;
#75323=CARTESIAN_POINT('Ctrl Pts',(-20.2438922431529,-29.3737252993574,
124.282207749836)) ;
#75324=CARTESIAN_POINT('Ctrl Pts',(-20.6825120255317,-29.5669775323866,
124.237867726883)) ;
#75325=CARTESIAN_POINT('Ctrl Pts',(-20.4278473773578,-29.3869884519678,
124.072677218546)) ;
#75326=CARTESIAN_POINT('Ctrl Pts',(-20.8392151517618,-29.5803024302904,
123.920338199531)) ;
#75327=CARTESIAN_POINT('Ctrl Pts',(-20.553226732279,-29.4003133498717,123.818635845126)) ;
#75328=CARTESIAN_POINT('Ctrl Pts',(-20.9074394905509,-29.5935581739061,
123.578684401658)) ;
#75329=CARTESIAN_POINT('Ctrl Pts',(-20.6078059447763,-29.4135690934873,
123.545295374543)) ;
#75330=CARTESIAN_POINT('Ctrl Pts',(-20.9137330389312,-29.6035175473534,
123.317072430937)) ;
#75331=CARTESIAN_POINT('Ctrl Pts',(-20.6128379811963,-29.4235284669346,
123.336009184031)) ;
#75332=CARTESIAN_POINT('Ctrl Pts',(-20.8748846542683,-29.6134613712803,
123.058630457431)) ;
#75333=CARTESIAN_POINT('Ctrl Pts',(-20.5817571955094,-29.4334722908616,
123.129255093572)) ;
#75334=CARTESIAN_POINT('Ctrl Pts',(-20.7906838438888,-29.6235093154276,
122.808386846947)) ;
#75335=CARTESIAN_POINT('Ctrl Pts',(-20.5143943808657,-29.4435202350089,
122.929061213128)) ;
#75336=CARTESIAN_POINT('Ctrl Pts',(-20.6669727396091,-29.6333602866458,
122.580969032594)) ;
#75337=CARTESIAN_POINT('Ctrl Pts',(-20.4154235694875,-29.4533712062271,
122.747128058925)) ;
#75338=CARTESIAN_POINT('Ctrl Pts',(-20.5042317391109,-29.6433321040879,
122.375617475146)) ;
#75339=CARTESIAN_POINT('Ctrl Pts',(-20.285229061277,-29.4633430236691,122.582848300707)) ;
#75340=CARTESIAN_POINT('Ctrl Pts',(-20.3077646578512,-29.65332752638,122.201218734674)) ;
#75341=CARTESIAN_POINT('Ctrl Pts',(-20.1280539536979,-29.4733384459612,
122.443331024174)) ;
#75342=CARTESIAN_POINT('Ctrl Pts',(-20.0830517817322,-29.6633605915037,
122.063322483004)) ;
#75343=CARTESIAN_POINT('Ctrl Pts',(-19.9482825016034,-29.4833715110849,
122.333015964112)) ;
#75344=CARTESIAN_POINT('Ctrl Pts',(-19.8419990548068,-29.6732259241689,
121.967921099616)) ;
#75345=CARTESIAN_POINT('Ctrl Pts',(-19.7554396557229,-29.4932368437501,
122.256697012164)) ;
#75346=CARTESIAN_POINT('Ctrl Pts',(-19.5857362753645,-29.6831864667665,
121.914563791479)) ;
#75347=CARTESIAN_POINT('Ctrl Pts',(-19.5504291017455,-29.5031973863477,
122.214013362556)) ;
#75348=CARTESIAN_POINT('Ctrl Pts',(-19.3221856204201,-29.6932201522682,
121.906899471653)) ;
#75349=CARTESIAN_POINT('Ctrl Pts',(-19.3395885271886,-29.5132310718494,
122.207884142788)) ;
#75350=CARTESIAN_POINT('Ctrl Pts',(-19.0650645565707,-29.7031049842585,
121.944106565248)) ;
#75351=CARTESIAN_POINT('Ctrl Pts',(-19.1338922165619,-29.5231159038397,
122.237651976139)) ;
#75352=CARTESIAN_POINT('Ctrl Pts',(-18.8138468784556,-29.7131724110183,
122.026926609353)) ;
#75353=CARTESIAN_POINT('Ctrl Pts',(-18.9329187385003,-29.5331833305995,
122.303910131109)) ;
#75354=CARTESIAN_POINT('Ctrl Pts',(-18.5859272207693,-29.7230109001771,
122.149077864709)) ;
#75355=CARTESIAN_POINT('Ctrl Pts',(-18.7505843444716,-29.5430218197584,
122.401632918194)) ;
#75356=CARTESIAN_POINT('Ctrl Pts',(-18.3778786570195,-29.7330743813672,
122.312276880573)) ;
#75357=CARTESIAN_POINT('Ctrl Pts',(-18.5841468108762,-29.5530853009485,
122.532193870255)) ;
#75358=CARTESIAN_POINT('Ctrl Pts',(-18.2044212592288,-29.7429685391823,
122.506008820016)) ;
#75359=CARTESIAN_POINT('Ctrl Pts',(-18.4453827052769,-29.5629794587636,
122.687180688913)) ;
#75360=CARTESIAN_POINT('Ctrl Pts',(-18.066004470774,-29.7529103959266,122.727551566426)) ;
#75361=CARTESIAN_POINT('Ctrl Pts',(-18.334651204385,-29.5729213155079,122.864415841661)) ;
#75362=CARTESIAN_POINT('Ctrl Pts',(-17.9674436495198,-29.7629128735981,
122.971267274074)) ;
#75363=CARTESIAN_POINT('Ctrl Pts',(-18.255804547113,-29.5829237931793,123.059389144256)) ;
#75364=CARTESIAN_POINT('Ctrl Pts',(-17.9129372901095,-29.7729476779024,
123.229259453653)) ;
#75365=CARTESIAN_POINT('Ctrl Pts',(-18.2122015796833,-29.5929585974836,
123.265783349704)) ;
#75366=CARTESIAN_POINT('Ctrl Pts',(-17.903787325648,-29.782792554748,123.487828320681)) ;
#75367=CARTESIAN_POINT('Ctrl Pts',(-18.2048837514533,-29.6028034743293,
123.472638064826)) ;
#75368=CARTESIAN_POINT('Ctrl Pts',(-17.9396889313481,-29.7927784343036,
123.747736250543)) ;
#75369=CARTESIAN_POINT('Ctrl Pts',(-18.2336070824238,-29.6127893538848,
123.680563995791)) ;
#75370=CARTESIAN_POINT('Ctrl Pts',(-18.0196096203183,-29.8027131646621,
123.99633015852)) ;
#75371=CARTESIAN_POINT('Ctrl Pts',(-18.2975455112086,-29.6227240842433,
123.879438242773)) ;
#75372=CARTESIAN_POINT('Ctrl Pts',(-18.1431663386496,-29.8127709769749,
124.229931834486)) ;
#75373=CARTESIAN_POINT('Ctrl Pts',(-18.3963927784555,-29.6327818965562,
124.066318691056)) ;
#75374=CARTESIAN_POINT('Ctrl Pts',(-18.3012830487224,-29.8225915690993,
124.433951656965)) ;
#75375=CARTESIAN_POINT('Ctrl Pts',(-18.5228873635076,-29.6426024886806,
124.229532798967)) ;
#75376=CARTESIAN_POINT('Ctrl Pts',(-18.4969190823567,-29.8326581547091,
124.611938648254)) ;
#75377=CARTESIAN_POINT('Ctrl Pts',(-18.679397626606,-29.6526690742904,124.37192099675)) ;
#75378=CARTESIAN_POINT('Ctrl Pts',(-18.7169004533169,-29.842557735291,124.750929340438)) ;
#75379=CARTESIAN_POINT('Ctrl Pts',(-18.8553834510956,-29.6625686548722,
124.483111642557)) ;
#75380=CARTESIAN_POINT('Ctrl Pts',(-18.9612300161898,-29.8526093349692,
124.851178041626)) ;
#75381=CARTESIAN_POINT('Ctrl Pts',(-19.050847943237,-29.6726202545505,124.563308795822)) ;
#75382=CARTESIAN_POINT('Ctrl Pts',(-19.2147547487761,-29.8624835213862,
124.906699600803)) ;
#75383=CARTESIAN_POINT('Ctrl Pts',(-19.2536676428027,-29.6824944409674,
124.607724013081)) ;
#75384=CARTESIAN_POINT('Ctrl Pts',(-19.4787496446866,-29.8725399972671,
124.917720031987)) ;
#75385=CARTESIAN_POINT('Ctrl Pts',(-19.4648637461611,-29.6925509168483,
124.616538418507)) ;
#75386=CARTESIAN_POINT('Ctrl Pts',(-19.7365039466666,-29.8824329285696,
124.883386677923)) ;
#75387=CARTESIAN_POINT('Ctrl Pts',(-19.6710664653841,-29.7024438481509,
124.589069887457)) ;
#75388=CARTESIAN_POINT('Ctrl Pts',(-19.9885582401288,-29.8924957072823,
124.803550123719)) ;
#75389=CARTESIAN_POINT('Ctrl Pts',(-19.8727094596313,-29.7125066268636,
124.52519876481)) ;
#75390=CARTESIAN_POINT('Ctrl Pts',(-20.2179182729885,-29.9023382328635,
124.68392271181)) ;
#75391=CARTESIAN_POINT('Ctrl Pts',(-20.0561959904771,-29.7223491524447,
124.429495469086)) ;
#75392=CARTESIAN_POINT('Ctrl Pts',(-20.4264420362818,-29.9123289982884,
124.52445158431)) ;
#75393=CARTESIAN_POINT('Ctrl Pts',(-20.2230137897094,-29.7323399178696,
124.301917213795)) ;
#75394=CARTESIAN_POINT('Ctrl Pts',(-20.602990790598,-29.9222570742864,124.332343420882)) ;
#75395=CARTESIAN_POINT('Ctrl Pts',(-20.3642511922906,-29.7422679938676,
124.148229742484)) ;
#75396=CARTESIAN_POINT('Ctrl Pts',(-20.7447343009426,-29.9322449846734,
124.111422181903)) ;
#75397=CARTESIAN_POINT('Ctrl Pts',(-20.4776444559696,-29.7522559042547,
123.971491933959)) ;
#75398=CARTESIAN_POINT('Ctrl Pts',(-20.8460304546489,-29.9422808967983,
123.867929241407)) ;
#75399=CARTESIAN_POINT('Ctrl Pts',(-20.5586797287902,-29.7622918163796,
123.776696819529)) ;
#75400=CARTESIAN_POINT('Ctrl Pts',(-20.9028976476815,-29.952135909646,123.615249639793)) ;
#75401=CARTESIAN_POINT('Ctrl Pts',(-20.6041716209895,-29.7721468292273,
123.574553473142)) ;
#75402=CARTESIAN_POINT('Ctrl Pts',(-20.9155677102884,-29.9621348555623,
123.352835793813)) ;
#75403=CARTESIAN_POINT('Ctrl Pts',(-20.6143059849255,-29.7821457751435,
123.364622425134)) ;
#75404=CARTESIAN_POINT('Ctrl Pts',(-20.8830605295313,-29.9720317680103,
123.094753953396)) ;
#75405=CARTESIAN_POINT('Ctrl Pts',(-20.5882986910333,-29.7920426875915,
123.158157729796)) ;
#75406=CARTESIAN_POINT('Ctrl Pts',(-20.8050694040147,-29.9820855661038,
122.842358190295)) ;
#75407=CARTESIAN_POINT('Ctrl Pts',(-20.5259041888426,-29.802096485685,122.956241456897)) ;
#75408=CARTESIAN_POINT('Ctrl Pts',(-20.6865523392665,-29.9919664869304,
122.611290225782)) ;
#75409=CARTESIAN_POINT('Ctrl Pts',(-20.4310894079275,-29.8119774065117,
122.771388421395)) ;
#75410=CARTESIAN_POINT('Ctrl Pts',(-20.5281670016261,-30.0019710129282,
122.401483413307)) ;
#75411=CARTESIAN_POINT('Ctrl Pts',(-20.3043799645414,-29.8219819325095,
122.603543955252)) ;
#75412=CARTESIAN_POINT('Ctrl Pts',(-20.3360451640972,-30.0119549765457,
122.222739387127)) ;
#75413=CARTESIAN_POINT('Ctrl Pts',(-20.1506815650826,-29.8319658961269,
122.460549974152)) ;
#75414=CARTESIAN_POINT('Ctrl Pts',(-20.1144958156019,-30.021994617097,122.079517699104)) ;
#75415=CARTESIAN_POINT('Ctrl Pts',(-19.9734411337302,-29.8420055366782,
122.345973905275)) ;
#75416=CARTESIAN_POINT('Ctrl Pts',(-19.8762838854864,-30.0318386427117,
121.978637774612)) ;
#75417=CARTESIAN_POINT('Ctrl Pts',(-19.7828718281963,-29.8518495622929,
122.265271730029)) ;
#75418=CARTESIAN_POINT('Ctrl Pts',(-19.620581079662,-30.041829648529,121.919049659256)) ;
#75419=CARTESIAN_POINT('Ctrl Pts',(-19.5783094204032,-29.8618405681103,
122.217602616233)) ;
#75420=CARTESIAN_POINT('Ctrl Pts',(-19.3571576412115,-30.0518674400612,
121.905299416059)) ;
#75421=CARTESIAN_POINT('Ctrl Pts',(-19.3675704851451,-29.8718783596425,
122.206603915684)) ;
#75422=CARTESIAN_POINT('Ctrl Pts',(-19.1003268168812,-30.0617118398496,
121.936426083641)) ;
#75423=CARTESIAN_POINT('Ctrl Pts',(-19.1621069272286,-29.8817227594309,
122.231506534638)) ;
#75424=CARTESIAN_POINT('Ctrl Pts',(-18.8491638610949,-30.0716966404063,
122.012238721602)) ;
#75425=CARTESIAN_POINT('Ctrl Pts',(-18.9611771300981,-29.8917075599876,
122.292157833579)) ;
#75426=CARTESIAN_POINT('Ctrl Pts',(-18.6159274222677,-30.0816361638175,
122.129904287685)) ;
#75427=CARTESIAN_POINT('Ctrl Pts',(-18.774588942654,-29.9016470833988,122.386291228805)) ;
#75428=CARTESIAN_POINT('Ctrl Pts',(-18.404637738631,-30.0916758829185,122.287871780177)) ;
#75429=CARTESIAN_POINT('Ctrl Pts',(-18.6055578744043,-29.9116868024998,
122.512666327168)) ;
#75430=CARTESIAN_POINT('Ctrl Pts',(-18.2265933389439,-30.1015640548378,
122.477161788277)) ;
#75431=CARTESIAN_POINT('Ctrl Pts',(-18.4631237804811,-29.921574974419,122.664098660573)) ;
#75432=CARTESIAN_POINT('Ctrl Pts',(-18.0822626445638,-30.1115536172548,
122.696428624397)) ;
#75433=CARTESIAN_POINT('Ctrl Pts',(-18.3476602845798,-29.931564536836,122.839512622054)) ;
#75434=CARTESIAN_POINT('Ctrl Pts',(-17.9786995241007,-30.1215119894495,
122.936755300678)) ;
#75435=CARTESIAN_POINT('Ctrl Pts',(-18.2648110278588,-29.9415229090307,
123.031774118599)) ;
#75436=CARTESIAN_POINT('Ctrl Pts',(-17.9181786121027,-30.1314120636802,
123.189791746342)) ;
#75437=CARTESIAN_POINT('Ctrl Pts',(-18.2163954912986,-29.9514229832614,
123.234202841237)) ;
#75438=CARTESIAN_POINT('Ctrl Pts',(-17.902317704542,-30.1414581600538,123.453303427387)) ;
#75439=CARTESIAN_POINT('Ctrl Pts',(-18.2037078197734,-29.961469079635,123.445012405779)) ;
#75440=CARTESIAN_POINT('Ctrl Pts',(-17.932026969616,-30.1513667440509,123.712002752088)) ;
#75441=CARTESIAN_POINT('Ctrl Pts',(-18.2274762127078,-29.9713776636321,
123.651971093748)) ;
#75442=CARTESIAN_POINT('Ctrl Pts',(-18.0064982864425,-30.1613773226418,
123.964313150641)) ;
#75443=CARTESIAN_POINT('Ctrl Pts',(-18.2870541704328,-29.981388242223,123.853819106392)) ;
#75444=CARTESIAN_POINT('Ctrl Pts',(-18.1243449647309,-30.1714064807546,
124.200064581394)) ;
#75445=CARTESIAN_POINT('Ctrl Pts',(-18.3813325117191,-29.9914174003359,
124.042419843847)) ;
#75446=CARTESIAN_POINT('Ctrl Pts',(-18.2782623863154,-30.1812593625927,
124.40825332171)) ;
#75447=CARTESIAN_POINT('Ctrl Pts',(-18.5044666446186,-30.0012702821739,
124.208969431975)) ;
#75448=CARTESIAN_POINT('Ctrl Pts',(-18.4674836004479,-30.1912189237437,
124.589086196472)) ;
#75449=CARTESIAN_POINT('Ctrl Pts',(-18.6558438971189,-30.0112298433249,
124.35363489223)) ;
#75450=CARTESIAN_POINT('Ctrl Pts',(-18.6871993887811,-30.2012573583328,
124.735052040816)) ;
#75451=CARTESIAN_POINT('Ctrl Pts',(-18.8316171435154,-30.021268277914,124.470406880302)) ;
#75452=CARTESIAN_POINT('Ctrl Pts',(-18.9248025260777,-30.2111306305599,
124.839385850432)) ;
#75453=CARTESIAN_POINT('Ctrl Pts',(-19.0216991485207,-30.0311415501411,
124.553872836708)) ;
#75454=CARTESIAN_POINT('Ctrl Pts',(-19.181943910287,-30.2212038725534,124.902021223961)) ;
#75455=CARTESIAN_POINT('Ctrl Pts',(-19.2274127817706,-30.0412147921347,
124.603980422162)) ;
#75456=CARTESIAN_POINT('Ctrl Pts',(-19.4395127810936,-30.2310242040865,
124.918975069685)) ;
#75457=CARTESIAN_POINT('Ctrl Pts',(-19.433466684621,-30.0510351236678,124.617542685309)) ;
#75458=CARTESIAN_POINT('Ctrl Pts',(-19.7027659038586,-30.2411028653133,
124.89046761584)) ;
#75459=CARTESIAN_POINT('Ctrl Pts',(-19.6440694852678,-30.0611137848945,
124.594736008976)) ;
#75460=CARTESIAN_POINT('Ctrl Pts',(-19.9514865660773,-30.2509544606075,
124.818398357358)) ;
#75461=CARTESIAN_POINT('Ctrl Pts',(-19.8430448190709,-30.0709653801888,
124.537080268754)) ;
#75462=CARTESIAN_POINT('Ctrl Pts',(-20.1891444820708,-30.2610275958363,
124.701927251156)) ;
#75463=CARTESIAN_POINT('Ctrl Pts',(-20.0331712033916,-30.0810385154176,
124.44390269208)) ;
#75464=CARTESIAN_POINT('Ctrl Pts',(-20.3981066042544,-30.2708700313613,
124.549458419437)) ;
#75465=CARTESIAN_POINT('Ctrl Pts',(-20.2003396262217,-30.0908809509426,
124.321927803439)) ;
#75466=CARTESIAN_POINT('Ctrl Pts',(-20.5805436588615,-30.2808508004947,
124.361037704467)) ;
#75467=CARTESIAN_POINT('Ctrl Pts',(-20.3462888173977,-30.100861720076,124.171191137294)) ;
#75468=CARTESIAN_POINT('Ctrl Pts',(-20.7276313527924,-30.2908679017386,
124.142726286171)) ;
#75469=CARTESIAN_POINT('Ctrl Pts',(-20.4639585479526,-30.1108788213199,
123.99654171188)) ;
#75470=CARTESIAN_POINT('Ctrl Pts',(-20.8336603364787,-30.3007563493404,
123.905461600846)) ;
#75471=CARTESIAN_POINT('Ctrl Pts',(-20.5487810297276,-30.1207672689217,
123.806730589124)) ;
#75472=CARTESIAN_POINT('Ctrl Pts',(-20.8979668750265,-30.3108120635213,
123.649176787993)) ;
#75473=CARTESIAN_POINT('Ctrl Pts',(-20.6002259506018,-30.1308229831026,
123.601702402648)) ;
#75474=CARTESIAN_POINT('Ctrl Pts',(-20.9165011055826,-30.3206872699351,
123.390311340075)) ;
#75475=CARTESIAN_POINT('Ctrl Pts',(-20.6150528932545,-30.1406981895164,
123.39461094526)) ;
#75476=CARTESIAN_POINT('Ctrl Pts',(-20.8901135578881,-30.3306823224079,
123.128988240044)) ;
#75477=CARTESIAN_POINT('Ctrl Pts',(-20.5939426563615,-30.1506932419891,
123.185552627896)) ;
#75478=CARTESIAN_POINT('Ctrl Pts',(-20.8181453544981,-30.34070420637,122.875637484416)) ;
#75479=CARTESIAN_POINT('Ctrl Pts',(-20.5363677699957,-30.1607151259512,
122.982872078019)) ;
#75480=CARTESIAN_POINT('Ctrl Pts',(-20.7048988528547,-30.3506081788993,
122.641302484531)) ;
#75481=CARTESIAN_POINT('Ctrl Pts',(-20.4457706757612,-30.1706190984805,
122.795404879528)) ;
#75482=CARTESIAN_POINT('Ctrl Pts',(-20.5516896930271,-30.3605966755602,
122.428164932621)) ;
#75483=CARTESIAN_POINT('Ctrl Pts',(-20.3232033327596,-30.1806075951414,
122.624895080866)) ;
#75484=CARTESIAN_POINT('Ctrl Pts',(-20.3641515811643,-30.3705604728081,
122.245458339218)) ;
#75485=CARTESIAN_POINT('Ctrl Pts',(-20.17317296099,-30.1905713923894,122.478730202668)) ;
#75486=CARTESIAN_POINT('Ctrl Pts',(-20.1493641424426,-30.3804644961162,
122.098426355277)) ;
#75487=CARTESIAN_POINT('Ctrl Pts',(-20.0013436095708,-30.2004754156974,
122.361105071754)) ;
#75488=CARTESIAN_POINT('Ctrl Pts',(-19.9085262576958,-30.3905249994378,
121.98944865862)) ;
#75489=CARTESIAN_POINT('Ctrl Pts',(-19.8086730047828,-30.2105359190191,
122.273922884312)) ;
#75490=CARTESIAN_POINT('Ctrl Pts',(-19.6580405513077,-30.4003655345777,
121.925039834699)) ;
#75491=CARTESIAN_POINT('Ctrl Pts',(-19.6082855766348,-30.2203764541589,
122.222396127967)) ;
#75492=CARTESIAN_POINT('Ctrl Pts',(-19.3944577950564,-30.4104277552823,
121.904320740001)) ;
#75493=CARTESIAN_POINT('Ctrl Pts',(-19.3974190827422,-30.2304386748635,
122.205820754266)) ;
#75494=CARTESIAN_POINT('Ctrl Pts',(-19.1355824753034,-30.4203249090585,
121.929541442094)) ;
#75495=CARTESIAN_POINT('Ctrl Pts',(-19.1903196245163,-30.2403358286398,
122.225997234219)) ;
#75496=CARTESIAN_POINT('Ctrl Pts',(-18.8839449757673,-30.430256042444,121.998725089926)) ;
#75497=CARTESIAN_POINT('Ctrl Pts',(-18.9890101207813,-30.2502669620252,
122.281343781079)) ;
#75498=CARTESIAN_POINT('Ctrl Pts',(-18.6456264179533,-30.4402984175897,
122.1120674788)) ;
#75499=CARTESIAN_POINT('Ctrl Pts',(-18.7983550586508,-30.260309337171,122.372017626633)) ;
#75500=CARTESIAN_POINT('Ctrl Pts',(-18.4338243468948,-30.4501843553558,
122.262533293048)) ;
#75501=CARTESIAN_POINT('Ctrl Pts',(-18.6289139946321,-30.2701952749371,
122.492389609933)) ;
#75502=CARTESIAN_POINT('Ctrl Pts',(-18.2490727523449,-30.4601801983407,
122.449233759721)) ;
#75503=CARTESIAN_POINT('Ctrl Pts',(-18.4811126123803,-30.2801911179219,
122.641749654634)) ;
#75504=CARTESIAN_POINT('Ctrl Pts',(-18.1003554685412,-30.4701221762193,
122.664059702214)) ;
#75505=CARTESIAN_POINT('Ctrl Pts',(-18.3621388222961,-30.2901330958005,
122.813609831262)) ;
#75506=CARTESIAN_POINT('Ctrl Pts',(-17.9906956059889,-30.4800815507003,
122.901684237762)) ;
#75507=CARTESIAN_POINT('Ctrl Pts',(-18.2744107413088,-30.3000924702815,
123.003708954726)) ;
#75508=CARTESIAN_POINT('Ctrl Pts',(-17.9235701572944,-30.490078166534,123.155692351254)) ;
#75509=CARTESIAN_POINT('Ctrl Pts',(-18.2207100063737,-30.3100890861153,
123.206915221358)) ;
#75510=CARTESIAN_POINT('Ctrl Pts',(-17.9018377986433,-30.5001123851076,
123.418476175523)) ;
#75511=CARTESIAN_POINT('Ctrl Pts',(-18.203323782619,-30.3201233046888,123.417142364106)) ;
#75512=CARTESIAN_POINT('Ctrl Pts',(-17.9253133851057,-30.5099654523182,
123.676335153518)) ;
#75513=CARTESIAN_POINT('Ctrl Pts',(-18.2221037452179,-30.3299763718994,
123.623428491503)) ;
#75514=CARTESIAN_POINT('Ctrl Pts',(-17.9932051453704,-30.5199257101958,
123.929113114996)) ;
#75515=CARTESIAN_POINT('Ctrl Pts',(-18.2764164755412,-30.339936629777,123.825650660064)) ;
#75516=CARTESIAN_POINT('Ctrl Pts',(-18.1050124820185,-30.5299547369014,
124.167789386628)) ;
#75517=CARTESIAN_POINT('Ctrl Pts',(-18.3658619051834,-30.3499656564826,
124.016591970179)) ;
#75518=CARTESIAN_POINT('Ctrl Pts',(-18.2546907014381,-30.5398649439358,
124.380895877624)) ;
#75519=CARTESIAN_POINT('Ctrl Pts',(-18.4856036341333,-30.3598758635171,
124.18707690079)) ;
#75520=CARTESIAN_POINT('Ctrl Pts',(-18.439085172546,-30.5497998545834,124.565733592048)) ;
#75521=CARTESIAN_POINT('Ctrl Pts',(-18.633118334194,-30.3698107741647,124.334947200933)) ;
#75522=CARTESIAN_POINT('Ctrl Pts',(-18.6551854058233,-30.5598409847626,
124.717139371071)) ;
#75523=CARTESIAN_POINT('Ctrl Pts',(-18.805998270169,-30.3798519043439,124.456072442656)) ;
#75524=CARTESIAN_POINT('Ctrl Pts',(-18.8905691521893,-30.5697281251326,
124.827187732262)) ;
#75525=CARTESIAN_POINT('Ctrl Pts',(-18.994304219969,-30.3897390447139,124.544111408934)) ;
#75526=CARTESIAN_POINT('Ctrl Pts',(-19.1440074490073,-30.5797204026685,
124.895826199271)) ;
#75527=CARTESIAN_POINT('Ctrl Pts',(-19.1970544909255,-30.3997313222498,
124.599022913111)) ;
#75528=CARTESIAN_POINT('Ctrl Pts',(-19.4044083048239,-30.5896689459369,
124.919242869025)) ;
#75529=CARTESIAN_POINT('Ctrl Pts',(-19.405374674023,-30.4096798655181,124.61775698852)) ;
#75530=CARTESIAN_POINT('Ctrl Pts',(-19.6646066985236,-30.5996056207541,
124.897490651065)) ;
#75531=CARTESIAN_POINT('Ctrl Pts',(-19.6135329527055,-30.4196165403353,
124.600356125457)) ;
#75532=CARTESIAN_POINT('Ctrl Pts',(-19.918388569691,-30.6095890416904,124.830870140945)) ;
#75533=CARTESIAN_POINT('Ctrl Pts',(-19.816558494324,-30.4295999612717,124.547060681517)) ;
#75534=CARTESIAN_POINT('Ctrl Pts',(-20.1579384638651,-30.6196313568797,
124.720177686915)) ;
#75535=CARTESIAN_POINT('Ctrl Pts',(-20.0081988873676,-30.4396422764609,
124.458507428981)) ;
#75536=CARTESIAN_POINT('Ctrl Pts',(-20.3705238610146,-30.6294716743189,
124.572936951998)) ;
#75537=CARTESIAN_POINT('Ctrl Pts',(-20.1782668479969,-30.4494825939001,
124.340716237617)) ;
#75538=CARTESIAN_POINT('Ctrl Pts',(-20.5582851076625,-30.6395013783764,
124.387959911848)) ;
#75539=CARTESIAN_POINT('Ctrl Pts',(-20.3284766672307,-30.4595122979576,
124.192735318187)) ;
#75540=CARTESIAN_POINT('Ctrl Pts',(-20.7103623023871,-30.6495223350989,
124.1729709106)) ;
#75541=CARTESIAN_POINT('Ctrl Pts',(-20.450139188978,-30.4695332546801,124.020744631255)) ;
#75542=CARTESIAN_POINT('Ctrl Pts',(-20.8216762307173,-30.6593888774025,
123.938777584524)) ;
#75543=CARTESIAN_POINT('Ctrl Pts',(-20.5391909126625,-30.4793997969837,
123.833391248542)) ;
#75544=CARTESIAN_POINT('Ctrl Pts',(-20.8920560098693,-30.6694599773476,
123.683674797195)) ;
#75545=CARTESIAN_POINT('Ctrl Pts',(-20.5954958516475,-30.4894708969289,
123.629309014543)) ;
#75546=CARTESIAN_POINT('Ctrl Pts',(-20.9165006065957,-30.6793020515252,
123.426182698947)) ;
#75547=CARTESIAN_POINT('Ctrl Pts',(-20.6150525003073,-30.4993129711065,
123.423316470327)) ;
#75548=CARTESIAN_POINT('Ctrl Pts',(-20.8965796707046,-30.6892628461122,
123.165188338051)) ;
#75549=CARTESIAN_POINT('Ctrl Pts',(-20.5991170611532,-30.5092737656935,
123.214521207781)) ;
#75550=CARTESIAN_POINT('Ctrl Pts',(-20.8306367979859,-30.6993007190131,
122.909788435408)) ;
#75551=CARTESIAN_POINT('Ctrl Pts',(-20.5463638720667,-30.5193116385943,
123.010200889343)) ;
#75552=CARTESIAN_POINT('Ctrl Pts',(-20.7235512012053,-30.7091750045571,
122.673393853089)) ;
#75553=CARTESIAN_POINT('Ctrl Pts',(-20.4606968923866,-30.5291859241384,
122.821085433644)) ;
#75554=CARTESIAN_POINT('Ctrl Pts',(-20.5741723490005,-30.7192447549711,
122.455008665901)) ;
#75555=CARTESIAN_POINT('Ctrl Pts',(-20.3411947055965,-30.5392556745523,
122.646376333744)) ;
#75556=CARTESIAN_POINT('Ctrl Pts',(-20.3935486501348,-30.7290780395057,
122.270181067648)) ;
#75557=CARTESIAN_POINT('Ctrl Pts',(-20.1966973937778,-30.549088959087,122.498514076006)) ;
#75558=CARTESIAN_POINT('Ctrl Pts',(-20.1798297267622,-30.7391083803058,
122.115914599619)) ;
#75559=CARTESIAN_POINT('Ctrl Pts',(-20.0257230530562,-30.559119299887,122.375099677665)) ;
#75560=CARTESIAN_POINT('Ctrl Pts',(-19.9421798972876,-30.7491403043054,
122.001770363391)) ;
#75561=CARTESIAN_POINT('Ctrl Pts',(-19.8356036909516,-30.5691512238866,
122.28378308955)) ;
#75562=CARTESIAN_POINT('Ctrl Pts',(-19.6936420289433,-30.7589688392413,
121.931532551755)) ;
#75563=CARTESIAN_POINT('Ctrl Pts',(-19.6367747626622,-30.5789797588226,
122.227591754788)) ;
#75564=CARTESIAN_POINT('Ctrl Pts',(-19.4324272173861,-30.768962617006,121.90436106235)) ;
#75565=CARTESIAN_POINT('Ctrl Pts',(-19.4278031940052,-30.5889735365872,
122.205853025448)) ;
#75566=CARTESIAN_POINT('Ctrl Pts',(-19.1696001927658,-30.7789903274915,
121.923539411907)) ;
#75567=CARTESIAN_POINT('Ctrl Pts',(-19.2175414369296,-30.5990012470728,
122.221194254643)) ;
#75568=CARTESIAN_POINT('Ctrl Pts',(-18.9175710994539,-30.7888787383255,
121.98685039034)) ;
#75569=CARTESIAN_POINT('Ctrl Pts',(-19.0159184367103,-30.6088896579067,
122.271841400405)) ;
#75570=CARTESIAN_POINT('Ctrl Pts',(-18.6780751167971,-30.798855588861,122.093481958298)) ;
#75571=CARTESIAN_POINT('Ctrl Pts',(-18.8243211846636,-30.6188665084423,
122.357145104466)) ;
#75572=CARTESIAN_POINT('Ctrl Pts',(-18.4603462227965,-30.8088473854115,
122.240311680706)) ;
#75573=CARTESIAN_POINT('Ctrl Pts',(-18.6501372714632,-30.6288583049927,
122.474607479311)) ;
#75574=CARTESIAN_POINT('Ctrl Pts',(-18.2708493729533,-30.8188833915051,
122.423713476648)) ;
#75575=CARTESIAN_POINT('Ctrl Pts',(-18.4985386630892,-30.6388943110864,
122.621327853477)) ;
#75576=CARTESIAN_POINT('Ctrl Pts',(-18.1185854662254,-30.828734125768,122.633088418397)) ;
#75577=CARTESIAN_POINT('Ctrl Pts',(-18.376726707459,-30.6487450453492,122.788826190101)) ;
#75578=CARTESIAN_POINT('Ctrl Pts',(-18.0029869057309,-30.8387253842962,
122.86878945056)) ;
#75579=CARTESIAN_POINT('Ctrl Pts',(-18.2842463850415,-30.6587363038774,
122.97738614376)) ;
#75580=CARTESIAN_POINT('Ctrl Pts',(-17.9304364000927,-30.8486432791994,
123.119155041254)) ;
#75581=CARTESIAN_POINT('Ctrl Pts',(-18.2262044469805,-30.6686541987806,
123.177677695621)) ;
#75582=CARTESIAN_POINT('Ctrl Pts',(-17.9020877613563,-30.8586714208624,
123.381133283298)) ;
#75583=CARTESIAN_POINT('Ctrl Pts',(-18.2035238003672,-30.6786823404437,
123.387260129306)) ;
#75584=CARTESIAN_POINT('Ctrl Pts',(-17.9193001863973,-30.8685565889783,
123.640341140636)) ;
#75585=CARTESIAN_POINT('Ctrl Pts',(-18.2172919455385,-30.6885675085595,
123.594625944928)) ;
#75586=CARTESIAN_POINT('Ctrl Pts',(-17.9812908654965,-30.8785459524843,
123.895432047581)) ;
#75587=CARTESIAN_POINT('Ctrl Pts',(-18.2668826491316,-30.6985568720655,
123.798698988406)) ;
#75588=CARTESIAN_POINT('Ctrl Pts',(-18.0876859530598,-30.8885870874943,
124.136901868382)) ;
#75589=CARTESIAN_POINT('Ctrl Pts',(-18.3519971252596,-30.7085980070756,
123.991875626918)) ;
#75590=CARTESIAN_POINT('Ctrl Pts',(-18.2309896742037,-30.8984197556824,
124.351909547768)) ;
#75591=CARTESIAN_POINT('Ctrl Pts',(-18.4666381458969,-30.7184306752636,
124.163882156588)) ;
#75592=CARTESIAN_POINT('Ctrl Pts',(-18.4118327451986,-30.9084136586368,
124.542354351719)) ;
#75593=CARTESIAN_POINT('Ctrl Pts',(-18.6113111190892,-30.7284245782181,
124.316239274634)) ;
#75594=CARTESIAN_POINT('Ctrl Pts',(-18.6240784847576,-30.9184429437214,
124.698611210616)) ;
#75595=CARTESIAN_POINT('Ctrl Pts',(-18.78110661491,-30.7384538633026,124.441246278568)) ;
#75596=CARTESIAN_POINT('Ctrl Pts',(-18.8564336547717,-30.9283184721633,
124.814232094013)) ;
#75597=CARTESIAN_POINT('Ctrl Pts',(-18.96698940901,-30.7483293917445,124.533744474627)) ;
#75598=CARTESIAN_POINT('Ctrl Pts',(-19.1083519713404,-30.9383187547793,
124.888948210895)) ;
#75599=CARTESIAN_POINT('Ctrl Pts',(-19.168523414082,-30.7583296743606,124.593519235513)) ;
#75600=CARTESIAN_POINT('Ctrl Pts',(-19.3671515658178,-30.9482307708364,
124.918740815802)) ;
#75601=CARTESIAN_POINT('Ctrl Pts',(-19.3755624914892,-30.7682416904176,
124.617355261869)) ;
#75602=CARTESIAN_POINT('Ctrl Pts',(-19.6305583756984,-30.9582728461754,
124.903010863117)) ;
#75603=CARTESIAN_POINT('Ctrl Pts',(-19.5862881163539,-30.7782837657566,
124.604773299001)) ;
#75604=CARTESIAN_POINT('Ctrl Pts',(-19.883627140372,-30.9681726788315,124.842636497085)) ;
#75605=CARTESIAN_POINT('Ctrl Pts',(-19.7887432076105,-30.7881835984127,
124.55647584906)) ;
#75606=CARTESIAN_POINT('Ctrl Pts',(-20.1248202353474,-30.9781650794095,
124.738811837768)) ;
#75607=CARTESIAN_POINT('Ctrl Pts',(-19.9816984157365,-30.7981759989908,
124.473418063959)) ;
#75608=CARTESIAN_POINT('Ctrl Pts',(-20.3449819506754,-30.9881991011689,
124.593690835945)) ;
#75609=CARTESIAN_POINT('Ctrl Pts',(-20.157828908641,-30.8082100207501,124.357322942106)) ;
#75610=CARTESIAN_POINT('Ctrl Pts',(-20.5335886315247,-30.9980637120101,
124.415853378469)) ;
#75611=CARTESIAN_POINT('Ctrl Pts',(-20.3087153229984,-30.8180746315913,
124.215054797051)) ;
#75612=CARTESIAN_POINT('Ctrl Pts',(-20.6909778266609,-31.0080561114712,
124.205652827194)) ;
#75613=CARTESIAN_POINT('Ctrl Pts',(-20.4346283289395,-30.8280670310525,
124.046895699291)) ;
#75614=CARTESIAN_POINT('Ctrl Pts',(-20.8094832863514,-31.0180880648041,
123.970160489442)) ;
#75615=CARTESIAN_POINT('Ctrl Pts',(-20.5294345476933,-30.8380989843854,
123.85850276039)) ;
#75616=CARTESIAN_POINT('Ctrl Pts',(-20.8844320813034,-31.0279544237458,
123.721940205745)) ;
#75617=CARTESIAN_POINT('Ctrl Pts',(-20.5893954864046,-30.8479653433271,
123.659927538539)) ;
#75618=CARTESIAN_POINT('Ctrl Pts',(-20.9159397609847,-31.0379418992316,
123.461410041661)) ;
#75619=CARTESIAN_POINT('Ctrl Pts',(-20.6146037560401,-30.8579528188129,
123.451503763144)) ;
#75620=CARTESIAN_POINT('Ctrl Pts',(-20.901928788736,-31.0478868054201,123.200405236566)) ;
#75621=CARTESIAN_POINT('Ctrl Pts',(-20.6033971453962,-30.8678977250013,
123.242699989987)) ;
#75622=CARTESIAN_POINT('Ctrl Pts',(-20.8420850391347,-31.0579317700803,
122.943333258404)) ;
#75623=CARTESIAN_POINT('Ctrl Pts',(-20.5555242372743,-30.8779426896616,
123.037041905058)) ;
#75624=CARTESIAN_POINT('Ctrl Pts',(-20.740600364807,-31.0677935769852,122.704848430395)) ;
#75625=CARTESIAN_POINT('Ctrl Pts',(-20.4743386257341,-30.8878044965664,
122.846253507543)) ;
#75626=CARTESIAN_POINT('Ctrl Pts',(-20.5978221441658,-31.0777862492909,
122.484491140216)) ;
#75627=CARTESIAN_POINT('Ctrl Pts',(-20.3601179413071,-30.8977971688722,
122.669966539594)) ;
#75628=CARTESIAN_POINT('Ctrl Pts',(-20.4200444703825,-31.0877149202363,
122.293491950939)) ;
#75629=CARTESIAN_POINT('Ctrl Pts',(-20.2178975346058,-30.9077258398175,
122.517165820862)) ;
#75630=CARTESIAN_POINT('Ctrl Pts',(-20.2115893828335,-31.0976674624616,
122.135563380037)) ;
#75631=CARTESIAN_POINT('Ctrl Pts',(-20.0511349097933,-30.9176783820428,
122.390821266279)) ;
#75632=CARTESIAN_POINT('Ctrl Pts',(-19.9777608298646,-31.1076688184575,
122.015498299293)) ;
#75633=CARTESIAN_POINT('Ctrl Pts',(-19.864073138811,-30.9276797380387,122.29476724589)) ;
#75634=CARTESIAN_POINT('Ctrl Pts',(-19.72588370907,-31.1176974307322,121.938001760839)) ;
#75635=CARTESIAN_POINT('Ctrl Pts',(-19.6625721285863,-30.9377083503134,
122.2327679101)) ;
#75636=CARTESIAN_POINT('Ctrl Pts',(-19.4686784023186,-31.1275617652817,
121.905569609701)) ;
#75637=CARTESIAN_POINT('Ctrl Pts',(-19.4568083670694,-30.9475726848629,
122.206820002847)) ;
#75638=CARTESIAN_POINT('Ctrl Pts',(-19.2064222623086,-31.1375540893583,
121.918044378352)) ;
#75639=CARTESIAN_POINT('Ctrl Pts',(-19.2470034110608,-30.9575650089395,
122.21679756988)) ;
#75640=CARTESIAN_POINT('Ctrl Pts',(-18.9518724579804,-31.1474815817241,
121.975353810709)) ;
#75641=CARTESIAN_POINT('Ctrl Pts',(-19.043363176175,-30.9674925013054,122.262642901527)) ;
#75642=CARTESIAN_POINT('Ctrl Pts',(-18.7087875924744,-31.157508940275,122.076985697082)) ;
#75643=CARTESIAN_POINT('Ctrl Pts',(-18.8488944626726,-30.9775198598562,
122.343946315082)) ;
#75644=CARTESIAN_POINT('Ctrl Pts',(-18.489949403091,-31.1673953583261,122.217086575925)) ;
#75645=CARTESIAN_POINT('Ctrl Pts',(-18.6738227767691,-30.9874062779074,
122.456025072437)) ;
#75646=CARTESIAN_POINT('Ctrl Pts',(-18.2959218217768,-31.1774270930615,
122.395489361703)) ;
#75647=CARTESIAN_POINT('Ctrl Pts',(-18.5185992246313,-30.9974380126427,
122.59874560302)) ;
#75648=CARTESIAN_POINT('Ctrl Pts',(-18.1379570317047,-31.1873086743047,
122.601654224037)) ;
#75649=CARTESIAN_POINT('Ctrl Pts',(-18.3922256360828,-31.007319593886,122.763676083483)) ;
#75650=CARTESIAN_POINT('Ctrl Pts',(-18.0159864387132,-31.1973706523371,
122.836214609543)) ;
#75651=CARTESIAN_POINT('Ctrl Pts',(-18.2946471919646,-31.0173815719183,
122.951323289987)) ;
#75652=CARTESIAN_POINT('Ctrl Pts',(-17.9380997061781,-31.2072277306988,
123.083299705071)) ;
#75653=CARTESIAN_POINT('Ctrl Pts',(-18.2323356602816,-31.02723865028,123.148990682481)) ;
#75654=CARTESIAN_POINT('Ctrl Pts',(-17.9033134791433,-31.2172223038048,
123.343589981841)) ;
#75655=CARTESIAN_POINT('Ctrl Pts',(-18.204504458958,-31.037233223386,123.357222569661)) ;
#75656=CARTESIAN_POINT('Ctrl Pts',(-17.9140838362629,-31.2271481000924,
123.604243273491)) ;
#75657=CARTESIAN_POINT('Ctrl Pts',(-18.2131185010766,-31.0471590196736,
123.565745298409)) ;
#75658=CARTESIAN_POINT('Ctrl Pts',(-17.9704288396059,-31.2371734672621,
123.861581949271)) ;
#75659=CARTESIAN_POINT('Ctrl Pts',(-18.2581923330531,-31.0571843868434,
123.77161667508)) ;
#75660=CARTESIAN_POINT('Ctrl Pts',(-18.0692181289341,-31.247069546916,124.102157307111)) ;
#75661=CARTESIAN_POINT('Ctrl Pts',(-18.3372216027186,-31.0670804664972,
123.964077752132)) ;
#75662=CARTESIAN_POINT('Ctrl Pts',(-18.2092168772367,-31.2570646266215,
124.324401075044)) ;
#75663=CARTESIAN_POINT('Ctrl Pts',(-18.4492191754673,-31.0770755462028,
124.141874372406)) ;
#75664=CARTESIAN_POINT('Ctrl Pts',(-18.3865390045604,-31.2670897144374,
124.519239586953)) ;
#75665=CARTESIAN_POINT('Ctrl Pts',(-18.5910734554309,-31.0871006340186,
124.297744917431)) ;
#75666=CARTESIAN_POINT('Ctrl Pts',(-18.6602990640398,-31.2802735368046,
124.731576473169)) ;
#75667=CARTESIAN_POINT('Ctrl Pts',(-18.8100883440291,-31.1002844563859,
124.46762529973)) ;
#75668=CARTESIAN_POINT('Ctrl Pts',(-18.9862948594046,-31.2935956549506,
124.869711357403)) ;
#75669=CARTESIAN_POINT('Ctrl Pts',(-19.0709153826081,-31.1136065745318,
124.578138411476)) ;
#75670=CARTESIAN_POINT('Ctrl Pts',(-19.3347015527529,-31.3069748645782,
124.917347223271)) ;
#75671=CARTESIAN_POINT('Ctrl Pts',(-19.3495941692662,-31.1269857841594,
124.616238563571)) ;
#75672=CARTESIAN_POINT('Ctrl Pts',(-19.5930836021326,-31.3168131018224,
124.908057132402)) ;
#75673=CARTESIAN_POINT('Ctrl Pts',(-19.5563095018621,-31.1368240214036,
124.608810852484)) ;
#75674=CARTESIAN_POINT('Ctrl Pts',(-19.8519437779512,-31.3268860250811,
124.852876717785)) ;
#75675=CARTESIAN_POINT('Ctrl Pts',(-19.7633952063794,-31.1468969446624,
124.564668365869)) ;
#75676=CARTESIAN_POINT('Ctrl Pts',(-20.0920602273385,-31.3367426665362,
124.755670606762)) ;
#75677=CARTESIAN_POINT('Ctrl Pts',(-19.9554908730702,-31.1567535861175,
124.486904328256)) ;
#75678=CARTESIAN_POINT('Ctrl Pts',(-20.3148623984848,-31.3467280420423,
124.617067390119)) ;
#75679=CARTESIAN_POINT('Ctrl Pts',(-20.1337308377886,-31.1667389616235,
124.376027861451)) ;
#75680=CARTESIAN_POINT('Ctrl Pts',(-20.5745088880156,-31.3600120735027,
124.383813943034)) ;
#75681=CARTESIAN_POINT('Ctrl Pts',(-20.3414635227013,-31.180022993084,124.18940523939)) ;
#75682=CARTESIAN_POINT('Ctrl Pts',(-20.8154916493389,-31.376530865373,124.016626072698)) ;
#75683=CARTESIAN_POINT('Ctrl Pts',(-20.5342357532926,-31.1965417849543,
123.895695702942)) ;
#75684=CARTESIAN_POINT('Ctrl Pts',(-20.917307049365,-31.3933165823797,123.582394229594)) ;
#75685=CARTESIAN_POINT('Ctrl Pts',(-20.6157025962168,-31.2133275019609,
123.548246263072)) ;
#75686=CARTESIAN_POINT('Ctrl Pts',(-20.90651529499,-31.4064297308887,123.237879258047)) ;
#75687=CARTESIAN_POINT('Ctrl Pts',(-20.6070652302265,-31.2264406504699,
123.272686121829)) ;
#75688=CARTESIAN_POINT('Ctrl Pts',(-20.8536524124441,-31.4164652799689,
122.979546305383)) ;
#75689=CARTESIAN_POINT('Ctrl Pts',(-20.56477758318,-31.2364761995501,123.066008431127)) ;
#75690=CARTESIAN_POINT('Ctrl Pts',(-20.7561932614657,-31.4264813361483,
122.735008678748)) ;
#75691=CARTESIAN_POINT('Ctrl Pts',(-20.4868138633641,-31.2464922557295,
122.870382595949)) ;
#75692=CARTESIAN_POINT('Ctrl Pts',(-20.574735633146,-31.4396593720143,122.440107128118)) ;
#75693=CARTESIAN_POINT('Ctrl Pts',(-20.3416392942912,-31.2596702915955,
122.634448243853)) ;
#75694=CARTESIAN_POINT('Ctrl Pts',(-20.2550642401777,-31.4562612492014,
122.135837120559)) ;
#75695=CARTESIAN_POINT('Ctrl Pts',(-20.0859155602014,-31.2762721687826,
122.391041933051)) ;
#75696=CARTESIAN_POINT('Ctrl Pts',(-19.7659328720119,-31.4763243938173,
121.923514400655)) ;
#75697=CARTESIAN_POINT('Ctrl Pts',(-19.6946085896363,-31.2963353133985,
122.221176679855)) ;
#75698=CARTESIAN_POINT('Ctrl Pts',(-19.2406043647769,-31.496125283901,121.890949553515)) ;
#75699=CARTESIAN_POINT('Ctrl Pts',(-19.2743458623151,-31.3161362034822,
122.195122232715)) ;
#75700=CARTESIAN_POINT('Ctrl Pts',(-18.7318418664049,-31.5160684091797,
122.039356586139)) ;
#75701=CARTESIAN_POINT('Ctrl Pts',(-18.8673343450499,-31.3360793287609,
122.313844690629)) ;
#75702=CARTESIAN_POINT('Ctrl Pts',(-18.3053752398977,-31.5359664542993,
122.35209220287)) ;
#75703=CARTESIAN_POINT('Ctrl Pts',(-18.5261587181132,-31.3559773738805,
122.564031167843)) ;
#75704=CARTESIAN_POINT('Ctrl Pts',(-18.010266411361,-31.555852213926,122.79064987689)) ;
#75705=CARTESIAN_POINT('Ctrl Pts',(-18.2900689875788,-31.3758631335073,
122.914876579139)) ;
#75706=CARTESIAN_POINT('Ctrl Pts',(-17.8822137796121,-31.5759173891059,
123.308303291764)) ;
#75707=CARTESIAN_POINT('Ctrl Pts',(-18.1876243873306,-31.3959283086872,
123.328998110787)) ;
#75708=CARTESIAN_POINT('Ctrl Pts',(-17.9380242802495,-31.5957440322087,
123.832388879127)) ;
#75709=CARTESIAN_POINT('Ctrl Pts',(-18.2322702877505,-31.41575495179,123.748268249303)) ;
#75710=CARTESIAN_POINT('Ctrl Pts',(-18.1688732799424,-31.6156527416571,
124.308361931738)) ;
#75711=CARTESIAN_POINT('Ctrl Pts',(-18.4169480416883,-31.4356636612383,
124.129048386258)) ;
#75712=CARTESIAN_POINT('Ctrl Pts',(-18.5492284834429,-31.6356045786889,
124.678079899734)) ;
#75713=CARTESIAN_POINT('Ctrl Pts',(-18.7212312265001,-31.4556154982701,
124.424824341634)) ;
#75714=CARTESIAN_POINT('Ctrl Pts',(-19.0344540489787,-31.655613053392,124.895564294093)) ;
#75715=CARTESIAN_POINT('Ctrl Pts',(-19.1094107625724,-31.4756239729733,
124.598813645085)) ;
#75716=CARTESIAN_POINT('Ctrl Pts',(-19.5593044714974,-31.6754145121535,
124.9346386812)) ;
#75717=CARTESIAN_POINT('Ctrl Pts',(-19.529293065133,-31.4954254317348,124.630074897987)) ;
#75718=CARTESIAN_POINT('Ctrl Pts',(-20.0703188207623,-31.6953714003894,
124.792477849168)) ;
#75719=CARTESIAN_POINT('Ctrl Pts',(-19.9381052599703,-31.5153823199707,
124.516346913691)) ;
#75720=CARTESIAN_POINT('Ctrl Pts',(-20.5020147231409,-31.7153552378035,
124.483083841994)) ;
#75721=CARTESIAN_POINT('Ctrl Pts',(-20.2834628020649,-31.5353661573848,
124.268832576871)) ;
#75722=CARTESIAN_POINT('Ctrl Pts',(-20.8005129694073,-31.7351636770245,
124.049324638375)) ;
#75723=CARTESIAN_POINT('Ctrl Pts',(-20.5222631468944,-31.5551745966057,
123.921823569577)) ;
#75724=CARTESIAN_POINT('Ctrl Pts',(-20.9347328466543,-31.7551493864047,
123.535538119664)) ;
#75725=CARTESIAN_POINT('Ctrl Pts',(-20.629639166781,-31.5751603059859,123.510794112745)) ;
#75726=CARTESIAN_POINT('Ctrl Pts',(-20.8859933952237,-31.77501890942,123.009476827428)) ;
#75727=CARTESIAN_POINT('Ctrl Pts',(-20.5906472054233,-31.5950298290012,
123.089943545706)) ;
#75728=CARTESIAN_POINT('Ctrl Pts',(-20.6589290213738,-31.7950396485372,
122.528458277119)) ;
#75729=CARTESIAN_POINT('Ctrl Pts',(-20.4089954572022,-31.6150505681184,
122.705129026127)) ;
#75730=CARTESIAN_POINT('Ctrl Pts',(-20.2856318117537,-31.8148437135141,
122.157092624958)) ;
#75731=CARTESIAN_POINT('Ctrl Pts',(-20.1103554752544,-31.6348546330954,
122.408035494353)) ;
#75732=CARTESIAN_POINT('Ctrl Pts',(-19.8021889397238,-31.8349056772449,
121.932500294407)) ;
#75733=CARTESIAN_POINT('Ctrl Pts',(-19.7236013288936,-31.6549165968261,
122.228362959859)) ;
#75734=CARTESIAN_POINT('Ctrl Pts',(-19.2768672597624,-31.8547388575334,
121.887382590685)) ;
#75735=CARTESIAN_POINT('Ctrl Pts',(-19.3033420853306,-31.6747497771146,
122.192269707988)) ;
#75736=CARTESIAN_POINT('Ctrl Pts',(-18.7652950498468,-31.8746580548595,
122.023339535084)) ;
#75737=CARTESIAN_POINT('Ctrl Pts',(-18.894083985732,-31.6946689744407,122.301037293139)) ;
#75738=CARTESIAN_POINT('Ctrl Pts',(-18.3305352276094,-31.8945960799728,
122.326324931623)) ;
#75739=CARTESIAN_POINT('Ctrl Pts',(-18.5462767220526,-31.714606999554,122.543427492195)) ;
#75740=CARTESIAN_POINT('Ctrl Pts',(-18.0255423059976,-31.9144741260288,
122.757789608144)) ;
#75741=CARTESIAN_POINT('Ctrl Pts',(-18.3022836422757,-31.7344850456101,
122.888601425754)) ;
#75742=CARTESIAN_POINT('Ctrl Pts',(-17.8853325730449,-31.9344588603169,
123.270040998402)) ;
#75743=CARTESIAN_POINT('Ctrl Pts',(-18.190118198044,-31.7544697798982,123.298403291928)) ;
#75744=CARTESIAN_POINT('Ctrl Pts',(-17.928106557401,-31.9543696769954,123.797659471947)) ;
#75745=CARTESIAN_POINT('Ctrl Pts',(-18.2243400264694,-31.7743805965766,
123.720498525304)) ;
#75746=CARTESIAN_POINT('Ctrl Pts',(-18.1495333781648,-31.9743686525141,
124.280744001263)) ;
#75747=CARTESIAN_POINT('Ctrl Pts',(-18.4014839037645,-31.7943795720954,
124.106965091444)) ;
#75748=CARTESIAN_POINT('Ctrl Pts',(-18.5185878610474,-31.9941735731593,
124.656228575468)) ;
#75749=CARTESIAN_POINT('Ctrl Pts',(-18.6967305737938,-31.8141844927406,
124.407351675959)) ;
#75750=CARTESIAN_POINT('Ctrl Pts',(-18.9973682959975,-32.0141575334505,
124.885894562738)) ;
#75751=CARTESIAN_POINT('Ctrl Pts',(-19.0797564164797,-31.8341684530318,
124.59108154804)) ;
#75752=CARTESIAN_POINT('Ctrl Pts',(-19.5234477413655,-32.0340437371745,
124.937928873711)) ;
#75753=CARTESIAN_POINT('Ctrl Pts',(-19.5006209678039,-31.8540546567557,
124.632705726637)) ;
#75754=CARTESIAN_POINT('Ctrl Pts',(-20.0373301586024,-32.0539929154977,
124.807521706243)) ;
#75755=CARTESIAN_POINT('Ctrl Pts',(-19.9117263038171,-31.8740038350789,
124.528376628622)) ;
#75756=CARTESIAN_POINT('Ctrl Pts',(-20.4747803851677,-32.0738947147372,
124.510171457497)) ;
#75757=CARTESIAN_POINT('Ctrl Pts',(-20.261684750146,-31.8939056343185,124.290492599356)) ;
#75758=CARTESIAN_POINT('Ctrl Pts',(-20.7850691733475,-32.0937733197896,
124.082510674335)) ;
#75759=CARTESIAN_POINT('Ctrl Pts',(-20.5099133229686,-31.9137842393708,
123.948363354658)) ;
#75760=CARTESIAN_POINT('Ctrl Pts',(-20.9316880819993,-32.1138056795153,
123.570639458994)) ;
#75761=CARTESIAN_POINT('Ctrl Pts',(-20.6272030682315,-31.9338165990965,
123.538857703905)) ;
#75762=CARTESIAN_POINT('Ctrl Pts',(-20.9004840929352,-32.1303874054713,
123.131013871463)) ;
#75763=CARTESIAN_POINT('Ctrl Pts',(-20.6022414356194,-31.9503983250526,
123.18718139994)) ;
#75764=CARTESIAN_POINT('Ctrl Pts',(-20.7882628388064,-32.1435815757693,
122.802971043157)) ;
#75765=CARTESIAN_POINT('Ctrl Pts',(-20.5124528334552,-31.9635924953505,
122.924720353763)) ;
#75766=CARTESIAN_POINT('Ctrl Pts',(-20.6197762199755,-32.1568937538625,
122.49638698779)) ;
#75767=CARTESIAN_POINT('Ctrl Pts',(-20.3776944292789,-31.9769046734437,
122.679499995801)) ;
#75768=CARTESIAN_POINT('Ctrl Pts',(-20.315208446771,-32.1734599334558,122.178383590864)) ;
#75769=CARTESIAN_POINT('Ctrl Pts',(-20.1339927311637,-31.9934708530371,
122.425047213569)) ;
#75770=CARTESIAN_POINT('Ctrl Pts',(-19.919195114621,-32.190088128316,121.982318683978)) ;
#75771=CARTESIAN_POINT('Ctrl Pts',(-19.8172191413778,-32.0100990478972,
122.268225564694)) ;
#75772=CARTESIAN_POINT('Ctrl Pts',(-19.5767420543865,-32.2033767100257,
121.913670003238)) ;
#75773=CARTESIAN_POINT('Ctrl Pts',(-19.5432298830773,-32.023387629607,122.21329620248)) ;
#75774=CARTESIAN_POINT('Ctrl Pts',(-19.3148866166787,-32.2133449581293,
121.907334290393)) ;
#75775=CARTESIAN_POINT('Ctrl Pts',(-19.3337508380696,-32.0333558777106,
122.208232314246)) ;
#75776=CARTESIAN_POINT('Ctrl Pts',(-19.0572238635759,-32.2232597143854,
121.946033185514)) ;
#75777=CARTESIAN_POINT('Ctrl Pts',(-19.1276189170704,-32.0432706339667,
122.239193494291)) ;
#75778=CARTESIAN_POINT('Ctrl Pts',(-18.8076409322164,-32.2332728650367,
122.029433371306)) ;
#75779=CARTESIAN_POINT('Ctrl Pts',(-18.9279556714256,-32.0532837846179,
122.305913714308)) ;
#75780=CARTESIAN_POINT('Ctrl Pts',(-18.5765593856739,-32.2432855722387,
122.155251712084)) ;
#75781=CARTESIAN_POINT('Ctrl Pts',(-18.7430841787746,-32.0632964918199,
122.406578419691)) ;
#75782=CARTESIAN_POINT('Ctrl Pts',(-18.3044914721086,-32.25650486093,122.37133980811)) ;
#75783=CARTESIAN_POINT('Ctrl Pts',(-18.5254677230784,-32.0765157805112,
122.579410561966)) ;
#75784=CARTESIAN_POINT('Ctrl Pts',(-18.0412520384418,-32.273123541928,122.725865755981)) ;
#75785=CARTESIAN_POINT('Ctrl Pts',(-18.3148360322381,-32.0931344615093,
122.863088795251)) ;
#75786=CARTESIAN_POINT('Ctrl Pts',(-17.9146049569576,-32.2896884497015,
123.147620680719)) ;
#75787=CARTESIAN_POINT('Ctrl Pts',(-18.2135427847506,-32.1096993692827,
123.200444214174)) ;
#75788=CARTESIAN_POINT('Ctrl Pts',(-17.9043631044386,-32.3030869213123,
123.499558748907)) ;
#75789=CARTESIAN_POINT('Ctrl Pts',(-18.2053428096442,-32.1230978408936,
123.482028671522)) ;
#75790=CARTESIAN_POINT('Ctrl Pts',(-17.9415874188151,-32.3129281767992,
123.755505137572)) ;
#75791=CARTESIAN_POINT('Ctrl Pts',(-18.2351264004454,-32.1329390963805,
123.686778655729)) ;
#75792=CARTESIAN_POINT('Ctrl Pts',(-18.0233154439274,-32.3229144923875,
124.004839610879)) ;
#75793=CARTESIAN_POINT('Ctrl Pts',(-18.3005104402209,-32.1429254119687,
123.886247298971)) ;
#75794=CARTESIAN_POINT('Ctrl Pts',(-18.1464078762441,-32.3328510999739,
124.235179732751)) ;
#75795=CARTESIAN_POINT('Ctrl Pts',(-18.3989864852805,-32.1528620195551,
124.070517791497)) ;
#75796=CARTESIAN_POINT('Ctrl Pts',(-18.3095220074797,-32.3429009673422,
124.442853309924)) ;
#75797=CARTESIAN_POINT('Ctrl Pts',(-18.5294795023595,-32.1629118869234,
124.23665535116)) ;
#75798=CARTESIAN_POINT('Ctrl Pts',(-18.5022200305322,-32.352751462017,124.615730119518)) ;
#75799=CARTESIAN_POINT('Ctrl Pts',(-18.6836393679515,-32.1727623815982,
124.374955019593)) ;
#75800=CARTESIAN_POINT('Ctrl Pts',(-18.7243070866901,-32.3627232624115,
124.754758703719)) ;
#75801=CARTESIAN_POINT('Ctrl Pts',(-18.8613101252405,-32.1827341819927,
124.486175940165)) ;
#75802=CARTESIAN_POINT('Ctrl Pts',(-18.9678327868279,-32.3727192294373,
124.853354582508)) ;
#75803=CARTESIAN_POINT('Ctrl Pts',(-19.0561314683988,-32.1927301490186,
124.565050536217)) ;
#75804=CARTESIAN_POINT('Ctrl Pts',(-19.2258519489846,-32.3827566888185,
124.908029994952)) ;
#75805=CARTESIAN_POINT('Ctrl Pts',(-19.2625472401696,-32.2027676083997,
124.608788652274)) ;
#75806=CARTESIAN_POINT('Ctrl Pts',(-19.4843048557943,-32.3925973897192,
124.917387851488)) ;
#75807=CARTESIAN_POINT('Ctrl Pts',(-19.4693094439586,-32.2126083093005,
124.616272690437)) ;
#75808=CARTESIAN_POINT('Ctrl Pts',(-19.7458762677013,-32.4026454109866,
124.881367125356)) ;
#75809=CARTESIAN_POINT('Ctrl Pts',(-19.6785662481788,-32.2226563305678,
124.587453906341)) ;
#75810=CARTESIAN_POINT('Ctrl Pts',(-19.9945882738424,-32.4125928040693,
124.800883482225)) ;
#75811=CARTESIAN_POINT('Ctrl Pts',(-19.8775350535338,-32.2326037236505,
124.523064890071)) ;
#75812=CARTESIAN_POINT('Ctrl Pts',(-20.2250646864161,-32.4225029501157,
124.679595400732)) ;
#75813=CARTESIAN_POINT('Ctrl Pts',(-20.0619149780218,-32.2425138696969,
124.426032565424)) ;
#75814=CARTESIAN_POINT('Ctrl Pts',(-20.4338556735441,-32.4325618639653,
124.517526669019)) ;
#75815=CARTESIAN_POINT('Ctrl Pts',(-20.2289464252875,-32.2525727835465,
124.296375807091)) ;
#75816=CARTESIAN_POINT('Ctrl Pts',(-20.6077963924508,-32.4424026342546,
124.326112710834)) ;
#75817=CARTESIAN_POINT('Ctrl Pts',(-20.3680971502017,-32.2624135538358,
124.143243405943)) ;
#75818=CARTESIAN_POINT('Ctrl Pts',(-20.7492002051282,-32.4524655038332,
124.102692225391)) ;
#75819=CARTESIAN_POINT('Ctrl Pts',(-20.4812183762259,-32.2724764234145,
123.964505819681)) ;
#75820=CARTESIAN_POINT('Ctrl Pts',(-20.8478072363994,-32.4623598269637,
123.862073047609)) ;
#75821=CARTESIAN_POINT('Ctrl Pts',(-20.5601018691605,-32.2823707465449,
123.772009890152)) ;
#75822=CARTESIAN_POINT('Ctrl Pts',(-20.9040808602979,-32.4723016340582,
123.606978235606)) ;
#75823=CARTESIAN_POINT('Ctrl Pts',(-20.6051186298419,-32.2923125536394,
123.567933786065)) ;
#75824=CARTESIAN_POINT('Ctrl Pts',(-20.9153764258994,-32.4823041450135,
123.344329862465)) ;
#75825=CARTESIAN_POINT('Ctrl Pts',(-20.6141529513669,-32.3023150645948,
123.357815062894)) ;
#75826=CARTESIAN_POINT('Ctrl Pts',(-20.8803820948973,-32.4923388658319,
123.082976330984)) ;
#75827=CARTESIAN_POINT('Ctrl Pts',(-20.5861553344511,-32.3123497854131,
123.148732512367)) ;
#75828=CARTESIAN_POINT('Ctrl Pts',(-20.8024460213964,-32.5021840433376,
122.83625706858)) ;
#75829=CARTESIAN_POINT('Ctrl Pts',(-20.5238045816804,-32.3221949629189,
122.951358176035)) ;
#75830=CARTESIAN_POINT('Ctrl Pts',(-20.6816420858967,-32.5121688037387,
122.603373026564)) ;
#75831=CARTESIAN_POINT('Ctrl Pts',(-20.427159646758,-32.3321797233199,122.765052018463)) ;
#75832=CARTESIAN_POINT('Ctrl Pts',(-20.5230220508971,-32.5221077100551,
122.395822102381)) ;
#75833=CARTESIAN_POINT('Ctrl Pts',(-20.3002621303212,-32.3421186296363,
122.59901272905)) ;
#75834=CARTESIAN_POINT('Ctrl Pts',(-20.328762472991,-32.5321499376908,122.217239391527)) ;
#75835=CARTESIAN_POINT('Ctrl Pts',(-20.1448530337361,-32.3521608572721,
122.456148061873)) ;
#75836=CARTESIAN_POINT('Ctrl Pts',(-20.1099755421351,-32.5420351492752,
122.077133850334)) ;
#75837=CARTESIAN_POINT('Ctrl Pts',(-19.9698227394801,-32.3620460688564,
122.344065585937)) ;
#75838=CARTESIAN_POINT('Ctrl Pts',(-19.8676198087707,-32.5520340794771,
121.975708802739)) ;
#75839=CARTESIAN_POINT('Ctrl Pts',(-19.7759374551782,-32.3720449990584,
122.262927442215)) ;
#75840=CARTESIAN_POINT('Ctrl Pts',(-19.6133877400245,-32.5619515023875,
121.918164610149)) ;
#75841=CARTESIAN_POINT('Ctrl Pts',(-19.5725517025332,-32.3819624219688,
122.216894103057)) ;
#75842=CARTESIAN_POINT('Ctrl Pts',(-19.3496802081927,-32.5719994344663,
121.90552817767)) ;
#75843=CARTESIAN_POINT('Ctrl Pts',(-19.3615855024817,-32.3920103540475,
122.206786949623)) ;
#75844=CARTESIAN_POINT('Ctrl Pts',(-19.0921154350344,-32.5818768102757,
121.938063647329)) ;
#75845=CARTESIAN_POINT('Ctrl Pts',(-19.1555344414447,-32.4018877298569,
122.232817207828)) ;
#75846=CARTESIAN_POINT('Ctrl Pts',(-18.8397271603411,-32.5919307034436,
122.016043063016)) ;
#75847=CARTESIAN_POINT('Ctrl Pts',(-18.9536242958656,-32.4119416230248,
122.295202630568)) ;
#75848=CARTESIAN_POINT('Ctrl Pts',(-18.6083164557065,-32.6018243266969,
122.13467532395)) ;
#75849=CARTESIAN_POINT('Ctrl Pts',(-18.7684970311458,-32.4218352462781,
122.390109938702)) ;
#75850=CARTESIAN_POINT('Ctrl Pts',(-18.3975309341111,-32.6118869203199,
122.294276744081)) ;
#75851=CARTESIAN_POINT('Ctrl Pts',(-18.5998696580958,-32.4318978399011,
122.517792698231)) ;
#75852=CARTESIAN_POINT('Ctrl Pts',(-18.2214436963193,-32.6217294943089,
122.48377741207)) ;
#75853=CARTESIAN_POINT('Ctrl Pts',(-18.4590017343272,-32.4417404138902,
122.669394019431)) ;
#75854=CARTESIAN_POINT('Ctrl Pts',(-18.0783294581763,-32.6317202511919,
122.703848805857)) ;
#75855=CARTESIAN_POINT('Ctrl Pts',(-18.3445119383423,-32.4517311707731,
122.845452004202)) ;
#75856=CARTESIAN_POINT('Ctrl Pts',(-17.9762694761468,-32.6416483129498,
122.943971098635)) ;
#75857=CARTESIAN_POINT('Ctrl Pts',(-18.2628657760219,-32.4616592325311,
123.037550188827)) ;
#75858=CARTESIAN_POINT('Ctrl Pts',(-17.9166533726252,-32.651636288839,123.199595350727)) ;
#75859=CARTESIAN_POINT('Ctrl Pts',(-18.2151746225017,-32.4716472084202,
123.242049843833)) ;
#75860=CARTESIAN_POINT('Ctrl Pts',(-17.9027006001273,-32.6616719531954,
123.462944824452)) ;
#75861=CARTESIAN_POINT('Ctrl Pts',(-18.2040142137418,-32.4816828727767,
123.452729587914)) ;
#75862=CARTESIAN_POINT('Ctrl Pts',(-17.9337120200505,-32.6715278916151,
123.720099296873)) ;
#75863=CARTESIAN_POINT('Ctrl Pts',(-18.2288249953322,-32.4915388111963,
123.658452229222)) ;
#75864=CARTESIAN_POINT('Ctrl Pts',(-18.009543101107,-32.681523383012,123.971557376354)) ;
#75865=CARTESIAN_POINT('Ctrl Pts',(-18.2894914284038,-32.5015343025932,
123.859618092693)) ;
#75866=CARTESIAN_POINT('Ctrl Pts',(-18.1268171254845,-32.6914331879654,
124.204090672369)) ;
#75867=CARTESIAN_POINT('Ctrl Pts',(-18.3833118888715,-32.5114441075467,
124.045643510793)) ;
#75868=CARTESIAN_POINT('Ctrl Pts',(-18.283949331049,-32.7014454102322,124.415135395342)) ;
#75869=CARTESIAN_POINT('Ctrl Pts',(-18.509018896985,-32.5214563298134,124.214478314619)) ;
#75870=CARTESIAN_POINT('Ctrl Pts',(-18.4759885041696,-32.711473290925,124.595595889939)) ;
#75871=CARTESIAN_POINT('Ctrl Pts',(-18.6626514215253,-32.5314842105063,
124.358845523371)) ;
#75872=CARTESIAN_POINT('Ctrl Pts',(-18.6924294796263,-32.7213296869076,
124.737869480945)) ;
#75873=CARTESIAN_POINT('Ctrl Pts',(-18.8358044087005,-32.5413406064889,
124.472662626393)) ;
#75874=CARTESIAN_POINT('Ctrl Pts',(-18.9341360919436,-32.7313544840876,
124.842659911691)) ;
#75875=CARTESIAN_POINT('Ctrl Pts',(-19.0291703120113,-32.5513654036688,
124.556493611938)) ;
#75876=CARTESIAN_POINT('Ctrl Pts',(-19.1906775296602,-32.7413854140714,
124.903298738931)) ;
#75877=CARTESIAN_POINT('Ctrl Pts',(-19.2344038900453,-32.5613963336526,
124.605003114696)) ;
#75878=CARTESIAN_POINT('Ctrl Pts',(-19.4489157332654,-32.7512300165801,
124.918654695637)) ;
#75879=CARTESIAN_POINT('Ctrl Pts',(-19.4409936483921,-32.5712409361613,
124.617286306339)) ;
#75880=CARTESIAN_POINT('Ctrl Pts',(-19.7098139114715,-32.7612208678041,
124.889204775751)) ;
#75881=CARTESIAN_POINT('Ctrl Pts',(-19.6497118803502,-32.5812317873854,
124.593725014445)) ;
#75882=CARTESIAN_POINT('Ctrl Pts',(-19.9626440102893,-32.7712587008154,
124.81398793579)) ;
#75883=CARTESIAN_POINT('Ctrl Pts',(-19.8519756339455,-32.5912696203966,
124.533550073541)) ;
#75884=CARTESIAN_POINT('Ctrl Pts',(-20.1942400544796,-32.7811030892808,
124.698686780545)) ;
#75885=CARTESIAN_POINT('Ctrl Pts',(-20.037251000993,-32.6011140088621,124.441308307128)) ;
#75886=CARTESIAN_POINT('Ctrl Pts',(-20.4055373690986,-32.7910878936504,
124.543175419244)) ;
#75887=CARTESIAN_POINT('Ctrl Pts',(-20.2062879201296,-32.6110988132316,
124.316898288086)) ;
#75888=CARTESIAN_POINT('Ctrl Pts',(-20.5859328055609,-32.8010274131332,
124.354225946047)) ;
#75889=CARTESIAN_POINT('Ctrl Pts',(-20.3506030458168,-32.6210383327145,
124.16573814407)) ;
#75890=CARTESIAN_POINT('Ctrl Pts',(-20.7321570745328,-32.8110671441346,
124.134645385884)) ;
#75891=CARTESIAN_POINT('Ctrl Pts',(-20.4675814518196,-32.6310780637158,
123.990072882451)) ;
#75892=CARTESIAN_POINT('Ctrl Pts',(-20.8365696228961,-32.8209552723808,
123.896678841606)) ;
#75893=CARTESIAN_POINT('Ctrl Pts',(-20.551110037506,-32.6409661919621,123.79969981623)) ;
#75894=CARTESIAN_POINT('Ctrl Pts',(-20.8991776004823,-32.8309449975894,
123.641744550602)) ;
#75895=CARTESIAN_POINT('Ctrl Pts',(-20.6011952561969,-32.6509559171706,
123.595752273945)) ;
#75896=CARTESIAN_POINT('Ctrl Pts',(-20.9163259244539,-32.8409027622909,
123.380631029216)) ;
#75897=CARTESIAN_POINT('Ctrl Pts',(-20.6149126952404,-32.6609136818721,
123.386861725222)) ;
#75898=CARTESIAN_POINT('Ctrl Pts',(-20.8886398162672,-32.8508051037029,
123.121875613557)) ;
#75899=CARTESIAN_POINT('Ctrl Pts',(-20.5927628294816,-32.6708160232841,
123.179858200967)) ;
#75900=CARTESIAN_POINT('Ctrl Pts',(-20.8153934382436,-32.8608492994093,
122.868304834819)) ;
#75901=CARTESIAN_POINT('Ctrl Pts',(-20.5341646599949,-32.6808602189905,
122.977001723796)) ;
#75902=CARTESIAN_POINT('Ctrl Pts',(-20.7008271859404,-32.8707567001685,
122.634494488464)) ;
#75903=CARTESIAN_POINT('Ctrl Pts',(-20.4425109923345,-32.6907676197498,
122.789954502378)) ;
#75904=CARTESIAN_POINT('Ctrl Pts',(-20.546186232059,-32.8807673000429,122.421673048504)) ;
#75905=CARTESIAN_POINT('Ctrl Pts',(-20.3187974795829,-32.7007782196241,
122.619697941561)) ;
#75906=CARTESIAN_POINT('Ctrl Pts',(-20.3562127677178,-32.8907975959551,
122.238939688414)) ;
#75907=CARTESIAN_POINT('Ctrl Pts',(-20.1668179033373,-32.7108085155363,
122.473511971535)) ;
#75908=CARTESIAN_POINT('Ctrl Pts',(-20.1414444851977,-32.9006523756048,
122.094253937505)) ;
#75909=CARTESIAN_POINT('Ctrl Pts',(-19.9950035629509,-32.720663295186,122.35776475964)) ;
#75910=CARTESIAN_POINT('Ctrl Pts',(-19.9026572208849,-32.9106097038223,
121.98722381841)) ;
#75911=CARTESIAN_POINT('Ctrl Pts',(-19.8039737675108,-32.7306206234035,
122.272141549309)) ;
#75912=CARTESIAN_POINT('Ctrl Pts',(-19.6467435512294,-32.9206487367292,
121.923215339436)) ;
#75913=CARTESIAN_POINT('Ctrl Pts',(-19.5992424816828,-32.7406596563104,
122.220935620064)) ;
#75914=CARTESIAN_POINT('Ctrl Pts',(-19.3879265897754,-32.9305218486184,
121.904435880126)) ;
#75915=CARTESIAN_POINT('Ctrl Pts',(-19.3921897535148,-32.7505327681997,
122.205912911945)) ;
#75916=CARTESIAN_POINT('Ctrl Pts',(-19.1246518187911,-32.9405951336456,
121.931486510168)) ;
#75917=CARTESIAN_POINT('Ctrl Pts',(-19.18156967997,-32.7606060532268,122.227554264233)) ;
#75918=CARTESIAN_POINT('Ctrl Pts',(-18.8762664626963,-32.9504154533823,
122.001727342431)) ;
#75919=CARTESIAN_POINT('Ctrl Pts',(-18.9828627923026,-32.7704263729636,
122.283747296942)) ;
#75920=CARTESIAN_POINT('Ctrl Pts',(-18.6377418414705,-32.9604941187608,
122.116709479885)) ;
#75921=CARTESIAN_POINT('Ctrl Pts',(-18.7920430490926,-32.780505038342,122.375733780278)) ;
#75922=CARTESIAN_POINT('Ctrl Pts',(-18.4274927506515,-32.9703457092446,
122.267875972301)) ;
#75923=CARTESIAN_POINT('Ctrl Pts',(-18.623845014994,-32.7903566288258,122.496666887985)) ;
#75924=CARTESIAN_POINT('Ctrl Pts',(-18.2425317133348,-32.9804188595635,
122.457180219364)) ;
#75925=CARTESIAN_POINT('Ctrl Pts',(-18.4758763682574,-32.8004297791447,
122.648110955056)) ;
#75926=CARTESIAN_POINT('Ctrl Pts',(-18.0966577529287,-32.9902612395385,
122.670798846619)) ;
#75927=CARTESIAN_POINT('Ctrl Pts',(-18.3591783416525,-32.8102721591198,
122.819005262211)) ;
#75928=CARTESIAN_POINT('Ctrl Pts',(-17.9878239542767,-33.0002422157816,
122.909421734019)) ;
#75929=CARTESIAN_POINT('Ctrl Pts',(-18.272111762497,-32.8202531353628,123.009903514452)) ;
#75930=CARTESIAN_POINT('Ctrl Pts',(-17.9222646671379,-33.0102585441368,
123.164359426902)) ;
#75931=CARTESIAN_POINT('Ctrl Pts',(-18.2196648233517,-32.8302694637181,
123.213853781775)) ;
#75932=CARTESIAN_POINT('Ctrl Pts',(-17.9018796512239,-33.020156341128,123.423653833823)) ;
#75933=CARTESIAN_POINT('Ctrl Pts',(-18.2033572916693,-32.8401672607093,
123.421288551752)) ;
#75934=CARTESIAN_POINT('Ctrl Pts',(-17.9266701885692,-33.0301688978601,
123.685622214855)) ;
#75935=CARTESIAN_POINT('Ctrl Pts',(-18.2231900289858,-32.8501798174413,
123.630863208958)) ;
#75936=CARTESIAN_POINT('Ctrl Pts',(-17.9972994488125,-33.0402009327065,
123.939603199714)) ;
#75937=CARTESIAN_POINT('Ctrl Pts',(-18.2796939144183,-32.8602118522878,
123.834047973384)) ;
#75938=CARTESIAN_POINT('Ctrl Pts',(-18.1082062115513,-33.050040333522,124.173202825611)) ;
#75939=CARTESIAN_POINT('Ctrl Pts',(-18.3684190950603,-32.8700512531033,
124.020926481006)) ;
#75940=CARTESIAN_POINT('Ctrl Pts',(-18.2612411136302,-33.0601061191736,
124.388920029525)) ;
#75941=CARTESIAN_POINT('Ctrl Pts',(-18.4908474005065,-32.8801170387548,
124.193500344908)) ;
#75942=CARTESIAN_POINT('Ctrl Pts',(-18.4462566310749,-33.0699965742882,
124.571505176975)) ;
#75943=CARTESIAN_POINT('Ctrl Pts',(-18.6388594192354,-32.8900074938694,
124.339567673731)) ;
#75944=CARTESIAN_POINT('Ctrl Pts',(-18.6620084680825,-33.0799886929239,
124.721150558797)) ;
#75945=CARTESIAN_POINT('Ctrl Pts',(-18.8114608287963,-32.8999996125052,
124.459283763965)) ;
#75946=CARTESIAN_POINT('Ctrl Pts',(-18.8998759883015,-33.089951519687,124.830519144771)) ;
#75947=CARTESIAN_POINT('Ctrl Pts',(-19.0017545994413,-32.9099624392683,
124.546778293489)) ;
#75948=CARTESIAN_POINT('Ctrl Pts',(-19.1514920072982,-33.0998558029599,
124.897179406817)) ;
#75949=CARTESIAN_POINT('Ctrl Pts',(-19.2030466974503,-32.9198667225411,
124.600106275238)) ;
#75950=CARTESIAN_POINT('Ctrl Pts',(-19.4149143853566,-33.109916236907,124.919252762211)) ;
#75951=CARTESIAN_POINT('Ctrl Pts',(-19.4137848897019,-32.9299271564882,
124.617764888164)) ;
#75952=CARTESIAN_POINT('Ctrl Pts',(-19.6725102686818,-33.1197567895802,
124.896100987833)) ;
#75953=CARTESIAN_POINT('Ctrl Pts',(-19.6198604236689,-32.9397677091614,
124.599243563997)) ;
#75954=CARTESIAN_POINT('Ctrl Pts',(-19.9278232585539,-33.1298190095259,
124.827395120456)) ;
#75955=CARTESIAN_POINT('Ctrl Pts',(-19.824111120568,-32.9498299291071,124.544278865711)) ;
#75956=CARTESIAN_POINT('Ctrl Pts',(-20.1633223010503,-33.1397161488044,
124.716975844199)) ;
#75957=CARTESIAN_POINT('Ctrl Pts',(-20.0125096303553,-32.9597270683857,
124.455943788509)) ;
#75958=CARTESIAN_POINT('Ctrl Pts',(-20.3772875393631,-33.1496473409395,
124.567550900656)) ;
#75959=CARTESIAN_POINT('Ctrl Pts',(-20.1836814780393,-32.9696582605208,
124.336404350332)) ;
#75960=CARTESIAN_POINT('Ctrl Pts',(-20.563912219423,-33.1596894955846,124.380978396935)) ;
#75961=CARTESIAN_POINT('Ctrl Pts',(-20.3329814474512,-32.9797004151658,
124.187146334296)) ;
#75962=CARTESIAN_POINT('Ctrl Pts',(-20.7131557898249,-33.1695762566039,
124.168279265525)) ;
#75963=CARTESIAN_POINT('Ctrl Pts',(-20.4523759687857,-32.9895871761851,
124.016987866727)) ;
#75964=CARTESIAN_POINT('Ctrl Pts',(-20.8247334246548,-33.1795755583211,
123.930412036543)) ;
#75965=CARTESIAN_POINT('Ctrl Pts',(-20.5416382872207,-32.9995864779024,
123.826694322003)) ;
#75966=CARTESIAN_POINT('Ctrl Pts',(-20.8929652907576,-33.1894963564879,
123.67875334174)) ;
#75967=CARTESIAN_POINT('Ctrl Pts',(-20.5962239379931,-33.0095072760691,
123.625368054938)) ;
#75968=CARTESIAN_POINT('Ctrl Pts',(-20.9167545831049,-33.1995304100846,
123.416173818305)) ;
#75969=CARTESIAN_POINT('Ctrl Pts',(-20.6152557226043,-33.0195413296658,
123.415304354511)) ;
#75970=CARTESIAN_POINT('Ctrl Pts',(-20.8949864127053,-33.209453527651,123.156274431555)) ;
#75971=CARTESIAN_POINT('Ctrl Pts',(-20.5978416138883,-33.0294644472322,
123.207385423938)) ;
#75972=CARTESIAN_POINT('Ctrl Pts',(-20.8274911535787,-33.2195096511501,
122.900802570395)) ;
#75973=CARTESIAN_POINT('Ctrl Pts',(-20.5438456966334,-33.0395205707314,
123.003007611585)) ;
#75974=CARTESIAN_POINT('Ctrl Pts',(-20.7190711619547,-33.2293550928049,
122.66587466645)) ;
#75975=CARTESIAN_POINT('Ctrl Pts',(-20.4571105336298,-33.0493660123862,
122.815066148446)) ;
#75976=CARTESIAN_POINT('Ctrl Pts',(-20.5704789954132,-33.2393173939291,
122.450351068631)) ;
#75977=CARTESIAN_POINT('Ctrl Pts',(-20.3382375063864,-33.0593283135103,
122.64264722283)) ;
#75978=CARTESIAN_POINT('Ctrl Pts',(-20.3852299652327,-33.2493458732042,
122.262882911271)) ;
#75979=CARTESIAN_POINT('Ctrl Pts',(-20.1900385985285,-33.0693567927855,
122.492672276396)) ;
#75980=CARTESIAN_POINT('Ctrl Pts',(-20.1728523554224,-33.2592562267139,
122.112168057939)) ;
#75981=CARTESIAN_POINT('Ctrl Pts',(-20.020137396195,-33.0792671462951,122.37210035673)) ;
#75982=CARTESIAN_POINT('Ctrl Pts',(-19.9372239609751,-33.2691910988911,
121.99971673784)) ;
#75983=CARTESIAN_POINT('Ctrl Pts',(-19.8316354638329,-33.0892020184723,
122.282138886147)) ;
#75984=CARTESIAN_POINT('Ctrl Pts',(-19.6829095120149,-33.2792322364768,
121.929380340477)) ;
#75985=CARTESIAN_POINT('Ctrl Pts',(-19.6281839338197,-33.099243156058,122.225869101484)) ;
#75986=CARTESIAN_POINT('Ctrl Pts',(-19.4242673412643,-33.2891193856913,
121.90447101779)) ;
#75987=CARTESIAN_POINT('Ctrl Pts',(-19.4212710912674,-33.1091303052726,
122.205941031457)) ;
#75988=CARTESIAN_POINT('Ctrl Pts',(-19.1624743734759,-33.2991116204424,
121.924625119978)) ;
#75989=CARTESIAN_POINT('Ctrl Pts',(-19.2118368178498,-33.1191225400237,
122.222063502103)) ;
#75990=CARTESIAN_POINT('Ctrl Pts',(-18.9092537721771,-33.3090603260054,
121.989726729826)) ;
#75991=CARTESIAN_POINT('Ctrl Pts',(-19.009260561855,-33.1290712455866,122.274143925144)) ;
#75992=CARTESIAN_POINT('Ctrl Pts',(-18.6713579683,-33.3189963944291,122.097309682387)) ;
#75993=CARTESIAN_POINT('Ctrl Pts',(-18.8189440248541,-33.1390073140103,
122.360209282463)) ;
#75994=CARTESIAN_POINT('Ctrl Pts',(-18.4544730862857,-33.3289820786449,
122.245077547406)) ;
#75995=CARTESIAN_POINT('Ctrl Pts',(-18.6454357542757,-33.1489929982261,
122.478422680742)) ;
#75996=CARTESIAN_POINT('Ctrl Pts',(-18.2658309061673,-33.3390225052135,
122.429534786663)) ;
#75997=CARTESIAN_POINT('Ctrl Pts',(-18.494521322166,-33.1590334247948,122.625987962609)) ;
#75998=CARTESIAN_POINT('Ctrl Pts',(-18.1148023370234,-33.3488616186773,
122.639409270559)) ;
#75999=CARTESIAN_POINT('Ctrl Pts',(-18.3736983361703,-33.1688725382585,
122.793886113984)) ;
#76000=CARTESIAN_POINT('Ctrl Pts',(-17.9997997484808,-33.3588913528531,
122.876570796165)) ;
#76001=CARTESIAN_POINT('Ctrl Pts',(-18.2816952521632,-33.1789022724343,
122.983614938204)) ;
#76002=CARTESIAN_POINT('Ctrl Pts',(-17.9284390776432,-33.368913452359,123.130086625295)) ;
#76003=CARTESIAN_POINT('Ctrl Pts',(-18.2246058215283,-33.1889243719402,
123.186427373328)) ;
#76004=CARTESIAN_POINT('Ctrl Pts',(-17.9019339657946,-33.3787818922524,
123.388080969437)) ;
#76005=CARTESIAN_POINT('Ctrl Pts',(-18.2034007565293,-33.1987928118337,
123.3928218386)) ;
#76006=CARTESIAN_POINT('Ctrl Pts',(-17.9210110194768,-33.388850756938,123.651967424928)) ;
#76007=CARTESIAN_POINT('Ctrl Pts',(-18.2186613497739,-33.2088616765193,
123.603931380545)) ;
#76008=CARTESIAN_POINT('Ctrl Pts',(-17.9841657909926,-33.3986934300366,
123.902803793682)) ;
#76009=CARTESIAN_POINT('Ctrl Pts',(-18.2691838719648,-33.2187043496179,
123.804599731666)) ;
#76010=CARTESIAN_POINT('Ctrl Pts',(-18.0903011026987,-33.4086540641991,
124.142069897839)) ;
#76011=CARTESIAN_POINT('Ctrl Pts',(-18.3540908116242,-33.2286649837803,
123.996012840234)) ;
#76012=CARTESIAN_POINT('Ctrl Pts',(-18.2379303217283,-33.4186919798772,
124.360664605531)) ;
#76013=CARTESIAN_POINT('Ctrl Pts',(-18.4721932743968,-33.2387028994585,
124.170889351092)) ;
#76014=CARTESIAN_POINT('Ctrl Pts',(-18.4179673638291,-33.4285662547366,
124.547577121992)) ;
#76015=CARTESIAN_POINT('Ctrl Pts',(-18.6162214263879,-33.2485771743179,
124.320419667571)) ;
#76016=CARTESIAN_POINT('Ctrl Pts',(-18.631829456025,-33.4386360051118,124.703362669237)) ;
#76017=CARTESIAN_POINT('Ctrl Pts',(-18.7873105748439,-33.258646924693,124.445049300282)) ;
#76018=CARTESIAN_POINT('Ctrl Pts',(-18.8639015606076,-33.4484693004863,
124.8170675459)) ;
#76019=CARTESIAN_POINT('Ctrl Pts',(-18.9729667662246,-33.2684802200675,
124.536013921811)) ;
#76020=CARTESIAN_POINT('Ctrl Pts',(-19.1169286180859,-33.4584995979659,
124.890896842936)) ;
#76021=CARTESIAN_POINT('Ctrl Pts',(-19.1753880699453,-33.2785105175472,
124.595078779856)) ;
#76022=CARTESIAN_POINT('Ctrl Pts',(-19.3790808832742,-33.4685316844073,
124.918905806872)) ;
#76023=CARTESIAN_POINT('Ctrl Pts',(-19.3851098109455,-33.2885426039886,
124.617487248845)) ;
#76024=CARTESIAN_POINT('Ctrl Pts',(-19.63677762178,-33.4783596128963,124.901904690661)) ;
#76025=CARTESIAN_POINT('Ctrl Pts',(-19.5912662774906,-33.2983705324775,
124.603887836004)) ;
#76026=CARTESIAN_POINT('Ctrl Pts',(-19.8920737335498,-33.4883556540071,
124.840047977174)) ;
#76027=CARTESIAN_POINT('Ctrl Pts',(-19.7955034173776,-33.3083665735883,
124.554404008552)) ;
#76028=CARTESIAN_POINT('Ctrl Pts',(-20.133272867341,-33.4983814661083,124.734019156256)) ;
#76029=CARTESIAN_POINT('Ctrl Pts',(-19.9884633393389,-33.3183923856895,
124.469582272309)) ;
#76030=CARTESIAN_POINT('Ctrl Pts',(-20.3495536622169,-33.5082687010031,
124.590024685986)) ;
#76031=CARTESIAN_POINT('Ctrl Pts',(-20.1614882643308,-33.3282796205843,
124.35438833044)) ;
#76032=CARTESIAN_POINT('Ctrl Pts',(-20.5395336849035,-33.5182455672141,
124.409369154999)) ;
#76033=CARTESIAN_POINT('Ctrl Pts',(-20.3134732405899,-33.3382564867954,
124.209865210489)) ;
#76034=CARTESIAN_POINT('Ctrl Pts',(-20.6955808167285,-33.5282385110859,
124.198113299895)) ;
#76035=CARTESIAN_POINT('Ctrl Pts',(-20.4383121677193,-33.3482494306672,
124.040861581618)) ;
#76036=CARTESIAN_POINT('Ctrl Pts',(-20.812778041228,-33.5382764337573,123.961814580472)) ;
#76037=CARTESIAN_POINT('Ctrl Pts',(-20.5320713666861,-33.3582873533385,
123.851823229752)) ;
#76038=CARTESIAN_POINT('Ctrl Pts',(-20.8861474399922,-33.548124898019,123.713603887061)) ;
#76039=CARTESIAN_POINT('Ctrl Pts',(-20.5907682089124,-33.3681358176002,
123.653255920477)) ;
#76040=CARTESIAN_POINT('Ctrl Pts',(-20.9161879632352,-33.558116764763,123.45279073019)) ;
#76041=CARTESIAN_POINT('Ctrl Pts',(-20.6148023084948,-33.3781276843442,
123.444605723383)) ;
#76042=CARTESIAN_POINT('Ctrl Pts',(-20.9007460376538,-33.5680344968042,
123.192586764774)) ;
#76043=CARTESIAN_POINT('Ctrl Pts',(-20.6024505212769,-33.3880454163854,
123.236442905293)) ;
#76044=CARTESIAN_POINT('Ctrl Pts',(-20.839767398119,-33.5780626816995,122.936230922759)) ;
#76045=CARTESIAN_POINT('Ctrl Pts',(-20.5536692986984,-33.3980736012807,
123.031357801439)) ;
#76046=CARTESIAN_POINT('Ctrl Pts',(-20.7367825953331,-33.5879478397483,
122.697737712754)) ;
#76047=CARTESIAN_POINT('Ctrl Pts',(-20.4712833051947,-33.4079587593295,
122.840563075759)) ;
#76048=CARTESIAN_POINT('Ctrl Pts',(-20.5929810835081,-33.59793720029,122.478112272393)) ;
#76049=CARTESIAN_POINT('Ctrl Pts',(-20.3562437228865,-33.4179481198712,
122.664861808084)) ;
#76050=CARTESIAN_POINT('Ctrl Pts',(-20.4118953447664,-33.6079783572243,
122.28618599591)) ;
#76051=CARTESIAN_POINT('Ctrl Pts',(-20.211376372118,-33.4279892768056,122.511319516605)) ;
#76052=CARTESIAN_POINT('Ctrl Pts',(-20.2048905332115,-33.6178109406795,
122.131549195087)) ;
#76053=CARTESIAN_POINT('Ctrl Pts',(-20.0457742371618,-33.4378218602607,
122.387609057188)) ;
#76054=CARTESIAN_POINT('Ctrl Pts',(-19.9707238078084,-33.6278051606415,
122.012626278737)) ;
#76055=CARTESIAN_POINT('Ctrl Pts',(-19.8584418276612,-33.4478160802227,
122.292469026325)) ;
#76056=CARTESIAN_POINT('Ctrl Pts',(-19.7184472437262,-33.6378332624288,
121.936421881555)) ;
#76057=CARTESIAN_POINT('Ctrl Pts',(-19.6566211029712,-33.45784418201,122.231503711827)) ;
#76058=CARTESIAN_POINT('Ctrl Pts',(-19.4606834132715,-33.6477132070518,
121.905273090472)) ;
#76059=CARTESIAN_POINT('Ctrl Pts',(-19.450410798269,-33.4677241266331,122.206582828695)) ;
#76060=CARTESIAN_POINT('Ctrl Pts',(-19.1985284829014,-33.6577035336089,
121.919105510817)) ;
#76061=CARTESIAN_POINT('Ctrl Pts',(-19.2406868632452,-33.4777144531901,
122.217646778312)) ;
#76062=CARTESIAN_POINT('Ctrl Pts',(-18.9440006247373,-33.6676444652632,
121.977957452848)) ;
#76063=CARTESIAN_POINT('Ctrl Pts',(-19.037064402286,-33.4876553848444,122.264726340451)) ;
#76064=CARTESIAN_POINT('Ctrl Pts',(-18.7022824096252,-33.6776315837661,
122.080244334411)) ;
#76065=CARTESIAN_POINT('Ctrl Pts',(-18.8436891442797,-33.4976425033473,
122.346553933699)) ;
#76066=CARTESIAN_POINT('Ctrl Pts',(-18.4812344248133,-33.6876649166633,
122.223936502214)) ;
#76067=CARTESIAN_POINT('Ctrl Pts',(-18.6668496639801,-33.5076758362445,
122.461506021483)) ;
#76068=CARTESIAN_POINT('Ctrl Pts',(-18.2913247034352,-33.697531021108,122.40049026279)) ;
#76069=CARTESIAN_POINT('Ctrl Pts',(-18.514920867317,-33.5175419406893,122.602747196414)) ;
#76070=CARTESIAN_POINT('Ctrl Pts',(-18.1317726323922,-33.7075971349883,
122.611443968971)) ;
#76071=CARTESIAN_POINT('Ctrl Pts',(-18.3872775066212,-33.5276080545696,
122.771509020567)) ;
#76072=CARTESIAN_POINT('Ctrl Pts',(-18.0137527034609,-33.7174531467568,
122.842018843075)) ;
#76073=CARTESIAN_POINT('Ctrl Pts',(-18.2928599689319,-33.537464066338,122.955967544122)) ;
#76074=CARTESIAN_POINT('Ctrl Pts',(-17.9357556599611,-33.7274478503881,
123.09281337308)) ;
#76075=CARTESIAN_POINT('Ctrl Pts',(-18.2304603236921,-33.5474587699693,
123.156602459403)) ;
#76076=CARTESIAN_POINT('Ctrl Pts',(-17.902925994022,-33.7374791861129,123.354378720206)) ;
#76077=CARTESIAN_POINT('Ctrl Pts',(-18.2041945366287,-33.5574901056942,
123.365854477829)) ;
#76078=CARTESIAN_POINT('Ctrl Pts',(-17.9153845548777,-33.7473457113166,
123.613370405314)) ;
#76079=CARTESIAN_POINT('Ctrl Pts',(-18.2141592554439,-33.5673566308979,
123.573047516046)) ;
#76080=CARTESIAN_POINT('Ctrl Pts',(-17.9729030335176,-33.7573331393624,
123.869417371831)) ;
#76081=CARTESIAN_POINT('Ctrl Pts',(-18.2601719160976,-33.5773440589437,
123.777885465428)) ;
#76082=CARTESIAN_POINT('Ctrl Pts',(-18.0734724275079,-33.7672780690488,
124.110676065915)) ;
#76083=CARTESIAN_POINT('Ctrl Pts',(-18.3406253653803,-33.5872889886301,
123.970893079309)) ;
#76084=CARTESIAN_POINT('Ctrl Pts',(-18.2159131529167,-33.7773229871573,
124.332886434343)) ;
#76085=CARTESIAN_POINT('Ctrl Pts',(-18.4545761429792,-33.5973339067386,
124.14866254757)) ;
#76086=CARTESIAN_POINT('Ctrl Pts',(-18.391376037984,-33.7871849567712,124.523645046394)) ;
#76087=CARTESIAN_POINT('Ctrl Pts',(-18.5949446249841,-33.6071958763525,
124.301270653746)) ;
#76088=CARTESIAN_POINT('Ctrl Pts',(-18.5996633148783,-33.7971770247925,
124.683493416161)) ;
#76089=CARTESIAN_POINT('Ctrl Pts',(-18.7615730437336,-33.6171879443737,
124.429151053145)) ;
#76090=CARTESIAN_POINT('Ctrl Pts',(-18.8311757134358,-33.807107950167,124.803984732188)) ;
#76091=CARTESIAN_POINT('Ctrl Pts',(-18.9467817879391,-33.6271188697483,
124.525545974419)) ;
#76092=CARTESIAN_POINT('Ctrl Pts',(-19.0804210324895,-33.8170585783905,
124.883010582598)) ;
#76093=CARTESIAN_POINT('Ctrl Pts',(-19.1461772488705,-33.6370694979717,
124.588768739218)) ;
#76094=CARTESIAN_POINT('Ctrl Pts',(-19.3409209971881,-33.8270588174496,
124.917887618055)) ;
#76095=CARTESIAN_POINT('Ctrl Pts',(-19.3545768691479,-33.6470697370308,
124.616672564472)) ;
#76096=CARTESIAN_POINT('Ctrl Pts',(-19.6042058083213,-33.8370872728188,
124.906594290963)) ;
#76097=CARTESIAN_POINT('Ctrl Pts',(-19.5652047628629,-33.6570981924,124.607640132786)) ;
#76098=CARTESIAN_POINT('Ctrl Pts',(-19.8574687091676,-33.8469533074021,
124.851055548334)) ;
#76099=CARTESIAN_POINT('Ctrl Pts',(-19.767815408138,-33.6669642269833,124.563211299104)) ;
#76100=CARTESIAN_POINT('Ctrl Pts',(-20.1004399415892,-33.8569456291495,
124.751536397017)) ;
#76101=CARTESIAN_POINT('Ctrl Pts',(-19.9621930061691,-33.6769565487307,
124.483598313414)) ;
#76102=CARTESIAN_POINT('Ctrl Pts',(-20.3211678424229,-33.8668779188265,
124.612195664148)) ;
#76103=CARTESIAN_POINT('Ctrl Pts',(-20.1387771157398,-33.6868888384077,
124.372126818241)) ;
#76104=CARTESIAN_POINT('Ctrl Pts',(-20.5158504185052,-33.8768795637972,
124.435627299948)) ;
#76105=CARTESIAN_POINT('Ctrl Pts',(-20.2945221175348,-33.6968904833785,
124.230877050889)) ;
#76106=CARTESIAN_POINT('Ctrl Pts',(-20.730134344233,-33.8901921972132,124.159073181057)) ;
#76107=CARTESIAN_POINT('Ctrl Pts',(-20.4659641625927,-33.7102031167945,
124.009619650892)) ;
#76108=CARTESIAN_POINT('Ctrl Pts',(-20.8667466131401,-33.9034239465948,
123.835025634175)) ;
#76109=CARTESIAN_POINT('Ctrl Pts',(-20.5752544036822,-33.7234348661761,
123.750361646045)) ;
#76110=CARTESIAN_POINT('Ctrl Pts',(-20.9147529609459,-33.9167472114119,
123.488209575829)) ;
#76111=CARTESIAN_POINT('Ctrl Pts',(-20.613652637114,-33.7367581309931,123.47295053957)) ;
#76112=CARTESIAN_POINT('Ctrl Pts',(-20.9055507234748,-33.9266229176296,
123.228839180921)) ;
#76113=CARTESIAN_POINT('Ctrl Pts',(-20.6062950688991,-33.7466338372108,
123.265445862905)) ;
#76114=CARTESIAN_POINT('Ctrl Pts',(-20.8511725358369,-33.9366125087296,
122.972045792738)) ;
#76115=CARTESIAN_POINT('Ctrl Pts',(-20.5627941970681,-33.7566234283109,
123.060012946144)) ;
#76116=CARTESIAN_POINT('Ctrl Pts',(-20.7537843024059,-33.946539605185,122.729998734827)) ;
#76117=CARTESIAN_POINT('Ctrl Pts',(-20.4848858225803,-33.7665505247663,
122.866373858558)) ;
#76118=CARTESIAN_POINT('Ctrl Pts',(-20.6145413557594,-33.9565647536896,
122.506380398541)) ;
#76119=CARTESIAN_POINT('Ctrl Pts',(-20.3734933698443,-33.7765756732709,
122.687478231554)) ;
#76120=CARTESIAN_POINT('Ctrl Pts',(-20.4409482370031,-33.9664604078363,
122.312726536697)) ;
#76121=CARTESIAN_POINT('Ctrl Pts',(-20.2346204969347,-33.7864713274175,
122.532553555553)) ;
#76122=CARTESIAN_POINT('Ctrl Pts',(-20.2344050443402,-33.9764639422145,
122.15014179103)) ;
#76123=CARTESIAN_POINT('Ctrl Pts',(-20.0693873459231,-33.7964748617957,
122.402484058768)) ;
#76124=CARTESIAN_POINT('Ctrl Pts',(-20.0031251937128,-33.9864490806545,
122.026110363631)) ;
#76125=CARTESIAN_POINT('Ctrl Pts',(-19.8843645383385,-33.8064600002358,
122.303256977614)) ;
#76126=CARTESIAN_POINT('Ctrl Pts',(-19.7525232072427,-33.9964850052499,
121.943972168171)) ;
#76127=CARTESIAN_POINT('Ctrl Pts',(-19.6838837485256,-33.8164959248312,
122.237544337022)) ;
#76128=CARTESIAN_POINT('Ctrl Pts',(-19.4963012262172,-34.0063362806776,
121.906976170248)) ;
#76129=CARTESIAN_POINT('Ctrl Pts',(-19.4789062849549,-33.8263472002588,
122.207945321101)) ;
#76130=CARTESIAN_POINT('Ctrl Pts',(-19.2338112579633,-34.0163285418389,
121.914396519878)) ;
#76131=CARTESIAN_POINT('Ctrl Pts',(-19.2689142641197,-33.8363394614202,
122.213879435451)) ;
#76132=CARTESIAN_POINT('Ctrl Pts',(-18.9755284714403,-34.0263684258565,
121.968182550253)) ;
#76133=CARTESIAN_POINT('Ctrl Pts',(-19.0622876995497,-33.8463793454378,
122.256906084154)) ;
#76134=CARTESIAN_POINT('Ctrl Pts',(-18.7352293588576,-34.036203200359,122.063406918067)) ;
#76135=CARTESIAN_POINT('Ctrl Pts',(-18.8700473962123,-33.8562141199402,
122.333083630202)) ;
#76136=CARTESIAN_POINT('Ctrl Pts',(-18.5097194263929,-34.0462795813793,
122.202115742351)) ;
#76137=CARTESIAN_POINT('Ctrl Pts',(-18.6896381792612,-33.8662905009605,
122.444048990142)) ;
#76138=CARTESIAN_POINT('Ctrl Pts',(-18.3161370097304,-34.0561258545299,
122.373856170595)) ;
#76139=CARTESIAN_POINT('Ctrl Pts',(-18.534771813737,-33.8761367741112,122.581439034222)) ;
#76140=CARTESIAN_POINT('Ctrl Pts',(-18.0973641720039,-34.0694903758151,
122.648596301524)) ;
#76141=CARTESIAN_POINT('Ctrl Pts',(-18.3597451619224,-33.8895012953964,
122.801233992996)) ;
#76142=CARTESIAN_POINT('Ctrl Pts',(-17.9574233666502,-34.0826966202496,
122.970485787033)) ;
#76143=CARTESIAN_POINT('Ctrl Pts',(-18.2477846414627,-33.9027075398308,
123.058779978968)) ;
#76144=CARTESIAN_POINT('Ctrl Pts',(-17.9048166903055,-34.0959615749268,
123.315069758418)) ;
#76145=CARTESIAN_POINT('Ctrl Pts',(-18.2057090036201,-33.9159724945081,
123.334400438449)) ;
#76146=CARTESIAN_POINT('Ctrl Pts',(-17.9110068531444,-34.1059938554785,
123.57864144409)) ;
#76147=CARTESIAN_POINT('Ctrl Pts',(-18.2106566732483,-33.9260047750597,
123.545267055076)) ;
#76148=CARTESIAN_POINT('Ctrl Pts',(-17.9622064694979,-34.1159025889964,
123.83394390301)) ;
#76149=CARTESIAN_POINT('Ctrl Pts',(-18.2516149524503,-33.9359135085776,
123.749507096678)) ;
#76150=CARTESIAN_POINT('Ctrl Pts',(-18.0566040744256,-34.1258401398639,
124.077443630535)) ;
#76151=CARTESIAN_POINT('Ctrl Pts',(-18.3271318142154,-33.9458510594451,
123.944309004323)) ;
#76152=CARTESIAN_POINT('Ctrl Pts',(-18.1932746080378,-34.1358699874578,
124.302786499477)) ;
#76153=CARTESIAN_POINT('Ctrl Pts',(-18.4364641738599,-33.9558809070391,
124.124582034141)) ;
#76154=CARTESIAN_POINT('Ctrl Pts',(-18.4222258928421,-34.1491051273782,
124.564718290343)) ;
#76155=CARTESIAN_POINT('Ctrl Pts',(-18.6196353445962,-33.9691160469595,
124.334139139703)) ;
#76156=CARTESIAN_POINT('Ctrl Pts',(-18.79005327306,-34.1657735917494,124.811391878925)) ;
#76157=CARTESIAN_POINT('Ctrl Pts',(-18.9138856664441,-33.9857845113307,
124.531468849858)) ;
#76158=CARTESIAN_POINT('Ctrl Pts',(-19.302810003159,-34.1856446036233,124.93867473504)) ;
#76159=CARTESIAN_POINT('Ctrl Pts',(-19.3240782602018,-34.0056555232046,
124.633306456755)) ;
#76160=CARTESIAN_POINT('Ctrl Pts',(-19.7442781237736,-34.2023516880063,
124.892055705492)) ;
#76161=CARTESIAN_POINT('Ctrl Pts',(-19.6773043553831,-34.0223626075875,
124.596000463399)) ;
#76162=CARTESIAN_POINT('Ctrl Pts',(-20.0675644893063,-34.2155289693169,
124.767792583649)) ;
#76163=CARTESIAN_POINT('Ctrl Pts',(-19.935888328374,-34.0355398888981,124.496604100906)) ;
#76164=CARTESIAN_POINT('Ctrl Pts',(-20.3669683528388,-34.228796429831,124.589169379332)) ;
#76165=CARTESIAN_POINT('Ctrl Pts',(-20.1754272032707,-34.0488073494122,
124.353698951168)) ;
#76166=CARTESIAN_POINT('Ctrl Pts',(-20.6747925424677,-34.2454103205182,
124.272577564585)) ;
#76167=CARTESIAN_POINT('Ctrl Pts',(-20.4216796479605,-34.0654212400994,
124.100434565729)) ;
#76168=CARTESIAN_POINT('Ctrl Pts',(-20.8925501700645,-34.2653591199456,
123.789095141631)) ;
#76169=CARTESIAN_POINT('Ctrl Pts',(-20.5958914715679,-34.0853700395268,
123.713647108598)) ;
#76170=CARTESIAN_POINT('Ctrl Pts',(-20.9320934628984,-34.2852802314764,
123.261176948921)) ;
#76171=CARTESIAN_POINT('Ctrl Pts',(-20.627528243359,-34.1052911510577,123.29131282389)) ;
#76172=CARTESIAN_POINT('Ctrl Pts',(-20.7905220574422,-34.3051466796493,
122.752407298915)) ;
#76173=CARTESIAN_POINT('Ctrl Pts',(-20.5142733449368,-34.1251575992306,
122.884295234101)) ;
#76174=CARTESIAN_POINT('Ctrl Pts',(-20.4811847889184,-34.3251730262664,
122.319328242718)) ;
#76175=CARTESIAN_POINT('Ctrl Pts',(-20.2668055516656,-34.1451839458477,
122.537830873447)) ;
#76176=CARTESIAN_POINT('Ctrl Pts',(-20.046046929039,-34.345035070656,122.02027991162)) ;
#76177=CARTESIAN_POINT('Ctrl Pts',(-19.9186955596424,-34.1650459902372,
122.298589641338)) ;
#76178=CARTESIAN_POINT('Ctrl Pts',(-19.5332082975731,-34.3649803733371,
121.886348768539)) ;
#76179=CARTESIAN_POINT('Ctrl Pts',(-19.5084245595147,-34.1849912929184,
122.191442818576)) ;
#76180=CARTESIAN_POINT('Ctrl Pts',(-19.0066946738913,-34.384875680396,121.935430157998)) ;
#76181=CARTESIAN_POINT('Ctrl Pts',(-19.0872124491375,-34.2048865999772,
122.230706348824)) ;
#76182=CARTESIAN_POINT('Ctrl Pts',(-18.5281796662803,-34.4047689505636,
122.160351280657)) ;
#76183=CARTESIAN_POINT('Ctrl Pts',(-18.7043988887934,-34.2247798701449,
122.410642726589)) ;
#76184=CARTESIAN_POINT('Ctrl Pts',(-18.1538942484392,-34.424734543244,122.536474463876)) ;
#76185=CARTESIAN_POINT('Ctrl Pts',(-18.404969560696,-34.2447454628253,122.711540862601)) ;
#76186=CARTESIAN_POINT('Ctrl Pts',(-17.9310744456909,-34.4446098669289,
123.015467619832)) ;
#76187=CARTESIAN_POINT('Ctrl Pts',(-18.2267125107953,-34.2646207865101,
123.094736487549)) ;
#76188=CARTESIAN_POINT('Ctrl Pts',(-17.8843177629388,-34.4645849295038,
123.544333074605)) ;
#76189=CARTESIAN_POINT('Ctrl Pts',(-18.1893069457108,-34.2845958490851,
123.517829108664)) ;
#76190=CARTESIAN_POINT('Ctrl Pts',(-18.0214586110125,-34.484537339135,124.056594429995)) ;
#76191=CARTESIAN_POINT('Ctrl Pts',(-18.2990194229785,-34.3045482587162,
123.927638867659)) ;
#76192=CARTESIAN_POINT('Ctrl Pts',(-18.3225640751272,-34.504373393371,124.489356119878)) ;
#76193=CARTESIAN_POINT('Ctrl Pts',(-18.5399052793811,-34.3243843129523,
124.27384976748)) ;
#76194=CARTESIAN_POINT('Ctrl Pts',(-18.7560161142361,-34.5243513047886,
124.796045846315)) ;
#76195=CARTESIAN_POINT('Ctrl Pts',(-18.8866675828867,-34.3443622243698,
124.519201026929)) ;
#76196=CARTESIAN_POINT('Ctrl Pts',(-19.266703075915,-34.5442693542921,124.935377333692)) ;
#76197=CARTESIAN_POINT('Ctrl Pts',(-19.2952182947917,-34.3642802738733,
124.630665776378)) ;
#76198=CARTESIAN_POINT('Ctrl Pts',(-19.7932159078687,-34.5641374980602,
124.893556756137)) ;
#76199=CARTESIAN_POINT('Ctrl Pts',(-19.7164298223103,-34.3841484176414,
124.597207716313)) ;
#76200=CARTESIAN_POINT('Ctrl Pts',(-20.2777146691111,-34.5841883546475,
124.671918199615)) ;
#76201=CARTESIAN_POINT('Ctrl Pts',(-20.1040278270987,-34.4041992742287,
124.419895848041)) ;
#76202=CARTESIAN_POINT('Ctrl Pts',(-20.6529658815837,-34.6039687911034,
124.3034966869)) ;
#76203=CARTESIAN_POINT('Ctrl Pts',(-20.4042291464414,-34.4239797106846,
124.125155886527)) ;
#76204=CARTESIAN_POINT('Ctrl Pts',(-20.8834863291553,-34.6239988467812,
123.823760909357)) ;
#76205=CARTESIAN_POINT('Ctrl Pts',(-20.5886433844177,-34.4440097663624,
123.74136659525)) ;
#76206=CARTESIAN_POINT('Ctrl Pts',(-20.9351889706726,-34.643879951956,123.297798988624)) ;
#76207=CARTESIAN_POINT('Ctrl Pts',(-20.6300035954088,-34.4638908715372,
123.32059580445)) ;
#76208=CARTESIAN_POINT('Ctrl Pts',(-20.8057903344438,-34.6637604143238,
122.785553366856)) ;
#76209=CARTESIAN_POINT('Ctrl Pts',(-20.5264818601808,-34.483771333905,122.910799001557)) ;
#76210=CARTESIAN_POINT('Ctrl Pts',(-20.5076352220896,-34.6837455614681,
122.345932909979)) ;
#76211=CARTESIAN_POINT('Ctrl Pts',(-20.2879554585398,-34.5037564810494,
122.559104093687)) ;
#76212=CARTESIAN_POINT('Ctrl Pts',(-20.0793236955873,-34.7036361400045,
122.036027427031)) ;
#76213=CARTESIAN_POINT('Ctrl Pts',(-19.9453039222835,-34.5236470595857,
122.311181522728)) ;
#76214=CARTESIAN_POINT('Ctrl Pts',(-19.5711560383536,-34.7235301598789,
121.889965636208)) ;
#76215=CARTESIAN_POINT('Ctrl Pts',(-19.5387682446119,-34.5435410794601,
122.1943349732)) ;
#76216=CARTESIAN_POINT('Ctrl Pts',(-19.0429893283556,-34.7434516046053,
121.925987779799)) ;
#76217=CARTESIAN_POINT('Ctrl Pts',(-19.1162346135711,-34.5634625241865,
122.223156059284)) ;
#76218=CARTESIAN_POINT('Ctrl Pts',(-18.5587933442751,-34.7633497426607,
122.139065599322)) ;
#76219=CARTESIAN_POINT('Ctrl Pts',(-18.7288788359676,-34.583360662242,122.393621850554)) ;
#76220=CARTESIAN_POINT('Ctrl Pts',(-18.1739396123522,-34.7834204978768,
122.508326536846)) ;
#76221=CARTESIAN_POINT('Ctrl Pts',(-18.4209985757421,-34.603431417458,122.689032837873)) ;
#76222=CARTESIAN_POINT('Ctrl Pts',(-17.9412291316827,-34.803206047928,122.980030562357)) ;
#76223=CARTESIAN_POINT('Ctrl Pts',(-18.234833032526,-34.6232169675093,123.066398644646)) ;
#76224=CARTESIAN_POINT('Ctrl Pts',(-17.8816194221956,-34.8231891228054,
123.507694573196)) ;
#76225=CARTESIAN_POINT('Ctrl Pts',(-18.1871490553495,-34.6432000423866,
123.488530272471)) ;
#76226=CARTESIAN_POINT('Ctrl Pts',(-18.0060182322605,-34.8430982054513,
124.022021160896)) ;
#76227=CARTESIAN_POINT('Ctrl Pts',(-18.2866725880628,-34.6631091250326,
123.899991117196)) ;
#76228=CARTESIAN_POINT('Ctrl Pts',(-18.296486524571,-34.8629567645741,124.462795927033)) ;
#76229=CARTESIAN_POINT('Ctrl Pts',(-18.5190486895846,-34.6829676841553,
124.252608470384)) ;
#76230=CARTESIAN_POINT('Ctrl Pts',(-18.7241036773719,-34.8830002084128,
124.780319588306)) ;
#76231=CARTESIAN_POINT('Ctrl Pts',(-18.8611532239642,-34.703011127994,124.506625843281)) ;
#76232=CARTESIAN_POINT('Ctrl Pts',(-19.1443314362072,-34.899500273142,124.906184977556)) ;
#76233=CARTESIAN_POINT('Ctrl Pts',(-19.1973104768277,-34.7195111927232,
124.607308957452)) ;
#76234=CARTESIAN_POINT('Ctrl Pts',(-19.4959856145743,-34.9128900129909,
124.916808895256)) ;
#76235=CARTESIAN_POINT('Ctrl Pts',(-19.4786571226114,-34.7329009325721,
124.615810467763)) ;
#76236=CARTESIAN_POINT('Ctrl Pts',(-19.7523697501697,-34.9227469141993,
124.879642738645)) ;
#76237=CARTESIAN_POINT('Ctrl Pts',(-19.6837596469558,-34.7427578337805,
124.586074466439)) ;
#76238=CARTESIAN_POINT('Ctrl Pts',(-20.0018598352165,-34.9327384400458,
124.797951435876)) ;
#76239=CARTESIAN_POINT('Ctrl Pts',(-19.8833526563097,-34.752749359627,124.520719090591)) ;
#76240=CARTESIAN_POINT('Ctrl Pts',(-20.2319445661498,-34.9426631204967,
124.675054574877)) ;
#76241=CARTESIAN_POINT('Ctrl Pts',(-20.0674176841992,-34.762674040078,124.4224015819)) ;
#76242=CARTESIAN_POINT('Ctrl Pts',(-20.4389718038519,-34.9526737105411,
124.512809926681)) ;
#76243=CARTESIAN_POINT('Ctrl Pts',(-20.2330436587693,-34.7726846301224,
124.292596602303)) ;
#76244=CARTESIAN_POINT('Ctrl Pts',(-20.6720998991918,-34.9659329712448,
124.253723717927)) ;
#76245=CARTESIAN_POINT('Ctrl Pts',(-20.4195165683706,-34.7859438908261,
124.085363349355)) ;
#76246=CARTESIAN_POINT('Ctrl Pts',(-20.8329350806872,-34.9792840463951,
123.937545082289)) ;
#76247=CARTESIAN_POINT('Ctrl Pts',(-20.5482036204118,-34.7992949659763,
123.832398938157)) ;
#76248=CARTESIAN_POINT('Ctrl Pts',(-20.9051329386564,-34.9924903556299,
123.598017654261)) ;
#76249=CARTESIAN_POINT('Ctrl Pts',(-20.605960739995,-34.8125012752111,123.56076258238)) ;
#76250=CARTESIAN_POINT('Ctrl Pts',(-20.9148428908615,-35.0024771892202,
123.335798885089)) ;
#76251=CARTESIAN_POINT('Ctrl Pts',(-20.6137261079857,-34.8224881088014,
123.350990280824)) ;
#76252=CARTESIAN_POINT('Ctrl Pts',(-20.8791149641005,-35.0124299167163,
123.076657694383)) ;
#76253=CARTESIAN_POINT('Ctrl Pts',(-20.5851416344258,-34.8324408362975,
123.143676914264)) ;
#76254=CARTESIAN_POINT('Ctrl Pts',(-20.7979778137027,-35.0224780135579,
122.825409407671)) ;
#76255=CARTESIAN_POINT('Ctrl Pts',(-20.5202297765397,-34.8424889331391,
122.942679247368)) ;
#76256=CARTESIAN_POINT('Ctrl Pts',(-20.6772333062883,-35.0323194704297,
122.596674503365)) ;
#76257=CARTESIAN_POINT('Ctrl Pts',(-20.4236321706692,-34.8523303900109,
122.759692291335)) ;
#76258=CARTESIAN_POINT('Ctrl Pts',(-20.5167579761927,-35.0423057373431,
122.389083764438)) ;
#76259=CARTESIAN_POINT('Ctrl Pts',(-20.2952501539374,-34.8623166569244,
122.593621150654)) ;
#76260=CARTESIAN_POINT('Ctrl Pts',(-20.3236651758144,-35.0522423382436,
122.213233449204)) ;
#76261=CARTESIAN_POINT('Ctrl Pts',(-20.1407744379203,-34.8722532578248,
122.452942601343)) ;
#76262=CARTESIAN_POINT('Ctrl Pts',(-20.1004431976112,-35.0622922810306,
122.072138574623)) ;
#76263=CARTESIAN_POINT('Ctrl Pts',(-19.9621956872849,-34.8823032006119,
122.340068638975)) ;
#76264=CARTESIAN_POINT('Ctrl Pts',(-19.8610023890791,-35.0721424807164,
121.973740369794)) ;
#76265=CARTESIAN_POINT('Ctrl Pts',(-19.7706422695711,-34.8921534002976,
122.261352199334)) ;
#76266=CARTESIAN_POINT('Ctrl Pts',(-19.6051578614326,-35.0821153856485,
121.917057183001)) ;
#76267=CARTESIAN_POINT('Ctrl Pts',(-19.5659662526582,-34.9021263052297,
122.216007866642)) ;
#76268=CARTESIAN_POINT('Ctrl Pts',(-19.3426236375275,-35.0921137601281,
121.905710783853)) ;
#76269=CARTESIAN_POINT('Ctrl Pts',(-19.3559388367088,-34.9121246797094,
122.206932993469)) ;
#76270=CARTESIAN_POINT('Ctrl Pts',(-19.0816040718375,-35.1021339339981,
121.940379135777)) ;
#76271=CARTESIAN_POINT('Ctrl Pts',(-19.1471235237251,-34.9221448535794,
122.234669903381)) ;
#76272=CARTESIAN_POINT('Ctrl Pts',(-18.8334713867964,-35.1120349779401,
122.018687487748)) ;
#76273=CARTESIAN_POINT('Ctrl Pts',(-18.9486181859309,-34.9320458975213,
122.297318684873)) ;
#76274=CARTESIAN_POINT('Ctrl Pts',(-18.6004760333388,-35.1220237816644,
122.139585076193)) ;
#76275=CARTESIAN_POINT('Ctrl Pts',(-18.7622230038763,-34.9420347012456,
122.394038699726)) ;
#76276=CARTESIAN_POINT('Ctrl Pts',(-18.3926205882541,-35.1319892484962,
122.298870810945)) ;
#76277=CARTESIAN_POINT('Ctrl Pts',(-18.5959400898762,-34.9520001680775,
122.521469007001)) ;
#76278=CARTESIAN_POINT('Ctrl Pts',(-18.2161904040798,-35.1418928107692,
122.490230413677)) ;
#76279=CARTESIAN_POINT('Ctrl Pts',(-18.4547977047164,-34.9619037303504,
122.674558035766)) ;
#76280=CARTESIAN_POINT('Ctrl Pts',(-18.0736527311834,-35.1519534886472,
122.712860272245)) ;
#76281=CARTESIAN_POINT('Ctrl Pts',(-18.3407694238614,-34.9719644082284,
122.852663144503)) ;
#76282=CARTESIAN_POINT('Ctrl Pts',(-17.9738293171921,-35.1617937865966,
122.951450001388)) ;
#76283=CARTESIAN_POINT('Ctrl Pts',(-18.2609128496764,-34.9818047061779,
123.043535471726)) ;
#76284=CARTESIAN_POINT('Ctrl Pts',(-17.9153656042715,-35.1718567815061,
123.209316008971)) ;
#76285=CARTESIAN_POINT('Ctrl Pts',(-18.2141439991331,-34.9918677010873,
123.249828796046)) ;
#76286=CARTESIAN_POINT('Ctrl Pts',(-17.9029906880306,-35.1817510756532,
123.469061216251)) ;
#76287=CARTESIAN_POINT('Ctrl Pts',(-18.2042462718512,-35.0017619952345,
123.457624801608)) ;
#76288=CARTESIAN_POINT('Ctrl Pts',(-17.9353509723989,-35.1916928733501,
123.728277083036)) ;
#76289=CARTESIAN_POINT('Ctrl Pts',(-18.230136599556,-35.0117037929313,123.664997019035)) ;
#76290=CARTESIAN_POINT('Ctrl Pts',(-18.0126256103988,-35.2016954508792,
123.979555436244)) ;
#76291=CARTESIAN_POINT('Ctrl Pts',(-18.2919583264141,-35.0217063704604,
123.866019011557)) ;
#76292=CARTESIAN_POINT('Ctrl Pts',(-18.1330779755953,-35.2117299148002,
124.214117512303)) ;
#76293=CARTESIAN_POINT('Ctrl Pts',(-18.3883221539504,-35.0317408343815,
124.053667693136)) ;
#76294=CARTESIAN_POINT('Ctrl Pts',(-18.2891276129428,-35.2215760533213,
124.420521008454)) ;
#76295=CARTESIAN_POINT('Ctrl Pts',(-18.5131632916011,-35.0415869729026,
124.218788844697)) ;
#76296=CARTESIAN_POINT('Ctrl Pts',(-18.4808245708617,-35.2315572265583,
124.599517750244)) ;
#76297=CARTESIAN_POINT('Ctrl Pts',(-18.6665221721677,-35.0515681461396,
124.361984625144)) ;
#76298=CARTESIAN_POINT('Ctrl Pts',(-18.7001113066262,-35.2415095205156,
124.742060651138)) ;
#76299=CARTESIAN_POINT('Ctrl Pts',(-18.8419525117809,-35.0615204400968,
124.476017085114)) ;
#76300=CARTESIAN_POINT('Ctrl Pts',(-18.9418196622189,-35.2515083156502,
124.845159871801)) ;
#76301=CARTESIAN_POINT('Ctrl Pts',(-19.0353199196314,-35.0715192352314,
124.558494551332)) ;
#76302=CARTESIAN_POINT('Ctrl Pts',(-19.1988694220075,-35.261547423911,124.904462676916)) ;
#76303=CARTESIAN_POINT('Ctrl Pts',(-19.2409602470283,-35.0815583434922,
124.605934759269)) ;
#76304=CARTESIAN_POINT('Ctrl Pts',(-19.4566932433143,-35.2713723653501,
124.918494235249)) ;
#76305=CARTESIAN_POINT('Ctrl Pts',(-19.4472187973089,-35.0913832849314,
124.617157941595)) ;
#76306=CARTESIAN_POINT('Ctrl Pts',(-19.7190507496246,-35.2814270524245,
124.887257605377)) ;
#76307=CARTESIAN_POINT('Ctrl Pts',(-19.6571046535086,-35.1014379720058,
124.592166657345)) ;
#76308=CARTESIAN_POINT('Ctrl Pts',(-19.9690783925478,-35.2913698573647,
124.811356103784)) ;
#76309=CARTESIAN_POINT('Ctrl Pts',(-19.8571259192075,-35.1113807769459,
124.531443580824)) ;
#76310=CARTESIAN_POINT('Ctrl Pts',(-20.201572991337,-35.3012736433612,124.694371844352)) ;
#76311=CARTESIAN_POINT('Ctrl Pts',(-20.0431203471688,-35.1212845629424,
124.437854636998)) ;
#76312=CARTESIAN_POINT('Ctrl Pts',(-20.4131178490752,-35.311320459926,124.536438012356)) ;
#76313=CARTESIAN_POINT('Ctrl Pts',(-20.2123551289518,-35.1313313795072,
124.311505953245)) ;
#76314=CARTESIAN_POINT('Ctrl Pts',(-20.5915179796909,-35.3212159794047,
124.347180770811)) ;
#76315=CARTESIAN_POINT('Ctrl Pts',(-20.3550735141645,-35.1412268989859,
124.160099180785)) ;
#76316=CARTESIAN_POINT('Ctrl Pts',(-20.7367072779977,-35.3312780647291,
124.126231712298)) ;
#76317=CARTESIAN_POINT('Ctrl Pts',(-20.4712234236235,-35.1512889843104,
123.983338754042)) ;
#76318=CARTESIAN_POINT('Ctrl Pts',(-20.8392082178342,-35.341120775687,123.888720097005)) ;
#76319=CARTESIAN_POINT('Ctrl Pts',(-20.5532221538063,-35.1611316952683,
123.793329345071)) ;
#76320=CARTESIAN_POINT('Ctrl Pts',(-20.9004009017914,-35.3511114929931,
123.633439183863)) ;
#76321=CARTESIAN_POINT('Ctrl Pts',(-20.6021745071673,-35.1711224125743,
123.589104328749)) ;
#76322=CARTESIAN_POINT('Ctrl Pts',(-20.9161968439774,-35.3610395760897,
123.373005745108)) ;
#76323=CARTESIAN_POINT('Ctrl Pts',(-20.6148094255355,-35.1810504956709,
123.38075785787)) ;
#76324=CARTESIAN_POINT('Ctrl Pts',(-20.8868090726175,-35.3710275062014,
123.112172972234)) ;
#76325=CARTESIAN_POINT('Ctrl Pts',(-20.5912974941036,-35.1910384257827,
123.172091979698)) ;
#76326=CARTESIAN_POINT('Ctrl Pts',(-20.8118024545618,-35.3810633323287,
122.859341843784)) ;
#76327=CARTESIAN_POINT('Ctrl Pts',(-20.5312904395145,-35.20107425191,122.969827526995)) ;
#76328=CARTESIAN_POINT('Ctrl Pts',(-20.6965136130344,-35.3909186694423,
122.627413231275)) ;
#76329=CARTESIAN_POINT('Ctrl Pts',(-20.4390581291398,-35.2109295890236,
122.784286070346)) ;
#76330=CARTESIAN_POINT('Ctrl Pts',(-20.5408432692732,-35.4009164042925,
122.415802978971)) ;
#76331=CARTESIAN_POINT('Ctrl Pts',(-20.3145205770678,-35.2209273238737,
122.614998959278)) ;
#76332=CARTESIAN_POINT('Ctrl Pts',(-20.3525343320778,-35.4108243082769,
122.235974665566)) ;
#76333=CARTESIAN_POINT('Ctrl Pts',(-20.1638726660472,-35.2308352278582,
122.471137872087)) ;
#76334=CARTESIAN_POINT('Ctrl Pts',(-20.1338538120055,-35.4208353828254,
122.089706748556)) ;
#76335=CARTESIAN_POINT('Ctrl Pts',(-19.9889274042967,-35.2408463024066,
122.354124872877)) ;
#76336=CARTESIAN_POINT('Ctrl Pts',(-19.8924829761776,-35.430863238361,121.983948431129)) ;
#76337=CARTESIAN_POINT('Ctrl Pts',(-19.7958300154897,-35.2508741579423,
122.26951973446)) ;
#76338=CARTESIAN_POINT('Ctrl Pts',(-19.6408783355225,-35.4407208322662,
121.922312589323)) ;
#76339=CARTESIAN_POINT('Ctrl Pts',(-19.5945467001667,-35.2607317518475,
122.220212798044)) ;
#76340=CARTESIAN_POINT('Ctrl Pts',(-19.3779878358357,-35.4507475191043,
121.904471410779)) ;
#76341=CARTESIAN_POINT('Ctrl Pts',(-19.3842341773709,-35.2707584386856,
122.205941341526)) ;
#76342=CARTESIAN_POINT('Ctrl Pts',(-19.1160071597598,-35.4607761882581,
121.933207053229)) ;
#76343=CARTESIAN_POINT('Ctrl Pts',(-19.1746497551832,-35.2807871078393,
122.228931467457)) ;
#76344=CARTESIAN_POINT('Ctrl Pts',(-18.8675097602548,-35.4706213965395,
122.005176454191)) ;
#76345=CARTESIAN_POINT('Ctrl Pts',(-18.975853120482,-35.2906323161207,122.286508201954)) ;
#76346=CARTESIAN_POINT('Ctrl Pts',(-18.6315240045913,-35.4806120855026,
122.120258716162)) ;
#76347=CARTESIAN_POINT('Ctrl Pts',(-18.787065262531,-35.3006230050839,122.3785751853)) ;
#76348=CARTESIAN_POINT('Ctrl Pts',(-18.4184551336029,-35.4906499617849,
122.275766762473)) ;
#76349=CARTESIAN_POINT('Ctrl Pts',(-18.6166109641243,-35.3106608813661,
122.502982897611)) ;
#76350=CARTESIAN_POINT('Ctrl Pts',(-18.2388143580411,-35.5004943394271,
122.461939201229)) ;
#76351=CARTESIAN_POINT('Ctrl Pts',(-18.472900009195,-35.3205052590084,122.651921150758)) ;
#76352=CARTESIAN_POINT('Ctrl Pts',(-18.0917605509489,-35.5104791438185,
122.679207506893)) ;
#76353=CARTESIAN_POINT('Ctrl Pts',(-18.3552581535845,-35.3304900633998,
122.825736359485)) ;
#76354=CARTESIAN_POINT('Ctrl Pts',(-17.9850190705562,-35.5204186740371,
122.917641507262)) ;
#76355=CARTESIAN_POINT('Ctrl Pts',(-18.2698663114521,-35.3404295936183,
123.016483683079)) ;
#76356=CARTESIAN_POINT('Ctrl Pts',(-17.9207300902024,-35.530458362074,123.173500108598)) ;
#76357=CARTESIAN_POINT('Ctrl Pts',(-18.2184363504254,-35.3504692816552,
123.221170992911)) ;
#76358=CARTESIAN_POINT('Ctrl Pts',(-17.9019975599719,-35.5403466514423,
123.432693219791)) ;
#76359=CARTESIAN_POINT('Ctrl Pts',(-18.2034516388014,-35.3603575710235,
123.428524836043)) ;
#76360=CARTESIAN_POINT('Ctrl Pts',(-17.9283290133231,-35.5503357751271,
123.693863790496)) ;
#76361=CARTESIAN_POINT('Ctrl Pts',(-18.2245179343512,-35.3703466947083,
123.637461006412)) ;
#76362=CARTESIAN_POINT('Ctrl Pts',(-17.9995984432438,-35.5602957848017,
123.945708092108)) ;
#76363=CARTESIAN_POINT('Ctrl Pts',(-18.2815345383664,-35.3803067043829,
123.83893578616)) ;
#76364=CARTESIAN_POINT('Ctrl Pts',(-18.1122794988798,-35.5701962145059,
124.180223126133)) ;
#76365=CARTESIAN_POINT('Ctrl Pts',(-18.3716800348444,-35.3902071340872,
124.026546724073)) ;
#76366=CARTESIAN_POINT('Ctrl Pts',(-18.2661525939109,-35.5802392959127,
124.394633262536)) ;
#76367=CARTESIAN_POINT('Ctrl Pts',(-18.4947794676731,-35.4002502154939,
124.198074338897)) ;
#76368=CARTESIAN_POINT('Ctrl Pts',(-18.4523813316654,-35.5901466898203,
124.576598857735)) ;
#76369=CARTESIAN_POINT('Ctrl Pts',(-18.6437627318548,-35.4101576094016,
124.343645597368)) ;
#76370=CARTESIAN_POINT('Ctrl Pts',(-18.6693558213906,-35.6001584208095,
124.725406064424)) ;
#76371=CARTESIAN_POINT('Ctrl Pts',(-18.817342832175,-35.4201693403907,124.462690554545)) ;
#76372=CARTESIAN_POINT('Ctrl Pts',(-18.9095840015466,-35.6101906385243,
124.834028669313)) ;
#76373=CARTESIAN_POINT('Ctrl Pts',(-19.0095258944054,-35.4302015581055,
124.549587692303)) ;
#76374=CARTESIAN_POINT('Ctrl Pts',(-19.1603393482512,-35.6200431477704,
124.898453661769)) ;
#76375=CARTESIAN_POINT('Ctrl Pts',(-19.2101294376099,-35.4400540673517,
124.601126473367)) ;
#76376=CARTESIAN_POINT('Ctrl Pts',(-19.4211928177093,-35.6300010843134,
124.919386454417)) ;
#76377=CARTESIAN_POINT('Ctrl Pts',(-19.4188119019026,-35.4500120038947,
124.617871878894)) ;
#76378=CARTESIAN_POINT('Ctrl Pts',(-19.6837654584698,-35.6400399543217,
124.894038281301)) ;
#76379=CARTESIAN_POINT('Ctrl Pts',(-19.6288700585704,-35.460050873903,124.59759241855)) ;
#76380=CARTESIAN_POINT('Ctrl Pts',(-19.933939291399,-35.64991310948,124.825100619507)) ;
#76381=CARTESIAN_POINT('Ctrl Pts',(-19.8290080447909,-35.4699240290612,
124.542441760864)) ;
#76382=CARTESIAN_POINT('Ctrl Pts',(-20.1729716448269,-35.6599863843297,
124.711483830353)) ;
#76383=CARTESIAN_POINT('Ctrl Pts',(-20.0202338855392,-35.4799973039109,
124.451547444271)) ;
#76384=CARTESIAN_POINT('Ctrl Pts',(-20.3835167615807,-35.6698067015071,
124.562152640073)) ;
#76385=CARTESIAN_POINT('Ctrl Pts',(-20.1886685395271,-35.4898176210883,
124.332082614018)) ;
#76386=CARTESIAN_POINT('Ctrl Pts',(-20.5697933970756,-35.6798853873006,
124.373961088666)) ;
#76387=CARTESIAN_POINT('Ctrl Pts',(-20.337689632591,-35.4998963068818,124.1815286286)) ;
#76388=CARTESIAN_POINT('Ctrl Pts',(-20.7173141231038,-35.6897368986837,
124.161139832824)) ;
#76389=CARTESIAN_POINT('Ctrl Pts',(-20.4557050752507,-35.5097478182649,
124.011272119984)) ;
#76390=CARTESIAN_POINT('Ctrl Pts',(-20.8282376598515,-35.6998103449903,
123.920835993588)) ;
#76391=CARTESIAN_POINT('Ctrl Pts',(-20.5444435077093,-35.5198212645716,
123.81902847826)) ;
#76392=CARTESIAN_POINT('Ctrl Pts',(-20.8941975463074,-35.709651620115,123.670739828065)) ;
#76393=CARTESIAN_POINT('Ctrl Pts',(-20.5972105412205,-35.5296625396963,
123.618952491442)) ;
#76394=CARTESIAN_POINT('Ctrl Pts',(-20.9168565667125,-35.7196367197718,
123.409346913405)) ;
#76395=CARTESIAN_POINT('Ctrl Pts',(-20.6153373392901,-35.539647639353,123.409838356451)) ;
#76396=CARTESIAN_POINT('Ctrl Pts',(-20.8933643886205,-35.7296441959061,
123.147392528949)) ;
#76397=CARTESIAN_POINT('Ctrl Pts',(-20.5965431125166,-35.5496551154873,
123.200274949627)) ;
#76398=CARTESIAN_POINT('Ctrl Pts',(-20.8255661488253,-35.739566783615,122.895618637238)) ;
#76399=CARTESIAN_POINT('Ctrl Pts',(-20.5423042616246,-35.5595777031963,
122.998856548276)) ;
#76400=CARTESIAN_POINT('Ctrl Pts',(-20.7147391059378,-35.7495533878884,
122.657703592523)) ;
#76401=CARTESIAN_POINT('Ctrl Pts',(-20.4536424122356,-35.5695643074696,
122.80852482131)) ;
#76402=CARTESIAN_POINT('Ctrl Pts',(-20.5631005958561,-35.7595935162225,
122.44181432367)) ;
#76403=CARTESIAN_POINT('Ctrl Pts',(-20.3323311466458,-35.5796044358037,
122.635813545013)) ;
#76404=CARTESIAN_POINT('Ctrl Pts',(-20.3803788347583,-35.7694329507559,
122.258824742505)) ;
#76405=CARTESIAN_POINT('Ctrl Pts',(-20.1861543576817,-35.5894438703371,
122.489422939203)) ;
#76406=CARTESIAN_POINT('Ctrl Pts',(-20.1640017994707,-35.7794970052469,
122.106806406676)) ;
#76407=CARTESIAN_POINT('Ctrl Pts',(-20.0130523328328,-35.5995079248281,
122.36780830073)) ;
#76408=CARTESIAN_POINT('Ctrl Pts',(-19.9285321533721,-35.789387924484,121.996676734364)) ;
#76409=CARTESIAN_POINT('Ctrl Pts',(-19.8246772528639,-35.6093988440653,
122.279705175091)) ;
#76410=CARTESIAN_POINT('Ctrl Pts',(-19.6751379025665,-35.7993799177901,
121.927884966062)) ;
#76411=CARTESIAN_POINT('Ctrl Pts',(-19.6219619807546,-35.6193908373713,
122.224671942912)) ;
#76412=CARTESIAN_POINT('Ctrl Pts',(-19.414382263436,-35.8093427817494,121.904446853301)) ;
#76413=CARTESIAN_POINT('Ctrl Pts',(-19.4133578143958,-35.6293537013306,
122.205921690293)) ;
#76414=CARTESIAN_POINT('Ctrl Pts',(-19.1549680514834,-35.8192470415671,
121.925855666105)) ;
#76415=CARTESIAN_POINT('Ctrl Pts',(-19.2058271969419,-35.6392579611484,
122.223048715094)) ;
#76416=CARTESIAN_POINT('Ctrl Pts',(-18.899352673591,-35.8293075321386,121.993232864623)) ;
#76417=CARTESIAN_POINT('Ctrl Pts',(-19.001334645375,-35.6493184517198,122.276950638567)) ;
#76418=CARTESIAN_POINT('Ctrl Pts',(-18.6643671184451,-35.8391478817696,
122.101269435789)) ;
#76419=CARTESIAN_POINT('Ctrl Pts',(-18.8133472746285,-35.6591588013508,
122.363379411723)) ;
#76420=CARTESIAN_POINT('Ctrl Pts',(-18.4467771153148,-35.8492108572596,
122.251492745657)) ;
#76421=CARTESIAN_POINT('Ctrl Pts',(-18.6392749852965,-35.6692217768408,
122.483558171074)) ;
#76422=CARTESIAN_POINT('Ctrl Pts',(-18.2618359406519,-35.859105177403,122.43429871186)) ;
#76423=CARTESIAN_POINT('Ctrl Pts',(-18.491322616233,-35.6791160969842,122.629802358124)) ;
#76424=CARTESIAN_POINT('Ctrl Pts',(-18.1101865600528,-35.8690468905346,
122.646995886954)) ;
#76425=CARTESIAN_POINT('Ctrl Pts',(-18.3700032496171,-35.6890578101158,
122.799959569415)) ;
#76426=CARTESIAN_POINT('Ctrl Pts',(-17.9969449046416,-35.8790497803287,
122.884263259483)) ;
#76427=CARTESIAN_POINT('Ctrl Pts',(-18.2794097634867,-35.69906069991,122.989773283224)) ;
#76428=CARTESIAN_POINT('Ctrl Pts',(-17.9268443213951,-35.8890896374892,
123.138590645387)) ;
#76429=CARTESIAN_POINT('Ctrl Pts',(-18.2233291597186,-35.7091005570704,
123.193235305604)) ;
#76430=CARTESIAN_POINT('Ctrl Pts',(-17.9019122828192,-35.8989138183268,
123.395574782341)) ;
#76431=CARTESIAN_POINT('Ctrl Pts',(-18.2033834027197,-35.7189247379081,
123.398821321961)) ;
#76432=CARTESIAN_POINT('Ctrl Pts',(-17.9220883777704,-35.90897079183,123.659068393634)) ;
#76433=CARTESIAN_POINT('Ctrl Pts',(-18.2195239554329,-35.7289817114113,
123.609616505664)) ;
#76434=CARTESIAN_POINT('Ctrl Pts',(-17.987198604821,-35.9188989160171,123.91172955812)) ;
#76435=CARTESIAN_POINT('Ctrl Pts',(-18.271611742449,-35.7389098355983,123.811744931268)) ;
#76436=CARTESIAN_POINT('Ctrl Pts',(-18.0948259750303,-35.9288526110905,
124.150136156843)) ;
#76437=CARTESIAN_POINT('Ctrl Pts',(-18.3577130663129,-35.7488635306717,
124.002469995443)) ;
#76438=CARTESIAN_POINT('Ctrl Pts',(-18.2438917114854,-35.9388988046658,
124.368025600054)) ;
#76439=CARTESIAN_POINT('Ctrl Pts',(-18.4769654839936,-35.758909724247,124.176781901697)) ;
#76440=CARTESIAN_POINT('Ctrl Pts',(-18.4247087144737,-35.9487469070257,
124.553177298438)) ;
#76441=CARTESIAN_POINT('Ctrl Pts',(-18.6216180178333,-35.7687578266069,
124.324902741368)) ;
#76442=CARTESIAN_POINT('Ctrl Pts',(-18.6368680942893,-35.9587084952533,
124.706511430736)) ;
#76443=CARTESIAN_POINT('Ctrl Pts',(-18.7913448718134,-35.7787194148345,
124.44757032455)) ;
#76444=CARTESIAN_POINT('Ctrl Pts',(-18.8741832744465,-35.9687371654095,
124.821161297366)) ;
#76445=CARTESIAN_POINT('Ctrl Pts',(-18.9811968587923,-35.7887480849908,
124.539290720976)) ;
#76446=CARTESIAN_POINT('Ctrl Pts',(-19.1247583601931,-35.9786474682913,
124.892091064611)) ;
#76447=CARTESIAN_POINT('Ctrl Pts',(-19.1816561053087,-35.7986583878725,
124.59603486579)) ;
#76448=CARTESIAN_POINT('Ctrl Pts',(-19.3844352240808,-35.9885823520992,
124.919183512101)) ;
#76449=CARTESIAN_POINT('Ctrl Pts',(-19.3893969971606,-35.8085932716804,
124.617709476599)) ;
#76450=CARTESIAN_POINT('Ctrl Pts',(-19.6476231191656,-35.9986234937898,
124.900335055158)) ;
#76451=CARTESIAN_POINT('Ctrl Pts',(-19.5999475089394,-35.8186344133711,
124.602631349119)) ;
#76452=CARTESIAN_POINT('Ctrl Pts',(-19.8996824513268,-36.0085106149538,
124.83723224939)) ;
#76453=CARTESIAN_POINT('Ctrl Pts',(-19.8015943370243,-35.828521534535,124.552149980266)) ;
#76454=CARTESIAN_POINT('Ctrl Pts',(-20.1396295183262,-36.0185029578023,
124.730608252224)) ;
#76455=CARTESIAN_POINT('Ctrl Pts',(-19.9935521670757,-35.8385138773836,
124.466851580924)) ;
#76456=CARTESIAN_POINT('Ctrl Pts',(-20.3564426703824,-36.0284512590263,
124.584508836184)) ;
#76457=CARTESIAN_POINT('Ctrl Pts',(-20.1670027663451,-35.8484621786075,
124.34997293713)) ;
#76458=CARTESIAN_POINT('Ctrl Pts',(-20.544635127036,-36.0383888367084,124.403471920476)) ;
#76459=CARTESIAN_POINT('Ctrl Pts',(-20.3175569672634,-35.8583997562896,
124.205144391475)) ;
#76460=CARTESIAN_POINT('Ctrl Pts',(-20.6995297068178,-36.0483754111589,
124.191598913506)) ;
#76461=CARTESIAN_POINT('Ctrl Pts',(-20.4414732773456,-35.8683863307402,
124.035646689111)) ;
#76462=CARTESIAN_POINT('Ctrl Pts',(-20.8154914357091,-36.0584042210674,
123.95493766918)) ;
#76463=CARTESIAN_POINT('Ctrl Pts',(-20.5342434668736,-35.8784151406487,
123.846318005785)) ;
#76464=CARTESIAN_POINT('Ctrl Pts',(-20.8877452575708,-36.0682825423742,
123.705606150778)) ;
#76465=CARTESIAN_POINT('Ctrl Pts',(-20.5920471744882,-35.8882934619554,
123.646853866704)) ;
#76466=CARTESIAN_POINT('Ctrl Pts',(-20.9165435265095,-36.0782741897216,
123.444611225451)) ;
#76467=CARTESIAN_POINT('Ctrl Pts',(-20.6150868306485,-35.8982851093029,
123.438058194467)) ;
#76468=CARTESIAN_POINT('Ctrl Pts',(-20.8989774526659,-36.0883087131594,
123.181512331522)) ;
#76469=CARTESIAN_POINT('Ctrl Pts',(-20.6010349029805,-35.9083196327406,
123.227578932499)) ;
#76470=CARTESIAN_POINT('Ctrl Pts',(-20.8375844348363,-36.098172070038,122.929660650896)) ;
#76471=CARTESIAN_POINT('Ctrl Pts',(-20.55192174251,-35.9181829896192,123.026098230027)) ;
#76472=CARTESIAN_POINT('Ctrl Pts',(-20.7312794062395,-36.1082422967183,
122.687347241502)) ;
#76473=CARTESIAN_POINT('Ctrl Pts',(-20.4668785833512,-35.9282532162995,
122.832246790872)) ;
#76474=CARTESIAN_POINT('Ctrl Pts',(-20.5878041611875,-36.118084604853,122.472130151243)) ;
#76475=CARTESIAN_POINT('Ctrl Pts',(-20.3520998563727,-35.9380955244342,
122.660073387355)) ;
#76476=CARTESIAN_POINT('Ctrl Pts',(-20.4077016433411,-36.1280453368764,
122.282190824052)) ;
#76477=CARTESIAN_POINT('Ctrl Pts',(-20.2080190009201,-35.9480562564576,
122.50812127463)) ;
#76478=CARTESIAN_POINT('Ctrl Pts',(-20.1954179813538,-36.1380832260745,
122.125622966296)) ;
#76479=CARTESIAN_POINT('Ctrl Pts',(-20.0381926818535,-35.9580941456557,
122.382865981336)) ;
#76480=CARTESIAN_POINT('Ctrl Pts',(-19.9632011128063,-36.1479575089933,
122.009756791279)) ;
#76481=CARTESIAN_POINT('Ctrl Pts',(-19.852420481698,-35.9679684285746,122.290172259536)) ;
#76482=CARTESIAN_POINT('Ctrl Pts',(-19.7095295605518,-36.1580272536108,
121.934544304188)) ;
#76483=CARTESIAN_POINT('Ctrl Pts',(-19.6494833349554,-35.978038173192,122.230000967982)) ;
#76484=CARTESIAN_POINT('Ctrl Pts',(-19.4527844207,-36.1678605639564,121.905081249656)) ;
#76485=CARTESIAN_POINT('Ctrl Pts',(-19.4440883880503,-35.9878714835377,
122.206429346442)) ;
#76486=CARTESIAN_POINT('Ctrl Pts',(-19.1896400044827,-36.1778908073091,
121.920204651344)) ;
#76487=CARTESIAN_POINT('Ctrl Pts',(-19.2335727027001,-35.9979017268903,
122.218526613797)) ;
#76488=CARTESIAN_POINT('Ctrl Pts',(-18.9332371753913,-36.1879230952875,
121.981571396633)) ;
#76489=CARTESIAN_POINT('Ctrl Pts',(-19.0284500699383,-36.0079340148687,
122.267618766793)) ;
#76490=CARTESIAN_POINT('Ctrl Pts',(-18.6960884546882,-36.1977502717556,
122.083816541802)) ;
#76491=CARTESIAN_POINT('Ctrl Pts',(-18.838731476733,-36.0177611913368,122.349413165543)) ;
#76492=CARTESIAN_POINT('Ctrl Pts',(-18.4761127316543,-36.2077556546224,
122.227783640436)) ;
#76493=CARTESIAN_POINT('Ctrl Pts',(-18.6627501158308,-36.0277665742037,
122.464585522614)) ;
#76494=CARTESIAN_POINT('Ctrl Pts',(-18.2849106465247,-36.2177382936152,
122.407469429995)) ;
#76495=CARTESIAN_POINT('Ctrl Pts',(-18.5097875384203,-36.0377492131964,
122.60833293523)) ;
#76496=CARTESIAN_POINT('Ctrl Pts',(-18.1271511615544,-36.2277823607518,
122.61904959903)) ;
#76497=CARTESIAN_POINT('Ctrl Pts',(-18.3835787128746,-36.047793280333,122.777596301397)) ;
#76498=CARTESIAN_POINT('Ctrl Pts',(-18.0107408056711,-36.2376035795558,
122.84940714592)) ;
#76499=CARTESIAN_POINT('Ctrl Pts',(-18.2904495064269,-36.057614499137,122.961880755855)) ;
#76500=CARTESIAN_POINT('Ctrl Pts',(-17.9338160940377,-36.2476404184938,
123.101693464126)) ;
#76501=CARTESIAN_POINT('Ctrl Pts',(-18.2289081204975,-36.0676513380751,
123.163709405385)) ;
#76502=CARTESIAN_POINT('Ctrl Pts',(-17.9026486631105,-36.2576648305916,
123.36328314838)) ;
#76503=CARTESIAN_POINT('Ctrl Pts',(-18.2039726598348,-36.0776757501728,
123.372980991972)) ;
#76504=CARTESIAN_POINT('Ctrl Pts',(-17.9165495302579,-36.2675169149969,
123.621816862734)) ;
#76505=CARTESIAN_POINT('Ctrl Pts',(-18.2150916816491,-36.0875278345781,
123.579807245692)) ;
#76506=CARTESIAN_POINT('Ctrl Pts',(-17.9755567900493,-36.27750781174,123.877618050262)) ;
#76507=CARTESIAN_POINT('Ctrl Pts',(-18.2622957977157,-36.0975187313213,
123.784448445474)) ;
#76508=CARTESIAN_POINT('Ctrl Pts',(-18.077203160799,-36.287425803641,124.117648747787)) ;
#76509=CARTESIAN_POINT('Ctrl Pts',(-18.3436111230473,-36.1074367232222,
123.976473257481)) ;
#76510=CARTESIAN_POINT('Ctrl Pts',(-18.2204755142944,-36.297453919098,124.338803226276)) ;
#76511=CARTESIAN_POINT('Ctrl Pts',(-18.4582275584006,-36.1174648386792,
124.153397810827)) ;
#76512=CARTESIAN_POINT('Ctrl Pts',(-18.3973504808936,-36.3073390950401,
124.529066690631)) ;
#76513=CARTESIAN_POINT('Ctrl Pts',(-18.5997258423448,-36.1273500146213,
124.30560934978)) ;
#76514=CARTESIAN_POINT('Ctrl Pts',(-18.606372387198,-36.317328453447,124.687887703302)) ;
#76515=CARTESIAN_POINT('Ctrl Pts',(-18.7669421404985,-36.1373393730282,
124.43266756716)) ;
#76516=CARTESIAN_POINT('Ctrl Pts',(-18.8412552934067,-36.3273696010273,
124.808127004858)) ;
#76517=CARTESIAN_POINT('Ctrl Pts',(-18.9548477220754,-36.1473805206085,
124.528860620491)) ;
#76518=CARTESIAN_POINT('Ctrl Pts',(-19.0880822046811,-36.3372022240337,
124.884553235506)) ;
#76519=CARTESIAN_POINT('Ctrl Pts',(-19.1523079763883,-36.157213143615,124.590003139103)) ;
#76520=CARTESIAN_POINT('Ctrl Pts',(-19.3485418518616,-36.3471962951445,
124.918229067324)) ;
#76521=CARTESIAN_POINT('Ctrl Pts',(-19.3606753488184,-36.1672072147257,
124.616945728324)) ;
#76522=CARTESIAN_POINT('Ctrl Pts',(-19.6117962054369,-36.3572249527853,
124.905606556928)) ;
#76523=CARTESIAN_POINT('Ctrl Pts',(-19.571278932422,-36.1772358723666,124.606849593265)) ;
#76524=CARTESIAN_POINT('Ctrl Pts',(-19.8651977310147,-36.3671092789782,
124.848586979644)) ;
#76525=CARTESIAN_POINT('Ctrl Pts',(-19.7740000730835,-36.1871201985594,
124.561235916018)) ;
#76526=CARTESIAN_POINT('Ctrl Pts',(-20.1070919689102,-36.3770750224688,
124.748197482078)) ;
#76527=CARTESIAN_POINT('Ctrl Pts',(-19.9675160571563,-36.19708594205,124.480926240918)) ;
#76528=CARTESIAN_POINT('Ctrl Pts',(-20.3290461476905,-36.3871034016,124.606136879373)) ;
#76529=CARTESIAN_POINT('Ctrl Pts',(-20.1450804639494,-36.2071143211812,
124.367279397955)) ;
#76530=CARTESIAN_POINT('Ctrl Pts',(-20.5207969132136,-36.3970042478069,
124.430224963432)) ;
#76531=CARTESIAN_POINT('Ctrl Pts',(-20.2984821301222,-36.2170151673881,
124.226551616459)) ;
#76532=CARTESIAN_POINT('Ctrl Pts',(-20.6815114755106,-36.407062905224,124.220415524645)) ;
#76533=CARTESIAN_POINT('Ctrl Pts',(-20.4270554231223,-36.2270738248052,
124.058705203557)) ;
#76534=CARTESIAN_POINT('Ctrl Pts',(-20.8012013744469,-36.4169204680059,
123.990625446844)) ;
#76535=CARTESIAN_POINT('Ctrl Pts',(-20.5228088997045,-36.2369313875871,
123.874874540363)) ;
#76536=CARTESIAN_POINT('Ctrl Pts',(-20.8809810995095,-36.4269888705591,
123.738394192403)) ;
#76537=CARTESIAN_POINT('Ctrl Pts',(-20.5866346717548,-36.2469997901403,
123.673090038089)) ;
#76538=CARTESIAN_POINT('Ctrl Pts',(-20.9150001538279,-36.4368442692987,
123.481625971232)) ;
#76539=CARTESIAN_POINT('Ctrl Pts',(-20.6138518770455,-36.2568551888799,
123.467676224677)) ;
#76540=CARTESIAN_POINT('Ctrl Pts',(-20.9045521215067,-36.4468391363726,
123.219187981019)) ;
#76541=CARTESIAN_POINT('Ctrl Pts',(-20.6054955832144,-36.2668500559538,
123.257725827146)) ;
#76542=CARTESIAN_POINT('Ctrl Pts',(-20.8479327597184,-36.456870431356,122.961723074858)) ;
#76543=CARTESIAN_POINT('Ctrl Pts',(-20.5602021162859,-36.2768813509373,
123.051753458956)) ;
#76544=CARTESIAN_POINT('Ctrl Pts',(-20.7495006731803,-36.4667369560826,
122.721841789023)) ;
#76545=CARTESIAN_POINT('Ctrl Pts',(-20.4814585578185,-36.2867478756638,
122.859848009329)) ;
#76546=CARTESIAN_POINT('Ctrl Pts',(-20.6095919097615,-36.4767244267783,
122.499818683209)) ;
#76547=CARTESIAN_POINT('Ctrl Pts',(-20.36953342095,-36.2967353463596,122.68222845983)) ;
#76548=CARTESIAN_POINT('Ctrl Pts',(-20.4340715147178,-36.4866691863422,
122.306140896077)) ;
#76549=CARTESIAN_POINT('Ctrl Pts',(-20.2291188313566,-36.3066801059234,
122.527284917964)) ;
#76550=CARTESIAN_POINT('Ctrl Pts',(-20.2254502142626,-36.496714742291,122.144429454207)) ;
#76551=CARTESIAN_POINT('Ctrl Pts',(-20.0622230962988,-36.3167256618723,
122.397914055264)) ;
#76552=CARTESIAN_POINT('Ctrl Pts',(-19.9963181527687,-36.5065743306661,
122.023404638943)) ;
#76553=CARTESIAN_POINT('Ctrl Pts',(-19.8789187628921,-36.3265852502474,
122.301092445277)) ;
#76554=CARTESIAN_POINT('Ctrl Pts',(-19.7463087037806,-36.5165752858022,
121.942510562541)) ;
#76555=CARTESIAN_POINT('Ctrl Pts',(-19.6789119467519,-36.3365862053834,
122.236375109967)) ;
#76556=CARTESIAN_POINT('Ctrl Pts',(-19.488513689031,-36.5264795130797,121.906393185081)) ;
#76557=CARTESIAN_POINT('Ctrl Pts',(-19.472676448649,-36.346490432661,122.207479050223)) ;
#76558=CARTESIAN_POINT('Ctrl Pts',(-19.22481600771,-36.5365215899749,121.91563802328)) ;
#76559=CARTESIAN_POINT('Ctrl Pts',(-19.2617182336787,-36.3565325095561,
122.214872707114)) ;
#76560=CARTESIAN_POINT('Ctrl Pts',(-18.9700774883561,-36.546429202661,121.969685726369)) ;
#76561=CARTESIAN_POINT('Ctrl Pts',(-19.0579271360362,-36.3664401222423,
122.258108661664)) ;
#76562=CARTESIAN_POINT('Ctrl Pts',(-18.7250847627376,-36.5564837332768,
122.068538595385)) ;
#76563=CARTESIAN_POINT('Ctrl Pts',(-18.8619321279312,-36.376494652858,122.337188894249)) ;
#76564=CARTESIAN_POINT('Ctrl Pts',(-18.5051552712521,-36.5663445198256,
122.20564207096)) ;
#76565=CARTESIAN_POINT('Ctrl Pts',(-18.6859875392954,-36.3863554394069,
122.446869671373)) ;
#76566=CARTESIAN_POINT('Ctrl Pts',(-18.3095046249298,-36.5763382748967,
122.380772756674)) ;
#76567=CARTESIAN_POINT('Ctrl Pts',(-18.5294655677005,-36.396349194478,122.586972503952)) ;
#76568=CARTESIAN_POINT('Ctrl Pts',(-18.1481936176702,-36.5862636351367,
122.585788118873)) ;
#76569=CARTESIAN_POINT('Ctrl Pts',(-18.4004150621657,-36.406274554718,122.750983322731)) ;
#76570=CARTESIAN_POINT('Ctrl Pts',(-18.0236841921793,-36.596291564532,122.818002834844)) ;
#76571=CARTESIAN_POINT('Ctrl Pts',(-18.300805562702,-36.4163024841132,122.936753987693)) ;
#76572=CARTESIAN_POINT('Ctrl Pts',(-17.9422706635279,-36.6061778313313,
123.064758942324)) ;
#76573=CARTESIAN_POINT('Ctrl Pts',(-18.2356726313687,-36.4261887509125,
123.134158078855)) ;
#76574=CARTESIAN_POINT('Ctrl Pts',(-17.9042663341552,-36.6162096002296,
123.325585129756)) ;
#76575=CARTESIAN_POINT('Ctrl Pts',(-18.2052669459445,-36.4362205198108,
123.342818652238)) ;
#76576=CARTESIAN_POINT('Ctrl Pts',(-17.9117588181507,-36.6260911960731,
123.585201643662)) ;
#76577=CARTESIAN_POINT('Ctrl Pts',(-18.2112586694567,-36.4461021156544,
123.55051186725)) ;
#76578=CARTESIAN_POINT('Ctrl Pts',(-17.9650896019866,-36.6361530815411,
123.844142860271)) ;
#76579=CARTESIAN_POINT('Ctrl Pts',(-18.2539211167218,-36.4561640011224,
123.757665267779)) ;
#76580=CARTESIAN_POINT('Ctrl Pts',(-18.0605371632968,-36.6460105155599,
124.084996144614)) ;
#76581=CARTESIAN_POINT('Ctrl Pts',(-18.3302769065666,-36.4660214351412,
123.950348570272)) ;
#76582=CARTESIAN_POINT('Ctrl Pts',(-18.1977180728427,-36.6560037586019,
124.308890236656)) ;
#76583=CARTESIAN_POINT('Ctrl Pts',(-18.4400203090856,-36.4760146781832,
124.129465536782)) ;
#76584=CARTESIAN_POINT('Ctrl Pts',(-18.3706217887722,-36.6659345194883,
124.50438473476)) ;
#76585=CARTESIAN_POINT('Ctrl Pts',(-18.5783393320726,-36.4859454390695,
124.285860564829)) ;
#76586=CARTESIAN_POINT('Ctrl Pts',(-18.6449288885394,-36.6792835116855,
124.723100111682)) ;
#76587=CARTESIAN_POINT('Ctrl Pts',(-18.797794429001,-36.4992944312667,124.46084539929)) ;
#76588=CARTESIAN_POINT('Ctrl Pts',(-18.9682246085293,-36.6925518845019,
124.863897618104)) ;
#76589=CARTESIAN_POINT('Ctrl Pts',(-19.0564576791259,-36.5125628040832,
124.573487208325)) ;
#76590=CARTESIAN_POINT('Ctrl Pts',(-19.3133563776457,-36.7058348258862,
124.916340475297)) ;
#76591=CARTESIAN_POINT('Ctrl Pts',(-19.3325181777442,-36.5258457454675,
124.615432945298)) ;
#76592=CARTESIAN_POINT('Ctrl Pts',(-19.5771730601713,-36.7158776117285,
124.909887095893)) ;
#76593=CARTESIAN_POINT('Ctrl Pts',(-19.5435804546175,-36.5358885313097,
124.610274688818)) ;
#76594=CARTESIAN_POINT('Ctrl Pts',(-19.8309776236179,-36.7257275542806,
124.858999538659)) ;
#76595=CARTESIAN_POINT('Ctrl Pts',(-19.7466221103153,-36.5457384738618,
124.569566509396)) ;
#76596=CARTESIAN_POINT('Ctrl Pts',(-20.0759163398703,-36.7357247871995,
124.764028514436)) ;
#76597=CARTESIAN_POINT('Ctrl Pts',(-19.9425753637021,-36.5557357067808,
124.493590557892)) ;
#76598=CARTESIAN_POINT('Ctrl Pts',(-20.300851683239,-36.7457396825341,124.627366616285)) ;
#76599=CARTESIAN_POINT('Ctrl Pts',(-20.1225212573089,-36.5657506021153,
124.384267868071)) ;
#76600=CARTESIAN_POINT('Ctrl Pts',(-20.5625371626539,-36.7589793591723,
124.39808728951)) ;
#76601=CARTESIAN_POINT('Ctrl Pts',(-20.3318880358835,-36.5789902787535,
124.200821860388)) ;
#76602=CARTESIAN_POINT('Ctrl Pts',(-20.8079029754559,-36.7755265835776,
124.033128787395)) ;
#76603=CARTESIAN_POINT('Ctrl Pts',(-20.5281632731602,-36.5955375031589,
123.908899479938)) ;
#76604=CARTESIAN_POINT('Ctrl Pts',(-20.914868930944,-36.7921740207087,123.603796766482)) ;
#76605=CARTESIAN_POINT('Ctrl Pts',(-20.6137528357625,-36.6121849402899,
123.56536784602)) ;
#76606=CARTESIAN_POINT('Ctrl Pts',(-20.9083945688034,-36.8054635181869,
123.254597757713)) ;
#76607=CARTESIAN_POINT('Ctrl Pts',(-20.6085683029633,-36.6254744377682,
123.286061935331)) ;
#76608=CARTESIAN_POINT('Ctrl Pts',(-20.8593749514375,-36.8153369260093,
122.999807024194)) ;
#76609=CARTESIAN_POINT('Ctrl Pts',(-20.56935600526,-36.6353478455905,123.082217773299)) ;
#76610=CARTESIAN_POINT('Ctrl Pts',(-20.7652312033455,-36.825389303602,122.752998369498)) ;
#76611=CARTESIAN_POINT('Ctrl Pts',(-20.4940428185494,-36.6454002231832,
122.884773343294)) ;
#76612=CARTESIAN_POINT('Ctrl Pts',(-20.6315577728681,-36.8352929571429,
122.529670136129)) ;
#76613=CARTESIAN_POINT('Ctrl Pts',(-20.3871046825718,-36.6553038767241,
122.706108244707)) ;
#76614=CARTESIAN_POINT('Ctrl Pts',(-20.4609498468132,-36.8452372261382,
122.331765024451)) ;
#76615=CARTESIAN_POINT('Ctrl Pts',(-20.250623548332,-36.6652481457194,122.547784435435)) ;
#76616=CARTESIAN_POINT('Ctrl Pts',(-20.1896663856008,-36.8585682344709,
122.109990345242)) ;
#76617=CARTESIAN_POINT('Ctrl Pts',(-20.0335788518521,-36.6785791540521,
122.3703552458)) ;
#76618=CARTESIAN_POINT('Ctrl Pts',(-19.7868089892169,-36.8751898149952,
121.928852787631)) ;
#76619=CARTESIAN_POINT('Ctrl Pts',(-19.7113302438444,-36.6952007345764,
122.22544992753)) ;
#76620=CARTESIAN_POINT('Ctrl Pts',(-19.3483970122158,-36.8917324856935,
121.895325330599)) ;
#76621=CARTESIAN_POINT('Ctrl Pts',(-19.3605382150688,-36.7117434052748,
122.198625176032)) ;
#76622=CARTESIAN_POINT('Ctrl Pts',(-19.0036058958817,-36.9050816452565,
121.959959179147)) ;
#76623=CARTESIAN_POINT('Ctrl Pts',(-19.084756195026,-36.7250925648377,122.250326885057)) ;
#76624=CARTESIAN_POINT('Ctrl Pts',(-18.6780618920126,-36.918309795416,122.081981866983)) ;
#76625=CARTESIAN_POINT('Ctrl Pts',(-18.8243006830399,-36.7383207149972,
122.347949900398)) ;
#76626=CARTESIAN_POINT('Ctrl Pts',(-18.3181836590694,-36.9349404725535,
122.338513488484)) ;
#76627=CARTESIAN_POINT('Ctrl Pts',(-18.536409956563,-36.7549513921347,122.553165511551)) ;
#76628=CARTESIAN_POINT('Ctrl Pts',(-18.0180562107128,-36.9548434118416,
122.774198058424)) ;
#76629=CARTESIAN_POINT('Ctrl Pts',(-18.2963005856459,-36.7748543314228,
122.901714217013)) ;
#76630=CARTESIAN_POINT('Ctrl Pts',(-17.8841306987683,-36.9747462784449,
123.285845641886)) ;
#76631=CARTESIAN_POINT('Ctrl Pts',(-18.1891582490799,-36.7947571980261,
123.311031567695)) ;
#76632=CARTESIAN_POINT('Ctrl Pts',(-17.9320811340281,-36.9946594435497,
123.813046654352)) ;
#76633=CARTESIAN_POINT('Ctrl Pts',(-18.2275157048257,-36.8146703631309,
123.732793421951)) ;
#76634=CARTESIAN_POINT('Ctrl Pts',(-18.1591155085534,-37.014695272691,124.294661831173)) ;
#76635=CARTESIAN_POINT('Ctrl Pts',(-18.4091406225134,-36.8347061922723,
124.118086406354)) ;
#76636=CARTESIAN_POINT('Ctrl Pts',(-18.5326928560292,-37.0345138475691,
124.666191700526)) ;
#76637=CARTESIAN_POINT('Ctrl Pts',(-18.7080017265223,-36.8545247671503,
124.415313158299)) ;
#76638=CARTESIAN_POINT('Ctrl Pts',(-19.0136563927,-37.0544841486111,124.890270639993)) ;
#76639=CARTESIAN_POINT('Ctrl Pts',(-19.0927719398134,-36.8744950681923,
124.594578398497)) ;
#76640=CARTESIAN_POINT('Ctrl Pts',(-19.5404829664597,-37.0743756809756,
124.936789595274)) ;
#76641=CARTESIAN_POINT('Ctrl Pts',(-19.5142340085164,-36.8943866005569,
124.63179555628)) ;
#76642=CARTESIAN_POINT('Ctrl Pts',(-20.0545360586527,-37.0943987787921,
124.799534983154)) ;
#76643=CARTESIAN_POINT('Ctrl Pts',(-19.9254767467742,-36.9144096983734,
124.52199379209)) ;
#76644=CARTESIAN_POINT('Ctrl Pts',(-20.4863256455072,-37.1141955317121,
124.498745537884)) ;
#76645=CARTESIAN_POINT('Ctrl Pts',(-20.2709110786742,-36.9342064512933,
124.281362358102)) ;
#76646=CARTESIAN_POINT('Ctrl Pts',(-20.7931678600069,-37.1341566202009,
124.066005974666)) ;
#76647=CARTESIAN_POINT('Ctrl Pts',(-20.5163858339727,-36.9541675397821,
123.93517078883)) ;
#76648=CARTESIAN_POINT('Ctrl Pts',(-20.9329957735426,-37.154134889133,123.553712501951)) ;
#76649=CARTESIAN_POINT('Ctrl Pts',(-20.6282493161937,-36.9741458087143,
123.525336142619)) ;
#76650=CARTESIAN_POINT('Ctrl Pts',(-20.8907271346695,-37.173954903924,123.028678283214)) ;
#76651=CARTESIAN_POINT('Ctrl Pts',(-20.5944348575025,-36.9939658235053,
123.105306484844)) ;
#76652=CARTESIAN_POINT('Ctrl Pts',(-20.6717362479784,-37.1938933131759,
122.546084069882)) ;
#76653=CARTESIAN_POINT('Ctrl Pts',(-20.4192415860018,-37.0139042327571,
122.719230493431)) ;
#76654=CARTESIAN_POINT('Ctrl Pts',(-20.2983002158022,-37.2139404305683,
122.165933042797)) ;
#76655=CARTESIAN_POINT('Ctrl Pts',(-20.1204933529623,-37.0339513501496,
122.415110073134)) ;
#76656=CARTESIAN_POINT('Ctrl Pts',(-19.8223796113184,-37.2337866764021,
121.938614397135)) ;
#76657=CARTESIAN_POINT('Ctrl Pts',(-19.7397550078523,-37.0537975959834,
122.233254223609)) ;
#76658=CARTESIAN_POINT('Ctrl Pts',(-19.2975051439778,-37.2536356449142,
121.885263707543)) ;
#76659=CARTESIAN_POINT('Ctrl Pts',(-19.3198535804931,-37.0736465644954,
122.190574646049)) ;
#76660=CARTESIAN_POINT('Ctrl Pts',(-18.7809853426803,-37.2736859472255,
122.016176078783)) ;
#76661=CARTESIAN_POINT('Ctrl Pts',(-18.9066385592989,-37.0936968668067,
122.295305374503)) ;
#76662=CARTESIAN_POINT('Ctrl Pts',(-18.3447935795222,-37.2935208696567,
122.312469305254)) ;
#76663=CARTESIAN_POINT('Ctrl Pts',(-18.5576842939248,-37.113531789238,122.532341920129)) ;
#76664=CARTESIAN_POINT('Ctrl Pts',(-18.0337656488262,-37.3134512708826,
122.7410074397)) ;
#76665=CARTESIAN_POINT('Ctrl Pts',(-18.3088629320483,-37.1334621904638,
122.875174080636)) ;
#76666=CARTESIAN_POINT('Ctrl Pts',(-17.8872187177166,-37.3333362162414,
123.249003693798)) ;
#76667=CARTESIAN_POINT('Ctrl Pts',(-18.1916271520052,-37.1533471358227,
123.28157263407)) ;
#76668=CARTESIAN_POINT('Ctrl Pts',(-17.9240043990121,-37.3534088243928,
123.781130410534)) ;
#76669=CARTESIAN_POINT('Ctrl Pts',(-18.2210576286058,-37.1734197439741,
123.707273187308)) ;
#76670=CARTESIAN_POINT('Ctrl Pts',(-18.1371306277128,-37.373200140721,124.262126611291)) ;
#76671=CARTESIAN_POINT('Ctrl Pts',(-18.3915613312149,-37.1932110603022,
124.092070982679)) ;
#76672=CARTESIAN_POINT('Ctrl Pts',(-18.5035285318235,-37.3931649304882,
124.64589122131)) ;
#76673=CARTESIAN_POINT('Ctrl Pts',(-18.6846818764584,-37.2131758500695,
124.399080894642)) ;
#76674=CARTESIAN_POINT('Ctrl Pts',(-18.9799605391563,-37.4131478862385,
124.880632850291)) ;
#76675=CARTESIAN_POINT('Ctrl Pts',(-19.0658287233952,-37.2331588058198,
124.586871974143)) ;
#76676=CARTESIAN_POINT('Ctrl Pts',(-19.5032077670225,-37.4329564082147,
124.939278140905)) ;
#76677=CARTESIAN_POINT('Ctrl Pts',(-19.4844282141108,-37.2529673277959,
124.633785395356)) ;
#76678=CARTESIAN_POINT('Ctrl Pts',(-20.0196196743258,-37.4529419829505,
124.815366561312)) ;
#76679=CARTESIAN_POINT('Ctrl Pts',(-19.8975570540621,-37.2729529025317,
124.534652928844)) ;
#76680=CARTESIAN_POINT('Ctrl Pts',(-20.4606042547495,-37.4728246230189,
124.523953283935)) ;
#76681=CARTESIAN_POINT('Ctrl Pts',(-20.2503434533714,-37.2928355426001,
124.301519156789)) ;
#76682=CARTESIAN_POINT('Ctrl Pts',(-20.7770251298041,-37.4927799351508,
124.098432867977)) ;
#76683=CARTESIAN_POINT('Ctrl Pts',(-20.5034774694716,-37.312790854732,123.961100528127)) ;
#76684=CARTESIAN_POINT('Ctrl Pts',(-20.9290068708971,-37.5126542917586,
123.592447664155)) ;
#76685=CARTESIAN_POINT('Ctrl Pts',(-20.6250594668182,-37.3326652113398,
123.556310724529)) ;
#76686=CARTESIAN_POINT('Ctrl Pts',(-20.899389956278,-37.5326364986196,123.062239130192)) ;
#76687=CARTESIAN_POINT('Ctrl Pts',(-20.6013622688047,-37.3526474182009,
123.132144083971)) ;
#76688=CARTESIAN_POINT('Ctrl Pts',(-20.6908254811286,-37.5525675765696,
122.575167631193)) ;
#76689=CARTESIAN_POINT('Ctrl Pts',(-20.4345064463008,-37.3725784961509,
122.742488126059)) ;
#76690=CARTESIAN_POINT('Ctrl Pts',(-20.3288457045905,-37.5724945514246,
122.18869479083)) ;
#76691=CARTESIAN_POINT('Ctrl Pts',(-20.1449218052122,-37.3925054710058,
122.433312456316)) ;
#76692=CARTESIAN_POINT('Ctrl Pts',(-19.8592684233699,-37.5923270103735,
121.949075641599)) ;
#76693=CARTESIAN_POINT('Ctrl Pts',(-19.7692491705873,-37.4123379299547,
122.241620182198)) ;
#76694=CARTESIAN_POINT('Ctrl Pts',(-19.420065800467,-37.6089846945487,121.894159881115)) ;
#76695=CARTESIAN_POINT('Ctrl Pts',(-19.4179129229134,-37.4289956141299,
122.197692407191)) ;
#76696=CARTESIAN_POINT('Ctrl Pts',(-19.0750788995426,-37.6222339184558,
121.941806794285)) ;
#76697=CARTESIAN_POINT('Ctrl Pts',(-19.1418999521506,-37.442244838037,122.235812007745)) ;
#76698=CARTESIAN_POINT('Ctrl Pts',(-18.8237258576815,-37.632282939907,122.022687580648)) ;
#76699=CARTESIAN_POINT('Ctrl Pts',(-18.9408249160599,-37.4522938594882,
122.300516750014)) ;
#76700=CARTESIAN_POINT('Ctrl Pts',(-18.5945663208292,-37.6421429481375,
122.14362057706)) ;
#76701=CARTESIAN_POINT('Ctrl Pts',(-18.7574893710446,-37.4621538677187,
122.397273180662)) ;
#76702=CARTESIAN_POINT('Ctrl Pts',(-18.3180876793282,-37.6554264613621,
122.356789242103)) ;
#76703=CARTESIAN_POINT('Ctrl Pts',(-18.5363454539202,-37.4754373809433,
122.567770274827)) ;
#76704=CARTESIAN_POINT('Ctrl Pts',(-18.0500066418884,-37.6720723803629,
122.708670183385)) ;
#76705=CARTESIAN_POINT('Ctrl Pts',(-18.3218393587194,-37.4920832999442,
122.849331203031)) ;
#76706=CARTESIAN_POINT('Ctrl Pts',(-17.9182173115326,-37.688626358179,123.128486091683)) ;
#76707=CARTESIAN_POINT('Ctrl Pts',(-18.2164325852077,-37.5086372777602,
123.185138398988)) ;
#76708=CARTESIAN_POINT('Ctrl Pts',(-17.9032980830167,-37.7019860871506,
123.479244069039)) ;
#76709=CARTESIAN_POINT('Ctrl Pts',(-18.2044905709866,-37.5219970067318,
123.465776425923)) ;
#76710=CARTESIAN_POINT('Ctrl Pts',(-17.9373186786892,-37.7118791389473,
123.737005381488)) ;
#76711=CARTESIAN_POINT('Ctrl Pts',(-18.2317111977967,-37.5318900585285,
123.671978909914)) ;
#76712=CARTESIAN_POINT('Ctrl Pts',(-18.015993501647,-37.7218691042283,123.98743356221)) ;
#76713=CARTESIAN_POINT('Ctrl Pts',(-18.2946526703774,-37.5418800238096,
123.872322439341)) ;
#76714=CARTESIAN_POINT('Ctrl Pts',(-18.1363891804097,-37.7318209850891,
124.219643590522)) ;
#76715=CARTESIAN_POINT('Ctrl Pts',(-18.3909713400926,-37.5518319046704,
124.058088956669)) ;
#76716=CARTESIAN_POINT('Ctrl Pts',(-18.2969510924276,-37.741869336781,124.429245026143)) ;
#76717=CARTESIAN_POINT('Ctrl Pts',(-18.5194225674474,-37.5618802563622,
124.225768799345)) ;
#76718=CARTESIAN_POINT('Ctrl Pts',(-18.4872912315673,-37.7517106208872,
124.604366917824)) ;
#76719=CARTESIAN_POINT('Ctrl Pts',(-18.6716962379228,-37.5717215404684,
124.365864646808)) ;
#76720=CARTESIAN_POINT('Ctrl Pts',(-18.7080075971964,-37.7616973240128,
124.74626444655)) ;
#76721=CARTESIAN_POINT('Ctrl Pts',(-18.848270497138,-37.5817082435941,124.479380739021)) ;
#76722=CARTESIAN_POINT('Ctrl Pts',(-18.948783824352,-37.7716323528303,124.847344520093)) ;
#76723=CARTESIAN_POINT('Ctrl Pts',(-19.0408922983168,-37.5916432724115,
124.560242693313)) ;
#76724=CARTESIAN_POINT('Ctrl Pts',(-19.2065084133327,-37.7816881477372,
124.905549326616)) ;
#76725=CARTESIAN_POINT('Ctrl Pts',(-19.2470724255386,-37.6016990673184,
124.606804323034)) ;
#76726=CARTESIAN_POINT('Ctrl Pts',(-19.4645118314046,-37.7915165110265,
124.918239663675)) ;
#76727=CARTESIAN_POINT('Ctrl Pts',(-19.4534751612069,-37.6115274306077,
124.61695433475)) ;
#76728=CARTESIAN_POINT('Ctrl Pts',(-19.7268395348962,-37.8015774809244,
124.885556198789)) ;
#76729=CARTESIAN_POINT('Ctrl Pts',(-19.6633370066296,-37.6215884005056,
124.590805332165)) ;
#76730=CARTESIAN_POINT('Ctrl Pts',(-19.9758209773242,-37.8114917598142,
124.808729302342)) ;
#76731=CARTESIAN_POINT('Ctrl Pts',(-19.8625213953459,-37.6315026793954,
124.529341692583)) ;
#76732=CARTESIAN_POINT('Ctrl Pts',(-20.2101091149036,-37.8215007542824,
124.689174409391)) ;
#76733=CARTESIAN_POINT('Ctrl Pts',(-20.0499508319165,-37.6415116738637,
124.433695808887)) ;
#76734=CARTESIAN_POINT('Ctrl Pts',(-20.4201860705366,-37.8315305888462,
124.529999912154)) ;
#76735=CARTESIAN_POINT('Ctrl Pts',(-20.2180110082682,-37.6515415084274,
124.306354429914)) ;
#76736=CARTESIAN_POINT('Ctrl Pts',(-20.5967424361067,-37.8413888189184,
124.340392518971)) ;
#76737=CARTESIAN_POINT('Ctrl Pts',(-20.3592543312716,-37.6613997384997,
124.154667125539)) ;
#76738=CARTESIAN_POINT('Ctrl Pts',(-20.7399359738855,-37.8513875246608,
124.120135025767)) ;
#76739=CARTESIAN_POINT('Ctrl Pts',(-20.4738072491821,-37.6713984442421,
123.978459973914)) ;
#76740=CARTESIAN_POINT('Ctrl Pts',(-20.8419611024385,-37.8612821805796,
123.880914135992)) ;
#76741=CARTESIAN_POINT('Ctrl Pts',(-20.5554252348265,-37.6812931001609,
123.787082588274)) ;
#76742=CARTESIAN_POINT('Ctrl Pts',(-20.9018013799904,-37.8713452449635,
123.623373162073)) ;
#76743=CARTESIAN_POINT('Ctrl Pts',(-20.603295299142,-37.6913561645448,123.581049278094)) ;
#76744=CARTESIAN_POINT('Ctrl Pts',(-20.9159903078622,-37.8811849032434,
123.365144028712)) ;
#76745=CARTESIAN_POINT('Ctrl Pts',(-20.6146442263728,-37.7011958228247,
123.374466181267)) ;
#76746=CARTESIAN_POINT('Ctrl Pts',(-20.8847687943629,-37.8912480703253,
123.102580743035)) ;
#76747=CARTESIAN_POINT('Ctrl Pts',(-20.589664844702,-37.7112589899066,123.16441577383)) ;
#76748=CARTESIAN_POINT('Ctrl Pts',(-20.809484036213,-37.9011423154524,122.853677895853)) ;
#76749=CARTESIAN_POINT('Ctrl Pts',(-20.5294350133251,-37.7211532350337,
122.965294385449)) ;
#76750=CARTESIAN_POINT('Ctrl Pts',(-20.6922226402959,-37.911084137057,122.620247034539)) ;
#76751=CARTESIAN_POINT('Ctrl Pts',(-20.4356240768759,-37.7310950566383,
122.778550847944)) ;
#76752=CARTESIAN_POINT('Ctrl Pts',(-20.5352958891587,-37.9210866679751,
122.409330679818)) ;
#76753=CARTESIAN_POINT('Ctrl Pts',(-20.3100810068094,-37.7410975875563,
122.60981908937)) ;
#76754=CARTESIAN_POINT('Ctrl Pts',(-20.3432724836096,-37.9311212944326,
122.228617908645)) ;
#76755=CARTESIAN_POINT('Ctrl Pts',(-20.1564607864245,-37.7511322140138,
122.465250443075)) ;
#76756=CARTESIAN_POINT('Ctrl Pts',(-20.1271504516015,-37.940966829419,122.086359667604)) ;
#76757=CARTESIAN_POINT('Ctrl Pts',(-19.9835623661803,-37.7609777490003,
122.351445878483)) ;
#76758=CARTESIAN_POINT('Ctrl Pts',(-19.8865382084238,-37.950950254258,121.981841696319)) ;
#76759=CARTESIAN_POINT('Ctrl Pts',(-19.7910718730727,-37.7709611738393,
122.267833461775)) ;
#76760=CARTESIAN_POINT('Ctrl Pts',(-19.632237024873,-37.9609006446231,121.920936388856)) ;
#76761=CARTESIAN_POINT('Ctrl Pts',(-19.5876306530056,-37.7809115642044,
122.219111287148)) ;
#76762=CARTESIAN_POINT('Ctrl Pts',(-19.3699906918053,-37.9708982849202,
121.904681189233)) ;
#76763=CARTESIAN_POINT('Ctrl Pts',(-19.3778335442572,-37.7909092045014,
122.206109169459)) ;
#76764=CARTESIAN_POINT('Ctrl Pts',(-19.1079206636086,-37.9809373654834,
121.934852971081)) ;
#76765=CARTESIAN_POINT('Ctrl Pts',(-19.1681777138388,-37.8009482850646,
122.230248687512)) ;
#76766=CARTESIAN_POINT('Ctrl Pts',(-18.860240682619,-37.9907635162525,122.007929238494)) ;
#76767=CARTESIAN_POINT('Ctrl Pts',(-18.9700348973941,-37.8107744358337,
122.288711477367)) ;
#76768=CARTESIAN_POINT('Ctrl Pts',(-18.6234287246879,-38.0008200911816,
122.125206427467)) ;
#76769=CARTESIAN_POINT('Ctrl Pts',(-18.7805861344579,-37.8208310107629,
122.382535045153)) ;
#76770=CARTESIAN_POINT('Ctrl Pts',(-18.4132844278419,-38.0107606305619,
122.280394942206)) ;
#76771=CARTESIAN_POINT('Ctrl Pts',(-18.6124721241605,-37.8307715501431,
122.506687339545)) ;
#76772=CARTESIAN_POINT('Ctrl Pts',(-18.2333456790557,-38.0206650235383,
122.46846128284)) ;
#76773=CARTESIAN_POINT('Ctrl Pts',(-18.4685228183294,-37.8406759431195,
122.657141441045)) ;
#76774=CARTESIAN_POINT('Ctrl Pts',(-18.0868734495751,-38.0307116777432,
122.688093340425)) ;
#76775=CARTESIAN_POINT('Ctrl Pts',(-18.3513466170776,-37.8507225973244,
122.832848242214)) ;
#76776=CARTESIAN_POINT('Ctrl Pts',(-17.9821139834346,-38.0406072396816,
122.926149688443)) ;
#76777=CARTESIAN_POINT('Ctrl Pts',(-18.2675409920432,-37.8606181592628,
123.023293667874)) ;
#76778=CARTESIAN_POINT('Ctrl Pts',(-17.9192592235036,-38.0506693175272,
123.182952338483)) ;
#76779=CARTESIAN_POINT('Ctrl Pts',(-18.2172590200462,-37.8706802371084,
123.228736387907)) ;
#76780=CARTESIAN_POINT('Ctrl Pts',(-17.9021734627855,-38.0605120159409,
123.441072933948)) ;
#76781=CARTESIAN_POINT('Ctrl Pts',(-18.2035923555535,-37.8805229355222,
123.43523229754)) ;
#76782=CARTESIAN_POINT('Ctrl Pts',(-17.929962860664,-38.0705027909024,123.702111270604)) ;
#76783=CARTESIAN_POINT('Ctrl Pts',(-18.2258256600623,-37.8905137104836,
123.644062635813)) ;
#76784=CARTESIAN_POINT('Ctrl Pts',(-18.002248222922,-38.0804306559215,123.952806457273)) ;
#76785=CARTESIAN_POINT('Ctrl Pts',(-18.2836555848188,-37.9004415755027,
123.844617906558)) ;
#76786=CARTESIAN_POINT('Ctrl Pts',(-18.1172694269182,-38.0904194006877,
124.188763665536)) ;
#76787=CARTESIAN_POINT('Ctrl Pts',(-18.3756740525521,-37.9104303202689,
124.033382779807)) ;
#76788=CARTESIAN_POINT('Ctrl Pts',(-18.2725063779135,-38.1004521862746,
124.401872836947)) ;
#76789=CARTESIAN_POINT('Ctrl Pts',(-18.4998651103405,-37.9204631058559,
124.203869099965)) ;
#76790=CARTESIAN_POINT('Ctrl Pts',(-18.4590525160072,-38.1103188708953,
124.581942987187)) ;
#76791=CARTESIAN_POINT('Ctrl Pts',(-18.6491027477406,-37.9303297904765,
124.347923469176)) ;
#76792=CARTESIAN_POINT('Ctrl Pts',(-18.6756943059333,-38.1202807630584,
124.728918023336)) ;
#76793=CARTESIAN_POINT('Ctrl Pts',(-18.8224168656527,-37.9402916826396,
124.46550199026)) ;
#76794=CARTESIAN_POINT('Ctrl Pts',(-18.9164378070636,-38.130314239971,124.836426983347)) ;
#76795=CARTESIAN_POINT('Ctrl Pts',(-19.0150124287312,-37.9503251595522,
124.551507627464)) ;
#76796=CARTESIAN_POINT('Ctrl Pts',(-19.1683321359597,-38.1401985812193,
124.899959302474)) ;
#76797=CARTESIAN_POINT('Ctrl Pts',(-19.2165276738214,-37.9602095008005,
124.602331745054)) ;
#76798=CARTESIAN_POINT('Ctrl Pts',(-19.4320465863461,-38.1502615233404,
124.919128358808)) ;
#76799=CARTESIAN_POINT('Ctrl Pts',(-19.4274995576439,-37.9702724429217,
124.617665373635)) ;
#76800=CARTESIAN_POINT('Ctrl Pts',(-19.6895940464607,-38.16011192496,124.89290473406)) ;
#76801=CARTESIAN_POINT('Ctrl Pts',(-19.6335365291386,-37.9801228445412,
124.596684955515)) ;
#76802=CARTESIAN_POINT('Ctrl Pts',(-19.9432929414495,-38.1701388137496,
124.821745925564)) ;
#76803=CARTESIAN_POINT('Ctrl Pts',(-19.8364952746785,-37.9901497333309,
124.539756471089)) ;
#76804=CARTESIAN_POINT('Ctrl Pts',(-20.1805416770185,-38.1801674287058,
124.706967424715)) ;
#76805=CARTESIAN_POINT('Ctrl Pts',(-20.0262936087495,-38.0001783482871,
124.447932190044)) ;
#76806=CARTESIAN_POINT('Ctrl Pts',(-20.3906137721402,-38.1900126518259,
124.555971632275)) ;
#76807=CARTESIAN_POINT('Ctrl Pts',(-20.1943496685895,-38.0100235714072,
124.327134842774)) ;
#76808=CARTESIAN_POINT('Ctrl Pts',(-20.5744646117543,-38.2000033356319,
124.368535624732)) ;
#76809=CARTESIAN_POINT('Ctrl Pts',(-20.3414292436618,-38.0200142552131,
124.177185180511)) ;
#76810=CARTESIAN_POINT('Ctrl Pts',(-20.7231886884151,-38.2100412177043,
124.150677424846)) ;
#76811=CARTESIAN_POINT('Ctrl Pts',(-20.4604073258307,-38.0300521372856,
124.002897686156)) ;
#76812=CARTESIAN_POINT('Ctrl Pts',(-20.8301490997781,-38.2198855773431,
123.915113415495)) ;
#76813=CARTESIAN_POINT('Ctrl Pts',(-20.5459739843948,-38.0398964969244,
123.814446751513)) ;
#76814=CARTESIAN_POINT('Ctrl Pts',(-20.8959919669497,-38.2298704479579,
123.661153850829)) ;
#76815=CARTESIAN_POINT('Ctrl Pts',(-20.5986469676164,-38.0498813675391,
123.611278966283)) ;
#76816=CARTESIAN_POINT('Ctrl Pts',(-20.9167692457474,-38.2398097312865,
123.400748772404)) ;
#76817=CARTESIAN_POINT('Ctrl Pts',(-20.6152674855689,-38.0598206508678,
123.402955237377)) ;
#76818=CARTESIAN_POINT('Ctrl Pts',(-20.8916876626832,-38.2498503406597,
123.138114322837)) ;
#76819=CARTESIAN_POINT('Ctrl Pts',(-20.5952009193857,-38.0698612602409,
123.192847680362)) ;
#76820=CARTESIAN_POINT('Ctrl Pts',(-20.8226462972461,-38.2597351915729,
122.887662089214)) ;
#76821=CARTESIAN_POINT('Ctrl Pts',(-20.5399668195097,-38.0797461111542,
122.992486951818)) ;
#76822=CARTESIAN_POINT('Ctrl Pts',(-20.7101619938538,-38.2697371477417,
122.650150261897)) ;
#76823=CARTESIAN_POINT('Ctrl Pts',(-20.44997835604,-38.089748067323,122.802478099931)) ;
#76824=CARTESIAN_POINT('Ctrl Pts',(-20.5595370995574,-38.2796557444622,
122.437376954918)) ;
#76825=CARTESIAN_POINT('Ctrl Pts',(-20.3294778457341,-38.0996666640434,
122.632260578575)) ;
#76826=CARTESIAN_POINT('Ctrl Pts',(-20.3718806510346,-38.289702566538,122.251710845109)) ;
#76827=CARTESIAN_POINT('Ctrl Pts',(-20.1793517557982,-38.1097134861192,
122.483728389381)) ;
#76828=CARTESIAN_POINT('Ctrl Pts',(-20.1586361997341,-38.2995768476507,
122.103781930012)) ;
#76829=CARTESIAN_POINT('Ctrl Pts',(-20.0087562603686,-38.1195877672319,
122.365386632677)) ;
#76830=CARTESIAN_POINT('Ctrl Pts',(-19.9188009996672,-38.3096310476953,
121.993039914005)) ;
#76831=CARTESIAN_POINT('Ctrl Pts',(-19.8168874663292,-38.1296419672765,
122.276793896463)) ;
#76832=CARTESIAN_POINT('Ctrl Pts',(-19.6673495935164,-38.3195264773305,
121.926560228982)) ;
#76833=CARTESIAN_POINT('Ctrl Pts',(-19.615726790868,-38.1395373969118,122.223611339034)) ;
#76834=CARTESIAN_POINT('Ctrl Pts',(-19.4039095755327,-38.3295881056479,
121.904328761381)) ;
#76835=CARTESIAN_POINT('Ctrl Pts',(-19.4049744286583,-38.1495990252291,
122.20582716044)) ;
#76836=CARTESIAN_POINT('Ctrl Pts',(-19.1462446839962,-38.3394327344778,
121.92763291997)) ;
#76837=CARTESIAN_POINT('Ctrl Pts',(-19.1988436604768,-38.159443654059,122.224471403124)) ;
#76838=CARTESIAN_POINT('Ctrl Pts',(-18.8933810810539,-38.3493927820834,
121.995203018732)) ;
#76839=CARTESIAN_POINT('Ctrl Pts',(-18.9965533361364,-38.1694037016646,
122.278528153739)) ;
#76840=CARTESIAN_POINT('Ctrl Pts',(-18.6544538829117,-38.3594310882575,
122.106985936692)) ;
#76841=CARTESIAN_POINT('Ctrl Pts',(-18.8054118480748,-38.1794420078387,
122.367955372878)) ;
#76842=CARTESIAN_POINT('Ctrl Pts',(-18.4417836192416,-38.3693043876901,
122.255686315655)) ;
#76843=CARTESIAN_POINT('Ctrl Pts',(-18.6352768308471,-38.1893153072714,
122.486915811868)) ;
#76844=CARTESIAN_POINT('Ctrl Pts',(-18.2545726342933,-38.3793776492764,
122.442761738828)) ;
#76845=CARTESIAN_POINT('Ctrl Pts',(-18.4855083791044,-38.1993885688576,
122.636576970832)) ;
#76846=CARTESIAN_POINT('Ctrl Pts',(-18.1061577775642,-38.3891978752331,
122.653952115977)) ;
#76847=CARTESIAN_POINT('Ctrl Pts',(-18.3667778089366,-38.2092087948143,
122.805528675082)) ;
#76848=CARTESIAN_POINT('Ctrl Pts',(-17.9936243509506,-38.3992769391726,
122.89364946878)) ;
#76849=CARTESIAN_POINT('Ctrl Pts',(-18.2767515207265,-38.2192878587538,
122.997287189187)) ;
#76850=CARTESIAN_POINT('Ctrl Pts',(-17.9258375543996,-38.4091270291924,
123.143539427575)) ;
#76851=CARTESIAN_POINT('Ctrl Pts',(-18.2225229861537,-38.2291379487737,
123.197198298179)) ;
#76852=CARTESIAN_POINT('Ctrl Pts',(-17.901802683763,-38.4192057828062,123.40723841002)) ;
#76853=CARTESIAN_POINT('Ctrl Pts',(-18.2032956687307,-38.2392167023874,
123.408157924605)) ;
#76854=CARTESIAN_POINT('Ctrl Pts',(-17.9231669694518,-38.4290272500656,
123.664509279097)) ;
#76855=CARTESIAN_POINT('Ctrl Pts',(-18.2203875531494,-38.2490381696469,
123.613973301711)) ;
#76856=CARTESIAN_POINT('Ctrl Pts',(-17.9900867206305,-38.4390928484233,
123.920355248503)) ;
#76857=CARTESIAN_POINT('Ctrl Pts',(-18.2739238795727,-38.2591037680045,
123.818650252036)) ;
#76858=CARTESIAN_POINT('Ctrl Pts',(-18.0987428643618,-38.448995504198,124.156888509118)) ;
#76859=CARTESIAN_POINT('Ctrl Pts',(-18.3608489306835,-38.2690064237792,
124.007875995514)) ;
#76860=CARTESIAN_POINT('Ctrl Pts',(-18.2488988280731,-38.4590463300276,
124.374113939664)) ;
#76861=CARTESIAN_POINT('Ctrl Pts',(-18.4809742059933,-38.2790572496089,
124.181656254911)) ;
#76862=CARTESIAN_POINT('Ctrl Pts',(-18.4311282812426,-38.4689205343665,
124.558922029274)) ;
#76863=CARTESIAN_POINT('Ctrl Pts',(-18.6267574017553,-38.2889314539477,
124.329501781547)) ;
#76864=CARTESIAN_POINT('Ctrl Pts',(-18.6468226000267,-38.4789929844056,
124.712247945109)) ;
#76865=CARTESIAN_POINT('Ctrl Pts',(-18.7993133663225,-38.2990039039868,
124.452162386081)) ;
#76866=CARTESIAN_POINT('Ctrl Pts',(-18.8800743167449,-38.4888220011791,
124.823318123701)) ;
#76867=CARTESIAN_POINT('Ctrl Pts',(-18.985913767497,-38.3088329207603,124.54101769674)) ;
#76868=CARTESIAN_POINT('Ctrl Pts',(-19.1349034186405,-38.4988888470939,
124.894192497896)) ;
#76869=CARTESIAN_POINT('Ctrl Pts',(-19.18977742163,-38.3188997666751,124.597717046058)) ;
#76870=CARTESIAN_POINT('Ctrl Pts',(-19.3936404772046,-38.5087790183957,
124.919135574691)) ;
#76871=CARTESIAN_POINT('Ctrl Pts',(-19.3967662609791,-38.3287899379769,
124.6176711408)) ;
#76872=CARTESIAN_POINT('Ctrl Pts',(-19.6554475745785,-38.5187712120195,
124.899143715497)) ;
#76873=CARTESIAN_POINT('Ctrl Pts',(-19.6062117573264,-38.3387821316008,
124.601677525334)) ;
#76874=CARTESIAN_POINT('Ctrl Pts',(-19.9090056650596,-38.5287340226429,
124.833945501383)) ;
#76875=CARTESIAN_POINT('Ctrl Pts',(-19.8090578249638,-38.3487449422242,
124.549518845411)) ;
#76876=CARTESIAN_POINT('Ctrl Pts',(-20.1462891749029,-38.5386382954864,
124.726937805289)) ;
#76877=CARTESIAN_POINT('Ctrl Pts',(-19.9988839326754,-38.3586492150676,
124.463912964312)) ;
#76878=CARTESIAN_POINT('Ctrl Pts',(-20.364605703527,-38.548698787291,124.577884540277)) ;
#76879=CARTESIAN_POINT('Ctrl Pts',(-20.173537335335,-38.3687097068723,124.344670113735)) ;
#76880=CARTESIAN_POINT('Ctrl Pts',(-20.5498721513318,-38.5585391189633,
124.397423633109)) ;
#76881=CARTESIAN_POINT('Ctrl Pts',(-20.3217496440126,-38.3785500385446,
124.200302203012)) ;
#76882=CARTESIAN_POINT('Ctrl Pts',(-20.7046268369188,-38.5686021650551,
124.183029887314)) ;
#76883=CARTESIAN_POINT('Ctrl Pts',(-20.4455536256558,-38.3886130846363,
124.028787005913)) ;
#76884=CARTESIAN_POINT('Ctrl Pts',(-20.8177037944646,-38.5784962207502,
123.948871113665)) ;
#76885=CARTESIAN_POINT('Ctrl Pts',(-20.5360148493182,-38.3985071403314,
123.841460727974)) ;
#76886=CARTESIAN_POINT('Ctrl Pts',(-20.889425745964,-38.5884389210731,123.697654055554)) ;
#76887=CARTESIAN_POINT('Ctrl Pts',(-20.5933924604119,-38.4084498406544,
123.640487633951)) ;
#76888=CARTESIAN_POINT('Ctrl Pts',(-20.916667441635,-38.5984446620007,123.436101061358)) ;
#76889=CARTESIAN_POINT('Ctrl Pts',(-20.6151860207473,-38.418455581582,123.431245328084)) ;
#76890=CARTESIAN_POINT('Ctrl Pts',(-20.8977588228678,-38.6084655725163,
123.173448091047)) ;
#76891=CARTESIAN_POINT('Ctrl Pts',(-20.6000592553857,-38.4284764920975,
123.221122910589)) ;
#76892=CARTESIAN_POINT('Ctrl Pts',(-20.8346540511211,-38.6183563079662,
122.921298084091)) ;
#76893=CARTESIAN_POINT('Ctrl Pts',(-20.5495758458622,-38.4383672275475,
123.019403663293)) ;
#76894=CARTESIAN_POINT('Ctrl Pts',(-20.7280091757343,-38.6283478486951,
122.681375284334)) ;
#76895=CARTESIAN_POINT('Ctrl Pts',(-20.4642602954684,-38.4483587682763,
122.827465455942)) ;
#76896=CARTESIAN_POINT('Ctrl Pts',(-20.5819003599623,-38.6382957091167,
122.464600481012)) ;
#76897=CARTESIAN_POINT('Ctrl Pts',(-20.3473737456245,-38.458306628698,122.654045845982)) ;
#76898=CARTESIAN_POINT('Ctrl Pts',(-20.4007533562196,-38.6482423783031,
122.276140396781)) ;
#76899=CARTESIAN_POINT('Ctrl Pts',(-20.2024567640308,-38.4682532978843,
122.503277819394)) ;
#76900=CARTESIAN_POINT('Ctrl Pts',(-20.1873323482712,-38.6582904544387,
122.12067245953)) ;
#76901=CARTESIAN_POINT('Ctrl Pts',(-20.0317199988072,-38.4783013740199,
122.378903072768)) ;
#76902=CARTESIAN_POINT('Ctrl Pts',(-19.954975200177,-38.6681380524443,122.006738756119)) ;
#76903=CARTESIAN_POINT('Ctrl Pts',(-19.8458354617128,-38.4881489720256,
122.287756243606)) ;
#76904=CARTESIAN_POINT('Ctrl Pts',(-19.7037273294392,-38.6780997755288,
121.933263220615)) ;
#76905=CARTESIAN_POINT('Ctrl Pts',(-19.6448376844739,-38.49811069511,122.228975335749)) ;
#76906=CARTESIAN_POINT('Ctrl Pts',(-19.4417254602115,-38.6881284106118,
121.904664952623)) ;
#76907=CARTESIAN_POINT('Ctrl Pts',(-19.435236168815,-38.508139330193,122.206096194811)) ;
#76908=CARTESIAN_POINT('Ctrl Pts',(-19.1818626712989,-38.6980387189298,
121.921702009189)) ;
#76909=CARTESIAN_POINT('Ctrl Pts',(-19.2273466015253,-38.5180496385111,
122.219725252916)) ;
#76910=CARTESIAN_POINT('Ctrl Pts',(-18.9280968781733,-38.7079736160657,
121.983094997381)) ;
#76911=CARTESIAN_POINT('Ctrl Pts',(-19.0243343132026,-38.5279845356469,
122.268838827757)) ;
#76912=CARTESIAN_POINT('Ctrl Pts',(-18.6864010148736,-38.7180146990083,
122.088952068189)) ;
#76913=CARTESIAN_POINT('Ctrl Pts',(-18.830977224545,-38.5380256185895,122.353523948551)) ;
#76914=CARTESIAN_POINT('Ctrl Pts',(-18.470002959374,-38.7279020418365,122.232792348732)) ;
#76915=CARTESIAN_POINT('Ctrl Pts',(-18.6578590879055,-38.5479129614178,
122.468595134658)) ;
#76916=CARTESIAN_POINT('Ctrl Pts',(-18.2795943517483,-38.7378935567758,
122.413563464175)) ;
#76917=CARTESIAN_POINT('Ctrl Pts',(-18.5055317681181,-38.5579044763571,
122.613211332423)) ;
#76918=CARTESIAN_POINT('Ctrl Pts',(-18.1241690741951,-38.7478449479723,
122.623883939049)) ;
#76919=CARTESIAN_POINT('Ctrl Pts',(-18.3811911759621,-38.5678558675536,
122.781466905472)) ;
#76920=CARTESIAN_POINT('Ctrl Pts',(-18.0074429396935,-38.7577774813049,
122.857344924789)) ;
#76921=CARTESIAN_POINT('Ctrl Pts',(-18.2878097133205,-38.5777884008862,
122.968234824021)) ;
#76922=CARTESIAN_POINT('Ctrl Pts',(-17.9324451630924,-38.7677746392044,
123.109116894499)) ;
#76923=CARTESIAN_POINT('Ctrl Pts',(-18.2278106582551,-38.5877855587856,
123.1696520247)) ;
#76924=CARTESIAN_POINT('Ctrl Pts',(-17.9022350150064,-38.7777596493679,
123.369808873097)) ;
#76925=CARTESIAN_POINT('Ctrl Pts',(-18.2036416362819,-38.5977705689491,
123.378205317584)) ;
#76926=CARTESIAN_POINT('Ctrl Pts',(-17.9182204761014,-38.7878024759377,
123.633203162135)) ;
#76927=CARTESIAN_POINT('Ctrl Pts',(-18.2164291783058,-38.6078133955189,
123.588920944231)) ;
#76928=CARTESIAN_POINT('Ctrl Pts',(-17.9778363799748,-38.7976327102426,
123.884601181643)) ;
#76929=CARTESIAN_POINT('Ctrl Pts',(-18.2641206846296,-38.6176436298239,
123.790038464492)) ;
#76930=CARTESIAN_POINT('Ctrl Pts',(-18.0826097272587,-38.8077087354773,
124.12771836108)) ;
#76931=CARTESIAN_POINT('Ctrl Pts',(-18.3479385732616,-38.6277196550586,
123.984532923754)) ;
#76932=CARTESIAN_POINT('Ctrl Pts',(-18.2247229698765,-38.8175609719682,
124.344203206697)) ;
#76933=CARTESIAN_POINT('Ctrl Pts',(-18.4616277604428,-38.6375718915494,
124.157720543777)) ;
#76934=CARTESIAN_POINT('Ctrl Pts',(-18.4060166291927,-38.8276341784023,
124.537031920966)) ;
#76935=CARTESIAN_POINT('Ctrl Pts',(-18.6066621150346,-38.6476450979836,
124.311984493962)) ;
#76936=CARTESIAN_POINT('Ctrl Pts',(-18.6132523457623,-38.8374756879095,
124.691787453211)) ;
#76937=CARTESIAN_POINT('Ctrl Pts',(-18.7724492132766,-38.6574866074907,
124.435789153201)) ;
#76938=CARTESIAN_POINT('Ctrl Pts',(-18.8465449134699,-38.8474366346893,
124.810489310381)) ;
#76939=CARTESIAN_POINT('Ctrl Pts',(-18.9590823935704,-38.6674475542705,
124.530751641621)) ;
#76940=CARTESIAN_POINT('Ctrl Pts',(-19.098990635747,-38.8574744634893,124.886965770344)) ;
#76941=CARTESIAN_POINT('Ctrl Pts',(-19.1610387331382,-38.6774853830706,
124.591933962578)) ;
#76942=CARTESIAN_POINT('Ctrl Pts',(-19.3565960865139,-38.8673487732438,
124.918417832389)) ;
#76943=CARTESIAN_POINT('Ctrl Pts',(-19.3671221354591,-38.687359692825,124.617096782375)) ;
#76944=CARTESIAN_POINT('Ctrl Pts',(-19.6208093648921,-38.8774184709169,
124.904380279323)) ;
#76945=CARTESIAN_POINT('Ctrl Pts',(-19.5784931043603,-38.6974293904982,
124.605867998489)) ;
#76946=CARTESIAN_POINT('Ctrl Pts',(-19.8726090819025,-38.8872519422043,
124.84620010404)) ;
#76947=CARTESIAN_POINT('Ctrl Pts',(-19.779932174487,-38.7072628617856,124.559325358216)) ;
#76948=CARTESIAN_POINT('Ctrl Pts',(-20.1154997479341,-38.8972815887343,
124.743876964868)) ;
#76949=CARTESIAN_POINT('Ctrl Pts',(-19.9742453375795,-38.7172925083155,
124.477468165888)) ;
#76950=CARTESIAN_POINT('Ctrl Pts',(-20.3366133293016,-38.9073161030616,
124.60018424076)) ;
#76951=CARTESIAN_POINT('Ctrl Pts',(-20.1511369670628,-38.7273270226429,
124.362515034824)) ;
#76952=CARTESIAN_POINT('Ctrl Pts',(-20.5258195611414,-38.9171413885325,
124.424489905026)) ;
#76953=CARTESIAN_POINT('Ctrl Pts',(-20.3025021660536,-38.7371523081138,
124.221961312577)) ;
#76954=CARTESIAN_POINT('Ctrl Pts',(-20.6849082649732,-38.9271456300811,
124.215225042755)) ;
#76955=CARTESIAN_POINT('Ctrl Pts',(-20.4297743088031,-38.7471565496623,
124.054550406334)) ;
#76956=CARTESIAN_POINT('Ctrl Pts',(-20.8049240327782,-38.9371282751602,
123.98189798351)) ;
#76957=CARTESIAN_POINT('Ctrl Pts',(-20.5257881879668,-38.7571391947414,
123.867889603181)) ;
#76958=CARTESIAN_POINT('Ctrl Pts',(-20.8827806720489,-38.9471734722517,
123.729693087447)) ;
#76959=CARTESIAN_POINT('Ctrl Pts',(-20.5880749231069,-38.7671843918329,
123.666125997018)) ;
#76960=CARTESIAN_POINT('Ctrl Pts',(-20.9153734465156,-38.9569965880118,
123.473607472968)) ;
#76961=CARTESIAN_POINT('Ctrl Pts',(-20.6141505414293,-38.7770075075931,
123.461258688752)) ;
#76962=CARTESIAN_POINT('Ctrl Pts',(-20.9034051257654,-38.9670311998121,
123.210183840089)) ;
#76963=CARTESIAN_POINT('Ctrl Pts',(-20.6045775434522,-38.7870421193933,
123.250519622744)) ;
#76964=CARTESIAN_POINT('Ctrl Pts',(-20.845214157011,-38.9770562085853,122.953236014163)) ;
#76965=CARTESIAN_POINT('Ctrl Pts',(-20.5580262508377,-38.7970671281665,
123.044961006179)) ;
#76966=CARTESIAN_POINT('Ctrl Pts',(-20.7455751867444,-38.9869081334268,
122.714273478696)) ;
#76967=CARTESIAN_POINT('Ctrl Pts',(-20.4783168903162,-38.8069190530081,
122.853791094508)) ;
#76968=CARTESIAN_POINT('Ctrl Pts',(-20.6043472153065,-38.9968990717495,
122.492979055676)) ;
#76969=CARTESIAN_POINT('Ctrl Pts',(-20.3653360237467,-38.8169099913308,
122.676754754454)) ;
#76970=CARTESIAN_POINT('Ctrl Pts',(-20.4282184151708,-39.006817056896,122.300819554169)) ;
#76971=CARTESIAN_POINT('Ctrl Pts',(-20.2244345676972,-38.8268279764772,
122.523026321021)) ;
#76972=CARTESIAN_POINT('Ctrl Pts',(-20.2191839000124,-39.0168451577915,
122.140380206256)) ;
#76973=CARTESIAN_POINT('Ctrl Pts',(-20.0572079946836,-38.8368560773727,
122.394673443587)) ;
#76974=CARTESIAN_POINT('Ctrl Pts',(-19.988823563401,-39.026730398734,122.020299045281)) ;
#76975=CARTESIAN_POINT('Ctrl Pts',(-19.8729210602191,-38.8467413183153,
122.298607226252)) ;
#76976=CARTESIAN_POINT('Ctrl Pts',(-19.7387023265597,-39.0367195117007,
121.940602617632)) ;
#76977=CARTESIAN_POINT('Ctrl Pts',(-19.6728247564175,-38.8567304312819,
122.234848346961)) ;
#76978=CARTESIAN_POINT('Ctrl Pts',(-19.4771010747282,-39.0467615760415,
121.905935512444)) ;
#76979=CARTESIAN_POINT('Ctrl Pts',(-19.4635439135823,-38.8667724956227,
122.207112896485)) ;
#76980=CARTESIAN_POINT('Ctrl Pts',(-19.2190051557657,-39.056590777446,121.916489575478)) ;
#76981=CARTESIAN_POINT('Ctrl Pts',(-19.2570678745084,-38.8766016970272,
122.215554268652)) ;
#76982=CARTESIAN_POINT('Ctrl Pts',(-18.9620194272322,-39.0665976182042,
121.97212452845)) ;
#76983=CARTESIAN_POINT('Ctrl Pts',(-19.0514789416566,-38.8866085377854,
122.260060324957)) ;
#76984=CARTESIAN_POINT('Ctrl Pts',(-18.7190580246496,-39.0765851423961,
122.071516726023)) ;
#76985=CARTESIAN_POINT('Ctrl Pts',(-18.8571092146858,-38.8965960619773,
122.339572267112)) ;
#76986=CARTESIAN_POINT('Ctrl Pts',(-18.496263286166,-39.0866147882047,122.212294698835)) ;
#76987=CARTESIAN_POINT('Ctrl Pts',(-18.6788723982506,-38.9066257077859,
122.452193065279)) ;
#76988=CARTESIAN_POINT('Ctrl Pts',(-18.304074260206,-39.0964888189434,122.386670421032)) ;
#76989=CARTESIAN_POINT('Ctrl Pts',(-18.5251202815215,-38.9164997385247,
122.591691852851)) ;
#76990=CARTESIAN_POINT('Ctrl Pts',(-18.1428504126763,-39.1064881418075,
122.594116058551)) ;
#76991=CARTESIAN_POINT('Ctrl Pts',(-18.3961396994837,-38.9264990613888,
122.757647081838)) ;
#76992=CARTESIAN_POINT('Ctrl Pts',(-18.0209136490319,-39.1163989773831,
122.824305926525)) ;
#76993=CARTESIAN_POINT('Ctrl Pts',(-18.2985886964444,-38.9364098969644,
122.941797703191)) ;
#76994=CARTESIAN_POINT('Ctrl Pts',(-17.9397564184948,-39.1264532253572,
123.075703741541)) ;
#76995=CARTESIAN_POINT('Ctrl Pts',(-18.2336609864209,-38.9464641449384,
123.142915426417)) ;
#76996=CARTESIAN_POINT('Ctrl Pts',(-17.9038739772955,-39.1363119696199,
123.332330097257)) ;
#76997=CARTESIAN_POINT('Ctrl Pts',(-18.2049530965617,-38.9563228892011,
123.348215715669)) ;
#76998=CARTESIAN_POINT('Ctrl Pts',(-17.9131303555369,-39.1463800556929,
123.596708290319)) ;
#76999=CARTESIAN_POINT('Ctrl Pts',(-18.2123561545412,-38.9663909752741,
123.559718464088)) ;
#77000=CARTESIAN_POINT('Ctrl Pts',(-17.967021152229,-39.1562355388724,123.850053708691)) ;
#77001=CARTESIAN_POINT('Ctrl Pts',(-18.2554666875822,-38.9762464584537,
123.762394736116)) ;
#77002=CARTESIAN_POINT('Ctrl Pts',(-18.064713155992,-39.1662303846666,124.09385471535)) ;
#77003=CARTESIAN_POINT('Ctrl Pts',(-18.3336182833703,-38.9862413042478,
123.957436260119)) ;
#77004=CARTESIAN_POINT('Ctrl Pts',(-18.2042478280738,-39.1762616803291,
124.317515212266)) ;
#77005=CARTESIAN_POINT('Ctrl Pts',(-18.4452442635705,-38.9962725999104,
124.136365752348)) ;
#77006=CARTESIAN_POINT('Ctrl Pts',(-18.3772981541373,-39.186128223619,124.510610102703)) ;
#77007=CARTESIAN_POINT('Ctrl Pts',(-18.5836826763418,-39.0061391432003,
124.290842767909)) ;
#77008=CARTESIAN_POINT('Ctrl Pts',(-18.5834523133423,-39.1961156193824,
124.672993813523)) ;
#77009=CARTESIAN_POINT('Ctrl Pts',(-18.7486045943314,-39.0161265389636,
124.420751367233)) ;
#77010=CARTESIAN_POINT('Ctrl Pts',(-18.8136849280849,-39.2060606601123,
124.79674572474)) ;
#77011=CARTESIAN_POINT('Ctrl Pts',(-18.9327894986595,-39.0260715796936,
124.519754710555)) ;
#77012=CARTESIAN_POINT('Ctrl Pts',(-19.0643744384827,-39.2161051663291,
124.879300115925)) ;
#77013=CARTESIAN_POINT('Ctrl Pts',(-19.1333404484933,-39.0361160859103,
124.585800271082)) ;
#77014=CARTESIAN_POINT('Ctrl Pts',(-19.3209006976884,-39.2259686724664,
124.916631731258)) ;
#77015=CARTESIAN_POINT('Ctrl Pts',(-19.3385608066028,-39.0459795920477,
124.61566765999)) ;
#77016=CARTESIAN_POINT('Ctrl Pts',(-19.5833595972612,-39.2359615333025,
124.909220187244)) ;
#77017=CARTESIAN_POINT('Ctrl Pts',(-19.5485279119773,-39.0559724528837,
124.609740630112)) ;
#77018=CARTESIAN_POINT('Ctrl Pts',(-19.8389276222297,-39.2458877270214,
124.856807197051)) ;
#77019=CARTESIAN_POINT('Ctrl Pts',(-19.7529826014343,-39.0658986466027,
124.567812433635)) ;
#77020=CARTESIAN_POINT('Ctrl Pts',(-20.0837340012859,-39.255906653054,124.759990302434)) ;
#77021=CARTESIAN_POINT('Ctrl Pts',(-19.9488284801805,-39.0759175726352,
124.490360989848)) ;
#77022=CARTESIAN_POINT('Ctrl Pts',(-20.3058732170056,-39.2658216524216,
124.623740322537)) ;
#77023=CARTESIAN_POINT('Ctrl Pts',(-20.1265408661882,-39.0858325720028,
124.381362989768)) ;
#77024=CARTESIAN_POINT('Ctrl Pts',(-20.5036398439104,-39.2758764239789,
124.448561262055)) ;
#77025=CARTESIAN_POINT('Ctrl Pts',(-20.2847556360216,-39.0958873435601,
124.241221409002)) ;
#77026=CARTESIAN_POINT('Ctrl Pts',(-20.6649559414728,-39.2857353862764,
124.245785908709)) ;
#77027=CARTESIAN_POINT('Ctrl Pts',(-20.4138101229452,-39.1057463058577,
124.079002680325)) ;
#77028=CARTESIAN_POINT('Ctrl Pts',(-20.7907073338541,-39.2957296301143,
124.015257630053)) ;
#77029=CARTESIAN_POINT('Ctrl Pts',(-20.5144131818237,-39.1157405496955,
123.894581187682)) ;
#77030=CARTESIAN_POINT('Ctrl Pts',(-20.8740852787271,-39.3056548595385,
123.768075589562)) ;
#77031=CARTESIAN_POINT('Ctrl Pts',(-20.5811176317263,-39.1256657791198,
123.696836372389)) ;
#77032=CARTESIAN_POINT('Ctrl Pts',(-20.9136831802489,-39.31568282343,123.507578576394)) ;
#77033=CARTESIAN_POINT('Ctrl Pts',(-20.6127981700986,-39.1356937430112,
123.488439150127)) ;
#77034=CARTESIAN_POINT('Ctrl Pts',(-20.9078028794993,-39.3255690830604,
123.247805457991)) ;
#77035=CARTESIAN_POINT('Ctrl Pts',(-20.6080961812906,-39.1455800026416,
123.280620698185)) ;
#77036=CARTESIAN_POINT('Ctrl Pts',(-20.8563083056204,-39.3356008461382,
122.989304179188)) ;
#77037=CARTESIAN_POINT('Ctrl Pts',(-20.5669027458931,-39.1556117657195,
123.07381928786)) ;
#77038=CARTESIAN_POINT('Ctrl Pts',(-20.7623452755489,-39.3454824724324,
122.747171858477)) ;
#77039=CARTESIAN_POINT('Ctrl Pts',(-20.4917344390515,-39.1654933920136,
122.880112663831)) ;
#77040=CARTESIAN_POINT('Ctrl Pts',(-20.6254181999182,-39.3555442419185,
122.52102025999)) ;
#77041=CARTESIAN_POINT('Ctrl Pts',(-20.3821947440194,-39.1755551614998,
122.699190275451)) ;
#77042=CARTESIAN_POINT('Ctrl Pts',(-20.4548438165895,-39.365402109414,122.326007790047)) ;
#77043=CARTESIAN_POINT('Ctrl Pts',(-20.2457369371644,-39.1854130289952,
122.543178822639)) ;
#77044=CARTESIAN_POINT('Ctrl Pts',(-20.2506752049278,-39.3753937345313,
122.160957633264)) ;
#77045=CARTESIAN_POINT('Ctrl Pts',(-20.0824034879034,-39.1954046541126,
122.41113697398)) ;
#77046=CARTESIAN_POINT('Ctrl Pts',(-20.0221459359516,-39.3853305336396,
122.034581725448)) ;
#77047=CARTESIAN_POINT('Ctrl Pts',(-19.8995811564876,-39.2053414532208,
122.310034285515)) ;
#77048=CARTESIAN_POINT('Ctrl Pts',(-19.7739378812756,-39.3953213631969,
121.948989845714)) ;
#77049=CARTESIAN_POINT('Ctrl Pts',(-19.7010154745598,-39.2153322827782,
122.241558685224)) ;
#77050=CARTESIAN_POINT('Ctrl Pts',(-19.5137457792874,-39.4053445989101,
121.907963203236)) ;
#77051=CARTESIAN_POINT('Ctrl Pts',(-19.4928622206853,-39.2253555184914,
122.208735172086)) ;
#77052=CARTESIAN_POINT('Ctrl Pts',(-19.2537240353443,-39.4152409469393,
121.912457737663)) ;
#77053=CARTESIAN_POINT('Ctrl Pts',(-19.284844725392,-39.2352518665205,122.212328561207)) ;
#77054=CARTESIAN_POINT('Ctrl Pts',(-18.9959028450321,-39.4252305094418,
121.961952758508)) ;
#77055=CARTESIAN_POINT('Ctrl Pts',(-19.0785873514741,-39.245241429023,122.251922433717)) ;
#77056=CARTESIAN_POINT('Ctrl Pts',(-18.7495601440392,-39.4352708171263,
122.056425100512)) ;
#77057=CARTESIAN_POINT('Ctrl Pts',(-18.8815126089877,-39.2552817367076,
122.327498082193)) ;
#77058=CARTESIAN_POINT('Ctrl Pts',(-18.5275396488287,-39.4451131204735,
122.189149904803)) ;
#77059=CARTESIAN_POINT('Ctrl Pts',(-18.7038944864329,-39.2651240400548,
122.433676503167)) ;
#77060=CARTESIAN_POINT('Ctrl Pts',(-18.3281491908291,-39.4551368287526,
122.361220908114)) ;
#77061=CARTESIAN_POINT('Ctrl Pts',(-18.544382291125,-39.2751477483338,122.571330259957)) ;
#77062=CARTESIAN_POINT('Ctrl Pts',(-18.1083641387951,-39.4683590062203,
122.63041569829)) ;
#77063=CARTESIAN_POINT('Ctrl Pts',(-18.3685442466138,-39.2883699258015,
122.786691064912)) ;
#77064=CARTESIAN_POINT('Ctrl Pts',(-17.962805114068,-39.4816515912796,122.952220149213)) ;
#77065=CARTESIAN_POINT('Ctrl Pts',(-18.2520900201739,-39.3016625108608,
123.0441667538)) ;
#77066=CARTESIAN_POINT('Ctrl Pts',(-17.9061735339547,-39.4949364472012,
123.296785705765)) ;
#77067=CARTESIAN_POINT('Ctrl Pts',(-18.2067947639732,-39.3149473667824,
123.319772623799)) ;
#77068=CARTESIAN_POINT('Ctrl Pts',(-17.9090249686714,-39.504908674374,123.558791097665)) ;
#77069=CARTESIAN_POINT('Ctrl Pts',(-18.2090712941876,-39.3249195939552,
123.529386330433)) ;
#77070=CARTESIAN_POINT('Ctrl Pts',(-17.9565864888428,-39.514817290813,123.814831513886)) ;
#77071=CARTESIAN_POINT('Ctrl Pts',(-18.2471189493616,-39.3348282103942,
123.734216637461)) ;
#77072=CARTESIAN_POINT('Ctrl Pts',(-18.0492936761103,-39.5248704961967,
124.062190998766)) ;
#77073=CARTESIAN_POINT('Ctrl Pts',(-18.321283555231,-39.3448814157779,123.93210607372)) ;
#77074=CARTESIAN_POINT('Ctrl Pts',(-18.1809125137279,-39.5347356299569,
124.285566479039)) ;
#77075=CARTESIAN_POINT('Ctrl Pts',(-18.4265731937417,-39.3547465495382,
124.110805222555)) ;
#77076=CARTESIAN_POINT('Ctrl Pts',(-18.4080910891847,-39.5480746875833,
124.552496993398)) ;
#77077=CARTESIAN_POINT('Ctrl Pts',(-18.6083336756882,-39.3680856071645,
124.324363766932)) ;
#77078=CARTESIAN_POINT('Ctrl Pts',(-18.7706176278764,-39.5646438749164,
124.802631869013)) ;
#77079=CARTESIAN_POINT('Ctrl Pts',(-18.8983168389849,-39.3846547944977,
124.524458515266)) ;
#77080=CARTESIAN_POINT('Ctrl Pts',(-19.1984775012454,-39.5812890147675,
124.914837427725)) ;
#77081=CARTESIAN_POINT('Ctrl Pts',(-19.2406669700555,-39.4012999343487,
124.614238150144)) ;
#77082=CARTESIAN_POINT('Ctrl Pts',(-19.5473160626192,-39.5945613172409,
124.91294505077)) ;
#77083=CARTESIAN_POINT('Ctrl Pts',(-19.5196867817272,-39.4145722368221,
124.6127192198)) ;
#77084=CARTESIAN_POINT('Ctrl Pts',(-19.8054003622154,-39.6045422806885,
124.866324423739)) ;
#77085=CARTESIAN_POINT('Ctrl Pts',(-19.7261653890183,-39.4245532002698,
124.575425593905)) ;
#77086=CARTESIAN_POINT('Ctrl Pts',(-20.0506098850286,-39.6144841127578,
124.776085831138)) ;
#77087=CARTESIAN_POINT('Ctrl Pts',(-19.9223292887017,-39.4344950323391,
124.503237755022)) ;
#77088=CARTESIAN_POINT('Ctrl Pts',(-20.3531494019728,-39.6278036819732,
124.600140542003)) ;
#77089=CARTESIAN_POINT('Ctrl Pts',(-20.1643723390079,-39.4478146015545,
124.362474577121)) ;
#77090=CARTESIAN_POINT('Ctrl Pts',(-20.6634916789112,-39.644333836906,124.28900205581)) ;
#77091=CARTESIAN_POINT('Ctrl Pts',(-20.4126378083465,-39.4643447564872,
124.11357553459)) ;
#77092=CARTESIAN_POINT('Ctrl Pts',(-20.8878880489204,-39.6643555623981,
123.806632140315)) ;
#77093=CARTESIAN_POINT('Ctrl Pts',(-20.5921614310952,-39.4843664819793,
123.727677884978)) ;
#77094=CARTESIAN_POINT('Ctrl Pts',(-20.9340458411947,-39.6841669590049,
123.281975948013)) ;
#77095=CARTESIAN_POINT('Ctrl Pts',(-20.6290900257531,-39.5041778785861,
123.307952866676)) ;
#77096=CARTESIAN_POINT('Ctrl Pts',(-20.7981256341411,-39.7041522077137,
122.768612564894)) ;
#77097=CARTESIAN_POINT('Ctrl Pts',(-20.5203568572082,-39.524163127295,122.897261068082)) ;
#77098=CARTESIAN_POINT('Ctrl Pts',(-20.4961474223464,-39.7240462703497,
122.334473379735)) ;
#77099=CARTESIAN_POINT('Ctrl Pts',(-20.2787761236903,-39.5440571899309,
122.549947532651)) ;
#77100=CARTESIAN_POINT('Ctrl Pts',(-20.0638627447035,-39.7439779495233,
122.028277249688)) ;
#77101=CARTESIAN_POINT('Ctrl Pts',(-19.9329493834132,-39.5639888691045,
122.304988270493)) ;
#77102=CARTESIAN_POINT('Ctrl Pts',(-19.5521053130839,-39.7639420039953,
121.888081012809)) ;
#77103=CARTESIAN_POINT('Ctrl Pts',(-19.523543821286,-39.5839529235765,122.192828836387)) ;
#77104=CARTESIAN_POINT('Ctrl Pts',(-19.0253744539785,-39.7838229057582,
121.930361827019)) ;
#77105=CARTESIAN_POINT('Ctrl Pts',(-19.1021578729861,-39.6038338253394,
122.226651390255)) ;
#77106=CARTESIAN_POINT('Ctrl Pts',(-18.5431348409181,-39.8037615673665,
122.150015941266)) ;
#77107=CARTESIAN_POINT('Ctrl Pts',(-18.7163648705892,-39.6237724869478,
122.402373239355)) ;
#77108=CARTESIAN_POINT('Ctrl Pts',(-18.1655278032644,-39.8236580926219,
122.520218221283)) ;
#77109=CARTESIAN_POINT('Ctrl Pts',(-18.4142773121928,-39.6436690122031,
122.698534606389)) ;
#77110=CARTESIAN_POINT('Ctrl Pts',(-17.9361396476805,-39.8435531310762,
122.996669054424)) ;
#77111=CARTESIAN_POINT('Ctrl Pts',(-18.2307652509137,-39.6635640506575,
123.079695848156)) ;
#77112=CARTESIAN_POINT('Ctrl Pts',(-17.8830061324122,-39.8635169543823,
123.524568225154)) ;
#77113=CARTESIAN_POINT('Ctrl Pts',(-18.1882574093228,-39.6835278739635,
123.502015493419)) ;
#77114=CARTESIAN_POINT('Ctrl Pts',(-18.012259531642,-39.8833910785114,124.036771136657)) ;
#77115=CARTESIAN_POINT('Ctrl Pts',(-18.2916598855057,-39.7034019980926,
123.911779438151)) ;
#77116=CARTESIAN_POINT('Ctrl Pts',(-18.309630845073,-39.9033661542386,124.476606505104)) ;
#77117=CARTESIAN_POINT('Ctrl Pts',(-18.5295569287949,-39.7233770738199,
124.263648070586)) ;
#77118=CARTESIAN_POINT('Ctrl Pts',(-18.7392016865205,-39.9233197235952,
124.787593898563)) ;
#77119=CARTESIAN_POINT('Ctrl Pts',(-18.8732138714757,-39.7433306431764,
124.512438635764)) ;
#77120=CARTESIAN_POINT('Ctrl Pts',(-19.2458886960608,-39.943157633783,124.933442272074)) ;
#77121=CARTESIAN_POINT('Ctrl Pts',(-19.278565608068,-39.7631685533643,124.629117598788)) ;
#77122=CARTESIAN_POINT('Ctrl Pts',(-19.7756254405779,-39.963133462354,124.897944226736)) ;
#77123=CARTESIAN_POINT('Ctrl Pts',(-19.702355195912,-39.7831443819352,124.600718333619)) ;
#77124=CARTESIAN_POINT('Ctrl Pts',(-20.2597769713168,-39.9830515070642,
124.683907752949)) ;
#77125=CARTESIAN_POINT('Ctrl Pts',(-20.0896770292724,-39.8030624266455,
124.429488092088)) ;
#77126=CARTESIAN_POINT('Ctrl Pts',(-20.6419438141652,-40.0029217528519,
124.319255201544)) ;
#77127=CARTESIAN_POINT('Ctrl Pts',(-20.3954104744399,-39.8229326724332,
124.137764014872)) ;
#77128=CARTESIAN_POINT('Ctrl Pts',(-20.8780281937701,-40.0229707559515,
123.841688417879)) ;
#77129=CARTESIAN_POINT('Ctrl Pts',(-20.584276553681,-39.8429816755327,123.755710427859)) ;
#77130=CARTESIAN_POINT('Ctrl Pts',(-20.9367938162393,-40.0427499971923,
123.31912856274)) ;
#77131=CARTESIAN_POINT('Ctrl Pts',(-20.6312875872331,-39.8627609167736,
123.337660188172)) ;
#77132=CARTESIAN_POINT('Ctrl Pts',(-20.8129964069857,-40.0627800609012,
122.801479468791)) ;
#77133=CARTESIAN_POINT('Ctrl Pts',(-20.5322475926192,-39.8827909804824,
122.92354173138)) ;
#77134=CARTESIAN_POINT('Ctrl Pts',(-20.5213204072104,-40.0826623458031,
122.360731282059)) ;
#77135=CARTESIAN_POINT('Ctrl Pts',(-20.2989045254631,-39.9026732653844,
122.570943408871)) ;
#77136=CARTESIAN_POINT('Ctrl Pts',(-20.0977276287901,-40.1025446466961,
122.04487225265)) ;
#77137=CARTESIAN_POINT('Ctrl Pts',(-19.9600279171563,-39.9225555662774,
122.31825773152)) ;
#77138=CARTESIAN_POINT('Ctrl Pts',(-19.5891047472115,-40.1225277563145,
121.891899364557)) ;
#77139=CARTESIAN_POINT('Ctrl Pts',(-19.5531287369363,-39.9425386758957,
122.195882009548)) ;
#77140=CARTESIAN_POINT('Ctrl Pts',(-19.0612514000122,-40.1424181516924,
121.921603035581)) ;
#77141=CARTESIAN_POINT('Ctrl Pts',(-19.1308454119986,-39.9624290712736,
122.219647817995)) ;
#77142=CARTESIAN_POINT('Ctrl Pts',(-18.5748477162895,-40.1623149417266,
122.128947492309)) ;
#77143=CARTESIAN_POINT('Ctrl Pts',(-18.7417230650517,-39.9823258613079,
122.385526589855)) ;
#77144=CARTESIAN_POINT('Ctrl Pts',(-18.1875342171797,-40.1822319956683,
122.489841093168)) ;
#77145=CARTESIAN_POINT('Ctrl Pts',(-18.4318742437841,-40.0022429152495,
122.674244288826)) ;
#77146=CARTESIAN_POINT('Ctrl Pts',(-17.945715845596,-40.2022355438718,122.963405930305)) ;
#77147=CARTESIAN_POINT('Ctrl Pts',(-18.2384227101736,-40.022246463453,123.05309765344)) ;
#77148=CARTESIAN_POINT('Ctrl Pts',(-17.8810209348164,-40.2221738375244,
123.489343815256)) ;
#77149=CARTESIAN_POINT('Ctrl Pts',(-18.1866699625709,-40.0421847571056,
123.473848687239)) ;
#77150=CARTESIAN_POINT('Ctrl Pts',(-17.9977400536668,-40.2419953249573,
124.003081008366)) ;
#77151=CARTESIAN_POINT('Ctrl Pts',(-18.2800496556778,-40.0620062445386,
123.884838604969)) ;
#77152=CARTESIAN_POINT('Ctrl Pts',(-18.2845312147726,-40.2619737179482,
124.449892679413)) ;
#77153=CARTESIAN_POINT('Ctrl Pts',(-18.5094838885054,-40.0819846375294,
124.242285370891)) ;
#77154=CARTESIAN_POINT('Ctrl Pts',(-18.7051945464621,-40.2818720995619,
124.77055920549)) ;
#77155=CARTESIAN_POINT('Ctrl Pts',(-18.8460248106455,-40.1018830191431,
124.498817503231)) ;
#77156=CARTESIAN_POINT('Ctrl Pts',(-19.1255703487642,-40.2984550302918,
124.902674539554)) ;
#77157=CARTESIAN_POINT('Ctrl Pts',(-19.1823032071528,-40.118465949873,124.604500927526)) ;
#77158=CARTESIAN_POINT('Ctrl Pts',(-19.4741295857804,-40.3117292658806,
124.917986772778)) ;
#77159=CARTESIAN_POINT('Ctrl Pts',(-19.461172160329,-40.1317401854619,124.616752617202)) ;
#77160=CARTESIAN_POINT('Ctrl Pts',(-19.7358425463497,-40.3217756833368,
124.883469686285)) ;
#77161=CARTESIAN_POINT('Ctrl Pts',(-19.6705356336101,-40.1417866029181,
124.589137624141)) ;
#77162=CARTESIAN_POINT('Ctrl Pts',(-19.9826774778491,-40.3316209085561,
124.80588177867)) ;
#77163=CARTESIAN_POINT('Ctrl Pts',(-19.8680131815929,-40.1516318281373,
124.527058888594)) ;
#77164=CARTESIAN_POINT('Ctrl Pts',(-20.293982933637,-40.3449558795955,124.645032731984)) ;
#77165=CARTESIAN_POINT('Ctrl Pts',(-20.117012406976,-40.1649667991767,124.398409704518)) ;
#77166=CARTESIAN_POINT('Ctrl Pts',(-20.6198884115135,-40.3615387363881,
124.348182656284)) ;
#77167=CARTESIAN_POINT('Ctrl Pts',(-20.3777873723934,-40.1815496559694,
124.160882593775)) ;
#77168=CARTESIAN_POINT('Ctrl Pts',(-20.8256972516867,-40.3781817387375,
123.956743051185)) ;
#77169=CARTESIAN_POINT('Ctrl Pts',(-20.5424028051594,-40.1981926583188,
123.84776904717)) ;
#77170=CARTESIAN_POINT('Ctrl Pts',(-20.9027340823675,-40.3914254697692,
123.617264907888)) ;
#77171=CARTESIAN_POINT('Ctrl Pts',(-20.6040438274232,-40.2114363893504,
123.576158441857)) ;
#77172=CARTESIAN_POINT('Ctrl Pts',(-20.9155780418675,-40.4014798644438,
123.353409333887)) ;
#77173=CARTESIAN_POINT('Ctrl Pts',(-20.6143139039399,-40.221490784025,123.365079497654)) ;
#77174=CARTESIAN_POINT('Ctrl Pts',(-20.883436236748,-40.4113209258323,123.096754250343)) ;
#77175=CARTESIAN_POINT('Ctrl Pts',(-20.5885990123171,-40.2313318454136,
123.159754036855)) ;
#77176=CARTESIAN_POINT('Ctrl Pts',(-20.8057493250627,-40.4213871501888,
122.843935791891)) ;
#77177=CARTESIAN_POINT('Ctrl Pts',(-20.5264471820404,-40.2413980697701,
122.957500455723)) ;
#77178=CARTESIAN_POINT('Ctrl Pts',(-20.6874567828828,-40.4312677631085,
122.61274782881)) ;
#77179=CARTESIAN_POINT('Ctrl Pts',(-20.431811178883,-40.2512786826897,122.77255090532)) ;
#77180=CARTESIAN_POINT('Ctrl Pts',(-20.5294818312778,-40.4412610562681,
122.403016184091)) ;
#77181=CARTESIAN_POINT('Ctrl Pts',(-20.3054294355456,-40.2612719758493,
122.604767012198)) ;
#77182=CARTESIAN_POINT('Ctrl Pts',(-20.3383061145161,-40.4512120644917,
122.224524733041)) ;
#77183=CARTESIAN_POINT('Ctrl Pts',(-20.1524873435744,-40.271222984073,122.461975496637)) ;
#77184=CARTESIAN_POINT('Ctrl Pts',(-20.1168471521159,-40.4612605788537,
122.08075282336)) ;
#77185=CARTESIAN_POINT('Ctrl Pts',(-19.9753190159199,-40.281271498435,122.34695989764)) ;
#77186=CARTESIAN_POINT('Ctrl Pts',(-19.8788615309388,-40.4711020849164,
121.979450513816)) ;
#77187=CARTESIAN_POINT('Ctrl Pts',(-19.7849296059222,-40.2911130044976,
122.265920106906)) ;
#77188=CARTESIAN_POINT('Ctrl Pts',(-19.6234056665273,-40.4810877375461,
121.919608246961)) ;
#77189=CARTESIAN_POINT('Ctrl Pts',(-19.5805644621411,-40.3010986571273,
122.218048512511)) ;
#77190=CARTESIAN_POINT('Ctrl Pts',(-19.3625879444261,-40.491026746391,121.904994592933)) ;
#77191=CARTESIAN_POINT('Ctrl Pts',(-19.3719102147239,-40.3110376659722,
122.206359844841)) ;
#77192=CARTESIAN_POINT('Ctrl Pts',(-19.1006071741676,-40.501067671684,121.9362672369)) ;
#77193=CARTESIAN_POINT('Ctrl Pts',(-19.1623259175616,-40.3210785912652,
122.231380198729)) ;
#77194=CARTESIAN_POINT('Ctrl Pts',(-18.8517347176432,-40.5109579934389,
122.011275192516)) ;
#77195=CARTESIAN_POINT('Ctrl Pts',(-18.9632286807816,-40.3309689130201,
122.291388701103)) ;
#77196=CARTESIAN_POINT('Ctrl Pts',(-18.6170528303979,-40.5209539667723,
122.129240595586)) ;
#77197=CARTESIAN_POINT('Ctrl Pts',(-18.775484242593,-40.3409648863536,122.385763008815)) ;
#77198=CARTESIAN_POINT('Ctrl Pts',(-18.4077408550666,-40.5308853663543,
122.285152304455)) ;
#77199=CARTESIAN_POINT('Ctrl Pts',(-18.6080360869343,-40.3508962859356,
122.510494122467)) ;
#77200=CARTESIAN_POINT('Ctrl Pts',(-18.2270702113385,-40.5408909068314,
122.476201697445)) ;
#77201=CARTESIAN_POINT('Ctrl Pts',(-18.463501244713,-40.3609018264127,122.663335132753)) ;
#77202=CARTESIAN_POINT('Ctrl Pts',(-18.0823350470019,-40.5509238907627,
122.696568451473)) ;
#77203=CARTESIAN_POINT('Ctrl Pts',(-18.3477150174073,-40.370934810344,122.839629750178)) ;
#77204=CARTESIAN_POINT('Ctrl Pts',(-17.9794720036772,-40.5607795215895,
122.934283776529)) ;
#77205=CARTESIAN_POINT('Ctrl Pts',(-18.2654267150485,-40.3807904411708,
123.029802727258)) ;
#77206=CARTESIAN_POINT('Ctrl Pts',(-17.9182550888982,-40.5707789237827,
123.189781090314)) ;
#77207=CARTESIAN_POINT('Ctrl Pts',(-18.2164553726085,-40.390789843364,123.234201028577)) ;
#77208=CARTESIAN_POINT('Ctrl Pts',(-17.9021932201745,-40.5806733931438,
123.449349378983)) ;
#77209=CARTESIAN_POINT('Ctrl Pts',(-18.2036080982215,-40.400684312725,123.441855585745)) ;
#77210=CARTESIAN_POINT('Ctrl Pts',(-17.9320113008533,-40.590736507308,123.712065167668)) ;
#77211=CARTESIAN_POINT('Ctrl Pts',(-18.2274647737821,-40.4107474268893,
123.65202799485)) ;
#77212=CARTESIAN_POINT('Ctrl Pts',(-18.0050786319795,-40.6005761530244,
123.960147159089)) ;
#77213=CARTESIAN_POINT('Ctrl Pts',(-18.2859206557208,-40.4205870726056,
123.850492648776)) ;
#77214=CARTESIAN_POINT('Ctrl Pts',(-18.1223872400541,-40.6106393205801,
124.197113300206)) ;
#77215=CARTESIAN_POINT('Ctrl Pts',(-18.3797695138113,-40.4306502401614,
124.04006462666)) ;
#77216=CARTESIAN_POINT('Ctrl Pts',(-18.276645110429,-40.620533576375,124.406457589645)) ;
#77217=CARTESIAN_POINT('Ctrl Pts',(-18.5031774204624,-40.4405444959563,
124.207538542366)) ;
#77218=CARTESIAN_POINT('Ctrl Pts',(-18.4652776966271,-40.6304753548347,
124.587171422817)) ;
#77219=CARTESIAN_POINT('Ctrl Pts',(-18.6540848187046,-40.4504862744159,
124.352107914679)) ;
#77220=CARTESIAN_POINT('Ctrl Pts',(-18.6837565652189,-40.6404780476649,
124.733392656267)) ;
#77221=CARTESIAN_POINT('Ctrl Pts',(-18.8288690428585,-40.4604889672461,
124.469083093928)) ;
#77222=CARTESIAN_POINT('Ctrl Pts',(-18.9251772147338,-40.6505120696187,
124.839403238368)) ;
#77223=CARTESIAN_POINT('Ctrl Pts',(-19.0220064463768,-40.4705229891999,
124.553889578956)) ;
#77224=CARTESIAN_POINT('Ctrl Pts',(-19.1765096236115,-40.6603598607077,
124.901116406768)) ;
#77225=CARTESIAN_POINT('Ctrl Pts',(-19.2230724433567,-40.480370780289,124.603257935975)) ;
#77226=CARTESIAN_POINT('Ctrl Pts',(-19.4381766703667,-40.6703413852567,
124.9190603837)) ;
#77227=CARTESIAN_POINT('Ctrl Pts',(-19.4324060828598,-40.490352304838,124.617611036855)) ;
#77228=CARTESIAN_POINT('Ctrl Pts',(-19.6981676204885,-40.6802906087477,
124.891345054744)) ;
#77229=CARTESIAN_POINT('Ctrl Pts',(-19.6403984071711,-40.5003015283289,
124.595436730586)) ;
#77230=CARTESIAN_POINT('Ctrl Pts',(-19.9507242764869,-40.6902882649642,
124.818869487546)) ;
#77231=CARTESIAN_POINT('Ctrl Pts',(-19.8424430882566,-40.5102991845455,
124.537454338467)) ;
#77232=CARTESIAN_POINT('Ctrl Pts',(-20.1876076662256,-40.7003284780193,
124.702714148728)) ;
#77233=CARTESIAN_POINT('Ctrl Pts',(-20.0319489184708,-40.5203393976006,
124.444528159668)) ;
#77234=CARTESIAN_POINT('Ctrl Pts',(-20.3965794743813,-40.7101565252955,
124.550916691097)) ;
#77235=CARTESIAN_POINT('Ctrl Pts',(-20.1991246693014,-40.5301674448768,
124.323088910881)) ;
#77236=CARTESIAN_POINT('Ctrl Pts',(-20.5804267072891,-40.7202108723279,
124.361171005095)) ;
#77237=CARTESIAN_POINT('Ctrl Pts',(-20.346201090862,-40.5402217919092,124.171290919494)) ;
#77238=CARTESIAN_POINT('Ctrl Pts',(-20.7265146725053,-40.7301520086565,
124.144583500083)) ;
#77239=CARTESIAN_POINT('Ctrl Pts',(-20.4630696218111,-40.5501629282377,
123.998019996052)) ;
#77240=CARTESIAN_POINT('Ctrl Pts',(-20.8331181684414,-40.7400562417362,
123.907137322054)) ;
#77241=CARTESIAN_POINT('Ctrl Pts',(-20.5483504786271,-40.5600671613174,
123.808062650785)) ;
#77242=CARTESIAN_POINT('Ctrl Pts',(-20.8976239887769,-40.7501029385798,
123.651145500457)) ;
#77243=CARTESIAN_POINT('Ctrl Pts',(-20.5999532571857,-40.5701138581611,
123.603268634691)) ;
#77244=CARTESIAN_POINT('Ctrl Pts',(-20.9166549330674,-40.7599984898601,
123.391755647877)) ;
#77245=CARTESIAN_POINT('Ctrl Pts',(-20.6151760608745,-40.5800094094413,
123.395757077431)) ;
#77246=CARTESIAN_POINT('Ctrl Pts',(-20.8899239296394,-40.7700605676996,
123.128727559475)) ;
#77247=CARTESIAN_POINT('Ctrl Pts',(-20.5937893272539,-40.5900714872808,
123.18533465587)) ;
#77248=CARTESIAN_POINT('Ctrl Pts',(-20.8196225926542,-40.7799032767956,
122.879777795685)) ;
#77249=CARTESIAN_POINT('Ctrl Pts',(-20.5375466154367,-40.5999141963769,
122.98617602963)) ;
#77250=CARTESIAN_POINT('Ctrl Pts',(-20.7060594583862,-40.7898940090341,
122.643100332468)) ;
#77251=CARTESIAN_POINT('Ctrl Pts',(-20.4466945356706,-40.6099049286153,
122.796834968904)) ;
#77252=CARTESIAN_POINT('Ctrl Pts',(-20.5540244826181,-40.7998220342628,
122.431061345429)) ;
#77253=CARTESIAN_POINT('Ctrl Pts',(-20.3250653085112,-40.6198329538441,
122.627205154481)) ;
#77254=CARTESIAN_POINT('Ctrl Pts',(-20.3666704075029,-40.8098101809134,
122.247223536426)) ;
#77255=CARTESIAN_POINT('Ctrl Pts',(-20.1751809297172,-40.6298211004947,
122.480136252607)) ;
#77256=CARTESIAN_POINT('Ctrl Pts',(-20.1490005901118,-40.8198451987533,
122.098346117537)) ;
#77257=CARTESIAN_POINT('Ctrl Pts',(-20.0010440055564,-40.6398561183346,
122.361035777316)) ;
#77258=CARTESIAN_POINT('Ctrl Pts',(-19.9129860528095,-40.8297099958586,
121.991128079593)) ;
#77259=CARTESIAN_POINT('Ctrl Pts',(-19.8122322768596,-40.6497209154398,
122.275263239916)) ;
#77260=CARTESIAN_POINT('Ctrl Pts',(-19.6596753422192,-40.8396707282147,
121.92514335029)) ;
#77261=CARTESIAN_POINT('Ctrl Pts',(-19.6095835667024,-40.6596816477959,
122.222477106731)) ;
#77262=CARTESIAN_POINT('Ctrl Pts',(-19.3968323127535,-40.8497041906117,
121.90443177847)) ;
#77263=CARTESIAN_POINT('Ctrl Pts',(-19.3993089374676,-40.6697151101929,
122.205909546887)) ;
#77264=CARTESIAN_POINT('Ctrl Pts',(-19.1381719931568,-40.8595897248231,
121.928871855585)) ;
#77265=CARTESIAN_POINT('Ctrl Pts',(-19.1923814686727,-40.6796006444043,
122.225463173289)) ;
#77266=CARTESIAN_POINT('Ctrl Pts',(-18.8832051234587,-40.8696545655031,
121.999096372932)) ;
#77267=CARTESIAN_POINT('Ctrl Pts',(-18.9884082093164,-40.6896654850843,
122.281644418991)) ;
#77268=CARTESIAN_POINT('Ctrl Pts',(-18.6493502438583,-40.8795026972319,
122.110000505727)) ;
#77269=CARTESIAN_POINT('Ctrl Pts',(-18.8013257528878,-40.6995136168132,
122.370368822003)) ;
#77270=CARTESIAN_POINT('Ctrl Pts',(-18.4340900375978,-40.8895301942221,
122.261979815456)) ;
#77271=CARTESIAN_POINT('Ctrl Pts',(-18.6291184182037,-40.7095411138033,
122.49195350058)) ;
#77272=CARTESIAN_POINT('Ctrl Pts',(-18.2489515311722,-40.8995586462672,
122.449550692962)) ;
#77273=CARTESIAN_POINT('Ctrl Pts',(-18.4810087252179,-40.7195695658484,
122.642011378484)) ;
#77274=CARTESIAN_POINT('Ctrl Pts',(-18.1015397640265,-40.9094039128313,
122.66215418172)) ;
#77275=CARTESIAN_POINT('Ctrl Pts',(-18.3630810732943,-40.7294148324125,
122.812094300653)) ;
#77276=CARTESIAN_POINT('Ctrl Pts',(-17.9910357649292,-40.9193945857722,
122.9003183125)) ;
#77277=CARTESIAN_POINT('Ctrl Pts',(-18.2746791939818,-40.7394055053534,
123.002626045039)) ;
#77278=CARTESIAN_POINT('Ctrl Pts',(-17.923815012575,-40.9294324678607,123.155391667996)) ;
#77279=CARTESIAN_POINT('Ctrl Pts',(-18.2209040160254,-40.7494433874419,
123.206685215275)) ;
#77280=CARTESIAN_POINT('Ctrl Pts',(-17.9018757959,-40.9392768383003,123.413170064838)) ;
#77281=CARTESIAN_POINT('Ctrl Pts',(-18.2033541255179,-40.7592877578816,
123.41290711647)) ;
#77282=CARTESIAN_POINT('Ctrl Pts',(-17.9248387221279,-40.9492616656957,
123.674518463685)) ;
#77283=CARTESIAN_POINT('Ctrl Pts',(-18.2217257460994,-40.7692725852769,
123.621985522676)) ;
#77284=CARTESIAN_POINT('Ctrl Pts',(-17.9924288979243,-40.959201111101,123.926859520028)) ;
#77285=CARTESIAN_POINT('Ctrl Pts',(-18.2757990048026,-40.7792120306822,
123.823857616306)) ;
#77286=CARTESIAN_POINT('Ctrl Pts',(-18.1039644976458,-40.9692411153869,
124.165936540815)) ;
#77287=CARTESIAN_POINT('Ctrl Pts',(-18.3650287084099,-40.7892520349681,
124.015118795446)) ;
#77288=CARTESIAN_POINT('Ctrl Pts',(-18.2528993474394,-40.9791282245725,
124.378873025774)) ;
#77289=CARTESIAN_POINT('Ctrl Pts',(-18.4841771835395,-40.7991391441538,
124.185466648641)) ;
#77290=CARTESIAN_POINT('Ctrl Pts',(-18.4383623409316,-40.989128284475,124.564995129776)) ;
#77291=CARTESIAN_POINT('Ctrl Pts',(-18.6325483359507,-40.8091392040562,
124.334363415602)) ;
#77292=CARTESIAN_POINT('Ctrl Pts',(-18.6514890496994,-40.9990457003897,
124.715068772914)) ;
#77293=CARTESIAN_POINT('Ctrl Pts',(-18.8030498870585,-40.8190566199709,
124.454421071669)) ;
#77294=CARTESIAN_POINT('Ctrl Pts',(-18.8904730960072,-41.0090925151305,
124.827199842397)) ;
#77295=CARTESIAN_POINT('Ctrl Pts',(-18.9942377675479,-40.8291034347117,
124.54412495723)) ;
#77296=CARTESIAN_POINT('Ctrl Pts',(-19.1409580664959,-41.0189679923272,
124.89523536818)) ;
#77297=CARTESIAN_POINT('Ctrl Pts',(-19.1946252220464,-40.8389789119084,
124.59855210373)) ;
#77298=CARTESIAN_POINT('Ctrl Pts',(-19.4040773768786,-41.0290240880484,
124.919312459414)) ;
#77299=CARTESIAN_POINT('Ctrl Pts',(-19.4051209742534,-40.8490350076296,
124.617812738242)) ;
#77300=CARTESIAN_POINT('Ctrl Pts',(-19.663216707279,-41.0389172500634,124.897783110562)) ;
#77301=CARTESIAN_POINT('Ctrl Pts',(-19.612431616485,-40.8589281696447,124.600588287946)) ;
#77302=CARTESIAN_POINT('Ctrl Pts',(-19.9189173138886,-41.0489794860861,
124.830551760959)) ;
#77303=CARTESIAN_POINT('Ctrl Pts',(-19.816992096317,-40.8689904056673,124.546802153709)) ;
#77304=CARTESIAN_POINT('Ctrl Pts',(-20.1539134835789,-41.058823951715,124.7223429247)) ;
#77305=CARTESIAN_POINT('Ctrl Pts',(-20.0049876465229,-40.8788348712962,
124.460234605023)) ;
#77306=CARTESIAN_POINT('Ctrl Pts',(-20.3695735131552,-41.0687840444191,
124.574029278999)) ;
#77307=CARTESIAN_POINT('Ctrl Pts',(-20.1775149195478,-40.8887949640004,
124.34158324237)) ;
#77308=CARTESIAN_POINT('Ctrl Pts',(-20.5573002807769,-41.0788223334002,
124.388718288862)) ;
#77309=CARTESIAN_POINT('Ctrl Pts',(-20.3276957826536,-40.8988332529814,
124.193333707095)) ;
#77310=CARTESIAN_POINT('Ctrl Pts',(-20.7079273847676,-41.0886956565064,
124.177407956279)) ;
#77311=CARTESIAN_POINT('Ctrl Pts',(-20.4481962954603,-40.9087065760876,
124.024285712482)) ;
#77312=CARTESIAN_POINT('Ctrl Pts',(-20.821719687652,-41.0987688405915,123.938460528955)) ;
#77313=CARTESIAN_POINT('Ctrl Pts',(-20.5392295466057,-40.9187797601727,
123.833127110571)) ;
#77314=CARTESIAN_POINT('Ctrl Pts',(-20.8908771121847,-41.1085893528794,
123.689767340511)) ;
#77315=CARTESIAN_POINT('Ctrl Pts',(-20.5945544458289,-40.9286002724607,
123.634173561183)) ;
#77316=CARTESIAN_POINT('Ctrl Pts',(-20.9166985131135,-41.1186673489952,
123.426252975595)) ;
#77317=CARTESIAN_POINT('Ctrl Pts',(-20.615210932042,-40.9386782685765,123.423361632516)) ;
#77318=CARTESIAN_POINT('Ctrl Pts',(-20.8968766071767,-41.1285214239785,
123.16799763283)) ;
#77319=CARTESIAN_POINT('Ctrl Pts',(-20.5993528292853,-40.9485323435597,
123.21675844281)) ;
#77320=CARTESIAN_POINT('Ctrl Pts',(-20.8314512990884,-41.1385853055622,
122.911802236395)) ;
#77321=CARTESIAN_POINT('Ctrl Pts',(-20.5470119442779,-40.9585962251434,
123.011802002189)) ;
#77322=CARTESIAN_POINT('Ctrl Pts',(-20.7244059190005,-41.1484687315359,
122.675111707048)) ;
#77323=CARTESIAN_POINT('Ctrl Pts',(-20.461375448032,-40.9684796511172,122.822450609287)) ;
#77324=CARTESIAN_POINT('Ctrl Pts',(-20.5765499861108,-41.158469335457,122.457899543899)) ;
#77325=CARTESIAN_POINT('Ctrl Pts',(-20.3430903518895,-40.9784802550382,
122.648681253808)) ;
#77326=CARTESIAN_POINT('Ctrl Pts',(-20.3947593960527,-41.1683891197948,
122.270998373861)) ;
#77327=CARTESIAN_POINT('Ctrl Pts',(-20.1976579864223,-40.9884000393761,
122.499161080854)) ;
#77328=CARTESIAN_POINT('Ctrl Pts',(-20.1805968422417,-41.1784364701517,
122.116644489957)) ;
#77329=CARTESIAN_POINT('Ctrl Pts',(-20.0263275114058,-40.998447389733,122.37567824904)) ;
#77330=CARTESIAN_POINT('Ctrl Pts',(-19.9469565781319,-41.188313812386,122.003445575684)) ;
#77331=CARTESIAN_POINT('Ctrl Pts',(-19.8394159581554,-41.0083247319672,
122.285119878453)) ;
#77332=CARTESIAN_POINT('Ctrl Pts',(-19.6924393110827,-41.1983836934606,
121.931197405245)) ;
#77333=CARTESIAN_POINT('Ctrl Pts',(-19.6358017081943,-41.0183946130419,
122.227321635127)) ;
#77334=CARTESIAN_POINT('Ctrl Pts',(-19.4354489668102,-41.2082133986623,
121.904602386761)) ;
#77335=CARTESIAN_POINT('Ctrl Pts',(-19.430210627212,-41.0282243182436,122.206046078659)) ;
#77336=CARTESIAN_POINT('Ctrl Pts',(-19.1716002965665,-41.2182800598287,
121.92311830147)) ;
#77337=CARTESIAN_POINT('Ctrl Pts',(-19.2191313901848,-41.03829097941,122.220859076658)) ;
#77338=CARTESIAN_POINT('Ctrl Pts',(-18.9194385507668,-41.228170281696,121.986221032393)) ;
#77339=CARTESIAN_POINT('Ctrl Pts',(-19.0174028771925,-41.0481812012773,
122.271341336615)) ;
#77340=CARTESIAN_POINT('Ctrl Pts',(-18.6794263981933,-41.2381624578062,
122.092694865088)) ;
#77341=CARTESIAN_POINT('Ctrl Pts',(-18.825393369095,-41.0581733773874,122.356520462696)) ;
#77342=CARTESIAN_POINT('Ctrl Pts',(-18.4623191157902,-41.2481252879188,
122.239006352242)) ;
#77343=CARTESIAN_POINT('Ctrl Pts',(-18.6517079609517,-41.0681362075001,
122.473569619426)) ;
#77344=CARTESIAN_POINT('Ctrl Pts',(-18.2745423236798,-41.2580295003191,
122.419265967133)) ;
#77345=CARTESIAN_POINT('Ctrl Pts',(-18.5014870946545,-41.0780404199004,
122.617776816636)) ;
#77346=CARTESIAN_POINT('Ctrl Pts',(-18.118713573879,-41.268090214407,122.632804079634)) ;
#77347=CARTESIAN_POINT('Ctrl Pts',(-18.3768240055462,-41.0881011339882,
122.788607593364)) ;
#77348=CARTESIAN_POINT('Ctrl Pts',(-18.0045368874471,-41.2779297173898,
122.864848022262)) ;
#77349=CARTESIAN_POINT('Ctrl Pts',(-18.2854831831512,-41.097940636971,122.974241688555)) ;
#77350=CARTESIAN_POINT('Ctrl Pts',(-17.9304874745659,-41.2879958559562,
123.118755220542)) ;
#77351=CARTESIAN_POINT('Ctrl Pts',(-18.2262435039461,-41.1080067755374,
123.177367738535)) ;
#77352=CARTESIAN_POINT('Ctrl Pts',(-17.9022632242414,-41.2978783704422,
123.376958924442)) ;
#77353=CARTESIAN_POINT('Ctrl Pts',(-18.2036641643928,-41.1178892900235,
123.383929797729)) ;
#77354=CARTESIAN_POINT('Ctrl Pts',(-17.9189692033118,-41.3078706697977,
123.638973965505)) ;
#77355=CARTESIAN_POINT('Ctrl Pts',(-18.2170287674167,-41.127881589379,123.593541666519)) ;
#77356=CARTESIAN_POINT('Ctrl Pts',(-17.9806273076424,-41.3178237367511,
123.893199304598)) ;
#77357=CARTESIAN_POINT('Ctrl Pts',(-18.2663549772125,-41.1378346563324,
123.796921581805)) ;
#77358=CARTESIAN_POINT('Ctrl Pts',(-18.0864278199348,-41.3278584449564,
124.134724121219)) ;
#77359=CARTESIAN_POINT('Ctrl Pts',(-18.3509952924776,-41.1478693645376,
123.990141608418)) ;
#77360=CARTESIAN_POINT('Ctrl Pts',(-18.230286207724,-41.3377466658605,124.351140926616)) ;
#77361=CARTESIAN_POINT('Ctrl Pts',(-18.4660813609323,-41.1577575854418,
124.163274450491)) ;
#77362=CARTESIAN_POINT('Ctrl Pts',(-18.411128139942,-41.347741088891,124.541587743778)) ;
#77363=CARTESIAN_POINT('Ctrl Pts',(-18.6107545669795,-41.1677520084722,
124.31563199722)) ;
#77364=CARTESIAN_POINT('Ctrl Pts',(-18.6213277143798,-41.3576864283371,
124.696900401369)) ;
#77365=CARTESIAN_POINT('Ctrl Pts',(-18.7789136746949,-41.1776973479184,
124.439882070568)) ;
#77366=CARTESIAN_POINT('Ctrl Pts',(-18.8551198560188,-41.3676337729485,
124.813866561851)) ;
#77367=CARTESIAN_POINT('Ctrl Pts',(-18.9659467888428,-41.1876446925297,
124.533455168981)) ;
#77368=CARTESIAN_POINT('Ctrl Pts',(-19.1082663812301,-41.3776816683594,
124.888923688578)) ;
#77369=CARTESIAN_POINT('Ctrl Pts',(-19.1684641030672,-41.1976925879407,
124.593501257939)) ;
#77370=CARTESIAN_POINT('Ctrl Pts',(-19.365357688919,-41.3875293138388,124.918508593986)) ;
#77371=CARTESIAN_POINT('Ctrl Pts',(-19.374135991281,-41.2075402334201,124.617169451887)) ;
#77372=CARTESIAN_POINT('Ctrl Pts',(-19.6267063239591,-41.3974910277528,
124.903644555677)) ;
#77373=CARTESIAN_POINT('Ctrl Pts',(-19.5832145704097,-41.2175019473341,
124.605278846852)) ;
#77374=CARTESIAN_POINT('Ctrl Pts',(-19.8831669773534,-41.4075196520438,
124.842893155748)) ;
#77375=CARTESIAN_POINT('Ctrl Pts',(-19.7883832884811,-41.227530571625,124.556678216363)) ;
#77376=CARTESIAN_POINT('Ctrl Pts',(-20.1223364380346,-41.4174300127005,
124.739853154609)) ;
#77377=CARTESIAN_POINT('Ctrl Pts',(-19.9797184280272,-41.2374409322817,
124.474246990679)) ;
#77378=CARTESIAN_POINT('Ctrl Pts',(-20.3409126899482,-41.4273647112738,
124.597063389215)) ;
#77379=CARTESIAN_POINT('Ctrl Pts',(-20.1545793763586,-41.247375630855,124.360016063863)) ;
#77380=CARTESIAN_POINT('Ctrl Pts',(-20.5332339905812,-41.437406536128,124.416390285372)) ;
#77381=CARTESIAN_POINT('Ctrl Pts',(-20.3084369714252,-41.2574174557092,
124.215477948896)) ;
#77382=CARTESIAN_POINT('Ctrl Pts',(-20.6889942203536,-41.4472911098724,
124.208484214608)) ;
#77383=CARTESIAN_POINT('Ctrl Pts',(-20.4330452122912,-41.2673020294536,
124.049154187181)) ;
#77384=CARTESIAN_POINT('Ctrl Pts',(-20.8079337347241,-41.4572929592355,
123.974137087489)) ;
#77385=CARTESIAN_POINT('Ctrl Pts',(-20.5281974668487,-41.2773038788168,
123.861676944645)) ;
#77386=CARTESIAN_POINT('Ctrl Pts',(-20.8839492757702,-41.4672122608096,
123.724761737212)) ;
#77387=CARTESIAN_POINT('Ctrl Pts',(-20.5890105118696,-41.2872231803909,
123.662177488703)) ;
#77388=CARTESIAN_POINT('Ctrl Pts',(-20.9159063784772,-41.4772563691549,
123.462776779807)) ;
#77389=CARTESIAN_POINT('Ctrl Pts',(-20.6145770325687,-41.2972672887361,
123.452589454882)) ;
#77390=CARTESIAN_POINT('Ctrl Pts',(-20.9021882405905,-41.4871407925971,
123.20337470008)) ;
#77391=CARTESIAN_POINT('Ctrl Pts',(-20.6036034091239,-41.3071517121784,
123.245068567429)) ;
#77392=CARTESIAN_POINT('Ctrl Pts',(-20.8434269168873,-41.4971571545066,
122.946788139657)) ;
#77393=CARTESIAN_POINT('Ctrl Pts',(-20.5565953052322,-41.3171680740879,
123.039799101921)) ;
#77394=CARTESIAN_POINT('Ctrl Pts',(-20.7401692463216,-41.507193810012,122.704103736662)) ;
#77395=CARTESIAN_POINT('Ctrl Pts',(-20.4739898809288,-41.3272047295932,
122.845651168886)) ;
#77396=CARTESIAN_POINT('Ctrl Pts',(-20.5998669969204,-41.5170239402013,
122.487161714468)) ;
#77397=CARTESIAN_POINT('Ctrl Pts',(-20.3617495279934,-41.3370348597826,
122.672097974141)) ;
#77398=CARTESIAN_POINT('Ctrl Pts',(-20.4197517581222,-41.5270999932912,
122.293140547017)) ;
#77399=CARTESIAN_POINT('Ctrl Pts',(-20.2176578409717,-41.3471109128724,
122.516880105175)) ;
#77400=CARTESIAN_POINT('Ctrl Pts',(-20.2133740001991,-41.536952222477,122.136713686601)) ;
#77401=CARTESIAN_POINT('Ctrl Pts',(-20.0525570462563,-41.3569631420582,
122.391738386618)) ;
#77402=CARTESIAN_POINT('Ctrl Pts',(-19.9779921556305,-41.5470254302763,
122.015693380282)) ;
#77403=CARTESIAN_POINT('Ctrl Pts',(-19.8642517827859,-41.3670363498575,
122.294921027755)) ;
#77404=CARTESIAN_POINT('Ctrl Pts',(-19.7309096530858,-41.5568669416277,
121.939233606191)) ;
#77405=CARTESIAN_POINT('Ctrl Pts',(-19.6665870925325,-41.3768778612089,
122.233752494711)) ;
#77406=CARTESIAN_POINT('Ctrl Pts',(-19.4713417220691,-41.5668278796652,
121.905469506119)) ;
#77407=CARTESIAN_POINT('Ctrl Pts',(-19.4589332355636,-41.3868387992465,
122.206739977289)) ;
#77408=CARTESIAN_POINT('Ctrl Pts',(-19.2078592032228,-41.5768657415902,
121.91790709068)) ;
#77409=CARTESIAN_POINT('Ctrl Pts',(-19.2481470590052,-41.3968766611714,
122.216688878807)) ;
#77410=CARTESIAN_POINT('Ctrl Pts',(-18.9545877189853,-41.5867399275872,
121.974495320647)) ;
#77411=CARTESIAN_POINT('Ctrl Pts',(-19.0455303831215,-41.4067508471685,
122.261958038974)) ;
#77412=CARTESIAN_POINT('Ctrl Pts',(-18.7103088483372,-41.5968100871651,
122.076174219081)) ;
#77413=CARTESIAN_POINT('Ctrl Pts',(-18.8501065384056,-41.4168210067464,
122.343300089057)) ;
#77414=CARTESIAN_POINT('Ctrl Pts',(-18.4925316286567,-41.606641834591,122.215244290438)) ;
#77415=CARTESIAN_POINT('Ctrl Pts',(-18.675884926045,-41.4266527541722,122.454554491954)) ;
#77416=CARTESIAN_POINT('Ctrl Pts',(-18.2978201733215,-41.6166779146623,
122.393114575324)) ;
#77417=CARTESIAN_POINT('Ctrl Pts',(-18.5201147167768,-41.4366888342435,
122.596849707631)) ;
#77418=CARTESIAN_POINT('Ctrl Pts',(-18.1377661291007,-41.6266949615148,
122.602121409373)) ;
#77419=CARTESIAN_POINT('Ctrl Pts',(-18.3920704452954,-41.446705881096,122.764054368868)) ;
#77420=CARTESIAN_POINT('Ctrl Pts',(-18.0176363963573,-41.6365772196814,
122.832366722348)) ;
#77421=CARTESIAN_POINT('Ctrl Pts',(-18.2959657432194,-41.4565881392626,
122.948249322725)) ;
#77422=CARTESIAN_POINT('Ctrl Pts',(-17.9381960768741,-41.6465649024777,
123.082493245772)) ;
#77423=CARTESIAN_POINT('Ctrl Pts',(-18.2324121300775,-41.466575822059,123.148349941612)) ;
#77424=CARTESIAN_POINT('Ctrl Pts',(-17.9033168941864,-41.6565115591945,
123.341584277104)) ;
#77425=CARTESIAN_POINT('Ctrl Pts',(-18.2045073339234,-41.4765224787757,
123.355622202973)) ;
#77426=CARTESIAN_POINT('Ctrl Pts',(-17.9143411682113,-41.6665686172746,
123.605613842763)) ;
#77427=CARTESIAN_POINT('Ctrl Pts',(-18.2133253006572,-41.4865795368559,
123.56684609059)) ;
#77428=CARTESIAN_POINT('Ctrl Pts',(-17.9693550454836,-41.6763867968241,
123.857706729687)) ;
#77429=CARTESIAN_POINT('Ctrl Pts',(-18.2573346904217,-41.4963977164053,
123.768519739504)) ;
#77430=CARTESIAN_POINT('Ctrl Pts',(-18.0688075004659,-41.6864227312631,
124.101962974005)) ;
#77431=CARTESIAN_POINT('Ctrl Pts',(-18.3368951443602,-41.5064336508443,
123.963925444336)) ;
#77432=CARTESIAN_POINT('Ctrl Pts',(-18.2096507194061,-41.6964473856921,
124.324600663838)) ;
#77433=CARTESIAN_POINT('Ctrl Pts',(-18.4495684418936,-41.5164583052733,
124.142036426713)) ;
#77434=CARTESIAN_POINT('Ctrl Pts',(-18.3835301011871,-41.7062994052716,
124.516428432838)) ;
#77435=CARTESIAN_POINT('Ctrl Pts',(-18.5886701972633,-41.5263103248528,
124.295499139978)) ;
#77436=CARTESIAN_POINT('Ctrl Pts',(-18.5906854587567,-41.7162903189865,
124.677682956485)) ;
#77437=CARTESIAN_POINT('Ctrl Pts',(-18.7543933282232,-41.5363012385678,
124.424504019859)) ;
#77438=CARTESIAN_POINT('Ctrl Pts',(-18.8209758180989,-41.7262083078261,
124.799801737025)) ;
#77439=CARTESIAN_POINT('Ctrl Pts',(-18.9386244015868,-41.5462192274073,
124.522200358764)) ;
#77440=CARTESIAN_POINT('Ctrl Pts',(-19.0716562721094,-41.7362364185569,
124.881015168281)) ;
#77441=CARTESIAN_POINT('Ctrl Pts',(-19.1391682539512,-41.5562473381381,
124.587172769983)) ;
#77442=CARTESIAN_POINT('Ctrl Pts',(-19.3289219205446,-41.7461216164653,
124.917060930271)) ;
#77443=CARTESIAN_POINT('Ctrl Pts',(-19.3449799461922,-41.5661325360465,
124.616011040601)) ;
#77444=CARTESIAN_POINT('Ctrl Pts',(-19.5912951011669,-41.7561108917333,
124.908434150121)) ;
#77445=CARTESIAN_POINT('Ctrl Pts',(-19.554878426075,-41.5761218113145,124.609111482984)) ;
#77446=CARTESIAN_POINT('Ctrl Pts',(-19.849396039096,-41.7661523499028,124.853543537004)) ;
#77447=CARTESIAN_POINT('Ctrl Pts',(-19.7613596181265,-41.586163269484,124.565200709918)) ;
#77448=CARTESIAN_POINT('Ctrl Pts',(-20.0891213276133,-41.7759838136911,
124.75717410497)) ;
#77449=CARTESIAN_POINT('Ctrl Pts',(-19.9531398219293,-41.5959947332723,
124.488107167589)) ;
#77450=CARTESIAN_POINT('Ctrl Pts',(-20.3126159521527,-41.785988745995,124.618753527339)) ;
#77451=CARTESIAN_POINT('Ctrl Pts',(-20.1319364892421,-41.6059996655762,
124.377372384104)) ;
#77452=CARTESIAN_POINT('Ctrl Pts',(-20.5082790001234,-41.7959751098897,
124.443796510955)) ;
#77453=CARTESIAN_POINT('Ctrl Pts',(-20.2884681052533,-41.615986029471,124.237408279578)) ;
#77454=CARTESIAN_POINT('Ctrl Pts',(-20.671089662106,-41.8060047387756,124.236556568572)) ;
#77455=CARTESIAN_POINT('Ctrl Pts',(-20.4187181302531,-41.6260156583568,
124.071617471286)) ;
#77456=CARTESIAN_POINT('Ctrl Pts',(-20.7938478464056,-41.815879960884,124.007888084139)) ;
#77457=CARTESIAN_POINT('Ctrl Pts',(-20.5169261213944,-41.6358908804652,
123.88868407081)) ;
#77458=CARTESIAN_POINT('Ctrl Pts',(-20.87634772346,-41.8258811732811,123.758394357576)) ;
#77459=CARTESIAN_POINT('Ctrl Pts',(-20.5829278694143,-41.6458920928623,
123.689089793448)) ;
#77460=CARTESIAN_POINT('Ctrl Pts',(-20.9141799975385,-41.8357897525166,
123.500723797929)) ;
#77461=CARTESIAN_POINT('Ctrl Pts',(-20.6131956146695,-41.6558006720979,
123.482954012209)) ;
#77462=CARTESIAN_POINT('Ctrl Pts',(-20.9065096443948,-41.8458446050726,
123.236647196733)) ;
#77463=CARTESIAN_POINT('Ctrl Pts',(-20.607061323779,-41.6658555246539,123.271692585024)) ;
#77464=CARTESIAN_POINT('Ctrl Pts',(-20.854419806544,-41.8557031873474,122.982817801562)) ;
#77465=CARTESIAN_POINT('Ctrl Pts',(-20.5653915448547,-41.6757141069286,
123.068629169974)) ;
#77466=CARTESIAN_POINT('Ctrl Pts',(-20.7572019523048,-41.86577131679,122.736787999783)) ;
#77467=CARTESIAN_POINT('Ctrl Pts',(-20.4876191232104,-41.6857822363713,
122.871804461378)) ;
#77468=CARTESIAN_POINT('Ctrl Pts',(-20.6216170476979,-41.8756267884792,
122.516096462848)) ;
#77469=CARTESIAN_POINT('Ctrl Pts',(-20.3791532034229,-41.6956377080604,
122.695250586501)) ;
#77470=CARTESIAN_POINT('Ctrl Pts',(-20.4479526498512,-41.8856216368654,
122.319060072971)) ;
#77471=CARTESIAN_POINT('Ctrl Pts',(-20.2402233360119,-41.7056325564467,
122.537620125504)) ;
#77472=CARTESIAN_POINT('Ctrl Pts',(-20.241600860006,-41.8956529336499,122.155008415719)) ;
#77473=CARTESIAN_POINT('Ctrl Pts',(-20.0751431938009,-41.7156638532311,
122.406377179865)) ;
#77474=CARTESIAN_POINT('Ctrl Pts',(-20.0138985646959,-41.90551946986,122.030978291857)) ;
#77475=CARTESIAN_POINT('Ctrl Pts',(-19.8929827296992,-41.7255303894412,
122.307151422635)) ;
#77476=CARTESIAN_POINT('Ctrl Pts',(-19.7652803950065,-41.9155068928208,
121.946967065422)) ;
#77477=CARTESIAN_POINT('Ctrl Pts',(-19.6940889763465,-41.7355178124021,
122.23994043297)) ;
#77478=CARTESIAN_POINT('Ctrl Pts',(-19.5069103967406,-41.9254518318406,
121.907424800188)) ;
#77479=CARTESIAN_POINT('Ctrl Pts',(-19.4873934887718,-41.7454627514218,
122.208304514196)) ;
#77480=CARTESIAN_POINT('Ctrl Pts',(-19.2430300937738,-41.9354967177006,
121.913529164993)) ;
#77481=CARTESIAN_POINT('Ctrl Pts',(-19.2762891837712,-41.7555076372818,
122.213185853992)) ;
#77482=CARTESIAN_POINT('Ctrl Pts',(-18.9887092821682,-41.9453652527868,
121.964316287539)) ;
#77483=CARTESIAN_POINT('Ctrl Pts',(-19.072832435962,-41.7653761723681,122.253813365681)) ;
#77484=CARTESIAN_POINT('Ctrl Pts',(-18.7444398718254,-41.9553311207935,
122.058732418044)) ;
#77485=CARTESIAN_POINT('Ctrl Pts',(-18.8774162150229,-41.7753420403747,
122.329344164061)) ;
#77486=CARTESIAN_POINT('Ctrl Pts',(-18.5191258959852,-41.965353768246,122.195167959757)) ;
#77487=CARTESIAN_POINT('Ctrl Pts',(-18.6971639262968,-41.7853646878272,
122.438490705683)) ;
#77488=CARTESIAN_POINT('Ctrl Pts',(-18.3228580657316,-41.9752774072536,
122.366864085239)) ;
#77489=CARTESIAN_POINT('Ctrl Pts',(-18.5401483567963,-41.7952883268348,
122.575845826025)) ;
#77490=CARTESIAN_POINT('Ctrl Pts',(-18.1585632396792,-41.9852201322593,
122.570050124115)) ;
#77491=CARTESIAN_POINT('Ctrl Pts',(-18.4087108446553,-41.8052310518406,
122.738393149906)) ;
#77492=CARTESIAN_POINT('Ctrl Pts',(-18.0310264116148,-41.9952657383112,
122.801169420602)) ;
#77493=CARTESIAN_POINT('Ctrl Pts',(-18.3066794495729,-41.8152766578924,
122.923287501502)) ;
#77494=CARTESIAN_POINT('Ctrl Pts',(-17.946842431743,-42.0051271608323,123.04628607553)) ;
#77495=CARTESIAN_POINT('Ctrl Pts',(-18.2393302260419,-41.8251380804135,
123.119379900334)) ;
#77496=CARTESIAN_POINT('Ctrl Pts',(-17.905523159314,-42.0151207292815,123.305597710685)) ;
#77497=CARTESIAN_POINT('Ctrl Pts',(-18.2062726013886,-41.8351316488627,
123.326828797274)) ;
#77498=CARTESIAN_POINT('Ctrl Pts',(-17.9096925518551,-42.0250462000368,
123.56643384869)) ;
#77499=CARTESIAN_POINT('Ctrl Pts',(-18.2096058544786,-41.845057119618,123.535497626538)) ;
#77500=CARTESIAN_POINT('Ctrl Pts',(-17.959571383868,-42.0350738739927,123.825153894788)) ;
#77501=CARTESIAN_POINT('Ctrl Pts',(-18.2495067533621,-41.8550847935739,
123.742474085264)) ;
#77502=CARTESIAN_POINT('Ctrl Pts',(-18.0520856876344,-42.0449610520343,
124.067987197521)) ;
#77503=CARTESIAN_POINT('Ctrl Pts',(-18.3235158644063,-41.8649719716156,
123.93674127071)) ;
#77504=CARTESIAN_POINT('Ctrl Pts',(-18.1870669887321,-42.0549894314025,
124.294288291732)) ;
#77505=CARTESIAN_POINT('Ctrl Pts',(-18.4314996700195,-41.8750003509838,
124.117783890498)) ;
#77506=CARTESIAN_POINT('Ctrl Pts',(-18.3569254896537,-42.064883674124,124.491191504036)) ;
#77507=CARTESIAN_POINT('Ctrl Pts',(-18.5673820062169,-41.8848945937052,
124.275305521873)) ;
#77508=CARTESIAN_POINT('Ctrl Pts',(-18.6285705557633,-42.0782365907749,
124.7132697805)) ;
#77509=CARTESIAN_POINT('Ctrl Pts',(-18.7847096513815,-41.8982475103561,
124.452982209414)) ;
#77510=CARTESIAN_POINT('Ctrl Pts',(-18.9483775262574,-42.0914391085216,
124.857795814256)) ;
#77511=CARTESIAN_POINT('Ctrl Pts',(-19.0405786175282,-41.9114500281029,
124.568605567899)) ;
#77512=CARTESIAN_POINT('Ctrl Pts',(-19.2946442504988,-42.1047950138026,
124.914924015867)) ;
#77513=CARTESIAN_POINT('Ctrl Pts',(-19.3175485758015,-41.9248059333838,
124.614299551762)) ;
#77514=CARTESIAN_POINT('Ctrl Pts',(-19.5547381910692,-42.1146916624404,
124.912293117232)) ;
#77515=CARTESIAN_POINT('Ctrl Pts',(-19.5256324094928,-41.9347025820217,
124.612199382613)) ;
#77516=CARTESIAN_POINT('Ctrl Pts',(-19.8142993016443,-42.1247398004929,
124.86390602354)) ;
#77517=CARTESIAN_POINT('Ctrl Pts',(-19.7332792909241,-41.9447507200741,
124.573491312428)) ;
#77518=CARTESIAN_POINT('Ctrl Pts',(-20.0576759369306,-42.1346307606706,
124.772616402123)) ;
#77519=CARTESIAN_POINT('Ctrl Pts',(-19.9279820995287,-41.9546416802519,
124.500461812852)) ;
#77520=CARTESIAN_POINT('Ctrl Pts',(-20.2841432703892,-42.1446235965474,
124.639664036418)) ;
#77521=CARTESIAN_POINT('Ctrl Pts',(-20.1091567936653,-41.9646345161287,
124.394101924367)) ;
#77522=CARTESIAN_POINT('Ctrl Pts',(-20.4846006079206,-42.154662691549,124.468172605325)) ;
#77523=CARTESIAN_POINT('Ctrl Pts',(-20.269524451752,-41.9746736111302,124.256910062148)) ;
#77524=CARTESIAN_POINT('Ctrl Pts',(-20.6493590678742,-42.1645000474001,
124.268925825655)) ;
#77525=CARTESIAN_POINT('Ctrl Pts',(-20.4013316292031,-41.9845109669814,
124.097515752566)) ;
#77526=CARTESIAN_POINT('Ctrl Pts',(-20.8232941424942,-42.1778929953309,
123.963015567202)) ;
#77527=CARTESIAN_POINT('Ctrl Pts',(-20.5404892049295,-41.9979039149121,
123.85277973288)) ;
#77528=CARTESIAN_POINT('Ctrl Pts',(-20.9119427187392,-42.1910596717578,
123.624389608239)) ;
#77529=CARTESIAN_POINT('Ctrl Pts',(-20.6114090656495,-42.0110705913391,
123.581847590379)) ;
#77530=CARTESIAN_POINT('Ctrl Pts',(-20.9103198255733,-42.2044444531646,
123.272710611948)) ;
#77531=CARTESIAN_POINT('Ctrl Pts',(-20.6101088464383,-42.0244553727458,
123.300551791675)) ;
#77532=CARTESIAN_POINT('Ctrl Pts',(-20.8642332430024,-42.2143062358084,
123.017641919744)) ;
#77533=CARTESIAN_POINT('Ctrl Pts',(-20.5732425041568,-42.0343171553897,
123.096486611068)) ;
#77534=CARTESIAN_POINT('Ctrl Pts',(-20.773744130429,-42.2243053837615,122.771002649434)) ;
#77535=CARTESIAN_POINT('Ctrl Pts',(-20.5008532527009,-42.0443163033428,
122.899177173043)) ;
#77536=CARTESIAN_POINT('Ctrl Pts',(-20.6432311627546,-42.2342081763786,
122.545797674222)) ;
#77537=CARTESIAN_POINT('Ctrl Pts',(-20.3964433972298,-42.0542190959598,
122.71901073462)) ;
#77538=CARTESIAN_POINT('Ctrl Pts',(-20.4731343577762,-42.2442577562695,
122.343862138683)) ;
#77539=CARTESIAN_POINT('Ctrl Pts',(-20.2603721024993,-42.0642686758508,
122.557463185732)) ;
#77540=CARTESIAN_POINT('Ctrl Pts',(-20.2076003347488,-42.257444830079,122.1209956095)) ;
#77541=CARTESIAN_POINT('Ctrl Pts',(-20.0479240767754,-42.0774557496602,
122.379158188714)) ;
#77542=CARTESIAN_POINT('Ctrl Pts',(-19.804126587412,-42.2741976200502,121.933081385901)) ;
#77543=CARTESIAN_POINT('Ctrl Pts',(-19.7251863995672,-42.0942085396314,
122.228834129982)) ;
#77544=CARTESIAN_POINT('Ctrl Pts',(-19.3673812946802,-42.2906862721449,
121.894819463431)) ;
#77545=CARTESIAN_POINT('Ctrl Pts',(-19.3757249718531,-42.1106971917261,
122.198219603723)) ;
#77546=CARTESIAN_POINT('Ctrl Pts',(-19.0216618584833,-42.3040430983283,
121.955010873932)) ;
#77547=CARTESIAN_POINT('Ctrl Pts',(-19.0992014122385,-42.1240540179095,
122.246369156977)) ;
#77548=CARTESIAN_POINT('Ctrl Pts',(-18.7769948828995,-42.3139394832062,
122.043336388538)) ;
#77549=CARTESIAN_POINT('Ctrl Pts',(-18.9034558730959,-42.1339504027875,
122.31702867763)) ;
#77550=CARTESIAN_POINT('Ctrl Pts',(-18.5489107992709,-42.3239459977267,
122.174062497351)) ;
#77551=CARTESIAN_POINT('Ctrl Pts',(-18.7209920470431,-42.1439569173079,
122.421605740756)) ;
#77552=CARTESIAN_POINT('Ctrl Pts',(-18.2820313955466,-42.3371361212431,
122.395439854846)) ;
#77553=CARTESIAN_POINT('Ctrl Pts',(-18.5074779287399,-42.1571470408243,
122.598716881194)) ;
#77554=CARTESIAN_POINT('Ctrl Pts',(-18.0248416306268,-42.3539026823926,
122.759167368736)) ;
#77555=CARTESIAN_POINT('Ctrl Pts',(-18.3017330244153,-42.1739136019739,
122.889684714368)) ;
#77556=CARTESIAN_POINT('Ctrl Pts',(-17.8860485150125,-42.3736871711007,
123.266512292207)) ;
#77557=CARTESIAN_POINT('Ctrl Pts',(-18.190691850351,-42.1936980906819,123.295564709079)) ;
#77558=CARTESIAN_POINT('Ctrl Pts',(-17.9274046620384,-42.3936326186972,
123.79488101199)) ;
#77559=CARTESIAN_POINT('Ctrl Pts',(-18.2237744875469,-42.2136435382784,
123.718259302305)) ;
#77560=CARTESIAN_POINT('Ctrl Pts',(-18.1467300052085,-42.4135442808531,
124.276525573027)) ;
#77561=CARTESIAN_POINT('Ctrl Pts',(-18.3992319711091,-42.2335552004343,
124.103577050796)) ;
#77562=CARTESIAN_POINT('Ctrl Pts',(-18.5161004763007,-42.433436472872,124.654913018511)) ;
#77563=CARTESIAN_POINT('Ctrl Pts',(-18.6947270610426,-42.2534473924532,
124.40628936176)) ;
#77564=CARTESIAN_POINT('Ctrl Pts',(-18.9961947812733,-42.4534776034266,
124.885472692645)) ;
#77565=CARTESIAN_POINT('Ctrl Pts',(-19.0788009536354,-42.2734885230078,
124.590739459069)) ;
#77566=CARTESIAN_POINT('Ctrl Pts',(-19.5204288936145,-42.4732959380422,
124.938073342038)) ;
#77567=CARTESIAN_POINT('Ctrl Pts',(-19.4981894659672,-42.2933068576234,
124.632822663084)) ;
#77568=CARTESIAN_POINT('Ctrl Pts',(-20.0350303911452,-42.4932685032617,
124.808520139726)) ;
#77569=CARTESIAN_POINT('Ctrl Pts',(-19.9098714983823,-42.313279422843,124.529182116314)) ;
#77570=CARTESIAN_POINT('Ctrl Pts',(-20.4730875843371,-42.5131577194334,
124.512279231731)) ;
#77571=CARTESIAN_POINT('Ctrl Pts',(-20.2603191389922,-42.3331686390146,
124.292190423348)) ;
#77572=CARTESIAN_POINT('Ctrl Pts',(-20.7853676285857,-42.5331812937561,
124.081500341459)) ;
#77573=CARTESIAN_POINT('Ctrl Pts',(-20.510144598529,-42.3531922133373,123.947568642154)) ;
#77574=CARTESIAN_POINT('Ctrl Pts',(-20.930672852745,-42.5529784568443,123.575689148446)) ;
#77575=CARTESIAN_POINT('Ctrl Pts',(-20.6263909037281,-42.3729893764256,
123.542918090147)) ;
#77576=CARTESIAN_POINT('Ctrl Pts',(-20.89563526975,-42.5729439506681,123.046309019456)) ;
#77577=CARTESIAN_POINT('Ctrl Pts',(-20.5983617160724,-42.3929548702494,
123.119413476898)) ;
#77578=CARTESIAN_POINT('Ctrl Pts',(-20.6814765720691,-42.5928976584095,
122.560980844354)) ;
#77579=CARTESIAN_POINT('Ctrl Pts',(-20.4270354944749,-42.4129085779908,
122.731150136192)) ;
#77580=CARTESIAN_POINT('Ctrl Pts',(-20.3156068294738,-42.6128050351361,
122.178926648518)) ;
#77581=CARTESIAN_POINT('Ctrl Pts',(-20.1343395078316,-42.4328159547174,
122.425505382769)) ;
#77582=CARTESIAN_POINT('Ctrl Pts',(-19.8430795028779,-42.6326572466847,
121.943950043766)) ;
#77583=CARTESIAN_POINT('Ctrl Pts',(-19.7563159223275,-42.4526681662659,
122.237523311971)) ;
#77584=CARTESIAN_POINT('Ctrl Pts',(-19.3129641321362,-42.6527296336304,
121.884197616133)) ;
#77585=CARTESIAN_POINT('Ctrl Pts',(-19.3322245789558,-42.4727405532116,
122.189721484159)) ;
#77586=CARTESIAN_POINT('Ctrl Pts',(-18.8004818960258,-42.6725675032707,
122.008159119994)) ;
#77587=CARTESIAN_POINT('Ctrl Pts',(-18.9222366927177,-42.4925784228519,
122.288891090315)) ;
#77588=CARTESIAN_POINT('Ctrl Pts',(-18.3595239815555,-42.6924181578238,
122.297834685057)) ;
#77589=CARTESIAN_POINT('Ctrl Pts',(-18.5694695547567,-42.5124290774051,
122.52063348008)) ;
#77590=CARTESIAN_POINT('Ctrl Pts',(-18.0413332377422,-42.7124700921642,
122.72531992571)) ;
#77591=CARTESIAN_POINT('Ctrl Pts',(-18.3149181158026,-42.5324810117455,
122.862621797376)) ;
#77592=CARTESIAN_POINT('Ctrl Pts',(-17.8898151801749,-42.7323032797303,
123.230332622457)) ;
#77593=CARTESIAN_POINT('Ctrl Pts',(-18.1937042468816,-42.5523141993116,
123.266634019015)) ;
#77594=CARTESIAN_POINT('Ctrl Pts',(-17.9188018274487,-42.752232491961,123.759028000025)) ;
#77595=CARTESIAN_POINT('Ctrl Pts',(-18.2168953694706,-42.5722434115422,
123.689590983492)) ;
#77596=CARTESIAN_POINT('Ctrl Pts',(-18.1255818945202,-42.7721174571754,
124.245626671877)) ;
#77597=CARTESIAN_POINT('Ctrl Pts',(-18.3823217704082,-42.5921283767566,
124.078870010309)) ;
#77598=CARTESIAN_POINT('Ctrl Pts',(-18.4898112909711,-42.79219119832,124.635336040319)) ;
#77599=CARTESIAN_POINT('Ctrl Pts',(-18.6737062691616,-42.6122021179012,
124.390635650376)) ;
#77600=CARTESIAN_POINT('Ctrl Pts',(-18.9586591559989,-42.8119843801004,
124.874120892194)) ;
#77601=CARTESIAN_POINT('Ctrl Pts',(-19.0487871981899,-42.6319952996816,
124.581662463708)) ;
#77602=CARTESIAN_POINT('Ctrl Pts',(-19.4849952307076,-42.8319470881031,
124.94071639769)) ;
#77603=CARTESIAN_POINT('Ctrl Pts',(-19.4698566611138,-42.6519580076843,
124.634936088449)) ;
#77604=CARTESIAN_POINT('Ctrl Pts',(-20.0027532085584,-42.8519300398455,
124.822320272829)) ;
#77605=CARTESIAN_POINT('Ctrl Pts',(-19.8840626043544,-42.6719409594268,
124.540216680374)) ;
#77606=CARTESIAN_POINT('Ctrl Pts',(-20.4457748039355,-42.8717406596177,
124.537685736261)) ;
#77607=CARTESIAN_POINT('Ctrl Pts',(-20.2384794300186,-42.6917515791989,
124.312505791514)) ;
#77608=CARTESIAN_POINT('Ctrl Pts',(-20.7682626055725,-42.8917243756506,
124.115808826905)) ;
#77609=CARTESIAN_POINT('Ctrl Pts',(-20.496467127968,-42.7117352952318,123.975002213064)) ;
#77610=CARTESIAN_POINT('Ctrl Pts',(-20.9266062653621,-42.9116058395479,
123.611535793614)) ;
#77611=CARTESIAN_POINT('Ctrl Pts',(-20.6231390533387,-42.7316167591292,
123.571582135576)) ;
#77612=CARTESIAN_POINT('Ctrl Pts',(-20.9036603573347,-42.9315611693923,
123.081759157347)) ;
#77613=CARTESIAN_POINT('Ctrl Pts',(-20.6047789224965,-42.7515720889735,
123.147760755325)) ;
#77614=CARTESIAN_POINT('Ctrl Pts',(-20.7024014511909,-42.9514366301977,
122.593252469711)) ;
#77615=CARTESIAN_POINT('Ctrl Pts',(-20.4437676559676,-42.771447549779,122.756956211372)) ;
#77616=CARTESIAN_POINT('Ctrl Pts',(-20.3449003201924,-42.9714209502493,
122.200502446614)) ;
#77617=CARTESIAN_POINT('Ctrl Pts',(-20.1577657851218,-42.7914318698305,
122.442758885575)) ;
#77618=CARTESIAN_POINT('Ctrl Pts',(-19.8758679528794,-42.9913489830389,
121.954198379495)) ;
#77619=CARTESIAN_POINT('Ctrl Pts',(-19.7825308096546,-42.8113599026202,
122.24571839476)) ;
#77620=CARTESIAN_POINT('Ctrl Pts',(-19.4385731677938,-43.0079577449787,
121.894584975547)) ;
#77621=CARTESIAN_POINT('Ctrl Pts',(-19.4327162628233,-42.82796866456,122.198032510649)) ;
#77622=CARTESIAN_POINT('Ctrl Pts',(-19.0946716816844,-43.0211453836688,
121.937615803006)) ;
#77623=CARTESIAN_POINT('Ctrl Pts',(-19.1575750804821,-42.84115630325,122.232458887897)) ;
#77624=CARTESIAN_POINT('Ctrl Pts',(-18.8437153065947,-43.0311318180289,
122.014331379979)) ;
#77625=CARTESIAN_POINT('Ctrl Pts',(-18.9568164411077,-42.8511427376102,
122.293831610718)) ;
#77626=CARTESIAN_POINT('Ctrl Pts',(-18.6094527008609,-43.0411411919883,
122.133980200426)) ;
#77627=CARTESIAN_POINT('Ctrl Pts',(-18.7693988622901,-42.8611521115695,
122.38956024232)) ;
#77628=CARTESIAN_POINT('Ctrl Pts',(-18.3305857336054,-43.0544312255535,
122.344252306503)) ;
#77629=CARTESIAN_POINT('Ctrl Pts',(-18.5463444103637,-42.8744421451348,
122.55774111295)) ;
#77630=CARTESIAN_POINT('Ctrl Pts',(-18.058791901131,-43.071025213216,122.691613440091)) ;
#77631=CARTESIAN_POINT('Ctrl Pts',(-18.3288675517154,-42.8910361327973,
122.835684012626)) ;
#77632=CARTESIAN_POINT('Ctrl Pts',(-17.9215463023581,-43.0876574684915,
123.111805423994)) ;
#77633=CARTESIAN_POINT('Ctrl Pts',(-18.2190954252728,-42.9076683880728,
123.171796586433)) ;
#77634=CARTESIAN_POINT('Ctrl Pts',(-17.9026645542889,-43.1008998521594,
123.459298795026)) ;
#77635=CARTESIAN_POINT('Ctrl Pts',(-18.203983606276,-42.9209107717406,123.449819411052)) ;
#77636=CARTESIAN_POINT('Ctrl Pts',(-17.933115438378,-43.1108140603868,123.718057560293)) ;
#77637=CARTESIAN_POINT('Ctrl Pts',(-18.2283482599857,-42.9308249799681,
123.656820588526)) ;
#77638=CARTESIAN_POINT('Ctrl Pts',(-18.0093888247414,-43.1208706996585,
123.971069080724)) ;
#77639=CARTESIAN_POINT('Ctrl Pts',(-18.2893690473881,-42.9408816192397,
123.859230933456)) ;
#77640=CARTESIAN_POINT('Ctrl Pts',(-18.1256799000597,-43.1307165060786,
124.202224696473)) ;
#77641=CARTESIAN_POINT('Ctrl Pts',(-18.3824021684236,-42.9507274256599,
124.044152714525)) ;
#77642=CARTESIAN_POINT('Ctrl Pts',(-18.2830849970075,-43.1407615057118,
124.414117164537)) ;
#77643=CARTESIAN_POINT('Ctrl Pts',(-18.5083351697391,-42.960772425293,124.21367093415)) ;
#77644=CARTESIAN_POINT('Ctrl Pts',(-18.5370432518798,-43.1540425280845,
124.653504054307)) ;
#77645=CARTESIAN_POINT('Ctrl Pts',(-18.7114678288813,-42.9740534476658,
124.405150550178)) ;
#77646=CARTESIAN_POINT('Ctrl Pts',(-18.8452649773072,-43.1672399746092,
124.820961905298)) ;
#77647=CARTESIAN_POINT('Ctrl Pts',(-18.9580634355738,-42.9872508941904,
124.539134958599)) ;
#77648=CARTESIAN_POINT('Ctrl Pts',(-19.1881152199905,-43.1806542724161,
124.902985566074)) ;
#77649=CARTESIAN_POINT('Ctrl Pts',(-19.232360308715,-43.0006651919974,124.604753983446)) ;
#77650=CARTESIAN_POINT('Ctrl Pts',(-19.4462101896767,-43.1904933378189,
124.918723959431)) ;
#77651=CARTESIAN_POINT('Ctrl Pts',(-19.4388332239247,-43.0105042574002,
124.617341843955)) ;
#77652=CARTESIAN_POINT('Ctrl Pts',(-19.70691664246,-43.2004765440966,124.889671060907)) ;
#77653=CARTESIAN_POINT('Ctrl Pts',(-19.6473989352599,-43.0204874636778,
124.594097446698)) ;
#77654=CARTESIAN_POINT('Ctrl Pts',(-19.9578281238574,-43.2104277790094,
124.815931888738)) ;
#77655=CARTESIAN_POINT('Ctrl Pts',(-19.8481272005172,-43.0304386985906,
124.535103914391)) ;
#77656=CARTESIAN_POINT('Ctrl Pts',(-20.1934350690433,-43.220428778711,124.699450982001)) ;
#77657=CARTESIAN_POINT('Ctrl Pts',(-20.0366117625381,-43.0404396982923,
124.441917204073)) ;
#77658=CARTESIAN_POINT('Ctrl Pts',(-20.4056235279115,-43.2304601244984,
124.543033701411)) ;
#77659=CARTESIAN_POINT('Ctrl Pts',(-20.206361135427,-43.0504710440796,124.316781584499)) ;
#77660=CARTESIAN_POINT('Ctrl Pts',(-20.5844761556789,-43.2403138892034,
124.355767995635)) ;
#77661=CARTESIAN_POINT('Ctrl Pts',(-20.3494415434613,-43.0603248087846,
124.166967530126)) ;
#77662=CARTESIAN_POINT('Ctrl Pts',(-20.7303004788891,-43.2502845428717,
124.138111587117)) ;
#77663=CARTESIAN_POINT('Ctrl Pts',(-20.4660990801308,-43.0702954624529,
123.992841228193)) ;
#77664=CARTESIAN_POINT('Ctrl Pts',(-20.8364178790176,-43.2602817865289,
123.897736472971)) ;
#77665=CARTESIAN_POINT('Ctrl Pts',(-20.5509909214164,-43.0802927061101,
123.800540288638)) ;
#77666=CARTESIAN_POINT('Ctrl Pts',(-20.8990697974947,-43.270315242473,123.641641842378)) ;
#77667=CARTESIAN_POINT('Ctrl Pts',(-20.6011102563004,-43.0903261620543,
123.595664077152)) ;
#77668=CARTESIAN_POINT('Ctrl Pts',(-20.9164201485292,-43.2801707467735,
123.38320598339)) ;
#77669=CARTESIAN_POINT('Ctrl Pts',(-20.6149882875894,-43.1001816663547,
123.388915428103)) ;
#77670=CARTESIAN_POINT('Ctrl Pts',(-20.8885847143256,-43.2901701830595,
123.121956715694)) ;
#77671=CARTESIAN_POINT('Ctrl Pts',(-20.5927177264753,-43.1101811026408,
123.17991632247)) ;
#77672=CARTESIAN_POINT('Ctrl Pts',(-20.8168337006827,-43.3000646425755,
122.871985466919)) ;
#77673=CARTESIAN_POINT('Ctrl Pts',(-20.5353148477446,-43.1200755621567,
122.979940136269)) ;
#77674=CARTESIAN_POINT('Ctrl Pts',(-20.7007964615209,-43.3101277620271,
122.634405971044)) ;
#77675=CARTESIAN_POINT('Ctrl Pts',(-20.4424830472007,-43.1301386816084,
122.789877488713)) ;
#77676=CARTESIAN_POINT('Ctrl Pts',(-20.548903419078,-43.3199673964391,122.425092863754)) ;
#77677=CARTESIAN_POINT('Ctrl Pts',(-20.3209670269666,-43.1399783160204,
122.622428563072)) ;
#77678=CARTESIAN_POINT('Ctrl Pts',(-20.3590408300739,-43.3300306039249,
122.241063679027)) ;
#77679=CARTESIAN_POINT('Ctrl Pts',(-20.1690754107749,-43.1500415235061,
122.475206756355)) ;
#77680=CARTESIAN_POINT('Ctrl Pts',(-20.1436111274477,-43.3399247113041,
122.095429795612)) ;
#77681=CARTESIAN_POINT('Ctrl Pts',(-19.9967306388888,-43.1599356308853,
122.358701616965)) ;
#77682=CARTESIAN_POINT('Ctrl Pts',(-19.9053553865349,-43.3498670434965,
121.988285686003)) ;
#77683=CARTESIAN_POINT('Ctrl Pts',(-19.8061253596654,-43.1698779630777,
122.272988371083)) ;
#77684=CARTESIAN_POINT('Ctrl Pts',(-19.6505873376489,-43.3598676698115,
121.923617759832)) ;
#77685=CARTESIAN_POINT('Ctrl Pts',(-19.6023104651923,-43.1798785893927,
122.221256110046)) ;
#77686=CARTESIAN_POINT('Ctrl Pts',(-19.387412643394,-43.3699094040934,121.904584247436)) ;
#77687=CARTESIAN_POINT('Ctrl Pts',(-19.391770525899,-43.1899203236746,122.206031467427)) ;
#77688=CARTESIAN_POINT('Ctrl Pts',(-19.1304837624311,-43.3797348300425,
121.930388446554)) ;
#77689=CARTESIAN_POINT('Ctrl Pts',(-19.1862281367957,-43.1997457496237,
122.226676884756)) ;
#77690=CARTESIAN_POINT('Ctrl Pts',(-18.8760169234249,-43.3897916565701,
122.001672515935)) ;
#77691=CARTESIAN_POINT('Ctrl Pts',(-18.9826551632411,-43.2098025761514,
122.283706165014)) ;
#77692=CARTESIAN_POINT('Ctrl Pts',(-18.6409865992332,-43.3997190896917,
122.11493089705)) ;
#77693=CARTESIAN_POINT('Ctrl Pts',(-18.7946320604858,-43.219730009273,122.374314665372)) ;
#77694=CARTESIAN_POINT('Ctrl Pts',(-18.4282774407741,-43.4096690820979,
122.26701392931)) ;
#77695=CARTESIAN_POINT('Ctrl Pts',(-18.6244661072569,-43.2296800016792,
122.495982618452)) ;
#77696=CARTESIAN_POINT('Ctrl Pts',(-18.2436237168823,-43.4197242831719,
122.456000772631)) ;
#77697=CARTESIAN_POINT('Ctrl Pts',(-18.4767445661238,-43.2397352027532,
122.647173618493)) ;
#77698=CARTESIAN_POINT('Ctrl Pts',(-18.0976352136823,-43.4295465572242,
122.668893815901)) ;
#77699=CARTESIAN_POINT('Ctrl Pts',(-18.3599557989295,-43.2495574768055,
122.817488687827)) ;
#77700=CARTESIAN_POINT('Ctrl Pts',(-17.9878760753137,-43.4396024511835,
122.90925930799)) ;
#77701=CARTESIAN_POINT('Ctrl Pts',(-18.272150254971,-43.2596133707647,123.009781985742)) ;
#77702=CARTESIAN_POINT('Ctrl Pts',(-17.9227225616892,-43.4495431730286,
123.162245934155)) ;
#77703=CARTESIAN_POINT('Ctrl Pts',(-18.2200294874287,-43.2695540926099,
123.212171536294)) ;
#77704=CARTESIAN_POINT('Ctrl Pts',(-17.9017472035659,-43.4594475171152,
123.421680109374)) ;
#77705=CARTESIAN_POINT('Ctrl Pts',(-18.2032511636437,-43.2794584366965,
123.41971860684)) ;
#77706=CARTESIAN_POINT('Ctrl Pts',(-17.9266517283389,-43.4694941844147,
123.684496298944)) ;
#77707=CARTESIAN_POINT('Ctrl Pts',(-18.2231767399461,-43.2895051039959,
123.629971456514)) ;
#77708=CARTESIAN_POINT('Ctrl Pts',(-17.9955444786617,-43.4793897428646,
123.935293204417)) ;
#77709=CARTESIAN_POINT('Ctrl Pts',(-18.2782926706353,-43.2994006624459,
123.830608021522)) ;
#77710=CARTESIAN_POINT('Ctrl Pts',(-18.1087774585217,-43.4894518215693,
124.174200467504)) ;
#77711=CARTESIAN_POINT('Ctrl Pts',(-18.3688808575243,-43.3094627411505,
124.021733139343)) ;
#77712=CARTESIAN_POINT('Ctrl Pts',(-18.2583544804656,-43.4992945200351,
124.385256639801)) ;
#77713=CARTESIAN_POINT('Ctrl Pts',(-18.4885436261305,-43.3193054396163,
124.19057641101)) ;
#77714=CARTESIAN_POINT('Ctrl Pts',(-18.4445910637564,-43.5092852939295,
124.570269448504)) ;
#77715=CARTESIAN_POINT('Ctrl Pts',(-18.6375340693141,-43.3292962135108,
124.338585274364)) ;
#77716=CARTESIAN_POINT('Ctrl Pts',(-18.6588280253522,-43.5192131631644,
124.719179491555)) ;
#77717=CARTESIAN_POINT('Ctrl Pts',(-18.8089243549263,-43.3392240827457,
124.457711595414)) ;
#77718=CARTESIAN_POINT('Ctrl Pts',(-18.8969249830117,-43.5292018921343,
124.829722059104)) ;
#77719=CARTESIAN_POINT('Ctrl Pts',(-18.9994025173376,-43.3492128117156,
124.546144008221)) ;
#77720=CARTESIAN_POINT('Ctrl Pts',(-19.1519853154848,-43.5392412941181,
124.897107997011)) ;
#77721=CARTESIAN_POINT('Ctrl Pts',(-19.2034513317484,-43.3592522136993,
124.600051019993)) ;
#77722=CARTESIAN_POINT('Ctrl Pts',(-19.4096395220042,-43.5490814618548,
124.919256070224)) ;
#77723=CARTESIAN_POINT('Ctrl Pts',(-19.4095740497206,-43.3690923814361,
124.617767680726)) ;
#77724=CARTESIAN_POINT('Ctrl Pts',(-19.6726790144128,-43.5591296722293,
124.896233588378)) ;
#77725=CARTESIAN_POINT('Ctrl Pts',(-19.6200056228297,-43.3791405918106,
124.599348022425)) ;
#77726=CARTESIAN_POINT('Ctrl Pts',(-19.9250688422625,-43.5690768425171,
124.828171804115)) ;
#77727=CARTESIAN_POINT('Ctrl Pts',(-19.8219167126913,-43.3890877620984,
124.544896996661)) ;
#77728=CARTESIAN_POINT('Ctrl Pts',(-20.1612764163258,-43.5789876907722,
124.718431010674)) ;
#77729=CARTESIAN_POINT('Ctrl Pts',(-20.0108816130576,-43.3989986103534,
124.457103131757)) ;
#77730=CARTESIAN_POINT('Ctrl Pts',(-20.3778135164168,-43.5890440184499,
124.566965650314)) ;
#77731=CARTESIAN_POINT('Ctrl Pts',(-20.1841104958632,-43.4090549380312,
124.335929390239)) ;
#77732=CARTESIAN_POINT('Ctrl Pts',(-20.5611126310766,-43.5988944312185,
124.384166137537)) ;
#77733=CARTESIAN_POINT('Ctrl Pts',(-20.3307480642774,-43.4189053507997,
124.189689229524)) ;
#77734=CARTESIAN_POINT('Ctrl Pts',(-20.7130674437035,-43.6089213170522,
124.168903399336)) ;
#77735=CARTESIAN_POINT('Ctrl Pts',(-20.4523107179373,-43.4289322366334,
124.017478157488)) ;
#77736=CARTESIAN_POINT('Ctrl Pts',(-20.8247441402527,-43.618949932683,123.930180059056)) ;
#77737=CARTESIAN_POINT('Ctrl Pts',(-20.5416506341111,-43.4389608522643,
123.82649874937)) ;
#77738=CARTESIAN_POINT('Ctrl Pts',(-20.8924859436322,-43.6287951560605,
123.680497788529)) ;
#77739=CARTESIAN_POINT('Ctrl Pts',(-20.5958423726042,-43.4488060756417,
123.626753399107)) ;
#77740=CARTESIAN_POINT('Ctrl Pts',(-20.9168945753088,-43.6387858381621,
123.419083293923)) ;
#77741=CARTESIAN_POINT('Ctrl Pts',(-20.6153678869585,-43.4587967577433,
123.417621830856)) ;
#77742=CARTESIAN_POINT('Ctrl Pts',(-20.8948561360982,-43.6488237267945,
123.15622317163)) ;
#77743=CARTESIAN_POINT('Ctrl Pts',(-20.5977356311787,-43.4688346463758,
123.207333751848)) ;
#77744=CARTESIAN_POINT('Ctrl Pts',(-20.8292438814433,-43.6586680618977,
122.905971997086)) ;
#77745=CARTESIAN_POINT('Ctrl Pts',(-20.5452447033601,-43.4786789814789,
123.00713407774)) ;
#77746=CARTESIAN_POINT('Ctrl Pts',(-20.7201211840923,-43.6686530240952,
122.667383970139)) ;
#77747=CARTESIAN_POINT('Ctrl Pts',(-20.4579454445687,-43.4886639436764,
122.816264379379)) ;
#77748=CARTESIAN_POINT('Ctrl Pts',(-20.5719738573376,-43.6785919656286,
122.452232949028)) ;
#77749=CARTESIAN_POINT('Ctrl Pts',(-20.3394267805854,-43.4986028852098,
122.644144644649)) ;
#77750=CARTESIAN_POINT('Ctrl Pts',(-20.3868068905276,-43.6886338506,122.264249292285)) ;
#77751=CARTESIAN_POINT('Ctrl Pts',(-20.1912922023766,-43.5086447701812,
122.493758541871)) ;
#77752=CARTESIAN_POINT('Ctrl Pts',(-20.175193466136,-43.6985203985083,122.113473137237)) ;
#77753=CARTESIAN_POINT('Ctrl Pts',(-20.0220013410477,-43.5185313180895,
122.373139073177)) ;
#77754=CARTESIAN_POINT('Ctrl Pts',(-19.9382875920077,-43.7085143240083,
122.000193047027)) ;
#77755=CARTESIAN_POINT('Ctrl Pts',(-19.8324762632877,-43.5285252435895,
122.282516123217)) ;
#77756=CARTESIAN_POINT('Ctrl Pts',(-19.6867374287738,-43.7184504151347,
121.930037797463)) ;
#77757=CARTESIAN_POINT('Ctrl Pts',(-19.631236272687,-43.538461334716,122.226393150879)) ;
#77758=CARTESIAN_POINT('Ctrl Pts',(-19.4244597082905,-43.7284796841147,
121.904445450398)) ;
#77759=CARTESIAN_POINT('Ctrl Pts',(-19.4214139225834,-43.5484906036959,
122.205920422987)) ;
#77760=CARTESIAN_POINT('Ctrl Pts',(-19.1654713412094,-43.738362066674,121.924160359711)) ;
#77761=CARTESIAN_POINT('Ctrl Pts',(-19.2142241183985,-43.5583729862552,
122.221693371168)) ;
#77762=CARTESIAN_POINT('Ctrl Pts',(-18.9095644693569,-43.7484145837619,
121.989548406025)) ;
#77763=CARTESIAN_POINT('Ctrl Pts',(-19.0094986897132,-43.5684255033431,
122.274004889728)) ;
#77764=CARTESIAN_POINT('Ctrl Pts',(-18.6725555427022,-43.7583087045857,
122.096577505289)) ;
#77765=CARTESIAN_POINT('Ctrl Pts',(-18.8198926461261,-43.578319624167,122.359628808823)) ;
#77766=CARTESIAN_POINT('Ctrl Pts',(-18.4541166119818,-43.7683706840062,
122.245521781362)) ;
#77767=CARTESIAN_POINT('Ctrl Pts',(-18.6451418602276,-43.5883816035874,
122.478785221664)) ;
#77768=CARTESIAN_POINT('Ctrl Pts',(-18.2688956918236,-43.7782152172351,
122.426149066482)) ;
#77769=CARTESIAN_POINT('Ctrl Pts',(-18.4969665901332,-43.5982261368164,
122.623287037953)) ;
#77770=CARTESIAN_POINT('Ctrl Pts',(-18.1153222214093,-43.7881752961414,
122.638095379922)) ;
#77771=CARTESIAN_POINT('Ctrl Pts',(-18.3741086705153,-43.6081862157226,
122.792844257825)) ;
#77772=CARTESIAN_POINT('Ctrl Pts',(-18.0004538038229,-43.798213572714,122.875554226938)) ;
#77773=CARTESIAN_POINT('Ctrl Pts',(-18.2822147043336,-43.6182244922952,
122.982811851236)) ;
#77774=CARTESIAN_POINT('Ctrl Pts',(-17.9292494151495,-43.8080869592518,
123.125095646761)) ;
#77775=CARTESIAN_POINT('Ctrl Pts',(-18.225252205665,-43.6280978788331,123.182444339761)) ;
#77776=CARTESIAN_POINT('Ctrl Pts',(-17.9020001551184,-43.8181599020189,
123.388344568529)) ;
#77777=CARTESIAN_POINT('Ctrl Pts',(-18.2034535746662,-43.6381708216001,
123.393043900429)) ;
#77778=CARTESIAN_POINT('Ctrl Pts',(-17.9200947061093,-43.8279813161472,
123.64585694239)) ;
#77779=CARTESIAN_POINT('Ctrl Pts',(-18.2179298642884,-43.6479922357285,
123.599052510802)) ;
#77780=CARTESIAN_POINT('Ctrl Pts',(-17.9839061110821,-43.8380559462195,
123.902752660062)) ;
#77781=CARTESIAN_POINT('Ctrl Pts',(-18.2689797188223,-43.6580668658008,
123.804569272354)) ;
#77782=CARTESIAN_POINT('Ctrl Pts',(-18.0892674356352,-43.8479225835364,
124.139701464769)) ;
#77783=CARTESIAN_POINT('Ctrl Pts',(-18.353269010714,-43.6679335031176,123.99412714447)) ;
#77784=CARTESIAN_POINT('Ctrl Pts',(-18.2358881550093,-43.8579461289082,
124.358516056975)) ;
#77785=CARTESIAN_POINT('Ctrl Pts',(-18.4705660406864,-43.6779570484894,
124.169178557313)) ;
#77786=CARTESIAN_POINT('Ctrl Pts',(-18.4187926357284,-43.8679718804254,
124.548170374681)) ;
#77787=CARTESIAN_POINT('Ctrl Pts',(-18.6168901651521,-43.6879828000066,
124.320901587011)) ;
#77788=CARTESIAN_POINT('Ctrl Pts',(-18.6279123308631,-43.8778254674347,
124.700856473508)) ;
#77789=CARTESIAN_POINT('Ctrl Pts',(-18.7841853999482,-43.697836387016,124.443049376181)) ;
#77790=CARTESIAN_POINT('Ctrl Pts',(-18.8629865023104,-43.8878024276627,
124.816974766351)) ;
#77791=CARTESIAN_POINT('Ctrl Pts',(-18.9722446774819,-43.7078133472439,
124.535943532528)) ;
#77792=CARTESIAN_POINT('Ctrl Pts',(-19.1158727505967,-43.8978235706912,
124.890405499209)) ;
#77793=CARTESIAN_POINT('Ctrl Pts',(-19.1745538313907,-43.7178344902724,
124.594687628449)) ;
#77794=CARTESIAN_POINT('Ctrl Pts',(-19.3740398930862,-43.9077061767111,
124.918943559818)) ;
#77795=CARTESIAN_POINT('Ctrl Pts',(-19.3810867133437,-43.7277170962923,
124.617517603467)) ;
#77796=CARTESIAN_POINT('Ctrl Pts',(-19.6380282810984,-43.9177746473438,
124.901808569006)) ;
#77797=CARTESIAN_POINT('Ctrl Pts',(-19.5922777253755,-43.737785566925,124.603809182427)) ;
#77798=CARTESIAN_POINT('Ctrl Pts',(-19.8891040806478,-43.9276047305275,
124.840852015911)) ;
#77799=CARTESIAN_POINT('Ctrl Pts',(-19.7931370891346,-43.7476156501087,
124.555043909552)) ;
#77800=CARTESIAN_POINT('Ctrl Pts',(-20.1315321755266,-43.9376712902079,
124.735084209489)) ;
#77801=CARTESIAN_POINT('Ctrl Pts',(-19.9870797585783,-43.7576822097891,
124.470429312396)) ;
#77802=CARTESIAN_POINT('Ctrl Pts',(-20.3480256593749,-43.947561540037,124.591215461455)) ;
#77803=CARTESIAN_POINT('Ctrl Pts',(-20.1602736880261,-43.7675724596183,
124.355334538994)) ;
#77804=CARTESIAN_POINT('Ctrl Pts',(-20.5385520108474,-43.9575537057859,
124.410544001572)) ;
#77805=CARTESIAN_POINT('Ctrl Pts',(-20.3126945474677,-43.7775646253671,
124.210797386208)) ;
#77806=CARTESIAN_POINT('Ctrl Pts',(-20.6941599748475,-43.967516549382,124.199999732242)) ;
#77807=CARTESIAN_POINT('Ctrl Pts',(-20.4371805360489,-43.7875274689632,
124.042362141687)) ;
#77808=CARTESIAN_POINT('Ctrl Pts',(-20.8107661786946,-43.9774207182097,
123.967284902369)) ;
#77809=CARTESIAN_POINT('Ctrl Pts',(-20.5304651300537,-43.797431637791,123.856190933871)) ;
#77810=CARTESIAN_POINT('Ctrl Pts',(-20.8861267322825,-43.9874815931041,
123.713900101294)) ;
#77811=CARTESIAN_POINT('Ctrl Pts',(-20.5907535610701,-43.8074925126853,
123.653482792957)) ;
#77812=CARTESIAN_POINT('Ctrl Pts',(-20.9160480544074,-43.9973204964335,
123.457038808337)) ;
#77813=CARTESIAN_POINT('Ctrl Pts',(-20.6146904768429,-43.8173314160147,
123.44799493269)) ;
#77814=CARTESIAN_POINT('Ctrl Pts',(-20.9008215570039,-44.0073888728073,
123.192934464744)) ;
#77815=CARTESIAN_POINT('Ctrl Pts',(-20.6025093217577,-43.8273997923886,
123.236711133605)) ;
#77816=CARTESIAN_POINT('Ctrl Pts',(-20.8409996768118,-44.01726948944,122.940227571299)) ;
#77817=CARTESIAN_POINT('Ctrl Pts',(-20.5546520629352,-43.8372804090212,
123.034546490848)) ;
#77818=CARTESIAN_POINT('Ctrl Pts',(-20.7375752827161,-44.027260649669,122.698940269749)) ;
#77819=CARTESIAN_POINT('Ctrl Pts',(-20.4719127723535,-43.8472715692502,
122.841516743795)) ;
#77820=CARTESIAN_POINT('Ctrl Pts',(-20.5943672383573,-44.0372137231011,
122.48002524176)) ;
#77821=CARTESIAN_POINT('Ctrl Pts',(-20.357346713871,-43.8572246426823,122.666384965214)) ;
#77822=CARTESIAN_POINT('Ctrl Pts',(-20.4138140211053,-44.0472495587137,
122.28781904811)) ;
#77823=CARTESIAN_POINT('Ctrl Pts',(-20.212904171313,-43.867260478295,122.512619815452)) ;
#77824=CARTESIAN_POINT('Ctrl Pts',(-20.205771627624,-44.0571396854439,122.132010547395)) ;
#77825=CARTESIAN_POINT('Ctrl Pts',(-20.0464710629452,-43.8771506050251,
122.387973367554)) ;
#77826=CARTESIAN_POINT('Ctrl Pts',(-19.9716606493193,-44.0671318672132,
122.01311881931)) ;
#77827=CARTESIAN_POINT('Ctrl Pts',(-19.8591825691405,-43.8871427867944,
122.292859783673)) ;
#77828=CARTESIAN_POINT('Ctrl Pts',(-19.7215859697083,-44.0770778071876,
121.937116648919)) ;
#77829=CARTESIAN_POINT('Ctrl Pts',(-19.6591233631449,-43.8970887267689,
122.232057912344)) ;
#77830=CARTESIAN_POINT('Ctrl Pts',(-19.4621316011736,-44.0870249909471,
121.905158079353)) ;
#77831=CARTESIAN_POINT('Ctrl Pts',(-19.4515603759915,-43.9070359105284,
122.206490695908)) ;
#77832=CARTESIAN_POINT('Ctrl Pts',(-19.1984633098355,-44.0970729292374,
121.919166261337)) ;
#77833=CARTESIAN_POINT('Ctrl Pts',(-19.2406255245606,-43.9170838488187,
122.217696907762)) ;
#77834=CARTESIAN_POINT('Ctrl Pts',(-18.9462999516844,-44.106920564051,121.977344862688)) ;
#77835=CARTESIAN_POINT('Ctrl Pts',(-19.0388958389278,-43.9269314836323,
122.264239147175)) ;
#77836=CARTESIAN_POINT('Ctrl Pts',(-18.705003034918,-44.1168822777489,122.078833023543)) ;
#77837=CARTESIAN_POINT('Ctrl Pts',(-18.8458584060323,-43.9368931973302,
122.345428976242)) ;
#77838=CARTESIAN_POINT('Ctrl Pts',(-18.4836721334417,-44.1269109135701,
122.221925766964)) ;
#77839=CARTESIAN_POINT('Ctrl Pts',(-18.6687933369296,-43.9469218331514,
122.459902775154)) ;
#77840=CARTESIAN_POINT('Ctrl Pts',(-18.2927904239881,-44.1368212283219,
122.399078178107)) ;
#77841=CARTESIAN_POINT('Ctrl Pts',(-18.5160881141208,-43.9568321479032,
122.601623829949)) ;
#77842=CARTESIAN_POINT('Ctrl Pts',(-18.1346189320246,-44.1467560989846,
122.60679979721)) ;
#77843=CARTESIAN_POINT('Ctrl Pts',(-18.3895506742922,-43.9667670185658,
122.767800273057)) ;
#77844=CARTESIAN_POINT('Ctrl Pts',(-18.0138706730866,-44.1567972813863,
122.841409864092)) ;
#77845=CARTESIAN_POINT('Ctrl Pts',(-18.2929514212946,-43.9768082009676,
122.955488165132)) ;
#77846=CARTESIAN_POINT('Ctrl Pts',(-17.9366823754351,-44.1666842528511,
123.089522739993)) ;
#77847=CARTESIAN_POINT('Ctrl Pts',(-18.2312003631439,-43.9866951724323,
123.153977453905)) ;
#77848=CARTESIAN_POINT('Ctrl Pts',(-17.9030484193325,-44.1766836851137,
123.350101781406)) ;
#77849=CARTESIAN_POINT('Ctrl Pts',(-18.2042924372665,-43.9966946046949,
123.36244046689)) ;
#77850=CARTESIAN_POINT('Ctrl Pts',(-17.91490147005,-44.1866037503703,123.610552838721)) ;
#77851=CARTESIAN_POINT('Ctrl Pts',(-18.213774030704,-44.0066146699516,123.570800751409)) ;
#77852=CARTESIAN_POINT('Ctrl Pts',(-17.9724055289825,-44.1966406029545,
123.867950986187)) ;
#77853=CARTESIAN_POINT('Ctrl Pts',(-18.2597764896288,-44.0166515225357,
123.776719574248)) ;
#77854=CARTESIAN_POINT('Ctrl Pts',(-18.072489495882,-44.2065532622945,124.108457083353)) ;
#77855=CARTESIAN_POINT('Ctrl Pts',(-18.33984264497,-44.0265641818757,123.969124165985)) ;
#77856=CARTESIAN_POINT('Ctrl Pts',(-18.2134492761072,-44.2165444742093,
124.329987229875)) ;
#77857=CARTESIAN_POINT('Ctrl Pts',(-18.4526095642665,-44.0365553937906,
124.146348659042)) ;
#77858=CARTESIAN_POINT('Ctrl Pts',(-18.3920400927289,-44.2265861156124,
124.524226386367)) ;
#77859=CARTESIAN_POINT('Ctrl Pts',(-18.5954817048883,-44.0465970351937,
124.301740649263)) ;
#77860=CARTESIAN_POINT('Ctrl Pts',(-18.5968513118153,-44.2364149098195,
124.681658511615)) ;
#77861=CARTESIAN_POINT('Ctrl Pts',(-18.7593291698146,-44.0564258294008,
124.427686424433)) ;
#77862=CARTESIAN_POINT('Ctrl Pts',(-18.831525371307,-44.2464913209408,124.804205426274)) ;
#77863=CARTESIAN_POINT('Ctrl Pts',(-18.9470682569457,-44.066502240522,124.525725008789)) ;
#77864=CARTESIAN_POINT('Ctrl Pts',(-19.078357884535,-44.2563434539832,124.882525082064)) ;
#77865=CARTESIAN_POINT('Ctrl Pts',(-19.1445330139973,-44.0763543735645,
124.588381422117)) ;
#77866=CARTESIAN_POINT('Ctrl Pts',(-19.3406710042033,-44.2664166883245,
124.917774928985)) ;
#77867=CARTESIAN_POINT('Ctrl Pts',(-19.3543836827224,-44.0864276079058,
124.616582420438)) ;
#77868=CARTESIAN_POINT('Ctrl Pts',(-19.5990935689859,-44.2762581896512,
124.907117526499)) ;
#77869=CARTESIAN_POINT('Ctrl Pts',(-19.5611207373312,-44.0962691092324,
124.608057610087)) ;
#77870=CARTESIAN_POINT('Ctrl Pts',(-19.8549900005476,-44.286219141246,124.852048008069)) ;
#77871=CARTESIAN_POINT('Ctrl Pts',(-19.7658378370726,-44.1062300608272,
124.56400332464)) ;
#77872=CARTESIAN_POINT('Ctrl Pts',(-20.0991093096475,-44.2962569589666,
124.752132918125)) ;
#77873=CARTESIAN_POINT('Ctrl Pts',(-19.9611338268518,-44.1162678785479,
124.484072297486)) ;
#77874=CARTESIAN_POINT('Ctrl Pts',(-20.3188305768952,-44.3061313082237,
124.614027246314)) ;
#77875=CARTESIAN_POINT('Ctrl Pts',(-20.1369108352661,-44.1261422278049,
124.373589272937)) ;
#77876=CARTESIAN_POINT('Ctrl Pts',(-20.5149750944299,-44.3162008589659,
124.43646009171)) ;
#77877=CARTESIAN_POINT('Ctrl Pts',(-20.2938275119669,-44.1362117785471,
124.231536305792)) ;
#77878=CARTESIAN_POINT('Ctrl Pts',(-20.6736665783671,-44.3260348784745,
124.232462693765)) ;
#77879=CARTESIAN_POINT('Ctrl Pts',(-20.4207810991636,-44.1460457980557,
124.068340001014)) ;
#77880=CARTESIAN_POINT('Ctrl Pts',(-20.7975823821295,-44.336069033054,123.999722159429)) ;
#77881=CARTESIAN_POINT('Ctrl Pts',(-20.5199150654758,-44.1560799526353,
123.88214817752)) ;
#77882=CARTESIAN_POINT('Ctrl Pts',(-20.8784453197295,-44.3460849588765,
123.749227159085)) ;
#77883=CARTESIAN_POINT('Ctrl Pts',(-20.5846066615164,-44.1660958784577,
123.681752589755)) ;
#77884=CARTESIAN_POINT('Ctrl Pts',(-20.9145638047595,-44.3559672140707,
123.49205122072)) ;
#77885=CARTESIAN_POINT('Ctrl Pts',(-20.613502746607,-44.175978133652,123.476012754182)) ;
#77886=CARTESIAN_POINT('Ctrl Pts',(-20.9057075528945,-44.3659560205816,
123.229734225028)) ;
#77887=CARTESIAN_POINT('Ctrl Pts',(-20.6064192252653,-44.1859669401629,
123.266159268691)) ;
#77888=CARTESIAN_POINT('Ctrl Pts',(-20.8518375941901,-44.3759045878444,
122.973864298025)) ;
#77889=CARTESIAN_POINT('Ctrl Pts',(-20.563324813657,-44.1959155074256,123.061463372867)) ;
#77890=CARTESIAN_POINT('Ctrl Pts',(-20.753082557148,-44.3859593931464,122.728813985301)) ;
#77891=CARTESIAN_POINT('Ctrl Pts',(-20.4843220736738,-44.2059703127276,
122.86542241497)) ;
#77892=CARTESIAN_POINT('Ctrl Pts',(-20.616855401544,-44.3957781764099,122.509662800828)) ;
#77893=CARTESIAN_POINT('Ctrl Pts',(-20.3753421837085,-44.2157890959912,
122.690101516828)) ;
#77894=CARTESIAN_POINT('Ctrl Pts',(-20.4413805689647,-44.4058139487705,
122.312790934057)) ;
#77895=CARTESIAN_POINT('Ctrl Pts',(-20.2349635031074,-44.2258248683518,
122.532602849493)) ;
#77896=CARTESIAN_POINT('Ctrl Pts',(-20.2341379247197,-44.4158386477992,
122.150140067288)) ;
#77897=CARTESIAN_POINT('Ctrl Pts',(-20.0691703136329,-44.2358495673804,
122.402480945821)) ;
#77898=CARTESIAN_POINT('Ctrl Pts',(-20.0060783373224,-44.4256906510582,
122.027581366455)) ;
#77899=CARTESIAN_POINT('Ctrl Pts',(-19.8867241261111,-44.2457015706395,
122.304432930007)) ;
#77900=CARTESIAN_POINT('Ctrl Pts',(-19.7568956897804,-44.4356815854555,
121.94497080337)) ;
#77901=CARTESIAN_POINT('Ctrl Pts',(-19.6873786743973,-44.2556925050367,
122.238342904726)) ;
#77902=CARTESIAN_POINT('Ctrl Pts',(-19.4990141869597,-44.4455995078866,
121.906980973372)) ;
#77903=CARTESIAN_POINT('Ctrl Pts',(-19.4810741764347,-44.2656104274678,
122.207949395468)) ;
#77904=CARTESIAN_POINT('Ctrl Pts',(-19.2356052976656,-44.4556278635689,
121.914367687835)) ;
#77905=CARTESIAN_POINT('Ctrl Pts',(-19.2703469878274,-44.2756387831502,
122.213857026739)) ;
#77906=CARTESIAN_POINT('Ctrl Pts',(-18.9811319609968,-44.4655121480795,
121.966499520209)) ;
#77907=CARTESIAN_POINT('Ctrl Pts',(-19.0667685443539,-44.2855230676607,
122.255560647816)) ;
#77908=CARTESIAN_POINT('Ctrl Pts',(-18.7367176525128,-44.4755048319874,
122.062515901557)) ;
#77909=CARTESIAN_POINT('Ctrl Pts',(-18.871236522365,-44.2955157515686,122.332371983472)) ;
#77910=CARTESIAN_POINT('Ctrl Pts',(-18.5121188960051,-44.4855335689951,
122.200401078734)) ;
#77911=CARTESIAN_POINT('Ctrl Pts',(-18.6915565682666,-44.3055444885763,
122.442678613519)) ;
#77912=CARTESIAN_POINT('Ctrl Pts',(-18.3174591680508,-44.495418965624,122.372439116278)) ;
#77913=CARTESIAN_POINT('Ctrl Pts',(-18.5358279827225,-44.3154298852052,
122.580307299376)) ;
#77914=CARTESIAN_POINT('Ctrl Pts',(-18.1536797929993,-44.5054068510379,
122.57750876057)) ;
#77915=CARTESIAN_POINT('Ctrl Pts',(-18.4048030832296,-44.3254177706191,
122.744361731314)) ;
#77916=CARTESIAN_POINT('Ctrl Pts',(-18.0283271818047,-44.5153575536985,
122.807042074276)) ;
#77917=CARTESIAN_POINT('Ctrl Pts',(-18.3045194438468,-44.3353684732797,
122.927987235333)) ;
#77918=CARTESIAN_POINT('Ctrl Pts',(-17.9441368873553,-44.5253978717959,
123.057070192347)) ;
#77919=CARTESIAN_POINT('Ctrl Pts',(-18.2371653982975,-44.3454087913771,
123.128009182656)) ;
#77920=CARTESIAN_POINT('Ctrl Pts',(-17.9050280765353,-44.5352724371291,
123.313629339721)) ;
#77921=CARTESIAN_POINT('Ctrl Pts',(-18.2058765291738,-44.3552833567104,
123.333255668068)) ;
#77922=CARTESIAN_POINT('Ctrl Pts',(-17.9108009162363,-44.5452720971902,
123.576303554654)) ;
#77923=CARTESIAN_POINT('Ctrl Pts',(-18.2104928246366,-44.3652830167714,
123.543394997243)) ;
#77924=CARTESIAN_POINT('Ctrl Pts',(-17.9614015775647,-44.5551810923579,
123.83178501251)) ;
#77925=CARTESIAN_POINT('Ctrl Pts',(-18.2509713159387,-44.3751920119392,
123.747780179525)) ;
#77926=CARTESIAN_POINT('Ctrl Pts',(-18.0570243117927,-44.5652358335212,
124.078057381531)) ;
#77927=CARTESIAN_POINT('Ctrl Pts',(-18.3274676754747,-44.3852467531024,
123.944798879371)) ;
#77928=CARTESIAN_POINT('Ctrl Pts',(-18.1910740417786,-44.5750944454349,
124.299808917712)) ;
#77929=CARTESIAN_POINT('Ctrl Pts',(-18.4347054549292,-44.3951053650162,
124.122200713057)) ;
#77930=CARTESIAN_POINT('Ctrl Pts',(-18.3650377632803,-44.5851625677143,
124.49910396342)) ;
#77931=CARTESIAN_POINT('Ctrl Pts',(-18.5738749680476,-44.4051734872955,
124.281638189971)) ;
#77932=CARTESIAN_POINT('Ctrl Pts',(-18.5666736485411,-44.5950180384175,
124.661680062397)) ;
#77933=CARTESIAN_POINT('Ctrl Pts',(-18.7351820039692,-44.4150289579987,
124.411700348019)) ;
#77934=CARTESIAN_POINT('Ctrl Pts',(-18.7962745857529,-44.6050128979108,
124.78921896705)) ;
#77935=CARTESIAN_POINT('Ctrl Pts',(-18.9188616496907,-44.4250238174921,
124.513733295613)) ;
#77936=CARTESIAN_POINT('Ctrl Pts',(-19.045634886817,-44.6150441512528,124.874734939546)) ;
#77937=CARTESIAN_POINT('Ctrl Pts',(-19.1183492174815,-44.435055070834,124.582148031688)) ;
#77938=CARTESIAN_POINT('Ctrl Pts',(-19.3017226630641,-44.6249108501259,
124.915389460371)) ;
#77939=CARTESIAN_POINT('Ctrl Pts',(-19.3232187005312,-44.4449217697071,
124.614673670169)) ;
#77940=CARTESIAN_POINT('Ctrl Pts',(-19.5641051552201,-44.6348976658771,
124.911339609396)) ;
#77941=CARTESIAN_POINT('Ctrl Pts',(-19.5331246292621,-44.4549085854583,
124.611435943813)) ;
#77942=CARTESIAN_POINT('Ctrl Pts',(-19.820862633576,-44.6448448710725,124.862095013868)) ;
#77943=CARTESIAN_POINT('Ctrl Pts',(-19.7385308356951,-44.4648557906538,
124.572042423977)) ;
#77944=CARTESIAN_POINT('Ctrl Pts',(-20.0674296682217,-44.6548878591988,
124.768031081774)) ;
#77945=CARTESIAN_POINT('Ctrl Pts',(-19.9357852426788,-44.4748987787801,
124.496793284832)) ;
#77946=CARTESIAN_POINT('Ctrl Pts',(-20.2900606909921,-44.6647552138203,
124.635070010774)) ;
#77947=CARTESIAN_POINT('Ctrl Pts',(-20.1138908853131,-44.4847661334015,
124.390426455139)) ;
#77948=CARTESIAN_POINT('Ctrl Pts',(-20.4886282484317,-44.6747211071184,
124.464326907959)) ;
#77949=CARTESIAN_POINT('Ctrl Pts',(-20.2727462890408,-44.4947320266996,
124.253833725483)) ;
#77950=CARTESIAN_POINT('Ctrl Pts',(-20.6553026894902,-44.6847448844945,
124.26032841296)) ;
#77951=CARTESIAN_POINT('Ctrl Pts',(-20.4060875193306,-44.5047558040757,
124.090636341466)) ;
#77952=CARTESIAN_POINT('Ctrl Pts',(-20.7828007334858,-44.6946704324262,
124.032794984421)) ;
#77953=CARTESIAN_POINT('Ctrl Pts',(-20.5080877807566,-44.5146813520074,
123.908610839297)) ;
#77954=CARTESIAN_POINT('Ctrl Pts',(-20.8695762748802,-44.7046109088472,
123.786387153768)) ;
#77955=CARTESIAN_POINT('Ctrl Pts',(-20.5775102739201,-44.5246218284284,
123.711485441995)) ;
#77956=CARTESIAN_POINT('Ctrl Pts',(-20.9124006494163,-44.7146571185101,
123.525895807859)) ;
#77957=CARTESIAN_POINT('Ctrl Pts',(-20.6117719585213,-44.5346680380913,
123.503092741529)) ;
#77958=CARTESIAN_POINT('Ctrl Pts',(-20.9096780312337,-44.7245183751719,
123.266743788831)) ;
#77959=CARTESIAN_POINT('Ctrl Pts',(-20.6095960943389,-44.5445292947531,
123.295771314812)) ;
#77960=CARTESIAN_POINT('Ctrl Pts',(-20.8618140136245,-44.7345120034472,
123.008558951092)) ;
#77961=CARTESIAN_POINT('Ctrl Pts',(-20.5713071019526,-44.5545229230284,
123.089223095259)) ;
#77962=CARTESIAN_POINT('Ctrl Pts',(-20.7705763698278,-44.7444374007574,
122.764165937538)) ;
#77963=CARTESIAN_POINT('Ctrl Pts',(-20.498319127258,-44.5644483203386,122.893707997254)) ;
#77964=CARTESIAN_POINT('Ctrl Pts',(-20.6369673170005,-44.7544653086676,
122.537064718107)) ;
#77965=CARTESIAN_POINT('Ctrl Pts',(-20.3914338502099,-44.5744762282489,
122.712025924337)) ;
#77966=CARTESIAN_POINT('Ctrl Pts',(-20.468527288973,-44.7643516243368,122.339213894273)) ;
#77967=CARTESIAN_POINT('Ctrl Pts',(-20.2566836019861,-44.584362543918,122.553743877924)) ;
#77968=CARTESIAN_POINT('Ctrl Pts',(-20.2655021978524,-44.7743832192406,
122.171124667689)) ;
#77969=CARTESIAN_POINT('Ctrl Pts',(-20.0942650101056,-44.5943941388218,
122.419270793338)) ;
#77970=CARTESIAN_POINT('Ctrl Pts',(-20.0398318506842,-44.7842654621923,
122.042531241713)) ;
#77971=CARTESIAN_POINT('Ctrl Pts',(-19.9137298912166,-44.6042763817735,
122.316394121493)) ;
#77972=CARTESIAN_POINT('Ctrl Pts',(-19.7909809655127,-44.7943249332221,
121.953425884344)) ;
#77973=CARTESIAN_POINT('Ctrl Pts',(-19.7146500072838,-44.6143358528034,
122.24510773456)) ;
#77974=CARTESIAN_POINT('Ctrl Pts',(-19.535389413835,-44.8041913778853,121.90976454012)) ;
#77975=CARTESIAN_POINT('Ctrl Pts',(-19.5101771563229,-44.6242022974665,
122.210176441665)) ;
#77976=CARTESIAN_POINT('Ctrl Pts',(-19.2734974473608,-44.8141575023339,
121.910332881199)) ;
#77977=CARTESIAN_POINT('Ctrl Pts',(-19.300663601662,-44.6341684219152,122.210628864892)) ;
#77978=CARTESIAN_POINT('Ctrl Pts',(-19.0140941941799,-44.8241877457251,
121.957079096009)) ;
#77979=CARTESIAN_POINT('Ctrl Pts',(-19.0931406459017,-44.6441986653064,
122.248023646285)) ;
#77980=CARTESIAN_POINT('Ctrl Pts',(-18.7699778546142,-44.8340807806781,
122.046571668305)) ;
#77981=CARTESIAN_POINT('Ctrl Pts',(-18.8978469009694,-44.6540917002594,
122.319615481204)) ;
#77982=CARTESIAN_POINT('Ctrl Pts',(-18.5415249218086,-44.844131694915,122.179088598148)) ;
#77983=CARTESIAN_POINT('Ctrl Pts',(-18.7150830028236,-44.6641426144963,
122.425627556527)) ;
#77984=CARTESIAN_POINT('Ctrl Pts',(-18.3427444001269,-44.8540215211396,
122.346531093199)) ;
#77985=CARTESIAN_POINT('Ctrl Pts',(-18.5560590226922,-44.6740324407208,
122.55957796272)) ;
#77986=CARTESIAN_POINT('Ctrl Pts',(-18.1174461021074,-44.8673563361865,
122.614979486974)) ;
#77987=CARTESIAN_POINT('Ctrl Pts',(-18.3758085267228,-44.6873672557678,
122.774344354257)) ;
#77988=CARTESIAN_POINT('Ctrl Pts',(-17.9686335760007,-44.880633427358,122.934896659111)) ;
#77989=CARTESIAN_POINT('Ctrl Pts',(-18.2567530298792,-44.7006443469392,
123.030306574973)) ;
#77990=CARTESIAN_POINT('Ctrl Pts',(-17.9076731561745,-44.8938817159563,
123.277709414337)) ;
#77991=CARTESIAN_POINT('Ctrl Pts',(-18.2079946998203,-44.7138926355375,
123.304511413503)) ;
#77992=CARTESIAN_POINT('Ctrl Pts',(-17.907462316396,-44.9039365574504,123.541899571291)) ;
#77993=CARTESIAN_POINT('Ctrl Pts',(-18.2078213171443,-44.7239474770316,
123.515872463229)) ;
#77994=CARTESIAN_POINT('Ctrl Pts',(-17.9516919898159,-44.9137675467579,
123.796479325877)) ;
#77995=CARTESIAN_POINT('Ctrl Pts',(-18.2432033587368,-44.7337784663392,
123.719534329518)) ;
#77996=CARTESIAN_POINT('Ctrl Pts',(-18.0414310832695,-44.9238441110811,
124.045563596341)) ;
#77997=CARTESIAN_POINT('Ctrl Pts',(-18.3149935556506,-44.7438550306624,
123.918803730498)) ;
#77998=CARTESIAN_POINT('Ctrl Pts',(-18.1701298254972,-44.9336934362151,
124.270160085641)) ;
#77999=CARTESIAN_POINT('Ctrl Pts',(-18.4179464132743,-44.7537043557963,
124.098479058977)) ;
#78000=CARTESIAN_POINT('Ctrl Pts',(-18.3940753258165,-44.9470414358523,
124.540160290247)) ;
#78001=CARTESIAN_POINT('Ctrl Pts',(-18.5971230250769,-44.7670523554336,
124.314496251429)) ;
#78002=CARTESIAN_POINT('Ctrl Pts',(-18.7539725180516,-44.9636261953889,
124.794623795702)) ;
#78003=CARTESIAN_POINT('Ctrl Pts',(-18.8849990055932,-44.7836371149701,
124.518050456276)) ;
#78004=CARTESIAN_POINT('Ctrl Pts',(-19.1783954642858,-44.980194746737,124.911954796684)) ;
#78005=CARTESIAN_POINT('Ctrl Pts',(-19.2246019623236,-44.8002056663183,
124.611932785891)) ;
#78006=CARTESIAN_POINT('Ctrl Pts',(-19.5295000394713,-44.993554571556,124.914496420858)) ;
#78007=CARTESIAN_POINT('Ctrl Pts',(-19.5054328311711,-44.8135654911373,
124.613960044086)) ;
#78008=CARTESIAN_POINT('Ctrl Pts',(-19.7862085515655,-45.0034599803866,
124.871351922851)) ;
#78009=CARTESIAN_POINT('Ctrl Pts',(-19.7108114579357,-44.8234708999679,
124.579447577859)) ;
#78010=CARTESIAN_POINT('Ctrl Pts',(-20.032977047638,-45.0134200069707,124.784181635909)) ;
#78011=CARTESIAN_POINT('Ctrl Pts',(-19.9082219143351,-44.833430926552,124.509714796774)) ;
#78012=CARTESIAN_POINT('Ctrl Pts',(-20.3365929404085,-45.026677591156,124.613239797364)) ;
#78013=CARTESIAN_POINT('Ctrl Pts',(-20.151128683135,-44.8466885107373,124.372952796465)) ;
#78014=CARTESIAN_POINT('Ctrl Pts',(-20.6530388479444,-45.0433288026507,
124.303846929817)) ;
#78015=CARTESIAN_POINT('Ctrl Pts',(-20.4042740591769,-44.8633397222319,
124.125452733239)) ;
#78016=CARTESIAN_POINT('Ctrl Pts',(-20.8822225929633,-45.063247016761,123.826665489828)) ;
#78017=CARTESIAN_POINT('Ctrl Pts',(-20.5876289589755,-44.8832579363422,
123.743704995004)) ;
#78018=CARTESIAN_POINT('Ctrl Pts',(-20.9358462101618,-45.0831247799818,
123.300999284686)) ;
#78019=CARTESIAN_POINT('Ctrl Pts',(-20.6305301436153,-44.9031356995631,
123.323172734801)) ;
#78020=CARTESIAN_POINT('Ctrl Pts',(-20.8055712372193,-45.103137447769,122.785395465284)) ;
#78021=CARTESIAN_POINT('Ctrl Pts',(-20.5263138314019,-44.9231483673502,
122.910688665346)) ;
#78022=CARTESIAN_POINT('Ctrl Pts',(-20.5104525720228,-45.1229499704356,
122.349160972127)) ;
#78023=CARTESIAN_POINT('Ctrl Pts',(-20.2902207745244,-44.9429608900168,
122.561698343085)) ;
#78024=CARTESIAN_POINT('Ctrl Pts',(-20.0811678726187,-45.1429332704355,
122.036595982183)) ;
#78025=CARTESIAN_POINT('Ctrl Pts',(-19.946794629083,-44.9629441900167,122.311643931763)) ;
#78026=CARTESIAN_POINT('Ctrl Pts',(-19.57298082711,-45.1628275475368,121.890260817319)) ;
#78027=CARTESIAN_POINT('Ctrl Pts',(-19.5402450431835,-44.982838467118,122.194572859151)) ;
#78028=CARTESIAN_POINT('Ctrl Pts',(-19.0443792387932,-45.1827603092946,
121.925363493161)) ;
#78029=CARTESIAN_POINT('Ctrl Pts',(-19.1173630609288,-45.0027712288758,
122.222652560923)) ;
#78030=CARTESIAN_POINT('Ctrl Pts',(-18.5588123388125,-45.2027263150593,
122.139444767392)) ;
#78031=CARTESIAN_POINT('Ctrl Pts',(-18.7289082955966,-45.0227372346405,
122.393915435072)) ;
#78032=CARTESIAN_POINT('Ctrl Pts',(-18.1768400074988,-45.2226048472241,
122.504512707819)) ;
#78033=CARTESIAN_POINT('Ctrl Pts',(-18.4233281318735,-45.0426157668054,
122.685968958821)) ;
#78034=CARTESIAN_POINT('Ctrl Pts',(-17.9412382745813,-45.2425445138845,
122.97916517489)) ;
#78035=CARTESIAN_POINT('Ctrl Pts',(-18.2348448067827,-45.0625554334657,
123.065690634958)) ;
#78036=CARTESIAN_POINT('Ctrl Pts',(-17.8817201356207,-45.2624393885298,
123.504633155358)) ;
#78037=CARTESIAN_POINT('Ctrl Pts',(-18.1872285519615,-45.0824503081111,
123.48606590208)) ;
#78038=CARTESIAN_POINT('Ctrl Pts',(-18.0046155636141,-45.2823465278232,
124.01913650114)) ;
#78039=CARTESIAN_POINT('Ctrl Pts',(-18.2855439122614,-45.1023574474044,
123.897669917515)) ;
#78040=CARTESIAN_POINT('Ctrl Pts',(-18.295159268459,-45.3022570759017,124.461637555443)) ;
#78041=CARTESIAN_POINT('Ctrl Pts',(-18.5179788419764,-45.1222679954829,
124.251671936744)) ;
#78042=CARTESIAN_POINT('Ctrl Pts',(-18.7231289192016,-45.3223256612588,
124.779793280971)) ;
#78043=CARTESIAN_POINT('Ctrl Pts',(-18.8603532666718,-45.1423365808401,
124.506196853283)) ;
#78044=CARTESIAN_POINT('Ctrl Pts',(-19.2267990765267,-45.3421074585736,
124.931211593248)) ;
#78045=CARTESIAN_POINT('Ctrl Pts',(-19.2632917257971,-45.1621183781549,
124.627332840506)) ;
#78046=CARTESIAN_POINT('Ctrl Pts',(-19.7575625515269,-45.3621150055181,
124.902127405281)) ;
#78047=CARTESIAN_POINT('Ctrl Pts',(-19.6879025560016,-45.1821259250994,
124.604065538221)) ;
#78048=CARTESIAN_POINT('Ctrl Pts',(-20.2423289587941,-45.381936743821,124.695488931226)) ;
#78049=CARTESIAN_POINT('Ctrl Pts',(-20.0757176520892,-45.2019476634022,
124.438753696871)) ;
#78050=CARTESIAN_POINT('Ctrl Pts',(-20.6310564600135,-45.4019167637251,
124.333814619523)) ;
#78051=CARTESIAN_POINT('Ctrl Pts',(-20.3866992414769,-45.2219276833064,
124.149413465804)) ;
#78052=CARTESIAN_POINT('Ctrl Pts',(-20.8717000556849,-45.4218342149874,
123.862278018849)) ;
#78053=CARTESIAN_POINT('Ctrl Pts',(-20.579213919715,-45.2418451345686,123.77218297004)) ;
#78054=CARTESIAN_POINT('Ctrl Pts',(-20.9380767681867,-45.4417091361601,
123.338188475179)) ;
#78055=CARTESIAN_POINT('Ctrl Pts',(-20.6323140215928,-45.2617200557413,
123.352909817565)) ;
#78056=CARTESIAN_POINT('Ctrl Pts',(-20.8204289202188,-45.4617335047109,
122.819174892969)) ;
#78057=CARTESIAN_POINT('Ctrl Pts',(-20.5381943820615,-45.2817444242922,
122.937699557393)) ;
#78058=CARTESIAN_POINT('Ctrl Pts',(-20.5348026192867,-45.4816001890844,
122.374971928314)) ;
#78059=CARTESIAN_POINT('Ctrl Pts',(-20.3096913007445,-45.3016111086656,
122.582336913759)) ;
#78060=CARTESIAN_POINT('Ctrl Pts',(-20.1137378287957,-45.5015440109306,
122.053072103638)) ;
#78061=CARTESIAN_POINT('Ctrl Pts',(-19.9728377986509,-45.3215549305118,
122.324818360673)) ;
#78062=CARTESIAN_POINT('Ctrl Pts',(-19.6089136734413,-45.5214513801821,
121.894620584334)) ;
#78063=CARTESIAN_POINT('Ctrl Pts',(-19.5689770139582,-45.3414622997634,
122.198058922414)) ;
#78064=CARTESIAN_POINT('Ctrl Pts',(-19.0811541092008,-45.5413260779288,
121.916926618905)) ;
#78065=CARTESIAN_POINT('Ctrl Pts',(-19.1467684454857,-45.3613369975101,
122.215906404225)) ;
#78066=CARTESIAN_POINT('Ctrl Pts',(-18.58996630322,-45.5613080204505,122.1189694923)) ;
#78067=CARTESIAN_POINT('Ctrl Pts',(-18.7538191655351,-45.3813189400318,
122.377543293856)) ;
#78068=CARTESIAN_POINT('Ctrl Pts',(-18.1991325995825,-45.5812106873614,
122.475351878696)) ;
#78069=CARTESIAN_POINT('Ctrl Pts',(-18.4411535104022,-45.4012216069426,
122.662651767787)) ;
#78070=CARTESIAN_POINT('Ctrl Pts',(-17.9525130135342,-45.6010660449001,
122.941989689351)) ;
#78071=CARTESIAN_POINT('Ctrl Pts',(-18.2438603264457,-45.4210769644813,
123.035964382293)) ;
#78072=CARTESIAN_POINT('Ctrl Pts',(-17.8797853305759,-45.6211300836161,
123.470193368156)) ;
#78073=CARTESIAN_POINT('Ctrl Pts',(-18.1856815073262,-45.4411410031973,
123.458527308833)) ;
#78074=CARTESIAN_POINT('Ctrl Pts',(-17.9907738385285,-45.6409852633412,
123.986308188062)) ;
#78075=CARTESIAN_POINT('Ctrl Pts',(-18.2744755604141,-45.4609961829224,
123.871419313323)) ;
#78076=CARTESIAN_POINT('Ctrl Pts',(-18.2724161799127,-45.6609653680056,
124.43626592713)) ;
#78077=CARTESIAN_POINT('Ctrl Pts',(-18.4997930441946,-45.4809762875868,
124.231383659367)) ;
#78078=CARTESIAN_POINT('Ctrl Pts',(-18.6870078951733,-45.6807744731754,
124.761025281419)) ;
#78079=CARTESIAN_POINT('Ctrl Pts',(-18.8314673456426,-45.5007853927566,
124.491189117074)) ;
#78080=CARTESIAN_POINT('Ctrl Pts',(-19.1916999501291,-45.7007670935161,
124.926741074953)) ;
#78081=CARTESIAN_POINT('Ctrl Pts',(-19.235230041018,-45.5207780130973,124.623756847041)) ;
#78082=CARTESIAN_POINT('Ctrl Pts',(-19.6312118173509,-45.7173065760202,
124.913196410059)) ;
#78083=CARTESIAN_POINT('Ctrl Pts',(-19.5868155436623,-45.5373174956014,
124.612921459841)) ;
#78084=CARTESIAN_POINT('Ctrl Pts',(-19.967499356913,-45.7306708940844,124.812112387731)) ;
#78085=CARTESIAN_POINT('Ctrl Pts',(-19.8558719099428,-45.5506818136656,
124.532044502846)) ;
#78086=CARTESIAN_POINT('Ctrl Pts',(-20.2779790595161,-45.7438884965859,
124.656227492498)) ;
#78087=CARTESIAN_POINT('Ctrl Pts',(-20.1042094374621,-45.5638994161671,
124.407362610249)) ;
#78088=CARTESIAN_POINT('Ctrl Pts',(-20.6088613726439,-45.7605460908637,
124.362235325812)) ;
#78089=CARTESIAN_POINT('Ctrl Pts',(-20.3689615158667,-45.5805570104449,
124.172135807522)) ;
#78090=CARTESIAN_POINT('Ctrl Pts',(-20.8603771682476,-45.7804117929054,
123.897882286003)) ;
#78091=CARTESIAN_POINT('Ctrl Pts',(-20.5701552926539,-45.6004227124867,
123.800652558022)) ;
#78092=CARTESIAN_POINT('Ctrl Pts',(-20.9262145452714,-45.7970415195954,
123.460911151539)) ;
#78093=CARTESIAN_POINT('Ctrl Pts',(-20.6228240067414,-45.6170524391767,
123.451100564137)) ;
#78094=CARTESIAN_POINT('Ctrl Pts',(-20.8869828200651,-45.8103306347333,
123.113835882206)) ;
#78095=CARTESIAN_POINT('Ctrl Pts',(-20.5914361114732,-45.6303415543145,
123.17341573683)) ;
#78096=CARTESIAN_POINT('Ctrl Pts',(-20.8131372217182,-45.8202949817104,
122.862628158014)) ;
#78097=CARTESIAN_POINT('Ctrl Pts',(-20.532359431995,-45.6403059012916,122.97245700907)) ;
#78098=CARTESIAN_POINT('Ctrl Pts',(-20.6973720959794,-45.8302233497119,
122.628822672063)) ;
#78099=CARTESIAN_POINT('Ctrl Pts',(-20.4397374777452,-45.6502342692931,
122.785404651052)) ;
#78100=CARTESIAN_POINT('Ctrl Pts',(-20.4910362460861,-45.8435067828006,
122.34720320038)) ;
#78101=CARTESIAN_POINT('Ctrl Pts',(-20.2747057229162,-45.6635177023819,
122.560148879039)) ;
#78102=CARTESIAN_POINT('Ctrl Pts',(-20.1458260850277,-45.8601588605409,
122.070280119453)) ;
#78103=CARTESIAN_POINT('Ctrl Pts',(-19.9984819208062,-45.6801697801222,
122.338567916265)) ;
#78104=CARTESIAN_POINT('Ctrl Pts',(-19.7294257177757,-45.8767102298418,
121.928426697249)) ;
#78105=CARTESIAN_POINT('Ctrl Pts',(-19.6654083759465,-45.696721149423,122.22511130924)) ;
#78106=CARTESIAN_POINT('Ctrl Pts',(-19.3810452958552,-45.8899976579907,
121.904492705502)) ;
#78107=CARTESIAN_POINT('Ctrl Pts',(-19.386670912546,-45.710008577572,122.205956446535)) ;
#78108=CARTESIAN_POINT('Ctrl Pts',(-19.1186091401468,-45.9000421976908,
121.932658290934)) ;
#78109=CARTESIAN_POINT('Ctrl Pts',(-19.1767289258844,-45.7200531172721,
122.228493281736)) ;
#78110=CARTESIAN_POINT('Ctrl Pts',(-18.8700233534811,-45.9098850395147,
122.004195045043)) ;
#78111=CARTESIAN_POINT('Ctrl Pts',(-18.9778591118884,-45.7298959590959,
122.285724283644)) ;
#78112=CARTESIAN_POINT('Ctrl Pts',(-18.6340661749748,-45.9198693237616,
122.118877741104)) ;
#78113=CARTESIAN_POINT('Ctrl Pts',(-18.7890948938155,-45.7398802433429,
122.377472601013)) ;
#78114=CARTESIAN_POINT('Ctrl Pts',(-18.4223444457329,-45.9298189691608,
122.272320772544)) ;
#78115=CARTESIAN_POINT('Ctrl Pts',(-18.6197187508759,-45.749829888742,122.500228781122)) ;
#78116=CARTESIAN_POINT('Ctrl Pts',(-18.2393318882481,-45.9398187308492,
122.460918444128)) ;
#78117=CARTESIAN_POINT('Ctrl Pts',(-18.4733104024896,-45.7598296504304,
122.65110845724)) ;
#78118=CARTESIAN_POINT('Ctrl Pts',(-18.0917505486385,-45.9498500768081,
122.679344429102)) ;
#78119=CARTESIAN_POINT('Ctrl Pts',(-18.3552472195982,-45.7698609963893,
122.825850469655)) ;
#78120=CARTESIAN_POINT('Ctrl Pts',(-17.9858757131845,-45.9597050312852,
122.915697061974)) ;
#78121=CARTESIAN_POINT('Ctrl Pts',(-18.2705494534768,-45.7797159508665,
123.014933412963)) ;
#78122=CARTESIAN_POINT('Ctrl Pts',(-17.9213083460047,-45.9696775692857,
123.169658598785)) ;
#78123=CARTESIAN_POINT('Ctrl Pts',(-18.218897762685,-45.789688488867,123.218103106479)) ;
#78124=CARTESIAN_POINT('Ctrl Pts',(-17.9017881316043,-45.9796725630207,
123.431630618321)) ;
#78125=CARTESIAN_POINT('Ctrl Pts',(-18.2032838339912,-45.7996834826019,
123.427680825471)) ;
#78126=CARTESIAN_POINT('Ctrl Pts',(-17.9284695514912,-45.9897066218148,
123.693939039822)) ;
#78127=CARTESIAN_POINT('Ctrl Pts',(-18.2246312126076,-45.809717541396,123.637527304085)) ;
#78128=CARTESIAN_POINT('Ctrl Pts',(-17.9986278341986,-45.9995619646378,
123.943270201428)) ;
#78129=CARTESIAN_POINT('Ctrl Pts',(-18.2807599457767,-45.819572884219,123.83699144443)) ;
#78130=CARTESIAN_POINT('Ctrl Pts',(-18.1123057056129,-46.0095614439834,
124.180132595311)) ;
#78131=CARTESIAN_POINT('Ctrl Pts',(-18.3717042256828,-45.8295723635646,
124.026480327799)) ;
#78132=CARTESIAN_POINT('Ctrl Pts',(-18.2635910838051,-46.0194558927387,
124.391666206139)) ;
#78133=CARTESIAN_POINT('Ctrl Pts',(-18.4927342046914,-45.8394668123199,
124.195705758367)) ;
#78134=CARTESIAN_POINT('Ctrl Pts',(-18.452459857194,-46.0295190121732,124.576699295131)) ;
#78135=CARTESIAN_POINT('Ctrl Pts',(-18.6438307990039,-45.8495299317544,
124.343730662622)) ;
#78136=CARTESIAN_POINT('Ctrl Pts',(-18.6656547762832,-46.0393586574144,
124.72309430415)) ;
#78137=CARTESIAN_POINT('Ctrl Pts',(-18.8143877068013,-45.8593695769957,
124.460844668667)) ;
#78138=CARTESIAN_POINT('Ctrl Pts',(-18.9061641632202,-46.0494218216005,
124.832954725834)) ;
#78139=CARTESIAN_POINT('Ctrl Pts',(-19.0067961563735,-45.8694327411817,
124.5487310367)) ;
#78140=CARTESIAN_POINT('Ctrl Pts',(-19.1579188976932,-46.0593160913493,
124.898075179744)) ;
#78141=CARTESIAN_POINT('Ctrl Pts',(-19.2082002369437,-45.8793270109305,
124.600825207935)) ;
#78142=CARTESIAN_POINT('Ctrl Pts',(-19.4182795982726,-46.0692578173631,
124.919290922773)) ;
#78143=CARTESIAN_POINT('Ctrl Pts',(-19.4164887608804,-45.8892687369444,
124.617795648672)) ;
#78144=CARTESIAN_POINT('Ctrl Pts',(-19.6800549446115,-46.0792607060225,
124.894933738413)) ;
#78145=CARTESIAN_POINT('Ctrl Pts',(-19.6259087706948,-45.8992716256037,
124.598307788373)) ;
#78146=CARTESIAN_POINT('Ctrl Pts',(-19.9343703358669,-46.0893005548165,
124.824788939951)) ;
#78147=CARTESIAN_POINT('Ctrl Pts',(-19.8293605316926,-45.9093114743977,
124.542189846149)) ;
#78148=CARTESIAN_POINT('Ctrl Pts',(-20.1678185634453,-46.0991247702773,
124.714495173591)) ;
#78149=CARTESIAN_POINT('Ctrl Pts',(-20.0161177505501,-45.9191356898586,
124.453953133522)) ;
#78150=CARTESIAN_POINT('Ctrl Pts',(-20.3837390423847,-46.1091816137709,
124.56213586375)) ;
#78151=CARTESIAN_POINT('Ctrl Pts',(-20.1888529869787,-45.9291925333521,
124.332063944319)) ;
#78152=CARTESIAN_POINT('Ctrl Pts',(-20.5673296044637,-46.1191102231669,
124.376727071072)) ;
#78153=CARTESIAN_POINT('Ctrl Pts',(-20.3357237457142,-45.9391211427481,
124.183735605175)) ;
#78154=CARTESIAN_POINT('Ctrl Pts',(-20.7168895336448,-46.1290621072048,
124.162174745033)) ;
#78155=CARTESIAN_POINT('Ctrl Pts',(-20.4553698831515,-45.949073026786,124.012092764765)) ;
#78156=CARTESIAN_POINT('Ctrl Pts',(-20.8275975548222,-46.1391150600124,
123.92232919589)) ;
#78157=CARTESIAN_POINT('Ctrl Pts',(-20.5439344348876,-45.9591259795936,
123.820215369618)) ;
#78158=CARTESIAN_POINT('Ctrl Pts',(-20.8939114403287,-46.1489379364785,
123.672837152812)) ;
#78159=CARTESIAN_POINT('Ctrl Pts',(-20.5969834127684,-45.9689488560598,
123.620621818295)) ;
#78160=CARTESIAN_POINT('Ctrl Pts',(-20.9168785395535,-46.1589936690487,
123.409601144835)) ;
#78161=CARTESIAN_POINT('Ctrl Pts',(-20.6153551246797,-45.9790045886299,
123.410032751232)) ;
#78162=CARTESIAN_POINT('Ctrl Pts',(-20.8935915401081,-46.1689344340363,
123.14939855817)) ;
#78163=CARTESIAN_POINT('Ctrl Pts',(-20.5967235160762,-45.9889453536176,
123.201871130652)) ;
#78164=CARTESIAN_POINT('Ctrl Pts',(-20.8265158341053,-46.178838766942,122.897909377588)) ;
#78165=CARTESIAN_POINT('Ctrl Pts',(-20.5430611920399,-45.9988496865232,
123.000680697245)) ;
#78166=CARTESIAN_POINT('Ctrl Pts',(-20.7150751052144,-46.1888854358227,
122.65859044673)) ;
#78167=CARTESIAN_POINT('Ctrl Pts',(-20.4539067994353,-46.0088963554039,
122.809226303556)) ;
#78168=CARTESIAN_POINT('Ctrl Pts',(-20.5662066576584,-46.1987809991285,
122.445321690462)) ;
#78169=CARTESIAN_POINT('Ctrl Pts',(-20.3348107319398,-46.0187919187097,
122.638612781793)) ;
#78170=CARTESIAN_POINT('Ctrl Pts',(-20.3795364262212,-46.2088430568288,
122.2580991555)) ;
#78171=CARTESIAN_POINT('Ctrl Pts',(-20.1854730795545,-46.02885397641,122.488836010064)) ;
#78172=CARTESIAN_POINT('Ctrl Pts',(-20.1679385536173,-46.2186858344563,
122.109285146135)) ;
#78173=CARTESIAN_POINT('Ctrl Pts',(-20.0161942548949,-46.0386967540375,
122.369786757822)) ;
#78174=CARTESIAN_POINT('Ctrl Pts',(-19.9305238988676,-46.2286763127081,
121.997288664803)) ;
#78175=CARTESIAN_POINT('Ctrl Pts',(-19.8262618842319,-46.0486872322894,
122.280191270744)) ;
#78176=CARTESIAN_POINT('Ctrl Pts',(-19.6787697821967,-46.2386052853517,
121.928664786083)) ;
#78177=CARTESIAN_POINT('Ctrl Pts',(-19.6248584943409,-46.0586162049329,
122.225294020736)) ;
#78178=CARTESIAN_POINT('Ctrl Pts',(-19.4173499655244,-46.2485964222312,
121.904240994582)) ;
#78179=CARTESIAN_POINT('Ctrl Pts',(-19.4157226100633,-46.0686073418125,
122.205756739917)) ;
#78180=CARTESIAN_POINT('Ctrl Pts',(-19.1548721753353,-46.2586185397202,
121.925962509157)) ;
#78181=CARTESIAN_POINT('Ctrl Pts',(-19.2057405118503,-46.0786294593014,
122.22313574868)) ;
#78182=CARTESIAN_POINT('Ctrl Pts',(-18.903182216174,-46.2685190501224,121.991878228726)) ;
#78183=CARTESIAN_POINT('Ctrl Pts',(-19.0043894985658,-46.0885299697036,
122.275869893625)) ;
#78184=CARTESIAN_POINT('Ctrl Pts',(-18.6644805817481,-46.2785080428685,
122.101090338697)) ;
#78185=CARTESIAN_POINT('Ctrl Pts',(-18.8134290284549,-46.0985189624497,
122.363241059296)) ;
#78186=CARTESIAN_POINT('Ctrl Pts',(-18.4489924496805,-46.2884732869191,
122.249880282416)) ;
#78187=CARTESIAN_POINT('Ctrl Pts',(-18.6410397168517,-46.1084842065003,
122.482274286718)) ;
#78188=CARTESIAN_POINT('Ctrl Pts',(-18.263300225065,-46.2983775514323,122.432284741279)) ;
#78189=CARTESIAN_POINT('Ctrl Pts',(-18.4924874591841,-46.1183884710135,
122.628198618205)) ;
#78190=CARTESIAN_POINT('Ctrl Pts',(-18.1099129936779,-46.3084356431305,
122.647513729993)) ;
#78191=CARTESIAN_POINT('Ctrl Pts',(-18.3697789069092,-46.1284465627118,
122.800382913545)) ;
#78192=CARTESIAN_POINT('Ctrl Pts',(-17.998387777928,-46.3182855835589,122.881119052178)) ;
#78193=CARTESIAN_POINT('Ctrl Pts',(-18.2805605437885,-46.1382965031402,
122.98726711269)) ;
#78194=CARTESIAN_POINT('Ctrl Pts',(-17.9272509866256,-46.3283125947325,
123.134829512523)) ;
#78195=CARTESIAN_POINT('Ctrl Pts',(-18.2236525328705,-46.1483235143137,
123.190235911234)) ;
#78196=CARTESIAN_POINT('Ctrl Pts',(-17.9019257693424,-46.3383411813445,
123.397163125625)) ;
#78197=CARTESIAN_POINT('Ctrl Pts',(-18.2033939634236,-46.1583521009257,
123.400103012758)) ;
#78198=CARTESIAN_POINT('Ctrl Pts',(-17.9216676871515,-46.3481863954572,
123.655117412468)) ;
#78199=CARTESIAN_POINT('Ctrl Pts',(-18.2191889474225,-46.1681973150384,
123.606465432505)) ;
#78200=CARTESIAN_POINT('Ctrl Pts',(-17.986172659598,-46.3581771436368,123.909622518297)) ;
#78201=CARTESIAN_POINT('Ctrl Pts',(-18.2707942272682,-46.178188063218,123.810069025763)) ;
#78202=CARTESIAN_POINT('Ctrl Pts',(-18.0949209307698,-46.3682147772222,
124.149940691099)) ;
#78203=CARTESIAN_POINT('Ctrl Pts',(-18.3577942543388,-46.1882256968035,
124.002323042482)) ;
#78204=CARTESIAN_POINT('Ctrl Pts',(-18.2405394895008,-46.3780600664351,
124.36379877282)) ;
#78205=CARTESIAN_POINT('Ctrl Pts',(-18.4742897414031,-46.1980709860163,
124.173407939844)) ;
#78206=CARTESIAN_POINT('Ctrl Pts',(-18.4231399413535,-46.3880414672409,
124.552075901783)) ;
#78207=CARTESIAN_POINT('Ctrl Pts',(-18.6203708816344,-46.2080523868222,
124.324028590119)) ;
#78208=CARTESIAN_POINT('Ctrl Pts',(-18.6350962163198,-46.3979937002309,
124.705303329943)) ;
#78209=CARTESIAN_POINT('Ctrl Pts',(-18.7899363575204,-46.2180046198121,
124.446609255118)) ;
#78210=CARTESIAN_POINT('Ctrl Pts',(-18.8714017008393,-46.4079925116875,
124.820247929174)) ;
#78211=CARTESIAN_POINT('Ctrl Pts',(-18.9789811859863,-46.2280034312688,
124.538563781757)) ;
#78212=CARTESIAN_POINT('Ctrl Pts',(-19.125198539865,-46.4180316156182,124.892209201569)) ;
#78213=CARTESIAN_POINT('Ctrl Pts',(-19.1820191456136,-46.2380425351995,
124.596131542575)) ;
#78214=CARTESIAN_POINT('Ctrl Pts',(-19.3820108279092,-46.4278565580375,
124.918993385685)) ;
#78215=CARTESIAN_POINT('Ctrl Pts',(-19.387468008186,-46.2478674776188,124.61755756467)) ;
#78216=CARTESIAN_POINT('Ctrl Pts',(-19.6455932892847,-46.4379112455134,
124.900789356812)) ;
#78217=CARTESIAN_POINT('Ctrl Pts',(-19.5983341049394,-46.2579221650947,
124.602993203772)) ;
#78218=CARTESIAN_POINT('Ctrl Pts',(-19.8990733415678,-46.4478540478703,
124.83736478161)) ;
#78219=CARTESIAN_POINT('Ctrl Pts',(-19.8011174177466,-46.2678649674515,
124.552252461191)) ;
#78220=CARTESIAN_POINT('Ctrl Pts',(-20.1370762828853,-46.45775784381,124.732039091005)) ;
#78221=CARTESIAN_POINT('Ctrl Pts',(-19.9915187270784,-46.2777687633913,
124.467991228943)) ;
#78222=CARTESIAN_POINT('Ctrl Pts',(-20.3561848751974,-46.4678046231851,
124.584777991466)) ;
#78223=CARTESIAN_POINT('Ctrl Pts',(-20.1668051376118,-46.2878155427663,
124.350181357414)) ;
#78224=CARTESIAN_POINT('Ctrl Pts',(-20.5437352890552,-46.4777002814797,
124.404584546191)) ;
#78225=CARTESIAN_POINT('Ctrl Pts',(-20.3168442299365,-46.2977112010609,
124.206026364736)) ;
#78226=CARTESIAN_POINT('Ctrl Pts',(-20.6997061795062,-46.4877618487303,
124.191114977076)) ;
#78227=CARTESIAN_POINT('Ctrl Pts',(-20.4416202696434,-46.3077727683115,
124.035249895047)) ;
#78228=CARTESIAN_POINT('Ctrl Pts',(-20.8137834733619,-46.4976064931676,
123.958907813351)) ;
#78229=CARTESIAN_POINT('Ctrl Pts',(-20.5328807279198,-46.3176174127489,
123.849484665839)) ;
#78230=CARTESIAN_POINT('Ctrl Pts',(-20.8875519245094,-46.5075665394103,
123.70778216214)) ;
#78231=CARTESIAN_POINT('Ctrl Pts',(-20.5918946247474,-46.3275774589915,
123.648584272298)) ;
#78232=CARTESIAN_POINT('Ctrl Pts',(-20.9163089328195,-46.5176048354286,
123.445571143075)) ;
#78233=CARTESIAN_POINT('Ctrl Pts',(-20.6148993352014,-46.3376157550099,
123.438815228034)) ;
#78234=CARTESIAN_POINT('Ctrl Pts',(-20.8998770458328,-46.527478176847,123.186591367231)) ;
#78235=CARTESIAN_POINT('Ctrl Pts',(-20.6017530884054,-46.3474890964282,
123.231632356186)) ;
#78236=CARTESIAN_POINT('Ctrl Pts',(-20.8374336991102,-46.5375512806463,
122.92940409919)) ;
#78237=CARTESIAN_POINT('Ctrl Pts',(-20.5517975371544,-46.3575622002275,
123.025882403029)) ;
#78238=CARTESIAN_POINT('Ctrl Pts',(-20.7341962066847,-46.5473720957652,
122.692815045751)) ;
#78239=CARTESIAN_POINT('Ctrl Pts',(-20.4692073631793,-46.3673830153464,
122.836612591769)) ;
#78240=CARTESIAN_POINT('Ctrl Pts',(-20.5880342150586,-46.5574489608432,
122.472055591204)) ;
#78241=CARTESIAN_POINT('Ctrl Pts',(-20.3522770187593,-46.3774598804244,
122.660005096316)) ;
#78242=CARTESIAN_POINT('Ctrl Pts',(-20.4094709147566,-46.5673137004984,
122.2840805988)) ;
#78243=CARTESIAN_POINT('Ctrl Pts',(-20.2094265518685,-46.3873246200797,
122.509626284042)) ;
#78244=CARTESIAN_POINT('Ctrl Pts',(-20.1980943114243,-46.5773361037398,
122.126973882659)) ;
#78245=CARTESIAN_POINT('Ctrl Pts',(-20.0403249282567,-46.397347023321,122.383941308971)) ;
#78246=CARTESIAN_POINT('Ctrl Pts',(-19.9622532730963,-46.5873618280283,
122.009494285036)) ;
#78247=CARTESIAN_POINT('Ctrl Pts',(-19.8516517311113,-46.4073727476095,
122.289958211651)) ;
#78248=CARTESIAN_POINT('Ctrl Pts',(-19.7140632034565,-46.5972166110496,
121.935594664528)) ;
#78249=CARTESIAN_POINT('Ctrl Pts',(-19.6531005311567,-46.4172275306308,
122.230839367749)) ;
#78250=CARTESIAN_POINT('Ctrl Pts',(-19.4536310994498,-46.6071954547728,
121.90485653267)) ;
#78251=CARTESIAN_POINT('Ctrl Pts',(-19.4447550642986,-46.4272063743541,
122.206249292798)) ;
#78252=CARTESIAN_POINT('Ctrl Pts',(-19.1908123744506,-46.6172143470095,
121.920317600712)) ;
#78253=CARTESIAN_POINT('Ctrl Pts',(-19.2345001020312,-46.4372252665907,
122.218618661177)) ;
#78254=CARTESIAN_POINT('Ctrl Pts',(-18.9379696063757,-46.6270975560505,
121.97984075854)) ;
#78255=CARTESIAN_POINT('Ctrl Pts',(-19.0322268301204,-46.4471084756317,
122.266237355114)) ;
#78256=CARTESIAN_POINT('Ctrl Pts',(-18.6949496716239,-46.6371658653907,
122.084353103982)) ;
#78257=CARTESIAN_POINT('Ctrl Pts',(-18.8378107414872,-46.4571767849719,
122.349847736102)) ;
#78258=CARTESIAN_POINT('Ctrl Pts',(-18.4787605240188,-46.6469959907234,
122.225836194855)) ;
#78259=CARTESIAN_POINT('Ctrl Pts',(-18.6648606358559,-46.4670069103046,
122.463033810365)) ;
#78260=CARTESIAN_POINT('Ctrl Pts',(-18.2857214965471,-46.6570625431004,
122.406651152133)) ;
#78261=CARTESIAN_POINT('Ctrl Pts',(-18.5104293493474,-46.4770734626816,
122.607686172701)) ;
#78262=CARTESIAN_POINT('Ctrl Pts',(-18.1298739185928,-46.6669527799941,
122.614687511518)) ;
#78263=CARTESIAN_POINT('Ctrl Pts',(-18.3857520197668,-46.4869636995753,
122.774114761019)) ;
#78264=CARTESIAN_POINT('Ctrl Pts',(-18.0108157652608,-46.6769450047881,
122.848713195594)) ;
#78265=CARTESIAN_POINT('Ctrl Pts',(-18.2905057011773,-46.4969559243693,
122.96133522007)) ;
#78266=CARTESIAN_POINT('Ctrl Pts',(-17.9346569101183,-46.686907625139,123.099193972025)) ;
#78267=CARTESIAN_POINT('Ctrl Pts',(-18.2295789196735,-46.5069185447203,
123.161719551088)) ;
#78268=CARTESIAN_POINT('Ctrl Pts',(-17.9026865141076,-46.6968126279022,
123.357534213857)) ;
#78269=CARTESIAN_POINT('Ctrl Pts',(-18.2040027337092,-46.5168235474834,
123.368391006395)) ;
#78270=CARTESIAN_POINT('Ctrl Pts',(-17.9164439567275,-46.7068703903003,
123.621460054298)) ;
#78271=CARTESIAN_POINT('Ctrl Pts',(-18.2150087894346,-46.5268813098816,
123.579531944023)) ;
#78272=CARTESIAN_POINT('Ctrl Pts',(-17.9743972614119,-46.7167209096791,
123.873771940595)) ;
#78273=CARTESIAN_POINT('Ctrl Pts',(-18.2613712111539,-46.5367318292604,
123.781380349578)) ;
#78274=CARTESIAN_POINT('Ctrl Pts',(-18.0765858906852,-46.7267524866773,
124.116760874198)) ;
#78275=CARTESIAN_POINT('Ctrl Pts',(-18.343122043701,-46.5467634062585,123.97577162832)) ;
#78276=CARTESIAN_POINT('Ctrl Pts',(-18.2195527491153,-46.7367622217822,
124.337596889002)) ;
#78277=CARTESIAN_POINT('Ctrl Pts',(-18.4574955266173,-46.5567731413635,
124.15244040257)) ;
#78278=CARTESIAN_POINT('Ctrl Pts',(-18.3966970018278,-46.7466717984085,
124.528446109124)) ;
#78279=CARTESIAN_POINT('Ctrl Pts',(-18.5992104071735,-46.5666827179897,
124.30511928162)) ;
#78280=CARTESIAN_POINT('Ctrl Pts',(-18.6042842737798,-46.7565991842651,
124.686473857412)) ;
#78281=CARTESIAN_POINT('Ctrl Pts',(-18.7652796215495,-46.5766101038464,
124.431541287681)) ;
#78282=CARTESIAN_POINT('Ctrl Pts',(-18.8389799600408,-46.7666441187554,
124.807271873862)) ;
#78283=CARTESIAN_POINT('Ctrl Pts',(-18.9530362508393,-46.5866550383367,
124.528179918756)) ;
#78284=CARTESIAN_POINT('Ctrl Pts',(-19.0870750670497,-46.7765300509434,
124.884401576639)) ;
#78285=CARTESIAN_POINT('Ctrl Pts',(-19.1515114465665,-46.5965409705246,
124.589883612155)) ;
#78286=CARTESIAN_POINT('Ctrl Pts',(-19.3475046537305,-46.7865233568964,
124.918084459539)) ;
#78287=CARTESIAN_POINT('Ctrl Pts',(-19.3598549143501,-46.6065342764777,
124.616830206673)) ;
#78288=CARTESIAN_POINT('Ctrl Pts',(-19.6085865454019,-46.7964689946783,
124.905990634187)) ;
#78289=CARTESIAN_POINT('Ctrl Pts',(-19.5687199653506,-46.6164799142595,
124.607155453148)) ;
#78290=CARTESIAN_POINT('Ctrl Pts',(-19.8637733414105,-46.8064162630242,
124.849258887839)) ;
#78291=CARTESIAN_POINT('Ctrl Pts',(-19.7728690447604,-46.6264271826054,
124.561770566073)) ;
#78292=CARTESIAN_POINT('Ctrl Pts',(-20.1075420667497,-46.8164641651613,
124.747800719741)) ;
#78293=CARTESIAN_POINT('Ctrl Pts',(-19.9678843424592,-46.6364750847425,
124.480604273047)) ;
#78294=CARTESIAN_POINT('Ctrl Pts',(-20.3256846822347,-46.8263118600015,
124.608569806592)) ;
#78295=CARTESIAN_POINT('Ctrl Pts',(-20.1423977064483,-46.6463227795827,
124.369220481856)) ;
#78296=CARTESIAN_POINT('Ctrl Pts',(-20.5190914281009,-46.8362733697459,
124.432171593208)) ;
#78297=CARTESIAN_POINT('Ctrl Pts',(-20.297123242795,-46.6562842893271,124.2281026054)) ;
#78298=CARTESIAN_POINT('Ctrl Pts',(-20.679753909111,-46.8463027613547,124.223227378261)) ;
#78299=CARTESIAN_POINT('Ctrl Pts',(-20.42565368723,-46.666313680936,124.060947484944)) ;
#78300=CARTESIAN_POINT('Ctrl Pts',(-20.8003366055936,-46.8562102569095,
123.992472885765)) ;
#78301=CARTESIAN_POINT('Ctrl Pts',(-20.5221200032968,-46.6762211764908,
123.876344781865)) ;
#78302=CARTESIAN_POINT('Ctrl Pts',(-20.8798121650525,-46.8661556485725,
123.743517316014)) ;
#78303=CARTESIAN_POINT('Ctrl Pts',(-20.5857009581305,-46.6861665681538,
123.6771809766)) ;
#78304=CARTESIAN_POINT('Ctrl Pts',(-20.9152146258605,-46.8761575661699,
123.483036674984)) ;
#78305=CARTESIAN_POINT('Ctrl Pts',(-20.614023626857,-46.6961684857511,123.468796661138)) ;
#78306=CARTESIAN_POINT('Ctrl Pts',(-20.9043274470116,-46.8861976337221,
123.219443241595)) ;
#78307=CARTESIAN_POINT('Ctrl Pts',(-20.605314478917,-46.7062085533033,123.257921751627)) ;
#78308=CARTESIAN_POINT('Ctrl Pts',(-20.8496146261628,-46.8960219451619,
122.967111685202)) ;
#78309=CARTESIAN_POINT('Ctrl Pts',(-20.5615452065626,-46.7160328647431,
123.056057541106)) ;
#78310=CARTESIAN_POINT('Ctrl Pts',(-20.7499690604386,-46.906078186318,122.722378927974)) ;
#78311=CARTESIAN_POINT('Ctrl Pts',(-20.481829431188,-46.7260891058992,122.860270789842)) ;
#78312=CARTESIAN_POINT('Ctrl Pts',(-20.6108065948764,-46.9160091080536,
122.501569334486)) ;
#78313=CARTESIAN_POINT('Ctrl Pts',(-20.3705003850126,-46.7360200276349,
122.683623170689)) ;
#78314=CARTESIAN_POINT('Ctrl Pts',(-20.4356383206303,-46.9259523441298,
122.307725777392)) ;
#78315=CARTESIAN_POINT('Ctrl Pts',(-20.2303667445202,-46.7459632637111,
122.528548091162)) ;
#78316=CARTESIAN_POINT('Ctrl Pts',(-20.2287819479569,-46.9359336281423,
122.146383450033)) ;
#78317=CARTESIAN_POINT('Ctrl Pts',(-20.0648823935122,-46.7559445477236,
122.399473615786)) ;
#78318=CARTESIAN_POINT('Ctrl Pts',(-19.9954418662729,-46.945977929768,122.02306909361)) ;
#78319=CARTESIAN_POINT('Ctrl Pts',(-19.8782105832335,-46.7659888493492,
122.300821320702)) ;
#78320=CARTESIAN_POINT('Ctrl Pts',(-19.7497569427487,-46.9558060109874,
121.943291660732)) ;
#78321=CARTESIAN_POINT('Ctrl Pts',(-19.6816640439892,-46.7758169305687,
122.236998801319)) ;
#78322=CARTESIAN_POINT('Ctrl Pts',(-19.4875976586558,-46.9658826138366,
121.906362635557)) ;
#78323=CARTESIAN_POINT('Ctrl Pts',(-19.4719364151813,-46.7858935334178,
122.207454534728)) ;
#78324=CARTESIAN_POINT('Ctrl Pts',(-19.2287886486828,-46.9757346929551,
121.915184765321)) ;
#78325=CARTESIAN_POINT('Ctrl Pts',(-19.2648901580032,-46.7957456125364,
122.214511170181)) ;
#78326=CARTESIAN_POINT('Ctrl Pts',(-18.9698079849052,-46.985807951264,121.969772870526)) ;
#78327=CARTESIAN_POINT('Ctrl Pts',(-19.0577050887598,-46.8058188708453,
122.258180656131)) ;
#78328=CARTESIAN_POINT('Ctrl Pts',(-18.7298606158463,-46.9956494106443,
122.066316849494)) ;
#78329=CARTESIAN_POINT('Ctrl Pts',(-18.8657477611846,-46.8156603302256,
122.335414457744)) ;
#78330=CARTESIAN_POINT('Ctrl Pts',(-18.507158497472,-47.0056105060567,122.203869923483)) ;
#78331=CARTESIAN_POINT('Ctrl Pts',(-18.6875856641331,-46.8256214256379,
122.445455650075)) ;
#78332=CARTESIAN_POINT('Ctrl Pts',(-18.3105700405973,-47.0156477904534,
122.379722097199)) ;
#78333=CARTESIAN_POINT('Ctrl Pts',(-18.5303140387269,-46.8356587100347,
122.586136582411)) ;
#78334=CARTESIAN_POINT('Ctrl Pts',(-18.1497383799776,-47.0255241291887,
122.583459652744)) ;
#78335=CARTESIAN_POINT('Ctrl Pts',(-18.4016482050606,-46.8455350487699,
122.749125213228)) ;
#78336=CARTESIAN_POINT('Ctrl Pts',(-18.0243973838488,-47.0355862553419,
122.816248967661)) ;
#78337=CARTESIAN_POINT('Ctrl Pts',(-18.3013741678358,-46.8555971749232,
122.935356256442)) ;
#78338=CARTESIAN_POINT('Ctrl Pts',(-17.942900261106,-47.0454544293185,123.062469015804)) ;
#78339=CARTESIAN_POINT('Ctrl Pts',(-18.2361754986026,-46.8654653488997,
123.132331099916)) ;
#78340=CARTESIAN_POINT('Ctrl Pts',(-17.9043551711864,-47.0554599778223,
123.322528432359)) ;
#78341=CARTESIAN_POINT('Ctrl Pts',(-18.2053380449325,-46.8754708974035,
123.340378359643)) ;
#78342=CARTESIAN_POINT('Ctrl Pts',(-17.9116262441301,-47.0654426097179,
123.584808795431)) ;
#78343=CARTESIAN_POINT('Ctrl Pts',(-18.2111535111412,-46.8854535292991,
123.55020250964)) ;
#78344=CARTESIAN_POINT('Ctrl Pts',(-17.9649058187744,-47.0754865521397,
123.843296984573)) ;
#78345=CARTESIAN_POINT('Ctrl Pts',(-18.2537758946358,-46.8954974717209,
123.756993455038)) ;
#78346=CARTESIAN_POINT('Ctrl Pts',(-18.0598529384755,-47.0853147001668,
124.083485382838)) ;
#78347=CARTESIAN_POINT('Ctrl Pts',(-18.3297319083217,-46.9053256197481,
123.949143731469)) ;
#78348=CARTESIAN_POINT('Ctrl Pts',(-18.1965689478695,-47.0953045675412,
124.307600675778)) ;
#78349=CARTESIAN_POINT('Ctrl Pts',(-18.4391033021549,-46.9153154871225,
124.128436666438)) ;
#78350=CARTESIAN_POINT('Ctrl Pts',(-18.3715713483997,-47.1053483064967,
124.505180389763)) ;
#78351=CARTESIAN_POINT('Ctrl Pts',(-18.5791042261939,-46.925359226078,124.286501476418)) ;
#78352=CARTESIAN_POINT('Ctrl Pts',(-18.5733188648225,-47.1151700550347,
124.666164420657)) ;
#78353=CARTESIAN_POINT('Ctrl Pts',(-18.7405004989235,-46.9351809746159,
124.41528928464)) ;
#78354=CARTESIAN_POINT('Ctrl Pts',(-18.8045645527925,-47.1252050326444,
124.792922450464)) ;
#78355=CARTESIAN_POINT('Ctrl Pts',(-18.9254963238758,-46.9452159522256,
124.516697207204)) ;
#78356=CARTESIAN_POINT('Ctrl Pts',(-19.0542980945305,-47.1352299454021,
124.87682516273)) ;
#78357=CARTESIAN_POINT('Ctrl Pts',(-19.1252826902165,-46.9552408649833,
124.583820828544)) ;
#78358=CARTESIAN_POINT('Ctrl Pts',(-19.3102255315823,-47.1450818884959,
124.915973694031)) ;
#78359=CARTESIAN_POINT('Ctrl Pts',(-19.3300235960743,-46.9650928080772,
124.615141143761)) ;
#78360=CARTESIAN_POINT('Ctrl Pts',(-19.5726863790216,-47.155072849825,124.910409512918)) ;
#78361=CARTESIAN_POINT('Ctrl Pts',(-19.5399921733102,-46.9750837694063,
124.61069150596)) ;
#78362=CARTESIAN_POINT('Ctrl Pts',(-19.8284072327493,-47.1649907246935,
124.859887472804)) ;
#78363=CARTESIAN_POINT('Ctrl Pts',(-19.7445687433349,-46.9850016442747,
124.570275659941)) ;
#78364=CARTESIAN_POINT('Ctrl Pts',(-20.0741511052673,-47.1750192436947,
124.764752235733)) ;
#78365=CARTESIAN_POINT('Ctrl Pts',(-19.9411644966269,-46.9950301632759,
124.494169084387)) ;
#78366=CARTESIAN_POINT('Ctrl Pts',(-20.2964844790249,-47.1849029224925,
124.630459757741)) ;
#78367=CARTESIAN_POINT('Ctrl Pts',(-20.1190316002392,-47.0049138420738,
124.386736915918)) ;
#78368=CARTESIAN_POINT('Ctrl Pts',(-20.4946972414239,-47.1948978659322,
124.45812275425)) ;
#78369=CARTESIAN_POINT('Ctrl Pts',(-20.2776029447661,-47.0149087855135,
124.248868788224)) ;
#78370=CARTESIAN_POINT('Ctrl Pts',(-20.6601527761512,-47.2049247197547,
124.253049913834)) ;
#78371=CARTESIAN_POINT('Ctrl Pts',(-20.4099687724888,-47.0249356393359,
124.084811622413)) ;
#78372=CARTESIAN_POINT('Ctrl Pts',(-20.7859931801088,-47.2148088840936,
124.025810555401)) ;
#78373=CARTESIAN_POINT('Ctrl Pts',(-20.5106424360365,-47.0348198036749,
123.90302151066)) ;
#78374=CARTESIAN_POINT('Ctrl Pts',(-20.8716717235175,-47.224796982136,123.777738571877)) ;
#78375=CARTESIAN_POINT('Ctrl Pts',(-20.5791870192374,-47.0448079017172,
123.704564663885)) ;
#78376=CARTESIAN_POINT('Ctrl Pts',(-20.9129754353913,-47.2347480885931,
123.519483140435)) ;
#78377=CARTESIAN_POINT('Ctrl Pts',(-20.6122318336066,-47.0547590081743,
123.497960883868)) ;
#78378=CARTESIAN_POINT('Ctrl Pts',(-20.9086243004651,-47.2447931397612,
123.255561025819)) ;
#78379=CARTESIAN_POINT('Ctrl Pts',(-20.6087528155346,-47.0648040593424,
123.286823089854)) ;
#78380=CARTESIAN_POINT('Ctrl Pts',(-20.8595658746091,-47.2546549001195,
123.001088343686)) ;
#78381=CARTESIAN_POINT('Ctrl Pts',(-20.5695080656259,-47.0746658197007,
123.083245164195)) ;
#78382=CARTESIAN_POINT('Ctrl Pts',(-20.7668750533367,-47.2646177169499,
122.756231591788)) ;
#78383=CARTESIAN_POINT('Ctrl Pts',(-20.4953573697405,-47.0846286365312,
122.887359233057)) ;
#78384=CARTESIAN_POINT('Ctrl Pts',(-20.6317297454447,-47.2746523982307,
122.529807845328)) ;
#78385=CARTESIAN_POINT('Ctrl Pts',(-20.3872427942103,-47.0946633178119,
122.706219207797)) ;
#78386=CARTESIAN_POINT('Ctrl Pts',(-20.4621990513722,-47.2845374280114,
122.332938363935)) ;
#78387=CARTESIAN_POINT('Ctrl Pts',(-20.2516200615866,-47.1045483475927,
122.548722648107)) ;
#78388=CARTESIAN_POINT('Ctrl Pts',(-20.2574099722964,-47.2946030214095,
122.165588379843)) ;
#78389=CARTESIAN_POINT('Ctrl Pts',(-20.0877899799016,-47.1146139409907,
122.414841027643)) ;
#78390=CARTESIAN_POINT('Ctrl Pts',(-20.0319196600013,-47.304442189771,122.038978242799)) ;
#78391=CARTESIAN_POINT('Ctrl Pts',(-19.9073992209969,-47.1244531093522,
122.313551415424)) ;
#78392=CARTESIAN_POINT('Ctrl Pts',(-19.782518300832,-47.3145047875124,121.951182502159)) ;
#78393=CARTESIAN_POINT('Ctrl Pts',(-19.7078787262288,-47.1345157070937,
122.243312822989)) ;
#78394=CARTESIAN_POINT('Ctrl Pts',(-19.5258624977705,-47.3244017999194,
121.909002520916)) ;
#78395=CARTESIAN_POINT('Ctrl Pts',(-19.502554784226,-47.1444127195006,122.209566874311)) ;
#78396=CARTESIAN_POINT('Ctrl Pts',(-19.2648924723444,-47.334333121745,121.911168475281)) ;
#78397=CARTESIAN_POINT('Ctrl Pts',(-19.2937789864561,-47.1543440413262,
122.211297494334)) ;
#78398=CARTESIAN_POINT('Ctrl Pts',(-19.0054588236184,-47.3443748844995,
121.959423773116)) ;
#78399=CARTESIAN_POINT('Ctrl Pts',(-19.0862316578282,-47.1643858040807,
122.249899661236)) ;
#78400=CARTESIAN_POINT('Ctrl Pts',(-18.7620408415113,-47.3542630833902,
122.050409572589)) ;
#78401=CARTESIAN_POINT('Ctrl Pts',(-18.8914968446578,-47.1742740029714,
122.322686186617)) ;
#78402=CARTESIAN_POINT('Ctrl Pts',(-18.5355442147044,-47.36425702199,122.183311500813)) ;
#78403=CARTESIAN_POINT('Ctrl Pts',(-18.7102985172249,-47.1842679415713,
122.429005819235)) ;
#78404=CARTESIAN_POINT('Ctrl Pts',(-18.3366094811182,-47.3741978430269,
122.352654795941)) ;
#78405=CARTESIAN_POINT('Ctrl Pts',(-18.551149473623,-47.1942087626082,122.564478686452)) ;
#78406=CARTESIAN_POINT('Ctrl Pts',(-18.1695526329319,-47.3841572253151,
122.554106931981)) ;
#78407=CARTESIAN_POINT('Ctrl Pts',(-18.417502400572,-47.2041681448964,122.725638889882)) ;
#78408=CARTESIAN_POINT('Ctrl Pts',(-18.0393553531157,-47.3941549849675,
122.782338451479)) ;
#78409=CARTESIAN_POINT('Ctrl Pts',(-18.3133427031119,-47.2141659045487,
122.908222957332)) ;
#78410=CARTESIAN_POINT('Ctrl Pts',(-17.9507774144696,-47.4041911211698,
123.030750867637)) ;
#78411=CARTESIAN_POINT('Ctrl Pts',(-18.2424783105885,-47.224202040751,123.106952144432)) ;
#78412=CARTESIAN_POINT('Ctrl Pts',(-17.9071905132183,-47.4140419186607,
123.285921661665)) ;
#78413=CARTESIAN_POINT('Ctrl Pts',(-18.2076066786079,-47.2340528382419,
123.311088103092)) ;
#78414=CARTESIAN_POINT('Ctrl Pts',(-17.9078079176154,-47.424002783737,123.547672833058)) ;
#78415=CARTESIAN_POINT('Ctrl Pts',(-18.2080983638521,-47.2440137033182,
123.520488944659)) ;
#78416=CARTESIAN_POINT('Ctrl Pts',(-17.9544972056364,-47.4340316513674,
123.807067402993)) ;
#78417=CARTESIAN_POINT('Ctrl Pts',(-18.2454476048845,-47.2540425709486,
123.728004959381)) ;
#78418=CARTESIAN_POINT('Ctrl Pts',(-18.04435585215,-47.4439418875038,124.051493099934)) ;
#78419=CARTESIAN_POINT('Ctrl Pts',(-18.3173323750563,-47.263952807085,123.923546127263)) ;
#78420=CARTESIAN_POINT('Ctrl Pts',(-18.1750338401963,-47.4538768408183,
124.277524030933)) ;
#78421=CARTESIAN_POINT('Ctrl Pts',(-18.4218727658216,-47.2738877603996,
124.10437190683)) ;
#78422=CARTESIAN_POINT('Ctrl Pts',(-18.3449402388799,-47.4639177712279,
124.479398422779)) ;
#78423=CARTESIAN_POINT('Ctrl Pts',(-18.5577961461573,-47.2839286908091,
124.265872834734)) ;
#78424=CARTESIAN_POINT('Ctrl Pts',(-18.5441394208456,-47.4738056680095,
124.64626268792)) ;
#78425=CARTESIAN_POINT('Ctrl Pts',(-18.717153951654,-47.2938165875907,124.399365886383)) ;
#78426=CARTESIAN_POINT('Ctrl Pts',(-18.7713398491189,-47.4837951196682,
124.777752129338)) ;
#78427=CARTESIAN_POINT('Ctrl Pts',(-18.8989131176986,-47.3038060392494,
124.504559363541)) ;
#78428=CARTESIAN_POINT('Ctrl Pts',(-19.0172406223809,-47.4937542100335,
124.867323859669)) ;
#78429=CARTESIAN_POINT('Ctrl Pts',(-19.0956328934438,-47.3137651296148,
124.576218838424)) ;
#78430=CARTESIAN_POINT('Ctrl Pts',(-19.2732681589841,-47.5036515223399,
124.913214982572)) ;
#78431=CARTESIAN_POINT('Ctrl Pts',(-19.3004544847699,-47.3236624419211,
124.612933948275)) ;
#78432=CARTESIAN_POINT('Ctrl Pts',(-19.5375180334374,-47.5137079482401,
124.913840319069)) ;
#78433=CARTESIAN_POINT('Ctrl Pts',(-19.5118543105369,-47.3337188678213,
124.613436469234)) ;
#78434=CARTESIAN_POINT('Ctrl Pts',(-19.7931038035364,-47.5235779508299,
124.86953541512)) ;
#78435=CARTESIAN_POINT('Ctrl Pts',(-19.7163232953093,-47.3435888704111,
124.577994777982)) ;
#78436=CARTESIAN_POINT('Ctrl Pts',(-20.0405538778999,-47.5335818840071,
124.780842159474)) ;
#78437=CARTESIAN_POINT('Ctrl Pts',(-19.9142841000956,-47.3535928035883,
124.507042257219)) ;
#78438=CARTESIAN_POINT('Ctrl Pts',(-20.2684557085734,-47.543569144471,124.650592871709)) ;
#78439=CARTESIAN_POINT('Ctrl Pts',(-20.096606520165,-47.3635800640522,124.402844965088)) ;
#78440=CARTESIAN_POINT('Ctrl Pts',(-20.470938720647,-47.5535961960567,124.48200287069)) ;
#78441=CARTESIAN_POINT('Ctrl Pts',(-20.2585947483738,-47.3736071156379,
124.267974120626)) ;
#78442=CARTESIAN_POINT('Ctrl Pts',(-20.6389889195146,-47.5634872858828,
124.283677447636)) ;
#78443=CARTESIAN_POINT('Ctrl Pts',(-20.3930350147794,-47.383498205464,124.109317524504)) ;
#78444=CARTESIAN_POINT('Ctrl Pts',(-20.8155222737349,-47.5767850406638,
123.982153460003)) ;
#78445=CARTESIAN_POINT('Ctrl Pts',(-20.5342723572746,-47.3967959602451,
123.86808831075)) ;
#78446=CARTESIAN_POINT('Ctrl Pts',(-20.9091627272302,-47.589983100272,123.644050843678)) ;
#78447=CARTESIAN_POINT('Ctrl Pts',(-20.6091851817961,-47.4099940198532,
123.597577609492)) ;
#78448=CARTESIAN_POINT('Ctrl Pts',(-20.9119614688863,-47.6033798408412,
123.292030999212)) ;
#78449=CARTESIAN_POINT('Ctrl Pts',(-20.6114219138469,-47.4233907604224,
123.316008249511)) ;
#78450=CARTESIAN_POINT('Ctrl Pts',(-20.8692234170747,-47.6132507529146,
123.036128094881)) ;
#78451=CARTESIAN_POINT('Ctrl Pts',(-20.5772346237464,-47.4332616724959,
123.111276038365)) ;
#78452=CARTESIAN_POINT('Ctrl Pts',(-20.7809529679851,-47.6233243146827,
122.786617518481)) ;
#78453=CARTESIAN_POINT('Ctrl Pts',(-20.5066201804174,-47.443335234264,122.911669620032)) ;
#78454=CARTESIAN_POINT('Ctrl Pts',(-20.6541739490914,-47.6331457272711,
122.561735103864)) ;
#78455=CARTESIAN_POINT('Ctrl Pts',(-20.405198506557,-47.4531566468523,122.731761296753)) ;
#78456=CARTESIAN_POINT('Ctrl Pts',(-20.4863320286393,-47.6432197445021,
122.357091382096)) ;
#78457=CARTESIAN_POINT('Ctrl Pts',(-20.2709276233739,-47.4632306640834,
122.568046598626)) ;
#78458=CARTESIAN_POINT('Ctrl Pts',(-20.2240587467642,-47.6563785314667,
122.13161591523)) ;
#78459=CARTESIAN_POINT('Ctrl Pts',(-20.0611061721674,-47.4763894510479,
122.387657331464)) ;
#78460=CARTESIAN_POINT('Ctrl Pts',(-19.9043966118388,-47.6697446345609,
121.976897634907)) ;
#78461=CARTESIAN_POINT('Ctrl Pts',(-19.8053424387584,-47.4897555541421,
122.263873680573)) ;
#78462=CARTESIAN_POINT('Ctrl Pts',(-19.5604802160081,-47.6830585694499,
121.912018372338)) ;
#78463=CARTESIAN_POINT('Ctrl Pts',(-19.5302562121692,-47.5030694890312,
122.211981762191)) ;
#78464=CARTESIAN_POINT('Ctrl Pts',(-19.3003815270674,-47.6929586088974,
121.90833318309)) ;
#78465=CARTESIAN_POINT('Ctrl Pts',(-19.322167620802,-47.5129695284786,122.209028724385)) ;
#78466=CARTESIAN_POINT('Ctrl Pts',(-19.041800524058,-47.7029230120319,121.949706845945)) ;
#78467=CARTESIAN_POINT('Ctrl Pts',(-19.1153050560258,-47.5229339316132,
122.242126300754)) ;
#78468=CARTESIAN_POINT('Ctrl Pts',(-18.7927924421726,-47.712952979153,122.036134213091)) ;
#78469=CARTESIAN_POINT('Ctrl Pts',(-18.9160968262407,-47.5329638987343,
122.311266676217)) ;
#78470=CARTESIAN_POINT('Ctrl Pts',(-18.5654632173557,-47.7228552557621,
122.162745640251)) ;
#78471=CARTESIAN_POINT('Ctrl Pts',(-18.734234498539,-47.5428661753434,122.412551849973)) ;
#78472=CARTESIAN_POINT('Ctrl Pts',(-18.2943866085651,-47.7361211849313,
122.382011147365)) ;
#78473=CARTESIAN_POINT('Ctrl Pts',(-18.5173605390981,-47.5561321045125,
122.587974585937)) ;
#78474=CARTESIAN_POINT('Ctrl Pts',(-18.0346303796322,-47.7527427160376,
122.739250673767)) ;
#78475=CARTESIAN_POINT('Ctrl Pts',(-18.3095657843141,-47.5727536356189,
122.873754271504)) ;
#78476=CARTESIAN_POINT('Ctrl Pts',(-17.8876997700459,-47.7726175446823,
123.246720784375)) ;
#78477=CARTESIAN_POINT('Ctrl Pts',(-18.192010176043,-47.5926284642636,123.27971738618)) ;
#78478=CARTESIAN_POINT('Ctrl Pts',(-17.9170005926413,-47.7892907527842,
123.688848718137)) ;
#78479=CARTESIAN_POINT('Ctrl Pts',(-18.2154597786599,-47.6093016723655,
123.63347188355)) ;
#78480=CARTESIAN_POINT('Ctrl Pts',(-18.0293936751226,-47.8025418777655,
124.018462677724)) ;
#78481=CARTESIAN_POINT('Ctrl Pts',(-18.305361509496,-47.6225527973467,123.897116801206)) ;
#78482=CARTESIAN_POINT('Ctrl Pts',(-18.1961054879698,-47.8157841965863,
124.323995100804)) ;
#78483=CARTESIAN_POINT('Ctrl Pts',(-18.4387378061925,-47.6357951161676,
124.141559984397)) ;
#78484=CARTESIAN_POINT('Ctrl Pts',(-18.5033373266332,-47.8325174369258,
124.645448284641)) ;
#78485=CARTESIAN_POINT('Ctrl Pts',(-18.6845128198436,-47.652528356507,124.398713602975)) ;
#78486=CARTESIAN_POINT('Ctrl Pts',(-18.9757346113062,-47.8523465851138,
124.87933604937)) ;
#78487=CARTESIAN_POINT('Ctrl Pts',(-19.0624327890952,-47.672357504695,124.585830613588)) ;
#78488=CARTESIAN_POINT('Ctrl Pts',(-19.5017537469011,-47.8722712802144,
124.9395166783)) ;
#78489=CARTESIAN_POINT('Ctrl Pts',(-19.4832476587856,-47.6922821997956,
124.633977069387)) ;
#78490=CARTESIAN_POINT('Ctrl Pts',(-20.0168758619817,-47.8921945087978,
124.816493222179)) ;
#78491=CARTESIAN_POINT('Ctrl Pts',(-19.8953467115458,-47.7122054283791,
124.535561030838)) ;
#78492=CARTESIAN_POINT('Ctrl Pts',(-20.4591503181284,-47.9121216479239,
124.525228376987)) ;
#78493=CARTESIAN_POINT('Ctrl Pts',(-20.2491681384619,-47.7321325675052,
124.302550855083)) ;
#78494=CARTESIAN_POINT('Ctrl Pts',(-20.7752836477804,-47.9319981105396,
124.101934449812)) ;
#78495=CARTESIAN_POINT('Ctrl Pts',(-20.5020771966928,-47.7520090301208,
123.963916114928)) ;
#78496=CARTESIAN_POINT('Ctrl Pts',(-20.9290246639703,-47.9519753391449,
123.59372436111)) ;
#78497=CARTESIAN_POINT('Ctrl Pts',(-20.6250718773028,-47.7719862587261,
123.557348393509)) ;
#78498=CARTESIAN_POINT('Ctrl Pts',(-20.8997496415045,-47.9719101971186,
123.064652071542)) ;
#78499=CARTESIAN_POINT('Ctrl Pts',(-20.6016537118098,-47.7919211166998,
123.134089837888)) ;
#78500=CARTESIAN_POINT('Ctrl Pts',(-20.6926191392944,-47.9918066460494,
122.578134849527)) ;
#78501=CARTESIAN_POINT('Ctrl Pts',(-20.4359502844163,-47.8118175656306,
122.744874452236)) ;
#78502=CARTESIAN_POINT('Ctrl Pts',(-20.331839327964,-48.011727930116,122.1905714448)) ;
#78503=CARTESIAN_POINT('Ctrl Pts',(-20.147326663776,-47.8317388496972,122.434822343269)) ;
#78504=CARTESIAN_POINT('Ctrl Pts',(-19.8595433796949,-48.0316845797869,
121.949105900336)) ;
#78505=CARTESIAN_POINT('Ctrl Pts',(-19.7694899560227,-47.8516954993682,
122.241648817227)) ;
#78506=CARTESIAN_POINT('Ctrl Pts',(-19.3354077539435,-48.0515618728986,
121.883411775876)) ;
#78507=CARTESIAN_POINT('Ctrl Pts',(-19.3501800444516,-47.8715727924798,
122.189092575261)) ;
#78508=CARTESIAN_POINT('Ctrl Pts',(-18.8196458601966,-48.071448345127,121.999233714831)) ;
#78509=CARTESIAN_POINT('Ctrl Pts',(-18.9375691001692,-47.8914592647082,
122.281750583357)) ;
#78510=CARTESIAN_POINT('Ctrl Pts',(-18.3709126385294,-48.091509911051,122.287270877135)) ;
#78511=CARTESIAN_POINT('Ctrl Pts',(-18.578583226595,-47.9115208306322,122.512179806311)) ;
#78512=CARTESIAN_POINT('Ctrl Pts',(-18.0514008753301,-48.1113503185918,
122.70674475677)) ;
#78513=CARTESIAN_POINT('Ctrl Pts',(-18.3229724703465,-47.931361238173,122.847760542803)) ;
#78514=CARTESIAN_POINT('Ctrl Pts',(-17.892005383859,-48.1312016425647,123.209726070952)) ;
#78515=CARTESIAN_POINT('Ctrl Pts',(-18.1954566722783,-47.9512125621459,
123.250147612826)) ;
#78516=CARTESIAN_POINT('Ctrl Pts',(-17.914844951633,-48.1512549125161,123.742150506215)) ;
#78517=CARTESIAN_POINT('Ctrl Pts',(-18.2137292815851,-47.9712658320974,
123.676086505446)) ;
#78518=CARTESIAN_POINT('Ctrl Pts',(-18.1156214422084,-48.1710755698994,
124.229345578923)) ;
#78519=CARTESIAN_POINT('Ctrl Pts',(-18.3743523078456,-47.9910864894807,
124.065843886977)) ;
#78520=CARTESIAN_POINT('Ctrl Pts',(-18.4724496627576,-48.1910469912299,
124.622086302339)) ;
#78521=CARTESIAN_POINT('Ctrl Pts',(-18.659816387674,-48.0110579108112,124.380035522052)) ;
#78522=CARTESIAN_POINT('Ctrl Pts',(-18.9403084788602,-48.2109404835936,
124.868804641601)) ;
#78523=CARTESIAN_POINT('Ctrl Pts',(-19.03410518183,-48.0309514031749,124.577408955661)) ;
#78524=CARTESIAN_POINT('Ctrl Pts',(-19.4674642242585,-48.2309645698347,
124.941135895806)) ;
#78525=CARTESIAN_POINT('Ctrl Pts',(-19.4558298576854,-48.050975489416,124.635271999274)) ;
#78526=CARTESIAN_POINT('Ctrl Pts',(-19.9821868641335,-48.2507694489476,
124.830704772389)) ;
#78527=CARTESIAN_POINT('Ctrl Pts',(-19.867609211054,-48.0707803685288,124.546924581979)) ;
#78528=CARTESIAN_POINT('Ctrl Pts',(-20.432501328611,-48.2707284646455,124.55033776454)) ;
#78529=CARTESIAN_POINT('Ctrl Pts',(-20.227859532346,-48.0907393842267,124.32262844544)) ;
#78530=CARTESIAN_POINT('Ctrl Pts',(-20.75958556185,-48.2907144882745,124.131795730235)) ;
#78531=CARTESIAN_POINT('Ctrl Pts',(-20.4895249857821,-48.1107254078558,
123.987793147059)) ;
#78532=CARTESIAN_POINT('Ctrl Pts',(-20.9237469670183,-48.310522984035,123.631516939099)) ;
#78533=CARTESIAN_POINT('Ctrl Pts',(-20.6208517088242,-48.1305339036163,
123.587567868658)) ;
#78534=CARTESIAN_POINT('Ctrl Pts',(-20.90785637785,-48.3305056231406,123.100761863408)) ;
#78535=CARTESIAN_POINT('Ctrl Pts',(-20.6081359619185,-48.1505165427219,
123.162963825818)) ;
#78536=CARTESIAN_POINT('Ctrl Pts',(-20.7125774922686,-48.3503870709346,
122.609609792236)) ;
#78537=CARTESIAN_POINT('Ctrl Pts',(-20.4519095117402,-48.1703979905159,
122.770042764306)) ;
#78538=CARTESIAN_POINT('Ctrl Pts',(-20.3605699835349,-48.3703435376721,
122.212992650378)) ;
#78539=CARTESIAN_POINT('Ctrl Pts',(-20.1703007092997,-48.1903544572534,
122.452751209908)) ;
#78540=CARTESIAN_POINT('Ctrl Pts',(-19.8961915070814,-48.3902209346277,
121.960894036754)) ;
#78541=CARTESIAN_POINT('Ctrl Pts',(-19.7987956286007,-48.210231854209,122.2510753083)) ;
#78542=CARTESIAN_POINT('Ctrl Pts',(-19.3710944052857,-48.410202880803,121.881710834877)) ;
#78543=CARTESIAN_POINT('Ctrl Pts',(-19.3787173826546,-48.2302138003843,
122.1877323754)) ;
#78544=CARTESIAN_POINT('Ctrl Pts',(-18.8517658004978,-48.4301319798398,
121.986485154986)) ;
#78545=CARTESIAN_POINT('Ctrl Pts',(-18.9632548451584,-48.250142899421,122.271556232587)) ;
#78546=CARTESIAN_POINT('Ctrl Pts',(-18.3995108076941,-48.4500606030523,
122.262000851755)) ;
#78547=CARTESIAN_POINT('Ctrl Pts',(-18.6014532429342,-48.2700715226336,
122.491970142446)) ;
#78548=CARTESIAN_POINT('Ctrl Pts',(-18.0691275875029,-48.4698949271588,
122.672852581585)) ;
#78549=CARTESIAN_POINT('Ctrl Pts',(-18.337147399175,-48.28990584674,122.820662663942)) ;
#78550=CARTESIAN_POINT('Ctrl Pts',(-17.9257131669283,-48.4865472145422,
123.091471777947)) ;
#78551=CARTESIAN_POINT('Ctrl Pts',(-18.2224260058625,-48.3065581341234,
123.155533896471)) ;
#78552=CARTESIAN_POINT('Ctrl Pts',(-17.9020712050021,-48.4998077155644,
123.439203218315)) ;
#78553=CARTESIAN_POINT('Ctrl Pts',(-18.2035092593179,-48.3198186351457,
123.433741819018)) ;
#78554=CARTESIAN_POINT('Ctrl Pts',(-17.9295520561369,-48.5098091927657,
123.700586123917)) ;
#78555=CARTESIAN_POINT('Ctrl Pts',(-18.2254971398453,-48.3298201123469,
123.642843255364)) ;
#78556=CARTESIAN_POINT('Ctrl Pts',(-18.0026504045817,-48.5198412136252,
123.953887639464)) ;
#78557=CARTESIAN_POINT('Ctrl Pts',(-18.2839780158191,-48.3398521332064,
123.845485394046)) ;
#78558=CARTESIAN_POINT('Ctrl Pts',(-18.1163811920468,-48.5297047573507,
124.186799307469)) ;
#78559=CARTESIAN_POINT('Ctrl Pts',(-18.3749628126578,-48.349715676932,124.031812191722)) ;
#78560=CARTESIAN_POINT('Ctrl Pts',(-18.2698960729777,-48.5396734710209,
124.399078392918)) ;
#78561=CARTESIAN_POINT('Ctrl Pts',(-18.4977838735188,-48.3596843906021,
124.201640071483)) ;
#78562=CARTESIAN_POINT('Ctrl Pts',(-18.5219675225245,-48.5530192184246,
124.64288817391)) ;
#78563=CARTESIAN_POINT('Ctrl Pts',(-18.6994062245984,-48.3730301380058,
124.396656830868)) ;
#78564=CARTESIAN_POINT('Ctrl Pts',(-18.8271260676844,-48.5661697734973,
124.813370161001)) ;
#78565=CARTESIAN_POINT('Ctrl Pts',(-18.9435542458751,-48.3861806930785,
124.533062412033)) ;
#78566=CARTESIAN_POINT('Ctrl Pts',(-19.1680417733559,-48.5795551540471,
124.899907926096)) ;
#78567=CARTESIAN_POINT('Ctrl Pts',(-19.2163009890961,-48.3995660736284,
124.602291912706)) ;
#78568=CARTESIAN_POINT('Ctrl Pts',(-19.4272046606689,-48.5894430900399,
124.91913276081)) ;
#78569=CARTESIAN_POINT('Ctrl Pts',(-19.4236288223874,-48.4094540096212,
124.617669122976)) ;
#78570=CARTESIAN_POINT('Ctrl Pts',(-19.688447434272,-48.5994342798526,124.893240945858)) ;
#78571=CARTESIAN_POINT('Ctrl Pts',(-19.6326235030201,-48.4194451994339,
124.596953556144)) ;
#78572=CARTESIAN_POINT('Ctrl Pts',(-19.9403393905488,-48.6093863783909,
124.82274784363)) ;
#78573=CARTESIAN_POINT('Ctrl Pts',(-19.834136251256,-48.4293972979721,124.540556882283)) ;
#78574=CARTESIAN_POINT('Ctrl Pts',(-20.1782692262565,-48.6194326348414,
124.708388111994)) ;
#78575=CARTESIAN_POINT('Ctrl Pts',(-20.0244791282803,-48.4394435544226,
124.449067115827)) ;
#78576=CARTESIAN_POINT('Ctrl Pts',(-20.3886560574177,-48.6292820822355,
124.557608789949)) ;
#78577=CARTESIAN_POINT('Ctrl Pts',(-20.1927872963318,-48.4492930018168,
124.328441805435)) ;
#78578=CARTESIAN_POINT('Ctrl Pts',(-20.5723260959942,-48.6392447347306,
124.371049479752)) ;
#78579=CARTESIAN_POINT('Ctrl Pts',(-20.3397216706453,-48.4592556543119,
124.179192818539)) ;
#78580=CARTESIAN_POINT('Ctrl Pts',(-20.7214277474001,-48.6492678203728,
124.153918077439)) ;
#78581=CARTESIAN_POINT('Ctrl Pts',(-20.4590011009063,-48.469278739954,124.005486461818)) ;
#78582=CARTESIAN_POINT('Ctrl Pts',(-20.8297802316799,-48.6591929361297,
123.916635975677)) ;
#78583=CARTESIAN_POINT('Ctrl Pts',(-20.5456810096503,-48.479203855711,123.815659897724)) ;
#78584=CARTESIAN_POINT('Ctrl Pts',(-20.8960112319061,-48.6692454145295,
123.660930444422)) ;
#78585=CARTESIAN_POINT('Ctrl Pts',(-20.5986636102316,-48.4892563341108,
123.611094951253)) ;
#78586=CARTESIAN_POINT('Ctrl Pts',(-20.916598068242,-48.6790969132322,123.402843889694)) ;
#78587=CARTESIAN_POINT('Ctrl Pts',(-20.6151308203117,-48.4991078328135,
123.404625622349)) ;
#78588=CARTESIAN_POINT('Ctrl Pts',(-20.892445735592,-48.6890686524347,123.141945824764)) ;
#78589=CARTESIAN_POINT('Ctrl Pts',(-20.5958067228006,-48.509079572016,123.195907470545)) ;
#78590=CARTESIAN_POINT('Ctrl Pts',(-20.8231457687366,-48.6990638602004,
122.888545055551)) ;
#78591=CARTESIAN_POINT('Ctrl Pts',(-20.5403646013204,-48.5190747797817,
122.993187508509)) ;
#78592=CARTESIAN_POINT('Ctrl Pts',(-20.7102015280108,-48.7090978616695,
122.650301300799)) ;
#78593=CARTESIAN_POINT('Ctrl Pts',(-20.4500071819512,-48.5291087812508,
122.802593499085)) ;
#78594=CARTESIAN_POINT('Ctrl Pts',(-20.5606310889798,-48.7189532197619,
122.438836911288)) ;
#78595=CARTESIAN_POINT('Ctrl Pts',(-20.3303491093556,-48.5389641393431,
122.633423436185)) ;
#78596=CARTESIAN_POINT('Ctrl Pts',(-20.3742255769114,-48.7289526953552,
122.253690036809)) ;
#78597=CARTESIAN_POINT('Ctrl Pts',(-20.1812231766611,-48.5489636149364,
122.485307572519)) ;
#78598=CARTESIAN_POINT('Ctrl Pts',(-20.1608603227047,-48.7388471438503,
122.104999075686)) ;
#78599=CARTESIAN_POINT('Ctrl Pts',(-20.0105298816174,-48.5588580634315,
122.366356738769)) ;
#78600=CARTESIAN_POINT('Ctrl Pts',(-19.9209501104199,-48.748910268078,121.993860313516)) ;
#78601=CARTESIAN_POINT('Ctrl Pts',(-19.8186007515957,-48.5689211876593,
122.277447732973)) ;
#78602=CARTESIAN_POINT('Ctrl Pts',(-19.6710512311484,-48.7587498944066,
121.927273469852)) ;
#78603=CARTESIAN_POINT('Ctrl Pts',(-19.6186814015643,-48.5787608139879,
122.224180469347)) ;
#78604=CARTESIAN_POINT('Ctrl Pts',(-19.4076398792597,-48.7688131294496,
121.904256633468)) ;
#78605=CARTESIAN_POINT('Ctrl Pts',(-19.4079520936183,-48.5888240490308,
122.205769170456)) ;
#78606=CARTESIAN_POINT('Ctrl Pts',(-19.1486188793757,-48.7787071346836,
121.927163232739)) ;
#78607=CARTESIAN_POINT('Ctrl Pts',(-19.2007357506879,-48.5987180542649,
122.224096613958)) ;
#78608=CARTESIAN_POINT('Ctrl Pts',(-18.8961432338801,-48.7886498478994,
121.994321818682)) ;
#78609=CARTESIAN_POINT('Ctrl Pts',(-18.9987559919676,-48.6086607674806,
122.27782549784)) ;
#78610=CARTESIAN_POINT('Ctrl Pts',(-18.6575880746569,-48.7986555876975,
122.104972809837)) ;
#78611=CARTESIAN_POINT('Ctrl Pts',(-18.8079128155078,-48.6186665072788,
122.366348201292)) ;
#78612=CARTESIAN_POINT('Ctrl Pts',(-18.4417397385288,-48.808676489844,122.255816146029)) ;
#78613=CARTESIAN_POINT('Ctrl Pts',(-18.6352354003947,-48.6286874094252,
122.487024632224)) ;
#78614=CARTESIAN_POINT('Ctrl Pts',(-18.2575608010827,-48.8185672598928,
122.439229061403)) ;
#78615=CARTESIAN_POINT('Ctrl Pts',(-18.4878939926653,-48.6385781794741,
122.633756241431)) ;
#78616=CARTESIAN_POINT('Ctrl Pts',(-18.1061936758401,-48.8285586706726,
122.653759103607)) ;
#78617=CARTESIAN_POINT('Ctrl Pts',(-18.3668020674057,-48.6485695902538,
122.805381400602)) ;
#78618=CARTESIAN_POINT('Ctrl Pts',(-17.9949337391282,-48.838507016337,122.890328842187)) ;
#78619=CARTESIAN_POINT('Ctrl Pts',(-18.2777961188115,-48.6585179359183,
122.994637890624)) ;
#78620=CARTESIAN_POINT('Ctrl Pts',(-17.9259246878583,-48.8484518743983,
123.14241755187)) ;
#78621=CARTESIAN_POINT('Ctrl Pts',(-18.2225909149543,-48.6684627939795,
123.196309167332)) ;
#78622=CARTESIAN_POINT('Ctrl Pts',(-17.9018586344331,-48.8585067097912,
123.405524737978)) ;
#78623=CARTESIAN_POINT('Ctrl Pts',(-18.2033401477523,-48.6785176293724,
123.406795195145)) ;
#78624=CARTESIAN_POINT('Ctrl Pts',(-17.9228907004356,-48.8683290818927,
123.662811089187)) ;
#78625=CARTESIAN_POINT('Ctrl Pts',(-18.2201677808873,-48.6883400014739,
123.612623483924)) ;
#78626=CARTESIAN_POINT('Ctrl Pts',(-17.9893599290001,-48.8783849493364,
123.918552606294)) ;
#78627=CARTESIAN_POINT('Ctrl Pts',(-18.2733451048243,-48.6983958689176,
123.817216284864)) ;
#78628=CARTESIAN_POINT('Ctrl Pts',(-18.0984022474381,-48.8883256791943,
124.155949320451)) ;
#78629=CARTESIAN_POINT('Ctrl Pts',(-18.360580702555,-48.7083365987755,124.007132560782)) ;
#78630=CARTESIAN_POINT('Ctrl Pts',(-18.2457897777886,-48.8982300177454,
124.370478803573)) ;
#78631=CARTESIAN_POINT('Ctrl Pts',(-18.4784920796112,-48.7182409373267,
124.178754699922)) ;
#78632=CARTESIAN_POINT('Ctrl Pts',(-18.4309099578096,-48.9082766991739,
124.558689346478)) ;
#78633=CARTESIAN_POINT('Ctrl Pts',(-18.6265896773682,-48.7282876187551,
124.329321820861)) ;
#78634=CARTESIAN_POINT('Ctrl Pts',(-18.6425771224203,-48.9181722066431,
124.709824664165)) ;
#78635=CARTESIAN_POINT('Ctrl Pts',(-18.7959241464339,-48.7381831262244,
124.450228239053)) ;
#78636=CARTESIAN_POINT('Ctrl Pts',(-18.881153587665,-48.9282344751418,124.823761366659)) ;
#78637=CARTESIAN_POINT('Ctrl Pts',(-18.986786280884,-48.748245394723,124.541375925979)) ;
#78638=CARTESIAN_POINT('Ctrl Pts',(-19.1303382919455,-48.9380764654124,
124.893166471183)) ;
#78639=CARTESIAN_POINT('Ctrl Pts',(-19.18613388542,-48.7580873849936,124.596897991502)) ;
#78640=CARTESIAN_POINT('Ctrl Pts',(-19.3916192445902,-48.9480698822934,
124.919216288569)) ;
#78641=CARTESIAN_POINT('Ctrl Pts',(-19.3951586909665,-48.7680808018746,
124.617736026515)) ;
#78642=CARTESIAN_POINT('Ctrl Pts',(-19.6517180268425,-48.9579943701455,
124.899657271401)) ;
#78643=CARTESIAN_POINT('Ctrl Pts',(-19.6032371787446,-48.7780052897268,
124.602087041937)) ;
#78644=CARTESIAN_POINT('Ctrl Pts',(-19.9064040385357,-48.967994004054,124.835026142102)) ;
#78645=CARTESIAN_POINT('Ctrl Pts',(-19.8069854638334,-48.7880049236352,
124.550380450082)) ;
#78646=CARTESIAN_POINT('Ctrl Pts',(-20.1457345660607,-48.9779801143107,
124.727283799791)) ;
#78647=CARTESIAN_POINT('Ctrl Pts',(-19.9984490348426,-48.797991033892,124.464185028181)) ;
#78648=CARTESIAN_POINT('Ctrl Pts',(-20.3635957586943,-48.9880160654979,
124.578693439251)) ;
#78649=CARTESIAN_POINT('Ctrl Pts',(-20.1727370240025,-48.8080269850791,
124.345311205248)) ;
#78650=CARTESIAN_POINT('Ctrl Pts',(-20.5492835774954,-48.9978727038327,
124.398066759138)) ;
#78651=CARTESIAN_POINT('Ctrl Pts',(-20.321285535719,-48.8178836234139,124.200809123624)) ;
#78652=CARTESIAN_POINT('Ctrl Pts',(-20.7032232577426,-49.0078716639107,
124.185175408086)) ;
#78653=CARTESIAN_POINT('Ctrl Pts',(-20.4444358521844,-48.8278825834919,
124.030495143245)) ;
#78654=CARTESIAN_POINT('Ctrl Pts',(-20.8169628557573,-49.0177668942244,
123.951284539001)) ;
#78655=CARTESIAN_POINT('Ctrl Pts',(-20.5354258074483,-48.8377778138057,
123.84338226399)) ;
#78656=CARTESIAN_POINT('Ctrl Pts',(-20.8895070311637,-49.0278274066931,
123.697088016927)) ;
#78657=CARTESIAN_POINT('Ctrl Pts',(-20.5934596252462,-48.8478383262744,
123.640024411145)) ;
#78658=CARTESIAN_POINT('Ctrl Pts',(-20.9163903856303,-49.0376766982393,
123.439638200356)) ;
#78659=CARTESIAN_POINT('Ctrl Pts',(-20.6149646209664,-48.8576876178205,
123.434065220729)) ;
#78660=CARTESIAN_POINT('Ctrl Pts',(-20.8985020838412,-49.0477038841715,
123.17674881798)) ;
#78661=CARTESIAN_POINT('Ctrl Pts',(-20.6006524960591,-48.8677148037527,
123.223753784893)) ;
#78662=CARTESIAN_POINT('Ctrl Pts',(-20.8345541010976,-49.0577324206308,
122.921071960527)) ;
#78663=CARTESIAN_POINT('Ctrl Pts',(-20.5494925272255,-48.8777433402121,
123.019212637237)) ;
#78664=CARTESIAN_POINT('Ctrl Pts',(-20.7296054274072,-49.0675776605958,
122.684606145175)) ;
#78665=CARTESIAN_POINT('Ctrl Pts',(-20.4655325601765,-48.887588580177,122.830041421681)) ;
#78666=CARTESIAN_POINT('Ctrl Pts',(-20.583631751647,-49.077568355519,122.466374760931)) ;
#78667=CARTESIAN_POINT('Ctrl Pts',(-20.3487525572943,-48.8975792751002,
122.655457213119)) ;
#78668=CARTESIAN_POINT('Ctrl Pts',(-20.4007099669967,-49.0876061762776,
122.276320211613)) ;
#78669=CARTESIAN_POINT('Ctrl Pts',(-20.202413975225,-48.9076170958588,122.503414537184)) ;
#78670=CARTESIAN_POINT('Ctrl Pts',(-20.1919240684328,-49.0974507700545,
122.123545795029)) ;
#78671=CARTESIAN_POINT('Ctrl Pts',(-20.0353851785869,-48.9174616896358,
122.381196695483)) ;
#78672=CARTESIAN_POINT('Ctrl Pts',(-19.9567693977437,-49.1074347654306,
122.007237918763)) ;
#78673=CARTESIAN_POINT('Ctrl Pts',(-19.8472610587631,-48.9274456850118,
122.288151648235)) ;
#78674=CARTESIAN_POINT('Ctrl Pts',(-19.7058304590674,-49.117383813992,121.933802444952)) ;
#78675=CARTESIAN_POINT('Ctrl Pts',(-19.646509912876,-48.9373947335732,122.229404623023)) ;
#78676=CARTESIAN_POINT('Ctrl Pts',(-19.4445921214441,-49.1273862529665,
121.904618015558)) ;
#78677=CARTESIAN_POINT('Ctrl Pts',(-19.437519186954,-48.9473971725478,122.206058321962)) ;
#78678=CARTESIAN_POINT('Ctrl Pts',(-19.181792231299,-49.1374074942629,121.921624060286)) ;
#78679=CARTESIAN_POINT('Ctrl Pts',(-19.2272793333639,-48.9574184138441,
122.219664472921)) ;
#78680=CARTESIAN_POINT('Ctrl Pts',(-18.9291459750835,-49.1473001727024,
121.982897915604)) ;
#78681=CARTESIAN_POINT('Ctrl Pts',(-19.025163319022,-48.9673110922836,122.268684604712)) ;
#78682=CARTESIAN_POINT('Ctrl Pts',(-18.6884670363389,-49.15729022665,122.087747388098)) ;
#78683=CARTESIAN_POINT('Ctrl Pts',(-18.8326207934705,-48.9773011462313,
122.352565175257)) ;
#78684=CARTESIAN_POINT('Ctrl Pts',(-18.4704519829709,-49.1672485877985,
122.232485671744)) ;
#78685=CARTESIAN_POINT('Ctrl Pts',(-18.6582097022475,-48.9872595073797,
122.468356610712)) ;
#78686=CARTESIAN_POINT('Ctrl Pts',(-18.2815383414992,-49.1771482146833,
122.411369259827)) ;
#78687=CARTESIAN_POINT('Ctrl Pts',(-18.5070800263305,-48.9971591342646,
122.611463763631)) ;
#78688=CARTESIAN_POINT('Ctrl Pts',(-18.124334533003,-49.1871961114867,122.623486945932)) ;
#78689=CARTESIAN_POINT('Ctrl Pts',(-18.3813177411218,-49.0072070310679,
122.781158694447)) ;
#78690=CARTESIAN_POINT('Ctrl Pts',(-18.0079271716233,-49.1970914691227,
122.856062333949)) ;
#78691=CARTESIAN_POINT('Ctrl Pts',(-18.2881931003449,-49.0171023887039,
122.967218812396)) ;
#78692=CARTESIAN_POINT('Ctrl Pts',(-17.932406893039,-49.2071531215793,123.109426695874)) ;
#78693=CARTESIAN_POINT('Ctrl Pts',(-18.2277777834536,-49.0271640411606,
123.169910844373)) ;
#78694=CARTESIAN_POINT('Ctrl Pts',(-17.9026375540909,-49.2169977258513,
123.366423552931)) ;
#78695=CARTESIAN_POINT('Ctrl Pts',(-18.2039634417627,-49.0370086454325,
123.375507396247)) ;
#78696=CARTESIAN_POINT('Ctrl Pts',(-17.9171858177311,-49.2269578475493,
123.627756075223)) ;
#78697=CARTESIAN_POINT('Ctrl Pts',(-18.2156028245757,-49.0469687671305,
123.584573004918)) ;
#78698=CARTESIAN_POINT('Ctrl Pts',(-17.9778519476595,-49.2369958819118,
123.884464098771)) ;
#78699=CARTESIAN_POINT('Ctrl Pts',(-18.2641366483863,-49.0570068014931,
123.789939339049)) ;
#78700=CARTESIAN_POINT('Ctrl Pts',(-18.0800477462609,-49.2468701944983,
124.12301444571)) ;
#78701=CARTESIAN_POINT('Ctrl Pts',(-18.3458936691752,-49.0668811140795,
123.980778477681)) ;
#78702=CARTESIAN_POINT('Ctrl Pts',(-18.2248917332872,-49.256939675281,124.34442449373)) ;
#78703=CARTESIAN_POINT('Ctrl Pts',(-18.4617697106575,-49.0769505948622,
124.157906347072)) ;
#78704=CARTESIAN_POINT('Ctrl Pts',(-18.4016886196437,-49.2667740112981,
124.53295491212)) ;
#78705=CARTESIAN_POINT('Ctrl Pts',(-18.6032069775405,-49.0867849308793,
124.308729299601)) ;
#78706=CARTESIAN_POINT('Ctrl Pts',(-18.6122540928525,-49.2768069690263,
124.691612235834)) ;
#78707=CARTESIAN_POINT('Ctrl Pts',(-18.7716597901353,-49.0968178886076,
124.435654741883)) ;
#78708=CARTESIAN_POINT('Ctrl Pts',(-18.8472145112235,-49.2868273676015,
124.8105056569)) ;
#78709=CARTESIAN_POINT('Ctrl Pts',(-18.9596285027308,-49.1068382871827,
124.530768800945)) ;
#78710=CARTESIAN_POINT('Ctrl Pts',(-19.0951813191126,-49.2966929413727,
124.886249263536)) ;
#78711=CARTESIAN_POINT('Ctrl Pts',(-19.158001200267,-49.116703860954,124.59136281955)) ;
#78712=CARTESIAN_POINT('Ctrl Pts',(-19.3577881565879,-49.3067618160288,
124.91843560293)) ;
#78713=CARTESIAN_POINT('Ctrl Pts',(-19.3680870720684,-49.12677273561,124.617111322248)) ;
#78714=CARTESIAN_POINT('Ctrl Pts',(-19.6161749842787,-49.3166072469343,
124.904881658566)) ;
#78715=CARTESIAN_POINT('Ctrl Pts',(-19.5747953751554,-49.1366181665155,
124.606267622671)) ;
#78716=CARTESIAN_POINT('Ctrl Pts',(-19.8718870581338,-49.326586871805,124.846704436952)) ;
#78717=CARTESIAN_POINT('Ctrl Pts',(-19.7793647044864,-49.1465977913862,
124.55972551948)) ;
#78718=CARTESIAN_POINT('Ctrl Pts',(-20.1143655070177,-49.3366055547191,
124.744152692603)) ;
#78719=CARTESIAN_POINT('Ctrl Pts',(-19.9733472699668,-49.1566164743003,
124.477683643661)) ;
#78720=CARTESIAN_POINT('Ctrl Pts',(-20.3326993755422,-49.3464888199029,
124.603431043447)) ;
#78721=CARTESIAN_POINT('Ctrl Pts',(-20.148013421792,-49.1664997394842,124.365106482365)) ;
#78722=CARTESIAN_POINT('Ctrl Pts',(-20.5267164376053,-49.3565571139943,
124.423600519454)) ;
#78723=CARTESIAN_POINT('Ctrl Pts',(-20.3032270348823,-49.1765680335755,
124.221241540364)) ;
#78724=CARTESIAN_POINT('Ctrl Pts',(-20.6830755385478,-49.3663872441796,
124.217913860269)) ;
#78725=CARTESIAN_POINT('Ctrl Pts',(-20.4283133065888,-49.1863981637609,
124.056692994351)) ;
#78726=CARTESIAN_POINT('Ctrl Pts',(-20.8044543032016,-49.3764537923947,
123.982913211167)) ;
#78727=CARTESIAN_POINT('Ctrl Pts',(-20.5254162463695,-49.196464711976,123.868692079819)) ;
#78728=CARTESIAN_POINT('Ctrl Pts',(-20.8816750148595,-49.3863440410833,
123.734710364359)) ;
#78729=CARTESIAN_POINT('Ctrl Pts',(-20.5871922922867,-49.2063549606646,
123.670130518056)) ;
#78730=CARTESIAN_POINT('Ctrl Pts',(-20.9155298640661,-49.3963362228594,
123.474333218866)) ;
#78731=CARTESIAN_POINT('Ctrl Pts',(-20.6142760088709,-49.2163471424406,
123.461828953088)) ;
#78732=CARTESIAN_POINT('Ctrl Pts',(-20.9034492217782,-49.4062990034872,
123.212805454259)) ;
#78733=CARTESIAN_POINT('Ctrl Pts',(-20.6046113070106,-49.2263099230684,
123.252607116101)) ;
#78734=CARTESIAN_POINT('Ctrl Pts',(-20.8471090806343,-49.4162034081609,
122.958679801281)) ;
#78735=CARTESIAN_POINT('Ctrl Pts',(-20.5595393178523,-49.2362143277422,
123.04930733304)) ;
#78736=CARTESIAN_POINT('Ctrl Pts',(-20.7457693980936,-49.42626340264,122.714534227901)) ;
#78737=CARTESIAN_POINT('Ctrl Pts',(-20.4784673873757,-49.2462743222212,
122.853990658576)) ;
#78738=CARTESIAN_POINT('Ctrl Pts',(-20.6067290421162,-49.4361120246098,
122.496219298876)) ;
#78739=CARTESIAN_POINT('Ctrl Pts',(-20.3672356811197,-49.256122944191,122.679339680775)) ;
#78740=CARTESIAN_POINT('Ctrl Pts',(-20.429127558002,-49.4461424640216,122.301465539504)) ;
#78741=CARTESIAN_POINT('Ctrl Pts',(-20.2251545164189,-49.2661533836029,
122.523536525192)) ;
#78742=CARTESIAN_POINT('Ctrl Pts',(-20.2204806965802,-49.4561521796563,
122.141233524229)) ;
#78743=CARTESIAN_POINT('Ctrl Pts',(-20.0582370435673,-49.2761630992376,
122.395350947196)) ;
#78744=CARTESIAN_POINT('Ctrl Pts',(-19.9896519589879,-49.466062932349,122.02066491153)) ;
#78745=CARTESIAN_POINT('Ctrl Pts',(-19.8735747112757,-49.2860738519302,
122.298896350739)) ;
#78746=CARTESIAN_POINT('Ctrl Pts',(-19.7410945155474,-49.4759922052954,
121.94122468313)) ;
#78747=CARTESIAN_POINT('Ctrl Pts',(-19.674729389547,-49.2960031248766,122.235344147617)) ;
#78748=CARTESIAN_POINT('Ctrl Pts',(-19.4795590978959,-49.4860348966881,
121.905973034216)) ;
#78749=CARTESIAN_POINT('Ctrl Pts',(-19.4655009066754,-49.3060458162693,
122.207142650007)) ;
#78750=CARTESIAN_POINT('Ctrl Pts',(-19.2199428620433,-49.4959214299056,
121.916333239369)) ;
#78751=CARTESIAN_POINT('Ctrl Pts',(-19.2578087796181,-49.3159323494868,
122.215430581112)) ;
#78752=CARTESIAN_POINT('Ctrl Pts',(-18.9632658837111,-49.5059145748376,
121.97176876514)) ;
#78753=CARTESIAN_POINT('Ctrl Pts',(-19.0524672904058,-49.3259254944189,
122.259778662686)) ;
#78754=CARTESIAN_POINT('Ctrl Pts',(-18.7212920166706,-49.5158602556741,
122.070557018446)) ;
#78755=CARTESIAN_POINT('Ctrl Pts',(-18.8588885297617,-49.3358711752553,
122.338808821512)) ;
#78756=CARTESIAN_POINT('Ctrl Pts',(-18.4998162839576,-49.5258075128226,
122.209435357168)) ;
#78757=CARTESIAN_POINT('Ctrl Pts',(-18.6817081096544,-49.3458184324039,
122.449910892272)) ;
#78758=CARTESIAN_POINT('Ctrl Pts',(-18.3040709556288,-49.5358554166946,
122.386637839502)) ;
#78759=CARTESIAN_POINT('Ctrl Pts',(-18.5251114670603,-49.3558663362759,
122.591672756877)) ;
#78760=CARTESIAN_POINT('Ctrl Pts',(-18.1451172425397,-49.5457031157926,
122.590856449705)) ;
#78761=CARTESIAN_POINT('Ctrl Pts',(-18.3979488685203,-49.3657140353738,
122.755046516047)) ;
#78762=CARTESIAN_POINT('Ctrl Pts',(-18.0219137175214,-49.5556646067713,
122.821817640646)) ;
#78763=CARTESIAN_POINT('Ctrl Pts',(-18.2993856846161,-49.3756755263525,
122.939814861468)) ;
#78764=CARTESIAN_POINT('Ctrl Pts',(-17.9404590218548,-49.5656940691852,
123.072489705615)) ;
#78765=CARTESIAN_POINT('Ctrl Pts',(-18.2342214104261,-49.3857049887665,
123.140352429838)) ;
#78766=CARTESIAN_POINT('Ctrl Pts',(-17.9040753302903,-49.5756013002851,
123.330287135658)) ;
#78767=CARTESIAN_POINT('Ctrl Pts',(-18.2051140105785,-49.3956122198664,
123.346589589261)) ;
#78768=CARTESIAN_POINT('Ctrl Pts',(-17.9125098781886,-49.5855476789625,
123.59151601534)) ;
#78769=CARTESIAN_POINT('Ctrl Pts',(-18.2118609481446,-49.4055585985438,
123.555572243342)) ;
#78770=CARTESIAN_POINT('Ctrl Pts',(-17.9664056108719,-49.5955524477714,
123.848870528839)) ;
#78771=CARTESIAN_POINT('Ctrl Pts',(-18.2549768267066,-49.4155633673526,
123.761455926636)) ;
#78772=CARTESIAN_POINT('Ctrl Pts',(-18.0645967712818,-49.6055735687916,
124.093218904673)) ;
#78773=CARTESIAN_POINT('Ctrl Pts',(-18.3335291813953,-49.4255844883728,
123.95693488968)) ;
#78774=CARTESIAN_POINT('Ctrl Pts',(-18.20166916916,-49.6154644346442,124.314070124089)) ;
#78775=CARTESIAN_POINT('Ctrl Pts',(-18.4431860779359,-49.4354753542255,
124.133615557219)) ;
#78776=CARTESIAN_POINT('Ctrl Pts',(-18.3764527036545,-49.6254552434035,
124.509963683003)) ;
#78777=CARTESIAN_POINT('Ctrl Pts',(-18.5830121977067,-49.4454661629847,
124.290330807483)) ;
#78778=CARTESIAN_POINT('Ctrl Pts',(-18.5818191090548,-49.6354059015838,
124.671858407303)) ;
#78779=CARTESIAN_POINT('Ctrl Pts',(-18.747304497956,-49.4554168211651,124.41984693504)) ;
#78780=CARTESIAN_POINT('Ctrl Pts',(-18.8116465770786,-49.6453421112259,
124.795748611769)) ;
#78781=CARTESIAN_POINT('Ctrl Pts',(-18.9311656103158,-49.4653530308072,
124.518959622352)) ;
#78782=CARTESIAN_POINT('Ctrl Pts',(-19.060609101934,-49.6553252779508,124.878578886169)) ;
#78783=CARTESIAN_POINT('Ctrl Pts',(-19.1303351363198,-49.475336197532,124.585224676569)) ;
#78784=CARTESIAN_POINT('Ctrl Pts',(-19.3217571085301,-49.6653690751611,
124.91666347962)) ;
#78785=CARTESIAN_POINT('Ctrl Pts',(-19.3392535710715,-49.4853799947423,
124.615693198187)) ;
#78786=CARTESIAN_POINT('Ctrl Pts',(-19.5799756953144,-49.6751972913293,
124.909602893017)) ;
#78787=CARTESIAN_POINT('Ctrl Pts',(-19.5458273138333,-49.4952082109106,
124.610045737877)) ;
#78788=CARTESIAN_POINT('Ctrl Pts',(-19.8393726054502,-49.6852738587986,
124.85664781928)) ;
#78789=CARTESIAN_POINT('Ctrl Pts',(-19.7533453820382,-49.5052847783798,
124.567682597387)) ;
#78790=CARTESIAN_POINT('Ctrl Pts',(-20.0802989167195,-49.695125944488,124.761703259133)) ;
#78791=CARTESIAN_POINT('Ctrl Pts',(-19.9460858927394,-49.5151368640692,
124.491728274294)) ;
#78792=CARTESIAN_POINT('Ctrl Pts',(-20.3060674976868,-49.7051992118934,
124.62357472207)) ;
#78793=CARTESIAN_POINT('Ctrl Pts',(-20.1267015988155,-49.5252101314746,
124.381226205106)) ;
#78794=CARTESIAN_POINT('Ctrl Pts',(-20.4998566128569,-49.715040628317,124.452283158296)) ;
#78795=CARTESIAN_POINT('Ctrl Pts',(-20.2817328184751,-49.5350515478982,
124.244194445969)) ;
#78796=CARTESIAN_POINT('Ctrl Pts',(-20.6636690760732,-49.7250018864597,
124.248115309329)) ;
#78797=CARTESIAN_POINT('Ctrl Pts',(-20.412783592269,-49.545012806041,124.080861225897)) ;
#78798=CARTESIAN_POINT('Ctrl Pts',(-20.7900512078552,-49.7350385628917,
124.01661886947)) ;
#78799=CARTESIAN_POINT('Ctrl Pts',(-20.5138903779245,-49.5550494824729,
123.895664546268)) ;
#78800=CARTESIAN_POINT('Ctrl Pts',(-20.8734168717332,-49.7449171707555,
123.770739635638)) ;
#78801=CARTESIAN_POINT('Ctrl Pts',(-20.5805838585332,-49.5649280903367,
123.698962322209)) ;
#78802=CARTESIAN_POINT('Ctrl Pts',(-20.9135969835831,-49.7549773993943,
123.509473505383)) ;
#78803=CARTESIAN_POINT('Ctrl Pts',(-20.6127292533526,-49.5749883189755,
123.489949387837)) ;
#78804=CARTESIAN_POINT('Ctrl Pts',(-20.9079881466067,-49.7648443835551,
123.25020659995)) ;
#78805=CARTESIAN_POINT('Ctrl Pts',(-20.6082434986379,-49.5848553031363,
123.282536664813)) ;
#78806=CARTESIAN_POINT('Ctrl Pts',(-20.8572486897129,-49.7748499498078,
122.992248524987)) ;
#78807=CARTESIAN_POINT('Ctrl Pts',(-20.5676533267145,-49.594860869389,123.076169999909)) ;
#78808=CARTESIAN_POINT('Ctrl Pts',(-20.762604793853,-49.7848337382224,122.74750089323)) ;
#78809=CARTESIAN_POINT('Ctrl Pts',(-20.4919395690296,-49.6048446578036,
122.88037156088)) ;
#78810=CARTESIAN_POINT('Ctrl Pts',(-20.6258474890098,-49.794879595025,122.521714953376)) ;
#78811=CARTESIAN_POINT('Ctrl Pts',(-20.3825347960662,-49.6148905146063,
122.699742010315)) ;
#78812=CARTESIAN_POINT('Ctrl Pts',(-20.4560100049864,-49.8047054722409,
122.327215170004)) ;
#78813=CARTESIAN_POINT('Ctrl Pts',(-20.246666541654,-49.6247163918222,122.544142037423)) ;
#78814=CARTESIAN_POINT('Ctrl Pts',(-20.2521537954512,-49.8146959480823,
122.161777820805)) ;
#78815=CARTESIAN_POINT('Ctrl Pts',(-20.0835826717048,-49.6347068676635,
122.411791024612)) ;
#78816=CARTESIAN_POINT('Ctrl Pts',(-20.0211126978838,-49.8247395239811,
122.034178353224)) ;
#78817=CARTESIAN_POINT('Ctrl Pts',(-19.8987503848234,-49.6447504435623,
122.30971013817)) ;
#78818=CARTESIAN_POINT('Ctrl Pts',(-19.777116224908,-49.8345613162791,121.95001127881)) ;
#78819=CARTESIAN_POINT('Ctrl Pts',(-19.7035546511395,-49.6545722358604,
122.242375346219)) ;
#78820=CARTESIAN_POINT('Ctrl Pts',(-19.5167805110233,-49.844596281905,121.907971037186)) ;
#78821=CARTESIAN_POINT('Ctrl Pts',(-19.4952862619387,-49.6646072014862,
122.208741497832)) ;
#78822=CARTESIAN_POINT('Ctrl Pts',(-19.2533683214203,-49.8546211988381,
121.912502122714)) ;
#78823=CARTESIAN_POINT('Ctrl Pts',(-19.2845564644904,-49.6746321184193,
122.212364842142)) ;
#78824=CARTESIAN_POINT('Ctrl Pts',(-18.9991000929057,-49.8644731372142,
121.961278882202)) ;
#78825=CARTESIAN_POINT('Ctrl Pts',(-19.0811423664437,-49.6844840567954,
122.251384496068)) ;
#78826=CARTESIAN_POINT('Ctrl Pts',(-18.7536426684916,-49.8744641132389,
122.05437660085)) ;
#78827=CARTESIAN_POINT('Ctrl Pts',(-18.8847759503893,-49.6944750328202,
122.325861028897)) ;
#78828=CARTESIAN_POINT('Ctrl Pts',(-18.5295831348585,-49.8843819340426,
122.187580190372)) ;
#78829=CARTESIAN_POINT('Ctrl Pts',(-18.7055278321113,-49.7043928536238,
122.432422178777)) ;
#78830=CARTESIAN_POINT('Ctrl Pts',(-18.3298664401023,-49.8944106546072,
122.359492881443)) ;
#78831=CARTESIAN_POINT('Ctrl Pts',(-18.5457533183806,-49.7144215741884,
122.569951033302)) ;
#78832=CARTESIAN_POINT('Ctrl Pts',(-18.1652873216249,-49.9042935812163,
122.560433756627)) ;
#78833=CARTESIAN_POINT('Ctrl Pts',(-18.4140890357409,-49.7243045007976,
122.730702147218)) ;
#78834=CARTESIAN_POINT('Ctrl Pts',(-18.0361983460719,-49.9142978663359,
122.789426912429)) ;
#78835=CARTESIAN_POINT('Ctrl Pts',(-18.3108162891678,-49.7343087859171,
122.913895707216)) ;
#78836=CARTESIAN_POINT('Ctrl Pts',(-17.9490142971123,-49.9242815475437,
123.036925185825)) ;
#78837=CARTESIAN_POINT('Ctrl Pts',(-18.2410673737591,-49.7442924671249,
123.111893582383)) ;
#78838=CARTESIAN_POINT('Ctrl Pts',(-17.9061915788502,-49.9343225462736,
123.297274155858)) ;
#78839=CARTESIAN_POINT('Ctrl Pts',(-18.2068074268591,-49.7543334658549,
123.32017254399)) ;
#78840=CARTESIAN_POINT('Ctrl Pts',(-17.9087977232919,-49.9441549911407,
123.555650792529)) ;
#78841=CARTESIAN_POINT('Ctrl Pts',(-18.2088904958492,-49.764165910722,123.526873108748)) ;
#78842=CARTESIAN_POINT('Ctrl Pts',(-17.9562480237733,-49.9541499895711,
123.813979871575)) ;
#78843=CARTESIAN_POINT('Ctrl Pts',(-18.2468487951362,-49.7741609091523,
123.733536626353)) ;
#78844=CARTESIAN_POINT('Ctrl Pts',(-18.0487030673203,-49.9641815383207,
124.060868718032)) ;
#78845=CARTESIAN_POINT('Ctrl Pts',(-18.3208110873252,-49.7841924579019,
123.93104838714)) ;
#78846=CARTESIAN_POINT('Ctrl Pts',(-18.1801084382228,-49.9740469166262,
124.284334653775)) ;
#78847=CARTESIAN_POINT('Ctrl Pts',(-18.4259334333969,-49.7940578362074,
124.109821606921)) ;
#78848=CARTESIAN_POINT('Ctrl Pts',(-18.349414443886,-49.9840087640865,124.48401461094)) ;
#78849=CARTESIAN_POINT('Ctrl Pts',(-18.56137656749,-49.8040196836677,124.269566724914)) ;
#78850=CARTESIAN_POINT('Ctrl Pts',(-18.5525546908774,-49.9940437049007,
124.652146083555)) ;
#78851=CARTESIAN_POINT('Ctrl Pts',(-18.7238875347409,-49.814054624482,124.404073431929)) ;
#78852=CARTESIAN_POINT('Ctrl Pts',(-18.7782043026968,-50.0039286659178,
124.780909685904)) ;
#78853=CARTESIAN_POINT('Ctrl Pts',(-18.9044058329455,-49.8239395854991,
124.507085842024)) ;
#78854=CARTESIAN_POINT('Ctrl Pts',(-19.0271970939987,-50.0139942748367,
124.870056934582)) ;
#78855=CARTESIAN_POINT('Ctrl Pts',(-19.1035994992475,-49.8340051944179,
124.578405575516)) ;
#78856=CARTESIAN_POINT('Ctrl Pts',(-19.2820603187376,-50.0238334498784,
124.913884244328)) ;
#78857=CARTESIAN_POINT('Ctrl Pts',(-19.3074891770789,-49.8438443694597,
124.613469338266)) ;
#78858=CARTESIAN_POINT('Ctrl Pts',(-19.5464617510488,-50.0338960053783,
124.91313355718)) ;
#78859=CARTESIAN_POINT('Ctrl Pts',(-19.5190104339783,-49.8539069249596,
124.61287087145)) ;
#78860=CARTESIAN_POINT('Ctrl Pts',(-19.8024340996591,-50.0437931800712,
124.86696663086)) ;
#78861=CARTESIAN_POINT('Ctrl Pts',(-19.7237883101448,-49.8638040996525,
124.575939415286)) ;
#78862=CARTESIAN_POINT('Ctrl Pts',(-20.0476128623271,-50.0537238949946,
124.777581121099)) ;
#78863=CARTESIAN_POINT('Ctrl Pts',(-19.9199318279951,-49.8737348145758,
124.504433101703)) ;
#78864=CARTESIAN_POINT('Ctrl Pts',(-20.2759720547415,-50.0637679230722,
124.645229703626)) ;
#78865=CARTESIAN_POINT('Ctrl Pts',(-20.1026202614428,-49.8837788426534,
124.398553782836)) ;
#78866=CARTESIAN_POINT('Ctrl Pts',(-20.4748580560747,-50.0736541249255,
124.478049523045)) ;
#78867=CARTESIAN_POINT('Ctrl Pts',(-20.2617301731961,-49.8936650445067,
124.264811487387)) ;
#78868=CARTESIAN_POINT('Ctrl Pts',(-20.6437749691382,-50.0836472913923,
124.277011182786)) ;
#78869=CARTESIAN_POINT('Ctrl Pts',(-20.396865308046,-49.9036582109736,124.103982270604)) ;
#78870=CARTESIAN_POINT('Ctrl Pts',(-20.7746102356371,-50.0935867623795,
124.050904663403)) ;
#78871=CARTESIAN_POINT('Ctrl Pts',(-20.5015353032639,-49.9135976819608,
123.92309830424)) ;
#78872=CARTESIAN_POINT('Ctrl Pts',(-20.8649209946815,-50.1036032767337,
123.803687665005)) ;
#78873=CARTESIAN_POINT('Ctrl Pts',(-20.5737859376745,-49.9236141963149,
123.725325490292)) ;
#78874=CARTESIAN_POINT('Ctrl Pts',(-20.9107662308834,-50.1135333032105,
123.546758707782)) ;
#78875=CARTESIAN_POINT('Ctrl Pts',(-20.610464245172,-49.9335442227918,123.519782903442)) ;
#78876=CARTESIAN_POINT('Ctrl Pts',(-20.911194011502,-50.12358583872,123.282611468906)) ;
#78877=CARTESIAN_POINT('Ctrl Pts',(-20.6108086511653,-49.9435967583012,
123.308465098402)) ;
#78878=CARTESIAN_POINT('Ctrl Pts',(-20.8668229607976,-50.1334322419396,
123.027681885346)) ;
#78879=CARTESIAN_POINT('Ctrl Pts',(-20.5753140241265,-49.9534431615209,
123.104521371413)) ;
#78880=CARTESIAN_POINT('Ctrl Pts',(-20.7786326899319,-50.1433942847937,
122.781207115412)) ;
#78881=CARTESIAN_POINT('Ctrl Pts',(-20.5047639491462,-49.963405204375,122.907340893886)) ;
#78882=CARTESIAN_POINT('Ctrl Pts',(-20.6478070136151,-50.1534228355844,
122.552412487801)) ;
#78883=CARTESIAN_POINT('Ctrl Pts',(-20.400105350936,-49.9734337551656,122.724304121501)) ;
#78884=CARTESIAN_POINT('Ctrl Pts',(-20.4813154003197,-50.163333161302,122.352163354397)) ;
#78885=CARTESIAN_POINT('Ctrl Pts',(-20.2669138792127,-49.9833440808833,
122.564103520818)) ;
#78886=CARTESIAN_POINT('Ctrl Pts',(-20.2825162867926,-50.1732680731316,
122.182913771869)) ;
#78887=CARTESIAN_POINT('Ctrl Pts',(-20.107876126385,-49.9932789927128,122.42870221035)) ;
#78888=CARTESIAN_POINT('Ctrl Pts',(-20.0548359116222,-50.1833090798997,
122.04955872531)) ;
#78889=CARTESIAN_POINT('Ctrl Pts',(-19.9257329909012,-50.0033199994809,
122.322016258521)) ;
#78890=CARTESIAN_POINT('Ctrl Pts',(-19.8112788264557,-50.1931967127318,
121.958995011296)) ;
#78891=CARTESIAN_POINT('Ctrl Pts',(-19.7308882259912,-50.0132076323131,
122.249563225972)) ;
#78892=CARTESIAN_POINT('Ctrl Pts',(-19.5531495649776,-50.2031871438299,
121.911155500874)) ;
#78893=CARTESIAN_POINT('Ctrl Pts',(-19.5243852785124,-50.0231980634112,
122.211289414015)) ;
#78894=CARTESIAN_POINT('Ctrl Pts',(-19.2915318676023,-50.2131425803871,
121.909011127538)) ;
#78895=CARTESIAN_POINT('Ctrl Pts',(-19.3150912261265,-50.0331534999684,
122.209571651062)) ;
#78896=CARTESIAN_POINT('Ctrl Pts',(-19.0346123538188,-50.2230535284865,
121.951656547233)) ;
#78897=CARTESIAN_POINT('Ctrl Pts',(-19.1095552462161,-50.0430644480677,
122.243685801554)) ;
#78898=CARTESIAN_POINT('Ctrl Pts',(-18.7863546985277,-50.2330656045842,
122.038872975881)) ;
#78899=CARTESIAN_POINT('Ctrl Pts',(-18.9109485915979,-50.0530765241654,
122.31345662738)) ;
#78900=CARTESIAN_POINT('Ctrl Pts',(-18.556965523036,-50.2430929266591,122.16850540643)) ;
#78901=CARTESIAN_POINT('Ctrl Pts',(-18.727435583092,-50.0631038462404,122.417161230504)) ;
#78902=CARTESIAN_POINT('Ctrl Pts',(-18.3565173091168,-50.2529517016133,
122.332725267608)) ;
#78903=CARTESIAN_POINT('Ctrl Pts',(-18.5670778973102,-50.0729626211945,
122.548532925854)) ;
#78904=CARTESIAN_POINT('Ctrl Pts',(-18.1268538969883,-50.2663778944257,
122.600443072319)) ;
#78905=CARTESIAN_POINT('Ctrl Pts',(-18.3833334664102,-50.086388814007,122.762717346392)) ;
#78906=CARTESIAN_POINT('Ctrl Pts',(-17.975652168658,-50.2794619102071,122.913754436158)) ;
#78907=CARTESIAN_POINT('Ctrl Pts',(-18.2623681321715,-50.0994728297884,
123.013391525604)) ;
#78908=CARTESIAN_POINT('Ctrl Pts',(-17.9092019313838,-50.2929353589624,
123.261460162953)) ;
#78909=CARTESIAN_POINT('Ctrl Pts',(-18.2092179634923,-50.1129462785436,
123.291511896051)) ;
#78910=CARTESIAN_POINT('Ctrl Pts',(-17.9058612706005,-50.3027683167682,
123.519872041666)) ;
#78911=CARTESIAN_POINT('Ctrl Pts',(-18.2065406001334,-50.1227792363495,
123.498250245797)) ;
#78912=CARTESIAN_POINT('Ctrl Pts',(-17.9468858270987,-50.3127315902189,
123.778444889139)) ;
#78913=CARTESIAN_POINT('Ctrl Pts',(-18.2393587805037,-50.1327425098001,
123.705106558061)) ;
#78914=CARTESIAN_POINT('Ctrl Pts',(-18.0333597050335,-50.3227686640368,
124.027627149713)) ;
#78915=CARTESIAN_POINT('Ctrl Pts',(-18.3085355866663,-50.1427795836181,
123.904453627933)) ;
#78916=CARTESIAN_POINT('Ctrl Pts',(-18.1593001785433,-50.3326436670485,
124.254558222545)) ;
#78917=CARTESIAN_POINT('Ctrl Pts',(-18.409286108333,-50.1526545866297,124.085999460383)) ;
#78918=CARTESIAN_POINT('Ctrl Pts',(-18.325884168104,-50.3427113466747,124.46004911197)) ;
#78919=CARTESIAN_POINT('Ctrl Pts',(-18.5425518166163,-50.1627222662559,
124.250393776869)) ;
#78920=CARTESIAN_POINT('Ctrl Pts',(-18.5210703742666,-50.3525521968924,
124.62974311494)) ;
#78921=CARTESIAN_POINT('Ctrl Pts',(-18.6986983036897,-50.1725631164736,
124.386149592484)) ;
#78922=CARTESIAN_POINT('Ctrl Pts',(-18.8210606852306,-50.3658883953684,
124.810877501162)) ;
#78923=CARTESIAN_POINT('Ctrl Pts',(-18.9386954921332,-50.1858993149496,
124.531065583499)) ;
#78924=CARTESIAN_POINT('Ctrl Pts',(-19.1585310682842,-50.3791059191828,
124.908576997296)) ;
#78925=CARTESIAN_POINT('Ctrl Pts',(-19.2087060042156,-50.199116838764,124.609228123008)) ;
#78926=CARTESIAN_POINT('Ctrl Pts',(-19.5088595130128,-50.392440845674,124.91604614796)) ;
#78927=CARTESIAN_POINT('Ctrl Pts',(-19.4889209379206,-50.2124517652553,
124.615199985815)) ;
#78928=CARTESIAN_POINT('Ctrl Pts',(-19.7681867122677,-50.4024239462686,
124.876091752278)) ;
#78929=CARTESIAN_POINT('Ctrl Pts',(-19.696392649381,-50.2224348658499,124.583239677521)) ;
#78930=CARTESIAN_POINT('Ctrl Pts',(-20.0179829922509,-50.4124687221682,
124.790847910307)) ;
#78931=CARTESIAN_POINT('Ctrl Pts',(-19.896227454566,-50.2324796417495,124.515046638421)) ;
#78932=CARTESIAN_POINT('Ctrl Pts',(-20.2442444734349,-50.4222866453541,
124.666833014675)) ;
#78933=CARTESIAN_POINT('Ctrl Pts',(-20.0772393601815,-50.2422975649354,
124.415835165722)) ;
#78934=CARTESIAN_POINT('Ctrl Pts',(-20.4505999319598,-50.4323359593095,
124.502045800935)) ;
#78935=CARTESIAN_POINT('Ctrl Pts',(-20.2423227107125,-50.2523468788908,
124.284011299718)) ;
#78936=CARTESIAN_POINT('Ctrl Pts',(-20.681214714332,-50.4456396999321,124.239319481613)) ;
#78937=CARTESIAN_POINT('Ctrl Pts',(-20.4268261522775,-50.2656506195133,
124.073810794489)) ;
#78938=CARTESIAN_POINT('Ctrl Pts',(-20.8766371021415,-50.4621298954088,
123.846918741784)) ;
#78939=CARTESIAN_POINT('Ctrl Pts',(-20.5831565547659,-50.28214081499,123.759929216494)) ;
#78940=CARTESIAN_POINT('Ctrl Pts',(-20.9269267934179,-50.4788490603334,
123.405534034858)) ;
#78941=CARTESIAN_POINT('Ctrl Pts',(-20.6233943759952,-50.2988599799146,
123.406758446571)) ;
#78942=CARTESIAN_POINT('Ctrl Pts',(-20.8757804022393,-50.4920100540035,
123.063406602107)) ;
#78943=CARTESIAN_POINT('Ctrl Pts',(-20.5824794341171,-50.3120209735847,
123.13310677555)) ;
#78944=CARTESIAN_POINT('Ctrl Pts',(-20.7933286315034,-50.5020062761088,
122.814013822148)) ;
#78945=CARTESIAN_POINT('Ctrl Pts',(-20.5165192334636,-50.32201719569,122.933581356952)) ;
#78946=CARTESIAN_POINT('Ctrl Pts',(-20.6679470249481,-50.5120301156425,
122.582347913138)) ;
#78947=CARTESIAN_POINT('Ctrl Pts',(-20.4162173324879,-50.3320410352238,
122.748251908727)) ;
#78948=CARTESIAN_POINT('Ctrl Pts',(-20.4530703196355,-50.5252234376358,
122.310222407872)) ;
#78949=CARTESIAN_POINT('Ctrl Pts',(-20.2443087067898,-50.345234357217,122.530542413722)) ;
#78950=CARTESIAN_POINT('Ctrl Pts',(-20.0984605249762,-50.5418826094131,
122.045150356545)) ;
#78951=CARTESIAN_POINT('Ctrl Pts',(-19.9606321286751,-50.3618935289943,
122.318489942363)) ;
#78952=CARTESIAN_POINT('Ctrl Pts',(-19.591771529195,-50.5617927848988,121.892456854746)) ;
#78953=CARTESIAN_POINT('Ctrl Pts',(-19.5552782569538,-50.38180370448,122.196329454903)) ;
#78954=CARTESIAN_POINT('Ctrl Pts',(-19.0638261203275,-50.5816827727432,
121.920703930823)) ;
#78955=CARTESIAN_POINT('Ctrl Pts',(-19.132921841017,-50.4016936923244,122.218924915738)) ;
#78956=CARTESIAN_POINT('Ctrl Pts',(-18.5747132438271,-50.601688220758,122.12899945868)) ;
#78957=CARTESIAN_POINT('Ctrl Pts',(-18.7416302351988,-50.4216991403392,
122.385558456999)) ;
#78958=CARTESIAN_POINT('Ctrl Pts',(-18.188781745609,-50.6215246147853,122.488396022967)) ;
#78959=CARTESIAN_POINT('Ctrl Pts',(-18.4328823682395,-50.4415355343665,
122.673074725378)) ;
#78960=CARTESIAN_POINT('Ctrl Pts',(-17.9465286196628,-50.6415324086819,
122.961624501233)) ;
#78961=CARTESIAN_POINT('Ctrl Pts',(-18.2390777138567,-50.4615433282632,
123.051656336489)) ;
#78962=CARTESIAN_POINT('Ctrl Pts',(-17.8806923532301,-50.6613590449759,
123.484550765064)) ;
#78963=CARTESIAN_POINT('Ctrl Pts',(-18.1864063185633,-50.4813699645572,
123.469998611925)) ;
#78964=CARTESIAN_POINT('Ctrl Pts',(-17.9971845805368,-50.6813379879298,
124.002602226852)) ;
#78965=CARTESIAN_POINT('Ctrl Pts',(-18.2795984569262,-50.501348907511,123.884440399758)) ;
#78966=CARTESIAN_POINT('Ctrl Pts',(-18.2835587249482,-50.7012697897989,
124.448196582392)) ;
#78967=CARTESIAN_POINT('Ctrl Pts',(-18.5086966003631,-50.5212807093801,
124.240917422711)) ;
#78968=CARTESIAN_POINT('Ctrl Pts',(-18.7016353947585,-50.7210940902964,
124.769140330271)) ;
#78969=CARTESIAN_POINT('Ctrl Pts',(-18.843158485295,-50.5411050098776,124.497674650865)) ;
#78970=CARTESIAN_POINT('Ctrl Pts',(-19.2109425558759,-50.7411900916362,
124.929317666307)) ;
#78971=CARTESIAN_POINT('Ctrl Pts',(-19.2506040110265,-50.5612010112175,
124.625816398005)) ;
#78972=CARTESIAN_POINT('Ctrl Pts',(-19.7359254653231,-50.7609485077402,
124.907008256573)) ;
#78973=CARTESIAN_POINT('Ctrl Pts',(-19.6705889099247,-50.5809594273214,
124.607973339329)) ;
#78974=CARTESIAN_POINT('Ctrl Pts',(-20.2295077366304,-50.7810422006242,
124.703903011823)) ;
#78975=CARTESIAN_POINT('Ctrl Pts',(-20.0654722041603,-50.6010531202055,
124.445475287471)) ;
#78976=CARTESIAN_POINT('Ctrl Pts',(-20.4872438679076,-50.7941531665309,
124.46905554134)) ;
#78977=CARTESIAN_POINT('Ctrl Pts',(-20.2716279488377,-50.6141640861122,
124.257625239002)) ;
#78978=CARTESIAN_POINT('Ctrl Pts',(-20.5950497967993,-50.8008665413188,
124.330315451458)) ;
#78979=CARTESIAN_POINT('Ctrl Pts',(-20.357892637621,-50.6208774609001,124.146615798218)) ;
#78980=CARTESIAN_POINT('Ctrl Pts',(-18.357854658548,-12.0237682964362,124.08784748689)) ;
#78981=CARTESIAN_POINT('Ctrl Pts',(-18.3365087757883,-12.0362829650914,
124.094103730057)) ;
#78982=CARTESIAN_POINT('Ctrl Pts',(-18.3147575215239,-12.0487813483325,
124.09965999913)) ;
#78983=CARTESIAN_POINT('Ctrl Pts',(-18.2929280361859,-12.0610923942012,
124.104426038987)) ;
#78984=CARTESIAN_POINT('Ctrl Pts',(-18.2713540954504,-12.0732593220902,
124.109136285693)) ;
#78985=CARTESIAN_POINT('Ctrl Pts',(-18.249704020901,-12.0852432736665,124.113074478837)) ;
#78986=CARTESIAN_POINT('Ctrl Pts',(-18.2283156882755,-12.0968791175651,
124.116199920138)) ;
#78987=CARTESIAN_POINT('Ctrl Pts',(-18.2227099783691,-12.0999287786375,
124.117019073158)) ;
#78988=CARTESIAN_POINT('Ctrl Pts',(-18.2171223536073,-12.1029545273125,
124.117782654151)) ;
#78989=CARTESIAN_POINT('Ctrl Pts',(-18.2115591098138,-12.1059533903454,
124.118490483479)) ;
#78990=CARTESIAN_POINT('Ctrl Pts',(-18.18871992723,-12.1182648372088,124.121396385838)) ;
#78991=CARTESIAN_POINT('Ctrl Pts',(-18.1654844706787,-12.1305575882187,
124.123462876928)) ;
#78992=CARTESIAN_POINT('Ctrl Pts',(-18.1422288201718,-12.1426193191337,
124.124534691556)) ;
#78993=CARTESIAN_POINT('Ctrl Pts',(-18.1247251875183,-12.1516977195438,
124.125341405156)) ;
#78994=CARTESIAN_POINT('Ctrl Pts',(-18.1072106532554,-12.1606452459923,
124.125585421888)) ;
#78995=CARTESIAN_POINT('Ctrl Pts',(-18.0898543520415,-12.1693713464509,
124.125218065099)) ;
#78996=CARTESIAN_POINT('Ctrl Pts',(-20.5005102612951,-12.2002209833368,
122.802143462197)) ;
#78997=CARTESIAN_POINT('Ctrl Pts',(-20.541093837296,-12.219219492016,122.806247489297)) ;
#78998=CARTESIAN_POINT('Ctrl Pts',(-20.5830951416339,-12.2380808775341,
122.814354667494)) ;
#78999=CARTESIAN_POINT('Ctrl Pts',(-20.6474219049173,-12.2647855663232,
122.837495408728)) ;
#79000=CARTESIAN_POINT('Ctrl Pts',(-20.6724144804817,-12.2745814626532,
122.849334969911)) ;
#79001=CARTESIAN_POINT('Ctrl Pts',(-20.7094156327346,-12.2874767103628,
122.874746786746)) ;
#79002=CARTESIAN_POINT('Ctrl Pts',(-20.7230455646647,-12.2917830191842,
122.886284215876)) ;
#79003=CARTESIAN_POINT('Ctrl Pts',(-20.7432461326241,-12.2970233590185,
122.908954347183)) ;
#79004=CARTESIAN_POINT('Ctrl Pts',(-20.7506335985086,-12.2985684592622,
122.919056120632)) ;
#79005=CARTESIAN_POINT('Ctrl Pts',(-20.7590911123199,-12.2996582019218,
122.933919924051)) ;
#79006=CARTESIAN_POINT('Ctrl Pts',(-20.7611608911784,-12.2998488756498,
122.937926648299)) ;
#79007=CARTESIAN_POINT('Ctrl Pts',(-20.7653472287969,-12.3000477257932,
122.94693639312)) ;
#79008=CARTESIAN_POINT('Ctrl Pts',(-20.7673793575462,-12.3000112231311,
122.951954892876)) ;
#79009=CARTESIAN_POINT('Ctrl Pts',(-20.7693310884309,-12.2998090284859,
122.957583705285)) ;
#79010=CARTESIAN_POINT('Ctrl Pts',(-20.7695054962804,-12.2997892287744,
122.958095078672)) ;
#79011=CARTESIAN_POINT('Ctrl Pts',(-20.7696845881009,-12.2997670653285,
122.958629049888)) ;
#79012=CARTESIAN_POINT('Ctrl Pts',(-20.7696918833559,-12.2997661592856,
122.958650816641)) ;
#79013=CARTESIAN_POINT('Ctrl Pts',(-20.769705894931,-12.2997644129052,122.958692652767)) ;
#79014=CARTESIAN_POINT('Ctrl Pts',(-20.7697126114251,-12.2997635730312,
122.958712720312)) ;
#79015=CARTESIAN_POINT('Ctrl Pts',(-20.7697224091429,-12.2997623438578,
122.958742013309)) ;
#79016=CARTESIAN_POINT('Ctrl Pts',(-20.7697254935453,-12.2997619563241,
122.958751237791)) ;
#79017=CARTESIAN_POINT('Ctrl Pts',(-20.7697308745325,-12.2997612792286,
122.958767335535)) ;
#79018=CARTESIAN_POINT('Ctrl Pts',(-20.7697331715033,-12.2997609898763,
122.958774208704)) ;
#79019=CARTESIAN_POINT('Ctrl Pts',(-20.7697378791215,-12.2997603961915,
122.958788298387)) ;
#79020=CARTESIAN_POINT('Ctrl Pts',(-20.7697402897172,-12.2997600918325,
122.958795514906)) ;
#79021=CARTESIAN_POINT('Ctrl Pts',(-20.7697463513703,-12.2997593256021,
122.958813665796)) ;
#79022=CARTESIAN_POINT('Ctrl Pts',(-20.7697500017654,-12.2997588633541,
122.958824600409)) ;
#79023=CARTESIAN_POINT('Ctrl Pts',(-20.7697641085656,-12.2997570738623,
122.958866872028)) ;
#79024=CARTESIAN_POINT('Ctrl Pts',(-20.7697745563457,-12.2997557418272,
122.958898211664)) ;
#79025=CARTESIAN_POINT('Ctrl Pts',(-20.7716678466195,-12.2995131409472,
122.964583297981)) ;
#79026=CARTESIAN_POINT('Ctrl Pts',(-20.7732253610465,-12.2990951061691,
122.970317141544)) ;
#79027=CARTESIAN_POINT('Ctrl Pts',(-20.7766185838289,-12.2974760939754,
122.986230079433)) ;
#79028=CARTESIAN_POINT('Ctrl Pts',(-20.7777752979968,-12.2959381602225,
122.996417279488)) ;
#79029=CARTESIAN_POINT('Ctrl Pts',(-20.7784284793249,-12.2910064741822,
123.021765385816)) ;
#79030=CARTESIAN_POINT('Ctrl Pts',(-20.7768380405423,-12.2871205346287,
123.036695790602)) ;
#79031=CARTESIAN_POINT('Ctrl Pts',(-20.7692015154357,-12.2758025819446,
123.072886879007)) ;
#79032=CARTESIAN_POINT('Ctrl Pts',(-20.7612984889414,-12.2675400841427,
123.093650774925)) ;
#79033=CARTESIAN_POINT('Ctrl Pts',(-20.7293644524945,-12.2382702301405,
123.157267294964)) ;
#79034=CARTESIAN_POINT('Ctrl Pts',(-20.6937666914365,-12.2110963893297,
123.201398141947)) ;
#79035=CARTESIAN_POINT('Ctrl Pts',(-20.6477460536494,-12.1788358604101,
123.242468690928)) ;
#79036=CARTESIAN_POINT('Origin',(-5.63784594171726E-6,12.,130.056019952763)) ;
#79037=CARTESIAN_POINT('',(-21.1595576762002,12.3,122.812674418818)) ;
#79038=CARTESIAN_POINT('',(-21.1596428393339,11.6999371236922,122.812655579117)) ;
#79039=CARTESIAN_POINT('Ctrl Pts',(-21.1595576760718,12.3,122.812674418862)) ;
#79040=CARTESIAN_POINT('Ctrl Pts',(-21.1231857045382,12.3022605407561,122.701878867478)) ;
#79041=CARTESIAN_POINT('Ctrl Pts',(-21.0335185861001,12.2002215949571,122.572974429341)) ;
#79042=CARTESIAN_POINT('Ctrl Pts',(-21.0066064330477,12.0208669735961,122.543615355704)) ;
#79043=CARTESIAN_POINT('Ctrl Pts',(-21.0129499559569,11.937009842197,122.550313273341)) ;
#79044=CARTESIAN_POINT('Ctrl Pts',(-21.0334141863148,11.8415941256325,122.576365669548)) ;
#79045=CARTESIAN_POINT('Ctrl Pts',(-21.0906762596813,11.7344433920243,122.653153592077)) ;
#79046=CARTESIAN_POINT('Ctrl Pts',(-21.1409524880335,11.6999402726311,122.758036674297)) ;
#79047=CARTESIAN_POINT('Ctrl Pts',(-21.1596428393339,11.6999371236922,122.812655579117)) ;
#79048=CARTESIAN_POINT('',(-5.63784594223766E-6,11.7,130.056019952763)) ;
#79049=CARTESIAN_POINT('Ctrl Pts',(-21.1596428393339,11.6999371236922,122.812655579117)) ;
#79050=CARTESIAN_POINT('Ctrl Pts',(-21.1783331906335,11.6999339747533,122.867274483935)) ;
#79051=CARTESIAN_POINT('Ctrl Pts',(-21.2028183674824,11.7344244983881,122.98086702099)) ;
#79052=CARTESIAN_POINT('Ctrl Pts',(-21.2047930541468,11.8416345270515,123.076798355982)) ;
#79053=CARTESIAN_POINT('Ctrl Pts',(-21.2043581510169,11.9369444204252,123.109719701306)) ;
#79054=CARTESIAN_POINT('Ctrl Pts',(-21.2039085683262,12.0210152953098,123.119325478645)) ;
#79055=CARTESIAN_POINT('Ctrl Pts',(-21.205181447895,12.1418774804202,123.09162894974)) ;
#79056=CARTESIAN_POINT('Ctrl Pts',(-21.2026565890277,12.2655504187303,122.980780809732)) ;
#79057=CARTESIAN_POINT('Ctrl Pts',(-21.1785313959741,12.3001251310309,122.867342837561)) ;
#79058=CARTESIAN_POINT('Ctrl Pts',(-21.1595576760718,12.3,122.812674418862)) ;
#79059=CARTESIAN_POINT('Ctrl Pts',(-21.1595576760718,12.3,122.812674418862)) ;
#79060=CARTESIAN_POINT('Ctrl Pts',(-21.1231857045382,12.3022605407561,122.701878867478)) ;
#79061=CARTESIAN_POINT('Ctrl Pts',(-21.0335185861001,12.2002215949571,122.572974429341)) ;
#79062=CARTESIAN_POINT('Ctrl Pts',(-21.0066064330477,12.0208669735961,122.543615355704)) ;
#79063=CARTESIAN_POINT('Ctrl Pts',(-21.0129499559569,11.937009842197,122.550313273341)) ;
#79064=CARTESIAN_POINT('Ctrl Pts',(-21.0334141863148,11.8415941256325,122.576365669548)) ;
#79065=CARTESIAN_POINT('Ctrl Pts',(-21.0906762596813,11.7344433920243,122.653153592077)) ;
#79066=CARTESIAN_POINT('Ctrl Pts',(-21.1660906022086,11.6826887129352,122.810478215405)) ;
#79067=CARTESIAN_POINT('Ctrl Pts',(-21.2028183674824,11.7344244983881,122.98086702099)) ;
#79068=CARTESIAN_POINT('Ctrl Pts',(-21.2047930541468,11.8416345270515,123.076798355982)) ;
#79069=CARTESIAN_POINT('Ctrl Pts',(-21.2043581510169,11.9369444204252,123.109719701306)) ;
#79070=CARTESIAN_POINT('Ctrl Pts',(-21.2039085683262,12.0210152953098,123.119325478645)) ;
#79071=CARTESIAN_POINT('Ctrl Pts',(-21.205181447895,12.1418774804202,123.09162894974)) ;
#79072=CARTESIAN_POINT('Ctrl Pts',(-21.2026565890277,12.2655504187303,122.980780809732)) ;
#79073=CARTESIAN_POINT('Ctrl Pts',(-21.1785313959741,12.3001251310309,122.867342837561)) ;
#79074=CARTESIAN_POINT('Ctrl Pts',(-21.1595576760718,12.3,122.812674418862)) ;
#79075=CARTESIAN_POINT('Ctrl Pts',(-21.3014729215226,12.4500000043639,122.764093940449)) ;
#79076=CARTESIAN_POINT('Ctrl Pts',(-21.2417386817332,12.4533908072994,122.58468313231)) ;
#79077=CARTESIAN_POINT('Ctrl Pts',(-21.1183669661588,12.3003323944147,122.368106075024)) ;
#79078=CARTESIAN_POINT('Ctrl Pts',(-21.0828841600767,12.0313004597594,122.317703938634)) ;
#79079=CARTESIAN_POINT('Ctrl Pts',(-21.0912110587446,11.9055147635765,122.329236338449)) ;
#79080=CARTESIAN_POINT('Ctrl Pts',(-21.1188098709144,11.7623911882616,122.373395814998)) ;
#79081=CARTESIAN_POINT('Ctrl Pts',(-21.1966797848952,11.6016650881281,122.503047298049)) ;
#79082=CARTESIAN_POINT('Ctrl Pts',(-21.3085421953233,11.5240330679577,122.761739092861)) ;
#79083=CARTESIAN_POINT('Ctrl Pts',(-21.3785516269951,11.6016367477315,123.03446770917)) ;
#79084=CARTESIAN_POINT('Ctrl Pts',(-21.3966874043036,11.7624517905451,123.184919968199)) ;
#79085=CARTESIAN_POINT('Ctrl Pts',(-21.4016453124917,11.905416630659,123.236367319138)) ;
#79086=CARTESIAN_POINT('Ctrl Pts',(-21.4027247828246,12.0315229430405,123.251325161369)) ;
#79087=CARTESIAN_POINT('Ctrl Pts',(-21.3995856881047,12.2128162203883,123.208193040234)) ;
#79088=CARTESIAN_POINT('Ctrl Pts',(-21.3783532801531,12.3983256286576,123.034306001354)) ;
#79089=CARTESIAN_POINT('Ctrl Pts',(-21.3321155076486,12.450187696004,122.852788427119)) ;
#79090=CARTESIAN_POINT('Ctrl Pts',(-21.3014729215226,12.4500000043639,122.764093940449)) ;
#79091=CARTESIAN_POINT('',(-21.1595576760718,12.3,122.812674418862)) ;
#79092=CARTESIAN_POINT('Origin',(-5.63784594171726E-6,12.,130.056019952763)) ;
#79093=CARTESIAN_POINT('',(-17.6588963672735,11.6999371505335,124.011011800868)) ;
#79094=CARTESIAN_POINT('',(-5.63784594223766E-6,11.7,130.056019952763)) ;
#79095=CARTESIAN_POINT('',(-17.6589816018599,12.3,124.010992891173)) ;
#79096=CARTESIAN_POINT('Ctrl Pts',(-17.6588963672735,11.6999371505335,124.011011800868)) ;
#79097=CARTESIAN_POINT('Ctrl Pts',(-17.6402059616163,11.6999340236683,123.956392954847)) ;
#79098=CARTESIAN_POINT('Ctrl Pts',(-17.6157209902082,11.734424479462,123.842800166528)) ;
#79099=CARTESIAN_POINT('Ctrl Pts',(-17.6137462730154,11.841634502012,123.746868949177)) ;
#79100=CARTESIAN_POINT('Ctrl Pts',(-17.6141812884147,11.9369442552144,123.713947499122)) ;
#79101=CARTESIAN_POINT('Ctrl Pts',(-17.614630652896,12.0210152204092,123.704342009584)) ;
#79102=CARTESIAN_POINT('Ctrl Pts',(-17.6133579093719,12.1418772592244,123.732038413223)) ;
#79103=CARTESIAN_POINT('Ctrl Pts',(-17.615882601329,12.265550626992,123.842886461929)) ;
#79104=CARTESIAN_POINT('Ctrl Pts',(-17.6400079287178,12.3001250268061,123.956324488906)) ;
#79105=CARTESIAN_POINT('Ctrl Pts',(-17.6589816021521,12.3,124.010992891073)) ;
#79106=CARTESIAN_POINT('Ctrl Pts',(-17.6589816021521,12.3,124.010992891073)) ;
#79107=CARTESIAN_POINT('Ctrl Pts',(-17.695354537387,12.3022593030227,124.121784712804)) ;
#79108=CARTESIAN_POINT('Ctrl Pts',(-17.7850200523455,12.20022254417,124.250695376743)) ;
#79109=CARTESIAN_POINT('Ctrl Pts',(-17.811932580282,12.0208678335766,124.280054163229)) ;
#79110=CARTESIAN_POINT('Ctrl Pts',(-17.8055896930183,11.9370093101012,124.273352046235)) ;
#79111=CARTESIAN_POINT('Ctrl Pts',(-17.7851245667583,11.8415943650359,124.247302411162)) ;
#79112=CARTESIAN_POINT('Ctrl Pts',(-17.7278634241582,11.7344432406589,124.170513242669)) ;
#79113=CARTESIAN_POINT('Ctrl Pts',(-17.6775867729323,11.6999402773988,124.065630646894)) ;
#79114=CARTESIAN_POINT('Ctrl Pts',(-17.6588963672735,11.6999371505335,124.011011800868)) ;
#79115=CARTESIAN_POINT('Ctrl Pts',(-17.6589816021521,12.3,124.010992891073)) ;
#79116=CARTESIAN_POINT('Ctrl Pts',(-17.695354537387,12.3022593030227,124.121784712804)) ;
#79117=CARTESIAN_POINT('Ctrl Pts',(-17.7850200523455,12.20022254417,124.250695376743)) ;
#79118=CARTESIAN_POINT('Ctrl Pts',(-17.811932580282,12.0208678335766,124.280054163229)) ;
#79119=CARTESIAN_POINT('Ctrl Pts',(-17.8055896930183,11.9370093101012,124.273352046235)) ;
#79120=CARTESIAN_POINT('Ctrl Pts',(-17.7851245667583,11.8415943650359,124.247302411162)) ;
#79121=CARTESIAN_POINT('Ctrl Pts',(-17.7278634241582,11.7344432406589,124.170513242669)) ;
#79122=CARTESIAN_POINT('Ctrl Pts',(-17.6524484473213,11.6826887957701,124.01318934901)) ;
#79123=CARTESIAN_POINT('Ctrl Pts',(-17.6157209902082,11.734424479462,123.842800166528)) ;
#79124=CARTESIAN_POINT('Ctrl Pts',(-17.6137462730154,11.841634502012,123.746868949177)) ;
#79125=CARTESIAN_POINT('Ctrl Pts',(-17.6141812884147,11.9369442552144,123.713947499122)) ;
#79126=CARTESIAN_POINT('Ctrl Pts',(-17.614630652896,12.0210152204092,123.704342009584)) ;
#79127=CARTESIAN_POINT('Ctrl Pts',(-17.6133579093719,12.1418772592244,123.732038413223)) ;
#79128=CARTESIAN_POINT('Ctrl Pts',(-17.615882601329,12.265550626992,123.842886461929)) ;
#79129=CARTESIAN_POINT('Ctrl Pts',(-17.6400079287178,12.3001250268061,123.956324488906)) ;
#79130=CARTESIAN_POINT('Ctrl Pts',(-17.6589816021521,12.3,124.010992891073)) ;
#79131=CARTESIAN_POINT('Ctrl Pts',(-17.5170663566028,12.4500000035941,124.059573369615)) ;
#79132=CARTESIAN_POINT('Ctrl Pts',(-17.5768010750503,12.4533889497169,124.238978500622)) ;
#79133=CARTESIAN_POINT('Ctrl Pts',(-17.7001719976827,12.3003338187364,124.455565035223)) ;
#79134=CARTESIAN_POINT('Ctrl Pts',(-17.735655182611,12.0313017495778,124.505966784337)) ;
#79135=CARTESIAN_POINT('Ctrl Pts',(-17.727328311671,11.9055139654912,124.494427918119)) ;
#79136=CARTESIAN_POINT('Ctrl Pts',(-17.6997289374594,11.7623915473154,124.450272614137)) ;
#79137=CARTESIAN_POINT('Ctrl Pts',(-17.6218598761679,11.6016648611214,124.320619335508)) ;
#79138=CARTESIAN_POINT('Ctrl Pts',(-17.5099968647986,11.5240331921794,124.061928577266)) ;
#79139=CARTESIAN_POINT('Ctrl Pts',(-17.4399877214087,11.6016367193622,123.789199422435)) ;
#79140=CARTESIAN_POINT('Ctrl Pts',(-17.4218519288077,11.7624517529768,123.638747342328)) ;
#79141=CARTESIAN_POINT('Ctrl Pts',(-17.4168941310285,11.9054163828466,123.587299846138)) ;
#79142=CARTESIAN_POINT('Ctrl Pts',(-17.415814460062,12.0315228305656,123.572342418142)) ;
#79143=CARTESIAN_POINT('Ctrl Pts',(-17.4189536889037,12.2128158889338,123.615474365746)) ;
#79144=CARTESIAN_POINT('Ctrl Pts',(-17.4401858916256,12.3983259401867,123.789361234211)) ;
#79145=CARTESIAN_POINT('Ctrl Pts',(-17.486423826463,12.4501875413069,123.970878916215)) ;
#79146=CARTESIAN_POINT('Ctrl Pts',(-17.5170663566028,12.4500000035941,124.059573369615)) ;
#79147=CARTESIAN_POINT('',(-17.6589816021521,12.3,124.010992891073)) ;
#79148=CARTESIAN_POINT('Origin',(-5.63784594070025E-6,-12.,130.056019952763)) ;
#79149=CARTESIAN_POINT('',(-17.6589027590969,-11.6999371236917,124.011030194063)) ;
#79150=CARTESIAN_POINT('',(-5.63784594017984E-6,-11.7,130.056019952763)) ;
#79151=CARTESIAN_POINT('',(-17.65898160186,-12.3,124.010992891173)) ;
#79152=CARTESIAN_POINT('Ctrl Pts',(-17.6589027590969,-11.6999371236917,
124.011030194063)) ;
#79153=CARTESIAN_POINT('Ctrl Pts',(-17.6776053053521,-11.6999339747542,
124.065644924303)) ;
#79154=CARTESIAN_POINT('Ctrl Pts',(-17.72786935392,-11.7344244983967,124.170412828578)) ;
#79155=CARTESIAN_POINT('Ctrl Pts',(-17.7850982943228,-11.8416345270247,
124.247429507382)) ;
#79156=CARTESIAN_POINT('Ctrl Pts',(-17.8056170712146,-11.9369444204012,
124.27317798136)) ;
#79157=CARTESIAN_POINT('Ctrl Pts',(-17.8118590245238,-12.021015295271,124.280493109677)) ;
#79158=CARTESIAN_POINT('Ctrl Pts',(-17.7938799763284,-12.1418774804083,
124.259386907686)) ;
#79159=CARTESIAN_POINT('Ctrl Pts',(-17.7279443615378,-12.2655504187416,
124.17024556063)) ;
#79160=CARTESIAN_POINT('Ctrl Pts',(-17.6774905688518,-12.3001251310252,
124.065820404267)) ;
#79161=CARTESIAN_POINT('Ctrl Pts',(-17.6589816021521,-12.3,124.010992891073)) ;
#79162=CARTESIAN_POINT('Ctrl Pts',(-17.6589816021521,-12.3,124.010992891073)) ;
#79163=CARTESIAN_POINT('Ctrl Pts',(-17.6198247664454,-12.302260540837,123.901150655369)) ;
#79164=CARTESIAN_POINT('Ctrl Pts',(-17.6116850160222,-12.2002215949029,
123.744337739047)) ;
#79165=CARTESIAN_POINT('Ctrl Pts',(-17.6149593962428,-12.0208669736416,
123.704645200407)) ;
#79166=CARTESIAN_POINT('Ctrl Pts',(-17.6140513077368,-11.9370098422088,
123.713825492269)) ;
#79167=CARTESIAN_POINT('Ctrl Pts',(-17.6138457601763,-11.8415941256522,
123.746953574365)) ;
#79168=CARTESIAN_POINT('Ctrl Pts',(-17.6156540763921,-11.7344433920138,
123.842724447157)) ;
#79169=CARTESIAN_POINT('Ctrl Pts',(-17.6402002128438,-11.6999402726293,
123.956415463829)) ;
#79170=CARTESIAN_POINT('Ctrl Pts',(-17.6589027590969,-11.6999371236917,
124.011030194063)) ;
#79171=CARTESIAN_POINT('Origin',(-5.63784594070025E-6,-12.,130.056019952763)) ;
#79172=CARTESIAN_POINT('',(-21.1595576754736,-12.3,122.812674419067)) ;
#79173=CARTESIAN_POINT('',(-21.1596366183962,-11.6999371505325,122.812637127424)) ;
#79174=CARTESIAN_POINT('Ctrl Pts',(-21.1595576755874,-12.3,122.812674419028)) ;
#79175=CARTESIAN_POINT('Ctrl Pts',(-21.1987114653594,-12.3022593030704,
122.922514297446)) ;
#79176=CARTESIAN_POINT('Ctrl Pts',(-21.2068562966847,-12.2002225441948,
123.079331151619)) ;
#79177=CARTESIAN_POINT('Ctrl Pts',(-21.2035814449539,-12.020867833611,123.1190236928)) ;
#79178=CARTESIAN_POINT('Ctrl Pts',(-21.2044864574362,-11.937009310127,123.109840472177)) ;
#79179=CARTESIAN_POINT('Ctrl Pts',(-21.204694405188,-11.8415943650587,123.076714022891)) ;
#79180=CARTESIAN_POINT('Ctrl Pts',(-21.2028845898013,-11.7344432406558,
122.980942735961)) ;
#79181=CARTESIAN_POINT('Ctrl Pts',(-21.1783390856595,-11.6999402773968,
122.867251844514)) ;
#79182=CARTESIAN_POINT('Ctrl Pts',(-21.1596366183962,-11.6999371505325,
122.812637127424)) ;
#79183=CARTESIAN_POINT('',(-5.63784594017984E-6,-11.7,130.056019952763)) ;
#79184=CARTESIAN_POINT('Ctrl Pts',(-21.1596366183962,-11.6999371505325,
122.812637127424)) ;
#79185=CARTESIAN_POINT('Ctrl Pts',(-21.1409341511322,-11.6999340236682,
122.758022410332)) ;
#79186=CARTESIAN_POINT('Ctrl Pts',(-21.0906697862186,-11.7344244794726,
122.653254433413)) ;
#79187=CARTESIAN_POINT('Ctrl Pts',(-21.0334409420522,-11.8416345019856,
122.576237828854)) ;
#79188=CARTESIAN_POINT('Ctrl Pts',(-21.0129220122535,-11.9369442551916,
122.550489340921)) ;
#79189=CARTESIAN_POINT('Ctrl Pts',(-21.0066804077936,-12.0210152203759,
122.543174306292)) ;
#79190=CARTESIAN_POINT('Ctrl Pts',(-21.0246592715631,-12.1418772592091,
122.564280492712)) ;
#79191=CARTESIAN_POINT('Ctrl Pts',(-21.0905949626881,-12.2655506269821,
122.653421665207)) ;
#79192=CARTESIAN_POINT('Ctrl Pts',(-21.141048681955,-12.3001250267877,122.757846947397)) ;
#79193=CARTESIAN_POINT('Ctrl Pts',(-21.1595576755874,-12.3,122.812674419028)) ;
#79194=CARTESIAN_POINT('Ctrl Pts',(-21.1595576755874,-12.3,122.812674419028)) ;
#79195=CARTESIAN_POINT('Ctrl Pts',(-21.1987114653594,-12.3022593030704,
122.922514297446)) ;
#79196=CARTESIAN_POINT('Ctrl Pts',(-21.2068562966847,-12.2002225441948,
123.079331151619)) ;
#79197=CARTESIAN_POINT('Ctrl Pts',(-21.2035814449539,-12.020867833611,123.1190236928)) ;
#79198=CARTESIAN_POINT('Ctrl Pts',(-21.2044864574362,-11.937009310127,123.109840472177)) ;
#79199=CARTESIAN_POINT('Ctrl Pts',(-21.204694405188,-11.8415943650587,123.076714022891)) ;
#79200=CARTESIAN_POINT('Ctrl Pts',(-21.2028845898013,-11.7344432406558,
122.980942735961)) ;
#79201=CARTESIAN_POINT('Ctrl Pts',(-21.166066333588,-11.6826887957666,122.810406398789)) ;
#79202=CARTESIAN_POINT('Ctrl Pts',(-21.0906697862186,-11.7344244794726,
122.653254433413)) ;
#79203=CARTESIAN_POINT('Ctrl Pts',(-21.0334409420522,-11.8416345019856,
122.576237828854)) ;
#79204=CARTESIAN_POINT('Ctrl Pts',(-21.0129220122535,-11.9369442551916,
122.550489340921)) ;
#79205=CARTESIAN_POINT('Ctrl Pts',(-21.0066804077936,-12.0210152203759,
122.543174306292)) ;
#79206=CARTESIAN_POINT('Ctrl Pts',(-21.0246592715631,-12.1418772592091,
122.564280492712)) ;
#79207=CARTESIAN_POINT('Ctrl Pts',(-21.0905949626881,-12.2655506269821,
122.653421665207)) ;
#79208=CARTESIAN_POINT('Ctrl Pts',(-21.141048681955,-12.3001250267877,122.757846947397)) ;
#79209=CARTESIAN_POINT('Ctrl Pts',(-21.1595576755874,-12.3,122.812674419028)) ;
#79210=CARTESIAN_POINT('Ctrl Pts',(-21.3014729215271,-12.4500000013844,
122.764093940462)) ;
#79211=CARTESIAN_POINT('Ctrl Pts',(-21.3642139707748,-12.4533889553457,
122.942469943529)) ;
#79212=CARTESIAN_POINT('Ctrl Pts',(-21.3994544235377,-12.3003338159049,
123.189225332334)) ;
#79213=CARTESIAN_POINT('Ctrl Pts',(-21.4023026040227,-12.031301750527,123.250798708205)) ;
#79214=CARTESIAN_POINT('Ctrl Pts',(-21.4018113001397,-11.9055139651401,
123.236577567789)) ;
#79215=CARTESIAN_POINT('Ctrl Pts',(-21.3965611953891,-11.7623915476468,
123.184771653818)) ;
#79216=CARTESIAN_POINT('Ctrl Pts',(-21.3786395141694,-11.6016648610055,
123.034597166172)) ;
#79217=CARTESIAN_POINT('Ctrl Pts',(-21.3085026878959,-11.5240331923606,
122.761622685277)) ;
#79218=CARTESIAN_POINT('Ctrl Pts',(-21.1966891219787,-11.6016367190622,
122.503204035368)) ;
#79219=CARTESIAN_POINT('Ctrl Pts',(-21.118819138729,-11.7624517530713,122.373200185185)) ;
#79220=CARTESIAN_POINT('Ctrl Pts',(-21.0912084270103,-11.9054163827587,
122.329507242695)) ;
#79221=CARTESIAN_POINT('Ctrl Pts',(-21.0828952761476,-12.0315228306677,
122.317025982144)) ;
#79222=CARTESIAN_POINT('Ctrl Pts',(-21.1068470535444,-12.212815888551,122.353033370586)) ;
#79223=CARTESIAN_POINT('Ctrl Pts',(-21.1966316872743,-12.3983259410573,
122.503453345861)) ;
#79224=CARTESIAN_POINT('Ctrl Pts',(-21.2713327489301,-12.450187539844,122.675227520146)) ;
#79225=CARTESIAN_POINT('Ctrl Pts',(-21.3014729215271,-12.4500000013844,
122.764093940462)) ;
#79226=CARTESIAN_POINT('',(-21.1595576755874,-12.3,122.812674419028)) ;
#79227=CARTESIAN_POINT('Ctrl Pts',(-17.6589816021521,-12.3,124.010992891073)) ;
#79228=CARTESIAN_POINT('Ctrl Pts',(-17.6198247664454,-12.302260540837,123.901150655369)) ;
#79229=CARTESIAN_POINT('Ctrl Pts',(-17.6116850160222,-12.2002215949029,
123.744337739047)) ;
#79230=CARTESIAN_POINT('Ctrl Pts',(-17.6149593962428,-12.0208669736416,
123.704645200407)) ;
#79231=CARTESIAN_POINT('Ctrl Pts',(-17.6140513077368,-11.9370098422088,
123.713825492269)) ;
#79232=CARTESIAN_POINT('Ctrl Pts',(-17.6138457601763,-11.8415941256522,
123.746953574365)) ;
#79233=CARTESIAN_POINT('Ctrl Pts',(-17.6156540763921,-11.7344433920138,
123.842724447157)) ;
#79234=CARTESIAN_POINT('Ctrl Pts',(-17.6524732810711,-11.682688712935,124.013260972172)) ;
#79235=CARTESIAN_POINT('Ctrl Pts',(-17.72786935392,-11.7344244983967,124.170412828578)) ;
#79236=CARTESIAN_POINT('Ctrl Pts',(-17.7850982943228,-11.8416345270247,
124.247429507382)) ;
#79237=CARTESIAN_POINT('Ctrl Pts',(-17.8056170712146,-11.9369444204012,
124.27317798136)) ;
#79238=CARTESIAN_POINT('Ctrl Pts',(-17.8118590245238,-12.021015295271,124.280493109677)) ;
#79239=CARTESIAN_POINT('Ctrl Pts',(-17.7938799763284,-12.1418774804083,
124.259386907686)) ;
#79240=CARTESIAN_POINT('Ctrl Pts',(-17.7279443615378,-12.2655504187416,
124.17024556063)) ;
#79241=CARTESIAN_POINT('Ctrl Pts',(-17.6774905688518,-12.3001251310252,
124.065820404267)) ;
#79242=CARTESIAN_POINT('Ctrl Pts',(-17.6589816021521,-12.3,124.010992891073)) ;
#79243=CARTESIAN_POINT('Ctrl Pts',(-17.5170663564952,-12.4500000035939,
124.059573369301)) ;
#79244=CARTESIAN_POINT('Ctrl Pts',(-17.4543214499664,-12.4533908062079,
123.881193173708)) ;
#79245=CARTESIAN_POINT('Ctrl Pts',(-17.4190874317839,-12.3003323949396,
123.634444787988)) ;
#79246=CARTESIAN_POINT('Ctrl Pts',(-17.4162387146148,-12.0313004596384,
123.572871338394)) ;
#79247=CARTESIAN_POINT('Ctrl Pts',(-17.4167260337872,-11.905514763682,123.587087385896)) ;
#79248=CARTESIAN_POINT('Ctrl Pts',(-17.4219791397424,-11.76239118819,123.638896252699)) ;
#79249=CARTESIAN_POINT('Ctrl Pts',(-17.4398990467708,-11.6016650883087,
123.789069843982)) ;
#79250=CARTESIAN_POINT('Ctrl Pts',(-17.5100369831582,-11.5240330679591,
124.062044775725)) ;
#79251=CARTESIAN_POINT('Ctrl Pts',(-17.6218499912451,-11.6016367475424,
124.320463176737)) ;
#79252=CARTESIAN_POINT('Ctrl Pts',(-17.6997200962288,-11.7624517905878,
124.450467158943)) ;
#79253=CARTESIAN_POINT('Ctrl Pts',(-17.7273306316869,-11.9054166305896,
124.494160054312)) ;
#79254=CARTESIAN_POINT('Ctrl Pts',(-17.7356441949461,-12.0315229428807,
124.50664151924)) ;
#79255=CARTESIAN_POINT('Ctrl Pts',(-17.7116922052291,-12.2128162206925,
124.470634075889)) ;
#79256=CARTESIAN_POINT('Ctrl Pts',(-17.6219076292031,-12.3983256278298,
124.320213840095)) ;
#79257=CARTESIAN_POINT('Ctrl Pts',(-17.5472065053376,-12.4501876978419,
124.148439850519)) ;
#79258=CARTESIAN_POINT('Ctrl Pts',(-17.5170663564952,-12.4500000035939,
124.059573369301)) ;
#79259=CARTESIAN_POINT('',(-17.6589816021521,-12.3,124.010992891073)) ;
#196737=UNCERTAINTY_MEASURE_WITH_UNIT(LENGTH_MEASURE(0.01),#196742,
'DISTANCE_ACCURACY_VALUE',
'Maximum model space distance between geometric entities at asserted c
onnectivities') ;
#196738=UNCERTAINTY_MEASURE_WITH_UNIT(LENGTH_MEASURE(0.01),#196742,
'DISTANCE_ACCURACY_VALUE',
'Maximum model space distance between geometric entities at asserted c
onnectivities') ;
#196740=(
GEOMETRIC_REPRESENTATION_CONTEXT(3)
GLOBAL_UNCERTAINTY_ASSIGNED_CONTEXT((#196737))
GLOBAL_UNIT_ASSIGNED_CONTEXT((#196742,#196744,#196745))
REPRESENTATION_CONTEXT('','3D')
) ;
#196741=(
GEOMETRIC_REPRESENTATION_CONTEXT(3)
GLOBAL_UNCERTAINTY_ASSIGNED_CONTEXT((#196738))
GLOBAL_UNIT_ASSIGNED_CONTEXT((#196742,#196744,#196745))
REPRESENTATION_CONTEXT('','3D')
) ;
#196742=(
LENGTH_UNIT()
NAMED_UNIT(*)
SI_UNIT(.MILLI.,.METRE.)
) ;
#196744=(
NAMED_UNIT(*)
PLANE_ANGLE_UNIT()
SI_UNIT($,.RADIAN.)
) ;
#196745=(
NAMED_UNIT(*)
SI_UNIT($,.STERADIAN.)
SOLID_ANGLE_UNIT()
) ;
#196753=PRODUCT_DEFINITION_CONTEXT('part definition',#196761,'design') ;
#196761=APPLICATION_CONTEXT(
'Core Data for Automotive Mechanical Design Process') ;
#196762=PRODUCT_CONTEXT('part definition',#196761,'mechanical') ;
#196765=PRESENTATION_STYLE_ASSIGNMENT((#196767)) ;
#196767=SURFACE_STYLE_USAGE(.BOTH.,#196769) ;
#196769=SURFACE_SIDE_STYLE('',(#196771)) ;
#196771=SURFACE_STYLE_FILL_AREA(#196773) ;
#196773=FILL_AREA_STYLE('Steel - Satin',(#196775)) ;
#196775=FILL_AREA_STYLE_COLOUR('Steel - Satin',#196777) ;
#196777=COLOUR_RGB('Steel - Satin', 0.09019608, 0.27058824, 0.51372549) ;
#196803=CARTESIAN_POINT ( '', ( 0.0, 0.0, 0.0 ) ) ;
#196804=DIRECTION ( '', ( 0.0, 0.0, 1.0 ) ) ;
#196805=DIRECTION ( '', ( 1.0, 0.0, 0.0 ) ) ;
#196806=AXIS2_PLACEMENT_3D ( '', #196803, #196804, #196805 ) ;
#196807=ADVANCED_BREP_SHAPE_REPRESENTATION ( 'Arbor', ( #339, #196806, #196817, #197251 ), #196740 ) ;
#196808=PRODUCT( 'Arbor', 'Arbor', '', ( #196762 ) ) ;
#196809=PRODUCT_DEFINITION_FORMATION ( '', '', #196808 ) ;
#196810=PRODUCT_DEFINITION( 'Arbor', 'Arbor', #196809, #196753 ) ;
#196811=PRODUCT_DEFINITION_SHAPE ( '', '', #196810 ) ;
#196812=SHAPE_DEFINITION_REPRESENTATION ( #196811, #196807 ) ;
#196814=CARTESIAN_POINT ( '', ( 0.0, 0.0, 0.0 ) ) ;
#196815=DIRECTION ( '', ( 0.0, 0.0, 1.0 ) ) ;
#196816=DIRECTION ( '', ( 1.0, 0.0, 0.0 ) ) ;
#196817=AXIS2_PLACEMENT_3D ( '', #196814, #196815, #196816 ) ;
#197248=CARTESIAN_POINT ( '', ( 0.0, 0.0, 0.0 ) ) ;
#197249=DIRECTION ( '', ( 0.0, 0.0, 1.0 ) ) ;
#197250=DIRECTION ( '', ( 1.0, 0.0, 0.0 ) ) ;
#197251=AXIS2_PLACEMENT_3D ( '', #197248, #197249, #197250 ) ;
ENDSEC;
END-ISO-10303-21;
